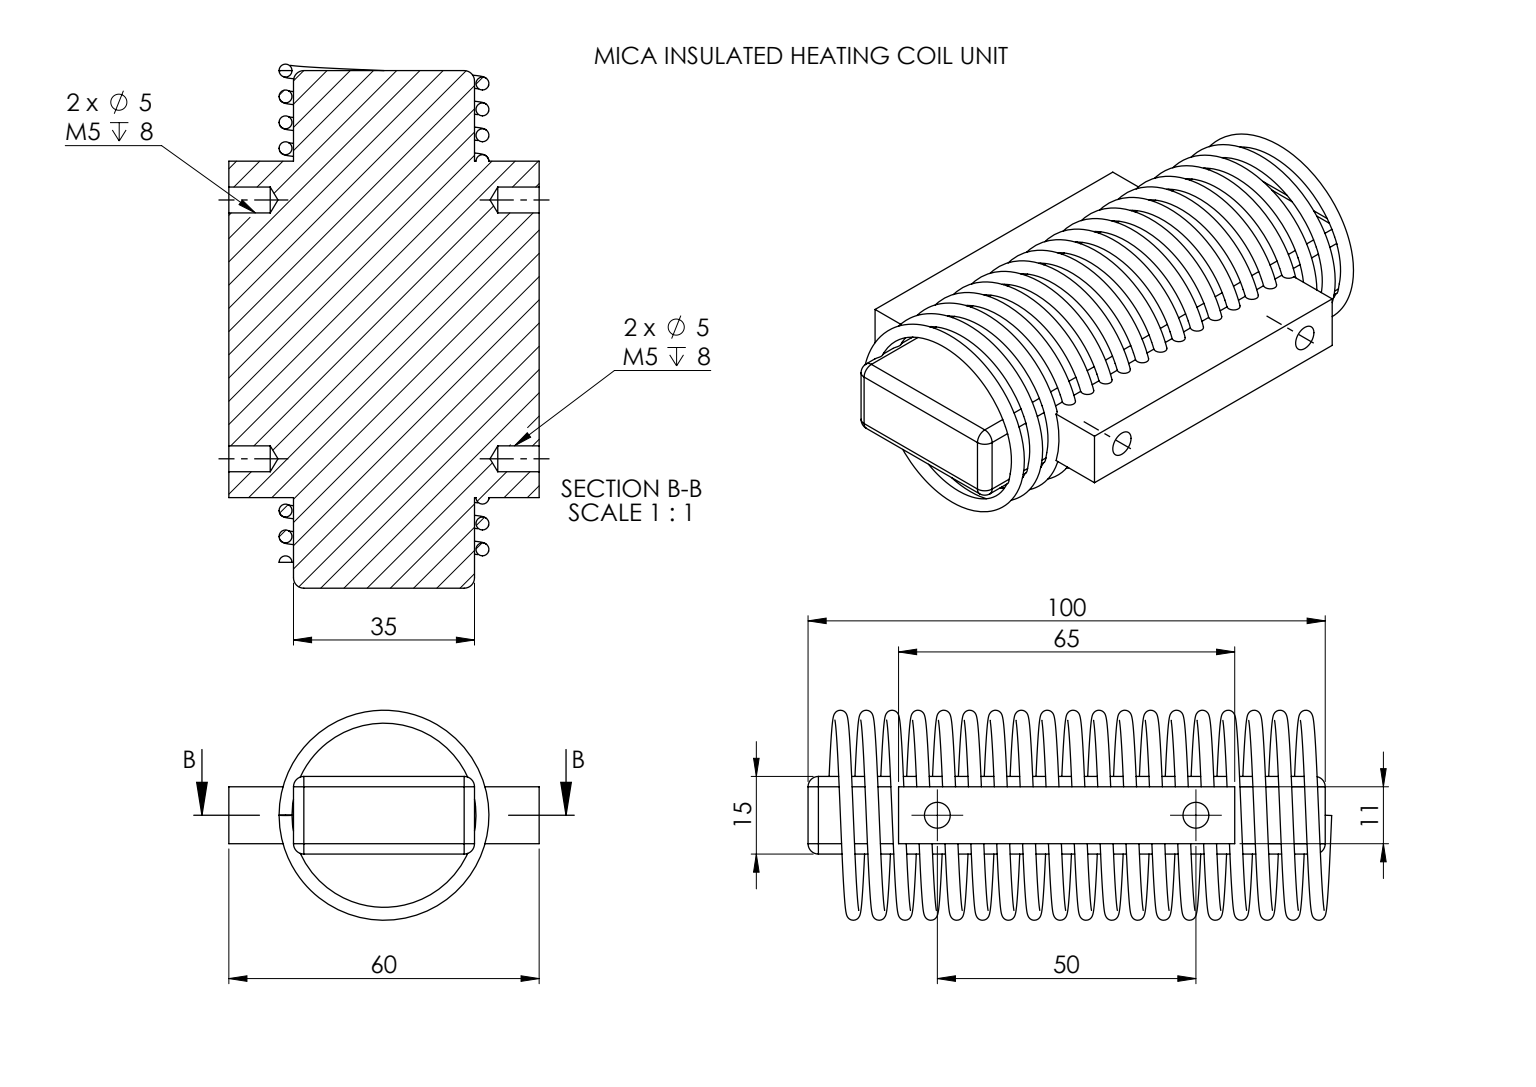
ISO-10303-21;
HEADER;
FILE_DESCRIPTION (('STEP AP214'),
    '1' );
FILE_NAME ('Mica Insulated Heating Coil Unit.step',
    '2026-10-04T13:31:42',
    ( '' ),
    ( '' ),
    'SwSTEP 2.0',
    'SolidWorks 2026',
    '' );
FILE_SCHEMA (( 'AUTOMOTIVE_DESIGN' ));
ENDSEC;

DATA;
#1=CARTESIAN_POINT ( 'NONE',  ( -19.03943276465977164, 0.05219959533909376836, 71.24890960531435269 ) ) ;
#2=CARTESIAN_POINT ( 'NONE',  ( 4.379528057220339221, -16.55341960407611168, 72.70724293864769550 ) ) ;
#3=CARTESIAN_POINT ( 'NONE',  ( 19.05341960407617918, -5.049401038297876454, 86.04275706135233293 ) ) ;
#4=CARTESIAN_POINT ( 'NONE',  ( 21.53943276465977519, -0.05219959533907433946, 43.74890960531435979 ) ) ;
#6=CARTESIAN_POINT ( 'NONE',  ( -19.05341960407611168, -5.049401038298163336, 21.45724293864768839 ) ) ;
#7=CARTESIAN_POINT ( 'NONE',  ( -16.18388926212240264, -7.379444403734405356, 30.43953151366152809 ) ) ;
#8=CARTESIAN_POINT ( 'NONE',  ( 5.049401038298161559, -19.05341960407611168, 77.70724293864765286 ) ) ;
#9=CARTESIAN_POINT ( 'NONE',  ( 21.53943276465977519, -0.05219959533907433946, 73.74890960531433848 ) ) ;
#10=CARTESIAN_POINT ( 'NONE',  ( -8.314922557961024197, 14.29746914071037800, 97.91775706135236135 ) ) ;
#11=CARTESIAN_POINT ( 'NONE',  ( -5.049401038298153566, 19.05341960407611168, 75.20724293864769550 ) ) ;
#12=CARTESIAN_POINT ( 'NONE',  ( -9.564922557961040184, 16.46253265017147172, 72.91775706135233293 ) ) ;
#13=CARTESIAN_POINT ( 'NONE',  ( 5.823673210054444382, -21.52544592524334988, 85.20942372801901854 ) ) ;
#14=CARTESIAN_POINT ( 'NONE',  ( -15.80617190586745835, -15.72974639402198527, 56.87390960531436690 ) ) ;
#15=CARTESIAN_POINT ( 'NONE',  ( 21.52544592524344225, -5.823673210054117533, 23.54057627198102765 ) ) ;
#16=CARTESIAN_POINT ( 'NONE',  ( -19.02544592524342804, 5.153800228976336051, 36.04057627198100988 ) ) ;
#17=CARTESIAN_POINT ( 'NONE',  ( -4.379528057220086978, -16.55341960407618274, 94.79275706135234714 ) ) ;
#18=CARTESIAN_POINT ( 'NONE',  ( -19.05341960407611168, -5.049401038298163336, 56.45724293864768129 ) ) ;
#19=CARTESIAN_POINT ( 'NONE',  ( 14.29746914071037800, 8.314922557961029526, 26.66775706135235424 ) ) ;
#21=CARTESIAN_POINT ( 'NONE',  ( 18.67979575497194134, -10.72451020669871369, 110.8344237280190043 ) ) ;
#22=CARTESIAN_POINT ( 'NONE',  ( -14.29746914071049879, 8.314922557960819915, 55.83224293864770260 ) ) ;
#23=CARTESIAN_POINT ( 'NONE',  ( -0.05219959533907301413, -21.53943276465977519, 102.4989096053143811 ) ) ;
#24=CARTESIAN_POINT ( 'NONE',  ( 10.81492255796078972, 18.62759615963270932, 99.58224293864770971 ) ) ;
#26=CARTESIAN_POINT ( 'NONE',  ( -15.72974639402197994, 15.80617190586746368, 40.62390960531435269 ) ) ;
#27=CARTESIAN_POINT ( 'NONE',  ( -12.06949235617739369, -12.14591786802326823, 74.37609039468568994 ) ) ;
#28=CARTESIAN_POINT ( 'NONE',  ( -4.483927247898539470, -16.52544592524342804, 92.29057627198103830 ) ) ;
#29=CARTESIAN_POINT ( 'NONE',  ( 19.03943276465977164, -0.05219959533909143690, 58.74890960531435979 ) ) ;
#30=SHAPE_REPRESENTATION_RELATIONSHIP ( 'NONE' , 'NONE' ,  #65015, #146166 ) ;
#32=CARTESIAN_POINT ( 'NONE',  ( -12.06949235617739369, -12.14591786802326823, 109.3760903946857042 ) ) ;
#33=CARTESIAN_POINT ( 'NONE',  ( -5.719274019375665041, -21.55341960407619695, 34.79275706135235424 ) ) ;
#34=CARTESIAN_POINT ( 'NONE',  ( -19.05341960407611168, -5.049401038298163336, 91.45724293864766707 ) ) ;
#35=CARTESIAN_POINT ( 'NONE',  ( 21.55341960407619695, -5.719274019375665929, 71.04275706135234714 ) ) ;
#38=ORIENTED_EDGE ( 'NONE', *, *, #138549, .T. ) ;
#39=CARTESIAN_POINT ( 'NONE',  ( 10.72451020669871369, 18.67979575497193778, 57.08442372801901854 ) ) ;
#40=CARTESIAN_POINT ( 'NONE',  ( -0.05219959533909027116, -19.03943276465977164, 57.49890960531435979 ) ) ;
#41=CARTESIAN_POINT ( 'NONE',  ( 9.564922557960805705, 16.46253265017160317, 84.58224293864769550 ) ) ;
#42=CARTESIAN_POINT ( 'NONE',  ( -9.564922557961040184, 16.46253265017147172, 67.91775706135233293 ) ) ;
#43=CARTESIAN_POINT ( 'NONE',  ( 5.719274019375673035, 21.55341960407619339, 47.29275706135234003 ) ) ;
#44=CARTESIAN_POINT ( 'NONE',  ( -19.05341960407617563, 5.049401038297882671, 103.5427570613523329 ) ) ;
#45=CARTESIAN_POINT ( 'NONE',  ( -5.049401038297874678, -19.05341960407617918, 69.79275706135233293 ) ) ;
#46=CARTESIAN_POINT ( 'NONE',  ( 13.89961937509977652, -13.97604488694527269, 38.12390960531436690 ) ) ;
#47=CARTESIAN_POINT ( 'NONE',  ( 19.05341960407617918, -5.049401038297876454, 86.04275706135233293 ) ) ;
#48=CARTESIAN_POINT ( 'NONE',  ( -16.52544592524335698, -4.483927247898792601, 98.95942372801903275 ) ) ;
#49=CARTESIAN_POINT ( 'NONE',  ( 0.05219959533936267826, -19.03943276465977164, 80.00109039468567573 ) ) ;
#50=CARTESIAN_POINT ( 'NONE',  ( -12.14591786802309592, -12.06949235617757132, 31.87390960531435979 ) ) ;
#51=CARTESIAN_POINT ( 'NONE',  ( 16.51473224551083163, -9.474510206698727899, 45.83442372801900433 ) ) ;
#52=CARTESIAN_POINT ( 'NONE',  ( 15.80617190586769283, -15.72974639402175789, 100.6260903946857184 ) ) ;
#54=CARTESIAN_POINT ( 'NONE',  ( 19.05341960407617918, -5.049401038297876454, 21.04275706135232582 ) ) ;
#56=CARTESIAN_POINT ( 'NONE',  ( 0.05219959533909260263, 19.03943276465977164, 24.99890960531435269 ) ) ;
#57=CARTESIAN_POINT ( 'NONE',  ( -21.53943276465977519, -0.05219959533937600094, 83.75109039468568994 ) ) ;
#58=CARTESIAN_POINT ( 'NONE',  ( 8.314922557961029526, -14.29746914071037800, 30.41775706135234358 ) ) ;
#59=CARTESIAN_POINT ( 'NONE',  ( 19.02544592524343514, -5.153800228976328945, 98.54057627198100988 ) ) ;
#61=CARTESIAN_POINT ( 'NONE',  ( 0.05219959533909260263, 19.03943276465977164, 79.99890960531436690 ) ) ;
#62=DIRECTION ( 'NONE',  ( -0.000000000000000000, -0.000000000000000000, 1.000000000000000000 ) ) ;
#64=CARTESIAN_POINT ( 'NONE',  ( -16.51473224551082808, 9.474510206698731452, 83.33442372801899012 ) ) ;
#66=CARTESIAN_POINT ( 'NONE',  ( 0.05219959533909260263, 19.03943276465977164, 114.9989096053143669 ) ) ;
#67=CARTESIAN_POINT ( 'NONE',  ( -10.72451020669870658, -18.67979575497194134, 109.5844237280190328 ) ) ;
#68=CARTESIAN_POINT ( 'NONE',  ( -13.97604488694547697, 13.89961937509957934, 103.1260903946856473 ) ) ;
#69=CARTESIAN_POINT ( 'NONE',  ( -4.483927247898539470, -16.52544592524342804, 97.29057627198105251 ) ) ;
#70=CARTESIAN_POINT ( 'NONE',  ( -5.153800228976328057, -19.02544592524343514, 22.29057627198102765 ) ) ;
#71=CARTESIAN_POINT ( 'NONE',  ( -5.823673210054116645, -21.52544592524344225, 62.29057627198102409 ) ) ;
#73=CARTESIAN_POINT ( 'NONE',  ( 10.72451020669898902, -18.67979575497178502, 47.91557627198102409 ) ) ;
#74=CARTESIAN_POINT ( 'NONE',  ( 13.89961937509977652, -13.97604488694527269, 28.12390960531435624 ) ) ;
#76=CARTESIAN_POINT ( 'NONE',  ( 16.51473224551083163, -9.474510206698727899, 55.83442372801899722 ) ) ;
#77=CARTESIAN_POINT ( 'NONE',  ( -14.29746914071049879, 8.314922557960819915, 35.83224293864768839 ) ) ;
#78=CARTESIAN_POINT ( 'NONE',  ( 9.474510206698971260, -16.51473224551069308, 112.9155762719810383 ) ) ;
#79=CARTESIAN_POINT ( 'NONE',  ( -15.80617190586768217, 15.72974639402176855, 83.12609039468568994 ) ) ;
#80=CARTESIAN_POINT ( 'NONE',  ( -10.72451020669898014, 18.67979575497178502, 65.41557627198102409 ) ) ;
#81=CARTESIAN_POINT ( 'NONE',  ( 18.67979575497194134, -10.72451020669871369, 55.83442372801901854 ) ) ;
#82=CARTESIAN_POINT ( 'NONE',  ( 15.80617190586769283, -15.72974639402175789, 45.62609039468567573 ) ) ;
#83=CARTESIAN_POINT ( 'NONE',  ( 13.89961937509977652, -13.97604488694527269, 78.12390960531433848 ) ) ;
#84=CARTESIAN_POINT ( 'NONE',  ( -8.314922557961024197, 14.29746914071037800, 97.91775706135236135 ) ) ;
#85=CARTESIAN_POINT ( 'NONE',  ( -5.049401038298153566, 19.05341960407611168, 25.20724293864768484 ) ) ;
#87=CARTESIAN_POINT ( 'NONE',  ( -14.29746914071049879, 8.314922557960819915, 70.83224293864770971 ) ) ;
#88=CARTESIAN_POINT ( 'NONE',  ( 8.224510206698953496, -14.34966873604960469, 37.91557627198102409 ) ) ;
#89=CARTESIAN_POINT ( 'NONE',  ( 19.05341960407611168, 5.049401038298154454, 63.95724293864769550 ) ) ;
#90=CARTESIAN_POINT ( 'NONE',  ( -19.03943276465977164, 0.05219959533909376836, 36.24890960531436690 ) ) ;
#91=CARTESIAN_POINT ( 'NONE',  ( 15.72974639402199770, -15.80617190586745480, 43.12390960531435269 ) ) ;
#92=CARTESIAN_POINT ( 'NONE',  ( -19.02544592524334988, -5.153800228976617603, 33.95942372801897591 ) ) ;
#94=CARTESIAN_POINT ( 'NONE',  ( 16.55341960407611168, 4.379528057220329451, 48.95724293864770971 ) ) ;
#95=CARTESIAN_POINT ( 'NONE',  ( -10.72451020669898014, 18.67979575497178502, 30.41557627198101699 ) ) ;
#98=CARTESIAN_POINT ( 'NONE',  ( -8.314922557961024197, 14.29746914071037800, 72.91775706135234714 ) ) ;
#99=CARTESIAN_POINT ( 'NONE',  ( 13.97604488694548053, -13.89961937509957401, 70.62609039468567573 ) ) ;
#100=CARTESIAN_POINT ( 'NONE',  ( 16.53943276465976808, -0.05219959533910856209, 43.74890960531435979 ) ) ;
#102=CARTESIAN_POINT ( 'NONE',  ( -8.314922557960811034, -14.29746914071050412, 27.08224293864769550 ) ) ;
#103=CARTESIAN_POINT ( 'NONE',  ( 16.46253265017160672, -9.564922557960803928, 48.33224293864769550 ) ) ;
#104=CARTESIAN_POINT ( 'NONE',  ( 19.05341960407611168, 5.049401038298154454, 73.95724293864768129 ) ) ;
#105=CARTESIAN_POINT ( 'NONE',  ( -5.049401038298153566, 19.05341960407611168, 35.20724293864768839 ) ) ;
#106=CARTESIAN_POINT ( 'NONE',  ( 21.55341960407619695, -5.719274019375665929, 41.04275706135236135 ) ) ;
#107=CARTESIAN_POINT ( 'NONE',  ( 16.46253265017160672, -9.564922557960803928, 63.33224293864769550 ) ) ;
#109=CARTESIAN_POINT ( 'NONE',  ( -19.03943276465977164, 0.05219959533909376836, 46.24890960531435979 ) ) ;
#110=CARTESIAN_POINT ( 'NONE',  ( -0.05219959533907301413, -21.53943276465977519, 32.49890960531435979 ) ) ;
#111=B_SPLINE_CURVE_WITH_KNOTS ( 'NONE', 3,
 ( #132361, #22184, #54519, #149527, #68676, #38352 ),
 .UNSPECIFIED., .F., .F.,
 ( 4, 2, 4 ),
 ( 0.007228050697041336729, 0.007608510107494812283, 0.007988969517948286969 ),
 .UNSPECIFIED. ) ;
#112=CARTESIAN_POINT ( 'NONE',  ( 10.72451020669871369, 18.67979575497193778, 67.08442372801901854 ) ) ;
#113=CARTESIAN_POINT ( 'NONE',  ( 12.06949235617757843, -12.14591786802309237, 113.1239096053143953 ) ) ;
#114=CARTESIAN_POINT ( 'NONE',  ( -21.55341960407610458, -5.719274019375992779, 31.45724293864769550 ) ) ;
#115=CARTESIAN_POINT ( 'NONE',  ( 8.314922557961029526, -14.29746914071037800, 95.41775706135234714 ) ) ;
#116=CARTESIAN_POINT ( 'NONE',  ( 10.81492255796106328, -18.62759615963255655, 110.4177570613523756 ) ) ;
#117=CARTESIAN_POINT ( 'NONE',  ( -8.314922557961024197, 14.29746914071037800, 67.91775706135234714 ) ) ;
#118=CARTESIAN_POINT ( 'NONE',  ( -9.564922557960796823, -16.46253265017161027, 112.0822429386476955 ) ) ;
#119=CARTESIAN_POINT ( 'NONE',  ( -14.29746914071037622, -8.314922557961029526, 59.16775706135234714 ) ) ;
#120=CARTESIAN_POINT ( 'NONE',  ( -8.314922557961024197, 14.29746914071037800, 37.91775706135235424 ) ) ;
#121=CARTESIAN_POINT ( 'NONE',  ( -0.05219959533934338120, 16.53943276465976808, 102.5010903946856899 ) ) ;
#122=CARTESIAN_POINT ( 'NONE',  ( -15.72974639402176322, -15.80617190586768395, 54.37609039468568994 ) ) ;
#123=CARTESIAN_POINT ( 'NONE',  ( 4.379528057220092307, 16.55341960407617563, 22.29275706135235069 ) ) ;
#124=CARTESIAN_POINT ( 'NONE',  ( 5.719274019375991003, -21.55341960407610458, 112.7072429386476955 ) ) ;
#125=CARTESIAN_POINT ( 'NONE',  ( 8.224510206698742110, 14.34966873604972548, 27.08442372801901854 ) ) ;
#126=CARTESIAN_POINT ( 'NONE',  ( -12.14591786802326823, 12.06949235617739902, 83.12609039468568994 ) ) ;
#128=CARTESIAN_POINT ( 'NONE',  ( 18.67979575497194134, -10.72451020669871369, 85.83442372801901854 ) ) ;
#129=CARTESIAN_POINT ( 'NONE',  ( 16.46253265017146816, 9.564922557961045513, 81.66775706135233293 ) ) ;
#130=CARTESIAN_POINT ( 'NONE',  ( -4.379528057220328563, 16.55341960407611168, 60.20724293864768839 ) ) ;
#131=CARTESIAN_POINT ( 'NONE',  ( -4.379528057220328563, 16.55341960407611168, 40.20724293864769550 ) ) ;
#132=CARTESIAN_POINT ( 'NONE',  ( -14.29746914071049879, 8.314922557960819915, 105.8322429386476955 ) ) ;
#133=CARTESIAN_POINT ( 'NONE',  ( -16.46253265017146816, -9.564922557961047289, 49.16775706135233293 ) ) ;
#135=CARTESIAN_POINT ( 'NONE',  ( 0.05219959533937995610, -21.53943276465977519, 45.00109039468568284 ) ) ;
#136=CARTESIAN_POINT ( 'NONE',  ( 0.05219959533934541429, -16.53943276465976808, 20.00109039468568639 ) ) ;
#137=DIRECTION ( 'NONE',  ( 0.000000000000000000, 0.000000000000000000, -1.000000000000000000 ) ) ;
#138=CARTESIAN_POINT ( 'NONE',  ( 16.46253265017160672, -9.564922557960803928, 108.3322429386476955 ) ) ;
#139=CARTESIAN_POINT ( 'NONE',  ( 15.80617190586746368, 15.72974639402197994, 69.37390960531436690 ) ) ;
#140=CARTESIAN_POINT ( 'NONE',  ( -19.02544592524334988, -5.153800228976617603, 98.95942372801900433 ) ) ;
#141=CARTESIAN_POINT ( 'NONE',  ( -16.51473224551069308, -9.474510206698971260, 106.6655762719810383 ) ) ;
#143=CARTESIAN_POINT ( 'NONE',  ( 14.29746914071049879, -8.314922557960816363, 113.3322429386476955 ) ) ;
#144=CARTESIAN_POINT ( 'NONE',  ( -21.55341960407619339, 5.719274019375674811, 98.54275706135234714 ) ) ;
#145=CARTESIAN_POINT ( 'NONE',  ( 13.89961937509977652, -13.97604488694527269, 28.12390960531435624 ) ) ;
#146=CARTESIAN_POINT ( 'NONE',  ( 21.52544592524334988, 5.823673210054432836, 51.45942372801901854 ) ) ;
#147=CARTESIAN_POINT ( 'NONE',  ( -21.53943276465977519, -0.05219959533937600094, 93.75109039468567573 ) ) ;
#148=CARTESIAN_POINT ( 'NONE',  ( 14.29746914071037800, 8.314922557961029526, 86.66775706135234714 ) ) ;
#149=CARTESIAN_POINT ( 'NONE',  ( -5.719274019375665041, -21.55341960407619695, 39.79275706135235424 ) ) ;
#150=CARTESIAN_POINT ( 'NONE',  ( 21.52544592524334988, 5.823673210054432836, 36.45942372801901143 ) ) ;
#151=CARTESIAN_POINT ( 'NONE',  ( 5.049401038297881783, 19.05341960407617563, 67.29275706135234714 ) ) ;
#152=CARTESIAN_POINT ( 'NONE',  ( -16.51473224551069308, -9.474510206698971260, 81.66557627198103830 ) ) ;
#153=CARTESIAN_POINT ( 'NONE',  ( -0.05219959533910754901, -16.53943276465976808, 107.4989096053143669 ) ) ;
#154=CARTESIAN_POINT ( 'NONE',  ( -0.05219959533907301413, -21.53943276465977519, 82.49890960531436690 ) ) ;
#155=CARTESIAN_POINT ( 'NONE',  ( 12.14591786802309770, 12.06949235617756955, 64.37390960531435269 ) ) ;
#156=CARTESIAN_POINT ( 'NONE',  ( -21.52544592524334988, -5.823673210054445271, 103.9594237280190185 ) ) ;
#157=CARTESIAN_POINT ( 'NONE',  ( -8.224510206698948167, 14.34966873604960824, 90.41557627198103830 ) ) ;
#158=CARTESIAN_POINT ( 'NONE',  ( -19.02544592524342804, 5.153800228976336051, 41.04057627198103120 ) ) ;
#159=CARTESIAN_POINT ( 'NONE',  ( 19.02544592524334988, 5.153800228976608722, 66.45942372801899012 ) ) ;
#160=AXIS2_PLACEMENT_3D ( 'NONE', #57198, #41025, #151201 ) ;
#161=CARTESIAN_POINT ( 'NONE',  ( -8.224510206698948167, 14.34966873604960824, 50.41557627198103120 ) ) ;
#162=CARTESIAN_POINT ( 'NONE',  ( 5.823673210054444382, -21.52544592524334988, 95.20942372801903275 ) ) ;
#163=CARTESIAN_POINT ( 'NONE',  ( 13.97604488694527802, 13.89961937509977652, 89.37390960531436690 ) ) ;
#164=CARTESIAN_POINT ( 'NONE',  ( 5.153800228976615827, -19.02544592524334988, 55.20942372801899722 ) ) ;
#165=CARTESIAN_POINT ( 'NONE',  ( 0.05219959533907565091, 21.53943276465977519, 69.99890960531435269 ) ) ;
#166=CARTESIAN_POINT ( 'NONE',  ( 18.67979575497178502, 10.72451020669898547, 109.1655762719810383 ) ) ;
#167=CARTESIAN_POINT ( 'NONE',  ( 5.153800228976615827, -19.02544592524334988, 110.2094237280189901 ) ) ;
#168=CARTESIAN_POINT ( 'NONE',  ( 0.05219959533934541429, -16.53943276465976808, 80.00109039468568994 ) ) ;
#169=CARTESIAN_POINT ( 'NONE',  ( -5.153800228976328057, -19.02544592524343514, 22.29057627198102765 ) ) ;
#170=CARTESIAN_POINT ( 'NONE',  ( -10.72451020669870658, -18.67979575497194134, 24.58442372801901499 ) ) ;
#171=CARTESIAN_POINT ( 'NONE',  ( -14.29746914071049879, 8.314922557960819915, 110.8322429386476955 ) ) ;
#173=CARTESIAN_POINT ( 'NONE',  ( 8.314922557961029526, -14.29746914071037800, 45.41775706135234003 ) ) ;
#175=CARTESIAN_POINT ( 'NONE',  ( 16.53943276465976808, -0.05219959533910856209, 78.74890960531436690 ) ) ;
#176=CARTESIAN_POINT ( 'NONE',  ( -18.67979575497178146, -10.72451020669898902, 81.66557627198103830 ) ) ;
#177=CARTESIAN_POINT ( 'NONE',  ( -8.224510206698735004, -14.34966873604973081, 104.5844237280190185 ) ) ;
#178=CARTESIAN_POINT ( 'NONE',  ( -4.483927247898782831, 16.52544592524335698, 32.70942372801900433 ) ) ;
#179=CARTESIAN_POINT ( 'NONE',  ( 19.03943276465977164, -0.05219959533909143690, 38.74890960531436690 ) ) ;
#180=CARTESIAN_POINT ( 'NONE',  ( -16.53943276465976808, -0.05219959533934237506, 83.75109039468568994 ) ) ;
#181=CARTESIAN_POINT ( 'NONE',  ( -5.153800228976607833, 19.02544592524334988, 77.70942372801900433 ) ) ;
#182=CARTESIAN_POINT ( 'NONE',  ( 21.55341960407610458, 5.719274019375980345, 68.95724293864769550 ) ) ;
#183=CARTESIAN_POINT ( 'NONE',  ( -4.379528057220086978, -16.55341960407618274, 109.7927570613523613 ) ) ;
#184=CARTESIAN_POINT ( 'NONE',  ( 15.72974639402176855, 15.80617190586768217, 86.87609039468568994 ) ) ;
#185=CARTESIAN_POINT ( 'NONE',  ( -18.67979575497178146, -10.72451020669898902, 41.66557627198103120 ) ) ;
#186=EDGE_LOOP ( 'NONE', ( #96983, #147295, #14374 ) ) ;
#187=CARTESIAN_POINT ( 'NONE',  ( -14.34966873604972548, 8.224510206698743886, 98.33442372801901854 ) ) ;
#188=CARTESIAN_POINT ( 'NONE',  ( -18.62759615963270932, 10.81492255796079327, 50.83224293864770971 ) ) ;
#190=CARTESIAN_POINT ( 'NONE',  ( -0.05219959533907301413, -21.53943276465977519, 22.49890960531436335 ) ) ;
#191=CARTESIAN_POINT ( 'NONE',  ( 17.50000000000000355, 3.565345528327941160, 108.0750551319352581 ) ) ;
#192=CARTESIAN_POINT ( 'NONE',  ( -16.46253265017160317, 9.564922557960807481, 25.83224293864769194 ) ) ;
#193=CARTESIAN_POINT ( 'NONE',  ( 15.72974639402199770, -15.80617190586745480, 78.12390960531436690 ) ) ;
#194=CARTESIAN_POINT ( 'NONE',  ( 0.05219959533934541429, -16.53943276465976808, 105.0010903946856757 ) ) ;
#195=CARTESIAN_POINT ( 'NONE',  ( 21.53943276465977519, 0.05219959533937863772, 61.25109039468567573 ) ) ;
#196=CARTESIAN_POINT ( 'NONE',  ( -14.29746914071037622, -8.314922557961029526, 24.16775706135235424 ) ) ;
#197=CARTESIAN_POINT ( 'NONE',  ( 12.14591786802309770, 12.06949235617756955, 114.3739096053143527 ) ) ;
#198=CARTESIAN_POINT ( 'NONE',  ( -19.05341960407617563, 5.049401038297882671, 113.5427570613523471 ) ) ;
#199=CARTESIAN_POINT ( 'NONE',  ( -5.049401038298153566, 19.05341960407611168, 35.20724293864768839 ) ) ;
#201=CARTESIAN_POINT ( 'NONE',  ( -19.03943276465977164, 0.05219959533909376836, 111.2489096053143669 ) ) ;
#202=CARTESIAN_POINT ( 'NONE',  ( 0.05219959533934541429, -16.53943276465976808, 85.00109039468568994 ) ) ;
#203=CARTESIAN_POINT ( 'NONE',  ( -9.564922557961040184, 16.46253265017147172, 82.91775706135233293 ) ) ;
#204=CARTESIAN_POINT ( 'NONE',  ( 9.564922557961047289, -16.46253265017146816, 30.41775706135232937 ) ) ;
#205=CARTESIAN_POINT ( 'NONE',  ( 0.05219959533907565091, 21.53943276465977519, 59.99890960531436690 ) ) ;
#206=CARTESIAN_POINT ( 'NONE',  ( -14.34966873604972548, 8.224510206698743886, 83.33442372801903275 ) ) ;
#207=CARTESIAN_POINT ( 'NONE',  ( -16.46253265017146816, -9.564922557961047289, 99.16775706135233293 ) ) ;
#208=CARTESIAN_POINT ( 'NONE',  ( 19.05341960407611168, 5.049401038298154454, 53.95724293864770260 ) ) ;
#209=CARTESIAN_POINT ( 'NONE',  ( 16.46253265017160672, -9.564922557960803928, 98.33224293864769550 ) ) ;
#210=CARTESIAN_POINT ( 'NONE',  ( -0.05219959533937732626, 21.53943276465977519, 47.50109039468568994 ) ) ;
#211=CARTESIAN_POINT ( 'NONE',  ( -19.05341960407611168, -5.049401038298163336, 41.45724293864769550 ) ) ;
#213=CARTESIAN_POINT ( 'NONE',  ( -13.89961937509977652, 13.97604488694528158, 110.6239096053143243 ) ) ;
#214=CARTESIAN_POINT ( 'NONE',  ( 8.314922557960818139, 14.29746914071049879, 64.58224293864769550 ) ) ;
#215=CARTESIAN_POINT ( 'NONE',  ( -5.719274019375978568, 21.55341960407610458, 55.20724293864770260 ) ) ;
#217=CARTESIAN_POINT ( 'NONE',  ( -16.46253265017146816, -9.564922557961047289, 49.16775706135233293 ) ) ;
#219=CARTESIAN_POINT ( 'NONE',  ( -16.46253265017160317, 9.564922557960807481, 60.83224293864769550 ) ) ;
#220=CARTESIAN_POINT ( 'NONE',  ( 5.049401038298161559, -19.05341960407611168, 67.70724293864769550 ) ) ;
#222=CARTESIAN_POINT ( 'NONE',  ( 12.06949235617739724, 12.14591786802326823, 46.87609039468568994 ) ) ;
#224=CARTESIAN_POINT ( 'NONE',  ( 16.51473224551083163, -9.474510206698727899, 30.83442372801900433 ) ) ;
#226=CARTESIAN_POINT ( 'NONE',  ( -0.05219959533934338120, 16.53943276465976808, 92.50109039468567573 ) ) ;
#228=CARTESIAN_POINT ( 'NONE',  ( 16.52544592524335698, 4.483927247898782831, 81.45942372801900433 ) ) ;
#229=CARTESIAN_POINT ( 'NONE',  ( 4.483927247898790824, -16.52544592524335698, 60.20942372801902565 ) ) ;
#230=CARTESIAN_POINT ( 'NONE',  ( -5.823673210054431948, 21.52544592524334988, 112.7094237280190328 ) ) ;
#231=CARTESIAN_POINT ( 'NONE',  ( -5.049401038298153566, 19.05341960407611168, 50.20724293864770260 ) ) ;
#233=CARTESIAN_POINT ( 'NONE',  ( -10.72451020669870658, -18.67979575497194134, 69.58442372801900433 ) ) ;
#234=CARTESIAN_POINT ( 'NONE',  ( -19.03943276465977164, -0.05219959533935918106, 73.75109039468566152 ) ) ;
#235=CARTESIAN_POINT ( 'NONE',  ( -18.67979575497193778, 10.72451020669871902, 113.3344237280190328 ) ) ;
#236=CARTESIAN_POINT ( 'NONE',  ( 16.51473224551069308, 9.474510206698969483, 29.16557627198103475 ) ) ;
#237=CARTESIAN_POINT ( 'NONE',  ( 17.50000000000006750, 5.663021631379938192, 23.82188452050911209 ) ) ;
#238=CARTESIAN_POINT ( 'NONE',  ( -10.72451020669898014, 18.67979575497178502, 70.41557627198102409 ) ) ;
#239=CARTESIAN_POINT ( 'NONE',  ( 18.67979575497178502, 10.72451020669898547, 24.16557627198103120 ) ) ;
#240=CARTESIAN_POINT ( 'NONE',  ( 0.05219959533910956823, 16.53943276465976808, 114.9989096053143669 ) ) ;
#241=CARTESIAN_POINT ( 'NONE',  ( 4.379528057220092307, 16.55341960407617563, 37.29275706135235424 ) ) ;
#242=CARTESIAN_POINT ( 'NONE',  ( 14.34966873604960469, 8.224510206698951720, 24.16557627198103120 ) ) ;
#244=CARTESIAN_POINT ( 'NONE',  ( -15.72974639402176322, -15.80617190586768395, 24.37609039468567573 ) ) ;
#245=CARTESIAN_POINT ( 'NONE',  ( 4.483927247898545687, 16.52544592524342804, 34.79057627198103120 ) ) ;
#247=CARTESIAN_POINT ( 'NONE',  ( -13.89961937509957401, -13.97604488694547875, 109.3760903946856331 ) ) ;
#248=CARTESIAN_POINT ( 'NONE',  ( 16.46253265017146816, 9.564922557961045513, 21.66775706135233648 ) ) ;
#249=CARTESIAN_POINT ( 'NONE',  ( 12.14591786802309770, 12.06949235617756955, 49.37390960531436690 ) ) ;
#250=CARTESIAN_POINT ( 'NONE',  ( 18.67979575497178502, 10.72451020669898547, 99.16557627198100988 ) ) ;
#251=CARTESIAN_POINT ( 'NONE',  ( 17.50000000000000355, 5.622605283950888655, 33.81207310596111881 ) ) ;
#252=CARTESIAN_POINT ( 'NONE',  ( -15.72974639402197994, 15.80617190586746368, 60.62390960531437401 ) ) ;
#253=CARTESIAN_POINT ( 'NONE',  ( -0.05219959533909027116, -19.03943276465977164, 77.49890960531435269 ) ) ;
#254=CARTESIAN_POINT ( 'NONE',  ( 8.314922557960818139, 14.29746914071049879, 49.58224293864769550 ) ) ;
#255=CARTESIAN_POINT ( 'NONE',  ( 0.05219959533909260263, 19.03943276465977164, 89.99890960531436690 ) ) ;
#256=B_SPLINE_CURVE_WITH_KNOTS ( 'NONE', 3,
 ( #135702, #179228, #194389, #162034, #102364, #70032, #58838, #148877, #56868, #196396, #118543, #180233, #23530, #41702, #119537, #146865, #181220, #193382, #54858, #116532, #178220, #17313, #108315, #14325, #1126, #186178, #60815, #44673, #78968, #169995, #75990, #62800 ),
 .UNSPECIFIED., .F., .F.,
 ( 4, 2, 2, 2, 2, 2, 2, 2, 2, 2, 2, 2, 2, 2, 2, 4 ),
 ( 1.646036181032119693E-15, 0.0003712461730052185930, 0.0007424923460087911502, 0.001113738519012363653, 0.001484984692015936265, 0.002227477038023079753, 0.002598723211026658653, 0.002969969384030237119, 0.003341215557033815585, 0.003712461730037394485, 0.004083707903040972517, 0.004454954076044551417, 0.004826200249048129449, 0.005197446422051708349, 0.005568692595055286382, 0.005939938768058865282 ),
 .UNSPECIFIED. ) ;
#258=CARTESIAN_POINT ( 'NONE',  ( 0.05219959533936267826, -19.03943276465977164, 60.00109039468566863 ) ) ;
#259=CARTESIAN_POINT ( 'NONE',  ( 5.823673210054125526, 21.52544592524343514, 99.79057627198103830 ) ) ;
#260=CARTESIAN_POINT ( 'NONE',  ( 19.05341960407611168, 5.049401038298154454, 43.95724293864769550 ) ) ;
#261=CARTESIAN_POINT ( 'NONE',  ( -0.05219959533910754901, -16.53943276465976808, 102.4989096053143811 ) ) ;
#262=CARTESIAN_POINT ( 'NONE',  ( -10.81492255796105439, 18.62759615963255655, 47.91775706135234714 ) ) ;
#264=CARTESIAN_POINT ( 'NONE',  ( -16.52544592524342804, 4.483927247898546575, 26.04057627198103475 ) ) ;
#265=CARTESIAN_POINT ( 'NONE',  ( -13.89961937509977652, 13.97604488694528158, 55.62390960531434558 ) ) ;
#266=CARTESIAN_POINT ( 'NONE',  ( -13.89961937509977652, 13.97604488694528158, 105.6239096053143527 ) ) ;
#267=CARTESIAN_POINT ( 'NONE',  ( 5.823673210054125526, 21.52544592524343514, 59.79057627198103120 ) ) ;
#269=CARTESIAN_POINT ( 'NONE',  ( 0.05219959533909260263, 19.03943276465977164, 34.99890960531435979 ) ) ;
#270=CARTESIAN_POINT ( 'NONE',  ( -15.72974639402197994, 15.80617190586746368, 50.62390960531435979 ) ) ;
#271=CARTESIAN_POINT ( 'NONE',  ( 15.72974639402176855, 15.80617190586768217, 91.87609039468568994 ) ) ;
#273=CARTESIAN_POINT ( 'NONE',  ( -16.52544592524335698, -4.483927247898792601, 83.95942372801900433 ) ) ;
#274=CARTESIAN_POINT ( 'NONE',  ( 12.06949235617739724, 12.14591786802326823, 91.87609039468568994 ) ) ;
#275=CARTESIAN_POINT ( 'NONE',  ( 5.153800228976335163, 19.02544592524342804, 54.79057627198103120 ) ) ;
#276=CARTESIAN_POINT ( 'NONE',  ( 13.89961937509977652, -13.97604488694527269, 68.12390960531436690 ) ) ;
#278=CARTESIAN_POINT ( 'NONE',  ( -19.03943276465977164, -0.05219959533935918106, 28.75109039468566507 ) ) ;
#279=CARTESIAN_POINT ( 'NONE',  ( 14.29746914071037800, 8.314922557961029526, 76.66775706135234714 ) ) ;
#280=CARTESIAN_POINT ( 'NONE',  ( -18.67979575497193778, 10.72451020669871902, 113.3344237280190328 ) ) ;
#281=CARTESIAN_POINT ( 'NONE',  ( -19.05341960407611168, -5.049401038298163336, 71.45724293864766707 ) ) ;
#282=CARTESIAN_POINT ( 'NONE',  ( -21.52544592524343514, 5.823673210054127303, 36.04057627198102409 ) ) ;
#283=CARTESIAN_POINT ( 'NONE',  ( 14.34966873604972726, -8.224510206698740333, 25.83442372801901499 ) ) ;
#284=CARTESIAN_POINT ( 'NONE',  ( 0.05219959533937995610, -21.53943276465977519, 80.00109039468568994 ) ) ;
#285=CARTESIAN_POINT ( 'NONE',  ( -0.05219959533934338120, 16.53943276465976808, 52.50109039468567573 ) ) ;
#286=CARTESIAN_POINT ( 'NONE',  ( 10.72451020669898902, -18.67979575497178502, 97.91557627198103830 ) ) ;
#287=CARTESIAN_POINT ( 'NONE',  ( -16.51473224551082808, 9.474510206698731452, 113.3344237280190043 ) ) ;
#288=CARTESIAN_POINT ( 'NONE',  ( 13.89961937509977652, -13.97604488694527269, 73.12390960531436690 ) ) ;
#289=CARTESIAN_POINT ( 'NONE',  ( 4.483927247898790824, -16.52544592524335698, 25.20942372801901854 ) ) ;
#290=CARTESIAN_POINT ( 'NONE',  ( 13.97604488694527802, 13.89961937509977652, 44.37390960531435269 ) ) ;
#291=CARTESIAN_POINT ( 'NONE',  ( 16.46253265017146816, 9.564922557961045513, 111.6677570613523329 ) ) ;
#292=CARTESIAN_POINT ( 'NONE',  ( -12.06949235617756955, 12.14591786802309770, 75.62390960531439532 ) ) ;
#293=CARTESIAN_POINT ( 'NONE',  ( 4.379528057220092307, 16.55341960407617563, 87.29275706135236135 ) ) ;
#294=EDGE_CURVE ( 'NONE', #2008, #55198, #134552, .T. ) ;
#295=CARTESIAN_POINT ( 'NONE',  ( 21.52544592524334988, 5.823673210054432836, 31.45942372801901854 ) ) ;
#296=CARTESIAN_POINT ( 'NONE',  ( 0.05219959533909260263, 19.03943276465977164, 69.99890960531435269 ) ) ;
#297=CARTESIAN_POINT ( 'NONE',  ( 13.89961937509977652, -13.97604488694527269, 63.12390960531435979 ) ) ;
#298=CARTESIAN_POINT ( 'NONE',  ( 4.483927247898790824, -16.52544592524335698, 80.20942372801901854 ) ) ;
#302=CARTESIAN_POINT ( 'NONE',  ( -19.02544592524334988, -5.153800228976617603, 28.95942372801900433 ) ) ;
#303=CARTESIAN_POINT ( 'NONE',  ( -5.049401038298153566, 19.05341960407611168, 35.20724293864768839 ) ) ;
#304=CARTESIAN_POINT ( 'NONE',  ( 0.05219959533909260263, 19.03943276465977164, 109.9989096053143669 ) ) ;
#305=ORIENTED_EDGE ( 'NONE', *, *, #5230, .T. ) ;
#306=CARTESIAN_POINT ( 'NONE',  ( -12.14591786802326823, 12.06949235617739902, 33.12609039468569705 ) ) ;
#307=CARTESIAN_POINT ( 'NONE',  ( 9.474510206698729675, 16.51473224551082808, 52.08442372801900433 ) ) ;
#308=CARTESIAN_POINT ( 'NONE',  ( -16.52544592524335698, -4.483927247898792601, 38.95942372801901854 ) ) ;
#309=CARTESIAN_POINT ( 'NONE',  ( 0.05219959533909260263, 19.03943276465977164, 109.9989096053143669 ) ) ;
#310=CARTESIAN_POINT ( 'NONE',  ( -0.05219959533909027116, -19.03943276465977164, 67.49890960531436690 ) ) ;
#311=CARTESIAN_POINT ( 'NONE',  ( 15.80617190586746368, 15.72974639402197994, 99.37390960531436690 ) ) ;
#312=CARTESIAN_POINT ( 'NONE',  ( 16.51473224551069308, 9.474510206698969483, 94.16557627198103830 ) ) ;
#313=CARTESIAN_POINT ( 'NONE',  ( 19.02544592524343514, -5.153800228976328945, 23.54057627198102054 ) ) ;
#314=CARTESIAN_POINT ( 'NONE',  ( -9.564922557960796823, -16.46253265017161027, 67.08224293864769550 ) ) ;
#315=CARTESIAN_POINT ( 'NONE',  ( -12.06949235617739369, -12.14591786802326823, 109.3760903946857042 ) ) ;
#316=CARTESIAN_POINT ( 'NONE',  ( 9.474510206698971260, -16.51473224551069308, 27.91557627198103120 ) ) ;
#317=CARTESIAN_POINT ( 'NONE',  ( -9.474510206698720793, -16.51473224551083518, 34.58442372801899722 ) ) ;
#318=CARTESIAN_POINT ( 'NONE',  ( 12.14591786802309770, 12.06949235617756955, 59.37390960531436690 ) ) ;
#319=CARTESIAN_POINT ( 'NONE',  ( 21.55341960407619695, -5.719274019375665929, 101.0427570613523756 ) ) ;
#320=CARTESIAN_POINT ( 'NONE',  ( 19.05341960407611168, 5.049401038298154454, 38.95724293864767418 ) ) ;
#321=CARTESIAN_POINT ( 'NONE',  ( -8.224510206698735004, -14.34966873604973081, 54.58442372801901143 ) ) ;
#322=CARTESIAN_POINT ( 'NONE',  ( -8.224510206698948167, 14.34966873604960824, 45.41557627198103830 ) ) ;
#323=CARTESIAN_POINT ( 'NONE',  ( 18.67979575497194134, -10.72451020669871369, 85.83442372801901854 ) ) ;
#324=CARTESIAN_POINT ( 'NONE',  ( 13.89961937509977652, -13.97604488694527269, 83.12390960531436690 ) ) ;
#325=CARTESIAN_POINT ( 'NONE',  ( 5.049401038298161559, -19.05341960407611168, 92.70724293864769550 ) ) ;
#326=CARTESIAN_POINT ( 'NONE',  ( 16.53943276465976808, -0.05219959533910856209, 103.7489096053143669 ) ) ;
#327=CARTESIAN_POINT ( 'NONE',  ( 14.29746914071049879, -8.314922557960816363, 78.33224293864770971 ) ) ;
#328=CARTESIAN_POINT ( 'NONE',  ( 15.80617190586746368, 15.72974639402197994, 84.37390960531438111 ) ) ;
#329=CARTESIAN_POINT ( 'NONE',  ( 19.02544592524343514, -5.153800228976328945, 78.54057627198099567 ) ) ;
#330=CARTESIAN_POINT ( 'NONE',  ( 21.52544592524344225, -5.823673210054117533, 93.54057627198103830 ) ) ;
#331=CARTESIAN_POINT ( 'NONE',  ( 16.46253265017146816, 9.564922557961045513, 71.66775706135233293 ) ) ;
#332=CARTESIAN_POINT ( 'NONE',  ( 19.53037848336981952, -5.499999999999893419, 47.35532783611446916 ) ) ;
#333=CARTESIAN_POINT ( 'NONE',  ( -12.14591786802309592, -12.06949235617757132, 91.87390960531436690 ) ) ;
#334=CARTESIAN_POINT ( 'NONE',  ( 5.049401038298161559, -19.05341960407611168, 57.70724293864769550 ) ) ;
#335=CARTESIAN_POINT ( 'NONE',  ( 21.52544592524344225, -5.823673210054117533, 63.54057627198103830 ) ) ;
#336=CARTESIAN_POINT ( 'NONE',  ( -18.09867054820431775, -5.499999999999926281, 83.98393025253589883 ) ) ;
#337=CARTESIAN_POINT ( 'NONE',  ( 16.53943276465976808, -0.05219959533910856209, 23.74890960531435269 ) ) ;
#339=CARTESIAN_POINT ( 'NONE',  ( -0.05219959533934338120, 16.53943276465976808, 22.50109039468567573 ) ) ;
#340=CARTESIAN_POINT ( 'NONE',  ( -8.314922557960811034, -14.29746914071050412, 77.08224293864769550 ) ) ;
#341=CARTESIAN_POINT ( 'NONE',  ( -19.20446147854526231, -5.499999999999955591, 94.38999695167676407 ) ) ;
#342=CARTESIAN_POINT ( 'NONE',  ( -19.03943276465977164, 0.05219959533909376836, 76.24890960531435269 ) ) ;
#343=CARTESIAN_POINT ( 'NONE',  ( -16.46253265017160317, 9.564922557960807481, 35.83224293864768839 ) ) ;
#344=CARTESIAN_POINT ( 'NONE',  ( -8.224510206698948167, 14.34966873604960824, 65.41557627198102409 ) ) ;
#345=CARTESIAN_POINT ( 'NONE',  ( -10.81492255796078084, -18.62759615963271287, 22.08224293864769194 ) ) ;
#346=CARTESIAN_POINT ( 'NONE',  ( 5.153800228976615827, -19.02544592524334988, 95.20942372801897591 ) ) ;
#347=CARTESIAN_POINT ( 'NONE',  ( -19.03943276465977164, 0.05219959533909376836, 96.24890960531436690 ) ) ;
#348=CARTESIAN_POINT ( 'NONE',  ( -10.72451020669898014, 18.67979575497178502, 70.41557627198102409 ) ) ;
#349=CARTESIAN_POINT ( 'NONE',  ( 8.314922557961029526, -14.29746914071037800, 75.41775706135233293 ) ) ;
#350=CARTESIAN_POINT ( 'NONE',  ( -16.29526858892909758, 7.335722546919977383, 94.20329402199732272 ) ) ;
#351=CARTESIAN_POINT ( 'NONE',  ( 16.51473224551069308, 9.474510206698969483, 69.16557627198102409 ) ) ;
#352=CARTESIAN_POINT ( 'NONE',  ( 18.67979575497178502, 10.72451020669898547, 64.16557627198102409 ) ) ;
#353=CARTESIAN_POINT ( 'NONE',  ( 19.02544592524334988, 5.153800228976608722, 106.4594237280190185 ) ) ;
#354=CARTESIAN_POINT ( 'NONE',  ( -8.314922557960811034, -14.29746914071050412, 37.08224293864768129 ) ) ;
#355=CARTESIAN_POINT ( 'NONE',  ( 18.67979575497194134, -10.72451020669871369, 40.83442372801901854 ) ) ;
#357=CARTESIAN_POINT ( 'NONE',  ( 16.53943276465976808, 0.05219959533934440121, 76.25109039468568994 ) ) ;
#358=CARTESIAN_POINT ( 'NONE',  ( -0.05219959533909027116, -19.03943276465977164, 102.4989096053143669 ) ) ;
#359=CARTESIAN_POINT ( 'NONE',  ( 9.564922557960805705, 16.46253265017160317, 104.5822429386476955 ) ) ;
#361=CARTESIAN_POINT ( 'NONE',  ( -12.06949235617739369, -12.14591786802326823, 99.37609039468568994 ) ) ;
#362=CARTESIAN_POINT ( 'NONE',  ( 12.06949235617739724, 12.14591786802326823, 51.87609039468568284 ) ) ;
#363=CARTESIAN_POINT ( 'NONE',  ( -19.02544592524342804, 5.153800228976336051, 61.04057627198103120 ) ) ;
#364=CARTESIAN_POINT ( 'NONE',  ( 0.05219959533909260263, 19.03943276465977164, 69.99890960531435269 ) ) ;
#365=CARTESIAN_POINT ( 'NONE',  ( -18.62759615963255300, -10.81492255796106328, 54.16775706135235424 ) ) ;
#366=CARTESIAN_POINT ( 'NONE',  ( 14.34966873604972726, -8.224510206698740333, 65.83442372801900433 ) ) ;
#367=CARTESIAN_POINT ( 'NONE',  ( -0.05219959533910754901, -16.53943276465976808, 32.49890960531435979 ) ) ;
#368=CARTESIAN_POINT ( 'NONE',  ( -16.46253265017160317, 9.564922557960807481, 40.83224293864769550 ) ) ;
#369=CARTESIAN_POINT ( 'NONE',  ( -9.474510206698964154, 16.51473224551069663, 30.41557627198102054 ) ) ;
#370=CARTESIAN_POINT ( 'NONE',  ( -12.06949235617739369, -12.14591786802326823, 24.37609039468567573 ) ) ;
#371=CARTESIAN_POINT ( 'NONE',  ( 19.05341960407617918, -5.049401038297876454, 76.04275706135230450 ) ) ;
#372=CARTESIAN_POINT ( 'NONE',  ( -14.34966873604960291, -8.224510206698953496, 81.66557627198103830 ) ) ;
#373=CARTESIAN_POINT ( 'NONE',  ( -16.46253265017160317, 9.564922557960807481, 55.83224293864769550 ) ) ;
#374=CARTESIAN_POINT ( 'NONE',  ( 0.05219959533936267826, -19.03943276465977164, 85.00109039468567573 ) ) ;
#376=CARTESIAN_POINT ( 'NONE',  ( -21.52544592524334988, -5.823673210054445271, 93.95942372801903275 ) ) ;
#377=CARTESIAN_POINT ( 'NONE',  ( -14.34966873604972548, 8.224510206698743886, 48.33442372801902565 ) ) ;
#379=CARTESIAN_POINT ( 'NONE',  ( -15.80617190586745835, -15.72974639402198527, 51.87390960531437401 ) ) ;
#380=CARTESIAN_POINT ( 'NONE',  ( 16.55341960407618274, -4.379528057220086978, 36.04275706135234714 ) ) ;
#381=CARTESIAN_POINT ( 'NONE',  ( -19.35633801406909527, 5.499999999999580780, 69.13373818172763663 ) ) ;
#382=CARTESIAN_POINT ( 'NONE',  ( 9.564922557961047289, -16.46253265017146816, 45.41775706135232582 ) ) ;
#383=CARTESIAN_POINT ( 'NONE',  ( -19.03943276465977164, 0.05219959533909376836, 76.24890960531435269 ) ) ;
#384=CARTESIAN_POINT ( 'NONE',  ( 13.89961937509977652, -13.97604488694527269, 58.12390960531436690 ) ) ;
#385=CARTESIAN_POINT ( 'NONE',  ( 16.46253265017160672, -9.564922557960803928, 73.33224293864769550 ) ) ;
#386=CARTESIAN_POINT ( 'NONE',  ( -16.51473224551069308, -9.474510206698971260, 91.66557627198103830 ) ) ;
#387=CARTESIAN_POINT ( 'NONE',  ( -9.474510206698720793, -16.51473224551083518, 39.58442372801899722 ) ) ;
#388=CARTESIAN_POINT ( 'NONE',  ( 9.564922557961047289, -16.46253265017146816, 20.41775706135233293 ) ) ;
#389=CARTESIAN_POINT ( 'NONE',  ( -14.34966873604960291, -8.224510206698953496, 41.66557627198103120 ) ) ;
#390=CARTESIAN_POINT ( 'NONE',  ( 13.89961937509977652, -13.97604488694527269, 38.12390960531436690 ) ) ;
#391=CARTESIAN_POINT ( 'NONE',  ( -5.049401038298153566, 19.05341960407611168, 105.2072429386476671 ) ) ;
#392=CARTESIAN_POINT ( 'NONE',  ( -0.05219959533937732626, 21.53943276465977519, 82.50109039468568994 ) ) ;
#393=CARTESIAN_POINT ( 'NONE',  ( -13.97604488694527625, -13.89961937509977652, 56.87390960531434558 ) ) ;
#395=CARTESIAN_POINT ( 'NONE',  ( 18.67979575497194134, -10.72451020669871369, 85.83442372801901854 ) ) ;
#396=CARTESIAN_POINT ( 'NONE',  ( 18.67979575497178502, 10.72451020669898547, 39.16557627198102409 ) ) ;
#397=CARTESIAN_POINT ( 'NONE',  ( -15.80617190586768217, 15.72974639402176855, 23.12609039468567573 ) ) ;
#398=CARTESIAN_POINT ( 'NONE',  ( 19.05341960407617918, -5.049401038297876454, 51.04275706135231871 ) ) ;
#399=CARTESIAN_POINT ( 'NONE',  ( -0.05219959533909027116, -19.03943276465977164, 22.49890960531436690 ) ) ;
#400=CARTESIAN_POINT ( 'NONE',  ( 19.05341960407611168, 5.049401038298154454, 78.95724293864769550 ) ) ;
#401=CARTESIAN_POINT ( 'NONE',  ( 12.14591786802327356, -12.06949235617739191, 30.62609039468567929 ) ) ;
#402=CARTESIAN_POINT ( 'NONE',  ( -12.06949235617756955, 12.14591786802309770, 90.62390960531436690 ) ) ;
#403=CARTESIAN_POINT ( 'NONE',  ( -19.03943276465977164, 0.05219959533909376836, 56.24890960531435979 ) ) ;
#404=CARTESIAN_POINT ( 'NONE',  ( 0.05219959533907565091, 21.53943276465977519, 34.99890960531435979 ) ) ;
#405=CARTESIAN_POINT ( 'NONE',  ( -16.51473224551082808, 9.474510206698731452, 103.3344237280190043 ) ) ;
#406=CARTESIAN_POINT ( 'NONE',  ( -21.55341960407610458, -5.719274019375992779, 101.4572429386476955 ) ) ;
#407=CARTESIAN_POINT ( 'NONE',  ( 18.62759615963255655, 10.81492255796105972, 61.66775706135235424 ) ) ;
#408=CARTESIAN_POINT ( 'NONE',  ( -8.314922557961024197, 14.29746914071037800, 52.91775706135235424 ) ) ;
#409=CARTESIAN_POINT ( 'NONE',  ( -16.53943276465976808, -0.05219959533934237506, 73.75109039468567573 ) ) ;
#410=CARTESIAN_POINT ( 'NONE',  ( -13.89961937509977652, 13.97604488694528158, 60.62390960531436690 ) ) ;
#411=CARTESIAN_POINT ( 'NONE',  ( -16.53943276465976808, -0.05219959533934237506, 83.75109039468568994 ) ) ;
#412=CARTESIAN_POINT ( 'NONE',  ( -10.72451020669898014, 18.67979575497178502, 115.4155762719810241 ) ) ;
#413=CARTESIAN_POINT ( 'NONE',  ( -14.34966873604960291, -8.224510206698953496, 66.66557627198102409 ) ) ;
#414=CARTESIAN_POINT ( 'NONE',  ( 9.564922557960805705, 16.46253265017160317, 84.58224293864769550 ) ) ;
#415=CARTESIAN_POINT ( 'NONE',  ( 0.05219959533934541429, -16.53943276465976808, 75.00109039468568994 ) ) ;
#416=CARTESIAN_POINT ( 'NONE',  ( -5.719274019375665041, -21.55341960407619695, 54.79275706135235424 ) ) ;
#417=CARTESIAN_POINT ( 'NONE',  ( -0.05219959533934338120, 16.53943276465976808, 22.50109039468567573 ) ) ;
#418=CARTESIAN_POINT ( 'NONE',  ( -21.53943276465977519, -0.05219959533937600094, 18.75109039468568639 ) ) ;
#419=CARTESIAN_POINT ( 'NONE',  ( -4.379528057220328563, 16.55341960407611168, 60.20724293864768839 ) ) ;
#421=CARTESIAN_POINT ( 'NONE',  ( -17.26058549869091863, 6.457015423128480869, 73.62254162523936429 ) ) ;
#422=CARTESIAN_POINT ( 'NONE',  ( 21.53943276465977519, -0.05219959533907433946, 88.74890960531436690 ) ) ;
#423=CARTESIAN_POINT ( 'NONE',  ( 12.14591786802309770, 12.06949235617756955, 34.37390960531435979 ) ) ;
#426=CARTESIAN_POINT ( 'NONE',  ( -10.81492255796078084, -18.62759615963271287, 112.0822429386477097 ) ) ;
#427=CARTESIAN_POINT ( 'NONE',  ( -9.474510206698964154, 16.51473224551069663, 110.4155762719810383 ) ) ;
#428=CARTESIAN_POINT ( 'NONE',  ( 21.55341960407619695, -5.719274019375665929, 21.04275706135234714 ) ) ;
#429=CARTESIAN_POINT ( 'NONE',  ( -16.52544592524342804, 4.483927247898546575, 56.04057627198102409 ) ) ;
#430=CARTESIAN_POINT ( 'NONE',  ( -12.14591786802326823, 12.06949235617739902, 68.12609039468567573 ) ) ;
#431=CARTESIAN_POINT ( 'NONE',  ( -5.153800228976328057, -19.02544592524343514, 57.29057627198103120 ) ) ;
#432=CARTESIAN_POINT ( 'NONE',  ( -19.02544592524334988, -5.153800228976617603, 68.95942372801896170 ) ) ;
#433=CARTESIAN_POINT ( 'NONE',  ( -16.46253265017160317, 9.564922557960807481, 75.83224293864769550 ) ) ;
#434=CARTESIAN_POINT ( 'NONE',  ( -18.62759615963270932, 10.81492255796079327, 45.83224293864769550 ) ) ;
#436=CARTESIAN_POINT ( 'NONE',  ( 5.049401038298161559, -19.05341960407611168, 62.70724293864769550 ) ) ;
#437=CARTESIAN_POINT ( 'NONE',  ( -4.379528057220086978, -16.55341960407618274, 29.79275706135234358 ) ) ;
#438=CARTESIAN_POINT ( 'NONE',  ( -19.02544592524334988, -5.153800228976617603, 63.95942372801899012 ) ) ;
#439=CARTESIAN_POINT ( 'NONE',  ( 21.55341960407610458, 5.719274019375980345, 113.9572429386477239 ) ) ;
#440=CARTESIAN_POINT ( 'NONE',  ( 0.05219959533910956823, 16.53943276465976808, 49.99890960531437401 ) ) ;
#441=CARTESIAN_POINT ( 'NONE',  ( -16.46253265017160317, 9.564922557960807481, 95.83224293864769550 ) ) ;
#442=CARTESIAN_POINT ( 'NONE',  ( 21.55341960407610458, 5.719274019375980345, 58.95724293864770971 ) ) ;
#443=CARTESIAN_POINT ( 'NONE',  ( 21.52544592524344225, -5.823673210054117533, 93.54057627198103830 ) ) ;
#444=CARTESIAN_POINT ( 'NONE',  ( -0.05219959533934338120, 16.53943276465976808, 32.50109039468568284 ) ) ;
#445=CARTESIAN_POINT ( 'NONE',  ( -21.55341960407610458, -5.719274019375992779, 41.45724293864769550 ) ) ;
#446=CARTESIAN_POINT ( 'NONE',  ( -0.05219959533937732626, 21.53943276465977519, 82.50109039468568994 ) ) ;
#447=CARTESIAN_POINT ( 'NONE',  ( -13.97604488694527625, -13.89961937509977652, 81.87390960531436690 ) ) ;
#448=CARTESIAN_POINT ( 'NONE',  ( -9.564922557960796823, -16.46253265017161027, 37.08224293864768839 ) ) ;
#449=CARTESIAN_POINT ( 'NONE',  ( -16.51473224551069308, -9.474510206698971260, 101.6655762719810241 ) ) ;
#450=CARTESIAN_POINT ( 'NONE',  ( 16.52544592524342804, -4.483927247898539470, 103.5405762719810383 ) ) ;
#451=CARTESIAN_POINT ( 'NONE',  ( -9.474510206698964154, 16.51473224551069663, 65.41557627198102409 ) ) ;
#452=CARTESIAN_POINT ( 'NONE',  ( -19.05341960407617563, 5.049401038297882671, 113.5427570613523471 ) ) ;
#453=CARTESIAN_POINT ( 'NONE',  ( 17.50000000000001776, 3.471454075611646761, 33.01667418855640790 ) ) ;
#454=CARTESIAN_POINT ( 'NONE',  ( 10.72451020669871369, 18.67979575497193778, 97.08442372801904696 ) ) ;
#455=CARTESIAN_POINT ( 'NONE',  ( -0.05219959533907301413, -21.53943276465977519, 32.49890960531435979 ) ) ;
#456=CARTESIAN_POINT ( 'NONE',  ( -4.483927247898782831, 16.52544592524335698, 87.70942372801901854 ) ) ;
#458=CARTESIAN_POINT ( 'NONE',  ( -19.03943276465977164, -0.05219959533935918106, 63.75109039468566863 ) ) ;
#459=CARTESIAN_POINT ( 'NONE',  ( -19.02544592524334988, -5.153800228976617603, 33.95942372801897591 ) ) ;
#461=CARTESIAN_POINT ( 'NONE',  ( 19.02544592524343514, -5.153800228976328945, 28.54057627198102409 ) ) ;
#462=CARTESIAN_POINT ( 'NONE',  ( -8.314922557960811034, -14.29746914071050412, 37.08224293864768129 ) ) ;
#463=CARTESIAN_POINT ( 'NONE',  ( -19.03943276465977164, 0.05219959533909376836, 21.24890960531436335 ) ) ;
#464=CARTESIAN_POINT ( 'NONE',  ( -14.29746914071049879, 8.314922557960819915, 25.83224293864769194 ) ) ;
#466=CARTESIAN_POINT ( 'NONE',  ( 8.224510206698742110, 14.34966873604972548, 92.08442372801901854 ) ) ;
#467=CARTESIAN_POINT ( 'NONE',  ( -16.51473224551069308, -9.474510206698971260, 31.66557627198102054 ) ) ;
#469=CARTESIAN_POINT ( 'NONE',  ( -19.03943276465977164, -0.05219959533935918106, 18.75109039468567218 ) ) ;
#470=CARTESIAN_POINT ( 'NONE',  ( -12.06949235617739369, -12.14591786802326823, 24.37609039468567573 ) ) ;
#471=CARTESIAN_POINT ( 'NONE',  ( 15.72974639402176855, 15.80617190586768217, 81.87609039468568994 ) ) ;
#472=CARTESIAN_POINT ( 'NONE',  ( -19.02544592524334988, -5.153800228976617603, 53.95942372801898301 ) ) ;
#473=CARTESIAN_POINT ( 'NONE',  ( 19.03943276465977164, -0.05219959533909143690, 93.74890960531435269 ) ) ;
#474=CARTESIAN_POINT ( 'NONE',  ( 13.89961937509977652, -13.97604488694527269, 73.12390960531436690 ) ) ;
#475=CARTESIAN_POINT ( 'NONE',  ( -18.22780087662122028, 5.500000000000031086, 38.51540105326107266 ) ) ;
#476=CARTESIAN_POINT ( 'NONE',  ( -10.81492255796078084, -18.62759615963271287, 102.0822429386476955 ) ) ;
#477=CARTESIAN_POINT ( 'NONE',  ( 16.53943276465976808, -0.05219959533910856209, 68.74890960531435269 ) ) ;
#478=CARTESIAN_POINT ( 'NONE',  ( -18.67979575497178146, -10.72451020669898902, 56.66557627198103830 ) ) ;
#479=CARTESIAN_POINT ( 'NONE',  ( -9.564922557960796823, -16.46253265017161027, 62.08224293864769550 ) ) ;
#480=CARTESIAN_POINT ( 'NONE',  ( 0.05219959533907565091, 21.53943276465977519, 89.99890960531438111 ) ) ;
#481=CARTESIAN_POINT ( 'NONE',  ( 14.29746914071037800, 8.314922557961029526, 76.66775706135234714 ) ) ;
#484=CARTESIAN_POINT ( 'NONE',  ( -16.46253265017160317, 9.564922557960807481, 50.83224293864770260 ) ) ;
#485=CARTESIAN_POINT ( 'NONE',  ( -16.55341960407611168, -4.379528057220339221, 91.45724293864769550 ) ) ;
#487=CARTESIAN_POINT ( 'NONE',  ( 16.51473224551069308, 9.474510206698969483, 44.16557627198103120 ) ) ;
#488=CARTESIAN_POINT ( 'NONE',  ( 14.34966873604960469, 8.224510206698951720, 114.1655762719810383 ) ) ;
#489=CARTESIAN_POINT ( 'NONE',  ( -5.153800228976607833, 19.02544592524334988, 62.70942372801899722 ) ) ;
#490=CARTESIAN_POINT ( 'NONE',  ( -8.314922557960811034, -14.29746914071050412, 87.08224293864769550 ) ) ;
#491=CARTESIAN_POINT ( 'NONE',  ( 5.823673210054444382, -21.52544592524334988, 45.20942372801901854 ) ) ;
#492=CARTESIAN_POINT ( 'NONE',  ( 19.03943276465977164, -0.05219959533909143690, 38.74890960531436690 ) ) ;
#493=CARTESIAN_POINT ( 'NONE',  ( 15.80617190586746368, 15.72974639402197994, 109.3739096053143811 ) ) ;
#494=CARTESIAN_POINT ( 'NONE',  ( 16.53943276465976808, -0.05219959533910856209, 83.74890960531435269 ) ) ;
#496=B_SPLINE_CURVE_WITH_KNOTS ( 'NONE', 3,
 ( #116941, #89601, #151289, #149289, #100764, #162446, #23947, #117955, #85601, #178634, #147288, #70447, #132113, #86606, #55272, #148289, #9783, #123892, #138089, #105763, #32904, #171418, #125899, #139075, #1553, #61237 ),
 .UNSPECIFIED., .F., .F.,
 ( 4, 2, 2, 2, 2, 2, 2, 2, 2, 2, 2, 2, 4 ),
 ( 0.000000000000000000, 0.0004878035110667099800, 0.0007317052666000649699, 0.0009756070221334199599, 0.001097557899900097455, 0.001219508777666774950, 0.001341459655433452445, 0.001463410533200129940, 0.001707312288733484930, 0.001951214044266839920, 0.002439017555333544696, 0.002926821066400249038, 0.003902428088533665095 ),
 .UNSPECIFIED. ) ;
#497=CARTESIAN_POINT ( 'NONE',  ( 13.97604488694527802, 13.89961937509977652, 64.37390960531436690 ) ) ;
#498=CARTESIAN_POINT ( 'NONE',  ( 19.39056639909671276, 5.500000000000041744, 48.28948781074346641 ) ) ;
#499=CARTESIAN_POINT ( 'NONE',  ( 19.03943276465977164, 0.05219959533936151252, 96.25109039468567573 ) ) ;
#500=CARTESIAN_POINT ( 'NONE',  ( 13.89961937509977652, -13.97604488694527269, 103.1239096053143527 ) ) ;
#501=CARTESIAN_POINT ( 'NONE',  ( 5.823673210054444382, -21.52544592524334988, 30.20942372801902565 ) ) ;
#502=CARTESIAN_POINT ( 'NONE',  ( 16.46253265017160672, -9.564922557960803928, 88.33224293864769550 ) ) ;
#503=CARTESIAN_POINT ( 'NONE',  ( -16.46253265017146816, -9.564922557961047289, 69.16775706135233293 ) ) ;
#504=CARTESIAN_POINT ( 'NONE',  ( 9.564922557960805705, 16.46253265017160317, 59.58224293864769550 ) ) ;
#505=CARTESIAN_POINT ( 'NONE',  ( -14.34966873604960291, -8.224510206698953496, 71.66557627198100988 ) ) ;
#506=CARTESIAN_POINT ( 'NONE',  ( -0.05219959533910754901, -16.53943276465976808, 67.49890960531436690 ) ) ;
#507=CARTESIAN_POINT ( 'NONE',  ( 0.05219959533909260263, 19.03943276465977164, 89.99890960531436690 ) ) ;
#508=CARTESIAN_POINT ( 'NONE',  ( 5.823673210054125526, 21.52544592524343514, 104.7905762719810241 ) ) ;
#509=CARTESIAN_POINT ( 'NONE',  ( -5.049401038298153566, 19.05341960407611168, 90.20724293864766707 ) ) ;
#510=CARTESIAN_POINT ( 'NONE',  ( -5.153800228976607833, 19.02544592524334988, 27.70942372801899722 ) ) ;
#511=CARTESIAN_POINT ( 'NONE',  ( -9.474510206698964154, 16.51473224551069663, 30.41557627198102054 ) ) ;
#512=CARTESIAN_POINT ( 'NONE',  ( 16.53943276465976808, -0.05219959533910856209, 28.74890960531435624 ) ) ;
#513=CARTESIAN_POINT ( 'NONE',  ( 14.34966873604960469, 8.224510206698951720, 114.1655762719810383 ) ) ;
#514=CARTESIAN_POINT ( 'NONE',  ( 19.03943276465977164, 0.05219959533936151252, 106.2510903946856615 ) ) ;
#516=CARTESIAN_POINT ( 'NONE',  ( -0.05219959533937732626, 21.53943276465977519, 32.50109039468568284 ) ) ;
#517=CARTESIAN_POINT ( 'NONE',  ( 19.02544592524334988, 5.153800228976608722, 71.45942372801900433 ) ) ;
#518=CARTESIAN_POINT ( 'NONE',  ( -16.55341960407611168, -4.379528057220339221, 26.45724293864768839 ) ) ;
#519=CARTESIAN_POINT ( 'NONE',  ( 18.67979575497178502, 10.72451020669898547, 84.16557627198103830 ) ) ;
#520=CARTESIAN_POINT ( 'NONE',  ( -13.89961937509977652, 13.97604488694528158, 115.6239096053143669 ) ) ;
#521=CARTESIAN_POINT ( 'NONE',  ( 12.14591786802309770, 12.06949235617756955, 64.37390960531435269 ) ) ;
#522=CARTESIAN_POINT ( 'NONE',  ( -0.05219959533909027116, -19.03943276465977164, 32.49890960531435979 ) ) ;
#523=CARTESIAN_POINT ( 'NONE',  ( -5.153800228976607833, 19.02544592524334988, 27.70942372801899722 ) ) ;
#524=CARTESIAN_POINT ( 'NONE',  ( -4.483927247898782831, 16.52544592524335698, 92.70942372801901854 ) ) ;
#525=CARTESIAN_POINT ( 'NONE',  ( 14.34966873604972726, -8.224510206698740333, 50.83442372801901143 ) ) ;
#526=CARTESIAN_POINT ( 'NONE',  ( -21.55341960407610458, -5.719274019375992779, 21.45724293864769550 ) ) ;
#527=CARTESIAN_POINT ( 'NONE',  ( -18.67979575497193778, 10.72451020669871902, 113.3344237280190328 ) ) ;
#528=CARTESIAN_POINT ( 'NONE',  ( 9.564922557960805705, 16.46253265017160317, 79.58224293864769550 ) ) ;
#529=CARTESIAN_POINT ( 'NONE',  ( 0.05219959533934541429, -16.53943276465976808, 60.00109039468568284 ) ) ;
#530=CARTESIAN_POINT ( 'NONE',  ( -9.564922557960796823, -16.46253265017161027, 27.08224293864769550 ) ) ;
#531=CARTESIAN_POINT ( 'NONE',  ( 16.52544592524342804, -4.483927247898539470, 33.54057627198102409 ) ) ;
#532=CARTESIAN_POINT ( 'NONE',  ( -17.97161686093727795, 5.499999999999975131, 70.99637206859166838 ) ) ;
#533=CARTESIAN_POINT ( 'NONE',  ( -19.05341960407611168, -5.049401038298163336, 106.4572429386476955 ) ) ;
#534=CARTESIAN_POINT ( 'NONE',  ( 13.97604488694527802, 13.89961937509977652, 89.37390960531436690 ) ) ;
#535=CARTESIAN_POINT ( 'NONE',  ( 19.05341960407611168, 5.049401038298154454, 113.9572429386477097 ) ) ;
#536=CARTESIAN_POINT ( 'NONE',  ( -8.314922557960811034, -14.29746914071050412, 57.08224293864769550 ) ) ;
#537=CARTESIAN_POINT ( 'NONE',  ( 16.55341960407611168, 4.379528057220329451, 33.95724293864769550 ) ) ;
#538=CARTESIAN_POINT ( 'NONE',  ( 16.52544592524342804, -4.483927247898539470, 58.54057627198103120 ) ) ;
#539=CARTESIAN_POINT ( 'NONE',  ( -14.29746914071037622, -8.314922557961029526, 44.16775706135234714 ) ) ;
#541=CARTESIAN_POINT ( 'NONE',  ( -13.89961937509957401, -13.97604488694547875, 54.37609039468565442 ) ) ;
#542=CARTESIAN_POINT ( 'NONE',  ( 16.51473224551069308, 9.474510206698969483, 74.16557627198103830 ) ) ;
#543=CARTESIAN_POINT ( 'NONE',  ( 19.03943276465977164, 0.05219959533936151252, 66.25109039468567573 ) ) ;
#545=CARTESIAN_POINT ( 'NONE',  ( 16.51473224551083163, -9.474510206698727899, 55.83442372801899722 ) ) ;
#546=CARTESIAN_POINT ( 'NONE',  ( 5.153800228976615827, -19.02544592524334988, 100.2094237280190043 ) ) ;
#547=CARTESIAN_POINT ( 'NONE',  ( -16.55341960407617563, 4.379528057220093196, 78.54275706135236135 ) ) ;
#549=CARTESIAN_POINT ( 'NONE',  ( 19.02544592524343514, -5.153800228976328945, 23.54057627198102054 ) ) ;
#550=CARTESIAN_POINT ( 'NONE',  ( -13.89961937509977652, 13.97604488694528158, 105.6239096053143527 ) ) ;
#551=CARTESIAN_POINT ( 'NONE',  ( -21.55341960407619339, 5.719274019375674811, 43.54275706135235424 ) ) ;
#552=CARTESIAN_POINT ( 'NONE',  ( 0.05219959533936267826, -19.03943276465977164, 100.0010903946856757 ) ) ;
#554=CARTESIAN_POINT ( 'NONE',  ( 9.474510206698971260, -16.51473224551069308, 57.91557627198103120 ) ) ;
#555=CARTESIAN_POINT ( 'NONE',  ( -0.05219959533909027116, -19.03943276465977164, 102.4989096053143669 ) ) ;
#556=CARTESIAN_POINT ( 'NONE',  ( -12.06949235617756955, 12.14591786802309770, 65.62390960531436690 ) ) ;
#557=CARTESIAN_POINT ( 'NONE',  ( -13.97604488694527625, -13.89961937509977652, 56.87390960531434558 ) ) ;
#558=CARTESIAN_POINT ( 'NONE',  ( 13.89961937509977652, -13.97604488694527269, 58.12390960531436690 ) ) ;
#559=CARTESIAN_POINT ( 'NONE',  ( 13.89961937509957401, 13.97604488694547697, 81.87609039468564731 ) ) ;
#560=CARTESIAN_POINT ( 'NONE',  ( -15.80617190586745835, -15.72974639402198527, 51.87390960531437401 ) ) ;
#561=CARTESIAN_POINT ( 'NONE',  ( -9.474510206698720793, -16.51473224551083518, 49.58442372801899722 ) ) ;
#562=CARTESIAN_POINT ( 'NONE',  ( -13.97604488694527625, -13.89961937509977652, 76.87390960531433848 ) ) ;
#563=CARTESIAN_POINT ( 'NONE',  ( -18.62759615963270932, 10.81492255796079327, 80.83224293864769550 ) ) ;
#564=CARTESIAN_POINT ( 'NONE',  ( 16.53943276465976808, -0.05219959533910856209, 83.74890960531435269 ) ) ;
#565=CARTESIAN_POINT ( 'NONE',  ( -9.564922557961040184, 16.46253265017147172, 37.91775706135233293 ) ) ;
#566=CARTESIAN_POINT ( 'NONE',  ( 0.05219959533907565091, 21.53943276465977519, 54.99890960531435269 ) ) ;
#567=CARTESIAN_POINT ( 'NONE',  ( 15.80617190586746368, 15.72974639402197994, 39.37390960531436690 ) ) ;
#568=CARTESIAN_POINT ( 'NONE',  ( -13.89961937509977652, 13.97604488694528158, 70.62390960531432427 ) ) ;
#569=CARTESIAN_POINT ( 'NONE',  ( 16.53943276465976808, -0.05219959533910856209, 108.7489096053143669 ) ) ;
#570=CARTESIAN_POINT ( 'NONE',  ( -21.53943276465977519, -0.05219959533937600094, 23.75109039468567929 ) ) ;
#571=CARTESIAN_POINT ( 'NONE',  ( -18.22780087662126647, -5.499999999999827693, 48.98236817873107185 ) ) ;
#572=CARTESIAN_POINT ( 'NONE',  ( 15.80617190586769283, -15.72974639402175789, 45.62609039468567573 ) ) ;
#573=CARTESIAN_POINT ( 'NONE',  ( -19.03943276465977164, 0.05219959533909376836, 31.24890960531435979 ) ) ;
#574=CARTESIAN_POINT ( 'NONE',  ( -18.67979575497178146, -10.72451020669898902, 111.6655762719810525 ) ) ;
#575=CARTESIAN_POINT ( 'NONE',  ( -13.97604488694547697, 13.89961937509957934, 43.12609039468566152 ) ) ;
#576=CARTESIAN_POINT ( 'NONE',  ( 0.05219959533909260263, 19.03943276465977164, 24.99890960531435269 ) ) ;
#577=CARTESIAN_POINT ( 'NONE',  ( 19.35633801406909171, -5.499999999999570122, 76.63373818172759400 ) ) ;
#578=CARTESIAN_POINT ( 'NONE',  ( 17.35746358384380628, -5.713263725054876119, 21.25662004187655185 ) ) ;
#579=CARTESIAN_POINT ( 'NONE',  ( 16.53943276465976808, 0.05219959533934440121, 56.25109039468568284 ) ) ;
#580=CARTESIAN_POINT ( 'NONE',  ( -9.564922557960796823, -16.46253265017161027, 22.08224293864768839 ) ) ;
#582=CARTESIAN_POINT ( 'NONE',  ( 5.153800228976335163, 19.02544592524342804, 74.79057627198103830 ) ) ;
#583=CARTESIAN_POINT ( 'NONE',  ( 16.53943276465976808, -0.05219959533910856209, 103.7489096053143669 ) ) ;
#585=CARTESIAN_POINT ( 'NONE',  ( 0.05219959533907565091, 21.53943276465977519, 64.99890960531435269 ) ) ;
#586=CARTESIAN_POINT ( 'NONE',  ( -4.379528057220086978, -16.55341960407618274, 39.79275706135235424 ) ) ;
#587=CARTESIAN_POINT ( 'NONE',  ( -0.05219959533937732626, 21.53943276465977519, 102.5010903946856899 ) ) ;
#588=EDGE_CURVE ( 'NONE', #47139, #178804, #190478, .T. ) ;
#590=CARTESIAN_POINT ( 'NONE',  ( 4.483927247898545687, 16.52544592524342804, 24.79057627198103120 ) ) ;
#591=CARTESIAN_POINT ( 'NONE',  ( 16.53943276465976808, -0.05219959533910856209, 48.74890960531435979 ) ) ;
#592=CARTESIAN_POINT ( 'NONE',  ( 16.46253265017160672, -9.564922557960803928, 48.33224293864769550 ) ) ;
#593=CARTESIAN_POINT ( 'NONE',  ( -21.52544592524334988, -5.823673210054445271, 93.95942372801903275 ) ) ;
#594=CARTESIAN_POINT ( 'NONE',  ( -5.823673210054116645, -21.52544592524344225, 112.2905762719810241 ) ) ;
#595=CARTESIAN_POINT ( 'NONE',  ( 10.72451020669871369, 18.67979575497193778, 67.08442372801901854 ) ) ;
#596=CARTESIAN_POINT ( 'NONE',  ( 14.29746914071037800, 8.314922557961029526, 56.66775706135235424 ) ) ;
#597=CARTESIAN_POINT ( 'NONE',  ( 16.55341960407611168, 4.379528057220329451, 73.95724293864769550 ) ) ;
#598=CARTESIAN_POINT ( 'NONE',  ( -5.719274019375665041, -21.55341960407619695, 104.7927570613523898 ) ) ;
#600=CARTESIAN_POINT ( 'NONE',  ( -8.314922557961024197, 14.29746914071037800, 112.9177570613523329 ) ) ;
#602=CARTESIAN_POINT ( 'NONE',  ( -14.29746914071037622, -8.314922557961029526, 44.16775706135234714 ) ) ;
#603=CARTESIAN_POINT ( 'NONE',  ( -12.06949235617756955, 12.14591786802309770, 40.62390960531435269 ) ) ;
#604=CARTESIAN_POINT ( 'NONE',  ( 16.55341960407618274, -4.379528057220086978, 81.04275706135236135 ) ) ;
#605=CARTESIAN_POINT ( 'NONE',  ( 5.153800228976335163, 19.02544592524342804, 94.79057627198103830 ) ) ;
#606=CARTESIAN_POINT ( 'NONE',  ( 5.153800228976335163, 19.02544592524342804, 109.7905762719810099 ) ) ;
#607=CARTESIAN_POINT ( 'NONE',  ( 10.81492255796106328, -18.62759615963255655, 95.41775706135234714 ) ) ;
#608=CARTESIAN_POINT ( 'NONE',  ( 16.53943276465976808, 0.05219959533934440121, 96.25109039468568994 ) ) ;
#609=CARTESIAN_POINT ( 'NONE',  ( -4.379528057220328563, 16.55341960407611168, 75.20724293864769550 ) ) ;
#610=CARTESIAN_POINT ( 'NONE',  ( -19.05341960407611168, -5.049401038298163336, 76.45724293864769550 ) ) ;
#612=CARTESIAN_POINT ( 'NONE',  ( 12.06949235617739724, 12.14591786802326823, 31.87609039468567929 ) ) ;
#613=CARTESIAN_POINT ( 'NONE',  ( -16.51473224551069308, -9.474510206698971260, 26.66557627198103120 ) ) ;
#614=CARTESIAN_POINT ( 'NONE',  ( 13.89961937509977652, -13.97604488694527269, 88.12390960531438111 ) ) ;
#615=CARTESIAN_POINT ( 'NONE',  ( -8.224510206698735004, -14.34966873604973081, 34.58442372801900433 ) ) ;
#617=CARTESIAN_POINT ( 'NONE',  ( -9.564922557961040184, 16.46253265017147172, 37.91775706135233293 ) ) ;
#618=CARTESIAN_POINT ( 'NONE',  ( -4.379528057220086978, -16.55341960407618274, 89.79275706135236135 ) ) ;
#619=CARTESIAN_POINT ( 'NONE',  ( 16.46253265017160672, -9.564922557960803928, 28.33224293864769550 ) ) ;
#620=CARTESIAN_POINT ( 'NONE',  ( 16.53943276465976808, 0.05219959533934440121, 81.25109039468568994 ) ) ;
#621=CARTESIAN_POINT ( 'NONE',  ( 16.52544592524335698, 4.483927247898782831, 71.45942372801901854 ) ) ;
#622=CARTESIAN_POINT ( 'NONE',  ( -16.51473224551082808, 9.474510206698731452, 88.33442372801900433 ) ) ;
#623=CARTESIAN_POINT ( 'NONE',  ( -16.46253265017146816, -9.564922557961047289, 34.16775706135233293 ) ) ;
#624=CARTESIAN_POINT ( 'NONE',  ( 5.049401038298161559, -19.05341960407611168, 42.70724293864767418 ) ) ;
#625=CARTESIAN_POINT ( 'NONE',  ( 16.53943276465976808, -0.05219959533910856209, 88.74890960531436690 ) ) ;
#626=CARTESIAN_POINT ( 'NONE',  ( 5.153800228976615827, -19.02544592524334988, 50.20942372801897591 ) ) ;
#627=CARTESIAN_POINT ( 'NONE',  ( 5.719274019375991003, -21.55341960407610458, 47.70724293864770260 ) ) ;
#628=CARTESIAN_POINT ( 'NONE',  ( -16.46253265017146816, -9.564922557961047289, 34.16775706135233293 ) ) ;
#629=CARTESIAN_POINT ( 'NONE',  ( 9.474510206698971260, -16.51473224551069308, 102.9155762719810241 ) ) ;
#631=CARTESIAN_POINT ( 'NONE',  ( -10.72451020669898014, 18.67979575497178502, 75.41557627198102409 ) ) ;
#632=CARTESIAN_POINT ( 'NONE',  ( 9.564922557960805705, 16.46253265017160317, 114.5822429386476955 ) ) ;
#633=CARTESIAN_POINT ( 'NONE',  ( -5.153800228976607833, 19.02544592524334988, 92.70942372801901854 ) ) ;
#634=CARTESIAN_POINT ( 'NONE',  ( -17.49999999999999645, 3.565345528327981128, 109.4249448680647561 ) ) ;
#635=CARTESIAN_POINT ( 'NONE',  ( -19.05341960407617563, 5.049401038297882671, 108.5427570613523187 ) ) ;
#636=CARTESIAN_POINT ( 'NONE',  ( -19.05341960407611168, -5.049401038298163336, 31.45724293864769550 ) ) ;
#637=CARTESIAN_POINT ( 'NONE',  ( -9.564922557960796823, -16.46253265017161027, 92.08224293864769550 ) ) ;
#638=CARTESIAN_POINT ( 'NONE',  ( -18.62759615963270932, 10.81492255796079327, 80.83224293864769550 ) ) ;
#639=CARTESIAN_POINT ( 'NONE',  ( 4.379528057220092307, 16.55341960407617563, 42.29275706135235424 ) ) ;
#640=CARTESIAN_POINT ( 'NONE',  ( -5.823673210054431948, 21.52544592524334988, 42.70942372801901854 ) ) ;
#641=CARTESIAN_POINT ( 'NONE',  ( -9.564922557961040184, 16.46253265017147172, 87.91775706135233293 ) ) ;
#642=CARTESIAN_POINT ( 'NONE',  ( 16.46253265017146816, 9.564922557961045513, 21.66775706135233648 ) ) ;
#643=CARTESIAN_POINT ( 'NONE',  ( -8.224510206698735004, -14.34966873604973081, 104.5844237280190185 ) ) ;
#644=CARTESIAN_POINT ( 'NONE',  ( 0.05219959533909260263, 19.03943276465977164, 104.9989096053143669 ) ) ;
#645=CARTESIAN_POINT ( 'NONE',  ( -14.29746914071049879, 8.314922557960819915, 85.83224293864768129 ) ) ;
#646=CARTESIAN_POINT ( 'NONE',  ( 16.55341960407611168, 4.379528057220329451, 38.95724293864768839 ) ) ;
#647=CARTESIAN_POINT ( 'NONE',  ( -19.02544592524334988, -5.153800228976617603, 83.95942372801901854 ) ) ;
#648=CARTESIAN_POINT ( 'NONE',  ( -21.52544592524334988, -5.823673210054445271, 63.95942372801901854 ) ) ;
#649=CARTESIAN_POINT ( 'NONE',  ( -19.05341960407617563, 5.049401038297882671, 23.54275706135233648 ) ) ;
#650=CARTESIAN_POINT ( 'NONE',  ( 4.379528057220339221, -16.55341960407611168, 107.7072429386476955 ) ) ;
#651=CARTESIAN_POINT ( 'NONE',  ( -10.72451020669898014, 18.67979575497178502, 35.41557627198102409 ) ) ;
#652=CARTESIAN_POINT ( 'NONE',  ( -14.34966873604960291, -8.224510206698953496, 26.66557627198103475 ) ) ;
#653=CARTESIAN_POINT ( 'NONE',  ( 21.55341960407619695, -5.719274019375665929, 101.0427570613523756 ) ) ;
#654=CARTESIAN_POINT ( 'NONE',  ( 4.483927247898790824, -16.52544592524335698, 55.20942372801902565 ) ) ;
#655=CARTESIAN_POINT ( 'NONE',  ( -14.34966873604960291, -8.224510206698953496, 21.66557627198102409 ) ) ;
#656=CARTESIAN_POINT ( 'NONE',  ( 10.72451020669871369, 18.67979575497193778, 57.08442372801901854 ) ) ;
#657=CARTESIAN_POINT ( 'NONE',  ( 21.53943276465977519, 0.05219959533937863772, 56.25109039468568284 ) ) ;
#658=VERTEX_POINT ( 'NONE', #196492 ) ;
#659=CARTESIAN_POINT ( 'NONE',  ( 16.46253265017160672, -9.564922557960803928, 63.33224293864769550 ) ) ;
#660=CARTESIAN_POINT ( 'NONE',  ( 21.52544592524334988, 5.823673210054432836, 31.45942372801901854 ) ) ;
#661=CARTESIAN_POINT ( 'NONE',  ( -8.314922557960811034, -14.29746914071050412, 102.0822429386476955 ) ) ;
#662=CARTESIAN_POINT ( 'NONE',  ( -13.89961937509977652, 13.97604488694528158, 30.62390960531435269 ) ) ;
#663=CARTESIAN_POINT ( 'NONE',  ( -4.379528057220328563, 16.55341960407611168, 85.20724293864770971 ) ) ;
#664=CARTESIAN_POINT ( 'NONE',  ( 9.474510206698971260, -16.51473224551069308, 67.91557627198102409 ) ) ;
#665=CARTESIAN_POINT ( 'NONE',  ( 14.29746914071049879, -8.314922557960816363, 28.33224293864769550 ) ) ;
#666=CARTESIAN_POINT ( 'NONE',  ( -18.67979575497178146, -10.72451020669898902, 51.66557627198102409 ) ) ;
#667=CARTESIAN_POINT ( 'NONE',  ( 4.483927247898545687, 16.52544592524342804, 89.79057627198103830 ) ) ;
#668=CARTESIAN_POINT ( 'NONE',  ( -21.52544592524343514, 5.823673210054127303, 91.04057627198103830 ) ) ;
#669=CARTESIAN_POINT ( 'NONE',  ( 19.03943276465977164, -0.05219959533909143690, 103.7489096053143669 ) ) ;
#670=CARTESIAN_POINT ( 'NONE',  ( -19.05341960407611168, -5.049401038298163336, 46.45724293864768129 ) ) ;
#671=CARTESIAN_POINT ( 'NONE',  ( -9.564922557961040184, 16.46253265017147172, 102.9177570613523329 ) ) ;
#672=CARTESIAN_POINT ( 'NONE',  ( -10.81492255796078084, -18.62759615963271287, 42.08224293864769550 ) ) ;
#673=CARTESIAN_POINT ( 'NONE',  ( 21.55341960407619695, -5.719274019375665929, 86.04275706135236135 ) ) ;
#674=CARTESIAN_POINT ( 'NONE',  ( 9.474510206698971260, -16.51473224551069308, 72.91557627198102409 ) ) ;
#675=CARTESIAN_POINT ( 'NONE',  ( 13.89961937509977652, -13.97604488694527269, 103.1239096053143527 ) ) ;
#676=CARTESIAN_POINT ( 'NONE',  ( 16.52544592524335698, 4.483927247898782831, 76.45942372801901854 ) ) ;
#677=CARTESIAN_POINT ( 'NONE',  ( 10.72451020669871369, 18.67979575497193778, 57.08442372801901854 ) ) ;
#678=CARTESIAN_POINT ( 'NONE',  ( 15.72974639402176855, 15.80617190586768217, 86.87609039468568994 ) ) ;
#679=CARTESIAN_POINT ( 'NONE',  ( -15.72974639402176322, -15.80617190586768395, 19.37609039468568639 ) ) ;
#680=CARTESIAN_POINT ( 'NONE',  ( -18.67979575497193778, 10.72451020669871902, 43.33442372801901143 ) ) ;
#681=CARTESIAN_POINT ( 'NONE',  ( -14.29746914071037622, -8.314922557961029526, 79.16775706135234714 ) ) ;
#682=CARTESIAN_POINT ( 'NONE',  ( -21.55341960407610458, -5.719274019375992779, 76.45724293864769550 ) ) ;
#683=CARTESIAN_POINT ( 'NONE',  ( -5.153800228976607833, 19.02544592524334988, 32.70942372801899722 ) ) ;
#684=CARTESIAN_POINT ( 'NONE',  ( 21.52544592524344225, -5.823673210054117533, 43.54057627198103830 ) ) ;
#685=CARTESIAN_POINT ( 'NONE',  ( -16.46253265017160317, 9.564922557960807481, 75.83224293864769550 ) ) ;
#686=CARTESIAN_POINT ( 'NONE',  ( -12.14591786802309592, -12.06949235617757132, 26.87390960531435979 ) ) ;
#687=CARTESIAN_POINT ( 'NONE',  ( -17.44270441346512612, 5.991230190323082461, 63.63664920735770636 ) ) ;
#688=CARTESIAN_POINT ( 'NONE',  ( -19.02544592524342804, 5.153800228976336051, 106.0405762719810241 ) ) ;
#690=CARTESIAN_POINT ( 'NONE',  ( 16.46253265017146816, 9.564922557961045513, 96.66775706135233293 ) ) ;
#691=CARTESIAN_POINT ( 'NONE',  ( -21.52544592524343514, 5.823673210054127303, 76.04057627198102409 ) ) ;
#692=CARTESIAN_POINT ( 'NONE',  ( 14.34966873604960469, 8.224510206698951720, 44.16557627198103120 ) ) ;
#693=CARTESIAN_POINT ( 'NONE',  ( -16.51473224551082808, 9.474510206698731452, 113.3344237280190043 ) ) ;
#694=CARTESIAN_POINT ( 'NONE',  ( -5.049401038298153566, 19.05341960407611168, 30.20724293864768839 ) ) ;
#695=CARTESIAN_POINT ( 'NONE',  ( -4.379528057220086978, -16.55341960407618274, 19.79275706135235069 ) ) ;
#696=CARTESIAN_POINT ( 'NONE',  ( -5.823673210054116645, -21.52544592524344225, 97.29057627198105251 ) ) ;
#697=CARTESIAN_POINT ( 'NONE',  ( -5.049401038297874678, -19.05341960407617918, 64.79275706135233293 ) ) ;
#698=CARTESIAN_POINT ( 'NONE',  ( 16.53943276465976808, 0.05219959533934440121, 76.25109039468568994 ) ) ;
#699=CARTESIAN_POINT ( 'NONE',  ( 19.05341960407611168, 5.049401038298154454, 83.95724293864766707 ) ) ;
#700=CARTESIAN_POINT ( 'NONE',  ( 16.55341960407611168, 4.379528057220329451, 73.95724293864769550 ) ) ;
#701=CARTESIAN_POINT ( 'NONE',  ( -9.474510206698964154, 16.51473224551069663, 55.41557627198103120 ) ) ;
#702=CARTESIAN_POINT ( 'NONE',  ( -8.314922557960811034, -14.29746914071050412, 72.08224293864769550 ) ) ;
#703=CARTESIAN_POINT ( 'NONE',  ( -19.02544592524342804, 5.153800228976336051, 31.04057627198102409 ) ) ;
#705=CARTESIAN_POINT ( 'NONE',  ( -8.224510206698948167, 14.34966873604960824, 40.41557627198103120 ) ) ;
#706=CARTESIAN_POINT ( 'NONE',  ( 13.89961937509977652, -13.97604488694527269, 73.12390960531436690 ) ) ;
#708=CARTESIAN_POINT ( 'NONE',  ( 9.474510206698729675, 16.51473224551082808, 52.08442372801900433 ) ) ;
#709=CARTESIAN_POINT ( 'NONE',  ( 16.55341960407618274, -4.379528057220086978, 61.04275706135234714 ) ) ;
#710=CARTESIAN_POINT ( 'NONE',  ( 15.72974639402199770, -15.80617190586745480, 68.12390960531436690 ) ) ;
#711=CARTESIAN_POINT ( 'NONE',  ( 9.474510206698729675, 16.51473224551082808, 22.08442372801899722 ) ) ;
#712=CARTESIAN_POINT ( 'NONE',  ( -16.46253265017160317, 9.564922557960807481, 90.83224293864769550 ) ) ;
#714=CARTESIAN_POINT ( 'NONE',  ( 10.81492255796078972, 18.62759615963270932, 24.58224293864768839 ) ) ;
#715=CARTESIAN_POINT ( 'NONE',  ( 19.02544592524343514, -5.153800228976328945, 63.54057627198103830 ) ) ;
#716=CARTESIAN_POINT ( 'NONE',  ( 5.823673210054444382, -21.52544592524334988, 50.20942372801901854 ) ) ;
#717=CARTESIAN_POINT ( 'NONE',  ( 0.05219959533910956823, 16.53943276465976808, 109.9989096053143527 ) ) ;
#718=CARTESIAN_POINT ( 'NONE',  ( -10.81492255796078084, -18.62759615963271287, 97.08224293864770971 ) ) ;
#719=CARTESIAN_POINT ( 'NONE',  ( 19.03943276465977164, -0.05219959533909143690, 93.74890960531435269 ) ) ;
#721=CARTESIAN_POINT ( 'NONE',  ( 0.05219959533937995610, -21.53943276465977519, 45.00109039468568284 ) ) ;
#724=CARTESIAN_POINT ( 'NONE',  ( -19.05341960407611168, -5.049401038298163336, 91.45724293864766707 ) ) ;
#725=CARTESIAN_POINT ( 'NONE',  ( 19.36337904590692460, -5.499999999999940492, 82.91494137495615746 ) ) ;
#726=CARTESIAN_POINT ( 'NONE',  ( 15.72974639402199770, -15.80617190586745480, 88.12390960531436690 ) ) ;
#727=CARTESIAN_POINT ( 'NONE',  ( 16.51473224551069308, 9.474510206698969483, 49.16557627198102409 ) ) ;
#728=CARTESIAN_POINT ( 'NONE',  ( 4.379528057220092307, 16.55341960407617563, 27.29275706135234358 ) ) ;
#730=CARTESIAN_POINT ( 'NONE',  ( 19.03943276465977164, -0.05219959533909143690, 28.74890960531435624 ) ) ;
#731=CARTESIAN_POINT ( 'NONE',  ( 21.53943276465977519, 0.05219959533937863772, 86.25109039468568994 ) ) ;
#732=CARTESIAN_POINT ( 'NONE',  ( 13.89961937509977652, -13.97604488694527269, 78.12390960531433848 ) ) ;
#733=CARTESIAN_POINT ( 'NONE',  ( -18.62759615963255300, -10.81492255796106328, 49.16775706135234003 ) ) ;
#734=CARTESIAN_POINT ( 'NONE',  ( 15.72974639402176855, 15.80617190586768217, 26.87609039468567218 ) ) ;
#736=CARTESIAN_POINT ( 'NONE',  ( 16.51473224551069308, 9.474510206698969483, 99.16557627198102409 ) ) ;
#737=CARTESIAN_POINT ( 'NONE',  ( 19.53091890409951858, 5.500000000000028422, 62.56097431831421574 ) ) ;
#738=CARTESIAN_POINT ( 'NONE',  ( -8.314922557961024197, 14.29746914071037800, 42.91775706135235424 ) ) ;
#739=CARTESIAN_POINT ( 'NONE',  ( 16.52544592524335698, 4.483927247898782831, 66.45942372801903275 ) ) ;
#740=CARTESIAN_POINT ( 'NONE',  ( -10.72451020669870658, -18.67979575497194134, 44.58442372801901854 ) ) ;
#741=CARTESIAN_POINT ( 'NONE',  ( -18.67979575497193778, 10.72451020669871902, 73.33442372801901854 ) ) ;
#743=CARTESIAN_POINT ( 'NONE',  ( -9.474510206698720793, -16.51473224551083518, 109.5844237280190043 ) ) ;
#744=CARTESIAN_POINT ( 'NONE',  ( -13.97604488694527625, -13.89961937509977652, 61.87390960531435979 ) ) ;
#745=CARTESIAN_POINT ( 'NONE',  ( 13.89961937509977652, -13.97604488694527269, 98.12390960531433848 ) ) ;
#746=CARTESIAN_POINT ( 'NONE',  ( 8.224510206698953496, -14.34966873604960469, 112.9155762719810383 ) ) ;
#747=CARTESIAN_POINT ( 'NONE',  ( 4.483927247898545687, 16.52544592524342804, 99.79057627198103830 ) ) ;
#748=CARTESIAN_POINT ( 'NONE',  ( -5.823673210054116645, -21.52544592524344225, 32.29057627198102409 ) ) ;
#750=CARTESIAN_POINT ( 'NONE',  ( -8.314922557961024197, 14.29746914071037800, 82.91775706135234714 ) ) ;
#751=CARTESIAN_POINT ( 'NONE',  ( 16.55341960407611168, 4.379528057220329451, 73.95724293864769550 ) ) ;
#752=CARTESIAN_POINT ( 'NONE',  ( 5.153800228976335163, 19.02544592524342804, 49.79057627198100988 ) ) ;
#753=CARTESIAN_POINT ( 'NONE',  ( 15.80617190586769283, -15.72974639402175789, 80.62609039468567573 ) ) ;
#754=CARTESIAN_POINT ( 'NONE',  ( -21.52544592524334988, -5.823673210054445271, 68.95942372801901854 ) ) ;
#755=CARTESIAN_POINT ( 'NONE',  ( -19.03943276465977164, -0.05219959533935918106, 108.7510903946856615 ) ) ;
#756=CARTESIAN_POINT ( 'NONE',  ( -14.34966873604960291, -8.224510206698953496, 71.66557627198100988 ) ) ;
#757=CARTESIAN_POINT ( 'NONE',  ( -15.80617190586768217, 15.72974639402176855, 23.12609039468567573 ) ) ;
#758=CARTESIAN_POINT ( 'NONE',  ( 21.52544592524344225, -5.823673210054117533, 58.54057627198103120 ) ) ;
#759=CARTESIAN_POINT ( 'NONE',  ( -17.44270441346516520, -5.991230190323039828, 106.3633507926423363 ) ) ;
#761=CARTESIAN_POINT ( 'NONE',  ( 13.89961937509977652, -13.97604488694527269, 68.12390960531436690 ) ) ;
#762=CARTESIAN_POINT ( 'NONE',  ( 4.483927247898545687, 16.52544592524342804, 49.79057627198102409 ) ) ;
#763=CARTESIAN_POINT ( 'NONE',  ( 14.29746914071037800, 8.314922557961029526, 111.6677570613523613 ) ) ;
#764=CARTESIAN_POINT ( 'NONE',  ( 12.14591786802327356, -12.06949235617739191, 90.62609039468567573 ) ) ;
#765=CARTESIAN_POINT ( 'NONE',  ( -16.51473224551082808, 9.474510206698731452, 53.33442372801900433 ) ) ;
#767=CARTESIAN_POINT ( 'NONE',  ( -9.474510206698964154, 16.51473224551069663, 105.4155762719810383 ) ) ;
#768=CARTESIAN_POINT ( 'NONE',  ( 0.05219959533910956823, 16.53943276465976808, 74.99890960531435269 ) ) ;
#769=CARTESIAN_POINT ( 'NONE',  ( -9.564922557961040184, 16.46253265017147172, 42.91775706135234003 ) ) ;
#770=CARTESIAN_POINT ( 'NONE',  ( 5.153800228976335163, 19.02544592524342804, 34.79057627198102409 ) ) ;
#771=CARTESIAN_POINT ( 'NONE',  ( 10.72451020669898902, -18.67979575497178502, 37.91557627198102409 ) ) ;
#772=CARTESIAN_POINT ( 'NONE',  ( 10.81492255796078972, 18.62759615963270932, 54.58224293864769550 ) ) ;
#774=CARTESIAN_POINT ( 'NONE',  ( -16.52544592524342804, 4.483927247898546575, 101.0405762719810383 ) ) ;
#775=CARTESIAN_POINT ( 'NONE',  ( 8.314922557961029526, -14.29746914071037800, 50.41775706135235424 ) ) ;
#776=CARTESIAN_POINT ( 'NONE',  ( 14.34966873604960469, 8.224510206698951720, 89.16557627198102409 ) ) ;
#777=CARTESIAN_POINT ( 'NONE',  ( 30.00000000000000000, -5.510910596163089556E-15, 45.00000000000000000 ) ) ;
#779=CARTESIAN_POINT ( 'NONE',  ( -15.80617190586745835, -15.72974639402198527, 21.87390960531436690 ) ) ;
#783=CARTESIAN_POINT ( 'NONE',  ( 16.55341960407618274, -4.379528057220086978, 41.04275706135236135 ) ) ;
#784=CARTESIAN_POINT ( 'NONE',  ( 12.06949235617757843, -12.14591786802309237, 28.12390960531435979 ) ) ;
#785=CARTESIAN_POINT ( 'NONE',  ( 10.81492255796078972, 18.62759615963270932, 59.58224293864770260 ) ) ;
#786=CARTESIAN_POINT ( 'NONE',  ( 13.97604488694548053, -13.89961937509957401, 80.62609039468567573 ) ) ;
#787=CARTESIAN_POINT ( 'NONE',  ( 10.72451020669898902, -18.67979575497178502, 57.91557627198103120 ) ) ;
#788=CARTESIAN_POINT ( 'NONE',  ( 15.80617190586769283, -15.72974639402175789, 75.62609039468567573 ) ) ;
#790=CARTESIAN_POINT ( 'NONE',  ( -0.05219959533934338120, 16.53943276465976808, 52.50109039468567573 ) ) ;
#791=CARTESIAN_POINT ( 'NONE',  ( 9.564922557960805705, 16.46253265017160317, 34.58224293864770260 ) ) ;
#792=CARTESIAN_POINT ( 'NONE',  ( -19.05341960407611168, -5.049401038298163336, 101.4572429386476955 ) ) ;
#793=CARTESIAN_POINT ( 'NONE',  ( -16.51473224551069308, -9.474510206698971260, 41.66557627198103120 ) ) ;
#794=CARTESIAN_POINT ( 'NONE',  ( -16.55341960407611168, -4.379528057220339221, 106.4572429386477097 ) ) ;
#796=CARTESIAN_POINT ( 'NONE',  ( -16.46253265017160317, 9.564922557960807481, 95.83224293864769550 ) ) ;
#797=ORIENTED_EDGE ( 'NONE', *, *, #148993, .T. ) ;
#798=CARTESIAN_POINT ( 'NONE',  ( 14.29746914071037800, 8.314922557961029526, 71.66775706135234714 ) ) ;
#799=CARTESIAN_POINT ( 'NONE',  ( -10.81492255796078084, -18.62759615963271287, 92.08224293864769550 ) ) ;
#800=CARTESIAN_POINT ( 'NONE',  ( -13.89961937509977652, 13.97604488694528158, 60.62390960531436690 ) ) ;
#801=CARTESIAN_POINT ( 'NONE',  ( -5.823673210054431948, 21.52544592524334988, 22.70942372801901499 ) ) ;
#802=CARTESIAN_POINT ( 'NONE',  ( -5.049401038298153566, 19.05341960407611168, 85.20724293864766707 ) ) ;
#804=ORIENTED_EDGE ( 'NONE', *, *, #97826, .F. ) ;
#805=CARTESIAN_POINT ( 'NONE',  ( -21.55341960407610458, -5.719274019375992779, 111.4572429386476813 ) ) ;
#806=CARTESIAN_POINT ( 'NONE',  ( -16.51473224551069308, -9.474510206698971260, 26.66557627198103120 ) ) ;
#807=CARTESIAN_POINT ( 'NONE',  ( 5.153800228976335163, 19.02544592524342804, 109.7905762719810099 ) ) ;
#808=CARTESIAN_POINT ( 'NONE',  ( 19.05341960407617918, -5.049401038297876454, 71.04275706135234714 ) ) ;
#809=CARTESIAN_POINT ( 'NONE',  ( -0.05219959533936034679, 19.03943276465977164, 27.50109039468566507 ) ) ;
#810=CARTESIAN_POINT ( 'NONE',  ( 15.80617190586746368, 15.72974639402197994, 99.37390960531436690 ) ) ;
#811=CARTESIAN_POINT ( 'NONE',  ( 5.049401038297881783, 19.05341960407617563, 42.29275706135234003 ) ) ;
#812=CARTESIAN_POINT ( 'NONE',  ( -0.05219959533934338120, 16.53943276465976808, 77.50109039468567573 ) ) ;
#813=CARTESIAN_POINT ( 'NONE',  ( 9.474510206698971260, -16.51473224551069308, 102.9155762719810241 ) ) ;
#814=CARTESIAN_POINT ( 'NONE',  ( -0.05219959533909027116, -19.03943276465977164, 52.49890960531436690 ) ) ;
#815=CARTESIAN_POINT ( 'NONE',  ( 10.81492255796106328, -18.62759615963255655, 60.41775706135235424 ) ) ;
#816=CARTESIAN_POINT ( 'NONE',  ( 18.67979575497194134, -10.72451020669871369, 75.83442372801900433 ) ) ;
#817=CARTESIAN_POINT ( 'NONE',  ( 16.46253265017160672, -9.564922557960803928, 68.33224293864770971 ) ) ;
#818=CARTESIAN_POINT ( 'NONE',  ( 21.52544592524334988, 5.823673210054432836, 46.45942372801901854 ) ) ;
#819=CARTESIAN_POINT ( 'NONE',  ( 13.89961937509957401, 13.97604488694547697, 91.87609039468567573 ) ) ;
#820=CARTESIAN_POINT ( 'NONE',  ( -5.153800228976328057, -19.02544592524343514, 47.29057627198102409 ) ) ;
#821=CARTESIAN_POINT ( 'NONE',  ( 0.05219959533909260263, 19.03943276465977164, 99.99890960531436690 ) ) ;
#822=CARTESIAN_POINT ( 'NONE',  ( -19.05341960407611168, -5.049401038298163336, 71.45724293864766707 ) ) ;
#824=CARTESIAN_POINT ( 'NONE',  ( 16.46253265017160672, -9.564922557960803928, 53.33224293864768839 ) ) ;
#825=CARTESIAN_POINT ( 'NONE',  ( 15.72974639402199770, -15.80617190586745480, 98.12390960531436690 ) ) ;
#826=CARTESIAN_POINT ( 'NONE',  ( -12.06949235617739369, -12.14591786802326823, 69.37609039468567573 ) ) ;
#828=CARTESIAN_POINT ( 'NONE',  ( -16.51473224551082808, 9.474510206698731452, 38.33442372801899722 ) ) ;
#830=CARTESIAN_POINT ( 'NONE',  ( -5.049401038298153566, 19.05341960407611168, 70.20724293864769550 ) ) ;
#831=CARTESIAN_POINT ( 'NONE',  ( 12.06949235617757843, -12.14591786802309237, 53.12390960531436690 ) ) ;
#832=CARTESIAN_POINT ( 'NONE',  ( 12.14591786802309770, 12.06949235617756955, 89.37390960531435269 ) ) ;
#833=CARTESIAN_POINT ( 'NONE',  ( -19.05341960407611168, -5.049401038298163336, 111.4572429386476671 ) ) ;
#835=CARTESIAN_POINT ( 'NONE',  ( -19.05341960407611168, -5.049401038298163336, 86.45724293864769550 ) ) ;
#836=CARTESIAN_POINT ( 'NONE',  ( 5.153800228976335163, 19.02544592524342804, 104.7905762719809957 ) ) ;
#837=CARTESIAN_POINT ( 'NONE',  ( -15.80617190586768217, 15.72974639402176855, 108.1260903946856757 ) ) ;
#838=CARTESIAN_POINT ( 'NONE',  ( -0.05219959533934338120, 16.53943276465976808, 87.50109039468568994 ) ) ;
#839=CARTESIAN_POINT ( 'NONE',  ( -16.46253265017160317, 9.564922557960807481, 75.83224293864769550 ) ) ;
#840=CARTESIAN_POINT ( 'NONE',  ( -21.55341960407619339, 5.719274019375674811, 33.54275706135234714 ) ) ;
#841=CARTESIAN_POINT ( 'NONE',  ( -5.823673210054116645, -21.52544592524344225, 27.29057627198103120 ) ) ;
#842=CARTESIAN_POINT ( 'NONE',  ( -0.05219959533907301413, -21.53943276465977519, 97.49890960531436690 ) ) ;
#843=CARTESIAN_POINT ( 'NONE',  ( 12.14591786802309770, 12.06949235617756955, 64.37390960531435269 ) ) ;
#844=CARTESIAN_POINT ( 'NONE',  ( 16.51473224551069308, 9.474510206698969483, 54.16557627198103120 ) ) ;
#845=CARTESIAN_POINT ( 'NONE',  ( -16.53943276465976808, 0.05219959533911058130, 86.24890960531436690 ) ) ;
#846=CARTESIAN_POINT ( 'NONE',  ( 13.97604488694548053, -13.89961937509957401, 45.62609039468566863 ) ) ;
#847=CARTESIAN_POINT ( 'NONE',  ( 12.14591786802309770, 12.06949235617756955, 109.3739096053143811 ) ) ;
#848=CARTESIAN_POINT ( 'NONE',  ( 16.55341960407618274, -4.379528057220086978, 66.04275706135236135 ) ) ;
#849=CARTESIAN_POINT ( 'NONE',  ( 19.05341960407611168, 5.049401038298154454, 83.95724293864766707 ) ) ;
#851=CARTESIAN_POINT ( 'NONE',  ( -4.483927247898539470, -16.52544592524342804, 102.2905762719810383 ) ) ;
#853=CARTESIAN_POINT ( 'NONE',  ( -4.483927247898782831, 16.52544592524335698, 112.7094237280190328 ) ) ;
#854=CARTESIAN_POINT ( 'NONE',  ( -0.05219959533934338120, 16.53943276465976808, 27.50109039468567929 ) ) ;
#855=CARTESIAN_POINT ( 'NONE',  ( 15.72974639402176855, 15.80617190586768217, 91.87609039468568994 ) ) ;
#856=CARTESIAN_POINT ( 'NONE',  ( -13.89961937509977652, 13.97604488694528158, 85.62390960531433848 ) ) ;
#857=CARTESIAN_POINT ( 'NONE',  ( 18.67979575497194134, -10.72451020669871369, 25.83442372801901499 ) ) ;
#858=CARTESIAN_POINT ( 'NONE',  ( 0.05219959533909260263, 19.03943276465977164, 29.99890960531435979 ) ) ;
#859=CARTESIAN_POINT ( 'NONE',  ( -16.55341960407617563, 4.379528057220093196, 33.54275706135234714 ) ) ;
#860=CARTESIAN_POINT ( 'NONE',  ( -9.564922557961040184, 16.46253265017147172, 92.91775706135233293 ) ) ;
#861=CARTESIAN_POINT ( 'NONE',  ( 10.81492255796078972, 18.62759615963270932, 89.58224293864768129 ) ) ;
#862=CARTESIAN_POINT ( 'NONE',  ( 5.049401038297881783, 19.05341960407617563, 72.29275706135234714 ) ) ;
#863=CARTESIAN_POINT ( 'NONE',  ( -17.97058386085787163, -5.500000000000058620, 64.00390968646217971 ) ) ;
#864=CARTESIAN_POINT ( 'NONE',  ( 18.67979575497194134, -10.72451020669871369, 25.83442372801901499 ) ) ;
#866=CARTESIAN_POINT ( 'NONE',  ( -0.05219959533909027116, -19.03943276465977164, 87.49890960531436690 ) ) ;
#867=CARTESIAN_POINT ( 'NONE',  ( -0.05219959533934338120, 16.53943276465976808, 27.50109039468567929 ) ) ;
#869=CARTESIAN_POINT ( 'NONE',  ( -19.03943276465977164, -0.05219959533935918106, 53.75109039468566863 ) ) ;
#870=CARTESIAN_POINT ( 'NONE',  ( -21.52544592524343514, 5.823673210054127303, 116.0405762719810383 ) ) ;
#871=CARTESIAN_POINT ( 'NONE',  ( 14.29746914071049879, -8.314922557960816363, 73.33224293864769550 ) ) ;
#872=CARTESIAN_POINT ( 'NONE',  ( -19.05341960407611168, -5.049401038298163336, 81.45724293864769550 ) ) ;
#873=CARTESIAN_POINT ( 'NONE',  ( 8.224510206698742110, 14.34966873604972548, 52.08442372801901854 ) ) ;
#874=CARTESIAN_POINT ( 'NONE',  ( 13.97604488694548053, -13.89961937509957401, 55.62609039468566863 ) ) ;
#875=CARTESIAN_POINT ( 'NONE',  ( 10.72451020669871369, 18.67979575497193778, 72.08442372801899012 ) ) ;
#876=CARTESIAN_POINT ( 'NONE',  ( -4.483927247898782831, 16.52544592524335698, 22.70942372801901499 ) ) ;
#877=CARTESIAN_POINT ( 'NONE',  ( 19.03943276465977164, -0.05219959533909143690, 68.74890960531436690 ) ) ;
#878=CARTESIAN_POINT ( 'NONE',  ( -19.03943276465977164, -0.05219959533935918106, 83.75109039468567573 ) ) ;
#879=CARTESIAN_POINT ( 'NONE',  ( -14.34966873604972548, 8.224510206698743886, 58.33442372801901143 ) ) ;
#880=CARTESIAN_POINT ( 'NONE',  ( -18.62759615963255300, -10.81492255796106328, 99.16775706135234714 ) ) ;
#881=CARTESIAN_POINT ( 'NONE',  ( 16.51473224551083163, -9.474510206698727899, 65.83442372801900433 ) ) ;
#882=CARTESIAN_POINT ( 'NONE',  ( 9.474510206698971260, -16.51473224551069308, 52.91557627198102409 ) ) ;
#883=CARTESIAN_POINT ( 'NONE',  ( -21.53943276465977519, 0.05219959533907696930, 71.24890960531435269 ) ) ;
#884=CARTESIAN_POINT ( 'NONE',  ( -8.224510206698948167, 14.34966873604960824, 70.41557627198102409 ) ) ;
#885=CARTESIAN_POINT ( 'NONE',  ( -19.03943276465977164, -0.05219959533935918106, 83.75109039468567573 ) ) ;
#886=CARTESIAN_POINT ( 'NONE',  ( 16.88567814943160172, -6.947325034625743356, 61.20998877347415856 ) ) ;
#887=CARTESIAN_POINT ( 'NONE',  ( 19.03943276465977164, 0.05219959533936151252, 46.25109039468566863 ) ) ;
#888=CARTESIAN_POINT ( 'NONE',  ( -8.314922557961024197, 14.29746914071037800, 102.9177570613523756 ) ) ;
#889=CARTESIAN_POINT ( 'NONE',  ( -12.14591786802309592, -12.06949235617757132, 66.87390960531436690 ) ) ;
#890=CARTESIAN_POINT ( 'NONE',  ( 0.05219959533937995610, -21.53943276465977519, 100.0010903946857042 ) ) ;
#892=CARTESIAN_POINT ( 'NONE',  ( -18.67979575497178146, -10.72451020669898902, 106.6655762719810383 ) ) ;
#893=( BOUNDED_SURFACE ( )  B_SPLINE_SURFACE ( 3, 2, ( 
 ( #10534, #53015, #163206, #193554, #178386, #114694, #23699, #69191, #130857, #72198, #68187, #86359, #133872, #40861, #191538, #115706, #99522, #71201, #39850, #161204, #176389, #195562, #8524, #57036, #100522, #7507, #118709, #22699, #70202, #84346, #162201, #85347, #146024, #9534, #177394, #147040, #180399, #41871, #131869, #101516, #24710, #148044, #129839, #103537, #132864, #194553, #56023, #117701, #165212, #88347, #6507, #156744, #198526, #59997, #89353, #166209, #136842, #134884, #28698, #121664, #125407, #79892, #3051, #32402, #126389, #187104, #110227, #48574, #18238, #171908, #120672, #135867, #111220, #167200, #33396, #17233, #74198, #105515, #155735, #64727, #58031, #78885, #140564, #27710, #119701, #95055, #2053, #141562, #75170, #183359, #188086, #94057, #11545, #63732, #49557, #73213, #181384, #182372, #13505, #172913, #197538, #34391, #150040, #196560, #42862, #104528, #151043, #12533, #59006, #44841, #43849, #90334, #152019, #106497, #168174, #53531, #65709, #66705, #116209, #176902, #174892, #38373, #21203, #175893, #142553, #4031, #54536, #20201, #143535, #127375, #23210, #19227, #113203, #160713, #81847, #6023, #5022, #36358, #68696, #22204, #128368, #51540, #99022, #8022, #189086, #83854, #145535, #173910, #50559, #130351, #7014, #100028, #82859, #144537, #131371, #37364, #157738, #192050, #193060, #80876, #112220, #190064, #159705, #177899, #98010, #96050, #115209, #161715, #35379, #84853, #146530, #97030, #69704, #67702, #158711, #129360, #191056, #52528, #114189, #197060, #9042, #10044, #59508, #120194, #118218, #181884, #164724, #119216, #85867, #147556, #198041, #163726, #86869, #70712, #166717, #162712, #56541, #104039, #25228, #149546, #148553, #43362, #101027, #180901, #105033, #73717, #24217, #71704, #132380, #165719, #11041, #194073, #55535, #28221, #41376, #58528, #133372, #40369, #89862, #117208, #103042, #178901, #195062, #179910, #102042, #42376, #26218, #87858, #12054, #151544, #72716, #134389, #196075, #57547, #27215, #135390, #88861, #150555, #13034, #74700, #136364, #121183, #39368, #186871, #31176, #92826, #122175, #199030, #169680, #167703, #61497, #154512, #155506, #109995, #33164, #62488, #156501, #17001, #140328, #78653, #48340, #1818, #153512, #168677, #141325, #60499, #152518, #63498, #47345, #125173, #107994, #16008, #18003, #124159, #44358, #109001, #79656, #106017, #14006, #15009, #46338, #2814, #30177, #64492, #171675, #93826, #29200, #94824, #182877, #75673, #90834, #77666, #170681, #32169, #137350, #91820, #76670, #183866, #45352, #138348, #107004, #200028, #123166, #184854, #139335, #185859, #814, #172670, #84617, #50328, #173675, #34155, #53293, #49324, #143297, #190820, #111983, #36126, #35142, #6782, #187855, #5790, #68461, #160479, #110984, #96795, #157501, #52295, #97778, #18994, #95815, #114972, #128134, #145299, #19971, #127137, #176664, #80640, #189835, #142317, #81614, #4783, #3797, #129121, #65475, #158483, #98786, #38141, #188844, #66472, #51308, #112968, #174661, #21970, #159465, #144299, #20961, #113952, #83622, #82618, #67463, #130115, #175651, #37126, #191811, #99794, #161481, #22969, #146296, #7783, #126160, #196826, #119962, #149311, #43127, #42143, #26980, #165484, #135153, #103804, #40120, #55295, #27982, #86629, #88623, #134148, #193830, #24983, #72474, #181648, #177663, #195836, #57308, #89621, #54303, #179669, #117979, #131134, #23971, #150321, #41139, #87625, #10805, #11816, #192821, #151310, #118984, #69467, #115975, #25982, #180667, #163486, #147313, #73480, #58293, #166484, #104795, #39132, #8802, #100787, #162470, #116967, #85627, #70472, #132138, #102803, #178658, #101799, #148312, #9806, #164489, #194824, #71468, #133133, #56296, #59272, #169433, #199789, #61257, #120941, #29942, #75440, #137114, #171434, #170434, #78403, #92585, #28965, #140079, #184615, #123908, #91581, #153270, #32921, #108758, #74464, #44124 ),
 ( #182641, #183632, #94576, #93580, #14772, #155265, #138108, #154273, #105783, #167470, #12799, #198801, #60266, #90606, #1570, #136130, #76432, #77423, #121937, #122927, #45114, #16755, #197806, #15764, #63246, #47097, #152288, #106771, #13772, #139095, #46096, #168446, #107751, #124925, #30938, #31926, #569, #62240, #186622, #185607, #48094, #109750, #50079, #34896, #172423, #159220, #95569, #3554, #128878, #6535, #49085, #125917, #111740, #96552, #33911, #20715, #157255, #65232, #190578, #68215, #110742, #142068, #18749, #80396, #17756, #52054, #158239, #174417, #126892, #144060, #113710, #51062, #79413, #160234, #4534, #66226, #188598, #173427, #143055, #141083, #19730, #127887, #175407, #83377, #129867, #35886, #191565, #36875, #98540, #21724, #145054, #53044, #81371, #189590, #114724, #112724, #176417, #82371, #97533, #5541, #67220, #37892, #64250, #156254, #2568, #187615, #69220, #133900, #164247, #41899, #24737, #86387, #134909, #40889, #161232, #25742, #196586, #22726, #130888, #70230, #163237, #119727, #85377, #58056, #195591, #10561, #84374, #57063, #72225, #192578, #118738, #71228, #87388, #149073, #180426, #147070, #131898, #103565, #54061, #193582, #181410, #165240, #178414, #26734, #148071, #179424, #146051, #7535, #99550, #23728, #8554, #115735, #88373, #177422, #116725, #150067, #55054, #9562, #39878, #11572, #38893, #102562, #73238, #100550, #162229, #101545, #132891, #194580, #56050, #117729, #151067, #170188, #44868, #61995, #136868, #43875, #31682, #89378, #106524, #122683, #16512, #15520, #327, #138847, #108509, #77177, #13531, #28724, #1317, #60023, #123661, #107506, #167226, #198553, #45853, #155016, #12558, #169182, #30688, #120698, #74224, #185358, #92339, #46849, #168201, #29698, #78160, #184372, #104553, #154025, #139828, #166235, #135892, #75197, #91329, #62996, #90361, #124674, #93331, #42888, #27735, #197564, #59031, #182397, #105540, #14520, #152046, #121690, #183386, #153021, #76181, #137861, #199541, #61011, #6292, #66976, #64988, #128636, #111491, #65977, #32674, #94327, #144809, #110492, #33659, #156005, #113466, #109503, #3315, #50824, #172174, #96311, #95320, #190330, #47850, #127646, #51807, #20469, #171185, #157005, #17502, #112481, #157997, #79159, #140830, #175160, #188349, #5293, #80151, #187369, #36627, #2319, #49827, #64001, #141822, #126646, #125671, #189346, #48838, #18503, #158977, #98284, #173176, #34652, #19489, #81134, #142815, #82119, #4295, #174174, #35644, #97290, #143811, #159985, #21472, #83133, #67971, #186371, #68974, #145807, #116484, #114465, #8308, #39638, #102317, #56821, #180186, #37637, #132654, #117482, #7290, #99301, #164007, #194342, #71976, #54809, #178173, #164999, #70986, #191320, #55810, #26493, #52797, #160986, #100307, #193335, #149819, #115489, #88135, #25503, #40648, #176167, #87147, #148830, #22480, #10320, #101299, #179180, #133650, #195341, #177177, #161985, #118495, #84128, #23481, #11325, #41655, #69985, #103319, #162988, #9321, #130638, #192333, #129625, #53814, #38650, #85130, #146814, #131653, #24493, #86144, #147835, #183143, #197327, #153782, #134664, #152785, #15277, #107269, #57818, #182150, #104311, #137620, #44628, #165994, #181172, #88, #74962, #92094, #166985, #73987, #61758, #119490, #136624, #42649, #28488, #151806, #89137, #75946, #12322, #120459, #45617, #123426, #27495, #58791, #150825, #135656, #196350, #168940, #198305, #91097, #43635, #60771, #30447, #167965, #105297, #76937, #121451, #106280, #90122, #13297, #59783, #29464, #14276, #199304, #138606, #185119, #46609, #122443, #108271, #169949, #31440, #93094, #154778, #72995, #184135, #2087, #174930, #33430, #189121, #80909, #140597, #171941, #19263, #128403, #155769, #63767, #50593, #66742, #109265, #125440, #94090, #17267, #77927, #112252, #18271, #34424, #187136, #4065, #173944, #111254, #139594, #20234, #64760, #126422, #78920, #32436 ),
 ( #35411, #48608, #110260, #36393, #95089, #97063, #142586, #156778, #79924, #65743, #190100, #124436, #127411, #158745, #141597, #186132, #81882, #143574, #5057, #51575, #3084, #113239, #98047, #96083, #188120, #16275, #49591, #1080, #172946, #157772, #62755, #47611, #170944, #191093, #59306, #53572, #10838, #119018, #180701, #192089, #44157, #42177, #52568, #115249, #161753, #23248, #82896, #176941, #119995, #43162, #151344, #11851, #37405, #120975, #28016, #38411, #182673, #149342, #104829, #159745, #165518, #100068, #166518, #136165, #99063, #150354, #21242, #27014, #72508, #87657, #196861, #160751, #88658, #58327, #181681, #134183, #83892, #114228, #68734, #144574, #73516, #195870, #89658, #57343, #175933, #135187, #103837, #6061, #22243, #12833, #74499, #197840, #67739, #129397, #145575, #7052, #130392, #171467, #154307, #75473, #78439, #167504, #31959, #141116, #28999, #137146, #76466, #169468, #125950, #91616, #2605, #140113, #16789, #90639, #1604, #63280, #198834, #124960, #77456, #170469, #155299, #186657, #153304, #138143, #48127, #60298, #199823, #187648, #109784, #184648, #32955, #30969, #185640, #152321, #13807, #64283, #29977, #14805, #121972, #94610, #183664, #122961, #93614, #61291, #15796, #46130, #156289, #45149, #47132, #17790, #79446, #106805, #107783, #168479, #105817, #139127, #92616, #604, #62274, #123942, #108790, #143091, #50113, #37924, #95603, #112758, #18784, #4570, #127922, #65266, #52088, #188633, #96586, #21758, #99584, #142103, #34933, #126926, #111773, #110776, #83410, #51098, #67254, #158275, #36911, #145087, #144093, #172458, #53079, #97566, #159254, #173461, #19764, #35920, #33945, #189624, #20750, #6570, #176451, #161265, #128912, #22759, #68249, #129900, #191600, #114757, #84408, #81405, #66262, #7569, #174451, #146085, #113745, #82405, #5574, #175441, #69255, #157288, #98574, #160268, #190613, #130921, #49119, #80430, #3588, #24776, #150107, #73276, #181447, #41936, #70265, #151105, #58093, #9600, #12597, #179462, #134946, #74261, #195629, #71265, #196623, #166275, #131934, #180464, #192612, #57102, #102600, #86423, #26771, #193617, #118776, #88411, #11608, #56088, #116760, #23765, #101586, #54094, #103602, #132929, #119763, #148109, #85414, #165277, #194616, #115768, #147106, #42925, #25779, #87425, #104589, #117769, #40927, #27773, #89416, #149110, #177456, #38926, #164286, #10600, #100583, #8591, #162265, #72261, #133939, #55089, #178451, #39918, #163274, #77213, #135931, #197601, #92374, #62033, #29733, #13566, #138882, #362, #32710, #123697, #185395, #75233, #31718, #156041, #183419, #17538, #124711, #182433, #107542, #46886, #136904, #105575, #94362, #169218, #61046, #184408, #108546, #93366, #43913, #154060, #122718, #45889, #167261, #153057, #186409, #109539, #30727, #47886, #1354, #15555, #152081, #63033, #170225, #155053, #14559, #76217, #59067, #16548, #120734, #28760, #90397, #91366, #78195, #139865, #171221, #168237, #198591, #60059, #121727, #44903, #106560, #137896, #199578, #125707, #49861, #175197, #98321, #158032, #36662, #190367, #189381, #172210, #51843, #142850, #159012, #111527, #173212, #83169, #82153, #140867, #48874, #21508, #188384, #19523, #127681, #50858, #126680, #144843, #112516, #110529, #34688, #96345, #81168, #2356, #65024, #143849, #67012, #160021, #97326, #33694, #79198, #64037, #4329, #187406, #174210, #95357, #157042, #113502, #35678, #18539, #80186, #66013, #141858, #3349, #20505, #5328, #128671, #94023, #137553, #186064, #155704, #17199, #123362, #184066, #91032, #168874, #121388, #47547, #19, #140532, #92024, #152718, #32370, #15212, #183080, #14209, #110195, #93027, #154715, #78853, #138541, #46543, #170879, #2021, #16208, #18203, #44563, #169884, #108203, #106218, #75877, #63700, #31377, #77863, #1013, #125375, #167902, #141529, #62687, #59716, #29402, #139530, #109200, #153716, #199236, #124369, #187071 ),
 ( #48541, #171873, #45549, #76871, #33362, #95021, #60701, #156710, #79861, #107204, #61693, #122377, #30379, #185055, #23172, #83819, #81813, #145499, #128334, #82822, #49522, #111185, #161676, #127338, #50525, #172875, #130315, #126355, #20168, #67667, #189050, #113169, #112187, #6980, #64694, #144503, #68660, #37329, #188052, #173875, #34356, #129325, #174857, #96017, #157702, #192012, #4985, #22169, #96996, #3997, #53496, #19192, #66671, #80841, #158679, #143501, #142518, #5987, #65676, #35345, #175857, #115173, #190033, #51507, #36323, #97977, #159670, #98988, #21166, #191020, #52495, #114155, #160677, #176866, #38335, #99991, #84816, #3017, #85832, #162676, #133336, #131336, #25191, #56504, #119182, #73682, #197026, #26183, #120159, #180867, #104005, #42343, #12020, #165683, #117170, #132344, #104997, #163689, #27181, #11006, #70678, #102007, #149509, #58493, #54501, #72680, #134355, #24182, #116173, #88828, #196039, #150521, #135354, #195027, #177863, #181850, #7986, #57514, #43329, #69669, #39332, #178865, #10009, #166684, #194036, #28186, #146495, #193024, #100991, #147522, #9010, #55500, #40332, #118182, #86833, #148519, #71669, #179873, #41341, #103003, #164688, #87823, #34119, #50290, #52258, #96756, #51271, #17965, #79620, #130075, #95778, #18957, #141288, #98749, #94784, #188807, #36090, #157464, #81576, #80602, #113916, #33128, #112931, #175614, #5751, #156465, #142279, #2778, #97741, #143261, #64454, #126124, #160442, #173636, #190784, #65437, #172631, #21932, #187819, #35105, #49288, #127098, #111947, #110946, #174625, #3760, #158446, #144264, #83583, #19934, #4745, #66434, #128095, #189799, #67427, #159429, #20925, #82583, #129084, #37090, #145262, #6744, #68423, #191774, #53256, #171638, #131096, #101764, #99757, #193793, #24949, #87593, #42111, #165452, #194789, #88591, #149279, #72439, #10774, #180636, #134115, #85590, #100753, #73448, #132102, #195804, #179635, #39097, #70436, #117945, #26949, #22933, #41105, #102769, #192784, #84579, #57276, #164456, #118950, #103773, #163451, #146259, #150289, #176627, #25950, #11784, #38102, #7743, #147277, #178623, #135121, #162435, #196795, #114934, #161441, #69429, #54267, #115939, #177629, #23936, #86596, #8767, #55261, #116930, #40086, #148279, #9772, #71436, #56262, #133100, #104765, #16727, #182608, #105751, #166453, #185578, #181617, #75409, #122896, #44093, #168415, #167437, #139063, #119932, #138077, #541, #92555, #43096, #28934, #89591, #184585, #29910, #151278, #27950, #47069, #60235, #77393, #152256, #59240, #108729, #12767, #121906, #74431, #13741, #137081, #136098, #61225, #197774, #90575, #30907, #170406, #120909, #198769, #183599, #45083, #106740, #154243, #91550, #76401, #153237, #46066, #15734, #14740, #199758, #62212, #107720, #169401, #123880, #31898, #93551, #155237, #78375, #140051, #58263, #131616, #54775, #81345, #178137, #174390, #159192, #97506, #69951, #35860, #172394, #187588, #162953, #18720, #23447, #66197, #125888, #157228, #4507, #116449, #109724, #127860, #189564, #79386, #171408, #85094, #51036, #146779, #193300, #50050, #32894, #8273, #63217, #112698, #39604, #124897, #94546, #33883, #65204, #24459, #49057, #101263, #86109, #1541, #186596, #48068, #156227, #17728, #141055, #173398, #2541, #64223, #110712, #95540, #80367, #142040, #3528, #34869, #126863, #96523, #188570, #111712, #158213, #19703, #143029, #9285, #179146, #44595, #41622, #196317, #104279, #165961, #180153, #29433, #27462, #40614, #103286, #149787, #11290, #72963, #198274, #194307, #135623, #136594, #197294, #25470, #106251, #13268, #164966, #167933, #134632, #28457, #147800, #150794, #26459, #151775, #121421, #87110, #58757, #70950, #12290, #57786, #88102, #182117, #148796, #73955, #43603, #105268, #119457, #71944, #102284, #56789, #132620, #120426, #181141, #90093, #42615, #163973, #166954, #89103, #55773, #10286, #59751, #74931 ),
 ( #183113, #117447, #133614, #195308, #118461, #152751, #172914, #32403, #91064, #14241, #47579, #17234, #185087, #168907, #94058, #155736, #188087, #78886, #140565, #30413, #187105, #111221, #138574, #75912, #79893, #137586, #62720, #2055, #92060, #60737, #49558, #124403, #16243, #139563, #63733, #48575, #199269, #109231, #77895, #1047, #122410, #108237, #141563, #64728, #186097, #3052, #156745, #170910, #107236, #126390, #153749, #125408, #184100, #110228, #171909, #123395, #33397, #15244, #95056, #18240, #45583, #154747, #76903, #52, #61727, #46576, #169917, #31409, #93060, #66707, #65710, #7015, #190065, #157739, #189087, #84854, #67703, #129361, #68697, #113204, #21204, #145536, #130352, #191057, #193061, #19228, #144538, #82861, #96051, #50561, #192051, #6024, #52529, #175894, #176903, #80877, #116210, #37366, #34393, #142554, #114190, #160714, #128369, #112221, #99024, #22205, #131373, #83855, #53533, #173911, #115210, #54537, #81848, #4032, #23211, #127376, #38374, #100029, #35380, #97031, #158712, #161716, #20202, #146531, #143536, #8024, #69706, #5023, #51541, #174893, #36359, #98011, #159706, #26219, #147558, #150557, #39369, #104040, #13035, #101028, #9043, #148554, #41377, #198042, #163728, #74701, #12056, #88863, #162713, #73718, #135391, #70713, #197061, #149547, #42377, #27216, #58529, #25229, #10045, #120195, #181885, #11042, #165720, #40370, #56543, #43363, #103043, #57548, #24219, #85869, #136365, #102044, #86870, #132381, #105035, #194074, #166719, #179911, #196077, #71705, #28223, #89863, #72718, #55536, #151545, #87859, #134391, #117209, #178902, #164725, #133373, #118220, #119217, #59509, #177900, #195063, #180902, #94825, #93827, #78654, #17002, #186872, #155507, #91821, #107005, #79658, #138349, #140329, #185861, #32171, #44360, #168678, #77667, #29201, #124160, #109003, #199032, #90835, #1819, #47347, #63500, #48342, #169682, #152519, #125175, #182878, #170682, #156502, #106018, #14007, #153514, #184855, #141327, #30178, #18004, #109996, #171676, #167705, #33165, #2815, #75674, #121185, #92828, #137352, #60501, #122176, #15011, #76672, #183868, #45353, #154513, #200030, #61498, #123167, #46339, #107995, #815, #31177, #16010, #139336, #62489, #111985, #172671, #191813, #187856, #81615, #129123, #50329, #174662, #188845, #145300, #126161, #144301, #6783, #98787, #49325, #173676, #95817, #190821, #36127, #157502, #34156, #53294, #66473, #83623, #158484, #65476, #114973, #110985, #128136, #18995, #19972, #143298, #80641, #67464, #3798, #35143, #37127, #176666, #142318, #96797, #127138, #4784, #189836, #20962, #52296, #51309, #112970, #113953, #5791, #161482, #175653, #160481, #97779, #21971, #84618, #159467, #146297, #38142, #82619, #68462, #130116, #99795, #22970, #64494, #27983, #178659, #134149, #118985, #165485, #54304, #164490, #194825, #56298, #115976, #24985, #58295, #181649, #117980, #119963, #73482, #87626, #23973, #135154, #179670, #180668, #86630, #148313, #89623, #103805, #69468, #39133, #104797, #101800, #41141, #25983, #149312, #40122, #7785, #10806, #100788, #163487, #9808, #71469, #133134, #43128, #177664, #195837, #196827, #57310, #85628, #166485, #131135, #102804, #192823, #72476, #88625, #162471, #42145, #26981, #11817, #147314, #8804, #150322, #70473, #132139, #193832, #55296, #116968, #28966, #77424, #47098, #185609, #14773, #75441, #182642, #60267, #12800, #139096, #91582, #31927, #183633, #44125, #123910, #106773, #74466, #105785, #1572, #184616, #46097, #108759, #29943, #138110, #62241, #170436, #107752, #109751, #136131, #61258, #199790, #197807, #167471, #93581, #122928, #169435, #92586, #155266, #59273, #32922, #154275, #151311, #120943, #570, #90608, #171435, #16756, #168448, #152289, #30939, #78404, #13773, #15765, #153272, #140080, #124926, #137116, #63247, #198802, #186624, #48095, #45115, #121939, #76433, #20716, #190579, #128879, #158240 ),
 ( #188599, #173428, #110743, #97534, #33913, #142069, #67221, #145055, #187616, #80397, #172424, #95570, #156255, #52055, #96553, #112725, #3555, #82373, #113711, #189591, #17758, #98542, #143057, #4535, #157256, #18751, #81372, #79414, #34898, #66228, #175408, #21725, #6536, #174418, #68216, #36876, #160235, #83378, #129868, #191566, #65233, #126893, #53045, #111741, #114725, #159221, #5542, #141084, #50080, #51064, #2570, #144061, #176418, #19731, #64251, #94577, #125918, #49086, #127888, #35887, #7536, #10562, #99551, #164248, #73239, #161233, #69221, #8555, #101546, #58057, #23729, #134910, #72226, #149074, #22727, #133901, #195592, #130889, #57064, #9563, #102563, #87389, #118739, #85378, #70231, #180427, #41900, #71229, #25743, #100551, #116726, #103566, #39879, #56051, #147071, #165241, #26735, #132892, #84375, #88374, #86388, #148072, #177423, #54062, #24738, #146052, #178415, #194581, #150068, #11573, #196587, #117730, #119728, #37893, #192579, #115736, #38894, #162230, #131899, #193583, #55055, #163238, #179425, #40890, #92340, #104554, #167227, #137862, #89379, #184373, #169183, #59032, #151068, #15521, #45854, #123662, #46850, #29699, #12559, #154026, #42889, #107507, #16513, #166236, #74225, #152047, #44869, #1318, #28725, #78161, #77178, #138848, #27736, #328, #61996, #135893, #185359, #153022, #30689, #108510, #170189, #90362, #13532, #31683, #93332, #14521, #155017, #43876, #60024, #139829, #106525, #61012, #197565, #120699, #62997, #105541, #75198, #182398, #181411, #136869, #198554, #121691, #183387, #91330, #168202, #76182, #199542, #122684, #5294, #158978, #109504, #33660, #156006, #189347, #34653, #17503, #32675, #51808, #126647, #143812, #18504, #125672, #113467, #171186, #188350, #94328, #80152, #3316, #140831, #127647, #64002, #172175, #97291, #175161, #79160, #110493, #2320, #187370, #186372, #64989, #48839, #50825, #95321, #157006, #20470, #36628, #141823, #49828, #111492, #173177, #47851, #82120, #96312, #142816, #157998, #112482, #66977, #19490, #81135, #128637, #4296, #65978, #174175, #35645, #190331, #98285, #159986, #21473, #83134, #144810, #6293, #124675, #41656, #40649, #25504, #164008, #133651, #102318, #38651, #53815, #26494, #85131, #87148, #132655, #179181, #191321, #115490, #24494, #176168, #70987, #55811, #145808, #37638, #148831, #194343, #10321, #195342, #116485, #99302, #71977, #129626, #117483, #103320, #52798, #160987, #100308, #131654, #88136, #177178, #165000, #56822, #118496, #114466, #180187, #149820, #22481, #67972, #39639, #84129, #7291, #68975, #161986, #23482, #130639, #192334, #101300, #146815, #8309, #69986, #193336, #54810, #147836, #178174, #162989, #86145, #9322, #58792, #119491, #141358, #134665, #28489, #78683, #197328, #121452, #135657, #94854, #72996, #91098, #156535, #48371, #196351, #120460, #42650, #140359, #183144, #104312, #181173, #2845, #13298, #33195, #105298, #12323, #64523, #57819, #74963, #165995, #166986, #90123, #198306, #125204, #110028, #167966, #172702, #27496, #44629, #59784, #89138, #150826, #186900, #106281, #29465, #152786, #18034, #73988, #95847, #14277, #11326, #182151, #1847, #63529, #151807, #43636, #171706, #79688, #111015, #126190, #187886, #136625, #49353, #34186, #4815, #177693, #146326, #3827, #129153, #98816, #96829, #127167, #145331, #39161, #128165, #83653, #68491, #115003, #65506, #113984, #144331, #5820, #188876, #174693, #7815, #131164, #67496, #69499, #23003, #37157, #173706, #84649, #190850, #130146, #36157, #97809, #157531, #53324, #19025, #50358, #54333, #51339, #52327, #175682, #160510, #189865, #80671, #22000, #112017, #112999, #159498, #20994, #82649, #192854, #35174, #6813, #116004, #191843, #158513, #142347, #20001, #176697, #81644, #38171, #99826, #143328, #161511, #66502, #104830, #74500, #178692, #88659, #59307, #165519, #10839, #133165, #135188, #40154, #27015, #196862, #58328 ),
 ( #55326, #151345, #134184, #195871, #119996, #120976, #89659, #147346, #72509, #42178, #101830, #70502, #150355, #182674, #71498, #11852, #73517, #181682, #8834, #57344, #87658, #149343, #132170, #118011, #12834, #136166, #119019, #197841, #166519, #180702, #116997, #28017, #103838, #43163, #179700, #41172, #100819, #162502, #24003, #193861, #85659, #194856, #163517, #25016, #86659, #56329, #148343, #9839, #102835, #164521, #26014, #46131, #107784, #94611, #90640, #31960, #32956, #93615, #121973, #2606, #109785, #61292, #64284, #30970, #124961, #125951, #47133, #122962, #48128, #17791, #183665, #155300, #44158, #108791, #154308, #76467, #78440, #45150, #170470, #140114, #1605, #169469, #168480, #75474, #153305, #105818, #16790, #184649, #186658, #138144, #137147, #63281, #199824, #167505, #198835, #156290, #77457, #139128, #171468, #92617, #15797, #79447, #141117, #605, #29000, #152322, #62275, #123943, #13808, #60299, #106806, #185641, #29978, #91617, #14806, #49120, #69256, #128913, #187649, #110777, #144094, #113746, #81406, #65267, #190614, #52089, #84409, #175442, #36912, #126927, #83411, #7570, #34934, #19765, #21759, #188634, #98575, #145088, #6571, #51099, #111774, #18785, #96587, #172459, #160269, #127923, #68250, #143092, #80431, #129901, #4571, #33946, #142104, #37925, #20751, #82406, #191601, #66263, #174452, #53080, #114758, #5575, #146086, #95604, #97567, #35921, #157289, #3589, #176452, #159255, #67255, #99585, #161266, #50114, #173462, #22760, #158276, #189625, #112759, #57103, #24777, #8592, #133940, #72262, #27774, #118777, #180465, #70266, #26772, #151106, #178452, #12598, #119764, #177457, #102601, #195630, #131935, #100584, #41937, #130922, #101587, #103603, #165278, #88412, #38927, #87426, #117770, #179463, #162266, #148110, #181448, #104590, #40928, #42926, #196624, #10601, #147107, #58094, #164287, #150108, #9601, #71266, #192613, #11609, #54095, #73277, #115769, #134947, #166276, #23766, #89417, #25780, #85415, #193618, #55090, #116761, #163275, #39919, #86424, #149111, #132930, #194617, #56089, #155054, #199579, #154061, #120735, #182434, #32711, #198592, #121728, #43914, #1355, #197602, #91367, #138883, #60060, #184409, #183420, #16549, #139866, #122719, #105576, #46887, #135932, #363, #109540, #59068, #167262, #44904, #137897, #94363, #63034, #28761, #90398, #62034, #152082, #170226, #108547, #13567, #31719, #45890, #123698, #185396, #78196, #106561, #168238, #93367, #124712, #107543, #186410, #136905, #153058, #47887, #61047, #15556, #75234, #29734, #156042, #14560, #76218, #169219, #171222, #30728, #92375, #74262, #77214, #127682, #141859, #98322, #79199, #97327, #160022, #51844, #2357, #126681, #48875, #82154, #189382, #110530, #125708, #144844, #19524, #36663, #111528, #18540, #6327, #64038, #81169, #187407, #173213, #96346, #33695, #20506, #157043, #65025, #190369, #68007, #172211, #3350, #95358, #80187, #140868, #113503, #142851, #35679, #188385, #5329, #175198, #112517, #49862, #21509, #66014, #50859, #34689, #158033, #4330, #174211, #159013, #143850, #83170, #129659, #191355, #67013, #52833, #114502, #176204, #37673, #99338, #17539, #128672, #162021, #103355, #131688, #102351, #194376, #40681, #84162, #23517, #147869, #7324, #55843, #117517, #115525, #69008, #164040, #179215, #10355, #192368, #85163, #177213, #38686, #22515, #25539, #116519, #9355, #146851, #87183, #148864, #86179, #145842, #72012, #101333, #163022, #100342, #53851, #24528, #130674, #193369, #71020, #133685, #195378, #56856, #132688, #118531, #180220, #41690, #165033, #26526, #161021, #8344, #70019, #54845, #178207, #39671, #5988, #52496, #64695, #127339, #97978, #49523, #144504, #129326, #19193, #111186, #175858, #67668, #83820, #6981, #190034, #172876, #114156, #3018, #191021, #176867, #126356, #34357, #112188, #4986, #161677, #68661, #188053, #157703, #37330, #96018, #98989, #160678 ) ),
 .UNSPECIFIED., .T., .F., .F. ) 
 B_SPLINE_SURFACE_WITH_KNOTS ( ( 4, 3, 4 ),
 ( 3, 2, 2, 2, 2, 2, 2, 2, 2, 2, 2, 2, 2, 2, 2, 2, 2, 2, 2, 2, 2, 2, 2, 2, 2, 2, 2, 2, 2, 2, 2, 2, 2, 2, 2, 2, 2, 2, 2, 2, 2, 2, 2, 2, 2, 2, 2, 2, 2, 2, 2, 2, 2, 2, 2, 2, 2, 2, 2, 2, 2, 2, 2, 2, 2, 2, 2, 2, 2, 2, 2, 2, 2, 2, 2, 2, 2, 2, 2, 2, 2, 2, 2, 2, 2, 2, 2, 2, 2, 2, 2, 2, 2, 2, 2, 2, 2, 2, 2, 2, 2, 2, 2, 2, 2, 2, 2, 2, 2, 2, 2, 2, 2, 2, 2, 2, 2, 2, 2, 2, 2, 2, 2, 2, 2, 2, 2, 2, 2, 2, 2, 2, 2, 2, 2, 2, 2, 2, 2, 2, 2, 2, 2, 2, 2, 2, 2, 2, 2, 2, 2, 2, 2, 2, 2, 2, 2, 2, 2, 2, 2, 2, 2, 2, 2, 2, 2, 2, 2, 2, 2, 2, 2, 2, 2, 2, 2, 2, 2, 2, 2, 2, 2, 2, 2, 2, 2, 2, 2, 2, 2, 2, 2, 2, 2, 2, 2, 2, 2, 2, 2, 2, 2, 2, 2, 2, 2, 2, 2, 2, 2, 2, 2, 2, 2, 2, 2, 2, 2, 2, 2, 2, 2, 2, 2, 2, 2, 2, 3 ),
 ( 0.000000000000000000, 0.5000000000000000000, 1.000000000000000000 ),
 ( 0.000000000000000000, 0.004385964912280701511, 0.008771929824561403022, 0.01315789473684210453, 0.01754385964912280604, 0.02192982456140350755, 0.02631578947368420907, 0.03070175438596491058, 0.03508771929824561209, 0.03947368421052631360, 0.04385964912280701511, 0.04824561403508771662, 0.05263157894736841813, 0.05701754385964911964, 0.06140350877192982115, 0.06578947368421052266, 0.07017543859649122417, 0.07456140350877192569, 0.07894736842105262720, 0.08333333333333332871, 0.08771929824561403022, 0.09210526315789473173, 0.09649122807017543324, 0.1008771929824561348, 0.1052631578947368363, 0.1096491228070175378, 0.1140350877192982393, 0.1184210526315789408, 0.1228070175438596423, 0.1271929824561403577, 0.1315789473684210453, 0.1359649122807017607, 0.1403508771929824483, 0.1447368421052631637, 0.1491228070175438514, 0.1535087719298245668, 0.1578947368421052544, 0.1622807017543859698, 0.1666666666666666574, 0.1710526315789473728, 0.1754385964912280604, 0.1798245614035087758, 0.1842105263157894635, 0.1885964912280701788, 0.1929824561403508665, 0.1973684210526315819, 0.2017543859649122695, 0.2061403508771929849, 0.2105263157894736725, 0.2149122807017543879, 0.2192982456140350755, 0.2236842105263157909, 0.2280701754385964786, 0.2324561403508771940, 0.2368421052631578816, 0.2412280701754385970, 0.2456140350877192846, 0.2500000000000000000, 0.2543859649122807154, 0.2587719298245614308, 0.2631578947368420907, 0.2675438596491228060, 0.2719298245614035214, 0.2763157894736842368, 0.2807017543859648967, 0.2850877192982456121, 0.2894736842105263275, 0.2938596491228070429, 0.2982456140350877027, 0.3026315789473684181, 0.3070175438596491335, 0.3114035087719298489, 0.3157894736842105088, 0.3201754385964912242, 0.3245614035087719396, 0.3289473684210526550, 0.3333333333333333148, 0.3377192982456140302, 0.3421052631578947456, 0.3464912280701754610, 0.3508771929824561209, 0.3552631578947368363, 0.3596491228070175517, 0.3640350877192982670, 0.3684210526315789269, 0.3728070175438596423, 0.3771929824561403577, 0.3815789473684210731, 0.3859649122807017330, 0.3903508771929824483, 0.3947368421052631637, 0.3991228070175438791, 0.4035087719298245390, 0.4078947368421052544, 0.4122807017543859698, 0.4166666666666666852, 0.4210526315789473450, 0.4254385964912280604, 0.4298245614035087758, 0.4342105263157894912, 0.4385964912280701511, 0.4429824561403508665, 0.4473684210526315819, 0.4517543859649122973, 0.4561403508771929571, 0.4605263157894736725, 0.4649122807017543879, 0.4692982456140351033, 0.4736842105263157632, 0.4780701754385964786, 0.4824561403508771940, 0.4868421052631579093, 0.4912280701754385692, 0.4956140350877192846, 0.5000000000000000000, 0.5043859649122807154, 0.5087719298245614308, 0.5131578947368421462, 0.5175438596491228616, 0.5219298245614034659, 0.5263157894736841813, 0.5307017543859648967, 0.5350877192982456121, 0.5394736842105263275, 0.5438596491228070429, 0.5482456140350877583, 0.5526315789473684736, 0.5570175438596490780, 0.5614035087719297934, 0.5657894736842105088, 0.5701754385964912242, 0.5745614035087719396, 0.5789473684210526550, 0.5833333333333333703, 0.5877192982456140857, 0.5921052631578946901, 0.5964912280701754055, 0.6008771929824561209, 0.6052631578947368363, 0.6096491228070175517, 0.6140350877192982670, 0.6184210526315789824, 0.6228070175438596978, 0.6271929824561403022, 0.6315789473684210176, 0.6359649122807017330, 0.6403508771929824483, 0.6447368421052631637, 0.6491228070175438791, 0.6535087719298245945, 0.6578947368421053099, 0.6622807017543859143, 0.6666666666666666297, 0.6710526315789473450, 0.6754385964912280604, 0.6798245614035087758, 0.6842105263157894912, 0.6885964912280702066, 0.6929824561403509220, 0.6973684210526315264, 0.7017543859649122417, 0.7061403508771929571, 0.7105263157894736725, 0.7149122807017543879, 0.7192982456140351033, 0.7236842105263158187, 0.7280701754385965341, 0.7324561403508771384, 0.7368421052631578538, 0.7412280701754385692, 0.7456140350877192846, 0.7500000000000000000, 0.7543859649122807154, 0.7587719298245614308, 0.7631578947368421462, 0.7675438596491228616, 0.7719298245614034659, 0.7763157894736841813, 0.7807017543859648967, 0.7850877192982456121, 0.7894736842105263275, 0.7938596491228070429, 0.7982456140350877583, 0.8026315789473684736, 0.8070175438596490780, 0.8114035087719297934, 0.8157894736842105088, 0.8201754385964912242, 0.8245614035087719396, 0.8289473684210526550, 0.8333333333333333703, 0.8377192982456140857, 0.8421052631578946901, 0.8464912280701754055, 0.8508771929824561209, 0.8552631578947368363, 0.8596491228070175517, 0.8640350877192982670, 0.8684210526315789824, 0.8728070175438596978, 0.8771929824561403022, 0.8815789473684210176, 0.8859649122807017330, 0.8903508771929824483, 0.8947368421052631637, 0.8991228070175438791, 0.9035087719298245945, 0.9078947368421053099, 0.9122807017543859143, 0.9166666666666666297, 0.9210526315789473450, 0.9254385964912280604, 0.9298245614035087758, 0.9342105263157894912, 0.9385964912280702066, 0.9429824561403509220, 0.9473684210526315264, 0.9517543859649122417, 0.9561403508771929571, 0.9605263157894736725, 0.9649122807017543879, 0.9692982456140351033, 0.9736842105263158187, 0.9780701754385965341, 0.9824561403508771384, 0.9868421052631578538, 0.9912280701754385692, 0.9956140350877192846, 1.000000000000000000 ),
 .UNSPECIFIED. ) 
 GEOMETRIC_REPRESENTATION_ITEM ( )  RATIONAL_B_SPLINE_SURFACE ( (
 ( 1.000000000000000000, 0.9659258262890683122, 1.000000000000000000, 0.9659258262890683122, 1.000000000000000000, 0.9659258262890683122, 1.000000000000000000, 0.9659258262890683122, 1.000000000000000000, 0.9659258262890683122, 1.000000000000000000, 0.9659258262890683122, 1.000000000000000000, 0.9659258262890683122, 1.000000000000000000, 0.9659258262890683122, 1.000000000000000000, 0.9659258262890683122, 1.000000000000000000, 0.9659258262890683122, 1.000000000000000000, 0.9659258262890683122, 1.000000000000000000, 0.9659258262890683122, 1.000000000000000000, 0.9659258262890683122, 1.000000000000000000, 0.9659258262890683122, 1.000000000000000000, 0.9659258262890683122, 1.000000000000000000, 0.9659258262890683122, 1.000000000000000000, 0.9659258262890683122, 1.000000000000000000, 0.9659258262890683122, 1.000000000000000000, 0.9659258262890683122, 1.000000000000000000, 0.9659258262890683122, 1.000000000000000000, 0.9659258262890683122, 1.000000000000000000, 0.9659258262890683122, 1.000000000000000000, 0.9659258262890683122, 1.000000000000000000, 0.9659258262890683122, 1.000000000000000000, 0.9659258262890683122, 1.000000000000000000, 0.9659258262890683122, 1.000000000000000000, 0.9659258262890683122, 1.000000000000000000, 0.9659258262890683122, 1.000000000000000000, 0.9659258262890683122, 1.000000000000000000, 0.9659258262890683122, 1.000000000000000000, 0.9659258262890683122, 1.000000000000000000, 0.9659258262890683122, 1.000000000000000000, 0.9659258262890683122, 1.000000000000000000, 0.9659258262890683122, 1.000000000000000000, 0.9659258262890683122, 1.000000000000000000, 0.9659258262890683122, 1.000000000000000000, 0.9659258262890683122, 1.000000000000000000, 0.9659258262890683122, 1.000000000000000000, 0.9659258262890683122, 1.000000000000000000, 0.9659258262890683122, 1.000000000000000000, 0.9659258262890683122, 1.000000000000000000, 0.9659258262890683122, 1.000000000000000000, 0.9659258262890683122, 1.000000000000000000, 0.9659258262890683122, 1.000000000000000000, 0.9659258262890683122, 1.000000000000000000, 0.9659258262890683122, 1.000000000000000000, 0.9659258262890683122, 1.000000000000000000, 0.9659258262890683122, 1.000000000000000000, 0.9659258262890683122, 1.000000000000000000, 0.9659258262890683122, 1.000000000000000000, 0.9659258262890683122, 1.000000000000000000, 0.9659258262890683122, 1.000000000000000000, 0.9659258262890683122, 1.000000000000000000, 0.9659258262890683122, 1.000000000000000000, 0.9659258262890683122, 1.000000000000000000, 0.9659258262890683122, 1.000000000000000000, 0.9659258262890683122, 1.000000000000000000, 0.9659258262890683122, 1.000000000000000000, 0.9659258262890683122, 1.000000000000000000, 0.9659258262890683122, 1.000000000000000000, 0.9659258262890683122, 1.000000000000000000, 0.9659258262890683122, 1.000000000000000000, 0.9659258262890683122, 1.000000000000000000, 0.9659258262890683122, 1.000000000000000000, 0.9659258262890683122, 1.000000000000000000, 0.9659258262890683122, 1.000000000000000000, 0.9659258262890683122, 1.000000000000000000, 0.9659258262890683122, 1.000000000000000000, 0.9659258262890683122, 1.000000000000000000, 0.9659258262890683122, 1.000000000000000000, 0.9659258262890683122, 1.000000000000000000, 0.9659258262890683122, 1.000000000000000000, 0.9659258262890683122, 1.000000000000000000, 0.9659258262890683122, 1.000000000000000000, 0.9659258262890683122, 1.000000000000000000, 0.9659258262890683122, 1.000000000000000000, 0.9659258262890683122, 1.000000000000000000, 0.9659258262890683122, 1.000000000000000000, 0.9659258262890683122, 1.000000000000000000, 0.9659258262890683122, 1.000000000000000000, 0.9659258262890683122, 1.000000000000000000, 0.9659258262890683122, 1.000000000000000000, 0.9659258262890683122, 1.000000000000000000, 0.9659258262890683122, 1.000000000000000000, 0.9659258262890683122, 1.000000000000000000, 0.9659258262890683122, 1.000000000000000000, 0.9659258262890683122, 1.000000000000000000, 0.9659258262890683122, 1.000000000000000000, 0.9659258262890683122, 1.000000000000000000, 0.9659258262890683122, 1.000000000000000000, 0.9659258262890683122, 1.000000000000000000, 0.9659258262890683122, 1.000000000000000000, 0.9659258262890683122, 1.000000000000000000, 0.9659258262890683122, 1.000000000000000000, 0.9659258262890683122, 1.000000000000000000, 0.9659258262890683122, 1.000000000000000000, 0.9659258262890683122, 1.000000000000000000, 0.9659258262890683122, 1.000000000000000000, 0.9659258262890683122, 1.000000000000000000, 0.9659258262890683122, 1.000000000000000000, 0.9659258262890683122, 1.000000000000000000, 0.9659258262890683122, 1.000000000000000000, 0.9659258262890683122, 1.000000000000000000, 0.9659258262890683122, 1.000000000000000000, 0.9659258262890683122, 1.000000000000000000, 0.9659258262890683122, 1.000000000000000000, 0.9659258262890683122, 1.000000000000000000, 0.9659258262890683122, 1.000000000000000000, 0.9659258262890683122, 1.000000000000000000, 0.9659258262890683122, 1.000000000000000000, 0.9659258262890683122, 1.000000000000000000, 0.9659258262890683122, 1.000000000000000000, 0.9659258262890683122, 1.000000000000000000, 0.9659258262890683122, 1.000000000000000000, 0.9659258262890683122, 1.000000000000000000, 0.9659258262890683122, 1.000000000000000000, 0.9659258262890683122, 1.000000000000000000, 0.9659258262890683122, 1.000000000000000000, 0.9659258262890683122, 1.000000000000000000, 0.9659258262890683122, 1.000000000000000000, 0.9659258262890683122, 1.000000000000000000, 0.9659258262890683122, 1.000000000000000000, 0.9659258262890683122, 1.000000000000000000, 0.9659258262890683122, 1.000000000000000000, 0.9659258262890683122, 1.000000000000000000, 0.9659258262890683122, 1.000000000000000000, 0.9659258262890683122, 1.000000000000000000, 0.9659258262890683122, 1.000000000000000000, 0.9659258262890683122, 1.000000000000000000, 0.9659258262890683122, 1.000000000000000000, 0.9659258262890683122, 1.000000000000000000, 0.9659258262890683122, 1.000000000000000000, 0.9659258262890683122, 1.000000000000000000, 0.9659258262890683122, 1.000000000000000000, 0.9659258262890683122, 1.000000000000000000, 0.9659258262890683122, 1.000000000000000000, 0.9659258262890683122, 1.000000000000000000, 0.9659258262890683122, 1.000000000000000000, 0.9659258262890683122, 1.000000000000000000, 0.9659258262890683122, 1.000000000000000000, 0.9659258262890683122, 1.000000000000000000, 0.9659258262890683122, 1.000000000000000000, 0.9659258262890683122, 1.000000000000000000, 0.9659258262890683122, 1.000000000000000000, 0.9659258262890683122, 1.000000000000000000, 0.9659258262890683122, 1.000000000000000000, 0.9659258262890683122, 1.000000000000000000, 0.9659258262890683122, 1.000000000000000000, 0.9659258262890683122, 1.000000000000000000, 0.9659258262890683122, 1.000000000000000000, 0.9659258262890683122, 1.000000000000000000, 0.9659258262890683122, 1.000000000000000000, 0.9659258262890683122, 1.000000000000000000, 0.9659258262890683122, 1.000000000000000000, 0.9659258262890683122, 1.000000000000000000, 0.9659258262890683122, 1.000000000000000000, 0.9659258262890683122, 1.000000000000000000, 0.9659258262890683122, 1.000000000000000000, 0.9659258262890683122, 1.000000000000000000, 0.9659258262890683122, 1.000000000000000000, 0.9659258262890683122, 1.000000000000000000, 0.9659258262890683122, 1.000000000000000000, 0.9659258262890683122, 1.000000000000000000, 0.9659258262890683122, 1.000000000000000000, 0.9659258262890683122, 1.000000000000000000, 0.9659258262890683122, 1.000000000000000000, 0.9659258262890683122, 1.000000000000000000, 0.9659258262890683122, 1.000000000000000000, 0.9659258262890683122, 1.000000000000000000, 0.9659258262890683122, 1.000000000000000000, 0.9659258262890683122, 1.000000000000000000, 0.9659258262890683122, 1.000000000000000000, 0.9659258262890683122, 1.000000000000000000, 0.9659258262890683122, 1.000000000000000000, 0.9659258262890683122, 1.000000000000000000, 0.9659258262890683122, 1.000000000000000000, 0.9659258262890683122, 1.000000000000000000, 0.9659258262890683122, 1.000000000000000000, 0.9659258262890683122, 1.000000000000000000, 0.9659258262890683122, 1.000000000000000000, 0.9659258262890683122, 1.000000000000000000, 0.9659258262890683122, 1.000000000000000000, 0.9659258262890683122, 1.000000000000000000, 0.9659258262890683122, 1.000000000000000000, 0.9659258262890683122, 1.000000000000000000, 0.9659258262890683122, 1.000000000000000000, 0.9659258262890683122, 1.000000000000000000, 0.9659258262890683122, 1.000000000000000000, 0.9659258262890683122, 1.000000000000000000, 0.9659258262890683122, 1.000000000000000000, 0.9659258262890683122, 1.000000000000000000, 0.9659258262890683122, 1.000000000000000000, 0.9659258262890683122, 1.000000000000000000, 0.9659258262890683122, 1.000000000000000000, 0.9659258262890683122, 1.000000000000000000, 0.9659258262890683122, 1.000000000000000000, 0.9659258262890683122, 1.000000000000000000, 0.9659258262890683122, 1.000000000000000000, 0.9659258262890683122, 1.000000000000000000, 0.9659258262890683122, 1.000000000000000000, 0.9659258262890683122, 1.000000000000000000, 0.9659258262890683122, 1.000000000000000000, 0.9659258262890683122, 1.000000000000000000, 0.9659258262890683122, 1.000000000000000000, 0.9659258262890683122, 1.000000000000000000, 0.9659258262890683122, 1.000000000000000000, 0.9659258262890683122, 1.000000000000000000, 0.9659258262890683122, 1.000000000000000000, 0.9659258262890683122, 1.000000000000000000, 0.9659258262890683122, 1.000000000000000000, 0.9659258262890683122, 1.000000000000000000, 0.9659258262890683122, 1.000000000000000000, 0.9659258262890683122, 1.000000000000000000, 0.9659258262890683122, 1.000000000000000000, 0.9659258262890683122, 1.000000000000000000, 0.9659258262890683122, 1.000000000000000000, 0.9659258262890683122, 1.000000000000000000, 0.9659258262890683122, 1.000000000000000000, 0.9659258262890683122, 1.000000000000000000, 0.9659258262890683122, 1.000000000000000000, 0.9659258262890683122, 1.000000000000000000, 0.9659258262890683122, 1.000000000000000000, 0.9659258262890683122, 1.000000000000000000, 0.9659258262890683122, 1.000000000000000000, 0.9659258262890683122, 1.000000000000000000, 0.9659258262890683122, 1.000000000000000000, 0.9659258262890683122, 1.000000000000000000, 0.9659258262890683122, 1.000000000000000000),
 ( 0.3333333333333333703, 0.3219752754296894559, 0.3333333333333333703, 0.3219752754296894559, 0.3333333333333333703, 0.3219752754296894559, 0.3333333333333333703, 0.3219752754296894559, 0.3333333333333333703, 0.3219752754296894559, 0.3333333333333333703, 0.3219752754296894559, 0.3333333333333333703, 0.3219752754296894559, 0.3333333333333333703, 0.3219752754296894559, 0.3333333333333333703, 0.3219752754296894559, 0.3333333333333333703, 0.3219752754296894559, 0.3333333333333333703, 0.3219752754296894559, 0.3333333333333333703, 0.3219752754296894559, 0.3333333333333333703, 0.3219752754296894559, 0.3333333333333333703, 0.3219752754296894559, 0.3333333333333333703, 0.3219752754296894559, 0.3333333333333333703, 0.3219752754296894559, 0.3333333333333333703, 0.3219752754296894559, 0.3333333333333333703, 0.3219752754296894559, 0.3333333333333333703, 0.3219752754296894559, 0.3333333333333333703, 0.3219752754296894559, 0.3333333333333333703, 0.3219752754296894559, 0.3333333333333333703, 0.3219752754296894559, 0.3333333333333333703, 0.3219752754296894559, 0.3333333333333333703, 0.3219752754296894559, 0.3333333333333333703, 0.3219752754296894559, 0.3333333333333333703, 0.3219752754296894559, 0.3333333333333333703, 0.3219752754296894559, 0.3333333333333333703, 0.3219752754296894559, 0.3333333333333333703, 0.3219752754296894559, 0.3333333333333333703, 0.3219752754296894559, 0.3333333333333333703, 0.3219752754296894559, 0.3333333333333333703, 0.3219752754296894559, 0.3333333333333333703, 0.3219752754296894559, 0.3333333333333333703, 0.3219752754296894559, 0.3333333333333333703, 0.3219752754296894559, 0.3333333333333333703, 0.3219752754296894559, 0.3333333333333333703, 0.3219752754296894559, 0.3333333333333333703, 0.3219752754296894559, 0.3333333333333333703, 0.3219752754296894559, 0.3333333333333333703, 0.3219752754296894559, 0.3333333333333333703, 0.3219752754296894559, 0.3333333333333333703, 0.3219752754296894559, 0.3333333333333333703, 0.3219752754296894559, 0.3333333333333333703, 0.3219752754296894559, 0.3333333333333333703, 0.3219752754296894559, 0.3333333333333333703, 0.3219752754296894559, 0.3333333333333333703, 0.3219752754296894559, 0.3333333333333333703, 0.3219752754296894559, 0.3333333333333333703, 0.3219752754296894559, 0.3333333333333333703, 0.3219752754296894559, 0.3333333333333333703, 0.3219752754296894559, 0.3333333333333333703, 0.3219752754296894559, 0.3333333333333333703, 0.3219752754296894559, 0.3333333333333333703, 0.3219752754296894559, 0.3333333333333333703, 0.3219752754296894559, 0.3333333333333333703, 0.3219752754296894559, 0.3333333333333333703, 0.3219752754296894559, 0.3333333333333333703, 0.3219752754296894559, 0.3333333333333333703, 0.3219752754296894559, 0.3333333333333333703, 0.3219752754296894559, 0.3333333333333333703, 0.3219752754296894559, 0.3333333333333333703, 0.3219752754296894559, 0.3333333333333333703, 0.3219752754296894559, 0.3333333333333333703, 0.3219752754296894559, 0.3333333333333333703, 0.3219752754296894559, 0.3333333333333333703, 0.3219752754296894559, 0.3333333333333333703, 0.3219752754296894559, 0.3333333333333333703, 0.3219752754296894559, 0.3333333333333333703, 0.3219752754296894559, 0.3333333333333333703, 0.3219752754296894559, 0.3333333333333333703, 0.3219752754296894559, 0.3333333333333333703, 0.3219752754296894559, 0.3333333333333333703, 0.3219752754296894559, 0.3333333333333333703, 0.3219752754296894559, 0.3333333333333333703, 0.3219752754296894559, 0.3333333333333333703, 0.3219752754296894559, 0.3333333333333333703, 0.3219752754296894559, 0.3333333333333333703, 0.3219752754296894559, 0.3333333333333333703, 0.3219752754296894559, 0.3333333333333333703, 0.3219752754296894559, 0.3333333333333333703, 0.3219752754296894559, 0.3333333333333333703, 0.3219752754296894559, 0.3333333333333333703, 0.3219752754296894559, 0.3333333333333333703, 0.3219752754296894559, 0.3333333333333333703, 0.3219752754296894559, 0.3333333333333333703, 0.3219752754296894559, 0.3333333333333333703, 0.3219752754296894559, 0.3333333333333333703, 0.3219752754296894559, 0.3333333333333333703, 0.3219752754296894559, 0.3333333333333333703, 0.3219752754296894559, 0.3333333333333333703, 0.3219752754296894559, 0.3333333333333333703, 0.3219752754296894559, 0.3333333333333333703, 0.3219752754296894559, 0.3333333333333333703, 0.3219752754296894559, 0.3333333333333333703, 0.3219752754296894559, 0.3333333333333333703, 0.3219752754296894559, 0.3333333333333333703, 0.3219752754296894559, 0.3333333333333333703, 0.3219752754296894559, 0.3333333333333333703, 0.3219752754296894559, 0.3333333333333333703, 0.3219752754296894559, 0.3333333333333333703, 0.3219752754296894559, 0.3333333333333333703, 0.3219752754296894559, 0.3333333333333333703, 0.3219752754296894559, 0.3333333333333333703, 0.3219752754296894559, 0.3333333333333333703, 0.3219752754296894559, 0.3333333333333333703, 0.3219752754296894559, 0.3333333333333333703, 0.3219752754296894559, 0.3333333333333333703, 0.3219752754296894559, 0.3333333333333333703, 0.3219752754296894559, 0.3333333333333333703, 0.3219752754296894559, 0.3333333333333333703, 0.3219752754296894559, 0.3333333333333333703, 0.3219752754296894559, 0.3333333333333333703, 0.3219752754296894559, 0.3333333333333333703, 0.3219752754296894559, 0.3333333333333333703, 0.3219752754296894559, 0.3333333333333333703, 0.3219752754296894559, 0.3333333333333333703, 0.3219752754296894559, 0.3333333333333333703, 0.3219752754296894559, 0.3333333333333333703, 0.3219752754296894559, 0.3333333333333333703, 0.3219752754296894559, 0.3333333333333333703, 0.3219752754296894559, 0.3333333333333333703, 0.3219752754296894559, 0.3333333333333333703, 0.3219752754296894559, 0.3333333333333333703, 0.3219752754296894559, 0.3333333333333333703, 0.3219752754296894559, 0.3333333333333333703, 0.3219752754296894559, 0.3333333333333333703, 0.3219752754296894559, 0.3333333333333333703, 0.3219752754296894559, 0.3333333333333333703, 0.3219752754296894559, 0.3333333333333333703, 0.3219752754296894559, 0.3333333333333333703, 0.3219752754296894559, 0.3333333333333333703, 0.3219752754296894559, 0.3333333333333333703, 0.3219752754296894559, 0.3333333333333333703, 0.3219752754296894559, 0.3333333333333333703, 0.3219752754296894559, 0.3333333333333333703, 0.3219752754296894559, 0.3333333333333333703, 0.3219752754296894559, 0.3333333333333333703, 0.3219752754296894559, 0.3333333333333333703, 0.3219752754296894559, 0.3333333333333333703, 0.3219752754296894559, 0.3333333333333333703, 0.3219752754296894559, 0.3333333333333333703, 0.3219752754296894559, 0.3333333333333333703, 0.3219752754296894559, 0.3333333333333333703, 0.3219752754296894559, 0.3333333333333333703, 0.3219752754296894559, 0.3333333333333333703, 0.3219752754296894559, 0.3333333333333333703, 0.3219752754296894559, 0.3333333333333333703, 0.3219752754296894559, 0.3333333333333333703, 0.3219752754296894559, 0.3333333333333333703, 0.3219752754296894559, 0.3333333333333333703, 0.3219752754296894559, 0.3333333333333333703, 0.3219752754296894559, 0.3333333333333333703, 0.3219752754296894559, 0.3333333333333333703, 0.3219752754296894559, 0.3333333333333333703, 0.3219752754296894559, 0.3333333333333333703, 0.3219752754296894559, 0.3333333333333333703, 0.3219752754296894559, 0.3333333333333333703, 0.3219752754296894559, 0.3333333333333333703, 0.3219752754296894559, 0.3333333333333333703, 0.3219752754296894559, 0.3333333333333333703, 0.3219752754296894559, 0.3333333333333333703, 0.3219752754296894559, 0.3333333333333333703, 0.3219752754296894559, 0.3333333333333333703, 0.3219752754296894559, 0.3333333333333333703, 0.3219752754296894559, 0.3333333333333333703, 0.3219752754296894559, 0.3333333333333333703, 0.3219752754296894559, 0.3333333333333333703, 0.3219752754296894559, 0.3333333333333333703, 0.3219752754296894559, 0.3333333333333333703, 0.3219752754296894559, 0.3333333333333333703, 0.3219752754296894559, 0.3333333333333333703, 0.3219752754296894559, 0.3333333333333333703, 0.3219752754296894559, 0.3333333333333333703, 0.3219752754296894559, 0.3333333333333333703, 0.3219752754296894559, 0.3333333333333333703, 0.3219752754296894559, 0.3333333333333333703, 0.3219752754296894559, 0.3333333333333333703, 0.3219752754296894559, 0.3333333333333333703, 0.3219752754296894559, 0.3333333333333333703, 0.3219752754296894559, 0.3333333333333333703, 0.3219752754296894559, 0.3333333333333333703, 0.3219752754296894559, 0.3333333333333333703, 0.3219752754296894559, 0.3333333333333333703, 0.3219752754296894559, 0.3333333333333333703, 0.3219752754296894559, 0.3333333333333333703, 0.3219752754296894559, 0.3333333333333333703, 0.3219752754296894559, 0.3333333333333333703, 0.3219752754296894559, 0.3333333333333333703, 0.3219752754296894559, 0.3333333333333333703, 0.3219752754296894559, 0.3333333333333333703, 0.3219752754296894559, 0.3333333333333333703, 0.3219752754296894559, 0.3333333333333333703, 0.3219752754296894559, 0.3333333333333333703, 0.3219752754296894559, 0.3333333333333333703, 0.3219752754296894559, 0.3333333333333333703, 0.3219752754296894559, 0.3333333333333333703, 0.3219752754296894559, 0.3333333333333333703, 0.3219752754296894559, 0.3333333333333333703, 0.3219752754296894559, 0.3333333333333333703, 0.3219752754296894559, 0.3333333333333333703, 0.3219752754296894559, 0.3333333333333333703, 0.3219752754296894559, 0.3333333333333333703, 0.3219752754296894559, 0.3333333333333333703, 0.3219752754296894559, 0.3333333333333333703, 0.3219752754296894559, 0.3333333333333333703, 0.3219752754296894559, 0.3333333333333333703, 0.3219752754296894559, 0.3333333333333333703, 0.3219752754296894559, 0.3333333333333333703, 0.3219752754296894559, 0.3333333333333333703, 0.3219752754296894559, 0.3333333333333333703, 0.3219752754296894559, 0.3333333333333333703, 0.3219752754296894559, 0.3333333333333333703, 0.3219752754296894559, 0.3333333333333333703, 0.3219752754296894559, 0.3333333333333333703, 0.3219752754296894559, 0.3333333333333333703, 0.3219752754296894559, 0.3333333333333333703, 0.3219752754296894559, 0.3333333333333333703, 0.3219752754296894559, 0.3333333333333333703, 0.3219752754296894559, 0.3333333333333333703, 0.3219752754296894559, 0.3333333333333333703, 0.3219752754296894559, 0.3333333333333333703, 0.3219752754296894559, 0.3333333333333333703, 0.3219752754296894559, 0.3333333333333333703, 0.3219752754296894559, 0.3333333333333333703, 0.3219752754296894559, 0.3333333333333333703, 0.3219752754296894559, 0.3333333333333333703, 0.3219752754296894559, 0.3333333333333333703, 0.3219752754296894559, 0.3333333333333333703),
 ( 0.3333333333333333703, 0.3219752754296894559, 0.3333333333333333703, 0.3219752754296894559, 0.3333333333333333703, 0.3219752754296894559, 0.3333333333333333703, 0.3219752754296894559, 0.3333333333333333703, 0.3219752754296894559, 0.3333333333333333703, 0.3219752754296894559, 0.3333333333333333703, 0.3219752754296894559, 0.3333333333333333703, 0.3219752754296894559, 0.3333333333333333703, 0.3219752754296894559, 0.3333333333333333703, 0.3219752754296894559, 0.3333333333333333703, 0.3219752754296894559, 0.3333333333333333703, 0.3219752754296894559, 0.3333333333333333703, 0.3219752754296894559, 0.3333333333333333703, 0.3219752754296894559, 0.3333333333333333703, 0.3219752754296894559, 0.3333333333333333703, 0.3219752754296894559, 0.3333333333333333703, 0.3219752754296894559, 0.3333333333333333703, 0.3219752754296894559, 0.3333333333333333703, 0.3219752754296894559, 0.3333333333333333703, 0.3219752754296894559, 0.3333333333333333703, 0.3219752754296894559, 0.3333333333333333703, 0.3219752754296894559, 0.3333333333333333703, 0.3219752754296894559, 0.3333333333333333703, 0.3219752754296894559, 0.3333333333333333703, 0.3219752754296894559, 0.3333333333333333703, 0.3219752754296894559, 0.3333333333333333703, 0.3219752754296894559, 0.3333333333333333703, 0.3219752754296894559, 0.3333333333333333703, 0.3219752754296894559, 0.3333333333333333703, 0.3219752754296894559, 0.3333333333333333703, 0.3219752754296894559, 0.3333333333333333703, 0.3219752754296894559, 0.3333333333333333703, 0.3219752754296894559, 0.3333333333333333703, 0.3219752754296894559, 0.3333333333333333703, 0.3219752754296894559, 0.3333333333333333703, 0.3219752754296894559, 0.3333333333333333703, 0.3219752754296894559, 0.3333333333333333703, 0.3219752754296894559, 0.3333333333333333703, 0.3219752754296894559, 0.3333333333333333703, 0.3219752754296894559, 0.3333333333333333703, 0.3219752754296894559, 0.3333333333333333703, 0.3219752754296894559, 0.3333333333333333703, 0.3219752754296894559, 0.3333333333333333703, 0.3219752754296894559, 0.3333333333333333703, 0.3219752754296894559, 0.3333333333333333703, 0.3219752754296894559, 0.3333333333333333703, 0.3219752754296894559, 0.3333333333333333703, 0.3219752754296894559, 0.3333333333333333703, 0.3219752754296894559, 0.3333333333333333703, 0.3219752754296894559, 0.3333333333333333703, 0.3219752754296894559, 0.3333333333333333703, 0.3219752754296894559, 0.3333333333333333703, 0.3219752754296894559, 0.3333333333333333703, 0.3219752754296894559, 0.3333333333333333703, 0.3219752754296894559, 0.3333333333333333703, 0.3219752754296894559, 0.3333333333333333703, 0.3219752754296894559, 0.3333333333333333703, 0.3219752754296894559, 0.3333333333333333703, 0.3219752754296894559, 0.3333333333333333703, 0.3219752754296894559, 0.3333333333333333703, 0.3219752754296894559, 0.3333333333333333703, 0.3219752754296894559, 0.3333333333333333703, 0.3219752754296894559, 0.3333333333333333703, 0.3219752754296894559, 0.3333333333333333703, 0.3219752754296894559, 0.3333333333333333703, 0.3219752754296894559, 0.3333333333333333703, 0.3219752754296894559, 0.3333333333333333703, 0.3219752754296894559, 0.3333333333333333703, 0.3219752754296894559, 0.3333333333333333703, 0.3219752754296894559, 0.3333333333333333703, 0.3219752754296894559, 0.3333333333333333703, 0.3219752754296894559, 0.3333333333333333703, 0.3219752754296894559, 0.3333333333333333703, 0.3219752754296894559, 0.3333333333333333703, 0.3219752754296894559, 0.3333333333333333703, 0.3219752754296894559, 0.3333333333333333703, 0.3219752754296894559, 0.3333333333333333703, 0.3219752754296894559, 0.3333333333333333703, 0.3219752754296894559, 0.3333333333333333703, 0.3219752754296894559, 0.3333333333333333703, 0.3219752754296894559, 0.3333333333333333703, 0.3219752754296894559, 0.3333333333333333703, 0.3219752754296894559, 0.3333333333333333703, 0.3219752754296894559, 0.3333333333333333703, 0.3219752754296894559, 0.3333333333333333703, 0.3219752754296894559, 0.3333333333333333703, 0.3219752754296894559, 0.3333333333333333703, 0.3219752754296894559, 0.3333333333333333703, 0.3219752754296894559, 0.3333333333333333703, 0.3219752754296894559, 0.3333333333333333703, 0.3219752754296894559, 0.3333333333333333703, 0.3219752754296894559, 0.3333333333333333703, 0.3219752754296894559, 0.3333333333333333703, 0.3219752754296894559, 0.3333333333333333703, 0.3219752754296894559, 0.3333333333333333703, 0.3219752754296894559, 0.3333333333333333703, 0.3219752754296894559, 0.3333333333333333703, 0.3219752754296894559, 0.3333333333333333703, 0.3219752754296894559, 0.3333333333333333703, 0.3219752754296894559, 0.3333333333333333703, 0.3219752754296894559, 0.3333333333333333703, 0.3219752754296894559, 0.3333333333333333703, 0.3219752754296894559, 0.3333333333333333703, 0.3219752754296894559, 0.3333333333333333703, 0.3219752754296894559, 0.3333333333333333703, 0.3219752754296894559, 0.3333333333333333703, 0.3219752754296894559, 0.3333333333333333703, 0.3219752754296894559, 0.3333333333333333703, 0.3219752754296894559, 0.3333333333333333703, 0.3219752754296894559, 0.3333333333333333703, 0.3219752754296894559, 0.3333333333333333703, 0.3219752754296894559, 0.3333333333333333703, 0.3219752754296894559, 0.3333333333333333703, 0.3219752754296894559, 0.3333333333333333703, 0.3219752754296894559, 0.3333333333333333703, 0.3219752754296894559, 0.3333333333333333703, 0.3219752754296894559, 0.3333333333333333703, 0.3219752754296894559, 0.3333333333333333703, 0.3219752754296894559, 0.3333333333333333703, 0.3219752754296894559, 0.3333333333333333703, 0.3219752754296894559, 0.3333333333333333703, 0.3219752754296894559, 0.3333333333333333703, 0.3219752754296894559, 0.3333333333333333703, 0.3219752754296894559, 0.3333333333333333703, 0.3219752754296894559, 0.3333333333333333703, 0.3219752754296894559, 0.3333333333333333703, 0.3219752754296894559, 0.3333333333333333703, 0.3219752754296894559, 0.3333333333333333703, 0.3219752754296894559, 0.3333333333333333703, 0.3219752754296894559, 0.3333333333333333703, 0.3219752754296894559, 0.3333333333333333703, 0.3219752754296894559, 0.3333333333333333703, 0.3219752754296894559, 0.3333333333333333703, 0.3219752754296894559, 0.3333333333333333703, 0.3219752754296894559, 0.3333333333333333703, 0.3219752754296894559, 0.3333333333333333703, 0.3219752754296894559, 0.3333333333333333703, 0.3219752754296894559, 0.3333333333333333703, 0.3219752754296894559, 0.3333333333333333703, 0.3219752754296894559, 0.3333333333333333703, 0.3219752754296894559, 0.3333333333333333703, 0.3219752754296894559, 0.3333333333333333703, 0.3219752754296894559, 0.3333333333333333703, 0.3219752754296894559, 0.3333333333333333703, 0.3219752754296894559, 0.3333333333333333703, 0.3219752754296894559, 0.3333333333333333703, 0.3219752754296894559, 0.3333333333333333703, 0.3219752754296894559, 0.3333333333333333703, 0.3219752754296894559, 0.3333333333333333703, 0.3219752754296894559, 0.3333333333333333703, 0.3219752754296894559, 0.3333333333333333703, 0.3219752754296894559, 0.3333333333333333703, 0.3219752754296894559, 0.3333333333333333703, 0.3219752754296894559, 0.3333333333333333703, 0.3219752754296894559, 0.3333333333333333703, 0.3219752754296894559, 0.3333333333333333703, 0.3219752754296894559, 0.3333333333333333703, 0.3219752754296894559, 0.3333333333333333703, 0.3219752754296894559, 0.3333333333333333703, 0.3219752754296894559, 0.3333333333333333703, 0.3219752754296894559, 0.3333333333333333703, 0.3219752754296894559, 0.3333333333333333703, 0.3219752754296894559, 0.3333333333333333703, 0.3219752754296894559, 0.3333333333333333703, 0.3219752754296894559, 0.3333333333333333703, 0.3219752754296894559, 0.3333333333333333703, 0.3219752754296894559, 0.3333333333333333703, 0.3219752754296894559, 0.3333333333333333703, 0.3219752754296894559, 0.3333333333333333703, 0.3219752754296894559, 0.3333333333333333703, 0.3219752754296894559, 0.3333333333333333703, 0.3219752754296894559, 0.3333333333333333703, 0.3219752754296894559, 0.3333333333333333703, 0.3219752754296894559, 0.3333333333333333703, 0.3219752754296894559, 0.3333333333333333703, 0.3219752754296894559, 0.3333333333333333703, 0.3219752754296894559, 0.3333333333333333703, 0.3219752754296894559, 0.3333333333333333703, 0.3219752754296894559, 0.3333333333333333703, 0.3219752754296894559, 0.3333333333333333703, 0.3219752754296894559, 0.3333333333333333703, 0.3219752754296894559, 0.3333333333333333703, 0.3219752754296894559, 0.3333333333333333703, 0.3219752754296894559, 0.3333333333333333703, 0.3219752754296894559, 0.3333333333333333703, 0.3219752754296894559, 0.3333333333333333703, 0.3219752754296894559, 0.3333333333333333703, 0.3219752754296894559, 0.3333333333333333703, 0.3219752754296894559, 0.3333333333333333703, 0.3219752754296894559, 0.3333333333333333703, 0.3219752754296894559, 0.3333333333333333703, 0.3219752754296894559, 0.3333333333333333703, 0.3219752754296894559, 0.3333333333333333703, 0.3219752754296894559, 0.3333333333333333703, 0.3219752754296894559, 0.3333333333333333703, 0.3219752754296894559, 0.3333333333333333703, 0.3219752754296894559, 0.3333333333333333703, 0.3219752754296894559, 0.3333333333333333703, 0.3219752754296894559, 0.3333333333333333703, 0.3219752754296894559, 0.3333333333333333703, 0.3219752754296894559, 0.3333333333333333703, 0.3219752754296894559, 0.3333333333333333703, 0.3219752754296894559, 0.3333333333333333703, 0.3219752754296894559, 0.3333333333333333703, 0.3219752754296894559, 0.3333333333333333703, 0.3219752754296894559, 0.3333333333333333703, 0.3219752754296894559, 0.3333333333333333703, 0.3219752754296894559, 0.3333333333333333703, 0.3219752754296894559, 0.3333333333333333703, 0.3219752754296894559, 0.3333333333333333703, 0.3219752754296894559, 0.3333333333333333703, 0.3219752754296894559, 0.3333333333333333703, 0.3219752754296894559, 0.3333333333333333703, 0.3219752754296894559, 0.3333333333333333703, 0.3219752754296894559, 0.3333333333333333703, 0.3219752754296894559, 0.3333333333333333703, 0.3219752754296894559, 0.3333333333333333703, 0.3219752754296894559, 0.3333333333333333703, 0.3219752754296894559, 0.3333333333333333703, 0.3219752754296894559, 0.3333333333333333703, 0.3219752754296894559, 0.3333333333333333703, 0.3219752754296894559, 0.3333333333333333703, 0.3219752754296894559, 0.3333333333333333703, 0.3219752754296894559, 0.3333333333333333703, 0.3219752754296894559, 0.3333333333333333703, 0.3219752754296894559, 0.3333333333333333703, 0.3219752754296894559, 0.3333333333333333703, 0.3219752754296894559, 0.3333333333333333703),
 ( 1.000000000000000000, 0.9659258262890683122, 1.000000000000000000, 0.9659258262890683122, 1.000000000000000000, 0.9659258262890683122, 1.000000000000000000, 0.9659258262890683122, 1.000000000000000000, 0.9659258262890683122, 1.000000000000000000, 0.9659258262890683122, 1.000000000000000000, 0.9659258262890683122, 1.000000000000000000, 0.9659258262890683122, 1.000000000000000000, 0.9659258262890683122, 1.000000000000000000, 0.9659258262890683122, 1.000000000000000000, 0.9659258262890683122, 1.000000000000000000, 0.9659258262890683122, 1.000000000000000000, 0.9659258262890683122, 1.000000000000000000, 0.9659258262890683122, 1.000000000000000000, 0.9659258262890683122, 1.000000000000000000, 0.9659258262890683122, 1.000000000000000000, 0.9659258262890683122, 1.000000000000000000, 0.9659258262890683122, 1.000000000000000000, 0.9659258262890683122, 1.000000000000000000, 0.9659258262890683122, 1.000000000000000000, 0.9659258262890683122, 1.000000000000000000, 0.9659258262890683122, 1.000000000000000000, 0.9659258262890683122, 1.000000000000000000, 0.9659258262890683122, 1.000000000000000000, 0.9659258262890683122, 1.000000000000000000, 0.9659258262890683122, 1.000000000000000000, 0.9659258262890683122, 1.000000000000000000, 0.9659258262890683122, 1.000000000000000000, 0.9659258262890683122, 1.000000000000000000, 0.9659258262890683122, 1.000000000000000000, 0.9659258262890683122, 1.000000000000000000, 0.9659258262890683122, 1.000000000000000000, 0.9659258262890683122, 1.000000000000000000, 0.9659258262890683122, 1.000000000000000000, 0.9659258262890683122, 1.000000000000000000, 0.9659258262890683122, 1.000000000000000000, 0.9659258262890683122, 1.000000000000000000, 0.9659258262890683122, 1.000000000000000000, 0.9659258262890683122, 1.000000000000000000, 0.9659258262890683122, 1.000000000000000000, 0.9659258262890683122, 1.000000000000000000, 0.9659258262890683122, 1.000000000000000000, 0.9659258262890683122, 1.000000000000000000, 0.9659258262890683122, 1.000000000000000000, 0.9659258262890683122, 1.000000000000000000, 0.9659258262890683122, 1.000000000000000000, 0.9659258262890683122, 1.000000000000000000, 0.9659258262890683122, 1.000000000000000000, 0.9659258262890683122, 1.000000000000000000, 0.9659258262890683122, 1.000000000000000000, 0.9659258262890683122, 1.000000000000000000, 0.9659258262890683122, 1.000000000000000000, 0.9659258262890683122, 1.000000000000000000, 0.9659258262890683122, 1.000000000000000000, 0.9659258262890683122, 1.000000000000000000, 0.9659258262890683122, 1.000000000000000000, 0.9659258262890683122, 1.000000000000000000, 0.9659258262890683122, 1.000000000000000000, 0.9659258262890683122, 1.000000000000000000, 0.9659258262890683122, 1.000000000000000000, 0.9659258262890683122, 1.000000000000000000, 0.9659258262890683122, 1.000000000000000000, 0.9659258262890683122, 1.000000000000000000, 0.9659258262890683122, 1.000000000000000000, 0.9659258262890683122, 1.000000000000000000, 0.9659258262890683122, 1.000000000000000000, 0.9659258262890683122, 1.000000000000000000, 0.9659258262890683122, 1.000000000000000000, 0.9659258262890683122, 1.000000000000000000, 0.9659258262890683122, 1.000000000000000000, 0.9659258262890683122, 1.000000000000000000, 0.9659258262890683122, 1.000000000000000000, 0.9659258262890683122, 1.000000000000000000, 0.9659258262890683122, 1.000000000000000000, 0.9659258262890683122, 1.000000000000000000, 0.9659258262890683122, 1.000000000000000000, 0.9659258262890683122, 1.000000000000000000, 0.9659258262890683122, 1.000000000000000000, 0.9659258262890683122, 1.000000000000000000, 0.9659258262890683122, 1.000000000000000000, 0.9659258262890683122, 1.000000000000000000, 0.9659258262890683122, 1.000000000000000000, 0.9659258262890683122, 1.000000000000000000, 0.9659258262890683122, 1.000000000000000000, 0.9659258262890683122, 1.000000000000000000, 0.9659258262890683122, 1.000000000000000000, 0.9659258262890683122, 1.000000000000000000, 0.9659258262890683122, 1.000000000000000000, 0.9659258262890683122, 1.000000000000000000, 0.9659258262890683122, 1.000000000000000000, 0.9659258262890683122, 1.000000000000000000, 0.9659258262890683122, 1.000000000000000000, 0.9659258262890683122, 1.000000000000000000, 0.9659258262890683122, 1.000000000000000000, 0.9659258262890683122, 1.000000000000000000, 0.9659258262890683122, 1.000000000000000000, 0.9659258262890683122, 1.000000000000000000, 0.9659258262890683122, 1.000000000000000000, 0.9659258262890683122, 1.000000000000000000, 0.9659258262890683122, 1.000000000000000000, 0.9659258262890683122, 1.000000000000000000, 0.9659258262890683122, 1.000000000000000000, 0.9659258262890683122, 1.000000000000000000, 0.9659258262890683122, 1.000000000000000000, 0.9659258262890683122, 1.000000000000000000, 0.9659258262890683122, 1.000000000000000000, 0.9659258262890683122, 1.000000000000000000, 0.9659258262890683122, 1.000000000000000000, 0.9659258262890683122, 1.000000000000000000, 0.9659258262890683122, 1.000000000000000000, 0.9659258262890683122, 1.000000000000000000, 0.9659258262890683122, 1.000000000000000000, 0.9659258262890683122, 1.000000000000000000, 0.9659258262890683122, 1.000000000000000000, 0.9659258262890683122, 1.000000000000000000, 0.9659258262890683122, 1.000000000000000000, 0.9659258262890683122, 1.000000000000000000, 0.9659258262890683122, 1.000000000000000000, 0.9659258262890683122, 1.000000000000000000, 0.9659258262890683122, 1.000000000000000000, 0.9659258262890683122, 1.000000000000000000, 0.9659258262890683122, 1.000000000000000000, 0.9659258262890683122, 1.000000000000000000, 0.9659258262890683122, 1.000000000000000000, 0.9659258262890683122, 1.000000000000000000, 0.9659258262890683122, 1.000000000000000000, 0.9659258262890683122, 1.000000000000000000, 0.9659258262890683122, 1.000000000000000000, 0.9659258262890683122, 1.000000000000000000, 0.9659258262890683122, 1.000000000000000000, 0.9659258262890683122, 1.000000000000000000, 0.9659258262890683122, 1.000000000000000000, 0.9659258262890683122, 1.000000000000000000, 0.9659258262890683122, 1.000000000000000000, 0.9659258262890683122, 1.000000000000000000, 0.9659258262890683122, 1.000000000000000000, 0.9659258262890683122, 1.000000000000000000, 0.9659258262890683122, 1.000000000000000000, 0.9659258262890683122, 1.000000000000000000, 0.9659258262890683122, 1.000000000000000000, 0.9659258262890683122, 1.000000000000000000, 0.9659258262890683122, 1.000000000000000000, 0.9659258262890683122, 1.000000000000000000, 0.9659258262890683122, 1.000000000000000000, 0.9659258262890683122, 1.000000000000000000, 0.9659258262890683122, 1.000000000000000000, 0.9659258262890683122, 1.000000000000000000, 0.9659258262890683122, 1.000000000000000000, 0.9659258262890683122, 1.000000000000000000, 0.9659258262890683122, 1.000000000000000000, 0.9659258262890683122, 1.000000000000000000, 0.9659258262890683122, 1.000000000000000000, 0.9659258262890683122, 1.000000000000000000, 0.9659258262890683122, 1.000000000000000000, 0.9659258262890683122, 1.000000000000000000, 0.9659258262890683122, 1.000000000000000000, 0.9659258262890683122, 1.000000000000000000, 0.9659258262890683122, 1.000000000000000000, 0.9659258262890683122, 1.000000000000000000, 0.9659258262890683122, 1.000000000000000000, 0.9659258262890683122, 1.000000000000000000, 0.9659258262890683122, 1.000000000000000000, 0.9659258262890683122, 1.000000000000000000, 0.9659258262890683122, 1.000000000000000000, 0.9659258262890683122, 1.000000000000000000, 0.9659258262890683122, 1.000000000000000000, 0.9659258262890683122, 1.000000000000000000, 0.9659258262890683122, 1.000000000000000000, 0.9659258262890683122, 1.000000000000000000, 0.9659258262890683122, 1.000000000000000000, 0.9659258262890683122, 1.000000000000000000, 0.9659258262890683122, 1.000000000000000000, 0.9659258262890683122, 1.000000000000000000, 0.9659258262890683122, 1.000000000000000000, 0.9659258262890683122, 1.000000000000000000, 0.9659258262890683122, 1.000000000000000000, 0.9659258262890683122, 1.000000000000000000, 0.9659258262890683122, 1.000000000000000000, 0.9659258262890683122, 1.000000000000000000, 0.9659258262890683122, 1.000000000000000000, 0.9659258262890683122, 1.000000000000000000, 0.9659258262890683122, 1.000000000000000000, 0.9659258262890683122, 1.000000000000000000, 0.9659258262890683122, 1.000000000000000000, 0.9659258262890683122, 1.000000000000000000, 0.9659258262890683122, 1.000000000000000000, 0.9659258262890683122, 1.000000000000000000, 0.9659258262890683122, 1.000000000000000000, 0.9659258262890683122, 1.000000000000000000, 0.9659258262890683122, 1.000000000000000000, 0.9659258262890683122, 1.000000000000000000, 0.9659258262890683122, 1.000000000000000000, 0.9659258262890683122, 1.000000000000000000, 0.9659258262890683122, 1.000000000000000000, 0.9659258262890683122, 1.000000000000000000, 0.9659258262890683122, 1.000000000000000000, 0.9659258262890683122, 1.000000000000000000, 0.9659258262890683122, 1.000000000000000000, 0.9659258262890683122, 1.000000000000000000, 0.9659258262890683122, 1.000000000000000000, 0.9659258262890683122, 1.000000000000000000, 0.9659258262890683122, 1.000000000000000000, 0.9659258262890683122, 1.000000000000000000, 0.9659258262890683122, 1.000000000000000000, 0.9659258262890683122, 1.000000000000000000, 0.9659258262890683122, 1.000000000000000000, 0.9659258262890683122, 1.000000000000000000, 0.9659258262890683122, 1.000000000000000000, 0.9659258262890683122, 1.000000000000000000, 0.9659258262890683122, 1.000000000000000000, 0.9659258262890683122, 1.000000000000000000, 0.9659258262890683122, 1.000000000000000000, 0.9659258262890683122, 1.000000000000000000, 0.9659258262890683122, 1.000000000000000000, 0.9659258262890683122, 1.000000000000000000, 0.9659258262890683122, 1.000000000000000000, 0.9659258262890683122, 1.000000000000000000, 0.9659258262890683122, 1.000000000000000000, 0.9659258262890683122, 1.000000000000000000, 0.9659258262890683122, 1.000000000000000000, 0.9659258262890683122, 1.000000000000000000, 0.9659258262890683122, 1.000000000000000000, 0.9659258262890683122, 1.000000000000000000, 0.9659258262890683122, 1.000000000000000000, 0.9659258262890683122, 1.000000000000000000, 0.9659258262890683122, 1.000000000000000000, 0.9659258262890683122, 1.000000000000000000, 0.9659258262890683122, 1.000000000000000000),
 ( 0.3333333333333333703, 0.3219752754296894559, 0.3333333333333333703, 0.3219752754296894559, 0.3333333333333333703, 0.3219752754296894559, 0.3333333333333333703, 0.3219752754296894559, 0.3333333333333333703, 0.3219752754296894559, 0.3333333333333333703, 0.3219752754296894559, 0.3333333333333333703, 0.3219752754296894559, 0.3333333333333333703, 0.3219752754296894559, 0.3333333333333333703, 0.3219752754296894559, 0.3333333333333333703, 0.3219752754296894559, 0.3333333333333333703, 0.3219752754296894559, 0.3333333333333333703, 0.3219752754296894559, 0.3333333333333333703, 0.3219752754296894559, 0.3333333333333333703, 0.3219752754296894559, 0.3333333333333333703, 0.3219752754296894559, 0.3333333333333333703, 0.3219752754296894559, 0.3333333333333333703, 0.3219752754296894559, 0.3333333333333333703, 0.3219752754296894559, 0.3333333333333333703, 0.3219752754296894559, 0.3333333333333333703, 0.3219752754296894559, 0.3333333333333333703, 0.3219752754296894559, 0.3333333333333333703, 0.3219752754296894559, 0.3333333333333333703, 0.3219752754296894559, 0.3333333333333333703, 0.3219752754296894559, 0.3333333333333333703, 0.3219752754296894559, 0.3333333333333333703, 0.3219752754296894559, 0.3333333333333333703, 0.3219752754296894559, 0.3333333333333333703, 0.3219752754296894559, 0.3333333333333333703, 0.3219752754296894559, 0.3333333333333333703, 0.3219752754296894559, 0.3333333333333333703, 0.3219752754296894559, 0.3333333333333333703, 0.3219752754296894559, 0.3333333333333333703, 0.3219752754296894559, 0.3333333333333333703, 0.3219752754296894559, 0.3333333333333333703, 0.3219752754296894559, 0.3333333333333333703, 0.3219752754296894559, 0.3333333333333333703, 0.3219752754296894559, 0.3333333333333333703, 0.3219752754296894559, 0.3333333333333333703, 0.3219752754296894559, 0.3333333333333333703, 0.3219752754296894559, 0.3333333333333333703, 0.3219752754296894559, 0.3333333333333333703, 0.3219752754296894559, 0.3333333333333333703, 0.3219752754296894559, 0.3333333333333333703, 0.3219752754296894559, 0.3333333333333333703, 0.3219752754296894559, 0.3333333333333333703, 0.3219752754296894559, 0.3333333333333333703, 0.3219752754296894559, 0.3333333333333333703, 0.3219752754296894559, 0.3333333333333333703, 0.3219752754296894559, 0.3333333333333333703, 0.3219752754296894559, 0.3333333333333333703, 0.3219752754296894559, 0.3333333333333333703, 0.3219752754296894559, 0.3333333333333333703, 0.3219752754296894559, 0.3333333333333333703, 0.3219752754296894559, 0.3333333333333333703, 0.3219752754296894559, 0.3333333333333333703, 0.3219752754296894559, 0.3333333333333333703, 0.3219752754296894559, 0.3333333333333333703, 0.3219752754296894559, 0.3333333333333333703, 0.3219752754296894559, 0.3333333333333333703, 0.3219752754296894559, 0.3333333333333333703, 0.3219752754296894559, 0.3333333333333333703, 0.3219752754296894559, 0.3333333333333333703, 0.3219752754296894559, 0.3333333333333333703, 0.3219752754296894559, 0.3333333333333333703, 0.3219752754296894559, 0.3333333333333333703, 0.3219752754296894559, 0.3333333333333333703, 0.3219752754296894559, 0.3333333333333333703, 0.3219752754296894559, 0.3333333333333333703, 0.3219752754296894559, 0.3333333333333333703, 0.3219752754296894559, 0.3333333333333333703, 0.3219752754296894559, 0.3333333333333333703, 0.3219752754296894559, 0.3333333333333333703, 0.3219752754296894559, 0.3333333333333333703, 0.3219752754296894559, 0.3333333333333333703, 0.3219752754296894559, 0.3333333333333333703, 0.3219752754296894559, 0.3333333333333333703, 0.3219752754296894559, 0.3333333333333333703, 0.3219752754296894559, 0.3333333333333333703, 0.3219752754296894559, 0.3333333333333333703, 0.3219752754296894559, 0.3333333333333333703, 0.3219752754296894559, 0.3333333333333333703, 0.3219752754296894559, 0.3333333333333333703, 0.3219752754296894559, 0.3333333333333333703, 0.3219752754296894559, 0.3333333333333333703, 0.3219752754296894559, 0.3333333333333333703, 0.3219752754296894559, 0.3333333333333333703, 0.3219752754296894559, 0.3333333333333333703, 0.3219752754296894559, 0.3333333333333333703, 0.3219752754296894559, 0.3333333333333333703, 0.3219752754296894559, 0.3333333333333333703, 0.3219752754296894559, 0.3333333333333333703, 0.3219752754296894559, 0.3333333333333333703, 0.3219752754296894559, 0.3333333333333333703, 0.3219752754296894559, 0.3333333333333333703, 0.3219752754296894559, 0.3333333333333333703, 0.3219752754296894559, 0.3333333333333333703, 0.3219752754296894559, 0.3333333333333333703, 0.3219752754296894559, 0.3333333333333333703, 0.3219752754296894559, 0.3333333333333333703, 0.3219752754296894559, 0.3333333333333333703, 0.3219752754296894559, 0.3333333333333333703, 0.3219752754296894559, 0.3333333333333333703, 0.3219752754296894559, 0.3333333333333333703, 0.3219752754296894559, 0.3333333333333333703, 0.3219752754296894559, 0.3333333333333333703, 0.3219752754296894559, 0.3333333333333333703, 0.3219752754296894559, 0.3333333333333333703, 0.3219752754296894559, 0.3333333333333333703, 0.3219752754296894559, 0.3333333333333333703, 0.3219752754296894559, 0.3333333333333333703, 0.3219752754296894559, 0.3333333333333333703, 0.3219752754296894559, 0.3333333333333333703, 0.3219752754296894559, 0.3333333333333333703, 0.3219752754296894559, 0.3333333333333333703, 0.3219752754296894559, 0.3333333333333333703, 0.3219752754296894559, 0.3333333333333333703, 0.3219752754296894559, 0.3333333333333333703, 0.3219752754296894559, 0.3333333333333333703, 0.3219752754296894559, 0.3333333333333333703, 0.3219752754296894559, 0.3333333333333333703, 0.3219752754296894559, 0.3333333333333333703, 0.3219752754296894559, 0.3333333333333333703, 0.3219752754296894559, 0.3333333333333333703, 0.3219752754296894559, 0.3333333333333333703, 0.3219752754296894559, 0.3333333333333333703, 0.3219752754296894559, 0.3333333333333333703, 0.3219752754296894559, 0.3333333333333333703, 0.3219752754296894559, 0.3333333333333333703, 0.3219752754296894559, 0.3333333333333333703, 0.3219752754296894559, 0.3333333333333333703, 0.3219752754296894559, 0.3333333333333333703, 0.3219752754296894559, 0.3333333333333333703, 0.3219752754296894559, 0.3333333333333333703, 0.3219752754296894559, 0.3333333333333333703, 0.3219752754296894559, 0.3333333333333333703, 0.3219752754296894559, 0.3333333333333333703, 0.3219752754296894559, 0.3333333333333333703, 0.3219752754296894559, 0.3333333333333333703, 0.3219752754296894559, 0.3333333333333333703, 0.3219752754296894559, 0.3333333333333333703, 0.3219752754296894559, 0.3333333333333333703, 0.3219752754296894559, 0.3333333333333333703, 0.3219752754296894559, 0.3333333333333333703, 0.3219752754296894559, 0.3333333333333333703, 0.3219752754296894559, 0.3333333333333333703, 0.3219752754296894559, 0.3333333333333333703, 0.3219752754296894559, 0.3333333333333333703, 0.3219752754296894559, 0.3333333333333333703, 0.3219752754296894559, 0.3333333333333333703, 0.3219752754296894559, 0.3333333333333333703, 0.3219752754296894559, 0.3333333333333333703, 0.3219752754296894559, 0.3333333333333333703, 0.3219752754296894559, 0.3333333333333333703, 0.3219752754296894559, 0.3333333333333333703, 0.3219752754296894559, 0.3333333333333333703, 0.3219752754296894559, 0.3333333333333333703, 0.3219752754296894559, 0.3333333333333333703, 0.3219752754296894559, 0.3333333333333333703, 0.3219752754296894559, 0.3333333333333333703, 0.3219752754296894559, 0.3333333333333333703, 0.3219752754296894559, 0.3333333333333333703, 0.3219752754296894559, 0.3333333333333333703, 0.3219752754296894559, 0.3333333333333333703, 0.3219752754296894559, 0.3333333333333333703, 0.3219752754296894559, 0.3333333333333333703, 0.3219752754296894559, 0.3333333333333333703, 0.3219752754296894559, 0.3333333333333333703, 0.3219752754296894559, 0.3333333333333333703, 0.3219752754296894559, 0.3333333333333333703, 0.3219752754296894559, 0.3333333333333333703, 0.3219752754296894559, 0.3333333333333333703, 0.3219752754296894559, 0.3333333333333333703, 0.3219752754296894559, 0.3333333333333333703, 0.3219752754296894559, 0.3333333333333333703, 0.3219752754296894559, 0.3333333333333333703, 0.3219752754296894559, 0.3333333333333333703, 0.3219752754296894559, 0.3333333333333333703, 0.3219752754296894559, 0.3333333333333333703, 0.3219752754296894559, 0.3333333333333333703, 0.3219752754296894559, 0.3333333333333333703, 0.3219752754296894559, 0.3333333333333333703, 0.3219752754296894559, 0.3333333333333333703, 0.3219752754296894559, 0.3333333333333333703, 0.3219752754296894559, 0.3333333333333333703, 0.3219752754296894559, 0.3333333333333333703, 0.3219752754296894559, 0.3333333333333333703, 0.3219752754296894559, 0.3333333333333333703, 0.3219752754296894559, 0.3333333333333333703, 0.3219752754296894559, 0.3333333333333333703, 0.3219752754296894559, 0.3333333333333333703, 0.3219752754296894559, 0.3333333333333333703, 0.3219752754296894559, 0.3333333333333333703, 0.3219752754296894559, 0.3333333333333333703, 0.3219752754296894559, 0.3333333333333333703, 0.3219752754296894559, 0.3333333333333333703, 0.3219752754296894559, 0.3333333333333333703, 0.3219752754296894559, 0.3333333333333333703, 0.3219752754296894559, 0.3333333333333333703, 0.3219752754296894559, 0.3333333333333333703, 0.3219752754296894559, 0.3333333333333333703, 0.3219752754296894559, 0.3333333333333333703, 0.3219752754296894559, 0.3333333333333333703, 0.3219752754296894559, 0.3333333333333333703, 0.3219752754296894559, 0.3333333333333333703, 0.3219752754296894559, 0.3333333333333333703, 0.3219752754296894559, 0.3333333333333333703, 0.3219752754296894559, 0.3333333333333333703, 0.3219752754296894559, 0.3333333333333333703, 0.3219752754296894559, 0.3333333333333333703, 0.3219752754296894559, 0.3333333333333333703, 0.3219752754296894559, 0.3333333333333333703, 0.3219752754296894559, 0.3333333333333333703, 0.3219752754296894559, 0.3333333333333333703, 0.3219752754296894559, 0.3333333333333333703, 0.3219752754296894559, 0.3333333333333333703, 0.3219752754296894559, 0.3333333333333333703, 0.3219752754296894559, 0.3333333333333333703, 0.3219752754296894559, 0.3333333333333333703, 0.3219752754296894559, 0.3333333333333333703, 0.3219752754296894559, 0.3333333333333333703, 0.3219752754296894559, 0.3333333333333333703, 0.3219752754296894559, 0.3333333333333333703, 0.3219752754296894559, 0.3333333333333333703, 0.3219752754296894559, 0.3333333333333333703, 0.3219752754296894559, 0.3333333333333333703, 0.3219752754296894559, 0.3333333333333333703, 0.3219752754296894559, 0.3333333333333333703, 0.3219752754296894559, 0.3333333333333333703),
 ( 0.3333333333333333703, 0.3219752754296894559, 0.3333333333333333703, 0.3219752754296894559, 0.3333333333333333703, 0.3219752754296894559, 0.3333333333333333703, 0.3219752754296894559, 0.3333333333333333703, 0.3219752754296894559, 0.3333333333333333703, 0.3219752754296894559, 0.3333333333333333703, 0.3219752754296894559, 0.3333333333333333703, 0.3219752754296894559, 0.3333333333333333703, 0.3219752754296894559, 0.3333333333333333703, 0.3219752754296894559, 0.3333333333333333703, 0.3219752754296894559, 0.3333333333333333703, 0.3219752754296894559, 0.3333333333333333703, 0.3219752754296894559, 0.3333333333333333703, 0.3219752754296894559, 0.3333333333333333703, 0.3219752754296894559, 0.3333333333333333703, 0.3219752754296894559, 0.3333333333333333703, 0.3219752754296894559, 0.3333333333333333703, 0.3219752754296894559, 0.3333333333333333703, 0.3219752754296894559, 0.3333333333333333703, 0.3219752754296894559, 0.3333333333333333703, 0.3219752754296894559, 0.3333333333333333703, 0.3219752754296894559, 0.3333333333333333703, 0.3219752754296894559, 0.3333333333333333703, 0.3219752754296894559, 0.3333333333333333703, 0.3219752754296894559, 0.3333333333333333703, 0.3219752754296894559, 0.3333333333333333703, 0.3219752754296894559, 0.3333333333333333703, 0.3219752754296894559, 0.3333333333333333703, 0.3219752754296894559, 0.3333333333333333703, 0.3219752754296894559, 0.3333333333333333703, 0.3219752754296894559, 0.3333333333333333703, 0.3219752754296894559, 0.3333333333333333703, 0.3219752754296894559, 0.3333333333333333703, 0.3219752754296894559, 0.3333333333333333703, 0.3219752754296894559, 0.3333333333333333703, 0.3219752754296894559, 0.3333333333333333703, 0.3219752754296894559, 0.3333333333333333703, 0.3219752754296894559, 0.3333333333333333703, 0.3219752754296894559, 0.3333333333333333703, 0.3219752754296894559, 0.3333333333333333703, 0.3219752754296894559, 0.3333333333333333703, 0.3219752754296894559, 0.3333333333333333703, 0.3219752754296894559, 0.3333333333333333703, 0.3219752754296894559, 0.3333333333333333703, 0.3219752754296894559, 0.3333333333333333703, 0.3219752754296894559, 0.3333333333333333703, 0.3219752754296894559, 0.3333333333333333703, 0.3219752754296894559, 0.3333333333333333703, 0.3219752754296894559, 0.3333333333333333703, 0.3219752754296894559, 0.3333333333333333703, 0.3219752754296894559, 0.3333333333333333703, 0.3219752754296894559, 0.3333333333333333703, 0.3219752754296894559, 0.3333333333333333703, 0.3219752754296894559, 0.3333333333333333703, 0.3219752754296894559, 0.3333333333333333703, 0.3219752754296894559, 0.3333333333333333703, 0.3219752754296894559, 0.3333333333333333703, 0.3219752754296894559, 0.3333333333333333703, 0.3219752754296894559, 0.3333333333333333703, 0.3219752754296894559, 0.3333333333333333703, 0.3219752754296894559, 0.3333333333333333703, 0.3219752754296894559, 0.3333333333333333703, 0.3219752754296894559, 0.3333333333333333703, 0.3219752754296894559, 0.3333333333333333703, 0.3219752754296894559, 0.3333333333333333703, 0.3219752754296894559, 0.3333333333333333703, 0.3219752754296894559, 0.3333333333333333703, 0.3219752754296894559, 0.3333333333333333703, 0.3219752754296894559, 0.3333333333333333703, 0.3219752754296894559, 0.3333333333333333703, 0.3219752754296894559, 0.3333333333333333703, 0.3219752754296894559, 0.3333333333333333703, 0.3219752754296894559, 0.3333333333333333703, 0.3219752754296894559, 0.3333333333333333703, 0.3219752754296894559, 0.3333333333333333703, 0.3219752754296894559, 0.3333333333333333703, 0.3219752754296894559, 0.3333333333333333703, 0.3219752754296894559, 0.3333333333333333703, 0.3219752754296894559, 0.3333333333333333703, 0.3219752754296894559, 0.3333333333333333703, 0.3219752754296894559, 0.3333333333333333703, 0.3219752754296894559, 0.3333333333333333703, 0.3219752754296894559, 0.3333333333333333703, 0.3219752754296894559, 0.3333333333333333703, 0.3219752754296894559, 0.3333333333333333703, 0.3219752754296894559, 0.3333333333333333703, 0.3219752754296894559, 0.3333333333333333703, 0.3219752754296894559, 0.3333333333333333703, 0.3219752754296894559, 0.3333333333333333703, 0.3219752754296894559, 0.3333333333333333703, 0.3219752754296894559, 0.3333333333333333703, 0.3219752754296894559, 0.3333333333333333703, 0.3219752754296894559, 0.3333333333333333703, 0.3219752754296894559, 0.3333333333333333703, 0.3219752754296894559, 0.3333333333333333703, 0.3219752754296894559, 0.3333333333333333703, 0.3219752754296894559, 0.3333333333333333703, 0.3219752754296894559, 0.3333333333333333703, 0.3219752754296894559, 0.3333333333333333703, 0.3219752754296894559, 0.3333333333333333703, 0.3219752754296894559, 0.3333333333333333703, 0.3219752754296894559, 0.3333333333333333703, 0.3219752754296894559, 0.3333333333333333703, 0.3219752754296894559, 0.3333333333333333703, 0.3219752754296894559, 0.3333333333333333703, 0.3219752754296894559, 0.3333333333333333703, 0.3219752754296894559, 0.3333333333333333703, 0.3219752754296894559, 0.3333333333333333703, 0.3219752754296894559, 0.3333333333333333703, 0.3219752754296894559, 0.3333333333333333703, 0.3219752754296894559, 0.3333333333333333703, 0.3219752754296894559, 0.3333333333333333703, 0.3219752754296894559, 0.3333333333333333703, 0.3219752754296894559, 0.3333333333333333703, 0.3219752754296894559, 0.3333333333333333703, 0.3219752754296894559, 0.3333333333333333703, 0.3219752754296894559, 0.3333333333333333703, 0.3219752754296894559, 0.3333333333333333703, 0.3219752754296894559, 0.3333333333333333703, 0.3219752754296894559, 0.3333333333333333703, 0.3219752754296894559, 0.3333333333333333703, 0.3219752754296894559, 0.3333333333333333703, 0.3219752754296894559, 0.3333333333333333703, 0.3219752754296894559, 0.3333333333333333703, 0.3219752754296894559, 0.3333333333333333703, 0.3219752754296894559, 0.3333333333333333703, 0.3219752754296894559, 0.3333333333333333703, 0.3219752754296894559, 0.3333333333333333703, 0.3219752754296894559, 0.3333333333333333703, 0.3219752754296894559, 0.3333333333333333703, 0.3219752754296894559, 0.3333333333333333703, 0.3219752754296894559, 0.3333333333333333703, 0.3219752754296894559, 0.3333333333333333703, 0.3219752754296894559, 0.3333333333333333703, 0.3219752754296894559, 0.3333333333333333703, 0.3219752754296894559, 0.3333333333333333703, 0.3219752754296894559, 0.3333333333333333703, 0.3219752754296894559, 0.3333333333333333703, 0.3219752754296894559, 0.3333333333333333703, 0.3219752754296894559, 0.3333333333333333703, 0.3219752754296894559, 0.3333333333333333703, 0.3219752754296894559, 0.3333333333333333703, 0.3219752754296894559, 0.3333333333333333703, 0.3219752754296894559, 0.3333333333333333703, 0.3219752754296894559, 0.3333333333333333703, 0.3219752754296894559, 0.3333333333333333703, 0.3219752754296894559, 0.3333333333333333703, 0.3219752754296894559, 0.3333333333333333703, 0.3219752754296894559, 0.3333333333333333703, 0.3219752754296894559, 0.3333333333333333703, 0.3219752754296894559, 0.3333333333333333703, 0.3219752754296894559, 0.3333333333333333703, 0.3219752754296894559, 0.3333333333333333703, 0.3219752754296894559, 0.3333333333333333703, 0.3219752754296894559, 0.3333333333333333703, 0.3219752754296894559, 0.3333333333333333703, 0.3219752754296894559, 0.3333333333333333703, 0.3219752754296894559, 0.3333333333333333703, 0.3219752754296894559, 0.3333333333333333703, 0.3219752754296894559, 0.3333333333333333703, 0.3219752754296894559, 0.3333333333333333703, 0.3219752754296894559, 0.3333333333333333703, 0.3219752754296894559, 0.3333333333333333703, 0.3219752754296894559, 0.3333333333333333703, 0.3219752754296894559, 0.3333333333333333703, 0.3219752754296894559, 0.3333333333333333703, 0.3219752754296894559, 0.3333333333333333703, 0.3219752754296894559, 0.3333333333333333703, 0.3219752754296894559, 0.3333333333333333703, 0.3219752754296894559, 0.3333333333333333703, 0.3219752754296894559, 0.3333333333333333703, 0.3219752754296894559, 0.3333333333333333703, 0.3219752754296894559, 0.3333333333333333703, 0.3219752754296894559, 0.3333333333333333703, 0.3219752754296894559, 0.3333333333333333703, 0.3219752754296894559, 0.3333333333333333703, 0.3219752754296894559, 0.3333333333333333703, 0.3219752754296894559, 0.3333333333333333703, 0.3219752754296894559, 0.3333333333333333703, 0.3219752754296894559, 0.3333333333333333703, 0.3219752754296894559, 0.3333333333333333703, 0.3219752754296894559, 0.3333333333333333703, 0.3219752754296894559, 0.3333333333333333703, 0.3219752754296894559, 0.3333333333333333703, 0.3219752754296894559, 0.3333333333333333703, 0.3219752754296894559, 0.3333333333333333703, 0.3219752754296894559, 0.3333333333333333703, 0.3219752754296894559, 0.3333333333333333703, 0.3219752754296894559, 0.3333333333333333703, 0.3219752754296894559, 0.3333333333333333703, 0.3219752754296894559, 0.3333333333333333703, 0.3219752754296894559, 0.3333333333333333703, 0.3219752754296894559, 0.3333333333333333703, 0.3219752754296894559, 0.3333333333333333703, 0.3219752754296894559, 0.3333333333333333703, 0.3219752754296894559, 0.3333333333333333703, 0.3219752754296894559, 0.3333333333333333703, 0.3219752754296894559, 0.3333333333333333703, 0.3219752754296894559, 0.3333333333333333703, 0.3219752754296894559, 0.3333333333333333703, 0.3219752754296894559, 0.3333333333333333703, 0.3219752754296894559, 0.3333333333333333703, 0.3219752754296894559, 0.3333333333333333703, 0.3219752754296894559, 0.3333333333333333703, 0.3219752754296894559, 0.3333333333333333703, 0.3219752754296894559, 0.3333333333333333703, 0.3219752754296894559, 0.3333333333333333703, 0.3219752754296894559, 0.3333333333333333703, 0.3219752754296894559, 0.3333333333333333703, 0.3219752754296894559, 0.3333333333333333703, 0.3219752754296894559, 0.3333333333333333703, 0.3219752754296894559, 0.3333333333333333703, 0.3219752754296894559, 0.3333333333333333703, 0.3219752754296894559, 0.3333333333333333703, 0.3219752754296894559, 0.3333333333333333703, 0.3219752754296894559, 0.3333333333333333703, 0.3219752754296894559, 0.3333333333333333703, 0.3219752754296894559, 0.3333333333333333703, 0.3219752754296894559, 0.3333333333333333703, 0.3219752754296894559, 0.3333333333333333703, 0.3219752754296894559, 0.3333333333333333703, 0.3219752754296894559, 0.3333333333333333703, 0.3219752754296894559, 0.3333333333333333703, 0.3219752754296894559, 0.3333333333333333703, 0.3219752754296894559, 0.3333333333333333703, 0.3219752754296894559, 0.3333333333333333703, 0.3219752754296894559, 0.3333333333333333703, 0.3219752754296894559, 0.3333333333333333703),
 ( 1.000000000000000000, 0.9659258262890683122, 1.000000000000000000, 0.9659258262890683122, 1.000000000000000000, 0.9659258262890683122, 1.000000000000000000, 0.9659258262890683122, 1.000000000000000000, 0.9659258262890683122, 1.000000000000000000, 0.9659258262890683122, 1.000000000000000000, 0.9659258262890683122, 1.000000000000000000, 0.9659258262890683122, 1.000000000000000000, 0.9659258262890683122, 1.000000000000000000, 0.9659258262890683122, 1.000000000000000000, 0.9659258262890683122, 1.000000000000000000, 0.9659258262890683122, 1.000000000000000000, 0.9659258262890683122, 1.000000000000000000, 0.9659258262890683122, 1.000000000000000000, 0.9659258262890683122, 1.000000000000000000, 0.9659258262890683122, 1.000000000000000000, 0.9659258262890683122, 1.000000000000000000, 0.9659258262890683122, 1.000000000000000000, 0.9659258262890683122, 1.000000000000000000, 0.9659258262890683122, 1.000000000000000000, 0.9659258262890683122, 1.000000000000000000, 0.9659258262890683122, 1.000000000000000000, 0.9659258262890683122, 1.000000000000000000, 0.9659258262890683122, 1.000000000000000000, 0.9659258262890683122, 1.000000000000000000, 0.9659258262890683122, 1.000000000000000000, 0.9659258262890683122, 1.000000000000000000, 0.9659258262890683122, 1.000000000000000000, 0.9659258262890683122, 1.000000000000000000, 0.9659258262890683122, 1.000000000000000000, 0.9659258262890683122, 1.000000000000000000, 0.9659258262890683122, 1.000000000000000000, 0.9659258262890683122, 1.000000000000000000, 0.9659258262890683122, 1.000000000000000000, 0.9659258262890683122, 1.000000000000000000, 0.9659258262890683122, 1.000000000000000000, 0.9659258262890683122, 1.000000000000000000, 0.9659258262890683122, 1.000000000000000000, 0.9659258262890683122, 1.000000000000000000, 0.9659258262890683122, 1.000000000000000000, 0.9659258262890683122, 1.000000000000000000, 0.9659258262890683122, 1.000000000000000000, 0.9659258262890683122, 1.000000000000000000, 0.9659258262890683122, 1.000000000000000000, 0.9659258262890683122, 1.000000000000000000, 0.9659258262890683122, 1.000000000000000000, 0.9659258262890683122, 1.000000000000000000, 0.9659258262890683122, 1.000000000000000000, 0.9659258262890683122, 1.000000000000000000, 0.9659258262890683122, 1.000000000000000000, 0.9659258262890683122, 1.000000000000000000, 0.9659258262890683122, 1.000000000000000000, 0.9659258262890683122, 1.000000000000000000, 0.9659258262890683122, 1.000000000000000000, 0.9659258262890683122, 1.000000000000000000, 0.9659258262890683122, 1.000000000000000000, 0.9659258262890683122, 1.000000000000000000, 0.9659258262890683122, 1.000000000000000000, 0.9659258262890683122, 1.000000000000000000, 0.9659258262890683122, 1.000000000000000000, 0.9659258262890683122, 1.000000000000000000, 0.9659258262890683122, 1.000000000000000000, 0.9659258262890683122, 1.000000000000000000, 0.9659258262890683122, 1.000000000000000000, 0.9659258262890683122, 1.000000000000000000, 0.9659258262890683122, 1.000000000000000000, 0.9659258262890683122, 1.000000000000000000, 0.9659258262890683122, 1.000000000000000000, 0.9659258262890683122, 1.000000000000000000, 0.9659258262890683122, 1.000000000000000000, 0.9659258262890683122, 1.000000000000000000, 0.9659258262890683122, 1.000000000000000000, 0.9659258262890683122, 1.000000000000000000, 0.9659258262890683122, 1.000000000000000000, 0.9659258262890683122, 1.000000000000000000, 0.9659258262890683122, 1.000000000000000000, 0.9659258262890683122, 1.000000000000000000, 0.9659258262890683122, 1.000000000000000000, 0.9659258262890683122, 1.000000000000000000, 0.9659258262890683122, 1.000000000000000000, 0.9659258262890683122, 1.000000000000000000, 0.9659258262890683122, 1.000000000000000000, 0.9659258262890683122, 1.000000000000000000, 0.9659258262890683122, 1.000000000000000000, 0.9659258262890683122, 1.000000000000000000, 0.9659258262890683122, 1.000000000000000000, 0.9659258262890683122, 1.000000000000000000, 0.9659258262890683122, 1.000000000000000000, 0.9659258262890683122, 1.000000000000000000, 0.9659258262890683122, 1.000000000000000000, 0.9659258262890683122, 1.000000000000000000, 0.9659258262890683122, 1.000000000000000000, 0.9659258262890683122, 1.000000000000000000, 0.9659258262890683122, 1.000000000000000000, 0.9659258262890683122, 1.000000000000000000, 0.9659258262890683122, 1.000000000000000000, 0.9659258262890683122, 1.000000000000000000, 0.9659258262890683122, 1.000000000000000000, 0.9659258262890683122, 1.000000000000000000, 0.9659258262890683122, 1.000000000000000000, 0.9659258262890683122, 1.000000000000000000, 0.9659258262890683122, 1.000000000000000000, 0.9659258262890683122, 1.000000000000000000, 0.9659258262890683122, 1.000000000000000000, 0.9659258262890683122, 1.000000000000000000, 0.9659258262890683122, 1.000000000000000000, 0.9659258262890683122, 1.000000000000000000, 0.9659258262890683122, 1.000000000000000000, 0.9659258262890683122, 1.000000000000000000, 0.9659258262890683122, 1.000000000000000000, 0.9659258262890683122, 1.000000000000000000, 0.9659258262890683122, 1.000000000000000000, 0.9659258262890683122, 1.000000000000000000, 0.9659258262890683122, 1.000000000000000000, 0.9659258262890683122, 1.000000000000000000, 0.9659258262890683122, 1.000000000000000000, 0.9659258262890683122, 1.000000000000000000, 0.9659258262890683122, 1.000000000000000000, 0.9659258262890683122, 1.000000000000000000, 0.9659258262890683122, 1.000000000000000000, 0.9659258262890683122, 1.000000000000000000, 0.9659258262890683122, 1.000000000000000000, 0.9659258262890683122, 1.000000000000000000, 0.9659258262890683122, 1.000000000000000000, 0.9659258262890683122, 1.000000000000000000, 0.9659258262890683122, 1.000000000000000000, 0.9659258262890683122, 1.000000000000000000, 0.9659258262890683122, 1.000000000000000000, 0.9659258262890683122, 1.000000000000000000, 0.9659258262890683122, 1.000000000000000000, 0.9659258262890683122, 1.000000000000000000, 0.9659258262890683122, 1.000000000000000000, 0.9659258262890683122, 1.000000000000000000, 0.9659258262890683122, 1.000000000000000000, 0.9659258262890683122, 1.000000000000000000, 0.9659258262890683122, 1.000000000000000000, 0.9659258262890683122, 1.000000000000000000, 0.9659258262890683122, 1.000000000000000000, 0.9659258262890683122, 1.000000000000000000, 0.9659258262890683122, 1.000000000000000000, 0.9659258262890683122, 1.000000000000000000, 0.9659258262890683122, 1.000000000000000000, 0.9659258262890683122, 1.000000000000000000, 0.9659258262890683122, 1.000000000000000000, 0.9659258262890683122, 1.000000000000000000, 0.9659258262890683122, 1.000000000000000000, 0.9659258262890683122, 1.000000000000000000, 0.9659258262890683122, 1.000000000000000000, 0.9659258262890683122, 1.000000000000000000, 0.9659258262890683122, 1.000000000000000000, 0.9659258262890683122, 1.000000000000000000, 0.9659258262890683122, 1.000000000000000000, 0.9659258262890683122, 1.000000000000000000, 0.9659258262890683122, 1.000000000000000000, 0.9659258262890683122, 1.000000000000000000, 0.9659258262890683122, 1.000000000000000000, 0.9659258262890683122, 1.000000000000000000, 0.9659258262890683122, 1.000000000000000000, 0.9659258262890683122, 1.000000000000000000, 0.9659258262890683122, 1.000000000000000000, 0.9659258262890683122, 1.000000000000000000, 0.9659258262890683122, 1.000000000000000000, 0.9659258262890683122, 1.000000000000000000, 0.9659258262890683122, 1.000000000000000000, 0.9659258262890683122, 1.000000000000000000, 0.9659258262890683122, 1.000000000000000000, 0.9659258262890683122, 1.000000000000000000, 0.9659258262890683122, 1.000000000000000000, 0.9659258262890683122, 1.000000000000000000, 0.9659258262890683122, 1.000000000000000000, 0.9659258262890683122, 1.000000000000000000, 0.9659258262890683122, 1.000000000000000000, 0.9659258262890683122, 1.000000000000000000, 0.9659258262890683122, 1.000000000000000000, 0.9659258262890683122, 1.000000000000000000, 0.9659258262890683122, 1.000000000000000000, 0.9659258262890683122, 1.000000000000000000, 0.9659258262890683122, 1.000000000000000000, 0.9659258262890683122, 1.000000000000000000, 0.9659258262890683122, 1.000000000000000000, 0.9659258262890683122, 1.000000000000000000, 0.9659258262890683122, 1.000000000000000000, 0.9659258262890683122, 1.000000000000000000, 0.9659258262890683122, 1.000000000000000000, 0.9659258262890683122, 1.000000000000000000, 0.9659258262890683122, 1.000000000000000000, 0.9659258262890683122, 1.000000000000000000, 0.9659258262890683122, 1.000000000000000000, 0.9659258262890683122, 1.000000000000000000, 0.9659258262890683122, 1.000000000000000000, 0.9659258262890683122, 1.000000000000000000, 0.9659258262890683122, 1.000000000000000000, 0.9659258262890683122, 1.000000000000000000, 0.9659258262890683122, 1.000000000000000000, 0.9659258262890683122, 1.000000000000000000, 0.9659258262890683122, 1.000000000000000000, 0.9659258262890683122, 1.000000000000000000, 0.9659258262890683122, 1.000000000000000000, 0.9659258262890683122, 1.000000000000000000, 0.9659258262890683122, 1.000000000000000000, 0.9659258262890683122, 1.000000000000000000, 0.9659258262890683122, 1.000000000000000000, 0.9659258262890683122, 1.000000000000000000, 0.9659258262890683122, 1.000000000000000000, 0.9659258262890683122, 1.000000000000000000, 0.9659258262890683122, 1.000000000000000000, 0.9659258262890683122, 1.000000000000000000, 0.9659258262890683122, 1.000000000000000000, 0.9659258262890683122, 1.000000000000000000, 0.9659258262890683122, 1.000000000000000000, 0.9659258262890683122, 1.000000000000000000, 0.9659258262890683122, 1.000000000000000000, 0.9659258262890683122, 1.000000000000000000, 0.9659258262890683122, 1.000000000000000000, 0.9659258262890683122, 1.000000000000000000, 0.9659258262890683122, 1.000000000000000000, 0.9659258262890683122, 1.000000000000000000, 0.9659258262890683122, 1.000000000000000000, 0.9659258262890683122, 1.000000000000000000, 0.9659258262890683122, 1.000000000000000000, 0.9659258262890683122, 1.000000000000000000, 0.9659258262890683122, 1.000000000000000000, 0.9659258262890683122, 1.000000000000000000, 0.9659258262890683122, 1.000000000000000000, 0.9659258262890683122, 1.000000000000000000, 0.9659258262890683122, 1.000000000000000000, 0.9659258262890683122, 1.000000000000000000, 0.9659258262890683122, 1.000000000000000000) ) ) 
 REPRESENTATION_ITEM ( '' )  SURFACE ( )  );
#894=CARTESIAN_POINT ( 'NONE',  ( 5.049401038298161559, -19.05341960407611168, 62.70724293864769550 ) ) ;
#895=CARTESIAN_POINT ( 'NONE',  ( 21.52544592524334988, 5.823673210054432836, 66.45942372801903275 ) ) ;
#896=CARTESIAN_POINT ( 'NONE',  ( 13.89961937509977652, -13.97604488694527269, 53.12390960531434558 ) ) ;
#897=CARTESIAN_POINT ( 'NONE',  ( 19.03943276465977164, -0.05219959533909143690, 28.74890960531435624 ) ) ;
#898=CARTESIAN_POINT ( 'NONE',  ( 9.564922557960805705, 16.46253265017160317, 114.5822429386476955 ) ) ;
#899=CARTESIAN_POINT ( 'NONE',  ( -4.379528057220328563, 16.55341960407611168, 65.20724293864768129 ) ) ;
#900=CARTESIAN_POINT ( 'NONE',  ( 19.05341960407611168, 5.049401038298154454, 23.95724293864769194 ) ) ;
#901=CARTESIAN_POINT ( 'NONE',  ( -8.314922557960811034, -14.29746914071050412, 87.08224293864769550 ) ) ;
#902=CARTESIAN_POINT ( 'NONE',  ( -21.55341960407610458, -5.719274019375992779, 101.4572429386476955 ) ) ;
#903=CARTESIAN_POINT ( 'NONE',  ( 5.719274019375673035, 21.55341960407619339, 37.29275706135235424 ) ) ;
#905=CARTESIAN_POINT ( 'NONE',  ( 16.53943276465976808, 0.05219959533934440121, 46.25109039468567573 ) ) ;
#906=CARTESIAN_POINT ( 'NONE',  ( 18.62759615963271287, -10.81492255796078972, 98.33224293864769550 ) ) ;
#907=CARTESIAN_POINT ( 'NONE',  ( 9.564922557961047289, -16.46253265017146816, 30.41775706135232937 ) ) ;
#908=CARTESIAN_POINT ( 'NONE',  ( 5.049401038298161559, -19.05341960407611168, 112.7072429386476813 ) ) ;
#909=CARTESIAN_POINT ( 'NONE',  ( -5.719274019375665041, -21.55341960407619695, 44.79275706135234714 ) ) ;
#911=CARTESIAN_POINT ( 'NONE',  ( -10.72451020669898014, 18.67979575497178502, 40.41557627198103120 ) ) ;
#912=CARTESIAN_POINT ( 'NONE',  ( -12.14591786802309592, -12.06949235617757132, 21.87390960531436690 ) ) ;
#913=CARTESIAN_POINT ( 'NONE',  ( 21.53943276465977519, 0.05219959533937863772, 61.25109039468567573 ) ) ;
#914=CARTESIAN_POINT ( 'NONE',  ( 18.62759615963255655, 10.81492255796105972, 96.66775706135234714 ) ) ;
#915=CARTESIAN_POINT ( 'NONE',  ( 0.05219959533936267826, -19.03943276465977164, 25.00109039468566152 ) ) ;
#916=CARTESIAN_POINT ( 'NONE',  ( -14.34966873604972548, 8.224510206698743886, 83.33442372801903275 ) ) ;
#917=CARTESIAN_POINT ( 'NONE',  ( 0.05219959533937995610, -21.53943276465977519, 50.00109039468568994 ) ) ;
#918=CARTESIAN_POINT ( 'NONE',  ( -19.03943276465977164, 0.05219959533909376836, 46.24890960531435979 ) ) ;
#919=CARTESIAN_POINT ( 'NONE',  ( -19.03943276465977164, -0.05219959533935918106, 23.75109039468566152 ) ) ;
#920=CARTESIAN_POINT ( 'NONE',  ( -0.05219959533907301413, -21.53943276465977519, 27.49890960531435269 ) ) ;
#921=CARTESIAN_POINT ( 'NONE',  ( 10.81492255796078972, 18.62759615963270932, 114.5822429386477097 ) ) ;
#922=CARTESIAN_POINT ( 'NONE',  ( -5.823673210054116645, -21.52544592524344225, 72.29057627198102409 ) ) ;
#923=CARTESIAN_POINT ( 'NONE',  ( -8.224510206698735004, -14.34966873604973081, 39.58442372801901143 ) ) ;
#925=CARTESIAN_POINT ( 'NONE',  ( 18.67979575497178502, 10.72451020669898547, 74.16557627198102409 ) ) ;
#926=CARTESIAN_POINT ( 'NONE',  ( -16.53943276465976808, -0.05219959533934237506, 68.75109039468568994 ) ) ;
#927=CARTESIAN_POINT ( 'NONE',  ( -4.483927247898539470, -16.52544592524342804, 57.29057627198103120 ) ) ;
#929=CARTESIAN_POINT ( 'NONE',  ( 19.05341960407617918, -5.049401038297876454, 106.0427570613523471 ) ) ;
#931=CARTESIAN_POINT ( 'NONE',  ( 4.483927247898790824, -16.52544592524335698, 45.20942372801901854 ) ) ;
#932=CARTESIAN_POINT ( 'NONE',  ( -21.53943276465977519, 0.05219959533907696930, 106.2489096053143811 ) ) ;
#933=CARTESIAN_POINT ( 'NONE',  ( 10.81492255796078972, 18.62759615963270932, 29.58224293864769905 ) ) ;
#934=CARTESIAN_POINT ( 'NONE',  ( 16.55341960407618274, -4.379528057220086978, 51.04275706135234714 ) ) ;
#935=CARTESIAN_POINT ( 'NONE',  ( -16.51473224551069308, -9.474510206698971260, 71.66557627198102409 ) ) ;
#936=CARTESIAN_POINT ( 'NONE',  ( -0.05219959533937732626, 21.53943276465977519, 42.50109039468567573 ) ) ;
#937=CARTESIAN_POINT ( 'NONE',  ( -19.05341960407617563, 5.049401038297882671, 113.5427570613523471 ) ) ;
#938=CARTESIAN_POINT ( 'NONE',  ( -0.05219959533907301413, -21.53943276465977519, 22.49890960531436335 ) ) ;
#939=CARTESIAN_POINT ( 'NONE',  ( -19.02544592524334988, -5.153800228976617603, 23.95942372801900078 ) ) ;
#940=CARTESIAN_POINT ( 'NONE',  ( 4.483927247898790824, -16.52544592524335698, 40.20942372801901854 ) ) ;
#941=CARTESIAN_POINT ( 'NONE',  ( -9.564922557960796823, -16.46253265017161027, 107.0822429386476955 ) ) ;
#942=CARTESIAN_POINT ( 'NONE',  ( 21.53943276465977519, -0.05219959533907433946, 98.74890960531438111 ) ) ;
#943=CARTESIAN_POINT ( 'NONE',  ( -9.474510206698964154, 16.51473224551069663, 70.41557627198102409 ) ) ;
#944=CARTESIAN_POINT ( 'NONE',  ( -17.48847506799967988, 5.747544572773784388, 25.82697437843280497 ) ) ;
#945=CARTESIAN_POINT ( 'NONE',  ( 16.53943276465976808, -0.05219959533910856209, 78.74890960531436690 ) ) ;
#946=CARTESIAN_POINT ( 'NONE',  ( -16.51473224551069308, -9.474510206698971260, 111.6655762719810383 ) ) ;
#948=CARTESIAN_POINT ( 'NONE',  ( 0.05219959533934541429, -16.53943276465976808, 70.00109039468568994 ) ) ;
#949=CARTESIAN_POINT ( 'NONE',  ( 15.80617190586746368, 15.72974639402197994, 99.37390960531436690 ) ) ;
#950=CARTESIAN_POINT ( 'NONE',  ( 5.049401038297881783, 19.05341960407617563, 67.29275706135234714 ) ) ;
#951=CARTESIAN_POINT ( 'NONE',  ( -15.80617190586745835, -15.72974639402198527, 26.87390960531435979 ) ) ;
#952=CARTESIAN_POINT ( 'NONE',  ( 9.564922557960805705, 16.46253265017160317, 29.58224293864769550 ) ) ;
#953=CARTESIAN_POINT ( 'NONE',  ( 15.80617190586746368, 15.72974639402197994, 74.37390960531436690 ) ) ;
#954=CARTESIAN_POINT ( 'NONE',  ( 5.049401038298161559, -19.05341960407611168, 102.7072429386476955 ) ) ;
#956=CARTESIAN_POINT ( 'NONE',  ( -18.67979575497193778, 10.72451020669871902, 93.33442372801901854 ) ) ;
#957=CARTESIAN_POINT ( 'NONE',  ( -0.05219959533909027116, -19.03943276465977164, 52.49890960531436690 ) ) ;
#958=CARTESIAN_POINT ( 'NONE',  ( -4.483927247898539470, -16.52544592524342804, 92.29057627198103830 ) ) ;
#959=CARTESIAN_POINT ( 'NONE',  ( 14.29746914071037800, 8.314922557961029526, 41.66775706135235424 ) ) ;
#960=CARTESIAN_POINT ( 'NONE',  ( -5.049401038298153566, 19.05341960407611168, 60.20724293864768129 ) ) ;
#961=CARTESIAN_POINT ( 'NONE',  ( 0.05219959533937995610, -21.53943276465977519, 80.00109039468568994 ) ) ;
#963=CARTESIAN_POINT ( 'NONE',  ( -19.02544592524334988, -5.153800228976617603, 38.95942372801900433 ) ) ;
#964=CARTESIAN_POINT ( 'NONE',  ( 19.03943276465977164, 0.05219959533936151252, 41.25109039468566152 ) ) ;
#965=CARTESIAN_POINT ( 'NONE',  ( 18.62759615963255655, 10.81492255796105972, 31.66775706135234358 ) ) ;
#967=CARTESIAN_POINT ( 'NONE',  ( 16.51473224551083163, -9.474510206698727899, 35.83442372801899722 ) ) ;
#968=CARTESIAN_POINT ( 'NONE',  ( -13.97604488694527625, -13.89961937509977652, 81.87390960531436690 ) ) ;
#969=CARTESIAN_POINT ( 'NONE',  ( 5.153800228976335163, 19.02544592524342804, 74.79057627198103830 ) ) ;
#970=CARTESIAN_POINT ( 'NONE',  ( -8.224510206698948167, 14.34966873604960824, 30.41557627198101699 ) ) ;
#971=CARTESIAN_POINT ( 'NONE',  ( -16.46253265017160317, 9.564922557960807481, 110.8322429386476955 ) ) ;
#972=CARTESIAN_POINT ( 'NONE',  ( -15.80617190586768217, 15.72974639402176855, 83.12609039468568994 ) ) ;
#975=CARTESIAN_POINT ( 'NONE',  ( 0.05219959533937995610, -21.53943276465977519, 100.0010903946857042 ) ) ;
#976=CARTESIAN_POINT ( 'NONE',  ( 17.40805194822031154, -6.112264579159331745, 43.33371272510611760 ) ) ;
#977=CARTESIAN_POINT ( 'NONE',  ( 13.97604488694527802, 13.89961937509977652, 114.3739096053143669 ) ) ;
#979=CARTESIAN_POINT ( 'NONE',  ( 14.34966873604972726, -8.224510206698740333, 50.83442372801901143 ) ) ;
#980=CARTESIAN_POINT ( 'NONE',  ( -15.72974639402197994, 15.80617190586746368, 75.62390960531439532 ) ) ;
#982=CARTESIAN_POINT ( 'NONE',  ( 8.314922557960818139, 14.29746914071049879, 29.58224293864769905 ) ) ;
#983=CARTESIAN_POINT ( 'NONE',  ( 4.483927247898545687, 16.52544592524342804, 114.7905762719810383 ) ) ;
#984=CARTESIAN_POINT ( 'NONE',  ( 9.564922557960805705, 16.46253265017160317, 99.58224293864770971 ) ) ;
#985=CARTESIAN_POINT ( 'NONE',  ( 19.03943276465977164, 0.05219959533936151252, 26.25109039468566507 ) ) ;
#986=CARTESIAN_POINT ( 'NONE',  ( 9.564922557960805705, 16.46253265017160317, 24.58224293864769194 ) ) ;
#987=CARTESIAN_POINT ( 'NONE',  ( -5.719274019375665041, -21.55341960407619695, 64.79275706135234714 ) ) ;
#988=CARTESIAN_POINT ( 'NONE',  ( -16.46253265017160317, 9.564922557960807481, 110.8322429386476955 ) ) ;
#989=CARTESIAN_POINT ( 'NONE',  ( -8.314922557961024197, 14.29746914071037800, 107.9177570613523471 ) ) ;
#990=CARTESIAN_POINT ( 'NONE',  ( 9.564922557961047289, -16.46253265017146816, 65.41775706135233293 ) ) ;
#992=CARTESIAN_POINT ( 'NONE',  ( -19.05341960407611168, -5.049401038298163336, 106.4572429386476955 ) ) ;
#993=CARTESIAN_POINT ( 'NONE',  ( 16.55341960407611168, 4.379528057220329451, 93.95724293864770971 ) ) ;
#994=CARTESIAN_POINT ( 'NONE',  ( 19.02544592524334988, 5.153800228976608722, 61.45942372801900433 ) ) ;
#995=CARTESIAN_POINT ( 'NONE',  ( 13.89961937509977652, -13.97604488694527269, 83.12390960531436690 ) ) ;
#996=CARTESIAN_POINT ( 'NONE',  ( -12.14591786802309592, -12.06949235617757132, 66.87390960531436690 ) ) ;
#997=CARTESIAN_POINT ( 'NONE',  ( 9.474510206698729675, 16.51473224551082808, 97.08442372801900433 ) ) ;
#998=CARTESIAN_POINT ( 'NONE',  ( -5.719274019375978568, 21.55341960407610458, 55.20724293864770260 ) ) ;
#1000=CARTESIAN_POINT ( 'NONE',  ( -13.89961937509977652, 13.97604488694528158, 25.62390960531434558 ) ) ;
#1001=CARTESIAN_POINT ( 'NONE',  ( -9.474510206698720793, -16.51473224551083518, 99.58442372801900433 ) ) ;
#1002=CARTESIAN_POINT ( 'NONE',  ( -19.03943276465977164, 0.05219959533909376836, 71.24890960531435269 ) ) ;
#1003=CARTESIAN_POINT ( 'NONE',  ( -18.67979575497178146, -10.72451020669898902, 81.66557627198103830 ) ) ;
#1004=CARTESIAN_POINT ( 'NONE',  ( 4.379528057220092307, 16.55341960407617563, 92.29275706135236135 ) ) ;
#1005=CARTESIAN_POINT ( 'NONE',  ( 9.474510206698971260, -16.51473224551069308, 67.91557627198102409 ) ) ;
#1006=CARTESIAN_POINT ( 'NONE',  ( -0.05219959533936034679, 19.03943276465977164, 67.50109039468566152 ) ) ;
#1007=CARTESIAN_POINT ( 'NONE',  ( 5.823673210054444382, -21.52544592524334988, 75.20942372801901854 ) ) ;
#1008=CARTESIAN_POINT ( 'NONE',  ( -15.80617190586745835, -15.72974639402198527, 66.87390960531436690 ) ) ;
#1009=CARTESIAN_POINT ( 'NONE',  ( 15.72974639402199770, -15.80617190586745480, 23.12390960531436335 ) ) ;
#1010=CARTESIAN_POINT ( 'NONE',  ( -5.153800228976328057, -19.02544592524343514, 42.29057627198101699 ) ) ;
#1011=CARTESIAN_POINT ( 'NONE',  ( 0.05219959533934541429, -16.53943276465976808, 105.0010903946856757 ) ) ;
#1012=CARTESIAN_POINT ( 'NONE',  ( 0.05219959533909260263, 19.03943276465977164, 54.99890960531435979 ) ) ;
#1013=CARTESIAN_POINT ( 'NONE',  ( 16.53943276465976808, 0.05219959533934440121, 21.25109039468567218 ) ) ;
#1015=CARTESIAN_POINT ( 'NONE',  ( -21.52544592524334988, -5.823673210054445271, 108.9594237280190185 ) ) ;
#1016=CARTESIAN_POINT ( 'NONE',  ( 12.14591786802309770, 12.06949235617756955, 59.37390960531436690 ) ) ;
#1018=CARTESIAN_POINT ( 'NONE',  ( -10.72451020669898014, 18.67979575497178502, 100.4155762719810241 ) ) ;
#1019=CARTESIAN_POINT ( 'NONE',  ( -15.80617190586745835, -15.72974639402198527, 106.8739096053143811 ) ) ;
#1020=CARTESIAN_POINT ( 'NONE',  ( 17.48853670773245383, -5.747243402303092275, 96.16671299749991420 ) ) ;
#1021=CARTESIAN_POINT ( 'NONE',  ( -10.72451020669898014, 18.67979575497178502, 50.41557627198103120 ) ) ;
#1022=CARTESIAN_POINT ( 'NONE',  ( 14.29746914071037800, 8.314922557961029526, 76.66775706135234714 ) ) ;
#1023=CARTESIAN_POINT ( 'NONE',  ( -14.29746914071049879, 8.314922557960819915, 85.83224293864768129 ) ) ;
#1024=CARTESIAN_POINT ( 'NONE',  ( -19.02544592524342804, 5.153800228976336051, 46.04057627198101699 ) ) ;
#1027=CARTESIAN_POINT ( 'NONE',  ( 4.379528057220339221, -16.55341960407611168, 22.70724293864769194 ) ) ;
#1028=CARTESIAN_POINT ( 'NONE',  ( -0.05219959533937732626, 21.53943276465977519, 27.50109039468567929 ) ) ;
#1029=CARTESIAN_POINT ( 'NONE',  ( -13.97604488694527625, -13.89961937509977652, 91.87390960531432427 ) ) ;
#1030=CARTESIAN_POINT ( 'NONE',  ( 10.72451020669871369, 18.67979575497193778, 62.08442372801901143 ) ) ;
#1032=CARTESIAN_POINT ( 'NONE',  ( 9.564922557960805705, 16.46253265017160317, 29.58224293864769550 ) ) ;
#1034=CARTESIAN_POINT ( 'NONE',  ( 18.67979575497194134, -10.72451020669871369, 60.83442372801901854 ) ) ;
#1035=CARTESIAN_POINT ( 'NONE',  ( -19.02544592524342804, 5.153800228976336051, 56.04057627198100988 ) ) ;
#1036=CARTESIAN_POINT ( 'NONE',  ( -19.05341960407611168, -5.049401038298163336, 111.4572429386476671 ) ) ;
#1037=CARTESIAN_POINT ( 'NONE',  ( 16.46253265017160672, -9.564922557960803928, 93.33224293864769550 ) ) ;
#1038=CARTESIAN_POINT ( 'NONE',  ( -19.02544592524334988, -5.153800228976617603, 68.95942372801896170 ) ) ;
#1039=CARTESIAN_POINT ( 'NONE',  ( -10.72451020669870658, -18.67979575497194134, 39.58442372801901143 ) ) ;
#1040=CARTESIAN_POINT ( 'NONE',  ( -13.97604488694547697, 13.89961937509957934, 103.1260903946856473 ) ) ;
#1041=CARTESIAN_POINT ( 'NONE',  ( -19.02544592524334988, -5.153800228976617603, 78.95942372801900433 ) ) ;
#1042=CARTESIAN_POINT ( 'NONE',  ( 19.03943276465977164, -0.05219959533909143690, 43.74890960531435979 ) ) ;
#1043=CARTESIAN_POINT ( 'NONE',  ( -16.52544592524335698, -4.483927247898792601, 103.9594237280190185 ) ) ;
#1044=CARTESIAN_POINT ( 'NONE',  ( 9.564922557961047289, -16.46253265017146816, 70.41775706135233293 ) ) ;
#1045=CARTESIAN_POINT ( 'NONE',  ( -14.29746914071049879, 8.314922557960819915, 25.83224293864769194 ) ) ;
#1046=CARTESIAN_POINT ( 'NONE',  ( 0.05219959533936267826, -19.03943276465977164, 45.00109039468566863 ) ) ;
#1047=CARTESIAN_POINT ( 'NONE',  ( 15.80617190586769283, -15.72974639402175789, 105.6260903946856899 ) ) ;
#1048=CARTESIAN_POINT ( 'NONE',  ( 16.51473224551083163, -9.474510206698727899, 30.83442372801900433 ) ) ;
#1049=CARTESIAN_POINT ( 'NONE',  ( -16.46253265017160317, 9.564922557960807481, 30.83224293864769550 ) ) ;
#1050=CARTESIAN_POINT ( 'NONE',  ( -21.55341960407619339, 5.719274019375674811, 93.54275706135234714 ) ) ;
#1051=CARTESIAN_POINT ( 'NONE',  ( 14.29746914071037800, 8.314922557961029526, 26.66775706135235424 ) ) ;
#1052=CARTESIAN_POINT ( 'NONE',  ( -5.153800228976328057, -19.02544592524343514, 87.29057627198103830 ) ) ;
#1053=AXIS2_PLACEMENT_3D ( 'NONE', #11334, #147844, #73005 ) ;
#1055=CARTESIAN_POINT ( 'NONE',  ( 19.05341960407611168, 5.049401038298154454, 83.95724293864766707 ) ) ;
#1056=CARTESIAN_POINT ( 'NONE',  ( -17.05587630539706367, 6.762274262136686254, 100.7418030903728408 ) ) ;
#1057=CARTESIAN_POINT ( 'NONE',  ( 13.89961937509957401, 13.97604488694547697, 81.87609039468564731 ) ) ;
#1058=CARTESIAN_POINT ( 'NONE',  ( -9.474510206698964154, 16.51473224551069663, 110.4155762719810383 ) ) ;
#1059=CARTESIAN_POINT ( 'NONE',  ( -18.67979575497193778, 10.72451020669871902, 98.33442372801901854 ) ) ;
#1060=CARTESIAN_POINT ( 'NONE',  ( 14.34966873604960469, 8.224510206698951720, 104.1655762719810241 ) ) ;
#1062=CARTESIAN_POINT ( 'NONE',  ( 0.05219959533907565091, 21.53943276465977519, 59.99890960531436690 ) ) ;
#1063=CARTESIAN_POINT ( 'NONE',  ( 10.72451020669898902, -18.67979575497178502, 42.91557627198103120 ) ) ;
#1064=CARTESIAN_POINT ( 'NONE',  ( -9.564922557960796823, -16.46253265017161027, 22.08224293864768839 ) ) ;
#1066=CARTESIAN_POINT ( 'NONE',  ( -16.46253265017146816, -9.564922557961047289, 54.16775706135234003 ) ) ;
#1067=CARTESIAN_POINT ( 'NONE',  ( -4.379528057220328563, 16.55341960407611168, 40.20724293864769550 ) ) ;
#1068=CARTESIAN_POINT ( 'NONE',  ( 5.719274019375991003, -21.55341960407610458, 22.70724293864769194 ) ) ;
#1069=CARTESIAN_POINT ( 'NONE',  ( -15.72974639402176322, -15.80617190586768395, 74.37609039468568994 ) ) ;
#1070=CARTESIAN_POINT ( 'NONE',  ( -10.81492255796078084, -18.62759615963271287, 72.08224293864769550 ) ) ;
#1071=CARTESIAN_POINT ( 'NONE',  ( -18.62759615963255300, -10.81492255796106328, 54.16775706135235424 ) ) ;
#1072=CARTESIAN_POINT ( 'NONE',  ( -5.823673210054116645, -21.52544592524344225, 97.29057627198105251 ) ) ;
#1073=CARTESIAN_POINT ( 'NONE',  ( -0.05219959533937732626, 21.53943276465977519, 52.50109039468567573 ) ) ;
#1074=CARTESIAN_POINT ( 'NONE',  ( -5.153800228976328057, -19.02544592524343514, 32.29057627198102409 ) ) ;
#1075=CARTESIAN_POINT ( 'NONE',  ( -13.97604488694527625, -13.89961937509977652, 76.87390960531433848 ) ) ;
#1076=CARTESIAN_POINT ( 'NONE',  ( 0.05219959533934541429, -16.53943276465976808, 85.00109039468568994 ) ) ;
#1077=CARTESIAN_POINT ( 'NONE',  ( 19.03943276465977164, -0.05219959533909143690, 28.74890960531435624 ) ) ;
#1079=CARTESIAN_POINT ( 'NONE',  ( -16.52544592524342804, 4.483927247898546575, 56.04057627198102409 ) ) ;
#1080=CARTESIAN_POINT ( 'NONE',  ( -12.14591786802326823, 12.06949235617739902, 108.1260903946856757 ) ) ;
#1081=CARTESIAN_POINT ( 'NONE',  ( -19.02544592524342804, 5.153800228976336051, 71.04057627198099567 ) ) ;
#1082=CARTESIAN_POINT ( 'NONE',  ( 19.02544592524343514, -5.153800228976328945, 38.54057627198103120 ) ) ;
#1083=CARTESIAN_POINT ( 'NONE',  ( 5.823673210054125526, 21.52544592524343514, 49.79057627198102409 ) ) ;
#1084=CARTESIAN_POINT ( 'NONE',  ( 9.474510206698729675, 16.51473224551082808, 42.08442372801900433 ) ) ;
#1086=CARTESIAN_POINT ( 'NONE',  ( 8.314922557960818139, 14.29746914071049879, 49.58224293864769550 ) ) ;
#1087=CARTESIAN_POINT ( 'NONE',  ( 5.823673210054125526, 21.52544592524343514, 29.79057627198102409 ) ) ;
#1089=CARTESIAN_POINT ( 'NONE',  ( -16.53943276465976808, -0.05219959533934237506, 68.75109039468568994 ) ) ;
#1090=CARTESIAN_POINT ( 'NONE',  ( -19.05341960407617563, 5.049401038297882671, 63.54275706135234003 ) ) ;
#1091=CARTESIAN_POINT ( 'NONE',  ( -16.55341960407611168, -4.379528057220339221, 36.45724293864768839 ) ) ;
#1093=CARTESIAN_POINT ( 'NONE',  ( -14.29746914071049879, 8.314922557960819915, 30.83224293864770260 ) ) ;
#1094=CARTESIAN_POINT ( 'NONE',  ( -16.46253265017160317, 9.564922557960807481, 40.83224293864769550 ) ) ;
#1095=CARTESIAN_POINT ( 'NONE',  ( 5.049401038298161559, -19.05341960407611168, 62.70724293864769550 ) ) ;
#1096=CARTESIAN_POINT ( 'NONE',  ( -19.05341960407611168, -5.049401038298163336, 21.45724293864768839 ) ) ;
#1097=CARTESIAN_POINT ( 'NONE',  ( 21.55341960407619695, -5.719274019375665929, 36.04275706135234714 ) ) ;
#1098=CARTESIAN_POINT ( 'NONE',  ( 16.46253265017160672, -9.564922557960803928, 58.33224293864769550 ) ) ;
#1100=CARTESIAN_POINT ( 'NONE',  ( 13.97604488694527802, 13.89961937509977652, 44.37390960531435269 ) ) ;
#1101=CARTESIAN_POINT ( 'NONE',  ( -10.72451020669898014, 18.67979575497178502, 35.41557627198102409 ) ) ;
#1102=CARTESIAN_POINT ( 'NONE',  ( 10.81492255796106328, -18.62759615963255655, 60.41775706135235424 ) ) ;
#1103=CARTESIAN_POINT ( 'NONE',  ( -19.05341960407611168, -5.049401038298163336, 21.45724293864768839 ) ) ;
#1104=CARTESIAN_POINT ( 'NONE',  ( 15.80617190586746368, 15.72974639402197994, 24.37390960531435979 ) ) ;
#1106=CARTESIAN_POINT ( 'NONE',  ( 16.52544592524335698, 4.483927247898782831, 96.45942372801901854 ) ) ;
#1108=CARTESIAN_POINT ( 'NONE',  ( -21.52544592524334988, -5.823673210054445271, 108.9594237280190185 ) ) ;
#1109=CARTESIAN_POINT ( 'NONE',  ( -12.14591786802326823, 12.06949235617739902, 63.12609039468568994 ) ) ;
#1110=CARTESIAN_POINT ( 'NONE',  ( -9.474510206698964154, 16.51473224551069663, 110.4155762719810383 ) ) ;
#1111=CARTESIAN_POINT ( 'NONE',  ( 16.53943276465976808, 0.05219959533934440121, 51.25109039468568994 ) ) ;
#1112=CARTESIAN_POINT ( 'NONE',  ( 4.379528057220092307, 16.55341960407617563, 32.29275706135235424 ) ) ;
#1113=CARTESIAN_POINT ( 'NONE',  ( -14.29746914071037622, -8.314922557961029526, 94.16775706135237556 ) ) ;
#1114=CARTESIAN_POINT ( 'NONE',  ( -18.62759615963255300, -10.81492255796106328, 49.16775706135234003 ) ) ;
#1115=CARTESIAN_POINT ( 'NONE',  ( 0.05219959533934541429, -16.53943276465976808, 20.00109039468568639 ) ) ;
#1116=CARTESIAN_POINT ( 'NONE',  ( 18.62759615963271287, -10.81492255796078972, 113.3322429386476955 ) ) ;
#1117=CARTESIAN_POINT ( 'NONE',  ( 4.379528057220092307, 16.55341960407617563, 27.29275706135234358 ) ) ;
#1118=CARTESIAN_POINT ( 'NONE',  ( -16.55341960407617563, 4.379528057220093196, 88.54275706135236135 ) ) ;
#1120=CARTESIAN_POINT ( 'NONE',  ( -21.53943276465977519, -0.05219959533937600094, 93.75109039468567573 ) ) ;
#1121=CARTESIAN_POINT ( 'NONE',  ( -9.564922557961040184, 16.46253265017147172, 87.91775706135233293 ) ) ;
#1122=CARTESIAN_POINT ( 'NONE',  ( 4.379528057220339221, -16.55341960407611168, 62.70724293864769550 ) ) ;
#1123=CARTESIAN_POINT ( 'NONE',  ( -4.483927247898539470, -16.52544592524342804, 37.29057627198102409 ) ) ;
#1124=CARTESIAN_POINT ( 'NONE',  ( -12.14591786802309592, -12.06949235617757132, 111.8739096053143669 ) ) ;
#1125=CARTESIAN_POINT ( 'NONE',  ( 19.05341960407617918, -5.049401038297876454, 51.04275706135231871 ) ) ;
#1126=CARTESIAN_POINT ( 'NONE',  ( 17.12812012977052589, -6.668231424565583154, 56.14051240676855059 ) ) ;
#1127=CARTESIAN_POINT ( 'NONE',  ( -18.67979575497193778, 10.72451020669871902, 53.33442372801901854 ) ) ;
#1128=CARTESIAN_POINT ( 'NONE',  ( 16.46253265017146816, 9.564922557961045513, 106.6677570613523471 ) ) ;
#1130=CARTESIAN_POINT ( 'NONE',  ( -19.02544592524342804, 5.153800228976336051, 101.0405762719810241 ) ) ;
#1131=CARTESIAN_POINT ( 'NONE',  ( 15.72974639402199770, -15.80617190586745480, 63.12390960531435979 ) ) ;
#1132=CARTESIAN_POINT ( 'NONE',  ( 0.05219959533936267826, -19.03943276465977164, 100.0010903946856757 ) ) ;
#1133=CARTESIAN_POINT ( 'NONE',  ( 13.97604488694527802, 13.89961937509977652, 89.37390960531436690 ) ) ;
#1134=CARTESIAN_POINT ( 'NONE',  ( -18.62759615963270932, 10.81492255796079327, 50.83224293864770971 ) ) ;
#1135=CARTESIAN_POINT ( 'NONE',  ( -12.06949235617756955, 12.14591786802309770, 110.6239096053143669 ) ) ;
#1136=CARTESIAN_POINT ( 'NONE',  ( -19.03943276465977164, 0.05219959533909376836, 76.24890960531435269 ) ) ;
#1137=CARTESIAN_POINT ( 'NONE',  ( 5.049401038298161559, -19.05341960407611168, 32.70724293864768129 ) ) ;
#1138=CARTESIAN_POINT ( 'NONE',  ( 10.81492255796106328, -18.62759615963255655, 35.41775706135234003 ) ) ;
#1139=CARTESIAN_POINT ( 'NONE',  ( 21.55341960407619695, -5.719274019375665929, 86.04275706135236135 ) ) ;
#1140=CARTESIAN_POINT ( 'NONE',  ( 14.34966873604972726, -8.224510206698740333, 95.83442372801903275 ) ) ;
#1141=CARTESIAN_POINT ( 'NONE',  ( -15.72974639402176322, -15.80617190586768395, 34.37609039468568284 ) ) ;
#1142=CARTESIAN_POINT ( 'NONE',  ( 5.719274019375673035, 21.55341960407619339, 37.29275706135235424 ) ) ;
#1143=CARTESIAN_POINT ( 'NONE',  ( 5.153800228976615827, -19.02544592524334988, 60.20942372801899012 ) ) ;
#1144=CARTESIAN_POINT ( 'NONE',  ( -5.049401038298153566, 19.05341960407611168, 75.20724293864769550 ) ) ;
#1145=CARTESIAN_POINT ( 'NONE',  ( 18.67979575497194134, -10.72451020669871369, 80.83442372801901854 ) ) ;
#1146=CARTESIAN_POINT ( 'NONE',  ( 15.80617190586746368, 15.72974639402197994, 89.37390960531435269 ) ) ;
#1147=CARTESIAN_POINT ( 'NONE',  ( -14.29746914071049879, 8.314922557960819915, 65.83224293864769550 ) ) ;
#1148=CARTESIAN_POINT ( 'NONE',  ( -5.823673210054431948, 21.52544592524334988, 107.7094237280190328 ) ) ;
#1149=CARTESIAN_POINT ( 'NONE',  ( -16.53943276465976808, 0.05219959533911058130, 86.24890960531436690 ) ) ;
#1150=CARTESIAN_POINT ( 'NONE',  ( -13.97604488694527625, -13.89961937509977652, 31.87390960531435979 ) ) ;
#1151=CARTESIAN_POINT ( 'NONE',  ( 0.05219959533936267826, -19.03943276465977164, 65.00109039468567573 ) ) ;
#1152=CARTESIAN_POINT ( 'NONE',  ( -12.06949235617756955, 12.14591786802309770, 30.62390960531436335 ) ) ;
#1153=CARTESIAN_POINT ( 'NONE',  ( -10.81492255796105439, 18.62759615963255655, 92.91775706135236135 ) ) ;
#1154=CARTESIAN_POINT ( 'NONE',  ( 9.564922557960805705, 16.46253265017160317, 94.58224293864769550 ) ) ;
#1155=CARTESIAN_POINT ( 'NONE',  ( 9.564922557961047289, -16.46253265017146816, 65.41775706135233293 ) ) ;
#1156=CARTESIAN_POINT ( 'NONE',  ( 10.81492255796078972, 18.62759615963270932, 64.58224293864769550 ) ) ;
#1157=CARTESIAN_POINT ( 'NONE',  ( -18.62759615963255300, -10.81492255796106328, 19.16775706135234714 ) ) ;
#1158=CARTESIAN_POINT ( 'NONE',  ( 19.05341960407617918, -5.049401038297876454, 106.0427570613523471 ) ) ;
#1159=CARTESIAN_POINT ( 'NONE',  ( 12.14591786802327356, -12.06949235617739191, 85.62609039468568994 ) ) ;
#1160=CARTESIAN_POINT ( 'NONE',  ( 16.31925111598459210, 7.325300261831489301, 62.33575461032749132 ) ) ;
#1161=CARTESIAN_POINT ( 'NONE',  ( -10.81492255796105439, 18.62759615963255655, 22.91775706135235069 ) ) ;
#1162=CARTESIAN_POINT ( 'NONE',  ( -16.53943276465976808, 0.05219959533911058130, 101.2489096053143669 ) ) ;
#1164=CARTESIAN_POINT ( 'NONE',  ( -12.14591786802326823, 12.06949235617739902, 43.12609039468568284 ) ) ;
#1165=CARTESIAN_POINT ( 'NONE',  ( 15.72974639402199770, -15.80617190586745480, 68.12390960531436690 ) ) ;
#1166=CARTESIAN_POINT ( 'NONE',  ( 14.34966873604972726, -8.224510206698740333, 110.8344237280190043 ) ) ;
#1167=CARTESIAN_POINT ( 'NONE',  ( -0.05219959533934338120, 16.53943276465976808, 42.50109039468567573 ) ) ;
#1168=CARTESIAN_POINT ( 'NONE',  ( 16.46253265017160672, -9.564922557960803928, 48.33224293864769550 ) ) ;
#1169=CARTESIAN_POINT ( 'NONE',  ( 14.29746914071037800, 8.314922557961029526, 81.66775706135236135 ) ) ;
#1170=CARTESIAN_POINT ( 'NONE',  ( -16.51473224551082808, 9.474510206698731452, 78.33442372801900433 ) ) ;
#1171=CARTESIAN_POINT ( 'NONE',  ( 18.67979575497178502, 10.72451020669898547, 69.16557627198102409 ) ) ;
#1172=CARTESIAN_POINT ( 'NONE',  ( 16.52544592524335698, 4.483927247898782831, 91.45942372801901854 ) ) ;
#1173=CARTESIAN_POINT ( 'NONE',  ( 5.719274019375673035, 21.55341960407619339, 82.29275706135234714 ) ) ;
#1174=CARTESIAN_POINT ( 'NONE',  ( 15.80617190586746368, 15.72974639402197994, 64.37390960531435269 ) ) ;
#1175=CARTESIAN_POINT ( 'NONE',  ( -0.05219959533907301413, -21.53943276465977519, 52.49890960531435979 ) ) ;
#1176=VERTEX_POINT ( 'NONE', #135799 ) ;
#1177=CARTESIAN_POINT ( 'NONE',  ( -8.314922557961024197, 14.29746914071037800, 77.91775706135231871 ) ) ;
#1178=CARTESIAN_POINT ( 'NONE',  ( -10.81492255796078084, -18.62759615963271287, 47.08224293864770260 ) ) ;
#1180=CARTESIAN_POINT ( 'NONE',  ( -19.02544592524342804, 5.153800228976336051, 116.0405762719810383 ) ) ;
#1182=CARTESIAN_POINT ( 'NONE',  ( -5.153800228976328057, -19.02544592524343514, 22.29057627198102765 ) ) ;
#1183=CARTESIAN_POINT ( 'NONE',  ( 10.81492255796078972, 18.62759615963270932, 74.58224293864768129 ) ) ;
#1184=CARTESIAN_POINT ( 'NONE',  ( -16.52544592524335698, -4.483927247898792601, 98.95942372801903275 ) ) ;
#1185=CARTESIAN_POINT ( 'NONE',  ( 21.52544592524334988, 5.823673210054432836, 51.45942372801901854 ) ) ;
#1186=CARTESIAN_POINT ( 'NONE',  ( -5.153800228976607833, 19.02544592524334988, 107.7094237280189759 ) ) ;
#1187=CARTESIAN_POINT ( 'NONE',  ( 12.06949235617757843, -12.14591786802309237, 113.1239096053143953 ) ) ;
#1188=CARTESIAN_POINT ( 'NONE',  ( 0.05219959533936267826, -19.03943276465977164, 105.0010903946856615 ) ) ;
#1189=CARTESIAN_POINT ( 'NONE',  ( -5.153800228976328057, -19.02544592524343514, 42.29057627198101699 ) ) ;
#1192=CARTESIAN_POINT ( 'NONE',  ( 5.153800228976335163, 19.02544592524342804, 94.79057627198103830 ) ) ;
#1193=CARTESIAN_POINT ( 'NONE',  ( 12.14591786802327356, -12.06949235617739191, 70.62609039468567573 ) ) ;
#1194=CARTESIAN_POINT ( 'NONE',  ( -16.46253265017146816, -9.564922557961047289, 84.16775706135233293 ) ) ;
#1195=CARTESIAN_POINT ( 'NONE',  ( 0.05219959533936267826, -19.03943276465977164, 20.00109039468567218 ) ) ;
#1196=CARTESIAN_POINT ( 'NONE',  ( 5.823673210054125526, 21.52544592524343514, 59.79057627198103120 ) ) ;
#1197=CARTESIAN_POINT ( 'NONE',  ( 12.06949235617739724, 12.14591786802326823, 81.87609039468568994 ) ) ;
#1199=CARTESIAN_POINT ( 'NONE',  ( 19.02544592524334988, 5.153800228976608722, 81.45942372801897591 ) ) ;
#1200=CARTESIAN_POINT ( 'NONE',  ( -0.05219959533909027116, -19.03943276465977164, 37.49890960531436690 ) ) ;
#1201=CARTESIAN_POINT ( 'NONE',  ( 5.049401038298161559, -19.05341960407611168, 97.70724293864766707 ) ) ;
#1202=CARTESIAN_POINT ( 'NONE',  ( -18.62759615963255300, -10.81492255796106328, 54.16775706135235424 ) ) ;
#1203=CARTESIAN_POINT ( 'NONE',  ( -16.51473224551069308, -9.474510206698971260, 46.66557627198102409 ) ) ;
#1205=CARTESIAN_POINT ( 'NONE',  ( -0.05219959533909027116, -19.03943276465977164, 112.4989096053143669 ) ) ;
#1206=CARTESIAN_POINT ( 'NONE',  ( -14.29746914071049879, 8.314922557960819915, 70.83224293864770971 ) ) ;
#1207=CARTESIAN_POINT ( 'NONE',  ( 5.823673210054125526, 21.52544592524343514, 64.79057627198103830 ) ) ;
#1209=CARTESIAN_POINT ( 'NONE',  ( 5.049401038297881783, 19.05341960407617563, 42.29275706135234003 ) ) ;
#1211=CARTESIAN_POINT ( 'NONE',  ( 19.05341960407611168, 5.049401038298154454, 58.95724293864768129 ) ) ;
#1212=CARTESIAN_POINT ( 'NONE',  ( -19.05341960407611168, -5.049401038298163336, 76.45724293864769550 ) ) ;
#1213=CARTESIAN_POINT ( 'NONE',  ( 8.224510206698742110, 14.34966873604972548, 52.08442372801901854 ) ) ;
#1216=CARTESIAN_POINT ( 'NONE',  ( -16.53943276465976808, -0.05219959533934237506, 83.75109039468568994 ) ) ;
#1218=CARTESIAN_POINT ( 'NONE',  ( -8.224510206698735004, -14.34966873604973081, 84.58442372801903275 ) ) ;
#1219=CARTESIAN_POINT ( 'NONE',  ( 12.14591786802327356, -12.06949235617739191, 50.62609039468568994 ) ) ;
#1220=CARTESIAN_POINT ( 'NONE',  ( -5.049401038297874678, -19.05341960407617918, 29.79275706135232227 ) ) ;
#1221=CARTESIAN_POINT ( 'NONE',  ( 19.03943276465977164, -0.05219959533909143690, 48.74890960531435979 ) ) ;
#1223=CARTESIAN_POINT ( 'NONE',  ( 0.05219959533937995610, -21.53943276465977519, 55.00109039468568284 ) ) ;
#1224=CARTESIAN_POINT ( 'NONE',  ( 13.97604488694548053, -13.89961937509957401, 55.62609039468566863 ) ) ;
#1225=CARTESIAN_POINT ( 'NONE',  ( -5.719274019375665041, -21.55341960407619695, 109.7927570613523613 ) ) ;
#1226=CARTESIAN_POINT ( 'NONE',  ( -0.05219959533909027116, -19.03943276465977164, 32.49890960531435979 ) ) ;
#1228=CARTESIAN_POINT ( 'NONE',  ( 0.05219959533907565091, 21.53943276465977519, 69.99890960531435269 ) ) ;
#1229=CARTESIAN_POINT ( 'NONE',  ( 9.474510206698971260, -16.51473224551069308, 112.9155762719810383 ) ) ;
#1230=CARTESIAN_POINT ( 'NONE',  ( 8.224510206698953496, -14.34966873604960469, 107.9155762719810241 ) ) ;
#1231=CARTESIAN_POINT ( 'NONE',  ( 8.224510206698742110, 14.34966873604972548, 37.08442372801901143 ) ) ;
#1232=CARTESIAN_POINT ( 'NONE',  ( -8.314922557960811034, -14.29746914071050412, 32.08224293864769550 ) ) ;
#1234=CARTESIAN_POINT ( 'NONE',  ( -21.53943276465977519, 0.05219959533907696930, 116.2489096053143669 ) ) ;
#1235=CARTESIAN_POINT ( 'NONE',  ( -4.483927247898539470, -16.52544592524342804, 42.29057627198103120 ) ) ;
#1236=CARTESIAN_POINT ( 'NONE',  ( 19.05341960407611168, 5.049401038298154454, 113.9572429386477097 ) ) ;
#1237=CARTESIAN_POINT ( 'NONE',  ( 0.05219959533936267826, -19.03943276465977164, 110.0010903946856757 ) ) ;
#1238=CARTESIAN_POINT ( 'NONE',  ( -5.153800228976607833, 19.02544592524334988, 22.70942372801899012 ) ) ;
#1239=CARTESIAN_POINT ( 'NONE',  ( -12.06949235617756955, 12.14591786802309770, 30.62390960531436335 ) ) ;
#1240=CARTESIAN_POINT ( 'NONE',  ( 21.52544592524344225, -5.823673210054117533, 103.5405762719810383 ) ) ;
#1241=DIRECTION ( 'NONE',  ( 0.000000000000000000, 0.000000000000000000, -1.000000000000000000 ) ) ;
#1242=CARTESIAN_POINT ( 'NONE',  ( -0.05219959533907301413, -21.53943276465977519, 62.49890960531436690 ) ) ;
#1243=CARTESIAN_POINT ( 'NONE',  ( -5.049401038298153566, 19.05341960407611168, 75.20724293864769550 ) ) ;
#1244=CARTESIAN_POINT ( 'NONE',  ( 8.314922557960818139, 14.29746914071049879, 54.58224293864769550 ) ) ;
#1245=CARTESIAN_POINT ( 'NONE',  ( 5.153800228976335163, 19.02544592524342804, 84.79057627198099567 ) ) ;
#1247=CARTESIAN_POINT ( 'NONE',  ( -19.02544592524334988, -5.153800228976617603, 58.95942372801900433 ) ) ;
#1248=CARTESIAN_POINT ( 'NONE',  ( 0.05219959533907565091, 21.53943276465977519, 99.99890960531436690 ) ) ;
#1249=CARTESIAN_POINT ( 'NONE',  ( 14.29746914071049879, -8.314922557960816363, 98.33224293864769550 ) ) ;
#1252=CARTESIAN_POINT ( 'NONE',  ( 0.05219959533937995610, -21.53943276465977519, 55.00109039468568284 ) ) ;
#1254=CARTESIAN_POINT ( 'NONE',  ( 4.379528057220339221, -16.55341960407611168, 27.70724293864769905 ) ) ;
#1255=CARTESIAN_POINT ( 'NONE',  ( -9.474510206698964154, 16.51473224551069663, 35.41557627198102409 ) ) ;
#1256=CARTESIAN_POINT ( 'NONE',  ( 16.51473224551069308, 9.474510206698969483, 99.16557627198102409 ) ) ;
#1257=CARTESIAN_POINT ( 'NONE',  ( -10.81492255796078084, -18.62759615963271287, 67.08224293864770971 ) ) ;
#1259=CARTESIAN_POINT ( 'NONE',  ( -0.05219959533909027116, -19.03943276465977164, 27.49890960531435624 ) ) ;
#1260=CARTESIAN_POINT ( 'NONE',  ( 15.80617190586746368, 15.72974639402197994, 54.37390960531435979 ) ) ;
#1261=CARTESIAN_POINT ( 'NONE',  ( 18.67979575497194134, -10.72451020669871369, 70.83442372801901854 ) ) ;
#1263=CARTESIAN_POINT ( 'NONE',  ( 16.53943276465976808, 0.05219959533934440121, 76.25109039468568994 ) ) ;
#1264=CARTESIAN_POINT ( 'NONE',  ( -9.564922557960796823, -16.46253265017161027, 57.08224293864769550 ) ) ;
#1265=CARTESIAN_POINT ( 'NONE',  ( 13.97604488694527802, 13.89961937509977652, 59.37390960531434558 ) ) ;
#1267=CARTESIAN_POINT ( 'NONE',  ( 13.89961937509957401, 13.97604488694547697, 21.87609039468566152 ) ) ;
#1268=CARTESIAN_POINT ( 'NONE',  ( 16.53943276465976808, 0.05219959533934440121, 81.25109039468568994 ) ) ;
#1269=CARTESIAN_POINT ( 'NONE',  ( 10.72451020669871369, 18.67979575497193778, 102.0844237280190185 ) ) ;
#1270=CARTESIAN_POINT ( 'NONE',  ( 13.89961937509977652, -13.97604488694527269, 73.12390960531436690 ) ) ;
#1271=CARTESIAN_POINT ( 'NONE',  ( -10.72451020669898014, 18.67979575497178502, 40.41557627198103120 ) ) ;
#1272=CARTESIAN_POINT ( 'NONE',  ( -19.03943276465977164, -0.05219959533935918106, 108.7510903946856615 ) ) ;
#1273=CARTESIAN_POINT ( 'NONE',  ( -10.72451020669870658, -18.67979575497194134, 79.58442372801903275 ) ) ;
#1274=CARTESIAN_POINT ( 'NONE',  ( -8.314922557961024197, 14.29746914071037800, 47.91775706135234714 ) ) ;
#1275=CARTESIAN_POINT ( 'NONE',  ( 15.80617190586746368, 15.72974639402197994, 94.37390960531436690 ) ) ;
#1276=CARTESIAN_POINT ( 'NONE',  ( -19.03943276465977164, -0.05219959533935918106, 113.7510903946856757 ) ) ;
#1277=CARTESIAN_POINT ( 'NONE',  ( -5.049401038298153566, 19.05341960407611168, 80.20724293864769550 ) ) ;
#1278=CARTESIAN_POINT ( 'NONE',  ( 9.474510206698729675, 16.51473224551082808, 112.0844237280190043 ) ) ;
#1279=CARTESIAN_POINT ( 'NONE',  ( 19.03943276465977164, -0.05219959533909143690, 43.74890960531435979 ) ) ;
#1281=CARTESIAN_POINT ( 'NONE',  ( 19.03943276465977164, 0.05219959533936151252, 111.2510903946856757 ) ) ;
#1282=CARTESIAN_POINT ( 'NONE',  ( -12.14591786802309592, -12.06949235617757132, 71.87390960531438111 ) ) ;
#1283=CARTESIAN_POINT ( 'NONE',  ( 16.55341960407618274, -4.379528057220086978, 71.04275706135234714 ) ) ;
#1284=CARTESIAN_POINT ( 'NONE',  ( -10.81492255796105439, 18.62759615963255655, 27.91775706135234358 ) ) ;
#1285=CARTESIAN_POINT ( 'NONE',  ( 13.89961937509977652, -13.97604488694527269, 53.12390960531434558 ) ) ;
#1286=CARTESIAN_POINT ( 'NONE',  ( 0.05219959533909260263, 19.03943276465977164, 69.99890960531435269 ) ) ;
#1287=CARTESIAN_POINT ( 'NONE',  ( 4.483927247898790824, -16.52544592524335698, 75.20942372801901854 ) ) ;
#1288=CARTESIAN_POINT ( 'NONE',  ( -17.50000000000000711, -5.499999999999944045, 81.28230962303565832 ) ) ;
#1290=CARTESIAN_POINT ( 'NONE',  ( -19.02544592524334988, -5.153800228976617603, 23.95942372801900078 ) ) ;
#1291=CARTESIAN_POINT ( 'NONE',  ( 19.03943276465977164, -0.05219959533909143690, 33.74890960531435979 ) ) ;
#1292=CARTESIAN_POINT ( 'NONE',  ( 17.50000000000000000, 5.499999999999992895, 66.70309617465828467 ) ) ;
#1294=CARTESIAN_POINT ( 'NONE',  ( -16.55341960407617563, 4.379528057220093196, 28.54275706135234358 ) ) ;
#1295=CARTESIAN_POINT ( 'NONE',  ( -19.05341960407617563, 5.049401038297882671, 58.54275706135234003 ) ) ;
#1296=CARTESIAN_POINT ( 'NONE',  ( -8.314922557961024197, 14.29746914071037800, 37.91775706135235424 ) ) ;
#1297=CARTESIAN_POINT ( 'NONE',  ( 5.049401038298161559, -19.05341960407611168, 37.70724293864768839 ) ) ;
#1298=CARTESIAN_POINT ( 'NONE',  ( 19.02544592524343514, -5.153800228976328945, 108.5405762719810383 ) ) ;
#1299=CARTESIAN_POINT ( 'NONE',  ( 13.97604488694527802, 13.89961937509977652, 59.37390960531434558 ) ) ;
#1300=CARTESIAN_POINT ( 'NONE',  ( 15.80617190586746368, 15.72974639402197994, 94.37390960531436690 ) ) ;
#1301=CARTESIAN_POINT ( 'NONE',  ( 9.474510206698971260, -16.51473224551069308, 87.91557627198102409 ) ) ;
#1303=CARTESIAN_POINT ( 'NONE',  ( 19.02544592524343514, -5.153800228976328945, 68.54057627198103830 ) ) ;
#1304=CARTESIAN_POINT ( 'NONE',  ( 14.34966873604972726, -8.224510206698740333, 110.8344237280190043 ) ) ;
#1306=CARTESIAN_POINT ( 'NONE',  ( -16.46253265017146816, -9.564922557961047289, 99.16775706135233293 ) ) ;
#1307=EDGE_CURVE ( 'NONE', #113002, #29646, #193703, .T. ) ;
#1308=CARTESIAN_POINT ( 'NONE',  ( 9.474510206698729675, 16.51473224551082808, 22.08442372801899722 ) ) ;
#1309=CARTESIAN_POINT ( 'NONE',  ( 4.379528057220339221, -16.55341960407611168, 62.70724293864769550 ) ) ;
#1310=CARTESIAN_POINT ( 'NONE',  ( 18.67979575497194134, -10.72451020669871369, 95.83442372801903275 ) ) ;
#1311=CARTESIAN_POINT ( 'NONE',  ( 16.51473224551069308, 9.474510206698969483, 44.16557627198103120 ) ) ;
#1312=CARTESIAN_POINT ( 'NONE',  ( 4.379528057220339221, -16.55341960407611168, 27.70724293864769905 ) ) ;
#1313=CARTESIAN_POINT ( 'NONE',  ( -15.72974639402176322, -15.80617190586768395, 84.37609039468570415 ) ) ;
#1314=CARTESIAN_POINT ( 'NONE',  ( -19.02544592524342804, 5.153800228976336051, 81.04057627198103830 ) ) ;
#1315=CARTESIAN_POINT ( 'NONE',  ( 19.05341960407611168, 5.049401038298154454, 93.95724293864769550 ) ) ;
#1316=CARTESIAN_POINT ( 'NONE',  ( 8.314922557960818139, 14.29746914071049879, 89.58224293864768129 ) ) ;
#1317=CARTESIAN_POINT ( 'NONE',  ( -8.314922557960811034, -14.29746914071050412, 77.08224293864769550 ) ) ;
#1318=CARTESIAN_POINT ( 'NONE',  ( -15.72974639402197994, 15.80617190586746368, 85.62390960531436690 ) ) ;
#1319=CARTESIAN_POINT ( 'NONE',  ( 13.89961937509977652, -13.97604488694527269, 78.12390960531433848 ) ) ;
#1320=CARTESIAN_POINT ( 'NONE',  ( 18.67979575497178502, 10.72451020669898547, 79.16557627198103830 ) ) ;
#1321=CARTESIAN_POINT ( 'NONE',  ( -13.97604488694547697, 13.89961937509957934, 73.12609039468568994 ) ) ;
#1323=CARTESIAN_POINT ( 'NONE',  ( -14.34966873604960291, -8.224510206698953496, 86.66557627198102409 ) ) ;
#1324=CARTESIAN_POINT ( 'NONE',  ( 5.049401038298161559, -19.05341960407611168, 62.70724293864769550 ) ) ;
#1325=CARTESIAN_POINT ( 'NONE',  ( 21.53943276465977519, -0.05219959533907433946, 63.74890960531435979 ) ) ;
#1327=CARTESIAN_POINT ( 'NONE',  ( -12.14591786802309592, -12.06949235617757132, 21.87390960531436690 ) ) ;
#1329=CARTESIAN_POINT ( 'NONE',  ( 5.049401038297881783, 19.05341960407617563, 112.2927570613523471 ) ) ;
#1330=CARTESIAN_POINT ( 'NONE',  ( -4.483927247898539470, -16.52544592524342804, 82.29057627198103830 ) ) ;
#1331=CARTESIAN_POINT ( 'NONE',  ( -19.35543954521080323, -5.499999999999531042, 94.58901960356449479 ) ) ;
#1332=CARTESIAN_POINT ( 'NONE',  ( -16.46253265017160317, 9.564922557960807481, 70.83224293864770971 ) ) ;
#1333=CARTESIAN_POINT ( 'NONE',  ( 19.02544592524343514, -5.153800228976328945, 38.54057627198103120 ) ) ;
#1334=CARTESIAN_POINT ( 'NONE',  ( -8.314922557960811034, -14.29746914071050412, 72.08224293864769550 ) ) ;
#1335=CARTESIAN_POINT ( 'NONE',  ( -19.02544592524342804, 5.153800228976336051, 101.0405762719810241 ) ) ;
#1336=CARTESIAN_POINT ( 'NONE',  ( -13.89961937509957401, -13.97604488694547875, 84.37609039468567573 ) ) ;
#1337=CARTESIAN_POINT ( 'NONE',  ( -9.564922557960796823, -16.46253265017161027, 82.08224293864768129 ) ) ;
#1338=CARTESIAN_POINT ( 'NONE',  ( -19.03943276465977164, 0.05219959533909376836, 86.24890960531436690 ) ) ;
#1339=CARTESIAN_POINT ( 'NONE',  ( 5.823673210054125526, 21.52544592524343514, 79.79057627198102409 ) ) ;
#1340=CARTESIAN_POINT ( 'NONE',  ( -4.483927247898782831, 16.52544592524335698, 67.70942372801901854 ) ) ;
#1341=CARTESIAN_POINT ( 'NONE',  ( 13.89961937509957579, 13.97604488694547520, 111.8760903946856757 ) ) ;
#1342=CARTESIAN_POINT ( 'NONE',  ( 19.05341960407611168, 5.049401038298154454, 68.95724293864769550 ) ) ;
#1343=CARTESIAN_POINT ( 'NONE',  ( -21.55341960407610458, -5.719274019375992779, 66.45724293864768129 ) ) ;
#1344=CARTESIAN_POINT ( 'NONE',  ( 13.89961937509957401, 13.97604488694547697, 91.87609039468567573 ) ) ;
#1345=CARTESIAN_POINT ( 'NONE',  ( 8.314922557960818139, 14.29746914071049879, 44.58224293864769550 ) ) ;
#1346=CARTESIAN_POINT ( 'NONE',  ( 21.52544592524334988, 5.823673210054432836, 46.45942372801901854 ) ) ;
#1349=CARTESIAN_POINT ( 'NONE',  ( -14.34966873604972548, 8.224510206698743886, 73.33442372801901854 ) ) ;
#1350=CARTESIAN_POINT ( 'NONE',  ( 16.46253265017160672, -9.564922557960803928, 103.3322429386476955 ) ) ;
#1353=CARTESIAN_POINT ( 'NONE',  ( -16.53943276465976808, -0.05219959533934237506, 88.75109039468567573 ) ) ;
#1354=CARTESIAN_POINT ( 'NONE',  ( 8.314922557961029526, -14.29746914071037800, 45.41775706135234003 ) ) ;
#1355=CARTESIAN_POINT ( 'NONE',  ( 19.03943276465977164, -0.05219959533909143690, 63.74890960531435979 ) ) ;
#1356=CARTESIAN_POINT ( 'NONE',  ( 0.05219959533909260263, 19.03943276465977164, 59.99890960531436690 ) ) ;
#1357=CARTESIAN_POINT ( 'NONE',  ( -15.80617190586768217, 15.72974639402176855, 53.12609039468568284 ) ) ;
#1358=CARTESIAN_POINT ( 'NONE',  ( 4.379528057220092307, 16.55341960407617563, 62.29275706135236845 ) ) ;
#1359=CARTESIAN_POINT ( 'NONE',  ( -16.55341960407611168, -4.379528057220339221, 31.45724293864769550 ) ) ;
#1360=CARTESIAN_POINT ( 'NONE',  ( -16.46253265017160317, 9.564922557960807481, 35.83224293864768839 ) ) ;
#1361=CARTESIAN_POINT ( 'NONE',  ( 19.02544592524343514, -5.153800228976328945, 28.54057627198102409 ) ) ;
#1362=CARTESIAN_POINT ( 'NONE',  ( -12.14591786802326823, 12.06949235617739902, 28.12609039468568284 ) ) ;
#1363=CARTESIAN_POINT ( 'NONE',  ( 5.049401038297881783, 19.05341960407617563, 87.29275706135234714 ) ) ;
#1364=CARTESIAN_POINT ( 'NONE',  ( 8.224510206698953496, -14.34966873604960469, 82.91557627198103830 ) ) ;
#1365=CARTESIAN_POINT ( 'NONE',  ( -0.05219959533909027116, -19.03943276465977164, 52.49890960531436690 ) ) ;
#1366=CARTESIAN_POINT ( 'NONE',  ( -13.89961937509957401, -13.97604488694547875, 84.37609039468567573 ) ) ;
#1368=CARTESIAN_POINT ( 'NONE',  ( 21.52544592524334988, 5.823673210054432836, 91.45942372801901854 ) ) ;
#1369=CARTESIAN_POINT ( 'NONE',  ( 8.224510206698742110, 14.34966873604972548, 52.08442372801901854 ) ) ;
#1371=CARTESIAN_POINT ( 'NONE',  ( 10.72451020669898902, -18.67979575497178502, 47.91557627198102409 ) ) ;
#1372=CARTESIAN_POINT ( 'NONE',  ( -8.224510206698735004, -14.34966873604973081, 44.58442372801901854 ) ) ;
#1373=CARTESIAN_POINT ( 'NONE',  ( -0.05219959533909027116, -19.03943276465977164, 32.49890960531435979 ) ) ;
#1374=CARTESIAN_POINT ( 'NONE',  ( 16.46253265017146816, 9.564922557961045513, 31.66775706135232937 ) ) ;
#1375=CARTESIAN_POINT ( 'NONE',  ( 13.89961937509977652, -13.97604488694527269, 73.12390960531436690 ) ) ;
#1376=CARTESIAN_POINT ( 'NONE',  ( 17.50000000000000000, -5.499999999999992895, 66.21769037696435589 ) ) ;
#1377=CARTESIAN_POINT ( 'NONE',  ( 19.02544592524343514, -5.153800228976328945, 58.54057627198102409 ) ) ;
#1379=CARTESIAN_POINT ( 'NONE',  ( 19.05341960407611168, 5.049401038298154454, 73.95724293864768129 ) ) ;
#1380=CARTESIAN_POINT ( 'NONE',  ( 17.50000000000014921, -3.292511757969696973, 112.5652027021053669 ) ) ;
#1381=CARTESIAN_POINT ( 'NONE',  ( -16.46253265017146816, -9.564922557961047289, 29.16775706135232937 ) ) ;
#1382=CARTESIAN_POINT ( 'NONE',  ( -13.89961937509957401, -13.97604488694547875, 19.37609039468566507 ) ) ;
#1383=CARTESIAN_POINT ( 'NONE',  ( -8.314922557960811034, -14.29746914071050412, 32.08224293864769550 ) ) ;
#1384=CARTESIAN_POINT ( 'NONE',  ( 13.89961937509977652, -13.97604488694527269, 48.12390960531435979 ) ) ;
#1385=CARTESIAN_POINT ( 'NONE',  ( -9.564922557960796823, -16.46253265017161027, 107.0822429386476955 ) ) ;
#1386=CARTESIAN_POINT ( 'NONE',  ( 15.72974639402176855, 15.80617190586768217, 66.87609039468568994 ) ) ;
#1387=CARTESIAN_POINT ( 'NONE',  ( 0.05219959533909260263, 19.03943276465977164, 49.99890960531435979 ) ) ;
#1388=CARTESIAN_POINT ( 'NONE',  ( -15.72974639402176322, -15.80617190586768395, 74.37609039468568994 ) ) ;
#1389=CARTESIAN_POINT ( 'NONE',  ( -10.81492255796078084, -18.62759615963271287, 27.08224293864769550 ) ) ;
#1390=CARTESIAN_POINT ( 'NONE',  ( 16.51473224551069308, 9.474510206698969483, 34.16557627198102409 ) ) ;
#1391=CARTESIAN_POINT ( 'NONE',  ( -15.72974639402176322, -15.80617190586768395, 29.37609039468568284 ) ) ;
#1392=CARTESIAN_POINT ( 'NONE',  ( 0.05219959533936267826, -19.03943276465977164, 50.00109039468566863 ) ) ;
#1393=CARTESIAN_POINT ( 'NONE',  ( 16.51473224551069308, 9.474510206698969483, 34.16557627198102409 ) ) ;
#1394=CARTESIAN_POINT ( 'NONE',  ( -16.46253265017160317, 9.564922557960807481, 80.83224293864769550 ) ) ;
#1395=CARTESIAN_POINT ( 'NONE',  ( 16.55341960407618274, -4.379528057220086978, 21.04275706135234714 ) ) ;
#1397=CARTESIAN_POINT ( 'NONE',  ( 12.14591786802309770, 12.06949235617756955, 69.37390960531436690 ) ) ;
#1398=CARTESIAN_POINT ( 'NONE',  ( -21.53943276465977519, 0.05219959533907696930, 36.24890960531435979 ) ) ;
#1399=CARTESIAN_POINT ( 'NONE',  ( 19.05341960407617918, -5.049401038297876454, 106.0427570613523471 ) ) ;
#1400=CARTESIAN_POINT ( 'NONE',  ( 5.823673210054125526, 21.52544592524343514, 104.7905762719810241 ) ) ;
#1401=CARTESIAN_POINT ( 'NONE',  ( 18.62759615963255655, 10.81492255796105972, 56.66775706135235424 ) ) ;
#1402=B_SPLINE_CURVE_WITH_KNOTS ( 'NONE', 3,
 ( #110750, #139103, #2578, #64258, #187623, #33920, #577, #123917, #81380, #159229, #23738, #191575, #192587, #22735, #98550, #160244, #99559, #144069, #20724, #65241 ),
 .UNSPECIFIED., .F., .F.,
 ( 4, 2, 2, 2, 2, 2, 2, 2, 2, 4 ),
 ( 0.004000878361811950439, 0.004499404418915936912, 0.004997930476019924254, 0.005496456533123910727, 0.005994982590227897201, 0.006244245618779890872, 0.006493508647331884542, 0.006992034704435875353, 0.007490560761539866164, 0.007989086818643856974 ),
 .UNSPECIFIED. ) ;
#1403=CARTESIAN_POINT ( 'NONE',  ( -0.05219959533934338120, 16.53943276465976808, 57.50109039468568994 ) ) ;
#1404=CARTESIAN_POINT ( 'NONE',  ( 16.53943276465976808, 0.05219959533934440121, 56.25109039468568284 ) ) ;
#1405=CARTESIAN_POINT ( 'NONE',  ( 19.03943276465977164, -0.05219959533909143690, 53.74890960531436690 ) ) ;
#1406=CARTESIAN_POINT ( 'NONE',  ( 12.14591786802327356, -12.06949235617739191, 85.62609039468568994 ) ) ;
#1407=CARTESIAN_POINT ( 'NONE',  ( -18.62759615963270932, 10.81492255796079327, 110.8322429386476955 ) ) ;
#1408=CARTESIAN_POINT ( 'NONE',  ( -8.314922557960811034, -14.29746914071050412, 47.08224293864770260 ) ) ;
#1409=CARTESIAN_POINT ( 'NONE',  ( 5.153800228976335163, 19.02544592524342804, 84.79057627198099567 ) ) ;
#1410=CARTESIAN_POINT ( 'NONE',  ( -12.06949235617739369, -12.14591786802326823, 69.37609039468567573 ) ) ;
#1411=CARTESIAN_POINT ( 'NONE',  ( 15.72974639402176855, 15.80617190586768217, 46.87609039468568994 ) ) ;
#1412=CARTESIAN_POINT ( 'NONE',  ( -5.153800228976607833, 19.02544592524334988, 107.7094237280189759 ) ) ;
#1413=CARTESIAN_POINT ( 'NONE',  ( 10.81492255796106328, -18.62759615963255655, 20.41775706135234714 ) ) ;
#1414=CARTESIAN_POINT ( 'NONE',  ( -0.05219959533910754901, -16.53943276465976808, 47.49890960531435979 ) ) ;
#1416=CARTESIAN_POINT ( 'NONE',  ( -17.49999999999999645, 5.499999999999992895, 73.71769037696435589 ) ) ;
#1417=CARTESIAN_POINT ( 'NONE',  ( -18.67979575497178146, -10.72451020669898902, 91.66557627198103830 ) ) ;
#1418=CARTESIAN_POINT ( 'NONE',  ( -12.14591786802309592, -12.06949235617757132, 26.87390960531435979 ) ) ;
#1421=CARTESIAN_POINT ( 'NONE',  ( 5.719274019375673035, 21.55341960407619339, 22.29275706135235069 ) ) ;
#1422=CARTESIAN_POINT ( 'NONE',  ( -0.05219959533909027116, -19.03943276465977164, 107.4989096053143527 ) ) ;
#1423=CARTESIAN_POINT ( 'NONE',  ( -10.72451020669870658, -18.67979575497194134, 19.58442372801901143 ) ) ;
#1424=CARTESIAN_POINT ( 'NONE',  ( -12.06949235617756955, 12.14591786802309770, 50.62390960531435979 ) ) ;
#1426=CARTESIAN_POINT ( 'NONE',  ( 4.483927247898790824, -16.52544592524335698, 60.20942372801902565 ) ) ;
#1427=CARTESIAN_POINT ( 'NONE',  ( -19.02544592524342804, 5.153800228976336051, 66.04057627198103830 ) ) ;
#1428=CARTESIAN_POINT ( 'NONE',  ( 19.03943276465977164, 0.05219959533936151252, 71.25109039468566152 ) ) ;
#1429=CARTESIAN_POINT ( 'NONE',  ( 5.049401038298161559, -19.05341960407611168, 77.70724293864765286 ) ) ;
#1431=CARTESIAN_POINT ( 'NONE',  ( 18.67979575497178502, 10.72451020669898547, 34.16557627198102409 ) ) ;
#1433=CARTESIAN_POINT ( 'NONE',  ( -19.05341960407611168, -5.049401038298163336, 41.45724293864769550 ) ) ;
#1434=CARTESIAN_POINT ( 'NONE',  ( 16.53943276465976808, 0.05219959533934440121, 21.25109039468567218 ) ) ;
#1435=CARTESIAN_POINT ( 'NONE',  ( 0.05219959533936267826, -19.03943276465977164, 60.00109039468566863 ) ) ;
#1436=CARTESIAN_POINT ( 'NONE',  ( -5.719274019375978568, 21.55341960407610458, 105.2072429386477097 ) ) ;
#1437=CARTESIAN_POINT ( 'NONE',  ( 16.52544592524342804, -4.483927247898539470, 38.54057627198103120 ) ) ;
#1438=CARTESIAN_POINT ( 'NONE',  ( -19.05341960407611168, -5.049401038298163336, 86.45724293864769550 ) ) ;
#1439=CARTESIAN_POINT ( 'NONE',  ( 21.53943276465977519, -0.05219959533907433946, 53.74890960531437401 ) ) ;
#1440=CARTESIAN_POINT ( 'NONE',  ( 15.80617190586746368, 15.72974639402197994, 99.37390960531436690 ) ) ;
#1441=CARTESIAN_POINT ( 'NONE',  ( -8.314922557961024197, 14.29746914071037800, 37.91775706135235424 ) ) ;
#1442=CARTESIAN_POINT ( 'NONE',  ( -5.823673210054116645, -21.52544592524344225, 37.29057627198102409 ) ) ;
#1443=CARTESIAN_POINT ( 'NONE',  ( 5.719274019375673035, 21.55341960407619339, 82.29275706135234714 ) ) ;
#1444=CARTESIAN_POINT ( 'NONE',  ( -5.153800228976328057, -19.02544592524343514, 92.29057627198099567 ) ) ;
#1445=CARTESIAN_POINT ( 'NONE',  ( 5.049401038298161559, -19.05341960407611168, 32.70724293864768129 ) ) ;
#1446=CARTESIAN_POINT ( 'NONE',  ( -13.89961937509977652, 13.97604488694528158, 90.62390960531432427 ) ) ;
#1447=CARTESIAN_POINT ( 'NONE',  ( -14.29746914071049879, 8.314922557960819915, 105.8322429386476955 ) ) ;
#1448=CARTESIAN_POINT ( 'NONE',  ( 13.97604488694527802, 13.89961937509977652, 64.37390960531436690 ) ) ;
#1449=CARTESIAN_POINT ( 'NONE',  ( -4.483927247898782831, 16.52544592524335698, 27.70942372801901854 ) ) ;
#1451=CARTESIAN_POINT ( 'NONE',  ( 21.55341960407619695, -5.719274019375665929, 101.0427570613523756 ) ) ;
#1452=CARTESIAN_POINT ( 'NONE',  ( -19.03943276465977164, 0.05219959533909376836, 111.2489096053143669 ) ) ;
#1453=CARTESIAN_POINT ( 'NONE',  ( 8.314922557961029526, -14.29746914071037800, 85.41775706135236135 ) ) ;
#1455=CARTESIAN_POINT ( 'NONE',  ( 9.474510206698729675, 16.51473224551082808, 67.08442372801900433 ) ) ;
#1456=CARTESIAN_POINT ( 'NONE',  ( -19.05341960407617563, 5.049401038297882671, 28.54275706135232937 ) ) ;
#1458=CARTESIAN_POINT ( 'NONE',  ( 16.51473224551069308, 9.474510206698969483, 24.16557627198102765 ) ) ;
#1459=CARTESIAN_POINT ( 'NONE',  ( 0.05219959533910956823, 16.53943276465976808, 34.99890960531435979 ) ) ;
#1460=CARTESIAN_POINT ( 'NONE',  ( 13.97604488694527802, 13.89961937509977652, 24.37390960531435624 ) ) ;
#1461=CARTESIAN_POINT ( 'NONE',  ( -12.06949235617756955, 12.14591786802309770, 30.62390960531436335 ) ) ;
#1463=CARTESIAN_POINT ( 'NONE',  ( -12.06949235617739369, -12.14591786802326823, 94.37609039468568994 ) ) ;
#1464=CARTESIAN_POINT ( 'NONE',  ( -19.02544592524342804, 5.153800228976336051, 41.04057627198103120 ) ) ;
#1465=CARTESIAN_POINT ( 'NONE',  ( 15.80617190586769283, -15.72974639402175789, 90.62609039468567573 ) ) ;
#1466=CARTESIAN_POINT ( 'NONE',  ( -19.03943276465977164, -0.05219959533935918106, 98.75109039468567573 ) ) ;
#1467=CARTESIAN_POINT ( 'NONE',  ( -15.80617190586768217, 15.72974639402176855, 78.12609039468570415 ) ) ;
#1468=CARTESIAN_POINT ( 'NONE',  ( -19.05341960407617563, 5.049401038297882671, 53.54275706135231871 ) ) ;
#1469=CARTESIAN_POINT ( 'NONE',  ( 19.03943276465977164, -0.05219959533909143690, 98.74890960531436690 ) ) ;
#1470=CARTESIAN_POINT ( 'NONE',  ( 16.46253265017160672, -9.564922557960803928, 68.33224293864770971 ) ) ;
#1471=CARTESIAN_POINT ( 'NONE',  ( 16.61371651742599909, 7.165104196376162804, 73.64584930007004004 ) ) ;
#1472=CARTESIAN_POINT ( 'NONE',  ( -12.14591786802309592, -12.06949235617757132, 66.87390960531436690 ) ) ;
#1473=CARTESIAN_POINT ( 'NONE',  ( 5.719274019375991003, -21.55341960407610458, 67.70724293864769550 ) ) ;
#1474=CARTESIAN_POINT ( 'NONE',  ( 5.049401038298161559, -19.05341960407611168, 57.70724293864769550 ) ) ;
#1475=CARTESIAN_POINT ( 'NONE',  ( -15.72974639402197994, 15.80617190586746368, 80.62390960531438111 ) ) ;
#1476=CARTESIAN_POINT ( 'NONE',  ( -14.29746914071037622, -8.314922557961029526, 74.16775706135231871 ) ) ;
#1477=ORIENTED_EDGE ( 'NONE', *, *, #126618, .F. ) ;
#1478=CARTESIAN_POINT ( 'NONE',  ( 19.05341960407611168, 5.049401038298154454, 48.95724293864768129 ) ) ;
#1480=CARTESIAN_POINT ( 'NONE',  ( -12.06949235617756955, 12.14591786802309770, 75.62390960531439532 ) ) ;
#1482=CARTESIAN_POINT ( 'NONE',  ( -9.474510206698964154, 16.51473224551069663, 50.41557627198102409 ) ) ;
#1483=CARTESIAN_POINT ( 'NONE',  ( -16.51473224551069308, -9.474510206698971260, 21.66557627198102765 ) ) ;
#1484=CARTESIAN_POINT ( 'NONE',  ( -13.89961937509957401, -13.97604488694547875, 69.37609039468564731 ) ) ;
#1485=CARTESIAN_POINT ( 'NONE',  ( -8.314922557960811034, -14.29746914071050412, 82.08224293864768129 ) ) ;
#1486=CARTESIAN_POINT ( 'NONE',  ( 21.55341960407619695, -5.719274019375665929, 41.04275706135236135 ) ) ;
#1487=CARTESIAN_POINT ( 'NONE',  ( -5.153800228976328057, -19.02544592524343514, 37.29057627198102409 ) ) ;
#1488=CARTESIAN_POINT ( 'NONE',  ( -15.72974639402197994, 15.80617190586746368, 100.6239096053143811 ) ) ;
#1489=CARTESIAN_POINT ( 'NONE',  ( 5.049401038298161559, -19.05341960407611168, 112.7072429386476813 ) ) ;
#1490=CARTESIAN_POINT ( 'NONE',  ( 8.224510206698953496, -14.34966873604960469, 87.91557627198103830 ) ) ;
#1492=CARTESIAN_POINT ( 'NONE',  ( 9.564922557960805705, 16.46253265017160317, 44.58224293864769550 ) ) ;
#1493=CARTESIAN_POINT ( 'NONE',  ( 16.88567814943161238, 6.947325034625693618, 113.7900112265259054 ) ) ;
#1494=CARTESIAN_POINT ( 'NONE',  ( -0.05219959533936034679, 19.03943276465977164, 97.50109039468567573 ) ) ;
#1495=CARTESIAN_POINT ( 'NONE',  ( 5.049401038298161559, -19.05341960407611168, 92.70724293864769550 ) ) ;
#1496=CARTESIAN_POINT ( 'NONE',  ( -15.72974639402176322, -15.80617190586768395, 39.37609039468567573 ) ) ;
#1497=CARTESIAN_POINT ( 'NONE',  ( -19.02544592524342804, 5.153800228976336051, 81.04057627198103830 ) ) ;
#1498=CARTESIAN_POINT ( 'NONE',  ( -5.049401038297874678, -19.05341960407617918, 69.79275706135233293 ) ) ;
#1499=CARTESIAN_POINT ( 'NONE',  ( -13.97604488694527625, -13.89961937509977652, 41.87390960531435979 ) ) ;
#1500=CARTESIAN_POINT ( 'NONE',  ( -8.224510206698948167, 14.34966873604960824, 70.41557627198102409 ) ) ;
#1501=CARTESIAN_POINT ( 'NONE',  ( 0.05219959533910956823, 16.53943276465976808, 69.99890960531435269 ) ) ;
#1502=CARTESIAN_POINT ( 'NONE',  ( 5.049401038298161559, -19.05341960407611168, 77.70724293864765286 ) ) ;
#1503=CARTESIAN_POINT ( 'NONE',  ( -10.72451020669898014, 18.67979575497178502, 100.4155762719810241 ) ) ;
#1504=CARTESIAN_POINT ( 'NONE',  ( -19.02544592524342804, 5.153800228976336051, 66.04057627198103830 ) ) ;
#1505=VECTOR ( 'NONE', #166542, 1000.000000000000000 ) ;
#1506=CARTESIAN_POINT ( 'NONE',  ( 5.049401038297881783, 19.05341960407617563, 22.29275706135233648 ) ) ;
#1507=CARTESIAN_POINT ( 'NONE',  ( -19.05341960407611168, -5.049401038298163336, 36.45724293864766707 ) ) ;
#1508=CARTESIAN_POINT ( 'NONE',  ( -4.483927247898539470, -16.52544592524342804, 27.29057627198103120 ) ) ;
#1509=CARTESIAN_POINT ( 'NONE',  ( -14.34966873604960291, -8.224510206698953496, 106.6655762719810383 ) ) ;
#1510=CARTESIAN_POINT ( 'NONE',  ( 5.049401038297881783, 19.05341960407617563, 102.2927570613523045 ) ) ;
#1512=CARTESIAN_POINT ( 'NONE',  ( 18.67979575497194134, -10.72451020669871369, 25.83442372801901499 ) ) ;
#1513=CARTESIAN_POINT ( 'NONE',  ( -13.97604488694547697, 13.89961937509957934, 63.12609039468566152 ) ) ;
#1514=CARTESIAN_POINT ( 'NONE',  ( -12.14591786802326823, 12.06949235617739902, 113.1260903946856899 ) ) ;
#1515=CARTESIAN_POINT ( 'NONE',  ( 15.72974639402199770, -15.80617190586745480, 68.12390960531436690 ) ) ;
#1516=CARTESIAN_POINT ( 'NONE',  ( -16.46253265017160317, 9.564922557960807481, 110.8322429386476955 ) ) ;
#1517=CARTESIAN_POINT ( 'NONE',  ( 4.379528057220339221, -16.55341960407611168, 57.70724293864770260 ) ) ;
#1518=CARTESIAN_POINT ( 'NONE',  ( 13.97604488694527802, 13.89961937509977652, 29.37390960531435979 ) ) ;
#1519=CARTESIAN_POINT ( 'NONE',  ( 13.97604488694548053, -13.89961937509957401, 20.62609039468567573 ) ) ;
#1520=CARTESIAN_POINT ( 'NONE',  ( -16.53943276465976808, -0.05219959533934237506, 83.75109039468568994 ) ) ;
#1521=CARTESIAN_POINT ( 'NONE',  ( -0.05219959533934338120, 16.53943276465976808, 52.50109039468567573 ) ) ;
#1522=CARTESIAN_POINT ( 'NONE',  ( 10.81492255796078972, 18.62759615963270932, 24.58224293864768839 ) ) ;
#1523=CARTESIAN_POINT ( 'NONE',  ( 5.719274019375673035, 21.55341960407619339, 112.2927570613523471 ) ) ;
#1524=CARTESIAN_POINT ( 'NONE',  ( -13.97604488694527625, -13.89961937509977652, 81.87390960531436690 ) ) ;
#1525=CARTESIAN_POINT ( 'NONE',  ( 16.55341960407618274, -4.379528057220086978, 66.04275706135236135 ) ) ;
#1526=CARTESIAN_POINT ( 'NONE',  ( -14.34966873604960291, -8.224510206698953496, 111.6655762719810525 ) ) ;
#1527=CARTESIAN_POINT ( 'NONE',  ( -4.483927247898539470, -16.52544592524342804, 22.29057627198102765 ) ) ;
#1529=CARTESIAN_POINT ( 'NONE',  ( -10.81492255796105439, 18.62759615963255655, 67.91775706135234714 ) ) ;
#1530=CARTESIAN_POINT ( 'NONE',  ( -19.05341960407611168, -5.049401038298163336, 91.45724293864766707 ) ) ;
#1531=CARTESIAN_POINT ( 'NONE',  ( 19.02544592524343514, -5.153800228976328945, 83.54057627198100988 ) ) ;
#1532=CARTESIAN_POINT ( 'NONE',  ( -5.049401038298153566, 19.05341960407611168, 105.2072429386476671 ) ) ;
#1534=CARTESIAN_POINT ( 'NONE',  ( 4.379528057220339221, -16.55341960407611168, 57.70724293864770260 ) ) ;
#1536=CARTESIAN_POINT ( 'NONE',  ( -14.34966873604972548, 8.224510206698743886, 108.3344237280190185 ) ) ;
#1537=CARTESIAN_POINT ( 'NONE',  ( 12.06949235617757843, -12.14591786802309237, 48.12390960531436690 ) ) ;
#1538=CARTESIAN_POINT ( 'NONE',  ( 0.05219959533934541429, -16.53943276465976808, 40.00109039468567573 ) ) ;
#1539=CARTESIAN_POINT ( 'NONE',  ( 18.22780087662125226, -5.499999999999864997, 61.01540105326109398 ) ) ;
#1541=CARTESIAN_POINT ( 'NONE',  ( 9.564922557961047289, -16.46253265017146816, 35.41775706135233293 ) ) ;
#1542=CARTESIAN_POINT ( 'NONE',  ( -9.564922557960796823, -16.46253265017161027, 82.08224293864768129 ) ) ;
#1543=CARTESIAN_POINT ( 'NONE',  ( 13.89961937509957401, 13.97604488694547697, 56.87609039468564731 ) ) ;
#1544=CARTESIAN_POINT ( 'NONE',  ( -9.564922557961040184, 16.46253265017147172, 57.91775706135233293 ) ) ;
#1545=CARTESIAN_POINT ( 'NONE',  ( 9.474510206698729675, 16.51473224551082808, 97.08442372801900433 ) ) ;
#1546=CARTESIAN_POINT ( 'NONE',  ( 14.34966873604972726, -8.224510206698740333, 80.83442372801901854 ) ) ;
#1549=CARTESIAN_POINT ( 'NONE',  ( -16.51473224551069308, -9.474510206698971260, 26.66557627198103120 ) ) ;
#1550=CARTESIAN_POINT ( 'NONE',  ( 19.05341960407611168, 5.049401038298154454, 103.9572429386476671 ) ) ;
#1551=CARTESIAN_POINT ( 'NONE',  ( -5.823673210054431948, 21.52544592524334988, 37.70942372801900433 ) ) ;
#1552=CARTESIAN_POINT ( 'NONE',  ( -13.89961937509957401, -13.97604488694547875, 84.37609039468567573 ) ) ;
#1553=CARTESIAN_POINT ( 'NONE',  ( 17.50000000000000355, 5.185212231016174123, 23.70589219561835392 ) ) ;
#1554=CARTESIAN_POINT ( 'NONE',  ( -19.03943276465977164, 0.05219959533909376836, 61.24890960531436690 ) ) ;
#1555=CARTESIAN_POINT ( 'NONE',  ( -9.564922557960796823, -16.46253265017161027, 102.0822429386477097 ) ) ;
#1556=CARTESIAN_POINT ( 'NONE',  ( -12.14591786802309592, -12.06949235617757132, 61.87390960531436690 ) ) ;
#1557=CARTESIAN_POINT ( 'NONE',  ( -16.46253265017160317, 9.564922557960807481, 65.83224293864769550 ) ) ;
#1558=CARTESIAN_POINT ( 'NONE',  ( -16.51473224551069308, -9.474510206698971260, 61.66557627198103120 ) ) ;
#1559=CARTESIAN_POINT ( 'NONE',  ( -16.46253265017146816, -9.564922557961047289, 59.16775706135233293 ) ) ;
#1560=CARTESIAN_POINT ( 'NONE',  ( 18.67979575497178502, 10.72451020669898547, 49.16557627198102409 ) ) ;
#1561=CARTESIAN_POINT ( 'NONE',  ( 5.049401038297881783, 19.05341960407617563, 42.29275706135234003 ) ) ;
#1562=CARTESIAN_POINT ( 'NONE',  ( -16.46253265017160317, 9.564922557960807481, 75.83224293864769550 ) ) ;
#1563=CARTESIAN_POINT ( 'NONE',  ( 5.719274019375991003, -21.55341960407610458, 82.70724293864770971 ) ) ;
#1564=CARTESIAN_POINT ( 'NONE',  ( 8.314922557960818139, 14.29746914071049879, 84.58224293864769550 ) ) ;
#1565=CARTESIAN_POINT ( 'NONE',  ( 0.05219959533936267826, -19.03943276465977164, 35.00109039468566863 ) ) ;
#1566=CARTESIAN_POINT ( 'NONE',  ( -18.67979575497178146, -10.72451020669898902, 46.66557627198102409 ) ) ;
#1567=CARTESIAN_POINT ( 'NONE',  ( 10.81492255796078972, 18.62759615963270932, 34.58224293864770260 ) ) ;
#1568=CARTESIAN_POINT ( 'NONE',  ( -19.03943276465977164, 0.05219959533909376836, 66.24890960531436690 ) ) ;
#1569=CARTESIAN_POINT ( 'NONE',  ( -13.97604488694527625, -13.89961937509977652, 56.87390960531434558 ) ) ;
#1570=CARTESIAN_POINT ( 'NONE',  ( 14.29746914071049879, -8.314922557960816363, 113.3322429386476955 ) ) ;
#1571=AXIS2_PLACEMENT_3D ( 'NONE', #136288, #181809, #132303 ) ;
#1572=CARTESIAN_POINT ( 'NONE',  ( -21.52544592524334988, -5.823673210054445271, 28.95942372801902209 ) ) ;
#1573=CARTESIAN_POINT ( 'NONE',  ( -9.474510206698964154, 16.51473224551069663, 110.4155762719810383 ) ) ;
#1574=CARTESIAN_POINT ( 'NONE',  ( -21.53943276465977519, -0.05219959533937600094, 33.75109039468568284 ) ) ;
#1575=CARTESIAN_POINT ( 'NONE',  ( 13.89961937509977652, -13.97604488694527269, 33.12390960531434558 ) ) ;
#1576=CARTESIAN_POINT ( 'NONE',  ( -10.81492255796078084, -18.62759615963271287, 112.0822429386477097 ) ) ;
#1577=CARTESIAN_POINT ( 'NONE',  ( -19.05341960407617563, 5.049401038297882671, 43.54275706135232582 ) ) ;
#1578=CARTESIAN_POINT ( 'NONE',  ( 13.89961937509977652, -13.97604488694527269, 28.12390960531435624 ) ) ;
#1580=CARTESIAN_POINT ( 'NONE',  ( 17.15686820162335025, -6.332220283772392655, 21.21893983122704341 ) ) ;
#1581=CARTESIAN_POINT ( 'NONE',  ( 4.379528057220092307, 16.55341960407617563, 62.29275706135236845 ) ) ;
#1582=CARTESIAN_POINT ( 'NONE',  ( -13.97604488694527625, -13.89961937509977652, 31.87390960531435979 ) ) ;
#1584=CARTESIAN_POINT ( 'NONE',  ( 13.97604488694527802, 13.89961937509977652, 69.37390960531436690 ) ) ;
#1585=CARTESIAN_POINT ( 'NONE',  ( -12.14591786802309592, -12.06949235617757132, 111.8739096053143669 ) ) ;
#1586=CARTESIAN_POINT ( 'NONE',  ( -21.53943276465977519, 0.05219959533907696930, 66.24890960531436690 ) ) ;
#1587=CARTESIAN_POINT ( 'NONE',  ( 4.379528057220339221, -16.55341960407611168, 82.70724293864770971 ) ) ;
#1588=CARTESIAN_POINT ( 'NONE',  ( -16.52544592524335698, -4.483927247898792601, 28.95942372801902209 ) ) ;
#1589=CARTESIAN_POINT ( 'NONE',  ( 5.719274019375673035, 21.55341960407619339, 92.29275706135236135 ) ) ;
#1590=CARTESIAN_POINT ( 'NONE',  ( 16.46253265017160672, -9.564922557960803928, 28.33224293864769550 ) ) ;
#1591=CARTESIAN_POINT ( 'NONE',  ( 0.05219959533934541429, -16.53943276465976808, 110.0010903946856757 ) ) ;
#1592=CARTESIAN_POINT ( 'NONE',  ( 16.55341960407611168, 4.379528057220329451, 58.95724293864770971 ) ) ;
#1593=CARTESIAN_POINT ( 'NONE',  ( -5.153800228976328057, -19.02544592524343514, 52.29057627198100988 ) ) ;
#1594=CARTESIAN_POINT ( 'NONE',  ( 21.53943276465977519, 0.05219959533937863772, 96.25109039468568994 ) ) ;
#1595=CARTESIAN_POINT ( 'NONE',  ( -5.719274019375978568, 21.55341960407610458, 110.2072429386477239 ) ) ;
#1596=CARTESIAN_POINT ( 'NONE',  ( 10.72451020669871369, 18.67979575497193778, 72.08442372801899012 ) ) ;
#1597=CARTESIAN_POINT ( 'NONE',  ( 12.14591786802327356, -12.06949235617739191, 45.62609039468567573 ) ) ;
#1598=CARTESIAN_POINT ( 'NONE',  ( -14.34966873604960291, -8.224510206698953496, 76.66557627198103830 ) ) ;
#1599=CARTESIAN_POINT ( 'NONE',  ( 5.719274019375673035, 21.55341960407619339, 87.29275706135236135 ) ) ;
#1600=CARTESIAN_POINT ( 'NONE',  ( -14.34966873604960291, -8.224510206698953496, 26.66557627198103475 ) ) ;
#1601=CARTESIAN_POINT ( 'NONE',  ( -17.40861289039002457, 6.110651285853324843, 113.6276752917256800 ) ) ;
#1602=CARTESIAN_POINT ( 'NONE',  ( 16.55341960407618274, -4.379528057220086978, 46.04275706135234714 ) ) ;
#1603=CARTESIAN_POINT ( 'NONE',  ( 12.06949235617757843, -12.14591786802309237, 38.12390960531436690 ) ) ;
#1604=CARTESIAN_POINT ( 'NONE',  ( 0.05219959533934541429, -16.53943276465976808, 90.00109039468567573 ) ) ;
#1605=CARTESIAN_POINT ( 'NONE',  ( 9.564922557960805705, 16.46253265017160317, 99.58224293864770971 ) ) ;
#1606=CARTESIAN_POINT ( 'NONE',  ( -0.05219959533907301413, -21.53943276465977519, 22.49890960531436335 ) ) ;
#1607=CARTESIAN_POINT ( 'NONE',  ( -5.823673210054431948, 21.52544592524334988, 102.7094237280190185 ) ) ;
#1608=CARTESIAN_POINT ( 'NONE',  ( 12.06949235617739724, 12.14591786802326823, 106.8760903946856899 ) ) ;
#1609=CARTESIAN_POINT ( 'NONE',  ( 14.29746914071049879, -8.314922557960816363, 73.33224293864769550 ) ) ;
#1610=CARTESIAN_POINT ( 'NONE',  ( 9.474510206698971260, -16.51473224551069308, 87.91557627198102409 ) ) ;
#1612=CARTESIAN_POINT ( 'NONE',  ( 4.483927247898790824, -16.52544592524335698, 25.20942372801901854 ) ) ;
#1613=CARTESIAN_POINT ( 'NONE',  ( 13.89961937509977652, -13.97604488694527269, 33.12390960531434558 ) ) ;
#1614=CARTESIAN_POINT ( 'NONE',  ( 19.02544592524343514, -5.153800228976328945, 88.54057627198102409 ) ) ;
#1615=CARTESIAN_POINT ( 'NONE',  ( -8.314922557961024197, 14.29746914071037800, 37.91775706135235424 ) ) ;
#1617=CARTESIAN_POINT ( 'NONE',  ( 19.03943276465977164, 0.05219959533936151252, 41.25109039468566152 ) ) ;
#1618=CARTESIAN_POINT ( 'NONE',  ( 16.55341960407618274, -4.379528057220086978, 96.04275706135236135 ) ) ;
#1619=CARTESIAN_POINT ( 'NONE',  ( 13.97604488694548053, -13.89961937509957401, 110.6260903946856615 ) ) ;
#1620=CARTESIAN_POINT ( 'NONE',  ( -9.564922557960796823, -16.46253265017161027, 32.08224293864769550 ) ) ;
#1621=CARTESIAN_POINT ( 'NONE',  ( -14.34966873604972548, 8.224510206698743886, 83.33442372801903275 ) ) ;
#1622=CARTESIAN_POINT ( 'NONE',  ( 14.29746914071037800, 8.314922557961029526, 71.66775706135234714 ) ) ;
#1623=CARTESIAN_POINT ( 'NONE',  ( 9.564922557961047289, -16.46253265017146816, 85.41775706135233293 ) ) ;
#1625=CARTESIAN_POINT ( 'NONE',  ( -21.53943276465977519, -0.05219959533937600094, 108.7510903946857042 ) ) ;
#1626=CARTESIAN_POINT ( 'NONE',  ( -19.05341960407611168, -5.049401038298163336, 41.45724293864769550 ) ) ;
#1627=CARTESIAN_POINT ( 'NONE',  ( -19.02544592524342804, 5.153800228976336051, 91.04057627198100988 ) ) ;
#1628=CARTESIAN_POINT ( 'NONE',  ( -8.224510206698948167, 14.34966873604960824, 80.41557627198103830 ) ) ;
#1630=CARTESIAN_POINT ( 'NONE',  ( -9.474510206698720793, -16.51473224551083518, 49.58442372801899722 ) ) ;
#1631=CARTESIAN_POINT ( 'NONE',  ( -21.53943276465977519, 0.05219959533907696930, 51.24890960531436690 ) ) ;
#1632=CARTESIAN_POINT ( 'NONE',  ( -5.153800228976607833, 19.02544592524334988, 27.70942372801899722 ) ) ;
#1633=CARTESIAN_POINT ( 'NONE',  ( -13.97604488694527625, -13.89961937509977652, 86.87390960531436690 ) ) ;
#1634=CARTESIAN_POINT ( 'NONE',  ( -13.97604488694547697, 13.89961937509957934, 28.12609039468565797 ) ) ;
#1635=CARTESIAN_POINT ( 'NONE',  ( 5.823673210054125526, 21.52544592524343514, 69.79057627198102409 ) ) ;
#1636=CARTESIAN_POINT ( 'NONE',  ( 5.049401038298161559, -19.05341960407611168, 107.7072429386476955 ) ) ;
#1637=CARTESIAN_POINT ( 'NONE',  ( 19.05341960407617918, -5.049401038297876454, 91.04275706135234714 ) ) ;
#1638=CARTESIAN_POINT ( 'NONE',  ( -17.50000000000002132, 4.049696124445919310, 109.1803967066594794 ) ) ;
#1639=CARTESIAN_POINT ( 'NONE',  ( 0.05219959533936267826, -19.03943276465977164, 105.0010903946856615 ) ) ;
#1640=CARTESIAN_POINT ( 'NONE',  ( 13.97604488694527802, 13.89961937509977652, 29.37390960531435979 ) ) ;
#1641=CARTESIAN_POINT ( 'NONE',  ( -19.02544592524342804, 5.153800228976336051, 91.04057627198100988 ) ) ;
#1642=CARTESIAN_POINT ( 'NONE',  ( 10.72451020669898902, -18.67979575497178502, 82.91557627198103830 ) ) ;
#1643=CARTESIAN_POINT ( 'NONE',  ( 16.52544592524335698, 4.483927247898782831, 46.45942372801901854 ) ) ;
#1644=CARTESIAN_POINT ( 'NONE',  ( 18.62759615963255655, 10.81492255796105972, 51.66775706135234714 ) ) ;
#1645=CARTESIAN_POINT ( 'NONE',  ( 16.51473224551083163, -9.474510206698727899, 95.83442372801900433 ) ) ;
#1646=CARTESIAN_POINT ( 'NONE',  ( 15.80617190586769283, -15.72974639402175789, 100.6260903946857184 ) ) ;
#1647=CARTESIAN_POINT ( 'NONE',  ( -16.53943276465976808, -0.05219959533934237506, 93.75109039468567573 ) ) ;
#1648=CARTESIAN_POINT ( 'NONE',  ( -16.46253265017160317, 9.564922557960807481, 105.8322429386476955 ) ) ;
#1649=CARTESIAN_POINT ( 'NONE',  ( 0.05219959533910956823, 16.53943276465976808, 84.99890960531436690 ) ) ;
#1650=CARTESIAN_POINT ( 'NONE',  ( 4.379528057220339221, -16.55341960407611168, 32.70724293864770260 ) ) ;
#1651=CARTESIAN_POINT ( 'NONE',  ( -16.46253265017146816, -9.564922557961047289, 74.16775706135234714 ) ) ;
#1652=CARTESIAN_POINT ( 'NONE',  ( 15.80617190586769283, -15.72974639402175789, 55.62609039468568284 ) ) ;
#1653=CARTESIAN_POINT ( 'NONE',  ( 16.46253265017146816, 9.564922557961045513, 31.66775706135232937 ) ) ;
#1654=CARTESIAN_POINT ( 'NONE',  ( 16.53943276465976808, -0.05219959533910856209, 93.74890960531436690 ) ) ;
#1655=CARTESIAN_POINT ( 'NONE',  ( 15.72974639402199770, -15.80617190586745480, 33.12390960531435979 ) ) ;
#1656=CARTESIAN_POINT ( 'NONE',  ( -0.05219959533934338120, 16.53943276465976808, 112.5010903946857042 ) ) ;
#1658=CARTESIAN_POINT ( 'NONE',  ( -18.67979575497193778, 10.72451020669871902, 103.3344237280190043 ) ) ;
#1659=CARTESIAN_POINT ( 'NONE',  ( -4.379528057220086978, -16.55341960407618274, 59.79275706135234714 ) ) ;
#1660=CARTESIAN_POINT ( 'NONE',  ( -12.06949235617739369, -12.14591786802326823, 109.3760903946857042 ) ) ;
#1661=CARTESIAN_POINT ( 'NONE',  ( -18.62759615963255300, -10.81492255796106328, 49.16775706135234003 ) ) ;
#1662=CARTESIAN_POINT ( 'NONE',  ( 15.80617190586769283, -15.72974639402175789, 60.62609039468567573 ) ) ;
#1663=ORIENTED_EDGE ( 'NONE', *, *, #80326, .T. ) ;
#1664=CARTESIAN_POINT ( 'NONE',  ( -10.81492255796105439, 18.62759615963255655, 32.91775706135234714 ) ) ;
#1665=CARTESIAN_POINT ( 'NONE',  ( 14.34966873604960469, 8.224510206698951720, 99.16557627198100988 ) ) ;
#1666=CARTESIAN_POINT ( 'NONE',  ( 13.89961937509977652, -13.97604488694527269, 23.12390960531436335 ) ) ;
#1667=CARTESIAN_POINT ( 'NONE',  ( -0.05219959533910754901, -16.53943276465976808, 62.49890960531436690 ) ) ;
#1668=CARTESIAN_POINT ( 'NONE',  ( 5.049401038298161559, -19.05341960407611168, 72.70724293864768129 ) ) ;
#1669=CARTESIAN_POINT ( 'NONE',  ( 14.34966873604972726, -8.224510206698740333, 110.8344237280190043 ) ) ;
#1670=CARTESIAN_POINT ( 'NONE',  ( 10.81492255796078972, 18.62759615963270932, 54.58224293864769550 ) ) ;
#1671=CARTESIAN_POINT ( 'NONE',  ( -12.14591786802309592, -12.06949235617757132, 96.87390960531436690 ) ) ;
#1672=CARTESIAN_POINT ( 'NONE',  ( -5.823673210054116645, -21.52544592524344225, 87.29057627198103830 ) ) ;
#1673=CARTESIAN_POINT ( 'NONE',  ( 19.02544592524343514, -5.153800228976328945, 103.5405762719809957 ) ) ;
#1674=CARTESIAN_POINT ( 'NONE',  ( -13.89961937509977652, 13.97604488694528158, 45.62390960531433848 ) ) ;
#1675=CARTESIAN_POINT ( 'NONE',  ( 19.05341960407617918, -5.049401038297876454, 111.0427570613523329 ) ) ;
#1676=CARTESIAN_POINT ( 'NONE',  ( 15.72974639402199770, -15.80617190586745480, 48.12390960531436690 ) ) ;
#1677=CARTESIAN_POINT ( 'NONE',  ( 5.823673210054444382, -21.52544592524334988, 70.20942372801904696 ) ) ;
#1678=CARTESIAN_POINT ( 'NONE',  ( 5.153800228976335163, 19.02544592524342804, 69.79057627198103830 ) ) ;
#1679=CARTESIAN_POINT ( 'NONE',  ( 19.02544592524343514, -5.153800228976328945, 93.54057627198102409 ) ) ;
#1680=CARTESIAN_POINT ( 'NONE',  ( -14.34966873604972548, 8.224510206698743886, 68.33442372801900433 ) ) ;
#1681=CARTESIAN_POINT ( 'NONE',  ( -0.05219959533937732626, 21.53943276465977519, 47.50109039468568994 ) ) ;
#1682=CARTESIAN_POINT ( 'NONE',  ( -18.67979575497193778, 10.72451020669871902, 83.33442372801903275 ) ) ;
#1683=CARTESIAN_POINT ( 'NONE',  ( -21.53943276465977519, 0.05219959533907696930, 96.24890960531435269 ) ) ;
#1685=CARTESIAN_POINT ( 'NONE',  ( 10.81492255796106328, -18.62759615963255655, 40.41775706135234714 ) ) ;
#1686=CARTESIAN_POINT ( 'NONE',  ( 14.34966873604972726, -8.224510206698740333, 80.83442372801901854 ) ) ;
#1687=CARTESIAN_POINT ( 'NONE',  ( -0.05219959533907301413, -21.53943276465977519, 77.49890960531433848 ) ) ;
#1688=CARTESIAN_POINT ( 'NONE',  ( -19.05341960407617563, 5.049401038297882671, 38.54275706135233293 ) ) ;
#1689=CIRCLE ( 'NONE', #85550, 2.500000000000002220 ) ;
#1690=CARTESIAN_POINT ( 'NONE',  ( 0.05219959533909260263, 19.03943276465977164, 79.99890960531436690 ) ) ;
#1691=CARTESIAN_POINT ( 'NONE',  ( 8.224510206698742110, 14.34966873604972548, 112.0844237280190185 ) ) ;
#1693=CARTESIAN_POINT ( 'NONE',  ( 13.89961937509977652, -13.97604488694527269, 98.12390960531433848 ) ) ;
#1695=CARTESIAN_POINT ( 'NONE',  ( -9.564922557961040184, 16.46253265017147172, 97.91775706135233293 ) ) ;
#1696=CARTESIAN_POINT ( 'NONE',  ( 5.823673210054125526, 21.52544592524343514, 54.79057627198104541 ) ) ;
#1697=CARTESIAN_POINT ( 'NONE',  ( 12.06949235617757843, -12.14591786802309237, 38.12390960531436690 ) ) ;
#1698=CARTESIAN_POINT ( 'NONE',  ( -9.564922557961040184, 16.46253265017147172, 107.9177570613523471 ) ) ;
#1699=CARTESIAN_POINT ( 'NONE',  ( 0.05219959533909260263, 19.03943276465977164, 24.99890960531435269 ) ) ;
#1700=CARTESIAN_POINT ( 'NONE',  ( -19.03943276465977164, -0.05219959533935918106, 108.7510903946856615 ) ) ;
#1701=CARTESIAN_POINT ( 'NONE',  ( -15.80617190586745835, -15.72974639402198527, 101.8739096053143811 ) ) ;
#1702=CARTESIAN_POINT ( 'NONE',  ( 19.05341960407617918, -5.049401038297876454, 76.04275706135230450 ) ) ;
#1703=CARTESIAN_POINT ( 'NONE',  ( 16.52544592524335698, 4.483927247898782831, 86.45942372801901854 ) ) ;
#1704=CARTESIAN_POINT ( 'NONE',  ( 9.564922557960805705, 16.46253265017160317, 64.58224293864769550 ) ) ;
#1705=CARTESIAN_POINT ( 'NONE',  ( -4.379528057220328563, 16.55341960407611168, 80.20724293864769550 ) ) ;
#1706=CARTESIAN_POINT ( 'NONE',  ( -19.05341960407611168, -5.049401038298163336, 56.45724293864768129 ) ) ;
#1707=CARTESIAN_POINT ( 'NONE',  ( 14.34966873604960469, 8.224510206698951720, 64.16557627198102409 ) ) ;
#1708=CARTESIAN_POINT ( 'NONE',  ( 16.46253265017160672, -9.564922557960803928, 23.33224293864769194 ) ) ;
#1710=CARTESIAN_POINT ( 'NONE',  ( 8.224510206698953496, -14.34966873604960469, 47.91557627198102409 ) ) ;
#1711=CARTESIAN_POINT ( 'NONE',  ( -13.89961937509977652, 13.97604488694528158, 75.62390960531438111 ) ) ;
#1713=CARTESIAN_POINT ( 'NONE',  ( 19.05341960407617918, -5.049401038297876454, 36.04275706135234003 ) ) ;
#1714=CARTESIAN_POINT ( 'NONE',  ( 8.224510206698742110, 14.34966873604972548, 62.08442372801901143 ) ) ;
#1715=CARTESIAN_POINT ( 'NONE',  ( 21.53943276465977519, -0.05219959533907433946, 68.74890960531435269 ) ) ;
#1716=CARTESIAN_POINT ( 'NONE',  ( 5.719274019375673035, 21.55341960407619339, 112.2927570613523471 ) ) ;
#1717=CARTESIAN_POINT ( 'NONE',  ( -9.564922557960796823, -16.46253265017161027, 72.08224293864770971 ) ) ;
#1719=CARTESIAN_POINT ( 'NONE',  ( -21.53943276465977519, 0.05219959533907696930, 21.24890960531436690 ) ) ;
#1720=CARTESIAN_POINT ( 'NONE',  ( 16.51473224551069308, 9.474510206698969483, 64.16557627198102409 ) ) ;
#1721=CARTESIAN_POINT ( 'NONE',  ( -21.52544592524334988, -5.823673210054445271, 38.95942372801901854 ) ) ;
#1722=CARTESIAN_POINT ( 'NONE',  ( -8.224510206698948167, 14.34966873604960824, 110.4155762719810383 ) ) ;
#1723=CARTESIAN_POINT ( 'NONE',  ( 18.62759615963271287, -10.81492255796078972, 103.3322429386476955 ) ) ;
#1724=CARTESIAN_POINT ( 'NONE',  ( 19.02544592524343514, -5.153800228976328945, 93.54057627198102409 ) ) ;
#1726=CARTESIAN_POINT ( 'NONE',  ( -0.05219959533937732626, 21.53943276465977519, 22.50109039468567573 ) ) ;
#1727=ORIENTED_EDGE ( 'NONE', *, *, #192158, .T. ) ;
#1728=CARTESIAN_POINT ( 'NONE',  ( -5.153800228976328057, -19.02544592524343514, 82.29057627198103830 ) ) ;
#1730=CARTESIAN_POINT ( 'NONE',  ( 10.81492255796078972, 18.62759615963270932, 99.58224293864770971 ) ) ;
#1731=CARTESIAN_POINT ( 'NONE',  ( -13.89961937509977652, 13.97604488694528158, 50.62390960531435979 ) ) ;
#1732=CARTESIAN_POINT ( 'NONE',  ( 9.474510206698729675, 16.51473224551082808, 102.0844237280190043 ) ) ;
#1734=CARTESIAN_POINT ( 'NONE',  ( -19.02544592524342804, 5.153800228976336051, 31.04057627198102409 ) ) ;
#1735=CARTESIAN_POINT ( 'NONE',  ( 21.52544592524334988, 5.823673210054432836, 91.45942372801901854 ) ) ;
#1736=CARTESIAN_POINT ( 'NONE',  ( -9.564922557960796823, -16.46253265017161027, 72.08224293864770971 ) ) ;
#1737=CARTESIAN_POINT ( 'NONE',  ( 15.72974639402176855, 15.80617190586768217, 41.87609039468568284 ) ) ;
#1738=CARTESIAN_POINT ( 'NONE',  ( -10.81492255796105439, 18.62759615963255655, 27.91775706135234358 ) ) ;
#1740=CARTESIAN_POINT ( 'NONE',  ( -16.51473224551069308, -9.474510206698971260, 86.66557627198102409 ) ) ;
#1741=CARTESIAN_POINT ( 'NONE',  ( 19.49671883438228193, 5.499999999999968914, 62.39279849105682985 ) ) ;
#1742=CARTESIAN_POINT ( 'NONE',  ( -12.06949235617739369, -12.14591786802326823, 44.37609039468567573 ) ) ;
#1743=CARTESIAN_POINT ( 'NONE',  ( -21.55341960407610458, -5.719274019375992779, 46.45724293864769550 ) ) ;
#1744=CARTESIAN_POINT ( 'NONE',  ( -10.72451020669870658, -18.67979575497194134, 39.58442372801901143 ) ) ;
#1745=CARTESIAN_POINT ( 'NONE',  ( -5.823673210054431948, 21.52544592524334988, 77.70942372801900433 ) ) ;
#1747=CARTESIAN_POINT ( 'NONE',  ( 0.05219959533936267826, -19.03943276465977164, 110.0010903946856757 ) ) ;
#1748=CARTESIAN_POINT ( 'NONE',  ( -19.02544592524342804, 5.153800228976336051, 56.04057627198100988 ) ) ;
#1749=CARTESIAN_POINT ( 'NONE',  ( 19.03943276465977164, -0.05219959533909143690, 88.74890960531436690 ) ) ;
#1750=CARTESIAN_POINT ( 'NONE',  ( 14.34966873604960469, 8.224510206698951720, 104.1655762719810241 ) ) ;
#1751=CARTESIAN_POINT ( 'NONE',  ( 16.53943276465976808, -0.05219959533910856209, 103.7489096053143669 ) ) ;
#1752=CARTESIAN_POINT ( 'NONE',  ( -15.80617190586745835, -15.72974639402198527, 21.87390960531436690 ) ) ;
#1753=CARTESIAN_POINT ( 'NONE',  ( -0.05219959533934338120, 16.53943276465976808, 82.50109039468568994 ) ) ;
#1754=CARTESIAN_POINT ( 'NONE',  ( -16.52544592524342804, 4.483927247898546575, 76.04057627198102409 ) ) ;
#1755=CARTESIAN_POINT ( 'NONE',  ( -16.46253265017160317, 9.564922557960807481, 55.83224293864769550 ) ) ;
#1756=CARTESIAN_POINT ( 'NONE',  ( -10.72451020669870658, -18.67979575497194134, 79.58442372801903275 ) ) ;
#1757=CARTESIAN_POINT ( 'NONE',  ( 18.62759615963255655, 10.81492255796105972, 71.66775706135234714 ) ) ;
#1758=CARTESIAN_POINT ( 'NONE',  ( 19.05341960407617918, -5.049401038297876454, 106.0427570613523471 ) ) ;
#1759=CARTESIAN_POINT ( 'NONE',  ( -8.224510206698948167, 14.34966873604960824, 65.41557627198102409 ) ) ;
#1760=CARTESIAN_POINT ( 'NONE',  ( 5.823673210054444382, -21.52544592524334988, 30.20942372801902565 ) ) ;
#1761=CARTESIAN_POINT ( 'NONE',  ( -10.81492255796078084, -18.62759615963271287, 67.08224293864770971 ) ) ;
#1763=CARTESIAN_POINT ( 'NONE',  ( 19.25176906914650843, 5.499999999999742428, 73.49927264242276692 ) ) ;
#1765=CARTESIAN_POINT ( 'NONE',  ( 13.89961937509977652, -13.97604488694527269, 73.12390960531436690 ) ) ;
#1766=CARTESIAN_POINT ( 'NONE',  ( 14.34966873604960469, 8.224510206698951720, 39.16557627198102409 ) ) ;
#1767=CARTESIAN_POINT ( 'NONE',  ( 0.05219959533934541429, -16.53943276465976808, 110.0010903946856757 ) ) ;
#1768=CARTESIAN_POINT ( 'NONE',  ( -16.55341960407617563, 4.379528057220093196, 93.54275706135234714 ) ) ;
#1769=CARTESIAN_POINT ( 'NONE',  ( 5.153800228976615827, -19.02544592524334988, 55.20942372801899722 ) ) ;
#1770=CARTESIAN_POINT ( 'NONE',  ( 16.19135201231368981, 7.376712067591808974, 47.68680854052031748 ) ) ;
#1771=CARTESIAN_POINT ( 'NONE',  ( -5.153800228976328057, -19.02544592524343514, 102.2905762719810383 ) ) ;
#1772=CARTESIAN_POINT ( 'NONE',  ( -14.29746914071049879, 8.314922557960819915, 80.83224293864769550 ) ) ;
#1773=CARTESIAN_POINT ( 'NONE',  ( 0.05219959533936267826, -19.03943276465977164, 40.00109039468566152 ) ) ;
#1774=CARTESIAN_POINT ( 'NONE',  ( -16.51473224551069308, -9.474510206698971260, 21.66557627198102765 ) ) ;
#1775=CARTESIAN_POINT ( 'NONE',  ( 18.62759615963271287, -10.81492255796078972, 28.33224293864769550 ) ) ;
#1776=CARTESIAN_POINT ( 'NONE',  ( 10.72451020669898902, -18.67979575497178502, 57.91557627198103120 ) ) ;
#1777=CARTESIAN_POINT ( 'NONE',  ( 8.314922557960818139, 14.29746914071049879, 94.58224293864769550 ) ) ;
#1778=CARTESIAN_POINT ( 'NONE',  ( -4.379528057220086978, -16.55341960407618274, 49.79275706135234714 ) ) ;
#1780=CARTESIAN_POINT ( 'NONE',  ( -16.52544592524342804, 4.483927247898546575, 96.04057627198102409 ) ) ;
#1782=CARTESIAN_POINT ( 'NONE',  ( -16.21995358207306381, 7.366697692864089042, 49.93551001512157939 ) ) ;
#1783=CARTESIAN_POINT ( 'NONE',  ( 0.05219959533909260263, 19.03943276465977164, 109.9989096053143669 ) ) ;
#1787=CARTESIAN_POINT ( 'NONE',  ( -8.314922557961024197, 14.29746914071037800, 42.91775706135235424 ) ) ;
#1788=CARTESIAN_POINT ( 'NONE',  ( 4.379528057220339221, -16.55341960407611168, 27.70724293864769905 ) ) ;
#1789=CARTESIAN_POINT ( 'NONE',  ( -18.62759615963270932, 10.81492255796079327, 55.83224293864770260 ) ) ;
#1790=CARTESIAN_POINT ( 'NONE',  ( 0.05219959533936267826, -19.03943276465977164, 90.00109039468567573 ) ) ;
#1791=CARTESIAN_POINT ( 'NONE',  ( 21.53943276465977519, -0.05219959533907433946, 53.74890960531437401 ) ) ;
#1792=CARTESIAN_POINT ( 'NONE',  ( -18.62759615963255300, -10.81492255796106328, 84.16775706135234714 ) ) ;
#1794=CARTESIAN_POINT ( 'NONE',  ( -4.483927247898782831, 16.52544592524335698, 37.70942372801900433 ) ) ;
#1795=CARTESIAN_POINT ( 'NONE',  ( -19.02544592524342804, 5.153800228976336051, 41.04057627198103120 ) ) ;
#1796=CARTESIAN_POINT ( 'NONE',  ( 9.474510206698971260, -16.51473224551069308, 97.91557627198102409 ) ) ;
#1797=CARTESIAN_POINT ( 'NONE',  ( -5.153800228976328057, -19.02544592524343514, 32.29057627198102409 ) ) ;
#1798=CARTESIAN_POINT ( 'NONE',  ( -16.52544592524342804, 4.483927247898546575, 101.0405762719810383 ) ) ;
#1799=CARTESIAN_POINT ( 'NONE',  ( -5.049401038298153566, 19.05341960407611168, 95.20724293864770971 ) ) ;
#1800=ORIENTED_EDGE ( 'NONE', *, *, #195432, .F. ) ;
#1801=CARTESIAN_POINT ( 'NONE',  ( 12.06949235617739724, 12.14591786802326823, 51.87609039468568284 ) ) ;
#1802=CARTESIAN_POINT ( 'NONE',  ( -21.55341960407610458, -5.719274019375992779, 96.45724293864770971 ) ) ;
#1803=CARTESIAN_POINT ( 'NONE',  ( -19.02544592524342804, 5.153800228976336051, 61.04057627198103120 ) ) ;
#1804=CARTESIAN_POINT ( 'NONE',  ( -10.72451020669870658, -18.67979575497194134, 24.58442372801901499 ) ) ;
#1805=CARTESIAN_POINT ( 'NONE',  ( 19.03943276465977164, -0.05219959533909143690, 83.74890960531436690 ) ) ;
#1808=CARTESIAN_POINT ( 'NONE',  ( 16.53943276465976808, 0.05219959533934440121, 41.25109039468568284 ) ) ;
#1809=CARTESIAN_POINT ( 'NONE',  ( 0.05219959533937995610, -21.53943276465977519, 25.00109039468567218 ) ) ;
#1810=CARTESIAN_POINT ( 'NONE',  ( 5.153800228976335163, 19.02544592524342804, 24.79057627198102765 ) ) ;
#1811=CARTESIAN_POINT ( 'NONE',  ( 9.474510206698971260, -16.51473224551069308, 102.9155762719810241 ) ) ;
#1812=CARTESIAN_POINT ( 'NONE',  ( 0.05219959533936267826, -19.03943276465977164, 70.00109039468566152 ) ) ;
#1813=CARTESIAN_POINT ( 'NONE',  ( 9.474510206698729675, 16.51473224551082808, 32.08442372801900433 ) ) ;
#1814=CARTESIAN_POINT ( 'NONE',  ( -21.53943276465977519, 0.05219959533907696930, 86.24890960531436690 ) ) ;
#1815=CARTESIAN_POINT ( 'NONE',  ( -16.46253265017146816, -9.564922557961047289, 39.16775706135234003 ) ) ;
#1816=CARTESIAN_POINT ( 'NONE',  ( -8.224510206698735004, -14.34966873604973081, 74.58442372801901854 ) ) ;
#1817=CARTESIAN_POINT ( 'NONE',  ( -9.564922557960796823, -16.46253265017161027, 112.0822429386476955 ) ) ;
#1818=CARTESIAN_POINT ( 'NONE',  ( -13.97604488694527625, -13.89961937509977652, 61.87390960531435979 ) ) ;
#1819=CARTESIAN_POINT ( 'NONE',  ( -18.67979575497193778, 10.72451020669871902, 68.33442372801900433 ) ) ;
#1820=CARTESIAN_POINT ( 'NONE',  ( 21.53943276465977519, 0.05219959533937863772, 86.25109039468568994 ) ) ;
#1821=CARTESIAN_POINT ( 'NONE',  ( -19.03943276465977164, 0.05219959533909376836, 71.24890960531435269 ) ) ;
#1822=CARTESIAN_POINT ( 'NONE',  ( 21.52544592524334988, 5.823673210054432836, 51.45942372801901854 ) ) ;
#1823=CARTESIAN_POINT ( 'NONE',  ( -19.05341960407617563, 5.049401038297882671, 93.54275706135234714 ) ) ;
#1824=CARTESIAN_POINT ( 'NONE',  ( -13.97604488694527625, -13.89961937509977652, 56.87390960531434558 ) ) ;
#1825=CARTESIAN_POINT ( 'NONE',  ( 19.02544592524343514, -5.153800228976328945, 103.5405762719809957 ) ) ;
#1826=CARTESIAN_POINT ( 'NONE',  ( -9.564922557960796823, -16.46253265017161027, 62.08224293864769550 ) ) ;
#1827=CARTESIAN_POINT ( 'NONE',  ( 16.46253265017160672, -9.564922557960803928, 113.3322429386476955 ) ) ;
#1828=CARTESIAN_POINT ( 'NONE',  ( -5.153800228976328057, -19.02544592524343514, 47.29057627198102409 ) ) ;
#1829=CARTESIAN_POINT ( 'NONE',  ( -5.823673210054116645, -21.52544592524344225, 102.2905762719810383 ) ) ;
#1830=CARTESIAN_POINT ( 'NONE',  ( -12.14591786802326823, 12.06949235617739902, 73.12609039468567573 ) ) ;
#1832=CARTESIAN_POINT ( 'NONE',  ( 16.51473224551083163, -9.474510206698727899, 30.83442372801900433 ) ) ;
#1833=CARTESIAN_POINT ( 'NONE',  ( -0.05219959533909027116, -19.03943276465977164, 72.49890960531435269 ) ) ;
#1834=CARTESIAN_POINT ( 'NONE',  ( -8.224510206698948167, 14.34966873604960824, 60.41557627198102409 ) ) ;
#1835=CARTESIAN_POINT ( 'NONE',  ( -8.314922557960811034, -14.29746914071050412, 92.08224293864769550 ) ) ;
#1836=CARTESIAN_POINT ( 'NONE',  ( 0.05219959533909260263, 19.03943276465977164, 94.99890960531436690 ) ) ;
#1837=CARTESIAN_POINT ( 'NONE',  ( 9.474510206698971260, -16.51473224551069308, 97.91557627198102409 ) ) ;
#1838=CARTESIAN_POINT ( 'NONE',  ( -16.46253265017160317, 9.564922557960807481, 105.8322429386476955 ) ) ;
#1839=CARTESIAN_POINT ( 'NONE',  ( 19.03943276465977164, 0.05219959533936151252, 21.25109039468565797 ) ) ;
#1840=CARTESIAN_POINT ( 'NONE',  ( -14.29746914071037622, -8.314922557961029526, 94.16775706135237556 ) ) ;
#1841=CARTESIAN_POINT ( 'NONE',  ( -10.81492255796105439, 18.62759615963255655, 37.91775706135235424 ) ) ;
#1842=CARTESIAN_POINT ( 'NONE',  ( 10.81492255796078972, 18.62759615963270932, 29.58224293864769905 ) ) ;
#1843=CARTESIAN_POINT ( 'NONE',  ( -5.823673210054116645, -21.52544592524344225, 102.2905762719810383 ) ) ;
#1844=CARTESIAN_POINT ( 'NONE',  ( -12.06949235617756955, 12.14591786802309770, 65.62390960531436690 ) ) ;
#1845=CARTESIAN_POINT ( 'NONE',  ( 0.05219959533909260263, 19.03943276465977164, 49.99890960531435979 ) ) ;
#1846=CARTESIAN_POINT ( 'NONE',  ( -16.52544592524342804, 4.483927247898546575, 81.04057627198102409 ) ) ;
#1847=CARTESIAN_POINT ( 'NONE',  ( 10.81492255796078972, 18.62759615963270932, 39.58224293864769550 ) ) ;
#1848=CARTESIAN_POINT ( 'NONE',  ( -5.049401038297874678, -19.05341960407617918, 49.79275706135231871 ) ) ;
#1849=CARTESIAN_POINT ( 'NONE',  ( -12.14591786802309592, -12.06949235617757132, 111.8739096053143669 ) ) ;
#1850=VERTEX_POINT ( 'NONE', #97199 ) ;
#1851=CARTESIAN_POINT ( 'NONE',  ( 8.224510206698742110, 14.34966873604972548, 67.08442372801901854 ) ) ;
#1852=CARTESIAN_POINT ( 'NONE',  ( 5.153800228976335163, 19.02544592524342804, 64.79057627198100988 ) ) ;
#1854=CARTESIAN_POINT ( 'NONE',  ( -16.55341960407611168, -4.379528057220339221, 86.45724293864770971 ) ) ;
#1855=CARTESIAN_POINT ( 'NONE',  ( -5.823673210054116645, -21.52544592524344225, 37.29057627198102409 ) ) ;
#1857=CARTESIAN_POINT ( 'NONE',  ( 16.55341960407618274, -4.379528057220086978, 106.0427570613523471 ) ) ;
#1858=CARTESIAN_POINT ( 'NONE',  ( 16.53943276465976808, 0.05219959533934440121, 31.25109039468568639 ) ) ;
#1859=CARTESIAN_POINT ( 'NONE',  ( -18.62759615963255300, -10.81492255796106328, 99.16775706135234714 ) ) ;
#1860=CARTESIAN_POINT ( 'NONE',  ( -19.02544592524342804, 5.153800228976336051, 86.04057627198103830 ) ) ;
#1861=CARTESIAN_POINT ( 'NONE',  ( -21.53943276465977519, 0.05219959533907696930, 116.2489096053143669 ) ) ;
#1862=CARTESIAN_POINT ( 'NONE',  ( -19.02544592524342804, 5.153800228976336051, 31.04057627198102409 ) ) ;
#1863=CARTESIAN_POINT ( 'NONE',  ( -8.224510206698735004, -14.34966873604973081, 24.58442372801901499 ) ) ;
#1865=CARTESIAN_POINT ( 'NONE',  ( -13.89961937509957401, -13.97604488694547875, 89.37609039468563310 ) ) ;
#1866=CARTESIAN_POINT ( 'NONE',  ( 21.55341960407610458, 5.719274019375980345, 88.95724293864769550 ) ) ;
#1867=CARTESIAN_POINT ( 'NONE',  ( 13.97604488694548053, -13.89961937509957401, 65.62609039468567573 ) ) ;
#1869=CARTESIAN_POINT ( 'NONE',  ( 15.80617190586746368, 15.72974639402197994, 114.3739096053143527 ) ) ;
#1870=CARTESIAN_POINT ( 'NONE',  ( 18.22780087662123805, -5.499999999999976019, 73.51763182126894947 ) ) ;
#1871=CARTESIAN_POINT ( 'NONE',  ( -9.474510206698964154, 16.51473224551069663, 80.41557627198103830 ) ) ;
#1872=CARTESIAN_POINT ( 'NONE',  ( 8.224510206698742110, 14.34966873604972548, 27.08442372801901854 ) ) ;
#1874=CARTESIAN_POINT ( 'NONE',  ( 9.564922557961047289, -16.46253265017146816, 65.41775706135233293 ) ) ;
#1875=CARTESIAN_POINT ( 'NONE',  ( -15.80617190586768217, 15.72974639402176855, 23.12609039468567573 ) ) ;
#1876=CARTESIAN_POINT ( 'NONE',  ( -16.55341960407611168, -4.379528057220339221, 71.45724293864769550 ) ) ;
#1877=CARTESIAN_POINT ( 'NONE',  ( 0.05219959533909260263, 19.03943276465977164, 79.99890960531436690 ) ) ;
#1878=CARTESIAN_POINT ( 'NONE',  ( -12.14591786802326823, 12.06949235617739902, 43.12609039468568284 ) ) ;
#1879=CARTESIAN_POINT ( 'NONE',  ( -16.51473224551082808, 9.474510206698731452, 38.33442372801899722 ) ) ;
#1880=CARTESIAN_POINT ( 'NONE',  ( -21.55341960407619339, 5.719274019375674811, 68.54275706135234714 ) ) ;
#1881=CARTESIAN_POINT ( 'NONE',  ( -9.474510206698720793, -16.51473224551083518, 104.5844237280190043 ) ) ;
#1882=CARTESIAN_POINT ( 'NONE',  ( 9.564922557960805705, 16.46253265017160317, 59.58224293864769550 ) ) ;
#1883=CARTESIAN_POINT ( 'NONE',  ( -19.03943276465977164, -0.05219959533935918106, 88.75109039468567573 ) ) ;
#1884=CARTESIAN_POINT ( 'NONE',  ( -16.53943276465976808, -0.05219959533934237506, 53.75109039468568994 ) ) ;
#1885=CARTESIAN_POINT ( 'NONE',  ( 10.81492255796106328, -18.62759615963255655, 100.4177570613523471 ) ) ;
#1886=CARTESIAN_POINT ( 'NONE',  ( -9.474510206698720793, -16.51473224551083518, 64.58442372801900433 ) ) ;
#1887=CARTESIAN_POINT ( 'NONE',  ( -19.05341960407611168, -5.049401038298163336, 56.45724293864768129 ) ) ;
#1888=CARTESIAN_POINT ( 'NONE',  ( -18.67979575497178146, -10.72451020669898902, 66.66557627198102409 ) ) ;
#1889=CARTESIAN_POINT ( 'NONE',  ( 16.55341960407611168, 4.379528057220329451, 68.95724293864769550 ) ) ;
#1890=CARTESIAN_POINT ( 'NONE',  ( -19.03943276465977164, -0.05219959533935918106, 63.75109039468566863 ) ) ;
#1892=CARTESIAN_POINT ( 'NONE',  ( 0.05219959533936267826, -19.03943276465977164, 40.00109039468566152 ) ) ;
#1894=CARTESIAN_POINT ( 'NONE',  ( -4.379528057220086978, -16.55341960407618274, 94.79275706135234714 ) ) ;
#1895=CARTESIAN_POINT ( 'NONE',  ( 12.06949235617757843, -12.14591786802309237, 68.12390960531436690 ) ) ;
#1896=CARTESIAN_POINT ( 'NONE',  ( 10.81492255796106328, -18.62759615963255655, 90.41775706135236135 ) ) ;
#1898=CARTESIAN_POINT ( 'NONE',  ( -10.81492255796078084, -18.62759615963271287, 92.08224293864769550 ) ) ;
#1899=CARTESIAN_POINT ( 'NONE',  ( 13.89961937509977652, -13.97604488694527269, 48.12390960531435979 ) ) ;
#1900=CARTESIAN_POINT ( 'NONE',  ( 18.62759615963255655, 10.81492255796105972, 76.66775706135234714 ) ) ;
#1901=CARTESIAN_POINT ( 'NONE',  ( 19.03943276465977164, -0.05219959533909143690, 53.74890960531436690 ) ) ;
#1903=CARTESIAN_POINT ( 'NONE',  ( 5.153800228976335163, 19.02544592524342804, 64.79057627198100988 ) ) ;
#1904=CARTESIAN_POINT ( 'NONE',  ( 12.14591786802309770, 12.06949235617756955, 114.3739096053143527 ) ) ;
#1905=CARTESIAN_POINT ( 'NONE',  ( -21.53943276465977519, 0.05219959533907696930, 21.24890960531436690 ) ) ;
#1907=CARTESIAN_POINT ( 'NONE',  ( 14.34966873604960469, 8.224510206698951720, 49.16557627198102409 ) ) ;
#1908=CARTESIAN_POINT ( 'NONE',  ( 9.474510206698971260, -16.51473224551069308, 27.91557627198103120 ) ) ;
#1909=CARTESIAN_POINT ( 'NONE',  ( -16.53943276465976808, 0.05219959533911058130, 86.24890960531436690 ) ) ;
#1910=CARTESIAN_POINT ( 'NONE',  ( -10.81492255796078084, -18.62759615963271287, 102.0822429386476955 ) ) ;
#1911=CARTESIAN_POINT ( 'NONE',  ( 21.53943276465977519, 0.05219959533937863772, 31.25109039468568639 ) ) ;
#1913=CARTESIAN_POINT ( 'NONE',  ( -14.29746914071037622, -8.314922557961029526, 49.16775706135234003 ) ) ;
#1914=CARTESIAN_POINT ( 'NONE',  ( -18.62759615963270932, 10.81492255796079327, 90.83224293864769550 ) ) ;
#1915=CARTESIAN_POINT ( 'NONE',  ( -21.53943276465977519, -0.05219959533937600094, 108.7510903946857042 ) ) ;
#1916=CARTESIAN_POINT ( 'NONE',  ( 0.05219959533909260263, 19.03943276465977164, 109.9989096053143669 ) ) ;
#1917=CARTESIAN_POINT ( 'NONE',  ( 0.05219959533937995610, -21.53943276465977519, 50.00109039468568994 ) ) ;
#1918=CARTESIAN_POINT ( 'NONE',  ( -18.62759615963270932, 10.81492255796079327, 40.83224293864769550 ) ) ;
#1919=CARTESIAN_POINT ( 'NONE',  ( 4.483927247898790824, -16.52544592524335698, 100.2094237280190043 ) ) ;
#1920=CARTESIAN_POINT ( 'NONE',  ( 5.823673210054444382, -21.52544592524334988, 60.20942372801902565 ) ) ;
#1921=CARTESIAN_POINT ( 'NONE',  ( 0.05219959533937995610, -21.53943276465977519, 100.0010903946857042 ) ) ;
#1922=CARTESIAN_POINT ( 'NONE',  ( 16.46253265017146816, 9.564922557961045513, 36.66775706135233293 ) ) ;
#1923=CARTESIAN_POINT ( 'NONE',  ( -14.34966873604972548, 8.224510206698743886, 93.33442372801901854 ) ) ;
#1924=CARTESIAN_POINT ( 'NONE',  ( 15.72974639402176855, 15.80617190586768217, 36.87609039468568994 ) ) ;
#1925=CARTESIAN_POINT ( 'NONE',  ( -0.05219959533909027116, -19.03943276465977164, 42.49890960531435269 ) ) ;
#1926=CARTESIAN_POINT ( 'NONE',  ( -5.153800228976607833, 19.02544592524334988, 27.70942372801899722 ) ) ;
#1927=CARTESIAN_POINT ( 'NONE',  ( 21.52544592524344225, -5.823673210054117533, 23.54057627198102765 ) ) ;
#1928=CARTESIAN_POINT ( 'NONE',  ( -18.67979575497178146, -10.72451020669898902, 111.6655762719810525 ) ) ;
#1929=CARTESIAN_POINT ( 'NONE',  ( 21.53943276465977519, -0.05219959533907433946, 78.74890960531436690 ) ) ;
#1930=CARTESIAN_POINT ( 'NONE',  ( 12.06949235617739724, 12.14591786802326823, 36.87609039468568994 ) ) ;
#1931=CARTESIAN_POINT ( 'NONE',  ( -17.49999999999999645, -7.500000000000000888, 22.00000000000000711 ) ) ;
#1932=CARTESIAN_POINT ( 'NONE',  ( -15.80617190586745835, -15.72974639402198527, 76.87390960531439532 ) ) ;
#1933=CARTESIAN_POINT ( 'NONE',  ( -4.379528057220086978, -16.55341960407618274, 69.79275706135234714 ) ) ;
#1934=CARTESIAN_POINT ( 'NONE',  ( 14.34966873604960469, 8.224510206698951720, 64.16557627198102409 ) ) ;
#1936=CARTESIAN_POINT ( 'NONE',  ( -0.05219959533936034679, 19.03943276465977164, 97.50109039468567573 ) ) ;
#1938=CARTESIAN_POINT ( 'NONE',  ( 16.55341960407618274, -4.379528057220086978, 41.04275706135236135 ) ) ;
#1939=CARTESIAN_POINT ( 'NONE',  ( 5.823673210054125526, 21.52544592524343514, 114.7905762719810383 ) ) ;
#1940=CARTESIAN_POINT ( 'NONE',  ( 18.67979575497178502, 10.72451020669898547, 69.16557627198102409 ) ) ;
#1941=CARTESIAN_POINT ( 'NONE',  ( -13.89961937509977652, 13.97604488694528158, 115.6239096053143669 ) ) ;
#1942=CARTESIAN_POINT ( 'NONE',  ( 12.14591786802327356, -12.06949235617739191, 60.62609039468567573 ) ) ;
#1943=CARTESIAN_POINT ( 'NONE',  ( 5.153800228976335163, 19.02544592524342804, 74.79057627198103830 ) ) ;
#1944=CARTESIAN_POINT ( 'NONE',  ( -21.52544592524334988, -5.823673210054445271, 43.95942372801902565 ) ) ;
#1945=CARTESIAN_POINT ( 'NONE',  ( 13.89961937509957401, 13.97604488694547697, 111.8760903946856757 ) ) ;
#1946=CARTESIAN_POINT ( 'NONE',  ( -19.02544592524342804, 5.153800228976336051, 106.0405762719810241 ) ) ;
#1948=CARTESIAN_POINT ( 'NONE',  ( 19.02544592524334988, 5.153800228976608722, 26.45942372801899722 ) ) ;
#1949=CARTESIAN_POINT ( 'NONE',  ( -16.53943276465976808, -0.05219959533934237506, 38.75109039468567573 ) ) ;
#1950=CARTESIAN_POINT ( 'NONE',  ( 13.97604488694527802, 13.89961937509977652, 104.3739096053143385 ) ) ;
#1951=CARTESIAN_POINT ( 'NONE',  ( 18.67979575497178502, 10.72451020669898547, 99.16557627198100988 ) ) ;
#1952=CARTESIAN_POINT ( 'NONE',  ( -5.153800228976328057, -19.02544592524343514, 57.29057627198103120 ) ) ;
#1953=CARTESIAN_POINT ( 'NONE',  ( -16.61371651742603461, 7.165104196376024248, 23.85415069992998482 ) ) ;
#1954=CARTESIAN_POINT ( 'NONE',  ( 8.224510206698953496, -14.34966873604960469, 77.91557627198102409 ) ) ;
#1955=CARTESIAN_POINT ( 'NONE',  ( 21.52544592524344225, -5.823673210054117533, 23.54057627198102765 ) ) ;
#1956=CARTESIAN_POINT ( 'NONE',  ( -16.18388926212241685, 7.379444403734376046, 34.56046848633846480 ) ) ;
#1957=CARTESIAN_POINT ( 'NONE',  ( 18.67979575497178502, 10.72451020669898547, 109.1655762719810383 ) ) ;
#1958=CARTESIAN_POINT ( 'NONE',  ( 19.03943276465977164, 0.05219959533936151252, 61.25109039468566863 ) ) ;
#1959=CARTESIAN_POINT ( 'NONE',  ( 21.53943276465977519, -0.05219959533907433946, 33.74890960531436690 ) ) ;
#1960=CARTESIAN_POINT ( 'NONE',  ( 13.97604488694527802, 13.89961937509977652, 29.37390960531435979 ) ) ;
#1961=CARTESIAN_POINT ( 'NONE',  ( 18.67979575497178502, 10.72451020669898547, 49.16557627198102409 ) ) ;
#1962=CARTESIAN_POINT ( 'NONE',  ( -19.03943276465977164, 0.05219959533909376836, 101.2489096053143669 ) ) ;
#1963=CARTESIAN_POINT ( 'NONE',  ( 10.72451020669871369, 18.67979575497193778, 82.08442372801901854 ) ) ;
#1964=CARTESIAN_POINT ( 'NONE',  ( 0.05219959533909260263, 19.03943276465977164, 49.99890960531435979 ) ) ;
#1965=CARTESIAN_POINT ( 'NONE',  ( 16.53943276465976808, -0.05219959533910856209, 88.74890960531436690 ) ) ;
#1966=CARTESIAN_POINT ( 'NONE',  ( 4.483927247898790824, -16.52544592524335698, 30.20942372801902565 ) ) ;
#1967=CARTESIAN_POINT ( 'NONE',  ( 5.153800228976335163, 19.02544592524342804, 54.79057627198103120 ) ) ;
#1968=CARTESIAN_POINT ( 'NONE',  ( 18.67979575497194134, -10.72451020669871369, 65.83442372801900433 ) ) ;
#1969=ORIENTED_EDGE ( 'NONE', *, *, #146153, .T. ) ;
#1970=CARTESIAN_POINT ( 'NONE',  ( 5.153800228976615827, -19.02544592524334988, 25.20942372801900433 ) ) ;
#1971=CARTESIAN_POINT ( 'NONE',  ( 5.049401038297881783, 19.05341960407617563, 42.29275706135234003 ) ) ;
#1973=CARTESIAN_POINT ( 'NONE',  ( -21.52544592524334988, -5.823673210054445271, 38.95942372801901854 ) ) ;
#1975=LINE ( 'NONE', #106172, #114116 ) ;
#1976=CARTESIAN_POINT ( 'NONE',  ( 5.049401038297881783, 19.05341960407617563, 32.29275706135233293 ) ) ;
#1977=CARTESIAN_POINT ( 'NONE',  ( -16.46253265017160317, 9.564922557960807481, 85.83224293864769550 ) ) ;
#1978=CARTESIAN_POINT ( 'NONE',  ( -19.03943276465977164, 0.05219959533909376836, 66.24890960531436690 ) ) ;
#1979=CARTESIAN_POINT ( 'NONE',  ( 12.06949235617757843, -12.14591786802309237, 23.12390960531436335 ) ) ;
#1980=CARTESIAN_POINT ( 'NONE',  ( 0.05219959533909260263, 19.03943276465977164, 114.9989096053143669 ) ) ;
#1981=CARTESIAN_POINT ( 'NONE',  ( 15.80617190586769283, -15.72974639402175789, 80.62609039468567573 ) ) ;
#1983=CARTESIAN_POINT ( 'NONE',  ( 16.36317988757058473, 7.306389748694949837, 58.40210391636776421 ) ) ;
#1984=CARTESIAN_POINT ( 'NONE',  ( 21.53943276465977519, 0.05219959533937863772, 81.25109039468568994 ) ) ;
#1985=CARTESIAN_POINT ( 'NONE',  ( 16.61371651742598843, -7.165104196376272938, 41.35415069992997417 ) ) ;
#1986=CARTESIAN_POINT ( 'NONE',  ( 5.153800228976335163, 19.02544592524342804, 104.7905762719809957 ) ) ;
#1989=CARTESIAN_POINT ( 'NONE',  ( 21.55341960407610458, 5.719274019375980345, 63.95724293864770260 ) ) ;
#1990=CARTESIAN_POINT ( 'NONE',  ( -8.314922557960811034, -14.29746914071050412, 22.08224293864769194 ) ) ;
#1991=CARTESIAN_POINT ( 'NONE',  ( 0.05219959533910956823, 16.53943276465976808, 109.9989096053143527 ) ) ;
#1992=CARTESIAN_POINT ( 'NONE',  ( 5.049401038298161559, -19.05341960407611168, 97.70724293864766707 ) ) ;
#1993=CARTESIAN_POINT ( 'NONE',  ( 10.72451020669871369, 18.67979575497193778, 112.0844237280190185 ) ) ;
#1994=CARTESIAN_POINT ( 'NONE',  ( -8.224510206698948167, 14.34966873604960824, 105.4155762719810383 ) ) ;
#1995=CARTESIAN_POINT ( 'NONE',  ( 21.52544592524334988, 5.823673210054432836, 66.45942372801903275 ) ) ;
#1996=CARTESIAN_POINT ( 'NONE',  ( 9.474510206698971260, -16.51473224551069308, 112.9155762719810383 ) ) ;
#1997=CARTESIAN_POINT ( 'NONE',  ( 8.314922557961029526, -14.29746914071037800, 105.4177570613523613 ) ) ;
#1998=CARTESIAN_POINT ( 'NONE',  ( -13.89961937509957401, -13.97604488694547875, 64.37609039468567573 ) ) ;
#2000=CARTESIAN_POINT ( 'NONE',  ( 19.02544592524343514, -5.153800228976328945, 103.5405762719809957 ) ) ;
#2001=CARTESIAN_POINT ( 'NONE',  ( 12.14591786802309770, 12.06949235617756955, 74.37390960531436690 ) ) ;
#2003=CARTESIAN_POINT ( 'NONE',  ( -13.89961937509957401, -13.97604488694547875, 59.37609039468566863 ) ) ;
#2004=CARTESIAN_POINT ( 'NONE',  ( 5.153800228976335163, 19.02544592524342804, 79.79057627198102409 ) ) ;
#2005=CARTESIAN_POINT ( 'NONE',  ( -16.52544592524342804, 4.483927247898546575, 66.04057627198103830 ) ) ;
#2006=CARTESIAN_POINT ( 'NONE',  ( -0.05219959533936034679, 19.03943276465977164, 97.50109039468567573 ) ) ;
#2007=CARTESIAN_POINT ( 'NONE',  ( 15.72974639402199770, -15.80617190586745480, 48.12390960531436690 ) ) ;
#2008=VERTEX_POINT ( 'NONE', #18414 ) ;
#2009=CARTESIAN_POINT ( 'NONE',  ( -13.97604488694527625, -13.89961937509977652, 21.87390960531435979 ) ) ;
#2010=CARTESIAN_POINT ( 'NONE',  ( 30.00000000000000000, -1.163414459189985801E-14, 92.50000000000000000 ) ) ;
#2011=CARTESIAN_POINT ( 'NONE',  ( -16.51473224551069308, -9.474510206698971260, 76.66557627198103830 ) ) ;
#2012=CARTESIAN_POINT ( 'NONE',  ( -15.72974639402197994, 15.80617190586746368, 65.62390960531436690 ) ) ;
#2013=CARTESIAN_POINT ( 'NONE',  ( -12.06949235617739369, -12.14591786802326823, 94.37609039468568994 ) ) ;
#2014=CARTESIAN_POINT ( 'NONE',  ( 16.46253265017160672, -9.564922557960803928, 78.33224293864769550 ) ) ;
#2015=CARTESIAN_POINT ( 'NONE',  ( 0.05219959533936267826, -19.03943276465977164, 50.00109039468566863 ) ) ;
#2016=CARTESIAN_POINT ( 'NONE',  ( 0.05219959533937995610, -21.53943276465977519, 80.00109039468568994 ) ) ;
#2017=CARTESIAN_POINT ( 'NONE',  ( -5.719274019375978568, 21.55341960407610458, 65.20724293864768129 ) ) ;
#2018=CARTESIAN_POINT ( 'NONE',  ( -5.153800228976328057, -19.02544592524343514, 112.2905762719810099 ) ) ;
#2019=CARTESIAN_POINT ( 'NONE',  ( 5.153800228976335163, 19.02544592524342804, 34.79057627198102409 ) ) ;
#2020=CARTESIAN_POINT ( 'NONE',  ( 4.379528057220092307, 16.55341960407617563, 107.2927570613523471 ) ) ;
#2021=CARTESIAN_POINT ( 'NONE',  ( -16.55341960407617563, 4.379528057220093196, 23.54275706135235424 ) ) ;
#2022=CARTESIAN_POINT ( 'NONE',  ( 16.61371651742603817, 7.165104196376042012, 53.64584930007004715 ) ) ;
#2023=CARTESIAN_POINT ( 'NONE',  ( -18.67979575497193778, 10.72451020669871902, 103.3344237280190043 ) ) ;
#2024=CARTESIAN_POINT ( 'NONE',  ( 16.55341960407611168, 4.379528057220329451, 53.95724293864770260 ) ) ;
#2025=CARTESIAN_POINT ( 'NONE',  ( 5.823673210054125526, 21.52544592524343514, 89.79057627198103830 ) ) ;
#2026=CARTESIAN_POINT ( 'NONE',  ( 18.62759615963271287, -10.81492255796078972, 88.33224293864769550 ) ) ;
#2028=CARTESIAN_POINT ( 'NONE',  ( 0.05219959533907565091, 21.53943276465977519, 39.99890960531436690 ) ) ;
#2029=CARTESIAN_POINT ( 'NONE',  ( 14.29746914071037800, 8.314922557961029526, 61.66775706135235424 ) ) ;
#2030=CARTESIAN_POINT ( 'NONE',  ( 12.14591786802309770, 12.06949235617756955, 89.37390960531435269 ) ) ;
#2031=CARTESIAN_POINT ( 'NONE',  ( -16.51473224551069308, -9.474510206698971260, 51.66557627198102409 ) ) ;
#2033=CARTESIAN_POINT ( 'NONE',  ( 16.52544592524335698, 4.483927247898782831, 101.4594237280190185 ) ) ;
#2034=CARTESIAN_POINT ( 'NONE',  ( -18.62759615963255300, -10.81492255796106328, 34.16775706135234714 ) ) ;
#2035=CARTESIAN_POINT ( 'NONE',  ( -0.05219959533909027116, -19.03943276465977164, 102.4989096053143669 ) ) ;
#2036=CARTESIAN_POINT ( 'NONE',  ( -5.823673210054431948, 21.52544592524334988, 67.70942372801901854 ) ) ;
#2038=CARTESIAN_POINT ( 'NONE',  ( -0.05219959533909027116, -19.03943276465977164, 27.49890960531435624 ) ) ;
#2040=CARTESIAN_POINT ( 'NONE',  ( 5.719274019375673035, 21.55341960407619339, 57.29275706135234714 ) ) ;
#2041=CARTESIAN_POINT ( 'NONE',  ( 5.153800228976335163, 19.02544592524342804, 49.79057627198100988 ) ) ;
#2042=CARTESIAN_POINT ( 'NONE',  ( 19.03943276465977164, -0.05219959533909143690, 113.7489096053143669 ) ) ;
#2043=CARTESIAN_POINT ( 'NONE',  ( 0.05219959533909260263, 19.03943276465977164, 89.99890960531436690 ) ) ;
#2044=CARTESIAN_POINT ( 'NONE',  ( 16.46253265017146816, 9.564922557961045513, 61.66775706135234003 ) ) ;
#2045=CARTESIAN_POINT ( 'NONE',  ( -5.823673210054431948, 21.52544592524334988, 47.70942372801902565 ) ) ;
#2047=CARTESIAN_POINT ( 'NONE',  ( 16.46253265017146816, 9.564922557961045513, 56.66775706135233293 ) ) ;
#2048=CARTESIAN_POINT ( 'NONE',  ( 13.97604488694527802, 13.89961937509977652, 39.37390960531435269 ) ) ;
#2049=CARTESIAN_POINT ( 'NONE',  ( -12.06949235617739369, -12.14591786802326823, 104.3760903946856899 ) ) ;
#2050=CARTESIAN_POINT ( 'NONE',  ( -9.474510206698720793, -16.51473224551083518, 74.58442372801900433 ) ) ;
#2051=CARTESIAN_POINT ( 'NONE',  ( -8.224510206698948167, 14.34966873604960824, 30.41557627198101699 ) ) ;
#2052=CARTESIAN_POINT ( 'NONE',  ( -5.049401038297874678, -19.05341960407617918, 49.79275706135231871 ) ) ;
#2053=CARTESIAN_POINT ( 'NONE',  ( 16.46253265017160672, -9.564922557960803928, 98.33224293864769550 ) ) ;
#2055=CARTESIAN_POINT ( 'NONE',  ( -15.80617190586768217, 15.72974639402176855, 108.1260903946856757 ) ) ;
#2056=CARTESIAN_POINT ( 'NONE',  ( 19.03943276465977164, 0.05219959533936151252, 31.25109039468566863 ) ) ;
#2057=CARTESIAN_POINT ( 'NONE',  ( 19.03943276465977164, -0.05219959533909143690, 33.74890960531435979 ) ) ;
#2058=CARTESIAN_POINT ( 'NONE',  ( 0.05219959533937995610, -21.53943276465977519, 90.00109039468567573 ) ) ;
#2059=CARTESIAN_POINT ( 'NONE',  ( -4.379528057220086978, -16.55341960407618274, 29.79275706135234358 ) ) ;
#2060=CARTESIAN_POINT ( 'NONE',  ( 5.049401038298161559, -19.05341960407611168, 92.70724293864769550 ) ) ;
#2062=CARTESIAN_POINT ( 'NONE',  ( 19.03943276465977164, -0.05219959533909143690, 73.74890960531435269 ) ) ;
#2063=CARTESIAN_POINT ( 'NONE',  ( -17.97161686094259636, 5.499999999999976907, 95.99637206859250682 ) ) ;
#2064=CARTESIAN_POINT ( 'NONE',  ( -19.02544592524334988, -5.153800228976617603, 88.95942372801897591 ) ) ;
#2065=CARTESIAN_POINT ( 'NONE',  ( 19.03943276465977164, -0.05219959533909143690, 103.7489096053143669 ) ) ;
#2066=CARTESIAN_POINT ( 'NONE',  ( -15.72974639402176322, -15.80617190586768395, 104.3760903946856899 ) ) ;
#2067=CARTESIAN_POINT ( 'NONE',  ( 8.314922557960818139, 14.29746914071049879, 99.58224293864770971 ) ) ;
#2069=CARTESIAN_POINT ( 'NONE',  ( -10.81492255796078084, -18.62759615963271287, 52.08224293864768839 ) ) ;
#2070=CARTESIAN_POINT ( 'NONE',  ( 18.67979575497178502, 10.72451020669898547, 39.16557627198102409 ) ) ;
#2071=CARTESIAN_POINT ( 'NONE',  ( -12.14591786802309592, -12.06949235617757132, 111.8739096053143669 ) ) ;
#2073=CARTESIAN_POINT ( 'NONE',  ( -9.564922557961040184, 16.46253265017147172, 62.91775706135233293 ) ) ;
#2074=CARTESIAN_POINT ( 'NONE',  ( 4.379528057220339221, -16.55341960407611168, 37.70724293864769550 ) ) ;
#2075=CARTESIAN_POINT ( 'NONE',  ( 0.05219959533907565091, 21.53943276465977519, 24.99890960531435624 ) ) ;
#2076=CARTESIAN_POINT ( 'NONE',  ( -0.05219959533937732626, 21.53943276465977519, 82.50109039468568994 ) ) ;
#2077=CARTESIAN_POINT ( 'NONE',  ( -18.67979575497178146, -10.72451020669898902, 76.66557627198103830 ) ) ;
#2078=CARTESIAN_POINT ( 'NONE',  ( -10.72451020669870658, -18.67979575497194134, 49.58442372801901143 ) ) ;
#2079=CARTESIAN_POINT ( 'NONE',  ( 15.72974639402199770, -15.80617190586745480, 93.12390960531436690 ) ) ;
#2080=CARTESIAN_POINT ( 'NONE',  ( 18.67979575497194134, -10.72451020669871369, 50.83442372801901143 ) ) ;
#2081=CARTESIAN_POINT ( 'NONE',  ( 19.03943276465977164, -0.05219959533909143690, 23.74890960531435269 ) ) ;
#2082=CARTESIAN_POINT ( 'NONE',  ( 19.05341960407611168, 5.049401038298154454, 83.95724293864766707 ) ) ;
#2083=CARTESIAN_POINT ( 'NONE',  ( -16.55341960407617563, 4.379528057220093196, 83.54275706135234714 ) ) ;
#2084=CARTESIAN_POINT ( 'NONE',  ( -16.53943276465976808, 0.05219959533911058130, 111.2489096053143669 ) ) ;
#2085=CARTESIAN_POINT ( 'NONE',  ( 19.05341960407611168, 5.049401038298154454, 108.9572429386477097 ) ) ;
#2086=CARTESIAN_POINT ( 'NONE',  ( 4.483927247898545687, 16.52544592524342804, 59.79057627198103120 ) ) ;
#2087=CARTESIAN_POINT ( 'NONE',  ( -0.05219959533910754901, -16.53943276465976808, 27.49890960531435269 ) ) ;
#2088=CARTESIAN_POINT ( 'NONE',  ( -5.049401038298153566, 19.05341960407611168, 70.20724293864769550 ) ) ;
#2089=CARTESIAN_POINT ( 'NONE',  ( 13.97604488694527802, 13.89961937509977652, 34.37390960531436690 ) ) ;
#2090=CARTESIAN_POINT ( 'NONE',  ( -21.53943276465977519, 0.05219959533907696930, 51.24890960531436690 ) ) ;
#2091=CARTESIAN_POINT ( 'NONE',  ( -9.474510206698720793, -16.51473224551083518, 34.58442372801899722 ) ) ;
#2092=CARTESIAN_POINT ( 'NONE',  ( -17.49999999999998579, -5.500000000000015099, 41.28230962303565832 ) ) ;
#2093=CARTESIAN_POINT ( 'NONE',  ( -8.314922557960811034, -14.29746914071050412, 32.08224293864769550 ) ) ;
#2094=CARTESIAN_POINT ( 'NONE',  ( 13.89961937509977652, -13.97604488694527269, 103.1239096053143527 ) ) ;
#2095=CARTESIAN_POINT ( 'NONE',  ( 21.52544592524334988, 5.823673210054432836, 66.45942372801903275 ) ) ;
#2096=CARTESIAN_POINT ( 'NONE',  ( 17.78921395495479629, -1.086248361263877582, 37.49999999999999289 ) ) ;
#2097=CARTESIAN_POINT ( 'NONE',  ( 16.53943276465976808, 0.05219959533934440121, 56.25109039468568284 ) ) ;
#2098=CARTESIAN_POINT ( 'NONE',  ( 19.02544592524334988, 5.153800228976608722, 56.45942372801898301 ) ) ;
#2099=CARTESIAN_POINT ( 'NONE',  ( -14.34966873604960291, -8.224510206698953496, 36.66557627198103120 ) ) ;
#2100=CARTESIAN_POINT ( 'NONE',  ( 16.79531203550644136, -7.028104445595668714, 51.24755011779560476 ) ) ;
#2101=CARTESIAN_POINT ( 'NONE',  ( 14.34966873604972726, -8.224510206698740333, 105.8344237280190328 ) ) ;
#2102=CARTESIAN_POINT ( 'NONE',  ( 5.153800228976335163, 19.02544592524342804, 39.79057627198100988 ) ) ;
#2103=CARTESIAN_POINT ( 'NONE',  ( -13.97604488694527625, -13.89961937509977652, 66.87390960531436690 ) ) ;
#2104=CARTESIAN_POINT ( 'NONE',  ( 9.564922557960805705, 16.46253265017160317, 29.58224293864769550 ) ) ;
#2105=CARTESIAN_POINT ( 'NONE',  ( 21.53943276465977519, 0.05219959533937863772, 26.25109039468567573 ) ) ;
#2106=CARTESIAN_POINT ( 'NONE',  ( -19.05341960407611168, -5.049401038298163336, 61.45724293864769550 ) ) ;
#2107=CARTESIAN_POINT ( 'NONE',  ( 16.51473224551069308, 9.474510206698969483, 114.1655762719810241 ) ) ;
#2108=CARTESIAN_POINT ( 'NONE',  ( 13.89961937509977652, -13.97604488694527269, 43.12390960531434558 ) ) ;
#2109=CARTESIAN_POINT ( 'NONE',  ( -21.55341960407610458, -5.719274019375992779, 26.45724293864768839 ) ) ;
#2110=CARTESIAN_POINT ( 'NONE',  ( -21.53943276465977519, -0.05219959533937600094, 53.75109039468568994 ) ) ;
#2111=CARTESIAN_POINT ( 'NONE',  ( 16.46253265017160672, -9.564922557960803928, 23.33224293864769194 ) ) ;
#2112=CARTESIAN_POINT ( 'NONE',  ( 21.52544592524344225, -5.823673210054117533, 33.54057627198102409 ) ) ;
#2113=CARTESIAN_POINT ( 'NONE',  ( -4.483927247898782831, 16.52544592524335698, 72.70942372801901854 ) ) ;
#2114=CARTESIAN_POINT ( 'NONE',  ( -15.80617190586768217, 15.72974639402176855, 103.1260903946856757 ) ) ;
#2115=CARTESIAN_POINT ( 'NONE',  ( 14.34966873604972726, -8.224510206698740333, 70.83442372801901854 ) ) ;
#2116=CARTESIAN_POINT ( 'NONE',  ( -19.03943276465977164, 0.05219959533909376836, 101.2489096053143669 ) ) ;
#2117=CARTESIAN_POINT ( 'NONE',  ( -14.34966873604972548, 8.224510206698743886, 48.33442372801902565 ) ) ;
#2118=CARTESIAN_POINT ( 'NONE',  ( 8.224510206698742110, 14.34966873604972548, 32.08442372801901854 ) ) ;
#2119=CARTESIAN_POINT ( 'NONE',  ( 8.224510206698742110, 14.34966873604972548, 102.0844237280190185 ) ) ;
#2120=CARTESIAN_POINT ( 'NONE',  ( -15.80617190586768217, 15.72974639402176855, 48.12609039468568284 ) ) ;
#2121=CARTESIAN_POINT ( 'NONE',  ( -19.02544592524334988, -5.153800228976617603, 108.9594237280189759 ) ) ;
#2122=CARTESIAN_POINT ( 'NONE',  ( -21.55341960407610458, -5.719274019375992779, 111.4572429386476813 ) ) ;
#2123=CARTESIAN_POINT ( 'NONE',  ( 4.379528057220339221, -16.55341960407611168, 102.7072429386476955 ) ) ;
#2124=CARTESIAN_POINT ( 'NONE',  ( 5.049401038297881783, 19.05341960407617563, 107.2927570613523187 ) ) ;
#2125=CARTESIAN_POINT ( 'NONE',  ( -16.53943276465976808, -0.05219959533934237506, 83.75109039468568994 ) ) ;
#2127=CARTESIAN_POINT ( 'NONE',  ( -16.51473224551082808, 9.474510206698731452, 88.33442372801900433 ) ) ;
#2129=CARTESIAN_POINT ( 'NONE',  ( -16.52544592524342804, 4.483927247898546575, 41.04057627198103120 ) ) ;
#2130=CARTESIAN_POINT ( 'NONE',  ( -4.483927247898539470, -16.52544592524342804, 47.29057627198103120 ) ) ;
#2131=CARTESIAN_POINT ( 'NONE',  ( 12.06949235617757843, -12.14591786802309237, 108.1239096053143811 ) ) ;
#2132=CARTESIAN_POINT ( 'NONE',  ( 13.89961937509957401, 13.97604488694547697, 46.87609039468565442 ) ) ;
#2133=CARTESIAN_POINT ( 'NONE',  ( -17.49999999999998579, 5.500000000000031974, 90.79690382534171533 ) ) ;
#2134=CARTESIAN_POINT ( 'NONE',  ( 0.05219959533937995610, -21.53943276465977519, 40.00109039468567573 ) ) ;
#2135=CARTESIAN_POINT ( 'NONE',  ( 8.314922557961029526, -14.29746914071037800, 20.41775706135234714 ) ) ;
#2137=CARTESIAN_POINT ( 'NONE',  ( -13.89961937509977652, 13.97604488694528158, 105.6239096053143527 ) ) ;
#2138=CARTESIAN_POINT ( 'NONE',  ( -10.72451020669898014, 18.67979575497178502, 60.41557627198102409 ) ) ;
#2139=CARTESIAN_POINT ( 'NONE',  ( 16.51473224551069308, 9.474510206698969483, 84.16557627198102409 ) ) ;
#2140=CARTESIAN_POINT ( 'NONE',  ( -21.52544592524343514, 5.823673210054127303, 51.04057627198103120 ) ) ;
#2141=CARTESIAN_POINT ( 'NONE',  ( 16.52544592524342804, -4.483927247898539470, 113.5405762719810383 ) ) ;
#2142=CARTESIAN_POINT ( 'NONE',  ( -9.474510206698964154, 16.51473224551069663, 70.41557627198102409 ) ) ;
#2144=CARTESIAN_POINT ( 'NONE',  ( -0.05219959533909027116, -19.03943276465977164, 32.49890960531435979 ) ) ;
#2146=CARTESIAN_POINT ( 'NONE',  ( 18.67979575497194134, -10.72451020669871369, 40.83442372801901854 ) ) ;
#2147=CARTESIAN_POINT ( 'NONE',  ( 18.62759615963255655, 10.81492255796105972, 76.66775706135234714 ) ) ;
#2148=CARTESIAN_POINT ( 'NONE',  ( -16.52544592524335698, -4.483927247898792601, 93.95942372801903275 ) ) ;
#2149=CARTESIAN_POINT ( 'NONE',  ( 21.52544592524334988, 5.823673210054432836, 31.45942372801901854 ) ) ;
#2150=CARTESIAN_POINT ( 'NONE',  ( -0.05219959533937732626, 21.53943276465977519, 32.50109039468568284 ) ) ;
#2151=CARTESIAN_POINT ( 'NONE',  ( 9.564922557961047289, -16.46253265017146816, 70.41775706135233293 ) ) ;
#2152=CARTESIAN_POINT ( 'NONE',  ( 16.51473224551069308, 9.474510206698969483, 79.16557627198103830 ) ) ;
#2153=CARTESIAN_POINT ( 'NONE',  ( 21.53943276465977519, 0.05219959533937863772, 86.25109039468568994 ) ) ;
#2154=CARTESIAN_POINT ( 'NONE',  ( 10.72451020669898902, -18.67979575497178502, 87.91557627198103830 ) ) ;
#2155=CARTESIAN_POINT ( 'NONE',  ( -12.06949235617756955, 12.14591786802309770, 60.62390960531437401 ) ) ;
#2156=CARTESIAN_POINT ( 'NONE',  ( -21.53943276465977519, -0.05219959533937600094, 98.75109039468568994 ) ) ;
#2157=CARTESIAN_POINT ( 'NONE',  ( 8.314922557960818139, 14.29746914071049879, 79.58224293864769550 ) ) ;
#2158=CARTESIAN_POINT ( 'NONE',  ( -9.564922557960796823, -16.46253265017161027, 27.08224293864769550 ) ) ;
#2159=CARTESIAN_POINT ( 'NONE',  ( -13.89961937509957401, -13.97604488694547875, 74.37609039468566152 ) ) ;
#2160=CARTESIAN_POINT ( 'NONE',  ( -14.34966873604960291, -8.224510206698953496, 31.66557627198102054 ) ) ;
#2161=CARTESIAN_POINT ( 'NONE',  ( -18.67979575497193778, 10.72451020669871902, 88.33442372801901854 ) ) ;
#2162=CARTESIAN_POINT ( 'NONE',  ( 13.89961937509977652, -13.97604488694527269, 88.12390960531438111 ) ) ;
#2163=CARTESIAN_POINT ( 'NONE',  ( 13.97604488694548053, -13.89961937509957401, 60.62609039468564731 ) ) ;
#2164=CARTESIAN_POINT ( 'NONE',  ( -21.55341960407610458, -5.719274019375992779, 71.45724293864769550 ) ) ;
#2165=CARTESIAN_POINT ( 'NONE',  ( -21.55341960407610458, -5.719274019375992779, 111.4572429386476813 ) ) ;
#2166=CARTESIAN_POINT ( 'NONE',  ( -19.02544592524334988, -5.153800228976617603, 108.9594237280189759 ) ) ;
#2167=CARTESIAN_POINT ( 'NONE',  ( 14.29746914071037800, 8.314922557961029526, 81.66775706135236135 ) ) ;
#2168=CARTESIAN_POINT ( 'NONE',  ( 17.31747979337950127, 6.344076630961019703, 63.87944868065186199 ) ) ;
#2169=CARTESIAN_POINT ( 'NONE',  ( -5.719274019375665041, -21.55341960407619695, 24.79275706135235779 ) ) ;
#2170=CARTESIAN_POINT ( 'NONE',  ( -12.14591786802309592, -12.06949235617757132, 106.8739096053143811 ) ) ;
#2172=CARTESIAN_POINT ( 'NONE',  ( -0.05219959533934338120, 16.53943276465976808, 32.50109039468568284 ) ) ;
#2173=CARTESIAN_POINT ( 'NONE',  ( -15.80617190586745835, -15.72974639402198527, 56.87390960531436690 ) ) ;
#2174=CARTESIAN_POINT ( 'NONE',  ( -12.06949235617739369, -12.14591786802326823, 109.3760903946857042 ) ) ;
#2175=CARTESIAN_POINT ( 'NONE',  ( 16.55341960407618274, -4.379528057220086978, 36.04275706135234714 ) ) ;
#2176=CARTESIAN_POINT ( 'NONE',  ( -9.564922557960796823, -16.46253265017161027, 37.08224293864768839 ) ) ;
#2177=CARTESIAN_POINT ( 'NONE',  ( -8.314922557961024197, 14.29746914071037800, 77.91775706135231871 ) ) ;
#2178=CARTESIAN_POINT ( 'NONE',  ( 13.97604488694548053, -13.89961937509957401, 75.62609039468564731 ) ) ;
#2179=CARTESIAN_POINT ( 'NONE',  ( 15.80617190586746368, 15.72974639402197994, 74.37390960531436690 ) ) ;
#2180=CARTESIAN_POINT ( 'NONE',  ( 16.53943276465976808, 0.05219959533934440121, 101.2510903946856757 ) ) ;
#2181=CARTESIAN_POINT ( 'NONE',  ( -18.67979575497193778, 10.72451020669871902, 88.33442372801901854 ) ) ;
#2182=CARTESIAN_POINT ( 'NONE',  ( -15.72974639402197994, 15.80617190586746368, 55.62390960531436690 ) ) ;
#2183=CARTESIAN_POINT ( 'NONE',  ( -5.823673210054116645, -21.52544592524344225, 47.29057627198103120 ) ) ;
#2184=CARTESIAN_POINT ( 'NONE',  ( -16.55341960407617563, 4.379528057220093196, 73.54275706135234714 ) ) ;
#2185=CARTESIAN_POINT ( 'NONE',  ( 5.823673210054125526, 21.52544592524343514, 49.79057627198102409 ) ) ;
#2186=ORIENTED_EDGE ( 'NONE', *, *, #107130, .T. ) ;
#2187=CARTESIAN_POINT ( 'NONE',  ( -5.153800228976328057, -19.02544592524343514, 112.2905762719810099 ) ) ;
#2189=CARTESIAN_POINT ( 'NONE',  ( 9.564922557960805705, 16.46253265017160317, 24.58224293864769194 ) ) ;
#2190=CARTESIAN_POINT ( 'NONE',  ( -21.52544592524343514, 5.823673210054127303, 56.04057627198102409 ) ) ;
#2191=CARTESIAN_POINT ( 'NONE',  ( 16.55341960407618274, -4.379528057220086978, 101.0427570613523756 ) ) ;
#2192=CARTESIAN_POINT ( 'NONE',  ( 5.823673210054444382, -21.52544592524334988, 40.20942372801901854 ) ) ;
#2193=CARTESIAN_POINT ( 'NONE',  ( -5.153800228976607833, 19.02544592524334988, 97.70942372801900433 ) ) ;
#2194=CARTESIAN_POINT ( 'NONE',  ( 4.483927247898545687, 16.52544592524342804, 114.7905762719810383 ) ) ;
#2195=CARTESIAN_POINT ( 'NONE',  ( 16.51473224551083163, -9.474510206698727899, 105.8344237280190043 ) ) ;
#2197=CARTESIAN_POINT ( 'NONE',  ( 13.97604488694527802, 13.89961937509977652, 39.37390960531435269 ) ) ;
#2199=CARTESIAN_POINT ( 'NONE',  ( 5.049401038298161559, -19.05341960407611168, 87.70724293864769550 ) ) ;
#2200=CARTESIAN_POINT ( 'NONE',  ( 8.224510206698742110, 14.34966873604972548, 72.08442372801899012 ) ) ;
#2201=CARTESIAN_POINT ( 'NONE',  ( -9.474510206698720793, -16.51473224551083518, 84.58442372801900433 ) ) ;
#2202=CARTESIAN_POINT ( 'NONE',  ( 5.049401038297881783, 19.05341960407617563, 22.29275706135233648 ) ) ;
#2203=CARTESIAN_POINT ( 'NONE',  ( -21.53943276465977519, 0.05219959533907696930, 56.24890960531436690 ) ) ;
#2204=CARTESIAN_POINT ( 'NONE',  ( -14.34966873604972548, 8.224510206698743886, 88.33442372801901854 ) ) ;
#2205=CARTESIAN_POINT ( 'NONE',  ( 19.03943276465977164, 0.05219959533936151252, 76.25109039468566152 ) ) ;
#2206=CARTESIAN_POINT ( 'NONE',  ( 0.05219959533909260263, 19.03943276465977164, 39.99890960531436690 ) ) ;
#2207=CARTESIAN_POINT ( 'NONE',  ( -5.049401038298153566, 19.05341960407611168, 75.20724293864769550 ) ) ;
#2208=CARTESIAN_POINT ( 'NONE',  ( -10.72451020669870658, -18.67979575497194134, 54.58442372801901143 ) ) ;
#2209=CARTESIAN_POINT ( 'NONE',  ( -13.89961937509977652, 13.97604488694528158, 45.62390960531433848 ) ) ;
#2210=CARTESIAN_POINT ( 'NONE',  ( -13.89961937509957401, -13.97604488694547875, 74.37609039468566152 ) ) ;
#2212=CARTESIAN_POINT ( 'NONE',  ( 0.05219959533909260263, 19.03943276465977164, 109.9989096053143669 ) ) ;
#2213=CARTESIAN_POINT ( 'NONE',  ( -12.14591786802309592, -12.06949235617757132, 66.87390960531436690 ) ) ;
#2214=CARTESIAN_POINT ( 'NONE',  ( 5.823673210054125526, 21.52544592524343514, 59.79057627198103120 ) ) ;
#2216=CARTESIAN_POINT ( 'NONE',  ( 19.03943276465977164, 0.05219959533936151252, 31.25109039468566863 ) ) ;
#2217=CARTESIAN_POINT ( 'NONE',  ( 5.049401038298161559, -19.05341960407611168, 57.70724293864769550 ) ) ;
#2218=CARTESIAN_POINT ( 'NONE',  ( 19.02544592524343514, -5.153800228976328945, 78.54057627198099567 ) ) ;
#2219=CARTESIAN_POINT ( 'NONE',  ( -4.379528057220086978, -16.55341960407618274, 44.79275706135234714 ) ) ;
#2221=CARTESIAN_POINT ( 'NONE',  ( -17.40805194822031510, 6.112264579159313982, 110.8337127251061247 ) ) ;
#2222=CARTESIAN_POINT ( 'NONE',  ( -14.29746914071037622, -8.314922557961029526, 89.16775706135236135 ) ) ;
#2223=CARTESIAN_POINT ( 'NONE',  ( -17.49999999999999645, 5.499999999999992895, 78.71769037696437010 ) ) ;
#2224=CARTESIAN_POINT ( 'NONE',  ( 0.05219959533934541429, -16.53943276465976808, 65.00109039468568994 ) ) ;
#2225=CARTESIAN_POINT ( 'NONE',  ( -16.52544592524335698, -4.483927247898792601, 38.95942372801901854 ) ) ;
#2226=CARTESIAN_POINT ( 'NONE',  ( 9.564922557960805705, 16.46253265017160317, 59.58224293864769550 ) ) ;
#2228=CARTESIAN_POINT ( 'NONE',  ( 21.55341960407619695, -5.719274019375665929, 56.04275706135235424 ) ) ;
#2229=CARTESIAN_POINT ( 'NONE',  ( 9.564922557961047289, -16.46253265017146816, 60.41775706135233293 ) ) ;
#2230=CARTESIAN_POINT ( 'NONE',  ( 0.05219959533937995610, -21.53943276465977519, 105.0010903946856757 ) ) ;
#2231=CARTESIAN_POINT ( 'NONE',  ( -19.02544592524342804, 5.153800228976336051, 36.04057627198100988 ) ) ;
#2233=CARTESIAN_POINT ( 'NONE',  ( 15.80617190586746368, 15.72974639402197994, 49.37390960531436690 ) ) ;
#2234=CARTESIAN_POINT ( 'NONE',  ( -19.05341960407611168, -5.049401038298163336, 111.4572429386476671 ) ) ;
#2235=CARTESIAN_POINT ( 'NONE',  ( -4.379528057220328563, 16.55341960407611168, 105.2072429386477097 ) ) ;
#2236=CARTESIAN_POINT ( 'NONE',  ( 16.53943276465976808, 0.05219959533934440121, 36.25109039468567573 ) ) ;
#2237=CARTESIAN_POINT ( 'NONE',  ( -16.55341960407611168, -4.379528057220339221, 31.45724293864769550 ) ) ;
#2239=CARTESIAN_POINT ( 'NONE',  ( -18.67979575497193778, 10.72451020669871902, 23.33442372801901499 ) ) ;
#2240=CARTESIAN_POINT ( 'NONE',  ( -4.379528057220328563, 16.55341960407611168, 40.20724293864769550 ) ) ;
#2241=CARTESIAN_POINT ( 'NONE',  ( 5.049401038298161559, -19.05341960407611168, 107.7072429386476955 ) ) ;
#2242=CARTESIAN_POINT ( 'NONE',  ( -13.97604488694547697, 13.89961937509957934, 113.1260903946856757 ) ) ;
#2243=CARTESIAN_POINT ( 'NONE',  ( -19.03943276465977164, -0.05219959533935918106, 23.75109039468566152 ) ) ;
#2244=CARTESIAN_POINT ( 'NONE',  ( 4.483927247898545687, 16.52544592524342804, 34.79057627198103120 ) ) ;
#2245=CARTESIAN_POINT ( 'NONE',  ( 21.53943276465977519, -0.05219959533907433946, 103.7489096053143669 ) ) ;
#2246=CARTESIAN_POINT ( 'NONE',  ( 18.62759615963271287, -10.81492255796078972, 63.33224293864770260 ) ) ;
#2247=CARTESIAN_POINT ( 'NONE',  ( -13.89961937509977652, 13.97604488694528158, 70.62390960531432427 ) ) ;
#2248=CARTESIAN_POINT ( 'NONE',  ( -12.14591786802309592, -12.06949235617757132, 51.87390960531437401 ) ) ;
#2249=CARTESIAN_POINT ( 'NONE',  ( 19.03943276465977164, -0.05219959533909143690, 93.74890960531435269 ) ) ;
#2250=B_SPLINE_CURVE_WITH_KNOTS ( 'NONE', 3,
 ( #76551, #27097, #62361, #16875, #170556, #81491 ),
 .UNSPECIFIED., .F., .F.,
 ( 4, 2, 4 ),
 ( 0.003989672132298188560, 0.004372778065220606601, 0.004755883998143024642 ),
 .UNSPECIFIED. ) ;
#2251=CARTESIAN_POINT ( 'NONE',  ( 0.05219959533909260263, 19.03943276465977164, 79.99890960531436690 ) ) ;
#2252=CARTESIAN_POINT ( 'NONE',  ( 19.02544592524334988, 5.153800228976608722, 41.45942372801900433 ) ) ;
#2253=CARTESIAN_POINT ( 'NONE',  ( -15.72974639402197994, 15.80617190586746368, 90.62390960531436690 ) ) ;
#2254=CARTESIAN_POINT ( 'NONE',  ( 14.29746914071049879, -8.314922557960816363, 93.33224293864769550 ) ) ;
#2255=CARTESIAN_POINT ( 'NONE',  ( -5.823673210054431948, 21.52544592524334988, 32.70942372801900433 ) ) ;
#2257=CARTESIAN_POINT ( 'NONE',  ( 16.55341960407611168, 4.379528057220329451, 23.95724293864769550 ) ) ;
#2258=CARTESIAN_POINT ( 'NONE',  ( 0.05219959533909260263, 19.03943276465977164, 29.99890960531435979 ) ) ;
#2259=CARTESIAN_POINT ( 'NONE',  ( 16.46253265017160672, -9.564922557960803928, 88.33224293864769550 ) ) ;
#2260=CARTESIAN_POINT ( 'NONE',  ( -21.55341960407610458, -5.719274019375992779, 61.45724293864770260 ) ) ;
#2262=CARTESIAN_POINT ( 'NONE',  ( -5.049401038298153566, 19.05341960407611168, 25.20724293864768484 ) ) ;
#2263=CARTESIAN_POINT ( 'NONE',  ( 5.719274019375991003, -21.55341960407610458, 57.70724293864770260 ) ) ;
#2264=CARTESIAN_POINT ( 'NONE',  ( 21.52544592524334988, 5.823673210054432836, 76.45942372801901854 ) ) ;
#2266=CARTESIAN_POINT ( 'NONE',  ( -8.224510206698735004, -14.34966873604973081, 69.58442372801900433 ) ) ;
#2267=CARTESIAN_POINT ( 'NONE',  ( -9.474510206698964154, 16.51473224551069663, 55.41557627198103120 ) ) ;
#2268=CARTESIAN_POINT ( 'NONE',  ( -9.474510206698964154, 16.51473224551069663, 70.41557627198102409 ) ) ;
#2270=CARTESIAN_POINT ( 'NONE',  ( -21.53943276465977519, -0.05219959533937600094, 113.7510903946856757 ) ) ;
#2271=CARTESIAN_POINT ( 'NONE',  ( 16.55341960407618274, -4.379528057220086978, 81.04275706135236135 ) ) ;
#2272=CARTESIAN_POINT ( 'NONE',  ( -21.55341960407619339, 5.719274019375674811, 103.5427570613523613 ) ) ;
#2273=CARTESIAN_POINT ( 'NONE',  ( 0.05219959533909260263, 19.03943276465977164, 59.99890960531436690 ) ) ;
#2274=CARTESIAN_POINT ( 'NONE',  ( 18.67979575497178502, 10.72451020669898547, 29.16557627198103120 ) ) ;
#2275=CARTESIAN_POINT ( 'NONE',  ( -9.564922557961040184, 16.46253265017147172, 102.9177570613523329 ) ) ;
#2276=CARTESIAN_POINT ( 'NONE',  ( 5.823673210054444382, -21.52544592524334988, 85.20942372801901854 ) ) ;
#2277=CARTESIAN_POINT ( 'NONE',  ( -8.314922557961024197, 14.29746914071037800, 42.91775706135235424 ) ) ;
#2278=CARTESIAN_POINT ( 'NONE',  ( -21.55341960407610458, -5.719274019375992779, 101.4572429386476955 ) ) ;
#2279=CARTESIAN_POINT ( 'NONE',  ( -19.03943276465977164, -0.05219959533935918106, 98.75109039468567573 ) ) ;
#2280=CARTESIAN_POINT ( 'NONE',  ( -16.46253265017160317, 9.564922557960807481, 80.83224293864769550 ) ) ;
#2281=CARTESIAN_POINT ( 'NONE',  ( 16.46253265017146816, 9.564922557961045513, 106.6677570613523471 ) ) ;
#2282=CARTESIAN_POINT ( 'NONE',  ( 0.05219959533909260263, 19.03943276465977164, 34.99890960531435979 ) ) ;
#2284=CARTESIAN_POINT ( 'NONE',  ( 0.05219959533934541429, -16.53943276465976808, 20.00109039468568639 ) ) ;
#2285=CARTESIAN_POINT ( 'NONE',  ( -16.52544592524342804, 4.483927247898546575, 61.04057627198103120 ) ) ;
#2286=CARTESIAN_POINT ( 'NONE',  ( 0.05219959533934541429, -16.53943276465976808, 75.00109039468568994 ) ) ;
#2287=CARTESIAN_POINT ( 'NONE',  ( 0.05219959533937995610, -21.53943276465977519, 30.00109039468568284 ) ) ;
#2288=CARTESIAN_POINT ( 'NONE',  ( -13.97604488694527625, -13.89961937509977652, 56.87390960531434558 ) ) ;
#2289=CARTESIAN_POINT ( 'NONE',  ( 5.049401038298161559, -19.05341960407611168, 67.70724293864769550 ) ) ;
#2290=CARTESIAN_POINT ( 'NONE',  ( -16.53943276465976808, -0.05219959533934237506, 73.75109039468567573 ) ) ;
#2293=CARTESIAN_POINT ( 'NONE',  ( 5.049401038297881783, 19.05341960407617563, 22.29275706135233648 ) ) ;
#2295=CARTESIAN_POINT ( 'NONE',  ( 9.564922557960805705, 16.46253265017160317, 29.58224293864769550 ) ) ;
#2297=CARTESIAN_POINT ( 'NONE',  ( 16.55341960407618274, -4.379528057220086978, 26.04275706135235779 ) ) ;
#2298=CARTESIAN_POINT ( 'NONE',  ( 19.03943276465977164, 0.05219959533936151252, 46.25109039468566863 ) ) ;
#2299=CARTESIAN_POINT ( 'NONE',  ( 12.06949235617739724, 12.14591786802326823, 41.87609039468568284 ) ) ;
#2300=CARTESIAN_POINT ( 'NONE',  ( 19.02544592524343514, -5.153800228976328945, 48.54057627198103120 ) ) ;
#2301=CARTESIAN_POINT ( 'NONE',  ( -13.97604488694527625, -13.89961937509977652, 101.8739096053143811 ) ) ;
#2302=CARTESIAN_POINT ( 'NONE',  ( -0.05219959533909027116, -19.03943276465977164, 57.49890960531435979 ) ) ;
#2303=CARTESIAN_POINT ( 'NONE',  ( -5.719274019375978568, 21.55341960407610458, 90.20724293864770971 ) ) ;
#2304=CARTESIAN_POINT ( 'NONE',  ( -19.05341960407611168, -5.049401038298163336, 76.45724293864769550 ) ) ;
#2305=CARTESIAN_POINT ( 'NONE',  ( -16.46253265017160317, 9.564922557960807481, 115.8322429386477097 ) ) ;
#2306=CARTESIAN_POINT ( 'NONE',  ( 16.46253265017160672, -9.564922557960803928, 63.33224293864769550 ) ) ;
#2308=CARTESIAN_POINT ( 'NONE',  ( -16.46253265017146816, -9.564922557961047289, 94.16775706135233293 ) ) ;
#2309=CARTESIAN_POINT ( 'NONE',  ( 19.05341960407617918, -5.049401038297876454, 21.04275706135232582 ) ) ;
#2310=CARTESIAN_POINT ( 'NONE',  ( -14.34966873604960291, -8.224510206698953496, 56.66557627198103830 ) ) ;
#2311=CARTESIAN_POINT ( 'NONE',  ( -10.72451020669870658, -18.67979575497194134, 89.58442372801901854 ) ) ;
#2312=CARTESIAN_POINT ( 'NONE',  ( -16.53943276465976808, 0.05219959533911058130, 116.2489096053143669 ) ) ;
#2313=CARTESIAN_POINT ( 'NONE',  ( -12.14591786802309592, -12.06949235617757132, 26.87390960531435979 ) ) ;
#2314=CARTESIAN_POINT ( 'NONE',  ( 21.52544592524334988, 5.823673210054432836, 91.45942372801901854 ) ) ;
#2315=CARTESIAN_POINT ( 'NONE',  ( 9.564922557960805705, 16.46253265017160317, 74.58224293864769550 ) ) ;
#2316=CARTESIAN_POINT ( 'NONE',  ( -10.72451020669870658, -18.67979575497194134, 44.58442372801901854 ) ) ;
#2317=CARTESIAN_POINT ( 'NONE',  ( 19.03943276465977164, -0.05219959533909143690, 78.74890960531436690 ) ) ;
#2318=CARTESIAN_POINT ( 'NONE',  ( 4.483927247898545687, 16.52544592524342804, 89.79057627198103830 ) ) ;
#2319=CARTESIAN_POINT ( 'NONE',  ( 4.483927247898545687, 16.52544592524342804, 59.79057627198103120 ) ) ;
#2320=CARTESIAN_POINT ( 'NONE',  ( -21.53943276465977519, 0.05219959533907696930, 71.24890960531435269 ) ) ;
#2321=CARTESIAN_POINT ( 'NONE',  ( 19.03943276465977164, -0.05219959533909143690, 78.74890960531436690 ) ) ;
#2322=CARTESIAN_POINT ( 'NONE',  ( -21.53943276465977519, 0.05219959533907696930, 91.24890960531436690 ) ) ;
#2323=CARTESIAN_POINT ( 'NONE',  ( 0.05219959533936267826, -19.03943276465977164, 80.00109039468567573 ) ) ;
#2324=CARTESIAN_POINT ( 'NONE',  ( 13.89961937509957579, 13.97604488694547520, 36.87609039468566863 ) ) ;
#2325=CARTESIAN_POINT ( 'NONE',  ( 12.14591786802309770, 12.06949235617756955, 79.37390960531436690 ) ) ;
#2327=CARTESIAN_POINT ( 'NONE',  ( -13.89961937509977652, 13.97604488694528158, 60.62390960531436690 ) ) ;
#2328=CARTESIAN_POINT ( 'NONE',  ( -5.823673210054116645, -21.52544592524344225, 72.29057627198102409 ) ) ;
#2329=CARTESIAN_POINT ( 'NONE',  ( 16.79531203550645202, -7.028104445595743321, 26.24755011779557989 ) ) ;
#2330=CARTESIAN_POINT ( 'NONE',  ( 8.314922557961029526, -14.29746914071037800, 110.4177570613523756 ) ) ;
#2332=CARTESIAN_POINT ( 'NONE',  ( 19.05341960407617918, -5.049401038297876454, 106.0427570613523471 ) ) ;
#2333=CARTESIAN_POINT ( 'NONE',  ( 4.379528057220339221, -16.55341960407611168, 87.70724293864769550 ) ) ;
#2334=CARTESIAN_POINT ( 'NONE',  ( -17.49999999999998579, 4.640572885337610920, 35.63788164548841308 ) ) ;
#2335=CARTESIAN_POINT ( 'NONE',  ( 5.153800228976335163, 19.02544592524342804, 79.79057627198102409 ) ) ;
#2336=CARTESIAN_POINT ( 'NONE',  ( -13.97604488694527625, -13.89961937509977652, 31.87390960531435979 ) ) ;
#2337=CARTESIAN_POINT ( 'NONE',  ( 0.05219959533910956823, 16.53943276465976808, 64.99890960531435269 ) ) ;
#2338=CARTESIAN_POINT ( 'NONE',  ( -19.03943276465977164, 0.05219959533909376836, 96.24890960531436690 ) ) ;
#2339=CARTESIAN_POINT ( 'NONE',  ( 9.564922557961047289, -16.46253265017146816, 95.41775706135233293 ) ) ;
#2340=CARTESIAN_POINT ( 'NONE',  ( -19.05341960407611168, -5.049401038298163336, 61.45724293864769550 ) ) ;
#2341=CARTESIAN_POINT ( 'NONE',  ( 9.564922557960805705, 16.46253265017160317, 89.58224293864769550 ) ) ;
#2342=CARTESIAN_POINT ( 'NONE',  ( 5.719274019375991003, -21.55341960407610458, 77.70724293864770971 ) ) ;
#2343=CARTESIAN_POINT ( 'NONE',  ( 14.29746914071037800, 8.314922557961029526, 71.66775706135234714 ) ) ;
#2344=CARTESIAN_POINT ( 'NONE',  ( -19.05341960407617918, 5.049401038297883559, 108.5427570613523329 ) ) ;
#2345=CARTESIAN_POINT ( 'NONE',  ( 5.049401038298161559, -19.05341960407611168, 62.70724293864769550 ) ) ;
#2346=CARTESIAN_POINT ( 'NONE',  ( 18.67979575497178502, 10.72451020669898547, 74.16557627198102409 ) ) ;
#2347=CARTESIAN_POINT ( 'NONE',  ( -5.153800228976607833, 19.02544592524334988, 97.70942372801900433 ) ) ;
#2348=CARTESIAN_POINT ( 'NONE',  ( 16.55341960407611168, 4.379528057220329451, 38.95724293864768839 ) ) ;
#2349=CARTESIAN_POINT ( 'NONE',  ( 21.55341960407619695, -5.719274019375665929, 46.04275706135234714 ) ) ;
#2351=CARTESIAN_POINT ( 'NONE',  ( 16.52544592524335698, 4.483927247898782831, 76.45942372801901854 ) ) ;
#2352=CARTESIAN_POINT ( 'NONE',  ( -0.05219959533909027116, -19.03943276465977164, 112.4989096053143669 ) ) ;
#2353=CARTESIAN_POINT ( 'NONE',  ( -5.049401038298153566, 19.05341960407611168, 105.2072429386476813 ) ) ;
#2354=CARTESIAN_POINT ( 'NONE',  ( -16.18388926212235290, -7.379444403734648716, 35.43953151366154941 ) ) ;
#2355=CARTESIAN_POINT ( 'NONE',  ( -16.53943276465976808, -0.05219959533934237506, 98.75109039468568994 ) ) ;
#2356=CARTESIAN_POINT ( 'NONE',  ( -16.52544592524335698, -4.483927247898792601, 33.95942372801901143 ) ) ;
#2357=CARTESIAN_POINT ( 'NONE',  ( -16.46253265017160317, 9.564922557960807481, 50.83224293864770260 ) ) ;
#2358=CARTESIAN_POINT ( 'NONE',  ( -9.474510206698964154, 16.51473224551069663, 55.41557627198103120 ) ) ;
#2359=CARTESIAN_POINT ( 'NONE',  ( 16.51473224551069308, 9.474510206698969483, 59.16557627198102409 ) ) ;
#2360=CARTESIAN_POINT ( 'NONE',  ( 15.80617190586769283, -15.72974639402175789, 50.62609039468568994 ) ) ;
#2361=CARTESIAN_POINT ( 'NONE',  ( -16.55341960407617563, 4.379528057220093196, 58.54275706135235424 ) ) ;
#2362=CARTESIAN_POINT ( 'NONE',  ( 14.34966873604960469, 8.224510206698951720, 34.16557627198102409 ) ) ;
#2363=CARTESIAN_POINT ( 'NONE',  ( -19.03943276465977164, 0.05219959533909376836, 46.24890960531435979 ) ) ;
#2364=CARTESIAN_POINT ( 'NONE',  ( -13.97604488694527625, -13.89961937509977652, 36.87390960531436690 ) ) ;
#2365=CARTESIAN_POINT ( 'NONE',  ( 14.34966873604972726, -8.224510206698740333, 25.83442372801901499 ) ) ;
#2367=CARTESIAN_POINT ( 'NONE',  ( 16.51473224551083163, -9.474510206698727899, 80.83442372801899012 ) ) ;
#2368=CARTESIAN_POINT ( 'NONE',  ( 14.34966873604960469, 8.224510206698951720, 79.16557627198103830 ) ) ;
#2369=CARTESIAN_POINT ( 'NONE',  ( -13.97604488694527625, -13.89961937509977652, 56.87390960531434558 ) ) ;
#2370=CARTESIAN_POINT ( 'NONE',  ( 9.474510206698729675, 16.51473224551082808, 82.08442372801899012 ) ) ;
#2372=CARTESIAN_POINT ( 'NONE',  ( -5.719274019375665041, -21.55341960407619695, 79.79275706135236135 ) ) ;
#2373=CARTESIAN_POINT ( 'NONE',  ( -16.55341960407617563, 4.379528057220093196, 58.54275706135235424 ) ) ;
#2375=CARTESIAN_POINT ( 'NONE',  ( -18.62759615963270932, 10.81492255796079327, 55.83224293864770260 ) ) ;
#2376=CARTESIAN_POINT ( 'NONE',  ( -0.05219959533934338120, 16.53943276465976808, 37.50109039468568284 ) ) ;
#2377=CARTESIAN_POINT ( 'NONE',  ( 19.05341960407611168, 5.049401038298154454, 23.95724293864769194 ) ) ;
#2378=CARTESIAN_POINT ( 'NONE',  ( -13.97604488694547697, 13.89961937509957934, 23.12609039468565442 ) ) ;
#2379=CARTESIAN_POINT ( 'NONE',  ( 19.02544592524343514, -5.153800228976328945, 83.54057627198100988 ) ) ;
#2381=CARTESIAN_POINT ( 'NONE',  ( 9.474510206698971260, -16.51473224551069308, 47.91557627198102409 ) ) ;
#2383=CARTESIAN_POINT ( 'NONE',  ( 5.153800228976335163, 19.02544592524342804, 69.79057627198103830 ) ) ;
#2384=CARTESIAN_POINT ( 'NONE',  ( 17.50000000000000355, -5.068104630630377194, 113.2281840534003265 ) ) ;
#2385=CARTESIAN_POINT ( 'NONE',  ( 19.03943276465977164, 0.05219959533936151252, 21.25109039468565797 ) ) ;
#2386=CARTESIAN_POINT ( 'NONE',  ( 12.06949235617757843, -12.14591786802309237, 38.12390960531436690 ) ) ;
#2387=CARTESIAN_POINT ( 'NONE',  ( 19.05341960407611168, 5.049401038298154454, 43.95724293864769550 ) ) ;
#2388=CARTESIAN_POINT ( 'NONE',  ( -13.89961937509977652, 13.97604488694528158, 110.6239096053143243 ) ) ;
#2389=CARTESIAN_POINT ( 'NONE',  ( -5.719274019375665041, -21.55341960407619695, 74.79275706135234714 ) ) ;
#2390=CARTESIAN_POINT ( 'NONE',  ( 13.97604488694527802, 13.89961937509977652, 54.37390960531435979 ) ) ;
#2391=CARTESIAN_POINT ( 'NONE',  ( -10.72451020669870658, -18.67979575497194134, 69.58442372801900433 ) ) ;
#2392=CARTESIAN_POINT ( 'NONE',  ( 21.52544592524344225, -5.823673210054117533, 28.54057627198103120 ) ) ;
#2393=CARTESIAN_POINT ( 'NONE',  ( -5.049401038298153566, 19.05341960407611168, 40.20724293864768839 ) ) ;
#2394=CARTESIAN_POINT ( 'NONE',  ( 15.80617190586769283, -15.72974639402175789, 30.62609039468567929 ) ) ;
#2395=CARTESIAN_POINT ( 'NONE',  ( -19.03943276465977164, -0.05219959533935918106, 48.75109039468566863 ) ) ;
#2396=CARTESIAN_POINT ( 'NONE',  ( -13.97604488694527625, -13.89961937509977652, 26.87390960531434558 ) ) ;
#2397=CARTESIAN_POINT ( 'NONE',  ( -19.05341960407611168, -5.049401038298163336, 71.45724293864766707 ) ) ;
#2398=CARTESIAN_POINT ( 'NONE',  ( 9.564922557961047289, -16.46253265017146816, 105.4177570613523471 ) ) ;
#2399=CARTESIAN_POINT ( 'NONE',  ( -14.34966873604960291, -8.224510206698953496, 71.66557627198100988 ) ) ;
#2400=CARTESIAN_POINT ( 'NONE',  ( 15.72974639402199770, -15.80617190586745480, 43.12390960531435269 ) ) ;
#2402=CARTESIAN_POINT ( 'NONE',  ( -9.474510206698720793, -16.51473224551083518, 99.58442372801900433 ) ) ;
#2403=CARTESIAN_POINT ( 'NONE',  ( 21.53943276465977519, -0.05219959533907433946, 103.7489096053143669 ) ) ;
#2404=CARTESIAN_POINT ( 'NONE',  ( 0.05219959533937995610, -21.53943276465977519, 55.00109039468568284 ) ) ;
#2405=CARTESIAN_POINT ( 'NONE',  ( 4.379528057220092307, 16.55341960407617563, 62.29275706135236845 ) ) ;
#2406=CARTESIAN_POINT ( 'NONE',  ( 16.53943276465976808, 0.05219959533934440121, 61.25109039468567573 ) ) ;
#2407=CARTESIAN_POINT ( 'NONE',  ( 5.823673210054125526, 21.52544592524343514, 69.79057627198102409 ) ) ;
#2408=CARTESIAN_POINT ( 'NONE',  ( 16.46253265017160672, -9.564922557960803928, 43.33224293864769550 ) ) ;
#2409=CARTESIAN_POINT ( 'NONE',  ( 16.52544592524335698, 4.483927247898782831, 91.45942372801901854 ) ) ;
#2410=CARTESIAN_POINT ( 'NONE',  ( -15.80617190586745835, -15.72974639402198527, 106.8739096053143811 ) ) ;
#2411=CARTESIAN_POINT ( 'NONE',  ( -8.314922557960811034, -14.29746914071050412, 57.08224293864769550 ) ) ;
#2412=CARTESIAN_POINT ( 'NONE',  ( -5.153800228976328057, -19.02544592524343514, 77.29057627198099567 ) ) ;
#2413=CARTESIAN_POINT ( 'NONE',  ( -12.14591786802326823, 12.06949235617739902, 78.12609039468570415 ) ) ;
#2414=CARTESIAN_POINT ( 'NONE',  ( -0.05219959533936034679, 19.03943276465977164, 112.5010903946856757 ) ) ;
#2415=CARTESIAN_POINT ( 'NONE',  ( -21.52544592524343514, 5.823673210054127303, 106.0405762719810525 ) ) ;
#2416=CARTESIAN_POINT ( 'NONE',  ( -14.29746914071049879, 8.314922557960819915, 45.83224293864769550 ) ) ;
#2418=CARTESIAN_POINT ( 'NONE',  ( -17.26058549869092573, 6.457015423128486198, 68.62254162523935008 ) ) ;
#2419=CARTESIAN_POINT ( 'NONE',  ( 10.72451020669898902, -18.67979575497178502, 87.91557627198103830 ) ) ;
#2420=ORIENTED_EDGE ( 'NONE', *, *, #94263, .F. ) ;
#2421=CARTESIAN_POINT ( 'NONE',  ( -16.52544592524342804, 4.483927247898546575, 26.04057627198103475 ) ) ;
#2422=ORIENTED_EDGE ( 'NONE', *, *, #150310, .F. ) ;
#2424=CARTESIAN_POINT ( 'NONE',  ( -21.53943276465977519, 0.05219959533907696930, 101.2489096053143669 ) ) ;
#2425=CARTESIAN_POINT ( 'NONE',  ( -13.89961937509977652, 13.97604488694528158, 105.6239096053143527 ) ) ;
#2426=CARTESIAN_POINT ( 'NONE',  ( 10.81492255796106328, -18.62759615963255655, 20.41775706135234714 ) ) ;
#2427=CARTESIAN_POINT ( 'NONE',  ( -8.224510206698948167, 14.34966873604960824, 50.41557627198103120 ) ) ;
#2428=CARTESIAN_POINT ( 'NONE',  ( 4.379528057220092307, 16.55341960407617563, 52.29275706135236135 ) ) ;
#2430=CARTESIAN_POINT ( 'NONE',  ( -9.474510206698964154, 16.51473224551069663, 55.41557627198103120 ) ) ;
#2431=CARTESIAN_POINT ( 'NONE',  ( 16.51473224551083163, -9.474510206698727899, 50.83442372801899722 ) ) ;
#2432=CARTESIAN_POINT ( 'NONE',  ( 5.153800228976335163, 19.02544592524342804, 79.79057627198102409 ) ) ;
#2433=CARTESIAN_POINT ( 'NONE',  ( 18.62759615963271287, -10.81492255796078972, 38.33224293864768839 ) ) ;
#2434=CARTESIAN_POINT ( 'NONE',  ( -9.474510206698964154, 16.51473224551069663, 40.41557627198103120 ) ) ;
#2435=CARTESIAN_POINT ( 'NONE',  ( -19.03943276465977164, -0.05219959533935918106, 113.7510903946856757 ) ) ;
#2436=CARTESIAN_POINT ( 'NONE',  ( 9.564922557961047289, -16.46253265017146816, 60.41775706135233293 ) ) ;
#2437=CARTESIAN_POINT ( 'NONE',  ( 15.80617190586746368, 15.72974639402197994, 104.3739096053143669 ) ) ;
#2438=CARTESIAN_POINT ( 'NONE',  ( -14.29746914071049879, 8.314922557960819915, 35.83224293864768839 ) ) ;
#2439=CARTESIAN_POINT ( 'NONE',  ( 9.564922557960805705, 16.46253265017160317, 74.58224293864769550 ) ) ;
#2440=CARTESIAN_POINT ( 'NONE',  ( -10.72451020669898014, 18.67979575497178502, 65.41557627198102409 ) ) ;
#2441=CARTESIAN_POINT ( 'NONE',  ( -15.72974639402197994, 15.80617190586746368, 95.62390960531436690 ) ) ;
#2442=CARTESIAN_POINT ( 'NONE',  ( 4.483927247898790824, -16.52544592524335698, 25.20942372801901854 ) ) ;
#2443=CARTESIAN_POINT ( 'NONE',  ( 9.474510206698971260, -16.51473224551069308, 112.9155762719810383 ) ) ;
#2444=CARTESIAN_POINT ( 'NONE',  ( -18.67979575497193778, 10.72451020669871902, 88.33442372801901854 ) ) ;
#2445=CARTESIAN_POINT ( 'NONE',  ( -19.02544592524342804, 5.153800228976336051, 81.04057627198103830 ) ) ;
#2446=CARTESIAN_POINT ( 'NONE',  ( -16.51473224551069308, -9.474510206698971260, 26.66557627198103120 ) ) ;
#2447=CARTESIAN_POINT ( 'NONE',  ( -19.02544592524342804, 5.153800228976336051, 81.04057627198103830 ) ) ;
#2448=CARTESIAN_POINT ( 'NONE',  ( 8.314922557960818139, 14.29746914071049879, 109.5822429386476955 ) ) ;
#2449=CARTESIAN_POINT ( 'NONE',  ( 19.02544592524343514, -5.153800228976328945, 68.54057627198103830 ) ) ;
#2450=CARTESIAN_POINT ( 'NONE',  ( 0.05219959533934541429, -16.53943276465976808, 25.00109039468567218 ) ) ;
#2451=CARTESIAN_POINT ( 'NONE',  ( 5.049401038297881783, 19.05341960407617918, 42.29275706135234003 ) ) ;
#2453=CARTESIAN_POINT ( 'NONE',  ( 21.53943276465977519, 0.05219959533937863772, 91.25109039468568994 ) ) ;
#2454=CARTESIAN_POINT ( 'NONE',  ( -19.03943276465977164, 0.05219959533909376836, 116.2489096053143669 ) ) ;
#2455=CARTESIAN_POINT ( 'NONE',  ( 14.29746914071037800, 8.314922557961029526, 86.66775706135234714 ) ) ;
#2457=CARTESIAN_POINT ( 'NONE',  ( -13.97604488694547697, 13.89961937509957934, 73.12609039468568994 ) ) ;
#2458=CARTESIAN_POINT ( 'NONE',  ( 9.564922557961047289, -16.46253265017146816, 25.41775706135234003 ) ) ;
#2460=CARTESIAN_POINT ( 'NONE',  ( -5.049401038298153566, 19.05341960407611168, 30.20724293864768839 ) ) ;
#2461=CARTESIAN_POINT ( 'NONE',  ( -16.52544592524342804, 4.483927247898546575, 36.04057627198102409 ) ) ;
#2463=CARTESIAN_POINT ( 'NONE',  ( 16.52544592524335698, 4.483927247898782831, 111.4594237280190328 ) ) ;
#2464=CARTESIAN_POINT ( 'NONE',  ( 16.62475595723700650, 7.163666690055261910, 66.97286648189530922 ) ) ;
#2465=CARTESIAN_POINT ( 'NONE',  ( -0.05219959533934338120, 16.53943276465976808, 82.50109039468568994 ) ) ;
#2466=CARTESIAN_POINT ( 'NONE',  ( 9.474510206698971260, -16.51473224551069308, 37.91557627198102409 ) ) ;
#2467=CARTESIAN_POINT ( 'NONE',  ( -15.72974639402176322, -15.80617190586768395, 99.37609039468568994 ) ) ;
#2468=CARTESIAN_POINT ( 'NONE',  ( 5.049401038297881783, 19.05341960407617563, 97.29275706135233293 ) ) ;
#2469=CARTESIAN_POINT ( 'NONE',  ( 0.05219959533937995610, -21.53943276465977519, 85.00109039468568994 ) ) ;
#2470=CARTESIAN_POINT ( 'NONE',  ( 13.97604488694548053, -13.89961937509957401, 50.62609039468566152 ) ) ;
#2471=CARTESIAN_POINT ( 'NONE',  ( -9.564922557960796823, -16.46253265017161027, 92.08224293864769550 ) ) ;
#2472=CARTESIAN_POINT ( 'NONE',  ( 19.02544592524343514, -5.153800228976328945, 73.54057627198103830 ) ) ;
#2473=CARTESIAN_POINT ( 'NONE',  ( 17.44279575226822843, 5.990770900252481823, 71.66442432485683867 ) ) ;
#2475=CARTESIAN_POINT ( 'NONE',  ( -14.29746914071049879, 8.314922557960819915, 65.83224293864769550 ) ) ;
#2476=CARTESIAN_POINT ( 'NONE',  ( -5.719274019375978568, 21.55341960407610458, 55.20724293864770260 ) ) ;
#2477=CARTESIAN_POINT ( 'NONE',  ( 9.564922557960805705, 16.46253265017160317, 49.58224293864770260 ) ) ;
#2478=CARTESIAN_POINT ( 'NONE',  ( 10.81492255796078972, 18.62759615963270932, 84.58224293864769550 ) ) ;
#2479=CARTESIAN_POINT ( 'NONE',  ( -8.224510206698735004, -14.34966873604973081, 74.58442372801901854 ) ) ;
#2480=VERTEX_POINT ( 'NONE', #101200 ) ;
#2481=CARTESIAN_POINT ( 'NONE',  ( 16.46253265017160672, -9.564922557960803928, 43.33224293864769550 ) ) ;
#2482=CARTESIAN_POINT ( 'NONE',  ( 14.29746914071049879, -8.314922557960816363, 73.33224293864769550 ) ) ;
#2484=CARTESIAN_POINT ( 'NONE',  ( 9.564922557960805705, 16.46253265017160317, 49.58224293864770260 ) ) ;
#2485=CARTESIAN_POINT ( 'NONE',  ( -19.02544592524342804, 5.153800228976336051, 26.04057627198103120 ) ) ;
#2486=CARTESIAN_POINT ( 'NONE',  ( 13.97604488694548053, -13.89961937509957401, 70.62609039468567573 ) ) ;
#2487=CARTESIAN_POINT ( 'NONE',  ( 14.34966873604960469, 8.224510206698951720, 74.16557627198102409 ) ) ;
#2488=CARTESIAN_POINT ( 'NONE',  ( -5.823673210054431948, 21.52544592524334988, 47.70942372801902565 ) ) ;
#2489=CARTESIAN_POINT ( 'NONE',  ( -9.564922557960796823, -16.46253265017161027, 37.08224293864768839 ) ) ;
#2490=CARTESIAN_POINT ( 'NONE',  ( 18.62759615963271287, -10.81492255796078972, 103.3322429386476955 ) ) ;
#2491=CARTESIAN_POINT ( 'NONE',  ( -5.049401038298153566, 19.05341960407611168, 115.2072429386477097 ) ) ;
#2492=CARTESIAN_POINT ( 'NONE',  ( 4.379528057220339221, -16.55341960407611168, 82.70724293864770971 ) ) ;
#2494=CARTESIAN_POINT ( 'NONE',  ( -19.03943276465977164, 0.05219959533909376836, 51.24890960531436690 ) ) ;
#2495=CARTESIAN_POINT ( 'NONE',  ( 19.25918095147781273, 5.499999999999579892, 46.95284276293937609 ) ) ;
#2496=CARTESIAN_POINT ( 'NONE',  ( 19.05341960407617918, -5.049401038297876454, 91.04275706135234714 ) ) ;
#2497=CARTESIAN_POINT ( 'NONE',  ( -21.53943276465977519, -0.05219959533937600094, 38.75109039468567573 ) ) ;
#2498=CARTESIAN_POINT ( 'NONE',  ( -19.03943276465977164, 0.05219959533909376836, 81.24890960531436690 ) ) ;
#2499=CARTESIAN_POINT ( 'NONE',  ( -19.03943276465977164, -0.05219959533935918106, 68.75109039468566152 ) ) ;
#2500=CARTESIAN_POINT ( 'NONE',  ( -9.474510206698964154, 16.51473224551069663, 40.41557627198103120 ) ) ;
#2502=CARTESIAN_POINT ( 'NONE',  ( -14.34966873604960291, -8.224510206698953496, 61.66557627198103120 ) ) ;
#2503=CARTESIAN_POINT ( 'NONE',  ( 4.379528057220339221, -16.55341960407611168, 67.70724293864769550 ) ) ;
#2504=CARTESIAN_POINT ( 'NONE',  ( -19.05341960407611168, -5.049401038298163336, 71.45724293864766707 ) ) ;
#2505=CARTESIAN_POINT ( 'NONE',  ( 10.81492255796078972, 18.62759615963270932, 99.58224293864770971 ) ) ;
#2506=CARTESIAN_POINT ( 'NONE',  ( 0.05219959533909260263, 19.03943276465977164, 74.99890960531435269 ) ) ;
#2507=CARTESIAN_POINT ( 'NONE',  ( -18.67979575497193778, 10.72451020669871902, 108.3344237280190185 ) ) ;
#2508=CARTESIAN_POINT ( 'NONE',  ( 13.97604488694527802, 13.89961937509977652, 39.37390960531435269 ) ) ;
#2509=CARTESIAN_POINT ( 'NONE',  ( -16.53943276465976808, 0.05219959533911058130, 21.24890960531436690 ) ) ;
#2510=CARTESIAN_POINT ( 'NONE',  ( -16.53943276465976808, 0.05219959533911058130, 111.2489096053143669 ) ) ;
#2511=CARTESIAN_POINT ( 'NONE',  ( -9.474510206698720793, -16.51473224551083518, 99.58442372801900433 ) ) ;
#2513=CARTESIAN_POINT ( 'NONE',  ( 10.72451020669871369, 18.67979575497193778, 37.08442372801901143 ) ) ;
#2514=CARTESIAN_POINT ( 'NONE',  ( 5.153800228976615827, -19.02544592524334988, 55.20942372801899722 ) ) ;
#2515=CARTESIAN_POINT ( 'NONE',  ( -8.314922557960811034, -14.29746914071050412, 22.08224293864769194 ) ) ;
#2516=CARTESIAN_POINT ( 'NONE',  ( -10.72451020669898014, 18.67979575497178502, 75.41557627198102409 ) ) ;
#2517=CARTESIAN_POINT ( 'NONE',  ( 18.67979575497178502, 10.72451020669898547, 24.16557627198103120 ) ) ;
#2518=CARTESIAN_POINT ( 'NONE',  ( -12.14591786802309592, -12.06949235617757132, 56.87390960531436690 ) ) ;
#2519=CARTESIAN_POINT ( 'NONE',  ( 19.03943276465977164, -0.05219959533909143690, 28.74890960531435624 ) ) ;
#2520=CARTESIAN_POINT ( 'NONE',  ( -19.03943276465977164, 0.05219959533909376836, 36.24890960531436690 ) ) ;
#2521=CARTESIAN_POINT ( 'NONE',  ( -19.02544592524334988, -5.153800228976617603, 28.95942372801900433 ) ) ;
#2522=CARTESIAN_POINT ( 'NONE',  ( 12.14591786802327356, -12.06949235617739191, 90.62609039468567573 ) ) ;
#2523=CARTESIAN_POINT ( 'NONE',  ( 16.53943276465976808, 0.05219959533934440121, 46.25109039468567573 ) ) ;
#2524=CARTESIAN_POINT ( 'NONE',  ( 5.823673210054125526, 21.52544592524343514, 24.79057627198103120 ) ) ;
#2525=CARTESIAN_POINT ( 'NONE',  ( 0.05219959533909260263, 19.03943276465977164, 59.99890960531436690 ) ) ;
#2526=CARTESIAN_POINT ( 'NONE',  ( -21.53943276465977519, -0.05219959533937600094, 88.75109039468567573 ) ) ;
#2527=CARTESIAN_POINT ( 'NONE',  ( -16.51473224551069308, -9.474510206698971260, 81.66557627198103830 ) ) ;
#2528=CARTESIAN_POINT ( 'NONE',  ( -14.29746914071037622, -8.314922557961029526, 64.16775706135234714 ) ) ;
#2529=CARTESIAN_POINT ( 'NONE',  ( 8.314922557960818139, 14.29746914071049879, 109.5822429386476955 ) ) ;
#2530=CARTESIAN_POINT ( 'NONE',  ( 8.314922557961029526, -14.29746914071037800, 110.4177570613523756 ) ) ;
#2532=CARTESIAN_POINT ( 'NONE',  ( 10.72451020669871369, 18.67979575497193778, 67.08442372801901854 ) ) ;
#2533=CARTESIAN_POINT ( 'NONE',  ( -13.97604488694527625, -13.89961937509977652, 86.87390960531436690 ) ) ;
#2534=CARTESIAN_POINT ( 'NONE',  ( -16.51473224551069308, -9.474510206698971260, 71.66557627198102409 ) ) ;
#2535=CARTESIAN_POINT ( 'NONE',  ( 16.51473224551069308, 9.474510206698969483, 114.1655762719810241 ) ) ;
#2536=CARTESIAN_POINT ( 'NONE',  ( -14.34966873604960291, -8.224510206698953496, 61.66557627198103120 ) ) ;
#2537=CARTESIAN_POINT ( 'NONE',  ( 12.06949235617739724, 12.14591786802326823, 111.8760903946856615 ) ) ;
#2538=CARTESIAN_POINT ( 'NONE',  ( 0.05219959533910956823, 16.53943276465976808, 34.99890960531435979 ) ) ;
#2539=CARTESIAN_POINT ( 'NONE',  ( -16.53943276465976808, -0.05219959533934237506, 43.75109039468568284 ) ) ;
#2541=CARTESIAN_POINT ( 'NONE',  ( -19.02544592524334988, -5.153800228976617603, 33.95942372801897591 ) ) ;
#2542=CARTESIAN_POINT ( 'NONE',  ( 5.153800228976335163, 19.02544592524342804, 74.79057627198103830 ) ) ;
#2543=CARTESIAN_POINT ( 'NONE',  ( 16.46253265017146816, 9.564922557961045513, 51.66775706135233293 ) ) ;
#2546=CARTESIAN_POINT ( 'NONE',  ( 0.05219959533936267826, -19.03943276465977164, 80.00109039468567573 ) ) ;
#2547=CARTESIAN_POINT ( 'NONE',  ( 4.483927247898790824, -16.52544592524335698, 80.20942372801901854 ) ) ;
#2549=CARTESIAN_POINT ( 'NONE',  ( -9.474510206698964154, 16.51473224551069663, 110.4155762719810383 ) ) ;
#2550=CARTESIAN_POINT ( 'NONE',  ( 0.05219959533937995610, -21.53943276465977519, 45.00109039468568284 ) ) ;
#2551=CARTESIAN_POINT ( 'NONE',  ( 5.153800228976615827, -19.02544592524334988, 95.20942372801897591 ) ) ;
#2553=CARTESIAN_POINT ( 'NONE',  ( -19.05341960407611168, -5.049401038298163336, 41.45724293864769550 ) ) ;
#2554=CARTESIAN_POINT ( 'NONE',  ( 19.05341960407611168, 5.049401038298154454, 108.9572429386477097 ) ) ;
#2555=CARTESIAN_POINT ( 'NONE',  ( -0.05219959533910754901, -16.53943276465976808, 62.49890960531436690 ) ) ;
#2556=CARTESIAN_POINT ( 'NONE',  ( 19.05341960407611168, 5.049401038298154454, 53.95724293864770260 ) ) ;
#2557=CARTESIAN_POINT ( 'NONE',  ( 5.049401038298161559, -19.05341960407611168, 62.70724293864769550 ) ) ;
#2558=CARTESIAN_POINT ( 'NONE',  ( -13.97604488694547697, 13.89961937509957934, 58.12609039468566863 ) ) ;
#2559=CARTESIAN_POINT ( 'NONE',  ( 19.05341960407617918, -5.049401038297876454, 46.04275706135233293 ) ) ;
#2560=CARTESIAN_POINT ( 'NONE',  ( 9.564922557960805705, 16.46253265017160317, 69.58224293864770971 ) ) ;
#2561=CARTESIAN_POINT ( 'NONE',  ( 5.823673210054125526, 21.52544592524343514, 74.79057627198105251 ) ) ;
#2562=CARTESIAN_POINT ( 'NONE',  ( -4.483927247898539470, -16.52544592524342804, 72.29057627198102409 ) ) ;
#2563=CARTESIAN_POINT ( 'NONE',  ( 5.153800228976615827, -19.02544592524334988, 40.20942372801898301 ) ) ;
#2564=CARTESIAN_POINT ( 'NONE',  ( -21.52544592524343514, 5.823673210054127303, 46.04057627198103830 ) ) ;
#2565=CARTESIAN_POINT ( 'NONE',  ( -21.52544592524343514, 5.823673210054127303, 36.04057627198102409 ) ) ;
#2566=CARTESIAN_POINT ( 'NONE',  ( -19.03943276465977164, 0.05219959533909376836, 61.24890960531436690 ) ) ;
#2567=CARTESIAN_POINT ( 'NONE',  ( -13.89961937509977652, 13.97604488694528158, 40.62390960531435979 ) ) ;
#2568=CARTESIAN_POINT ( 'NONE',  ( 8.314922557960818139, 14.29746914071049879, 94.58224293864769550 ) ) ;
#2570=CARTESIAN_POINT ( 'NONE',  ( -18.62759615963270932, 10.81492255796079327, 105.8322429386476955 ) ) ;
#2571=CARTESIAN_POINT ( 'NONE',  ( -0.05219959533909027116, -19.03943276465977164, 112.4989096053143669 ) ) ;
#2572=CARTESIAN_POINT ( 'NONE',  ( 10.72451020669871369, 18.67979575497193778, 27.08442372801901854 ) ) ;
#2573=CARTESIAN_POINT ( 'NONE',  ( -19.03943276465977164, 0.05219959533909376836, 41.24890960531435269 ) ) ;
#2574=CARTESIAN_POINT ( 'NONE',  ( 10.81492255796078972, 18.62759615963270932, 109.5822429386476955 ) ) ;
#2576=CARTESIAN_POINT ( 'NONE',  ( -9.474510206698720793, -16.51473224551083518, 49.58442372801899722 ) ) ;
#2577=CARTESIAN_POINT ( 'NONE',  ( 0.05219959533909260263, 19.03943276465977164, 29.99890960531435979 ) ) ;
#2578=CARTESIAN_POINT ( 'NONE',  ( 18.56197773271727414, -5.500000000000073719, 76.05066217314451649 ) ) ;
#2580=CARTESIAN_POINT ( 'NONE',  ( -16.55341960407617563, 4.379528057220093196, 48.54275706135234714 ) ) ;
#2581=CARTESIAN_POINT ( 'NONE',  ( -19.02544592524342804, 5.153800228976336051, 26.04057627198103120 ) ) ;
#2583=CARTESIAN_POINT ( 'NONE',  ( 5.153800228976335163, 19.02544592524342804, 69.79057627198103830 ) ) ;
#2584=CARTESIAN_POINT ( 'NONE',  ( -12.06949235617756955, 12.14591786802309770, 110.6239096053143669 ) ) ;
#2585=CARTESIAN_POINT ( 'NONE',  ( -5.823673210054116645, -21.52544592524344225, 52.29057627198102409 ) ) ;
#2586=CARTESIAN_POINT ( 'NONE',  ( -14.34966873604960291, -8.224510206698953496, 81.66557627198103830 ) ) ;
#2587=CARTESIAN_POINT ( 'NONE',  ( -4.483927247898782831, 16.52544592524335698, 37.70942372801900433 ) ) ;
#2588=CARTESIAN_POINT ( 'NONE',  ( 18.67979575497194134, -10.72451020669871369, 80.83442372801901854 ) ) ;
#2589=CARTESIAN_POINT ( 'NONE',  ( -19.03943276465977164, 0.05219959533909376836, 26.24890960531435624 ) ) ;
#2591=CARTESIAN_POINT ( 'NONE',  ( -4.483927247898782831, 16.52544592524335698, 107.7094237280190328 ) ) ;
#2592=CARTESIAN_POINT ( 'NONE',  ( -16.55341960407611168, -4.379528057220339221, 56.45724293864768839 ) ) ;
#2593=CARTESIAN_POINT ( 'NONE',  ( -16.46253265017160317, 9.564922557960807481, 50.83224293864770260 ) ) ;
#2594=CARTESIAN_POINT ( 'NONE',  ( -5.719274019375665041, -21.55341960407619695, 94.79275706135234714 ) ) ;
#2595=CARTESIAN_POINT ( 'NONE',  ( 21.52544592524344225, -5.823673210054117533, 103.5405762719810383 ) ) ;
#2596=CARTESIAN_POINT ( 'NONE',  ( -15.80617190586768217, 15.72974639402176855, 73.12609039468567573 ) ) ;
#2597=CARTESIAN_POINT ( 'NONE',  ( 16.55341960407618274, -4.379528057220086978, 36.04275706135234714 ) ) ;
#2598=CARTESIAN_POINT ( 'NONE',  ( -16.55341960407611168, -4.379528057220339221, 81.45724293864769550 ) ) ;
#2599=CARTESIAN_POINT ( 'NONE',  ( 18.62759615963255655, 10.81492255796105972, 91.66775706135234714 ) ) ;
#2601=CARTESIAN_POINT ( 'NONE',  ( 12.14591786802309770, 12.06949235617756955, 24.37390960531435979 ) ) ;
#2602=CARTESIAN_POINT ( 'NONE',  ( 18.22780087662125226, -5.499999999999864997, 61.01540105326109398 ) ) ;
#2603=CARTESIAN_POINT ( 'NONE',  ( 12.14591786802327356, -12.06949235617739191, 45.62609039468567573 ) ) ;
#2604=CARTESIAN_POINT ( 'NONE',  ( -16.53943276465976808, 0.05219959533911058130, 36.24890960531435979 ) ) ;
#2605=CARTESIAN_POINT ( 'NONE',  ( 14.34966873604972726, -8.224510206698740333, 90.83442372801901854 ) ) ;
#2606=CARTESIAN_POINT ( 'NONE',  ( 19.05341960407611168, 5.049401038298154454, 103.9572429386476671 ) ) ;
#2608=CARTESIAN_POINT ( 'NONE',  ( 9.564922557960805705, 16.46253265017160317, 94.58224293864769550 ) ) ;
#2609=CARTESIAN_POINT ( 'NONE',  ( 15.80617190586769283, -15.72974639402175789, 100.6260903946857184 ) ) ;
#2610=CARTESIAN_POINT ( 'NONE',  ( -16.52544592524335698, -4.483927247898792601, 98.95942372801903275 ) ) ;
#2611=CARTESIAN_POINT ( 'NONE',  ( -12.06949235617756955, 12.14591786802309770, 70.62390960531436690 ) ) ;
#2612=CARTESIAN_POINT ( 'NONE',  ( 16.46253265017160672, -9.564922557960803928, 83.33224293864768129 ) ) ;
#2614=CARTESIAN_POINT ( 'NONE',  ( 14.29746914071037800, 8.314922557961029526, 31.66775706135234358 ) ) ;
#2615=CARTESIAN_POINT ( 'NONE',  ( 5.153800228976335163, 19.02544592524342804, 24.79057627198102765 ) ) ;
#2616=CARTESIAN_POINT ( 'NONE',  ( -19.05341960407611168, -5.049401038298163336, 91.45724293864766707 ) ) ;
#2617=CARTESIAN_POINT ( 'NONE',  ( 16.53943276465976808, 0.05219959533934440121, 36.25109039468567573 ) ) ;
#2619=CARTESIAN_POINT ( 'NONE',  ( 0.05219959533936267826, -19.03943276465977164, 30.00109039468566863 ) ) ;
#2620=CARTESIAN_POINT ( 'NONE',  ( -14.34966873604972548, 8.224510206698743886, 93.33442372801901854 ) ) ;
#2621=CARTESIAN_POINT ( 'NONE',  ( 13.89961937509957401, 13.97604488694547697, 111.8760903946856757 ) ) ;
#2622=CARTESIAN_POINT ( 'NONE',  ( 13.97604488694527802, 13.89961937509977652, 29.37390960531435979 ) ) ;
#2623=CARTESIAN_POINT ( 'NONE',  ( -8.314922557961024197, 14.29746914071037800, 77.91775706135231871 ) ) ;
#2624=CARTESIAN_POINT ( 'NONE',  ( -16.52544592524335698, -4.483927247898792601, 63.95942372801901854 ) ) ;
#2625=CARTESIAN_POINT ( 'NONE',  ( -19.02544592524342804, 5.153800228976336051, 26.04057627198103120 ) ) ;
#2626=CARTESIAN_POINT ( 'NONE',  ( -13.97604488694547697, 13.89961937509957934, 68.12609039468563310 ) ) ;
#2627=CARTESIAN_POINT ( 'NONE',  ( -18.67979575497193778, 10.72451020669871902, 113.3344237280190328 ) ) ;
#2628=CARTESIAN_POINT ( 'NONE',  ( 5.049401038298161559, -19.05341960407611168, 47.70724293864770260 ) ) ;
#2629=CARTESIAN_POINT ( 'NONE',  ( 16.46253265017160672, -9.564922557960803928, 88.33224293864769550 ) ) ;
#2630=CARTESIAN_POINT ( 'NONE',  ( 14.34966873604960469, 8.224510206698951720, 84.16557627198103830 ) ) ;
#2632=CARTESIAN_POINT ( 'NONE',  ( 5.153800228976615827, -19.02544592524334988, 60.20942372801899012 ) ) ;
#2633=CARTESIAN_POINT ( 'NONE',  ( 21.53943276465977519, -0.05219959533907433946, 53.74890960531437401 ) ) ;
#2634=CARTESIAN_POINT ( 'NONE',  ( -19.02544592524334988, -5.153800228976617603, 18.95942372801899722 ) ) ;
#2635=CARTESIAN_POINT ( 'NONE',  ( 9.564922557960805705, 16.46253265017160317, 94.58224293864769550 ) ) ;
#2636=CARTESIAN_POINT ( 'NONE',  ( -13.97604488694547697, 13.89961937509957934, 23.12609039468565442 ) ) ;
#2637=CARTESIAN_POINT ( 'NONE',  ( -21.55341960407610458, -5.719274019375992779, 61.45724293864770260 ) ) ;
#2638=CARTESIAN_POINT ( 'NONE',  ( 19.05341960407611168, 5.049401038298154454, 113.9572429386477097 ) ) ;
#2639=CARTESIAN_POINT ( 'NONE',  ( 16.46253265017146816, 9.564922557961045513, 86.66775706135233293 ) ) ;
#2640=CARTESIAN_POINT ( 'NONE',  ( -17.50000000000148148, 3.202012800152246097, 109.9282241602726202 ) ) ;
#2641=CARTESIAN_POINT ( 'NONE',  ( -9.474510206698720793, -16.51473224551083518, 104.5844237280190043 ) ) ;
#2642=CARTESIAN_POINT ( 'NONE',  ( -8.224510206698948167, 14.34966873604960824, 110.4155762719810383 ) ) ;
#2643=CARTESIAN_POINT ( 'NONE',  ( 9.474510206698971260, -16.51473224551069308, 97.91557627198102409 ) ) ;
#2644=CARTESIAN_POINT ( 'NONE',  ( 15.72974639402199770, -15.80617190586745480, 73.12390960531436690 ) ) ;
#2645=CARTESIAN_POINT ( 'NONE',  ( -4.483927247898782831, 16.52544592524335698, 42.70942372801901854 ) ) ;
#2646=CARTESIAN_POINT ( 'NONE',  ( 5.719274019375673035, 21.55341960407619339, 47.29275706135234003 ) ) ;
#2647=CARTESIAN_POINT ( 'NONE',  ( 10.81492255796106328, -18.62759615963255655, 95.41775706135234714 ) ) ;
#2648=CARTESIAN_POINT ( 'NONE',  ( -16.53943276465976808, -0.05219959533934237506, 98.75109039468568994 ) ) ;
#2649=CARTESIAN_POINT ( 'NONE',  ( 19.02544592524343514, -5.153800228976328945, 93.54057627198102409 ) ) ;
#2650=CARTESIAN_POINT ( 'NONE',  ( -16.55341960407611168, -4.379528057220339221, 96.45724293864770971 ) ) ;
#2651=CARTESIAN_POINT ( 'NONE',  ( -14.34966873604960291, -8.224510206698953496, 36.66557627198103120 ) ) ;
#2652=CARTESIAN_POINT ( 'NONE',  ( -19.05341960407617563, 5.049401038297882671, 68.54275706135230450 ) ) ;
#2653=CARTESIAN_POINT ( 'NONE',  ( -5.719274019375665041, -21.55341960407619695, 44.79275706135234714 ) ) ;
#2654=CARTESIAN_POINT ( 'NONE',  ( -13.97604488694547697, 13.89961937509957934, 33.12609039468566863 ) ) ;
#2655=CARTESIAN_POINT ( 'NONE',  ( 12.14591786802309770, 12.06949235617756955, 89.37390960531435269 ) ) ;
#2656=CARTESIAN_POINT ( 'NONE',  ( -16.51473224551069308, -9.474510206698971260, 111.6655762719810383 ) ) ;
#2657=CARTESIAN_POINT ( 'NONE',  ( 16.53943276465976808, 0.05219959533934440121, 111.2510903946856899 ) ) ;
#2658=CARTESIAN_POINT ( 'NONE',  ( -0.05219959533937732626, 21.53943276465977519, 87.50109039468568994 ) ) ;
#2659=CARTESIAN_POINT ( 'NONE',  ( 4.379528057220092307, 16.55341960407617563, 62.29275706135236845 ) ) ;
#2660=CARTESIAN_POINT ( 'NONE',  ( -16.55341960407617563, 4.379528057220093196, 103.5427570613523613 ) ) ;
#2661=CARTESIAN_POINT ( 'NONE',  ( -15.80617190586768217, 15.72974639402176855, 48.12609039468568284 ) ) ;
#2663=CARTESIAN_POINT ( 'NONE',  ( -21.52544592524334988, -5.823673210054445271, 28.95942372801902209 ) ) ;
#2664=CARTESIAN_POINT ( 'NONE',  ( 12.06949235617757843, -12.14591786802309237, 103.1239096053143811 ) ) ;
#2665=CARTESIAN_POINT ( 'NONE',  ( -19.03943276465977164, 0.05219959533909376836, 21.24890960531436335 ) ) ;
#2666=CARTESIAN_POINT ( 'NONE',  ( -16.52544592524342804, 4.483927247898546575, 66.04057627198103830 ) ) ;
#2667=CARTESIAN_POINT ( 'NONE',  ( 16.51473224551069308, 9.474510206698969483, 74.16557627198103830 ) ) ;
#2668=CARTESIAN_POINT ( 'NONE',  ( 16.53943276465976808, 0.05219959533934440121, 101.2510903946856757 ) ) ;
#2669=CARTESIAN_POINT ( 'NONE',  ( -0.05219959533909027116, -19.03943276465977164, 42.49890960531435269 ) ) ;
#2670=CARTESIAN_POINT ( 'NONE',  ( 10.72451020669898902, -18.67979575497178502, 52.91557627198103830 ) ) ;
#2671=CARTESIAN_POINT ( 'NONE',  ( -0.05219959533910754901, -16.53943276465976808, 97.49890960531436690 ) ) ;
#2672=CARTESIAN_POINT ( 'NONE',  ( -10.81492255796078084, -18.62759615963271287, 97.08224293864770971 ) ) ;
#2673=CARTESIAN_POINT ( 'NONE',  ( 0.05219959533909260263, 19.03943276465977164, 94.99890960531436690 ) ) ;
#2674=CARTESIAN_POINT ( 'NONE',  ( 13.89961937509977652, -13.97604488694527269, 48.12390960531435979 ) ) ;
#2675=CARTESIAN_POINT ( 'NONE',  ( -5.153800228976607833, 19.02544592524334988, 97.70942372801900433 ) ) ;
#2676=CARTESIAN_POINT ( 'NONE',  ( -15.72974639402197994, 15.80617190586746368, 40.62390960531435269 ) ) ;
#2677=CARTESIAN_POINT ( 'NONE',  ( 0.05219959533937995610, -21.53943276465977519, 65.00109039468568994 ) ) ;
#2678=CARTESIAN_POINT ( 'NONE',  ( 13.97604488694527802, 13.89961937509977652, 59.37390960531434558 ) ) ;
#2679=CARTESIAN_POINT ( 'NONE',  ( 19.05341960407611168, 5.049401038298154454, 88.95724293864769550 ) ) ;
#2680=CARTESIAN_POINT ( 'NONE',  ( -0.05219959533934338120, 16.53943276465976808, 67.50109039468568994 ) ) ;
#2681=CARTESIAN_POINT ( 'NONE',  ( 0.05219959533937995610, -21.53943276465977519, 50.00109039468568994 ) ) ;
#2682=CARTESIAN_POINT ( 'NONE',  ( -5.823673210054431948, 21.52544592524334988, 92.70942372801901854 ) ) ;
#2683=CARTESIAN_POINT ( 'NONE',  ( 21.55341960407610458, 5.719274019375980345, 98.95724293864770971 ) ) ;
#2684=CARTESIAN_POINT ( 'NONE',  ( -10.72451020669870658, -18.67979575497194134, 39.58442372801901143 ) ) ;
#2685=CARTESIAN_POINT ( 'NONE',  ( 14.34966873604972726, -8.224510206698740333, 65.83442372801900433 ) ) ;
#2686=CARTESIAN_POINT ( 'NONE',  ( 15.72974639402199770, -15.80617190586745480, 63.12390960531435979 ) ) ;
#2687=CARTESIAN_POINT ( 'NONE',  ( 9.474510206698729675, 16.51473224551082808, 32.08442372801900433 ) ) ;
#2688=CARTESIAN_POINT ( 'NONE',  ( -9.564922557960796823, -16.46253265017161027, 62.08224293864769550 ) ) ;
#2689=CARTESIAN_POINT ( 'NONE',  ( 14.34966873604972726, -8.224510206698740333, 110.8344237280190043 ) ) ;
#2690=CARTESIAN_POINT ( 'NONE',  ( -17.50000000000000000, -5.500000000000000000, 106.2823096230357010 ) ) ;
#2691=CARTESIAN_POINT ( 'NONE',  ( -19.05341960407611168, -5.049401038298163336, 96.45724293864769550 ) ) ;
#2694=CARTESIAN_POINT ( 'NONE',  ( 9.564922557961047289, -16.46253265017146816, 85.41775706135233293 ) ) ;
#2695=CARTESIAN_POINT ( 'NONE',  ( 0.05219959533907565091, 21.53943276465977519, 54.99890960531435269 ) ) ;
#2696=CARTESIAN_POINT ( 'NONE',  ( -8.224510206698948167, 14.34966873604960824, 40.41557627198103120 ) ) ;
#2697=CARTESIAN_POINT ( 'NONE',  ( 5.153800228976615827, -19.02544592524334988, 110.2094237280189901 ) ) ;
#2698=CARTESIAN_POINT ( 'NONE',  ( -16.51473224551069308, -9.474510206698971260, 26.66557627198103120 ) ) ;
#2699=CARTESIAN_POINT ( 'NONE',  ( 5.153800228976615827, -19.02544592524334988, 110.2094237280189901 ) ) ;
#2700=CARTESIAN_POINT ( 'NONE',  ( -10.72451020669898014, 18.67979575497178502, 105.4155762719810383 ) ) ;
#2701=CARTESIAN_POINT ( 'NONE',  ( 9.474510206698729675, 16.51473224551082808, 67.08442372801900433 ) ) ;
#2702=CARTESIAN_POINT ( 'NONE',  ( 4.483927247898790824, -16.52544592524335698, 75.20942372801901854 ) ) ;
#2703=CARTESIAN_POINT ( 'NONE',  ( 16.46253265017160672, -9.564922557960803928, 73.33224293864769550 ) ) ;
#2704=CARTESIAN_POINT ( 'NONE',  ( -4.483927247898539470, -16.52544592524342804, 82.29057627198103830 ) ) ;
#2705=CARTESIAN_POINT ( 'NONE',  ( -19.02544592524342804, 5.153800228976336051, 61.04057627198103120 ) ) ;
#2706=CARTESIAN_POINT ( 'NONE',  ( 12.06949235617757843, -12.14591786802309237, 63.12390960531435979 ) ) ;
#2709=CARTESIAN_POINT ( 'NONE',  ( -4.483927247898539470, -16.52544592524342804, 47.29057627198103120 ) ) ;
#2710=CARTESIAN_POINT ( 'NONE',  ( -13.89961937509977652, 13.97604488694528158, 70.62390960531432427 ) ) ;
#2711=LINE ( 'NONE', #121077, #57362 ) ;
#2712=CARTESIAN_POINT ( 'NONE',  ( -16.46253265017146816, -9.564922557961047289, 44.16775706135232582 ) ) ;
#2713=CARTESIAN_POINT ( 'NONE',  ( 14.34966873604972726, -8.224510206698740333, 50.83442372801901143 ) ) ;
#2714=CARTESIAN_POINT ( 'NONE',  ( -5.719274019375978568, 21.55341960407610458, 60.20724293864768839 ) ) ;
#2715=CARTESIAN_POINT ( 'NONE',  ( -9.474510206698720793, -16.51473224551083518, 29.58442372801900433 ) ) ;
#2716=CARTESIAN_POINT ( 'NONE',  ( 19.02544592524343514, -5.153800228976328945, 78.54057627198099567 ) ) ;
#2718=CARTESIAN_POINT ( 'NONE',  ( -16.51473224551069308, -9.474510206698971260, 111.6655762719810383 ) ) ;
#2719=CARTESIAN_POINT ( 'NONE',  ( -10.81492255796105439, 18.62759615963255655, 42.91775706135235424 ) ) ;
#2720=CARTESIAN_POINT ( 'NONE',  ( 8.224510206698953496, -14.34966873604960469, 112.9155762719810383 ) ) ;
#2721=CARTESIAN_POINT ( 'NONE',  ( -18.62759615963270932, 10.81492255796079327, 95.83224293864770971 ) ) ;
#2722=CARTESIAN_POINT ( 'NONE',  ( 16.51473224551069308, 9.474510206698969483, 79.16557627198103830 ) ) ;
#2724=CARTESIAN_POINT ( 'NONE',  ( 0.05219959533937995610, -21.53943276465977519, 30.00109039468568284 ) ) ;
#2726=CARTESIAN_POINT ( 'NONE',  ( -19.03943276465977164, 0.05219959533909376836, 91.24890960531436690 ) ) ;
#2727=CARTESIAN_POINT ( 'NONE',  ( -17.97214573761834799, -5.500000000000021316, 76.46970049038655759 ) ) ;
#2728=CARTESIAN_POINT ( 'NONE',  ( 13.89961937509977652, -13.97604488694527269, 28.12390960531435624 ) ) ;
#2729=CARTESIAN_POINT ( 'NONE',  ( -13.97604488694547697, 13.89961937509957934, 103.1260903946856473 ) ) ;
#2731=CARTESIAN_POINT ( 'NONE',  ( -8.224510206698948167, 14.34966873604960824, 110.4155762719810383 ) ) ;
#2732=CARTESIAN_POINT ( 'NONE',  ( -21.52544592524334988, -5.823673210054445271, 78.95942372801901854 ) ) ;
#2733=CARTESIAN_POINT ( 'NONE',  ( -5.049401038298153566, 19.05341960407611168, 80.20724293864769550 ) ) ;
#2734=CARTESIAN_POINT ( 'NONE',  ( 5.823673210054444382, -21.52544592524334988, 45.20942372801901854 ) ) ;
#2735=CARTESIAN_POINT ( 'NONE',  ( 10.81492255796106328, -18.62759615963255655, 30.41775706135234358 ) ) ;
#2737=CARTESIAN_POINT ( 'NONE',  ( -19.05341960407611168, -5.049401038298163336, 86.45724293864769550 ) ) ;
#2739=CARTESIAN_POINT ( 'NONE',  ( 16.55341960407618274, -4.379528057220086978, 41.04275706135236135 ) ) ;
#2740=CARTESIAN_POINT ( 'NONE',  ( 18.62759615963271287, -10.81492255796078972, 38.33224293864768839 ) ) ;
#2741=CARTESIAN_POINT ( 'NONE',  ( 15.72974639402176855, 15.80617190586768217, 76.87609039468567573 ) ) ;
#2743=CARTESIAN_POINT ( 'NONE',  ( 13.89961937509957401, 13.97604488694547697, 111.8760903946856757 ) ) ;
#2744=CARTESIAN_POINT ( 'NONE',  ( -16.51473224551069308, -9.474510206698971260, 66.66557627198102409 ) ) ;
#2745=CARTESIAN_POINT ( 'NONE',  ( -16.46253265017160317, 9.564922557960807481, 85.83224293864769550 ) ) ;
#2747=CARTESIAN_POINT ( 'NONE',  ( -16.53943276465976808, 0.05219959533911058130, 106.2489096053143811 ) ) ;
#2748=CARTESIAN_POINT ( 'NONE',  ( 8.224510206698953496, -14.34966873604960469, 102.9155762719810383 ) ) ;
#2749=CARTESIAN_POINT ( 'NONE',  ( -9.474510206698964154, 16.51473224551069663, 105.4155762719810383 ) ) ;
#2750=CARTESIAN_POINT ( 'NONE',  ( 8.224510206698742110, 14.34966873604972548, 77.08442372801901854 ) ) ;
#2751=CARTESIAN_POINT ( 'NONE',  ( 14.34966873604960469, 8.224510206698951720, 54.16557627198103120 ) ) ;
#2752=CARTESIAN_POINT ( 'NONE',  ( 13.89961937509977652, -13.97604488694527269, 48.12390960531435979 ) ) ;
#2753=CARTESIAN_POINT ( 'NONE',  ( 21.53943276465977519, 0.05219959533937863772, 76.25109039468568994 ) ) ;
#2754=CARTESIAN_POINT ( 'NONE',  ( 5.719274019375673035, 21.55341960407619339, 77.29275706135234714 ) ) ;
#2755=CARTESIAN_POINT ( 'NONE',  ( -9.564922557961040184, 16.46253265017147172, 107.9177570613523471 ) ) ;
#2756=CARTESIAN_POINT ( 'NONE',  ( 16.55341960407611168, 4.379528057220329451, 68.95724293864769550 ) ) ;
#2757=CARTESIAN_POINT ( 'NONE',  ( -0.05219959533907301413, -21.53943276465977519, 107.4989096053143669 ) ) ;
#2758=CARTESIAN_POINT ( 'NONE',  ( -21.53943276465977519, 0.05219959533907696930, 66.24890960531436690 ) ) ;
#2759=CARTESIAN_POINT ( 'NONE',  ( 19.34837522270366961, 5.499999999999741540, 73.36337684832578532 ) ) ;
#2761=CARTESIAN_POINT ( 'NONE',  ( 16.46253265017160672, -9.564922557960803928, 63.33224293864769550 ) ) ;
#2762=CARTESIAN_POINT ( 'NONE',  ( 14.29746914071049879, -8.314922557960816363, 43.33224293864769550 ) ) ;
#2763=CARTESIAN_POINT ( 'NONE',  ( 8.314922557960818139, 14.29746914071049879, 24.58224293864768839 ) ) ;
#2764=CARTESIAN_POINT ( 'NONE',  ( -4.483927247898782831, 16.52544592524335698, 97.70942372801904696 ) ) ;
#2765=CARTESIAN_POINT ( 'NONE',  ( -19.02544592524334988, -5.153800228976617603, 48.95942372801900433 ) ) ;
#2766=CARTESIAN_POINT ( 'NONE',  ( -17.49999999999999645, -5.500000000000000888, 120.0000000000000142 ) ) ;
#2767=CARTESIAN_POINT ( 'NONE',  ( -16.51473224551069308, -9.474510206698971260, 86.66557627198102409 ) ) ;
#2769=CARTESIAN_POINT ( 'NONE',  ( -8.224510206698948167, 14.34966873604960824, 60.41557627198102409 ) ) ;
#2770=CARTESIAN_POINT ( 'NONE',  ( 16.51473224551069308, 9.474510206698969483, 24.16557627198102765 ) ) ;
#2771=CARTESIAN_POINT ( 'NONE',  ( -15.72974639402197994, 15.80617190586746368, 25.62390960531435624 ) ) ;
#2772=CARTESIAN_POINT ( 'NONE',  ( 15.80617190586746368, 15.72974639402197994, 49.37390960531436690 ) ) ;
#2774=CARTESIAN_POINT ( 'NONE',  ( 14.29746914071049879, -8.314922557960816363, 93.33224293864769550 ) ) ;
#2775=CARTESIAN_POINT ( 'NONE',  ( 12.06949235617739724, 12.14591786802326823, 56.87609039468568994 ) ) ;
#2776=CARTESIAN_POINT ( 'NONE',  ( -12.14591786802309592, -12.06949235617757132, 76.87390960531439532 ) ) ;
#2778=CARTESIAN_POINT ( 'NONE',  ( -19.02544592524334988, -5.153800228976617603, 78.95942372801900433 ) ) ;
#2779=CARTESIAN_POINT ( 'NONE',  ( -19.02544592524342804, 5.153800228976336051, 116.0405762719810383 ) ) ;
#2781=CARTESIAN_POINT ( 'NONE',  ( 19.17291183240702779, 5.499999999999965361, 101.8490549527296452 ) ) ;
#2782=CARTESIAN_POINT ( 'NONE',  ( -12.06949235617739369, -12.14591786802326823, 49.37609039468569705 ) ) ;
#2783=CARTESIAN_POINT ( 'NONE',  ( 16.52544592524342804, -4.483927247898539470, 28.54057627198103120 ) ) ;
#2784=CARTESIAN_POINT ( 'NONE',  ( -18.67979575497178146, -10.72451020669898902, 61.66557627198103120 ) ) ;
#2785=CARTESIAN_POINT ( 'NONE',  ( 9.564922557961047289, -16.46253265017146816, 80.41775706135234714 ) ) ;
#2786=CARTESIAN_POINT ( 'NONE',  ( 18.62759615963271287, -10.81492255796078972, 43.33224293864769550 ) ) ;
#2787=CARTESIAN_POINT ( 'NONE',  ( -21.55341960407619339, 5.719274019375674811, 78.54275706135236135 ) ) ;
#2788=CARTESIAN_POINT ( 'NONE',  ( -17.49999999999999289, 5.500000000000036415, 85.79690382534171533 ) ) ;
#2789=CARTESIAN_POINT ( 'NONE',  ( 14.34966873604972726, -8.224510206698740333, 30.83442372801902209 ) ) ;
#2790=CARTESIAN_POINT ( 'NONE',  ( -9.564922557960796823, -16.46253265017161027, 37.08224293864768839 ) ) ;
#2791=CARTESIAN_POINT ( 'NONE',  ( 16.51473224551069308, 9.474510206698969483, 104.1655762719810241 ) ) ;
#2792=CARTESIAN_POINT ( 'NONE',  ( -16.46253265017160317, 9.564922557960807481, 35.83224293864768839 ) ) ;
#2793=CARTESIAN_POINT ( 'NONE',  ( -12.14591786802309592, -12.06949235617757132, 106.8739096053143811 ) ) ;
#2795=CARTESIAN_POINT ( 'NONE',  ( 5.049401038298161559, -19.05341960407611168, 107.7072429386476955 ) ) ;
#2796=ORIENTED_EDGE ( 'NONE', *, *, #152637, .F. ) ;
#2797=CARTESIAN_POINT ( 'NONE',  ( -4.379528057220086978, -16.55341960407618274, 49.79275706135234714 ) ) ;
#2798=CARTESIAN_POINT ( 'NONE',  ( -5.719274019375978568, 21.55341960407610458, 90.20724293864770971 ) ) ;
#2799=CARTESIAN_POINT ( 'NONE',  ( -19.03943276465977164, 0.05219959533909376836, 41.24890960531435269 ) ) ;
#2800=CARTESIAN_POINT ( 'NONE',  ( -21.53943276465977519, -0.05219959533937600094, 33.75109039468568284 ) ) ;
#2801=CARTESIAN_POINT ( 'NONE',  ( 5.049401038298161559, -19.05341960407611168, 87.70724293864769550 ) ) ;
#2804=CARTESIAN_POINT ( 'NONE',  ( -14.34966873604972548, 8.224510206698743886, 48.33442372801902565 ) ) ;
#2805=CARTESIAN_POINT ( 'NONE',  ( -21.52544592524343514, 5.823673210054127303, 111.0405762719810525 ) ) ;
#2806=CARTESIAN_POINT ( 'NONE',  ( 4.379528057220339221, -16.55341960407611168, 102.7072429386476955 ) ) ;
#2807=CARTESIAN_POINT ( 'NONE',  ( 19.02544592524343514, -5.153800228976328945, 98.54057627198100988 ) ) ;
#2808=CARTESIAN_POINT ( 'NONE',  ( -19.03943276465977164, -0.05219959533935918106, 68.75109039468566152 ) ) ;
#2809=CARTESIAN_POINT ( 'NONE',  ( -13.97604488694547697, 13.89961937509957934, 33.12609039468566863 ) ) ;
#2810=CARTESIAN_POINT ( 'NONE',  ( -10.81492255796078084, -18.62759615963271287, 82.08224293864768129 ) ) ;
#2811=CARTESIAN_POINT ( 'NONE',  ( 9.474510206698729675, 16.51473224551082808, 27.08442372801900433 ) ) ;
#2812=CARTESIAN_POINT ( 'NONE',  ( -12.14591786802326823, 12.06949235617739902, 78.12609039468570415 ) ) ;
#2813=CARTESIAN_POINT ( 'NONE',  ( -16.51473224551069308, -9.474510206698971260, 101.6655762719810241 ) ) ;
#2814=CARTESIAN_POINT ( 'NONE',  ( 5.049401038298161559, -19.05341960407611168, 57.70724293864769550 ) ) ;
#2815=CARTESIAN_POINT ( 'NONE',  ( -21.52544592524334988, -5.823673210054445271, 63.95942372801901854 ) ) ;
#2816=CARTESIAN_POINT ( 'NONE',  ( 21.52544592524334988, 5.823673210054432836, 61.45942372801901854 ) ) ;
#2817=CARTESIAN_POINT ( 'NONE',  ( -5.049401038298153566, 19.05341960407611168, 70.20724293864769550 ) ) ;
#2818=CARTESIAN_POINT ( 'NONE',  ( -0.05219959533937732626, 21.53943276465977519, 47.50109039468568994 ) ) ;
#2820=CARTESIAN_POINT ( 'NONE',  ( -16.46253265017146816, -9.564922557961047289, 94.16775706135233293 ) ) ;
#2821=CARTESIAN_POINT ( 'NONE',  ( 16.51473224551069308, 9.474510206698969483, 49.16557627198102409 ) ) ;
#2822=CARTESIAN_POINT ( 'NONE',  ( 16.51473224551069308, 9.474510206698969483, 94.16557627198103830 ) ) ;
#2823=CARTESIAN_POINT ( 'NONE',  ( 5.049401038298161559, -19.05341960407611168, 62.70724293864769550 ) ) ;
#2824=CARTESIAN_POINT ( 'NONE',  ( 9.564922557960805705, 16.46253265017160317, 114.5822429386476955 ) ) ;
#2825=CARTESIAN_POINT ( 'NONE',  ( 0.05219959533909260263, 19.03943276465977164, 49.99890960531435979 ) ) ;
#2826=CARTESIAN_POINT ( 'NONE',  ( -15.72974639402197994, 15.80617190586746368, 80.62390960531438111 ) ) ;
#2827=CARTESIAN_POINT ( 'NONE',  ( -16.53943276465976808, -0.05219959533934237506, 78.75109039468568994 ) ) ;
#2829=CARTESIAN_POINT ( 'NONE',  ( 13.97604488694548053, -13.89961937509957401, 25.62609039468566507 ) ) ;
#2830=CARTESIAN_POINT ( 'NONE',  ( -19.02544592524342804, 5.153800228976336051, 71.04057627198099567 ) ) ;
#2831=CARTESIAN_POINT ( 'NONE',  ( 4.483927247898545687, 16.52544592524342804, 59.79057627198103120 ) ) ;
#2832=CARTESIAN_POINT ( 'NONE',  ( -4.483927247898539470, -16.52544592524342804, 92.29057627198103830 ) ) ;
#2833=CARTESIAN_POINT ( 'NONE',  ( -19.03943276465977164, 0.05219959533909376836, 96.24890960531436690 ) ) ;
#2834=CARTESIAN_POINT ( 'NONE',  ( 16.46253265017160672, -9.564922557960803928, 98.33224293864769550 ) ) ;
#2835=CARTESIAN_POINT ( 'NONE',  ( 0.05219959533937995610, -21.53943276465977519, 45.00109039468568284 ) ) ;
#2836=CARTESIAN_POINT ( 'NONE',  ( 16.46253265017160672, -9.564922557960803928, 103.3322429386476955 ) ) ;
#2837=CARTESIAN_POINT ( 'NONE',  ( 5.719274019375673035, 21.55341960407619339, 112.2927570613523471 ) ) ;
#2838=CARTESIAN_POINT ( 'NONE',  ( 14.34966873604972726, -8.224510206698740333, 75.83442372801900433 ) ) ;
#2839=CARTESIAN_POINT ( 'NONE',  ( -21.55341960407619339, 5.719274019375674811, 43.54275706135235424 ) ) ;
#2840=CARTESIAN_POINT ( 'NONE',  ( -10.72451020669898014, 18.67979575497178502, 25.41557627198103120 ) ) ;
#2841=CARTESIAN_POINT ( 'NONE',  ( 5.719274019375991003, -21.55341960407610458, 97.70724293864772392 ) ) ;
#2842=CARTESIAN_POINT ( 'NONE',  ( -14.29746914071049879, 8.314922557960819915, 60.83224293864769550 ) ) ;
#2843=CARTESIAN_POINT ( 'NONE',  ( 16.46253265017160672, -9.564922557960803928, 58.33224293864769550 ) ) ;
#2844=CARTESIAN_POINT ( 'NONE',  ( -8.314922557960811034, -14.29746914071050412, 77.08224293864769550 ) ) ;
#2845=CARTESIAN_POINT ( 'NONE',  ( -21.52544592524343514, 5.823673210054127303, 46.04057627198103830 ) ) ;
#2846=CARTESIAN_POINT ( 'NONE',  ( 5.049401038297881783, 19.05341960407617563, 47.29275706135231161 ) ) ;
#2847=CARTESIAN_POINT ( 'NONE',  ( -13.97604488694527625, -13.89961937509977652, 21.87390960531435979 ) ) ;
#2849=CARTESIAN_POINT ( 'NONE',  ( 4.483927247898790824, -16.52544592524335698, 70.20942372801904696 ) ) ;
#2850=CARTESIAN_POINT ( 'NONE',  ( 13.89961937509977652, -13.97604488694527269, 73.12390960531436690 ) ) ;
#2852=CARTESIAN_POINT ( 'NONE',  ( -16.55341960407611168, -4.379528057220339221, 91.45724293864769550 ) ) ;
#2853=CARTESIAN_POINT ( 'NONE',  ( -0.05219959533907301413, -21.53943276465977519, 42.49890960531435979 ) ) ;
#2855=CARTESIAN_POINT ( 'NONE',  ( -16.55341960407617563, 4.379528057220093196, 103.5427570613523613 ) ) ;
#2856=CARTESIAN_POINT ( 'NONE',  ( -19.03943276465977164, -0.05219959533935918106, 108.7510903946856615 ) ) ;
#2857=CARTESIAN_POINT ( 'NONE',  ( -21.53943276465977519, -0.05219959533937600094, 73.75109039468567573 ) ) ;
#2858=CARTESIAN_POINT ( 'NONE',  ( 13.89961937509977652, -13.97604488694527269, 93.12390960531436690 ) ) ;
#2859=CARTESIAN_POINT ( 'NONE',  ( -15.80617190586745835, -15.72974639402198527, 101.8739096053143811 ) ) ;
#2860=CARTESIAN_POINT ( 'NONE',  ( 16.53943276465976808, 0.05219959533934440121, 56.25109039468568284 ) ) ;
#2861=CARTESIAN_POINT ( 'NONE',  ( 0.05219959533909260263, 19.03943276465977164, 34.99890960531435979 ) ) ;
#2862=CARTESIAN_POINT ( 'NONE',  ( -8.314922557961024197, 14.29746914071037800, 32.91775706135234714 ) ) ;
#2863=CARTESIAN_POINT ( 'NONE',  ( -19.03943276465977164, -0.05219959533935918106, 98.75109039468567573 ) ) ;
#2864=B_SPLINE_CURVE_WITH_KNOTS ( 'NONE', 3,
 ( #190179, #24336, #51654, #25347, #83975, #85986 ),
 .UNSPECIFIED., .F., .F.,
 ( 4, 2, 4 ),
 ( 0.000000000000000000, 0.0003837532665634992165, 0.0007675065331269984329 ),
 .UNSPECIFIED. ) ;
#2865=CARTESIAN_POINT ( 'NONE',  ( -15.72974639402197994, 15.80617190586746368, 90.62390960531436690 ) ) ;
#2866=CARTESIAN_POINT ( 'NONE',  ( -16.51473224551082808, 9.474510206698731452, 53.33442372801900433 ) ) ;
#2867=DIRECTION ( 'NONE',  ( 0.000000000000000000, -1.000000000000000000, 0.000000000000000000 ) ) ;
#2868=CARTESIAN_POINT ( 'NONE',  ( -5.823673210054116645, -21.52544592524344225, 107.2905762719810525 ) ) ;
#2870=CARTESIAN_POINT ( 'NONE',  ( 19.03943276465977164, -0.05219959533909143690, 73.74890960531435269 ) ) ;
#2871=CARTESIAN_POINT ( 'NONE',  ( -12.06949235617739369, -12.14591786802326823, 39.37609039468567573 ) ) ;
#2872=CARTESIAN_POINT ( 'NONE',  ( -18.09805431107524143, 5.499999999999980460, 101.0160622929189032 ) ) ;
#2873=CARTESIAN_POINT ( 'NONE',  ( -19.05341960407617563, 5.049401038297882671, 58.54275706135234003 ) ) ;
#2874=CARTESIAN_POINT ( 'NONE',  ( 5.719274019375673035, 21.55341960407619339, 22.29275706135235069 ) ) ;
#2875=CARTESIAN_POINT ( 'NONE',  ( -8.224510206698948167, 14.34966873604960824, 60.41557627198102409 ) ) ;
#2876=CARTESIAN_POINT ( 'NONE',  ( -0.05219959533909027116, -19.03943276465977164, 72.49890960531435269 ) ) ;
#2877=CARTESIAN_POINT ( 'NONE',  ( 16.52544592524335698, 4.483927247898782831, 41.45942372801901143 ) ) ;
#2878=CARTESIAN_POINT ( 'NONE',  ( 13.89961937509957401, 13.97604488694547697, 41.87609039468566152 ) ) ;
#2879=CARTESIAN_POINT ( 'NONE',  ( 5.719274019375673035, 21.55341960407619339, 47.29275706135234003 ) ) ;
#2880=CARTESIAN_POINT ( 'NONE',  ( 16.51473224551083163, -9.474510206698727899, 110.8344237280190043 ) ) ;
#2881=CARTESIAN_POINT ( 'NONE',  ( 9.474510206698971260, -16.51473224551069308, 52.91557627198102409 ) ) ;
#2882=CARTESIAN_POINT ( 'NONE',  ( 16.51473224551083163, -9.474510206698727899, 75.83442372801900433 ) ) ;
#2883=CARTESIAN_POINT ( 'NONE',  ( -5.823673210054431948, 21.52544592524334988, 97.70942372801904696 ) ) ;
#2884=CARTESIAN_POINT ( 'NONE',  ( 13.89961937509957401, 13.97604488694547697, 66.87609039468567573 ) ) ;
#2885=CARTESIAN_POINT ( 'NONE',  ( 5.049401038298161559, -19.05341960407611168, 42.70724293864767418 ) ) ;
#2886=CARTESIAN_POINT ( 'NONE',  ( -10.72451020669898014, 18.67979575497178502, 75.41557627198102409 ) ) ;
#2887=CARTESIAN_POINT ( 'NONE',  ( 14.34966873604960469, 8.224510206698951720, 59.16557627198103120 ) ) ;
#2888=CARTESIAN_POINT ( 'NONE',  ( -16.46253265017146816, -9.564922557961047289, 64.16775706135233293 ) ) ;
#2890=CARTESIAN_POINT ( 'NONE',  ( 19.05341960407617918, -5.049401038297876454, 26.04275706135233293 ) ) ;
#2891=CARTESIAN_POINT ( 'NONE',  ( 4.379528057220092307, 16.55341960407617563, 92.29275706135236135 ) ) ;
#2892=CARTESIAN_POINT ( 'NONE',  ( -16.52544592524342804, 4.483927247898546575, 51.04057627198103120 ) ) ;
#2893=CARTESIAN_POINT ( 'NONE',  ( -15.72974639402176322, -15.80617190586768395, 84.37609039468570415 ) ) ;
#2895=CARTESIAN_POINT ( 'NONE',  ( 21.55341960407610458, 5.719274019375980345, 93.95724293864770971 ) ) ;
#2896=CARTESIAN_POINT ( 'NONE',  ( 19.05341960407611168, 5.049401038298154454, 48.95724293864768129 ) ) ;
#2897=CARTESIAN_POINT ( 'NONE',  ( 5.823673210054444382, -21.52544592524334988, 65.20942372801901854 ) ) ;
#2898=CARTESIAN_POINT ( 'NONE',  ( 16.51473224551069308, 9.474510206698969483, 44.16557627198103120 ) ) ;
#2900=CARTESIAN_POINT ( 'NONE',  ( 16.46253265017160672, -9.564922557960803928, 63.33224293864769550 ) ) ;
#2901=CARTESIAN_POINT ( 'NONE',  ( 16.52544592524342804, -4.483927247898539470, 108.5405762719810241 ) ) ;
#2902=CARTESIAN_POINT ( 'NONE',  ( -13.89961937509977652, 13.97604488694528158, 105.6239096053143527 ) ) ;
#2903=CARTESIAN_POINT ( 'NONE',  ( 4.483927247898545687, 16.52544592524342804, 59.79057627198103120 ) ) ;
#2904=CARTESIAN_POINT ( 'NONE',  ( -5.153800228976328057, -19.02544592524343514, 32.29057627198102409 ) ) ;
#2905=CARTESIAN_POINT ( 'NONE',  ( 16.52544592524342804, -4.483927247898539470, 88.54057627198103830 ) ) ;
#2906=CARTESIAN_POINT ( 'NONE',  ( -15.80617190586745835, -15.72974639402198527, 96.87390960531436690 ) ) ;
#2907=CARTESIAN_POINT ( 'NONE',  ( -21.52544592524334988, -5.823673210054445271, 28.95942372801902209 ) ) ;
#2909=CARTESIAN_POINT ( 'NONE',  ( -16.52544592524335698, -4.483927247898792601, 48.95942372801902565 ) ) ;
#2910=CARTESIAN_POINT ( 'NONE',  ( -21.53943276465977519, 0.05219959533907696930, 86.24890960531436690 ) ) ;
#2911=CARTESIAN_POINT ( 'NONE',  ( -18.62759615963255300, -10.81492255796106328, 104.1677570613523471 ) ) ;
#2912=CARTESIAN_POINT ( 'NONE',  ( -19.03943276465977164, 0.05219959533909376836, 96.24890960531436690 ) ) ;
#2913=CARTESIAN_POINT ( 'NONE',  ( -21.55341960407619339, 5.719274019375674811, 48.54275706135234714 ) ) ;
#2915=CARTESIAN_POINT ( 'NONE',  ( -18.62759615963270932, 10.81492255796079327, 35.83224293864768839 ) ) ;
#2916=CARTESIAN_POINT ( 'NONE',  ( -8.314922557961024197, 14.29746914071037800, 102.9177570613523756 ) ) ;
#2917=CARTESIAN_POINT ( 'NONE',  ( 0.05219959533937995610, -21.53943276465977519, 60.00109039468568284 ) ) ;
#2918=CARTESIAN_POINT ( 'NONE',  ( 21.53943276465977519, 0.05219959533937863772, 81.25109039468568994 ) ) ;
#2919=CARTESIAN_POINT ( 'NONE',  ( 5.049401038297881783, 19.05341960407617563, 37.29275706135232582 ) ) ;
#2920=CARTESIAN_POINT ( 'NONE',  ( -8.314922557961024197, 14.29746914071037800, 87.91775706135234714 ) ) ;
#2921=CARTESIAN_POINT ( 'NONE',  ( 5.719274019375673035, 21.55341960407619339, 42.29275706135235424 ) ) ;
#2922=CARTESIAN_POINT ( 'NONE',  ( 19.03943276465977164, -0.05219959533909143690, 43.74890960531435979 ) ) ;
#2923=CARTESIAN_POINT ( 'NONE',  ( -18.67979575497193778, 10.72451020669871902, 108.3344237280190185 ) ) ;
#2924=CARTESIAN_POINT ( 'NONE',  ( -21.55341960407610458, -5.719274019375992779, 21.45724293864769550 ) ) ;
#2925=CARTESIAN_POINT ( 'NONE',  ( 0.05219959533907565091, 21.53943276465977519, 114.9989096053143669 ) ) ;
#2926=CARTESIAN_POINT ( 'NONE',  ( 18.67979575497178502, 10.72451020669898547, 79.16557627198103830 ) ) ;
#2928=CARTESIAN_POINT ( 'NONE',  ( 0.05219959533907565091, 21.53943276465977519, 69.99890960531435269 ) ) ;
#2929=CARTESIAN_POINT ( 'NONE',  ( -16.52544592524335698, -4.483927247898792601, 53.95942372801900433 ) ) ;
#2930=CARTESIAN_POINT ( 'NONE',  ( 14.29746914071049879, -8.314922557960816363, 58.33224293864768839 ) ) ;
#2932=CARTESIAN_POINT ( 'NONE',  ( -19.03943276465977164, -0.05219959533935918106, 93.75109039468566152 ) ) ;
#2934=CARTESIAN_POINT ( 'NONE',  ( 14.29746914071037800, 8.314922557961029526, 26.66775706135235424 ) ) ;
#2935=CARTESIAN_POINT ( 'NONE',  ( 0.05219959533907565091, 21.53943276465977519, 99.99890960531436690 ) ) ;
#2936=CARTESIAN_POINT ( 'NONE',  ( -15.80617190586745835, -15.72974639402198527, 71.87390960531438111 ) ) ;
#2937=CARTESIAN_POINT ( 'NONE',  ( -16.51473224551069308, -9.474510206698971260, 111.6655762719810383 ) ) ;
#2938=CARTESIAN_POINT ( 'NONE',  ( 0.05219959533934541429, -16.53943276465976808, 55.00109039468568284 ) ) ;
#2939=CARTESIAN_POINT ( 'NONE',  ( -5.153800228976328057, -19.02544592524343514, 72.29057627198102409 ) ) ;
#2940=CARTESIAN_POINT ( 'NONE',  ( 15.80617190586769283, -15.72974639402175789, 45.62609039468567573 ) ) ;
#2941=CARTESIAN_POINT ( 'NONE',  ( -4.379528057220086978, -16.55341960407618274, 19.79275706135235069 ) ) ;
#2942=CARTESIAN_POINT ( 'NONE',  ( -13.89961937509977652, 13.97604488694528158, 110.6239096053143243 ) ) ;
#2943=CARTESIAN_POINT ( 'NONE',  ( -19.02544592524334988, -5.153800228976617603, 28.95942372801900433 ) ) ;
#2944=CARTESIAN_POINT ( 'NONE',  ( 0.05219959533909260263, 19.03943276465977164, 104.9989096053143669 ) ) ;
#2945=CARTESIAN_POINT ( 'NONE',  ( -10.72451020669898014, 18.67979575497178502, 105.4155762719810383 ) ) ;
#2946=CARTESIAN_POINT ( 'NONE',  ( 5.153800228976335163, 19.02544592524342804, 64.79057627198100988 ) ) ;
#2948=CARTESIAN_POINT ( 'NONE',  ( 12.06949235617757843, -12.14591786802309237, 83.12390960531436690 ) ) ;
#2949=CARTESIAN_POINT ( 'NONE',  ( -0.05219959533909027116, -19.03943276465977164, 112.4989096053143669 ) ) ;
#2950=CARTESIAN_POINT ( 'NONE',  ( -16.79531203550644491, 7.028104445595745098, 33.74755011779555502 ) ) ;
#2951=CARTESIAN_POINT ( 'NONE',  ( -10.81492255796078084, -18.62759615963271287, 107.0822429386476955 ) ) ;
#2952=CARTESIAN_POINT ( 'NONE',  ( -19.03943276465977164, -0.05219959533935918106, 63.75109039468566863 ) ) ;
#2953=CARTESIAN_POINT ( 'NONE',  ( 13.97604488694527802, 13.89961937509977652, 109.3739096053143669 ) ) ;
#2954=CARTESIAN_POINT ( 'NONE',  ( -9.564922557960796823, -16.46253265017161027, 32.08224293864769550 ) ) ;
#2955=CARTESIAN_POINT ( 'NONE',  ( -0.05219959533907301413, -21.53943276465977519, 57.49890960531435979 ) ) ;
#2956=CARTESIAN_POINT ( 'NONE',  ( -9.474510206698964154, 16.51473224551069663, 95.41557627198102409 ) ) ;
#2957=CARTESIAN_POINT ( 'NONE',  ( -18.62759615963255300, -10.81492255796106328, 79.16775706135234714 ) ) ;
#2958=CARTESIAN_POINT ( 'NONE',  ( -13.97604488694527625, -13.89961937509977652, 46.87390960531435979 ) ) ;
#2959=CARTESIAN_POINT ( 'NONE',  ( 4.483927247898545687, 16.52544592524342804, 84.79057627198102409 ) ) ;
#2960=CARTESIAN_POINT ( 'NONE',  ( -16.53943276465976808, -0.05219959533934237506, 33.75109039468568284 ) ) ;
#2961=CARTESIAN_POINT ( 'NONE',  ( 5.823673210054444382, -21.52544592524334988, 70.20942372801904696 ) ) ;
#2963=CARTESIAN_POINT ( 'NONE',  ( -16.51473224551082808, 9.474510206698731452, 23.33442372801900078 ) ) ;
#2964=CARTESIAN_POINT ( 'NONE',  ( -5.153800228976607833, 19.02544592524334988, 82.70942372801897591 ) ) ;
#2965=CARTESIAN_POINT ( 'NONE',  ( 5.049401038297881783, 19.05341960407617563, 37.29275706135232582 ) ) ;
#2967=CARTESIAN_POINT ( 'NONE',  ( 15.72974639402176855, 15.80617190586768217, 36.87609039468568994 ) ) ;
#2968=CARTESIAN_POINT ( 'NONE',  ( -19.52851543214742946, -5.500000000000037303, 45.39357721762583964 ) ) ;
#2969=CARTESIAN_POINT ( 'NONE',  ( -9.564922557961040184, 16.46253265017147172, 27.91775706135232582 ) ) ;
#2970=CARTESIAN_POINT ( 'NONE',  ( -5.153800228976328057, -19.02544592524343514, 72.29057627198102409 ) ) ;
#2971=CARTESIAN_POINT ( 'NONE',  ( -8.224510206698948167, 14.34966873604960824, 25.41557627198103120 ) ) ;
#2972=CARTESIAN_POINT ( 'NONE',  ( -10.81492255796078084, -18.62759615963271287, 27.08224293864769550 ) ) ;
#2973=CARTESIAN_POINT ( 'NONE',  ( -5.719274019375665041, -21.55341960407619695, 89.79275706135236135 ) ) ;
#2974=CIRCLE ( 'NONE', #183833, 2.500000000000002220 ) ;
#2976=CARTESIAN_POINT ( 'NONE',  ( -17.50000000000015277, -3.292511757969575292, 34.93479729789483201 ) ) ;
#2977=CARTESIAN_POINT ( 'NONE',  ( 15.80617190586769283, -15.72974639402175789, 80.62609039468567573 ) ) ;
#2978=CARTESIAN_POINT ( 'NONE',  ( 17.13100169013300089, -6.664070546373147330, 43.26789835699850784 ) ) ;
#2979=CARTESIAN_POINT ( 'NONE',  ( -19.05341960407611168, -5.049401038298163336, 106.4572429386476955 ) ) ;
#2981=CARTESIAN_POINT ( 'NONE',  ( 13.89961937509977652, -13.97604488694527269, 48.12390960531435979 ) ) ;
#2982=CARTESIAN_POINT ( 'NONE',  ( -5.823673210054116645, -21.52544592524344225, 52.29057627198102409 ) ) ;
#2983=CARTESIAN_POINT ( 'NONE',  ( -0.05219959533910754901, -16.53943276465976808, 32.49890960531435979 ) ) ;
#2984=CARTESIAN_POINT ( 'NONE',  ( -14.29746914071049879, 8.314922557960819915, 110.8322429386476955 ) ) ;
#2985=CARTESIAN_POINT ( 'NONE',  ( 19.02544592524343514, -5.153800228976328945, 88.54057627198102409 ) ) ;
#2986=CARTESIAN_POINT ( 'NONE',  ( 19.02544592524334988, 5.153800228976608722, 26.45942372801899722 ) ) ;
#2988=CARTESIAN_POINT ( 'NONE',  ( -16.53943276465976808, 0.05219959533911058130, 96.24890960531435269 ) ) ;
#2989=CARTESIAN_POINT ( 'NONE',  ( -21.53943276465977519, -0.05219959533937600094, 58.75109039468568994 ) ) ;
#2990=CARTESIAN_POINT ( 'NONE',  ( -0.05219959533909027116, -19.03943276465977164, 112.4989096053143669 ) ) ;
#2991=CARTESIAN_POINT ( 'NONE',  ( -16.52544592524335698, -4.483927247898792601, 103.9594237280190185 ) ) ;
#2992=CARTESIAN_POINT ( 'NONE',  ( -19.03943276465977164, -0.05219959533935918106, 63.75109039468566863 ) ) ;
#2994=CARTESIAN_POINT ( 'NONE',  ( 16.51473224551069308, 9.474510206698969483, 114.1655762719810241 ) ) ;
#2995=CARTESIAN_POINT ( 'NONE',  ( -16.53943276465976808, 0.05219959533911058130, 76.24890960531435269 ) ) ;
#2996=CARTESIAN_POINT ( 'NONE',  ( -13.97604488694547697, 13.89961937509957934, 63.12609039468566152 ) ) ;
#2997=CARTESIAN_POINT ( 'NONE',  ( 13.97604488694527802, 13.89961937509977652, 64.37390960531436690 ) ) ;
#2999=CARTESIAN_POINT ( 'NONE',  ( -16.52544592524342804, 4.483927247898546575, 56.04057627198102409 ) ) ;
#3000=CARTESIAN_POINT ( 'NONE',  ( -9.474510206698720793, -16.51473224551083518, 94.58442372801900433 ) ) ;
#3001=CARTESIAN_POINT ( 'NONE',  ( 21.53943276465977519, -0.05219959533907433946, 53.74890960531437401 ) ) ;
#3004=CARTESIAN_POINT ( 'NONE',  ( -16.55341960407611168, -4.379528057220339221, 101.4572429386476955 ) ) ;
#3005=CARTESIAN_POINT ( 'NONE',  ( -16.36317988757057762, -7.306389748694950725, 30.90210391636774290 ) ) ;
#3006=CARTESIAN_POINT ( 'NONE',  ( 5.153800228976335163, 19.02544592524342804, 64.79057627198100988 ) ) ;
#3007=CARTESIAN_POINT ( 'NONE',  ( 5.719274019375991003, -21.55341960407610458, 57.70724293864770260 ) ) ;
#3008=CARTESIAN_POINT ( 'NONE',  ( 12.14591786802327356, -12.06949235617739191, 90.62609039468567573 ) ) ;
#3009=CARTESIAN_POINT ( 'NONE',  ( 0.05219959533909260263, 19.03943276465977164, 79.99890960531436690 ) ) ;
#3010=CARTESIAN_POINT ( 'NONE',  ( -9.474510206698720793, -16.51473224551083518, 59.58442372801900433 ) ) ;
#3011=CARTESIAN_POINT ( 'NONE',  ( 15.72974639402176855, 15.80617190586768217, 81.87609039468568994 ) ) ;
#3012=ORIENTED_EDGE ( 'NONE', *, *, #25923, .F. ) ;
#3013=CARTESIAN_POINT ( 'NONE',  ( -18.62759615963270932, 10.81492255796079327, 65.83224293864769550 ) ) ;
#3014=CARTESIAN_POINT ( 'NONE',  ( -19.02544592524342804, 5.153800228976336051, 101.0405762719810241 ) ) ;
#3015=CARTESIAN_POINT ( 'NONE',  ( -19.03943276465977164, 0.05219959533909376836, 41.24890960531435269 ) ) ;
#3016=CARTESIAN_POINT ( 'NONE',  ( -14.29746914071037622, -8.314922557961029526, 89.16775706135236135 ) ) ;
#3017=CARTESIAN_POINT ( 'NONE',  ( -5.153800228976607833, 19.02544592524334988, 97.70942372801900433 ) ) ;
#3018=CARTESIAN_POINT ( 'NONE',  ( 16.51473224551069308, 9.474510206698969483, 24.16557627198102765 ) ) ;
#3019=CARTESIAN_POINT ( 'NONE',  ( 17.05116617787827238, 6.768360034955700932, 53.84324446740803438 ) ) ;
#3020=CARTESIAN_POINT ( 'NONE',  ( 10.72451020669871369, 18.67979575497193778, 92.08442372801901854 ) ) ;
#3022=CARTESIAN_POINT ( 'NONE',  ( 16.52544592524342804, -4.483927247898539470, 63.54057627198103830 ) ) ;
#3023=CARTESIAN_POINT ( 'NONE',  ( -16.53943276465976808, 0.05219959533911058130, 71.24890960531435269 ) ) ;
#3024=CARTESIAN_POINT ( 'NONE',  ( 10.81492255796078972, 18.62759615963270932, 94.58224293864769550 ) ) ;
#3025=CARTESIAN_POINT ( 'NONE',  ( -10.72451020669898014, 18.67979575497178502, 90.41557627198103830 ) ) ;
#3026=CARTESIAN_POINT ( 'NONE',  ( 16.29526858892875296, -7.335722546920107945, 96.70329402199793378 ) ) ;
#3027=CARTESIAN_POINT ( 'NONE',  ( 15.80617190586746368, 15.72974639402197994, 49.37390960531436690 ) ) ;
#3028=CARTESIAN_POINT ( 'NONE',  ( 8.314922557961029526, -14.29746914071037800, 65.41775706135234714 ) ) ;
#3029=CARTESIAN_POINT ( 'NONE',  ( -16.53943276465976808, 0.05219959533911058130, 91.24890960531436690 ) ) ;
#3030=CARTESIAN_POINT ( 'NONE',  ( -13.89961937509977652, 13.97604488694528158, 40.62390960531435979 ) ) ;
#3032=CARTESIAN_POINT ( 'NONE',  ( -4.483927247898782831, 16.52544592524335698, 92.70942372801901854 ) ) ;
#3033=CARTESIAN_POINT ( 'NONE',  ( -15.72974639402176322, -15.80617190586768395, 34.37609039468568284 ) ) ;
#3034=CARTESIAN_POINT ( 'NONE',  ( 13.97604488694527802, 13.89961937509977652, 79.37390960531435269 ) ) ;
#3035=CARTESIAN_POINT ( 'NONE',  ( -5.823673210054431948, 21.52544592524334988, 72.70942372801901854 ) ) ;
#3038=ORIENTED_EDGE ( 'NONE', *, *, #106448, .F. ) ;
#3039=CARTESIAN_POINT ( 'NONE',  ( 10.81492255796106328, -18.62759615963255655, 55.41775706135234714 ) ) ;
#3040=CARTESIAN_POINT ( 'NONE',  ( -19.05341960407611168, -5.049401038298163336, 36.45724293864766707 ) ) ;
#3041=CARTESIAN_POINT ( 'NONE',  ( 16.46253265017160672, -9.564922557960803928, 113.3322429386476955 ) ) ;
#3042=CARTESIAN_POINT ( 'NONE',  ( 16.46253265017160672, -9.564922557960803928, 88.33224293864769550 ) ) ;
#3043=CARTESIAN_POINT ( 'NONE',  ( 13.97604488694548053, -13.89961937509957401, 60.62609039468564731 ) ) ;
#3044=CARTESIAN_POINT ( 'NONE',  ( 15.80617190586769283, -15.72974639402175789, 30.62609039468567929 ) ) ;
#3045=CARTESIAN_POINT ( 'NONE',  ( -16.46253265017146816, -9.564922557961047289, 54.16775706135234003 ) ) ;
#3046=CARTESIAN_POINT ( 'NONE',  ( 16.46253265017160672, -9.564922557960803928, 43.33224293864769550 ) ) ;
#3047=CARTESIAN_POINT ( 'NONE',  ( -16.55341960407617563, 4.379528057220093196, 98.54275706135234714 ) ) ;
#3048=CARTESIAN_POINT ( 'NONE',  ( -13.89961937509957401, -13.97604488694547875, 69.37609039468564731 ) ) ;
#3049=CARTESIAN_POINT ( 'NONE',  ( -4.379528057220328563, 16.55341960407611168, 25.20724293864769550 ) ) ;
#3050=CARTESIAN_POINT ( 'NONE',  ( -19.03943276465977164, -0.05219959533935918106, 53.75109039468566863 ) ) ;
#3051=CARTESIAN_POINT ( 'NONE',  ( 16.46253265017160672, -9.564922557960803928, 103.3322429386476955 ) ) ;
#3052=CARTESIAN_POINT ( 'NONE',  ( -15.72974639402176322, -15.80617190586768395, 104.3760903946856899 ) ) ;
#3053=CARTESIAN_POINT ( 'NONE',  ( -18.67979575497193778, 10.72451020669871902, 108.3344237280190185 ) ) ;
#3055=CARTESIAN_POINT ( 'NONE',  ( 21.55341960407619695, -5.719274019375665929, 86.04275706135236135 ) ) ;
#3056=CARTESIAN_POINT ( 'NONE',  ( -12.06949235617739369, -12.14591786802326823, 29.37609039468568284 ) ) ;
#3057=CARTESIAN_POINT ( 'NONE',  ( -5.153800228976328057, -19.02544592524343514, 97.29057627198099567 ) ) ;
#3059=CARTESIAN_POINT ( 'NONE',  ( -5.049401038298153566, 19.05341960407611168, 85.20724293864766707 ) ) ;
#3060=DIRECTION ( 'NONE',  ( -1.000000000000000000, -0.000000000000000000, -0.000000000000000000 ) ) ;
#3061=CARTESIAN_POINT ( 'NONE',  ( -0.05219959533936034679, 19.03943276465977164, 67.50109039468566152 ) ) ;
#3062=CARTESIAN_POINT ( 'NONE',  ( -9.564922557960796823, -16.46253265017161027, 112.0822429386476955 ) ) ;
#3063=CARTESIAN_POINT ( 'NONE',  ( 21.53943276465977519, 0.05219959533937863772, 101.2510903946856757 ) ) ;
#3064=CARTESIAN_POINT ( 'NONE',  ( 14.34966873604960469, 8.224510206698951720, 99.16557627198100988 ) ) ;
#3065=CARTESIAN_POINT ( 'NONE',  ( -15.72974639402197994, 15.80617190586746368, 50.62390960531435979 ) ) ;
#3066=CARTESIAN_POINT ( 'NONE',  ( -21.55341960407610458, -5.719274019375992779, 31.45724293864769550 ) ) ;
#3067=CARTESIAN_POINT ( 'NONE',  ( -8.314922557960811034, -14.29746914071050412, 102.0822429386476955 ) ) ;
#3069=CARTESIAN_POINT ( 'NONE',  ( -19.02544592524334988, -5.153800228976617603, 53.95942372801898301 ) ) ;
#3070=CARTESIAN_POINT ( 'NONE',  ( -12.06949235617756955, 12.14591786802309770, 30.62390960531436335 ) ) ;
#3071=B_SPLINE_CURVE_WITH_KNOTS ( 'NONE', 3,
 ( #188981, #130245, #82752, #4917, #145428, #37259, #66600, #116102, #175785, #34287, #80772, #98917, #160609, #128264, #189962, #53425, #115102, #131265, #176794, #38267, #142450, #99921, #23100, #69598, #51437, #3928, #127268, #146423, #113097, #174788, #7914, #192953 ),
 .UNSPECIFIED., .F., .F.,
 ( 4, 2, 2, 2, 2, 2, 2, 2, 2, 2, 2, 2, 2, 2, 2, 4 ),
 ( 2.969368287472575283E-17, 0.0003712461730036993547, 0.0007424923460073690022, 0.001113738519011038758, 0.001484984692014708297, 0.002227477038022045424, 0.002598723211025721468, 0.002969969384029397079, 0.003341215557033072690, 0.003712461730036748300, 0.004083707903040423477, 0.004454954076044099522, 0.004826200249047774699, 0.005197446422051450743, 0.005568692595055125920, 0.005939938768058801964 ),
 .UNSPECIFIED. ) ;
#3072=CARTESIAN_POINT ( 'NONE',  ( -19.02544592524342804, 5.153800228976336051, 106.0405762719810241 ) ) ;
#3073=CARTESIAN_POINT ( 'NONE',  ( 15.72974639402176855, 15.80617190586768217, 81.87609039468568994 ) ) ;
#3074=CARTESIAN_POINT ( 'NONE',  ( 18.67979575497178502, 10.72451020669898547, 69.16557627198102409 ) ) ;
#3075=CARTESIAN_POINT ( 'NONE',  ( 15.72974639402176855, 15.80617190586768217, 41.87609039468568284 ) ) ;
#3076=CARTESIAN_POINT ( 'NONE',  ( 15.80617190586746368, 15.72974639402197994, 99.37390960531436690 ) ) ;
#3077=CARTESIAN_POINT ( 'NONE',  ( -15.72974639402176322, -15.80617190586768395, 49.37609039468569705 ) ) ;
#3078=CARTESIAN_POINT ( 'NONE',  ( 9.564922557960805705, 16.46253265017160317, 29.58224293864769550 ) ) ;
#3079=CARTESIAN_POINT ( 'NONE',  ( 19.03943276465977164, -0.05219959533909143690, 88.74890960531436690 ) ) ;
#3080=CARTESIAN_POINT ( 'NONE',  ( -14.29746914071037622, -8.314922557961029526, 79.16775706135234714 ) ) ;
#3081=CARTESIAN_POINT ( 'NONE',  ( -16.55341960407611168, -4.379528057220339221, 106.4572429386477097 ) ) ;
#3082=CARTESIAN_POINT ( 'NONE',  ( 19.02544592524343514, -5.153800228976328945, 113.5405762719810241 ) ) ;
#3083=CARTESIAN_POINT ( 'NONE',  ( 8.314922557960818139, 14.29746914071049879, 59.58224293864770260 ) ) ;
#3084=CARTESIAN_POINT ( 'NONE',  ( -8.224510206698735004, -14.34966873604973081, 109.5844237280190328 ) ) ;
#3085=CARTESIAN_POINT ( 'NONE',  ( 5.153800228976335163, 19.02544592524342804, 49.79057627198100988 ) ) ;
#3086=CARTESIAN_POINT ( 'NONE',  ( -19.02544592524342804, 5.153800228976336051, 31.04057627198102409 ) ) ;
#3087=CARTESIAN_POINT ( 'NONE',  ( -10.81492255796078084, -18.62759615963271287, 47.08224293864770260 ) ) ;
#3088=CARTESIAN_POINT ( 'NONE',  ( -19.03943276465977164, -0.05219959533935918106, 33.75109039468566863 ) ) ;
#3089=LINE ( 'NONE', #34429, #184950 ) ;
#3090=CARTESIAN_POINT ( 'NONE',  ( 0.05219959533910956823, 16.53943276465976808, 29.99890960531435979 ) ) ;
#3091=CARTESIAN_POINT ( 'NONE',  ( -21.52544592524334988, -5.823673210054445271, 43.95942372801902565 ) ) ;
#3093=CARTESIAN_POINT ( 'NONE',  ( -4.379528057220086978, -16.55341960407618274, 54.79275706135235424 ) ) ;
#3094=CARTESIAN_POINT ( 'NONE',  ( -16.46253265017146816, -9.564922557961047289, 64.16775706135233293 ) ) ;
#3095=CARTESIAN_POINT ( 'NONE',  ( -12.06949235617756955, 12.14591786802309770, 25.62390960531435624 ) ) ;
#3096=CARTESIAN_POINT ( 'NONE',  ( -18.22780087662123094, -5.499999999999984901, 76.48459894673894155 ) ) ;
#3097=CARTESIAN_POINT ( 'NONE',  ( -8.314922557961024197, 14.29746914071037800, 102.9177570613523756 ) ) ;
#3098=CARTESIAN_POINT ( 'NONE',  ( 19.03943276465977164, -0.05219959533909143690, 33.74890960531435979 ) ) ;
#3099=CARTESIAN_POINT ( 'NONE',  ( 0.05219959533909260263, 19.03943276465977164, 64.99890960531436690 ) ) ;
#3100=CARTESIAN_POINT ( 'NONE',  ( -13.89961937509977652, 13.97604488694528158, 30.62390960531435269 ) ) ;
#3101=CARTESIAN_POINT ( 'NONE',  ( -18.67979575497193778, 10.72451020669871902, 38.33442372801900433 ) ) ;
#3102=CARTESIAN_POINT ( 'NONE',  ( 5.049401038298161559, -19.05341960407611168, 42.70724293864767418 ) ) ;
#3103=CARTESIAN_POINT ( 'NONE',  ( -5.153800228976328057, -19.02544592524343514, 112.2905762719810099 ) ) ;
#3104=CARTESIAN_POINT ( 'NONE',  ( -5.153800228976328057, -19.02544592524343514, 42.29057627198101699 ) ) ;
#3106=CARTESIAN_POINT ( 'NONE',  ( 16.46253265017160672, -9.564922557960803928, 113.3322429386476955 ) ) ;
#3108=CARTESIAN_POINT ( 'NONE',  ( 15.80617190586769283, -15.72974639402175789, 55.62609039468568284 ) ) ;
#3109=CARTESIAN_POINT ( 'NONE',  ( -8.224510206698948167, 14.34966873604960824, 115.4155762719810241 ) ) ;
#3110=CARTESIAN_POINT ( 'NONE',  ( 0.05219959533907565091, 21.53943276465977519, 29.99890960531435979 ) ) ;
#3111=CARTESIAN_POINT ( 'NONE',  ( 14.29746914071037800, 8.314922557961029526, 71.66775706135234714 ) ) ;
#3112=CARTESIAN_POINT ( 'NONE',  ( 10.72451020669871369, 18.67979575497193778, 97.08442372801904696 ) ) ;
#3113=CARTESIAN_POINT ( 'NONE',  ( 0.05219959533934541429, -16.53943276465976808, 50.00109039468568994 ) ) ;
#3114=CARTESIAN_POINT ( 'NONE',  ( 9.474510206698971260, -16.51473224551069308, 92.91557627198103830 ) ) ;
#3115=ADVANCED_FACE ( 'NONE', ( #114370 ), #176313, .T. ) ;
#3116=CARTESIAN_POINT ( 'NONE',  ( -0.05219959533934338120, 16.53943276465976808, 47.50109039468568994 ) ) ;
#3117=CARTESIAN_POINT ( 'NONE',  ( -8.224510206698735004, -14.34966873604973081, 24.58442372801901499 ) ) ;
#3118=CARTESIAN_POINT ( 'NONE',  ( 12.14591786802327356, -12.06949235617739191, 95.62609039468568994 ) ) ;
#3119=CARTESIAN_POINT ( 'NONE',  ( 15.72974639402176855, 15.80617190586768217, 56.87609039468568994 ) ) ;
#3120=CARTESIAN_POINT ( 'NONE',  ( 19.03943276465977164, 0.05219959533936151252, 101.2510903946856757 ) ) ;
#3121=CARTESIAN_POINT ( 'NONE',  ( 5.719274019375991003, -21.55341960407610458, 107.7072429386476955 ) ) ;
#3122=CARTESIAN_POINT ( 'NONE',  ( -4.483927247898539470, -16.52544592524342804, 97.29057627198105251 ) ) ;
#3123=CARTESIAN_POINT ( 'NONE',  ( -19.03943276465977164, -0.05219959533935918106, 103.7510903946856757 ) ) ;
#3124=CARTESIAN_POINT ( 'NONE',  ( -4.379528057220086978, -16.55341960407618274, 74.79275706135234714 ) ) ;
#3125=CARTESIAN_POINT ( 'NONE',  ( -17.49999999999999645, 5.499999999999992895, 43.71769037696436300 ) ) ;
#3126=CARTESIAN_POINT ( 'NONE',  ( 9.474510206698729675, 16.51473224551082808, 77.08442372801900433 ) ) ;
#3127=CARTESIAN_POINT ( 'NONE',  ( -14.34966873604960291, -8.224510206698953496, 46.66557627198102409 ) ) ;
#3128=CARTESIAN_POINT ( 'NONE',  ( 14.29746914071049879, -8.314922557960816363, 48.33224293864770260 ) ) ;
#3129=CARTESIAN_POINT ( 'NONE',  ( -16.55341960407611168, -4.379528057220339221, 96.45724293864770971 ) ) ;
#3130=CARTESIAN_POINT ( 'NONE',  ( 19.02544592524334988, 5.153800228976608722, 31.45942372801900433 ) ) ;
#3131=CARTESIAN_POINT ( 'NONE',  ( -17.50000000000001066, 5.622605283950872668, 88.68792689403889540 ) ) ;
#3132=CARTESIAN_POINT ( 'NONE',  ( -15.72974639402176322, -15.80617190586768395, 34.37609039468568284 ) ) ;
#3133=CARTESIAN_POINT ( 'NONE',  ( 19.03943276465977164, 0.05219959533936151252, 101.2510903946856757 ) ) ;
#3135=CARTESIAN_POINT ( 'NONE',  ( 19.02544592524343514, -5.153800228976328945, 93.54057627198102409 ) ) ;
#3136=CARTESIAN_POINT ( 'NONE',  ( 16.46253265017160672, -9.564922557960803928, 93.33224293864769550 ) ) ;
#3137=CARTESIAN_POINT ( 'NONE',  ( 21.55341960407610458, 5.719274019375980345, 58.95724293864770971 ) ) ;
#3138=CARTESIAN_POINT ( 'NONE',  ( -16.52544592524342804, 4.483927247898546575, 96.04057627198102409 ) ) ;
#3139=CARTESIAN_POINT ( 'NONE',  ( -16.51473224551069308, -9.474510206698971260, 76.66557627198103830 ) ) ;
#3140=CARTESIAN_POINT ( 'NONE',  ( -19.02544592524342804, 5.153800228976336051, 26.04057627198103120 ) ) ;
#3141=CARTESIAN_POINT ( 'NONE',  ( 21.53943276465977519, 0.05219959533937863772, 41.25109039468568284 ) ) ;
#3143=CARTESIAN_POINT ( 'NONE',  ( -5.719274019375665041, -21.55341960407619695, 69.79275706135234714 ) ) ;
#3144=CARTESIAN_POINT ( 'NONE',  ( 0.05219959533934541429, -16.53943276465976808, 90.00109039468567573 ) ) ;
#3145=CARTESIAN_POINT ( 'NONE',  ( 18.67979575497194134, -10.72451020669871369, 30.83442372801902209 ) ) ;
#3146=CARTESIAN_POINT ( 'NONE',  ( 10.81492255796106328, -18.62759615963255655, 30.41775706135234358 ) ) ;
#3147=CARTESIAN_POINT ( 'NONE',  ( -9.564922557961040184, 16.46253265017147172, 57.91775706135233293 ) ) ;
#3148=CARTESIAN_POINT ( 'NONE',  ( -19.02544592524342804, 5.153800228976336051, 81.04057627198103830 ) ) ;
#3149=CARTESIAN_POINT ( 'NONE',  ( -10.72451020669870658, -18.67979575497194134, 89.58442372801901854 ) ) ;
#3151=CARTESIAN_POINT ( 'NONE',  ( 10.81492255796078972, 18.62759615963270932, 79.58224293864769550 ) ) ;
#3152=CARTESIAN_POINT ( 'NONE',  ( 14.29746914071049879, -8.314922557960816363, 53.33224293864769550 ) ) ;
#3153=CARTESIAN_POINT ( 'NONE',  ( 5.719274019375673035, 21.55341960407619339, 97.29275706135234714 ) ) ;
#3154=CARTESIAN_POINT ( 'NONE',  ( -0.05219959533936034679, 19.03943276465977164, 32.50109039468566863 ) ) ;
#3155=CARTESIAN_POINT ( 'NONE',  ( -16.55341960407611168, -4.379528057220339221, 71.45724293864769550 ) ) ;
#3156=CARTESIAN_POINT ( 'NONE',  ( -0.05219959533910754901, -16.53943276465976808, 112.4989096053143669 ) ) ;
#3157=CARTESIAN_POINT ( 'NONE',  ( 16.51473224551083163, -9.474510206698727899, 70.83442372801900433 ) ) ;
#3158=CARTESIAN_POINT ( 'NONE',  ( 8.314922557960818139, 14.29746914071049879, 39.58224293864769550 ) ) ;
#3159=CARTESIAN_POINT ( 'NONE',  ( 5.719274019375673035, 21.55341960407619339, 82.29275706135234714 ) ) ;
#3160=CARTESIAN_POINT ( 'NONE',  ( 19.03943276465977164, -0.05219959533909143690, 78.74890960531436690 ) ) ;
#3161=CARTESIAN_POINT ( 'NONE',  ( -9.564922557961040184, 16.46253265017147172, 62.91775706135233293 ) ) ;
#3162=CARTESIAN_POINT ( 'NONE',  ( 5.719274019375991003, -21.55341960407610458, 62.70724293864769550 ) ) ;
#3163=CARTESIAN_POINT ( 'NONE',  ( 21.52544592524344225, -5.823673210054117533, 113.5405762719810383 ) ) ;
#3164=CARTESIAN_POINT ( 'NONE',  ( -9.474510206698720793, -16.51473224551083518, 109.5844237280190043 ) ) ;
#3165=CARTESIAN_POINT ( 'NONE',  ( -16.55341960407617563, 4.379528057220093196, 78.54275706135236135 ) ) ;
#3166=CARTESIAN_POINT ( 'NONE',  ( 16.79531203550650176, 7.028104445595486638, 63.75244988220443787 ) ) ;
#3167=CARTESIAN_POINT ( 'NONE',  ( 21.53943276465977519, 0.05219959533937863772, 21.25109039468567218 ) ) ;
#3168=CARTESIAN_POINT ( 'NONE',  ( 14.34966873604960469, 8.224510206698951720, 104.1655762719810241 ) ) ;
#3170=CARTESIAN_POINT ( 'NONE',  ( -16.55341960407617563, 4.379528057220093196, 33.54275706135234714 ) ) ;
#3171=CARTESIAN_POINT ( 'NONE',  ( 5.719274019375991003, -21.55341960407610458, 62.70724293864769550 ) ) ;
#3172=CARTESIAN_POINT ( 'NONE',  ( 8.314922557961029526, -14.29746914071037800, 110.4177570613523756 ) ) ;
#3173=CARTESIAN_POINT ( 'NONE',  ( -13.89961937509977652, 13.97604488694528158, 35.62390960531435269 ) ) ;
#3174=CARTESIAN_POINT ( 'NONE',  ( 14.34966873604972726, -8.224510206698740333, 60.83442372801901854 ) ) ;
#3175=CARTESIAN_POINT ( 'NONE',  ( 5.049401038297881783, 19.05341960407617563, 77.29275706135231871 ) ) ;
#3176=CARTESIAN_POINT ( 'NONE',  ( 10.72451020669871369, 18.67979575497193778, 47.08442372801901854 ) ) ;
#3177=CARTESIAN_POINT ( 'NONE',  ( 5.823673210054125526, 21.52544592524343514, 54.79057627198104541 ) ) ;
#3178=CARTESIAN_POINT ( 'NONE',  ( -16.53943276465976808, -0.05219959533934237506, 98.75109039468568994 ) ) ;
#3179=CARTESIAN_POINT ( 'NONE',  ( 21.53943276465977519, 0.05219959533937863772, 86.25109039468568994 ) ) ;
#3180=CARTESIAN_POINT ( 'NONE',  ( 10.81492255796078972, 18.62759615963270932, 49.58224293864769550 ) ) ;
#3181=CARTESIAN_POINT ( 'NONE',  ( -5.823673210054116645, -21.52544592524344225, 52.29057627198102409 ) ) ;
#3182=CARTESIAN_POINT ( 'NONE',  ( 12.14591786802327356, -12.06949235617739191, 75.62609039468567573 ) ) ;
#3183=CARTESIAN_POINT ( 'NONE',  ( 21.53943276465977519, -0.05219959533907433946, 48.74890960531435979 ) ) ;
#3185=CARTESIAN_POINT ( 'NONE',  ( 13.89961937509977652, -13.97604488694527269, 103.1239096053143527 ) ) ;
#3187=CARTESIAN_POINT ( 'NONE',  ( -16.46253265017160317, 9.564922557960807481, 30.83224293864769550 ) ) ;
#3188=CARTESIAN_POINT ( 'NONE',  ( 5.719274019375991003, -21.55341960407610458, 62.70724293864769550 ) ) ;
#3189=CARTESIAN_POINT ( 'NONE',  ( 16.53943276465976808, 0.05219959533934440121, 91.25109039468568994 ) ) ;
#3190=CARTESIAN_POINT ( 'NONE',  ( 21.53943276465977519, 0.05219959533937863772, 46.25109039468567573 ) ) ;
#3191=CARTESIAN_POINT ( 'NONE',  ( -19.02544592524334988, -5.153800228976617603, 108.9594237280189759 ) ) ;
#3192=CARTESIAN_POINT ( 'NONE',  ( 14.34966873604960469, 8.224510206698951720, 104.1655762719810241 ) ) ;
#3193=CARTESIAN_POINT ( 'NONE',  ( 0.05219959533934541429, -16.53943276465976808, 20.00109039468568639 ) ) ;
#3194=CARTESIAN_POINT ( 'NONE',  ( 9.564922557960805705, 16.46253265017160317, 44.58224293864769550 ) ) ;
#3196=CARTESIAN_POINT ( 'NONE',  ( -9.564922557960796823, -16.46253265017161027, 92.08224293864769550 ) ) ;
#3197=CARTESIAN_POINT ( 'NONE',  ( -0.05219959533934338120, 16.53943276465976808, 77.50109039468567573 ) ) ;
#3198=CARTESIAN_POINT ( 'NONE',  ( -10.72451020669870658, -18.67979575497194134, 104.5844237280190185 ) ) ;
#3199=CARTESIAN_POINT ( 'NONE',  ( 18.62759615963271287, -10.81492255796078972, 68.33224293864769550 ) ) ;
#3200=CARTESIAN_POINT ( 'NONE',  ( 4.379528057220092307, 16.55341960407617563, 87.29275706135236135 ) ) ;
#3201=CARTESIAN_POINT ( 'NONE',  ( 16.51473224551083163, -9.474510206698727899, 80.83442372801899012 ) ) ;
#3202=CARTESIAN_POINT ( 'NONE',  ( -19.03943276465977164, 0.05219959533909376836, 31.24890960531435979 ) ) ;
#3203=CARTESIAN_POINT ( 'NONE',  ( 5.153800228976335163, 19.02544592524342804, 79.79057627198102409 ) ) ;
#3204=CARTESIAN_POINT ( 'NONE',  ( 9.564922557960805705, 16.46253265017160317, 29.58224293864769550 ) ) ;
#3205=CARTESIAN_POINT ( 'NONE',  ( 5.049401038297881783, 19.05341960407617563, 67.29275706135234714 ) ) ;
#3207=CARTESIAN_POINT ( 'NONE',  ( -0.05219959533909027116, -19.03943276465977164, 107.4989096053143527 ) ) ;
#3208=CARTESIAN_POINT ( 'NONE',  ( -4.379528057220328563, 16.55341960407611168, 70.20724293864769550 ) ) ;
#3209=CARTESIAN_POINT ( 'NONE',  ( -5.719274019375978568, 21.55341960407610458, 60.20724293864768839 ) ) ;
#3211=CARTESIAN_POINT ( 'NONE',  ( 13.89961937509957401, 13.97604488694547697, 31.87609039468566863 ) ) ;
#3213=CARTESIAN_POINT ( 'NONE',  ( 13.89961937509977652, -13.97604488694527269, 68.12390960531436690 ) ) ;
#3214=CARTESIAN_POINT ( 'NONE',  ( -13.97604488694527625, -13.89961937509977652, 76.87390960531433848 ) ) ;
#3215=CARTESIAN_POINT ( 'NONE',  ( -4.483927247898782831, 16.52544592524335698, 52.70942372801902565 ) ) ;
#3217=CARTESIAN_POINT ( 'NONE',  ( -16.62475595723701005, 7.163666690055290331, 110.5271335181047760 ) ) ;
#3218=CARTESIAN_POINT ( 'NONE',  ( -16.55341960407617563, 4.379528057220093196, 73.54275706135234714 ) ) ;
#3220=CARTESIAN_POINT ( 'NONE',  ( -12.14591786802326823, 12.06949235617739902, 63.12609039468568994 ) ) ;
#3221=CARTESIAN_POINT ( 'NONE',  ( 14.34966873604972726, -8.224510206698740333, 35.83442372801901143 ) ) ;
#3222=CARTESIAN_POINT ( 'NONE',  ( -5.049401038298153566, 19.05341960407611168, 60.20724293864768129 ) ) ;
#3224=CARTESIAN_POINT ( 'NONE',  ( -15.72974639402176322, -15.80617190586768395, 54.37609039468568994 ) ) ;
#3225=CARTESIAN_POINT ( 'NONE',  ( -19.05341960407617563, 5.049401038297882671, 63.54275706135234003 ) ) ;
#3226=CARTESIAN_POINT ( 'NONE',  ( 10.72451020669871369, 18.67979575497193778, 112.0844237280190185 ) ) ;
#3227=CARTESIAN_POINT ( 'NONE',  ( 19.05341960407611168, 5.049401038298154454, 28.95724293864769550 ) ) ;
#3229=CARTESIAN_POINT ( 'NONE',  ( 10.72451020669898902, -18.67979575497178502, 57.91557627198103120 ) ) ;
#3230=CARTESIAN_POINT ( 'NONE',  ( -19.03943276465977164, 0.05219959533909376836, 106.2489096053143669 ) ) ;
#3231=CARTESIAN_POINT ( 'NONE',  ( 14.34966873604960469, 8.224510206698951720, 104.1655762719810241 ) ) ;
#3232=CARTESIAN_POINT ( 'NONE',  ( -0.05219959533934338120, 16.53943276465976808, 42.50109039468567573 ) ) ;
#3233=CARTESIAN_POINT ( 'NONE',  ( 8.224510206698953496, -14.34966873604960469, 27.91557627198103830 ) ) ;
#3234=ORIENTED_EDGE ( 'NONE', *, *, #131252, .T. ) ;
#3235=CARTESIAN_POINT ( 'NONE',  ( 5.719274019375991003, -21.55341960407610458, 97.70724293864772392 ) ) ;
#3236=CARTESIAN_POINT ( 'NONE',  ( -14.29746914071049879, 8.314922557960819915, 40.83224293864769550 ) ) ;
#3237=CARTESIAN_POINT ( 'NONE',  ( 16.46253265017160672, -9.564922557960803928, 113.3322429386476955 ) ) ;
#3238=CARTESIAN_POINT ( 'NONE',  ( 9.564922557961047289, -16.46253265017146816, 90.41775706135234714 ) ) ;
#3239=CARTESIAN_POINT ( 'NONE',  ( -19.05341960407617563, 5.049401038297882671, 23.54275706135233648 ) ) ;
#3240=CARTESIAN_POINT ( 'NONE',  ( -4.483927247898539470, -16.52544592524342804, 27.29057627198103120 ) ) ;
#3241=CARTESIAN_POINT ( 'NONE',  ( -21.52544592524343514, 5.823673210054127303, 101.0405762719810383 ) ) ;
#3242=CARTESIAN_POINT ( 'NONE',  ( 15.80617190586746368, 15.72974639402197994, 49.37390960531436690 ) ) ;
#3243=CARTESIAN_POINT ( 'NONE',  ( -19.03943276465977164, 0.05219959533909376836, 76.24890960531435269 ) ) ;
#3244=CARTESIAN_POINT ( 'NONE',  ( -0.05219959533910754901, -16.53943276465976808, 42.49890960531435979 ) ) ;
#3245=CARTESIAN_POINT ( 'NONE',  ( -5.153800228976328057, -19.02544592524343514, 92.29057627198099567 ) ) ;
#3246=VECTOR ( 'NONE', #122823, 1000.000000000000000 ) ;
#3249=CARTESIAN_POINT ( 'NONE',  ( 9.474510206698729675, 16.51473224551082808, 37.08442372801899722 ) ) ;
#3250=CARTESIAN_POINT ( 'NONE',  ( 21.53943276465977519, -0.05219959533907433946, 83.74890960531435269 ) ) ;
#3251=CARTESIAN_POINT ( 'NONE',  ( 0.05219959533910956823, 16.53943276465976808, 104.9989096053143669 ) ) ;
#3252=CARTESIAN_POINT ( 'NONE',  ( -18.67979575497193778, 10.72451020669871902, 33.33442372801900433 ) ) ;
#3254=CARTESIAN_POINT ( 'NONE',  ( -8.314922557961024197, 14.29746914071037800, 112.9177570613523329 ) ) ;
#3255=CARTESIAN_POINT ( 'NONE',  ( -16.51473224551069308, -9.474510206698971260, 41.66557627198103120 ) ) ;
#3256=CARTESIAN_POINT ( 'NONE',  ( -16.51473224551069308, -9.474510206698971260, 81.66557627198103830 ) ) ;
#3257=CARTESIAN_POINT ( 'NONE',  ( -19.52217212775657273, 5.500000000000115463, 44.93993709005262360 ) ) ;
#3258=CARTESIAN_POINT ( 'NONE',  ( 19.03943276465977164, -0.05219959533909143690, 33.74890960531435979 ) ) ;
#3259=CARTESIAN_POINT ( 'NONE',  ( -0.05219959533910754901, -16.53943276465976808, 37.49890960531436690 ) ) ;
#3261=CARTESIAN_POINT ( 'NONE',  ( -0.05219959533937732626, 21.53943276465977519, 72.50109039468568994 ) ) ;
#3263=CARTESIAN_POINT ( 'NONE',  ( -14.29746914071037622, -8.314922557961029526, 69.16775706135234714 ) ) ;
#3264=CARTESIAN_POINT ( 'NONE',  ( 5.049401038298161559, -19.05341960407611168, 57.70724293864769550 ) ) ;
#3265=CARTESIAN_POINT ( 'NONE',  ( -16.51473224551069308, -9.474510206698971260, 66.66557627198102409 ) ) ;
#3268=CARTESIAN_POINT ( 'NONE',  ( 5.719274019375673035, 21.55341960407619339, 102.2927570613523613 ) ) ;
#3269=CARTESIAN_POINT ( 'NONE',  ( -12.06949235617739369, -12.14591786802326823, 69.37609039468567573 ) ) ;
#3270=CARTESIAN_POINT ( 'NONE',  ( -15.72974639402176322, -15.80617190586768395, 99.37609039468568994 ) ) ;
#3271=CARTESIAN_POINT ( 'NONE',  ( -19.03943276465977164, 0.05219959533909376836, 61.24890960531436690 ) ) ;
#3272=CARTESIAN_POINT ( 'NONE',  ( 5.719274019375991003, -21.55341960407610458, 32.70724293864770260 ) ) ;
#3273=CARTESIAN_POINT ( 'NONE',  ( 13.97604488694548053, -13.89961937509957401, 100.6260903946856615 ) ) ;
#3274=CARTESIAN_POINT ( 'NONE',  ( 21.55341960407619695, -5.719274019375665929, 66.04275706135236135 ) ) ;
#3275=CARTESIAN_POINT ( 'NONE',  ( -4.379528057220086978, -16.55341960407618274, 54.79275706135235424 ) ) ;
#3276=CARTESIAN_POINT ( 'NONE',  ( -15.80617190586745835, -15.72974639402198527, 101.8739096053143811 ) ) ;
#3277=CARTESIAN_POINT ( 'NONE',  ( -19.02544592524334988, -5.153800228976617603, 103.9594237280190043 ) ) ;
#3278=CARTESIAN_POINT ( 'NONE',  ( 5.049401038298161559, -19.05341960407611168, 77.70724293864765286 ) ) ;
#3279=CARTESIAN_POINT ( 'NONE',  ( -9.474510206698720793, -16.51473224551083518, 104.5844237280190043 ) ) ;
#3281=CARTESIAN_POINT ( 'NONE',  ( -19.03943276465977164, -0.05219959533935918106, 113.7510903946856757 ) ) ;
#3282=CARTESIAN_POINT ( 'NONE',  ( -12.14591786802309592, -12.06949235617757132, 61.87390960531436690 ) ) ;
#3283=CARTESIAN_POINT ( 'NONE',  ( -0.05219959533934338120, 16.53943276465976808, 67.50109039468568994 ) ) ;
#3284=CARTESIAN_POINT ( 'NONE',  ( 5.823673210054444382, -21.52544592524334988, 20.20942372801900788 ) ) ;
#3285=CARTESIAN_POINT ( 'NONE',  ( -19.05341960407611168, -5.049401038298163336, 46.45724293864768129 ) ) ;
#3286=CARTESIAN_POINT ( 'NONE',  ( -0.05219959533909027116, -19.03943276465977164, 67.49890960531436690 ) ) ;
#3287=CARTESIAN_POINT ( 'NONE',  ( -4.379528057220086978, -16.55341960407618274, 74.79275706135234714 ) ) ;
#3290=CARTESIAN_POINT ( 'NONE',  ( -19.05341960407617563, 5.049401038297882671, 23.54275706135233648 ) ) ;
#3291=CARTESIAN_POINT ( 'NONE',  ( -16.46253265017160317, 9.564922557960807481, 40.83224293864769550 ) ) ;
#3293=CARTESIAN_POINT ( 'NONE',  ( 8.224510206698742110, 14.34966873604972548, 22.08442372801901143 ) ) ;
#3294=CARTESIAN_POINT ( 'NONE',  ( 0.05219959533936267826, -19.03943276465977164, 40.00109039468566152 ) ) ;
#3295=CARTESIAN_POINT ( 'NONE',  ( -14.29746914071037622, -8.314922557961029526, 29.16775706135234003 ) ) ;
#3296=CARTESIAN_POINT ( 'NONE',  ( 19.02544592524343514, -5.153800228976328945, 38.54057627198103120 ) ) ;
#3297=CARTESIAN_POINT ( 'NONE',  ( 19.05341960407611168, 5.049401038298154454, 68.95724293864769550 ) ) ;
#3298=CARTESIAN_POINT ( 'NONE',  ( -18.67979575497178146, -10.72451020669898902, 86.66557627198102409 ) ) ;
#3299=CARTESIAN_POINT ( 'NONE',  ( 16.51473224551069308, 9.474510206698969483, 114.1655762719810241 ) ) ;
#3300=CARTESIAN_POINT ( 'NONE',  ( -9.474510206698964154, 16.51473224551069663, 55.41557627198103120 ) ) ;
#3302=CARTESIAN_POINT ( 'NONE',  ( 16.51473224551083163, -9.474510206698727899, 95.83442372801900433 ) ) ;
#3303=CARTESIAN_POINT ( 'NONE',  ( -10.72451020669898014, 18.67979575497178502, 70.41557627198102409 ) ) ;
#3304=CARTESIAN_POINT ( 'NONE',  ( -16.51473224551082808, 9.474510206698731452, 23.33442372801900078 ) ) ;
#3305=CARTESIAN_POINT ( 'NONE',  ( 8.224510206698953496, -14.34966873604960469, 62.91557627198102409 ) ) ;
#3306=CARTESIAN_POINT ( 'NONE',  ( 15.72974639402176855, 15.80617190586768217, 91.87609039468568994 ) ) ;
#3307=CARTESIAN_POINT ( 'NONE',  ( 13.97604488694527802, 13.89961937509977652, 29.37390960531435979 ) ) ;
#3308=CARTESIAN_POINT ( 'NONE',  ( -18.62759615963255300, -10.81492255796106328, 94.16775706135237556 ) ) ;
#3309=CARTESIAN_POINT ( 'NONE',  ( 0.05219959533910956823, 16.53943276465976808, 24.99890960531435624 ) ) ;
#3310=CARTESIAN_POINT ( 'NONE',  ( -10.81492255796105439, 18.62759615963255655, 87.91775706135234714 ) ) ;
#3311=CARTESIAN_POINT ( 'NONE',  ( 19.03943276465977164, -0.05219959533909143690, 73.74890960531435269 ) ) ;
#3312=CARTESIAN_POINT ( 'NONE',  ( -18.62759615963255300, -10.81492255796106328, 39.16775706135235424 ) ) ;
#3313=CARTESIAN_POINT ( 'NONE',  ( -16.46253265017160317, 9.564922557960807481, 75.83224293864769550 ) ) ;
#3314=CARTESIAN_POINT ( 'NONE',  ( -16.55341960407611168, -4.379528057220339221, 96.45724293864770971 ) ) ;
#3315=CARTESIAN_POINT ( 'NONE',  ( 8.314922557960818139, 14.29746914071049879, 64.58224293864769550 ) ) ;
#3316=CARTESIAN_POINT ( 'NONE',  ( 15.72974639402199770, -15.80617190586745480, 73.12390960531436690 ) ) ;
#3317=CARTESIAN_POINT ( 'NONE',  ( -9.474510206698964154, 16.51473224551069663, 75.41557627198103830 ) ) ;
#3318=CARTESIAN_POINT ( 'NONE',  ( -10.72451020669898014, 18.67979575497178502, 90.41557627198103830 ) ) ;
#3319=CARTESIAN_POINT ( 'NONE',  ( -9.564922557961040184, 16.46253265017147172, 82.91775706135233293 ) ) ;
#3320=CARTESIAN_POINT ( 'NONE',  ( 16.51473224551083163, -9.474510206698727899, 30.83442372801900433 ) ) ;
#3321=CARTESIAN_POINT ( 'NONE',  ( -8.314922557960811034, -14.29746914071050412, 82.08224293864768129 ) ) ;
#3322=CARTESIAN_POINT ( 'NONE',  ( -21.55341960407610458, -5.719274019375992779, 51.45724293864770260 ) ) ;
#3324=CARTESIAN_POINT ( 'NONE',  ( -12.14591786802326823, 12.06949235617739902, 103.1260903946856757 ) ) ;
#3326=CARTESIAN_POINT ( 'NONE',  ( -0.05219959533936034679, 19.03943276465977164, 107.5010903946856615 ) ) ;
#3327=CARTESIAN_POINT ( 'NONE',  ( 8.224510206698953496, -14.34966873604960469, 67.91557627198102409 ) ) ;
#3329=CARTESIAN_POINT ( 'NONE',  ( -16.46253265017160317, 9.564922557960807481, 60.83224293864769550 ) ) ;
#3330=CARTESIAN_POINT ( 'NONE',  ( -12.14591786802309592, -12.06949235617757132, 56.87390960531436690 ) ) ;
#3331=CARTESIAN_POINT ( 'NONE',  ( 19.02544592524343514, -5.153800228976328945, 103.5405762719809957 ) ) ;
#3332=CARTESIAN_POINT ( 'NONE',  ( 9.564922557961047289, -16.46253265017146816, 90.41775706135234714 ) ) ;
#3333=CARTESIAN_POINT ( 'NONE',  ( -0.05219959533909027116, -19.03943276465977164, 62.49890960531435979 ) ) ;
#3334=CARTESIAN_POINT ( 'NONE',  ( -19.02544592524342804, 5.153800228976336051, 86.04057627198103830 ) ) ;
#3335=CARTESIAN_POINT ( 'NONE',  ( 13.89961937509977652, -13.97604488694527269, 83.12390960531436690 ) ) ;
#3336=CARTESIAN_POINT ( 'NONE',  ( 18.67979575497178502, 10.72451020669898547, 59.16557627198103120 ) ) ;
#3337=CARTESIAN_POINT ( 'NONE',  ( -14.34966873604972548, 8.224510206698743886, 58.33442372801901143 ) ) ;
#3338=CARTESIAN_POINT ( 'NONE',  ( -13.89961937509957401, -13.97604488694547697, 104.3760903946856757 ) ) ;
#3339=CARTESIAN_POINT ( 'NONE',  ( -19.03943276465977164, 0.05219959533909376836, 61.24890960531436690 ) ) ;
#3340=CARTESIAN_POINT ( 'NONE',  ( -18.62759615963270932, 10.81492255796079327, 65.83224293864769550 ) ) ;
#3341=CARTESIAN_POINT ( 'NONE',  ( 16.51473224551083163, -9.474510206698727899, 95.83442372801900433 ) ) ;
#3342=CARTESIAN_POINT ( 'NONE',  ( -14.34966873604960291, -8.224510206698953496, 26.66557627198103475 ) ) ;
#3343=CARTESIAN_POINT ( 'NONE',  ( 0.05219959533937995610, -21.53943276465977519, 50.00109039468568994 ) ) ;
#3345=CARTESIAN_POINT ( 'NONE',  ( -16.55341960407617563, 4.379528057220093196, 68.54275706135234714 ) ) ;
#3346=CARTESIAN_POINT ( 'NONE',  ( -8.314922557961024197, 14.29746914071037800, 97.91775706135236135 ) ) ;
#3347=CARTESIAN_POINT ( 'NONE',  ( 19.52837319214027900, -5.499999999999891642, 42.10471352585535953 ) ) ;
#3348=CARTESIAN_POINT ( 'NONE',  ( -16.52544592524335698, -4.483927247898792601, 78.95942372801901854 ) ) ;
#3349=CARTESIAN_POINT ( 'NONE',  ( -4.379528057220086978, -16.55341960407618274, 29.79275706135234358 ) ) ;
#3350=CARTESIAN_POINT ( 'NONE',  ( -13.89961937509977652, 13.97604488694528158, 45.62390960531433848 ) ) ;
#3351=CARTESIAN_POINT ( 'NONE',  ( 5.153800228976335163, 19.02544592524342804, 54.79057627198103120 ) ) ;
#3352=CARTESIAN_POINT ( 'NONE',  ( -19.03943276465977164, 0.05219959533909376836, 61.24890960531436690 ) ) ;
#3353=CARTESIAN_POINT ( 'NONE',  ( 18.62759615963255655, 10.81492255796105972, 51.66775706135234714 ) ) ;
#3354=CARTESIAN_POINT ( 'NONE',  ( 16.55341960407618274, -4.379528057220086978, 46.04275706135234714 ) ) ;
#3355=CARTESIAN_POINT ( 'NONE',  ( 16.55341960407611168, 4.379528057220329451, 38.95724293864768839 ) ) ;
#3356=CARTESIAN_POINT ( 'NONE',  ( 19.03943276465977164, -0.05219959533909143690, 33.74890960531435979 ) ) ;
#3357=CARTESIAN_POINT ( 'NONE',  ( 0.05219959533909260263, 19.03943276465977164, 39.99890960531436690 ) ) ;
#3358=CARTESIAN_POINT ( 'NONE',  ( 16.52544592524335698, 4.483927247898782831, 31.45942372801901854 ) ) ;
#3359=CARTESIAN_POINT ( 'NONE',  ( 5.049401038297881783, 19.05341960407617563, 82.29275706135229029 ) ) ;
#3360=CARTESIAN_POINT ( 'NONE',  ( 12.06949235617757843, -12.14591786802309237, 88.12390960531436690 ) ) ;
#3361=CARTESIAN_POINT ( 'NONE',  ( -0.05219959533909027116, -19.03943276465977164, 57.49890960531435979 ) ) ;
#3362=CARTESIAN_POINT ( 'NONE',  ( -9.474510206698720793, -16.51473224551083518, 79.58442372801899012 ) ) ;
#3363=CARTESIAN_POINT ( 'NONE',  ( 17.44279575226822132, 5.990770900252482711, 76.66442432485679603 ) ) ;
#3364=CARTESIAN_POINT ( 'NONE',  ( -21.53943276465977519, -0.05219959533937600094, 78.75109039468568994 ) ) ;
#3365=CARTESIAN_POINT ( 'NONE',  ( -16.55341960407617563, 4.379528057220093196, 53.54275706135234714 ) ) ;
#3366=CARTESIAN_POINT ( 'NONE',  ( 17.31728774477273092, 6.344390552232407998, 36.68093348310681279 ) ) ;
#3367=CARTESIAN_POINT ( 'NONE',  ( -15.80617190586745835, -15.72974639402198527, 36.87390960531435979 ) ) ;
#3368=CARTESIAN_POINT ( 'NONE',  ( 8.224510206698742110, 14.34966873604972548, 32.08442372801901854 ) ) ;
#3370=CARTESIAN_POINT ( 'NONE',  ( 19.03943276465977164, 0.05219959533936151252, 26.25109039468566507 ) ) ;
#3372=CARTESIAN_POINT ( 'NONE',  ( -13.97604488694527625, -13.89961937509977652, 41.87390960531435979 ) ) ;
#3374=CARTESIAN_POINT ( 'NONE',  ( 19.05341960407611168, 5.049401038298154454, 68.95724293864769550 ) ) ;
#3375=CARTESIAN_POINT ( 'NONE',  ( -19.49190055781010145, -5.500000000000053291, 55.56116087098782685 ) ) ;
#3376=CARTESIAN_POINT ( 'NONE',  ( 15.80617190586769283, -15.72974639402175789, 110.6260903946857042 ) ) ;
#3377=CARTESIAN_POINT ( 'NONE',  ( 8.314922557960818139, 14.29746914071049879, 34.58224293864770260 ) ) ;
#3378=CARTESIAN_POINT ( 'NONE',  ( 19.05341960407611168, 5.049401038298154454, 38.95724293864767418 ) ) ;
#3379=CARTESIAN_POINT ( 'NONE',  ( -19.05341960407611168, -5.049401038298163336, 111.4572429386476671 ) ) ;
#3380=CARTESIAN_POINT ( 'NONE',  ( 18.67979575497194134, -10.72451020669871369, 75.83442372801900433 ) ) ;
#3381=CARTESIAN_POINT ( 'NONE',  ( -13.89961937509977652, 13.97604488694528158, 55.62390960531434558 ) ) ;
#3382=CARTESIAN_POINT ( 'NONE',  ( 21.53943276465977519, 0.05219959533937863772, 71.25109039468568994 ) ) ;
#3383=CARTESIAN_POINT ( 'NONE',  ( 5.049401038298161559, -19.05341960407611168, 112.7072429386476813 ) ) ;
#3384=CARTESIAN_POINT ( 'NONE',  ( 19.03943276465977164, -0.05219959533909143690, 38.74890960531436690 ) ) ;
#3385=CARTESIAN_POINT ( 'NONE',  ( -21.55341960407619339, 5.719274019375674811, 23.54275706135235424 ) ) ;
#3386=CARTESIAN_POINT ( 'NONE',  ( 5.049401038297881783, 19.05341960407617563, 42.29275706135234003 ) ) ;
#3387=CARTESIAN_POINT ( 'NONE',  ( -12.14591786802309592, -12.06949235617757132, 106.8739096053143811 ) ) ;
#3388=CARTESIAN_POINT ( 'NONE',  ( -9.474510206698964154, 16.51473224551069663, 65.41557627198102409 ) ) ;
#3389=CARTESIAN_POINT ( 'NONE',  ( 14.29746914071037800, 8.314922557961029526, 21.66775706135235069 ) ) ;
#3390=CARTESIAN_POINT ( 'NONE',  ( -8.224510206698948167, 14.34966873604960824, 75.41557627198102409 ) ) ;
#3391=CARTESIAN_POINT ( 'NONE',  ( 18.62759615963271287, -10.81492255796078972, 28.33224293864769550 ) ) ;
#3392=CARTESIAN_POINT ( 'NONE',  ( -9.564922557961040184, 16.46253265017147172, 107.9177570613523471 ) ) ;
#3393=CARTESIAN_POINT ( 'NONE',  ( -15.72974639402197994, 15.80617190586746368, 110.6239096053143669 ) ) ;
#3394=CARTESIAN_POINT ( 'NONE',  ( -10.81492255796105439, 18.62759615963255655, 52.91775706135235424 ) ) ;
#3395=CARTESIAN_POINT ( 'NONE',  ( 16.53943276465976808, 0.05219959533934440121, 61.25109039468567573 ) ) ;
#3396=CARTESIAN_POINT ( 'NONE',  ( 14.29746914071037800, 8.314922557961029526, 56.66775706135235424 ) ) ;
#3397=CARTESIAN_POINT ( 'NONE',  ( -5.823673210054116645, -21.52544592524344225, 52.29057627198102409 ) ) ;
#3398=CARTESIAN_POINT ( 'NONE',  ( -5.049401038298153566, 19.05341960407611168, 50.20724293864770260 ) ) ;
#3399=CARTESIAN_POINT ( 'NONE',  ( 16.55341960407618274, -4.379528057220086978, 81.04275706135236135 ) ) ;
#3400=CARTESIAN_POINT ( 'NONE',  ( -21.52544592524343514, 5.823673210054127303, 96.04057627198102409 ) ) ;
#3401=CARTESIAN_POINT ( 'NONE',  ( 16.55341960407611168, 4.379528057220329451, 48.95724293864770971 ) ) ;
#3402=CARTESIAN_POINT ( 'NONE',  ( -19.02544592524342804, 5.153800228976336051, 71.04057627198099567 ) ) ;
#3403=CARTESIAN_POINT ( 'NONE',  ( -4.483927247898782831, 16.52544592524335698, 77.70942372801900433 ) ) ;
#3404=CARTESIAN_POINT ( 'NONE',  ( -19.03943276465977164, -0.05219959533935918106, 113.7510903946856757 ) ) ;
#3405=CARTESIAN_POINT ( 'NONE',  ( -15.72974639402197994, 15.80617190586746368, 100.6239096053143811 ) ) ;
#3406=CARTESIAN_POINT ( 'NONE',  ( 8.224510206698953496, -14.34966873604960469, 47.91557627198102409 ) ) ;
#3408=CARTESIAN_POINT ( 'NONE',  ( -16.62475595723698518, 7.163666690055228159, 75.52713351810470499 ) ) ;
#3409=CARTESIAN_POINT ( 'NONE',  ( -15.72974639402197994, 15.80617190586746368, 85.62390960531436690 ) ) ;
#3410=CARTESIAN_POINT ( 'NONE',  ( 12.06949235617757843, -12.14591786802309237, 23.12390960531436335 ) ) ;
#3413=CARTESIAN_POINT ( 'NONE',  ( -15.80617190586745835, -15.72974639402198527, 101.8739096053143811 ) ) ;
#3414=CARTESIAN_POINT ( 'NONE',  ( 19.02544592524343514, -5.153800228976328945, 98.54057627198100988 ) ) ;
#3415=CARTESIAN_POINT ( 'NONE',  ( -5.823673210054431948, 21.52544592524334988, 22.70942372801901499 ) ) ;
#3416=CARTESIAN_POINT ( 'NONE',  ( 12.06949235617757843, -12.14591786802309237, 33.12390960531435979 ) ) ;
#3417=CARTESIAN_POINT ( 'NONE',  ( -12.06949235617739369, -12.14591786802326823, 44.37609039468567573 ) ) ;
#3418=CARTESIAN_POINT ( 'NONE',  ( 5.153800228976335163, 19.02544592524342804, 44.79057627198103830 ) ) ;
#3419=CARTESIAN_POINT ( 'NONE',  ( 16.46253265017146816, 9.564922557961045513, 46.66775706135233293 ) ) ;
#3420=CARTESIAN_POINT ( 'NONE',  ( 9.564922557960805705, 16.46253265017160317, 79.58224293864769550 ) ) ;
#3421=CARTESIAN_POINT ( 'NONE',  ( 10.81492255796078972, 18.62759615963270932, 34.58224293864770260 ) ) ;
#3423=CARTESIAN_POINT ( 'NONE',  ( -4.483927247898782831, 16.52544592524335698, 22.70942372801901499 ) ) ;
#3424=CARTESIAN_POINT ( 'NONE',  ( 0.05219959533936267826, -19.03943276465977164, 50.00109039468566863 ) ) ;
#3425=CARTESIAN_POINT ( 'NONE',  ( 18.62759615963271287, -10.81492255796078972, 103.3322429386476955 ) ) ;
#3426=CARTESIAN_POINT ( 'NONE',  ( -8.224510206698948167, 14.34966873604960824, 35.41557627198102409 ) ) ;
#3427=CARTESIAN_POINT ( 'NONE',  ( -16.46253265017160317, 9.564922557960807481, 80.83224293864769550 ) ) ;
#3428=CARTESIAN_POINT ( 'NONE',  ( -21.52544592524343514, 5.823673210054127303, 66.04057627198103830 ) ) ;
#3429=CARTESIAN_POINT ( 'NONE',  ( -18.67979575497178146, -10.72451020669898902, 101.6655762719810383 ) ) ;
#3430=CARTESIAN_POINT ( 'NONE',  ( -16.53943276465976808, -0.05219959533934237506, 28.75109039468567929 ) ) ;
#3431=CARTESIAN_POINT ( 'NONE',  ( 18.67979575497178502, 10.72451020669898547, 29.16557627198103120 ) ) ;
#3432=CARTESIAN_POINT ( 'NONE',  ( -0.05219959533937732626, 21.53943276465977519, 87.50109039468568994 ) ) ;
#3433=CARTESIAN_POINT ( 'NONE',  ( 5.049401038298161559, -19.05341960407611168, 82.70724293864770971 ) ) ;
#3434=CARTESIAN_POINT ( 'NONE',  ( 19.05341960407611168, 5.049401038298154454, 23.95724293864769194 ) ) ;
#3435=CARTESIAN_POINT ( 'NONE',  ( 19.02544592524343514, -5.153800228976328945, 88.54057627198102409 ) ) ;
#3436=CARTESIAN_POINT ( 'NONE',  ( 14.29746914071049879, -8.314922557960816363, 108.3322429386477097 ) ) ;
#3437=CARTESIAN_POINT ( 'NONE',  ( -16.51473224551069308, -9.474510206698971260, 66.66557627198102409 ) ) ;
#3438=CARTESIAN_POINT ( 'NONE',  ( 14.29746914071037800, 8.314922557961029526, 26.66775706135235424 ) ) ;
#3439=CARTESIAN_POINT ( 'NONE',  ( 17.50000000000147082, 3.202012800152225669, 32.57177583972737978 ) ) ;
#3440=CARTESIAN_POINT ( 'NONE',  ( 5.049401038298161559, -19.05341960407611168, 72.70724293864768129 ) ) ;
#3441=CARTESIAN_POINT ( 'NONE',  ( -15.80617190586768217, 15.72974639402176855, 103.1260903946856757 ) ) ;
#3442=CARTESIAN_POINT ( 'NONE',  ( 5.719274019375991003, -21.55341960407610458, 22.70724293864769194 ) ) ;
#3443=CARTESIAN_POINT ( 'NONE',  ( -8.224510206698735004, -14.34966873604973081, 89.58442372801901854 ) ) ;
#3445=CARTESIAN_POINT ( 'NONE',  ( 5.049401038297881783, 19.05341960407617563, 72.29275706135234714 ) ) ;
#3446=CARTESIAN_POINT ( 'NONE',  ( 18.67979575497194134, -10.72451020669871369, 110.8344237280190043 ) ) ;
#3447=CARTESIAN_POINT ( 'NONE',  ( -17.40861289039002813, -6.110651285853281323, 46.37232470827434838 ) ) ;
#3448=CARTESIAN_POINT ( 'NONE',  ( -5.049401038298153566, 19.05341960407611168, 25.20724293864768484 ) ) ;
#3449=CARTESIAN_POINT ( 'NONE',  ( -12.14591786802309592, -12.06949235617757132, 31.87390960531435979 ) ) ;
#3451=CARTESIAN_POINT ( 'NONE',  ( -12.14591786802326823, 12.06949235617739902, 103.1260903946856757 ) ) ;
#3452=CARTESIAN_POINT ( 'NONE',  ( -18.87255363501902750, -5.500000000000067502, 86.32513748171830059 ) ) ;
#3453=CARTESIAN_POINT ( 'NONE',  ( 8.314922557961029526, -14.29746914071037800, 80.41775706135234714 ) ) ;
#3454=CARTESIAN_POINT ( 'NONE',  ( -9.564922557960796823, -16.46253265017161027, 37.08224293864768839 ) ) ;
#3455=CARTESIAN_POINT ( 'NONE',  ( 21.53943276465977519, 0.05219959533937863772, 96.25109039468568994 ) ) ;
#3456=CARTESIAN_POINT ( 'NONE',  ( 13.97604488694548053, -13.89961937509957401, 95.62609039468563310 ) ) ;
#3457=CARTESIAN_POINT ( 'NONE',  ( -18.67979575497193778, 10.72451020669871902, 78.33442372801901854 ) ) ;
#3458=CARTESIAN_POINT ( 'NONE',  ( -16.51473224551082808, 9.474510206698731452, 48.33442372801900433 ) ) ;
#3459=CARTESIAN_POINT ( 'NONE',  ( -5.153800228976328057, -19.02544592524343514, 77.29057627198099567 ) ) ;
#3460=CARTESIAN_POINT ( 'NONE',  ( 5.153800228976335163, 19.02544592524342804, 69.79057627198103830 ) ) ;
#3461=CARTESIAN_POINT ( 'NONE',  ( 17.50000000000000000, 5.499999999999997335, 120.0000000000000142 ) ) ;
#3462=CARTESIAN_POINT ( 'NONE',  ( 8.224510206698953496, -14.34966873604960469, 67.91557627198102409 ) ) ;
#3463=CARTESIAN_POINT ( 'NONE',  ( 18.62759615963271287, -10.81492255796078972, 53.33224293864769550 ) ) ;
#3464=CARTESIAN_POINT ( 'NONE',  ( 5.049401038298161559, -19.05341960407611168, 47.70724293864770260 ) ) ;
#3465=CARTESIAN_POINT ( 'NONE',  ( 15.80617190586746368, 15.72974639402197994, 84.37390960531438111 ) ) ;
#3466=CARTESIAN_POINT ( 'NONE',  ( 16.52544592524335698, 4.483927247898782831, 81.45942372801900433 ) ) ;
#3468=CARTESIAN_POINT ( 'NONE',  ( 8.224510206698953496, -14.34966873604960469, 77.91557627198102409 ) ) ;
#3470=CARTESIAN_POINT ( 'NONE',  ( -8.224510206698735004, -14.34966873604973081, 44.58442372801901854 ) ) ;
#3471=CARTESIAN_POINT ( 'NONE',  ( -14.29746914071049879, 8.314922557960819915, 110.8322429386476955 ) ) ;
#3472=CARTESIAN_POINT ( 'NONE',  ( -0.05219959533936034679, 19.03943276465977164, 72.50109039468566152 ) ) ;
#3473=CARTESIAN_POINT ( 'NONE',  ( -12.06949235617756955, 12.14591786802309770, 65.62390960531436690 ) ) ;
#3474=CARTESIAN_POINT ( 'NONE',  ( -5.719274019375665041, -21.55341960407619695, 44.79275706135234714 ) ) ;
#3475=DIRECTION ( 'NONE',  ( 0.000000000000000000, -1.000000000000000000, 0.000000000000000000 ) ) ;
#3476=CARTESIAN_POINT ( 'NONE',  ( -21.52544592524343514, 5.823673210054127303, 96.04057627198102409 ) ) ;
#3477=CARTESIAN_POINT ( 'NONE',  ( 17.50000000000000000, 5.499999999999992895, 91.70309617465828467 ) ) ;
#3478=CARTESIAN_POINT ( 'NONE',  ( -14.34966873604960291, -8.224510206698953496, 81.66557627198103830 ) ) ;
#3480=CARTESIAN_POINT ( 'NONE',  ( 9.564922557960805705, 16.46253265017160317, 39.58224293864768839 ) ) ;
#3482=CARTESIAN_POINT ( 'NONE',  ( -19.02544592524334988, -5.153800228976617603, 78.95942372801900433 ) ) ;
#3483=CARTESIAN_POINT ( 'NONE',  ( -21.53943276465977519, -0.05219959533937600094, 33.75109039468568284 ) ) ;
#3484=CARTESIAN_POINT ( 'NONE',  ( 19.03943276465977164, -0.05219959533909143690, 68.74890960531436690 ) ) ;
#3485=CARTESIAN_POINT ( 'NONE',  ( 0.05219959533936267826, -19.03943276465977164, 55.00109039468566863 ) ) ;
#3486=CARTESIAN_POINT ( 'NONE',  ( -13.89961937509977652, 13.97604488694528158, 50.62390960531435979 ) ) ;
#3487=CARTESIAN_POINT ( 'NONE',  ( 16.52544592524342804, -4.483927247898539470, 58.54057627198103120 ) ) ;
#3488=CARTESIAN_POINT ( 'NONE',  ( -4.483927247898539470, -16.52544592524342804, 57.29057627198103120 ) ) ;
#3489=CARTESIAN_POINT ( 'NONE',  ( 5.153800228976335163, 19.02544592524342804, 69.79057627198103830 ) ) ;
#3490=CARTESIAN_POINT ( 'NONE',  ( -21.55341960407610458, -5.719274019375992779, 101.4572429386476955 ) ) ;
#3491=CARTESIAN_POINT ( 'NONE',  ( -13.97604488694527625, -13.89961937509977652, 66.87390960531436690 ) ) ;
#3492=CARTESIAN_POINT ( 'NONE',  ( -15.72974639402197994, 15.80617190586746368, 80.62390960531438111 ) ) ;
#3493=EDGE_CURVE ( 'NONE', #90870, #121091, #171835, .T. ) ;
#3494=CARTESIAN_POINT ( 'NONE',  ( -18.67979575497193778, 10.72451020669871902, 113.3344237280190328 ) ) ;
#3495=CARTESIAN_POINT ( 'NONE',  ( -0.05219959533909027116, -19.03943276465977164, 32.49890960531435979 ) ) ;
#3496=CARTESIAN_POINT ( 'NONE',  ( -12.06949235617739369, -12.14591786802326823, 104.3760903946856899 ) ) ;
#3497=CARTESIAN_POINT ( 'NONE',  ( -4.379528057220328563, 16.55341960407611168, 100.2072429386476955 ) ) ;
#3498=CARTESIAN_POINT ( 'NONE',  ( 13.97604488694548053, -13.89961937509957401, 110.6260903946856615 ) ) ;
#3500=CARTESIAN_POINT ( 'NONE',  ( 0.05219959533937995610, -21.53943276465977519, 30.00109039468568284 ) ) ;
#3501=CARTESIAN_POINT ( 'NONE',  ( -5.049401038297874678, -19.05341960407617918, 59.79275706135231871 ) ) ;
#3502=CARTESIAN_POINT ( 'NONE',  ( -12.14591786802309592, -12.06949235617757132, 26.87390960531435979 ) ) ;
#3503=CARTESIAN_POINT ( 'NONE',  ( -21.52544592524343514, 5.823673210054127303, 76.04057627198102409 ) ) ;
#3504=CARTESIAN_POINT ( 'NONE',  ( -13.97604488694527625, -13.89961937509977652, 101.8739096053143811 ) ) ;
#3505=CARTESIAN_POINT ( 'NONE',  ( -16.52544592524342804, 4.483927247898546575, 61.04057627198103120 ) ) ;
#3506=CARTESIAN_POINT ( 'NONE',  ( -5.153800228976328057, -19.02544592524343514, 27.29057627198103120 ) ) ;
#3507=CARTESIAN_POINT ( 'NONE',  ( -9.474510206698964154, 16.51473224551069663, 40.41557627198103120 ) ) ;
#3508=CARTESIAN_POINT ( 'NONE',  ( 5.153800228976615827, -19.02544592524334988, 30.20942372801900433 ) ) ;
#3509=CARTESIAN_POINT ( 'NONE',  ( -0.05219959533934338120, 16.53943276465976808, 92.50109039468567573 ) ) ;
#3510=CARTESIAN_POINT ( 'NONE',  ( 10.81492255796106328, -18.62759615963255655, 40.41775706135234714 ) ) ;
#3511=CARTESIAN_POINT ( 'NONE',  ( -8.314922557961024197, 14.29746914071037800, 47.91775706135234714 ) ) ;
#3512=CARTESIAN_POINT ( 'NONE',  ( 21.55341960407610458, 5.719274019375980345, 28.95724293864769905 ) ) ;
#3513=CARTESIAN_POINT ( 'NONE',  ( 5.049401038298161559, -19.05341960407611168, 47.70724293864770260 ) ) ;
#3514=CARTESIAN_POINT ( 'NONE',  ( -0.05219959533937732626, 21.53943276465977519, 92.50109039468567573 ) ) ;
#3515=CARTESIAN_POINT ( 'NONE',  ( -5.049401038298153566, 19.05341960407611168, 75.20724293864769550 ) ) ;
#3516=CARTESIAN_POINT ( 'NONE',  ( -14.34966873604972548, 8.224510206698743886, 58.33442372801901143 ) ) ;
#3517=CARTESIAN_POINT ( 'NONE',  ( -16.52544592524342804, 4.483927247898546575, 101.0405762719810383 ) ) ;
#3518=CARTESIAN_POINT ( 'NONE',  ( -4.379528057220086978, -16.55341960407618274, 109.7927570613523613 ) ) ;
#3520=CARTESIAN_POINT ( 'NONE',  ( 10.72451020669871369, 18.67979575497193778, 62.08442372801901143 ) ) ;
#3521=CARTESIAN_POINT ( 'NONE',  ( 9.474510206698971260, -16.51473224551069308, 97.91557627198102409 ) ) ;
#3522=CARTESIAN_POINT ( 'NONE',  ( -19.03943276465977164, 0.05219959533909376836, 81.24890960531436690 ) ) ;
#3523=CARTESIAN_POINT ( 'NONE',  ( 16.46253265017160672, -9.564922557960803928, 113.3322429386476955 ) ) ;
#3524=CARTESIAN_POINT ( 'NONE',  ( 0.05219959533910956823, 16.53943276465976808, 44.99890960531435979 ) ) ;
#3525=CARTESIAN_POINT ( 'NONE',  ( 8.314922557960818139, 14.29746914071049879, 24.58224293864768839 ) ) ;
#3526=CARTESIAN_POINT ( 'NONE',  ( 4.379528057220339221, -16.55341960407611168, 37.70724293864769550 ) ) ;
#3528=CARTESIAN_POINT ( 'NONE',  ( -5.153800228976607833, 19.02544592524334988, 32.70942372801899722 ) ) ;
#3529=CARTESIAN_POINT ( 'NONE',  ( 5.153800228976335163, 19.02544592524342804, 79.79057627198102409 ) ) ;
#3530=CARTESIAN_POINT ( 'NONE',  ( -0.05219959533936034679, 19.03943276465977164, 57.50109039468566863 ) ) ;
#3532=CARTESIAN_POINT ( 'NONE',  ( -0.05219959533936034679, 19.03943276465977164, 82.50109039468567573 ) ) ;
#3533=CARTESIAN_POINT ( 'NONE',  ( -12.14591786802326823, 12.06949235617739902, 73.12609039468567573 ) ) ;
#3535=CARTESIAN_POINT ( 'NONE',  ( 0.05219959533909260263, 19.03943276465977164, 109.9989096053143669 ) ) ;
#3536=CARTESIAN_POINT ( 'NONE',  ( 18.62759615963255655, 10.81492255796105972, 26.66775706135235424 ) ) ;
#3537=CARTESIAN_POINT ( 'NONE',  ( 19.05341960407617918, -5.049401038297876454, 96.04275706135231871 ) ) ;
#3538=CARTESIAN_POINT ( 'NONE',  ( 19.05341960407611168, 5.049401038298154454, 53.95724293864770260 ) ) ;
#3539=CARTESIAN_POINT ( 'NONE',  ( -16.46253265017160317, 9.564922557960807481, 95.83224293864769550 ) ) ;
#3540=CARTESIAN_POINT ( 'NONE',  ( -12.14591786802309592, -12.06949235617757132, 56.87390960531436690 ) ) ;
#3541=CARTESIAN_POINT ( 'NONE',  ( 5.049401038298161559, -19.05341960407611168, 52.70724293864767418 ) ) ;
#3542=CARTESIAN_POINT ( 'NONE',  ( 5.153800228976335163, 19.02544592524342804, 59.79057627198100988 ) ) ;
#3543=CARTESIAN_POINT ( 'NONE',  ( 9.474510206698729675, 16.51473224551082808, 67.08442372801900433 ) ) ;
#3544=CARTESIAN_POINT ( 'NONE',  ( -19.03943276465977164, -0.05219959533935918106, 28.75109039468566507 ) ) ;
#3545=CARTESIAN_POINT ( 'NONE',  ( -13.89961937509977652, 13.97604488694528158, 60.62390960531436690 ) ) ;
#3546=CARTESIAN_POINT ( 'NONE',  ( -0.05219959533907301413, -21.53943276465977519, 67.49890960531436690 ) ) ;
#3547=CARTESIAN_POINT ( 'NONE',  ( -14.34966873604960291, -8.224510206698953496, 71.66557627198100988 ) ) ;
#3548=CARTESIAN_POINT ( 'NONE',  ( 9.564922557961047289, -16.46253265017146816, 30.41775706135232937 ) ) ;
#3549=CARTESIAN_POINT ( 'NONE',  ( 30.00000000000000000, -5.204748896376250896E-15, 47.50000000000000000 ) ) ;
#3550=CARTESIAN_POINT ( 'NONE',  ( 15.72974639402199770, -15.80617190586745480, 48.12390960531436690 ) ) ;
#3551=CARTESIAN_POINT ( 'NONE',  ( 18.62759615963271287, -10.81492255796078972, 23.33224293864769194 ) ) ;
#3552=CARTESIAN_POINT ( 'NONE',  ( 13.97604488694527802, 13.89961937509977652, 54.37390960531435979 ) ) ;
#3553=CARTESIAN_POINT ( 'NONE',  ( -19.03943276465977164, 0.05219959533909376836, 41.24890960531435269 ) ) ;
#3554=CARTESIAN_POINT ( 'NONE',  ( -16.55341960407611168, -4.379528057220339221, 106.4572429386477097 ) ) ;
#3555=CARTESIAN_POINT ( 'NONE',  ( 10.72451020669898902, -18.67979575497178502, 112.9155762719810383 ) ) ;
#3556=CARTESIAN_POINT ( 'NONE',  ( 13.89961937509977652, -13.97604488694527269, 108.1239096053143669 ) ) ;
#3557=CARTESIAN_POINT ( 'NONE',  ( -21.55341960407619339, 5.719274019375674811, 33.54275706135234714 ) ) ;
#3558=CARTESIAN_POINT ( 'NONE',  ( 12.06949235617757843, -12.14591786802309237, 113.1239096053143953 ) ) ;
#3559=CARTESIAN_POINT ( 'NONE',  ( -10.72451020669870658, -18.67979575497194134, 84.58442372801903275 ) ) ;
#3560=CARTESIAN_POINT ( 'NONE',  ( 10.72451020669898902, -18.67979575497178502, 87.91557627198103830 ) ) ;
#3561=CARTESIAN_POINT ( 'NONE',  ( -16.46253265017146816, -9.564922557961047289, 39.16775706135234003 ) ) ;
#3563=CARTESIAN_POINT ( 'NONE',  ( 9.564922557960805705, 16.46253265017160317, 24.58224293864769194 ) ) ;
#3565=CARTESIAN_POINT ( 'NONE',  ( 16.55341960407618274, -4.379528057220086978, 41.04275706135236135 ) ) ;
#3566=CARTESIAN_POINT ( 'NONE',  ( -9.474510206698964154, 16.51473224551069663, 30.41557627198102054 ) ) ;
#3568=CARTESIAN_POINT ( 'NONE',  ( -0.05219959533909027116, -19.03943276465977164, 67.49890960531436690 ) ) ;
#3569=CARTESIAN_POINT ( 'NONE',  ( 4.379528057220339221, -16.55341960407611168, 87.70724293864769550 ) ) ;
#3570=CARTESIAN_POINT ( 'NONE',  ( -10.72451020669898014, 18.67979575497178502, 50.41557627198103120 ) ) ;
#3571=CARTESIAN_POINT ( 'NONE',  ( 8.224510206698953496, -14.34966873604960469, 82.91557627198103830 ) ) ;
#3572=CARTESIAN_POINT ( 'NONE',  ( 0.05219959533934541429, -16.53943276465976808, 30.00109039468568284 ) ) ;
#3573=CARTESIAN_POINT ( 'NONE',  ( -21.52544592524334988, -5.823673210054445271, 83.95942372801900433 ) ) ;
#3574=CARTESIAN_POINT ( 'NONE',  ( 5.049401038298161559, -19.05341960407611168, 32.70724293864768129 ) ) ;
#3575=CARTESIAN_POINT ( 'NONE',  ( 16.52544592524335698, 4.483927247898782831, 101.4594237280190185 ) ) ;
#3576=CARTESIAN_POINT ( 'NONE',  ( -8.314922557960811034, -14.29746914071050412, 47.08224293864770260 ) ) ;
#3577=CARTESIAN_POINT ( 'NONE',  ( -0.05219959533909027116, -19.03943276465977164, 52.49890960531436690 ) ) ;
#3578=CARTESIAN_POINT ( 'NONE',  ( -5.823673210054431948, 21.52544592524334988, 97.70942372801904696 ) ) ;
#3579=CARTESIAN_POINT ( 'NONE',  ( -10.81492255796078084, -18.62759615963271287, 102.0822429386476955 ) ) ;
#3580=CARTESIAN_POINT ( 'NONE',  ( -18.62759615963255300, -10.81492255796106328, 54.16775706135235424 ) ) ;
#3581=CARTESIAN_POINT ( 'NONE',  ( 4.483927247898790824, -16.52544592524335698, 35.20942372801901854 ) ) ;
#3582=CARTESIAN_POINT ( 'NONE',  ( -14.29746914071049879, 8.314922557960819915, 60.83224293864769550 ) ) ;
#3583=CARTESIAN_POINT ( 'NONE',  ( -5.823673210054431948, 21.52544592524334988, 92.70942372801901854 ) ) ;
#3584=CARTESIAN_POINT ( 'NONE',  ( 12.06949235617757843, -12.14591786802309237, 23.12390960531436335 ) ) ;
#3585=CARTESIAN_POINT ( 'NONE',  ( 16.21995358207275117, -7.366697692864356384, 47.43551001512066989 ) ) ;
#3586=CARTESIAN_POINT ( 'NONE',  ( -19.25176906914649422, -5.499999999999740652, 65.99927264242279534 ) ) ;
#3587=CARTESIAN_POINT ( 'NONE',  ( 4.483927247898545687, 16.52544592524342804, 39.79057627198103830 ) ) ;
#3588=CARTESIAN_POINT ( 'NONE',  ( 8.224510206698742110, 14.34966873604972548, 67.08442372801901854 ) ) ;
#3589=CARTESIAN_POINT ( 'NONE',  ( -19.05341960407611168, -5.049401038298163336, 81.45724293864769550 ) ) ;
#3590=CARTESIAN_POINT ( 'NONE',  ( -19.03943276465977164, 0.05219959533909376836, 106.2489096053143669 ) ) ;
#3591=CARTESIAN_POINT ( 'NONE',  ( -18.62759615963255300, -10.81492255796106328, 84.16775706135234714 ) ) ;
#3592=CARTESIAN_POINT ( 'NONE',  ( -4.379528057220086978, -16.55341960407618274, 84.79275706135234714 ) ) ;
#3593=CARTESIAN_POINT ( 'NONE',  ( 16.52544592524342804, -4.483927247898539470, 73.54057627198102409 ) ) ;
#3594=CARTESIAN_POINT ( 'NONE',  ( 19.02544592524343514, -5.153800228976328945, 78.54057627198099567 ) ) ;
#3596=CARTESIAN_POINT ( 'NONE',  ( -8.224510206698735004, -14.34966873604973081, 29.58442372801901854 ) ) ;
#3597=CARTESIAN_POINT ( 'NONE',  ( 19.03943276465977164, -0.05219959533909143690, 23.74890960531435269 ) ) ;
#3598=CARTESIAN_POINT ( 'NONE',  ( 5.049401038298161559, -19.05341960407611168, 97.70724293864766707 ) ) ;
#3599=CARTESIAN_POINT ( 'NONE',  ( -8.314922557961024197, 14.29746914071037800, 27.91775706135234358 ) ) ;
#3601=CARTESIAN_POINT ( 'NONE',  ( 21.52544592524334988, 5.823673210054432836, 111.4594237280190328 ) ) ;
#3602=CARTESIAN_POINT ( 'NONE',  ( -12.06949235617739369, -12.14591786802326823, 89.37609039468568994 ) ) ;
#3603=CARTESIAN_POINT ( 'NONE',  ( 16.46253265017146816, 9.564922557961045513, 106.6677570613523471 ) ) ;
#3604=CARTESIAN_POINT ( 'NONE',  ( 0.05219959533909260263, 19.03943276465977164, 29.99890960531435979 ) ) ;
#3605=CARTESIAN_POINT ( 'NONE',  ( 14.34966873604972726, -8.224510206698740333, 80.83442372801901854 ) ) ;
#3606=CARTESIAN_POINT ( 'NONE',  ( 0.05219959533934541429, -16.53943276465976808, 70.00109039468568994 ) ) ;
#3608=CARTESIAN_POINT ( 'NONE',  ( 16.46253265017146816, 9.564922557961045513, 66.66775706135233293 ) ) ;
#3609=CARTESIAN_POINT ( 'NONE',  ( 16.46253265017146816, 9.564922557961045513, 21.66775706135233648 ) ) ;
#3610=CARTESIAN_POINT ( 'NONE',  ( -16.51473224551069308, -9.474510206698971260, 46.66557627198102409 ) ) ;
#3611=CARTESIAN_POINT ( 'NONE',  ( -16.46253265017160317, 9.564922557960807481, 95.83224293864769550 ) ) ;
#3612=CARTESIAN_POINT ( 'NONE',  ( -16.53943276465976808, 0.05219959533911058130, 91.24890960531436690 ) ) ;
#3613=CARTESIAN_POINT ( 'NONE',  ( 16.46253265017146816, 9.564922557961045513, 51.66775706135233293 ) ) ;
#3614=CARTESIAN_POINT ( 'NONE',  ( -18.67979575497178146, -10.72451020669898902, 46.66557627198102409 ) ) ;
#3615=CARTESIAN_POINT ( 'NONE',  ( -15.72974639402176322, -15.80617190586768395, 104.3760903946856899 ) ) ;
#3616=CARTESIAN_POINT ( 'NONE',  ( -9.564922557960796823, -16.46253265017161027, 87.08224293864769550 ) ) ;
#3617=CARTESIAN_POINT ( 'NONE',  ( -10.72451020669870658, -18.67979575497194134, 109.5844237280190328 ) ) ;
#3618=CARTESIAN_POINT ( 'NONE',  ( 21.53943276465977519, -0.05219959533907433946, 68.74890960531435269 ) ) ;
#3619=CARTESIAN_POINT ( 'NONE',  ( -0.05219959533909027116, -19.03943276465977164, 92.49890960531436690 ) ) ;
#3620=CARTESIAN_POINT ( 'NONE',  ( 0.05219959533936267826, -19.03943276465977164, 85.00109039468567573 ) ) ;
#3621=CARTESIAN_POINT ( 'NONE',  ( 13.89961937509977652, -13.97604488694527269, 108.1239096053143669 ) ) ;
#3622=CARTESIAN_POINT ( 'NONE',  ( -16.46253265017146816, -9.564922557961047289, 104.1677570613523329 ) ) ;
#3623=CARTESIAN_POINT ( 'NONE',  ( -12.14591786802309592, -12.06949235617757132, 111.8739096053143669 ) ) ;
#3624=CARTESIAN_POINT ( 'NONE',  ( 0.05219959533909260263, 19.03943276465977164, 79.99890960531436690 ) ) ;
#3625=CARTESIAN_POINT ( 'NONE',  ( -21.53943276465977519, 0.05219959533907696930, 76.24890960531435269 ) ) ;
#3626=CARTESIAN_POINT ( 'NONE',  ( -0.05219959533934338120, 16.53943276465976808, 42.50109039468567573 ) ) ;
#3627=CARTESIAN_POINT ( 'NONE',  ( -5.823673210054431948, 21.52544592524334988, 47.70942372801902565 ) ) ;
#3628=CARTESIAN_POINT ( 'NONE',  ( -10.81492255796105439, 18.62759615963255655, 102.9177570613523756 ) ) ;
#3629=CARTESIAN_POINT ( 'NONE',  ( -4.379528057220086978, -16.55341960407618274, 89.79275706135236135 ) ) ;
#3630=CARTESIAN_POINT ( 'NONE',  ( -9.474510206698964154, 16.51473224551069663, 85.41557627198102409 ) ) ;
#3631=CARTESIAN_POINT ( 'NONE',  ( -0.05219959533910754901, -16.53943276465976808, 97.49890960531436690 ) ) ;
#3632=CARTESIAN_POINT ( 'NONE',  ( 4.379528057220339221, -16.55341960407611168, 27.70724293864769905 ) ) ;
#3633=CARTESIAN_POINT ( 'NONE',  ( -19.03943276465977164, -0.05219959533935918106, 63.75109039468566863 ) ) ;
#3634=ADVANCED_FACE ( 'NONE', ( #17223 ), #51107, .T. ) ;
#3635=CARTESIAN_POINT ( 'NONE',  ( 21.53943276465977519, 0.05219959533937863772, 41.25109039468568284 ) ) ;
#3636=CARTESIAN_POINT ( 'NONE',  ( -9.474510206698720793, -16.51473224551083518, 24.58442372801900078 ) ) ;
#3637=CARTESIAN_POINT ( 'NONE',  ( -8.314922557960811034, -14.29746914071050412, 97.08224293864770971 ) ) ;
#3638=CARTESIAN_POINT ( 'NONE',  ( 13.89961937509977652, -13.97604488694527269, 113.1239096053143527 ) ) ;
#3639=CARTESIAN_POINT ( 'NONE',  ( -8.224510206698948167, 14.34966873604960824, 25.41557627198103120 ) ) ;
#3640=CARTESIAN_POINT ( 'NONE',  ( -21.52544592524334988, -5.823673210054445271, 78.95942372801901854 ) ) ;
#3641=CARTESIAN_POINT ( 'NONE',  ( -4.483927247898782831, 16.52544592524335698, 52.70942372801902565 ) ) ;
#3642=CARTESIAN_POINT ( 'NONE',  ( 0.05219959533934541429, -16.53943276465976808, 100.0010903946857042 ) ) ;
#3643=CARTESIAN_POINT ( 'NONE',  ( 18.67979575497194134, -10.72451020669871369, 55.83442372801901854 ) ) ;
#3645=CARTESIAN_POINT ( 'NONE',  ( 18.67979575497194134, -10.72451020669871369, 25.83442372801901499 ) ) ;
#3646=CARTESIAN_POINT ( 'NONE',  ( -16.53943276465976808, 0.05219959533911058130, 101.2489096053143669 ) ) ;
#3647=CARTESIAN_POINT ( 'NONE',  ( 19.05341960407611168, 5.049401038298154454, 28.95724293864769550 ) ) ;
#3648=CARTESIAN_POINT ( 'NONE',  ( -8.314922557960811034, -14.29746914071050412, 72.08224293864769550 ) ) ;
#3649=CARTESIAN_POINT ( 'NONE',  ( 19.02544592524343514, -5.153800228976328945, 68.54057627198103830 ) ) ;
#3650=CARTESIAN_POINT ( 'NONE',  ( 8.224510206698742110, 14.34966873604972548, 102.0844237280190185 ) ) ;
#3651=CARTESIAN_POINT ( 'NONE',  ( -5.153800228976328057, -19.02544592524343514, 37.29057627198102409 ) ) ;
#3652=CARTESIAN_POINT ( 'NONE',  ( -10.72451020669898014, 18.67979575497178502, 50.41557627198103120 ) ) ;
#3653=CARTESIAN_POINT ( 'NONE',  ( 12.06949235617757843, -12.14591786802309237, 88.12390960531436690 ) ) ;
#3654=CARTESIAN_POINT ( 'NONE',  ( 21.53943276465977519, -0.05219959533907433946, 88.74890960531436690 ) ) ;
#3655=CARTESIAN_POINT ( 'NONE',  ( 0.05219959533909260263, 19.03943276465977164, 89.99890960531436690 ) ) ;
#3656=CARTESIAN_POINT ( 'NONE',  ( -19.02544592524342804, 5.153800228976336051, 46.04057627198101699 ) ) ;
#3657=CARTESIAN_POINT ( 'NONE',  ( 19.02544592524334988, 5.153800228976608722, 86.45942372801900433 ) ) ;
#3658=CARTESIAN_POINT ( 'NONE',  ( 15.80617190586746368, 15.72974639402197994, 39.37390960531436690 ) ) ;
#3659=CARTESIAN_POINT ( 'NONE',  ( -18.62759615963255300, -10.81492255796106328, 74.16775706135231871 ) ) ;
#3660=CARTESIAN_POINT ( 'NONE',  ( 9.474510206698971260, -16.51473224551069308, 57.91557627198103120 ) ) ;
#3661=CARTESIAN_POINT ( 'NONE',  ( 5.049401038298161559, -19.05341960407611168, 87.70724293864769550 ) ) ;
#3662=CARTESIAN_POINT ( 'NONE',  ( 16.52544592524335698, 4.483927247898782831, 66.45942372801903275 ) ) ;
#3663=CARTESIAN_POINT ( 'NONE',  ( -10.81492255796105439, 18.62759615963255655, 37.91775706135235424 ) ) ;
#3664=CARTESIAN_POINT ( 'NONE',  ( 5.719274019375673035, 21.55341960407619339, 72.29275706135236135 ) ) ;
#3665=CARTESIAN_POINT ( 'NONE',  ( 9.564922557960805705, 16.46253265017160317, 114.5822429386476955 ) ) ;
#3666=CARTESIAN_POINT ( 'NONE',  ( 18.62759615963271287, -10.81492255796078972, 103.3322429386476955 ) ) ;
#3667=CARTESIAN_POINT ( 'NONE',  ( -21.55341960407619339, 5.719274019375674811, 33.54275706135234714 ) ) ;
#3668=CARTESIAN_POINT ( 'NONE',  ( 0.05219959533934541429, -16.53943276465976808, 70.00109039468568994 ) ) ;
#3669=CARTESIAN_POINT ( 'NONE',  ( 21.53943276465977519, -0.05219959533907433946, 68.74890960531435269 ) ) ;
#3670=CARTESIAN_POINT ( 'NONE',  ( -19.03943276465977164, -0.05219959533935918106, 38.75109039468566152 ) ) ;
#3671=CARTESIAN_POINT ( 'NONE',  ( 19.03943276465977164, -0.05219959533909143690, 68.74890960531436690 ) ) ;
#3672=CARTESIAN_POINT ( 'NONE',  ( -12.06949235617739369, -12.14591786802326823, 109.3760903946857042 ) ) ;
#3674=CARTESIAN_POINT ( 'NONE',  ( 5.153800228976335163, 19.02544592524342804, 104.7905762719809957 ) ) ;
#3675=CARTESIAN_POINT ( 'NONE',  ( 17.50000000000000000, 5.499999999999992895, 96.70309617465829888 ) ) ;
#3676=CARTESIAN_POINT ( 'NONE',  ( 16.46253265017146816, 9.564922557961045513, 81.66775706135233293 ) ) ;
#3677=CARTESIAN_POINT ( 'NONE',  ( -5.719274019375978568, 21.55341960407610458, 60.20724293864768839 ) ) ;
#3678=CARTESIAN_POINT ( 'NONE',  ( -8.314922557960811034, -14.29746914071050412, 37.08224293864768129 ) ) ;
#3679=CARTESIAN_POINT ( 'NONE',  ( -9.564922557961040184, 16.46253265017147172, 112.9177570613523329 ) ) ;
#3680=CARTESIAN_POINT ( 'NONE',  ( 9.474510206698971260, -16.51473224551069308, 37.91557627198102409 ) ) ;
#3681=CARTESIAN_POINT ( 'NONE',  ( 13.89961937509957401, 13.97604488694547697, 106.8760903946856757 ) ) ;
#3682=CARTESIAN_POINT ( 'NONE',  ( 10.72451020669898902, -18.67979575497178502, 92.91557627198103830 ) ) ;
#3683=CARTESIAN_POINT ( 'NONE',  ( -5.153800228976607833, 19.02544592524334988, 62.70942372801899722 ) ) ;
#3684=CARTESIAN_POINT ( 'NONE',  ( 8.314922557961029526, -14.29746914071037800, 75.41775706135233293 ) ) ;
#3685=CARTESIAN_POINT ( 'NONE',  ( -19.05341960407611168, -5.049401038298163336, 66.45724293864769550 ) ) ;
#3686=CARTESIAN_POINT ( 'NONE',  ( -8.314922557960811034, -14.29746914071050412, 72.08224293864769550 ) ) ;
#3687=CARTESIAN_POINT ( 'NONE',  ( -19.03943276465977164, 0.05219959533909376836, 51.24890960531436690 ) ) ;
#3688=CARTESIAN_POINT ( 'NONE',  ( -16.53943276465976808, 0.05219959533911058130, 51.24890960531436690 ) ) ;
#3689=CARTESIAN_POINT ( 'NONE',  ( 19.03943276465977164, -0.05219959533909143690, 23.74890960531435269 ) ) ;
#3691=CARTESIAN_POINT ( 'NONE',  ( 12.06949235617757843, -12.14591786802309237, 23.12390960531436335 ) ) ;
#3692=CARTESIAN_POINT ( 'NONE',  ( 19.03943276465977164, -0.05219959533909143690, 73.74890960531435269 ) ) ;
#3694=CARTESIAN_POINT ( 'NONE',  ( -5.153800228976607833, 19.02544592524334988, 42.70942372801901143 ) ) ;
#3695=CARTESIAN_POINT ( 'NONE',  ( 8.314922557961029526, -14.29746914071037800, 40.41775706135234714 ) ) ;
#3696=CARTESIAN_POINT ( 'NONE',  ( 18.62759615963271287, -10.81492255796078972, 63.33224293864770260 ) ) ;
#3697=CARTESIAN_POINT ( 'NONE',  ( 19.05341960407617918, -5.049401038297876454, 21.04275706135232582 ) ) ;
#3698=CARTESIAN_POINT ( 'NONE',  ( -9.474510206698964154, 16.51473224551069663, 80.41557627198103830 ) ) ;
#3700=CARTESIAN_POINT ( 'NONE',  ( 19.05341960407611168, 5.049401038298154454, 103.9572429386476671 ) ) ;
#3701=CARTESIAN_POINT ( 'NONE',  ( -18.67979575497193778, 10.72451020669871902, 38.33442372801900433 ) ) ;
#3702=CARTESIAN_POINT ( 'NONE',  ( 16.53943276465976808, -0.05219959533910856209, 108.7489096053143669 ) ) ;
#3704=CARTESIAN_POINT ( 'NONE',  ( -5.823673210054116645, -21.52544592524344225, 102.2905762719810383 ) ) ;
#3705=CARTESIAN_POINT ( 'NONE',  ( 9.474510206698971260, -16.51473224551069308, 82.91557627198103830 ) ) ;
#3707=CARTESIAN_POINT ( 'NONE',  ( -0.05219959533937732626, 21.53943276465977519, 27.50109039468567929 ) ) ;
#3709=CARTESIAN_POINT ( 'NONE',  ( -0.05219959533909027116, -19.03943276465977164, 82.49890960531436690 ) ) ;
#3710=CARTESIAN_POINT ( 'NONE',  ( 18.87075004821567603, -5.500000000000079936, 81.17408112101045958 ) ) ;
#3712=CARTESIAN_POINT ( 'NONE',  ( -14.29746914071049879, 8.314922557960819915, 115.8322429386477097 ) ) ;
#3713=CARTESIAN_POINT ( 'NONE',  ( -0.05219959533909027116, -19.03943276465977164, 27.49890960531435624 ) ) ;
#3714=CARTESIAN_POINT ( 'NONE',  ( -19.03943276465977164, -0.05219959533935918106, 103.7510903946856757 ) ) ;
#3716=CARTESIAN_POINT ( 'NONE',  ( 16.52544592524342804, -4.483927247898539470, 108.5405762719810241 ) ) ;
#3717=CARTESIAN_POINT ( 'NONE',  ( 5.823673210054444382, -21.52544592524334988, 85.20942372801901854 ) ) ;
#3718=CARTESIAN_POINT ( 'NONE',  ( 19.03943276465977164, -0.05219959533909143690, 68.74890960531436690 ) ) ;
#3719=CARTESIAN_POINT ( 'NONE',  ( 0.05219959533937995610, -21.53943276465977519, 50.00109039468568994 ) ) ;
#3720=CARTESIAN_POINT ( 'NONE',  ( 18.62759615963255655, 10.81492255796105972, 26.66775706135235424 ) ) ;
#3722=CARTESIAN_POINT ( 'NONE',  ( 13.89961937509977652, -13.97604488694527269, 88.12390960531438111 ) ) ;
#3724=CARTESIAN_POINT ( 'NONE',  ( 14.29746914071037800, 8.314922557961029526, 31.66775706135234358 ) ) ;
#3725=CARTESIAN_POINT ( 'NONE',  ( -18.62759615963270932, 10.81492255796079327, 40.83224293864769550 ) ) ;
#3726=CARTESIAN_POINT ( 'NONE',  ( 5.719274019375673035, 21.55341960407619339, 77.29275706135234714 ) ) ;
#3727=CARTESIAN_POINT ( 'NONE',  ( 13.97604488694527802, 13.89961937509977652, 109.3739096053143669 ) ) ;
#3728=CARTESIAN_POINT ( 'NONE',  ( -0.05219959533936034679, 19.03943276465977164, 102.5010903946856757 ) ) ;
#3729=CARTESIAN_POINT ( 'NONE',  ( -9.564922557960796823, -16.46253265017161027, 62.08224293864769550 ) ) ;
#3730=CARTESIAN_POINT ( 'NONE',  ( 19.05341960407611168, 5.049401038298154454, 88.95724293864769550 ) ) ;
#3731=CARTESIAN_POINT ( 'NONE',  ( -4.379528057220328563, 16.55341960407611168, 105.2072429386477097 ) ) ;
#3732=CARTESIAN_POINT ( 'NONE',  ( 0.05219959533910956823, 16.53943276465976808, 104.9989096053143669 ) ) ;
#3733=CARTESIAN_POINT ( 'NONE',  ( -16.46253265017160317, 9.564922557960807481, 115.8322429386477097 ) ) ;
#3734=CARTESIAN_POINT ( 'NONE',  ( 16.52544592524335698, 4.483927247898782831, 76.45942372801901854 ) ) ;
#3735=CARTESIAN_POINT ( 'NONE',  ( -14.34966873604960291, -8.224510206698953496, 61.66557627198103120 ) ) ;
#3736=CARTESIAN_POINT ( 'NONE',  ( -19.03943276465977164, 0.05219959533909376836, 36.24890960531436690 ) ) ;
#3737=CARTESIAN_POINT ( 'NONE',  ( -5.823673210054431948, 21.52544592524334988, 72.70942372801901854 ) ) ;
#3738=CARTESIAN_POINT ( 'NONE',  ( -16.51473224551082808, 9.474510206698731452, 88.33442372801900433 ) ) ;
#3739=CARTESIAN_POINT ( 'NONE',  ( 4.379528057220339221, -16.55341960407611168, 67.70724293864769550 ) ) ;
#3740=CARTESIAN_POINT ( 'NONE',  ( -18.62759615963255300, -10.81492255796106328, 19.16775706135234714 ) ) ;
#3741=CARTESIAN_POINT ( 'NONE',  ( 5.823673210054125526, 21.52544592524343514, 49.79057627198102409 ) ) ;
#3742=LINE ( 'NONE', #186814, #122762 ) ;
#3744=CARTESIAN_POINT ( 'NONE',  ( 5.153800228976335163, 19.02544592524342804, 69.79057627198103830 ) ) ;
#3745=CARTESIAN_POINT ( 'NONE',  ( 12.06949235617757843, -12.14591786802309237, 43.12390960531435269 ) ) ;
#3746=CARTESIAN_POINT ( 'NONE',  ( 4.379528057220339221, -16.55341960407611168, 22.70724293864769194 ) ) ;
#3747=CARTESIAN_POINT ( 'NONE',  ( -16.55341960407617563, 4.379528057220093196, 83.54275706135234714 ) ) ;
#3748=CARTESIAN_POINT ( 'NONE',  ( -5.049401038297874678, -19.05341960407617918, 44.79275706135232582 ) ) ;
#3750=CARTESIAN_POINT ( 'NONE',  ( 13.89961937509977652, -13.97604488694527269, 98.12390960531433848 ) ) ;
#3751=CARTESIAN_POINT ( 'NONE',  ( -12.14591786802309592, -12.06949235617757132, 56.87390960531436690 ) ) ;
#3752=CARTESIAN_POINT ( 'NONE',  ( 16.20579543436678094, -7.371946100355078357, 101.9347916582813127 ) ) ;
#3753=CARTESIAN_POINT ( 'NONE',  ( -19.02544592524342804, 5.153800228976336051, 116.0405762719810383 ) ) ;
#3754=CARTESIAN_POINT ( 'NONE',  ( -15.72974639402197994, 15.80617190586746368, 50.62390960531435979 ) ) ;
#3756=CARTESIAN_POINT ( 'NONE',  ( -16.53943276465976808, 0.05219959533911058130, 101.2489096053143669 ) ) ;
#3757=CARTESIAN_POINT ( 'NONE',  ( -8.224510206698735004, -14.34966873604973081, 39.58442372801901143 ) ) ;
#3758=CARTESIAN_POINT ( 'NONE',  ( 4.483927247898545687, 16.52544592524342804, 84.79057627198102409 ) ) ;
#3760=CARTESIAN_POINT ( 'NONE',  ( 5.153800228976615827, -19.02544592524334988, 75.20942372801896170 ) ) ;
#3761=CARTESIAN_POINT ( 'NONE',  ( -0.05219959533907301413, -21.53943276465977519, 27.49890960531435269 ) ) ;
#3764=CARTESIAN_POINT ( 'NONE',  ( 14.34966873604972726, -8.224510206698740333, 35.83442372801901143 ) ) ;
#3765=CARTESIAN_POINT ( 'NONE',  ( -16.55341960407611168, -4.379528057220339221, 31.45724293864769550 ) ) ;
#3766=CARTESIAN_POINT ( 'NONE',  ( -21.55341960407610458, -5.719274019375992779, 51.45724293864770260 ) ) ;
#3767=CARTESIAN_POINT ( 'NONE',  ( -9.564922557961040184, 16.46253265017147172, 72.91775706135233293 ) ) ;
#3768=CARTESIAN_POINT ( 'NONE',  ( 18.62759615963271287, -10.81492255796078972, 53.33224293864769550 ) ) ;
#3769=CARTESIAN_POINT ( 'NONE',  ( -10.81492255796105439, 18.62759615963255655, 62.91775706135236135 ) ) ;
#3771=CARTESIAN_POINT ( 'NONE',  ( -16.53943276465976808, -0.05219959533934237506, 38.75109039468567573 ) ) ;
#3772=CARTESIAN_POINT ( 'NONE',  ( -13.89961937509977652, 13.97604488694528158, 30.62390960531435269 ) ) ;
#3773=CARTESIAN_POINT ( 'NONE',  ( -16.46253265017160317, 9.564922557960807481, 90.83224293864769550 ) ) ;
#3774=CARTESIAN_POINT ( 'NONE',  ( -16.51473224551069308, -9.474510206698971260, 31.66557627198102054 ) ) ;
#3775=CARTESIAN_POINT ( 'NONE',  ( -0.05219959533910754901, -16.53943276465976808, 102.4989096053143811 ) ) ;
#3777=CARTESIAN_POINT ( 'NONE',  ( 0.05219959533909260263, 19.03943276465977164, 99.99890960531436690 ) ) ;
#3778=VERTEX_POINT ( 'NONE', #101192 ) ;
#3779=CARTESIAN_POINT ( 'NONE',  ( -4.379528057220086978, -16.55341960407618274, 59.79275706135234714 ) ) ;
#3780=CARTESIAN_POINT ( 'NONE',  ( -21.52544592524343514, 5.823673210054127303, 91.04057627198103830 ) ) ;
#3781=CARTESIAN_POINT ( 'NONE',  ( 13.97604488694527802, 13.89961937509977652, 49.37390960531434558 ) ) ;
#3782=CARTESIAN_POINT ( 'NONE',  ( 0.05219959533936267826, -19.03943276465977164, 75.00109039468566152 ) ) ;
#3783=CARTESIAN_POINT ( 'NONE',  ( 18.62759615963255655, 10.81492255796105972, 31.66775706135234358 ) ) ;
#3784=CARTESIAN_POINT ( 'NONE',  ( 19.03943276465977164, -0.05219959533909143690, 73.74890960531435269 ) ) ;
#3785=CARTESIAN_POINT ( 'NONE',  ( -13.89961937509977652, 13.97604488694528158, 100.6239096053143669 ) ) ;
#3787=CARTESIAN_POINT ( 'NONE',  ( -4.483927247898782831, 16.52544592524335698, 37.70942372801900433 ) ) ;
#3788=CARTESIAN_POINT ( 'NONE',  ( 5.719274019375673035, 21.55341960407619339, 22.29275706135235069 ) ) ;
#3789=CARTESIAN_POINT ( 'NONE',  ( -4.379528057220328563, 16.55341960407611168, 105.2072429386477097 ) ) ;
#3790=CARTESIAN_POINT ( 'NONE',  ( -19.02544592524342804, 5.153800228976336051, 96.04057627198103830 ) ) ;
#3791=CARTESIAN_POINT ( 'NONE',  ( 19.02544592524334988, 5.153800228976608722, 71.45942372801900433 ) ) ;
#3792=CARTESIAN_POINT ( 'NONE',  ( 18.67979575497178502, 10.72451020669898547, 89.16557627198102409 ) ) ;
#3793=CARTESIAN_POINT ( 'NONE',  ( 0.05219959533910956823, 16.53943276465976808, 49.99890960531437401 ) ) ;
#3794=CARTESIAN_POINT ( 'NONE',  ( 19.03943276465977164, 0.05219959533936151252, 26.25109039468566507 ) ) ;
#3795=CARTESIAN_POINT ( 'NONE',  ( -12.06949235617739369, -12.14591786802326823, 74.37609039468568994 ) ) ;
#3796=CARTESIAN_POINT ( 'NONE',  ( 5.153800228976335163, 19.02544592524342804, 89.79057627198102409 ) ) ;
#3797=CARTESIAN_POINT ( 'NONE',  ( 0.05219959533909260263, 19.03943276465977164, 44.99890960531435979 ) ) ;
#3798=CARTESIAN_POINT ( 'NONE',  ( 5.719274019375673035, 21.55341960407619339, 52.29275706135236135 ) ) ;
#3799=CARTESIAN_POINT ( 'NONE',  ( 21.53943276465977519, 0.05219959533937863772, 71.25109039468568994 ) ) ;
#3800=CARTESIAN_POINT ( 'NONE',  ( -9.474510206698964154, 16.51473224551069663, 55.41557627198103120 ) ) ;
#3801=CARTESIAN_POINT ( 'NONE',  ( 10.72451020669871369, 18.67979575497193778, 37.08442372801901143 ) ) ;
#3802=CARTESIAN_POINT ( 'NONE',  ( -19.03943276465977164, -0.05219959533935918106, 83.75109039468567573 ) ) ;
#3803=CARTESIAN_POINT ( 'NONE',  ( -9.564922557960796823, -16.46253265017161027, 37.08224293864768839 ) ) ;
#3804=CARTESIAN_POINT ( 'NONE',  ( 8.224510206698742110, 14.34966873604972548, 92.08442372801901854 ) ) ;
#3805=CARTESIAN_POINT ( 'NONE',  ( -9.564922557960796823, -16.46253265017161027, 67.08224293864769550 ) ) ;
#3806=CARTESIAN_POINT ( 'NONE',  ( -9.474510206698964154, 16.51473224551069663, 110.4155762719810383 ) ) ;
#3807=CARTESIAN_POINT ( 'NONE',  ( -16.46253265017160317, 9.564922557960807481, 50.83224293864770260 ) ) ;
#3808=CARTESIAN_POINT ( 'NONE',  ( 0.05219959533907565091, 21.53943276465977519, 89.99890960531438111 ) ) ;
#3809=CARTESIAN_POINT ( 'NONE',  ( -8.314922557961024197, 14.29746914071037800, 77.91775706135231871 ) ) ;
#3811=CARTESIAN_POINT ( 'NONE',  ( 5.049401038297881783, 19.05341960407617563, 32.29275706135233293 ) ) ;
#3812=CARTESIAN_POINT ( 'NONE',  ( -16.51473224551069308, -9.474510206698971260, 61.66557627198103120 ) ) ;
#3813=CARTESIAN_POINT ( 'NONE',  ( -4.483927247898539470, -16.52544592524342804, 52.29057627198102409 ) ) ;
#3814=CARTESIAN_POINT ( 'NONE',  ( 12.06949235617757843, -12.14591786802309237, 78.12390960531436690 ) ) ;
#3815=CARTESIAN_POINT ( 'NONE',  ( -9.474510206698964154, 16.51473224551069663, 100.4155762719810241 ) ) ;
#3816=CARTESIAN_POINT ( 'NONE',  ( 16.46253265017160672, -9.564922557960803928, 93.33224293864769550 ) ) ;
#3817=CARTESIAN_POINT ( 'NONE',  ( 18.62759615963255655, 10.81492255796105972, 51.66775706135234714 ) ) ;
#3818=CARTESIAN_POINT ( 'NONE',  ( 19.03943276465977164, -0.05219959533909143690, 108.7489096053143527 ) ) ;
#3819=CARTESIAN_POINT ( 'NONE',  ( 5.823673210054444382, -21.52544592524334988, 110.2094237280190185 ) ) ;
#3820=CARTESIAN_POINT ( 'NONE',  ( 16.52544592524335698, 4.483927247898782831, 76.45942372801901854 ) ) ;
#3821=CARTESIAN_POINT ( 'NONE',  ( 15.72974639402176855, 15.80617190586768217, 36.87609039468568994 ) ) ;
#3822=CARTESIAN_POINT ( 'NONE',  ( 19.02544592524343514, -5.153800228976328945, 108.5405762719810383 ) ) ;
#3823=CARTESIAN_POINT ( 'NONE',  ( 21.53943276465977519, -0.05219959533907433946, 108.7489096053143669 ) ) ;
#3824=CARTESIAN_POINT ( 'NONE',  ( 12.14591786802309770, 12.06949235617756955, 54.37390960531435979 ) ) ;
#3825=CARTESIAN_POINT ( 'NONE',  ( 19.02544592524343514, -5.153800228976328945, 58.54057627198102409 ) ) ;
#3826=CARTESIAN_POINT ( 'NONE',  ( 14.34966873604960469, 8.224510206698951720, 79.16557627198103830 ) ) ;
#3827=CARTESIAN_POINT ( 'NONE',  ( -21.55341960407610458, -5.719274019375992779, 36.45724293864768839 ) ) ;
#3828=CARTESIAN_POINT ( 'NONE',  ( -19.02544592524334988, -5.153800228976617603, 38.95942372801900433 ) ) ;
#3829=CARTESIAN_POINT ( 'NONE',  ( 8.224510206698953496, -14.34966873604960469, 112.9155762719810383 ) ) ;
#3830=VERTEX_POINT ( 'NONE', #148727 ) ;
#3831=CARTESIAN_POINT ( 'NONE',  ( -16.53943276465976808, -0.05219959533934237506, 63.75109039468568284 ) ) ;
#3832=CARTESIAN_POINT ( 'NONE',  ( -9.474510206698964154, 16.51473224551069663, 65.41557627198102409 ) ) ;
#3834=CARTESIAN_POINT ( 'NONE',  ( -16.52544592524342804, 4.483927247898546575, 91.04057627198103830 ) ) ;
#3835=CARTESIAN_POINT ( 'NONE',  ( -21.52544592524343514, 5.823673210054127303, 41.04057627198103120 ) ) ;
#3836=ORIENTED_EDGE ( 'NONE', *, *, #177334, .F. ) ;
#3837=CARTESIAN_POINT ( 'NONE',  ( -14.34966873604972548, 8.224510206698743886, 108.3344237280190185 ) ) ;
#3838=CARTESIAN_POINT ( 'NONE',  ( -13.89961937509957401, -13.97604488694547875, 104.3760903946856757 ) ) ;
#3839=CARTESIAN_POINT ( 'NONE',  ( -15.80617190586768217, 15.72974639402176855, 78.12609039468570415 ) ) ;
#3840=CARTESIAN_POINT ( 'NONE',  ( 16.46253265017160672, -9.564922557960803928, 88.33224293864769550 ) ) ;
#3841=CARTESIAN_POINT ( 'NONE',  ( 15.80617190586746368, 15.72974639402197994, 104.3739096053143669 ) ) ;
#3842=CARTESIAN_POINT ( 'NONE',  ( -14.29746914071037622, -8.314922557961029526, 49.16775706135234003 ) ) ;
#3843=CARTESIAN_POINT ( 'NONE',  ( 13.89961937509977652, -13.97604488694527269, 28.12390960531435624 ) ) ;
#3844=CARTESIAN_POINT ( 'NONE',  ( 8.224510206698742110, 14.34966873604972548, 27.08442372801901854 ) ) ;
#3845=CARTESIAN_POINT ( 'NONE',  ( 5.153800228976615827, -19.02544592524334988, 95.20942372801897591 ) ) ;
#3846=CARTESIAN_POINT ( 'NONE',  ( 21.53943276465977519, -0.05219959533907433946, 93.74890960531436690 ) ) ;
#3847=CARTESIAN_POINT ( 'NONE',  ( -13.89961937509957401, -13.97604488694547875, 59.37609039468566863 ) ) ;
#3848=CARTESIAN_POINT ( 'NONE',  ( -17.49999999999999645, 5.499999999999997335, 120.0000000000000142 ) ) ;
#3849=CARTESIAN_POINT ( 'NONE',  ( 21.55341960407610458, 5.719274019375980345, 108.9572429386476955 ) ) ;
#3850=CARTESIAN_POINT ( 'NONE',  ( 16.46253265017160672, -9.564922557960803928, 73.33224293864769550 ) ) ;
#3851=CARTESIAN_POINT ( 'NONE',  ( 5.049401038298161559, -19.05341960407611168, 72.70724293864768129 ) ) ;
#3853=CARTESIAN_POINT ( 'NONE',  ( -16.55341960407617563, 4.379528057220093196, 33.54275706135234714 ) ) ;
#3855=CARTESIAN_POINT ( 'NONE',  ( -10.72451020669870658, -18.67979575497194134, 24.58442372801901499 ) ) ;
#3856=CARTESIAN_POINT ( 'NONE',  ( 8.224510206698953496, -14.34966873604960469, 62.91557627198102409 ) ) ;
#3857=CARTESIAN_POINT ( 'NONE',  ( 5.153800228976335163, 19.02544592524342804, 74.79057627198103830 ) ) ;
#3858=CARTESIAN_POINT ( 'NONE',  ( -14.34966873604972548, 8.224510206698743886, 43.33442372801901143 ) ) ;
#3859=CARTESIAN_POINT ( 'NONE',  ( 16.46253265017146816, 9.564922557961045513, 46.66775706135233293 ) ) ;
#3860=CARTESIAN_POINT ( 'NONE',  ( 5.719274019375673035, 21.55341960407619339, 57.29275706135234714 ) ) ;
#3861=CARTESIAN_POINT ( 'NONE',  ( -16.46253265017146816, -9.564922557961047289, 104.1677570613523329 ) ) ;
#3862=CARTESIAN_POINT ( 'NONE',  ( -19.05341960407611168, -5.049401038298163336, 56.45724293864768129 ) ) ;
#3863=EDGE_CURVE ( 'NONE', #25133, #53699, #36920, .T. ) ;
#3864=CARTESIAN_POINT ( 'NONE',  ( -19.02544592524334988, -5.153800228976617603, 83.95942372801901854 ) ) ;
#3865=CARTESIAN_POINT ( 'NONE',  ( 5.823673210054444382, -21.52544592524334988, 85.20942372801901854 ) ) ;
#3866=CARTESIAN_POINT ( 'NONE',  ( 19.02544592524334988, 5.153800228976608722, 66.45942372801899012 ) ) ;
#3867=CARTESIAN_POINT ( 'NONE',  ( 13.89961937509977652, -13.97604488694527269, 38.12390960531436690 ) ) ;
#3868=CARTESIAN_POINT ( 'NONE',  ( -21.55341960407610458, -5.719274019375992779, 56.45724293864768839 ) ) ;
#3869=CARTESIAN_POINT ( 'NONE',  ( -16.55341960407611168, -4.379528057220339221, 61.45724293864770260 ) ) ;
#3870=CARTESIAN_POINT ( 'NONE',  ( -9.474510206698720793, -16.51473224551083518, 64.58442372801900433 ) ) ;
#3871=CARTESIAN_POINT ( 'NONE',  ( -16.18388926212235646, -7.379444403734649605, 25.43953151366155296 ) ) ;
#3872=CARTESIAN_POINT ( 'NONE',  ( 13.97604488694548053, -13.89961937509957401, 25.62609039468566507 ) ) ;
#3873=CARTESIAN_POINT ( 'NONE',  ( -4.379528057220086978, -16.55341960407618274, 99.79275706135234714 ) ) ;
#3874=CARTESIAN_POINT ( 'NONE',  ( 12.06949235617757843, -12.14591786802309237, 58.12390960531435979 ) ) ;
#3875=CARTESIAN_POINT ( 'NONE',  ( -21.55341960407619339, 5.719274019375674811, 93.54275706135234714 ) ) ;
#3877=CARTESIAN_POINT ( 'NONE',  ( -18.67979575497193778, 10.72451020669871902, 93.33442372801901854 ) ) ;
#3878=CARTESIAN_POINT ( 'NONE',  ( 0.05219959533907565091, 21.53943276465977519, 94.99890960531436690 ) ) ;
#3879=CARTESIAN_POINT ( 'NONE',  ( 9.564922557960805705, 16.46253265017160317, 54.58224293864769550 ) ) ;
#3880=CARTESIAN_POINT ( 'NONE',  ( 21.53943276465977519, 0.05219959533937863772, 66.25109039468567573 ) ) ;
#3881=CARTESIAN_POINT ( 'NONE',  ( 5.153800228976335163, 19.02544592524342804, 54.79057627198103120 ) ) ;
#3882=CARTESIAN_POINT ( 'NONE',  ( -5.049401038298153566, 19.05341960407611168, 70.20724293864769550 ) ) ;
#3883=CARTESIAN_POINT ( 'NONE',  ( -12.06949235617756955, 12.14591786802309770, 110.6239096053143669 ) ) ;
#3884=CARTESIAN_POINT ( 'NONE',  ( 10.72451020669898902, -18.67979575497178502, 22.91557627198102765 ) ) ;
#3885=CARTESIAN_POINT ( 'NONE',  ( -8.314922557960811034, -14.29746914071050412, 52.08224293864768839 ) ) ;
#3886=CARTESIAN_POINT ( 'NONE',  ( -16.51473224551069308, -9.474510206698971260, 26.66557627198103120 ) ) ;
#3887=CARTESIAN_POINT ( 'NONE',  ( -8.314922557960811034, -14.29746914071050412, 77.08224293864769550 ) ) ;
#3888=CARTESIAN_POINT ( 'NONE',  ( -21.53943276465977519, 0.05219959533907696930, 91.24890960531436690 ) ) ;
#3889=CARTESIAN_POINT ( 'NONE',  ( 21.53943276465977519, 0.05219959533937863772, 36.25109039468567573 ) ) ;
#3891=CARTESIAN_POINT ( 'NONE',  ( -14.29746914071037622, -8.314922557961029526, 39.16775706135235424 ) ) ;
#3892=CARTESIAN_POINT ( 'NONE',  ( 15.80617190586746368, 15.72974639402197994, 84.37390960531438111 ) ) ;
#3893=PRODUCT_DEFINITION_CONTEXT ( 'detailed design', #36479, 'design' ) ;
#3894=CARTESIAN_POINT ( 'NONE',  ( -21.55341960407619339, 5.719274019375674811, 113.5427570613523756 ) ) ;
#3895=CARTESIAN_POINT ( 'NONE',  ( 5.049401038298161559, -19.05341960407611168, 87.70724293864769550 ) ) ;
#3896=CARTESIAN_POINT ( 'NONE',  ( 10.72451020669871369, 18.67979575497193778, 47.08442372801901854 ) ) ;
#3897=CARTESIAN_POINT ( 'NONE',  ( -18.62759615963270932, 10.81492255796079327, 25.83224293864769194 ) ) ;
#3898=CARTESIAN_POINT ( 'NONE',  ( -16.53943276465976808, -0.05219959533934237506, 98.75109039468568994 ) ) ;
#3899=CARTESIAN_POINT ( 'NONE',  ( -15.72974639402176322, -15.80617190586768395, 49.37609039468569705 ) ) ;
#3900=CARTESIAN_POINT ( 'NONE',  ( -21.53943276465977519, -0.05219959533937600094, 88.75109039468567573 ) ) ;
#3901=CARTESIAN_POINT ( 'NONE',  ( -13.89961937509957401, -13.97604488694547875, 29.37609039468565797 ) ) ;
#3902=CARTESIAN_POINT ( 'NONE',  ( -4.379528057220086978, -16.55341960407618274, 89.79275706135236135 ) ) ;
#3903=CARTESIAN_POINT ( 'NONE',  ( 10.81492255796106328, -18.62759615963255655, 45.41775706135234003 ) ) ;
#3904=CARTESIAN_POINT ( 'NONE',  ( -5.153800228976328057, -19.02544592524343514, 32.29057627198102409 ) ) ;
#3905=CARTESIAN_POINT ( 'NONE',  ( -21.55341960407619339, 5.719274019375674811, 98.54275706135234714 ) ) ;
#3906=CARTESIAN_POINT ( 'NONE',  ( 5.153800228976335163, 19.02544592524342804, 104.7905762719809957 ) ) ;
#3907=CARTESIAN_POINT ( 'NONE',  ( 5.719274019375991003, -21.55341960407610458, 107.7072429386476955 ) ) ;
#3908=CARTESIAN_POINT ( 'NONE',  ( -18.67979575497178146, -10.72451020669898902, 61.66557627198103120 ) ) ;
#3909=DIRECTION ( 'NONE',  ( 0.000000000000000000, -1.000000000000000000, 0.000000000000000000 ) ) ;
#3910=CARTESIAN_POINT ( 'NONE',  ( 10.72451020669898902, -18.67979575497178502, 62.91557627198102409 ) ) ;
#3911=CARTESIAN_POINT ( 'NONE',  ( 12.06949235617739724, 12.14591786802326823, 46.87609039468568994 ) ) ;
#3912=CARTESIAN_POINT ( 'NONE',  ( -12.14591786802309592, -12.06949235617757132, 56.87390960531436690 ) ) ;
#3914=CARTESIAN_POINT ( 'NONE',  ( 19.02544592524334988, 5.153800228976608722, 96.45942372801897591 ) ) ;
#3916=CARTESIAN_POINT ( 'NONE',  ( 16.52544592524335698, 4.483927247898782831, 21.45942372801901499 ) ) ;
#3917=CARTESIAN_POINT ( 'NONE',  ( -0.05219959533907301413, -21.53943276465977519, 92.49890960531436690 ) ) ;
#3918=CARTESIAN_POINT ( 'NONE',  ( -21.53943276465977519, 0.05219959533907696930, 76.24890960531435269 ) ) ;
#3919=CARTESIAN_POINT ( 'NONE',  ( -5.049401038298153566, 19.05341960407611168, 110.2072429386476671 ) ) ;
#3920=CARTESIAN_POINT ( 'NONE',  ( -8.314922557961024197, 14.29746914071037800, 52.91775706135235424 ) ) ;
#3921=CARTESIAN_POINT ( 'NONE',  ( 19.03943276465977164, -0.05219959533909143690, 73.74890960531435269 ) ) ;
#3922=CARTESIAN_POINT ( 'NONE',  ( -5.719274019375665041, -21.55341960407619695, 29.79275706135234358 ) ) ;
#3923=CARTESIAN_POINT ( 'NONE',  ( 16.51473224551083163, -9.474510206698727899, 105.8344237280190043 ) ) ;
#3924=CARTESIAN_POINT ( 'NONE',  ( -13.97604488694527625, -13.89961937509977652, 106.8739096053143669 ) ) ;
#3925=CARTESIAN_POINT ( 'NONE',  ( 16.51473224551069308, 9.474510206698969483, 84.16557627198102409 ) ) ;
#3926=CARTESIAN_POINT ( 'NONE',  ( -5.719274019375978568, 21.55341960407610458, 85.20724293864770971 ) ) ;
#3927=CARTESIAN_POINT ( 'NONE',  ( 5.049401038298161559, -19.05341960407611168, 62.70724293864769550 ) ) ;
#3928=CARTESIAN_POINT ( 'NONE',  ( -17.26058549869089376, -6.457015423128632747, 61.37745837476070676 ) ) ;
#3929=CARTESIAN_POINT ( 'NONE',  ( 14.34966873604960469, 8.224510206698951720, 64.16557627198102409 ) ) ;
#3930=CARTESIAN_POINT ( 'NONE',  ( -16.46253265017160317, 9.564922557960807481, 115.8322429386477097 ) ) ;
#3932=CARTESIAN_POINT ( 'NONE',  ( 15.72974639402199770, -15.80617190586745480, 108.1239096053143811 ) ) ;
#3933=CARTESIAN_POINT ( 'NONE',  ( 16.51473224551083163, -9.474510206698727899, 60.83442372801900433 ) ) ;
#3934=CARTESIAN_POINT ( 'NONE',  ( 19.02544592524343514, -5.153800228976328945, 108.5405762719810383 ) ) ;
#3935=CARTESIAN_POINT ( 'NONE',  ( 9.474510206698971260, -16.51473224551069308, 27.91557627198103120 ) ) ;
#3936=CARTESIAN_POINT ( 'NONE',  ( 21.52544592524344225, -5.823673210054117533, 58.54057627198103120 ) ) ;
#3937=CARTESIAN_POINT ( 'NONE',  ( -13.97604488694527625, -13.89961937509977652, 86.87390960531436690 ) ) ;
#3938=CARTESIAN_POINT ( 'NONE',  ( 5.719274019375673035, 21.55341960407619339, 82.29275706135234714 ) ) ;
#3939=CARTESIAN_POINT ( 'NONE',  ( -19.02544592524342804, 5.153800228976336051, 56.04057627198100988 ) ) ;
#3941=CARTESIAN_POINT ( 'NONE',  ( -16.55341960407611168, -4.379528057220339221, 81.45724293864769550 ) ) ;
#3942=CARTESIAN_POINT ( 'NONE',  ( -14.29746914071037622, -8.314922557961029526, 34.16775706135234714 ) ) ;
#3943=CARTESIAN_POINT ( 'NONE',  ( -15.72974639402176322, -15.80617190586768395, 69.37609039468567573 ) ) ;
#3945=CARTESIAN_POINT ( 'NONE',  ( -19.02544592524334988, -5.153800228976617603, 23.95942372801900078 ) ) ;
#3946=CARTESIAN_POINT ( 'NONE',  ( 5.049401038297881783, 19.05341960407617563, 77.29275706135231871 ) ) ;
#3947=CARTESIAN_POINT ( 'NONE',  ( -19.03943276465977164, -0.05219959533935918106, 38.75109039468566152 ) ) ;
#3949=CARTESIAN_POINT ( 'NONE',  ( -18.67979575497193778, 10.72451020669871902, 43.33442372801901143 ) ) ;
#3950=DIRECTION ( 'NONE',  ( 4.336808689942018229E-16, -1.000000000000000000, -0.000000000000000000 ) ) ;
#3951=CARTESIAN_POINT ( 'NONE',  ( -0.05219959533936034679, 19.03943276465977164, 32.50109039468566863 ) ) ;
#3952=CARTESIAN_POINT ( 'NONE',  ( -9.474510206698964154, 16.51473224551069663, 50.41557627198102409 ) ) ;
#3953=CARTESIAN_POINT ( 'NONE',  ( -5.049401038297874678, -19.05341960407617918, 29.79275706135232227 ) ) ;
#3954=CARTESIAN_POINT ( 'NONE',  ( -16.52544592524335698, -4.483927247898792601, 98.95942372801903275 ) ) ;
#3955=CARTESIAN_POINT ( 'NONE',  ( 13.97604488694527802, 13.89961937509977652, 109.3739096053143669 ) ) ;
#3956=CARTESIAN_POINT ( 'NONE',  ( -0.05219959533937732626, 21.53943276465977519, 82.50109039468568994 ) ) ;
#3959=CARTESIAN_POINT ( 'NONE',  ( -15.72974639402176322, -15.80617190586768395, 89.37609039468568994 ) ) ;
#3961=CARTESIAN_POINT ( 'NONE',  ( -16.51473224551069308, -9.474510206698971260, 106.6655762719810383 ) ) ;
#3963=CARTESIAN_POINT ( 'NONE',  ( -13.89961937509977652, 13.97604488694528158, 55.62390960531434558 ) ) ;
#3964=CARTESIAN_POINT ( 'NONE',  ( 21.53943276465977519, -0.05219959533907433946, 53.74890960531437401 ) ) ;
#3965=CARTESIAN_POINT ( 'NONE',  ( 14.34966873604960469, 8.224510206698951720, 24.16557627198103120 ) ) ;
#3966=CARTESIAN_POINT ( 'NONE',  ( 12.06949235617757843, -12.14591786802309237, 98.12390960531436690 ) ) ;
#3967=CARTESIAN_POINT ( 'NONE',  ( 13.89961937509977652, -13.97604488694527269, 93.12390960531436690 ) ) ;
#3968=CARTESIAN_POINT ( 'NONE',  ( 9.564922557961047289, -16.46253265017146816, 25.41775706135234003 ) ) ;
#3969=CARTESIAN_POINT ( 'NONE',  ( -19.03943276465977164, 0.05219959533909376836, 36.24890960531436690 ) ) ;
#3970=CARTESIAN_POINT ( 'NONE',  ( 4.379528057220339221, -16.55341960407611168, 107.7072429386476955 ) ) ;
#3971=CARTESIAN_POINT ( 'NONE',  ( -15.80617190586768217, 15.72974639402176855, 53.12609039468568284 ) ) ;
#3972=CARTESIAN_POINT ( 'NONE',  ( -16.53943276465976808, -0.05219959533934237506, 108.7510903946857042 ) ) ;
#3973=CARTESIAN_POINT ( 'NONE',  ( 5.049401038297881783, 19.05341960407617563, 62.29275706135234003 ) ) ;
#3975=CARTESIAN_POINT ( 'NONE',  ( -16.46253265017160317, 9.564922557960807481, 110.8322429386476955 ) ) ;
#3976=CARTESIAN_POINT ( 'NONE',  ( 14.34966873604960469, 8.224510206698951720, 79.16557627198103830 ) ) ;
#3977=CARTESIAN_POINT ( 'NONE',  ( -19.05341960407617563, 5.049401038297882671, 43.54275706135232582 ) ) ;
#3978=CARTESIAN_POINT ( 'NONE',  ( 0.05219959533909260263, 19.03943276465977164, 64.99890960531436690 ) ) ;
#3979=CARTESIAN_POINT ( 'NONE',  ( -4.483927247898539470, -16.52544592524342804, 57.29057627198103120 ) ) ;
#3980=CARTESIAN_POINT ( 'NONE',  ( 5.153800228976615827, -19.02544592524334988, 85.20942372801900433 ) ) ;
#3981=CARTESIAN_POINT ( 'NONE',  ( -21.55341960407610458, -5.719274019375992779, 36.45724293864768839 ) ) ;
#3982=ORIENTED_EDGE ( 'NONE', *, *, #6380, .F. ) ;
#3983=CARTESIAN_POINT ( 'NONE',  ( 8.224510206698953496, -14.34966873604960469, 107.9155762719810241 ) ) ;
#3985=CARTESIAN_POINT ( 'NONE',  ( 16.51473224551069308, 9.474510206698969483, 59.16557627198102409 ) ) ;
#3986=CARTESIAN_POINT ( 'NONE',  ( 5.823673210054125526, 21.52544592524343514, 59.79057627198103120 ) ) ;
#3987=CARTESIAN_POINT ( 'NONE',  ( -13.97604488694527625, -13.89961937509977652, 41.87390960531435979 ) ) ;
#3988=CARTESIAN_POINT ( 'NONE',  ( 16.52544592524335698, 4.483927247898782831, 91.45942372801901854 ) ) ;
#3989=CARTESIAN_POINT ( 'NONE',  ( 13.89961937509977652, -13.97604488694527269, 78.12390960531433848 ) ) ;
#3990=CARTESIAN_POINT ( 'NONE',  ( -5.049401038297874678, -19.05341960407617918, 59.79275706135231871 ) ) ;
#3991=CARTESIAN_POINT ( 'NONE',  ( -15.80617190586768217, 15.72974639402176855, 73.12609039468567573 ) ) ;
#3992=CARTESIAN_POINT ( 'NONE',  ( -5.719274019375978568, 21.55341960407610458, 45.20724293864769550 ) ) ;
#3993=CARTESIAN_POINT ( 'NONE',  ( -0.05219959533909027116, -19.03943276465977164, 102.4989096053143669 ) ) ;
#3994=CARTESIAN_POINT ( 'NONE',  ( 9.564922557960805705, 16.46253265017160317, 29.58224293864769550 ) ) ;
#3995=CARTESIAN_POINT ( 'NONE',  ( -14.34966873604972548, 8.224510206698743886, 88.33442372801901854 ) ) ;
#3997=CARTESIAN_POINT ( 'NONE',  ( -19.05341960407617563, 5.049401038297882671, 103.5427570613523329 ) ) ;
#4000=CARTESIAN_POINT ( 'NONE',  ( 21.52544592524334988, 5.823673210054432836, 96.45942372801901854 ) ) ;
#4001=CARTESIAN_POINT ( 'NONE',  ( 16.52544592524342804, -4.483927247898539470, 58.54057627198103120 ) ) ;
#4002=CARTESIAN_POINT ( 'NONE',  ( 16.52544592524342804, -4.483927247898539470, 68.54057627198103830 ) ) ;
#4003=CARTESIAN_POINT ( 'NONE',  ( 5.719274019375991003, -21.55341960407610458, 97.70724293864772392 ) ) ;
#4004=CARTESIAN_POINT ( 'NONE',  ( 10.72451020669898902, -18.67979575497178502, 82.91557627198103830 ) ) ;
#4006=CARTESIAN_POINT ( 'NONE',  ( 21.55341960407610458, 5.719274019375980345, 38.95724293864768839 ) ) ;
#4007=CARTESIAN_POINT ( 'NONE',  ( -4.483927247898782831, 16.52544592524335698, 62.70942372801902565 ) ) ;
#4008=CARTESIAN_POINT ( 'NONE',  ( 8.314922557960818139, 14.29746914071049879, 89.58224293864768129 ) ) ;
#4009=CARTESIAN_POINT ( 'NONE',  ( 0.05219959533909260263, 19.03943276465977164, 39.99890960531436690 ) ) ;
#4012=CARTESIAN_POINT ( 'NONE',  ( 14.29746914071037800, 8.314922557961029526, 96.66775706135234714 ) ) ;
#4013=CARTESIAN_POINT ( 'NONE',  ( 15.72974639402176855, 15.80617190586768217, 31.87609039468567929 ) ) ;
#4014=CARTESIAN_POINT ( 'NONE',  ( 19.05341960407611168, 5.049401038298154454, 78.95724293864769550 ) ) ;
#4015=CARTESIAN_POINT ( 'NONE',  ( 15.80617190586769283, -15.72974639402175789, 65.62609039468568994 ) ) ;
#4016=CARTESIAN_POINT ( 'NONE',  ( 9.564922557960805705, 16.46253265017160317, 109.5822429386476955 ) ) ;
#4019=CARTESIAN_POINT ( 'NONE',  ( -18.67979575497193778, 10.72451020669871902, 63.33442372801900433 ) ) ;
#4020=CARTESIAN_POINT ( 'NONE',  ( -19.03943276465977164, 0.05219959533909376836, 41.24890960531435269 ) ) ;
#4021=CARTESIAN_POINT ( 'NONE',  ( 5.153800228976335163, 19.02544592524342804, 114.7905762719810241 ) ) ;
#4022=CARTESIAN_POINT ( 'NONE',  ( 0.05219959533936267826, -19.03943276465977164, 65.00109039468567573 ) ) ;
#4023=CARTESIAN_POINT ( 'NONE',  ( -5.823673210054431948, 21.52544592524334988, 22.70942372801901499 ) ) ;
#4024=CARTESIAN_POINT ( 'NONE',  ( -9.474510206698720793, -16.51473224551083518, 54.58442372801899722 ) ) ;
#4025=CARTESIAN_POINT ( 'NONE',  ( 5.049401038298161559, -19.05341960407611168, 27.70724293864769550 ) ) ;
#4026=CARTESIAN_POINT ( 'NONE',  ( -12.14591786802326823, 12.06949235617739902, 98.12609039468570415 ) ) ;
#4027=CARTESIAN_POINT ( 'NONE',  ( -19.02544592524334988, -5.153800228976617603, 63.95942372801899012 ) ) ;
#4028=CARTESIAN_POINT ( 'NONE',  ( 4.379528057220339221, -16.55341960407611168, 22.70724293864769194 ) ) ;
#4029=CARTESIAN_POINT ( 'NONE',  ( 16.46253265017146816, 9.564922557961045513, 46.66775706135233293 ) ) ;
#4031=CARTESIAN_POINT ( 'NONE',  ( -5.049401038298153566, 19.05341960407611168, 90.20724293864766707 ) ) ;
#4032=CARTESIAN_POINT ( 'NONE',  ( 5.823673210054444382, -21.52544592524334988, 90.20942372801903275 ) ) ;
#4033=CARTESIAN_POINT ( 'NONE',  ( -18.67979575497193778, 10.72451020669871902, 113.3344237280190328 ) ) ;
#4034=CARTESIAN_POINT ( 'NONE',  ( -22.00000000000000000, -1.163414459189985801E-14, 95.00000000000000000 ) ) ;
#4035=CARTESIAN_POINT ( 'NONE',  ( -18.62759615963255300, -10.81492255796106328, 89.16775706135236135 ) ) ;
#4036=CARTESIAN_POINT ( 'NONE',  ( 14.29746914071037800, 8.314922557961029526, 36.66775706135234714 ) ) ;
#4037=CARTESIAN_POINT ( 'NONE',  ( 9.474510206698971260, -16.51473224551069308, 87.91557627198102409 ) ) ;
#4038=CARTESIAN_POINT ( 'NONE',  ( -0.05219959533907301413, -21.53943276465977519, 32.49890960531435979 ) ) ;
#4041=CARTESIAN_POINT ( 'NONE',  ( -13.97604488694527625, -13.89961937509977652, 81.87390960531436690 ) ) ;
#4042=CARTESIAN_POINT ( 'NONE',  ( -19.25176906914649777, -5.499999999999744205, 40.99927264242279534 ) ) ;
#4043=CARTESIAN_POINT ( 'NONE',  ( 19.05341960407617918, -5.049401038297876454, 66.04275706135233293 ) ) ;
#4044=CARTESIAN_POINT ( 'NONE',  ( -13.89961937509977652, 13.97604488694528158, 100.6239096053143669 ) ) ;
#4045=CARTESIAN_POINT ( 'NONE',  ( -21.53943276465977519, -0.05219959533937600094, 103.7510903946857042 ) ) ;
#4046=CARTESIAN_POINT ( 'NONE',  ( 12.14591786802309770, 12.06949235617756955, 99.37390960531436690 ) ) ;
#4047=CARTESIAN_POINT ( 'NONE',  ( -21.55341960407610458, -5.719274019375992779, 46.45724293864769550 ) ) ;
#4048=CARTESIAN_POINT ( 'NONE',  ( -10.72451020669898014, 18.67979575497178502, 35.41557627198102409 ) ) ;
#4049=CARTESIAN_POINT ( 'NONE',  ( 16.55341960407611168, 4.379528057220329451, 108.9572429386476955 ) ) ;
#4051=CARTESIAN_POINT ( 'NONE',  ( 19.02544592524334988, 5.153800228976608722, 61.45942372801900433 ) ) ;
#4052=CARTESIAN_POINT ( 'NONE',  ( -14.34966873604972548, 8.224510206698743886, 113.3344237280190328 ) ) ;
#4053=CARTESIAN_POINT ( 'NONE',  ( -19.05341960407611168, -5.049401038298163336, 96.45724293864769550 ) ) ;
#4054=CARTESIAN_POINT ( 'NONE',  ( -18.67979575497193778, 10.72451020669871902, 78.33442372801901854 ) ) ;
#4055=CARTESIAN_POINT ( 'NONE',  ( -21.53943276465977519, 0.05219959533907696930, 61.24890960531435979 ) ) ;
#4056=CARTESIAN_POINT ( 'NONE',  ( 21.53943276465977519, 0.05219959533937863772, 41.25109039468568284 ) ) ;
#4057=CARTESIAN_POINT ( 'NONE',  ( 10.81492255796078972, 18.62759615963270932, 94.58224293864769550 ) ) ;
#4058=CARTESIAN_POINT ( 'NONE',  ( -10.72451020669870658, -18.67979575497194134, 39.58442372801901143 ) ) ;
#4059=CARTESIAN_POINT ( 'NONE',  ( 9.474510206698971260, -16.51473224551069308, 27.91557627198103120 ) ) ;
#4060=CARTESIAN_POINT ( 'NONE',  ( -9.474510206698964154, 16.51473224551069663, 80.41557627198103830 ) ) ;
#4061=CARTESIAN_POINT ( 'NONE',  ( 8.224510206698742110, 14.34966873604972548, 77.08442372801901854 ) ) ;
#4062=CARTESIAN_POINT ( 'NONE',  ( -14.34966873604960291, -8.224510206698953496, 101.6655762719810383 ) ) ;
#4063=CARTESIAN_POINT ( 'NONE',  ( 13.89961937509977652, -13.97604488694527269, 113.1239096053143527 ) ) ;
#4064=CARTESIAN_POINT ( 'NONE',  ( -16.53943276465976808, 0.05219959533911058130, 56.24890960531436690 ) ) ;
#4065=CARTESIAN_POINT ( 'NONE',  ( 8.224510206698953496, -14.34966873604960469, 22.91557627198102765 ) ) ;
#4066=CARTESIAN_POINT ( 'NONE',  ( 9.474510206698971260, -16.51473224551069308, 47.91557627198102409 ) ) ;
#4067=CARTESIAN_POINT ( 'NONE',  ( -13.89961937509977652, 13.97604488694528158, 30.62390960531435269 ) ) ;
#4068=CARTESIAN_POINT ( 'NONE',  ( -18.67979575497178146, -10.72451020669898902, 41.66557627198103120 ) ) ;
#4070=CARTESIAN_POINT ( 'NONE',  ( 19.02544592524334988, 5.153800228976608722, 21.45942372801899012 ) ) ;
#4071=CARTESIAN_POINT ( 'NONE',  ( -17.49999999999998934, -5.622605283950890431, 41.31207310596112592 ) ) ;
#4072=CARTESIAN_POINT ( 'NONE',  ( 4.379528057220339221, -16.55341960407611168, 32.70724293864770260 ) ) ;
#4073=CARTESIAN_POINT ( 'NONE',  ( -5.719274019375665041, -21.55341960407619695, 49.79275706135234714 ) ) ;
#4074=CARTESIAN_POINT ( 'NONE',  ( 16.51473224551069308, 9.474510206698969483, 114.1655762719810241 ) ) ;
#4075=CARTESIAN_POINT ( 'NONE',  ( -8.314922557961024197, 14.29746914071037800, 62.91775706135236135 ) ) ;
#4076=CARTESIAN_POINT ( 'NONE',  ( 19.05341960407617918, -5.049401038297876454, 66.04275706135233293 ) ) ;
#4077=CARTESIAN_POINT ( 'NONE',  ( -14.34966873604960291, -8.224510206698953496, 31.66557627198102054 ) ) ;
#4078=CARTESIAN_POINT ( 'NONE',  ( 12.14591786802327356, -12.06949235617739191, 100.6260903946857184 ) ) ;
#4079=CARTESIAN_POINT ( 'NONE',  ( -0.05219959533909027116, -19.03943276465977164, 37.49890960531436690 ) ) ;
#4080=CARTESIAN_POINT ( 'NONE',  ( 5.153800228976335163, 19.02544592524342804, 59.79057627198100988 ) ) ;
#4081=CARTESIAN_POINT ( 'NONE',  ( -9.474510206698964154, 16.51473224551069663, 25.41557627198103120 ) ) ;
#4082=CARTESIAN_POINT ( 'NONE',  ( 15.80617190586769283, -15.72974639402175789, 30.62609039468567929 ) ) ;
#4083=CARTESIAN_POINT ( 'NONE',  ( -19.03943276465977164, 0.05219959533909376836, 51.24890960531436690 ) ) ;
#4085=CARTESIAN_POINT ( 'NONE',  ( -9.564922557960796823, -16.46253265017161027, 47.08224293864769550 ) ) ;
#4086=CARTESIAN_POINT ( 'NONE',  ( 13.97604488694527802, 13.89961937509977652, 114.3739096053143669 ) ) ;
#4087=CARTESIAN_POINT ( 'NONE',  ( 10.72451020669871369, 18.67979575497193778, 62.08442372801901143 ) ) ;
#4088=CARTESIAN_POINT ( 'NONE',  ( -8.224510206698948167, 14.34966873604960824, 110.4155762719810383 ) ) ;
#4089=CARTESIAN_POINT ( 'NONE',  ( 19.03943276465977164, -0.05219959533909143690, 108.7489096053143527 ) ) ;
#4090=CARTESIAN_POINT ( 'NONE',  ( 16.53943276465976808, 0.05219959533934440121, 81.25109039468568994 ) ) ;
#4091=CARTESIAN_POINT ( 'NONE',  ( 15.72974639402176855, 15.80617190586768217, 86.87609039468568994 ) ) ;
#4092=CARTESIAN_POINT ( 'NONE',  ( -8.224510206698735004, -14.34966873604973081, 49.58442372801901143 ) ) ;
#4093=CARTESIAN_POINT ( 'NONE',  ( -5.049401038298153566, 19.05341960407611168, 100.2072429386476955 ) ) ;
#4094=CARTESIAN_POINT ( 'NONE',  ( -14.29746914071037622, -8.314922557961029526, 44.16775706135234714 ) ) ;
#4095=CARTESIAN_POINT ( 'NONE',  ( 14.29746914071037800, 8.314922557961029526, 26.66775706135235424 ) ) ;
#4096=CARTESIAN_POINT ( 'NONE',  ( 12.06949235617739724, 12.14591786802326823, 86.87609039468568994 ) ) ;
#4097=CARTESIAN_POINT ( 'NONE',  ( 13.97604488694548053, -13.89961937509957401, 110.6260903946856615 ) ) ;
#4098=CARTESIAN_POINT ( 'NONE',  ( 21.55341960407610458, 5.719274019375980345, 103.9572429386476813 ) ) ;
#4099=CARTESIAN_POINT ( 'NONE',  ( 4.483927247898545687, 16.52544592524342804, 109.7905762719810383 ) ) ;
#4100=CARTESIAN_POINT ( 'NONE',  ( -16.46253265017146816, -9.564922557961047289, 99.16775706135233293 ) ) ;
#4101=CARTESIAN_POINT ( 'NONE',  ( -12.14591786802326823, 12.06949235617739902, 68.12609039468567573 ) ) ;
#4103=CARTESIAN_POINT ( 'NONE',  ( 5.153800228976615827, -19.02544592524334988, 65.20942372801900433 ) ) ;
#4104=CARTESIAN_POINT ( 'NONE',  ( 8.224510206698953496, -14.34966873604960469, 42.91557627198103120 ) ) ;
#4105=CARTESIAN_POINT ( 'NONE',  ( 0.05219959533910956823, 16.53943276465976808, 34.99890960531435979 ) ) ;
#4106=CARTESIAN_POINT ( 'NONE',  ( -16.52544592524342804, 4.483927247898546575, 91.04057627198103830 ) ) ;
#4107=CARTESIAN_POINT ( 'NONE',  ( -5.049401038297874678, -19.05341960407617918, 29.79275706135232227 ) ) ;
#4109=CARTESIAN_POINT ( 'NONE',  ( 18.67979575497194134, -10.72451020669871369, 40.83442372801901854 ) ) ;
#4110=CARTESIAN_POINT ( 'NONE',  ( 0.05219959533936267826, -19.03943276465977164, 100.0010903946856757 ) ) ;
#4112=CARTESIAN_POINT ( 'NONE',  ( 9.474510206698971260, -16.51473224551069308, 87.91557627198102409 ) ) ;
#4113=CARTESIAN_POINT ( 'NONE',  ( 0.05219959533909260263, 19.03943276465977164, 89.99890960531436690 ) ) ;
#4114=CARTESIAN_POINT ( 'NONE',  ( -10.72451020669898014, 18.67979575497178502, 55.41557627198102409 ) ) ;
#4115=CARTESIAN_POINT ( 'NONE',  ( 14.29746914071049879, -8.314922557960816363, 88.33224293864769550 ) ) ;
#4116=CARTESIAN_POINT ( 'NONE',  ( -5.049401038298153566, 19.05341960407611168, 75.20724293864769550 ) ) ;
#4117=CARTESIAN_POINT ( 'NONE',  ( 19.02544592524343514, -5.153800228976328945, 33.54057627198102409 ) ) ;
#4118=CARTESIAN_POINT ( 'NONE',  ( 15.80617190586769283, -15.72974639402175789, 35.62609039468568994 ) ) ;
#4119=CARTESIAN_POINT ( 'NONE',  ( 5.719274019375673035, 21.55341960407619339, 77.29275706135234714 ) ) ;
#4120=CARTESIAN_POINT ( 'NONE',  ( 13.97604488694527802, 13.89961937509977652, 59.37390960531434558 ) ) ;
#4121=CARTESIAN_POINT ( 'NONE',  ( -16.55341960407617563, 4.379528057220093196, 78.54275706135236135 ) ) ;
#4123=CARTESIAN_POINT ( 'NONE',  ( 10.72451020669871369, 18.67979575497193778, 32.08442372801901854 ) ) ;
#4124=CARTESIAN_POINT ( 'NONE',  ( 0.05219959533937995610, -21.53943276465977519, 20.00109039468568639 ) ) ;
#4125=CARTESIAN_POINT ( 'NONE',  ( -19.05341960407617563, 5.049401038297882671, 48.54275706135233293 ) ) ;
#4126=CARTESIAN_POINT ( 'NONE',  ( 13.89961937509977652, -13.97604488694527269, 78.12390960531433848 ) ) ;
#4127=CARTESIAN_POINT ( 'NONE',  ( -19.05341960407617563, 5.049401038297882671, 28.54275706135232937 ) ) ;
#4128=CARTESIAN_POINT ( 'NONE',  ( -10.72451020669870658, -18.67979575497194134, 84.58442372801903275 ) ) ;
#4129=CARTESIAN_POINT ( 'NONE',  ( 18.67979575497178502, 10.72451020669898547, 69.16557627198102409 ) ) ;
#4130=CARTESIAN_POINT ( 'NONE',  ( -16.53943276465976808, 0.05219959533911058130, 56.24890960531436690 ) ) ;
#4131=CARTESIAN_POINT ( 'NONE',  ( 0.05219959533937995610, -21.53943276465977519, 95.00109039468568994 ) ) ;
#4132=CARTESIAN_POINT ( 'NONE',  ( 13.97604488694548053, -13.89961937509957401, 25.62609039468566507 ) ) ;
#4133=CARTESIAN_POINT ( 'NONE',  ( 4.379528057220339221, -16.55341960407611168, 72.70724293864769550 ) ) ;
#4134=CARTESIAN_POINT ( 'NONE',  ( 9.474510206698971260, -16.51473224551069308, 27.91557627198103120 ) ) ;
#4135=CARTESIAN_POINT ( 'NONE',  ( 0.05219959533936267826, -19.03943276465977164, 75.00109039468566152 ) ) ;
#4136=CARTESIAN_POINT ( 'NONE',  ( -4.379528057220328563, 16.55341960407611168, 40.20724293864769550 ) ) ;
#4137=CARTESIAN_POINT ( 'NONE',  ( -15.72974639402176322, -15.80617190586768395, 79.37609039468567573 ) ) ;
#4138=CARTESIAN_POINT ( 'NONE',  ( -9.564922557960796823, -16.46253265017161027, 77.08224293864769550 ) ) ;
#4139=CARTESIAN_POINT ( 'NONE',  ( -13.89961937509957401, -13.97604488694547875, 44.37609039468566863 ) ) ;
#4140=CARTESIAN_POINT ( 'NONE',  ( -10.81492255796078084, -18.62759615963271287, 52.08224293864768839 ) ) ;
#4141=CARTESIAN_POINT ( 'NONE',  ( -21.52544592524334988, -5.823673210054445271, 18.95942372801901143 ) ) ;
#4142=CARTESIAN_POINT ( 'NONE',  ( 16.52544592524335698, 4.483927247898782831, 21.45942372801901499 ) ) ;
#4143=CARTESIAN_POINT ( 'NONE',  ( -4.483927247898782831, 16.52544592524335698, 72.70942372801901854 ) ) ;
#4145=CARTESIAN_POINT ( 'NONE',  ( -15.80617190586745835, -15.72974639402198527, 111.8739096053143669 ) ) ;
#4146=CARTESIAN_POINT ( 'NONE',  ( -14.34966873604960291, -8.224510206698953496, 106.6655762719810383 ) ) ;
#4147=CARTESIAN_POINT ( 'NONE',  ( -17.49999999999998579, -3.237210098469594399, 30.28763012620448691 ) ) ;
#4148=CARTESIAN_POINT ( 'NONE',  ( 16.53943276465976808, 0.05219959533934440121, 41.25109039468568284 ) ) ;
#4149=CARTESIAN_POINT ( 'NONE',  ( -18.67979575497178146, -10.72451020669898902, 66.66557627198102409 ) ) ;
#4150=CARTESIAN_POINT ( 'NONE',  ( 4.483927247898790824, -16.52544592524335698, 105.2094237280190328 ) ) ;
#4151=CARTESIAN_POINT ( 'NONE',  ( -0.05219959533909027116, -19.03943276465977164, 37.49890960531436690 ) ) ;
#4152=CARTESIAN_POINT ( 'NONE',  ( -14.34966873604972548, 8.224510206698743886, 68.33442372801900433 ) ) ;
#4153=CARTESIAN_POINT ( 'NONE',  ( -16.51473224551082808, 9.474510206698731452, 58.33442372801900433 ) ) ;
#4154=CARTESIAN_POINT ( 'NONE',  ( -5.719274019375665041, -21.55341960407619695, 39.79275706135235424 ) ) ;
#4155=CARTESIAN_POINT ( 'NONE',  ( -10.81492255796078084, -18.62759615963271287, 62.08224293864769550 ) ) ;
#4156=CARTESIAN_POINT ( 'NONE',  ( 14.29746914071037800, 8.314922557961029526, 101.6677570613523613 ) ) ;
#4157=CARTESIAN_POINT ( 'NONE',  ( 21.55341960407619695, -5.719274019375665929, 81.04275706135236135 ) ) ;
#4158=CARTESIAN_POINT ( 'NONE',  ( 21.53943276465977519, -0.05219959533907433946, 58.74890960531436690 ) ) ;
#4159=CARTESIAN_POINT ( 'NONE',  ( -21.52544592524343514, 5.823673210054127303, 41.04057627198103120 ) ) ;
#4161=CARTESIAN_POINT ( 'NONE',  ( -4.483927247898782831, 16.52544592524335698, 82.70942372801900433 ) ) ;
#4162=CARTESIAN_POINT ( 'NONE',  ( 15.72974639402199770, -15.80617190586745480, 43.12390960531435269 ) ) ;
#4164=CARTESIAN_POINT ( 'NONE',  ( -19.05341960407611168, -5.049401038298163336, 96.45724293864769550 ) ) ;
#4165=CARTESIAN_POINT ( 'NONE',  ( 12.06949235617739724, 12.14591786802326823, 111.8760903946856615 ) ) ;
#4167=CARTESIAN_POINT ( 'NONE',  ( -19.03943276465977164, 0.05219959533909376836, 26.24890960531435624 ) ) ;
#4168=CARTESIAN_POINT ( 'NONE',  ( -18.67979575497178146, -10.72451020669898902, 61.66557627198103120 ) ) ;
#4169=CARTESIAN_POINT ( 'NONE',  ( -16.55341960407617563, 4.379528057220093196, 88.54275706135236135 ) ) ;
#4170=CARTESIAN_POINT ( 'NONE',  ( -21.55341960407619339, 5.719274019375674811, 43.54275706135235424 ) ) ;
#4171=CARTESIAN_POINT ( 'NONE',  ( -16.51473224551082808, 9.474510206698731452, 108.3344237280190043 ) ) ;
#4172=CARTESIAN_POINT ( 'NONE',  ( 12.06949235617757843, -12.14591786802309237, 103.1239096053143811 ) ) ;
#4173=CARTESIAN_POINT ( 'NONE',  ( 0.05219959533936267826, -19.03943276465977164, 110.0010903946856757 ) ) ;
#4174=CARTESIAN_POINT ( 'NONE',  ( 16.46253265017160672, -9.564922557960803928, 38.33224293864768839 ) ) ;
#4176=CARTESIAN_POINT ( 'NONE',  ( -19.05341960407611168, -5.049401038298163336, 91.45724293864766707 ) ) ;
#4177=CARTESIAN_POINT ( 'NONE',  ( 12.06949235617739724, 12.14591786802326823, 71.87609039468568994 ) ) ;
#4178=CARTESIAN_POINT ( 'NONE',  ( 15.72974639402176855, 15.80617190586768217, 101.8760903946857042 ) ) ;
#4179=CARTESIAN_POINT ( 'NONE',  ( 18.62759615963271287, -10.81492255796078972, 58.33224293864768839 ) ) ;
#4180=CARTESIAN_POINT ( 'NONE',  ( 14.29746914071037800, 8.314922557961029526, 91.66775706135234714 ) ) ;
#4181=CARTESIAN_POINT ( 'NONE',  ( -19.02544592524334988, -5.153800228976617603, 78.95942372801900433 ) ) ;
#4182=CARTESIAN_POINT ( 'NONE',  ( -19.02544592524342804, 5.153800228976336051, 31.04057627198102409 ) ) ;
#4183=CARTESIAN_POINT ( 'NONE',  ( 19.05341960407611168, 5.049401038298154454, 83.95724293864766707 ) ) ;
#4184=CARTESIAN_POINT ( 'NONE',  ( 13.89961937509977652, -13.97604488694527269, 28.12390960531435624 ) ) ;
#4185=CARTESIAN_POINT ( 'NONE',  ( -13.97604488694547697, 13.89961937509957934, 68.12609039468563310 ) ) ;
#4187=CARTESIAN_POINT ( 'NONE',  ( 9.564922557960805705, 16.46253265017160317, 94.58224293864769550 ) ) ;
#4188=CARTESIAN_POINT ( 'NONE',  ( -0.05219959533910754901, -16.53943276465976808, 47.49890960531435979 ) ) ;
#4189=CARTESIAN_POINT ( 'NONE',  ( -18.67979575497178146, -10.72451020669898902, 56.66557627198103830 ) ) ;
#4190=CARTESIAN_POINT ( 'NONE',  ( 17.50000000000000000, -5.499999999999992895, 91.21769037696437010 ) ) ;
#4191=( BOUNDED_SURFACE ( )  B_SPLINE_SURFACE ( 3, 2, ( 
 ( #118549, #161040, #22534, #147888, #41708, #84181, #148883, #165051, #145861, #53870, #115544, #193388, #24548, #177232, #38704, #100361, #23536, #40700, #164059, #39690, #85182, #70038, #86198, #8363, #9374, #116538, #178226, #71039, #55862, #25558, #87202, #10374, #136678, #90175, #106333, #168993, #16328, #92148, #42703, #105350, #166048, #44680, #30497, #121504, #45669, #122496, #141, #135709, #138660, #77978, #15331, #76989, #75997, #153834, #14332, #107320, #119544, #137671, #198360, #27548, #59835, #61810, #197380, #89189, #123480, #12375, #168019, #152838, #75013, #199357, #60822, #184187, #28539, #196402, #74038, #46663, #185172, #170002, #29515, #108322, #91149, #57872, #31493, #151858, #181227, #93146, #183198, #154830, #104364, #150881, #58845, #13349, #120512, #182204, #43688, #167037, #65792, #173991, #79978, #18321, #110311, #95139, #141646, #188170, #80959, #125491, #66787, #51622, #98097, #50639, #3136, #112301, #157821, #156828, #19311, #49643, #35460, #111306, #189167, #34473, #96132, #36442, #190147, #126472, #97111, #142635, #4113, #47666, #158794, #1133, #109318, #127461, #128451, #62807, #20283, #5106, #32490, #159795, #94143, #64811, #172995, #186185, #155822, #139645, #113287, #81929, #143621, #174978, #21290, #124489, #170998, #17319, #78974, #140649, #2139, #63818, #187188, #48659, #171993, #33481, #23295, #176991, #193145, #55620, #103130, #178988, #129446, #192141, #52619, #131458, #117293, #8112, #132465, #9131, #86957, #22293, #25315, #164811, #102129, #163813, #162796, #40455, #101110, #148641, #41465, #82947, #24305, #191145, #70797, #179998, #53622, #177982, #39449, #144625, #133461, #69790, #10131, #85954, #147642, #114281, #71792, #6108, #175984, #194156, #195151, #67789, #56632, #118306, #37452, #99113, #160805, #161800, #54617, #83944, #145624, #7103, #68785, #130442, #115298, #116292, #38461, #100117, #84939, #146620, #121267, #104125, #28305, #45431, #138427, #149634, #165807, #44444, #166805, #120276, #136445, #199113, #46420, #122256, #72807, #135475, #196162, #74783, #60580, #151626, #75756, #152599, #30259, #27304, #168756, #108078, #107084, #91902, #106098, #183946, #167784, #137433, #200107, #61575, #26306, #59593, #90914, #76752, #14090, #57636, #182961, #153594, #29283, #87946, #42461, #15092, #197143, #105119, #13119, #88951, #11132, #123244, #134477, #184935, #119302, #181968, #180985, #150642, #12138, #73802, #58610, #43451, #89945, #198126, #127220, #92907, #157583, #34238, #78736, #80724, #139413, #3881, #33249, #124247, #77747, #81696, #1901, #126242, #31257, #896, #169762, #143379, #51391, #35227, #63581, #185942, #142402, #64577, #47427, #171760, #188933, #4871, #154593, #109083, #187937, #110080, #125255, #79741, #65560, #189916, #50411, #16089, #140412, #62570, #18086, #112071, #94907, #19076, #95900, #173759, #170762, #96880, #32251, #158564, #20053, #49406, #66555, #111069, #128219, #93909, #155587, #17082, #2898, #186954, #48424, #156591, #141410, #172758, #132223, #131218, #174744, #129206, #147400, #83705, #191895, #38223, #114037, #113052, #193916, #194908, #117049, #86712, #6865, #177747, #55379, #71552, #148397, #24059, #101887, #36207, #178744, #70556, #97861, #100872, #39216, #22054, #85714, #82702, #8888, #176749, #67548, #21048, #25069, #145383, #69554, #159551, #144386, #5872, #9891, #190904, #40208, #68544, #52380, #163569, #133217, #175735, #37213, #54386, #98869, #162554, #160565, #130200, #7868, #192909, #53379, #115057, #99878, #161562, #116059, #23055, #84700, #146380, #118065, #26065, #151397, #45205, #179755, #152375, #122029, #149394, #153360, #10889, #135241, #166571, #102886, #72562, #56383, #183719, #121030, #182728, #43215, #76523, #73568, #28071, #14862, #74550, #196913, #150409, #89712, #29052, #138200, #13860, #164571, #165569, #87708, #104883, #90692, #181734, #105871, #44212, #60356, #195922, #198888 ),
 ( #167558, #134237, #12887, #75527, #136217, #41225, #57398, #137202, #27068, #58380, #197892, #119070, #180752, #106859, #42228, #168533, #30031, #11904, #91669, #103889, #88714, #120047, #59361, #188691, #199882, #18843, #157348, #123017, #187705, #64341, #108848, #110835, #169524, #34004, #63343, #154362, #107840, #111829, #32018, #156348, #61346, #31024, #184702, #173517, #81461, #65324, #93676, #15856, #172519, #80488, #158331, #46187, #141174, #92674, #49177, #96643, #170528, #94669, #17848, #19820, #50172, #186716, #95660, #2664, #126010, #77514, #142162, #139186, #661, #79505, #34989, #62331, #3646, #126984, #124001, #185699, #47188, #78499, #109841, #155359, #16848, #140172, #1665, #125020, #48186, #171526, #33014, #160327, #53138, #42737, #37987, #20807, #145146, #165084, #57905, #66318, #82463, #180272, #113803, #21817, #68308, #144149, #143147, #26578, #27584, #149905, #119577, #36971, #7630, #88221, #104399, #181260, #54154, #134753, #4628, #11412, #103406, #127979, #130980, #69314, #52146, #118582, #112815, #41742, #6629, #97622, #51154, #166081, #175498, #99643, #189682, #174508, #35975, #159312, #5634, #73082, #98632, #67311, #196435, #128970, #190670, #83469, #84465, #129959, #192671, #191659, #114817, #161326, #22819, #176509, #146143, #168051, #92183, #60854, #122529, #135742, #15365, #150916, #197413, #14365, #123512, #12409, #153867, #61843, #120545, #170036, #58879, #121537, #91181, #74071, #43723, #89222, #154864, #77021, #138693, #184220, #182238, #137706, #107352, #105384, #175, #183232, #45701, #93179, #167071, #90209, #44713, #185205, #169025, #199390, #30530, #31526, #28573, #151892, #198393, #46696, #106369, #108357, #13382, #75046, #136712, #59870, #29548, #152870, #76030, #63383, #60393, #168570, #33055, #154403, #153403, #44250, #702, #61385, #152410, #123057, #78539, #122065, #13898, #32060, #137240, #31066, #77555, #199922, #139227, #94710, #105907, #198925, #62374, #184743, #14901, #92714, #93716, #141216, #16888, #167593, #30068, #90727, #169569, #155398, #46228, #170569, #47231, #125060, #186757, #29088, #75564, #183757, #140214, #124044, #1707, #185743, #48227, #156388, #17892, #2706, #15897, #108890, #171566, #109882, #45243, #79546, #121072, #182766, #106897, #91709, #76563, #138238, #107882, #189726, #65367, #64383, #83511, #146186, #68350, #38030, #158375, #129014, #145188, #22861, #99686, #175541, #53185, #126051, #6672, #21861, #187748, #52187, #190714, #173563, #37016, #34047, #98677, #128024, #18885, #172561, #176555, #96687, #20854, #49218, #95704, #110876, #161370, #157392, #130001, #19864, #80531, #160370, #191701, #84508, #142205, #5678, #3688, #113845, #127027, #35032, #159356, #82510, #188734, #114860, #51199, #50219, #67354, #111873, #81504, #143192, #4672, #66364, #144192, #112860, #174551, #36018, #97667, #100682, #104693, #162364, #86524, #117873, #54197, #23865, #7671, #135051, #72366, #134040, #194720, #27877, #24875, #179563, #166381, #102699, #85516, #9702, #26876, #148208, #196727, #71366, #133030, #56190, #195733, #42039, #41033, #164387, #178550, #163378, #25880, #87525, #149212, #193722, #58195, #119863, #89518, #118881, #10703, #180565, #57206, #103703, #165383, #88519, #115869, #132033, #69355, #131024, #150215, #181548, #11712, #43027, #73379, #192713, #177558, #39027, #147204, #8695, #70365, #55190, #116859, #40016, #101689, #186518, #155159, #76324, #60162, #14663, #138001, #199685, #197702, #93472, #61150, #15659, #170329, #77318, #47992, #1461, #105679, #92479, #183525, #184512, #137006, #122822, #198696, #16651, #120837, #123803, #78298, #31822, #63139, #45992, #109646, #138986, #107647, #151208, #91474, #139972, #44018, #90503, #464, #121831, #182536, #124818, #32816, #74362, #171328, #152185, #45008, #12696, #169324, #106668, #136028, #30831, #153162, #167365, #154168, #108651, #13669, #28863, #62139, #75336, #185501 ),
 ( #168341, #46992, #59168, #29837, #129764, #5435, #83275, #94467, #113609, #51949, #17646, #2463, #175303, #156148, #64145, #189485, #144949, #79306, #190476, #160129, #187512, #191460, #48978, #173319, #4432, #140975, #110633, #125809, #21617, #159117, #20612, #81270, #114612, #111634, #66120, #52938, #50963, #172314, #96449, #36769, #6430, #33803, #95463, #112622, #34794, #188491, #127785, #67119, #176311, #98433, #157149, #3451, #18644, #142952, #128777, #19628, #143955, #82263, #68112, #80290, #141962, #65128, #126785, #49970, #174314, #158136, #35784, #97431, #11468, #149962, #57959, #71125, #102457, #88274, #164145, #7431, #132791, #56961, #55950, #99446, #53956, #72121, #8451, #116624, #163131, #38791, #37782, #118634, #119630, #41794, #73139, #131796, #25642, #180326, #196489, #134809, #148971, #26631, #161126, #103461, #195486, #22622, #87287, #10460, #146963, #133794, #69115, #165140, #101440, #192473, #145950, #84269, #70124, #194478, #130781, #115631, #177320, #100448, #162128, #23624, #193475, #85272, #54952, #178313, #39776, #24634, #179324, #86282, #147973, #9462, #117626, #40788, #137757, #78061, #31581, #168101, #15418, #184272, #45755, #153924, #1218, #77076, #27639, #90262, #150970, #29599, #138746, #106420, #30586, #107407, #185261, #46753, #166137, #89280, #12465, #228, #60909, #61896, #199441, #92238, #154916, #93231, #62895, #14417, #169080, #16414, #123566, #74125, #76081, #108412, #122585, #42792, #197467, #170087, #151945, #59922, #91230, #182296, #181313, #139729, #104454, #135796, #58933, #75098, #120602, #43776, #105440, #167125, #28625, #13434, #136765, #198451, #121590, #183285, #44767, #152921, #33566, #38298, #94228, #161638, #188255, #79062, #32575, #39293, #156914, #81044, #186272, #155909, #124576, #100950, #8969, #192986, #18411, #140735, #99952, #146455, #85793, #47751, #65878, #171084, #115134, #24141, #95228, #19395, #142720, #147479, #177823, #111397, #23132, #127552, #189253, #17405, #7948, #109405, #2224, #4200, #116134, #63906, #84777, #54464, #125576, #187274, #48743, #3220, #34559, #110397, #172079, #80060, #162634, #53458, #176826, #173082, #141730, #64894, #96217, #126555, #69631, #49729, #157906, #131297, #182802, #193996, #148479, #88788, #10965, #164648, #180826, #178822, #89785, #150481, #28145, #11976, #120119, #44285, #105943, #90763, #103965, #135312, #121108, #196985, #40293, #165643, #151470, #73641, #132304, #86792, #104957, #41302, #149470, #196000, #71630, #70638, #12959, #152446, #74623, #167628, #26143, #58451, #136289, #29125, #55458, #181810, #59435, #117129, #197965, #101967, #163648, #43288, #166643, #179832, #25150, #9970, #133296, #134314, #194986, #56464, #118142, #102963, #27141, #87785, #72639, #57473, #119145, #42304, #79581, #46264, #30104, #125095, #33089, #172595, #95739, #155433, #60427, #1742, #110909, #184778, #108925, #170605, #34081, #64416, #738, #48264, #16923, #78576, #122101, #94745, #75599, #183791, #32095, #2739, #137278, #109918, #141250, #106931, #13932, #168604, #92750, #124080, #45278, #91744, #198960, #126085, #140250, #63420, #62410, #153439, #31102, #185781, #14937, #93752, #76597, #15932, #156425, #187781, #138273, #199956, #186793, #154438, #107919, #47268, #171601, #61421, #17926, #123092, #169604, #77591, #49251, #139262, #82547, #6706, #83545, #161403, #22895, #142239, #3724, #113879, #20889, #80564, #96721, #190748, #98712, #192747, #65401, #111909, #50253, #54230, #84541, #144229, #66398, #5713, #67390, #129047, #127062, #99719, #52222, #21895, #176589, #145224, #115901, #7706, #173597, #160406, #189762, #175576, #143226, #37053, #4708, #146218, #188769, #130036, #69389, #38063, #131058, #68384, #177591, #191735, #53217, #157425, #97703, #39058, #35066, #158409, #114895, #128060, #19898, #18919, #81539, #51234, #112895, #174589, #36054, #159394, #134075, #133063, #23899, #180597, #41068 ),
 ( #194753, #100716, #178585, #151238, #27909, #74393, #149244, #12727, #195765, #162396, #42071, #56225, #85552, #89552, #179596, #136058, #182568, #57239, #58225, #117907, #197733, #102731, #164420, #87557, #26908, #135082, #25913, #10735, #71399, #72399, #118913, #103735, #165415, #86557, #59199, #120868, #147238, #11744, #88551, #73411, #150250, #196758, #119894, #181579, #8730, #24910, #70399, #132067, #43057, #193756, #104723, #55224, #166415, #116893, #40049, #101725, #163414, #148241, #9735, #137037, #183556, #108684, #153193, #75367, #186551, #125842, #167398, #48023, #45042, #91506, #156181, #77352, #76359, #28894, #123835, #184543, #198728, #46023, #1494, #106700, #60194, #155193, #121864, #154201, #499, #122855, #62171, #185533, #170362, #138036, #44051, #168373, #94499, #171361, #17680, #92512, #79338, #139019, #105711, #47026, #199717, #90534, #32849, #107679, #141008, #152216, #31854, #63172, #61183, #2496, #169356, #30866, #15691, #93507, #78332, #16682, #140005, #14697, #124851, #109680, #64177, #13700, #29869, #114644, #99475, #145978, #98465, #66151, #160159, #5467, #142984, #67149, #97460, #33835, #111666, #187544, #7460, #128807, #176342, #143986, #37814, #21650, #190506, #50992, #110666, #126818, #20642, #51980, #22652, #172346, #141994, #80321, #84299, #191489, #112653, #96479, #174344, #35814, #159146, #95495, #129792, #82295, #113638, #6460, #175333, #69144, #161156, #3482, #36800, #19659, #83303, #173353, #144980, #34824, #52967, #157181, #68141, #49011, #18675, #65159, #188524, #50001, #158167, #81300, #4462, #127814, #189519, #70154, #164173, #72149, #166167, #115659, #85300, #23652, #27668, #134838, #55979, #39804, #194506, #117656, #179353, #177349, #73168, #40816, #195516, #149991, #56989, #89308, #181341, #146992, #133825, #163160, #25671, #116651, #102486, #178342, #196517, #100477, #103490, #57988, #11497, #42820, #87316, #151001, #118663, #149000, #130811, #71154, #119659, #8479, #131824, #180354, #101470, #162156, #104483, #12492, #53986, #192502, #193505, #24663, #38819, #10489, #86312, #54982, #41823, #132820, #148001, #165168, #88303, #9491, #26661, #185290, #90290, #184304, #30616, #152949, #92269, #153953, #258, #106451, #74154, #151974, #124606, #1247, #47781, #122614, #186301, #107437, #135825, #15449, #168130, #197495, #62926, #14448, #109433, #155938, #169109, #31611, #91258, #171115, #76111, #137788, #60939, #61927, #108441, #199472, #45785, #44796, #29626, #77107, #138777, #123596, #59952, #32605, #94258, #58962, #46782, #170117, #93261, #154947, #16443, #78092, #139761, #120630, #198480, #182327, #43806, #105469, #167155, #28655, #13462, #75126, #136794, #121619, #183314, #64922, #129560, #50760, #49758, #140763, #97225, #157933, #48772, #19424, #175093, #156941, #110427, #128570, #33594, #127582, #174109, #96245, #35579, #158912, #143746, #111426, #17434, #95258, #67907, #144741, #191259, #65909, #52734, #112417, #79090, #20403, #173112, #2252, #6228, #81071, #114401, #99235, #82051, #36562, #34588, #176102, #142750, #4230, #189282, #5225, #51742, #66907, #190265, #188284, #113403, #98217, #159920, #21409, #3249, #37572, #63934, #125603, #83066, #187301, #172108, #18438, #80089, #141757, #126582, #7225, #85063, #160922, #119425, #179115, #88069, #117417, #149755, #71912, #40583, #24428, #84065, #100239, #194276, #102253, #196286, #145744, #115423, #53749, #57755, #164936, #86076, #69918, #147767, #9253, #70920, #68910, #103254, #132587, #25438, #180122, #87079, #181109, #11258, #177112, #163941, #193268, #55743, #146745, #148764, #8240, #26429, #130570, #133584, #72931, #41590, #134600, #10253, #42583, #195274, #56757, #22415, #101231, #192267, #38583, #161921, #118429, #131584, #23415, #54742, #116414, #178104, #39572, #162919, #77865, #16210, #124371, #137555, #168876, #154717, #30381, #73922, #199238, #123364, #122379, #165929, #120395, #138543 ),
 ( #198245, #27426, #93029, #183082, #31379, #186066, #60703, #61695, #121390, #139532, #44565, #106220, #91034, #92026, #21, #167904, #29404, #74901, #59718, #152720, #14211, #45551, #90063, #1015, #62689, #104246, #15214, #75879, #76873, #184068, #107206, #153718, #185057, #150762, #28426, #89071, #12259, #46545, #135592, #108205, #197264, #169886, #58726, #182089, #43572, #105237, #166925, #151745, #13238, #136564, #2023, #140534, #82826, #51510, #172878, #156712, #111188, #34359, #96020, #94025, #190036, #157705, #112190, #66674, #173878, #144507, #97981, #63702, #189053, #79863, #80844, #33364, #19195, #95023, #113172, #17201, #20170, #174861, #128337, #159674, #142521, #5991, #35348, #4000, #47549, #188055, #36327, #125377, #187073, #96999, #18205, #78855, #21170, #129329, #170881, #67671, #49525, #64697, #65679, #158682, #81816, #127341, #126358, #141532, #3020, #50528, #143504, #4988, #109202, #32372, #155706, #48543, #110197, #171875, #163694, #9015, #146500, #70683, #100996, #37333, #115178, #191024, #149514, #132349, #118187, #147527, #179878, #102012, #194041, #54506, #114159, #130320, #24187, #55505, #26188, #175861, #145504, #83823, #87828, #195032, #116178, #99996, #177868, #39337, #162681, #98992, #133341, #85837, #117175, #10014, #178870, #11011, #41346, #6985, #40337, #23177, #25196, #176871, #86838, #38340, #56509, #160681, #148524, #103008, #71674, #164693, #72685, #52499, #22173, #68665, #192017, #131341, #53501, #161681, #84821, #7991, #69674, #193029, #79375, #18712, #57519, #141046, #73687, #181855, #49047, #170397, #166688, #119187, #16716, #74668, #165688, #136335, #94535, #135359, #27186, #48059, #150526, #44329, #93542, #13005, #155227, #78366, #63208, #28191, #134360, #12025, #187579, #64213, #110702, #182846, #172382, #31888, #196044, #140040, #89833, #180872, #125879, #198009, #33873, #42348, #1529, #156217, #151513, #95532, #2532, #17717, #157219, #124888, #104010, #186587, #109715, #88833, #59479, #197031, #58498, #120164, #171398, #43334, #105002, #121153, #108720, #32885, #22690, #19695, #127851, #192541, #113675, #112689, #3520, #160197, #20678, #111704, #82333, #37854, #81337, #173390, #191529, #96515, #190542, #36837, #159183, #98502, #21687, #6498, #174381, #80359, #158205, #130849, #7499, #54024, #128843, #115697, #175369, #142032, #83340, #35851, #65196, #69183, #144023, #177386, #162193, #145017, #99513, #97497, #38857, #5504, #67186, #52016, #68178, #114685, #129830, #53006, #51028, #176380, #161194, #84337, #146016, #66189, #100514, #126855, #188561, #50040, #34860, #143020, #4498, #189556, #103529, #133863, #70194, #148037, #23691, #182363, #41863, #151036, #180392, #12526, #134876, #165204, #87352, #147032, #163198, #57028, #26699, #58999, #8516, #178378, #116688, #120665, #27702, #149038, #132856, #10526, #72189, #195554, #131861, #166201, #118701, #88339, #42855, #150030, #43841, #74191, #39842, #11537, #56015, #73205, #9526, #196553, #71192, #89345, #193545, #58024, #119694, #181377, #85339, #164210, #135860, #101508, #24702, #104520, #194544, #55018, #197531, #105506, #86351, #117693, #179390, #40853, #102527, #25707, #199509, #90326, #46816, #107472, #198517, #169149, #124641, #106488, #59988, #78127, #183350, #77144, #123630, #45821, #185326, #108476, #93296, #60975, #167193, #44833, #17469, #94293, #140798, #15487, #79125, #295, #28690, #170154, #122651, #152011, #155972, #30653, #2287, #48806, #61963, #186336, #184339, #63969, #92307, #153990, #138814, #154982, #1284, #31647, #16477, #137826, #139795, #62960, #47818, #109467, #152986, #125639, #187336, #13497, #171151, #32639, #75162, #136834, #121656, #168166, #29663, #91295, #14485, #76147, #52764, #158944, #144775, #20433, #83099, #190296, #97256, #65943, #33628, #126614, #35611, #82084, #129592, #95290, #141790, #3284, #191288, #159951, #189314, #34620, #127614, #67939, #6259 ),
 ( #36593, #114433, #172141, #64955, #143777, #4263, #19457, #112450, #51773, #176134, #5258, #110460, #66941, #156974, #98249, #128603, #174139, #188316, #96279, #113433, #175126, #18471, #49794, #111460, #173145, #80121, #157965, #21439, #81104, #142782, #50791, #63630, #47475, #76803, #77793, #155637, #110129, #17132, #126286, #141461, #45480, #32303, #123293, #124295, #138474, #16138, #200155, #94954, #60632, #125306, #156638, #171807, #2945, #185992, #49453, #78784, #109132, #90963, #31304, #79788, #183997, #30310, #140461, #61625, #122306, #33295, #172804, #14140, #18134, #91953, #184985, #64624, #170810, #46469, #75807, #93958, #92957, #107136, #154643, #48472, #153646, #168806, #1951, #15141, #942, #187002, #169813, #187983, #111115, #152650, #108129, #137485, #139462, #199165, #62617, #7912, #82750, #146421, #67593, #34285, #114082, #128262, #95945, #23098, #113095, #161604, #116100, #129252, #191939, #51435, #84745, #174786, #36252, #21093, #160607, #68587, #97905, #159596, #4915, #189960, #144430, #5916, #175783, #20098, #69596, #131263, #192951, #145426, #190947, #6909, #52424, #37257, #98915, #22097, #80770, #158608, #157631, #83747, #66598, #130243, #53423, #115100, #176792, #81742, #54430, #19120, #142448, #38265, #99919, #3926, #65606, #127266, #188979, #50455, #112114, #143429, #173806, #35271, #96926, #104922, #134278, #166609, #88754, #195966, #41266, #100914, #117093, #10931, #119111, #12922, #162599, #132268, #70601, #74586, #181773, #102928, #86757, #164613, #135278, #150447, #57438, #163612, #26107, #42271, #196950, #103929, #136254, #28111, #193959, #180792, #9935, #72604, #25113, #87750, #148440, #43254, #147444, #11943, #89749, #58418, #151435, #165609, #197930, #27108, #73607, #177788, #118108, #59398, #55422, #178788, #120085, #71594, #8932, #39258, #24103, #85757, #40257, #101930, #133260, #194951, #56428, #179797, #149435, #40567, #149740, #72916, #104231, #90048, #165912, #9237, #134585, #58710, #57740, #101214, #55727, #73907, #10236, #118413, #164919, #102237, #39557, #120380, #121373, #43556, #13223, #133567, #27410, #182073, #198229, #74886, #150747, #28411, #162903, #105222, #197249, #24412, #89056, #12245, #148748, #135577, #70904, #166910, #103237, #194260, #147750, #86061, #151730, #180106, #136548, #132571, #196271, #59701, #56742, #117400, #41574, #26413, #88052, #179098, #163925, #11241, #119410, #71896, #195258, #181093, #42568, #25421, #87063, #110181, #95007, #141515, #94009, #61678, #155690, #998, #138526, #62672, #93012, #29387, #107188, #183066, #3001, #124353, #171860, #139515, #33348, #17185, #186048, #46527, #106204, #122362, #16193, #47531, #18189, #167888, #137539, #75863, #79846, #187057, #108187, #92007, #169868, #140517, #78839, #109186, #168859, #31362, #170865, #2007, #32356, #64678, #156695, #199221, #63686, #15196, #77848, #30364, #154698, #153701, #48527, #152704, #125360, #44549, #91018, #14193, #60687, #184051, #45534, #76855, #4, #123347, #185040, #19177, #65661, #191006, #35329, #157686, #68647, #7973, #49507, #130303, #127323, #173861, #38323, #159656, #158663, #52482, #6967, #20154, #114141, #128320, #83807, #189035, #80825, #37316, #142503, #36309, #82808, #4971, #144490, #5973, #175842, #81799, #126340, #3981, #176854, #53483, #99979, #174844, #161664, #21153, #188037, #67653, #143486, #23160, #129310, #50510, #190019, #145487, #84803, #111170, #112173, #98974, #66657, #51493, #97964, #160664, #146482, #22156, #172860, #96982, #96002, #191997, #115161, #113154, #34341, #196027, #73669, #135341, #54489, #116161, #177851, #88817, #149498, #27170, #87812, #147507, #39320, #70665, #179860, #102990, #134344, #120147, #57502, #100979, #164676, #150510, #10995, #131323, #85820, #103992, #40318, #148507, #195015, #132332, #69656, #12008, #151497, #197015, #43318, #163676, #119171, #58480, #28174, #104985, #180855, #181838, #193012 ),
 ( #101994, #25178, #71657, #118169, #72667, #55486, #166672, #89816, #162663, #42331, #9997, #165671, #24169, #86820, #8997, #41330, #194023, #117156, #178852, #133324, #56491, #26171, #169634, #140279, #124111, #31130, #76624, #136318, #152474, #46291, #154468, #48292, #197993, #167657, #105972, #109948, #16951, #138302, #122130, #199983, #170634, #185811, #92779, #198987, #61450, #77620, #32123, #139290, #171629, #63449, #29153, #123120, #767, #93780, #62437, #33117, #125125, #90790, #15960, #45307, #107948, #60455, #184805, #183817, #78605, #182831, #47297, #1771, #155461, #186822, #108954, #94774, #12989, #74652, #59464, #153467, #121137, #13960, #75627, #44313, #106957, #137306, #168631, #30131, #91773, #14964, #95767, #3750, #68411, #189789, #188797, #20915, #37080, #50280, #144254, #158436, #113905, #157453, #49278, #67417, #172622, #66424, #112920, #35094, #174615, #36080, #82573, #111937, #156456, #34110, #6733, #83573, #130064, #4735, #191763, #51260, #17955, #97729, #173624, #79608, #145252, #96746, #53246, #38092, #159419, #175603, #19923, #114924, #81565, #143251, #128085, #5741, #190773, #129072, #52248, #127088, #98739, #160432, #21922, #176617, #142267, #141278, #2767, #64443, #126114, #187809, #110936, #18947, #80592, #65427, #9760, #146247, #23925, #99747, #58252, #117934, #26936, #56252, #88578, #10762, #179623, #163441, #22923, #39087, #133088, #41095, #135108, #84569, #54258, #192774, #196784, #103762, #24938, #8756, #86584, #57266, #72426, #102759, #85580, #161431, #164446, #193782, #7733, #150276, #178612, #11772, #181606, #194778, #118940, #116919, #73437, #40075, #101753, #148268, #25940, #134104, #71424, #87583, #70427, #55251, #149270, #195794, #180625, #147266, #119920, #69419, #131085, #42097, #165441, #115929, #177619, #100743, #162424, #132093, #92288, #170134, #43084, #4245, #63951, #173128, #2268, #34603, #156956, #125620, #109449, #169130, #185307, #79106, #187318, #81087, #30635, #276, #138795, #142765, #49776, #171132, #154963, #32621, #3265, #18453, #48789, #31628, #94275, #110443, #64938, #172124, #65925, #96262, #61945, #33610, #78108, #140779, #93278, #155953, #16459, #111441, #15469, #80104, #157948, #126597, #19439, #95273, #127598, #141772, #188299, #104751, #186317, #153972, #123612, #46798, #77126, #139777, #108457, #1265, #62942, #124622, #47799, #17450, #36576, #101246, #22428, #21421, #53762, #69934, #83081, #177127, #191271, #146760, #128585, #82067, #100254, #5241, #99249, #145757, #67921, #7239, #68924, #115436, #144757, #189297, #66921, #39587, #116431, #162935, #37587, #24442, #84078, #175107, #193283, #158928, #161935, #54757, #8254, #86091, #130586, #147782, #38598, #192281, #50774, #129574, #178119, #143760, #190279, #23430, #98231, #20417, #131598, #70934, #112434, #9268, #51755, #159934, #174123, #85077, #6242, #35594, #97240, #52746, #113416, #114415, #176116, #160936, #25454, #43587, #148779, #42598, #89086, #11272, #150778, #12273, #58741, #164949, #132601, #10268, #183098, #59735, #106235, #181124, #44579, #165944, #194291, #73938, #26442, #55757, #121404, #72945, #167918, #14226, #27444, #90077, #149770, #29418, #134615, #196299, #119439, #120410, #166939, #57769, #104261, #103269, #88084, #135607, #197278, #182102, #118442, #91049, #152736, #117431, #105253, #28442, #151760, #13253, #74916, #136579, #198259, #179129, #56770, #40597, #102268, #163956, #87094, #71927, #133597, #195289, #180135, #41604, #199254, #15229, #109217, #17218, #111205, #60721, #30397, #168892, #172897, #79879, #1032, #185072, #139547, #33381, #48560, #32388, #61710, #62704, #140550, #95039, #2038, #34376, #126375, #92044, #78870, #108222, #170896, #123380, #124387, #96036, #46560, #94043, #155721, #157723, #188072, #186082, #110213, #63718, #125393, #184084, #156730, #137571, #45568, #187090, #64713, #122395, #171894, #141548, #153733, #75896, #76888 ) ),
 .UNSPECIFIED., .T., .F., .F. ) 
 B_SPLINE_SURFACE_WITH_KNOTS ( ( 4, 3, 4 ),
 ( 3, 2, 2, 2, 2, 2, 2, 2, 2, 2, 2, 2, 2, 2, 2, 2, 2, 2, 2, 2, 2, 2, 2, 2, 2, 2, 2, 2, 2, 2, 2, 2, 2, 2, 2, 2, 2, 2, 2, 2, 2, 2, 2, 2, 2, 2, 2, 2, 2, 2, 2, 2, 2, 2, 2, 2, 2, 2, 2, 2, 2, 2, 2, 2, 2, 2, 2, 2, 2, 2, 2, 2, 2, 2, 2, 2, 2, 2, 2, 2, 2, 2, 2, 2, 2, 2, 2, 2, 2, 2, 2, 2, 2, 2, 2, 2, 2, 2, 2, 2, 2, 2, 2, 2, 2, 2, 2, 2, 2, 2, 2, 2, 2, 2, 2, 2, 2, 2, 2, 2, 2, 2, 2, 2, 2, 2, 2, 2, 2, 2, 2, 2, 2, 2, 2, 2, 2, 2, 2, 2, 2, 2, 2, 2, 2, 2, 2, 2, 2, 2, 2, 2, 2, 2, 2, 2, 2, 2, 2, 2, 2, 2, 2, 2, 2, 2, 2, 2, 2, 2, 2, 2, 2, 2, 2, 2, 2, 2, 2, 2, 2, 2, 2, 2, 2, 2, 2, 2, 2, 2, 2, 2, 2, 2, 2, 2, 2, 2, 2, 2, 2, 2, 2, 2, 2, 2, 2, 2, 2, 2, 2, 2, 2, 2, 2, 2, 2, 2, 2, 2, 2, 2, 2, 2, 2, 2, 2, 2, 3 ),
 ( 0.000000000000000000, 0.5000000000000000000, 1.000000000000000000 ),
 ( 0.000000000000000000, 0.004385964912280701511, 0.008771929824561403022, 0.01315789473684210453, 0.01754385964912280604, 0.02192982456140350755, 0.02631578947368420907, 0.03070175438596491058, 0.03508771929824561209, 0.03947368421052631360, 0.04385964912280701511, 0.04824561403508771662, 0.05263157894736841813, 0.05701754385964911964, 0.06140350877192982115, 0.06578947368421052266, 0.07017543859649122417, 0.07456140350877192569, 0.07894736842105262720, 0.08333333333333332871, 0.08771929824561403022, 0.09210526315789473173, 0.09649122807017543324, 0.1008771929824561348, 0.1052631578947368363, 0.1096491228070175378, 0.1140350877192982393, 0.1184210526315789408, 0.1228070175438596423, 0.1271929824561403577, 0.1315789473684210453, 0.1359649122807017607, 0.1403508771929824483, 0.1447368421052631637, 0.1491228070175438514, 0.1535087719298245668, 0.1578947368421052544, 0.1622807017543859698, 0.1666666666666666574, 0.1710526315789473728, 0.1754385964912280604, 0.1798245614035087758, 0.1842105263157894635, 0.1885964912280701788, 0.1929824561403508665, 0.1973684210526315819, 0.2017543859649122695, 0.2061403508771929849, 0.2105263157894736725, 0.2149122807017543879, 0.2192982456140350755, 0.2236842105263157909, 0.2280701754385964786, 0.2324561403508771940, 0.2368421052631578816, 0.2412280701754385970, 0.2456140350877192846, 0.2500000000000000000, 0.2543859649122807154, 0.2587719298245614308, 0.2631578947368420907, 0.2675438596491228060, 0.2719298245614035214, 0.2763157894736842368, 0.2807017543859648967, 0.2850877192982456121, 0.2894736842105263275, 0.2938596491228070429, 0.2982456140350877027, 0.3026315789473684181, 0.3070175438596491335, 0.3114035087719298489, 0.3157894736842105088, 0.3201754385964912242, 0.3245614035087719396, 0.3289473684210526550, 0.3333333333333333148, 0.3377192982456140302, 0.3421052631578947456, 0.3464912280701754610, 0.3508771929824561209, 0.3552631578947368363, 0.3596491228070175517, 0.3640350877192982670, 0.3684210526315789269, 0.3728070175438596423, 0.3771929824561403577, 0.3815789473684210731, 0.3859649122807017330, 0.3903508771929824483, 0.3947368421052631637, 0.3991228070175438791, 0.4035087719298245390, 0.4078947368421052544, 0.4122807017543859698, 0.4166666666666666852, 0.4210526315789473450, 0.4254385964912280604, 0.4298245614035087758, 0.4342105263157894912, 0.4385964912280701511, 0.4429824561403508665, 0.4473684210526315819, 0.4517543859649122973, 0.4561403508771929571, 0.4605263157894736725, 0.4649122807017543879, 0.4692982456140351033, 0.4736842105263157632, 0.4780701754385964786, 0.4824561403508771940, 0.4868421052631579093, 0.4912280701754385692, 0.4956140350877192846, 0.5000000000000000000, 0.5043859649122807154, 0.5087719298245614308, 0.5131578947368421462, 0.5175438596491228616, 0.5219298245614034659, 0.5263157894736841813, 0.5307017543859648967, 0.5350877192982456121, 0.5394736842105263275, 0.5438596491228070429, 0.5482456140350877583, 0.5526315789473684736, 0.5570175438596490780, 0.5614035087719297934, 0.5657894736842105088, 0.5701754385964912242, 0.5745614035087719396, 0.5789473684210526550, 0.5833333333333333703, 0.5877192982456140857, 0.5921052631578946901, 0.5964912280701754055, 0.6008771929824561209, 0.6052631578947368363, 0.6096491228070175517, 0.6140350877192982670, 0.6184210526315789824, 0.6228070175438596978, 0.6271929824561403022, 0.6315789473684210176, 0.6359649122807017330, 0.6403508771929824483, 0.6447368421052631637, 0.6491228070175438791, 0.6535087719298245945, 0.6578947368421053099, 0.6622807017543859143, 0.6666666666666666297, 0.6710526315789473450, 0.6754385964912280604, 0.6798245614035087758, 0.6842105263157894912, 0.6885964912280702066, 0.6929824561403509220, 0.6973684210526315264, 0.7017543859649122417, 0.7061403508771929571, 0.7105263157894736725, 0.7149122807017543879, 0.7192982456140351033, 0.7236842105263158187, 0.7280701754385965341, 0.7324561403508771384, 0.7368421052631578538, 0.7412280701754385692, 0.7456140350877192846, 0.7500000000000000000, 0.7543859649122807154, 0.7587719298245614308, 0.7631578947368421462, 0.7675438596491228616, 0.7719298245614034659, 0.7763157894736841813, 0.7807017543859648967, 0.7850877192982456121, 0.7894736842105263275, 0.7938596491228070429, 0.7982456140350877583, 0.8026315789473684736, 0.8070175438596490780, 0.8114035087719297934, 0.8157894736842105088, 0.8201754385964912242, 0.8245614035087719396, 0.8289473684210526550, 0.8333333333333333703, 0.8377192982456140857, 0.8421052631578946901, 0.8464912280701754055, 0.8508771929824561209, 0.8552631578947368363, 0.8596491228070175517, 0.8640350877192982670, 0.8684210526315789824, 0.8728070175438596978, 0.8771929824561403022, 0.8815789473684210176, 0.8859649122807017330, 0.8903508771929824483, 0.8947368421052631637, 0.8991228070175438791, 0.9035087719298245945, 0.9078947368421053099, 0.9122807017543859143, 0.9166666666666666297, 0.9210526315789473450, 0.9254385964912280604, 0.9298245614035087758, 0.9342105263157894912, 0.9385964912280702066, 0.9429824561403509220, 0.9473684210526315264, 0.9517543859649122417, 0.9561403508771929571, 0.9605263157894736725, 0.9649122807017543879, 0.9692982456140351033, 0.9736842105263158187, 0.9780701754385965341, 0.9824561403508771384, 0.9868421052631578538, 0.9912280701754385692, 0.9956140350877192846, 1.000000000000000000 ),
 .UNSPECIFIED. ) 
 GEOMETRIC_REPRESENTATION_ITEM ( )  RATIONAL_B_SPLINE_SURFACE ( (
 ( 1.000000000000000000, 0.9659258262890683122, 1.000000000000000000, 0.9659258262890683122, 1.000000000000000000, 0.9659258262890683122, 1.000000000000000000, 0.9659258262890683122, 1.000000000000000000, 0.9659258262890683122, 1.000000000000000000, 0.9659258262890683122, 1.000000000000000000, 0.9659258262890683122, 1.000000000000000000, 0.9659258262890683122, 1.000000000000000000, 0.9659258262890683122, 1.000000000000000000, 0.9659258262890683122, 1.000000000000000000, 0.9659258262890683122, 1.000000000000000000, 0.9659258262890683122, 1.000000000000000000, 0.9659258262890683122, 1.000000000000000000, 0.9659258262890683122, 1.000000000000000000, 0.9659258262890683122, 1.000000000000000000, 0.9659258262890683122, 1.000000000000000000, 0.9659258262890683122, 1.000000000000000000, 0.9659258262890683122, 1.000000000000000000, 0.9659258262890683122, 1.000000000000000000, 0.9659258262890683122, 1.000000000000000000, 0.9659258262890683122, 1.000000000000000000, 0.9659258262890683122, 1.000000000000000000, 0.9659258262890683122, 1.000000000000000000, 0.9659258262890683122, 1.000000000000000000, 0.9659258262890683122, 1.000000000000000000, 0.9659258262890683122, 1.000000000000000000, 0.9659258262890683122, 1.000000000000000000, 0.9659258262890683122, 1.000000000000000000, 0.9659258262890683122, 1.000000000000000000, 0.9659258262890683122, 1.000000000000000000, 0.9659258262890683122, 1.000000000000000000, 0.9659258262890683122, 1.000000000000000000, 0.9659258262890683122, 1.000000000000000000, 0.9659258262890683122, 1.000000000000000000, 0.9659258262890683122, 1.000000000000000000, 0.9659258262890683122, 1.000000000000000000, 0.9659258262890683122, 1.000000000000000000, 0.9659258262890683122, 1.000000000000000000, 0.9659258262890683122, 1.000000000000000000, 0.9659258262890683122, 1.000000000000000000, 0.9659258262890683122, 1.000000000000000000, 0.9659258262890683122, 1.000000000000000000, 0.9659258262890683122, 1.000000000000000000, 0.9659258262890683122, 1.000000000000000000, 0.9659258262890683122, 1.000000000000000000, 0.9659258262890683122, 1.000000000000000000, 0.9659258262890683122, 1.000000000000000000, 0.9659258262890683122, 1.000000000000000000, 0.9659258262890683122, 1.000000000000000000, 0.9659258262890683122, 1.000000000000000000, 0.9659258262890683122, 1.000000000000000000, 0.9659258262890683122, 1.000000000000000000, 0.9659258262890683122, 1.000000000000000000, 0.9659258262890683122, 1.000000000000000000, 0.9659258262890683122, 1.000000000000000000, 0.9659258262890683122, 1.000000000000000000, 0.9659258262890683122, 1.000000000000000000, 0.9659258262890683122, 1.000000000000000000, 0.9659258262890683122, 1.000000000000000000, 0.9659258262890683122, 1.000000000000000000, 0.9659258262890683122, 1.000000000000000000, 0.9659258262890683122, 1.000000000000000000, 0.9659258262890683122, 1.000000000000000000, 0.9659258262890683122, 1.000000000000000000, 0.9659258262890683122, 1.000000000000000000, 0.9659258262890683122, 1.000000000000000000, 0.9659258262890683122, 1.000000000000000000, 0.9659258262890683122, 1.000000000000000000, 0.9659258262890683122, 1.000000000000000000, 0.9659258262890683122, 1.000000000000000000, 0.9659258262890683122, 1.000000000000000000, 0.9659258262890683122, 1.000000000000000000, 0.9659258262890683122, 1.000000000000000000, 0.9659258262890683122, 1.000000000000000000, 0.9659258262890683122, 1.000000000000000000, 0.9659258262890683122, 1.000000000000000000, 0.9659258262890683122, 1.000000000000000000, 0.9659258262890683122, 1.000000000000000000, 0.9659258262890683122, 1.000000000000000000, 0.9659258262890683122, 1.000000000000000000, 0.9659258262890683122, 1.000000000000000000, 0.9659258262890683122, 1.000000000000000000, 0.9659258262890683122, 1.000000000000000000, 0.9659258262890683122, 1.000000000000000000, 0.9659258262890683122, 1.000000000000000000, 0.9659258262890683122, 1.000000000000000000, 0.9659258262890683122, 1.000000000000000000, 0.9659258262890683122, 1.000000000000000000, 0.9659258262890683122, 1.000000000000000000, 0.9659258262890683122, 1.000000000000000000, 0.9659258262890683122, 1.000000000000000000, 0.9659258262890683122, 1.000000000000000000, 0.9659258262890683122, 1.000000000000000000, 0.9659258262890683122, 1.000000000000000000, 0.9659258262890683122, 1.000000000000000000, 0.9659258262890683122, 1.000000000000000000, 0.9659258262890683122, 1.000000000000000000, 0.9659258262890683122, 1.000000000000000000, 0.9659258262890683122, 1.000000000000000000, 0.9659258262890683122, 1.000000000000000000, 0.9659258262890683122, 1.000000000000000000, 0.9659258262890683122, 1.000000000000000000, 0.9659258262890683122, 1.000000000000000000, 0.9659258262890683122, 1.000000000000000000, 0.9659258262890683122, 1.000000000000000000, 0.9659258262890683122, 1.000000000000000000, 0.9659258262890683122, 1.000000000000000000, 0.9659258262890683122, 1.000000000000000000, 0.9659258262890683122, 1.000000000000000000, 0.9659258262890683122, 1.000000000000000000, 0.9659258262890683122, 1.000000000000000000, 0.9659258262890683122, 1.000000000000000000, 0.9659258262890683122, 1.000000000000000000, 0.9659258262890683122, 1.000000000000000000, 0.9659258262890683122, 1.000000000000000000, 0.9659258262890683122, 1.000000000000000000, 0.9659258262890683122, 1.000000000000000000, 0.9659258262890683122, 1.000000000000000000, 0.9659258262890683122, 1.000000000000000000, 0.9659258262890683122, 1.000000000000000000, 0.9659258262890683122, 1.000000000000000000, 0.9659258262890683122, 1.000000000000000000, 0.9659258262890683122, 1.000000000000000000, 0.9659258262890683122, 1.000000000000000000, 0.9659258262890683122, 1.000000000000000000, 0.9659258262890683122, 1.000000000000000000, 0.9659258262890683122, 1.000000000000000000, 0.9659258262890683122, 1.000000000000000000, 0.9659258262890683122, 1.000000000000000000, 0.9659258262890683122, 1.000000000000000000, 0.9659258262890683122, 1.000000000000000000, 0.9659258262890683122, 1.000000000000000000, 0.9659258262890683122, 1.000000000000000000, 0.9659258262890683122, 1.000000000000000000, 0.9659258262890683122, 1.000000000000000000, 0.9659258262890683122, 1.000000000000000000, 0.9659258262890683122, 1.000000000000000000, 0.9659258262890683122, 1.000000000000000000, 0.9659258262890683122, 1.000000000000000000, 0.9659258262890683122, 1.000000000000000000, 0.9659258262890683122, 1.000000000000000000, 0.9659258262890683122, 1.000000000000000000, 0.9659258262890683122, 1.000000000000000000, 0.9659258262890683122, 1.000000000000000000, 0.9659258262890683122, 1.000000000000000000, 0.9659258262890683122, 1.000000000000000000, 0.9659258262890683122, 1.000000000000000000, 0.9659258262890683122, 1.000000000000000000, 0.9659258262890683122, 1.000000000000000000, 0.9659258262890683122, 1.000000000000000000, 0.9659258262890683122, 1.000000000000000000, 0.9659258262890683122, 1.000000000000000000, 0.9659258262890683122, 1.000000000000000000, 0.9659258262890683122, 1.000000000000000000, 0.9659258262890683122, 1.000000000000000000, 0.9659258262890683122, 1.000000000000000000, 0.9659258262890683122, 1.000000000000000000, 0.9659258262890683122, 1.000000000000000000, 0.9659258262890683122, 1.000000000000000000, 0.9659258262890683122, 1.000000000000000000, 0.9659258262890683122, 1.000000000000000000, 0.9659258262890683122, 1.000000000000000000, 0.9659258262890683122, 1.000000000000000000, 0.9659258262890683122, 1.000000000000000000, 0.9659258262890683122, 1.000000000000000000, 0.9659258262890683122, 1.000000000000000000, 0.9659258262890683122, 1.000000000000000000, 0.9659258262890683122, 1.000000000000000000, 0.9659258262890683122, 1.000000000000000000, 0.9659258262890683122, 1.000000000000000000, 0.9659258262890683122, 1.000000000000000000, 0.9659258262890683122, 1.000000000000000000, 0.9659258262890683122, 1.000000000000000000, 0.9659258262890683122, 1.000000000000000000, 0.9659258262890683122, 1.000000000000000000, 0.9659258262890683122, 1.000000000000000000, 0.9659258262890683122, 1.000000000000000000, 0.9659258262890683122, 1.000000000000000000, 0.9659258262890683122, 1.000000000000000000, 0.9659258262890683122, 1.000000000000000000, 0.9659258262890683122, 1.000000000000000000, 0.9659258262890683122, 1.000000000000000000, 0.9659258262890683122, 1.000000000000000000, 0.9659258262890683122, 1.000000000000000000, 0.9659258262890683122, 1.000000000000000000, 0.9659258262890683122, 1.000000000000000000, 0.9659258262890683122, 1.000000000000000000, 0.9659258262890683122, 1.000000000000000000, 0.9659258262890683122, 1.000000000000000000, 0.9659258262890683122, 1.000000000000000000, 0.9659258262890683122, 1.000000000000000000, 0.9659258262890683122, 1.000000000000000000, 0.9659258262890683122, 1.000000000000000000, 0.9659258262890683122, 1.000000000000000000, 0.9659258262890683122, 1.000000000000000000, 0.9659258262890683122, 1.000000000000000000, 0.9659258262890683122, 1.000000000000000000, 0.9659258262890683122, 1.000000000000000000, 0.9659258262890683122, 1.000000000000000000, 0.9659258262890683122, 1.000000000000000000, 0.9659258262890683122, 1.000000000000000000, 0.9659258262890683122, 1.000000000000000000, 0.9659258262890683122, 1.000000000000000000, 0.9659258262890683122, 1.000000000000000000, 0.9659258262890683122, 1.000000000000000000, 0.9659258262890683122, 1.000000000000000000, 0.9659258262890683122, 1.000000000000000000, 0.9659258262890683122, 1.000000000000000000, 0.9659258262890683122, 1.000000000000000000, 0.9659258262890683122, 1.000000000000000000, 0.9659258262890683122, 1.000000000000000000, 0.9659258262890683122, 1.000000000000000000, 0.9659258262890683122, 1.000000000000000000, 0.9659258262890683122, 1.000000000000000000, 0.9659258262890683122, 1.000000000000000000, 0.9659258262890683122, 1.000000000000000000, 0.9659258262890683122, 1.000000000000000000, 0.9659258262890683122, 1.000000000000000000, 0.9659258262890683122, 1.000000000000000000, 0.9659258262890683122, 1.000000000000000000, 0.9659258262890683122, 1.000000000000000000, 0.9659258262890683122, 1.000000000000000000, 0.9659258262890683122, 1.000000000000000000, 0.9659258262890683122, 1.000000000000000000, 0.9659258262890683122, 1.000000000000000000, 0.9659258262890683122, 1.000000000000000000, 0.9659258262890683122, 1.000000000000000000, 0.9659258262890683122, 1.000000000000000000),
 ( 0.3333333333333333703, 0.3219752754296894559, 0.3333333333333333703, 0.3219752754296894559, 0.3333333333333333703, 0.3219752754296894559, 0.3333333333333333703, 0.3219752754296894559, 0.3333333333333333703, 0.3219752754296894559, 0.3333333333333333703, 0.3219752754296894559, 0.3333333333333333703, 0.3219752754296894559, 0.3333333333333333703, 0.3219752754296894559, 0.3333333333333333703, 0.3219752754296894559, 0.3333333333333333703, 0.3219752754296894559, 0.3333333333333333703, 0.3219752754296894559, 0.3333333333333333703, 0.3219752754296894559, 0.3333333333333333703, 0.3219752754296894559, 0.3333333333333333703, 0.3219752754296894559, 0.3333333333333333703, 0.3219752754296894559, 0.3333333333333333703, 0.3219752754296894559, 0.3333333333333333703, 0.3219752754296894559, 0.3333333333333333703, 0.3219752754296894559, 0.3333333333333333703, 0.3219752754296894559, 0.3333333333333333703, 0.3219752754296894559, 0.3333333333333333703, 0.3219752754296894559, 0.3333333333333333703, 0.3219752754296894559, 0.3333333333333333703, 0.3219752754296894559, 0.3333333333333333703, 0.3219752754296894559, 0.3333333333333333703, 0.3219752754296894559, 0.3333333333333333703, 0.3219752754296894559, 0.3333333333333333703, 0.3219752754296894559, 0.3333333333333333703, 0.3219752754296894559, 0.3333333333333333703, 0.3219752754296894559, 0.3333333333333333703, 0.3219752754296894559, 0.3333333333333333703, 0.3219752754296894559, 0.3333333333333333703, 0.3219752754296894559, 0.3333333333333333703, 0.3219752754296894559, 0.3333333333333333703, 0.3219752754296894559, 0.3333333333333333703, 0.3219752754296894559, 0.3333333333333333703, 0.3219752754296894559, 0.3333333333333333703, 0.3219752754296894559, 0.3333333333333333703, 0.3219752754296894559, 0.3333333333333333703, 0.3219752754296894559, 0.3333333333333333703, 0.3219752754296894559, 0.3333333333333333703, 0.3219752754296894559, 0.3333333333333333703, 0.3219752754296894559, 0.3333333333333333703, 0.3219752754296894559, 0.3333333333333333703, 0.3219752754296894559, 0.3333333333333333703, 0.3219752754296894559, 0.3333333333333333703, 0.3219752754296894559, 0.3333333333333333703, 0.3219752754296894559, 0.3333333333333333703, 0.3219752754296894559, 0.3333333333333333703, 0.3219752754296894559, 0.3333333333333333703, 0.3219752754296894559, 0.3333333333333333703, 0.3219752754296894559, 0.3333333333333333703, 0.3219752754296894559, 0.3333333333333333703, 0.3219752754296894559, 0.3333333333333333703, 0.3219752754296894559, 0.3333333333333333703, 0.3219752754296894559, 0.3333333333333333703, 0.3219752754296894559, 0.3333333333333333703, 0.3219752754296894559, 0.3333333333333333703, 0.3219752754296894559, 0.3333333333333333703, 0.3219752754296894559, 0.3333333333333333703, 0.3219752754296894559, 0.3333333333333333703, 0.3219752754296894559, 0.3333333333333333703, 0.3219752754296894559, 0.3333333333333333703, 0.3219752754296894559, 0.3333333333333333703, 0.3219752754296894559, 0.3333333333333333703, 0.3219752754296894559, 0.3333333333333333703, 0.3219752754296894559, 0.3333333333333333703, 0.3219752754296894559, 0.3333333333333333703, 0.3219752754296894559, 0.3333333333333333703, 0.3219752754296894559, 0.3333333333333333703, 0.3219752754296894559, 0.3333333333333333703, 0.3219752754296894559, 0.3333333333333333703, 0.3219752754296894559, 0.3333333333333333703, 0.3219752754296894559, 0.3333333333333333703, 0.3219752754296894559, 0.3333333333333333703, 0.3219752754296894559, 0.3333333333333333703, 0.3219752754296894559, 0.3333333333333333703, 0.3219752754296894559, 0.3333333333333333703, 0.3219752754296894559, 0.3333333333333333703, 0.3219752754296894559, 0.3333333333333333703, 0.3219752754296894559, 0.3333333333333333703, 0.3219752754296894559, 0.3333333333333333703, 0.3219752754296894559, 0.3333333333333333703, 0.3219752754296894559, 0.3333333333333333703, 0.3219752754296894559, 0.3333333333333333703, 0.3219752754296894559, 0.3333333333333333703, 0.3219752754296894559, 0.3333333333333333703, 0.3219752754296894559, 0.3333333333333333703, 0.3219752754296894559, 0.3333333333333333703, 0.3219752754296894559, 0.3333333333333333703, 0.3219752754296894559, 0.3333333333333333703, 0.3219752754296894559, 0.3333333333333333703, 0.3219752754296894559, 0.3333333333333333703, 0.3219752754296894559, 0.3333333333333333703, 0.3219752754296894559, 0.3333333333333333703, 0.3219752754296894559, 0.3333333333333333703, 0.3219752754296894559, 0.3333333333333333703, 0.3219752754296894559, 0.3333333333333333703, 0.3219752754296894559, 0.3333333333333333703, 0.3219752754296894559, 0.3333333333333333703, 0.3219752754296894559, 0.3333333333333333703, 0.3219752754296894559, 0.3333333333333333703, 0.3219752754296894559, 0.3333333333333333703, 0.3219752754296894559, 0.3333333333333333703, 0.3219752754296894559, 0.3333333333333333703, 0.3219752754296894559, 0.3333333333333333703, 0.3219752754296894559, 0.3333333333333333703, 0.3219752754296894559, 0.3333333333333333703, 0.3219752754296894559, 0.3333333333333333703, 0.3219752754296894559, 0.3333333333333333703, 0.3219752754296894559, 0.3333333333333333703, 0.3219752754296894559, 0.3333333333333333703, 0.3219752754296894559, 0.3333333333333333703, 0.3219752754296894559, 0.3333333333333333703, 0.3219752754296894559, 0.3333333333333333703, 0.3219752754296894559, 0.3333333333333333703, 0.3219752754296894559, 0.3333333333333333703, 0.3219752754296894559, 0.3333333333333333703, 0.3219752754296894559, 0.3333333333333333703, 0.3219752754296894559, 0.3333333333333333703, 0.3219752754296894559, 0.3333333333333333703, 0.3219752754296894559, 0.3333333333333333703, 0.3219752754296894559, 0.3333333333333333703, 0.3219752754296894559, 0.3333333333333333703, 0.3219752754296894559, 0.3333333333333333703, 0.3219752754296894559, 0.3333333333333333703, 0.3219752754296894559, 0.3333333333333333703, 0.3219752754296894559, 0.3333333333333333703, 0.3219752754296894559, 0.3333333333333333703, 0.3219752754296894559, 0.3333333333333333703, 0.3219752754296894559, 0.3333333333333333703, 0.3219752754296894559, 0.3333333333333333703, 0.3219752754296894559, 0.3333333333333333703, 0.3219752754296894559, 0.3333333333333333703, 0.3219752754296894559, 0.3333333333333333703, 0.3219752754296894559, 0.3333333333333333703, 0.3219752754296894559, 0.3333333333333333703, 0.3219752754296894559, 0.3333333333333333703, 0.3219752754296894559, 0.3333333333333333703, 0.3219752754296894559, 0.3333333333333333703, 0.3219752754296894559, 0.3333333333333333703, 0.3219752754296894559, 0.3333333333333333703, 0.3219752754296894559, 0.3333333333333333703, 0.3219752754296894559, 0.3333333333333333703, 0.3219752754296894559, 0.3333333333333333703, 0.3219752754296894559, 0.3333333333333333703, 0.3219752754296894559, 0.3333333333333333703, 0.3219752754296894559, 0.3333333333333333703, 0.3219752754296894559, 0.3333333333333333703, 0.3219752754296894559, 0.3333333333333333703, 0.3219752754296894559, 0.3333333333333333703, 0.3219752754296894559, 0.3333333333333333703, 0.3219752754296894559, 0.3333333333333333703, 0.3219752754296894559, 0.3333333333333333703, 0.3219752754296894559, 0.3333333333333333703, 0.3219752754296894559, 0.3333333333333333703, 0.3219752754296894559, 0.3333333333333333703, 0.3219752754296894559, 0.3333333333333333703, 0.3219752754296894559, 0.3333333333333333703, 0.3219752754296894559, 0.3333333333333333703, 0.3219752754296894559, 0.3333333333333333703, 0.3219752754296894559, 0.3333333333333333703, 0.3219752754296894559, 0.3333333333333333703, 0.3219752754296894559, 0.3333333333333333703, 0.3219752754296894559, 0.3333333333333333703, 0.3219752754296894559, 0.3333333333333333703, 0.3219752754296894559, 0.3333333333333333703, 0.3219752754296894559, 0.3333333333333333703, 0.3219752754296894559, 0.3333333333333333703, 0.3219752754296894559, 0.3333333333333333703, 0.3219752754296894559, 0.3333333333333333703, 0.3219752754296894559, 0.3333333333333333703, 0.3219752754296894559, 0.3333333333333333703, 0.3219752754296894559, 0.3333333333333333703, 0.3219752754296894559, 0.3333333333333333703, 0.3219752754296894559, 0.3333333333333333703, 0.3219752754296894559, 0.3333333333333333703, 0.3219752754296894559, 0.3333333333333333703, 0.3219752754296894559, 0.3333333333333333703, 0.3219752754296894559, 0.3333333333333333703, 0.3219752754296894559, 0.3333333333333333703, 0.3219752754296894559, 0.3333333333333333703, 0.3219752754296894559, 0.3333333333333333703, 0.3219752754296894559, 0.3333333333333333703, 0.3219752754296894559, 0.3333333333333333703, 0.3219752754296894559, 0.3333333333333333703, 0.3219752754296894559, 0.3333333333333333703, 0.3219752754296894559, 0.3333333333333333703, 0.3219752754296894559, 0.3333333333333333703, 0.3219752754296894559, 0.3333333333333333703, 0.3219752754296894559, 0.3333333333333333703, 0.3219752754296894559, 0.3333333333333333703, 0.3219752754296894559, 0.3333333333333333703, 0.3219752754296894559, 0.3333333333333333703, 0.3219752754296894559, 0.3333333333333333703, 0.3219752754296894559, 0.3333333333333333703, 0.3219752754296894559, 0.3333333333333333703, 0.3219752754296894559, 0.3333333333333333703, 0.3219752754296894559, 0.3333333333333333703, 0.3219752754296894559, 0.3333333333333333703, 0.3219752754296894559, 0.3333333333333333703, 0.3219752754296894559, 0.3333333333333333703, 0.3219752754296894559, 0.3333333333333333703, 0.3219752754296894559, 0.3333333333333333703, 0.3219752754296894559, 0.3333333333333333703, 0.3219752754296894559, 0.3333333333333333703, 0.3219752754296894559, 0.3333333333333333703, 0.3219752754296894559, 0.3333333333333333703, 0.3219752754296894559, 0.3333333333333333703, 0.3219752754296894559, 0.3333333333333333703, 0.3219752754296894559, 0.3333333333333333703, 0.3219752754296894559, 0.3333333333333333703, 0.3219752754296894559, 0.3333333333333333703, 0.3219752754296894559, 0.3333333333333333703, 0.3219752754296894559, 0.3333333333333333703, 0.3219752754296894559, 0.3333333333333333703, 0.3219752754296894559, 0.3333333333333333703, 0.3219752754296894559, 0.3333333333333333703, 0.3219752754296894559, 0.3333333333333333703, 0.3219752754296894559, 0.3333333333333333703, 0.3219752754296894559, 0.3333333333333333703, 0.3219752754296894559, 0.3333333333333333703, 0.3219752754296894559, 0.3333333333333333703, 0.3219752754296894559, 0.3333333333333333703, 0.3219752754296894559, 0.3333333333333333703, 0.3219752754296894559, 0.3333333333333333703, 0.3219752754296894559, 0.3333333333333333703, 0.3219752754296894559, 0.3333333333333333703, 0.3219752754296894559, 0.3333333333333333703),
 ( 0.3333333333333333703, 0.3219752754296894559, 0.3333333333333333703, 0.3219752754296894559, 0.3333333333333333703, 0.3219752754296894559, 0.3333333333333333703, 0.3219752754296894559, 0.3333333333333333703, 0.3219752754296894559, 0.3333333333333333703, 0.3219752754296894559, 0.3333333333333333703, 0.3219752754296894559, 0.3333333333333333703, 0.3219752754296894559, 0.3333333333333333703, 0.3219752754296894559, 0.3333333333333333703, 0.3219752754296894559, 0.3333333333333333703, 0.3219752754296894559, 0.3333333333333333703, 0.3219752754296894559, 0.3333333333333333703, 0.3219752754296894559, 0.3333333333333333703, 0.3219752754296894559, 0.3333333333333333703, 0.3219752754296894559, 0.3333333333333333703, 0.3219752754296894559, 0.3333333333333333703, 0.3219752754296894559, 0.3333333333333333703, 0.3219752754296894559, 0.3333333333333333703, 0.3219752754296894559, 0.3333333333333333703, 0.3219752754296894559, 0.3333333333333333703, 0.3219752754296894559, 0.3333333333333333703, 0.3219752754296894559, 0.3333333333333333703, 0.3219752754296894559, 0.3333333333333333703, 0.3219752754296894559, 0.3333333333333333703, 0.3219752754296894559, 0.3333333333333333703, 0.3219752754296894559, 0.3333333333333333703, 0.3219752754296894559, 0.3333333333333333703, 0.3219752754296894559, 0.3333333333333333703, 0.3219752754296894559, 0.3333333333333333703, 0.3219752754296894559, 0.3333333333333333703, 0.3219752754296894559, 0.3333333333333333703, 0.3219752754296894559, 0.3333333333333333703, 0.3219752754296894559, 0.3333333333333333703, 0.3219752754296894559, 0.3333333333333333703, 0.3219752754296894559, 0.3333333333333333703, 0.3219752754296894559, 0.3333333333333333703, 0.3219752754296894559, 0.3333333333333333703, 0.3219752754296894559, 0.3333333333333333703, 0.3219752754296894559, 0.3333333333333333703, 0.3219752754296894559, 0.3333333333333333703, 0.3219752754296894559, 0.3333333333333333703, 0.3219752754296894559, 0.3333333333333333703, 0.3219752754296894559, 0.3333333333333333703, 0.3219752754296894559, 0.3333333333333333703, 0.3219752754296894559, 0.3333333333333333703, 0.3219752754296894559, 0.3333333333333333703, 0.3219752754296894559, 0.3333333333333333703, 0.3219752754296894559, 0.3333333333333333703, 0.3219752754296894559, 0.3333333333333333703, 0.3219752754296894559, 0.3333333333333333703, 0.3219752754296894559, 0.3333333333333333703, 0.3219752754296894559, 0.3333333333333333703, 0.3219752754296894559, 0.3333333333333333703, 0.3219752754296894559, 0.3333333333333333703, 0.3219752754296894559, 0.3333333333333333703, 0.3219752754296894559, 0.3333333333333333703, 0.3219752754296894559, 0.3333333333333333703, 0.3219752754296894559, 0.3333333333333333703, 0.3219752754296894559, 0.3333333333333333703, 0.3219752754296894559, 0.3333333333333333703, 0.3219752754296894559, 0.3333333333333333703, 0.3219752754296894559, 0.3333333333333333703, 0.3219752754296894559, 0.3333333333333333703, 0.3219752754296894559, 0.3333333333333333703, 0.3219752754296894559, 0.3333333333333333703, 0.3219752754296894559, 0.3333333333333333703, 0.3219752754296894559, 0.3333333333333333703, 0.3219752754296894559, 0.3333333333333333703, 0.3219752754296894559, 0.3333333333333333703, 0.3219752754296894559, 0.3333333333333333703, 0.3219752754296894559, 0.3333333333333333703, 0.3219752754296894559, 0.3333333333333333703, 0.3219752754296894559, 0.3333333333333333703, 0.3219752754296894559, 0.3333333333333333703, 0.3219752754296894559, 0.3333333333333333703, 0.3219752754296894559, 0.3333333333333333703, 0.3219752754296894559, 0.3333333333333333703, 0.3219752754296894559, 0.3333333333333333703, 0.3219752754296894559, 0.3333333333333333703, 0.3219752754296894559, 0.3333333333333333703, 0.3219752754296894559, 0.3333333333333333703, 0.3219752754296894559, 0.3333333333333333703, 0.3219752754296894559, 0.3333333333333333703, 0.3219752754296894559, 0.3333333333333333703, 0.3219752754296894559, 0.3333333333333333703, 0.3219752754296894559, 0.3333333333333333703, 0.3219752754296894559, 0.3333333333333333703, 0.3219752754296894559, 0.3333333333333333703, 0.3219752754296894559, 0.3333333333333333703, 0.3219752754296894559, 0.3333333333333333703, 0.3219752754296894559, 0.3333333333333333703, 0.3219752754296894559, 0.3333333333333333703, 0.3219752754296894559, 0.3333333333333333703, 0.3219752754296894559, 0.3333333333333333703, 0.3219752754296894559, 0.3333333333333333703, 0.3219752754296894559, 0.3333333333333333703, 0.3219752754296894559, 0.3333333333333333703, 0.3219752754296894559, 0.3333333333333333703, 0.3219752754296894559, 0.3333333333333333703, 0.3219752754296894559, 0.3333333333333333703, 0.3219752754296894559, 0.3333333333333333703, 0.3219752754296894559, 0.3333333333333333703, 0.3219752754296894559, 0.3333333333333333703, 0.3219752754296894559, 0.3333333333333333703, 0.3219752754296894559, 0.3333333333333333703, 0.3219752754296894559, 0.3333333333333333703, 0.3219752754296894559, 0.3333333333333333703, 0.3219752754296894559, 0.3333333333333333703, 0.3219752754296894559, 0.3333333333333333703, 0.3219752754296894559, 0.3333333333333333703, 0.3219752754296894559, 0.3333333333333333703, 0.3219752754296894559, 0.3333333333333333703, 0.3219752754296894559, 0.3333333333333333703, 0.3219752754296894559, 0.3333333333333333703, 0.3219752754296894559, 0.3333333333333333703, 0.3219752754296894559, 0.3333333333333333703, 0.3219752754296894559, 0.3333333333333333703, 0.3219752754296894559, 0.3333333333333333703, 0.3219752754296894559, 0.3333333333333333703, 0.3219752754296894559, 0.3333333333333333703, 0.3219752754296894559, 0.3333333333333333703, 0.3219752754296894559, 0.3333333333333333703, 0.3219752754296894559, 0.3333333333333333703, 0.3219752754296894559, 0.3333333333333333703, 0.3219752754296894559, 0.3333333333333333703, 0.3219752754296894559, 0.3333333333333333703, 0.3219752754296894559, 0.3333333333333333703, 0.3219752754296894559, 0.3333333333333333703, 0.3219752754296894559, 0.3333333333333333703, 0.3219752754296894559, 0.3333333333333333703, 0.3219752754296894559, 0.3333333333333333703, 0.3219752754296894559, 0.3333333333333333703, 0.3219752754296894559, 0.3333333333333333703, 0.3219752754296894559, 0.3333333333333333703, 0.3219752754296894559, 0.3333333333333333703, 0.3219752754296894559, 0.3333333333333333703, 0.3219752754296894559, 0.3333333333333333703, 0.3219752754296894559, 0.3333333333333333703, 0.3219752754296894559, 0.3333333333333333703, 0.3219752754296894559, 0.3333333333333333703, 0.3219752754296894559, 0.3333333333333333703, 0.3219752754296894559, 0.3333333333333333703, 0.3219752754296894559, 0.3333333333333333703, 0.3219752754296894559, 0.3333333333333333703, 0.3219752754296894559, 0.3333333333333333703, 0.3219752754296894559, 0.3333333333333333703, 0.3219752754296894559, 0.3333333333333333703, 0.3219752754296894559, 0.3333333333333333703, 0.3219752754296894559, 0.3333333333333333703, 0.3219752754296894559, 0.3333333333333333703, 0.3219752754296894559, 0.3333333333333333703, 0.3219752754296894559, 0.3333333333333333703, 0.3219752754296894559, 0.3333333333333333703, 0.3219752754296894559, 0.3333333333333333703, 0.3219752754296894559, 0.3333333333333333703, 0.3219752754296894559, 0.3333333333333333703, 0.3219752754296894559, 0.3333333333333333703, 0.3219752754296894559, 0.3333333333333333703, 0.3219752754296894559, 0.3333333333333333703, 0.3219752754296894559, 0.3333333333333333703, 0.3219752754296894559, 0.3333333333333333703, 0.3219752754296894559, 0.3333333333333333703, 0.3219752754296894559, 0.3333333333333333703, 0.3219752754296894559, 0.3333333333333333703, 0.3219752754296894559, 0.3333333333333333703, 0.3219752754296894559, 0.3333333333333333703, 0.3219752754296894559, 0.3333333333333333703, 0.3219752754296894559, 0.3333333333333333703, 0.3219752754296894559, 0.3333333333333333703, 0.3219752754296894559, 0.3333333333333333703, 0.3219752754296894559, 0.3333333333333333703, 0.3219752754296894559, 0.3333333333333333703, 0.3219752754296894559, 0.3333333333333333703, 0.3219752754296894559, 0.3333333333333333703, 0.3219752754296894559, 0.3333333333333333703, 0.3219752754296894559, 0.3333333333333333703, 0.3219752754296894559, 0.3333333333333333703, 0.3219752754296894559, 0.3333333333333333703, 0.3219752754296894559, 0.3333333333333333703, 0.3219752754296894559, 0.3333333333333333703, 0.3219752754296894559, 0.3333333333333333703, 0.3219752754296894559, 0.3333333333333333703, 0.3219752754296894559, 0.3333333333333333703, 0.3219752754296894559, 0.3333333333333333703, 0.3219752754296894559, 0.3333333333333333703, 0.3219752754296894559, 0.3333333333333333703, 0.3219752754296894559, 0.3333333333333333703, 0.3219752754296894559, 0.3333333333333333703, 0.3219752754296894559, 0.3333333333333333703, 0.3219752754296894559, 0.3333333333333333703, 0.3219752754296894559, 0.3333333333333333703, 0.3219752754296894559, 0.3333333333333333703, 0.3219752754296894559, 0.3333333333333333703, 0.3219752754296894559, 0.3333333333333333703, 0.3219752754296894559, 0.3333333333333333703, 0.3219752754296894559, 0.3333333333333333703, 0.3219752754296894559, 0.3333333333333333703, 0.3219752754296894559, 0.3333333333333333703, 0.3219752754296894559, 0.3333333333333333703, 0.3219752754296894559, 0.3333333333333333703, 0.3219752754296894559, 0.3333333333333333703, 0.3219752754296894559, 0.3333333333333333703, 0.3219752754296894559, 0.3333333333333333703, 0.3219752754296894559, 0.3333333333333333703, 0.3219752754296894559, 0.3333333333333333703, 0.3219752754296894559, 0.3333333333333333703, 0.3219752754296894559, 0.3333333333333333703, 0.3219752754296894559, 0.3333333333333333703, 0.3219752754296894559, 0.3333333333333333703, 0.3219752754296894559, 0.3333333333333333703, 0.3219752754296894559, 0.3333333333333333703, 0.3219752754296894559, 0.3333333333333333703, 0.3219752754296894559, 0.3333333333333333703, 0.3219752754296894559, 0.3333333333333333703, 0.3219752754296894559, 0.3333333333333333703, 0.3219752754296894559, 0.3333333333333333703, 0.3219752754296894559, 0.3333333333333333703, 0.3219752754296894559, 0.3333333333333333703, 0.3219752754296894559, 0.3333333333333333703, 0.3219752754296894559, 0.3333333333333333703, 0.3219752754296894559, 0.3333333333333333703, 0.3219752754296894559, 0.3333333333333333703, 0.3219752754296894559, 0.3333333333333333703, 0.3219752754296894559, 0.3333333333333333703, 0.3219752754296894559, 0.3333333333333333703, 0.3219752754296894559, 0.3333333333333333703, 0.3219752754296894559, 0.3333333333333333703, 0.3219752754296894559, 0.3333333333333333703),
 ( 1.000000000000000000, 0.9659258262890683122, 1.000000000000000000, 0.9659258262890683122, 1.000000000000000000, 0.9659258262890683122, 1.000000000000000000, 0.9659258262890683122, 1.000000000000000000, 0.9659258262890683122, 1.000000000000000000, 0.9659258262890683122, 1.000000000000000000, 0.9659258262890683122, 1.000000000000000000, 0.9659258262890683122, 1.000000000000000000, 0.9659258262890683122, 1.000000000000000000, 0.9659258262890683122, 1.000000000000000000, 0.9659258262890683122, 1.000000000000000000, 0.9659258262890683122, 1.000000000000000000, 0.9659258262890683122, 1.000000000000000000, 0.9659258262890683122, 1.000000000000000000, 0.9659258262890683122, 1.000000000000000000, 0.9659258262890683122, 1.000000000000000000, 0.9659258262890683122, 1.000000000000000000, 0.9659258262890683122, 1.000000000000000000, 0.9659258262890683122, 1.000000000000000000, 0.9659258262890683122, 1.000000000000000000, 0.9659258262890683122, 1.000000000000000000, 0.9659258262890683122, 1.000000000000000000, 0.9659258262890683122, 1.000000000000000000, 0.9659258262890683122, 1.000000000000000000, 0.9659258262890683122, 1.000000000000000000, 0.9659258262890683122, 1.000000000000000000, 0.9659258262890683122, 1.000000000000000000, 0.9659258262890683122, 1.000000000000000000, 0.9659258262890683122, 1.000000000000000000, 0.9659258262890683122, 1.000000000000000000, 0.9659258262890683122, 1.000000000000000000, 0.9659258262890683122, 1.000000000000000000, 0.9659258262890683122, 1.000000000000000000, 0.9659258262890683122, 1.000000000000000000, 0.9659258262890683122, 1.000000000000000000, 0.9659258262890683122, 1.000000000000000000, 0.9659258262890683122, 1.000000000000000000, 0.9659258262890683122, 1.000000000000000000, 0.9659258262890683122, 1.000000000000000000, 0.9659258262890683122, 1.000000000000000000, 0.9659258262890683122, 1.000000000000000000, 0.9659258262890683122, 1.000000000000000000, 0.9659258262890683122, 1.000000000000000000, 0.9659258262890683122, 1.000000000000000000, 0.9659258262890683122, 1.000000000000000000, 0.9659258262890683122, 1.000000000000000000, 0.9659258262890683122, 1.000000000000000000, 0.9659258262890683122, 1.000000000000000000, 0.9659258262890683122, 1.000000000000000000, 0.9659258262890683122, 1.000000000000000000, 0.9659258262890683122, 1.000000000000000000, 0.9659258262890683122, 1.000000000000000000, 0.9659258262890683122, 1.000000000000000000, 0.9659258262890683122, 1.000000000000000000, 0.9659258262890683122, 1.000000000000000000, 0.9659258262890683122, 1.000000000000000000, 0.9659258262890683122, 1.000000000000000000, 0.9659258262890683122, 1.000000000000000000, 0.9659258262890683122, 1.000000000000000000, 0.9659258262890683122, 1.000000000000000000, 0.9659258262890683122, 1.000000000000000000, 0.9659258262890683122, 1.000000000000000000, 0.9659258262890683122, 1.000000000000000000, 0.9659258262890683122, 1.000000000000000000, 0.9659258262890683122, 1.000000000000000000, 0.9659258262890683122, 1.000000000000000000, 0.9659258262890683122, 1.000000000000000000, 0.9659258262890683122, 1.000000000000000000, 0.9659258262890683122, 1.000000000000000000, 0.9659258262890683122, 1.000000000000000000, 0.9659258262890683122, 1.000000000000000000, 0.9659258262890683122, 1.000000000000000000, 0.9659258262890683122, 1.000000000000000000, 0.9659258262890683122, 1.000000000000000000, 0.9659258262890683122, 1.000000000000000000, 0.9659258262890683122, 1.000000000000000000, 0.9659258262890683122, 1.000000000000000000, 0.9659258262890683122, 1.000000000000000000, 0.9659258262890683122, 1.000000000000000000, 0.9659258262890683122, 1.000000000000000000, 0.9659258262890683122, 1.000000000000000000, 0.9659258262890683122, 1.000000000000000000, 0.9659258262890683122, 1.000000000000000000, 0.9659258262890683122, 1.000000000000000000, 0.9659258262890683122, 1.000000000000000000, 0.9659258262890683122, 1.000000000000000000, 0.9659258262890683122, 1.000000000000000000, 0.9659258262890683122, 1.000000000000000000, 0.9659258262890683122, 1.000000000000000000, 0.9659258262890683122, 1.000000000000000000, 0.9659258262890683122, 1.000000000000000000, 0.9659258262890683122, 1.000000000000000000, 0.9659258262890683122, 1.000000000000000000, 0.9659258262890683122, 1.000000000000000000, 0.9659258262890683122, 1.000000000000000000, 0.9659258262890683122, 1.000000000000000000, 0.9659258262890683122, 1.000000000000000000, 0.9659258262890683122, 1.000000000000000000, 0.9659258262890683122, 1.000000000000000000, 0.9659258262890683122, 1.000000000000000000, 0.9659258262890683122, 1.000000000000000000, 0.9659258262890683122, 1.000000000000000000, 0.9659258262890683122, 1.000000000000000000, 0.9659258262890683122, 1.000000000000000000, 0.9659258262890683122, 1.000000000000000000, 0.9659258262890683122, 1.000000000000000000, 0.9659258262890683122, 1.000000000000000000, 0.9659258262890683122, 1.000000000000000000, 0.9659258262890683122, 1.000000000000000000, 0.9659258262890683122, 1.000000000000000000, 0.9659258262890683122, 1.000000000000000000, 0.9659258262890683122, 1.000000000000000000, 0.9659258262890683122, 1.000000000000000000, 0.9659258262890683122, 1.000000000000000000, 0.9659258262890683122, 1.000000000000000000, 0.9659258262890683122, 1.000000000000000000, 0.9659258262890683122, 1.000000000000000000, 0.9659258262890683122, 1.000000000000000000, 0.9659258262890683122, 1.000000000000000000, 0.9659258262890683122, 1.000000000000000000, 0.9659258262890683122, 1.000000000000000000, 0.9659258262890683122, 1.000000000000000000, 0.9659258262890683122, 1.000000000000000000, 0.9659258262890683122, 1.000000000000000000, 0.9659258262890683122, 1.000000000000000000, 0.9659258262890683122, 1.000000000000000000, 0.9659258262890683122, 1.000000000000000000, 0.9659258262890683122, 1.000000000000000000, 0.9659258262890683122, 1.000000000000000000, 0.9659258262890683122, 1.000000000000000000, 0.9659258262890683122, 1.000000000000000000, 0.9659258262890683122, 1.000000000000000000, 0.9659258262890683122, 1.000000000000000000, 0.9659258262890683122, 1.000000000000000000, 0.9659258262890683122, 1.000000000000000000, 0.9659258262890683122, 1.000000000000000000, 0.9659258262890683122, 1.000000000000000000, 0.9659258262890683122, 1.000000000000000000, 0.9659258262890683122, 1.000000000000000000, 0.9659258262890683122, 1.000000000000000000, 0.9659258262890683122, 1.000000000000000000, 0.9659258262890683122, 1.000000000000000000, 0.9659258262890683122, 1.000000000000000000, 0.9659258262890683122, 1.000000000000000000, 0.9659258262890683122, 1.000000000000000000, 0.9659258262890683122, 1.000000000000000000, 0.9659258262890683122, 1.000000000000000000, 0.9659258262890683122, 1.000000000000000000, 0.9659258262890683122, 1.000000000000000000, 0.9659258262890683122, 1.000000000000000000, 0.9659258262890683122, 1.000000000000000000, 0.9659258262890683122, 1.000000000000000000, 0.9659258262890683122, 1.000000000000000000, 0.9659258262890683122, 1.000000000000000000, 0.9659258262890683122, 1.000000000000000000, 0.9659258262890683122, 1.000000000000000000, 0.9659258262890683122, 1.000000000000000000, 0.9659258262890683122, 1.000000000000000000, 0.9659258262890683122, 1.000000000000000000, 0.9659258262890683122, 1.000000000000000000, 0.9659258262890683122, 1.000000000000000000, 0.9659258262890683122, 1.000000000000000000, 0.9659258262890683122, 1.000000000000000000, 0.9659258262890683122, 1.000000000000000000, 0.9659258262890683122, 1.000000000000000000, 0.9659258262890683122, 1.000000000000000000, 0.9659258262890683122, 1.000000000000000000, 0.9659258262890683122, 1.000000000000000000, 0.9659258262890683122, 1.000000000000000000, 0.9659258262890683122, 1.000000000000000000, 0.9659258262890683122, 1.000000000000000000, 0.9659258262890683122, 1.000000000000000000, 0.9659258262890683122, 1.000000000000000000, 0.9659258262890683122, 1.000000000000000000, 0.9659258262890683122, 1.000000000000000000, 0.9659258262890683122, 1.000000000000000000, 0.9659258262890683122, 1.000000000000000000, 0.9659258262890683122, 1.000000000000000000, 0.9659258262890683122, 1.000000000000000000, 0.9659258262890683122, 1.000000000000000000, 0.9659258262890683122, 1.000000000000000000, 0.9659258262890683122, 1.000000000000000000, 0.9659258262890683122, 1.000000000000000000, 0.9659258262890683122, 1.000000000000000000, 0.9659258262890683122, 1.000000000000000000, 0.9659258262890683122, 1.000000000000000000, 0.9659258262890683122, 1.000000000000000000, 0.9659258262890683122, 1.000000000000000000, 0.9659258262890683122, 1.000000000000000000, 0.9659258262890683122, 1.000000000000000000, 0.9659258262890683122, 1.000000000000000000, 0.9659258262890683122, 1.000000000000000000, 0.9659258262890683122, 1.000000000000000000, 0.9659258262890683122, 1.000000000000000000, 0.9659258262890683122, 1.000000000000000000, 0.9659258262890683122, 1.000000000000000000, 0.9659258262890683122, 1.000000000000000000, 0.9659258262890683122, 1.000000000000000000, 0.9659258262890683122, 1.000000000000000000, 0.9659258262890683122, 1.000000000000000000, 0.9659258262890683122, 1.000000000000000000, 0.9659258262890683122, 1.000000000000000000, 0.9659258262890683122, 1.000000000000000000, 0.9659258262890683122, 1.000000000000000000, 0.9659258262890683122, 1.000000000000000000, 0.9659258262890683122, 1.000000000000000000, 0.9659258262890683122, 1.000000000000000000, 0.9659258262890683122, 1.000000000000000000, 0.9659258262890683122, 1.000000000000000000, 0.9659258262890683122, 1.000000000000000000, 0.9659258262890683122, 1.000000000000000000, 0.9659258262890683122, 1.000000000000000000, 0.9659258262890683122, 1.000000000000000000, 0.9659258262890683122, 1.000000000000000000, 0.9659258262890683122, 1.000000000000000000, 0.9659258262890683122, 1.000000000000000000, 0.9659258262890683122, 1.000000000000000000, 0.9659258262890683122, 1.000000000000000000, 0.9659258262890683122, 1.000000000000000000, 0.9659258262890683122, 1.000000000000000000, 0.9659258262890683122, 1.000000000000000000, 0.9659258262890683122, 1.000000000000000000, 0.9659258262890683122, 1.000000000000000000, 0.9659258262890683122, 1.000000000000000000, 0.9659258262890683122, 1.000000000000000000, 0.9659258262890683122, 1.000000000000000000, 0.9659258262890683122, 1.000000000000000000, 0.9659258262890683122, 1.000000000000000000),
 ( 0.3333333333333333703, 0.3219752754296894559, 0.3333333333333333703, 0.3219752754296894559, 0.3333333333333333703, 0.3219752754296894559, 0.3333333333333333703, 0.3219752754296894559, 0.3333333333333333703, 0.3219752754296894559, 0.3333333333333333703, 0.3219752754296894559, 0.3333333333333333703, 0.3219752754296894559, 0.3333333333333333703, 0.3219752754296894559, 0.3333333333333333703, 0.3219752754296894559, 0.3333333333333333703, 0.3219752754296894559, 0.3333333333333333703, 0.3219752754296894559, 0.3333333333333333703, 0.3219752754296894559, 0.3333333333333333703, 0.3219752754296894559, 0.3333333333333333703, 0.3219752754296894559, 0.3333333333333333703, 0.3219752754296894559, 0.3333333333333333703, 0.3219752754296894559, 0.3333333333333333703, 0.3219752754296894559, 0.3333333333333333703, 0.3219752754296894559, 0.3333333333333333703, 0.3219752754296894559, 0.3333333333333333703, 0.3219752754296894559, 0.3333333333333333703, 0.3219752754296894559, 0.3333333333333333703, 0.3219752754296894559, 0.3333333333333333703, 0.3219752754296894559, 0.3333333333333333703, 0.3219752754296894559, 0.3333333333333333703, 0.3219752754296894559, 0.3333333333333333703, 0.3219752754296894559, 0.3333333333333333703, 0.3219752754296894559, 0.3333333333333333703, 0.3219752754296894559, 0.3333333333333333703, 0.3219752754296894559, 0.3333333333333333703, 0.3219752754296894559, 0.3333333333333333703, 0.3219752754296894559, 0.3333333333333333703, 0.3219752754296894559, 0.3333333333333333703, 0.3219752754296894559, 0.3333333333333333703, 0.3219752754296894559, 0.3333333333333333703, 0.3219752754296894559, 0.3333333333333333703, 0.3219752754296894559, 0.3333333333333333703, 0.3219752754296894559, 0.3333333333333333703, 0.3219752754296894559, 0.3333333333333333703, 0.3219752754296894559, 0.3333333333333333703, 0.3219752754296894559, 0.3333333333333333703, 0.3219752754296894559, 0.3333333333333333703, 0.3219752754296894559, 0.3333333333333333703, 0.3219752754296894559, 0.3333333333333333703, 0.3219752754296894559, 0.3333333333333333703, 0.3219752754296894559, 0.3333333333333333703, 0.3219752754296894559, 0.3333333333333333703, 0.3219752754296894559, 0.3333333333333333703, 0.3219752754296894559, 0.3333333333333333703, 0.3219752754296894559, 0.3333333333333333703, 0.3219752754296894559, 0.3333333333333333703, 0.3219752754296894559, 0.3333333333333333703, 0.3219752754296894559, 0.3333333333333333703, 0.3219752754296894559, 0.3333333333333333703, 0.3219752754296894559, 0.3333333333333333703, 0.3219752754296894559, 0.3333333333333333703, 0.3219752754296894559, 0.3333333333333333703, 0.3219752754296894559, 0.3333333333333333703, 0.3219752754296894559, 0.3333333333333333703, 0.3219752754296894559, 0.3333333333333333703, 0.3219752754296894559, 0.3333333333333333703, 0.3219752754296894559, 0.3333333333333333703, 0.3219752754296894559, 0.3333333333333333703, 0.3219752754296894559, 0.3333333333333333703, 0.3219752754296894559, 0.3333333333333333703, 0.3219752754296894559, 0.3333333333333333703, 0.3219752754296894559, 0.3333333333333333703, 0.3219752754296894559, 0.3333333333333333703, 0.3219752754296894559, 0.3333333333333333703, 0.3219752754296894559, 0.3333333333333333703, 0.3219752754296894559, 0.3333333333333333703, 0.3219752754296894559, 0.3333333333333333703, 0.3219752754296894559, 0.3333333333333333703, 0.3219752754296894559, 0.3333333333333333703, 0.3219752754296894559, 0.3333333333333333703, 0.3219752754296894559, 0.3333333333333333703, 0.3219752754296894559, 0.3333333333333333703, 0.3219752754296894559, 0.3333333333333333703, 0.3219752754296894559, 0.3333333333333333703, 0.3219752754296894559, 0.3333333333333333703, 0.3219752754296894559, 0.3333333333333333703, 0.3219752754296894559, 0.3333333333333333703, 0.3219752754296894559, 0.3333333333333333703, 0.3219752754296894559, 0.3333333333333333703, 0.3219752754296894559, 0.3333333333333333703, 0.3219752754296894559, 0.3333333333333333703, 0.3219752754296894559, 0.3333333333333333703, 0.3219752754296894559, 0.3333333333333333703, 0.3219752754296894559, 0.3333333333333333703, 0.3219752754296894559, 0.3333333333333333703, 0.3219752754296894559, 0.3333333333333333703, 0.3219752754296894559, 0.3333333333333333703, 0.3219752754296894559, 0.3333333333333333703, 0.3219752754296894559, 0.3333333333333333703, 0.3219752754296894559, 0.3333333333333333703, 0.3219752754296894559, 0.3333333333333333703, 0.3219752754296894559, 0.3333333333333333703, 0.3219752754296894559, 0.3333333333333333703, 0.3219752754296894559, 0.3333333333333333703, 0.3219752754296894559, 0.3333333333333333703, 0.3219752754296894559, 0.3333333333333333703, 0.3219752754296894559, 0.3333333333333333703, 0.3219752754296894559, 0.3333333333333333703, 0.3219752754296894559, 0.3333333333333333703, 0.3219752754296894559, 0.3333333333333333703, 0.3219752754296894559, 0.3333333333333333703, 0.3219752754296894559, 0.3333333333333333703, 0.3219752754296894559, 0.3333333333333333703, 0.3219752754296894559, 0.3333333333333333703, 0.3219752754296894559, 0.3333333333333333703, 0.3219752754296894559, 0.3333333333333333703, 0.3219752754296894559, 0.3333333333333333703, 0.3219752754296894559, 0.3333333333333333703, 0.3219752754296894559, 0.3333333333333333703, 0.3219752754296894559, 0.3333333333333333703, 0.3219752754296894559, 0.3333333333333333703, 0.3219752754296894559, 0.3333333333333333703, 0.3219752754296894559, 0.3333333333333333703, 0.3219752754296894559, 0.3333333333333333703, 0.3219752754296894559, 0.3333333333333333703, 0.3219752754296894559, 0.3333333333333333703, 0.3219752754296894559, 0.3333333333333333703, 0.3219752754296894559, 0.3333333333333333703, 0.3219752754296894559, 0.3333333333333333703, 0.3219752754296894559, 0.3333333333333333703, 0.3219752754296894559, 0.3333333333333333703, 0.3219752754296894559, 0.3333333333333333703, 0.3219752754296894559, 0.3333333333333333703, 0.3219752754296894559, 0.3333333333333333703, 0.3219752754296894559, 0.3333333333333333703, 0.3219752754296894559, 0.3333333333333333703, 0.3219752754296894559, 0.3333333333333333703, 0.3219752754296894559, 0.3333333333333333703, 0.3219752754296894559, 0.3333333333333333703, 0.3219752754296894559, 0.3333333333333333703, 0.3219752754296894559, 0.3333333333333333703, 0.3219752754296894559, 0.3333333333333333703, 0.3219752754296894559, 0.3333333333333333703, 0.3219752754296894559, 0.3333333333333333703, 0.3219752754296894559, 0.3333333333333333703, 0.3219752754296894559, 0.3333333333333333703, 0.3219752754296894559, 0.3333333333333333703, 0.3219752754296894559, 0.3333333333333333703, 0.3219752754296894559, 0.3333333333333333703, 0.3219752754296894559, 0.3333333333333333703, 0.3219752754296894559, 0.3333333333333333703, 0.3219752754296894559, 0.3333333333333333703, 0.3219752754296894559, 0.3333333333333333703, 0.3219752754296894559, 0.3333333333333333703, 0.3219752754296894559, 0.3333333333333333703, 0.3219752754296894559, 0.3333333333333333703, 0.3219752754296894559, 0.3333333333333333703, 0.3219752754296894559, 0.3333333333333333703, 0.3219752754296894559, 0.3333333333333333703, 0.3219752754296894559, 0.3333333333333333703, 0.3219752754296894559, 0.3333333333333333703, 0.3219752754296894559, 0.3333333333333333703, 0.3219752754296894559, 0.3333333333333333703, 0.3219752754296894559, 0.3333333333333333703, 0.3219752754296894559, 0.3333333333333333703, 0.3219752754296894559, 0.3333333333333333703, 0.3219752754296894559, 0.3333333333333333703, 0.3219752754296894559, 0.3333333333333333703, 0.3219752754296894559, 0.3333333333333333703, 0.3219752754296894559, 0.3333333333333333703, 0.3219752754296894559, 0.3333333333333333703, 0.3219752754296894559, 0.3333333333333333703, 0.3219752754296894559, 0.3333333333333333703, 0.3219752754296894559, 0.3333333333333333703, 0.3219752754296894559, 0.3333333333333333703, 0.3219752754296894559, 0.3333333333333333703, 0.3219752754296894559, 0.3333333333333333703, 0.3219752754296894559, 0.3333333333333333703, 0.3219752754296894559, 0.3333333333333333703, 0.3219752754296894559, 0.3333333333333333703, 0.3219752754296894559, 0.3333333333333333703, 0.3219752754296894559, 0.3333333333333333703, 0.3219752754296894559, 0.3333333333333333703, 0.3219752754296894559, 0.3333333333333333703, 0.3219752754296894559, 0.3333333333333333703, 0.3219752754296894559, 0.3333333333333333703, 0.3219752754296894559, 0.3333333333333333703, 0.3219752754296894559, 0.3333333333333333703, 0.3219752754296894559, 0.3333333333333333703, 0.3219752754296894559, 0.3333333333333333703, 0.3219752754296894559, 0.3333333333333333703, 0.3219752754296894559, 0.3333333333333333703, 0.3219752754296894559, 0.3333333333333333703, 0.3219752754296894559, 0.3333333333333333703, 0.3219752754296894559, 0.3333333333333333703, 0.3219752754296894559, 0.3333333333333333703, 0.3219752754296894559, 0.3333333333333333703, 0.3219752754296894559, 0.3333333333333333703, 0.3219752754296894559, 0.3333333333333333703, 0.3219752754296894559, 0.3333333333333333703, 0.3219752754296894559, 0.3333333333333333703, 0.3219752754296894559, 0.3333333333333333703, 0.3219752754296894559, 0.3333333333333333703, 0.3219752754296894559, 0.3333333333333333703, 0.3219752754296894559, 0.3333333333333333703, 0.3219752754296894559, 0.3333333333333333703, 0.3219752754296894559, 0.3333333333333333703, 0.3219752754296894559, 0.3333333333333333703, 0.3219752754296894559, 0.3333333333333333703, 0.3219752754296894559, 0.3333333333333333703, 0.3219752754296894559, 0.3333333333333333703, 0.3219752754296894559, 0.3333333333333333703, 0.3219752754296894559, 0.3333333333333333703, 0.3219752754296894559, 0.3333333333333333703, 0.3219752754296894559, 0.3333333333333333703, 0.3219752754296894559, 0.3333333333333333703, 0.3219752754296894559, 0.3333333333333333703, 0.3219752754296894559, 0.3333333333333333703, 0.3219752754296894559, 0.3333333333333333703, 0.3219752754296894559, 0.3333333333333333703, 0.3219752754296894559, 0.3333333333333333703, 0.3219752754296894559, 0.3333333333333333703, 0.3219752754296894559, 0.3333333333333333703, 0.3219752754296894559, 0.3333333333333333703, 0.3219752754296894559, 0.3333333333333333703, 0.3219752754296894559, 0.3333333333333333703, 0.3219752754296894559, 0.3333333333333333703, 0.3219752754296894559, 0.3333333333333333703, 0.3219752754296894559, 0.3333333333333333703, 0.3219752754296894559, 0.3333333333333333703, 0.3219752754296894559, 0.3333333333333333703, 0.3219752754296894559, 0.3333333333333333703, 0.3219752754296894559, 0.3333333333333333703, 0.3219752754296894559, 0.3333333333333333703),
 ( 0.3333333333333333703, 0.3219752754296894559, 0.3333333333333333703, 0.3219752754296894559, 0.3333333333333333703, 0.3219752754296894559, 0.3333333333333333703, 0.3219752754296894559, 0.3333333333333333703, 0.3219752754296894559, 0.3333333333333333703, 0.3219752754296894559, 0.3333333333333333703, 0.3219752754296894559, 0.3333333333333333703, 0.3219752754296894559, 0.3333333333333333703, 0.3219752754296894559, 0.3333333333333333703, 0.3219752754296894559, 0.3333333333333333703, 0.3219752754296894559, 0.3333333333333333703, 0.3219752754296894559, 0.3333333333333333703, 0.3219752754296894559, 0.3333333333333333703, 0.3219752754296894559, 0.3333333333333333703, 0.3219752754296894559, 0.3333333333333333703, 0.3219752754296894559, 0.3333333333333333703, 0.3219752754296894559, 0.3333333333333333703, 0.3219752754296894559, 0.3333333333333333703, 0.3219752754296894559, 0.3333333333333333703, 0.3219752754296894559, 0.3333333333333333703, 0.3219752754296894559, 0.3333333333333333703, 0.3219752754296894559, 0.3333333333333333703, 0.3219752754296894559, 0.3333333333333333703, 0.3219752754296894559, 0.3333333333333333703, 0.3219752754296894559, 0.3333333333333333703, 0.3219752754296894559, 0.3333333333333333703, 0.3219752754296894559, 0.3333333333333333703, 0.3219752754296894559, 0.3333333333333333703, 0.3219752754296894559, 0.3333333333333333703, 0.3219752754296894559, 0.3333333333333333703, 0.3219752754296894559, 0.3333333333333333703, 0.3219752754296894559, 0.3333333333333333703, 0.3219752754296894559, 0.3333333333333333703, 0.3219752754296894559, 0.3333333333333333703, 0.3219752754296894559, 0.3333333333333333703, 0.3219752754296894559, 0.3333333333333333703, 0.3219752754296894559, 0.3333333333333333703, 0.3219752754296894559, 0.3333333333333333703, 0.3219752754296894559, 0.3333333333333333703, 0.3219752754296894559, 0.3333333333333333703, 0.3219752754296894559, 0.3333333333333333703, 0.3219752754296894559, 0.3333333333333333703, 0.3219752754296894559, 0.3333333333333333703, 0.3219752754296894559, 0.3333333333333333703, 0.3219752754296894559, 0.3333333333333333703, 0.3219752754296894559, 0.3333333333333333703, 0.3219752754296894559, 0.3333333333333333703, 0.3219752754296894559, 0.3333333333333333703, 0.3219752754296894559, 0.3333333333333333703, 0.3219752754296894559, 0.3333333333333333703, 0.3219752754296894559, 0.3333333333333333703, 0.3219752754296894559, 0.3333333333333333703, 0.3219752754296894559, 0.3333333333333333703, 0.3219752754296894559, 0.3333333333333333703, 0.3219752754296894559, 0.3333333333333333703, 0.3219752754296894559, 0.3333333333333333703, 0.3219752754296894559, 0.3333333333333333703, 0.3219752754296894559, 0.3333333333333333703, 0.3219752754296894559, 0.3333333333333333703, 0.3219752754296894559, 0.3333333333333333703, 0.3219752754296894559, 0.3333333333333333703, 0.3219752754296894559, 0.3333333333333333703, 0.3219752754296894559, 0.3333333333333333703, 0.3219752754296894559, 0.3333333333333333703, 0.3219752754296894559, 0.3333333333333333703, 0.3219752754296894559, 0.3333333333333333703, 0.3219752754296894559, 0.3333333333333333703, 0.3219752754296894559, 0.3333333333333333703, 0.3219752754296894559, 0.3333333333333333703, 0.3219752754296894559, 0.3333333333333333703, 0.3219752754296894559, 0.3333333333333333703, 0.3219752754296894559, 0.3333333333333333703, 0.3219752754296894559, 0.3333333333333333703, 0.3219752754296894559, 0.3333333333333333703, 0.3219752754296894559, 0.3333333333333333703, 0.3219752754296894559, 0.3333333333333333703, 0.3219752754296894559, 0.3333333333333333703, 0.3219752754296894559, 0.3333333333333333703, 0.3219752754296894559, 0.3333333333333333703, 0.3219752754296894559, 0.3333333333333333703, 0.3219752754296894559, 0.3333333333333333703, 0.3219752754296894559, 0.3333333333333333703, 0.3219752754296894559, 0.3333333333333333703, 0.3219752754296894559, 0.3333333333333333703, 0.3219752754296894559, 0.3333333333333333703, 0.3219752754296894559, 0.3333333333333333703, 0.3219752754296894559, 0.3333333333333333703, 0.3219752754296894559, 0.3333333333333333703, 0.3219752754296894559, 0.3333333333333333703, 0.3219752754296894559, 0.3333333333333333703, 0.3219752754296894559, 0.3333333333333333703, 0.3219752754296894559, 0.3333333333333333703, 0.3219752754296894559, 0.3333333333333333703, 0.3219752754296894559, 0.3333333333333333703, 0.3219752754296894559, 0.3333333333333333703, 0.3219752754296894559, 0.3333333333333333703, 0.3219752754296894559, 0.3333333333333333703, 0.3219752754296894559, 0.3333333333333333703, 0.3219752754296894559, 0.3333333333333333703, 0.3219752754296894559, 0.3333333333333333703, 0.3219752754296894559, 0.3333333333333333703, 0.3219752754296894559, 0.3333333333333333703, 0.3219752754296894559, 0.3333333333333333703, 0.3219752754296894559, 0.3333333333333333703, 0.3219752754296894559, 0.3333333333333333703, 0.3219752754296894559, 0.3333333333333333703, 0.3219752754296894559, 0.3333333333333333703, 0.3219752754296894559, 0.3333333333333333703, 0.3219752754296894559, 0.3333333333333333703, 0.3219752754296894559, 0.3333333333333333703, 0.3219752754296894559, 0.3333333333333333703, 0.3219752754296894559, 0.3333333333333333703, 0.3219752754296894559, 0.3333333333333333703, 0.3219752754296894559, 0.3333333333333333703, 0.3219752754296894559, 0.3333333333333333703, 0.3219752754296894559, 0.3333333333333333703, 0.3219752754296894559, 0.3333333333333333703, 0.3219752754296894559, 0.3333333333333333703, 0.3219752754296894559, 0.3333333333333333703, 0.3219752754296894559, 0.3333333333333333703, 0.3219752754296894559, 0.3333333333333333703, 0.3219752754296894559, 0.3333333333333333703, 0.3219752754296894559, 0.3333333333333333703, 0.3219752754296894559, 0.3333333333333333703, 0.3219752754296894559, 0.3333333333333333703, 0.3219752754296894559, 0.3333333333333333703, 0.3219752754296894559, 0.3333333333333333703, 0.3219752754296894559, 0.3333333333333333703, 0.3219752754296894559, 0.3333333333333333703, 0.3219752754296894559, 0.3333333333333333703, 0.3219752754296894559, 0.3333333333333333703, 0.3219752754296894559, 0.3333333333333333703, 0.3219752754296894559, 0.3333333333333333703, 0.3219752754296894559, 0.3333333333333333703, 0.3219752754296894559, 0.3333333333333333703, 0.3219752754296894559, 0.3333333333333333703, 0.3219752754296894559, 0.3333333333333333703, 0.3219752754296894559, 0.3333333333333333703, 0.3219752754296894559, 0.3333333333333333703, 0.3219752754296894559, 0.3333333333333333703, 0.3219752754296894559, 0.3333333333333333703, 0.3219752754296894559, 0.3333333333333333703, 0.3219752754296894559, 0.3333333333333333703, 0.3219752754296894559, 0.3333333333333333703, 0.3219752754296894559, 0.3333333333333333703, 0.3219752754296894559, 0.3333333333333333703, 0.3219752754296894559, 0.3333333333333333703, 0.3219752754296894559, 0.3333333333333333703, 0.3219752754296894559, 0.3333333333333333703, 0.3219752754296894559, 0.3333333333333333703, 0.3219752754296894559, 0.3333333333333333703, 0.3219752754296894559, 0.3333333333333333703, 0.3219752754296894559, 0.3333333333333333703, 0.3219752754296894559, 0.3333333333333333703, 0.3219752754296894559, 0.3333333333333333703, 0.3219752754296894559, 0.3333333333333333703, 0.3219752754296894559, 0.3333333333333333703, 0.3219752754296894559, 0.3333333333333333703, 0.3219752754296894559, 0.3333333333333333703, 0.3219752754296894559, 0.3333333333333333703, 0.3219752754296894559, 0.3333333333333333703, 0.3219752754296894559, 0.3333333333333333703, 0.3219752754296894559, 0.3333333333333333703, 0.3219752754296894559, 0.3333333333333333703, 0.3219752754296894559, 0.3333333333333333703, 0.3219752754296894559, 0.3333333333333333703, 0.3219752754296894559, 0.3333333333333333703, 0.3219752754296894559, 0.3333333333333333703, 0.3219752754296894559, 0.3333333333333333703, 0.3219752754296894559, 0.3333333333333333703, 0.3219752754296894559, 0.3333333333333333703, 0.3219752754296894559, 0.3333333333333333703, 0.3219752754296894559, 0.3333333333333333703, 0.3219752754296894559, 0.3333333333333333703, 0.3219752754296894559, 0.3333333333333333703, 0.3219752754296894559, 0.3333333333333333703, 0.3219752754296894559, 0.3333333333333333703, 0.3219752754296894559, 0.3333333333333333703, 0.3219752754296894559, 0.3333333333333333703, 0.3219752754296894559, 0.3333333333333333703, 0.3219752754296894559, 0.3333333333333333703, 0.3219752754296894559, 0.3333333333333333703, 0.3219752754296894559, 0.3333333333333333703, 0.3219752754296894559, 0.3333333333333333703, 0.3219752754296894559, 0.3333333333333333703, 0.3219752754296894559, 0.3333333333333333703, 0.3219752754296894559, 0.3333333333333333703, 0.3219752754296894559, 0.3333333333333333703, 0.3219752754296894559, 0.3333333333333333703, 0.3219752754296894559, 0.3333333333333333703, 0.3219752754296894559, 0.3333333333333333703, 0.3219752754296894559, 0.3333333333333333703, 0.3219752754296894559, 0.3333333333333333703, 0.3219752754296894559, 0.3333333333333333703, 0.3219752754296894559, 0.3333333333333333703, 0.3219752754296894559, 0.3333333333333333703, 0.3219752754296894559, 0.3333333333333333703, 0.3219752754296894559, 0.3333333333333333703, 0.3219752754296894559, 0.3333333333333333703, 0.3219752754296894559, 0.3333333333333333703, 0.3219752754296894559, 0.3333333333333333703, 0.3219752754296894559, 0.3333333333333333703, 0.3219752754296894559, 0.3333333333333333703, 0.3219752754296894559, 0.3333333333333333703, 0.3219752754296894559, 0.3333333333333333703, 0.3219752754296894559, 0.3333333333333333703, 0.3219752754296894559, 0.3333333333333333703, 0.3219752754296894559, 0.3333333333333333703, 0.3219752754296894559, 0.3333333333333333703, 0.3219752754296894559, 0.3333333333333333703, 0.3219752754296894559, 0.3333333333333333703, 0.3219752754296894559, 0.3333333333333333703, 0.3219752754296894559, 0.3333333333333333703, 0.3219752754296894559, 0.3333333333333333703, 0.3219752754296894559, 0.3333333333333333703, 0.3219752754296894559, 0.3333333333333333703, 0.3219752754296894559, 0.3333333333333333703, 0.3219752754296894559, 0.3333333333333333703, 0.3219752754296894559, 0.3333333333333333703, 0.3219752754296894559, 0.3333333333333333703, 0.3219752754296894559, 0.3333333333333333703, 0.3219752754296894559, 0.3333333333333333703, 0.3219752754296894559, 0.3333333333333333703, 0.3219752754296894559, 0.3333333333333333703, 0.3219752754296894559, 0.3333333333333333703, 0.3219752754296894559, 0.3333333333333333703, 0.3219752754296894559, 0.3333333333333333703, 0.3219752754296894559, 0.3333333333333333703),
 ( 1.000000000000000000, 0.9659258262890683122, 1.000000000000000000, 0.9659258262890683122, 1.000000000000000000, 0.9659258262890683122, 1.000000000000000000, 0.9659258262890683122, 1.000000000000000000, 0.9659258262890683122, 1.000000000000000000, 0.9659258262890683122, 1.000000000000000000, 0.9659258262890683122, 1.000000000000000000, 0.9659258262890683122, 1.000000000000000000, 0.9659258262890683122, 1.000000000000000000, 0.9659258262890683122, 1.000000000000000000, 0.9659258262890683122, 1.000000000000000000, 0.9659258262890683122, 1.000000000000000000, 0.9659258262890683122, 1.000000000000000000, 0.9659258262890683122, 1.000000000000000000, 0.9659258262890683122, 1.000000000000000000, 0.9659258262890683122, 1.000000000000000000, 0.9659258262890683122, 1.000000000000000000, 0.9659258262890683122, 1.000000000000000000, 0.9659258262890683122, 1.000000000000000000, 0.9659258262890683122, 1.000000000000000000, 0.9659258262890683122, 1.000000000000000000, 0.9659258262890683122, 1.000000000000000000, 0.9659258262890683122, 1.000000000000000000, 0.9659258262890683122, 1.000000000000000000, 0.9659258262890683122, 1.000000000000000000, 0.9659258262890683122, 1.000000000000000000, 0.9659258262890683122, 1.000000000000000000, 0.9659258262890683122, 1.000000000000000000, 0.9659258262890683122, 1.000000000000000000, 0.9659258262890683122, 1.000000000000000000, 0.9659258262890683122, 1.000000000000000000, 0.9659258262890683122, 1.000000000000000000, 0.9659258262890683122, 1.000000000000000000, 0.9659258262890683122, 1.000000000000000000, 0.9659258262890683122, 1.000000000000000000, 0.9659258262890683122, 1.000000000000000000, 0.9659258262890683122, 1.000000000000000000, 0.9659258262890683122, 1.000000000000000000, 0.9659258262890683122, 1.000000000000000000, 0.9659258262890683122, 1.000000000000000000, 0.9659258262890683122, 1.000000000000000000, 0.9659258262890683122, 1.000000000000000000, 0.9659258262890683122, 1.000000000000000000, 0.9659258262890683122, 1.000000000000000000, 0.9659258262890683122, 1.000000000000000000, 0.9659258262890683122, 1.000000000000000000, 0.9659258262890683122, 1.000000000000000000, 0.9659258262890683122, 1.000000000000000000, 0.9659258262890683122, 1.000000000000000000, 0.9659258262890683122, 1.000000000000000000, 0.9659258262890683122, 1.000000000000000000, 0.9659258262890683122, 1.000000000000000000, 0.9659258262890683122, 1.000000000000000000, 0.9659258262890683122, 1.000000000000000000, 0.9659258262890683122, 1.000000000000000000, 0.9659258262890683122, 1.000000000000000000, 0.9659258262890683122, 1.000000000000000000, 0.9659258262890683122, 1.000000000000000000, 0.9659258262890683122, 1.000000000000000000, 0.9659258262890683122, 1.000000000000000000, 0.9659258262890683122, 1.000000000000000000, 0.9659258262890683122, 1.000000000000000000, 0.9659258262890683122, 1.000000000000000000, 0.9659258262890683122, 1.000000000000000000, 0.9659258262890683122, 1.000000000000000000, 0.9659258262890683122, 1.000000000000000000, 0.9659258262890683122, 1.000000000000000000, 0.9659258262890683122, 1.000000000000000000, 0.9659258262890683122, 1.000000000000000000, 0.9659258262890683122, 1.000000000000000000, 0.9659258262890683122, 1.000000000000000000, 0.9659258262890683122, 1.000000000000000000, 0.9659258262890683122, 1.000000000000000000, 0.9659258262890683122, 1.000000000000000000, 0.9659258262890683122, 1.000000000000000000, 0.9659258262890683122, 1.000000000000000000, 0.9659258262890683122, 1.000000000000000000, 0.9659258262890683122, 1.000000000000000000, 0.9659258262890683122, 1.000000000000000000, 0.9659258262890683122, 1.000000000000000000, 0.9659258262890683122, 1.000000000000000000, 0.9659258262890683122, 1.000000000000000000, 0.9659258262890683122, 1.000000000000000000, 0.9659258262890683122, 1.000000000000000000, 0.9659258262890683122, 1.000000000000000000, 0.9659258262890683122, 1.000000000000000000, 0.9659258262890683122, 1.000000000000000000, 0.9659258262890683122, 1.000000000000000000, 0.9659258262890683122, 1.000000000000000000, 0.9659258262890683122, 1.000000000000000000, 0.9659258262890683122, 1.000000000000000000, 0.9659258262890683122, 1.000000000000000000, 0.9659258262890683122, 1.000000000000000000, 0.9659258262890683122, 1.000000000000000000, 0.9659258262890683122, 1.000000000000000000, 0.9659258262890683122, 1.000000000000000000, 0.9659258262890683122, 1.000000000000000000, 0.9659258262890683122, 1.000000000000000000, 0.9659258262890683122, 1.000000000000000000, 0.9659258262890683122, 1.000000000000000000, 0.9659258262890683122, 1.000000000000000000, 0.9659258262890683122, 1.000000000000000000, 0.9659258262890683122, 1.000000000000000000, 0.9659258262890683122, 1.000000000000000000, 0.9659258262890683122, 1.000000000000000000, 0.9659258262890683122, 1.000000000000000000, 0.9659258262890683122, 1.000000000000000000, 0.9659258262890683122, 1.000000000000000000, 0.9659258262890683122, 1.000000000000000000, 0.9659258262890683122, 1.000000000000000000, 0.9659258262890683122, 1.000000000000000000, 0.9659258262890683122, 1.000000000000000000, 0.9659258262890683122, 1.000000000000000000, 0.9659258262890683122, 1.000000000000000000, 0.9659258262890683122, 1.000000000000000000, 0.9659258262890683122, 1.000000000000000000, 0.9659258262890683122, 1.000000000000000000, 0.9659258262890683122, 1.000000000000000000, 0.9659258262890683122, 1.000000000000000000, 0.9659258262890683122, 1.000000000000000000, 0.9659258262890683122, 1.000000000000000000, 0.9659258262890683122, 1.000000000000000000, 0.9659258262890683122, 1.000000000000000000, 0.9659258262890683122, 1.000000000000000000, 0.9659258262890683122, 1.000000000000000000, 0.9659258262890683122, 1.000000000000000000, 0.9659258262890683122, 1.000000000000000000, 0.9659258262890683122, 1.000000000000000000, 0.9659258262890683122, 1.000000000000000000, 0.9659258262890683122, 1.000000000000000000, 0.9659258262890683122, 1.000000000000000000, 0.9659258262890683122, 1.000000000000000000, 0.9659258262890683122, 1.000000000000000000, 0.9659258262890683122, 1.000000000000000000, 0.9659258262890683122, 1.000000000000000000, 0.9659258262890683122, 1.000000000000000000, 0.9659258262890683122, 1.000000000000000000, 0.9659258262890683122, 1.000000000000000000, 0.9659258262890683122, 1.000000000000000000, 0.9659258262890683122, 1.000000000000000000, 0.9659258262890683122, 1.000000000000000000, 0.9659258262890683122, 1.000000000000000000, 0.9659258262890683122, 1.000000000000000000, 0.9659258262890683122, 1.000000000000000000, 0.9659258262890683122, 1.000000000000000000, 0.9659258262890683122, 1.000000000000000000, 0.9659258262890683122, 1.000000000000000000, 0.9659258262890683122, 1.000000000000000000, 0.9659258262890683122, 1.000000000000000000, 0.9659258262890683122, 1.000000000000000000, 0.9659258262890683122, 1.000000000000000000, 0.9659258262890683122, 1.000000000000000000, 0.9659258262890683122, 1.000000000000000000, 0.9659258262890683122, 1.000000000000000000, 0.9659258262890683122, 1.000000000000000000, 0.9659258262890683122, 1.000000000000000000, 0.9659258262890683122, 1.000000000000000000, 0.9659258262890683122, 1.000000000000000000, 0.9659258262890683122, 1.000000000000000000, 0.9659258262890683122, 1.000000000000000000, 0.9659258262890683122, 1.000000000000000000, 0.9659258262890683122, 1.000000000000000000, 0.9659258262890683122, 1.000000000000000000, 0.9659258262890683122, 1.000000000000000000, 0.9659258262890683122, 1.000000000000000000, 0.9659258262890683122, 1.000000000000000000, 0.9659258262890683122, 1.000000000000000000, 0.9659258262890683122, 1.000000000000000000, 0.9659258262890683122, 1.000000000000000000, 0.9659258262890683122, 1.000000000000000000, 0.9659258262890683122, 1.000000000000000000, 0.9659258262890683122, 1.000000000000000000, 0.9659258262890683122, 1.000000000000000000, 0.9659258262890683122, 1.000000000000000000, 0.9659258262890683122, 1.000000000000000000, 0.9659258262890683122, 1.000000000000000000, 0.9659258262890683122, 1.000000000000000000, 0.9659258262890683122, 1.000000000000000000, 0.9659258262890683122, 1.000000000000000000, 0.9659258262890683122, 1.000000000000000000, 0.9659258262890683122, 1.000000000000000000, 0.9659258262890683122, 1.000000000000000000, 0.9659258262890683122, 1.000000000000000000, 0.9659258262890683122, 1.000000000000000000, 0.9659258262890683122, 1.000000000000000000, 0.9659258262890683122, 1.000000000000000000, 0.9659258262890683122, 1.000000000000000000, 0.9659258262890683122, 1.000000000000000000, 0.9659258262890683122, 1.000000000000000000, 0.9659258262890683122, 1.000000000000000000, 0.9659258262890683122, 1.000000000000000000, 0.9659258262890683122, 1.000000000000000000, 0.9659258262890683122, 1.000000000000000000, 0.9659258262890683122, 1.000000000000000000, 0.9659258262890683122, 1.000000000000000000, 0.9659258262890683122, 1.000000000000000000, 0.9659258262890683122, 1.000000000000000000, 0.9659258262890683122, 1.000000000000000000, 0.9659258262890683122, 1.000000000000000000, 0.9659258262890683122, 1.000000000000000000, 0.9659258262890683122, 1.000000000000000000, 0.9659258262890683122, 1.000000000000000000, 0.9659258262890683122, 1.000000000000000000, 0.9659258262890683122, 1.000000000000000000, 0.9659258262890683122, 1.000000000000000000, 0.9659258262890683122, 1.000000000000000000, 0.9659258262890683122, 1.000000000000000000, 0.9659258262890683122, 1.000000000000000000, 0.9659258262890683122, 1.000000000000000000, 0.9659258262890683122, 1.000000000000000000, 0.9659258262890683122, 1.000000000000000000, 0.9659258262890683122, 1.000000000000000000, 0.9659258262890683122, 1.000000000000000000, 0.9659258262890683122, 1.000000000000000000, 0.9659258262890683122, 1.000000000000000000, 0.9659258262890683122, 1.000000000000000000, 0.9659258262890683122, 1.000000000000000000, 0.9659258262890683122, 1.000000000000000000, 0.9659258262890683122, 1.000000000000000000, 0.9659258262890683122, 1.000000000000000000, 0.9659258262890683122, 1.000000000000000000, 0.9659258262890683122, 1.000000000000000000, 0.9659258262890683122, 1.000000000000000000, 0.9659258262890683122, 1.000000000000000000, 0.9659258262890683122, 1.000000000000000000, 0.9659258262890683122, 1.000000000000000000, 0.9659258262890683122, 1.000000000000000000, 0.9659258262890683122, 1.000000000000000000) ) ) 
 REPRESENTATION_ITEM ( '' )  SURFACE ( )  );
#4192=CARTESIAN_POINT ( 'NONE',  ( -16.51473224551082808, 9.474510206698731452, 28.33442372801900433 ) ) ;
#4194=CARTESIAN_POINT ( 'NONE',  ( -13.97604488694527625, -13.89961937509977652, 51.87390960531436690 ) ) ;
#4195=CARTESIAN_POINT ( 'NONE',  ( 19.02544592524343514, -5.153800228976328945, 68.54057627198103830 ) ) ;
#4196=CARTESIAN_POINT ( 'NONE',  ( 8.224510206698742110, 14.34966873604972548, 32.08442372801901854 ) ) ;
#4198=CARTESIAN_POINT ( 'NONE',  ( -16.79531203550645913, 7.028104445595614536, 108.7475501177955834 ) ) ;
#4199=CARTESIAN_POINT ( 'NONE',  ( 8.314922557961029526, -14.29746914071037800, 80.41775706135234714 ) ) ;
#4200=CARTESIAN_POINT ( 'NONE',  ( -4.379528057220086978, -16.55341960407618274, 64.79275706135234714 ) ) ;
#4201=CARTESIAN_POINT ( 'NONE',  ( -5.719274019375978568, 21.55341960407610458, 90.20724293864770971 ) ) ;
#4202=CARTESIAN_POINT ( 'NONE',  ( -8.314922557961024197, 14.29746914071037800, 47.91775706135234714 ) ) ;
#4203=CARTESIAN_POINT ( 'NONE',  ( -16.51473224551069308, -9.474510206698971260, 41.66557627198103120 ) ) ;
#4205=CARTESIAN_POINT ( 'NONE',  ( -21.53943276465977519, -0.05219959533937600094, 58.75109039468568994 ) ) ;
#4206=CARTESIAN_POINT ( 'NONE',  ( -13.97604488694547697, 13.89961937509957934, 68.12609039468563310 ) ) ;
#4207=CARTESIAN_POINT ( 'NONE',  ( -10.81492255796105439, 18.62759615963255655, 97.91775706135236135 ) ) ;
#4208=CARTESIAN_POINT ( 'NONE',  ( 5.049401038298161559, -19.05341960407611168, 32.70724293864768129 ) ) ;
#4210=CARTESIAN_POINT ( 'NONE',  ( -21.52544592524343514, 5.823673210054127303, 56.04057627198102409 ) ) ;
#4211=CARTESIAN_POINT ( 'NONE',  ( 5.153800228976335163, 19.02544592524342804, 99.79057627198102409 ) ) ;
#4212=CARTESIAN_POINT ( 'NONE',  ( 12.06949235617757843, -12.14591786802309237, 103.1239096053143811 ) ) ;
#4213=CARTESIAN_POINT ( 'NONE',  ( 4.379528057220092307, 16.55341960407617563, 42.29275706135235424 ) ) ;
#4214=CARTESIAN_POINT ( 'NONE',  ( -16.55341960407617563, 4.379528057220093196, 108.5427570613523756 ) ) ;
#4215=VERTEX_POINT ( 'NONE', #91986 ) ;
#4216=CARTESIAN_POINT ( 'NONE',  ( 18.62759615963271287, -10.81492255796078972, 108.3322429386477097 ) ) ;
#4218=CARTESIAN_POINT ( 'NONE',  ( 0.05219959533910956823, 16.53943276465976808, 34.99890960531435979 ) ) ;
#4219=CARTESIAN_POINT ( 'NONE',  ( -19.02544592524342804, 5.153800228976336051, 111.0405762719810099 ) ) ;
#4220=CARTESIAN_POINT ( 'NONE',  ( 9.564922557961047289, -16.46253265017146816, 95.41775706135233293 ) ) ;
#4221=CARTESIAN_POINT ( 'NONE',  ( -0.05219959533936034679, 19.03943276465977164, 22.50109039468566152 ) ) ;
#4222=CARTESIAN_POINT ( 'NONE',  ( -8.224510206698948167, 14.34966873604960824, 25.41557627198103120 ) ) ;
#4223=CARTESIAN_POINT ( 'NONE',  ( 0.05219959533907565091, 21.53943276465977519, 94.99890960531436690 ) ) ;
#4224=CARTESIAN_POINT ( 'NONE',  ( 10.72451020669898902, -18.67979575497178502, 52.91557627198103830 ) ) ;
#4225=CARTESIAN_POINT ( 'NONE',  ( -9.474510206698964154, 16.51473224551069663, 60.41557627198102409 ) ) ;
#4226=CARTESIAN_POINT ( 'NONE',  ( -8.224510206698948167, 14.34966873604960824, 35.41557627198102409 ) ) ;
#4227=CARTESIAN_POINT ( 'NONE',  ( -5.049401038298153566, 19.05341960407611168, 85.20724293864766707 ) ) ;
#4229=CARTESIAN_POINT ( 'NONE',  ( 18.22780087662125226, -5.499999999999864997, 61.01540105326109398 ) ) ;
#4230=CARTESIAN_POINT ( 'NONE',  ( -13.89961937509957401, -13.97604488694547875, 39.37609039468566152 ) ) ;
#4231=CARTESIAN_POINT ( 'NONE',  ( -21.52544592524343514, 5.823673210054127303, 86.04057627198102409 ) ) ;
#4232=CARTESIAN_POINT ( 'NONE',  ( 4.379528057220339221, -16.55341960407611168, 97.70724293864772392 ) ) ;
#4233=CARTESIAN_POINT ( 'NONE',  ( 10.72451020669871369, 18.67979575497193778, 37.08442372801901143 ) ) ;
#4235=CARTESIAN_POINT ( 'NONE',  ( -12.06949235617739369, -12.14591786802326823, 104.3760903946856899 ) ) ;
#4236=CARTESIAN_POINT ( 'NONE',  ( 5.049401038298161559, -19.05341960407611168, 37.70724293864768839 ) ) ;
#4237=CARTESIAN_POINT ( 'NONE',  ( -16.46253265017160317, 9.564922557960807481, 85.83224293864769550 ) ) ;
#4238=CARTESIAN_POINT ( 'NONE',  ( -19.26498983726237313, 5.499999999999599432, 45.55319577422005750 ) ) ;
#4239=CARTESIAN_POINT ( 'NONE',  ( 9.564922557960805705, 16.46253265017160317, 29.58224293864769550 ) ) ;
#4240=CARTESIAN_POINT ( 'NONE',  ( 8.224510206698953496, -14.34966873604960469, 47.91557627198102409 ) ) ;
#4241=CARTESIAN_POINT ( 'NONE',  ( -5.823673210054431948, 21.52544592524334988, 67.70942372801901854 ) ) ;
#4243=CARTESIAN_POINT ( 'NONE',  ( -12.14591786802326823, 12.06949235617739902, 73.12609039468567573 ) ) ;
#4244=CARTESIAN_POINT ( 'NONE',  ( 13.97604488694527802, 13.89961937509977652, 54.37390960531435979 ) ) ;
#4245=CARTESIAN_POINT ( 'NONE',  ( -19.02544592524342804, 5.153800228976336051, 71.04057627198099567 ) ) ;
#4247=CARTESIAN_POINT ( 'NONE',  ( 21.52544592524334988, 5.823673210054432836, 106.4594237280190328 ) ) ;
#4248=CARTESIAN_POINT ( 'NONE',  ( -16.55341960407617563, 4.379528057220093196, 78.54275706135236135 ) ) ;
#4249=B_SPLINE_CURVE_WITH_KNOTS ( 'NONE', 3,
 ( #199002, #121154, #154481, #199997, #182847, #186838 ),
 .UNSPECIFIED., .F., .F.,
 ( 4, 2, 4 ),
 ( 0.003239945802372220466, 0.003620412082092073526, 0.004000878361811927020 ),
 .UNSPECIFIED. ) ;
#4250=CARTESIAN_POINT ( 'NONE',  ( -18.67979575497193778, 10.72451020669871902, 98.33442372801901854 ) ) ;
#4251=CARTESIAN_POINT ( 'NONE',  ( -13.97604488694527625, -13.89961937509977652, 56.87390960531434558 ) ) ;
#4252=CARTESIAN_POINT ( 'NONE',  ( 21.53943276465977519, -0.05219959533907433946, 33.74890960531436690 ) ) ;
#4253=CARTESIAN_POINT ( 'NONE',  ( 5.153800228976615827, -19.02544592524334988, 110.2094237280189901 ) ) ;
#4254=CARTESIAN_POINT ( 'NONE',  ( -18.62759615963255300, -10.81492255796106328, 69.16775706135234714 ) ) ;
#4255=CARTESIAN_POINT ( 'NONE',  ( -16.52544592524335698, -4.483927247898792601, 48.95942372801902565 ) ) ;
#4256=CARTESIAN_POINT ( 'NONE',  ( 21.55341960407610458, 5.719274019375980345, 98.95724293864770971 ) ) ;
#4257=CARTESIAN_POINT ( 'NONE',  ( -9.564922557961040184, 16.46253265017147172, 92.91775706135233293 ) ) ;
#4258=CARTESIAN_POINT ( 'NONE',  ( -5.049401038298153566, 19.05341960407611168, 75.20724293864769550 ) ) ;
#4259=CARTESIAN_POINT ( 'NONE',  ( -19.05341960407617563, 5.049401038297882671, 103.5427570613523329 ) ) ;
#4260=CARTESIAN_POINT ( 'NONE',  ( -19.03943276465977164, -0.05219959533935918106, 108.7510903946856615 ) ) ;
#4261=CARTESIAN_POINT ( 'NONE',  ( -16.55341960407611168, -4.379528057220339221, 61.45724293864770260 ) ) ;
#4262=CARTESIAN_POINT ( 'NONE',  ( -0.05219959533934338120, 16.53943276465976808, 77.50109039468567573 ) ) ;
#4263=CARTESIAN_POINT ( 'NONE',  ( -5.719274019375978568, 21.55341960407610458, 115.2072429386476955 ) ) ;
#4264=CARTESIAN_POINT ( 'NONE',  ( 16.46253265017160672, -9.564922557960803928, 48.33224293864769550 ) ) ;
#4265=CARTESIAN_POINT ( 'NONE',  ( 5.153800228976335163, 19.02544592524342804, 59.79057627198100988 ) ) ;
#4266=CARTESIAN_POINT ( 'NONE',  ( 0.05219959533934541429, -16.53943276465976808, 75.00109039468568994 ) ) ;
#4267=ADVANCED_FACE ( 'NONE', ( #27388 ), #85950, .T. ) ;
#4270=CARTESIAN_POINT ( 'NONE',  ( 19.03943276465977164, 0.05219959533936151252, 21.25109039468565797 ) ) ;
#4271=CARTESIAN_POINT ( 'NONE',  ( 5.049401038298161559, -19.05341960407611168, 22.70724293864769194 ) ) ;
#4272=CARTESIAN_POINT ( 'NONE',  ( 14.29746914071037800, 8.314922557961029526, 21.66775706135235069 ) ) ;
#4273=CARTESIAN_POINT ( 'NONE',  ( 19.05341960407617918, -5.049401038297876454, 46.04275706135233293 ) ) ;
#4274=CARTESIAN_POINT ( 'NONE',  ( -16.55341960407617563, 4.379528057220093196, 23.54275706135235424 ) ) ;
#4275=CARTESIAN_POINT ( 'NONE',  ( -0.05219959533909027116, -19.03943276465977164, 37.49890960531436690 ) ) ;
#4276=B_SPLINE_CURVE_WITH_KNOTS ( 'NONE', 3,
 ( #133701, #28535, #45665, #168015, #199353, #10371, #13345, #135705, #165048, #30493, #148880, #59830, #12371, #73044, #137666, #90171, #72028, #26541, #182199, #103370, #29511, #121500, #91145, #60818, #75009, #195393, #151854, #197376, #122492, #89185, #104360, #149869 ),
 .UNSPECIFIED., .F., .F.,
 ( 4, 2, 2, 2, 2, 2, 2, 2, 2, 2, 2, 2, 2, 2, 2, 4 ),
 ( 2.453269466693398313E-17, 0.0003712461730037028783, 0.0007424923460073811453, 0.001113738519011059358, 0.001484984692014737788, 0.002227477038022087925, 0.002598723211025748790, 0.002969969384029409656, 0.003341215557033070088, 0.003712461730036730519, 0.004083707903040390517, 0.004454954076044050949, 0.004826200249047711381, 0.005197446422051372680, 0.005568692595055032245, 0.005939938768058692677 ),
 .UNSPECIFIED. ) ;
#4277=CARTESIAN_POINT ( 'NONE',  ( 5.153800228976335163, 19.02544592524342804, 59.79057627198100988 ) ) ;
#4278=CARTESIAN_POINT ( 'NONE',  ( -18.62759615963270932, 10.81492255796079327, 85.83224293864768129 ) ) ;
#4279=CARTESIAN_POINT ( 'NONE',  ( 5.153800228976335163, 19.02544592524342804, 114.7905762719810241 ) ) ;
#4280=CARTESIAN_POINT ( 'NONE',  ( -16.51473224551069308, -9.474510206698971260, 46.66557627198102409 ) ) ;
#4282=CARTESIAN_POINT ( 'NONE',  ( 13.89961937509957401, 13.97604488694547697, 101.8760903946856331 ) ) ;
#4283=CARTESIAN_POINT ( 'NONE',  ( -16.55341960407611168, -4.379528057220339221, 66.45724293864768129 ) ) ;
#4284=CARTESIAN_POINT ( 'NONE',  ( 13.97604488694548053, -13.89961937509957401, 20.62609039468567573 ) ) ;
#4285=CARTESIAN_POINT ( 'NONE',  ( -16.53943276465976808, 0.05219959533911058130, 61.24890960531435979 ) ) ;
#4286=CARTESIAN_POINT ( 'NONE',  ( 0.05219959533937995610, -21.53943276465977519, 90.00109039468567573 ) ) ;
#4287=CARTESIAN_POINT ( 'NONE',  ( 13.89961937509977652, -13.97604488694527269, 28.12390960531435624 ) ) ;
#4288=CARTESIAN_POINT ( 'NONE',  ( -0.05219959533937732626, 21.53943276465977519, 97.50109039468567573 ) ) ;
#4289=CARTESIAN_POINT ( 'NONE',  ( 14.29746914071049879, -8.314922557960816363, 23.33224293864769194 ) ) ;
#4290=CARTESIAN_POINT ( 'NONE',  ( 10.81492255796106328, -18.62759615963255655, 70.41775706135236135 ) ) ;
#4291=CARTESIAN_POINT ( 'NONE',  ( -19.02544592524342804, 5.153800228976336051, 86.04057627198103830 ) ) ;
#4292=CARTESIAN_POINT ( 'NONE',  ( -21.55341960407619339, 5.719274019375674811, 48.54275706135234714 ) ) ;
#4293=CARTESIAN_POINT ( 'NONE',  ( -16.51473224551069308, -9.474510206698971260, 81.66557627198103830 ) ) ;
#4294=CARTESIAN_POINT ( 'NONE',  ( 14.34966873604960469, 8.224510206698951720, 94.16557627198103830 ) ) ;
#4295=CARTESIAN_POINT ( 'NONE',  ( -16.53943276465976808, 0.05219959533911058130, 56.24890960531436690 ) ) ;
#4296=CARTESIAN_POINT ( 'NONE',  ( -21.53943276465977519, 0.05219959533907696930, 66.24890960531436690 ) ) ;
#4297=CARTESIAN_POINT ( 'NONE',  ( 16.51473224551069308, 9.474510206698969483, 74.16557627198103830 ) ) ;
#4298=CARTESIAN_POINT ( 'NONE',  ( 0.05219959533907565091, 21.53943276465977519, 79.99890960531435269 ) ) ;
#4299=CARTESIAN_POINT ( 'NONE',  ( -16.46253265017146816, -9.564922557961047289, 64.16775706135233293 ) ) ;
#4300=CARTESIAN_POINT ( 'NONE',  ( -13.97604488694547520, 13.89961937509957934, 28.12609039468566152 ) ) ;
#4301=CARTESIAN_POINT ( 'NONE',  ( -8.314922557960811034, -14.29746914071050412, 72.08224293864769550 ) ) ;
#4302=CARTESIAN_POINT ( 'NONE',  ( 15.72974639402199770, -15.80617190586745480, 48.12390960531436690 ) ) ;
#4304=CARTESIAN_POINT ( 'NONE',  ( -4.379528057220086978, -16.55341960407618274, 99.79275706135234714 ) ) ;
#4306=CARTESIAN_POINT ( 'NONE',  ( 9.474510206698729675, 16.51473224551082808, 97.08442372801900433 ) ) ;
#4307=CARTESIAN_POINT ( 'NONE',  ( 14.34966873604960469, 8.224510206698951720, 64.16557627198102409 ) ) ;
#4308=CARTESIAN_POINT ( 'NONE',  ( -17.50000000000001776, 3.305555262949595452, 34.62517152156593170 ) ) ;
#4309=CARTESIAN_POINT ( 'NONE',  ( 0.05219959533909260263, 19.03943276465977164, 54.99890960531435979 ) ) ;
#4310=CARTESIAN_POINT ( 'NONE',  ( 14.29746914071049879, -8.314922557960816363, 53.33224293864769550 ) ) ;
#4311=CARTESIAN_POINT ( 'NONE',  ( 9.564922557960805705, 16.46253265017160317, 99.58224293864770971 ) ) ;
#4312=CARTESIAN_POINT ( 'NONE',  ( 19.02544592524334988, 5.153800228976608722, 81.45942372801897591 ) ) ;
#4313=CARTESIAN_POINT ( 'NONE',  ( -13.89961937509977652, 13.97604488694528158, 70.62390960531432427 ) ) ;
#4314=CARTESIAN_POINT ( 'NONE',  ( -13.97604488694527625, -13.89961937509977652, 91.87390960531432427 ) ) ;
#4315=CARTESIAN_POINT ( 'NONE',  ( -16.46253265017160317, 9.564922557960807481, 80.83224293864769550 ) ) ;
#4316=CARTESIAN_POINT ( 'NONE',  ( 5.719274019375991003, -21.55341960407610458, 67.70724293864769550 ) ) ;
#4317=CARTESIAN_POINT ( 'NONE',  ( -4.379528057220086978, -16.55341960407618274, 54.79275706135235424 ) ) ;
#4319=CARTESIAN_POINT ( 'NONE',  ( -19.05341960407611168, -5.049401038298163336, 46.45724293864768129 ) ) ;
#4320=CARTESIAN_POINT ( 'NONE',  ( 5.719274019375991003, -21.55341960407610458, 52.70724293864769550 ) ) ;
#4321=CARTESIAN_POINT ( 'NONE',  ( -9.474510206698720793, -16.51473224551083518, 99.58442372801900433 ) ) ;
#4322=CARTESIAN_POINT ( 'NONE',  ( -4.379528057220328563, 16.55341960407611168, 30.20724293864769550 ) ) ;
#4323=CARTESIAN_POINT ( 'NONE',  ( 18.62759615963255655, 10.81492255796105972, 46.66775706135234714 ) ) ;
#4324=CARTESIAN_POINT ( 'NONE',  ( 5.049401038297881783, 19.05341960407617563, 37.29275706135232582 ) ) ;
#4325=CARTESIAN_POINT ( 'NONE',  ( -12.06949235617739369, -12.14591786802326823, 54.37609039468568994 ) ) ;
#4326=CARTESIAN_POINT ( 'NONE',  ( -16.53943276465976808, -0.05219959533934237506, 93.75109039468567573 ) ) ;
#4327=CARTESIAN_POINT ( 'NONE',  ( 18.87580814761073711, -5.500000000000038192, 43.37172394265759579 ) ) ;
#4328=CARTESIAN_POINT ( 'NONE',  ( 12.14591786802327356, -12.06949235617739191, 75.62609039468567573 ) ) ;
#4329=CARTESIAN_POINT ( 'NONE',  ( 8.224510206698742110, 14.34966873604972548, 32.08442372801901854 ) ) ;
#4330=CARTESIAN_POINT ( 'NONE',  ( -9.564922557960796823, -16.46253265017161027, 42.08224293864769550 ) ) ;
#4331=CARTESIAN_POINT ( 'NONE',  ( 9.474510206698971260, -16.51473224551069308, 52.91557627198102409 ) ) ;
#4332=CARTESIAN_POINT ( 'NONE',  ( -16.51473224551069308, -9.474510206698971260, 61.66557627198103120 ) ) ;
#4333=CARTESIAN_POINT ( 'NONE',  ( -15.72974639402176322, -15.80617190586768395, 54.37609039468568994 ) ) ;
#4334=CARTESIAN_POINT ( 'NONE',  ( 4.483927247898790824, -16.52544592524335698, 50.20942372801901854 ) ) ;
#4335=CARTESIAN_POINT ( 'NONE',  ( -8.314922557961024197, 14.29746914071037800, 112.9177570613523329 ) ) ;
#4336=CARTESIAN_POINT ( 'NONE',  ( -0.05219959533909027116, -19.03943276465977164, 22.49890960531436690 ) ) ;
#4337=CARTESIAN_POINT ( 'NONE',  ( -9.474510206698720793, -16.51473224551083518, 19.58442372801899722 ) ) ;
#4338=CARTESIAN_POINT ( 'NONE',  ( 9.474510206698729675, 16.51473224551082808, 112.0844237280190043 ) ) ;
#4339=CARTESIAN_POINT ( 'NONE',  ( -13.89961937509957401, -13.97604488694547875, 69.37609039468564731 ) ) ;
#4340=CARTESIAN_POINT ( 'NONE',  ( -12.14591786802309592, -12.06949235617757132, 81.87390960531435269 ) ) ;
#4341=CARTESIAN_POINT ( 'NONE',  ( 0.05219959533909260263, 19.03943276465977164, 39.99890960531436690 ) ) ;
#4342=CARTESIAN_POINT ( 'NONE',  ( 16.46253265017146816, 9.564922557961045513, 76.66775706135234714 ) ) ;
#4344=CARTESIAN_POINT ( 'NONE',  ( -10.81492255796105439, 18.62759615963255655, 82.91775706135234714 ) ) ;
#4345=CARTESIAN_POINT ( 'NONE',  ( 8.314922557961029526, -14.29746914071037800, 35.41775706135234003 ) ) ;
#4346=CARTESIAN_POINT ( 'NONE',  ( -17.50000000000000711, 4.049696124445808287, 24.18039670665952201 ) ) ;
#4347=CARTESIAN_POINT ( 'NONE',  ( -10.72451020669898014, 18.67979575497178502, 40.41557627198103120 ) ) ;
#4348=CARTESIAN_POINT ( 'NONE',  ( -4.379528057220086978, -16.55341960407618274, 24.79275706135235779 ) ) ;
#4349=CARTESIAN_POINT ( 'NONE',  ( 9.564922557960805705, 16.46253265017160317, 29.58224293864769550 ) ) ;
#4350=CARTESIAN_POINT ( 'NONE',  ( -19.03943276465977164, -0.05219959533935918106, 33.75109039468566863 ) ) ;
#4352=CARTESIAN_POINT ( 'NONE',  ( -5.049401038298153566, 19.05341960407611168, 35.20724293864768839 ) ) ;
#4354=CARTESIAN_POINT ( 'NONE',  ( 0.05219959533909260263, 19.03943276465977164, 64.99890960531436690 ) ) ;
#4355=CARTESIAN_POINT ( 'NONE',  ( 17.50000000000000355, -3.345213924137376171, 112.0876862309434756 ) ) ;
#4356=CARTESIAN_POINT ( 'NONE',  ( -21.52544592524334988, -5.823673210054445271, 108.9594237280190185 ) ) ;
#4357=CARTESIAN_POINT ( 'NONE',  ( 14.29746914071049879, -8.314922557960816363, 33.33224293864769550 ) ) ;
#4358=CARTESIAN_POINT ( 'NONE',  ( 9.474510206698971260, -16.51473224551069308, 47.91557627198102409 ) ) ;
#4360=CARTESIAN_POINT ( 'NONE',  ( -5.049401038298153566, 19.05341960407611168, 90.20724293864766707 ) ) ;
#4361=CARTESIAN_POINT ( 'NONE',  ( -5.823673210054431948, 21.52544592524334988, 67.70942372801901854 ) ) ;
#4362=CARTESIAN_POINT ( 'NONE',  ( 16.51473224551069308, 9.474510206698969483, 49.16557627198102409 ) ) ;
#4364=CARTESIAN_POINT ( 'NONE',  ( -15.72974639402176322, -15.80617190586768395, 69.37609039468567573 ) ) ;
#4365=CARTESIAN_POINT ( 'NONE',  ( 15.80617190586746368, 15.72974639402197994, 24.37390960531435979 ) ) ;
#4366=CARTESIAN_POINT ( 'NONE',  ( 13.97604488694527802, 13.89961937509977652, 34.37390960531436690 ) ) ;
#4367=CARTESIAN_POINT ( 'NONE',  ( 5.823673210054125526, 21.52544592524343514, 114.7905762719810383 ) ) ;
#4368=CARTESIAN_POINT ( 'NONE',  ( 19.05341960407617918, -5.049401038297876454, 31.04275706135232227 ) ) ;
#4369=CARTESIAN_POINT ( 'NONE',  ( -0.05219959533910754901, -16.53943276465976808, 107.4989096053143669 ) ) ;
#4370=CARTESIAN_POINT ( 'NONE',  ( -13.97604488694527625, -13.89961937509977652, 66.87390960531436690 ) ) ;
#4371=CARTESIAN_POINT ( 'NONE',  ( -16.52544592524335698, -4.483927247898792601, 18.95942372801901143 ) ) ;
#4372=CARTESIAN_POINT ( 'NONE',  ( 8.314922557960818139, 14.29746914071049879, 74.58224293864768129 ) ) ;
#4373=CARTESIAN_POINT ( 'NONE',  ( -21.53943276465977519, 0.05219959533907696930, 26.24890960531435624 ) ) ;
#4374=CARTESIAN_POINT ( 'NONE',  ( 16.46253265017146816, 9.564922557961045513, 86.66775706135233293 ) ) ;
#4375=CARTESIAN_POINT ( 'NONE',  ( -18.67979575497178146, -10.72451020669898902, 111.6655762719810525 ) ) ;
#4376=CARTESIAN_POINT ( 'NONE',  ( 21.55341960407619695, -5.719274019375665929, 56.04275706135235424 ) ) ;
#4377=CARTESIAN_POINT ( 'NONE',  ( 14.29746914071037800, 8.314922557961029526, 61.66775706135235424 ) ) ;
#4378=CARTESIAN_POINT ( 'NONE',  ( -4.483927247898782831, 16.52544592524335698, 57.70942372801901143 ) ) ;
#4379=CARTESIAN_POINT ( 'NONE',  ( -10.81492255796078084, -18.62759615963271287, 52.08224293864768839 ) ) ;
#4380=CARTESIAN_POINT ( 'NONE',  ( -19.02544592524342804, 5.153800228976336051, 51.04057627198103120 ) ) ;
#4382=CARTESIAN_POINT ( 'NONE',  ( -0.05219959533934338120, 16.53943276465976808, 77.50109039468567573 ) ) ;
#4383=CARTESIAN_POINT ( 'NONE',  ( -18.62759615963270932, 10.81492255796079327, 100.8322429386477097 ) ) ;
#4384=CARTESIAN_POINT ( 'NONE',  ( -0.05219959533910754901, -16.53943276465976808, 52.49890960531435979 ) ) ;
#4385=CARTESIAN_POINT ( 'NONE',  ( 14.29746914071037800, 8.314922557961029526, 76.66775706135234714 ) ) ;
#4386=CARTESIAN_POINT ( 'NONE',  ( 16.51473224551083163, -9.474510206698727899, 105.8344237280190043 ) ) ;
#4387=CARTESIAN_POINT ( 'NONE',  ( 18.67979575497178502, 10.72451020669898547, 94.16557627198103830 ) ) ;
#4388=CARTESIAN_POINT ( 'NONE',  ( -0.05219959533910754901, -16.53943276465976808, 42.49890960531435979 ) ) ;
#4391=CARTESIAN_POINT ( 'NONE',  ( -16.29526858892875651, 7.335722546920117715, 69.20329402199793378 ) ) ;
#4392=CARTESIAN_POINT ( 'NONE',  ( 18.67979575497178502, 10.72451020669898547, 79.16557627198103830 ) ) ;
#4393=CARTESIAN_POINT ( 'NONE',  ( -14.34966873604972548, 8.224510206698743886, 113.3344237280190328 ) ) ;
#4395=CARTESIAN_POINT ( 'NONE',  ( -17.31728774477271671, -6.344390552232407110, 54.18093348310682700 ) ) ;
#4396=CARTESIAN_POINT ( 'NONE',  ( -18.62759615963270932, 10.81492255796079327, 95.83224293864770971 ) ) ;
#4397=CARTESIAN_POINT ( 'NONE',  ( -5.719274019375665041, -21.55341960407619695, 24.79275706135235779 ) ) ;
#4398=CARTESIAN_POINT ( 'NONE',  ( 4.483927247898545687, 16.52544592524342804, 34.79057627198103120 ) ) ;
#4399=CARTESIAN_POINT ( 'NONE',  ( -4.483927247898782831, 16.52544592524335698, 47.70942372801902565 ) ) ;
#4400=CARTESIAN_POINT ( 'NONE',  ( 19.03943276465977164, -0.05219959533909143690, 53.74890960531436690 ) ) ;
#4401=CARTESIAN_POINT ( 'NONE',  ( -13.97604488694527625, -13.89961937509977652, 81.87390960531436690 ) ) ;
#4403=CARTESIAN_POINT ( 'NONE',  ( 21.53943276465977519, -0.05219959533907433946, 28.74890960531435624 ) ) ;
#4405=CARTESIAN_POINT ( 'NONE',  ( 12.06949235617739724, 12.14591786802326823, 21.87609039468567573 ) ) ;
#4406=CARTESIAN_POINT ( 'NONE',  ( -9.474510206698720793, -16.51473224551083518, 49.58442372801899722 ) ) ;
#4407=CARTESIAN_POINT ( 'NONE',  ( 5.719274019375991003, -21.55341960407610458, 97.70724293864772392 ) ) ;
#4408=CARTESIAN_POINT ( 'NONE',  ( 0.05219959533910956823, 16.53943276465976808, 34.99890960531435979 ) ) ;
#4409=CARTESIAN_POINT ( 'NONE',  ( 0.05219959533909260263, 19.03943276465977164, 79.99890960531436690 ) ) ;
#4410=CARTESIAN_POINT ( 'NONE',  ( 5.719274019375991003, -21.55341960407610458, 57.70724293864770260 ) ) ;
#4411=CARTESIAN_POINT ( 'NONE',  ( 5.823673210054125526, 21.52544592524343514, 99.79057627198103830 ) ) ;
#4412=CARTESIAN_POINT ( 'NONE',  ( 16.55341960407618274, -4.379528057220086978, 26.04275706135235779 ) ) ;
#4413=CARTESIAN_POINT ( 'NONE',  ( 5.049401038298161559, -19.05341960407611168, 112.7072429386476813 ) ) ;
#4414=CARTESIAN_POINT ( 'NONE',  ( -15.80617190586768217, 15.72974639402176855, 83.12609039468568994 ) ) ;
#4415=CARTESIAN_POINT ( 'NONE',  ( -5.153800228976328057, -19.02544592524343514, 77.29057627198099567 ) ) ;
#4416=CARTESIAN_POINT ( 'NONE',  ( -19.03943276465977164, 0.05219959533909376836, 31.24890960531435979 ) ) ;
#4417=CARTESIAN_POINT ( 'NONE',  ( -13.97604488694527625, -13.89961937509977652, 86.87390960531436690 ) ) ;
#4418=CARTESIAN_POINT ( 'NONE',  ( 4.483927247898545687, 16.52544592524342804, 99.79057627198103830 ) ) ;
#4419=CARTESIAN_POINT ( 'NONE',  ( 5.153800228976615827, -19.02544592524334988, 110.2094237280189901 ) ) ;
#4422=CARTESIAN_POINT ( 'NONE',  ( 9.564922557960805705, 16.46253265017160317, 74.58224293864769550 ) ) ;
#4423=CARTESIAN_POINT ( 'NONE',  ( -5.719274019375665041, -21.55341960407619695, 94.79275706135234714 ) ) ;
#4424=CARTESIAN_POINT ( 'NONE',  ( -21.55341960407610458, -5.719274019375992779, 21.45724293864769550 ) ) ;
#4425=CARTESIAN_POINT ( 'NONE',  ( -4.483927247898782831, 16.52544592524335698, 92.70942372801901854 ) ) ;
#4427=CARTESIAN_POINT ( 'NONE',  ( -5.153800228976607833, 19.02544592524334988, 57.70942372801899012 ) ) ;
#4428=CARTESIAN_POINT ( 'NONE',  ( -19.05341960407617563, 5.049401038297882671, 23.54275706135233648 ) ) ;
#4429=CARTESIAN_POINT ( 'NONE',  ( -19.05341960407611168, -5.049401038298163336, 26.45724293864769550 ) ) ;
#4430=CARTESIAN_POINT ( 'NONE',  ( -16.55341960407611168, -4.379528057220339221, 26.45724293864768839 ) ) ;
#4432=CARTESIAN_POINT ( 'NONE',  ( -16.53943276465976808, -0.05219959533934237506, 108.7510903946857042 ) ) ;
#4434=CARTESIAN_POINT ( 'NONE',  ( 0.05219959533934541429, -16.53943276465976808, 80.00109039468568994 ) ) ;
#4435=CARTESIAN_POINT ( 'NONE',  ( -9.564922557960796823, -16.46253265017161027, 22.08224293864768839 ) ) ;
#4436=CARTESIAN_POINT ( 'NONE',  ( -15.72974639402176322, -15.80617190586768395, 89.37609039468568994 ) ) ;
#4437=CARTESIAN_POINT ( 'NONE',  ( 0.05219959533936267826, -19.03943276465977164, 105.0010903946856615 ) ) ;
#4438=CARTESIAN_POINT ( 'NONE',  ( -10.72451020669870658, -18.67979575497194134, 64.58442372801900433 ) ) ;
#4439=CARTESIAN_POINT ( 'NONE',  ( 0.05219959533936267826, -19.03943276465977164, 35.00109039468566863 ) ) ;
#4440=CARTESIAN_POINT ( 'NONE',  ( 0.05219959533909260263, 19.03943276465977164, 84.99890960531436690 ) ) ;
#4441=CARTESIAN_POINT ( 'NONE',  ( -16.51473224551069308, -9.474510206698971260, 76.66557627198103830 ) ) ;
#4443=CARTESIAN_POINT ( 'NONE',  ( 5.719274019375991003, -21.55341960407610458, 52.70724293864769550 ) ) ;
#4444=CARTESIAN_POINT ( 'NONE',  ( 9.474510206698971260, -16.51473224551069308, 47.91557627198102409 ) ) ;
#4445=CARTESIAN_POINT ( 'NONE',  ( -8.224510206698735004, -14.34966873604973081, 79.58442372801903275 ) ) ;
#4446=ORIENTED_EDGE ( 'NONE', *, *, #59341, .T. ) ;
#4447=CARTESIAN_POINT ( 'NONE',  ( -4.379528057220328563, 16.55341960407611168, 75.20724293864769550 ) ) ;
#4449=CARTESIAN_POINT ( 'NONE',  ( -16.52544592524335698, -4.483927247898792601, 43.95942372801902565 ) ) ;
#4450=CARTESIAN_POINT ( 'NONE',  ( -16.52544592524342804, 4.483927247898546575, 116.0405762719810383 ) ) ;
#4451=CARTESIAN_POINT ( 'NONE',  ( -0.05219959533936034679, 19.03943276465977164, 62.50109039468566863 ) ) ;
#4452=CARTESIAN_POINT ( 'NONE',  ( -14.34966873604960291, -8.224510206698953496, 71.66557627198100988 ) ) ;
#4453=CARTESIAN_POINT ( 'NONE',  ( -21.55341960407619339, 5.719274019375674811, 48.54275706135234714 ) ) ;
#4455=CYLINDRICAL_SURFACE ( 'NONE', #82707, 2.000000000000001776 ) ;
#4456=CARTESIAN_POINT ( 'NONE',  ( 21.55341960407610458, 5.719274019375980345, 88.95724293864769550 ) ) ;
#4457=CARTESIAN_POINT ( 'NONE',  ( 19.02544592524343514, -5.153800228976328945, 113.5405762719810241 ) ) ;
#4458=CARTESIAN_POINT ( 'NONE',  ( 14.34966873604960469, 8.224510206698951720, 69.16557627198102409 ) ) ;
#4460=CARTESIAN_POINT ( 'NONE',  ( 0.05219959533909260263, 19.03943276465977164, 39.99890960531436690 ) ) ;
#4462=CARTESIAN_POINT ( 'NONE',  ( 9.564922557961047289, -16.46253265017146816, 75.41775706135234714 ) ) ;
#4463=CARTESIAN_POINT ( 'NONE',  ( -10.81492255796105439, 18.62759615963255655, 22.91775706135235069 ) ) ;
#4464=CARTESIAN_POINT ( 'NONE',  ( 9.564922557960805705, 16.46253265017160317, 74.58224293864769550 ) ) ;
#4465=CARTESIAN_POINT ( 'NONE',  ( 9.564922557961047289, -16.46253265017146816, 50.41775706135233293 ) ) ;
#4466=CARTESIAN_POINT ( 'NONE',  ( -16.51473224551069308, -9.474510206698971260, 41.66557627198103120 ) ) ;
#4467=CARTESIAN_POINT ( 'NONE',  ( 14.29746914071049879, -8.314922557960816363, 58.33224293864768839 ) ) ;
#4468=CARTESIAN_POINT ( 'NONE',  ( 14.34966873604960469, 8.224510206698951720, 54.16557627198103120 ) ) ;
#4469=CARTESIAN_POINT ( 'NONE',  ( 0.05219959533909260263, 19.03943276465977164, 79.99890960531436690 ) ) ;
#4470=CARTESIAN_POINT ( 'NONE',  ( 21.55341960407610458, 5.719274019375980345, 83.95724293864770971 ) ) ;
#4471=CARTESIAN_POINT ( 'NONE',  ( -13.97604488694527625, -13.89961937509977652, 76.87390960531433848 ) ) ;
#4472=CARTESIAN_POINT ( 'NONE',  ( -0.05219959533907301413, -21.53943276465977519, 77.49890960531433848 ) ) ;
#4473=CARTESIAN_POINT ( 'NONE',  ( 5.153800228976615827, -19.02544592524334988, 20.20942372801899722 ) ) ;
#4474=CARTESIAN_POINT ( 'NONE',  ( 16.51473224551069308, 9.474510206698969483, 24.16557627198102765 ) ) ;
#4475=CARTESIAN_POINT ( 'NONE',  ( -12.14591786802326823, 12.06949235617739902, 103.1260903946856757 ) ) ;
#4476=CARTESIAN_POINT ( 'NONE',  ( 8.224510206698953496, -14.34966873604960469, 102.9155762719810383 ) ) ;
#4477=CARTESIAN_POINT ( 'NONE',  ( -19.05341960407617563, 5.049401038297882671, 108.5427570613523187 ) ) ;
#4478=ORIENTED_EDGE ( 'NONE', *, *, #588, .F. ) ;
#4479=CARTESIAN_POINT ( 'NONE',  ( 21.53943276465977519, 0.05219959533937863772, 36.25109039468567573 ) ) ;
#4480=CARTESIAN_POINT ( 'NONE',  ( -0.05219959533936034679, 19.03943276465977164, 47.50109039468566863 ) ) ;
#4481=CARTESIAN_POINT ( 'NONE',  ( 4.379528057220339221, -16.55341960407611168, 22.70724293864769194 ) ) ;
#4482=CARTESIAN_POINT ( 'NONE',  ( -18.62759615963270932, 10.81492255796079327, 70.83224293864770971 ) ) ;
#4483=CARTESIAN_POINT ( 'NONE',  ( 19.03943276465977164, -0.05219959533909143690, 103.7489096053143669 ) ) ;
#4484=CARTESIAN_POINT ( 'NONE',  ( -4.483927247898539470, -16.52544592524342804, 62.29057627198102409 ) ) ;
#4486=CARTESIAN_POINT ( 'NONE',  ( -16.51473224551069308, -9.474510206698971260, 36.66557627198102409 ) ) ;
#4487=CARTESIAN_POINT ( 'NONE',  ( -21.55341960407619339, 5.719274019375674811, 103.5427570613523613 ) ) ;
#4488=CARTESIAN_POINT ( 'NONE',  ( 14.34966873604972726, -8.224510206698740333, 85.83442372801901854 ) ) ;
#4489=CARTESIAN_POINT ( 'NONE',  ( 5.719274019375673035, 21.55341960407619339, 42.29275706135235424 ) ) ;
#4490=CARTESIAN_POINT ( 'NONE',  ( 14.34966873604972726, -8.224510206698740333, 45.83442372801901854 ) ) ;
#4491=CARTESIAN_POINT ( 'NONE',  ( 18.67979575497178502, 10.72451020669898547, 29.16557627198103120 ) ) ;
#4492=CARTESIAN_POINT ( 'NONE',  ( 0.05219959533909260263, 19.03943276465977164, 49.99890960531435979 ) ) ;
#4493=CARTESIAN_POINT ( 'NONE',  ( 0.05219959533909260263, 19.03943276465977164, 69.99890960531435269 ) ) ;
#4494=CARTESIAN_POINT ( 'NONE',  ( 14.29746914071037800, 8.314922557961029526, 56.66775706135235424 ) ) ;
#4495=CARTESIAN_POINT ( 'NONE',  ( 14.29746914071049879, -8.314922557960816363, 103.3322429386476955 ) ) ;
#4496=CARTESIAN_POINT ( 'NONE',  ( -8.224510206698735004, -14.34966873604973081, 109.5844237280190328 ) ) ;
#4498=CARTESIAN_POINT ( 'NONE',  ( 10.81492255796106328, -18.62759615963255655, 50.41775706135235424 ) ) ;
#4499=CARTESIAN_POINT ( 'NONE',  ( 0.05219959533909260263, 19.03943276465977164, 94.99890960531436690 ) ) ;
#4500=CARTESIAN_POINT ( 'NONE',  ( 16.51473224551069308, 9.474510206698969483, 84.16557627198102409 ) ) ;
#4501=CARTESIAN_POINT ( 'NONE',  ( 0.05219959533909260263, 19.03943276465977164, 99.99890960531436690 ) ) ;
#4502=CARTESIAN_POINT ( 'NONE',  ( -8.224510206698948167, 14.34966873604960824, 50.41557627198103120 ) ) ;
#4503=CARTESIAN_POINT ( 'NONE',  ( -16.55341960407617563, 4.379528057220093196, 113.5427570613523756 ) ) ;
#4505=CARTESIAN_POINT ( 'NONE',  ( -14.29746914071049879, 8.314922557960819915, 40.83224293864769550 ) ) ;
#4507=CARTESIAN_POINT ( 'NONE',  ( 13.97604488694548053, -13.89961937509957401, 40.62609039468564731 ) ) ;
#4508=CARTESIAN_POINT ( 'NONE',  ( -16.51473224551069308, -9.474510206698971260, 71.66557627198102409 ) ) ;
#4509=CARTESIAN_POINT ( 'NONE',  ( -19.02544592524334988, -5.153800228976617603, 58.95942372801900433 ) ) ;
#4512=CARTESIAN_POINT ( 'NONE',  ( 5.153800228976615827, -19.02544592524334988, 80.20942372801901854 ) ) ;
#4513=CARTESIAN_POINT ( 'NONE',  ( 16.53943276465976808, 0.05219959533934440121, 71.25109039468568994 ) ) ;
#4515=CARTESIAN_POINT ( 'NONE',  ( 9.564922557960805705, 16.46253265017160317, 104.5822429386476955 ) ) ;
#4516=CARTESIAN_POINT ( 'NONE',  ( 15.80617190586769283, -15.72974639402175789, 30.62609039468567929 ) ) ;
#4517=CARTESIAN_POINT ( 'NONE',  ( -19.02544592524334988, -5.153800228976617603, 88.95942372801897591 ) ) ;
#4518=CARTESIAN_POINT ( 'NONE',  ( 16.18388926212237067, 7.379444403734554569, 87.93953151366153520 ) ) ;
#4519=CARTESIAN_POINT ( 'NONE',  ( 19.05341960407611168, 5.049401038298154454, 48.95724293864768129 ) ) ;
#4520=CARTESIAN_POINT ( 'NONE',  ( -16.51473224551069308, -9.474510206698971260, 86.66557627198102409 ) ) ;
#4521=CARTESIAN_POINT ( 'NONE',  ( -12.06949235617756955, 12.14591786802309770, 45.62390960531436690 ) ) ;
#4522=CARTESIAN_POINT ( 'NONE',  ( 16.46253265017160672, -9.564922557960803928, 53.33224293864768839 ) ) ;
#4523=CARTESIAN_POINT ( 'NONE',  ( -0.05219959533936034679, 19.03943276465977164, 67.50109039468566152 ) ) ;
#4524=CARTESIAN_POINT ( 'NONE',  ( 16.46253265017146816, 9.564922557961045513, 26.66775706135234003 ) ) ;
#4525=CARTESIAN_POINT ( 'NONE',  ( -16.46253265017160317, 9.564922557960807481, 60.83224293864769550 ) ) ;
#4527=CARTESIAN_POINT ( 'NONE',  ( 5.823673210054125526, 21.52544592524343514, 59.79057627198103120 ) ) ;
#4528=CARTESIAN_POINT ( 'NONE',  ( 14.34966873604960469, 8.224510206698951720, 69.16557627198102409 ) ) ;
#4529=CARTESIAN_POINT ( 'NONE',  ( 5.719274019375673035, 21.55341960407619339, 112.2927570613523471 ) ) ;
#4531=CARTESIAN_POINT ( 'NONE',  ( -16.46253265017160317, 9.564922557960807481, 115.8322429386477097 ) ) ;
#4532=CARTESIAN_POINT ( 'NONE',  ( 19.02544592524343514, -5.153800228976328945, 53.54057627198102409 ) ) ;
#4533=CARTESIAN_POINT ( 'NONE',  ( -5.153800228976328057, -19.02544592524343514, 37.29057627198102409 ) ) ;
#4534=CARTESIAN_POINT ( 'NONE',  ( -14.29746914071049879, 8.314922557960819915, 100.8322429386477097 ) ) ;
#4535=CARTESIAN_POINT ( 'NONE',  ( -21.55341960407610458, -5.719274019375992779, 111.4572429386476813 ) ) ;
#4537=CARTESIAN_POINT ( 'NONE',  ( 5.823673210054444382, -21.52544592524334988, 30.20942372801902565 ) ) ;
#4538=CARTESIAN_POINT ( 'NONE',  ( -19.03943276465977164, 0.05219959533909376836, 26.24890960531435624 ) ) ;
#4539=CARTESIAN_POINT ( 'NONE',  ( -18.67979575497193778, 10.72451020669871902, 78.33442372801901854 ) ) ;
#4540=CARTESIAN_POINT ( 'NONE',  ( 15.72974639402199770, -15.80617190586745480, 93.12390960531436690 ) ) ;
#4541=CARTESIAN_POINT ( 'NONE',  ( 13.89961937509957401, 13.97604488694547697, 36.87609039468565442 ) ) ;
#4542=CARTESIAN_POINT ( 'NONE',  ( -16.51473224551069308, -9.474510206698971260, 21.66557627198102765 ) ) ;
#4545=CARTESIAN_POINT ( 'NONE',  ( -14.29746914071037622, -8.314922557961029526, 49.16775706135234003 ) ) ;
#4546=CARTESIAN_POINT ( 'NONE',  ( 4.379528057220339221, -16.55341960407611168, 102.7072429386476955 ) ) ;
#4549=CARTESIAN_POINT ( 'NONE',  ( 16.51473224551069308, 9.474510206698969483, 74.16557627198103830 ) ) ;
#4550=CARTESIAN_POINT ( 'NONE',  ( -14.34966873604960291, -8.224510206698953496, 96.66557627198102409 ) ) ;
#4551=CARTESIAN_POINT ( 'NONE',  ( -21.55341960407610458, -5.719274019375992779, 51.45724293864770260 ) ) ;
#4552=CARTESIAN_POINT ( 'NONE',  ( 14.34966873604960469, 8.224510206698951720, 69.16557627198102409 ) ) ;
#4553=CARTESIAN_POINT ( 'NONE',  ( 12.14591786802327356, -12.06949235617739191, 30.62609039468567929 ) ) ;
#4554=CARTESIAN_POINT ( 'NONE',  ( -21.53943276465977519, -0.05219959533937600094, 83.75109039468568994 ) ) ;
#4557=CARTESIAN_POINT ( 'NONE',  ( 12.06949235617739724, 12.14591786802326823, 91.87609039468568994 ) ) ;
#4558=CARTESIAN_POINT ( 'NONE',  ( 4.483927247898545687, 16.52544592524342804, 44.79057627198103120 ) ) ;
#4559=CARTESIAN_POINT ( 'NONE',  ( -19.02544592524342804, 5.153800228976336051, 36.04057627198100988 ) ) ;
#4560=CARTESIAN_POINT ( 'NONE',  ( 9.474510206698971260, -16.51473224551069308, 82.91557627198103830 ) ) ;
#4561=CARTESIAN_POINT ( 'NONE',  ( 15.80617190586746368, 15.72974639402197994, 114.3739096053143527 ) ) ;
#4562=CARTESIAN_POINT ( 'NONE',  ( 18.62759615963255655, 10.81492255796105972, 56.66775706135235424 ) ) ;
#4563=CARTESIAN_POINT ( 'NONE',  ( -8.314922557961024197, 14.29746914071037800, 37.91775706135235424 ) ) ;
#4564=CARTESIAN_POINT ( 'NONE',  ( -16.53943276465976808, 0.05219959533911058130, 61.24890960531435979 ) ) ;
#4565=CARTESIAN_POINT ( 'NONE',  ( 0.05219959533937995610, -21.53943276465977519, 85.00109039468568994 ) ) ;
#4566=CARTESIAN_POINT ( 'NONE',  ( -12.06949235617739369, -12.14591786802326823, 99.37609039468568994 ) ) ;
#4567=CARTESIAN_POINT ( 'NONE',  ( 16.18388926212245948, -7.379444403734571445, 47.06046848633767610 ) ) ;
#4568=CARTESIAN_POINT ( 'NONE',  ( -17.49999999999999645, 5.499999999999992895, 48.71769037696437010 ) ) ;
#4569=CARTESIAN_POINT ( 'NONE',  ( 12.14591786802309770, 12.06949235617756955, 34.37390960531435979 ) ) ;
#4570=CARTESIAN_POINT ( 'NONE',  ( -16.52544592524335698, -4.483927247898792601, 78.95942372801901854 ) ) ;
#4571=CARTESIAN_POINT ( 'NONE',  ( 0.05219959533909260263, 19.03943276465977164, 84.99890960531436690 ) ) ;
#4572=CARTESIAN_POINT ( 'NONE',  ( -9.564922557960796823, -16.46253265017161027, 97.08224293864769550 ) ) ;
#4573=CARTESIAN_POINT ( 'NONE',  ( -5.719274019375665041, -21.55341960407619695, 79.79275706135236135 ) ) ;
#4574=CARTESIAN_POINT ( 'NONE',  ( 16.53943276465976808, 0.05219959533934440121, 91.25109039468568994 ) ) ;
#4575=CARTESIAN_POINT ( 'NONE',  ( 16.52544592524342804, -4.483927247898539470, 58.54057627198103120 ) ) ;
#4576=CARTESIAN_POINT ( 'NONE',  ( 13.89961937509977652, -13.97604488694527269, 73.12390960531436690 ) ) ;
#4577=VERTEX_POINT ( 'NONE', #180648 ) ;
#4578=CARTESIAN_POINT ( 'NONE',  ( 14.34966873604972726, -8.224510206698740333, 25.83442372801901499 ) ) ;
#4579=CARTESIAN_POINT ( 'NONE',  ( -19.05341960407611168, -5.049401038298163336, 31.45724293864769550 ) ) ;
#4580=CARTESIAN_POINT ( 'NONE',  ( -16.51473224551069308, -9.474510206698971260, 81.66557627198103830 ) ) ;
#4581=CARTESIAN_POINT ( 'NONE',  ( -5.153800228976607833, 19.02544592524334988, 112.7094237280190043 ) ) ;
#4583=CARTESIAN_POINT ( 'NONE',  ( 16.46253265017146816, 9.564922557961045513, 21.66775706135233648 ) ) ;
#4584=CARTESIAN_POINT ( 'NONE',  ( 8.224510206698742110, 14.34966873604972548, 87.08442372801901854 ) ) ;
#4585=CARTESIAN_POINT ( 'NONE',  ( 5.153800228976615827, -19.02544592524334988, 110.2094237280189901 ) ) ;
#4586=CARTESIAN_POINT ( 'NONE',  ( 16.46253265017160672, -9.564922557960803928, 23.33224293864769194 ) ) ;
#4587=CARTESIAN_POINT ( 'NONE',  ( -16.53943276465976808, -0.05219959533934237506, 63.75109039468568284 ) ) ;
#4588=CARTESIAN_POINT ( 'NONE',  ( 16.55341960407618274, -4.379528057220086978, 56.04275706135235424 ) ) ;
#4589=CARTESIAN_POINT ( 'NONE',  ( 19.05341960407611168, 5.049401038298154454, 23.95724293864769194 ) ) ;
#4590=CARTESIAN_POINT ( 'NONE',  ( -9.474510206698720793, -16.51473224551083518, 74.58442372801900433 ) ) ;
#4591=CARTESIAN_POINT ( 'NONE',  ( -0.05219959533937732626, 21.53943276465977519, 107.5010903946856899 ) ) ;
#4592=CARTESIAN_POINT ( 'NONE',  ( -13.89961937509977652, 13.97604488694528158, 30.62390960531435269 ) ) ;
#4593=CARTESIAN_POINT ( 'NONE',  ( 9.564922557960805705, 16.46253265017160317, 84.58224293864769550 ) ) ;
#4594=CARTESIAN_POINT ( 'NONE',  ( -0.05219959533910754901, -16.53943276465976808, 77.49890960531433848 ) ) ;
#4596=CARTESIAN_POINT ( 'NONE',  ( -19.03943276465977164, -0.05219959533935918106, 38.75109039468566152 ) ) ;
#4597=CARTESIAN_POINT ( 'NONE',  ( -15.80617190586745835, -15.72974639402198527, 41.87390960531435979 ) ) ;
#4598=CARTESIAN_POINT ( 'NONE',  ( -5.049401038297874678, -19.05341960407617918, 19.79275706135233293 ) ) ;
#4599=CARTESIAN_POINT ( 'NONE',  ( 5.153800228976335163, 19.02544592524342804, 89.79057627198102409 ) ) ;
#4600=CARTESIAN_POINT ( 'NONE',  ( -21.55341960407619339, 5.719274019375674811, 103.5427570613523613 ) ) ;
#4601=CARTESIAN_POINT ( 'NONE',  ( 15.80617190586746368, 15.72974639402197994, 59.37390960531436690 ) ) ;
#4602=CARTESIAN_POINT ( 'NONE',  ( -9.564922557960796823, -16.46253265017161027, 102.0822429386477097 ) ) ;
#4603=CARTESIAN_POINT ( 'NONE',  ( -9.564922557961040184, 16.46253265017147172, 82.91775706135233293 ) ) ;
#4604=CARTESIAN_POINT ( 'NONE',  ( -13.97604488694527625, -13.89961937509977652, 101.8739096053143811 ) ) ;
#4605=CARTESIAN_POINT ( 'NONE',  ( -5.153800228976607833, 19.02544592524334988, 97.70942372801900433 ) ) ;
#4606=CARTESIAN_POINT ( 'NONE',  ( -8.224510206698948167, 14.34966873604960824, 115.4155762719810241 ) ) ;
#4607=CARTESIAN_POINT ( 'NONE',  ( 5.049401038298161559, -19.05341960407611168, 82.70724293864770971 ) ) ;
#4608=CARTESIAN_POINT ( 'NONE',  ( 21.55341960407610458, 5.719274019375980345, 63.95724293864770260 ) ) ;
#4609=CARTESIAN_POINT ( 'NONE',  ( -12.14591786802326823, 12.06949235617739902, 43.12609039468568284 ) ) ;
#4610=CARTESIAN_POINT ( 'NONE',  ( 0.05219959533937995610, -21.53943276465977519, 50.00109039468568994 ) ) ;
#4611=CARTESIAN_POINT ( 'NONE',  ( 10.81492255796106328, -18.62759615963255655, 100.4177570613523471 ) ) ;
#4612=CARTESIAN_POINT ( 'NONE',  ( 4.379528057220092307, 16.55341960407617563, 92.29275706135236135 ) ) ;
#4613=CARTESIAN_POINT ( 'NONE',  ( 9.564922557960805705, 16.46253265017160317, 89.58224293864769550 ) ) ;
#4614=CARTESIAN_POINT ( 'NONE',  ( -8.314922557960811034, -14.29746914071050412, 87.08224293864769550 ) ) ;
#4615=CARTESIAN_POINT ( 'NONE',  ( -16.52544592524342804, 4.483927247898546575, 26.04057627198103475 ) ) ;
#4616=CARTESIAN_POINT ( 'NONE',  ( -13.97604488694547697, 13.89961937509957934, 63.12609039468566152 ) ) ;
#4617=CARTESIAN_POINT ( 'NONE',  ( -10.72451020669870658, -18.67979575497194134, 39.58442372801901143 ) ) ;
#4619=CARTESIAN_POINT ( 'NONE',  ( -4.379528057220328563, 16.55341960407611168, 95.20724293864769550 ) ) ;
#4620=CARTESIAN_POINT ( 'NONE',  ( -13.97604488694527625, -13.89961937509977652, 106.8739096053143669 ) ) ;
#4621=CARTESIAN_POINT ( 'NONE',  ( 8.314922557961029526, -14.29746914071037800, 110.4177570613523756 ) ) ;
#4622=CARTESIAN_POINT ( 'NONE',  ( 21.53943276465977519, 0.05219959533937863772, 91.25109039468568994 ) ) ;
#4623=CARTESIAN_POINT ( 'NONE',  ( -14.29746914071037622, -8.314922557961029526, 64.16775706135234714 ) ) ;
#4624=CARTESIAN_POINT ( 'NONE',  ( 5.719274019375673035, 21.55341960407619339, 42.29275706135235424 ) ) ;
#4627=CARTESIAN_POINT ( 'NONE',  ( 0.05219959533937995610, -21.53943276465977519, 35.00109039468568284 ) ) ;
#4628=CARTESIAN_POINT ( 'NONE',  ( -0.05219959533910754901, -16.53943276465976808, 92.49890960531436690 ) ) ;
#4629=CARTESIAN_POINT ( 'NONE',  ( 19.05341960407611168, 5.049401038298154454, 23.95724293864769194 ) ) ;
#4630=CARTESIAN_POINT ( 'NONE',  ( 12.14591786802309770, 12.06949235617756955, 64.37390960531435269 ) ) ;
#4631=CARTESIAN_POINT ( 'NONE',  ( -5.049401038298153566, 19.05341960407611168, 60.20724293864768129 ) ) ;
#4632=CARTESIAN_POINT ( 'NONE',  ( 16.52544592524335698, 4.483927247898782831, 111.4594237280190328 ) ) ;
#4633=CARTESIAN_POINT ( 'NONE',  ( 16.46253265017160672, -9.564922557960803928, 38.33224293864768839 ) ) ;
#4634=CARTESIAN_POINT ( 'NONE',  ( 18.67979575497178502, 10.72451020669898547, 49.16557627198102409 ) ) ;
#4635=CARTESIAN_POINT ( 'NONE',  ( -16.53943276465976808, 0.05219959533911058130, 76.24890960531435269 ) ) ;
#4636=CARTESIAN_POINT ( 'NONE',  ( 18.62759615963271287, -10.81492255796078972, 88.33224293864769550 ) ) ;
#4637=CARTESIAN_POINT ( 'NONE',  ( -9.564922557960796823, -16.46253265017161027, 82.08224293864768129 ) ) ;
#4638=CARTESIAN_POINT ( 'NONE',  ( -5.049401038298153566, 19.05341960407611168, 50.20724293864770260 ) ) ;
#4639=CARTESIAN_POINT ( 'NONE',  ( 16.46253265017146816, 9.564922557961045513, 91.66775706135234714 ) ) ;
#4640=CARTESIAN_POINT ( 'NONE',  ( 18.67979575497178502, 10.72451020669898547, 44.16557627198103120 ) ) ;
#4641=CARTESIAN_POINT ( 'NONE',  ( -15.72974639402176322, -15.80617190586768395, 74.37609039468568994 ) ) ;
#4642=CARTESIAN_POINT ( 'NONE',  ( 16.46253265017160672, -9.564922557960803928, 48.33224293864769550 ) ) ;
#4643=CARTESIAN_POINT ( 'NONE',  ( 19.02544592524343514, -5.153800228976328945, 88.54057627198102409 ) ) ;
#4645=CARTESIAN_POINT ( 'NONE',  ( 12.06949235617739724, 12.14591786802326823, 61.87609039468568284 ) ) ;
#4646=CARTESIAN_POINT ( 'NONE',  ( 18.67979575497194134, -10.72451020669871369, 40.83442372801901854 ) ) ;
#4647=CARTESIAN_POINT ( 'NONE',  ( -0.05219959533937732626, 21.53943276465977519, 67.50109039468568994 ) ) ;
#4648=CARTESIAN_POINT ( 'NONE',  ( 10.72451020669898902, -18.67979575497178502, 22.91557627198102765 ) ) ;
#4649=CARTESIAN_POINT ( 'NONE',  ( -18.62759615963270932, 10.81492255796079327, 100.8322429386477097 ) ) ;
#4650=CARTESIAN_POINT ( 'NONE',  ( 15.72974639402176855, 15.80617190586768217, 31.87609039468567929 ) ) ;
#4651=CARTESIAN_POINT ( 'NONE',  ( 16.52544592524335698, 4.483927247898782831, 71.45942372801901854 ) ) ;
#4652=CARTESIAN_POINT ( 'NONE',  ( -5.719274019375978568, 21.55341960407610458, 60.20724293864768839 ) ) ;
#4653=CARTESIAN_POINT ( 'NONE',  ( 19.05341960407617918, -5.049401038297876454, 36.04275706135234003 ) ) ;
#4654=CARTESIAN_POINT ( 'NONE',  ( -16.46253265017160317, 9.564922557960807481, 65.83224293864769550 ) ) ;
#4655=CARTESIAN_POINT ( 'NONE',  ( 12.14591786802327356, -12.06949235617739191, 105.6260903946856899 ) ) ;
#4656=CARTESIAN_POINT ( 'NONE',  ( 18.22780087662123805, -5.499999999999976019, 83.51763182126894947 ) ) ;
#4657=CARTESIAN_POINT ( 'NONE',  ( -16.46253265017160317, 9.564922557960807481, 100.8322429386477097 ) ) ;
#4659=CARTESIAN_POINT ( 'NONE',  ( -0.05219959533936034679, 19.03943276465977164, 87.50109039468567573 ) ) ;
#4660=CARTESIAN_POINT ( 'NONE',  ( -15.80617190586745835, -15.72974639402198527, 51.87390960531437401 ) ) ;
#4661=CARTESIAN_POINT ( 'NONE',  ( 4.379528057220339221, -16.55341960407611168, 32.70724293864770260 ) ) ;
#4662=CARTESIAN_POINT ( 'NONE',  ( -9.474510206698720793, -16.51473224551083518, 104.5844237280190043 ) ) ;
#4664=CARTESIAN_POINT ( 'NONE',  ( -19.02544592524334988, -5.153800228976617603, 93.95942372801900433 ) ) ;
#4665=CARTESIAN_POINT ( 'NONE',  ( -10.81492255796078084, -18.62759615963271287, 82.08224293864768129 ) ) ;
#4666=CARTESIAN_POINT ( 'NONE',  ( -16.51473224551082808, 9.474510206698731452, 63.33442372801900433 ) ) ;
#4667=CARTESIAN_POINT ( 'NONE',  ( 16.55341960407618274, -4.379528057220086978, 76.04275706135237556 ) ) ;
#4668=CARTESIAN_POINT ( 'NONE',  ( 19.03943276465977164, -0.05219959533909143690, 63.74890960531435979 ) ) ;
#4669=CARTESIAN_POINT ( 'NONE',  ( 4.379528057220339221, -16.55341960407611168, 62.70724293864769550 ) ) ;
#4671=CARTESIAN_POINT ( 'NONE',  ( 9.474510206698971260, -16.51473224551069308, 52.91557627198102409 ) ) ;
#4672=CARTESIAN_POINT ( 'NONE',  ( 14.29746914071049879, -8.314922557960816363, 48.33224293864770260 ) ) ;
#4673=CARTESIAN_POINT ( 'NONE',  ( -19.05341960407611168, -5.049401038298163336, 21.45724293864768839 ) ) ;
#4675=CARTESIAN_POINT ( 'NONE',  ( 14.34966873604960469, 8.224510206698951720, 34.16557627198102409 ) ) ;
#4676=CARTESIAN_POINT ( 'NONE',  ( -0.05219959533909027116, -19.03943276465977164, 77.49890960531435269 ) ) ;
#4677=CARTESIAN_POINT ( 'NONE',  ( -18.22780087662122028, 5.500000000000031086, 73.51540105326107266 ) ) ;
#4678=CARTESIAN_POINT ( 'NONE',  ( -19.03943276465977164, -0.05219959533935918106, 43.75109039468566863 ) ) ;
#4679=CARTESIAN_POINT ( 'NONE',  ( 4.379528057220092307, 16.55341960407617563, 52.29275706135236135 ) ) ;
#4680=CARTESIAN_POINT ( 'NONE',  ( 18.67979575497178502, 10.72451020669898547, 54.16557627198103120 ) ) ;
#4681=CARTESIAN_POINT ( 'NONE',  ( 0.05219959533937995610, -21.53943276465977519, 100.0010903946857042 ) ) ;
#4682=CARTESIAN_POINT ( 'NONE',  ( 5.049401038298161559, -19.05341960407611168, 72.70724293864768129 ) ) ;
#4683=LINE ( 'NONE', #52198, #69514 ) ;
#4684=CARTESIAN_POINT ( 'NONE',  ( -13.89961937509977652, 13.97604488694528158, 105.6239096053143527 ) ) ;
#4685=CARTESIAN_POINT ( 'NONE',  ( 15.72974639402176855, 15.80617190586768217, 41.87609039468568284 ) ) ;
#4686=CARTESIAN_POINT ( 'NONE',  ( 0.05219959533910956823, 16.53943276465976808, 94.99890960531436690 ) ) ;
#4687=CARTESIAN_POINT ( 'NONE',  ( 21.52544592524344225, -5.823673210054117533, 83.54057627198102409 ) ) ;
#4688=CARTESIAN_POINT ( 'NONE',  ( -19.02544592524342804, 5.153800228976336051, 86.04057627198103830 ) ) ;
#4690=CARTESIAN_POINT ( 'NONE',  ( -21.52544592524334988, -5.823673210054445271, 28.95942372801902209 ) ) ;
#4693=CARTESIAN_POINT ( 'NONE',  ( 9.564922557960805705, 16.46253265017160317, 84.58224293864769550 ) ) ;
#4694=FACE_OUTER_BOUND ( 'NONE', #155307, .T. ) ;
#4695=CARTESIAN_POINT ( 'NONE',  ( 16.51473224551069308, 9.474510206698969483, 24.16557627198102765 ) ) ;
#4696=CARTESIAN_POINT ( 'NONE',  ( -9.564922557960796823, -16.46253265017161027, 37.08224293864768839 ) ) ;
#4697=CARTESIAN_POINT ( 'NONE',  ( -9.564922557961040184, 16.46253265017147172, 112.9177570613523329 ) ) ;
#4700=CARTESIAN_POINT ( 'NONE',  ( 14.34966873604960469, 8.224510206698951720, 109.1655762719810383 ) ) ;
#4701=CARTESIAN_POINT ( 'NONE',  ( 21.53943276465977519, 0.05219959533937863772, 91.25109039468568994 ) ) ;
#4702=CARTESIAN_POINT ( 'NONE',  ( -5.153800228976328057, -19.02544592524343514, 62.29057627198100988 ) ) ;
#4703=CARTESIAN_POINT ( 'NONE',  ( 15.72974639402176855, 15.80617190586768217, 31.87609039468567929 ) ) ;
#4704=CARTESIAN_POINT ( 'NONE',  ( 5.719274019375673035, 21.55341960407619339, 32.29275706135235424 ) ) ;
#4706=CARTESIAN_POINT ( 'NONE',  ( -5.153800228976328057, -19.02544592524343514, 87.29057627198103830 ) ) ;
#4708=CARTESIAN_POINT ( 'NONE',  ( 0.05219959533934541429, -16.53943276465976808, 25.00109039468567218 ) ) ;
#4709=CARTESIAN_POINT ( 'NONE',  ( 18.67979575497178502, 10.72451020669898547, 49.16557627198102409 ) ) ;
#4710=CARTESIAN_POINT ( 'NONE',  ( 5.719274019375673035, 21.55341960407619339, 57.29275706135234714 ) ) ;
#4712=CARTESIAN_POINT ( 'NONE',  ( 0.05219959533909260263, 19.03943276465977164, 109.9989096053143669 ) ) ;
#4713=CARTESIAN_POINT ( 'NONE',  ( -0.05219959533936034679, 19.03943276465977164, 97.50109039468567573 ) ) ;
#4714=CARTESIAN_POINT ( 'NONE',  ( -13.97604488694527625, -13.89961937509977652, 66.87390960531436690 ) ) ;
#4715=CARTESIAN_POINT ( 'NONE',  ( -16.46253265017160317, 9.564922557960807481, 90.83224293864769550 ) ) ;
#4716=CARTESIAN_POINT ( 'NONE',  ( -0.05219959533910754901, -16.53943276465976808, 92.49890960531436690 ) ) ;
#4717=CARTESIAN_POINT ( 'NONE',  ( -0.05219959533910754901, -16.53943276465976808, 107.4989096053143669 ) ) ;
#4718=CARTESIAN_POINT ( 'NONE',  ( 13.89961937509977652, -13.97604488694527269, 113.1239096053143527 ) ) ;
#4719=CARTESIAN_POINT ( 'NONE',  ( -16.55341960407611168, -4.379528057220339221, 51.45724293864770260 ) ) ;
#4720=CARTESIAN_POINT ( 'NONE',  ( -16.46253265017160317, 9.564922557960807481, 35.83224293864768839 ) ) ;
#4721=CARTESIAN_POINT ( 'NONE',  ( -10.72451020669870658, -18.67979575497194134, 74.58442372801901854 ) ) ;
#4722=CARTESIAN_POINT ( 'NONE',  ( 16.51473224551083163, -9.474510206698727899, 90.83442372801900433 ) ) ;
#4723=CARTESIAN_POINT ( 'NONE',  ( -8.224510206698948167, 14.34966873604960824, 60.41557627198102409 ) ) ;
#4724=CARTESIAN_POINT ( 'NONE',  ( -15.80617190586745835, -15.72974639402198527, 106.8739096053143811 ) ) ;
#4725=CARTESIAN_POINT ( 'NONE',  ( 15.80617190586746368, 15.72974639402197994, 44.37390960531435979 ) ) ;
#4726=CARTESIAN_POINT ( 'NONE',  ( -16.51473224551069308, -9.474510206698971260, 111.6655762719810383 ) ) ;
#4728=CARTESIAN_POINT ( 'NONE',  ( -13.89961937509977652, 13.97604488694528158, 70.62390960531432427 ) ) ;
#4729=CARTESIAN_POINT ( 'NONE',  ( 14.34966873604960469, 8.224510206698951720, 34.16557627198102409 ) ) ;
#4731=CARTESIAN_POINT ( 'NONE',  ( 16.53943276465976808, 0.05219959533934440121, 106.2510903946856757 ) ) ;
#4732=CARTESIAN_POINT ( 'NONE',  ( 16.52544592524335698, 4.483927247898782831, 86.45942372801901854 ) ) ;
#4733=CARTESIAN_POINT ( 'NONE',  ( -9.474510206698720793, -16.51473224551083518, 44.58442372801900433 ) ) ;
#4735=CARTESIAN_POINT ( 'NONE',  ( 5.049401038298161559, -19.05341960407611168, 92.70724293864769550 ) ) ;
#4736=CARTESIAN_POINT ( 'NONE',  ( 13.97604488694527802, 13.89961937509977652, 44.37390960531435269 ) ) ;
#4737=CARTESIAN_POINT ( 'NONE',  ( 14.34966873604960469, 8.224510206698951720, 59.16557627198103120 ) ) ;
#4738=CARTESIAN_POINT ( 'NONE',  ( 17.13100169013300444, -6.664070546373146442, 103.2678983569984581 ) ) ;
#4739=CARTESIAN_POINT ( 'NONE',  ( 5.719274019375991003, -21.55341960407610458, 22.70724293864769194 ) ) ;
#4740=CARTESIAN_POINT ( 'NONE',  ( 15.72974639402199770, -15.80617190586745480, 58.12390960531435979 ) ) ;
#4741=CARTESIAN_POINT ( 'NONE',  ( -16.55341960407611168, -4.379528057220339221, 81.45724293864769550 ) ) ;
#4742=CARTESIAN_POINT ( 'NONE',  ( -16.55341960407617563, 4.379528057220093196, 33.54275706135234714 ) ) ;
#4743=CARTESIAN_POINT ( 'NONE',  ( 14.29746914071049879, -8.314922557960816363, 83.33224293864769550 ) ) ;
#4744=CARTESIAN_POINT ( 'NONE',  ( -19.49149378614657735, 5.499999999999777955, 64.43757513605362419 ) ) ;
#4745=CARTESIAN_POINT ( 'NONE',  ( -16.46253265017146816, -9.564922557961047289, 74.16775706135234714 ) ) ;
#4746=CARTESIAN_POINT ( 'NONE',  ( 13.89961937509977652, -13.97604488694527269, 113.1239096053143527 ) ) ;
#4749=CARTESIAN_POINT ( 'NONE',  ( -16.55341960407617563, 4.379528057220093196, 33.54275706135234714 ) ) ;
#4750=CARTESIAN_POINT ( 'NONE',  ( 12.14591786802327356, -12.06949235617739191, 105.6260903946856899 ) ) ;
#4751=CARTESIAN_POINT ( 'NONE',  ( -13.89961937509957401, -13.97604488694547875, 69.37609039468564731 ) ) ;
#4752=CARTESIAN_POINT ( 'NONE',  ( -21.55341960407610458, -5.719274019375992779, 46.45724293864769550 ) ) ;
#4753=CARTESIAN_POINT ( 'NONE',  ( -21.52544592524334988, -5.823673210054445271, 73.95942372801901854 ) ) ;
#4755=CARTESIAN_POINT ( 'NONE',  ( 12.06949235617739724, 12.14591786802326823, 31.87609039468567929 ) ) ;
#4757=CARTESIAN_POINT ( 'NONE',  ( -19.05341960407611168, -5.049401038298163336, 91.45724293864766707 ) ) ;
#4759=CARTESIAN_POINT ( 'NONE',  ( -9.564922557960796823, -16.46253265017161027, 22.08224293864768839 ) ) ;
#4760=CARTESIAN_POINT ( 'NONE',  ( -0.05219959533910754901, -16.53943276465976808, 97.49890960531436690 ) ) ;
#4762=CARTESIAN_POINT ( 'NONE',  ( 19.03943276465977164, -0.05219959533909143690, 103.7489096053143669 ) ) ;
#4764=CARTESIAN_POINT ( 'NONE',  ( -12.06949235617739369, -12.14591786802326823, 59.37609039468568284 ) ) ;
#4765=CARTESIAN_POINT ( 'NONE',  ( -5.153800228976607833, 19.02544592524334988, 102.7094237280189759 ) ) ;
#4766=CARTESIAN_POINT ( 'NONE',  ( 18.62759615963271287, -10.81492255796078972, 83.33224293864769550 ) ) ;
#4767=CARTESIAN_POINT ( 'NONE',  ( 5.153800228976335163, 19.02544592524342804, 44.79057627198103830 ) ) ;
#4768=CARTESIAN_POINT ( 'NONE',  ( 5.049401038297881783, 19.05341960407617563, 72.29275706135234714 ) ) ;
#4769=CARTESIAN_POINT ( 'NONE',  ( -21.52544592524334988, -5.823673210054445271, 18.95942372801901143 ) ) ;
#4770=CARTESIAN_POINT ( 'NONE',  ( 16.51473224551069308, 9.474510206698969483, 69.16557627198102409 ) ) ;
#4771=CARTESIAN_POINT ( 'NONE',  ( 19.03943276465977164, -0.05219959533909143690, 108.7489096053143527 ) ) ;
#4772=ORIENTED_EDGE ( 'NONE', *, *, #189415, .T. ) ;
#4773=CARTESIAN_POINT ( 'NONE',  ( -8.224510206698735004, -14.34966873604973081, 29.58442372801901854 ) ) ;
#4774=CARTESIAN_POINT ( 'NONE',  ( 21.55341960407610458, 5.719274019375980345, 103.9572429386476813 ) ) ;
#4775=CARTESIAN_POINT ( 'NONE',  ( -0.05219959533910754901, -16.53943276465976808, 107.4989096053143669 ) ) ;
#4776=CARTESIAN_POINT ( 'NONE',  ( -9.474510206698964154, 16.51473224551069663, 95.41557627198102409 ) ) ;
#4777=CARTESIAN_POINT ( 'NONE',  ( -19.03943276465977164, -0.05219959533935918106, 73.75109039468566152 ) ) ;
#4778=CARTESIAN_POINT ( 'NONE',  ( 0.05219959533907565091, 21.53943276465977519, 84.99890960531436690 ) ) ;
#4779=CARTESIAN_POINT ( 'NONE',  ( 14.29746914071049879, -8.314922557960816363, 43.33224293864769550 ) ) ;
#4780=CARTESIAN_POINT ( 'NONE',  ( -10.81492255796105439, 18.62759615963255655, 112.9177570613523329 ) ) ;
#4781=CARTESIAN_POINT ( 'NONE',  ( -12.14591786802326823, 12.06949235617739902, 68.12609039468567573 ) ) ;
#4782=CARTESIAN_POINT ( 'NONE',  ( -9.474510206698964154, 16.51473224551069663, 90.41557627198103830 ) ) ;
#4783=CARTESIAN_POINT ( 'NONE',  ( -5.049401038298153566, 19.05341960407611168, 45.20724293864769550 ) ) ;
#4784=CARTESIAN_POINT ( 'NONE',  ( 18.67979575497194134, -10.72451020669871369, 50.83442372801901143 ) ) ;
#4785=CARTESIAN_POINT ( 'NONE',  ( 15.72974639402176855, 15.80617190586768217, 61.87609039468568284 ) ) ;
#4786=CARTESIAN_POINT ( 'NONE',  ( 5.153800228976335163, 19.02544592524342804, 59.79057627198100988 ) ) ;
#4787=CARTESIAN_POINT ( 'NONE',  ( 21.52544592524334988, 5.823673210054432836, 31.45942372801901854 ) ) ;
#4788=CARTESIAN_POINT ( 'NONE',  ( 9.564922557961047289, -16.46253265017146816, 70.41775706135233293 ) ) ;
#4789=CARTESIAN_POINT ( 'NONE',  ( -19.02544592524342804, 5.153800228976336051, 41.04057627198103120 ) ) ;
#4790=CARTESIAN_POINT ( 'NONE',  ( -8.224510206698735004, -14.34966873604973081, 84.58442372801903275 ) ) ;
#4791=CARTESIAN_POINT ( 'NONE',  ( -16.46253265017160317, 9.564922557960807481, 50.83224293864770260 ) ) ;
#4792=CARTESIAN_POINT ( 'NONE',  ( -19.05341960407611168, -5.049401038298163336, 106.4572429386476955 ) ) ;
#4793=CARTESIAN_POINT ( 'NONE',  ( -19.02544592524342804, 5.153800228976336051, 41.04057627198103120 ) ) ;
#4795=CARTESIAN_POINT ( 'NONE',  ( -21.52544592524343514, 5.823673210054127303, 81.04057627198102409 ) ) ;
#4796=CARTESIAN_POINT ( 'NONE',  ( -14.34966873604972548, 8.224510206698743886, 78.33442372801901854 ) ) ;
#4798=CARTESIAN_POINT ( 'NONE',  ( -9.564922557961040184, 16.46253265017147172, 32.91775706135233293 ) ) ;
#4799=CARTESIAN_POINT ( 'NONE',  ( -9.564922557960796823, -16.46253265017161027, 57.08224293864769550 ) ) ;
#4800=CARTESIAN_POINT ( 'NONE',  ( 14.29746914071049879, -8.314922557960816363, 43.33224293864769550 ) ) ;
#4801=CARTESIAN_POINT ( 'NONE',  ( 8.314922557960818139, 14.29746914071049879, 79.58224293864769550 ) ) ;
#4802=CARTESIAN_POINT ( 'NONE',  ( -16.51473224551069308, -9.474510206698971260, 106.6655762719810383 ) ) ;
#4803=CARTESIAN_POINT ( 'NONE',  ( 9.564922557960805705, 16.46253265017160317, 79.58224293864769550 ) ) ;
#4804=CARTESIAN_POINT ( 'NONE',  ( -15.72974639402176322, -15.80617190586768395, 54.37609039468568994 ) ) ;
#4805=CARTESIAN_POINT ( 'NONE',  ( 19.03943276465977164, -0.05219959533909143690, 98.74890960531436690 ) ) ;
#4806=CARTESIAN_POINT ( 'NONE',  ( -0.05219959533937732626, 21.53943276465977519, 102.5010903946856899 ) ) ;
#4807=CARTESIAN_POINT ( 'NONE',  ( 16.53943276465976808, 0.05219959533934440121, 81.25109039468568994 ) ) ;
#4809=CARTESIAN_POINT ( 'NONE',  ( 18.67979575497194134, -10.72451020669871369, 25.83442372801901499 ) ) ;
#4810=CARTESIAN_POINT ( 'NONE',  ( 18.67979575497178502, 10.72451020669898547, 109.1655762719810383 ) ) ;
#4811=CARTESIAN_POINT ( 'NONE',  ( -4.379528057220328563, 16.55341960407611168, 55.20724293864770260 ) ) ;
#4812=AXIS2_PLACEMENT_3D ( 'NONE', #26522, #196381, #195373 ) ;
#4813=CARTESIAN_POINT ( 'NONE',  ( -16.46253265017160317, 9.564922557960807481, 40.83224293864769550 ) ) ;
#4814=CARTESIAN_POINT ( 'NONE',  ( -4.379528057220328563, 16.55341960407611168, 65.20724293864768129 ) ) ;
#4815=CARTESIAN_POINT ( 'NONE',  ( -10.81492255796078084, -18.62759615963271287, 37.08224293864768129 ) ) ;
#4816=CARTESIAN_POINT ( 'NONE',  ( 9.474510206698729675, 16.51473224551082808, 37.08442372801899722 ) ) ;
#4817=CARTESIAN_POINT ( 'NONE',  ( -16.55341960407611168, -4.379528057220339221, 96.45724293864770971 ) ) ;
#4819=CARTESIAN_POINT ( 'NONE',  ( 16.53943276465976808, 0.05219959533934440121, 66.25109039468567573 ) ) ;
#4820=CARTESIAN_POINT ( 'NONE',  ( 19.03943276465977164, -0.05219959533909143690, 68.74890960531436690 ) ) ;
#4821=CARTESIAN_POINT ( 'NONE',  ( -16.99472585857189699, -5.499999999999960032, 20.67116795353343051 ) ) ;
#4822=CARTESIAN_POINT ( 'NONE',  ( 16.55341960407611168, 4.379528057220329451, 83.95724293864770971 ) ) ;
#4823=CARTESIAN_POINT ( 'NONE',  ( -21.55341960407610458, -5.719274019375992779, 31.45724293864769550 ) ) ;
#4824=CARTESIAN_POINT ( 'NONE',  ( 12.14591786802327356, -12.06949235617739191, 90.62609039468567573 ) ) ;
#4825=CARTESIAN_POINT ( 'NONE',  ( 4.483927247898790824, -16.52544592524335698, 20.20942372801900788 ) ) ;
#4826=CARTESIAN_POINT ( 'NONE',  ( -18.67979575497193778, 10.72451020669871902, 73.33442372801901854 ) ) ;
#4827=CARTESIAN_POINT ( 'NONE',  ( 13.97604488694527802, 13.89961937509977652, 94.37390960531436690 ) ) ;
#4828=CARTESIAN_POINT ( 'NONE',  ( 0.05219959533907565091, 21.53943276465977519, 104.9989096053143669 ) ) ;
#4829=CARTESIAN_POINT ( 'NONE',  ( -14.29746914071037622, -8.314922557961029526, 59.16775706135234714 ) ) ;
#4831=CARTESIAN_POINT ( 'NONE',  ( 16.53943276465976808, -0.05219959533910856209, 108.7489096053143669 ) ) ;
#4832=CARTESIAN_POINT ( 'NONE',  ( -14.29746914071037622, -8.314922557961029526, 19.16775706135234714 ) ) ;
#4833=CARTESIAN_POINT ( 'NONE',  ( 0.05219959533936267826, -19.03943276465977164, 75.00109039468566152 ) ) ;
#4834=CARTESIAN_POINT ( 'NONE',  ( 5.719274019375991003, -21.55341960407610458, 92.70724293864770971 ) ) ;
#4835=CARTESIAN_POINT ( 'NONE',  ( 19.02544592524334988, 5.153800228976608722, 51.45942372801900433 ) ) ;
#4836=CARTESIAN_POINT ( 'NONE',  ( 19.49149378614661998, -5.499999999999574563, 86.93757513605363840 ) ) ;
#4837=CARTESIAN_POINT ( 'NONE',  ( -21.53943276465977519, 0.05219959533907696930, 106.2489096053143811 ) ) ;
#4838=CARTESIAN_POINT ( 'NONE',  ( -17.49999999999999289, 5.500000000000036415, 85.79690382534171533 ) ) ;
#4839=CARTESIAN_POINT ( 'NONE',  ( -9.564922557960796823, -16.46253265017161027, 77.08224293864769550 ) ) ;
#4842=CARTESIAN_POINT ( 'NONE',  ( 4.483927247898790824, -16.52544592524335698, 35.20942372801901854 ) ) ;
#4844=CARTESIAN_POINT ( 'NONE',  ( 21.53943276465977519, -0.05219959533907433946, 98.74890960531438111 ) ) ;
#4845=CARTESIAN_POINT ( 'NONE',  ( -4.379528057220328563, 16.55341960407611168, 65.20724293864768129 ) ) ;
#4846=CARTESIAN_POINT ( 'NONE',  ( 5.153800228976335163, 19.02544592524342804, 64.79057627198100988 ) ) ;
#4848=CARTESIAN_POINT ( 'NONE',  ( 21.55341960407619695, -5.719274019375665929, 91.04275706135236135 ) ) ;
#4849=CARTESIAN_POINT ( 'NONE',  ( -4.379528057220328563, 16.55341960407611168, 95.20724293864769550 ) ) ;
#4850=CARTESIAN_POINT ( 'NONE',  ( -16.52544592524335698, -4.483927247898792601, 43.95942372801902565 ) ) ;
#4851=CARTESIAN_POINT ( 'NONE',  ( 16.46253265017146816, 9.564922557961045513, 41.66775706135234003 ) ) ;
#4852=CARTESIAN_POINT ( 'NONE',  ( -5.719274019375665041, -21.55341960407619695, 54.79275706135235424 ) ) ;
#4853=CARTESIAN_POINT ( 'NONE',  ( -13.97604488694547697, 13.89961937509957934, 113.1260903946856757 ) ) ;
#4854=CARTESIAN_POINT ( 'NONE',  ( -0.05219959533909027116, -19.03943276465977164, 52.49890960531436690 ) ) ;
#4855=CARTESIAN_POINT ( 'NONE',  ( 19.02544592524334988, 5.153800228976608722, 81.45942372801897591 ) ) ;
#4856=CARTESIAN_POINT ( 'NONE',  ( 18.67979575497194134, -10.72451020669871369, 80.83442372801901854 ) ) ;
#4857=CARTESIAN_POINT ( 'NONE',  ( -0.05219959533936034679, 19.03943276465977164, 72.50109039468566152 ) ) ;
#4858=CARTESIAN_POINT ( 'NONE',  ( 16.51473224551069308, 9.474510206698969483, 34.16557627198102409 ) ) ;
#4859=CARTESIAN_POINT ( 'NONE',  ( -10.72451020669898014, 18.67979575497178502, 60.41557627198102409 ) ) ;
#4860=CARTESIAN_POINT ( 'NONE',  ( 4.379528057220339221, -16.55341960407611168, 62.70724293864769550 ) ) ;
#4862=CARTESIAN_POINT ( 'NONE',  ( -9.564922557961040184, 16.46253265017147172, 27.91775706135232582 ) ) ;
#4863=CARTESIAN_POINT ( 'NONE',  ( -12.06949235617739369, -12.14591786802326823, 99.37609039468568994 ) ) ;
#4864=CARTESIAN_POINT ( 'NONE',  ( 8.314922557960818139, 14.29746914071049879, 59.58224293864770260 ) ) ;
#4865=CARTESIAN_POINT ( 'NONE',  ( -21.53943276465977519, -0.05219959533937600094, 88.75109039468567573 ) ) ;
#4866=CARTESIAN_POINT ( 'NONE',  ( -18.67979575497193778, 10.72451020669871902, 78.33442372801901854 ) ) ;
#4867=CARTESIAN_POINT ( 'NONE',  ( -18.62759615963270932, 10.81492255796079327, 90.83224293864769550 ) ) ;
#4869=CARTESIAN_POINT ( 'NONE',  ( 19.03943276465977164, -0.05219959533909143690, 53.74890960531436690 ) ) ;
#4870=CARTESIAN_POINT ( 'NONE',  ( 15.80617190586769283, -15.72974639402175789, 75.62609039468567573 ) ) ;
#4871=CARTESIAN_POINT ( 'NONE',  ( -13.89961937509977652, 13.97604488694528158, 50.62390960531435979 ) ) ;
#4873=CARTESIAN_POINT ( 'NONE',  ( 0.05219959533909260263, 19.03943276465977164, 69.99890960531435269 ) ) ;
#4874=CARTESIAN_POINT ( 'NONE',  ( 12.06949235617757843, -12.14591786802309237, 108.1239096053143811 ) ) ;
#4875=CARTESIAN_POINT ( 'NONE',  ( 9.474510206698971260, -16.51473224551069308, 92.91557627198103830 ) ) ;
#4876=CARTESIAN_POINT ( 'NONE',  ( 0.05219959533910956823, 16.53943276465976808, 59.99890960531436690 ) ) ;
#4877=CARTESIAN_POINT ( 'NONE',  ( 16.55341960407611168, 4.379528057220329451, 108.9572429386476955 ) ) ;
#4879=CARTESIAN_POINT ( 'NONE',  ( 10.72451020669898902, -18.67979575497178502, 82.91557627198103830 ) ) ;
#4880=CARTESIAN_POINT ( 'NONE',  ( -21.52544592524334988, -5.823673210054445271, 33.95942372801901143 ) ) ;
#4882=CARTESIAN_POINT ( 'NONE',  ( 16.55341960407618274, -4.379528057220086978, 36.04275706135234714 ) ) ;
#4883=CARTESIAN_POINT ( 'NONE',  ( -5.823673210054116645, -21.52544592524344225, 82.29057627198103830 ) ) ;
#4884=CARTESIAN_POINT ( 'NONE',  ( 21.53943276465977519, 0.05219959533937863772, 111.2510903946856899 ) ) ;
#4885=CARTESIAN_POINT ( 'NONE',  ( 16.51473224551069308, 9.474510206698969483, 94.16557627198103830 ) ) ;
#4886=CARTESIAN_POINT ( 'NONE',  ( -5.823673210054431948, 21.52544592524334988, 27.70942372801901854 ) ) ;
#4887=CARTESIAN_POINT ( 'NONE',  ( 21.55341960407610458, 5.719274019375980345, 28.95724293864769905 ) ) ;
#4888=CARTESIAN_POINT ( 'NONE',  ( -4.379528057220086978, -16.55341960407618274, 99.79275706135234714 ) ) ;
#4889=CARTESIAN_POINT ( 'NONE',  ( -0.05219959533937732626, 21.53943276465977519, 47.50109039468568994 ) ) ;
#4890=CARTESIAN_POINT ( 'NONE',  ( -0.05219959533937732626, 21.53943276465977519, 87.50109039468568994 ) ) ;
#4891=CARTESIAN_POINT ( 'NONE',  ( -21.53943276465977519, -0.05219959533937600094, 113.7510903946856757 ) ) ;
#4892=CARTESIAN_POINT ( 'NONE',  ( 0.05219959533934541429, -16.53943276465976808, 70.00109039468568994 ) ) ;
#4893=CARTESIAN_POINT ( 'NONE',  ( 15.72974639402176855, 15.80617190586768217, 46.87609039468568994 ) ) ;
#4894=CARTESIAN_POINT ( 'NONE',  ( -13.97604488694527625, -13.89961937509977652, 36.87390960531436690 ) ) ;
#4895=CARTESIAN_POINT ( 'NONE',  ( 21.53943276465977519, 0.05219959533937863772, 106.2510903946856757 ) ) ;
#4896=CARTESIAN_POINT ( 'NONE',  ( 19.03943276465977164, -0.05219959533909143690, 103.7489096053143669 ) ) ;
#4897=CARTESIAN_POINT ( 'NONE',  ( 15.80617190586746368, 15.72974639402197994, 99.37390960531436690 ) ) ;
#4899=CARTESIAN_POINT ( 'NONE',  ( 21.52544592524344225, -5.823673210054117533, 73.54057627198102409 ) ) ;
#4900=CARTESIAN_POINT ( 'NONE',  ( 16.53943276465976808, 0.05219959533934440121, 56.25109039468568284 ) ) ;
#4901=CARTESIAN_POINT ( 'NONE',  ( 16.52544592524342804, -4.483927247898539470, 43.54057627198103830 ) ) ;
#4902=CARTESIAN_POINT ( 'NONE',  ( 18.41295718396491310, -5.500000000000023093, 101.0176815517915969 ) ) ;
#4903=CARTESIAN_POINT ( 'NONE',  ( 9.564922557961047289, -16.46253265017146816, 95.41775706135233293 ) ) ;
#4905=CARTESIAN_POINT ( 'NONE',  ( 16.53943276465976808, 0.05219959533934440121, 26.25109039468567573 ) ) ;
#4906=CARTESIAN_POINT ( 'NONE',  ( 15.80617190586746368, 15.72974639402197994, 104.3739096053143669 ) ) ;
#4907=CARTESIAN_POINT ( 'NONE',  ( 0.05219959533907565091, 21.53943276465977519, 74.99890960531435269 ) ) ;
#4908=CARTESIAN_POINT ( 'NONE',  ( -9.474510206698964154, 16.51473224551069663, 110.4155762719810383 ) ) ;
#4909=CARTESIAN_POINT ( 'NONE',  ( 16.55341960407618274, -4.379528057220086978, 46.04275706135234714 ) ) ;
#4910=CARTESIAN_POINT ( 'NONE',  ( 19.05341960407611168, 5.049401038298154454, 73.95724293864768129 ) ) ;
#4911=CARTESIAN_POINT ( 'NONE',  ( -18.62759615963255300, -10.81492255796106328, 24.16775706135235424 ) ) ;
#4912=CARTESIAN_POINT ( 'NONE',  ( 13.89961937509957401, 13.97604488694547697, 101.8760903946856331 ) ) ;
#4913=CARTESIAN_POINT ( 'NONE',  ( 5.153800228976335163, 19.02544592524342804, 114.7905762719810241 ) ) ;
#4914=CARTESIAN_POINT ( 'NONE',  ( 9.564922557960805705, 16.46253265017160317, 89.58224293864769550 ) ) ;
#4915=CARTESIAN_POINT ( 'NONE',  ( -18.67979575497178146, -10.72451020669898902, 91.66557627198103830 ) ) ;
#4916=CARTESIAN_POINT ( 'NONE',  ( 9.564922557960805705, 16.46253265017160317, 54.58224293864769550 ) ) ;
#4917=CARTESIAN_POINT ( 'NONE',  ( -17.44279575226822487, -5.990770900252486264, 59.16442432485682446 ) ) ;
#4918=CARTESIAN_POINT ( 'NONE',  ( -4.483927247898539470, -16.52544592524342804, 62.29057627198102409 ) ) ;
#4919=CARTESIAN_POINT ( 'NONE',  ( -18.67979575497178146, -10.72451020669898902, 21.66557627198102409 ) ) ;
#4922=CARTESIAN_POINT ( 'NONE',  ( -10.81492255796078084, -18.62759615963271287, 92.08224293864769550 ) ) ;
#4923=CARTESIAN_POINT ( 'NONE',  ( -5.049401038297874678, -19.05341960407617918, 69.79275706135233293 ) ) ;
#4924=CARTESIAN_POINT ( 'NONE',  ( 21.52544592524344225, -5.823673210054117533, 23.54057627198102765 ) ) ;
#4925=CARTESIAN_POINT ( 'NONE',  ( 19.49671883438228548, 5.499999999999968026, 67.39279849105682274 ) ) ;
#4926=CARTESIAN_POINT ( 'NONE',  ( -21.52544592524343514, 5.823673210054127303, 61.04057627198103120 ) ) ;
#4927=CARTESIAN_POINT ( 'NONE',  ( 19.05341960407611168, 5.049401038298154454, 83.95724293864766707 ) ) ;
#4928=CARTESIAN_POINT ( 'NONE',  ( -18.62759615963255300, -10.81492255796106328, 84.16775706135234714 ) ) ;
#4929=CARTESIAN_POINT ( 'NONE',  ( -13.89961937509977652, 13.97604488694528158, 50.62390960531435979 ) ) ;
#4930=CARTESIAN_POINT ( 'NONE',  ( -8.314922557960811034, -14.29746914071050412, 77.08224293864769550 ) ) ;
#4931=CARTESIAN_POINT ( 'NONE',  ( -4.483927247898782831, 16.52544592524335698, 32.70942372801900433 ) ) ;
#4932=CARTESIAN_POINT ( 'NONE',  ( 21.53943276465977519, 0.05219959533937863772, 71.25109039468568994 ) ) ;
#4934=CARTESIAN_POINT ( 'NONE',  ( -13.89961937509957401, -13.97604488694547875, 19.37609039468566507 ) ) ;
#4935=CARTESIAN_POINT ( 'NONE',  ( 16.51473224551083163, -9.474510206698727899, 75.83442372801900433 ) ) ;
#4936=CARTESIAN_POINT ( 'NONE',  ( -18.62759615963255300, -10.81492255796106328, 39.16775706135235424 ) ) ;
#4938=CARTESIAN_POINT ( 'NONE',  ( 5.049401038297881783, 19.05341960407617563, 27.29275706135232937 ) ) ;
#4939=CARTESIAN_POINT ( 'NONE',  ( -19.02544592524342804, 5.153800228976336051, 56.04057627198100988 ) ) ;
#4940=CARTESIAN_POINT ( 'NONE',  ( -16.51473224551082808, 9.474510206698731452, 28.33442372801900433 ) ) ;
#4941=CARTESIAN_POINT ( 'NONE',  ( -8.314922557961024197, 14.29746914071037800, 107.9177570613523471 ) ) ;
#4942=CARTESIAN_POINT ( 'NONE',  ( 0.05219959533909260263, 19.03943276465977164, 99.99890960531436690 ) ) ;
#4943=CARTESIAN_POINT ( 'NONE',  ( -0.05219959533937732626, 21.53943276465977519, 72.50109039468568994 ) ) ;
#4946=CARTESIAN_POINT ( 'NONE',  ( -15.72974639402176322, -15.80617190586768395, 84.37609039468570415 ) ) ;
#4948=CARTESIAN_POINT ( 'NONE',  ( 5.153800228976335163, 19.02544592524342804, 99.79057627198102409 ) ) ;
#4949=CARTESIAN_POINT ( 'NONE',  ( -9.564922557961040184, 16.46253265017147172, 27.91775706135232582 ) ) ;
#4951=CARTESIAN_POINT ( 'NONE',  ( 5.153800228976335163, 19.02544592524342804, 34.79057627198102409 ) ) ;
#4952=CARTESIAN_POINT ( 'NONE',  ( 21.52544592524344225, -5.823673210054117533, 53.54057627198103120 ) ) ;
#4953=CARTESIAN_POINT ( 'NONE',  ( 12.14591786802309770, 12.06949235617756955, 24.37390960531435979 ) ) ;
#4954=CARTESIAN_POINT ( 'NONE',  ( -14.34966873604960291, -8.224510206698953496, 91.66557627198103830 ) ) ;
#4955=CARTESIAN_POINT ( 'NONE',  ( -9.474510206698964154, 16.51473224551069663, 75.41557627198103830 ) ) ;
#4956=CARTESIAN_POINT ( 'NONE',  ( 21.55341960407619695, -5.719274019375665929, 101.0427570613523756 ) ) ;
#4957=CARTESIAN_POINT ( 'NONE',  ( -9.474510206698964154, 16.51473224551069663, 35.41557627198102409 ) ) ;
#4958=CARTESIAN_POINT ( 'NONE',  ( 4.483927247898545687, 16.52544592524342804, 104.7905762719810241 ) ) ;
#4959=CARTESIAN_POINT ( 'NONE',  ( -0.05219959533937732626, 21.53943276465977519, 57.50109039468568994 ) ) ;
#4960=CARTESIAN_POINT ( 'NONE',  ( -15.72974639402197994, 15.80617190586746368, 80.62390960531438111 ) ) ;
#4961=CARTESIAN_POINT ( 'NONE',  ( 5.153800228976615827, -19.02544592524334988, 50.20942372801897591 ) ) ;
#4963=CARTESIAN_POINT ( 'NONE',  ( -9.474510206698964154, 16.51473224551069663, 105.4155762719810383 ) ) ;
#4964=CARTESIAN_POINT ( 'NONE',  ( -8.314922557960811034, -14.29746914071050412, 82.08224293864768129 ) ) ;
#4966=CARTESIAN_POINT ( 'NONE',  ( -5.049401038297874678, -19.05341960407617918, 44.79275706135232582 ) ) ;
#4967=CARTESIAN_POINT ( 'NONE',  ( -13.97604488694527625, -13.89961937509977652, 61.87390960531435979 ) ) ;
#4968=CARTESIAN_POINT ( 'NONE',  ( -16.53943276465976808, 0.05219959533911058130, 56.24890960531436690 ) ) ;
#4969=CARTESIAN_POINT ( 'NONE',  ( -19.05341960407617563, 5.049401038297882671, 73.54275706135233293 ) ) ;
#4971=CARTESIAN_POINT ( 'NONE',  ( 5.719274019375991003, -21.55341960407610458, 37.70724293864769550 ) ) ;
#4973=CARTESIAN_POINT ( 'NONE',  ( 12.06949235617757843, -12.14591786802309237, 98.12390960531436690 ) ) ;
#4974=CARTESIAN_POINT ( 'NONE',  ( -17.49999999999997158, -3.805241302050501151, 24.62647527217407628 ) ) ;
#4975=CARTESIAN_POINT ( 'NONE',  ( 9.474510206698971260, -16.51473224551069308, 62.91557627198102409 ) ) ;
#4976=CARTESIAN_POINT ( 'NONE',  ( 5.719274019375991003, -21.55341960407610458, 67.70724293864769550 ) ) ;
#4977=CARTESIAN_POINT ( 'NONE',  ( 19.05341960407611168, 5.049401038298154454, 33.95724293864769550 ) ) ;
#4978=CARTESIAN_POINT ( 'NONE',  ( -4.483927247898782831, 16.52544592524335698, 77.70942372801900433 ) ) ;
#4979=CARTESIAN_POINT ( 'NONE',  ( -13.97604488694527625, -13.89961937509977652, 66.87390960531436690 ) ) ;
#4980=CARTESIAN_POINT ( 'NONE',  ( 5.153800228976615827, -19.02544592524334988, 50.20942372801897591 ) ) ;
#4981=CARTESIAN_POINT ( 'NONE',  ( 21.52544592524334988, 5.823673210054432836, 66.45942372801903275 ) ) ;
#4982=CARTESIAN_POINT ( 'NONE',  ( 18.67979575497178502, 10.72451020669898547, 44.16557627198103120 ) ) ;
#4983=CARTESIAN_POINT ( 'NONE',  ( 5.153800228976335163, 19.02544592524342804, 29.79057627198102409 ) ) ;
#4984=CARTESIAN_POINT ( 'NONE',  ( 12.14591786802327356, -12.06949235617739191, 85.62609039468568994 ) ) ;
#4985=CARTESIAN_POINT ( 'NONE',  ( -16.46253265017146816, -9.564922557961047289, 104.1677570613523329 ) ) ;
#4986=CARTESIAN_POINT ( 'NONE',  ( 9.474510206698971260, -16.51473224551069308, 22.91557627198102765 ) ) ;
#4987=DIRECTION ( 'NONE',  ( -1.000000000000000000, 0.000000000000000000, 0.000000000000000000 ) ) ;
#4988=CARTESIAN_POINT ( 'NONE',  ( 21.52544592524334988, 5.823673210054432836, 91.45942372801901854 ) ) ;
#4991=CARTESIAN_POINT ( 'NONE',  ( -4.379528057220328563, 16.55341960407611168, 40.20724293864769550 ) ) ;
#4992=CARTESIAN_POINT ( 'NONE',  ( -4.379528057220328563, 16.55341960407611168, 55.20724293864770260 ) ) ;
#4993=CARTESIAN_POINT ( 'NONE',  ( 21.52544592524344225, -5.823673210054117533, 93.54057627198103830 ) ) ;
#4994=CARTESIAN_POINT ( 'NONE',  ( 18.62759615963271287, -10.81492255796078972, 93.33224293864769550 ) ) ;
#4996=CARTESIAN_POINT ( 'NONE',  ( -15.72974639402197994, 15.80617190586746368, 35.62390960531437401 ) ) ;
#4997=ADVANCED_FACE ( 'NONE', ( #193808 ), #113093, .T. ) ;
#4998=CARTESIAN_POINT ( 'NONE',  ( -8.314922557961024197, 14.29746914071037800, 72.91775706135234714 ) ) ;
#5000=CARTESIAN_POINT ( 'NONE',  ( 14.34966873604960469, 8.224510206698951720, 84.16557627198103830 ) ) ;
#5001=CARTESIAN_POINT ( 'NONE',  ( -9.564922557960796823, -16.46253265017161027, 47.08224293864769550 ) ) ;
#5004=CARTESIAN_POINT ( 'NONE',  ( 14.34966873604972726, -8.224510206698740333, 100.8344237280190185 ) ) ;
#5005=CARTESIAN_POINT ( 'NONE',  ( 21.53943276465977519, -0.05219959533907433946, 113.7489096053143527 ) ) ;
#5006=CARTESIAN_POINT ( 'NONE',  ( -16.46253265017160317, 9.564922557960807481, 80.83224293864769550 ) ) ;
#5007=CARTESIAN_POINT ( 'NONE',  ( 21.52544592524334988, 5.823673210054432836, 51.45942372801901854 ) ) ;
#5008=CARTESIAN_POINT ( 'NONE',  ( 0.05219959533909260263, 19.03943276465977164, 104.9989096053143669 ) ) ;
#5011=CARTESIAN_POINT ( 'NONE',  ( 5.823673210054444382, -21.52544592524334988, 45.20942372801901854 ) ) ;
#5012=CARTESIAN_POINT ( 'NONE',  ( 0.05219959533909260263, 19.03943276465977164, 39.99890960531436690 ) ) ;
#5013=CARTESIAN_POINT ( 'NONE',  ( -19.05341960407611168, -5.049401038298163336, 21.45724293864768839 ) ) ;
#5014=CARTESIAN_POINT ( 'NONE',  ( -13.89961937509957401, -13.97604488694547875, 59.37609039468566863 ) ) ;
#5015=CARTESIAN_POINT ( 'NONE',  ( -5.823673210054431948, 21.52544592524334988, 27.70942372801901854 ) ) ;
#5016=CARTESIAN_POINT ( 'NONE',  ( -9.474510206698720793, -16.51473224551083518, 64.58442372801900433 ) ) ;
#5017=CARTESIAN_POINT ( 'NONE',  ( -16.46253265017160317, 9.564922557960807481, 30.83224293864769550 ) ) ;
#5018=CARTESIAN_POINT ( 'NONE',  ( 16.55341960407618274, -4.379528057220086978, 96.04275706135236135 ) ) ;
#5019=CARTESIAN_POINT ( 'NONE',  ( 19.05341960407617918, -5.049401038297876454, 66.04275706135233293 ) ) ;
#5020=CARTESIAN_POINT ( 'NONE',  ( 14.34966873604972726, -8.224510206698740333, 110.8344237280190043 ) ) ;
#5022=CARTESIAN_POINT ( 'NONE',  ( 9.474510206698971260, -16.51473224551069308, 87.91557627198102409 ) ) ;
#5023=CARTESIAN_POINT ( 'NONE',  ( 5.719274019375673035, 21.55341960407619339, 87.29275706135236135 ) ) ;
#5024=CARTESIAN_POINT ( 'NONE',  ( -21.55341960407619339, 5.719274019375674811, 103.5427570613523613 ) ) ;
#5026=CARTESIAN_POINT ( 'NONE',  ( 0.05219959533909260263, 19.03943276465977164, 94.99890960531436690 ) ) ;
#5027=CARTESIAN_POINT ( 'NONE',  ( 15.72974639402176855, 15.80617190586768217, 71.87609039468568994 ) ) ;
#5028=CARTESIAN_POINT ( 'NONE',  ( 0.05219959533934541429, -16.53943276465976808, 25.00109039468567218 ) ) ;
#5029=CARTESIAN_POINT ( 'NONE',  ( 16.46253265017160672, -9.564922557960803928, 78.33224293864769550 ) ) ;
#5030=CARTESIAN_POINT ( 'NONE',  ( -15.80617190586745835, -15.72974639402198527, 31.87390960531435979 ) ) ;
#5032=CARTESIAN_POINT ( 'NONE',  ( 13.97604488694527802, 13.89961937509977652, 59.37390960531434558 ) ) ;
#5033=CARTESIAN_POINT ( 'NONE',  ( 16.55341960407618274, -4.379528057220086978, 111.0427570613523613 ) ) ;
#5034=CARTESIAN_POINT ( 'NONE',  ( -16.19135201231352639, 7.376712067591985722, 99.81319145947878724 ) ) ;
#5035=CARTESIAN_POINT ( 'NONE',  ( 19.02544592524334988, 5.153800228976608722, 71.45942372801900433 ) ) ;
#5036=CARTESIAN_POINT ( 'NONE',  ( -19.03943276465977164, 0.05219959533909376836, 101.2489096053143669 ) ) ;
#5037=CARTESIAN_POINT ( 'NONE',  ( 10.72451020669871369, 18.67979575497193778, 102.0844237280190185 ) ) ;
#5038=CARTESIAN_POINT ( 'NONE',  ( 8.314922557960818139, 14.29746914071049879, 84.58224293864769550 ) ) ;
#5039=CARTESIAN_POINT ( 'NONE',  ( -15.80617190586745835, -15.72974639402198527, 51.87390960531437401 ) ) ;
#5040=CARTESIAN_POINT ( 'NONE',  ( -15.72974639402197994, 15.80617190586746368, 35.62390960531437401 ) ) ;
#5041=CARTESIAN_POINT ( 'NONE',  ( -14.29746914071049879, 8.314922557960819915, 110.8322429386476955 ) ) ;
#5043=CARTESIAN_POINT ( 'NONE',  ( 19.03943276465977164, 0.05219959533936151252, 41.25109039468566152 ) ) ;
#5044=CARTESIAN_POINT ( 'NONE',  ( 8.224510206698953496, -14.34966873604960469, 22.91557627198102765 ) ) ;
#5045=CARTESIAN_POINT ( 'NONE',  ( 9.564922557960805705, 16.46253265017160317, 99.58224293864770971 ) ) ;
#5046=CARTESIAN_POINT ( 'NONE',  ( 15.80617190586769283, -15.72974639402175789, 70.62609039468567573 ) ) ;
#5047=CARTESIAN_POINT ( 'NONE',  ( 15.80617190586746368, 15.72974639402197994, 54.37390960531435979 ) ) ;
#5048=CARTESIAN_POINT ( 'NONE',  ( -5.719274019375665041, -21.55341960407619695, 44.79275706135234714 ) ) ;
#5049=CARTESIAN_POINT ( 'NONE',  ( 5.719274019375991003, -21.55341960407610458, 97.70724293864772392 ) ) ;
#5050=CARTESIAN_POINT ( 'NONE',  ( -18.67979575497193778, 10.72451020669871902, 33.33442372801900433 ) ) ;
#5051=CARTESIAN_POINT ( 'NONE',  ( 16.46253265017160672, -9.564922557960803928, 28.33224293864769550 ) ) ;
#5052=CARTESIAN_POINT ( 'NONE',  ( 0.05219959533936267826, -19.03943276465977164, 65.00109039468567573 ) ) ;
#5053=CARTESIAN_POINT ( 'NONE',  ( -8.224510206698948167, 14.34966873604960824, 110.4155762719810383 ) ) ;
#5054=CARTESIAN_POINT ( 'NONE',  ( -19.05341960407611168, -5.049401038298163336, 106.4572429386476955 ) ) ;
#5056=CARTESIAN_POINT ( 'NONE',  ( 8.224510206698953496, -14.34966873604960469, 57.91557627198103120 ) ) ;
#5057=CARTESIAN_POINT ( 'NONE',  ( 0.05219959533934541429, -16.53943276465976808, 110.0010903946856757 ) ) ;
#5058=CARTESIAN_POINT ( 'NONE',  ( -19.05341960407611168, -5.049401038298163336, 46.45724293864768129 ) ) ;
#5059=CARTESIAN_POINT ( 'NONE',  ( 16.53943276465976808, -0.05219959533910856209, 113.7489096053143527 ) ) ;
#5060=CARTESIAN_POINT ( 'NONE',  ( -15.72974639402197994, 15.80617190586746368, 30.62390960531436335 ) ) ;
#5061=CARTESIAN_POINT ( 'NONE',  ( -5.049401038297874678, -19.05341960407617918, 29.79275706135232227 ) ) ;
#5063=CARTESIAN_POINT ( 'NONE',  ( 16.53943276465976808, -0.05219959533910856209, 33.74890960531436690 ) ) ;
#5064=CARTESIAN_POINT ( 'NONE',  ( 10.72451020669871369, 18.67979575497193778, 47.08442372801901854 ) ) ;
#5065=CARTESIAN_POINT ( 'NONE',  ( 17.50000000000000000, -7.500000000000000888, 120.0000000000000142 ) ) ;
#5066=CARTESIAN_POINT ( 'NONE',  ( 8.224510206698742110, 14.34966873604972548, 62.08442372801901143 ) ) ;
#5068=CARTESIAN_POINT ( 'NONE',  ( 9.474510206698729675, 16.51473224551082808, 62.08442372801899722 ) ) ;
#5069=CARTESIAN_POINT ( 'NONE',  ( 4.483927247898545687, 16.52544592524342804, 29.79057627198102409 ) ) ;
#5070=CARTESIAN_POINT ( 'NONE',  ( 4.379528057220092307, 16.55341960407617563, 107.2927570613523471 ) ) ;
#5071=CARTESIAN_POINT ( 'NONE',  ( 19.05341960407611168, 5.049401038298154454, 33.95724293864769550 ) ) ;
#5072=CARTESIAN_POINT ( 'NONE',  ( 9.474510206698971260, -16.51473224551069308, 67.91557627198102409 ) ) ;
#5073=CARTESIAN_POINT ( 'NONE',  ( -5.153800228976328057, -19.02544592524343514, 27.29057627198103120 ) ) ;
#5074=CARTESIAN_POINT ( 'NONE',  ( 18.67979575497194134, -10.72451020669871369, 30.83442372801902209 ) ) ;
#5075=CARTESIAN_POINT ( 'NONE',  ( 19.03943276465977164, -0.05219959533909143690, 48.74890960531435979 ) ) ;
#5077=CARTESIAN_POINT ( 'NONE',  ( 19.03943276465977164, -0.05219959533909143690, 33.74890960531435979 ) ) ;
#5078=CARTESIAN_POINT ( 'NONE',  ( -0.05219959533909027116, -19.03943276465977164, 112.4989096053143669 ) ) ;
#5080=CARTESIAN_POINT ( 'NONE',  ( -10.72451020669870658, -18.67979575497194134, 64.58442372801900433 ) ) ;
#5081=CARTESIAN_POINT ( 'NONE',  ( -16.53943276465976808, 0.05219959533911058130, 101.2489096053143669 ) ) ;
#5082=CARTESIAN_POINT ( 'NONE',  ( -16.46253265017160317, 9.564922557960807481, 115.8322429386477097 ) ) ;
#5083=CARTESIAN_POINT ( 'NONE',  ( -14.29746914071037622, -8.314922557961029526, 84.16775706135234714 ) ) ;
#5084=CARTESIAN_POINT ( 'NONE',  ( -5.719274019375665041, -21.55341960407619695, 94.79275706135234714 ) ) ;
#5085=CARTESIAN_POINT ( 'NONE',  ( -12.14591786802326823, 12.06949235617739902, 48.12609039468568284 ) ) ;
#5086=CARTESIAN_POINT ( 'NONE',  ( 13.97604488694527802, 13.89961937509977652, 94.37390960531436690 ) ) ;
#5087=CARTESIAN_POINT ( 'NONE',  ( 16.55341960407618274, -4.379528057220086978, 36.04275706135234714 ) ) ;
#5088=CARTESIAN_POINT ( 'NONE',  ( 16.52544592524335698, 4.483927247898782831, 21.45942372801901499 ) ) ;
#5089=CARTESIAN_POINT ( 'NONE',  ( 16.52544592524335698, 4.483927247898782831, 81.45942372801900433 ) ) ;
#5090=CARTESIAN_POINT ( 'NONE',  ( -13.89961937509957401, -13.97604488694547875, 109.3760903946856331 ) ) ;
#5091=CARTESIAN_POINT ( 'NONE',  ( 18.62759615963271287, -10.81492255796078972, 93.33224293864769550 ) ) ;
#5092=CARTESIAN_POINT ( 'NONE',  ( 16.55341960407611168, 4.379528057220329451, 103.9572429386476813 ) ) ;
#5093=CARTESIAN_POINT ( 'NONE',  ( -16.51473224551082808, 9.474510206698731452, 98.33442372801900433 ) ) ;
#5094=CARTESIAN_POINT ( 'NONE',  ( 4.379528057220092307, 16.55341960407617563, 77.29275706135234714 ) ) ;
#5096=CARTESIAN_POINT ( 'NONE',  ( -19.02544592524334988, -5.153800228976617603, 63.95942372801899012 ) ) ;
#5097=CARTESIAN_POINT ( 'NONE',  ( -8.224510206698948167, 14.34966873604960824, 45.41557627198103830 ) ) ;
#5098=CARTESIAN_POINT ( 'NONE',  ( 8.224510206698953496, -14.34966873604960469, 92.91557627198103830 ) ) ;
#5099=CARTESIAN_POINT ( 'NONE',  ( 5.153800228976615827, -19.02544592524334988, 35.20942372801899722 ) ) ;
#5100=CARTESIAN_POINT ( 'NONE',  ( -19.49149378614659867, 5.499999999999578115, 89.43757513605359577 ) ) ;
#5101=CARTESIAN_POINT ( 'NONE',  ( 5.823673210054444382, -21.52544592524334988, 40.20942372801901854 ) ) ;
#5102=CARTESIAN_POINT ( 'NONE',  ( 16.51473224551083163, -9.474510206698727899, 95.83442372801900433 ) ) ;
#5103=CARTESIAN_POINT ( 'NONE',  ( -19.05341960407611168, -5.049401038298163336, 111.4572429386476671 ) ) ;
#5104=CARTESIAN_POINT ( 'NONE',  ( 16.51473224551069308, 9.474510206698969483, 94.16557627198103830 ) ) ;
#5105=CARTESIAN_POINT ( 'NONE',  ( 21.52544592524334988, 5.823673210054432836, 111.4594237280190328 ) ) ;
#5106=CARTESIAN_POINT ( 'NONE',  ( 13.89961937509977652, -13.97604488694527269, 88.12390960531438111 ) ) ;
#5107=CARTESIAN_POINT ( 'NONE',  ( -21.53943276465977519, 0.05219959533907696930, 61.24890960531435979 ) ) ;
#5108=CARTESIAN_POINT ( 'NONE',  ( 4.379528057220339221, -16.55341960407611168, 87.70724293864769550 ) ) ;
#5109=CARTESIAN_POINT ( 'NONE',  ( -19.05341960407611168, -5.049401038298163336, 66.45724293864769550 ) ) ;
#5110=CARTESIAN_POINT ( 'NONE',  ( 12.06949235617757843, -12.14591786802309237, 108.1239096053143811 ) ) ;
#5111=CARTESIAN_POINT ( 'NONE',  ( -21.52544592524334988, -5.823673210054445271, 43.95942372801902565 ) ) ;
#5112=CARTESIAN_POINT ( 'NONE',  ( -18.67979575497193778, 10.72451020669871902, 78.33442372801901854 ) ) ;
#5113=CARTESIAN_POINT ( 'NONE',  ( 5.153800228976335163, 19.02544592524342804, 49.79057627198100988 ) ) ;
#5114=CARTESIAN_POINT ( 'NONE',  ( -8.314922557961024197, 14.29746914071037800, 72.91775706135234714 ) ) ;
#5115=CARTESIAN_POINT ( 'NONE',  ( 21.53943276465977519, 0.05219959533937863772, 36.25109039468567573 ) ) ;
#5116=CARTESIAN_POINT ( 'NONE',  ( 21.55341960407619695, -5.719274019375665929, 26.04275706135235779 ) ) ;
#5117=CARTESIAN_POINT ( 'NONE',  ( -16.51473224551082808, 9.474510206698731452, 53.33442372801900433 ) ) ;
#5118=CARTESIAN_POINT ( 'NONE',  ( -13.97604488694527625, -13.89961937509977652, 66.87390960531436690 ) ) ;
#5119=CARTESIAN_POINT ( 'NONE',  ( 16.46253265017146816, 9.564922557961045513, 26.66775706135234003 ) ) ;
#5120=CARTESIAN_POINT ( 'NONE',  ( -0.05219959533937732626, 21.53943276465977519, 87.50109039468568994 ) ) ;
#5121=CARTESIAN_POINT ( 'NONE',  ( 21.53943276465977519, -0.05219959533907433946, 73.74890960531433848 ) ) ;
#5122=CARTESIAN_POINT ( 'NONE',  ( 8.314922557960818139, 14.29746914071049879, 49.58224293864769550 ) ) ;
#5123=CARTESIAN_POINT ( 'NONE',  ( 10.81492255796106328, -18.62759615963255655, 85.41775706135236135 ) ) ;
#5124=CARTESIAN_POINT ( 'NONE',  ( -16.46253265017146816, -9.564922557961047289, 24.16775706135233648 ) ) ;
#5125=CARTESIAN_POINT ( 'NONE',  ( -12.14591786802309592, -12.06949235617757132, 76.87390960531439532 ) ) ;
#5126=CARTESIAN_POINT ( 'NONE',  ( -16.46253265017160317, 9.564922557960807481, 25.83224293864769194 ) ) ;
#5127=CARTESIAN_POINT ( 'NONE',  ( -16.46253265017146816, -9.564922557961047289, 54.16775706135234003 ) ) ;
#5128=CARTESIAN_POINT ( 'NONE',  ( -12.14591786802309592, -12.06949235617757132, 31.87390960531435979 ) ) ;
#5129=CARTESIAN_POINT ( 'NONE',  ( 18.62759615963255655, 10.81492255796105972, 86.66775706135234714 ) ) ;
#5130=CARTESIAN_POINT ( 'NONE',  ( 16.51473224551069308, 9.474510206698969483, 79.16557627198103830 ) ) ;
#5131=CARTESIAN_POINT ( 'NONE',  ( 13.89961937509957401, 13.97604488694547697, 51.87609039468566863 ) ) ;
#5132=CARTESIAN_POINT ( 'NONE',  ( -18.67979575497178146, -10.72451020669898902, 46.66557627198102409 ) ) ;
#5134=CARTESIAN_POINT ( 'NONE',  ( -21.55341960407619339, 5.719274019375674811, 48.54275706135234714 ) ) ;
#5135=CARTESIAN_POINT ( 'NONE',  ( -21.55341960407610458, -5.719274019375992779, 96.45724293864770971 ) ) ;
#5136=CARTESIAN_POINT ( 'NONE',  ( 13.97604488694548053, -13.89961937509957401, 100.6260903946856615 ) ) ;
#5137=CARTESIAN_POINT ( 'NONE',  ( 8.224510206698742110, 14.34966873604972548, 62.08442372801901143 ) ) ;
#5139=CARTESIAN_POINT ( 'NONE',  ( 15.72974639402199770, -15.80617190586745480, 108.1239096053143811 ) ) ;
#5140=CARTESIAN_POINT ( 'NONE',  ( -12.14591786802309592, -12.06949235617757132, 96.87390960531436690 ) ) ;
#5141=DIRECTION ( 'NONE',  ( 0.000000000000000000, 0.000000000000000000, -1.000000000000000000 ) ) ;
#5142=CARTESIAN_POINT ( 'NONE',  ( 16.55341960407618274, -4.379528057220086978, 31.04275706135234714 ) ) ;
#5143=CARTESIAN_POINT ( 'NONE',  ( -10.72451020669898014, 18.67979575497178502, 65.41557627198102409 ) ) ;
#5144=CARTESIAN_POINT ( 'NONE',  ( -12.14591786802326823, 12.06949235617739902, 98.12609039468570415 ) ) ;
#5145=CARTESIAN_POINT ( 'NONE',  ( 13.89961937509977652, -13.97604488694527269, 28.12390960531435624 ) ) ;
#5146=CARTESIAN_POINT ( 'NONE',  ( -8.224510206698735004, -14.34966873604973081, 64.58442372801900433 ) ) ;
#5147=CARTESIAN_POINT ( 'NONE',  ( -16.46253265017146816, -9.564922557961047289, 59.16775706135233293 ) ) ;
#5148=CARTESIAN_POINT ( 'NONE',  ( -18.67979575497193778, 10.72451020669871902, 43.33442372801901143 ) ) ;
#5149=CARTESIAN_POINT ( 'NONE',  ( 21.55341960407610458, 5.719274019375980345, 58.95724293864770971 ) ) ;
#5150=CARTESIAN_POINT ( 'NONE',  ( -4.483927247898782831, 16.52544592524335698, 87.70942372801901854 ) ) ;
#5151=CARTESIAN_POINT ( 'NONE',  ( -21.53943276465977519, -0.05219959533937600094, 73.75109039468567573 ) ) ;
#5152=CARTESIAN_POINT ( 'NONE',  ( 5.719274019375991003, -21.55341960407610458, 57.70724293864770260 ) ) ;
#5153=CARTESIAN_POINT ( 'NONE',  ( 0.05219959533907565091, 21.53943276465977519, 39.99890960531436690 ) ) ;
#5154=CARTESIAN_POINT ( 'NONE',  ( 4.483927247898790824, -16.52544592524335698, 60.20942372801902565 ) ) ;
#5155=CARTESIAN_POINT ( 'NONE',  ( -18.62759615963270932, 10.81492255796079327, 35.83224293864768839 ) ) ;
#5157=CARTESIAN_POINT ( 'NONE',  ( 19.05341960407611168, 5.049401038298154454, 93.95724293864769550 ) ) ;
#5158=CARTESIAN_POINT ( 'NONE',  ( -12.14591786802326823, 12.06949235617739902, 113.1260903946856899 ) ) ;
#5160=CARTESIAN_POINT ( 'NONE',  ( 8.224510206698953496, -14.34966873604960469, 102.9155762719810383 ) ) ;
#5161=CARTESIAN_POINT ( 'NONE',  ( -15.72974639402197994, 15.80617190586746368, 65.62390960531436690 ) ) ;
#5162=CARTESIAN_POINT ( 'NONE',  ( 14.34966873604972726, -8.224510206698740333, 85.83442372801901854 ) ) ;
#5163=CARTESIAN_POINT ( 'NONE',  ( -15.72974639402176322, -15.80617190586768395, 49.37609039468569705 ) ) ;
#5164=CARTESIAN_POINT ( 'NONE',  ( -0.05219959533936034679, 19.03943276465977164, 107.5010903946856615 ) ) ;
#5165=CARTESIAN_POINT ( 'NONE',  ( 4.379528057220339221, -16.55341960407611168, 102.7072429386476955 ) ) ;
#5166=CARTESIAN_POINT ( 'NONE',  ( -9.564922557960796823, -16.46253265017161027, 52.08224293864768839 ) ) ;
#5168=CARTESIAN_POINT ( 'NONE',  ( 9.564922557960805705, 16.46253265017160317, 29.58224293864769550 ) ) ;
#5170=CARTESIAN_POINT ( 'NONE',  ( 5.153800228976335163, 19.02544592524342804, 89.79057627198102409 ) ) ;
#5171=CARTESIAN_POINT ( 'NONE',  ( -8.314922557961024197, 14.29746914071037800, 77.91775706135231871 ) ) ;
#5172=CARTESIAN_POINT ( 'NONE',  ( -5.719274019375665041, -21.55341960407619695, 99.79275706135234714 ) ) ;
#5173=CARTESIAN_POINT ( 'NONE',  ( 10.72451020669898902, -18.67979575497178502, 47.91557627198102409 ) ) ;
#5175=CARTESIAN_POINT ( 'NONE',  ( -14.34966873604972548, 8.224510206698743886, 78.33442372801901854 ) ) ;
#5176=CARTESIAN_POINT ( 'NONE',  ( 13.97604488694548053, -13.89961937509957401, 80.62609039468567573 ) ) ;
#5178=CARTESIAN_POINT ( 'NONE',  ( -13.97604488694527625, -13.89961937509977652, 36.87390960531436690 ) ) ;
#5179=CARTESIAN_POINT ( 'NONE',  ( -13.89961937509977652, 13.97604488694528158, 80.62390960531436690 ) ) ;
#5180=CARTESIAN_POINT ( 'NONE',  ( 13.89961937509977652, -13.97604488694527269, 38.12390960531436690 ) ) ;
#5181=CARTESIAN_POINT ( 'NONE',  ( -13.97604488694547697, 13.89961937509957934, 78.12609039468567573 ) ) ;
#5183=CARTESIAN_POINT ( 'NONE',  ( -0.05219959533909027116, -19.03943276465977164, 102.4989096053143669 ) ) ;
#5184=CARTESIAN_POINT ( 'NONE',  ( -12.06949235617756955, 12.14591786802309770, 55.62390960531436690 ) ) ;
#5185=CARTESIAN_POINT ( 'NONE',  ( -10.72451020669898014, 18.67979575497178502, 50.41557627198103120 ) ) ;
#5186=CARTESIAN_POINT ( 'NONE',  ( -17.50000000000000000, 3.209263204892625954, 104.7619682560627297 ) ) ;
#5187=CARTESIAN_POINT ( 'NONE',  ( 9.564922557961047289, -16.46253265017146816, 30.41775706135232937 ) ) ;
#5188=CARTESIAN_POINT ( 'NONE',  ( -17.50000000000000711, -5.499999999999944045, 81.28230962303565832 ) ) ;
#5189=CARTESIAN_POINT ( 'NONE',  ( -5.153800228976328057, -19.02544592524343514, 47.29057627198102409 ) ) ;
#5190=CARTESIAN_POINT ( 'NONE',  ( 16.55341960407618274, -4.379528057220086978, 36.04275706135234714 ) ) ;
#5191=CARTESIAN_POINT ( 'NONE',  ( -18.56399227203342051, -5.499999999999968914, 98.97830131249901342 ) ) ;
#5193=CARTESIAN_POINT ( 'NONE',  ( 4.379528057220092307, 16.55341960407617563, 82.29275706135234714 ) ) ;
#5194=CARTESIAN_POINT ( 'NONE',  ( 21.55341960407610458, 5.719274019375980345, 93.95724293864770971 ) ) ;
#5195=CARTESIAN_POINT ( 'NONE',  ( -0.05219959533934338120, 16.53943276465976808, 42.50109039468567573 ) ) ;
#5196=CARTESIAN_POINT ( 'NONE',  ( 13.89961937509977652, -13.97604488694527269, 38.12390960531436690 ) ) ;
#5197=CARTESIAN_POINT ( 'NONE',  ( -5.049401038298153566, 19.05341960407611168, 115.2072429386477097 ) ) ;
#5198=CARTESIAN_POINT ( 'NONE',  ( -21.55341960407619339, 5.719274019375674811, 38.54275706135234714 ) ) ;
#5199=CARTESIAN_POINT ( 'NONE',  ( 19.05341960407617918, -5.049401038297876454, 56.04275706135234714 ) ) ;
#5200=CARTESIAN_POINT ( 'NONE',  ( 21.55341960407619695, -5.719274019375665929, 96.04275706135236135 ) ) ;
#5203=CARTESIAN_POINT ( 'NONE',  ( -4.379528057220328563, 16.55341960407611168, 35.20724293864768839 ) ) ;
#5205=CARTESIAN_POINT ( 'NONE',  ( -15.80617190586745835, -15.72974639402198527, 56.87390960531436690 ) ) ;
#5207=CARTESIAN_POINT ( 'NONE',  ( -16.51473224551069308, -9.474510206698971260, 106.6655762719810383 ) ) ;
#5208=CARTESIAN_POINT ( 'NONE',  ( 14.29746914071049879, -8.314922557960816363, 108.3322429386477097 ) ) ;
#5209=CARTESIAN_POINT ( 'NONE',  ( -12.06949235617739369, -12.14591786802326823, 19.37609039468568639 ) ) ;
#5210=CARTESIAN_POINT ( 'NONE',  ( -4.379528057220086978, -16.55341960407618274, 109.7927570613523613 ) ) ;
#5212=CARTESIAN_POINT ( 'NONE',  ( 19.02544592524343514, -5.153800228976328945, 103.5405762719809957 ) ) ;
#5213=CARTESIAN_POINT ( 'NONE',  ( 5.719274019375991003, -21.55341960407610458, 102.7072429386476955 ) ) ;
#5214=CARTESIAN_POINT ( 'NONE',  ( -16.53943276465976808, 0.05219959533911058130, 31.24890960531435979 ) ) ;
#5215=CARTESIAN_POINT ( 'NONE',  ( -13.97604488694527625, -13.89961937509977652, 111.8739096053143243 ) ) ;
#5216=CARTESIAN_POINT ( 'NONE',  ( 13.97604488694548053, -13.89961937509957401, 90.62609039468567573 ) ) ;
#5217=CARTESIAN_POINT ( 'NONE',  ( 5.719274019375673035, 21.55341960407619339, 102.2927570613523613 ) ) ;
#5218=CARTESIAN_POINT ( 'NONE',  ( -4.379528057220328563, 16.55341960407611168, 30.20724293864769550 ) ) ;
#5219=CARTESIAN_POINT ( 'NONE',  ( -18.67979575497178146, -10.72451020669898902, 86.66557627198102409 ) ) ;
#5220=CARTESIAN_POINT ( 'NONE',  ( 21.55341960407610458, 5.719274019375980345, 48.95724293864770971 ) ) ;
#5221=CARTESIAN_POINT ( 'NONE',  ( 16.46253265017160672, -9.564922557960803928, 63.33224293864769550 ) ) ;
#5222=CARTESIAN_POINT ( 'NONE',  ( 0.05219959533910956823, 16.53943276465976808, 29.99890960531435979 ) ) ;
#5223=CARTESIAN_POINT ( 'NONE',  ( 5.049401038298161559, -19.05341960407611168, 77.70724293864765286 ) ) ;
#5224=CARTESIAN_POINT ( 'NONE',  ( 19.53037848336977333, -5.500000000000093259, 62.35532783611444074 ) ) ;
#5225=CARTESIAN_POINT ( 'NONE',  ( -19.02544592524334988, -5.153800228976617603, 38.95942372801900433 ) ) ;
#5226=CARTESIAN_POINT ( 'NONE',  ( -10.81492255796078084, -18.62759615963271287, 87.08224293864769550 ) ) ;
#5227=CARTESIAN_POINT ( 'NONE',  ( 0.05219959533910956823, 16.53943276465976808, 84.99890960531436690 ) ) ;
#5228=CARTESIAN_POINT ( 'NONE',  ( 10.72451020669871369, 18.67979575497193778, 42.08442372801901854 ) ) ;
#5230=EDGE_CURVE ( 'NONE', #13916, #15707, #123918, .T. ) ;
#5231=CARTESIAN_POINT ( 'NONE',  ( -14.34966873604972548, 8.224510206698743886, 108.3344237280190185 ) ) ;
#5232=CARTESIAN_POINT ( 'NONE',  ( -0.05219959533909027116, -19.03943276465977164, 22.49890960531436690 ) ) ;
#5233=CARTESIAN_POINT ( 'NONE',  ( -16.46253265017160317, 9.564922557960807481, 90.83224293864769550 ) ) ;
#5236=CARTESIAN_POINT ( 'NONE',  ( -16.52544592524342804, 4.483927247898546575, 41.04057627198103120 ) ) ;
#5237=CARTESIAN_POINT ( 'NONE',  ( 10.72451020669871369, 18.67979575497193778, 77.08442372801901854 ) ) ;
#5239=CARTESIAN_POINT ( 'NONE',  ( -4.379528057220086978, -16.55341960407618274, 69.79275706135234714 ) ) ;
#5240=CARTESIAN_POINT ( 'NONE',  ( -16.46253265017160317, 9.564922557960807481, 40.83224293864769550 ) ) ;
#5241=CARTESIAN_POINT ( 'NONE',  ( -13.89961937509977652, 13.97604488694528158, 55.62390960531434558 ) ) ;
#5243=CARTESIAN_POINT ( 'NONE',  ( 5.823673210054444382, -21.52544592524334988, 110.2094237280190185 ) ) ;
#5244=CARTESIAN_POINT ( 'NONE',  ( 14.34966873604972726, -8.224510206698740333, 65.83442372801900433 ) ) ;
#5245=CARTESIAN_POINT ( 'NONE',  ( 5.823673210054444382, -21.52544592524334988, 95.20942372801903275 ) ) ;
#5246=CARTESIAN_POINT ( 'NONE',  ( -13.89961937509977652, 13.97604488694528158, 115.6239096053143669 ) ) ;
#5247=CARTESIAN_POINT ( 'NONE',  ( -5.153800228976607833, 19.02544592524334988, 102.7094237280189759 ) ) ;
#5248=CARTESIAN_POINT ( 'NONE',  ( -5.823673210054431948, 21.52544592524334988, 72.70942372801901854 ) ) ;
#5249=CARTESIAN_POINT ( 'NONE',  ( 16.52544592524335698, 4.483927247898782831, 31.45942372801901854 ) ) ;
#5250=CARTESIAN_POINT ( 'NONE',  ( -10.81492255796078084, -18.62759615963271287, 92.08224293864769550 ) ) ;
#5251=CARTESIAN_POINT ( 'NONE',  ( -16.46253265017146816, -9.564922557961047289, 99.16775706135233293 ) ) ;
#5252=CARTESIAN_POINT ( 'NONE',  ( -19.03943276465977164, 0.05219959533909376836, 66.24890960531436690 ) ) ;
#5253=CARTESIAN_POINT ( 'NONE',  ( 5.153800228976615827, -19.02544592524334988, 110.2094237280189901 ) ) ;
#5254=CARTESIAN_POINT ( 'NONE',  ( 13.97604488694548053, -13.89961937509957401, 100.6260903946856615 ) ) ;
#5255=CARTESIAN_POINT ( 'NONE',  ( -4.483927247898539470, -16.52544592524342804, 62.29057627198102409 ) ) ;
#5256=CARTESIAN_POINT ( 'NONE',  ( 5.049401038297881783, 19.05341960407617563, 82.29275706135229029 ) ) ;
#5257=CARTESIAN_POINT ( 'NONE',  ( -4.483927247898782831, 16.52544592524335698, 72.70942372801901854 ) ) ;
#5258=CARTESIAN_POINT ( 'NONE',  ( 18.67979575497178502, 10.72451020669898547, 114.1655762719810383 ) ) ;
#5259=CARTESIAN_POINT ( 'NONE',  ( -9.474510206698964154, 16.51473224551069663, 35.41557627198102409 ) ) ;
#5260=CARTESIAN_POINT ( 'NONE',  ( -9.564922557960796823, -16.46253265017161027, 52.08224293864768839 ) ) ;
#5262=CARTESIAN_POINT ( 'NONE',  ( -16.53943276465976808, -0.05219959533934237506, 78.75109039468568994 ) ) ;
#5265=ORIENTED_EDGE ( 'NONE', *, *, #135302, .F. ) ;
#5266=CARTESIAN_POINT ( 'NONE',  ( -5.153800228976607833, 19.02544592524334988, 22.70942372801899012 ) ) ;
#5269=CARTESIAN_POINT ( 'NONE',  ( 4.379528057220092307, 16.55341960407617563, 22.29275706135235069 ) ) ;
#5270=B_SPLINE_CURVE_WITH_KNOTS ( 'NONE', 3,
 ( #154319, #121986, #64295, #157300, #139139, #155312 ),
 .UNSPECIFIED., .F., .F.,
 ( 4, 2, 4 ),
 ( 0.007228050697041574386, 0.007608510107495053409, 0.007988969517948531565 ),
 .UNSPECIFIED. ) ;
#5271=CARTESIAN_POINT ( 'NONE',  ( -15.72974639402197994, 15.80617190586746368, 45.62390960531436690 ) ) ;
#5272=CARTESIAN_POINT ( 'NONE',  ( -9.564922557961040184, 16.46253265017147172, 47.91775706135233293 ) ) ;
#5273=CARTESIAN_POINT ( 'NONE',  ( -16.52544592524335698, -4.483927247898792601, 33.95942372801901143 ) ) ;
#5274=CARTESIAN_POINT ( 'NONE',  ( 13.89961937509977652, -13.97604488694527269, 48.12390960531435979 ) ) ;
#5275=CARTESIAN_POINT ( 'NONE',  ( -9.474510206698964154, 16.51473224551069663, 55.41557627198103120 ) ) ;
#5276=CARTESIAN_POINT ( 'NONE',  ( 5.823673210054125526, 21.52544592524343514, 89.79057627198103830 ) ) ;
#5277=CARTESIAN_POINT ( 'NONE',  ( -19.03943276465977164, 0.05219959533909376836, 106.2489096053143669 ) ) ;
#5278=CARTESIAN_POINT ( 'NONE',  ( 19.05341960407611168, 5.049401038298154454, 48.95724293864768129 ) ) ;
#5280=CARTESIAN_POINT ( 'NONE',  ( -5.153800228976607833, 19.02544592524334988, 92.70942372801901854 ) ) ;
#5281=CARTESIAN_POINT ( 'NONE',  ( -4.483927247898539470, -16.52544592524342804, 62.29057627198102409 ) ) ;
#5282=CARTESIAN_POINT ( 'NONE',  ( -9.474510206698720793, -16.51473224551083518, 19.58442372801899722 ) ) ;
#5283=CARTESIAN_POINT ( 'NONE',  ( 5.823673210054125526, 21.52544592524343514, 99.79057627198103830 ) ) ;
#5284=CARTESIAN_POINT ( 'NONE',  ( 18.62759615963255655, 10.81492255796105972, 81.66775706135236135 ) ) ;
#5285=CARTESIAN_POINT ( 'NONE',  ( 16.46253265017160672, -9.564922557960803928, 23.33224293864769194 ) ) ;
#5286=CARTESIAN_POINT ( 'NONE',  ( -18.62759615963255300, -10.81492255796106328, 84.16775706135234714 ) ) ;
#5287=CARTESIAN_POINT ( 'NONE',  ( -14.34966873604972548, 8.224510206698743886, 113.3344237280190328 ) ) ;
#5288=CARTESIAN_POINT ( 'NONE',  ( 18.62759615963255655, 10.81492255796105972, 76.66775706135234714 ) ) ;
#5289=CARTESIAN_POINT ( 'NONE',  ( -5.049401038298153566, 19.05341960407611168, 65.20724293864765286 ) ) ;
#5290=CARTESIAN_POINT ( 'NONE',  ( -10.81492255796105439, 18.62759615963255655, 37.91775706135235424 ) ) ;
#5291=CARTESIAN_POINT ( 'NONE',  ( 16.46253265017160672, -9.564922557960803928, 78.33224293864769550 ) ) ;
#5292=CARTESIAN_POINT ( 'NONE',  ( 8.224510206698953496, -14.34966873604960469, 92.91557627198103830 ) ) ;
#5293=CARTESIAN_POINT ( 'NONE',  ( -12.06949235617756955, 12.14591786802309770, 60.62390960531437401 ) ) ;
#5294=CARTESIAN_POINT ( 'NONE',  ( -10.81492255796078084, -18.62759615963271287, 77.08224293864769550 ) ) ;
#5295=CARTESIAN_POINT ( 'NONE',  ( -13.89961937509977652, 13.97604488694528158, 60.62390960531436690 ) ) ;
#5296=CARTESIAN_POINT ( 'NONE',  ( 10.81492255796078972, 18.62759615963270932, 89.58224293864768129 ) ) ;
#5297=CARTESIAN_POINT ( 'NONE',  ( 16.51473224551083163, -9.474510206698727899, 60.83442372801900433 ) ) ;
#5298=CARTESIAN_POINT ( 'NONE',  ( 17.50000000000000000, 5.499999999999997335, 36.70309617465829177 ) ) ;
#5299=CARTESIAN_POINT ( 'NONE',  ( -8.314922557960811034, -14.29746914071050412, 77.08224293864769550 ) ) ;
#5300=CARTESIAN_POINT ( 'NONE',  ( -5.719274019375978568, 21.55341960407610458, 50.20724293864769550 ) ) ;
#5302=CARTESIAN_POINT ( 'NONE',  ( 16.53943276465976808, 0.05219959533934440121, 96.25109039468568994 ) ) ;
#5304=CARTESIAN_POINT ( 'NONE',  ( 16.46253265017146816, 9.564922557961045513, 96.66775706135233293 ) ) ;
#5305=CARTESIAN_POINT ( 'NONE',  ( 14.29746914071049879, -8.314922557960816363, 68.33224293864769550 ) ) ;
#5306=CARTESIAN_POINT ( 'NONE',  ( -17.50000000000001066, -5.499999999999943157, 86.28230962303568674 ) ) ;
#5307=CARTESIAN_POINT ( 'NONE',  ( -5.049401038298153566, 19.05341960407611168, 55.20724293864769550 ) ) ;
#5308=CARTESIAN_POINT ( 'NONE',  ( 14.29746914071049879, -8.314922557960816363, 58.33224293864768839 ) ) ;
#5309=CARTESIAN_POINT ( 'NONE',  ( -13.89961937509977652, 13.97604488694528158, 105.6239096053143527 ) ) ;
#5310=CARTESIAN_POINT ( 'NONE',  ( -13.97604488694547697, 13.89961937509957934, 73.12609039468568994 ) ) ;
#5311=CARTESIAN_POINT ( 'NONE',  ( -19.02544592524342804, 5.153800228976336051, 66.04057627198103830 ) ) ;
#5312=CARTESIAN_POINT ( 'NONE',  ( 13.89961937509977652, -13.97604488694527269, 88.12390960531438111 ) ) ;
#5313=CARTESIAN_POINT ( 'NONE',  ( 19.05341960407611168, 5.049401038298154454, 78.95724293864769550 ) ) ;
#5314=CARTESIAN_POINT ( 'NONE',  ( -5.823673210054116645, -21.52544592524344225, 67.29057627198103830 ) ) ;
#5315=CARTESIAN_POINT ( 'NONE',  ( -12.14591786802326823, 12.06949235617739902, 63.12609039468568994 ) ) ;
#5317=CARTESIAN_POINT ( 'NONE',  ( 9.564922557960805705, 16.46253265017160317, 44.58224293864769550 ) ) ;
#5318=CARTESIAN_POINT ( 'NONE',  ( 5.823673210054125526, 21.52544592524343514, 49.79057627198102409 ) ) ;
#5319=CARTESIAN_POINT ( 'NONE',  ( 9.474510206698729675, 16.51473224551082808, 92.08442372801900433 ) ) ;
#5320=CARTESIAN_POINT ( 'NONE',  ( -16.52544592524342804, 4.483927247898546575, 31.04057627198102409 ) ) ;
#5321=CARTESIAN_POINT ( 'NONE',  ( -10.72451020669870658, -18.67979575497194134, 29.58442372801901854 ) ) ;
#5322=CARTESIAN_POINT ( 'NONE',  ( 19.02544592524334988, 5.153800228976608722, 31.45942372801900433 ) ) ;
#5323=CARTESIAN_POINT ( 'NONE',  ( -0.05219959533934338120, 16.53943276465976808, 62.50109039468568284 ) ) ;
#5324=CARTESIAN_POINT ( 'NONE',  ( -0.05219959533934338120, 16.53943276465976808, 97.50109039468567573 ) ) ;
#5326=CARTESIAN_POINT ( 'NONE',  ( 4.483927247898790824, -16.52544592524335698, 80.20942372801901854 ) ) ;
#5327=CARTESIAN_POINT ( 'NONE',  ( 21.52544592524344225, -5.823673210054117533, 23.54057627198102765 ) ) ;
#5328=CARTESIAN_POINT ( 'NONE',  ( -12.06949235617739369, -12.14591786802326823, 29.37609039468568284 ) ) ;
#5329=CARTESIAN_POINT ( 'NONE',  ( 19.05341960407611168, 5.049401038298154454, 43.95724293864769550 ) ) ;
#5330=CARTESIAN_POINT ( 'NONE',  ( 9.564922557960805705, 16.46253265017160317, 49.58224293864770260 ) ) ;
#5331=CARTESIAN_POINT ( 'NONE',  ( 19.05341960407611168, 5.049401038298154454, 63.95724293864769550 ) ) ;
#5332=CARTESIAN_POINT ( 'NONE',  ( -0.05219959533937732626, 21.53943276465977519, 42.50109039468567573 ) ) ;
#5333=CARTESIAN_POINT ( 'NONE',  ( -8.224510206698735004, -14.34966873604973081, 49.58442372801901143 ) ) ;
#5334=CARTESIAN_POINT ( 'NONE',  ( -14.29746914071037622, -8.314922557961029526, 109.1677570613523613 ) ) ;
#5335=CARTESIAN_POINT ( 'NONE',  ( -19.02544592524342804, 5.153800228976336051, 31.04057627198102409 ) ) ;
#5336=CARTESIAN_POINT ( 'NONE',  ( -0.05219959533937732626, 21.53943276465977519, 107.5010903946856899 ) ) ;
#5337=CARTESIAN_POINT ( 'NONE',  ( -13.89961937509957401, -13.97604488694547875, 109.3760903946856331 ) ) ;
#5338=CARTESIAN_POINT ( 'NONE',  ( -19.03943276465977164, -0.05219959533935918106, 63.75109039468566863 ) ) ;
#5339=CARTESIAN_POINT ( 'NONE',  ( 12.14591786802309770, 12.06949235617756955, 64.37390960531435269 ) ) ;
#5340=CARTESIAN_POINT ( 'NONE',  ( 16.46253265017160672, -9.564922557960803928, 33.33224293864770260 ) ) ;
#5341=CARTESIAN_POINT ( 'NONE',  ( -0.05219959533936034679, 19.03943276465977164, 67.50109039468566152 ) ) ;
#5342=CARTESIAN_POINT ( 'NONE',  ( 17.48853670773245028, -5.747243402303091386, 91.16671299749991420 ) ) ;
#5343=CARTESIAN_POINT ( 'NONE',  ( -10.72451020669870658, -18.67979575497194134, 79.58442372801903275 ) ) ;
#5344=CARTESIAN_POINT ( 'NONE',  ( -4.379528057220086978, -16.55341960407618274, 34.79275706135235424 ) ) ;
#5345=CARTESIAN_POINT ( 'NONE',  ( 18.22780087662119897, -5.500000000000096811, 58.51763182126894947 ) ) ;
#5346=CARTESIAN_POINT ( 'NONE',  ( 10.81492255796078972, 18.62759615963270932, 39.58224293864769550 ) ) ;
#5347=CARTESIAN_POINT ( 'NONE',  ( -0.05219959533934338120, 16.53943276465976808, 32.50109039468568284 ) ) ;
#5348=CARTESIAN_POINT ( 'NONE',  ( 19.03943276465977164, -0.05219959533909143690, 23.74890960531435269 ) ) ;
#5349=CARTESIAN_POINT ( 'NONE',  ( 13.97604488694548053, -13.89961937509957401, 30.62609039468566863 ) ) ;
#5351=CARTESIAN_POINT ( 'NONE',  ( -19.03943276465977164, 0.05219959533909376836, 36.24890960531436690 ) ) ;
#5352=CARTESIAN_POINT ( 'NONE',  ( 13.89961937509957579, 13.97604488694547520, 56.87609039468566863 ) ) ;
#5353=CARTESIAN_POINT ( 'NONE',  ( -19.02544592524342804, 5.153800228976336051, 61.04057627198103120 ) ) ;
#5355=CARTESIAN_POINT ( 'NONE',  ( -19.25176906914649422, -5.499999999999741540, 55.99927264242278824 ) ) ;
#5356=CARTESIAN_POINT ( 'NONE',  ( -21.55341960407619339, 5.719274019375674811, 113.5427570613523756 ) ) ;
#5357=CARTESIAN_POINT ( 'NONE',  ( 14.34966873604960469, 8.224510206698951720, 24.16557627198103120 ) ) ;
#5358=CARTESIAN_POINT ( 'NONE',  ( -13.97604488694527625, -13.89961937509977652, 31.87390960531435979 ) ) ;
#5359=CARTESIAN_POINT ( 'NONE',  ( -19.03943276465977164, 0.05219959533909376836, 96.24890960531436690 ) ) ;
#5360=CARTESIAN_POINT ( 'NONE',  ( 21.52544592524334988, 5.823673210054432836, 71.45942372801901854 ) ) ;
#5361=CARTESIAN_POINT ( 'NONE',  ( 16.51473224551069308, 9.474510206698969483, 44.16557627198103120 ) ) ;
#5362=CARTESIAN_POINT ( 'NONE',  ( -15.72974639402176322, -15.80617190586768395, 64.37609039468568994 ) ) ;
#5363=CARTESIAN_POINT ( 'NONE',  ( 13.97604488694548053, -13.89961937509957401, 95.62609039468563310 ) ) ;
#5364=CARTESIAN_POINT ( 'NONE',  ( 10.72451020669898902, -18.67979575497178502, 22.91557627198102765 ) ) ;
#5365=CARTESIAN_POINT ( 'NONE',  ( -16.46253265017160317, 9.564922557960807481, 30.83224293864769550 ) ) ;
#5366=CARTESIAN_POINT ( 'NONE',  ( -18.67979575497178146, -10.72451020669898902, 106.6655762719810383 ) ) ;
#5367=CARTESIAN_POINT ( 'NONE',  ( 19.03943276465977164, 0.05219959533936151252, 31.25109039468566863 ) ) ;
#5368=CARTESIAN_POINT ( 'NONE',  ( 14.34966873604960469, 8.224510206698951720, 104.1655762719810241 ) ) ;
#5369=CARTESIAN_POINT ( 'NONE',  ( -19.03943276465977164, 0.05219959533909376836, 61.24890960531436690 ) ) ;
#5370=CARTESIAN_POINT ( 'NONE',  ( -5.153800228976607833, 19.02544592524334988, 107.7094237280189759 ) ) ;
#5371=CARTESIAN_POINT ( 'NONE',  ( 4.379528057220339221, -16.55341960407611168, 72.70724293864769550 ) ) ;
#5372=CARTESIAN_POINT ( 'NONE',  ( -5.049401038298153566, 19.05341960407611168, 115.2072429386477097 ) ) ;
#5373=CARTESIAN_POINT ( 'NONE',  ( -13.97604488694547697, 13.89961937509957934, 83.12609039468564731 ) ) ;
#5374=CARTESIAN_POINT ( 'NONE',  ( 21.52544592524344225, -5.823673210054117533, 88.54057627198103830 ) ) ;
#5375=CARTESIAN_POINT ( 'NONE',  ( 21.52544592524334988, 5.823673210054432836, 41.45942372801901143 ) ) ;
#5376=CARTESIAN_POINT ( 'NONE',  ( -8.224510206698735004, -14.34966873604973081, 49.58442372801901143 ) ) ;
#5377=CARTESIAN_POINT ( 'NONE',  ( 4.483927247898790824, -16.52544592524335698, 50.20942372801901854 ) ) ;
#5378=CARTESIAN_POINT ( 'NONE',  ( 5.823673210054444382, -21.52544592524334988, 55.20942372801902565 ) ) ;
#5379=CARTESIAN_POINT ( 'NONE',  ( -21.53943276465977519, 0.05219959533907696930, 61.24890960531435979 ) ) ;
#5380=( BOUNDED_CURVE ( )  B_SPLINE_CURVE ( 2, ( #51492, #21152, #144489, #25177, #86819, #148506, #52481, #66656, #115160, #99978, #113153, #114140, #37315 ),
 .UNSPECIFIED., .F., .F. ) 
 B_SPLINE_CURVE_WITH_KNOTS ( ( 3, 2, 2, 2, 2, 2, 3 ),
 ( 0.2393182215122932333, 0.2412280701754385970, 0.2456140350877192846, 0.2500000000000000000, 0.2543859649122807154, 0.2587719298245614308, 0.2607274583097970999 ),
 .UNSPECIFIED. ) 
 CURVE ( )  GEOMETRIC_REPRESENTATION_ITEM ( )  RATIONAL_B_SPLINE_CURVE ( ( 0.9832469066685285419, 0.9851625545550100060, 1.000000000000000000, 0.9659258262890683122, 1.000000000000000000, 0.9659258262890683122, 1.000000000000000000, 0.9659258262890683122, 1.000000000000000000, 0.9659258262890683122, 1.000000000000000000, 0.9848076720550081875, 0.9831626618144004848 ) ) 
 REPRESENTATION_ITEM ( '' )  );
#5381=CARTESIAN_POINT ( 'NONE',  ( 9.564922557960805705, 16.46253265017160317, 49.58224293864770260 ) ) ;
#5383=CARTESIAN_POINT ( 'NONE',  ( 14.34966873604972726, -8.224510206698740333, 75.83442372801900433 ) ) ;
#5384=CARTESIAN_POINT ( 'NONE',  ( -5.823673210054116645, -21.52544592524344225, 102.2905762719810383 ) ) ;
#5385=CARTESIAN_POINT ( 'NONE',  ( -12.14591786802309592, -12.06949235617757132, 56.87390960531436690 ) ) ;
#5386=CARTESIAN_POINT ( 'NONE',  ( 14.29746914071037800, 8.314922557961029526, 66.66775706135234714 ) ) ;
#5387=CARTESIAN_POINT ( 'NONE',  ( 19.02544592524334988, 5.153800228976608722, 96.45942372801897591 ) ) ;
#5388=CARTESIAN_POINT ( 'NONE',  ( -10.72451020669898014, 18.67979575497178502, 100.4155762719810241 ) ) ;
#5389=CARTESIAN_POINT ( 'NONE',  ( -8.224510206698948167, 14.34966873604960824, 45.41557627198103830 ) ) ;
#5391=CARTESIAN_POINT ( 'NONE',  ( 18.22780087662123805, -5.499999999999976019, 93.51763182126896368 ) ) ;
#5392=CARTESIAN_POINT ( 'NONE',  ( 18.62759615963271287, -10.81492255796078972, 78.33224293864770971 ) ) ;
#5393=CARTESIAN_POINT ( 'NONE',  ( -8.224510206698948167, 14.34966873604960824, 25.41557627198103120 ) ) ;
#5396=CARTESIAN_POINT ( 'NONE',  ( 5.719274019375991003, -21.55341960407610458, 107.7072429386476955 ) ) ;
#5397=CARTESIAN_POINT ( 'NONE',  ( -18.67979575497178146, -10.72451020669898902, 111.6655762719810525 ) ) ;
#5398=CARTESIAN_POINT ( 'NONE',  ( 8.224510206698953496, -14.34966873604960469, 42.91557627198103120 ) ) ;
#5399=CARTESIAN_POINT ( 'NONE',  ( 12.14591786802327356, -12.06949235617739191, 50.62609039468568994 ) ) ;
#5400=CARTESIAN_POINT ( 'NONE',  ( 19.02544592524343514, -5.153800228976328945, 53.54057627198102409 ) ) ;
#5401=CARTESIAN_POINT ( 'NONE',  ( 0.05219959533909260263, 19.03943276465977164, 69.99890960531435269 ) ) ;
#5403=CARTESIAN_POINT ( 'NONE',  ( 10.72451020669898902, -18.67979575497178502, 37.91557627198102409 ) ) ;
#5405=CARTESIAN_POINT ( 'NONE',  ( -5.153800228976607833, 19.02544592524334988, 107.7094237280189759 ) ) ;
#5406=CARTESIAN_POINT ( 'NONE',  ( -13.97604488694547697, 13.89961937509957934, 53.12609039468565442 ) ) ;
#5407=CARTESIAN_POINT ( 'NONE',  ( 21.53943276465977519, -0.05219959533907433946, 103.7489096053143669 ) ) ;
#5409=CARTESIAN_POINT ( 'NONE',  ( -8.314922557960811034, -14.29746914071050412, 32.08224293864769550 ) ) ;
#5410=CARTESIAN_POINT ( 'NONE',  ( 19.02544592524343514, -5.153800228976328945, 78.54057627198099567 ) ) ;
#5411=CARTESIAN_POINT ( 'NONE',  ( 21.52544592524344225, -5.823673210054117533, 43.54057627198103830 ) ) ;
#5412=CARTESIAN_POINT ( 'NONE',  ( -0.05219959533907301413, -21.53943276465977519, 87.49890960531436690 ) ) ;
#5413=CARTESIAN_POINT ( 'NONE',  ( 8.224510206698742110, 14.34966873604972548, 22.08442372801901143 ) ) ;
#5414=CARTESIAN_POINT ( 'NONE',  ( -9.474510206698964154, 16.51473224551069663, 115.4155762719810241 ) ) ;
#5415=CARTESIAN_POINT ( 'NONE',  ( 15.80617190586769283, -15.72974639402175789, 70.62609039468567573 ) ) ;
#5416=CARTESIAN_POINT ( 'NONE',  ( 16.46253265017160672, -9.564922557960803928, 78.33224293864769550 ) ) ;
#5417=CARTESIAN_POINT ( 'NONE',  ( 5.153800228976335163, 19.02544592524342804, 24.79057627198102765 ) ) ;
#5418=CARTESIAN_POINT ( 'NONE',  ( 0.05219959533909260263, 19.03943276465977164, 79.99890960531436690 ) ) ;
#5419=CARTESIAN_POINT ( 'NONE',  ( 8.314922557960818139, 14.29746914071049879, 94.58224293864769550 ) ) ;
#5421=CARTESIAN_POINT ( 'NONE',  ( -19.05341960407617563, 5.049401038297882671, 103.5427570613523329 ) ) ;
#5423=CARTESIAN_POINT ( 'NONE',  ( 16.46253265017160672, -9.564922557960803928, 78.33224293864769550 ) ) ;
#5424=CARTESIAN_POINT ( 'NONE',  ( 10.72451020669871369, 18.67979575497193778, 82.08442372801901854 ) ) ;
#5425=CARTESIAN_POINT ( 'NONE',  ( -16.46253265017160317, 9.564922557960807481, 110.8322429386476955 ) ) ;
#5426=CARTESIAN_POINT ( 'NONE',  ( -16.55341960407617563, 4.379528057220093196, 78.54275706135236135 ) ) ;
#5427=CARTESIAN_POINT ( 'NONE',  ( -17.26172910966779384, -6.454744622555833367, 74.19353091350777163 ) ) ;
#5428=CARTESIAN_POINT ( 'NONE',  ( -5.153800228976607833, 19.02544592524334988, 52.70942372801900433 ) ) ;
#5429=CARTESIAN_POINT ( 'NONE',  ( -0.05219959533936034679, 19.03943276465977164, 22.50109039468566152 ) ) ;
#5433=CARTESIAN_POINT ( 'NONE',  ( 12.06949235617757843, -12.14591786802309237, 28.12390960531435979 ) ) ;
#5435=CARTESIAN_POINT ( 'NONE',  ( -4.483927247898782831, 16.52544592524335698, 112.7094237280190328 ) ) ;
#5437=CARTESIAN_POINT ( 'NONE',  ( -0.05219959533934338120, 16.53943276465976808, 87.50109039468568994 ) ) ;
#5438=CARTESIAN_POINT ( 'NONE',  ( 15.80617190586769283, -15.72974639402175789, 100.6260903946857184 ) ) ;
#5439=CARTESIAN_POINT ( 'NONE',  ( 13.89961937509957401, 13.97604488694547697, 101.8760903946856331 ) ) ;
#5440=CARTESIAN_POINT ( 'NONE',  ( 21.55341960407619695, -5.719274019375665929, 61.04275706135234714 ) ) ;
#5441=CARTESIAN_POINT ( 'NONE',  ( 13.89961937509957401, 13.97604488694547697, 41.87609039468566152 ) ) ;
#5442=CARTESIAN_POINT ( 'NONE',  ( 16.46253265017160672, -9.564922557960803928, 83.33224293864768129 ) ) ;
#5443=CARTESIAN_POINT ( 'NONE',  ( -13.97604488694527625, -13.89961937509977652, 51.87390960531436690 ) ) ;
#5445=CARTESIAN_POINT ( 'NONE',  ( -0.05219959533907301413, -21.53943276465977519, 92.49890960531436690 ) ) ;
#5447=CARTESIAN_POINT ( 'NONE',  ( 18.67979575497178502, 10.72451020669898547, 49.16557627198102409 ) ) ;
#5448=CARTESIAN_POINT ( 'NONE',  ( 13.97604488694527802, 13.89961937509977652, 44.37390960531435269 ) ) ;
#5449=CARTESIAN_POINT ( 'NONE',  ( 14.29746914071037800, 8.314922557961029526, 66.66775706135234714 ) ) ;
#5452=CARTESIAN_POINT ( 'NONE',  ( -21.53943276465977519, -0.05219959533937600094, 38.75109039468567573 ) ) ;
#5453=CARTESIAN_POINT ( 'NONE',  ( -16.52544592524342804, 4.483927247898546575, 81.04057627198102409 ) ) ;
#5455=CARTESIAN_POINT ( 'NONE',  ( -4.483927247898782831, 16.52544592524335698, 42.70942372801901854 ) ) ;
#5456=CARTESIAN_POINT ( 'NONE',  ( 8.224510206698953496, -14.34966873604960469, 107.9155762719810241 ) ) ;
#5457=CARTESIAN_POINT ( 'NONE',  ( 19.02544592524334988, 5.153800228976608722, 51.45942372801900433 ) ) ;
#5458=VECTOR ( 'NONE', #88989, 1000.000000000000000 ) ;
#5459=CARTESIAN_POINT ( 'NONE',  ( -16.52544592524342804, 4.483927247898546575, 71.04057627198103830 ) ) ;
#5460=CARTESIAN_POINT ( 'NONE',  ( 21.52544592524334988, 5.823673210054432836, 36.45942372801901143 ) ) ;
#5461=CARTESIAN_POINT ( 'NONE',  ( 19.05341960407611168, 5.049401038298154454, 28.95724293864769550 ) ) ;
#5462=CARTESIAN_POINT ( 'NONE',  ( 5.823673210054125526, 21.52544592524343514, 84.79057627198102409 ) ) ;
#5463=CARTESIAN_POINT ( 'NONE',  ( 0.05219959533909260263, 19.03943276465977164, 99.99890960531436690 ) ) ;
#5464=CARTESIAN_POINT ( 'NONE',  ( 14.29746914071049879, -8.314922557960816363, 68.33224293864769550 ) ) ;
#5467=CARTESIAN_POINT ( 'NONE',  ( 13.89961937509957401, 13.97604488694547697, 86.87609039468567573 ) ) ;
#5468=CARTESIAN_POINT ( 'NONE',  ( -21.53943276465977519, -0.05219959533937600094, 28.75109039468567929 ) ) ;
#5469=CARTESIAN_POINT ( 'NONE',  ( -19.02544592524342804, 5.153800228976336051, 66.04057627198103830 ) ) ;
#5470=CARTESIAN_POINT ( 'NONE',  ( 0.05219959533936267826, -19.03943276465977164, 60.00109039468566863 ) ) ;
#5471=CARTESIAN_POINT ( 'NONE',  ( 9.564922557960805705, 16.46253265017160317, 44.58224293864769550 ) ) ;
#5472=CARTESIAN_POINT ( 'NONE',  ( -8.224510206698948167, 14.34966873604960824, 60.41557627198102409 ) ) ;
#5473=CARTESIAN_POINT ( 'NONE',  ( -8.224510206698948167, 14.34966873604960824, 55.41557627198102409 ) ) ;
#5474=CARTESIAN_POINT ( 'NONE',  ( 13.89961937509977652, -13.97604488694527269, 73.12390960531436690 ) ) ;
#5475=CARTESIAN_POINT ( 'NONE',  ( 18.67979575497178502, 10.72451020669898547, 89.16557627198102409 ) ) ;
#5476=CARTESIAN_POINT ( 'NONE',  ( 13.89961937509977652, -13.97604488694527269, 68.12390960531436690 ) ) ;
#5477=CARTESIAN_POINT ( 'NONE',  ( -18.62759615963270932, 10.81492255796079327, 85.83224293864768129 ) ) ;
#5478=CARTESIAN_POINT ( 'NONE',  ( -0.05219959533937732626, 21.53943276465977519, 112.5010903946857042 ) ) ;
#5479=CARTESIAN_POINT ( 'NONE',  ( -17.49999999999999645, -7.500000000000000888, 120.0000000000000142 ) ) ;
#5480=CARTESIAN_POINT ( 'NONE',  ( -0.05219959533910754901, -16.53943276465976808, 22.49890960531436335 ) ) ;
#5481=CARTESIAN_POINT ( 'NONE',  ( -0.05219959533910754901, -16.53943276465976808, 97.49890960531436690 ) ) ;
#5482=CARTESIAN_POINT ( 'NONE',  ( 13.89961937509957401, 13.97604488694547697, 91.87609039468567573 ) ) ;
#5483=EDGE_LOOP ( 'NONE', ( #52442, #128612, #179339 ) ) ;
#5484=CARTESIAN_POINT ( 'NONE',  ( 21.52544592524334988, 5.823673210054432836, 21.45942372801901499 ) ) ;
#5485=CARTESIAN_POINT ( 'NONE',  ( 9.564922557961047289, -16.46253265017146816, 50.41775706135233293 ) ) ;
#5486=CARTESIAN_POINT ( 'NONE',  ( -14.34966873604972548, 8.224510206698743886, 108.3344237280190185 ) ) ;
#5487=CARTESIAN_POINT ( 'NONE',  ( 16.46253265017146816, 9.564922557961045513, 46.66775706135233293 ) ) ;
#5488=CARTESIAN_POINT ( 'NONE',  ( 5.049401038298161559, -19.05341960407611168, 107.7072429386476955 ) ) ;
#5489=CARTESIAN_POINT ( 'NONE',  ( -8.314922557960811034, -14.29746914071050412, 62.08224293864769550 ) ) ;
#5490=CARTESIAN_POINT ( 'NONE',  ( -19.53037848336980886, 5.499999999999898748, 49.85532783611443364 ) ) ;
#5491=CARTESIAN_POINT ( 'NONE',  ( 13.89961937509977652, -13.97604488694527269, 33.12390960531434558 ) ) ;
#5492=CARTESIAN_POINT ( 'NONE',  ( 21.52544592524334988, 5.823673210054432836, 111.4594237280190328 ) ) ;
#5493=CARTESIAN_POINT ( 'NONE',  ( -4.379528057220086978, -16.55341960407618274, 79.79275706135236135 ) ) ;
#5494=CARTESIAN_POINT ( 'NONE',  ( -21.53943276465977519, -0.05219959533937600094, 43.75109039468568284 ) ) ;
#5495=CARTESIAN_POINT ( 'NONE',  ( -14.34966873604972548, 8.224510206698743886, 43.33442372801901143 ) ) ;
#5496=CARTESIAN_POINT ( 'NONE',  ( -9.564922557960796823, -16.46253265017161027, 102.0822429386477097 ) ) ;
#5497=CARTESIAN_POINT ( 'NONE',  ( 0.05219959533909260263, 19.03943276465977164, 54.99890960531435979 ) ) ;
#5498=CARTESIAN_POINT ( 'NONE',  ( -9.474510206698964154, 16.51473224551069663, 70.41557627198102409 ) ) ;
#5500=CARTESIAN_POINT ( 'NONE',  ( -12.06949235617739369, -12.14591786802326823, 49.37609039468569705 ) ) ;
#5501=CARTESIAN_POINT ( 'NONE',  ( 16.55341960407611168, 4.379528057220329451, 103.9572429386476813 ) ) ;
#5502=CARTESIAN_POINT ( 'NONE',  ( 12.14591786802309770, 12.06949235617756955, 24.37390960531435979 ) ) ;
#5504=CARTESIAN_POINT ( 'NONE',  ( -15.72974639402176322, -15.80617190586768395, 54.37609039468568994 ) ) ;
#5505=CARTESIAN_POINT ( 'NONE',  ( 16.46253265017160672, -9.564922557960803928, 88.33224293864769550 ) ) ;
#5506=CARTESIAN_POINT ( 'NONE',  ( -9.474510206698964154, 16.51473224551069663, 65.41557627198102409 ) ) ;
#5507=CARTESIAN_POINT ( 'NONE',  ( -5.153800228976328057, -19.02544592524343514, 97.29057627198099567 ) ) ;
#5509=CARTESIAN_POINT ( 'NONE',  ( 14.29746914071049879, -8.314922557960816363, 48.33224293864770260 ) ) ;
#5510=CARTESIAN_POINT ( 'NONE',  ( 4.379528057220339221, -16.55341960407611168, 22.70724293864769194 ) ) ;
#5511=CARTESIAN_POINT ( 'NONE',  ( -16.55341960407611168, -4.379528057220339221, 36.45724293864768839 ) ) ;
#5512=VERTEX_POINT ( 'NONE', #91590 ) ;
#5514=CARTESIAN_POINT ( 'NONE',  ( -5.153800228976328057, -19.02544592524343514, 67.29057627198102409 ) ) ;
#5515=CARTESIAN_POINT ( 'NONE',  ( 19.05341960407617918, -5.049401038297876454, 36.04275706135234003 ) ) ;
#5517=CARTESIAN_POINT ( 'NONE',  ( -5.153800228976328057, -19.02544592524343514, 67.29057627198102409 ) ) ;
#5518=CARTESIAN_POINT ( 'NONE',  ( -16.51473224551082808, 9.474510206698731452, 88.33442372801900433 ) ) ;
#5519=CARTESIAN_POINT ( 'NONE',  ( -8.314922557961024197, 14.29746914071037800, 62.91775706135236135 ) ) ;
#5521=CARTESIAN_POINT ( 'NONE',  ( -19.03943276465977164, 0.05219959533909376836, 96.24890960531436690 ) ) ;
#5522=CARTESIAN_POINT ( 'NONE',  ( 18.67979575497194134, -10.72451020669871369, 25.83442372801901499 ) ) ;
#5523=CARTESIAN_POINT ( 'NONE',  ( 16.46253265017146816, 9.564922557961045513, 86.66775706135233293 ) ) ;
#5524=CARTESIAN_POINT ( 'NONE',  ( 19.05341960407611168, 5.049401038298154454, 113.9572429386477097 ) ) ;
#5525=CARTESIAN_POINT ( 'NONE',  ( -9.564922557960796823, -16.46253265017161027, 42.08224293864769550 ) ) ;
#5526=CARTESIAN_POINT ( 'NONE',  ( -13.97604488694527625, -13.89961937509977652, 86.87390960531436690 ) ) ;
#5527=CARTESIAN_POINT ( 'NONE',  ( 12.06949235617757843, -12.14591786802309237, 53.12390960531436690 ) ) ;
#5528=CARTESIAN_POINT ( 'NONE',  ( -9.474510206698964154, 16.51473224551069663, 50.41557627198102409 ) ) ;
#5529=CARTESIAN_POINT ( 'NONE',  ( -5.049401038297874678, -19.05341960407617918, 69.79275706135233293 ) ) ;
#5530=ORIENTED_EDGE ( 'NONE', *, *, #127855, .T. ) ;
#5531=CARTESIAN_POINT ( 'NONE',  ( 12.06949235617757843, -12.14591786802309237, 83.12390960531436690 ) ) ;
#5532=CARTESIAN_POINT ( 'NONE',  ( -9.474510206698720793, -16.51473224551083518, 24.58442372801900078 ) ) ;
#5533=CARTESIAN_POINT ( 'NONE',  ( -9.564922557960796823, -16.46253265017161027, 72.08224293864770971 ) ) ;
#5534=CARTESIAN_POINT ( 'NONE',  ( -0.05219959533907301413, -21.53943276465977519, 57.49890960531435979 ) ) ;
#5535=CARTESIAN_POINT ( 'NONE',  ( -8.314922557960811034, -14.29746914071050412, 72.08224293864769550 ) ) ;
#5536=CARTESIAN_POINT ( 'NONE',  ( -9.474510206698720793, -16.51473224551083518, 24.58442372801900078 ) ) ;
#5537=CARTESIAN_POINT ( 'NONE',  ( 0.05219959533909260263, 19.03943276465977164, 109.9989096053143669 ) ) ;
#5538=CARTESIAN_POINT ( 'NONE',  ( 10.72451020669898902, -18.67979575497178502, 27.91557627198103830 ) ) ;
#5539=CARTESIAN_POINT ( 'NONE',  ( 19.02544592524343514, -5.153800228976328945, 48.54057627198103120 ) ) ;
#5540=CARTESIAN_POINT ( 'NONE',  ( 19.02544592524343514, -5.153800228976328945, 38.54057627198103120 ) ) ;
#5541=CARTESIAN_POINT ( 'NONE',  ( -12.06949235617756955, 12.14591786802309770, 95.62390960531436690 ) ) ;
#5542=CARTESIAN_POINT ( 'NONE',  ( -18.67979575497178146, -10.72451020669898902, 106.6655762719810383 ) ) ;
#5543=CARTESIAN_POINT ( 'NONE',  ( -19.03943276465977164, 0.05219959533909376836, 111.2489096053143669 ) ) ;
#5544=CARTESIAN_POINT ( 'NONE',  ( -15.80617190586768217, 15.72974639402176855, 23.12609039468567573 ) ) ;
#5545=CARTESIAN_POINT ( 'NONE',  ( -5.049401038298153566, 19.05341960407611168, 105.2072429386476671 ) ) ;
#5546=CARTESIAN_POINT ( 'NONE',  ( 9.474510206698971260, -16.51473224551069308, 22.91557627198102765 ) ) ;
#5547=CARTESIAN_POINT ( 'NONE',  ( 10.72451020669871369, 18.67979575497193778, 72.08442372801899012 ) ) ;
#5548=CARTESIAN_POINT ( 'NONE',  ( 5.719274019375991003, -21.55341960407610458, 92.70724293864770971 ) ) ;
#5549=CARTESIAN_POINT ( 'NONE',  ( 17.50000000000000000, -5.500000000000000888, 33.29690382534174375 ) ) ;
#5550=CARTESIAN_POINT ( 'NONE',  ( -5.153800228976328057, -19.02544592524343514, 52.29057627198101699 ) ) ;
#5552=CARTESIAN_POINT ( 'NONE',  ( 8.314922557961029526, -14.29746914071037800, 50.41775706135235424 ) ) ;
#5553=CARTESIAN_POINT ( 'NONE',  ( -4.379528057220328563, 16.55341960407611168, 110.2072429386477239 ) ) ;
#5555=CARTESIAN_POINT ( 'NONE',  ( -9.564922557960796823, -16.46253265017161027, 57.08224293864769550 ) ) ;
#5556=CARTESIAN_POINT ( 'NONE',  ( -14.34966873604960291, -8.224510206698953496, 91.66557627198103830 ) ) ;
#5557=CARTESIAN_POINT ( 'NONE',  ( 15.72974639402199770, -15.80617190586745480, 43.12390960531435269 ) ) ;
#5558=CARTESIAN_POINT ( 'NONE',  ( 14.29746914071049879, -8.314922557960816363, 68.33224293864769550 ) ) ;
#5559=CARTESIAN_POINT ( 'NONE',  ( -0.05219959533934338120, 16.53943276465976808, 22.50109039468567573 ) ) ;
#5560=CARTESIAN_POINT ( 'NONE',  ( 15.72974639402176855, 15.80617190586768217, 81.87609039468568994 ) ) ;
#5561=CARTESIAN_POINT ( 'NONE',  ( 17.40861289039004944, -6.110651285853252901, 76.12767529172570846 ) ) ;
#5562=CARTESIAN_POINT ( 'NONE',  ( -0.05219959533934338120, 16.53943276465976808, 97.50109039468567573 ) ) ;
#5563=CARTESIAN_POINT ( 'NONE',  ( -8.314922557960811034, -14.29746914071050412, 37.08224293864768129 ) ) ;
#5564=CARTESIAN_POINT ( 'NONE',  ( 19.03943276465977164, -0.05219959533909143690, 38.74890960531436690 ) ) ;
#5565=CARTESIAN_POINT ( 'NONE',  ( -16.51473224551069308, -9.474510206698971260, 86.66557627198102409 ) ) ;
#5566=CARTESIAN_POINT ( 'NONE',  ( 10.81492255796078972, 18.62759615963270932, 89.58224293864768129 ) ) ;
#5567=CARTESIAN_POINT ( 'NONE',  ( 8.314922557961029526, -14.29746914071037800, 45.41775706135234003 ) ) ;
#5568=CARTESIAN_POINT ( 'NONE',  ( 4.483927247898545687, 16.52544592524342804, 69.79057627198102409 ) ) ;
#5569=CARTESIAN_POINT ( 'NONE',  ( 18.67979575497194134, -10.72451020669871369, 80.83442372801901854 ) ) ;
#5570=CARTESIAN_POINT ( 'NONE',  ( -12.06949235617739369, -12.14591786802326823, 94.37609039468568994 ) ) ;
#5571=CARTESIAN_POINT ( 'NONE',  ( 17.31728774477213051, -6.344390552233675429, 48.31906651689307353 ) ) ;
#5572=CARTESIAN_POINT ( 'NONE',  ( -19.01529144963331674, -5.500000000000166978, 66.23431955728440812 ) ) ;
#5573=CARTESIAN_POINT ( 'NONE',  ( 16.53943276465976808, -0.05219959533910856209, 33.74890960531436690 ) ) ;
#5574=CARTESIAN_POINT ( 'NONE',  ( -14.29746914071037622, -8.314922557961029526, 69.16775706135234714 ) ) ;
#5575=CARTESIAN_POINT ( 'NONE',  ( 5.049401038298161559, -19.05341960407611168, 82.70724293864770971 ) ) ;
#5576=CARTESIAN_POINT ( 'NONE',  ( -19.02544592524342804, 5.153800228976336051, 96.04057627198103830 ) ) ;
#5577=CARTESIAN_POINT ( 'NONE',  ( 10.72451020669871369, 18.67979575497193778, 87.08442372801901854 ) ) ;
#5578=CARTESIAN_POINT ( 'NONE',  ( 8.224510206698742110, 14.34966873604972548, 87.08442372801901854 ) ) ;
#5579=CARTESIAN_POINT ( 'NONE',  ( -8.224510206698948167, 14.34966873604960824, 55.41557627198102409 ) ) ;
#5580=CARTESIAN_POINT ( 'NONE',  ( 13.89961937509977652, -13.97604488694527269, 63.12390960531435979 ) ) ;
#5581=ORIENTED_EDGE ( 'NONE', *, *, #50316, .F. ) ;
#5582=CARTESIAN_POINT ( 'NONE',  ( 19.03943276465977164, 0.05219959533936151252, 106.2510903946856615 ) ) ;
#5583=CARTESIAN_POINT ( 'NONE',  ( -4.379528057220328563, 16.55341960407611168, 110.2072429386477239 ) ) ;
#5584=CARTESIAN_POINT ( 'NONE',  ( -0.05219959533909027116, -19.03943276465977164, 72.49890960531435269 ) ) ;
#5585=CARTESIAN_POINT ( 'NONE',  ( -16.52544592524335698, -4.483927247898792601, 18.95942372801901143 ) ) ;
#5587=CARTESIAN_POINT ( 'NONE',  ( 5.153800228976615827, -19.02544592524334988, 20.20942372801899722 ) ) ;
#5588=CARTESIAN_POINT ( 'NONE',  ( -12.06949235617739369, -12.14591786802326823, 74.37609039468568994 ) ) ;
#5589=CARTESIAN_POINT ( 'NONE',  ( 19.02544592524334988, 5.153800228976608722, 106.4594237280190185 ) ) ;
#5590=CARTESIAN_POINT ( 'NONE',  ( -8.224510206698948167, 14.34966873604960824, 110.4155762719810383 ) ) ;
#5591=CARTESIAN_POINT ( 'NONE',  ( 0.05219959533934541429, -16.53943276465976808, 60.00109039468568284 ) ) ;
#5592=CARTESIAN_POINT ( 'NONE',  ( 4.379528057220092307, 16.55341960407617563, 52.29275706135236135 ) ) ;
#5593=CARTESIAN_POINT ( 'NONE',  ( -5.153800228976328057, -19.02544592524343514, 22.29057627198102765 ) ) ;
#5594=CARTESIAN_POINT ( 'NONE',  ( -16.46253265017146816, -9.564922557961047289, 64.16775706135233293 ) ) ;
#5595=CARTESIAN_POINT ( 'NONE',  ( -15.72974639402176322, -15.80617190586768395, 109.3760903946857042 ) ) ;
#5596=CARTESIAN_POINT ( 'NONE',  ( 19.05341960407611168, 5.049401038298154454, 33.95724293864769550 ) ) ;
#5597=CARTESIAN_POINT ( 'NONE',  ( 0.05219959533909260263, 19.03943276465977164, 84.99890960531436690 ) ) ;
#5598=CARTESIAN_POINT ( 'NONE',  ( 8.314922557960818139, 14.29746914071049879, 74.58224293864768129 ) ) ;
#5600=CARTESIAN_POINT ( 'NONE',  ( 5.153800228976615827, -19.02544592524334988, 35.20942372801899722 ) ) ;
#5601=CARTESIAN_POINT ( 'NONE',  ( -5.823673210054116645, -21.52544592524344225, 32.29057627198102409 ) ) ;
#5602=CARTESIAN_POINT ( 'NONE',  ( -16.46253265017146816, -9.564922557961047289, 19.16775706135233293 ) ) ;
#5603=CARTESIAN_POINT ( 'NONE',  ( -19.03943276465977164, 0.05219959533909376836, 86.24890960531436690 ) ) ;
#5604=CARTESIAN_POINT ( 'NONE',  ( -0.05219959533937732626, 21.53943276465977519, 112.5010903946857042 ) ) ;
#5605=CARTESIAN_POINT ( 'NONE',  ( -0.05219959533907301413, -21.53943276465977519, 62.49890960531436690 ) ) ;
#5606=CARTESIAN_POINT ( 'NONE',  ( -16.46253265017160317, 9.564922557960807481, 90.83224293864769550 ) ) ;
#5607=CARTESIAN_POINT ( 'NONE',  ( -19.03943276465977164, -0.05219959533935918106, 78.75109039468567573 ) ) ;
#5608=CARTESIAN_POINT ( 'NONE',  ( 19.03943276465977164, -0.05219959533909143690, 98.74890960531436690 ) ) ;
#5610=CARTESIAN_POINT ( 'NONE',  ( 9.474510206698729675, 16.51473224551082808, 102.0844237280190043 ) ) ;
#5611=CARTESIAN_POINT ( 'NONE',  ( 8.224510206698742110, 14.34966873604972548, 57.08442372801901854 ) ) ;
#5612=CARTESIAN_POINT ( 'NONE',  ( -16.53943276465976808, 0.05219959533911058130, 111.2489096053143669 ) ) ;
#5613=CARTESIAN_POINT ( 'NONE',  ( 9.564922557960805705, 16.46253265017160317, 79.58224293864769550 ) ) ;
#5614=CARTESIAN_POINT ( 'NONE',  ( 21.52544592524344225, -5.823673210054117533, 68.54057627198103830 ) ) ;
#5615=CARTESIAN_POINT ( 'NONE',  ( -4.379528057220086978, -16.55341960407618274, 34.79275706135235424 ) ) ;
#5616=CARTESIAN_POINT ( 'NONE',  ( -21.52544592524334988, -5.823673210054445271, 28.95942372801902209 ) ) ;
#5617=CARTESIAN_POINT ( 'NONE',  ( -15.72974639402176322, -15.80617190586768395, 84.37609039468570415 ) ) ;
#5618=CARTESIAN_POINT ( 'NONE',  ( -16.55341960407617563, 4.379528057220093196, 93.54275706135234714 ) ) ;
#5619=CARTESIAN_POINT ( 'NONE',  ( 16.46253265017160672, -9.564922557960803928, 93.33224293864769550 ) ) ;
#5620=CARTESIAN_POINT ( 'NONE',  ( -4.379528057220328563, 16.55341960407611168, 80.20724293864769550 ) ) ;
#5621=CARTESIAN_POINT ( 'NONE',  ( -16.53943276465976808, 0.05219959533911058130, 26.24890960531435624 ) ) ;
#5622=CARTESIAN_POINT ( 'NONE',  ( 9.564922557961047289, -16.46253265017146816, 75.41775706135234714 ) ) ;
#5624=CARTESIAN_POINT ( 'NONE',  ( -18.67979575497193778, 10.72451020669871902, 43.33442372801901143 ) ) ;
#5625=EDGE_CURVE ( 'NONE', #199940, #38283, #53651, .T. ) ;
#5626=CARTESIAN_POINT ( 'NONE',  ( -0.05219959533910754901, -16.53943276465976808, 87.49890960531436690 ) ) ;
#5627=CARTESIAN_POINT ( 'NONE',  ( -13.97604488694527625, -13.89961937509977652, 111.8739096053143243 ) ) ;
#5628=CARTESIAN_POINT ( 'NONE',  ( 12.14591786802327356, -12.06949235617739191, 105.6260903946856899 ) ) ;
#5629=CARTESIAN_POINT ( 'NONE',  ( -21.55341960407619339, 5.719274019375674811, 83.54275706135234714 ) ) ;
#5630=CARTESIAN_POINT ( 'NONE',  ( 0.05219959533934541429, -16.53943276465976808, 45.00109039468568284 ) ) ;
#5631=CARTESIAN_POINT ( 'NONE',  ( -18.67979575497193778, 10.72451020669871902, 43.33442372801901143 ) ) ;
#5632=ORIENTED_EDGE ( 'NONE', *, *, #5625, .T. ) ;
#5633=CARTESIAN_POINT ( 'NONE',  ( 18.62759615963255655, 10.81492255796105972, 21.66775706135235069 ) ) ;
#5634=CARTESIAN_POINT ( 'NONE',  ( 14.29746914071049879, -8.314922557960816363, 88.33224293864769550 ) ) ;
#5636=CARTESIAN_POINT ( 'NONE',  ( 12.06949235617757843, -12.14591786802309237, 63.12390960531435979 ) ) ;
#5637=CARTESIAN_POINT ( 'NONE',  ( -4.379528057220086978, -16.55341960407618274, 104.7927570613523898 ) ) ;
#5638=CARTESIAN_POINT ( 'NONE',  ( 16.51473224551069308, 9.474510206698969483, 34.16557627198102409 ) ) ;
#5639=CARTESIAN_POINT ( 'NONE',  ( -10.72451020669898014, 18.67979575497178502, 45.41557627198103830 ) ) ;
#5640=CARTESIAN_POINT ( 'NONE',  ( 4.379528057220339221, -16.55341960407611168, 72.70724293864769550 ) ) ;
#5641=CARTESIAN_POINT ( 'NONE',  ( -10.81492255796078084, -18.62759615963271287, 82.08224293864768129 ) ) ;
#5642=CARTESIAN_POINT ( 'NONE',  ( 5.153800228976335163, 19.02544592524342804, 84.79057627198099567 ) ) ;
#5643=CARTESIAN_POINT ( 'NONE',  ( -13.97604488694527625, -13.89961937509977652, 36.87390960531436690 ) ) ;
#5644=CARTESIAN_POINT ( 'NONE',  ( 19.03943276465977164, 0.05219959533936151252, 96.25109039468567573 ) ) ;
#5645=CARTESIAN_POINT ( 'NONE',  ( -10.81492255796078084, -18.62759615963271287, 37.08224293864768129 ) ) ;
#5646=CARTESIAN_POINT ( 'NONE',  ( -21.52544592524334988, -5.823673210054445271, 73.95942372801901854 ) ) ;
#5647=CARTESIAN_POINT ( 'NONE',  ( 16.51473224551069308, 9.474510206698969483, 59.16557627198102409 ) ) ;
#5648=CARTESIAN_POINT ( 'NONE',  ( -9.474510206698964154, 16.51473224551069663, 90.41557627198103830 ) ) ;
#5650=CARTESIAN_POINT ( 'NONE',  ( 12.06949235617739724, 12.14591786802326823, 66.87609039468568994 ) ) ;
#5651=CARTESIAN_POINT ( 'NONE',  ( -21.53943276465977519, -0.05219959533937600094, 48.75109039468568284 ) ) ;
#5652=ADVANCED_FACE ( 'NONE', ( #169444 ), #46105, .F. ) ;
#5653=CARTESIAN_POINT ( 'NONE',  ( 21.53943276465977519, 0.05219959533937863772, 76.25109039468568994 ) ) ;
#5654=CARTESIAN_POINT ( 'NONE',  ( 15.72974639402199770, -15.80617190586745480, 28.12390960531435979 ) ) ;
#5655=CARTESIAN_POINT ( 'NONE',  ( 0.05219959533907565091, 21.53943276465977519, 89.99890960531438111 ) ) ;
#5656=CARTESIAN_POINT ( 'NONE',  ( 18.67979575497194134, -10.72451020669871369, 25.83442372801901499 ) ) ;
#5657=CARTESIAN_POINT ( 'NONE',  ( -16.53943276465976808, -0.05219959533934237506, 58.75109039468568994 ) ) ;
#5658=CARTESIAN_POINT ( 'NONE',  ( 18.62759615963271287, -10.81492255796078972, 63.33224293864770260 ) ) ;
#5659=CARTESIAN_POINT ( 'NONE',  ( -19.02544592524334988, -5.153800228976617603, 18.95942372801899722 ) ) ;
#5660=CARTESIAN_POINT ( 'NONE',  ( -19.02544592524342804, 5.153800228976336051, 71.04057627198099567 ) ) ;
#5661=CARTESIAN_POINT ( 'NONE',  ( -16.52544592524335698, -4.483927247898792601, 103.9594237280190185 ) ) ;
#5663=CARTESIAN_POINT ( 'NONE',  ( 16.46253265017160672, -9.564922557960803928, 88.33224293864769550 ) ) ;
#5664=CARTESIAN_POINT ( 'NONE',  ( 4.379528057220092307, 16.55341960407617563, 37.29275706135235424 ) ) ;
#5665=CARTESIAN_POINT ( 'NONE',  ( 17.49999999999999645, 3.190838340304485321, 102.6087687570488498 ) ) ;
#5666=CARTESIAN_POINT ( 'NONE',  ( 5.153800228976615827, -19.02544592524334988, 80.20942372801901854 ) ) ;
#5667=CARTESIAN_POINT ( 'NONE',  ( 15.72974639402199770, -15.80617190586745480, 63.12390960531435979 ) ) ;
#5668=CARTESIAN_POINT ( 'NONE',  ( -8.314922557960811034, -14.29746914071050412, 22.08224293864769194 ) ) ;
#5669=CARTESIAN_POINT ( 'NONE',  ( 19.03943276465977164, 0.05219959533936151252, 96.25109039468567573 ) ) ;
#5670=CARTESIAN_POINT ( 'NONE',  ( -17.58332526062525858, 7.635886036038558977, 40.92334959558466778 ) ) ;
#5671=CARTESIAN_POINT ( 'NONE',  ( -5.153800228976607833, 19.02544592524334988, 97.70942372801900433 ) ) ;
#5672=CARTESIAN_POINT ( 'NONE',  ( -15.80617190586745835, -15.72974639402198527, 86.87390960531438111 ) ) ;
#5673=CARTESIAN_POINT ( 'NONE',  ( 19.02544592524334988, 5.153800228976608722, 61.45942372801900433 ) ) ;
#5675=CARTESIAN_POINT ( 'NONE',  ( 5.153800228976335163, 19.02544592524342804, 54.79057627198103120 ) ) ;
#5676=CARTESIAN_POINT ( 'NONE',  ( 8.224510206698953496, -14.34966873604960469, 57.91557627198103120 ) ) ;
#5677=CARTESIAN_POINT ( 'NONE',  ( 19.03943276465977164, -0.05219959533909143690, 48.74890960531435979 ) ) ;
#5678=CARTESIAN_POINT ( 'NONE',  ( -16.55341960407611168, -4.379528057220339221, 51.45724293864770260 ) ) ;
#5681=CARTESIAN_POINT ( 'NONE',  ( -16.55341960407611168, -4.379528057220339221, 31.45724293864769550 ) ) ;
#5682=CARTESIAN_POINT ( 'NONE',  ( -9.474510206698964154, 16.51473224551069663, 60.41557627198102409 ) ) ;
#5683=CARTESIAN_POINT ( 'NONE',  ( -13.97604488694547520, 13.89961937509957934, 73.12609039468567573 ) ) ;
#5684=CARTESIAN_POINT ( 'NONE',  ( 0.05219959533936267826, -19.03943276465977164, 45.00109039468566863 ) ) ;
#5685=CARTESIAN_POINT ( 'NONE',  ( 8.224510206698742110, 14.34966873604972548, 52.08442372801901854 ) ) ;
#5686=CARTESIAN_POINT ( 'NONE',  ( 10.72451020669898902, -18.67979575497178502, 47.91557627198102409 ) ) ;
#5687=CARTESIAN_POINT ( 'NONE',  ( -21.52544592524334988, -5.823673210054445271, 108.9594237280190185 ) ) ;
#5688=CARTESIAN_POINT ( 'NONE',  ( -19.02544592524342804, 5.153800228976336051, 71.04057627198099567 ) ) ;
#5690=CARTESIAN_POINT ( 'NONE',  ( -16.46253265017160317, 9.564922557960807481, 105.8322429386476955 ) ) ;
#5692=CARTESIAN_POINT ( 'NONE',  ( 15.72974639402176855, 15.80617190586768217, 36.87609039468568994 ) ) ;
#5693=CARTESIAN_POINT ( 'NONE',  ( 4.379528057220339221, -16.55341960407611168, 87.70724293864769550 ) ) ;
#5694=CARTESIAN_POINT ( 'NONE',  ( -10.81492255796078084, -18.62759615963271287, 82.08224293864768129 ) ) ;
#5695=CARTESIAN_POINT ( 'NONE',  ( 9.474510206698971260, -16.51473224551069308, 87.91557627198102409 ) ) ;
#5696=CARTESIAN_POINT ( 'NONE',  ( 13.89961937509977652, -13.97604488694527269, 93.12390960531436690 ) ) ;
#5697=CARTESIAN_POINT ( 'NONE',  ( -18.62759615963255300, -10.81492255796106328, 29.16775706135234003 ) ) ;
#5699=CARTESIAN_POINT ( 'NONE',  ( 5.153800228976335163, 19.02544592524342804, 74.79057627198103830 ) ) ;
#5701=CARTESIAN_POINT ( 'NONE',  ( 19.02544592524343514, -5.153800228976328945, 23.54057627198102054 ) ) ;
#5702=CARTESIAN_POINT ( 'NONE',  ( -9.474510206698964154, 16.51473224551069663, 30.41557627198102054 ) ) ;
#5703=CARTESIAN_POINT ( 'NONE',  ( 19.02544592524334988, 5.153800228976608722, 111.4594237280190043 ) ) ;
#5705=CARTESIAN_POINT ( 'NONE',  ( 14.29746914071049879, -8.314922557960816363, 108.3322429386477097 ) ) ;
#5706=CARTESIAN_POINT ( 'NONE',  ( -5.823673210054431948, 21.52544592524334988, 77.70942372801900433 ) ) ;
#5707=CARTESIAN_POINT ( 'NONE',  ( 9.474510206698971260, -16.51473224551069308, 62.91557627198102409 ) ) ;
#5708=CARTESIAN_POINT ( 'NONE',  ( 10.81492255796106328, -18.62759615963255655, 30.41775706135234358 ) ) ;
#5709=CARTESIAN_POINT ( 'NONE',  ( 18.62759615963271287, -10.81492255796078972, 113.3322429386476955 ) ) ;
#5711=CARTESIAN_POINT ( 'NONE',  ( 5.049401038298161559, -19.05341960407611168, 87.70724293864769550 ) ) ;
#5713=CARTESIAN_POINT ( 'NONE',  ( -16.55341960407617563, 4.379528057220093196, 28.54275706135234358 ) ) ;
#5714=CARTESIAN_POINT ( 'NONE',  ( 21.52544592524344225, -5.823673210054117533, 38.54057627198103120 ) ) ;
#5715=CARTESIAN_POINT ( 'NONE',  ( 5.719274019375673035, 21.55341960407619339, 67.29275706135234714 ) ) ;
#5716=CARTESIAN_POINT ( 'NONE',  ( -9.474510206698964154, 16.51473224551069663, 110.4155762719810383 ) ) ;
#5717=CARTESIAN_POINT ( 'NONE',  ( 13.97604488694548053, -13.89961937509957401, 100.6260903946856615 ) ) ;
#5718=CARTESIAN_POINT ( 'NONE',  ( -0.05219959533909027116, -19.03943276465977164, 47.49890960531435979 ) ) ;
#5719=CARTESIAN_POINT ( 'NONE',  ( -0.05219959533909027116, -19.03943276465977164, 82.49890960531436690 ) ) ;
#5720=CARTESIAN_POINT ( 'NONE',  ( -8.314922557960811034, -14.29746914071050412, 92.08224293864769550 ) ) ;
#5721=CARTESIAN_POINT ( 'NONE',  ( 12.06949235617757843, -12.14591786802309237, 93.12390960531436690 ) ) ;
#5722=CARTESIAN_POINT ( 'NONE',  ( 19.02544592524343514, -5.153800228976328945, 108.5405762719810383 ) ) ;
#5723=CARTESIAN_POINT ( 'NONE',  ( 0.05219959533910956823, 16.53943276465976808, 54.99890960531435269 ) ) ;
#5724=CARTESIAN_POINT ( 'NONE',  ( -19.05341960407611168, -5.049401038298163336, 46.45724293864768129 ) ) ;
#5725=CARTESIAN_POINT ( 'NONE',  ( 15.80617190586769283, -15.72974639402175789, 60.62609039468567573 ) ) ;
#5726=CARTESIAN_POINT ( 'NONE',  ( -5.049401038297874678, -19.05341960407617918, 99.79275706135234714 ) ) ;
#5727=CARTESIAN_POINT ( 'NONE',  ( 16.55341960407611168, 4.379528057220329451, 58.95724293864770971 ) ) ;
#5728=CARTESIAN_POINT ( 'NONE',  ( -15.72974639402197994, 15.80617190586746368, 110.6239096053143669 ) ) ;
#5729=CARTESIAN_POINT ( 'NONE',  ( -18.67979575497178146, -10.72451020669898902, 46.66557627198102409 ) ) ;
#5730=CARTESIAN_POINT ( 'NONE',  ( -19.02544592524342804, 5.153800228976336051, 116.0405762719810383 ) ) ;
#5732=CARTESIAN_POINT ( 'NONE',  ( -16.46253265017160317, 9.564922557960807481, 55.83224293864769550 ) ) ;
#5733=CARTESIAN_POINT ( 'NONE',  ( -4.483927247898539470, -16.52544592524342804, 32.29057627198102409 ) ) ;
#5734=AXIS2_PLACEMENT_3D ( 'NONE', #61704, #10514, #133851 ) ;
#5736=CARTESIAN_POINT ( 'NONE',  ( 16.52544592524335698, 4.483927247898782831, 106.4594237280190328 ) ) ;
#5737=CARTESIAN_POINT ( 'NONE',  ( -4.379528057220086978, -16.55341960407618274, 89.79275706135236135 ) ) ;
#5738=CARTESIAN_POINT ( 'NONE',  ( -5.049401038297874678, -19.05341960407617918, 34.79275706135233293 ) ) ;
#5741=CARTESIAN_POINT ( 'NONE',  ( 19.05341960407611168, 5.049401038298154454, 88.95724293864769550 ) ) ;
#5742=CARTESIAN_POINT ( 'NONE',  ( -0.05219959533909027116, -19.03943276465977164, 52.49890960531436690 ) ) ;
#5743=CARTESIAN_POINT ( 'NONE',  ( -14.29746914071049879, 8.314922557960819915, 60.83224293864769550 ) ) ;
#5744=CARTESIAN_POINT ( 'NONE',  ( 16.52216118717207394, -7.221426719304488984, 101.4240097895301034 ) ) ;
#5745=CARTESIAN_POINT ( 'NONE',  ( -21.52544592524343514, 5.823673210054127303, 26.04057627198103475 ) ) ;
#5746=CARTESIAN_POINT ( 'NONE',  ( -15.80617190586745835, -15.72974639402198527, 46.87390960531435979 ) ) ;
#5747=CARTESIAN_POINT ( 'NONE',  ( -14.34966873604960291, -8.224510206698953496, 81.66557627198103830 ) ) ;
#5748=CARTESIAN_POINT ( 'NONE',  ( -0.05219959533934338120, 16.53943276465976808, 32.50109039468568284 ) ) ;
#5749=CARTESIAN_POINT ( 'NONE',  ( -16.55341960407611168, -4.379528057220339221, 76.45724293864769550 ) ) ;
#5751=CARTESIAN_POINT ( 'NONE',  ( -9.474510206698720793, -16.51473224551083518, 79.58442372801899012 ) ) ;
#5752=CARTESIAN_POINT ( 'NONE',  ( 5.049401038298161559, -19.05341960407611168, 107.7072429386476955 ) ) ;
#5754=CARTESIAN_POINT ( 'NONE',  ( -0.05219959533909027116, -19.03943276465977164, 42.49890960531435269 ) ) ;
#5755=CARTESIAN_POINT ( 'NONE',  ( -8.224510206698735004, -14.34966873604973081, 29.58442372801901854 ) ) ;
#5756=CARTESIAN_POINT ( 'NONE',  ( -16.53943276465976808, -0.05219959533934237506, 103.7510903946857042 ) ) ;
#5757=CARTESIAN_POINT ( 'NONE',  ( -19.05341960407617563, 5.049401038297882671, 68.54275706135230450 ) ) ;
#5758=CARTESIAN_POINT ( 'NONE',  ( 18.67979575497178502, 10.72451020669898547, 44.16557627198103120 ) ) ;
#5759=CARTESIAN_POINT ( 'NONE',  ( -15.72974639402176322, -15.80617190586768395, 69.37609039468567573 ) ) ;
#5761=CARTESIAN_POINT ( 'NONE',  ( 16.55341960407618274, -4.379528057220086978, 41.04275706135236135 ) ) ;
#5762=CARTESIAN_POINT ( 'NONE',  ( 0.05219959533909260263, 19.03943276465977164, 29.99890960531435979 ) ) ;
#5763=CARTESIAN_POINT ( 'NONE',  ( -16.51473224551069308, -9.474510206698971260, 81.66557627198103830 ) ) ;
#5765=CARTESIAN_POINT ( 'NONE',  ( -19.05341960407611168, -5.049401038298163336, 26.45724293864769550 ) ) ;
#5766=CARTESIAN_POINT ( 'NONE',  ( 4.483927247898545687, 16.52544592524342804, 84.79057627198102409 ) ) ;
#5768=CARTESIAN_POINT ( 'NONE',  ( 0.05219959533909260263, 19.03943276465977164, 84.99890960531436690 ) ) ;
#5770=CARTESIAN_POINT ( 'NONE',  ( 19.05341960407617918, -5.049401038297876454, 101.0427570613523045 ) ) ;
#5771=CARTESIAN_POINT ( 'NONE',  ( 21.53943276465977519, -0.05219959533907433946, 78.74890960531436690 ) ) ;
#5772=CARTESIAN_POINT ( 'NONE',  ( -19.02544592524342804, 5.153800228976336051, 46.04057627198101699 ) ) ;
#5773=CARTESIAN_POINT ( 'NONE',  ( -5.049401038297874678, -19.05341960407617918, 69.79275706135233293 ) ) ;
#5774=CARTESIAN_POINT ( 'NONE',  ( 5.719274019375991003, -21.55341960407610458, 112.7072429386476955 ) ) ;
#5775=CARTESIAN_POINT ( 'NONE',  ( 5.153800228976335163, 19.02544592524342804, 64.79057627198100988 ) ) ;
#5776=CARTESIAN_POINT ( 'NONE',  ( 5.153800228976335163, 19.02544592524342804, 109.7905762719810099 ) ) ;
#5779=CARTESIAN_POINT ( 'NONE',  ( -16.53943276465976808, -0.05219959533934237506, 33.75109039468568284 ) ) ;
#5780=CARTESIAN_POINT ( 'NONE',  ( -10.72451020669898014, 18.67979575497178502, 105.4155762719810383 ) ) ;
#5781=CARTESIAN_POINT ( 'NONE',  ( -0.05219959533910754901, -16.53943276465976808, 112.4989096053143669 ) ) ;
#5782=CARTESIAN_POINT ( 'NONE',  ( -19.02544592524342804, 5.153800228976336051, 91.04057627198100988 ) ) ;
#5783=CARTESIAN_POINT ( 'NONE',  ( 5.153800228976615827, -19.02544592524334988, 55.20942372801899722 ) ) ;
#5784=CARTESIAN_POINT ( 'NONE',  ( 10.72451020669898902, -18.67979575497178502, 82.91557627198103830 ) ) ;
#5785=CARTESIAN_POINT ( 'NONE',  ( -12.06949235617756955, 12.14591786802309770, 45.62390960531436690 ) ) ;
#5786=CARTESIAN_POINT ( 'NONE',  ( -13.89961937509957401, -13.97604488694547875, 24.37609039468565442 ) ) ;
#5787=CARTESIAN_POINT ( 'NONE',  ( -14.29746914071037622, -8.314922557961029526, 64.16775706135234714 ) ) ;
#5789=CARTESIAN_POINT ( 'NONE',  ( 19.05341960407611168, 5.049401038298154454, 98.95724293864766707 ) ) ;
#5790=CARTESIAN_POINT ( 'NONE',  ( 13.97604488694527802, 13.89961937509977652, 49.37390960531434558 ) ) ;
#5791=CARTESIAN_POINT ( 'NONE',  ( -15.72974639402176322, -15.80617190586768395, 49.37609039468569705 ) ) ;
#5792=CARTESIAN_POINT ( 'NONE',  ( -5.823673210054431948, 21.52544592524334988, 67.70942372801901854 ) ) ;
#5793=CARTESIAN_POINT ( 'NONE',  ( -19.05341960407611168, -5.049401038298163336, 66.45724293864769550 ) ) ;
#5794=CARTESIAN_POINT ( 'NONE',  ( 15.80617190586769283, -15.72974639402175789, 30.62609039468567929 ) ) ;
#5795=CARTESIAN_POINT ( 'NONE',  ( -16.51473224551082808, 9.474510206698731452, 73.33442372801900433 ) ) ;
#5796=CARTESIAN_POINT ( 'NONE',  ( -13.97604488694547697, 13.89961937509957934, 73.12609039468568994 ) ) ;
#5797=CARTESIAN_POINT ( 'NONE',  ( 19.05341960407611168, 5.049401038298154454, 33.95724293864769550 ) ) ;
#5798=CARTESIAN_POINT ( 'NONE',  ( -4.379528057220086978, -16.55341960407618274, 89.79275706135236135 ) ) ;
#5799=CARTESIAN_POINT ( 'NONE',  ( 19.02544592524343514, -5.153800228976328945, 48.54057627198103120 ) ) ;
#5800=CARTESIAN_POINT ( 'NONE',  ( 5.153800228976335163, 19.02544592524342804, 24.79057627198102765 ) ) ;
#5801=CARTESIAN_POINT ( 'NONE',  ( -5.153800228976328057, -19.02544592524343514, 102.2905762719810383 ) ) ;
#5802=CARTESIAN_POINT ( 'NONE',  ( -5.153800228976328057, -19.02544592524343514, 32.29057627198102409 ) ) ;
#5803=CARTESIAN_POINT ( 'NONE',  ( -5.719274019375978568, 21.55341960407610458, 90.20724293864770971 ) ) ;
#5804=CARTESIAN_POINT ( 'NONE',  ( 8.314922557961029526, -14.29746914071037800, 60.41775706135235424 ) ) ;
#5805=CARTESIAN_POINT ( 'NONE',  ( 19.02544592524334988, 5.153800228976608722, 36.45942372801900433 ) ) ;
#5806=CARTESIAN_POINT ( 'NONE',  ( -13.97604488694527625, -13.89961937509977652, 46.87390960531435979 ) ) ;
#5807=CARTESIAN_POINT ( 'NONE',  ( 8.314922557960818139, 14.29746914071049879, 39.58224293864769550 ) ) ;
#5808=CARTESIAN_POINT ( 'NONE',  ( -16.52544592524342804, 4.483927247898546575, 76.04057627198102409 ) ) ;
#5809=CARTESIAN_POINT ( 'NONE',  ( -19.05341960407611168, -5.049401038298163336, 81.45724293864769550 ) ) ;
#5810=CARTESIAN_POINT ( 'NONE',  ( -9.564922557960796823, -16.46253265017161027, 77.08224293864769550 ) ) ;
#5811=CARTESIAN_POINT ( 'NONE',  ( 10.72451020669871369, 18.67979575497193778, 32.08442372801901854 ) ) ;
#5812=CARTESIAN_POINT ( 'NONE',  ( -9.564922557960796823, -16.46253265017161027, 87.08224293864769550 ) ) ;
#5813=CARTESIAN_POINT ( 'NONE',  ( -21.52544592524334988, -5.823673210054445271, 103.9594237280190185 ) ) ;
#5814=CARTESIAN_POINT ( 'NONE',  ( 16.53943276465976808, 0.05219959533934440121, 76.25109039468568994 ) ) ;
#5815=CARTESIAN_POINT ( 'NONE',  ( 5.719274019375673035, 21.55341960407619339, 22.29275706135235069 ) ) ;
#5816=CARTESIAN_POINT ( 'NONE',  ( 10.72451020669898902, -18.67979575497178502, 87.91557627198103830 ) ) ;
#5817=CARTESIAN_POINT ( 'NONE',  ( 8.224510206698953496, -14.34966873604960469, 47.91557627198102409 ) ) ;
#5818=CARTESIAN_POINT ( 'NONE',  ( -19.05341960407611168, -5.049401038298163336, 41.45724293864769550 ) ) ;
#5819=CARTESIAN_POINT ( 'NONE',  ( 12.06949235617757843, -12.14591786802309237, 73.12390960531436690 ) ) ;
#5820=CARTESIAN_POINT ( 'NONE',  ( 21.52544592524344225, -5.823673210054117533, 33.54057627198102409 ) ) ;
#5821=CARTESIAN_POINT ( 'NONE',  ( -5.049401038297874678, -19.05341960407617918, 29.79275706135232227 ) ) ;
#5822=CARTESIAN_POINT ( 'NONE',  ( -16.53943276465976808, 0.05219959533911058130, 106.2489096053143811 ) ) ;
#5823=CARTESIAN_POINT ( 'NONE',  ( -13.97604488694527625, -13.89961937509977652, 106.8739096053143669 ) ) ;
#5824=EDGE_LOOP ( 'NONE', ( #66134, #59358 ) ) ;
#5825=CARTESIAN_POINT ( 'NONE',  ( 16.55341960407618274, -4.379528057220086978, 51.04275706135234714 ) ) ;
#5826=CARTESIAN_POINT ( 'NONE',  ( 13.89961937509977652, -13.97604488694527269, 63.12390960531435979 ) ) ;
#5828=CARTESIAN_POINT ( 'NONE',  ( 15.72974639402199770, -15.80617190586745480, 23.12390960531436335 ) ) ;
#5829=CARTESIAN_POINT ( 'NONE',  ( -12.06949235617739369, -12.14591786802326823, 89.37609039468568994 ) ) ;
#5830=CARTESIAN_POINT ( 'NONE',  ( -8.224510206698735004, -14.34966873604973081, 19.58442372801901143 ) ) ;
#5831=CARTESIAN_POINT ( 'NONE',  ( 21.55341960407619695, -5.719274019375665929, 86.04275706135236135 ) ) ;
#5832=CARTESIAN_POINT ( 'NONE',  ( -9.474510206698964154, 16.51473224551069663, 75.41557627198103830 ) ) ;
#5833=CARTESIAN_POINT ( 'NONE',  ( 15.72974639402199770, -15.80617190586745480, 103.1239096053143811 ) ) ;
#5834=CARTESIAN_POINT ( 'NONE',  ( 16.53943276465976808, 0.05219959533934440121, 61.25109039468567573 ) ) ;
#5835=CARTESIAN_POINT ( 'NONE',  ( 12.14591786802309770, 12.06949235617756955, 114.3739096053143527 ) ) ;
#5836=CARTESIAN_POINT ( 'NONE',  ( 14.29746914071037800, 8.314922557961029526, 21.66775706135235069 ) ) ;
#5837=CARTESIAN_POINT ( 'NONE',  ( 9.564922557961047289, -16.46253265017146816, 85.41775706135233293 ) ) ;
#5838=CARTESIAN_POINT ( 'NONE',  ( -10.72451020669898014, 18.67979575497178502, 80.41557627198103830 ) ) ;
#5839=CARTESIAN_POINT ( 'NONE',  ( 19.05341960407617918, -5.049401038297876454, 56.04275706135234714 ) ) ;
#5841=CARTESIAN_POINT ( 'NONE',  ( -15.80617190586745835, -15.72974639402198527, 101.8739096053143811 ) ) ;
#5843=CARTESIAN_POINT ( 'NONE',  ( 19.02544592524343514, -5.153800228976328945, 78.54057627198099567 ) ) ;
#5845=CARTESIAN_POINT ( 'NONE',  ( 16.53943276465976808, 0.05219959533934440121, 21.25109039468567218 ) ) ;
#5847=CARTESIAN_POINT ( 'NONE',  ( -10.81492255796078084, -18.62759615963271287, 97.08224293864770971 ) ) ;
#5848=CARTESIAN_POINT ( 'NONE',  ( -4.379528057220328563, 16.55341960407611168, 70.20724293864769550 ) ) ;
#5849=CARTESIAN_POINT ( 'NONE',  ( 19.05341960407611168, 5.049401038298154454, 63.95724293864769550 ) ) ;
#5850=CARTESIAN_POINT ( 'NONE',  ( 0.05219959533937995610, -21.53943276465977519, 75.00109039468568994 ) ) ;
#5851=CARTESIAN_POINT ( 'NONE',  ( -0.05219959533934338120, 16.53943276465976808, 37.50109039468568284 ) ) ;
#5852=CARTESIAN_POINT ( 'NONE',  ( -0.05219959533936034679, 19.03943276465977164, 37.50109039468567573 ) ) ;
#5853=CARTESIAN_POINT ( 'NONE',  ( 21.53943276465977519, 0.05219959533937863772, 56.25109039468568284 ) ) ;
#5854=CARTESIAN_POINT ( 'NONE',  ( -5.719274019375978568, 21.55341960407610458, 65.20724293864768129 ) ) ;
#5855=CARTESIAN_POINT ( 'NONE',  ( 19.03943276465977164, 0.05219959533936151252, 106.2510903946856615 ) ) ;
#5856=CARTESIAN_POINT ( 'NONE',  ( -19.02544592524342804, 5.153800228976336051, 51.04057627198103120 ) ) ;
#5857=CARTESIAN_POINT ( 'NONE',  ( -9.474510206698720793, -16.51473224551083518, 74.58442372801900433 ) ) ;
#5858=CARTESIAN_POINT ( 'NONE',  ( -15.80617190586768217, 15.72974639402176855, 78.12609039468570415 ) ) ;
#5859=CARTESIAN_POINT ( 'NONE',  ( -13.97604488694547697, 13.89961937509957934, 48.12609039468566863 ) ) ;
#5860=CARTESIAN_POINT ( 'NONE',  ( -19.05341960407611168, -5.049401038298163336, 41.45724293864769550 ) ) ;
#5861=CARTESIAN_POINT ( 'NONE',  ( 21.55341960407610458, 5.719274019375980345, 63.95724293864770260 ) ) ;
#5862=CARTESIAN_POINT ( 'NONE',  ( -16.55341960407611168, -4.379528057220339221, 46.45724293864769550 ) ) ;
#5864=CARTESIAN_POINT ( 'NONE',  ( 9.564922557961047289, -16.46253265017146816, 25.41775706135234003 ) ) ;
#5865=CARTESIAN_POINT ( 'NONE',  ( 14.29746914071037800, 8.314922557961029526, 91.66775706135234714 ) ) ;
#5866=CARTESIAN_POINT ( 'NONE',  ( -0.05219959533910754901, -16.53943276465976808, 57.49890960531435979 ) ) ;
#5867=CARTESIAN_POINT ( 'NONE',  ( -18.67979575497193778, 10.72451020669871902, 83.33442372801903275 ) ) ;
#5868=CARTESIAN_POINT ( 'NONE',  ( -15.72974639402176322, -15.80617190586768395, 79.37609039468567573 ) ) ;
#5869=CARTESIAN_POINT ( 'NONE',  ( -21.52544592524343514, 5.823673210054127303, 76.04057627198102409 ) ) ;
#5870=CARTESIAN_POINT ( 'NONE',  ( 16.51473224551069308, 9.474510206698969483, 54.16557627198103120 ) ) ;
#5871=CARTESIAN_POINT ( 'NONE',  ( 21.55341960407619695, -5.719274019375665929, 56.04275706135235424 ) ) ;
#5872=CARTESIAN_POINT ( 'NONE',  ( 5.153800228976335163, 19.02544592524342804, 34.79057627198102409 ) ) ;
#5873=CARTESIAN_POINT ( 'NONE',  ( -9.474510206698964154, 16.51473224551069663, 50.41557627198102409 ) ) ;
#5874=CARTESIAN_POINT ( 'NONE',  ( 0.05219959533910956823, 16.53943276465976808, 109.9989096053143527 ) ) ;
#5875=CARTESIAN_POINT ( 'NONE',  ( -5.153800228976328057, -19.02544592524343514, 97.29057627198099567 ) ) ;
#5876=CARTESIAN_POINT ( 'NONE',  ( -4.483927247898539470, -16.52544592524342804, 47.29057627198103120 ) ) ;
#5877=CARTESIAN_POINT ( 'NONE',  ( 14.29746914071049879, -8.314922557960816363, 108.3322429386477097 ) ) ;
#5878=CARTESIAN_POINT ( 'NONE',  ( -0.05219959533907301413, -21.53943276465977519, 82.49890960531436690 ) ) ;
#5879=CARTESIAN_POINT ( 'NONE',  ( 15.80617190586769283, -15.72974639402175789, 20.62609039468568639 ) ) ;
#5881=CARTESIAN_POINT ( 'NONE',  ( 8.224510206698742110, 14.34966873604972548, 42.08442372801901854 ) ) ;
#5882=EDGE_LOOP ( 'NONE', ( #15030, #54670, #59880, #149688, #178120, #2796, #66506, #131779 ) ) ;
#5883=CARTESIAN_POINT ( 'NONE',  ( 10.72451020669898902, -18.67979575497178502, 67.91557627198102409 ) ) ;
#5885=CARTESIAN_POINT ( 'NONE',  ( 15.72974639402176855, 15.80617190586768217, 106.8760903946856899 ) ) ;
#5886=CARTESIAN_POINT ( 'NONE',  ( -19.02544592524342804, 5.153800228976336051, 96.04057627198103830 ) ) ;
#5887=CARTESIAN_POINT ( 'NONE',  ( 5.719274019375673035, 21.55341960407619339, 27.29275706135234358 ) ) ;
#5888=CARTESIAN_POINT ( 'NONE',  ( 5.823673210054125526, 21.52544592524343514, 29.79057627198102409 ) ) ;
#5889=CARTESIAN_POINT ( 'NONE',  ( 8.314922557961029526, -14.29746914071037800, 105.4177570613523613 ) ) ;
#5890=CARTESIAN_POINT ( 'NONE',  ( -18.67979575497193778, 10.72451020669871902, 53.33442372801901854 ) ) ;
#5891=CARTESIAN_POINT ( 'NONE',  ( -18.67979575497193778, 10.72451020669871902, 78.33442372801901854 ) ) ;
#5892=CARTESIAN_POINT ( 'NONE',  ( 10.81492255796106328, -18.62759615963255655, 110.4177570613523756 ) ) ;
#5893=CARTESIAN_POINT ( 'NONE',  ( 12.14591786802327356, -12.06949235617739191, 70.62609039468567573 ) ) ;
#5894=CARTESIAN_POINT ( 'NONE',  ( 21.53943276465977519, 0.05219959533937863772, 36.25109039468567573 ) ) ;
#5895=CARTESIAN_POINT ( 'NONE',  ( 9.474510206698971260, -16.51473224551069308, 27.91557627198103120 ) ) ;
#5896=CARTESIAN_POINT ( 'NONE',  ( -5.823673210054431948, 21.52544592524334988, 107.7094237280190328 ) ) ;
#5897=CARTESIAN_POINT ( 'NONE',  ( -19.02544592524342804, 5.153800228976336051, 106.0405762719810241 ) ) ;
#5898=CARTESIAN_POINT ( 'NONE',  ( 18.62759615963271287, -10.81492255796078972, 108.3322429386477097 ) ) ;
#5900=CARTESIAN_POINT ( 'NONE',  ( -21.52544592524343514, 5.823673210054127303, 71.04057627198103830 ) ) ;
#5901=CARTESIAN_POINT ( 'NONE',  ( -16.53943276465976808, -0.05219959533934237506, 53.75109039468568994 ) ) ;
#5902=CARTESIAN_POINT ( 'NONE',  ( 16.53943276465976808, -0.05219959533910856209, 43.74890960531435979 ) ) ;
#5904=CARTESIAN_POINT ( 'NONE',  ( 9.564922557961047289, -16.46253265017146816, 85.41775706135233293 ) ) ;
#5906=CARTESIAN_POINT ( 'NONE',  ( -16.53943276465976808, -0.05219959533934237506, 23.75109039468567929 ) ) ;
#5907=CARTESIAN_POINT ( 'NONE',  ( 21.52544592524344225, -5.823673210054117533, 93.54057627198103830 ) ) ;
#5908=CARTESIAN_POINT ( 'NONE',  ( 15.80617190586746368, 15.72974639402197994, 69.37390960531436690 ) ) ;
#5909=CARTESIAN_POINT ( 'NONE',  ( 9.474510206698971260, -16.51473224551069308, 107.9155762719810383 ) ) ;
#5910=CARTESIAN_POINT ( 'NONE',  ( -8.314922557961024197, 14.29746914071037800, 47.91775706135234714 ) ) ;
#5911=CARTESIAN_POINT ( 'NONE',  ( -9.474510206698964154, 16.51473224551069663, 55.41557627198103120 ) ) ;
#5912=CARTESIAN_POINT ( 'NONE',  ( 18.67979575497194134, -10.72451020669871369, 35.83442372801901143 ) ) ;
#5913=CARTESIAN_POINT ( 'NONE',  ( -0.05219959533936034679, 19.03943276465977164, 92.50109039468566152 ) ) ;
#5914=CARTESIAN_POINT ( 'NONE',  ( 16.46253265017160672, -9.564922557960803928, 103.3322429386476955 ) ) ;
#5915=CARTESIAN_POINT ( 'NONE',  ( 16.51473224551069308, 9.474510206698969483, 94.16557627198103830 ) ) ;
#5916=CARTESIAN_POINT ( 'NONE',  ( -21.52544592524343514, 5.823673210054127303, 91.04057627198103830 ) ) ;
#5917=CARTESIAN_POINT ( 'NONE',  ( -5.153800228976328057, -19.02544592524343514, 62.29057627198100988 ) ) ;
#5919=CARTESIAN_POINT ( 'NONE',  ( 8.314922557960818139, 14.29746914071049879, 69.58224293864769550 ) ) ;
#5920=CARTESIAN_POINT ( 'NONE',  ( 19.02544592524343514, -5.153800228976328945, 98.54057627198100988 ) ) ;
#5922=CARTESIAN_POINT ( 'NONE',  ( -5.049401038297874678, -19.05341960407617918, 79.79275706135233293 ) ) ;
#5923=CARTESIAN_POINT ( 'NONE',  ( -18.67979575497178146, -10.72451020669898902, 86.66557627198102409 ) ) ;
#5924=CARTESIAN_POINT ( 'NONE',  ( 19.03943276465977164, 0.05219959533936151252, 46.25109039468566863 ) ) ;
#5925=CARTESIAN_POINT ( 'NONE',  ( 15.80617190586746368, 15.72974639402197994, 24.37390960531435979 ) ) ;
#5926=SURFACE_STYLE_USAGE ( .BOTH. , #173815 ) ;
#5927=CARTESIAN_POINT ( 'NONE',  ( 21.55341960407610458, 5.719274019375980345, 58.95724293864770971 ) ) ;
#5928=CARTESIAN_POINT ( 'NONE',  ( 13.89961937509977652, -13.97604488694527269, 88.12390960531438111 ) ) ;
#5929=CARTESIAN_POINT ( 'NONE',  ( 21.53943276465977519, 0.05219959533937863772, 76.25109039468568994 ) ) ;
#5930=CARTESIAN_POINT ( 'NONE',  ( 5.049401038298161559, -19.05341960407611168, 37.70724293864768839 ) ) ;
#5931=CARTESIAN_POINT ( 'NONE',  ( -8.314922557960811034, -14.29746914071050412, 72.08224293864769550 ) ) ;
#5932=CARTESIAN_POINT ( 'NONE',  ( 4.379528057220092307, 16.55341960407617563, 27.29275706135234358 ) ) ;
#5933=CARTESIAN_POINT ( 'NONE',  ( 15.80617190586769283, -15.72974639402175789, 60.62609039468567573 ) ) ;
#5935=CARTESIAN_POINT ( 'NONE',  ( -13.97604488694547697, 13.89961937509957934, 28.12609039468565797 ) ) ;
#5936=CARTESIAN_POINT ( 'NONE',  ( 19.05341960407617918, -5.049401038297876454, 81.04275706135231871 ) ) ;
#5937=CARTESIAN_POINT ( 'NONE',  ( -17.60779699588841751, -5.499999999999947597, 91.34981316670105400 ) ) ;
#5938=CARTESIAN_POINT ( 'NONE',  ( -21.52544592524334988, -5.823673210054445271, 23.95942372801901143 ) ) ;
#5940=CARTESIAN_POINT ( 'NONE',  ( 10.81492255796106328, -18.62759615963255655, 110.4177570613523756 ) ) ;
#5941=CARTESIAN_POINT ( 'NONE',  ( -5.153800228976328057, -19.02544592524343514, 57.29057627198103120 ) ) ;
#5942=CARTESIAN_POINT ( 'NONE',  ( 19.03943276465977164, 0.05219959533936151252, 21.25109039468565797 ) ) ;
#5943=CARTESIAN_POINT ( 'NONE',  ( -8.224510206698735004, -14.34966873604973081, 104.5844237280190185 ) ) ;
#5944=CARTESIAN_POINT ( 'NONE',  ( -9.474510206698964154, 16.51473224551069663, 105.4155762719810383 ) ) ;
#5945=CARTESIAN_POINT ( 'NONE',  ( -21.55341960407619339, 5.719274019375674811, 78.54275706135236135 ) ) ;
#5948=CARTESIAN_POINT ( 'NONE',  ( 18.67979575497194134, -10.72451020669871369, 90.83442372801901854 ) ) ;
#5949=CARTESIAN_POINT ( 'NONE',  ( 21.52544592524334988, 5.823673210054432836, 101.4594237280190185 ) ) ;
#5951=CARTESIAN_POINT ( 'NONE',  ( 9.474510206698971260, -16.51473224551069308, 102.9155762719810241 ) ) ;
#5952=CARTESIAN_POINT ( 'NONE',  ( 9.564922557961047289, -16.46253265017146816, 20.41775706135233293 ) ) ;
#5954=CARTESIAN_POINT ( 'NONE',  ( -19.05341960407611168, -5.049401038298163336, 36.45724293864766707 ) ) ;
#5955=CARTESIAN_POINT ( 'NONE',  ( 10.72451020669898902, -18.67979575497178502, 57.91557627198103120 ) ) ;
#5956=CARTESIAN_POINT ( 'NONE',  ( 12.14591786802327356, -12.06949235617739191, 105.6260903946856899 ) ) ;
#5957=CARTESIAN_POINT ( 'NONE',  ( -14.29746914071049879, 8.314922557960819915, 100.8322429386477097 ) ) ;
#5958=CARTESIAN_POINT ( 'NONE',  ( 5.049401038298161559, -19.05341960407611168, 87.70724293864769550 ) ) ;
#5959=CARTESIAN_POINT ( 'NONE',  ( -21.53943276465977519, -0.05219959533937600094, 103.7510903946857042 ) ) ;
#5960=CARTESIAN_POINT ( 'NONE',  ( -5.049401038298153566, 19.05341960407611168, 35.20724293864768839 ) ) ;
#5961=CARTESIAN_POINT ( 'NONE',  ( 4.379528057220339221, -16.55341960407611168, 97.70724293864772392 ) ) ;
#5962=CARTESIAN_POINT ( 'NONE',  ( 15.80617190586769283, -15.72974639402175789, 60.62609039468567573 ) ) ;
#5963=CARTESIAN_POINT ( 'NONE',  ( 18.62759615963271287, -10.81492255796078972, 93.33224293864769550 ) ) ;
#5964=CARTESIAN_POINT ( 'NONE',  ( -9.474510206698720793, -16.51473224551083518, 54.58442372801899722 ) ) ;
#5965=CARTESIAN_POINT ( 'NONE',  ( 17.58332526062526568, -7.635886036038552760, 48.42334959558466778 ) ) ;
#5966=CARTESIAN_POINT ( 'NONE',  ( -16.51473224551069308, -9.474510206698971260, 96.66557627198102409 ) ) ;
#5967=CARTESIAN_POINT ( 'NONE',  ( -16.55341960407611168, -4.379528057220339221, 71.45724293864769550 ) ) ;
#5968=CARTESIAN_POINT ( 'NONE',  ( -16.51473224551082808, 9.474510206698731452, 38.33442372801899722 ) ) ;
#5969=CARTESIAN_POINT ( 'NONE',  ( -13.89961937509977652, 13.97604488694528158, 60.62390960531436690 ) ) ;
#5970=CARTESIAN_POINT ( 'NONE',  ( -8.314922557960811034, -14.29746914071050412, 47.08224293864770260 ) ) ;
#5971=CARTESIAN_POINT ( 'NONE',  ( -19.03943276465977164, -0.05219959533935918106, 73.75109039468566152 ) ) ;
#5972=CARTESIAN_POINT ( 'NONE',  ( 17.50000000000000000, -5.499999999999992895, 101.2176903769643559 ) ) ;
#5973=CARTESIAN_POINT ( 'NONE',  ( -5.823673210054116645, -21.52544592524344225, 37.29057627198102409 ) ) ;
#5974=CARTESIAN_POINT ( 'NONE',  ( -16.52544592524342804, 4.483927247898546575, 101.0405762719810383 ) ) ;
#5976=CARTESIAN_POINT ( 'NONE',  ( 5.049401038298161559, -19.05341960407611168, 57.70724293864769550 ) ) ;
#5977=CARTESIAN_POINT ( 'NONE',  ( 21.55341960407610458, 5.719274019375980345, 58.95724293864770971 ) ) ;
#5978=CARTESIAN_POINT ( 'NONE',  ( -19.02544592524342804, 5.153800228976336051, 31.04057627198102409 ) ) ;
#5979=CARTESIAN_POINT ( 'NONE',  ( -0.05219959533934338120, 16.53943276465976808, 72.50109039468568994 ) ) ;
#5980=CARTESIAN_POINT ( 'NONE',  ( -19.03943276465977164, 0.05219959533909376836, 61.24890960531436690 ) ) ;
#5981=CARTESIAN_POINT ( 'NONE',  ( 0.05219959533936267826, -19.03943276465977164, 55.00109039468566863 ) ) ;
#5982=CARTESIAN_POINT ( 'NONE',  ( -18.62759615963255300, -10.81492255796106328, 74.16775706135231871 ) ) ;
#5984=CARTESIAN_POINT ( 'NONE',  ( 5.719274019375991003, -21.55341960407610458, 47.70724293864770260 ) ) ;
#5985=CARTESIAN_POINT ( 'NONE',  ( 13.97604488694527802, 13.89961937509977652, 29.37390960531435979 ) ) ;
#5986=CARTESIAN_POINT ( 'NONE',  ( 4.379528057220092307, 16.55341960407617563, 82.29275706135234714 ) ) ;
#5987=CARTESIAN_POINT ( 'NONE',  ( 13.89961937509957401, 13.97604488694547697, 101.8760903946856331 ) ) ;
#5988=CARTESIAN_POINT ( 'NONE',  ( 5.049401038298161559, -19.05341960407611168, 27.70724293864769550 ) ) ;
#5990=CARTESIAN_POINT ( 'NONE',  ( -15.80617190586745835, -15.72974639402198527, 56.87390960531436690 ) ) ;
#5991=CARTESIAN_POINT ( 'NONE',  ( 15.72974639402176855, 15.80617190586768217, 96.87609039468568994 ) ) ;
#5993=CARTESIAN_POINT ( 'NONE',  ( 8.224510206698953496, -14.34966873604960469, 47.91557627198102409 ) ) ;
#5994=CARTESIAN_POINT ( 'NONE',  ( -16.55341960407611168, -4.379528057220339221, 51.45724293864770260 ) ) ;
#5995=CARTESIAN_POINT ( 'NONE',  ( -15.72974639402197994, 15.80617190586746368, 85.62390960531436690 ) ) ;
#5996=CARTESIAN_POINT ( 'NONE',  ( 15.72974639402199770, -15.80617190586745480, 93.12390960531436690 ) ) ;
#5998=CARTESIAN_POINT ( 'NONE',  ( 21.52544592524344225, -5.823673210054117533, 28.54057627198103120 ) ) ;
#5999=CARTESIAN_POINT ( 'NONE',  ( 8.224510206698742110, 14.34966873604972548, 67.08442372801901854 ) ) ;
#6000=CARTESIAN_POINT ( 'NONE',  ( 8.224510206698953496, -14.34966873604960469, 77.91557627198102409 ) ) ;
#6001=CARTESIAN_POINT ( 'NONE',  ( -5.153800228976328057, -19.02544592524343514, 32.29057627198102409 ) ) ;
#6004=CARTESIAN_POINT ( 'NONE',  ( 8.314922557961029526, -14.29746914071037800, 90.41775706135236135 ) ) ;
#6005=CARTESIAN_POINT ( 'NONE',  ( -21.53943276465977519, 0.05219959533907696930, 116.2489096053143669 ) ) ;
#6006=CARTESIAN_POINT ( 'NONE',  ( 5.049401038298161559, -19.05341960407611168, 77.70724293864765286 ) ) ;
#6007=CARTESIAN_POINT ( 'NONE',  ( -21.52544592524334988, -5.823673210054445271, 53.95942372801900433 ) ) ;
#6008=CARTESIAN_POINT ( 'NONE',  ( 5.049401038298161559, -19.05341960407611168, 107.7072429386476955 ) ) ;
#6012=CARTESIAN_POINT ( 'NONE',  ( 21.53943276465977519, 0.05219959533937863772, 41.25109039468568284 ) ) ;
#6013=CARTESIAN_POINT ( 'NONE',  ( 16.51473224551069308, 9.474510206698969483, 39.16557627198103120 ) ) ;
#6014=CARTESIAN_POINT ( 'NONE',  ( 9.474510206698971260, -16.51473224551069308, 97.91557627198102409 ) ) ;
#6015=CARTESIAN_POINT ( 'NONE',  ( 19.03943276465977164, 0.05219959533936151252, 56.25109039468566863 ) ) ;
#6016=CARTESIAN_POINT ( 'NONE',  ( -18.62759615963255300, -10.81492255796106328, 29.16775706135234003 ) ) ;
#6017=CARTESIAN_POINT ( 'NONE',  ( 9.564922557961047289, -16.46253265017146816, 45.41775706135232582 ) ) ;
#6018=CARTESIAN_POINT ( 'NONE',  ( 13.97604488694527802, 13.89961937509977652, 29.37390960531435979 ) ) ;
#6019=CARTESIAN_POINT ( 'NONE',  ( 16.52544592524335698, 4.483927247898782831, 96.45942372801901854 ) ) ;
#6020=CARTESIAN_POINT ( 'NONE',  ( 5.049401038297881783, 19.05341960407617563, 57.29275706135231871 ) ) ;
#6021=CARTESIAN_POINT ( 'NONE',  ( -16.53943276465976808, -0.05219959533934237506, 108.7510903946857042 ) ) ;
#6022=CARTESIAN_POINT ( 'NONE',  ( 17.72560187377285601, 5.500000000000046185, 86.57814504131317790 ) ) ;
#6023=CARTESIAN_POINT ( 'NONE',  ( 13.89961937509977652, -13.97604488694527269, 88.12390960531438111 ) ) ;
#6024=CARTESIAN_POINT ( 'NONE',  ( -5.719274019375665041, -21.55341960407619695, 94.79275706135234714 ) ) ;
#6025=CARTESIAN_POINT ( 'NONE',  ( 10.72451020669871369, 18.67979575497193778, 107.0844237280190043 ) ) ;
#6027=CARTESIAN_POINT ( 'NONE',  ( -9.564922557960796823, -16.46253265017161027, 107.0822429386476955 ) ) ;
#6028=CARTESIAN_POINT ( 'NONE',  ( -21.55341960407619339, 5.719274019375674811, 73.54275706135234714 ) ) ;
#6029=CARTESIAN_POINT ( 'NONE',  ( -5.153800228976607833, 19.02544592524334988, 112.7094237280190043 ) ) ;
#6030=CARTESIAN_POINT ( 'NONE',  ( 5.049401038298161559, -19.05341960407611168, 82.70724293864770971 ) ) ;
#6031=CARTESIAN_POINT ( 'NONE',  ( 21.52544592524344225, -5.823673210054117533, 33.54057627198102409 ) ) ;
#6032=CARTESIAN_POINT ( 'NONE',  ( -0.05219959533909027116, -19.03943276465977164, 92.49890960531436690 ) ) ;
#6034=CARTESIAN_POINT ( 'NONE',  ( 5.049401038298161559, -19.05341960407611168, 77.70724293864765286 ) ) ;
#6035=CARTESIAN_POINT ( 'NONE',  ( -9.564922557960796823, -16.46253265017161027, 62.08224293864769550 ) ) ;
#6036=CARTESIAN_POINT ( 'NONE',  ( 14.29746914071037800, 8.314922557961029526, 111.6677570613523613 ) ) ;
#6037=CARTESIAN_POINT ( 'NONE',  ( -16.20579543436698700, 7.371946100355027731, 99.43479165828048849 ) ) ;
#6038=CARTESIAN_POINT ( 'NONE',  ( -5.153800228976607833, 19.02544592524334988, 67.70942372801900433 ) ) ;
#6039=CARTESIAN_POINT ( 'NONE',  ( 9.564922557960805705, 16.46253265017160317, 99.58224293864770971 ) ) ;
#6040=CARTESIAN_POINT ( 'NONE',  ( 8.314922557960818139, 14.29746914071049879, 89.58224293864768129 ) ) ;
#6042=CARTESIAN_POINT ( 'NONE',  ( 10.72451020669898902, -18.67979575497178502, 47.91557627198102409 ) ) ;
#6043=CARTESIAN_POINT ( 'NONE',  ( 18.67979575497178502, 10.72451020669898547, 29.16557627198103120 ) ) ;
#6044=CARTESIAN_POINT ( 'NONE',  ( -12.14591786802309592, -12.06949235617757132, 106.8739096053143811 ) ) ;
#6045=CARTESIAN_POINT ( 'NONE',  ( -17.44270441346513678, 5.991230190323085125, 53.63664920735775610 ) ) ;
#6046=CARTESIAN_POINT ( 'NONE',  ( 5.049401038297881783, 19.05341960407617563, 42.29275706135234003 ) ) ;
#6047=CARTESIAN_POINT ( 'NONE',  ( -4.379528057220328563, 16.55341960407611168, 30.20724293864769550 ) ) ;
#6048=CARTESIAN_POINT ( 'NONE',  ( -13.97604488694527625, -13.89961937509977652, 106.8739096053143669 ) ) ;
#6049=CARTESIAN_POINT ( 'NONE',  ( 15.72974639402176855, 15.80617190586768217, 71.87609039468568994 ) ) ;
#6050=CARTESIAN_POINT ( 'NONE',  ( -18.67979575497178146, -10.72451020669898902, 61.66557627198103120 ) ) ;
#6051=CARTESIAN_POINT ( 'NONE',  ( 18.67979575497194134, -10.72451020669871369, 50.83442372801901143 ) ) ;
#6052=CARTESIAN_POINT ( 'NONE',  ( -5.823673210054116645, -21.52544592524344225, 82.29057627198103830 ) ) ;
#6053=CARTESIAN_POINT ( 'NONE',  ( 18.62759615963255655, 10.81492255796105972, 41.66775706135235424 ) ) ;
#6054=CARTESIAN_POINT ( 'NONE',  ( 12.06949235617757843, -12.14591786802309237, 113.1239096053143953 ) ) ;
#6055=CARTESIAN_POINT ( 'NONE',  ( -5.049401038297874678, -19.05341960407617918, 74.79275706135231871 ) ) ;
#6056=CARTESIAN_POINT ( 'NONE',  ( 16.51473224551069308, 9.474510206698969483, 39.16557627198103120 ) ) ;
#6057=CARTESIAN_POINT ( 'NONE',  ( -16.53943276465976808, 0.05219959533911058130, 86.24890960531436690 ) ) ;
#6058=CARTESIAN_POINT ( 'NONE',  ( 16.51473224551069308, 9.474510206698969483, 104.1655762719810241 ) ) ;
#6059=CARTESIAN_POINT ( 'NONE',  ( -19.05341960407611168, -5.049401038298163336, 26.45724293864769550 ) ) ;
#6060=CARTESIAN_POINT ( 'NONE',  ( 16.52544592524342804, -4.483927247898539470, 43.54057627198103830 ) ) ;
#6061=CARTESIAN_POINT ( 'NONE',  ( 12.14591786802327356, -12.06949235617739191, 95.62609039468568994 ) ) ;
#6062=CARTESIAN_POINT ( 'NONE',  ( 5.049401038298161559, -19.05341960407611168, 57.70724293864769550 ) ) ;
#6063=CARTESIAN_POINT ( 'NONE',  ( -13.89961937509977652, 13.97604488694528158, 25.62390960531434558 ) ) ;
#6064=CARTESIAN_POINT ( 'NONE',  ( -13.97604488694547697, 13.89961937509957934, 28.12609039468565797 ) ) ;
#6065=CARTESIAN_POINT ( 'NONE',  ( 0.05219959533909260263, 19.03943276465977164, 109.9989096053143669 ) ) ;
#6066=CARTESIAN_POINT ( 'NONE',  ( -14.29746914071049879, 8.314922557960819915, 35.83224293864768839 ) ) ;
#6067=CARTESIAN_POINT ( 'NONE',  ( 21.55341960407619695, -5.719274019375665929, 46.04275706135234714 ) ) ;
#6069=CARTESIAN_POINT ( 'NONE',  ( 14.29746914071037800, 8.314922557961029526, 61.66775706135235424 ) ) ;
#6070=CARTESIAN_POINT ( 'NONE',  ( 4.379528057220339221, -16.55341960407611168, 22.70724293864769194 ) ) ;
#6071=CARTESIAN_POINT ( 'NONE',  ( -4.379528057220086978, -16.55341960407618274, 109.7927570613523613 ) ) ;
#6072=CARTESIAN_POINT ( 'NONE',  ( -16.53943276465976808, -0.05219959533934237506, 23.75109039468567929 ) ) ;
#6073=CARTESIAN_POINT ( 'NONE',  ( -5.049401038298153566, 19.05341960407611168, 50.20724293864770260 ) ) ;
#6074=CARTESIAN_POINT ( 'NONE',  ( 16.53943276465976808, -0.05219959533910856209, 108.7489096053143669 ) ) ;
#6075=CARTESIAN_POINT ( 'NONE',  ( 5.823673210054125526, 21.52544592524343514, 114.7905762719810383 ) ) ;
#6076=CARTESIAN_POINT ( 'NONE',  ( -5.049401038298153566, 19.05341960407611168, 50.20724293864770260 ) ) ;
#6078=CARTESIAN_POINT ( 'NONE',  ( 9.474510206698971260, -16.51473224551069308, 27.91557627198103120 ) ) ;
#6079=CARTESIAN_POINT ( 'NONE',  ( -18.67979575497178146, -10.72451020669898902, 21.66557627198102409 ) ) ;
#6080=CARTESIAN_POINT ( 'NONE',  ( -17.44270441346516876, -5.991230190323022065, 36.36335079264227232 ) ) ;
#6081=CARTESIAN_POINT ( 'NONE',  ( 16.46253265017160672, -9.564922557960803928, 98.33224293864769550 ) ) ;
#6082=CARTESIAN_POINT ( 'NONE',  ( 5.719274019375673035, 21.55341960407619339, 47.29275706135234003 ) ) ;
#6083=CARTESIAN_POINT ( 'NONE',  ( -8.314922557960811034, -14.29746914071050412, 102.0822429386476955 ) ) ;
#6084=CARTESIAN_POINT ( 'NONE',  ( -5.049401038298153566, 19.05341960407611168, 105.2072429386476671 ) ) ;
#6086=CARTESIAN_POINT ( 'NONE',  ( 4.379528057220092307, 16.55341960407617563, 77.29275706135234714 ) ) ;
#6087=CARTESIAN_POINT ( 'NONE',  ( -21.53943276465977519, -0.05219959533937600094, 98.75109039468568994 ) ) ;
#6088=CARTESIAN_POINT ( 'NONE',  ( -12.06949235617739369, -12.14591786802326823, 54.37609039468568994 ) ) ;
#6089=CARTESIAN_POINT ( 'NONE',  ( 16.46253265017160672, -9.564922557960803928, 98.33224293864769550 ) ) ;
#6090=CARTESIAN_POINT ( 'NONE',  ( 0.05219959533934541429, -16.53943276465976808, 40.00109039468567573 ) ) ;
#6091=CARTESIAN_POINT ( 'NONE',  ( -5.153800228976607833, 19.02544592524334988, 107.7094237280189759 ) ) ;
#6092=CARTESIAN_POINT ( 'NONE',  ( -8.224510206698735004, -14.34966873604973081, 79.58442372801903275 ) ) ;
#6093=CARTESIAN_POINT ( 'NONE',  ( -16.46253265017146816, -9.564922557961047289, 109.1677570613523471 ) ) ;
#6094=CARTESIAN_POINT ( 'NONE',  ( -5.049401038298153566, 19.05341960407611168, 75.20724293864769550 ) ) ;
#6095=CARTESIAN_POINT ( 'NONE',  ( 18.62759615963271287, -10.81492255796078972, 103.3322429386476955 ) ) ;
#6096=CARTESIAN_POINT ( 'NONE',  ( 16.53943276465976808, -0.05219959533910856209, 103.7489096053143669 ) ) ;
#6097=CARTESIAN_POINT ( 'NONE',  ( 16.46253265017146816, 9.564922557961045513, 106.6677570613523471 ) ) ;
#6098=CARTESIAN_POINT ( 'NONE',  ( -14.29746914071037622, -8.314922557961029526, 69.16775706135234714 ) ) ;
#6099=CARTESIAN_POINT ( 'NONE',  ( 19.02544592524334988, 5.153800228976608722, 76.45942372801897591 ) ) ;
#6100=CARTESIAN_POINT ( 'NONE',  ( 4.483927247898545687, 16.52544592524342804, 34.79057627198103120 ) ) ;
#6101=CARTESIAN_POINT ( 'NONE',  ( 8.314922557960818139, 14.29746914071049879, 99.58224293864770971 ) ) ;
#6102=CARTESIAN_POINT ( 'NONE',  ( -19.03943276465977164, -0.05219959533935918106, 33.75109039468566863 ) ) ;
#6103=CARTESIAN_POINT ( 'NONE',  ( -5.823673210054431948, 21.52544592524334988, 42.70942372801901854 ) ) ;
#6104=CARTESIAN_POINT ( 'NONE',  ( -13.89961937509957401, -13.97604488694547875, 94.37609039468566152 ) ) ;
#6105=CARTESIAN_POINT ( 'NONE',  ( 13.89961937509977652, -13.97604488694527269, 113.1239096053143527 ) ) ;
#6106=CARTESIAN_POINT ( 'NONE',  ( 19.02544592524343514, -5.153800228976328945, 88.54057627198102409 ) ) ;
#6107=CARTESIAN_POINT ( 'NONE',  ( -18.62759615963255300, -10.81492255796106328, 109.1677570613523613 ) ) ;
#6108=CARTESIAN_POINT ( 'NONE',  ( 13.97604488694527802, 13.89961937509977652, 74.37390960531436690 ) ) ;
#6109=CARTESIAN_POINT ( 'NONE',  ( 21.52544592524344225, -5.823673210054117533, 43.54057627198103830 ) ) ;
#6110=CARTESIAN_POINT ( 'NONE',  ( 12.14591786802309770, 12.06949235617756955, 94.37390960531436690 ) ) ;
#6111=CARTESIAN_POINT ( 'NONE',  ( 9.564922557960805705, 16.46253265017160317, 59.58224293864769550 ) ) ;
#6112=CARTESIAN_POINT ( 'NONE',  ( -14.29746914071049879, 8.314922557960819915, 115.8322429386477097 ) ) ;
#6113=CARTESIAN_POINT ( 'NONE',  ( -0.05219959533937732626, 21.53943276465977519, 27.50109039468567929 ) ) ;
#6114=CARTESIAN_POINT ( 'NONE',  ( 15.80617190586769283, -15.72974639402175789, 80.62609039468567573 ) ) ;
#6115=CARTESIAN_POINT ( 'NONE',  ( -0.05219959533909027116, -19.03943276465977164, 42.49890960531435269 ) ) ;
#6116=CARTESIAN_POINT ( 'NONE',  ( 16.52544592524335698, 4.483927247898782831, 81.45942372801900433 ) ) ;
#6117=CARTESIAN_POINT ( 'NONE',  ( -15.72974639402176322, -15.80617190586768395, 19.37609039468568639 ) ) ;
#6119=CARTESIAN_POINT ( 'NONE',  ( -5.719274019375665041, -21.55341960407619695, 29.79275706135234358 ) ) ;
#6120=CARTESIAN_POINT ( 'NONE',  ( -13.97604488694547697, 13.89961937509957934, 48.12609039468566863 ) ) ;
#6121=CARTESIAN_POINT ( 'NONE',  ( -13.97604488694527625, -13.89961937509977652, 61.87390960531435979 ) ) ;
#6122=CARTESIAN_POINT ( 'NONE',  ( -0.05219959533936034679, 19.03943276465977164, 32.50109039468566863 ) ) ;
#6123=CARTESIAN_POINT ( 'NONE',  ( 5.719274019375673035, 21.55341960407619339, 77.29275706135234714 ) ) ;
#6124=CARTESIAN_POINT ( 'NONE',  ( 21.55341960407610458, 5.719274019375980345, 68.95724293864769550 ) ) ;
#6125=CARTESIAN_POINT ( 'NONE',  ( -16.53943276465976808, 0.05219959533911058130, 46.24890960531435979 ) ) ;
#6126=CARTESIAN_POINT ( 'NONE',  ( 21.52544592524334988, 5.823673210054432836, 86.45942372801901854 ) ) ;
#6127=CARTESIAN_POINT ( 'NONE',  ( 19.02544592524334988, 5.153800228976608722, 31.45942372801900433 ) ) ;
#6128=CARTESIAN_POINT ( 'NONE',  ( -4.379528057220328563, 16.55341960407611168, 75.20724293864769550 ) ) ;
#6129=CARTESIAN_POINT ( 'NONE',  ( -19.05341960407611168, -5.049401038298163336, 26.45724293864769550 ) ) ;
#6130=CARTESIAN_POINT ( 'NONE',  ( 13.89961937509957401, 13.97604488694547697, 61.87609039468566863 ) ) ;
#6131=CARTESIAN_POINT ( 'NONE',  ( -14.34966873604960291, -8.224510206698953496, 26.66557627198103475 ) ) ;
#6132=CARTESIAN_POINT ( 'NONE',  ( 18.67979575497194134, -10.72451020669871369, 80.83442372801901854 ) ) ;
#6133=CARTESIAN_POINT ( 'NONE',  ( -5.049401038297874678, -19.05341960407617918, 44.79275706135232582 ) ) ;
#6134=CARTESIAN_POINT ( 'NONE',  ( -15.80617190586745835, -15.72974639402198527, 56.87390960531436690 ) ) ;
#6135=CARTESIAN_POINT ( 'NONE',  ( 21.53943276465977519, 0.05219959533937863772, 41.25109039468568284 ) ) ;
#6137=CARTESIAN_POINT ( 'NONE',  ( 18.62759615963271287, -10.81492255796078972, 98.33224293864769550 ) ) ;
#6138=CARTESIAN_POINT ( 'NONE',  ( 16.51473224551083163, -9.474510206698727899, 100.8344237280190043 ) ) ;
#6139=CARTESIAN_POINT ( 'NONE',  ( 12.14591786802327356, -12.06949235617739191, 70.62609039468567573 ) ) ;
#6140=CARTESIAN_POINT ( 'NONE',  ( 17.50000000000000000, -5.500000000000031086, 98.29690382534174375 ) ) ;
#6141=CARTESIAN_POINT ( 'NONE',  ( -21.52544592524343514, 5.823673210054127303, 106.0405762719810525 ) ) ;
#6142=CARTESIAN_POINT ( 'NONE',  ( -4.379528057220328563, 16.55341960407611168, 95.20724293864769550 ) ) ;
#6143=LINE ( 'NONE', #113321, #114368 ) ;
#6144=CARTESIAN_POINT ( 'NONE',  ( 12.06949235617739724, 12.14591786802326823, 41.87609039468568284 ) ) ;
#6146=CARTESIAN_POINT ( 'NONE',  ( 15.72974639402199770, -15.80617190586745480, 43.12390960531435269 ) ) ;
#6147=CARTESIAN_POINT ( 'NONE',  ( 16.53943276465976808, 0.05219959533934440121, 96.25109039468568994 ) ) ;
#6148=CARTESIAN_POINT ( 'NONE',  ( 13.97604488694527802, 13.89961937509977652, 24.37390960531435624 ) ) ;
#6150=CARTESIAN_POINT ( 'NONE',  ( -16.53943276465976808, -0.05219959533934237506, 63.75109039468568284 ) ) ;
#6151=CARTESIAN_POINT ( 'NONE',  ( 0.05219959533937995610, -21.53943276465977519, 40.00109039468567573 ) ) ;
#6152=CARTESIAN_POINT ( 'NONE',  ( 18.62759615963271287, -10.81492255796078972, 63.33224293864770260 ) ) ;
#6153=CARTESIAN_POINT ( 'NONE',  ( 8.314922557961029526, -14.29746914071037800, 80.41775706135234714 ) ) ;
#6154=CARTESIAN_POINT ( 'NONE',  ( 18.67979575497194134, -10.72451020669871369, 70.83442372801901854 ) ) ;
#6155=CARTESIAN_POINT ( 'NONE',  ( 15.72974639402199770, -15.80617190586745480, 58.12390960531435979 ) ) ;
#6156=CARTESIAN_POINT ( 'NONE',  ( 15.72974639402199770, -15.80617190586745480, 38.12390960531436690 ) ) ;
#6157=CARTESIAN_POINT ( 'NONE',  ( 0.05219959533934541429, -16.53943276465976808, 60.00109039468568284 ) ) ;
#6158=CARTESIAN_POINT ( 'NONE',  ( -21.55341960407610458, -5.719274019375992779, 36.45724293864768839 ) ) ;
#6160=CARTESIAN_POINT ( 'NONE',  ( -0.05219959533909027116, -19.03943276465977164, 102.4989096053143669 ) ) ;
#6161=CARTESIAN_POINT ( 'NONE',  ( 8.224510206698742110, 14.34966873604972548, 107.0844237280190043 ) ) ;
#6162=CARTESIAN_POINT ( 'NONE',  ( -18.09867054820431775, -5.499999999999927169, 78.98393025253584199 ) ) ;
#6163=CARTESIAN_POINT ( 'NONE',  ( 0.05219959533910956823, 16.53943276465976808, 114.9989096053143669 ) ) ;
#6164=CARTESIAN_POINT ( 'NONE',  ( 18.67979575497178502, 10.72451020669898547, 59.16557627198103120 ) ) ;
#6165=CARTESIAN_POINT ( 'NONE',  ( 19.05341960407611168, 5.049401038298154454, 38.95724293864767418 ) ) ;
#6166=CARTESIAN_POINT ( 'NONE',  ( 16.53943276465976808, 0.05219959533934440121, 96.25109039468568994 ) ) ;
#6167=CARTESIAN_POINT ( 'NONE',  ( 10.72451020669871369, 18.67979575497193778, 37.08442372801901143 ) ) ;
#6168=CARTESIAN_POINT ( 'NONE',  ( 0.05219959533936267826, -19.03943276465977164, 95.00109039468567573 ) ) ;
#6169=CARTESIAN_POINT ( 'NONE',  ( 12.06949235617757843, -12.14591786802309237, 108.1239096053143811 ) ) ;
#6170=CARTESIAN_POINT ( 'NONE',  ( 9.564922557960805705, 16.46253265017160317, 59.58224293864769550 ) ) ;
#6172=FACE_BOUND ( 'NONE', #14736, .T. ) ;
#6173=CARTESIAN_POINT ( 'NONE',  ( 9.564922557960805705, 16.46253265017160317, 79.58224293864769550 ) ) ;
#6174=CARTESIAN_POINT ( 'NONE',  ( 16.52544592524335698, 4.483927247898782831, 61.45942372801901854 ) ) ;
#6175=CARTESIAN_POINT ( 'NONE',  ( 10.81492255796106328, -18.62759615963255655, 100.4177570613523471 ) ) ;
#6176=CARTESIAN_POINT ( 'NONE',  ( 21.53943276465977519, -0.05219959533907433946, 48.74890960531435979 ) ) ;
#6177=CARTESIAN_POINT ( 'NONE',  ( -0.05219959533934338120, 16.53943276465976808, 72.50109039468568994 ) ) ;
#6178=CARTESIAN_POINT ( 'NONE',  ( -16.46253265017146816, -9.564922557961047289, 64.16775706135233293 ) ) ;
#6180=CARTESIAN_POINT ( 'NONE',  ( -15.72974639402176322, -15.80617190586768395, 69.37609039468567573 ) ) ;
#6181=CARTESIAN_POINT ( 'NONE',  ( 5.153800228976335163, 19.02544592524342804, 69.79057627198103830 ) ) ;
#6182=CARTESIAN_POINT ( 'NONE',  ( 9.474510206698971260, -16.51473224551069308, 32.91557627198102409 ) ) ;
#6183=CARTESIAN_POINT ( 'NONE',  ( 9.474510206698729675, 16.51473224551082808, 62.08442372801899722 ) ) ;
#6184=CARTESIAN_POINT ( 'NONE',  ( 5.153800228976335163, 19.02544592524342804, 109.7905762719810099 ) ) ;
#6185=CARTESIAN_POINT ( 'NONE',  ( 13.97604488694527802, 13.89961937509977652, 99.37390960531436690 ) ) ;
#6186=CARTESIAN_POINT ( 'NONE',  ( -16.52544592524342804, 4.483927247898546575, 56.04057627198102409 ) ) ;
#6187=CARTESIAN_POINT ( 'NONE',  ( -10.81492255796078084, -18.62759615963271287, 52.08224293864768839 ) ) ;
#6189=CARTESIAN_POINT ( 'NONE',  ( 5.153800228976615827, -19.02544592524334988, 30.20942372801900433 ) ) ;
#6191=CARTESIAN_POINT ( 'NONE',  ( 9.564922557960805705, 16.46253265017160317, 49.58224293864770260 ) ) ;
#6192=CARTESIAN_POINT ( 'NONE',  ( 12.14591786802327356, -12.06949235617739191, 35.62609039468568994 ) ) ;
#6195=CARTESIAN_POINT ( 'NONE',  ( -14.29746914071037622, -8.314922557961029526, 74.16775706135231871 ) ) ;
#6196=CARTESIAN_POINT ( 'NONE',  ( -15.80617190586745835, -15.72974639402198527, 96.87390960531436690 ) ) ;
#6198=CARTESIAN_POINT ( 'NONE',  ( -19.05341960407611168, -5.049401038298163336, 36.45724293864766707 ) ) ;
#6200=CARTESIAN_POINT ( 'NONE',  ( 5.719274019375673035, 21.55341960407619339, 37.29275706135235424 ) ) ;
#6201=CARTESIAN_POINT ( 'NONE',  ( -19.05341960407617563, 5.049401038297882671, 48.54275706135233293 ) ) ;
#6202=CARTESIAN_POINT ( 'NONE',  ( 9.564922557960805705, 16.46253265017160317, 44.58224293864769550 ) ) ;
#6203=CARTESIAN_POINT ( 'NONE',  ( 21.53943276465977519, 0.05219959533937863772, 101.2510903946856757 ) ) ;
#6204=CARTESIAN_POINT ( 'NONE',  ( 16.52216118717209525, 7.221426719304514741, 98.57599021046996768 ) ) ;
#6205=CARTESIAN_POINT ( 'NONE',  ( 8.314922557960818139, 14.29746914071049879, 34.58224293864770260 ) ) ;
#6206=CARTESIAN_POINT ( 'NONE',  ( 18.56399227203344893, 5.499999999999817923, 41.47830131249902763 ) ) ;
#6207=CARTESIAN_POINT ( 'NONE',  ( -0.05219959533907301413, -21.53943276465977519, 57.49890960531435979 ) ) ;
#6209=CARTESIAN_POINT ( 'NONE',  ( -16.51473224551069308, -9.474510206698971260, 96.66557627198102409 ) ) ;
#6210=CARTESIAN_POINT ( 'NONE',  ( -4.483927247898539470, -16.52544592524342804, 92.29057627198103830 ) ) ;
#6211=CARTESIAN_POINT ( 'NONE',  ( -19.03943276465977164, -0.05219959533935918106, 113.7510903946856757 ) ) ;
#6212=EDGE_CURVE ( 'NONE', #48812, #162452, #31629, .T. ) ;
#6213=CARTESIAN_POINT ( 'NONE',  ( -16.53943276465976808, -0.05219959533934237506, 103.7510903946857042 ) ) ;
#6215=CARTESIAN_POINT ( 'NONE',  ( 9.474510206698971260, -16.51473224551069308, 97.91557627198102409 ) ) ;
#6216=CARTESIAN_POINT ( 'NONE',  ( 5.823673210054125526, 21.52544592524343514, 99.79057627198103830 ) ) ;
#6217=CARTESIAN_POINT ( 'NONE',  ( -14.34966873604960291, -8.224510206698953496, 21.66557627198102409 ) ) ;
#6218=CARTESIAN_POINT ( 'NONE',  ( 9.474510206698971260, -16.51473224551069308, 97.91557627198102409 ) ) ;
#6219=CARTESIAN_POINT ( 'NONE',  ( -9.474510206698720793, -16.51473224551083518, 99.58442372801900433 ) ) ;
#6220=CARTESIAN_POINT ( 'NONE',  ( -21.52544592524334988, -5.823673210054445271, 108.9594237280190185 ) ) ;
#6221=CARTESIAN_POINT ( 'NONE',  ( 21.55341960407610458, 5.719274019375980345, 83.95724293864770971 ) ) ;
#6222=CARTESIAN_POINT ( 'NONE',  ( -10.72451020669898014, 18.67979575497178502, 45.41557627198103830 ) ) ;
#6223=CARTESIAN_POINT ( 'NONE',  ( 13.89961937509977652, -13.97604488694527269, 58.12390960531436690 ) ) ;
#6224=CARTESIAN_POINT ( 'NONE',  ( 12.06949235617757843, -12.14591786802309237, 38.12390960531436690 ) ) ;
#6225=CARTESIAN_POINT ( 'NONE',  ( 16.46253265017160672, -9.564922557960803928, 83.33224293864768129 ) ) ;
#6227=CARTESIAN_POINT ( 'NONE',  ( 18.87255363501903105, 5.499999999999944045, 58.82513748171828638 ) ) ;
#6228=CARTESIAN_POINT ( 'NONE',  ( 19.03943276465977164, 0.05219959533936151252, 41.25109039468566152 ) ) ;
#6229=CARTESIAN_POINT ( 'NONE',  ( -5.719274019375978568, 21.55341960407610458, 80.20724293864769550 ) ) ;
#6230=CARTESIAN_POINT ( 'NONE',  ( -8.224510206698948167, 14.34966873604960824, 80.41557627198103830 ) ) ;
#6231=CARTESIAN_POINT ( 'NONE',  ( -5.719274019375978568, 21.55341960407610458, 115.2072429386476955 ) ) ;
#6233=CARTESIAN_POINT ( 'NONE',  ( -4.483927247898782831, 16.52544592524335698, 112.7094237280190328 ) ) ;
#6234=CARTESIAN_POINT ( 'NONE',  ( 19.03943276465977164, -0.05219959533909143690, 28.74890960531435624 ) ) ;
#6235=CARTESIAN_POINT ( 'NONE',  ( -0.05219959533909027116, -19.03943276465977164, 92.49890960531436690 ) ) ;
#6238=CARTESIAN_POINT ( 'NONE',  ( 16.52544592524342804, -4.483927247898539470, 48.54057627198103120 ) ) ;
#6239=CARTESIAN_POINT ( 'NONE',  ( -15.80617190586768217, 15.72974639402176855, 63.12609039468568994 ) ) ;
#6241=CARTESIAN_POINT ( 'NONE',  ( 9.474510206698971260, -16.51473224551069308, 37.91557627198102409 ) ) ;
#6242=CARTESIAN_POINT ( 'NONE',  ( -16.51473224551069308, -9.474510206698971260, 46.66557627198102409 ) ) ;
#6243=ORIENTED_EDGE ( 'NONE', *, *, #128983, .F. ) ;
#6244=CARTESIAN_POINT ( 'NONE',  ( 21.53943276465977519, 0.05219959533937863772, 111.2510903946856899 ) ) ;
#6245=CARTESIAN_POINT ( 'NONE',  ( -16.52544592524335698, -4.483927247898792601, 63.95942372801901854 ) ) ;
#6246=CARTESIAN_POINT ( 'NONE',  ( 15.72974639402176855, 15.80617190586768217, 86.87609039468568994 ) ) ;
#6247=CARTESIAN_POINT ( 'NONE',  ( 13.97604488694527802, 13.89961937509977652, 114.3739096053143669 ) ) ;
#6248=CARTESIAN_POINT ( 'NONE',  ( 16.46253265017146816, 9.564922557961045513, 96.66775706135233293 ) ) ;
#6249=CARTESIAN_POINT ( 'NONE',  ( -21.55341960407619339, 5.719274019375674811, 63.54275706135234003 ) ) ;
#6250=CARTESIAN_POINT ( 'NONE',  ( -8.224510206698735004, -14.34966873604973081, 29.58442372801901854 ) ) ;
#6251=CARTESIAN_POINT ( 'NONE',  ( -18.67979575497178146, -10.72451020669898902, 81.66557627198103830 ) ) ;
#6252=CARTESIAN_POINT ( 'NONE',  ( -16.51473224551082808, 9.474510206698731452, 103.3344237280190043 ) ) ;
#6253=CARTESIAN_POINT ( 'NONE',  ( -5.153800228976328057, -19.02544592524343514, 62.29057627198100988 ) ) ;
#6254=CARTESIAN_POINT ( 'NONE',  ( 5.049401038297881783, 19.05341960407617563, 97.29275706135233293 ) ) ;
#6255=CARTESIAN_POINT ( 'NONE',  ( 16.51473224551083163, -9.474510206698727899, 100.8344237280190043 ) ) ;
#6256=CARTESIAN_POINT ( 'NONE',  ( -14.34966873604960291, -8.224510206698953496, 56.66557627198103830 ) ) ;
#6257=CARTESIAN_POINT ( 'NONE',  ( 0.05219959533936267826, -19.03943276465977164, 80.00109039468567573 ) ) ;
#6258=CARTESIAN_POINT ( 'NONE',  ( -12.14591786802326823, 12.06949235617739902, 63.12609039468568994 ) ) ;
#6259=CARTESIAN_POINT ( 'NONE',  ( -21.53943276465977519, -0.05219959533937600094, 18.75109039468568639 ) ) ;
#6260=CARTESIAN_POINT ( 'NONE',  ( -9.564922557960796823, -16.46253265017161027, 32.08224293864769550 ) ) ;
#6261=CARTESIAN_POINT ( 'NONE',  ( 16.51473224551069308, 9.474510206698969483, 54.16557627198103120 ) ) ;
#6262=CARTESIAN_POINT ( 'NONE',  ( -8.314922557961024197, 14.29746914071037800, 62.91775706135236135 ) ) ;
#6265=CARTESIAN_POINT ( 'NONE',  ( 9.564922557960805705, 16.46253265017160317, 104.5822429386476955 ) ) ;
#6268=CARTESIAN_POINT ( 'NONE',  ( 19.05341960407617918, -5.049401038297876454, 111.0427570613523329 ) ) ;
#6270=CARTESIAN_POINT ( 'NONE',  ( 18.62759615963271287, -10.81492255796078972, 38.33224293864768839 ) ) ;
#6271=CARTESIAN_POINT ( 'NONE',  ( -0.05219959533936034679, 19.03943276465977164, 42.50109039468566152 ) ) ;
#6272=CARTESIAN_POINT ( 'NONE',  ( 16.55341960407618274, -4.379528057220086978, 26.04275706135235779 ) ) ;
#6273=CARTESIAN_POINT ( 'NONE',  ( 19.05341960407611168, 5.049401038298154454, 23.95724293864769194 ) ) ;
#6274=CARTESIAN_POINT ( 'NONE',  ( -19.02544592524342804, 5.153800228976336051, 51.04057627198103120 ) ) ;
#6275=CARTESIAN_POINT ( 'NONE',  ( -21.55341960407610458, -5.719274019375992779, 86.45724293864770971 ) ) ;
#6276=CARTESIAN_POINT ( 'NONE',  ( -16.46253265017160317, 9.564922557960807481, 110.8322429386476955 ) ) ;
#6277=CARTESIAN_POINT ( 'NONE',  ( 16.51473224551069308, 9.474510206698969483, 54.16557627198103120 ) ) ;
#6279=CARTESIAN_POINT ( 'NONE',  ( -16.51473224551082808, 9.474510206698731452, 83.33442372801899012 ) ) ;
#6280=CARTESIAN_POINT ( 'NONE',  ( -4.483927247898539470, -16.52544592524342804, 67.29057627198103830 ) ) ;
#6281=CARTESIAN_POINT ( 'NONE',  ( 21.55341960407619695, -5.719274019375665929, 106.0427570613523471 ) ) ;
#6282=CARTESIAN_POINT ( 'NONE',  ( 18.67979575497178502, 10.72451020669898547, 104.1655762719810241 ) ) ;
#6283=CARTESIAN_POINT ( 'NONE',  ( 21.55341960407619695, -5.719274019375665929, 86.04275706135236135 ) ) ;
#6284=CARTESIAN_POINT ( 'NONE',  ( 21.52544592524334988, 5.823673210054432836, 81.45942372801900433 ) ) ;
#6285=CARTESIAN_POINT ( 'NONE',  ( 16.46253265017160672, -9.564922557960803928, 103.3322429386476955 ) ) ;
#6286=CARTESIAN_POINT ( 'NONE',  ( 8.314922557961029526, -14.29746914071037800, 110.4177570613523756 ) ) ;
#6287=CARTESIAN_POINT ( 'NONE',  ( 5.823673210054444382, -21.52544592524334988, 80.20942372801901854 ) ) ;
#6288=CARTESIAN_POINT ( 'NONE',  ( -19.05341960407611168, -5.049401038298163336, 61.45724293864769550 ) ) ;
#6289=CARTESIAN_POINT ( 'NONE',  ( 21.55341960407619695, -5.719274019375665929, 46.04275706135234714 ) ) ;
#6290=CARTESIAN_POINT ( 'NONE',  ( 5.153800228976335163, 19.02544592524342804, 84.79057627198099567 ) ) ;
#6291=CARTESIAN_POINT ( 'NONE',  ( 14.29746914071049879, -8.314922557960816363, 83.33224293864769550 ) ) ;
#6292=CARTESIAN_POINT ( 'NONE',  ( -0.05219959533910754901, -16.53943276465976808, 67.49890960531436690 ) ) ;
#6293=CARTESIAN_POINT ( 'NONE',  ( 18.67979575497178502, 10.72451020669898547, 64.16557627198102409 ) ) ;
#6294=CARTESIAN_POINT ( 'NONE',  ( -19.03943276465977164, 0.05219959533909376836, 56.24890960531435979 ) ) ;
#6295=CARTESIAN_POINT ( 'NONE',  ( -21.52544592524343514, 5.823673210054127303, 71.04057627198103830 ) ) ;
#6296=CARTESIAN_POINT ( 'NONE',  ( -19.02544592524334988, -5.153800228976617603, 58.95942372801900433 ) ) ;
#6297=CARTESIAN_POINT ( 'NONE',  ( 9.474510206698729675, 16.51473224551082808, 37.08442372801899722 ) ) ;
#6298=CARTESIAN_POINT ( 'NONE',  ( 12.06949235617757843, -12.14591786802309237, 73.12390960531436690 ) ) ;
#6299=CARTESIAN_POINT ( 'NONE',  ( -15.80617190586745835, -15.72974639402198527, 51.87390960531437401 ) ) ;
#6302=CARTESIAN_POINT ( 'NONE',  ( 12.14591786802327356, -12.06949235617739191, 100.6260903946857184 ) ) ;
#6304=CARTESIAN_POINT ( 'NONE',  ( -5.153800228976607833, 19.02544592524334988, 107.7094237280189759 ) ) ;
#6305=CARTESIAN_POINT ( 'NONE',  ( -4.379528057220328563, 16.55341960407611168, 65.20724293864768129 ) ) ;
#6306=CARTESIAN_POINT ( 'NONE',  ( -17.49999999999999645, 5.499999999999992895, 68.71769037696435589 ) ) ;
#6307=CARTESIAN_POINT ( 'NONE',  ( 13.89961937509977652, -13.97604488694527269, 63.12390960531435979 ) ) ;
#6308=CARTESIAN_POINT ( 'NONE',  ( 14.34966873604960469, 8.224510206698951720, 49.16557627198102409 ) ) ;
#6309=CARTESIAN_POINT ( 'NONE',  ( 19.05341960407611168, 5.049401038298154454, 88.95724293864769550 ) ) ;
#6310=CARTESIAN_POINT ( 'NONE',  ( 5.049401038297881783, 19.05341960407617563, 77.29275706135231871 ) ) ;
#6311=CARTESIAN_POINT ( 'NONE',  ( 5.153800228976335163, 19.02544592524342804, 64.79057627198100988 ) ) ;
#6312=CARTESIAN_POINT ( 'NONE',  ( 19.03943276465977164, -0.05219959533909143690, 83.74890960531436690 ) ) ;
#6313=CARTESIAN_POINT ( 'NONE',  ( 5.049401038298161559, -19.05341960407611168, 67.70724293864769550 ) ) ;
#6314=CARTESIAN_POINT ( 'NONE',  ( -15.80617190586745835, -15.72974639402198527, 61.87390960531436690 ) ) ;
#6315=CARTESIAN_POINT ( 'NONE',  ( -0.05219959533934338120, 16.53943276465976808, 62.50109039468568284 ) ) ;
#6316=CARTESIAN_POINT ( 'NONE',  ( -9.474510206698720793, -16.51473224551083518, 104.5844237280190043 ) ) ;
#6317=CARTESIAN_POINT ( 'NONE',  ( -5.049401038298153566, 19.05341960407611168, 55.20724293864769550 ) ) ;
#6318=CARTESIAN_POINT ( 'NONE',  ( 0.05219959533907565091, 21.53943276465977519, 54.99890960531435269 ) ) ;
#6319=CARTESIAN_POINT ( 'NONE',  ( 5.049401038297881783, 19.05341960407617563, 82.29275706135229029 ) ) ;
#6320=CARTESIAN_POINT ( 'NONE',  ( -0.05219959533934338120, 16.53943276465976808, 112.5010903946857042 ) ) ;
#6321=CARTESIAN_POINT ( 'NONE',  ( -0.05219959533936034679, 19.03943276465977164, 42.50109039468566152 ) ) ;
#6322=CARTESIAN_POINT ( 'NONE',  ( -12.06949235617739369, -12.14591786802326823, 64.37609039468568994 ) ) ;
#6323=CARTESIAN_POINT ( 'NONE',  ( -0.05219959533934338120, 16.53943276465976808, 92.50109039468567573 ) ) ;
#6325=CARTESIAN_POINT ( 'NONE',  ( 12.06949235617739724, 12.14591786802326823, 81.87609039468568994 ) ) ;
#6326=CARTESIAN_POINT ( 'NONE',  ( 15.72974639402199770, -15.80617190586745480, 28.12390960531435979 ) ) ;
#6327=CARTESIAN_POINT ( 'NONE',  ( 16.46253265017160672, -9.564922557960803928, 48.33224293864769550 ) ) ;
#6328=CARTESIAN_POINT ( 'NONE',  ( -9.564922557960796823, -16.46253265017161027, 47.08224293864769550 ) ) ;
#6329=CARTESIAN_POINT ( 'NONE',  ( -5.153800228976328057, -19.02544592524343514, 47.29057627198102409 ) ) ;
#6330=CARTESIAN_POINT ( 'NONE',  ( 18.67979575497194134, -10.72451020669871369, 35.83442372801901143 ) ) ;
#6331=CARTESIAN_POINT ( 'NONE',  ( 16.52544592524335698, 4.483927247898782831, 51.45942372801901854 ) ) ;
#6332=CARTESIAN_POINT ( 'NONE',  ( -12.06949235617756955, 12.14591786802309770, 25.62390960531435624 ) ) ;
#6333=CARTESIAN_POINT ( 'NONE',  ( -5.153800228976328057, -19.02544592524343514, 27.29057627198103120 ) ) ;
#6334=CARTESIAN_POINT ( 'NONE',  ( 9.564922557961047289, -16.46253265017146816, 20.41775706135233293 ) ) ;
#6335=CARTESIAN_POINT ( 'NONE',  ( -9.564922557961040184, 16.46253265017147172, 112.9177570613523329 ) ) ;
#6336=CARTESIAN_POINT ( 'NONE',  ( -13.97604488694547697, 13.89961937509957934, 63.12609039468566152 ) ) ;
#6337=CARTESIAN_POINT ( 'NONE',  ( -12.06949235617756955, 12.14591786802309770, 65.62390960531436690 ) ) ;
#6338=CARTESIAN_POINT ( 'NONE',  ( -5.049401038298153566, 19.05341960407611168, 40.20724293864768839 ) ) ;
#6339=CARTESIAN_POINT ( 'NONE',  ( 9.474510206698729675, 16.51473224551082808, 77.08442372801900433 ) ) ;
#6340=CARTESIAN_POINT ( 'NONE',  ( 16.81555441253551564, 7.025013491695499823, 76.86314554665744936 ) ) ;
#6341=CARTESIAN_POINT ( 'NONE',  ( -18.62759615963255300, -10.81492255796106328, 79.16775706135234714 ) ) ;
#6342=CARTESIAN_POINT ( 'NONE',  ( -8.224510206698735004, -14.34966873604973081, 39.58442372801901143 ) ) ;
#6344=CARTESIAN_POINT ( 'NONE',  ( 21.52544592524344225, -5.823673210054117533, 33.54057627198102409 ) ) ;
#6345=CARTESIAN_POINT ( 'NONE',  ( 14.29746914071037800, 8.314922557961029526, 31.66775706135234358 ) ) ;
#6346=CARTESIAN_POINT ( 'NONE',  ( 17.97214573761835510, 5.499999999999910294, 88.96970049038655759 ) ) ;
#6347=CARTESIAN_POINT ( 'NONE',  ( 0.05219959533937995610, -21.53943276465977519, 110.0010903946856757 ) ) ;
#6349=CARTESIAN_POINT ( 'NONE',  ( 0.05219959533909260263, 19.03943276465977164, 34.99890960531435979 ) ) ;
#6351=CARTESIAN_POINT ( 'NONE',  ( -19.03943276465977164, 0.05219959533909376836, 51.24890960531436690 ) ) ;
#6352=CARTESIAN_POINT ( 'NONE',  ( 21.55341960407619695, -5.719274019375665929, 66.04275706135236135 ) ) ;
#6353=CARTESIAN_POINT ( 'NONE',  ( 5.049401038297881783, 19.05341960407617563, 22.29275706135233648 ) ) ;
#6354=CARTESIAN_POINT ( 'NONE',  ( 0.05219959533910956823, 16.53943276465976808, 29.99890960531435979 ) ) ;
#6355=CARTESIAN_POINT ( 'NONE',  ( 9.564922557960805705, 16.46253265017160317, 29.58224293864769550 ) ) ;
#6356=CARTESIAN_POINT ( 'NONE',  ( -5.153800228976328057, -19.02544592524343514, 97.29057627198099567 ) ) ;
#6357=CARTESIAN_POINT ( 'NONE',  ( 5.823673210054444382, -21.52544592524334988, 50.20942372801901854 ) ) ;
#6358=CARTESIAN_POINT ( 'NONE',  ( 9.474510206698971260, -16.51473224551069308, 37.91557627198102409 ) ) ;
#6359=CARTESIAN_POINT ( 'NONE',  ( -21.52544592524334988, -5.823673210054445271, 63.95942372801901854 ) ) ;
#6360=CARTESIAN_POINT ( 'NONE',  ( 9.564922557961047289, -16.46253265017146816, 90.41775706135234714 ) ) ;
#6361=CARTESIAN_POINT ( 'NONE',  ( 5.153800228976335163, 19.02544592524342804, 109.7905762719810099 ) ) ;
#6362=CARTESIAN_POINT ( 'NONE',  ( -16.51473224551069308, -9.474510206698971260, 21.66557627198102765 ) ) ;
#6363=CARTESIAN_POINT ( 'NONE',  ( -21.53943276465977519, 0.05219959533907696930, 106.2489096053143811 ) ) ;
#6364=CARTESIAN_POINT ( 'NONE',  ( -9.564922557961040184, 16.46253265017147172, 32.91775706135233293 ) ) ;
#6365=CARTESIAN_POINT ( 'NONE',  ( 16.55341960407611168, 4.379528057220329451, 108.9572429386476955 ) ) ;
#6366=CARTESIAN_POINT ( 'NONE',  ( 5.153800228976335163, 19.02544592524342804, 59.79057627198100988 ) ) ;
#6367=CARTESIAN_POINT ( 'NONE',  ( 5.153800228976615827, -19.02544592524334988, 100.2094237280190043 ) ) ;
#6368=CARTESIAN_POINT ( 'NONE',  ( 14.34966873604960469, 8.224510206698951720, 64.16557627198102409 ) ) ;
#6369=CARTESIAN_POINT ( 'NONE',  ( 0.05219959533907565091, 21.53943276465977519, 24.99890960531435624 ) ) ;
#6370=CARTESIAN_POINT ( 'NONE',  ( 19.03943276465977164, 0.05219959533936151252, 91.25109039468566152 ) ) ;
#6371=CARTESIAN_POINT ( 'NONE',  ( -10.81492255796078084, -18.62759615963271287, 97.08224293864770971 ) ) ;
#6372=CARTESIAN_POINT ( 'NONE',  ( 10.72451020669871369, 18.67979575497193778, 42.08442372801901854 ) ) ;
#6373=CARTESIAN_POINT ( 'NONE',  ( -16.55341960407617563, 4.379528057220093196, 38.54275706135234714 ) ) ;
#6374=CARTESIAN_POINT ( 'NONE',  ( 12.06949235617739724, 12.14591786802326823, 41.87609039468568284 ) ) ;
#6375=CARTESIAN_POINT ( 'NONE',  ( 15.80617190586769283, -15.72974639402175789, 55.62609039468568284 ) ) ;
#6376=CARTESIAN_POINT ( 'NONE',  ( 18.62759615963271287, -10.81492255796078972, 53.33224293864769550 ) ) ;
#6377=CARTESIAN_POINT ( 'NONE',  ( 13.97604488694527802, 13.89961937509977652, 34.37390960531436690 ) ) ;
#6379=CARTESIAN_POINT ( 'NONE',  ( 0.05219959533934541429, -16.53943276465976808, 70.00109039468568994 ) ) ;
#6380=EDGE_CURVE ( 'NONE', #65463, #186347, #182275, .T. ) ;
#6381=CARTESIAN_POINT ( 'NONE',  ( 10.81492255796078972, 18.62759615963270932, 104.5822429386477097 ) ) ;
#6382=CARTESIAN_POINT ( 'NONE',  ( -8.314922557960811034, -14.29746914071050412, 42.08224293864769550 ) ) ;
#6383=CARTESIAN_POINT ( 'NONE',  ( 14.29746914071037800, 8.314922557961029526, 61.66775706135235424 ) ) ;
#6384=CARTESIAN_POINT ( 'NONE',  ( 19.02544592524334988, 5.153800228976608722, 101.4594237280189759 ) ) ;
#6385=CARTESIAN_POINT ( 'NONE',  ( 21.55341960407610458, 5.719274019375980345, 93.95724293864770971 ) ) ;
#6386=CARTESIAN_POINT ( 'NONE',  ( -14.34966873604960291, -8.224510206698953496, 31.66557627198102054 ) ) ;
#6388=CARTESIAN_POINT ( 'NONE',  ( -12.06949235617739369, -12.14591786802326823, 74.37609039468568994 ) ) ;
#6390=CARTESIAN_POINT ( 'NONE',  ( -5.719274019375978568, 21.55341960407610458, 70.20724293864769550 ) ) ;
#6391=CARTESIAN_POINT ( 'NONE',  ( 14.29746914071037800, 8.314922557961029526, 111.6677570613523613 ) ) ;
#6394=CARTESIAN_POINT ( 'NONE',  ( -10.72451020669898014, 18.67979575497178502, 105.4155762719810383 ) ) ;
#6395=CARTESIAN_POINT ( 'NONE',  ( -0.05219959533907301413, -21.53943276465977519, 112.4989096053143669 ) ) ;
#6396=CARTESIAN_POINT ( 'NONE',  ( -4.379528057220328563, 16.55341960407611168, 35.20724293864768839 ) ) ;
#6397=CARTESIAN_POINT ( 'NONE',  ( -14.34966873604972548, 8.224510206698743886, 43.33442372801901143 ) ) ;
#6398=CARTESIAN_POINT ( 'NONE',  ( 13.89961937509977652, -13.97604488694527269, 53.12390960531434558 ) ) ;
#6399=CARTESIAN_POINT ( 'NONE',  ( 9.474510206698971260, -16.51473224551069308, 67.91557627198102409 ) ) ;
#6400=CARTESIAN_POINT ( 'NONE',  ( -19.02544592524342804, 5.153800228976336051, 111.0405762719810099 ) ) ;
#6402=CARTESIAN_POINT ( 'NONE',  ( 19.03943276465977164, 0.05219959533936151252, 101.2510903946856757 ) ) ;
#6403=CARTESIAN_POINT ( 'NONE',  ( 9.564922557961047289, -16.46253265017146816, 50.41775706135233293 ) ) ;
#6404=CARTESIAN_POINT ( 'NONE',  ( 18.62759615963271287, -10.81492255796078972, 93.33224293864769550 ) ) ;
#6405=CARTESIAN_POINT ( 'NONE',  ( -8.314922557961024197, 14.29746914071037800, 112.9177570613523329 ) ) ;
#6406=CARTESIAN_POINT ( 'NONE',  ( 0.05219959533907565091, 21.53943276465977519, 49.99890960531437401 ) ) ;
#6407=CARTESIAN_POINT ( 'NONE',  ( -10.81492255796078084, -18.62759615963271287, 77.08224293864769550 ) ) ;
#6408=CARTESIAN_POINT ( 'NONE',  ( 19.03943276465977164, 0.05219959533936151252, 111.2510903946856757 ) ) ;
#6409=CARTESIAN_POINT ( 'NONE',  ( 16.46253265017160672, -9.564922557960803928, 113.3322429386476955 ) ) ;
#6410=CARTESIAN_POINT ( 'NONE',  ( -15.72974639402176322, -15.80617190586768395, 79.37609039468567573 ) ) ;
#6411=CARTESIAN_POINT ( 'NONE',  ( -19.02544592524342804, 5.153800228976336051, 76.04057627198102409 ) ) ;
#6414=CARTESIAN_POINT ( 'NONE',  ( 5.153800228976335163, 19.02544592524342804, 69.79057627198103830 ) ) ;
#6415=CARTESIAN_POINT ( 'NONE',  ( -14.29746914071049879, 8.314922557960819915, 85.83224293864768129 ) ) ;
#6417=CARTESIAN_POINT ( 'NONE',  ( 13.97604488694548053, -13.89961937509957401, 110.6260903946856615 ) ) ;
#6419=CARTESIAN_POINT ( 'NONE',  ( -9.564922557960796823, -16.46253265017161027, 77.08224293864769550 ) ) ;
#6420=CARTESIAN_POINT ( 'NONE',  ( -5.719274019375665041, -21.55341960407619695, 89.79275706135236135 ) ) ;
#6421=CARTESIAN_POINT ( 'NONE',  ( -19.03943276465977164, 0.05219959533909376836, 106.2489096053143669 ) ) ;
#6422=CARTESIAN_POINT ( 'NONE',  ( 12.14591786802327356, -12.06949235617739191, 80.62609039468567573 ) ) ;
#6423=CARTESIAN_POINT ( 'NONE',  ( -16.61371651742603106, -7.165104196376148593, 76.14584930007006847 ) ) ;
#6424=CARTESIAN_POINT ( 'NONE',  ( 19.03943276465977164, 0.05219959533936151252, 51.25109039468567573 ) ) ;
#6425=CARTESIAN_POINT ( 'NONE',  ( -5.719274019375665041, -21.55341960407619695, 109.7927570613523613 ) ) ;
#6428=CARTESIAN_POINT ( 'NONE',  ( -8.224510206698948167, 14.34966873604960824, 25.41557627198103120 ) ) ;
#6430=CARTESIAN_POINT ( 'NONE',  ( 8.314922557961029526, -14.29746914071037800, 105.4177570613523613 ) ) ;
#6432=CARTESIAN_POINT ( 'NONE',  ( 16.55341960407618274, -4.379528057220086978, 81.04275706135236135 ) ) ;
#6433=CARTESIAN_POINT ( 'NONE',  ( -18.62759615963255300, -10.81492255796106328, 79.16775706135234714 ) ) ;
#6434=CARTESIAN_POINT ( 'NONE',  ( -5.049401038297874678, -19.05341960407617918, 89.79275706135230450 ) ) ;
#6435=CARTESIAN_POINT ( 'NONE',  ( -16.51473224551082808, 9.474510206698731452, 33.33442372801899722 ) ) ;
#6436=CARTESIAN_POINT ( 'NONE',  ( 9.564922557960805705, 16.46253265017160317, 74.58224293864769550 ) ) ;
#6437=CARTESIAN_POINT ( 'NONE',  ( 16.51473224551069308, 9.474510206698969483, 54.16557627198103120 ) ) ;
#6438=CARTESIAN_POINT ( 'NONE',  ( 17.50000000000000711, -5.499999999999978684, 41.21769037696436300 ) ) ;
#6439=CARTESIAN_POINT ( 'NONE',  ( 5.823673210054125526, 21.52544592524343514, 89.79057627198103830 ) ) ;
#6441=CARTESIAN_POINT ( 'NONE',  ( 5.823673210054125526, 21.52544592524343514, 44.79057627198103120 ) ) ;
#6442=CARTESIAN_POINT ( 'NONE',  ( 19.02544592524343514, -5.153800228976328945, 43.54057627198103120 ) ) ;
#6443=CARTESIAN_POINT ( 'NONE',  ( -0.05219959533934338120, 16.53943276465976808, 67.50109039468568994 ) ) ;
#6444=EDGE_CURVE ( 'NONE', #40791, #194062, #8567, .T. ) ;
#6446=CARTESIAN_POINT ( 'NONE',  ( 10.72451020669871369, 18.67979575497193778, 47.08442372801901854 ) ) ;
#6447=CARTESIAN_POINT ( 'NONE',  ( 4.379528057220339221, -16.55341960407611168, 67.70724293864769550 ) ) ;
#6449=CARTESIAN_POINT ( 'NONE',  ( -12.14591786802326823, 12.06949235617739902, 33.12609039468569705 ) ) ;
#6450=CARTESIAN_POINT ( 'NONE',  ( -8.314922557960811034, -14.29746914071050412, 97.08224293864770971 ) ) ;
#6451=CARTESIAN_POINT ( 'NONE',  ( 13.89961937509957401, 13.97604488694547697, 46.87609039468565442 ) ) ;
#6452=CARTESIAN_POINT ( 'NONE',  ( -8.314922557960811034, -14.29746914071050412, 77.08224293864769550 ) ) ;
#6453=CARTESIAN_POINT ( 'NONE',  ( 21.52544592524334988, 5.823673210054432836, 31.45942372801901854 ) ) ;
#6454=CARTESIAN_POINT ( 'NONE',  ( -19.02544592524342804, 5.153800228976336051, 26.04057627198103120 ) ) ;
#6455=CARTESIAN_POINT ( 'NONE',  ( -15.72974639402197994, 15.80617190586746368, 95.62390960531436690 ) ) ;
#6456=CARTESIAN_POINT ( 'NONE',  ( -13.89961937509977652, 13.97604488694528158, 100.6239096053143669 ) ) ;
#6457=CARTESIAN_POINT ( 'NONE',  ( -14.29746914071049879, 8.314922557960819915, 70.83224293864770971 ) ) ;
#6458=CARTESIAN_POINT ( 'NONE',  ( -9.474510206698964154, 16.51473224551069663, 115.4155762719810241 ) ) ;
#6460=CARTESIAN_POINT ( 'NONE',  ( -5.049401038297874678, -19.05341960407617918, 79.79275706135233293 ) ) ;
#6461=CARTESIAN_POINT ( 'NONE',  ( -21.55341960407619339, 5.719274019375674811, 23.54275706135235424 ) ) ;
#6462=CARTESIAN_POINT ( 'NONE',  ( -19.05341960407611168, -5.049401038298163336, 66.45724293864769550 ) ) ;
#6463=CARTESIAN_POINT ( 'NONE',  ( 5.049401038297881783, 19.05341960407617563, 52.29275706135234003 ) ) ;
#6464=CARTESIAN_POINT ( 'NONE',  ( -16.46253265017160317, 9.564922557960807481, 30.83224293864769550 ) ) ;
#6465=CARTESIAN_POINT ( 'NONE',  ( 10.72451020669871369, 18.67979575497193778, 77.08442372801901854 ) ) ;
#6466=CARTESIAN_POINT ( 'NONE',  ( 0.05219959533910956823, 16.53943276465976808, 64.99890960531435269 ) ) ;
#6467=CARTESIAN_POINT ( 'NONE',  ( 16.52544592524342804, -4.483927247898539470, 53.54057627198103120 ) ) ;
#6468=CARTESIAN_POINT ( 'NONE',  ( -5.153800228976328057, -19.02544592524343514, 62.29057627198100988 ) ) ;
#6469=CARTESIAN_POINT ( 'NONE',  ( 10.72451020669898902, -18.67979575497178502, 82.91557627198103830 ) ) ;
#6470=CARTESIAN_POINT ( 'NONE',  ( 13.97604488694527802, 13.89961937509977652, 54.37390960531435979 ) ) ;
#6471=ORIENTED_EDGE ( 'NONE', *, *, #12002, .T. ) ;
#6472=CARTESIAN_POINT ( 'NONE',  ( -15.80617190586745835, -15.72974639402198527, 76.87390960531439532 ) ) ;
#6473=CARTESIAN_POINT ( 'NONE',  ( 15.80617190586769283, -15.72974639402175789, 100.6260903946857184 ) ) ;
#6475=CARTESIAN_POINT ( 'NONE',  ( 14.34966873604972726, -8.224510206698740333, 110.8344237280190043 ) ) ;
#6476=CARTESIAN_POINT ( 'NONE',  ( -16.55341960407611168, -4.379528057220339221, 101.4572429386476955 ) ) ;
#6477=CARTESIAN_POINT ( 'NONE',  ( 19.05341960407617918, -5.049401038297876454, 91.04275706135234714 ) ) ;
#6479=CARTESIAN_POINT ( 'NONE',  ( 15.72974639402176855, 15.80617190586768217, 21.87609039468567573 ) ) ;
#6480=CARTESIAN_POINT ( 'NONE',  ( -13.89961937509957401, -13.97604488694547875, 59.37609039468566863 ) ) ;
#6481=CARTESIAN_POINT ( 'NONE',  ( -16.55341960407617563, 4.379528057220093196, 98.54275706135234714 ) ) ;
#6482=CARTESIAN_POINT ( 'NONE',  ( 9.474510206698729675, 16.51473224551082808, 37.08442372801899722 ) ) ;
#6483=CARTESIAN_POINT ( 'NONE',  ( 16.46253265017160672, -9.564922557960803928, 98.33224293864769550 ) ) ;
#6484=CARTESIAN_POINT ( 'NONE',  ( 5.719274019375991003, -21.55341960407610458, 67.70724293864769550 ) ) ;
#6486=CARTESIAN_POINT ( 'NONE',  ( 13.97604488694527802, 13.89961937509977652, 29.37390960531435979 ) ) ;
#6487=CARTESIAN_POINT ( 'NONE',  ( -15.72974639402176322, -15.80617190586768395, 109.3760903946857042 ) ) ;
#6488=CARTESIAN_POINT ( 'NONE',  ( 12.14591786802327356, -12.06949235617739191, 70.62609039468567573 ) ) ;
#6489=CARTESIAN_POINT ( 'NONE',  ( 10.81492255796106328, -18.62759615963255655, 25.41775706135235779 ) ) ;
#6490=CARTESIAN_POINT ( 'NONE',  ( -14.34966873604972548, 8.224510206698743886, 48.33442372801902565 ) ) ;
#6491=CARTESIAN_POINT ( 'NONE',  ( 13.89961937509977652, -13.97604488694527269, 108.1239096053143669 ) ) ;
#6492=CARTESIAN_POINT ( 'NONE',  ( 16.51473224551069308, 9.474510206698969483, 54.16557627198103120 ) ) ;
#6493=CARTESIAN_POINT ( 'NONE',  ( -19.05341960407611168, -5.049401038298163336, 71.45724293864766707 ) ) ;
#6494=CARTESIAN_POINT ( 'NONE',  ( 16.55341960407618274, -4.379528057220086978, 41.04275706135236135 ) ) ;
#6495=CARTESIAN_POINT ( 'NONE',  ( -16.55341960407611168, -4.379528057220339221, 96.45724293864770971 ) ) ;
#6496=CARTESIAN_POINT ( 'NONE',  ( 16.52544592524335698, 4.483927247898782831, 106.4594237280190328 ) ) ;
#6498=CARTESIAN_POINT ( 'NONE',  ( -21.52544592524334988, -5.823673210054445271, 58.95942372801902565 ) ) ;
#6499=CARTESIAN_POINT ( 'NONE',  ( 16.46253265017160672, -9.564922557960803928, 78.33224293864769550 ) ) ;
#6500=CARTESIAN_POINT ( 'NONE',  ( 13.89961937509977652, -13.97604488694527269, 63.12390960531435979 ) ) ;
#6501=CARTESIAN_POINT ( 'NONE',  ( -13.97604488694527625, -13.89961937509977652, 96.87390960531433848 ) ) ;
#6502=CARTESIAN_POINT ( 'NONE',  ( -16.53943276465976808, 0.05219959533911058130, 51.24890960531436690 ) ) ;
#6503=CARTESIAN_POINT ( 'NONE',  ( 14.34966873604972726, -8.224510206698740333, 95.83442372801903275 ) ) ;
#6504=CARTESIAN_POINT ( 'NONE',  ( 8.224510206698953496, -14.34966873604960469, 42.91557627198103120 ) ) ;
#6506=CARTESIAN_POINT ( 'NONE',  ( -16.51473224551082808, 9.474510206698731452, 38.33442372801899722 ) ) ;
#6507=CARTESIAN_POINT ( 'NONE',  ( -16.46253265017160317, 9.564922557960807481, 105.8322429386476955 ) ) ;
#6508=CARTESIAN_POINT ( 'NONE',  ( -19.05341960407611168, -5.049401038298163336, 66.45724293864769550 ) ) ;
#6509=CARTESIAN_POINT ( 'NONE',  ( 16.46253265017146816, 9.564922557961045513, 41.66775706135234003 ) ) ;
#6512=CARTESIAN_POINT ( 'NONE',  ( 17.72662750342724891, 5.500000000000079048, 58.90179492283742491 ) ) ;
#6513=CARTESIAN_POINT ( 'NONE',  ( 16.51473224551083163, -9.474510206698727899, 90.83442372801900433 ) ) ;
#6514=CARTESIAN_POINT ( 'NONE',  ( 16.55341960407618274, -4.379528057220086978, 71.04275706135234714 ) ) ;
#6516=CARTESIAN_POINT ( 'NONE',  ( 9.474510206698971260, -16.51473224551069308, 87.91557627198102409 ) ) ;
#6517=CARTESIAN_POINT ( 'NONE',  ( -15.72974639402176322, -15.80617190586768395, 34.37609039468568284 ) ) ;
#6518=CARTESIAN_POINT ( 'NONE',  ( -16.46253265017146816, -9.564922557961047289, 79.16775706135234714 ) ) ;
#6520=CARTESIAN_POINT ( 'NONE',  ( -13.97604488694527625, -13.89961937509977652, 41.87390960531435979 ) ) ;
#6521=CARTESIAN_POINT ( 'NONE',  ( 9.474510206698971260, -16.51473224551069308, 92.91557627198103830 ) ) ;
#6522=CARTESIAN_POINT ( 'NONE',  ( -16.52544592524342804, 4.483927247898546575, 51.04057627198103120 ) ) ;
#6523=CARTESIAN_POINT ( 'NONE',  ( 9.564922557960805705, 16.46253265017160317, 34.58224293864770260 ) ) ;
#6524=CARTESIAN_POINT ( 'NONE',  ( -9.564922557961040184, 16.46253265017147172, 47.91775706135233293 ) ) ;
#6525=CARTESIAN_POINT ( 'NONE',  ( -4.483927247898539470, -16.52544592524342804, 92.29057627198103830 ) ) ;
#6526=CARTESIAN_POINT ( 'NONE',  ( -9.474510206698720793, -16.51473224551083518, 29.58442372801900433 ) ) ;
#6527=CARTESIAN_POINT ( 'NONE',  ( 19.05341960407611168, 5.049401038298154454, 63.95724293864769550 ) ) ;
#6528=CARTESIAN_POINT ( 'NONE',  ( 5.823673210054125526, 21.52544592524343514, 69.79057627198102409 ) ) ;
#6529=CARTESIAN_POINT ( 'NONE',  ( 16.53943276465976808, -0.05219959533910856209, 68.74890960531435269 ) ) ;
#6530=CARTESIAN_POINT ( 'NONE',  ( -16.46253265017146816, -9.564922557961047289, 19.16775706135233293 ) ) ;
#6531=CARTESIAN_POINT ( 'NONE',  ( 0.05219959533909260263, 19.03943276465977164, 99.99890960531436690 ) ) ;
#6532=CARTESIAN_POINT ( 'NONE',  ( -21.52544592524343514, 5.823673210054127303, 26.04057627198103475 ) ) ;
#6533=CARTESIAN_POINT ( 'NONE',  ( 16.51473224551069308, 9.474510206698969483, 49.16557627198102409 ) ) ;
#6534=CARTESIAN_POINT ( 'NONE',  ( -9.474510206698964154, 16.51473224551069663, 35.41557627198102409 ) ) ;
#6535=CARTESIAN_POINT ( 'NONE',  ( -16.52544592524342804, 4.483927247898546575, 106.0405762719810525 ) ) ;
#6536=CARTESIAN_POINT ( 'NONE',  ( 10.81492255796078972, 18.62759615963270932, 109.5822429386476955 ) ) ;
#6537=CARTESIAN_POINT ( 'NONE',  ( -5.049401038298153566, 19.05341960407611168, 95.20724293864770971 ) ) ;
#6538=CARTESIAN_POINT ( 'NONE',  ( 10.81492255796078972, 18.62759615963270932, 109.5822429386476955 ) ) ;
#6539=CARTESIAN_POINT ( 'NONE',  ( 9.564922557960805705, 16.46253265017160317, 104.5822429386476955 ) ) ;
#6540=CARTESIAN_POINT ( 'NONE',  ( -16.53943276465976808, 0.05219959533911058130, 116.2489096053143669 ) ) ;
#6541=CARTESIAN_POINT ( 'NONE',  ( -21.53943276465977519, -0.05219959533937600094, 83.75109039468568994 ) ) ;
#6542=CARTESIAN_POINT ( 'NONE',  ( -10.72451020669898014, 18.67979575497178502, 90.41557627198103830 ) ) ;
#6544=CARTESIAN_POINT ( 'NONE',  ( -19.03943276465977164, -0.05219959533935918106, 18.75109039468567218 ) ) ;
#6545=CARTESIAN_POINT ( 'NONE',  ( 5.153800228976335163, 19.02544592524342804, 59.79057627198101699 ) ) ;
#6546=CARTESIAN_POINT ( 'NONE',  ( 16.53943276465976808, 0.05219959533934440121, 46.25109039468567573 ) ) ;
#6547=CARTESIAN_POINT ( 'NONE',  ( 14.34966873604960469, 8.224510206698951720, 109.1655762719810383 ) ) ;
#6548=CARTESIAN_POINT ( 'NONE',  ( -17.50000000000147082, -3.202012800152271854, 110.0717758397273798 ) ) ;
#6549=CARTESIAN_POINT ( 'NONE',  ( -5.153800228976328057, -19.02544592524343514, 57.29057627198103120 ) ) ;
#6550=CARTESIAN_POINT ( 'NONE',  ( -8.224510206698948167, 14.34966873604960824, 100.4155762719810241 ) ) ;
#6552=CARTESIAN_POINT ( 'NONE',  ( 18.62759615963271287, -10.81492255796078972, 43.33224293864769550 ) ) ;
#6553=CARTESIAN_POINT ( 'NONE',  ( -16.55341960407611168, -4.379528057220339221, 66.45724293864768129 ) ) ;
#6554=CARTESIAN_POINT ( 'NONE',  ( -16.51473224551082808, 9.474510206698731452, 113.3344237280190043 ) ) ;
#6555=CARTESIAN_POINT ( 'NONE',  ( -18.67979575497193778, 10.72451020669871902, 68.33442372801900433 ) ) ;
#6557=CARTESIAN_POINT ( 'NONE',  ( -16.52544592524335698, -4.483927247898792601, 103.9594237280190185 ) ) ;
#6558=CARTESIAN_POINT ( 'NONE',  ( -16.53943276465976808, 0.05219959533911058130, 41.24890960531435269 ) ) ;
#6559=CARTESIAN_POINT ( 'NONE',  ( -9.564922557960796823, -16.46253265017161027, 42.08224293864769550 ) ) ;
#6560=CARTESIAN_POINT ( 'NONE',  ( 19.03943276465977164, -0.05219959533909143690, 93.74890960531435269 ) ) ;
#6561=CARTESIAN_POINT ( 'NONE',  ( 18.67979575497178502, 10.72451020669898547, 94.16557627198103830 ) ) ;
#6562=( BOUNDED_SURFACE ( )  B_SPLINE_SURFACE ( 3, 2, ( 
 ( #143243, #5730, #54248, #146237, #11506, #73177, #68402, #175595, #99737, #81557, #36072, #196526, #21913, #97721, #57997, #26671, #52240, #88312, #35085, #160424, #98731, #83564, #4726, #66416, #7724, #150000, #159411, #69410, #114914, #115920, #53237, #119667, #96738, #20906, #190765, #158427, #84559, #128077, #192765, #130054, #131076, #177610, #113897, #145243, #189780, #82565, #144246, #67409, #6724, #30624, #169119, #266, #13471, #90298, #93269, #137797, #58970, #16450, #75134, #61934, #120638, #31619, #60947, #154954, #92277, #74162, #44804, #122622, #42828, #138785, #104493, #181349, #78099, #170124, #199481, #76119, #106459, #184312, #29634, #166175, #27676, #182336, #1256, #168138, #153961, #14456, #123603, #89316, #135834, #197503, #139768, #45793, #15459, #151009, #107445, #12500, #91267, #62933, #108448, #43814, #77115, #185298, #167164, #105477, #28663, #46789, #151983, #136804, #198488, #59961, #121627, #183323, #152958, #36569, #6235, #35586, #96253, #189289, #187309, #141764, #49768, #155945, #5233, #48780, #17441, #34595, #95265, #157940, #79097, #50767, #140770, #19431, #128578, #81078, #2259, #126589, #63942, #159927, #110434, #125610, #82059, #124613, #142757, #97232, #51749, #172116, #4237, #113410, #112425, #175101, #158920, #65917, #94266, #127590, #98224, #21416, #83074, #143753, #156948, #33602, #174116, #18445, #80096, #20410, #66914, #144750, #3256, #47789, #111433, #64930, #188291, #186308, #173120, #190272, #109440, #171123, #32612, #37578, #71920, #25446, #69925, #39579, #84071, #54749, #52740, #146752, #178111, #40590, #195282, #149763, #179122, #101238, #132594, #130578, #85070, #193276, #99241, #148771, #192273, #160930, #162927, #38591, #24435, #22421, #194284, #145750, #86083, #133591, #147774, #7231, #131591, #68916, #103261, #53755, #115429, #87086, #67914, #9261, #102261, #56764, #177120, #70927, #118436, #55750, #180129, #163948, #117424, #100246, #10260, #41597, #164943, #26436, #88077, #161928, #23422, #129567, #8247, #116423, #191265, #114407, #176108, #73931, #134607, #198253, #135600, #120404, #169894, #59728, #30389, #61703, #90071, #105246, #181117, #15222, #168884, #13246, #183091, #27436, #121398, #196293, #151753, #44573, #184076, #138552, #123372, #91042, #185065, #199246, #104254, #74909, #152729, #72938, #92036, #57763, #11266, #46553, #29, #167912, #106228, #136573, #29412, #14219, #119433, #42591, #12267, #31388, #75888, #60713, #137563, #153726, #165937, #89079, #150770, #108215, #122387, #45560, #197272, #107214, #58734, #76881, #93037, #182097, #43581, #166933, #28435, #140543, #16220, #155714, #20180, #170889, #2031, #173889, #128346, #63711, #51519, #66684, #190045, #35358, #65688, #113181, #174871, #188064, #95032, #19205, #139540, #17210, #36337, #141541, #78863, #154725, #143513, #171886, #5001, #77873, #79872, #18214, #156722, #1024, #62697, #127352, #124379, #32381, #189066, #34368, #97009, #172889, #186074, #96029, #111197, #80854, #81826, #47557, #112199, #125386, #94035, #157715, #187083, #48552, #142531, #126368, #109210, #110206, #33374, #3030, #64706, #49535, #4009, #50537, #158691, #148534, #176881, #192027, #67680, #102022, #55515, #100006, #69685, #114168, #84831, #82836, #38351, #8001, #70693, #25207, #10025, #177879, #71685, #85846, #191033, #161693, #39347, #159684, #117186, #21181, #97990, #133351, #86849, #54518, #193040, #23188, #116190, #146511, #144516, #6001, #99001, #118197, #131352, #147536, #101006, #40347, #129338, #52508, #175871, #195042, #162690, #9024, #37343, #24196, #160691, #132360, #179889, #56519, #22182, #194052, #178880, #83832, #145513, #6994, #163705, #68675, #130330, #53511, #115188, #88842, #138328, #153493, #14989, #123146, #152498, #13014, #105996, #104019, #58507, #166697, #74678, #73697, #44339, #26199, #30156, #89842, #167683, #150534, #136345, #91799, #164703, #137330, #134369 ),
 ( #76650, #149525, #60479, #199011, #197040, #87838, #11021, #122154, #198020, #200009, #105013, #61475, #72694, #29179, #59489, #196053, #12034, #183843, #13986, #41356, #103020, #121164, #181864, #90815, #57528, #42357, #119197, #28200, #165698, #180882, #27196, #120173, #135369, #43343, #151523, #182857, #75652, #45332, #106982, #168656, #173651, #62466, #157480, #64472, #65452, #2793, #46319, #794, #18972, #155486, #143276, #110962, #111961, #142295, #17981, #79635, #80618, #63476, #78632, #184833, #77646, #187834, #31157, #140307, #34134, #172646, #3775, #16978, #93807, #96771, #141304, #124139, #19949, #1798, #127115, #185838, #47325, #188821, #126139, #95793, #125151, #108981, #49304, #50304, #81590, #35119, #158460, #186850, #48319, #107974, #4760, #169661, #109974, #92806, #66448, #170661, #171654, #154493, #15988, #33143, #139315, #32149, #94801, #156480, #146273, #86609, #68437, #83597, #163466, #162449, #129098, #24963, #36104, #147291, #23950, #145277, #174639, #97756, #85605, #22947, #148292, #191789, #178637, #159444, #115954, #161456, #20939, #98763, #8781, #39111, #101778, #9786, #84593, #130091, #192799, #112946, #190798, #128109, #114948, #52272, #189814, #116944, #6758, #40100, #51285, #53270, #176641, #38117, #82596, #144278, #100767, #5766, #67441, #70451, #7760, #132116, #69443, #113930, #175630, #193809, #160456, #37104, #54282, #55274, #21948, #131111, #177643, #99771, #150301, #165466, #71448, #164469, #74447, #117958, #26962, #120924, #59255, #90590, #103786, #180649, #183615, #27963, #149292, #106755, #88605, #152272, #10786, #72453, #75424, #89604, #197789, #11797, #134128, #136113, #12781, #168430, #182623, #137098, #73461, #135135, #194801, #44108, #56275, #196809, #179649, #105766, #195817, #58276, #198784, #167453, #119945, #151293, #60250, #43110, #181630, #28949, #41119, #121921, #104778, #13756, #118965, #166466, #45098, #102783, #29926, #25963, #91565, #153253, #133113, #87606, #57289, #42124, #32907, #64237, #122912, #79399, #184600, #140065, #34883, #142054, #46081, #141070, #187602, #556, #76416, #15749, #80382, #30922, #62227, #33897, #188584, #123895, #111726, #126878, #50065, #96538, #125903, #186609, #2555, #77408, #31912, #1556, #107736, #95554, #139078, #169417, #124911, #185594, #48081, #92570, #49071, #154258, #109737, #18735, #171421, #47083, #16740, #108744, #173412, #170420, #93565, #172408, #14755, #94561, #110727, #3540, #155251, #156240, #65218, #157241, #138092, #199773, #78389, #17742, #61240, #63232, #85363, #55041, #115721, #128865, #174405, #161218, #97520, #5527, #37878, #129854, #131884, #20701, #81359, #145040, #82357, #67207, #116711, #6522, #177409, #8539, #36860, #52040, #127874, #162216, #38880, #160220, #191552, #35874, #68201, #143043, #98527, #53029, #130874, #147055, #70217, #99536, #193569, #146038, #51050, #21710, #22713, #19717, #100537, #4521, #158227, #178401, #39865, #114710, #176403, #83364, #84360, #7522, #66214, #189578, #159207, #112712, #69206, #192564, #54047, #23715, #144045, #190565, #113696, #175392, #181398, #73226, #75183, #164233, #24724, #88361, #25729, #10548, #60011, #150054, #120686, #152033, #180413, #195577, #71215, #105528, #59019, #103552, #134897, #117715, #11560, #86373, #41885, #196574, #74212, #28711, #13518, #42876, #136855, #89366, #194567, #165227, #104541, #163223, #182385, #148058, #101531, #198540, #90347, #58044, #119714, #26722, #166222, #27723, #9549, #132878, #102549, #121678, #151055, #12546, #135880, #43863, #56037, #179411, #40876, #183374, #197551, #167214, #87375, #149060, #72212, #133886, #57050, #118725, #153008, #171173, #20211, #30674, #106511, #45841, #113216, #60999, #92327, #66719, #21216, #154013, #144551, #159719, #82873, #129373, #155992, #16500, #109490, #107493, #61983, #170176, #76169, #128380, #169170, #137849, #155003, #15508, #78148, #199530, #32660, #122671, #139817 ),
 ( #36370, #184360, #81859, #124662, #190076, #62983, #168188, #77165, #143547, #138835, #6036, #94314, #174906, #5033, #1304, #186358, #51552, #47838, #185347, #98024, #29685, #315, #67715, #31669, #123649, #44855, #91317, #46837, #14507, #108497, #93319, #54550, #193075, #175907, #37379, #102057, #179924, #68709, #163742, #70727, #71718, #9056, #52542, #7027, #25242, #161728, #149560, #117222, #118233, #148568, #24232, #85883, #86883, #69719, #84866, #191069, #83867, #194087, #99036, #146544, #40383, #178916, #10058, #23223, #100042, #103056, #147571, #130366, #26233, #8037, #133386, #192063, #53545, #195077, #132394, #56556, #131386, #115223, #55549, #41391, #87872, #164738, #11056, #116223, #177914, #114203, #72731, #160726, #39382, #22218, #145549, #176915, #101041, #38386, #162727, #182891, #152532, #138360, #106030, #166732, #137364, #119231, #123179, #44374, #199043, #181898, #29214, #184868, #57561, #30191, #27229, #167716, #200041, #16021, #61510, #88877, #104053, #14019, #92839, #74715, #89876, #169693, #168690, #135404, #31187, #42390, #153526, #91833, #151559, #180915, #165733, #15023, #90847, #154524, #198055, #46350, #150570, #122188, #75685, #12069, #105048, #76684, #45365, #108008, #134404, #196091, #60513, #183880, #59521, #107018, #73731, #197075, #58542, #120208, #43376, #121198, #28236, #13048, #136378, #62501, #32182, #170693, #112982, #95829, #127149, #185873, #142329, #47359, #2827, #97792, #4796, #109014, #3809, #50340, #63512, #139347, #78665, #143309, #93838, #125187, #96810, #51321, #186883, #174675, #189847, #36140, #159481, #188857, #49335, #65487, #140342, #94836, #64505, #155518, #158496, #1830, #17013, #187867, #48353, #110997, #110007, #111997, #171688, #172683, #81626, #34167, #33177, #79669, #156515, #77678, #18016, #141340, #35154, #826, #157513, #173688, #66485, #126172, #19007, #128147, #19983, #124172, #80653, #99809, #39146, #177678, #147329, #148327, #117995, #178673, #191827, #37141, #23986, #160494, #68475, #100801, #192836, #194839, #83636, #144314, #7799, #145313, #130130, #179684, #69483, #40137, #71483, #161495, #114986, #190834, #25000, #101814, #22983, #54317, #98800, #131148, #5804, #84633, #115989, #193845, #9822, #133148, #162485, #56312, #8816, #113967, #146310, #85643, #82632, #163502, #67477, #20975, #41156, #102819, #129137, #52310, #175666, #132152, #70486, #55309, #6797, #38155, #116981, #21984, #86644, #53308, #176679, #74481, #135169, #197822, #195852, #28981, #57324, #59288, #168462, #120957, #180683, #166500, #103819, #199806, #150336, #42159, #121954, #164504, #182656, #75455, #91597, #88640, #44140, #153287, #152304, #14788, #198816, #43142, #105799, #167485, #90622, #76448, #61273, #183647, #196842, #165499, #13789, #26995, #11831, #137129, #136146, #138125, #73497, #87640, #151326, #58309, #119977, #122943, #12814, #45129, #184632, #104811, #181663, #134163, #29960, #106788, #27998, #60281, #89637, #46113, #149326, #25998, #10820, #72490, #119000, #158258, #187632, #19748, #95587, #586, #171451, #49102, #169451, #65250, #30953, #107766, #81389, #96570, #64267, #2587, #32939, #125933, #156272, #92600, #154290, #108774, #127906, #94594, #157271, #141100, #50097, #15780, #62258, #123926, #143075, #110760, #18767, #77439, #172441, #139111, #17774, #189608, #34914, #185624, #33929, #80414, #93597, #47115, #170452, #173446, #31943, #155283, #126910, #4553, #16773, #142086, #3572, #78421, #188616, #140097, #79429, #1588, #66246, #63263, #111757, #124943, #186640, #48111, #109767, #116744, #67238, #36894, #70250, #24760, #98559, #148092, #163258, #86407, #132913, #162250, #22744, #115753, #113729, #68232, #176436, #82390, #131918, #175426, #144078, #161250, #21743, #84393, #5559, #177441, #128897, #146069, #55074, #7554, #190596, #53063, #52073, #9583, #160253, #83395, #69240, #23749, #35905, #85398, #39902, #145072, #147091 ),
 ( #8575, #129885, #6554, #51082, #191585, #54079, #97551, #114742, #100568, #38911, #193602, #37910, #99569, #71249, #130906, #192596, #112742, #178434, #101567, #174435, #159239, #20733, #151088, #120718, #88395, #72245, #197584, #135913, #91349, #182416, #198573, #196606, #58077, #117752, #59051, #179445, #119747, #102584, #167245, #133922, #134929, #60043, #43896, #42908, #12579, #121711, #166256, #26755, #105559, #40911, #183404, #104574, #28744, #41920, #89399, #44887, #164268, #90380, #25763, #149094, #87409, #29717, #74244, #152065, #10584, #13550, #195613, #181430, #14540, #106544, #57085, #75216, #136888, #180448, #56072, #118759, #168220, #103586, #165261, #153041, #76201, #150088, #194600, #11592, #73260, #27756, #48856, #109522, #2339, #346, #155036, #63016, #169202, #18522, #62015, #30708, #47869, #108529, #171204, #92358, #64020, #154044, #32694, #141841, #94345, #15539, #139847, #77197, #173194, #123679, #107525, #126663, #3332, #137880, #110511, #65006, #185378, #156024, #188367, #125689, #49844, #172192, #16531, #17521, #79179, #187388, #111508, #34670, #95339, #170208, #138866, #140850, #46868, #31701, #33677, #157024, #96328, #93350, #61030, #124695, #78178, #1336, #158015, #186392, #80169, #19506, #199561, #122702, #184392, #45872, #7308, #175178, #144826, #174192, #21491, #4312, #113484, #83152, #22499, #53834, #177196, #191338, #38669, #37656, #112498, #98303, #52816, #81151, #68993, #65995, #142833, #23499, #162003, #114484, #176187, #6310, #99321, #67988, #189364, #35660, #143830, #127664, #129642, #130658, #161005, #100324, #50841, #97308, #84146, #158994, #20487, #145825, #85147, #192351, #146833, #5310, #82136, #66994, #115508, #128653, #190348, #51824, #36644, #160003, #77840, #95993, #32348, #20145, #188029, #189026, #19168, #95000, #156686, #157678, #140509, #155682, #61670, #154690, #64670, #108178, #17177, #111162, #49500, #80817, #94001, #170857, #173853, #18180, #139507, #96973, #78831, #142495, #990, #62664, #65653, #79837, #172851, #1998, #124344, #126332, #2992, #158654, #34332, #127315, #63677, #125352, #185032, #3973, #46519, #187049, #169859, #50500, #186039, #48519, #112164, #35319, #110173, #141507, #81790, #33340, #171852, #143477, #31353, #123339, #93004, #16185, #109178, #47522, #194015, #128309, #100970, #97955, #38316, #70657, #86812, #132323, #159647, #174835, #23151, #163668, #145477, #160655, #40311, #39311, #5964, #101987, #113145, #24161, #162655, #22147, #51483, #36300, #85812, #99971, #25170, #68638, #55478, #21143, #193005, #161655, #82798, #175833, #147498, #116152, #178843, #4961, #84795, #6958, #69649, #190009, #67642, #66647, #191988, #129301, #177843, #190997, #144480, #52473, #117148, #114132, #37306, #8989, #98965, #83797, #130294, #53475, #115152, #176845, #146474, #7966, #131315, #54482, #165663, #73661, #179851, #29145, #72659, #41322, #58472, #119163, #181830, #102982, #12980, #164667, #43309, #152466, #104977, #26163, #150501, #87804, #183810, #134334, #118161, #137298, #13952, #148498, #59455, #75618, #196018, #166664, #198979, #136310, #60446, #182823, #27161, #28165, #89807, #74644, #122121, #45298, #105964, #180846, #149490, #151489, #10986, #57494, #197985, #120139, #106950, #42323, #71649, #135333, #103984, #88809, #168623, #197006, #167649, #30123, #11998, #121129, #44305, #9989, #90782, #133316, #195005, #56483, #181944, #58587, #64312, #29259, #167761, #125980, #16817, #32986, #28283, #89922, #149610, #93644, #11108, #151604, #134453, #1634, #165784, #166782, #94639, #155329, #74761, #44421, #156320, #198103, #120253, #78468, #72783, #17820, #136423, #140142, #73778, #121244, #79478, #196138, #124990, #119278, #59569, #141146, #110806, #2636, #180961, #57609, #106074, #187678, #13095, #43427, #27279, #88927, #49148, #26281, #105096, #182938, #87923, #63311, #186686, #42438, #48156, #104101, #109814, #171497, #150619 ),
 ( #12115, #135451, #197120, #192642, #35949, #160299, #5604, #114789, #157319, #126955, #65296, #7600, #190643, #21789, #80459, #36943, #142133, #97595, #54125, #99616, #3617, #98605, #145118, #158305, #33976, #173491, #37958, #188664, #19793, #191631, #146116, #81434, #69286, #84438, #130952, #172488, #83440, #144123, #6602, #34964, #189655, #159283, #50143, #53111, #96616, #111803, #82435, #143120, #67284, #4600, #68281, #66292, #128942, #176482, #52119, #127951, #174482, #51128, #95632, #112788, #20780, #161296, #22792, #18815, #129932, #113775, #175471, #133972, #42958, #103635, #166310, #150141, #194650, #195663, #72293, #41968, #104621, #12628, #73309, #86455, #131964, #118810, #55121, #163308, #57134, #87456, #89448, #178482, #38957, #102632, #39948, #24806, #74293, #164317, #134980, #27807, #56120, #9631, #85446, #119795, #148140, #135962, #165312, #151137, #196657, #149142, #10633, #11643, #117802, #71298, #115798, #8624, #180496, #162296, #132961, #26806, #88446, #58126, #179495, #40960, #197632, #181479, #193649, #177488, #25810, #100614, #116790, #101619, #23796, #147136, #70296, #91403, #94396, #62067, #395, #156077, #46921, #63069, #61079, #122752, #182465, #123732, #43946, #184442, #167296, #31752, #198627, #199613, #124748, #185431, #107576, #77246, #186444, #30761, #153091, #108581, #105608, #47920, #169254, #170258, #106595, #154094, #109574, #28792, #155087, #152117, #92408, #171257, #140905, #32744, #13600, #90431, #138914, #17573, #45922, #14595, #79234, #93401, #60093, #59099, #75268, #78229, #16581, #76251, #136938, #121761, #139900, #15588, #120764, #1388, #183454, #44939, #168271, #29768, #137929, #173246, #21542, #113536, #176236, #37707, #35712, #142882, #67046, #187440, #3382, #99369, #189416, #65057, #161052, #191388, #19557, #52865, #2391, #4364, #51877, #159045, #175230, #48908, #36695, #114536, #80220, #98356, #82188, #83202, #20539, #64070, #18573, #160055, #125740, #144877, #129691, #22547, #143881, #84193, #190401, #95391, #66047, #5362, #110562, #6359, #172243, #33730, #157077, #141891, #128704, #97359, #127714, #68039, #50891, #126714, #188418, #49895, #111562, #112549, #34721, #96379, #158066, #81201, #174244, #38716, #181237, #164069, #195407, #53882, #10384, #115557, #71050, #166058, #73058, #177244, #72041, #118559, #131719, #7356, #146884, #11388, #162052, #193401, #165061, #119554, #54876, #42713, #57882, #104375, #27559, #56885, #117547, #133715, #8376, #163052, #132716, #100374, #26555, #70051, #23548, #55874, #116550, #179246, #85196, #180249, #178239, #40712, #149882, #102381, #39700, #147898, #101363, #145873, #24559, #86208, #134730, #196412, #69041, #41719, #130706, #9384, #25568, #192400, #103383, #194404, #88198, #87212, #148894, #45678, #15342, #16338, #186195, #46672, #59847, #105361, #92157, #28549, #136688, #169002, #60831, #62816, #151869, #12386, #76007, #13359, #198370, #47676, #137682, #108332, #139654, #168028, #183209, #58855, #93156, #170012, #91158, #122506, #167048, #30506, #89199, #171009, #107329, #154841, #184196, #121514, #153844, #74048, #77987, #199367, #76998, #44690, #138670, #1142, #135719, #185182, #182215, #150, #124500, #150892, #109327, #43699, #120522, #61819, #197390, #29525, #106344, #90186, #123489, #75023, #152847, #14341, #31503, #128461, #188180, #78983, #2150, #190157, #127471, #67802, #96142, #82959, #140658, #20293, #65803, #63828, #3146, #51633, #143632, #6119, #129457, #189177, #173005, #97121, #17328, #33490, #191156, #19322, #95148, #52629, #21302, #49652, #144636, #32500, #34484, #81941, #50650, #5116, #125500, #66798, #114293, #110321, #113297, #112311, #174988, #174001, #94152, #48669, #36452, #64820, #155831, #158804, #159807, #98110, #35472, #187198, #172002, #111316, #126482, #156837, #18332, #79987, #141655, #157831, #80969, #142645, #4124, #8123, #84949, #87958, #132477, #53634, #11144 ),
 ( #180009, #177992, #39459, #99126, #40467, #160816, #101120, #83955, #148654, #115311, #116303, #41476, #102139, #24315, #177003, #103140, #164822, #131469, #69801, #72818, #178999, #117303, #134487, #163824, #26318, #162806, #85964, #22304, #25325, #145635, #147653, #7115, #10142, #38472, #9141, #149646, #86967, #70808, #194166, #196174, #55630, #193156, #71802, #68797, #57646, #133471, #195162, #23305, #56643, #175995, #130456, #118316, #192153, #37465, #100129, #161810, #146631, #54628, #88963, #137447, #77758, #59607, #74794, #154605, #153607, #120288, #16100, #27316, #138437, #15103, #136456, #165819, #150653, #76764, #14101, #139424, #182973, #169774, #12151, #107096, #152611, #73816, #89957, #200118, #30269, #92919, #906, #75769, #121280, #183956, #104137, #181981, #119312, #106111, #43463, #180998, #108090, #135486, #91914, #105131, #197156, #31268, #123255, #42474, #61587, #46431, #166817, #199126, #58621, #168766, #28318, #184946, #198137, #60593, #122268, #45443, #151637, #13132, #44457, #167795, #29295, #90925, #1914, #110093, #142414, #34251, #36218, #125268, #185954, #49419, #186966, #171771, #21061, #111081, #81708, #113062, #141423, #156604, #32264, #66565, #20064, #64588, #144398, #155599, #2910, #112082, #19087, #35238, #47438, #173772, #51402, #140424, #96892, #3892, #143392, #80735, #124259, #78747, #158575, #33260, #82715, #188946, #189927, #4883, #95911, #157595, #128230, #126253, #18098, #62581, #17094, #65572, #109095, #79753, #174754, #50423, #97871, #94918, #187950, #159562, #127231, #63593, #170774, #172771, #93921, #48436, #145394, #9903, #71563, #161573, #38233, #41236, #8899, #147411, #102897, #193927, #133228, #7878, #69564, #129218, #70567, #190915, #131230, #114049, #178755, #6877, #146390, #194919, #132235, #54397, #24069, #56394, #177757, #99888, #55390, #52392, #118077, #116069, #117060, #53391, #100882, #179767, #175747, #101898, #98882, #39226, #164582, #87720, #26076, #160576, #37225, #85724, #5883, #192919, #23066, #67560, #40220, #68555, #22065, #83716, #25080, #163580, #84712, #130211, #191906, #86723, #162565, #115069, #148408, #176761, #195935, #137212, #182740, #57409, #120058, #168543, #60367, #123028, #184714, #44224, #89723, #13870, #134248, #150421, #46198, #136228, #11916, #107851, #29063, #196924, #61357, #31036, #122039, #121044, #75537, #73580, #166583, #74561, #180763, #30041, #135252, #42239, #59372, #181745, #105882, #103900, #198899, #165581, #167569, #153372, #90702, #27079, #138211, #119081, #183729, #58391, #88725, #199893, #14874, #149405, #45215, #76535, #43227, #152385, #169536, #106870, #10900, #91680, #28083, #72573, #104894, #151409, #12897, #197903, #50185, #63354, #108860, #95675, #32029, #140184, #172531, #64353, #66331, #155370, #15867, #79517, #16859, #1676, #51168, #141187, #111842, #143160, #171537, #186727, #62343, #96656, #173532, #94680, #126022, #170539, #34017, #92685, #174520, #154373, #65336, #19832, #4640, #157361, #127992, #80501, #185710, #156359, #18855, #77525, #35001, #139197, #672, #189695, #81473, #49189, #187718, #17862, #110847, #2676, #124012, #47200, #93687, #112828, #142174, #3658, #126996, #158343, #78510, #125031, #48198, #109852, #188703, #33025, #144160, #103420, #5645, #161337, #58894, #166097, #67322, #165099, #11426, #21828, #97634, #36983, #104414, #52157, #83480, #57920, #12424, #145158, #135757, #150931, #56922, #197428, #176522, #191670, #74087, #73096, #98645, #120560, #128984, #119591, #134767, #53149, #82475, #190682, #196450, #133753, #35987, #99653, #89237, #113814, #26592, #72079, #175509, #6642, #181274, #149920, #159323, #20819, #195447, #37998, #88235, #160339, #68320, #129970, #22829, #114828, #84476, #118597, #148931, #10421, #180287, #41755, #42751, #27599, #154880, #167086, #93195, #171047, #59886, #16378, #61859, #62857, #190, #43739, #198409, #78025, #152885, #140697, #108376 ),
 ( #170052, #1180, #14380, #91195, #94190, #138709, #121552, #17367, #76046, #124539, #183248, #44729, #186236, #47715, #137722, #199406, #79022, #185222, #123528, #2187, #31543, #109365, #184236, #45717, #105400, #46713, #28588, #107370, #90224, #139694, #106385, #122546, #32537, #155870, #30548, #63869, #182254, #153884, #60869, #151908, #13397, #75061, #92200, #136727, #29564, #77038, #168066, #169042, #15381, #18373, #158846, #191195, #7158, #52670, #80025, #95190, #175030, #113338, #144675, #157872, #34523, #37504, #81983, #3185, #160856, #19361, #6160, #64858, #126520, #129496, #114333, #81010, #142685, #22346, #128503, #66840, #83997, #36495, #176036, #127512, #189216, #48706, #190198, #110359, #50695, #33528, #98149, #188219, #65842, #99166, #51676, #174044, #143676, #145676, #97161, #4164, #159849, #172041, #125540, #35513, #21342, #173046, #20334, #187236, #156876, #83000, #141694, #5157, #49692, #111357, #96183, #112353, #67840, #87011, #27357, #9185, #24357, #104179, #103185, #69844, #165861, #177045, #88001, #164866, #86008, #115355, #38515, #26361, #163870, #89003, #132519, #119357, #100171, #56686, #102182, #161853, #39502, #149689, #180053, #42516, #150694, #25369, #70850, #133514, #53678, #131512, #68841, #55673, #193198, #130500, #148697, #116345, #192196, #23347, #194208, #118360, #10185, #41522, #84992, #11187, #57689, #146673, #72862, #71845, #134532, #195206, #8168, #54671, #196219, #101162, #178034, #181041, #162850, #147697, #117347, #179043, #40511, #90964, #106152, #12192, #105170, #15142, #58660, #167834, #120326, #138475, #184986, #198176, #73857, #13171, #77794, #28358, #59646, #31305, #185993, #121320, #109133, #124296, #47476, #93959, #123294, #183998, #76804, #74834, #29335, #137486, #43504, #92958, #136496, #166856, #122307, #183012, #45481, #89996, #200156, #151678, #107137, #16139, #168807, #44496, #943, #182021, #46470, #152651, #14141, #62618, #139463, #135526, #108130, #170811, #75808, #30311, #32304, #61626, #197197, #169814, #199166, #91954, #153647, #154644, #60633, #52425, #113096, #126287, #171808, #158609, #94955, #2946, #35272, #127267, #129253, #18135, #78785, #142449, #79789, #64625, #114083, #3927, #174787, #5917, #34286, #49454, #125307, #159597, #36253, #157632, #188980, #33296, #96927, #155638, #37258, #17133, #128263, #82751, #67594, #20099, #190948, #143430, #48473, #19121, #81743, #140462, #97906, #1952, #63631, #175784, #144431, #112115, #50456, #80771, #173807, #65607, #187003, #110130, #156639, #141462, #4916, #66599, #189961, #21094, #187984, #111116, #172805, #95946, #51436, #148441, #6910, #163613, #68588, #24104, #119112, #26108, #87751, #23099, #117094, #149436, #86758, #10932, #133261, #177789, #178789, #55423, #25114, #72605, #195967, #56429, #69597, #115101, #101931, #38266, #146422, #40258, #70602, #134279, #161605, #22098, #85758, #84746, #7913, #57439, #147445, #118109, #180793, #39259, #192952, #130244, #102929, #179798, #100915, #132269, #176793, #9936, #98916, #160608, #83748, #71595, #145427, #191940, #194952, #53424, #41267, #99920, #162600, #164614, #131264, #54431, #116101, #8933, #193960, #31067, #198926, #137241, #105908, #60394, #90728, #103930, #88755, #43255, #62375, #167594, #30069, #75565, #184744, #27109, #196951, #135279, #77556, #122066, #91710, #150448, #106898, #11944, #29089, #124045, #169570, #73608, #168571, #14902, #28112, #165610, #104923, #107883, #58419, #89750, #61386, #15898, #151436, #139228, #154404, #703, #42272, #153404, #13899, #76564, #166610, #59399, #152411, #120086, #123058, #12923, #181774, #183758, #74587, #45244, #136255, #138239, #197931, #199923, #46229, #92715, #121073, #182767, #44251, #96688, #109883, #155399, #174552, #189727, #185744, #158376, #63384, #19865, #65368, #66365, #3689, #47232, #1708, #81505, #156389, #144193, #111874, #112861, #143193, #18886, #80532, #4673, #64384 ) ),
 .UNSPECIFIED., .T., .F., .T. ) 
 B_SPLINE_SURFACE_WITH_KNOTS ( ( 4, 3, 4 ),
 ( 3, 2, 2, 2, 2, 2, 2, 2, 2, 2, 2, 2, 2, 2, 2, 2, 2, 2, 2, 2, 2, 2, 2, 2, 2, 2, 2, 2, 2, 2, 2, 2, 2, 2, 2, 2, 2, 2, 2, 2, 2, 2, 2, 2, 2, 2, 2, 2, 2, 2, 2, 2, 2, 2, 2, 2, 2, 2, 2, 2, 2, 2, 2, 2, 2, 2, 2, 2, 2, 2, 2, 2, 2, 2, 2, 2, 2, 2, 2, 2, 2, 2, 2, 2, 2, 2, 2, 2, 2, 2, 2, 2, 2, 2, 2, 2, 2, 2, 2, 2, 2, 2, 2, 2, 2, 2, 2, 2, 2, 2, 2, 2, 2, 2, 2, 2, 2, 2, 2, 2, 2, 2, 2, 2, 2, 2, 2, 2, 2, 2, 2, 2, 2, 2, 2, 2, 2, 2, 2, 2, 2, 2, 2, 2, 2, 2, 2, 2, 2, 2, 2, 2, 2, 2, 2, 2, 2, 2, 2, 2, 2, 2, 2, 2, 2, 2, 2, 2, 2, 2, 2, 2, 2, 2, 2, 2, 2, 2, 2, 2, 2, 2, 2, 2, 2, 2, 2, 2, 2, 2, 2, 2, 2, 2, 2, 2, 2, 2, 2, 2, 2, 2, 2, 2, 2, 2, 2, 2, 2, 2, 2, 2, 2, 2, 2, 2, 2, 2, 2, 2, 2, 2, 2, 2, 2, 2, 2, 2, 3 ),
 ( 0.000000000000000000, 0.5000000000000000000, 1.000000000000000000 ),
 ( 0.000000000000000000, 0.004385964912280701511, 0.008771929824561403022, 0.01315789473684210453, 0.01754385964912280604, 0.02192982456140350755, 0.02631578947368420907, 0.03070175438596491058, 0.03508771929824561209, 0.03947368421052631360, 0.04385964912280701511, 0.04824561403508771662, 0.05263157894736841813, 0.05701754385964911964, 0.06140350877192982115, 0.06578947368421052266, 0.07017543859649122417, 0.07456140350877192569, 0.07894736842105262720, 0.08333333333333332871, 0.08771929824561403022, 0.09210526315789473173, 0.09649122807017543324, 0.1008771929824561348, 0.1052631578947368363, 0.1096491228070175378, 0.1140350877192982393, 0.1184210526315789408, 0.1228070175438596423, 0.1271929824561403577, 0.1315789473684210453, 0.1359649122807017607, 0.1403508771929824483, 0.1447368421052631637, 0.1491228070175438514, 0.1535087719298245668, 0.1578947368421052544, 0.1622807017543859698, 0.1666666666666666574, 0.1710526315789473728, 0.1754385964912280604, 0.1798245614035087758, 0.1842105263157894635, 0.1885964912280701788, 0.1929824561403508665, 0.1973684210526315819, 0.2017543859649122695, 0.2061403508771929849, 0.2105263157894736725, 0.2149122807017543879, 0.2192982456140350755, 0.2236842105263157909, 0.2280701754385964786, 0.2324561403508771940, 0.2368421052631578816, 0.2412280701754385970, 0.2456140350877192846, 0.2500000000000000000, 0.2543859649122807154, 0.2587719298245614308, 0.2631578947368420907, 0.2675438596491228060, 0.2719298245614035214, 0.2763157894736842368, 0.2807017543859648967, 0.2850877192982456121, 0.2894736842105263275, 0.2938596491228070429, 0.2982456140350877027, 0.3026315789473684181, 0.3070175438596491335, 0.3114035087719298489, 0.3157894736842105088, 0.3201754385964912242, 0.3245614035087719396, 0.3289473684210526550, 0.3333333333333333148, 0.3377192982456140302, 0.3421052631578947456, 0.3464912280701754610, 0.3508771929824561209, 0.3552631578947368363, 0.3596491228070175517, 0.3640350877192982670, 0.3684210526315789269, 0.3728070175438596423, 0.3771929824561403577, 0.3815789473684210731, 0.3859649122807017330, 0.3903508771929824483, 0.3947368421052631637, 0.3991228070175438791, 0.4035087719298245390, 0.4078947368421052544, 0.4122807017543859698, 0.4166666666666666852, 0.4210526315789473450, 0.4254385964912280604, 0.4298245614035087758, 0.4342105263157894912, 0.4385964912280701511, 0.4429824561403508665, 0.4473684210526315819, 0.4517543859649122973, 0.4561403508771929571, 0.4605263157894736725, 0.4649122807017543879, 0.4692982456140351033, 0.4736842105263157632, 0.4780701754385964786, 0.4824561403508771940, 0.4868421052631579093, 0.4912280701754385692, 0.4956140350877192846, 0.5000000000000000000, 0.5043859649122807154, 0.5087719298245614308, 0.5131578947368421462, 0.5175438596491228616, 0.5219298245614034659, 0.5263157894736841813, 0.5307017543859648967, 0.5350877192982456121, 0.5394736842105263275, 0.5438596491228070429, 0.5482456140350877583, 0.5526315789473684736, 0.5570175438596490780, 0.5614035087719297934, 0.5657894736842105088, 0.5701754385964912242, 0.5745614035087719396, 0.5789473684210526550, 0.5833333333333333703, 0.5877192982456140857, 0.5921052631578946901, 0.5964912280701754055, 0.6008771929824561209, 0.6052631578947368363, 0.6096491228070175517, 0.6140350877192982670, 0.6184210526315789824, 0.6228070175438596978, 0.6271929824561403022, 0.6315789473684210176, 0.6359649122807017330, 0.6403508771929824483, 0.6447368421052631637, 0.6491228070175438791, 0.6535087719298245945, 0.6578947368421053099, 0.6622807017543859143, 0.6666666666666666297, 0.6710526315789473450, 0.6754385964912280604, 0.6798245614035087758, 0.6842105263157894912, 0.6885964912280702066, 0.6929824561403509220, 0.6973684210526315264, 0.7017543859649122417, 0.7061403508771929571, 0.7105263157894736725, 0.7149122807017543879, 0.7192982456140351033, 0.7236842105263158187, 0.7280701754385965341, 0.7324561403508771384, 0.7368421052631578538, 0.7412280701754385692, 0.7456140350877192846, 0.7500000000000000000, 0.7543859649122807154, 0.7587719298245614308, 0.7631578947368421462, 0.7675438596491228616, 0.7719298245614034659, 0.7763157894736841813, 0.7807017543859648967, 0.7850877192982456121, 0.7894736842105263275, 0.7938596491228070429, 0.7982456140350877583, 0.8026315789473684736, 0.8070175438596490780, 0.8114035087719297934, 0.8157894736842105088, 0.8201754385964912242, 0.8245614035087719396, 0.8289473684210526550, 0.8333333333333333703, 0.8377192982456140857, 0.8421052631578946901, 0.8464912280701754055, 0.8508771929824561209, 0.8552631578947368363, 0.8596491228070175517, 0.8640350877192982670, 0.8684210526315789824, 0.8728070175438596978, 0.8771929824561403022, 0.8815789473684210176, 0.8859649122807017330, 0.8903508771929824483, 0.8947368421052631637, 0.8991228070175438791, 0.9035087719298245945, 0.9078947368421053099, 0.9122807017543859143, 0.9166666666666666297, 0.9210526315789473450, 0.9254385964912280604, 0.9298245614035087758, 0.9342105263157894912, 0.9385964912280702066, 0.9429824561403509220, 0.9473684210526315264, 0.9517543859649122417, 0.9561403508771929571, 0.9605263157894736725, 0.9649122807017543879, 0.9692982456140351033, 0.9736842105263158187, 0.9780701754385965341, 0.9824561403508771384, 0.9868421052631578538, 0.9912280701754385692, 0.9956140350877192846, 1.000000000000000000 ),
 .UNSPECIFIED. ) 
 GEOMETRIC_REPRESENTATION_ITEM ( )  RATIONAL_B_SPLINE_SURFACE ( (
 ( 1.000000000000000000, 0.9659258262890683122, 1.000000000000000000, 0.9659258262890683122, 1.000000000000000000, 0.9659258262890683122, 1.000000000000000000, 0.9659258262890683122, 1.000000000000000000, 0.9659258262890683122, 1.000000000000000000, 0.9659258262890683122, 1.000000000000000000, 0.9659258262890683122, 1.000000000000000000, 0.9659258262890683122, 1.000000000000000000, 0.9659258262890683122, 1.000000000000000000, 0.9659258262890683122, 1.000000000000000000, 0.9659258262890683122, 1.000000000000000000, 0.9659258262890683122, 1.000000000000000000, 0.9659258262890683122, 1.000000000000000000, 0.9659258262890683122, 1.000000000000000000, 0.9659258262890683122, 1.000000000000000000, 0.9659258262890683122, 1.000000000000000000, 0.9659258262890683122, 1.000000000000000000, 0.9659258262890683122, 1.000000000000000000, 0.9659258262890683122, 1.000000000000000000, 0.9659258262890683122, 1.000000000000000000, 0.9659258262890683122, 1.000000000000000000, 0.9659258262890683122, 1.000000000000000000, 0.9659258262890683122, 1.000000000000000000, 0.9659258262890683122, 1.000000000000000000, 0.9659258262890683122, 1.000000000000000000, 0.9659258262890683122, 1.000000000000000000, 0.9659258262890683122, 1.000000000000000000, 0.9659258262890683122, 1.000000000000000000, 0.9659258262890683122, 1.000000000000000000, 0.9659258262890683122, 1.000000000000000000, 0.9659258262890683122, 1.000000000000000000, 0.9659258262890683122, 1.000000000000000000, 0.9659258262890683122, 1.000000000000000000, 0.9659258262890683122, 1.000000000000000000, 0.9659258262890683122, 1.000000000000000000, 0.9659258262890683122, 1.000000000000000000, 0.9659258262890683122, 1.000000000000000000, 0.9659258262890683122, 1.000000000000000000, 0.9659258262890683122, 1.000000000000000000, 0.9659258262890683122, 1.000000000000000000, 0.9659258262890683122, 1.000000000000000000, 0.9659258262890683122, 1.000000000000000000, 0.9659258262890683122, 1.000000000000000000, 0.9659258262890683122, 1.000000000000000000, 0.9659258262890683122, 1.000000000000000000, 0.9659258262890683122, 1.000000000000000000, 0.9659258262890683122, 1.000000000000000000, 0.9659258262890683122, 1.000000000000000000, 0.9659258262890683122, 1.000000000000000000, 0.9659258262890683122, 1.000000000000000000, 0.9659258262890683122, 1.000000000000000000, 0.9659258262890683122, 1.000000000000000000, 0.9659258262890683122, 1.000000000000000000, 0.9659258262890683122, 1.000000000000000000, 0.9659258262890683122, 1.000000000000000000, 0.9659258262890683122, 1.000000000000000000, 0.9659258262890683122, 1.000000000000000000, 0.9659258262890683122, 1.000000000000000000, 0.9659258262890683122, 1.000000000000000000, 0.9659258262890683122, 1.000000000000000000, 0.9659258262890683122, 1.000000000000000000, 0.9659258262890683122, 1.000000000000000000, 0.9659258262890683122, 1.000000000000000000, 0.9659258262890683122, 1.000000000000000000, 0.9659258262890683122, 1.000000000000000000, 0.9659258262890683122, 1.000000000000000000, 0.9659258262890683122, 1.000000000000000000, 0.9659258262890683122, 1.000000000000000000, 0.9659258262890683122, 1.000000000000000000, 0.9659258262890683122, 1.000000000000000000, 0.9659258262890683122, 1.000000000000000000, 0.9659258262890683122, 1.000000000000000000, 0.9659258262890683122, 1.000000000000000000, 0.9659258262890683122, 1.000000000000000000, 0.9659258262890683122, 1.000000000000000000, 0.9659258262890683122, 1.000000000000000000, 0.9659258262890683122, 1.000000000000000000, 0.9659258262890683122, 1.000000000000000000, 0.9659258262890683122, 1.000000000000000000, 0.9659258262890683122, 1.000000000000000000, 0.9659258262890683122, 1.000000000000000000, 0.9659258262890683122, 1.000000000000000000, 0.9659258262890683122, 1.000000000000000000, 0.9659258262890683122, 1.000000000000000000, 0.9659258262890683122, 1.000000000000000000, 0.9659258262890683122, 1.000000000000000000, 0.9659258262890683122, 1.000000000000000000, 0.9659258262890683122, 1.000000000000000000, 0.9659258262890683122, 1.000000000000000000, 0.9659258262890683122, 1.000000000000000000, 0.9659258262890683122, 1.000000000000000000, 0.9659258262890683122, 1.000000000000000000, 0.9659258262890683122, 1.000000000000000000, 0.9659258262890683122, 1.000000000000000000, 0.9659258262890683122, 1.000000000000000000, 0.9659258262890683122, 1.000000000000000000, 0.9659258262890683122, 1.000000000000000000, 0.9659258262890683122, 1.000000000000000000, 0.9659258262890683122, 1.000000000000000000, 0.9659258262890683122, 1.000000000000000000, 0.9659258262890683122, 1.000000000000000000, 0.9659258262890683122, 1.000000000000000000, 0.9659258262890683122, 1.000000000000000000, 0.9659258262890683122, 1.000000000000000000, 0.9659258262890683122, 1.000000000000000000, 0.9659258262890683122, 1.000000000000000000, 0.9659258262890683122, 1.000000000000000000, 0.9659258262890683122, 1.000000000000000000, 0.9659258262890683122, 1.000000000000000000, 0.9659258262890683122, 1.000000000000000000, 0.9659258262890683122, 1.000000000000000000, 0.9659258262890683122, 1.000000000000000000, 0.9659258262890683122, 1.000000000000000000, 0.9659258262890683122, 1.000000000000000000, 0.9659258262890683122, 1.000000000000000000, 0.9659258262890683122, 1.000000000000000000, 0.9659258262890683122, 1.000000000000000000, 0.9659258262890683122, 1.000000000000000000, 0.9659258262890683122, 1.000000000000000000, 0.9659258262890683122, 1.000000000000000000, 0.9659258262890683122, 1.000000000000000000, 0.9659258262890683122, 1.000000000000000000, 0.9659258262890683122, 1.000000000000000000, 0.9659258262890683122, 1.000000000000000000, 0.9659258262890683122, 1.000000000000000000, 0.9659258262890683122, 1.000000000000000000, 0.9659258262890683122, 1.000000000000000000, 0.9659258262890683122, 1.000000000000000000, 0.9659258262890683122, 1.000000000000000000, 0.9659258262890683122, 1.000000000000000000, 0.9659258262890683122, 1.000000000000000000, 0.9659258262890683122, 1.000000000000000000, 0.9659258262890683122, 1.000000000000000000, 0.9659258262890683122, 1.000000000000000000, 0.9659258262890683122, 1.000000000000000000, 0.9659258262890683122, 1.000000000000000000, 0.9659258262890683122, 1.000000000000000000, 0.9659258262890683122, 1.000000000000000000, 0.9659258262890683122, 1.000000000000000000, 0.9659258262890683122, 1.000000000000000000, 0.9659258262890683122, 1.000000000000000000, 0.9659258262890683122, 1.000000000000000000, 0.9659258262890683122, 1.000000000000000000, 0.9659258262890683122, 1.000000000000000000, 0.9659258262890683122, 1.000000000000000000, 0.9659258262890683122, 1.000000000000000000, 0.9659258262890683122, 1.000000000000000000, 0.9659258262890683122, 1.000000000000000000, 0.9659258262890683122, 1.000000000000000000, 0.9659258262890683122, 1.000000000000000000, 0.9659258262890683122, 1.000000000000000000, 0.9659258262890683122, 1.000000000000000000, 0.9659258262890683122, 1.000000000000000000, 0.9659258262890683122, 1.000000000000000000, 0.9659258262890683122, 1.000000000000000000, 0.9659258262890683122, 1.000000000000000000, 0.9659258262890683122, 1.000000000000000000, 0.9659258262890683122, 1.000000000000000000, 0.9659258262890683122, 1.000000000000000000, 0.9659258262890683122, 1.000000000000000000, 0.9659258262890683122, 1.000000000000000000, 0.9659258262890683122, 1.000000000000000000, 0.9659258262890683122, 1.000000000000000000, 0.9659258262890683122, 1.000000000000000000, 0.9659258262890683122, 1.000000000000000000, 0.9659258262890683122, 1.000000000000000000, 0.9659258262890683122, 1.000000000000000000, 0.9659258262890683122, 1.000000000000000000, 0.9659258262890683122, 1.000000000000000000, 0.9659258262890683122, 1.000000000000000000, 0.9659258262890683122, 1.000000000000000000, 0.9659258262890683122, 1.000000000000000000, 0.9659258262890683122, 1.000000000000000000, 0.9659258262890683122, 1.000000000000000000, 0.9659258262890683122, 1.000000000000000000, 0.9659258262890683122, 1.000000000000000000, 0.9659258262890683122, 1.000000000000000000, 0.9659258262890683122, 1.000000000000000000, 0.9659258262890683122, 1.000000000000000000, 0.9659258262890683122, 1.000000000000000000, 0.9659258262890683122, 1.000000000000000000, 0.9659258262890683122, 1.000000000000000000, 0.9659258262890683122, 1.000000000000000000, 0.9659258262890683122, 1.000000000000000000, 0.9659258262890683122, 1.000000000000000000, 0.9659258262890683122, 1.000000000000000000, 0.9659258262890683122, 1.000000000000000000, 0.9659258262890683122, 1.000000000000000000, 0.9659258262890683122, 1.000000000000000000, 0.9659258262890683122, 1.000000000000000000, 0.9659258262890683122, 1.000000000000000000, 0.9659258262890683122, 1.000000000000000000, 0.9659258262890683122, 1.000000000000000000, 0.9659258262890683122, 1.000000000000000000, 0.9659258262890683122, 1.000000000000000000, 0.9659258262890683122, 1.000000000000000000, 0.9659258262890683122, 1.000000000000000000, 0.9659258262890683122, 1.000000000000000000, 0.9659258262890683122, 1.000000000000000000, 0.9659258262890683122, 1.000000000000000000, 0.9659258262890683122, 1.000000000000000000, 0.9659258262890683122, 1.000000000000000000, 0.9659258262890683122, 1.000000000000000000, 0.9659258262890683122, 1.000000000000000000, 0.9659258262890683122, 1.000000000000000000, 0.9659258262890683122, 1.000000000000000000, 0.9659258262890683122, 1.000000000000000000, 0.9659258262890683122, 1.000000000000000000, 0.9659258262890683122, 1.000000000000000000, 0.9659258262890683122, 1.000000000000000000, 0.9659258262890683122, 1.000000000000000000, 0.9659258262890683122, 1.000000000000000000, 0.9659258262890683122, 1.000000000000000000, 0.9659258262890683122, 1.000000000000000000, 0.9659258262890683122, 1.000000000000000000, 0.9659258262890683122, 1.000000000000000000, 0.9659258262890683122, 1.000000000000000000, 0.9659258262890683122, 1.000000000000000000, 0.9659258262890683122, 1.000000000000000000, 0.9659258262890683122, 1.000000000000000000, 0.9659258262890683122, 1.000000000000000000, 0.9659258262890683122, 1.000000000000000000, 0.9659258262890683122, 1.000000000000000000, 0.9659258262890683122, 1.000000000000000000, 0.9659258262890683122, 1.000000000000000000, 0.9659258262890683122, 1.000000000000000000, 0.9659258262890683122, 1.000000000000000000, 0.9659258262890683122, 1.000000000000000000),
 ( 0.3333333333333333703, 0.3219752754296894559, 0.3333333333333333703, 0.3219752754296894559, 0.3333333333333333703, 0.3219752754296894559, 0.3333333333333333703, 0.3219752754296894559, 0.3333333333333333703, 0.3219752754296894559, 0.3333333333333333703, 0.3219752754296894559, 0.3333333333333333703, 0.3219752754296894559, 0.3333333333333333703, 0.3219752754296894559, 0.3333333333333333703, 0.3219752754296894559, 0.3333333333333333703, 0.3219752754296894559, 0.3333333333333333703, 0.3219752754296894559, 0.3333333333333333703, 0.3219752754296894559, 0.3333333333333333703, 0.3219752754296894559, 0.3333333333333333703, 0.3219752754296894559, 0.3333333333333333703, 0.3219752754296894559, 0.3333333333333333703, 0.3219752754296894559, 0.3333333333333333703, 0.3219752754296894559, 0.3333333333333333703, 0.3219752754296894559, 0.3333333333333333703, 0.3219752754296894559, 0.3333333333333333703, 0.3219752754296894559, 0.3333333333333333703, 0.3219752754296894559, 0.3333333333333333703, 0.3219752754296894559, 0.3333333333333333703, 0.3219752754296894559, 0.3333333333333333703, 0.3219752754296894559, 0.3333333333333333703, 0.3219752754296894559, 0.3333333333333333703, 0.3219752754296894559, 0.3333333333333333703, 0.3219752754296894559, 0.3333333333333333703, 0.3219752754296894559, 0.3333333333333333703, 0.3219752754296894559, 0.3333333333333333703, 0.3219752754296894559, 0.3333333333333333703, 0.3219752754296894559, 0.3333333333333333703, 0.3219752754296894559, 0.3333333333333333703, 0.3219752754296894559, 0.3333333333333333703, 0.3219752754296894559, 0.3333333333333333703, 0.3219752754296894559, 0.3333333333333333703, 0.3219752754296894559, 0.3333333333333333703, 0.3219752754296894559, 0.3333333333333333703, 0.3219752754296894559, 0.3333333333333333703, 0.3219752754296894559, 0.3333333333333333703, 0.3219752754296894559, 0.3333333333333333703, 0.3219752754296894559, 0.3333333333333333703, 0.3219752754296894559, 0.3333333333333333703, 0.3219752754296894559, 0.3333333333333333703, 0.3219752754296894559, 0.3333333333333333703, 0.3219752754296894559, 0.3333333333333333703, 0.3219752754296894559, 0.3333333333333333703, 0.3219752754296894559, 0.3333333333333333703, 0.3219752754296894559, 0.3333333333333333703, 0.3219752754296894559, 0.3333333333333333703, 0.3219752754296894559, 0.3333333333333333703, 0.3219752754296894559, 0.3333333333333333703, 0.3219752754296894559, 0.3333333333333333703, 0.3219752754296894559, 0.3333333333333333703, 0.3219752754296894559, 0.3333333333333333703, 0.3219752754296894559, 0.3333333333333333703, 0.3219752754296894559, 0.3333333333333333703, 0.3219752754296894559, 0.3333333333333333703, 0.3219752754296894559, 0.3333333333333333703, 0.3219752754296894559, 0.3333333333333333703, 0.3219752754296894559, 0.3333333333333333703, 0.3219752754296894559, 0.3333333333333333703, 0.3219752754296894559, 0.3333333333333333703, 0.3219752754296894559, 0.3333333333333333703, 0.3219752754296894559, 0.3333333333333333703, 0.3219752754296894559, 0.3333333333333333703, 0.3219752754296894559, 0.3333333333333333703, 0.3219752754296894559, 0.3333333333333333703, 0.3219752754296894559, 0.3333333333333333703, 0.3219752754296894559, 0.3333333333333333703, 0.3219752754296894559, 0.3333333333333333703, 0.3219752754296894559, 0.3333333333333333703, 0.3219752754296894559, 0.3333333333333333703, 0.3219752754296894559, 0.3333333333333333703, 0.3219752754296894559, 0.3333333333333333703, 0.3219752754296894559, 0.3333333333333333703, 0.3219752754296894559, 0.3333333333333333703, 0.3219752754296894559, 0.3333333333333333703, 0.3219752754296894559, 0.3333333333333333703, 0.3219752754296894559, 0.3333333333333333703, 0.3219752754296894559, 0.3333333333333333703, 0.3219752754296894559, 0.3333333333333333703, 0.3219752754296894559, 0.3333333333333333703, 0.3219752754296894559, 0.3333333333333333703, 0.3219752754296894559, 0.3333333333333333703, 0.3219752754296894559, 0.3333333333333333703, 0.3219752754296894559, 0.3333333333333333703, 0.3219752754296894559, 0.3333333333333333703, 0.3219752754296894559, 0.3333333333333333703, 0.3219752754296894559, 0.3333333333333333703, 0.3219752754296894559, 0.3333333333333333703, 0.3219752754296894559, 0.3333333333333333703, 0.3219752754296894559, 0.3333333333333333703, 0.3219752754296894559, 0.3333333333333333703, 0.3219752754296894559, 0.3333333333333333703, 0.3219752754296894559, 0.3333333333333333703, 0.3219752754296894559, 0.3333333333333333703, 0.3219752754296894559, 0.3333333333333333703, 0.3219752754296894559, 0.3333333333333333703, 0.3219752754296894559, 0.3333333333333333703, 0.3219752754296894559, 0.3333333333333333703, 0.3219752754296894559, 0.3333333333333333703, 0.3219752754296894559, 0.3333333333333333703, 0.3219752754296894559, 0.3333333333333333703, 0.3219752754296894559, 0.3333333333333333703, 0.3219752754296894559, 0.3333333333333333703, 0.3219752754296894559, 0.3333333333333333703, 0.3219752754296894559, 0.3333333333333333703, 0.3219752754296894559, 0.3333333333333333703, 0.3219752754296894559, 0.3333333333333333703, 0.3219752754296894559, 0.3333333333333333703, 0.3219752754296894559, 0.3333333333333333703, 0.3219752754296894559, 0.3333333333333333703, 0.3219752754296894559, 0.3333333333333333703, 0.3219752754296894559, 0.3333333333333333703, 0.3219752754296894559, 0.3333333333333333703, 0.3219752754296894559, 0.3333333333333333703, 0.3219752754296894559, 0.3333333333333333703, 0.3219752754296894559, 0.3333333333333333703, 0.3219752754296894559, 0.3333333333333333703, 0.3219752754296894559, 0.3333333333333333703, 0.3219752754296894559, 0.3333333333333333703, 0.3219752754296894559, 0.3333333333333333703, 0.3219752754296894559, 0.3333333333333333703, 0.3219752754296894559, 0.3333333333333333703, 0.3219752754296894559, 0.3333333333333333703, 0.3219752754296894559, 0.3333333333333333703, 0.3219752754296894559, 0.3333333333333333703, 0.3219752754296894559, 0.3333333333333333703, 0.3219752754296894559, 0.3333333333333333703, 0.3219752754296894559, 0.3333333333333333703, 0.3219752754296894559, 0.3333333333333333703, 0.3219752754296894559, 0.3333333333333333703, 0.3219752754296894559, 0.3333333333333333703, 0.3219752754296894559, 0.3333333333333333703, 0.3219752754296894559, 0.3333333333333333703, 0.3219752754296894559, 0.3333333333333333703, 0.3219752754296894559, 0.3333333333333333703, 0.3219752754296894559, 0.3333333333333333703, 0.3219752754296894559, 0.3333333333333333703, 0.3219752754296894559, 0.3333333333333333703, 0.3219752754296894559, 0.3333333333333333703, 0.3219752754296894559, 0.3333333333333333703, 0.3219752754296894559, 0.3333333333333333703, 0.3219752754296894559, 0.3333333333333333703, 0.3219752754296894559, 0.3333333333333333703, 0.3219752754296894559, 0.3333333333333333703, 0.3219752754296894559, 0.3333333333333333703, 0.3219752754296894559, 0.3333333333333333703, 0.3219752754296894559, 0.3333333333333333703, 0.3219752754296894559, 0.3333333333333333703, 0.3219752754296894559, 0.3333333333333333703, 0.3219752754296894559, 0.3333333333333333703, 0.3219752754296894559, 0.3333333333333333703, 0.3219752754296894559, 0.3333333333333333703, 0.3219752754296894559, 0.3333333333333333703, 0.3219752754296894559, 0.3333333333333333703, 0.3219752754296894559, 0.3333333333333333703, 0.3219752754296894559, 0.3333333333333333703, 0.3219752754296894559, 0.3333333333333333703, 0.3219752754296894559, 0.3333333333333333703, 0.3219752754296894559, 0.3333333333333333703, 0.3219752754296894559, 0.3333333333333333703, 0.3219752754296894559, 0.3333333333333333703, 0.3219752754296894559, 0.3333333333333333703, 0.3219752754296894559, 0.3333333333333333703, 0.3219752754296894559, 0.3333333333333333703, 0.3219752754296894559, 0.3333333333333333703, 0.3219752754296894559, 0.3333333333333333703, 0.3219752754296894559, 0.3333333333333333703, 0.3219752754296894559, 0.3333333333333333703, 0.3219752754296894559, 0.3333333333333333703, 0.3219752754296894559, 0.3333333333333333703, 0.3219752754296894559, 0.3333333333333333703, 0.3219752754296894559, 0.3333333333333333703, 0.3219752754296894559, 0.3333333333333333703, 0.3219752754296894559, 0.3333333333333333703, 0.3219752754296894559, 0.3333333333333333703, 0.3219752754296894559, 0.3333333333333333703, 0.3219752754296894559, 0.3333333333333333703, 0.3219752754296894559, 0.3333333333333333703, 0.3219752754296894559, 0.3333333333333333703, 0.3219752754296894559, 0.3333333333333333703, 0.3219752754296894559, 0.3333333333333333703, 0.3219752754296894559, 0.3333333333333333703, 0.3219752754296894559, 0.3333333333333333703, 0.3219752754296894559, 0.3333333333333333703, 0.3219752754296894559, 0.3333333333333333703, 0.3219752754296894559, 0.3333333333333333703, 0.3219752754296894559, 0.3333333333333333703, 0.3219752754296894559, 0.3333333333333333703, 0.3219752754296894559, 0.3333333333333333703, 0.3219752754296894559, 0.3333333333333333703, 0.3219752754296894559, 0.3333333333333333703, 0.3219752754296894559, 0.3333333333333333703, 0.3219752754296894559, 0.3333333333333333703, 0.3219752754296894559, 0.3333333333333333703, 0.3219752754296894559, 0.3333333333333333703, 0.3219752754296894559, 0.3333333333333333703, 0.3219752754296894559, 0.3333333333333333703, 0.3219752754296894559, 0.3333333333333333703, 0.3219752754296894559, 0.3333333333333333703, 0.3219752754296894559, 0.3333333333333333703, 0.3219752754296894559, 0.3333333333333333703, 0.3219752754296894559, 0.3333333333333333703, 0.3219752754296894559, 0.3333333333333333703, 0.3219752754296894559, 0.3333333333333333703, 0.3219752754296894559, 0.3333333333333333703, 0.3219752754296894559, 0.3333333333333333703, 0.3219752754296894559, 0.3333333333333333703, 0.3219752754296894559, 0.3333333333333333703, 0.3219752754296894559, 0.3333333333333333703, 0.3219752754296894559, 0.3333333333333333703, 0.3219752754296894559, 0.3333333333333333703, 0.3219752754296894559, 0.3333333333333333703, 0.3219752754296894559, 0.3333333333333333703, 0.3219752754296894559, 0.3333333333333333703, 0.3219752754296894559, 0.3333333333333333703, 0.3219752754296894559, 0.3333333333333333703, 0.3219752754296894559, 0.3333333333333333703, 0.3219752754296894559, 0.3333333333333333703, 0.3219752754296894559, 0.3333333333333333703, 0.3219752754296894559, 0.3333333333333333703, 0.3219752754296894559, 0.3333333333333333703, 0.3219752754296894559, 0.3333333333333333703, 0.3219752754296894559, 0.3333333333333333703, 0.3219752754296894559, 0.3333333333333333703, 0.3219752754296894559, 0.3333333333333333703, 0.3219752754296894559, 0.3333333333333333703),
 ( 0.3333333333333333703, 0.3219752754296894559, 0.3333333333333333703, 0.3219752754296894559, 0.3333333333333333703, 0.3219752754296894559, 0.3333333333333333703, 0.3219752754296894559, 0.3333333333333333703, 0.3219752754296894559, 0.3333333333333333703, 0.3219752754296894559, 0.3333333333333333703, 0.3219752754296894559, 0.3333333333333333703, 0.3219752754296894559, 0.3333333333333333703, 0.3219752754296894559, 0.3333333333333333703, 0.3219752754296894559, 0.3333333333333333703, 0.3219752754296894559, 0.3333333333333333703, 0.3219752754296894559, 0.3333333333333333703, 0.3219752754296894559, 0.3333333333333333703, 0.3219752754296894559, 0.3333333333333333703, 0.3219752754296894559, 0.3333333333333333703, 0.3219752754296894559, 0.3333333333333333703, 0.3219752754296894559, 0.3333333333333333703, 0.3219752754296894559, 0.3333333333333333703, 0.3219752754296894559, 0.3333333333333333703, 0.3219752754296894559, 0.3333333333333333703, 0.3219752754296894559, 0.3333333333333333703, 0.3219752754296894559, 0.3333333333333333703, 0.3219752754296894559, 0.3333333333333333703, 0.3219752754296894559, 0.3333333333333333703, 0.3219752754296894559, 0.3333333333333333703, 0.3219752754296894559, 0.3333333333333333703, 0.3219752754296894559, 0.3333333333333333703, 0.3219752754296894559, 0.3333333333333333703, 0.3219752754296894559, 0.3333333333333333703, 0.3219752754296894559, 0.3333333333333333703, 0.3219752754296894559, 0.3333333333333333703, 0.3219752754296894559, 0.3333333333333333703, 0.3219752754296894559, 0.3333333333333333703, 0.3219752754296894559, 0.3333333333333333703, 0.3219752754296894559, 0.3333333333333333703, 0.3219752754296894559, 0.3333333333333333703, 0.3219752754296894559, 0.3333333333333333703, 0.3219752754296894559, 0.3333333333333333703, 0.3219752754296894559, 0.3333333333333333703, 0.3219752754296894559, 0.3333333333333333703, 0.3219752754296894559, 0.3333333333333333703, 0.3219752754296894559, 0.3333333333333333703, 0.3219752754296894559, 0.3333333333333333703, 0.3219752754296894559, 0.3333333333333333703, 0.3219752754296894559, 0.3333333333333333703, 0.3219752754296894559, 0.3333333333333333703, 0.3219752754296894559, 0.3333333333333333703, 0.3219752754296894559, 0.3333333333333333703, 0.3219752754296894559, 0.3333333333333333703, 0.3219752754296894559, 0.3333333333333333703, 0.3219752754296894559, 0.3333333333333333703, 0.3219752754296894559, 0.3333333333333333703, 0.3219752754296894559, 0.3333333333333333703, 0.3219752754296894559, 0.3333333333333333703, 0.3219752754296894559, 0.3333333333333333703, 0.3219752754296894559, 0.3333333333333333703, 0.3219752754296894559, 0.3333333333333333703, 0.3219752754296894559, 0.3333333333333333703, 0.3219752754296894559, 0.3333333333333333703, 0.3219752754296894559, 0.3333333333333333703, 0.3219752754296894559, 0.3333333333333333703, 0.3219752754296894559, 0.3333333333333333703, 0.3219752754296894559, 0.3333333333333333703, 0.3219752754296894559, 0.3333333333333333703, 0.3219752754296894559, 0.3333333333333333703, 0.3219752754296894559, 0.3333333333333333703, 0.3219752754296894559, 0.3333333333333333703, 0.3219752754296894559, 0.3333333333333333703, 0.3219752754296894559, 0.3333333333333333703, 0.3219752754296894559, 0.3333333333333333703, 0.3219752754296894559, 0.3333333333333333703, 0.3219752754296894559, 0.3333333333333333703, 0.3219752754296894559, 0.3333333333333333703, 0.3219752754296894559, 0.3333333333333333703, 0.3219752754296894559, 0.3333333333333333703, 0.3219752754296894559, 0.3333333333333333703, 0.3219752754296894559, 0.3333333333333333703, 0.3219752754296894559, 0.3333333333333333703, 0.3219752754296894559, 0.3333333333333333703, 0.3219752754296894559, 0.3333333333333333703, 0.3219752754296894559, 0.3333333333333333703, 0.3219752754296894559, 0.3333333333333333703, 0.3219752754296894559, 0.3333333333333333703, 0.3219752754296894559, 0.3333333333333333703, 0.3219752754296894559, 0.3333333333333333703, 0.3219752754296894559, 0.3333333333333333703, 0.3219752754296894559, 0.3333333333333333703, 0.3219752754296894559, 0.3333333333333333703, 0.3219752754296894559, 0.3333333333333333703, 0.3219752754296894559, 0.3333333333333333703, 0.3219752754296894559, 0.3333333333333333703, 0.3219752754296894559, 0.3333333333333333703, 0.3219752754296894559, 0.3333333333333333703, 0.3219752754296894559, 0.3333333333333333703, 0.3219752754296894559, 0.3333333333333333703, 0.3219752754296894559, 0.3333333333333333703, 0.3219752754296894559, 0.3333333333333333703, 0.3219752754296894559, 0.3333333333333333703, 0.3219752754296894559, 0.3333333333333333703, 0.3219752754296894559, 0.3333333333333333703, 0.3219752754296894559, 0.3333333333333333703, 0.3219752754296894559, 0.3333333333333333703, 0.3219752754296894559, 0.3333333333333333703, 0.3219752754296894559, 0.3333333333333333703, 0.3219752754296894559, 0.3333333333333333703, 0.3219752754296894559, 0.3333333333333333703, 0.3219752754296894559, 0.3333333333333333703, 0.3219752754296894559, 0.3333333333333333703, 0.3219752754296894559, 0.3333333333333333703, 0.3219752754296894559, 0.3333333333333333703, 0.3219752754296894559, 0.3333333333333333703, 0.3219752754296894559, 0.3333333333333333703, 0.3219752754296894559, 0.3333333333333333703, 0.3219752754296894559, 0.3333333333333333703, 0.3219752754296894559, 0.3333333333333333703, 0.3219752754296894559, 0.3333333333333333703, 0.3219752754296894559, 0.3333333333333333703, 0.3219752754296894559, 0.3333333333333333703, 0.3219752754296894559, 0.3333333333333333703, 0.3219752754296894559, 0.3333333333333333703, 0.3219752754296894559, 0.3333333333333333703, 0.3219752754296894559, 0.3333333333333333703, 0.3219752754296894559, 0.3333333333333333703, 0.3219752754296894559, 0.3333333333333333703, 0.3219752754296894559, 0.3333333333333333703, 0.3219752754296894559, 0.3333333333333333703, 0.3219752754296894559, 0.3333333333333333703, 0.3219752754296894559, 0.3333333333333333703, 0.3219752754296894559, 0.3333333333333333703, 0.3219752754296894559, 0.3333333333333333703, 0.3219752754296894559, 0.3333333333333333703, 0.3219752754296894559, 0.3333333333333333703, 0.3219752754296894559, 0.3333333333333333703, 0.3219752754296894559, 0.3333333333333333703, 0.3219752754296894559, 0.3333333333333333703, 0.3219752754296894559, 0.3333333333333333703, 0.3219752754296894559, 0.3333333333333333703, 0.3219752754296894559, 0.3333333333333333703, 0.3219752754296894559, 0.3333333333333333703, 0.3219752754296894559, 0.3333333333333333703, 0.3219752754296894559, 0.3333333333333333703, 0.3219752754296894559, 0.3333333333333333703, 0.3219752754296894559, 0.3333333333333333703, 0.3219752754296894559, 0.3333333333333333703, 0.3219752754296894559, 0.3333333333333333703, 0.3219752754296894559, 0.3333333333333333703, 0.3219752754296894559, 0.3333333333333333703, 0.3219752754296894559, 0.3333333333333333703, 0.3219752754296894559, 0.3333333333333333703, 0.3219752754296894559, 0.3333333333333333703, 0.3219752754296894559, 0.3333333333333333703, 0.3219752754296894559, 0.3333333333333333703, 0.3219752754296894559, 0.3333333333333333703, 0.3219752754296894559, 0.3333333333333333703, 0.3219752754296894559, 0.3333333333333333703, 0.3219752754296894559, 0.3333333333333333703, 0.3219752754296894559, 0.3333333333333333703, 0.3219752754296894559, 0.3333333333333333703, 0.3219752754296894559, 0.3333333333333333703, 0.3219752754296894559, 0.3333333333333333703, 0.3219752754296894559, 0.3333333333333333703, 0.3219752754296894559, 0.3333333333333333703, 0.3219752754296894559, 0.3333333333333333703, 0.3219752754296894559, 0.3333333333333333703, 0.3219752754296894559, 0.3333333333333333703, 0.3219752754296894559, 0.3333333333333333703, 0.3219752754296894559, 0.3333333333333333703, 0.3219752754296894559, 0.3333333333333333703, 0.3219752754296894559, 0.3333333333333333703, 0.3219752754296894559, 0.3333333333333333703, 0.3219752754296894559, 0.3333333333333333703, 0.3219752754296894559, 0.3333333333333333703, 0.3219752754296894559, 0.3333333333333333703, 0.3219752754296894559, 0.3333333333333333703, 0.3219752754296894559, 0.3333333333333333703, 0.3219752754296894559, 0.3333333333333333703, 0.3219752754296894559, 0.3333333333333333703, 0.3219752754296894559, 0.3333333333333333703, 0.3219752754296894559, 0.3333333333333333703, 0.3219752754296894559, 0.3333333333333333703, 0.3219752754296894559, 0.3333333333333333703, 0.3219752754296894559, 0.3333333333333333703, 0.3219752754296894559, 0.3333333333333333703, 0.3219752754296894559, 0.3333333333333333703, 0.3219752754296894559, 0.3333333333333333703, 0.3219752754296894559, 0.3333333333333333703, 0.3219752754296894559, 0.3333333333333333703, 0.3219752754296894559, 0.3333333333333333703, 0.3219752754296894559, 0.3333333333333333703, 0.3219752754296894559, 0.3333333333333333703, 0.3219752754296894559, 0.3333333333333333703, 0.3219752754296894559, 0.3333333333333333703, 0.3219752754296894559, 0.3333333333333333703, 0.3219752754296894559, 0.3333333333333333703, 0.3219752754296894559, 0.3333333333333333703, 0.3219752754296894559, 0.3333333333333333703, 0.3219752754296894559, 0.3333333333333333703, 0.3219752754296894559, 0.3333333333333333703, 0.3219752754296894559, 0.3333333333333333703, 0.3219752754296894559, 0.3333333333333333703, 0.3219752754296894559, 0.3333333333333333703, 0.3219752754296894559, 0.3333333333333333703, 0.3219752754296894559, 0.3333333333333333703, 0.3219752754296894559, 0.3333333333333333703, 0.3219752754296894559, 0.3333333333333333703, 0.3219752754296894559, 0.3333333333333333703, 0.3219752754296894559, 0.3333333333333333703, 0.3219752754296894559, 0.3333333333333333703, 0.3219752754296894559, 0.3333333333333333703, 0.3219752754296894559, 0.3333333333333333703, 0.3219752754296894559, 0.3333333333333333703, 0.3219752754296894559, 0.3333333333333333703, 0.3219752754296894559, 0.3333333333333333703, 0.3219752754296894559, 0.3333333333333333703, 0.3219752754296894559, 0.3333333333333333703, 0.3219752754296894559, 0.3333333333333333703, 0.3219752754296894559, 0.3333333333333333703, 0.3219752754296894559, 0.3333333333333333703, 0.3219752754296894559, 0.3333333333333333703, 0.3219752754296894559, 0.3333333333333333703, 0.3219752754296894559, 0.3333333333333333703, 0.3219752754296894559, 0.3333333333333333703, 0.3219752754296894559, 0.3333333333333333703, 0.3219752754296894559, 0.3333333333333333703, 0.3219752754296894559, 0.3333333333333333703, 0.3219752754296894559, 0.3333333333333333703, 0.3219752754296894559, 0.3333333333333333703, 0.3219752754296894559, 0.3333333333333333703),
 ( 1.000000000000000000, 0.9659258262890683122, 1.000000000000000000, 0.9659258262890683122, 1.000000000000000000, 0.9659258262890683122, 1.000000000000000000, 0.9659258262890683122, 1.000000000000000000, 0.9659258262890683122, 1.000000000000000000, 0.9659258262890683122, 1.000000000000000000, 0.9659258262890683122, 1.000000000000000000, 0.9659258262890683122, 1.000000000000000000, 0.9659258262890683122, 1.000000000000000000, 0.9659258262890683122, 1.000000000000000000, 0.9659258262890683122, 1.000000000000000000, 0.9659258262890683122, 1.000000000000000000, 0.9659258262890683122, 1.000000000000000000, 0.9659258262890683122, 1.000000000000000000, 0.9659258262890683122, 1.000000000000000000, 0.9659258262890683122, 1.000000000000000000, 0.9659258262890683122, 1.000000000000000000, 0.9659258262890683122, 1.000000000000000000, 0.9659258262890683122, 1.000000000000000000, 0.9659258262890683122, 1.000000000000000000, 0.9659258262890683122, 1.000000000000000000, 0.9659258262890683122, 1.000000000000000000, 0.9659258262890683122, 1.000000000000000000, 0.9659258262890683122, 1.000000000000000000, 0.9659258262890683122, 1.000000000000000000, 0.9659258262890683122, 1.000000000000000000, 0.9659258262890683122, 1.000000000000000000, 0.9659258262890683122, 1.000000000000000000, 0.9659258262890683122, 1.000000000000000000, 0.9659258262890683122, 1.000000000000000000, 0.9659258262890683122, 1.000000000000000000, 0.9659258262890683122, 1.000000000000000000, 0.9659258262890683122, 1.000000000000000000, 0.9659258262890683122, 1.000000000000000000, 0.9659258262890683122, 1.000000000000000000, 0.9659258262890683122, 1.000000000000000000, 0.9659258262890683122, 1.000000000000000000, 0.9659258262890683122, 1.000000000000000000, 0.9659258262890683122, 1.000000000000000000, 0.9659258262890683122, 1.000000000000000000, 0.9659258262890683122, 1.000000000000000000, 0.9659258262890683122, 1.000000000000000000, 0.9659258262890683122, 1.000000000000000000, 0.9659258262890683122, 1.000000000000000000, 0.9659258262890683122, 1.000000000000000000, 0.9659258262890683122, 1.000000000000000000, 0.9659258262890683122, 1.000000000000000000, 0.9659258262890683122, 1.000000000000000000, 0.9659258262890683122, 1.000000000000000000, 0.9659258262890683122, 1.000000000000000000, 0.9659258262890683122, 1.000000000000000000, 0.9659258262890683122, 1.000000000000000000, 0.9659258262890683122, 1.000000000000000000, 0.9659258262890683122, 1.000000000000000000, 0.9659258262890683122, 1.000000000000000000, 0.9659258262890683122, 1.000000000000000000, 0.9659258262890683122, 1.000000000000000000, 0.9659258262890683122, 1.000000000000000000, 0.9659258262890683122, 1.000000000000000000, 0.9659258262890683122, 1.000000000000000000, 0.9659258262890683122, 1.000000000000000000, 0.9659258262890683122, 1.000000000000000000, 0.9659258262890683122, 1.000000000000000000, 0.9659258262890683122, 1.000000000000000000, 0.9659258262890683122, 1.000000000000000000, 0.9659258262890683122, 1.000000000000000000, 0.9659258262890683122, 1.000000000000000000, 0.9659258262890683122, 1.000000000000000000, 0.9659258262890683122, 1.000000000000000000, 0.9659258262890683122, 1.000000000000000000, 0.9659258262890683122, 1.000000000000000000, 0.9659258262890683122, 1.000000000000000000, 0.9659258262890683122, 1.000000000000000000, 0.9659258262890683122, 1.000000000000000000, 0.9659258262890683122, 1.000000000000000000, 0.9659258262890683122, 1.000000000000000000, 0.9659258262890683122, 1.000000000000000000, 0.9659258262890683122, 1.000000000000000000, 0.9659258262890683122, 1.000000000000000000, 0.9659258262890683122, 1.000000000000000000, 0.9659258262890683122, 1.000000000000000000, 0.9659258262890683122, 1.000000000000000000, 0.9659258262890683122, 1.000000000000000000, 0.9659258262890683122, 1.000000000000000000, 0.9659258262890683122, 1.000000000000000000, 0.9659258262890683122, 1.000000000000000000, 0.9659258262890683122, 1.000000000000000000, 0.9659258262890683122, 1.000000000000000000, 0.9659258262890683122, 1.000000000000000000, 0.9659258262890683122, 1.000000000000000000, 0.9659258262890683122, 1.000000000000000000, 0.9659258262890683122, 1.000000000000000000, 0.9659258262890683122, 1.000000000000000000, 0.9659258262890683122, 1.000000000000000000, 0.9659258262890683122, 1.000000000000000000, 0.9659258262890683122, 1.000000000000000000, 0.9659258262890683122, 1.000000000000000000, 0.9659258262890683122, 1.000000000000000000, 0.9659258262890683122, 1.000000000000000000, 0.9659258262890683122, 1.000000000000000000, 0.9659258262890683122, 1.000000000000000000, 0.9659258262890683122, 1.000000000000000000, 0.9659258262890683122, 1.000000000000000000, 0.9659258262890683122, 1.000000000000000000, 0.9659258262890683122, 1.000000000000000000, 0.9659258262890683122, 1.000000000000000000, 0.9659258262890683122, 1.000000000000000000, 0.9659258262890683122, 1.000000000000000000, 0.9659258262890683122, 1.000000000000000000, 0.9659258262890683122, 1.000000000000000000, 0.9659258262890683122, 1.000000000000000000, 0.9659258262890683122, 1.000000000000000000, 0.9659258262890683122, 1.000000000000000000, 0.9659258262890683122, 1.000000000000000000, 0.9659258262890683122, 1.000000000000000000, 0.9659258262890683122, 1.000000000000000000, 0.9659258262890683122, 1.000000000000000000, 0.9659258262890683122, 1.000000000000000000, 0.9659258262890683122, 1.000000000000000000, 0.9659258262890683122, 1.000000000000000000, 0.9659258262890683122, 1.000000000000000000, 0.9659258262890683122, 1.000000000000000000, 0.9659258262890683122, 1.000000000000000000, 0.9659258262890683122, 1.000000000000000000, 0.9659258262890683122, 1.000000000000000000, 0.9659258262890683122, 1.000000000000000000, 0.9659258262890683122, 1.000000000000000000, 0.9659258262890683122, 1.000000000000000000, 0.9659258262890683122, 1.000000000000000000, 0.9659258262890683122, 1.000000000000000000, 0.9659258262890683122, 1.000000000000000000, 0.9659258262890683122, 1.000000000000000000, 0.9659258262890683122, 1.000000000000000000, 0.9659258262890683122, 1.000000000000000000, 0.9659258262890683122, 1.000000000000000000, 0.9659258262890683122, 1.000000000000000000, 0.9659258262890683122, 1.000000000000000000, 0.9659258262890683122, 1.000000000000000000, 0.9659258262890683122, 1.000000000000000000, 0.9659258262890683122, 1.000000000000000000, 0.9659258262890683122, 1.000000000000000000, 0.9659258262890683122, 1.000000000000000000, 0.9659258262890683122, 1.000000000000000000, 0.9659258262890683122, 1.000000000000000000, 0.9659258262890683122, 1.000000000000000000, 0.9659258262890683122, 1.000000000000000000, 0.9659258262890683122, 1.000000000000000000, 0.9659258262890683122, 1.000000000000000000, 0.9659258262890683122, 1.000000000000000000, 0.9659258262890683122, 1.000000000000000000, 0.9659258262890683122, 1.000000000000000000, 0.9659258262890683122, 1.000000000000000000, 0.9659258262890683122, 1.000000000000000000, 0.9659258262890683122, 1.000000000000000000, 0.9659258262890683122, 1.000000000000000000, 0.9659258262890683122, 1.000000000000000000, 0.9659258262890683122, 1.000000000000000000, 0.9659258262890683122, 1.000000000000000000, 0.9659258262890683122, 1.000000000000000000, 0.9659258262890683122, 1.000000000000000000, 0.9659258262890683122, 1.000000000000000000, 0.9659258262890683122, 1.000000000000000000, 0.9659258262890683122, 1.000000000000000000, 0.9659258262890683122, 1.000000000000000000, 0.9659258262890683122, 1.000000000000000000, 0.9659258262890683122, 1.000000000000000000, 0.9659258262890683122, 1.000000000000000000, 0.9659258262890683122, 1.000000000000000000, 0.9659258262890683122, 1.000000000000000000, 0.9659258262890683122, 1.000000000000000000, 0.9659258262890683122, 1.000000000000000000, 0.9659258262890683122, 1.000000000000000000, 0.9659258262890683122, 1.000000000000000000, 0.9659258262890683122, 1.000000000000000000, 0.9659258262890683122, 1.000000000000000000, 0.9659258262890683122, 1.000000000000000000, 0.9659258262890683122, 1.000000000000000000, 0.9659258262890683122, 1.000000000000000000, 0.9659258262890683122, 1.000000000000000000, 0.9659258262890683122, 1.000000000000000000, 0.9659258262890683122, 1.000000000000000000, 0.9659258262890683122, 1.000000000000000000, 0.9659258262890683122, 1.000000000000000000, 0.9659258262890683122, 1.000000000000000000, 0.9659258262890683122, 1.000000000000000000, 0.9659258262890683122, 1.000000000000000000, 0.9659258262890683122, 1.000000000000000000, 0.9659258262890683122, 1.000000000000000000, 0.9659258262890683122, 1.000000000000000000, 0.9659258262890683122, 1.000000000000000000, 0.9659258262890683122, 1.000000000000000000, 0.9659258262890683122, 1.000000000000000000, 0.9659258262890683122, 1.000000000000000000, 0.9659258262890683122, 1.000000000000000000, 0.9659258262890683122, 1.000000000000000000, 0.9659258262890683122, 1.000000000000000000, 0.9659258262890683122, 1.000000000000000000, 0.9659258262890683122, 1.000000000000000000, 0.9659258262890683122, 1.000000000000000000, 0.9659258262890683122, 1.000000000000000000, 0.9659258262890683122, 1.000000000000000000, 0.9659258262890683122, 1.000000000000000000, 0.9659258262890683122, 1.000000000000000000, 0.9659258262890683122, 1.000000000000000000, 0.9659258262890683122, 1.000000000000000000, 0.9659258262890683122, 1.000000000000000000, 0.9659258262890683122, 1.000000000000000000, 0.9659258262890683122, 1.000000000000000000, 0.9659258262890683122, 1.000000000000000000, 0.9659258262890683122, 1.000000000000000000, 0.9659258262890683122, 1.000000000000000000, 0.9659258262890683122, 1.000000000000000000, 0.9659258262890683122, 1.000000000000000000, 0.9659258262890683122, 1.000000000000000000, 0.9659258262890683122, 1.000000000000000000, 0.9659258262890683122, 1.000000000000000000, 0.9659258262890683122, 1.000000000000000000, 0.9659258262890683122, 1.000000000000000000, 0.9659258262890683122, 1.000000000000000000, 0.9659258262890683122, 1.000000000000000000, 0.9659258262890683122, 1.000000000000000000, 0.9659258262890683122, 1.000000000000000000, 0.9659258262890683122, 1.000000000000000000, 0.9659258262890683122, 1.000000000000000000, 0.9659258262890683122, 1.000000000000000000, 0.9659258262890683122, 1.000000000000000000, 0.9659258262890683122, 1.000000000000000000, 0.9659258262890683122, 1.000000000000000000),
 ( 0.3333333333333333703, 0.3219752754296894559, 0.3333333333333333703, 0.3219752754296894559, 0.3333333333333333703, 0.3219752754296894559, 0.3333333333333333703, 0.3219752754296894559, 0.3333333333333333703, 0.3219752754296894559, 0.3333333333333333703, 0.3219752754296894559, 0.3333333333333333703, 0.3219752754296894559, 0.3333333333333333703, 0.3219752754296894559, 0.3333333333333333703, 0.3219752754296894559, 0.3333333333333333703, 0.3219752754296894559, 0.3333333333333333703, 0.3219752754296894559, 0.3333333333333333703, 0.3219752754296894559, 0.3333333333333333703, 0.3219752754296894559, 0.3333333333333333703, 0.3219752754296894559, 0.3333333333333333703, 0.3219752754296894559, 0.3333333333333333703, 0.3219752754296894559, 0.3333333333333333703, 0.3219752754296894559, 0.3333333333333333703, 0.3219752754296894559, 0.3333333333333333703, 0.3219752754296894559, 0.3333333333333333703, 0.3219752754296894559, 0.3333333333333333703, 0.3219752754296894559, 0.3333333333333333703, 0.3219752754296894559, 0.3333333333333333703, 0.3219752754296894559, 0.3333333333333333703, 0.3219752754296894559, 0.3333333333333333703, 0.3219752754296894559, 0.3333333333333333703, 0.3219752754296894559, 0.3333333333333333703, 0.3219752754296894559, 0.3333333333333333703, 0.3219752754296894559, 0.3333333333333333703, 0.3219752754296894559, 0.3333333333333333703, 0.3219752754296894559, 0.3333333333333333703, 0.3219752754296894559, 0.3333333333333333703, 0.3219752754296894559, 0.3333333333333333703, 0.3219752754296894559, 0.3333333333333333703, 0.3219752754296894559, 0.3333333333333333703, 0.3219752754296894559, 0.3333333333333333703, 0.3219752754296894559, 0.3333333333333333703, 0.3219752754296894559, 0.3333333333333333703, 0.3219752754296894559, 0.3333333333333333703, 0.3219752754296894559, 0.3333333333333333703, 0.3219752754296894559, 0.3333333333333333703, 0.3219752754296894559, 0.3333333333333333703, 0.3219752754296894559, 0.3333333333333333703, 0.3219752754296894559, 0.3333333333333333703, 0.3219752754296894559, 0.3333333333333333703, 0.3219752754296894559, 0.3333333333333333703, 0.3219752754296894559, 0.3333333333333333703, 0.3219752754296894559, 0.3333333333333333703, 0.3219752754296894559, 0.3333333333333333703, 0.3219752754296894559, 0.3333333333333333703, 0.3219752754296894559, 0.3333333333333333703, 0.3219752754296894559, 0.3333333333333333703, 0.3219752754296894559, 0.3333333333333333703, 0.3219752754296894559, 0.3333333333333333703, 0.3219752754296894559, 0.3333333333333333703, 0.3219752754296894559, 0.3333333333333333703, 0.3219752754296894559, 0.3333333333333333703, 0.3219752754296894559, 0.3333333333333333703, 0.3219752754296894559, 0.3333333333333333703, 0.3219752754296894559, 0.3333333333333333703, 0.3219752754296894559, 0.3333333333333333703, 0.3219752754296894559, 0.3333333333333333703, 0.3219752754296894559, 0.3333333333333333703, 0.3219752754296894559, 0.3333333333333333703, 0.3219752754296894559, 0.3333333333333333703, 0.3219752754296894559, 0.3333333333333333703, 0.3219752754296894559, 0.3333333333333333703, 0.3219752754296894559, 0.3333333333333333703, 0.3219752754296894559, 0.3333333333333333703, 0.3219752754296894559, 0.3333333333333333703, 0.3219752754296894559, 0.3333333333333333703, 0.3219752754296894559, 0.3333333333333333703, 0.3219752754296894559, 0.3333333333333333703, 0.3219752754296894559, 0.3333333333333333703, 0.3219752754296894559, 0.3333333333333333703, 0.3219752754296894559, 0.3333333333333333703, 0.3219752754296894559, 0.3333333333333333703, 0.3219752754296894559, 0.3333333333333333703, 0.3219752754296894559, 0.3333333333333333703, 0.3219752754296894559, 0.3333333333333333703, 0.3219752754296894559, 0.3333333333333333703, 0.3219752754296894559, 0.3333333333333333703, 0.3219752754296894559, 0.3333333333333333703, 0.3219752754296894559, 0.3333333333333333703, 0.3219752754296894559, 0.3333333333333333703, 0.3219752754296894559, 0.3333333333333333703, 0.3219752754296894559, 0.3333333333333333703, 0.3219752754296894559, 0.3333333333333333703, 0.3219752754296894559, 0.3333333333333333703, 0.3219752754296894559, 0.3333333333333333703, 0.3219752754296894559, 0.3333333333333333703, 0.3219752754296894559, 0.3333333333333333703, 0.3219752754296894559, 0.3333333333333333703, 0.3219752754296894559, 0.3333333333333333703, 0.3219752754296894559, 0.3333333333333333703, 0.3219752754296894559, 0.3333333333333333703, 0.3219752754296894559, 0.3333333333333333703, 0.3219752754296894559, 0.3333333333333333703, 0.3219752754296894559, 0.3333333333333333703, 0.3219752754296894559, 0.3333333333333333703, 0.3219752754296894559, 0.3333333333333333703, 0.3219752754296894559, 0.3333333333333333703, 0.3219752754296894559, 0.3333333333333333703, 0.3219752754296894559, 0.3333333333333333703, 0.3219752754296894559, 0.3333333333333333703, 0.3219752754296894559, 0.3333333333333333703, 0.3219752754296894559, 0.3333333333333333703, 0.3219752754296894559, 0.3333333333333333703, 0.3219752754296894559, 0.3333333333333333703, 0.3219752754296894559, 0.3333333333333333703, 0.3219752754296894559, 0.3333333333333333703, 0.3219752754296894559, 0.3333333333333333703, 0.3219752754296894559, 0.3333333333333333703, 0.3219752754296894559, 0.3333333333333333703, 0.3219752754296894559, 0.3333333333333333703, 0.3219752754296894559, 0.3333333333333333703, 0.3219752754296894559, 0.3333333333333333703, 0.3219752754296894559, 0.3333333333333333703, 0.3219752754296894559, 0.3333333333333333703, 0.3219752754296894559, 0.3333333333333333703, 0.3219752754296894559, 0.3333333333333333703, 0.3219752754296894559, 0.3333333333333333703, 0.3219752754296894559, 0.3333333333333333703, 0.3219752754296894559, 0.3333333333333333703, 0.3219752754296894559, 0.3333333333333333703, 0.3219752754296894559, 0.3333333333333333703, 0.3219752754296894559, 0.3333333333333333703, 0.3219752754296894559, 0.3333333333333333703, 0.3219752754296894559, 0.3333333333333333703, 0.3219752754296894559, 0.3333333333333333703, 0.3219752754296894559, 0.3333333333333333703, 0.3219752754296894559, 0.3333333333333333703, 0.3219752754296894559, 0.3333333333333333703, 0.3219752754296894559, 0.3333333333333333703, 0.3219752754296894559, 0.3333333333333333703, 0.3219752754296894559, 0.3333333333333333703, 0.3219752754296894559, 0.3333333333333333703, 0.3219752754296894559, 0.3333333333333333703, 0.3219752754296894559, 0.3333333333333333703, 0.3219752754296894559, 0.3333333333333333703, 0.3219752754296894559, 0.3333333333333333703, 0.3219752754296894559, 0.3333333333333333703, 0.3219752754296894559, 0.3333333333333333703, 0.3219752754296894559, 0.3333333333333333703, 0.3219752754296894559, 0.3333333333333333703, 0.3219752754296894559, 0.3333333333333333703, 0.3219752754296894559, 0.3333333333333333703, 0.3219752754296894559, 0.3333333333333333703, 0.3219752754296894559, 0.3333333333333333703, 0.3219752754296894559, 0.3333333333333333703, 0.3219752754296894559, 0.3333333333333333703, 0.3219752754296894559, 0.3333333333333333703, 0.3219752754296894559, 0.3333333333333333703, 0.3219752754296894559, 0.3333333333333333703, 0.3219752754296894559, 0.3333333333333333703, 0.3219752754296894559, 0.3333333333333333703, 0.3219752754296894559, 0.3333333333333333703, 0.3219752754296894559, 0.3333333333333333703, 0.3219752754296894559, 0.3333333333333333703, 0.3219752754296894559, 0.3333333333333333703, 0.3219752754296894559, 0.3333333333333333703, 0.3219752754296894559, 0.3333333333333333703, 0.3219752754296894559, 0.3333333333333333703, 0.3219752754296894559, 0.3333333333333333703, 0.3219752754296894559, 0.3333333333333333703, 0.3219752754296894559, 0.3333333333333333703, 0.3219752754296894559, 0.3333333333333333703, 0.3219752754296894559, 0.3333333333333333703, 0.3219752754296894559, 0.3333333333333333703, 0.3219752754296894559, 0.3333333333333333703, 0.3219752754296894559, 0.3333333333333333703, 0.3219752754296894559, 0.3333333333333333703, 0.3219752754296894559, 0.3333333333333333703, 0.3219752754296894559, 0.3333333333333333703, 0.3219752754296894559, 0.3333333333333333703, 0.3219752754296894559, 0.3333333333333333703, 0.3219752754296894559, 0.3333333333333333703, 0.3219752754296894559, 0.3333333333333333703, 0.3219752754296894559, 0.3333333333333333703, 0.3219752754296894559, 0.3333333333333333703, 0.3219752754296894559, 0.3333333333333333703, 0.3219752754296894559, 0.3333333333333333703, 0.3219752754296894559, 0.3333333333333333703, 0.3219752754296894559, 0.3333333333333333703, 0.3219752754296894559, 0.3333333333333333703, 0.3219752754296894559, 0.3333333333333333703, 0.3219752754296894559, 0.3333333333333333703, 0.3219752754296894559, 0.3333333333333333703, 0.3219752754296894559, 0.3333333333333333703, 0.3219752754296894559, 0.3333333333333333703, 0.3219752754296894559, 0.3333333333333333703, 0.3219752754296894559, 0.3333333333333333703, 0.3219752754296894559, 0.3333333333333333703, 0.3219752754296894559, 0.3333333333333333703, 0.3219752754296894559, 0.3333333333333333703, 0.3219752754296894559, 0.3333333333333333703, 0.3219752754296894559, 0.3333333333333333703, 0.3219752754296894559, 0.3333333333333333703, 0.3219752754296894559, 0.3333333333333333703, 0.3219752754296894559, 0.3333333333333333703, 0.3219752754296894559, 0.3333333333333333703, 0.3219752754296894559, 0.3333333333333333703, 0.3219752754296894559, 0.3333333333333333703, 0.3219752754296894559, 0.3333333333333333703, 0.3219752754296894559, 0.3333333333333333703, 0.3219752754296894559, 0.3333333333333333703, 0.3219752754296894559, 0.3333333333333333703, 0.3219752754296894559, 0.3333333333333333703, 0.3219752754296894559, 0.3333333333333333703, 0.3219752754296894559, 0.3333333333333333703, 0.3219752754296894559, 0.3333333333333333703, 0.3219752754296894559, 0.3333333333333333703, 0.3219752754296894559, 0.3333333333333333703, 0.3219752754296894559, 0.3333333333333333703, 0.3219752754296894559, 0.3333333333333333703, 0.3219752754296894559, 0.3333333333333333703, 0.3219752754296894559, 0.3333333333333333703, 0.3219752754296894559, 0.3333333333333333703, 0.3219752754296894559, 0.3333333333333333703, 0.3219752754296894559, 0.3333333333333333703, 0.3219752754296894559, 0.3333333333333333703, 0.3219752754296894559, 0.3333333333333333703, 0.3219752754296894559, 0.3333333333333333703, 0.3219752754296894559, 0.3333333333333333703, 0.3219752754296894559, 0.3333333333333333703, 0.3219752754296894559, 0.3333333333333333703, 0.3219752754296894559, 0.3333333333333333703, 0.3219752754296894559, 0.3333333333333333703, 0.3219752754296894559, 0.3333333333333333703),
 ( 0.3333333333333333703, 0.3219752754296894559, 0.3333333333333333703, 0.3219752754296894559, 0.3333333333333333703, 0.3219752754296894559, 0.3333333333333333703, 0.3219752754296894559, 0.3333333333333333703, 0.3219752754296894559, 0.3333333333333333703, 0.3219752754296894559, 0.3333333333333333703, 0.3219752754296894559, 0.3333333333333333703, 0.3219752754296894559, 0.3333333333333333703, 0.3219752754296894559, 0.3333333333333333703, 0.3219752754296894559, 0.3333333333333333703, 0.3219752754296894559, 0.3333333333333333703, 0.3219752754296894559, 0.3333333333333333703, 0.3219752754296894559, 0.3333333333333333703, 0.3219752754296894559, 0.3333333333333333703, 0.3219752754296894559, 0.3333333333333333703, 0.3219752754296894559, 0.3333333333333333703, 0.3219752754296894559, 0.3333333333333333703, 0.3219752754296894559, 0.3333333333333333703, 0.3219752754296894559, 0.3333333333333333703, 0.3219752754296894559, 0.3333333333333333703, 0.3219752754296894559, 0.3333333333333333703, 0.3219752754296894559, 0.3333333333333333703, 0.3219752754296894559, 0.3333333333333333703, 0.3219752754296894559, 0.3333333333333333703, 0.3219752754296894559, 0.3333333333333333703, 0.3219752754296894559, 0.3333333333333333703, 0.3219752754296894559, 0.3333333333333333703, 0.3219752754296894559, 0.3333333333333333703, 0.3219752754296894559, 0.3333333333333333703, 0.3219752754296894559, 0.3333333333333333703, 0.3219752754296894559, 0.3333333333333333703, 0.3219752754296894559, 0.3333333333333333703, 0.3219752754296894559, 0.3333333333333333703, 0.3219752754296894559, 0.3333333333333333703, 0.3219752754296894559, 0.3333333333333333703, 0.3219752754296894559, 0.3333333333333333703, 0.3219752754296894559, 0.3333333333333333703, 0.3219752754296894559, 0.3333333333333333703, 0.3219752754296894559, 0.3333333333333333703, 0.3219752754296894559, 0.3333333333333333703, 0.3219752754296894559, 0.3333333333333333703, 0.3219752754296894559, 0.3333333333333333703, 0.3219752754296894559, 0.3333333333333333703, 0.3219752754296894559, 0.3333333333333333703, 0.3219752754296894559, 0.3333333333333333703, 0.3219752754296894559, 0.3333333333333333703, 0.3219752754296894559, 0.3333333333333333703, 0.3219752754296894559, 0.3333333333333333703, 0.3219752754296894559, 0.3333333333333333703, 0.3219752754296894559, 0.3333333333333333703, 0.3219752754296894559, 0.3333333333333333703, 0.3219752754296894559, 0.3333333333333333703, 0.3219752754296894559, 0.3333333333333333703, 0.3219752754296894559, 0.3333333333333333703, 0.3219752754296894559, 0.3333333333333333703, 0.3219752754296894559, 0.3333333333333333703, 0.3219752754296894559, 0.3333333333333333703, 0.3219752754296894559, 0.3333333333333333703, 0.3219752754296894559, 0.3333333333333333703, 0.3219752754296894559, 0.3333333333333333703, 0.3219752754296894559, 0.3333333333333333703, 0.3219752754296894559, 0.3333333333333333703, 0.3219752754296894559, 0.3333333333333333703, 0.3219752754296894559, 0.3333333333333333703, 0.3219752754296894559, 0.3333333333333333703, 0.3219752754296894559, 0.3333333333333333703, 0.3219752754296894559, 0.3333333333333333703, 0.3219752754296894559, 0.3333333333333333703, 0.3219752754296894559, 0.3333333333333333703, 0.3219752754296894559, 0.3333333333333333703, 0.3219752754296894559, 0.3333333333333333703, 0.3219752754296894559, 0.3333333333333333703, 0.3219752754296894559, 0.3333333333333333703, 0.3219752754296894559, 0.3333333333333333703, 0.3219752754296894559, 0.3333333333333333703, 0.3219752754296894559, 0.3333333333333333703, 0.3219752754296894559, 0.3333333333333333703, 0.3219752754296894559, 0.3333333333333333703, 0.3219752754296894559, 0.3333333333333333703, 0.3219752754296894559, 0.3333333333333333703, 0.3219752754296894559, 0.3333333333333333703, 0.3219752754296894559, 0.3333333333333333703, 0.3219752754296894559, 0.3333333333333333703, 0.3219752754296894559, 0.3333333333333333703, 0.3219752754296894559, 0.3333333333333333703, 0.3219752754296894559, 0.3333333333333333703, 0.3219752754296894559, 0.3333333333333333703, 0.3219752754296894559, 0.3333333333333333703, 0.3219752754296894559, 0.3333333333333333703, 0.3219752754296894559, 0.3333333333333333703, 0.3219752754296894559, 0.3333333333333333703, 0.3219752754296894559, 0.3333333333333333703, 0.3219752754296894559, 0.3333333333333333703, 0.3219752754296894559, 0.3333333333333333703, 0.3219752754296894559, 0.3333333333333333703, 0.3219752754296894559, 0.3333333333333333703, 0.3219752754296894559, 0.3333333333333333703, 0.3219752754296894559, 0.3333333333333333703, 0.3219752754296894559, 0.3333333333333333703, 0.3219752754296894559, 0.3333333333333333703, 0.3219752754296894559, 0.3333333333333333703, 0.3219752754296894559, 0.3333333333333333703, 0.3219752754296894559, 0.3333333333333333703, 0.3219752754296894559, 0.3333333333333333703, 0.3219752754296894559, 0.3333333333333333703, 0.3219752754296894559, 0.3333333333333333703, 0.3219752754296894559, 0.3333333333333333703, 0.3219752754296894559, 0.3333333333333333703, 0.3219752754296894559, 0.3333333333333333703, 0.3219752754296894559, 0.3333333333333333703, 0.3219752754296894559, 0.3333333333333333703, 0.3219752754296894559, 0.3333333333333333703, 0.3219752754296894559, 0.3333333333333333703, 0.3219752754296894559, 0.3333333333333333703, 0.3219752754296894559, 0.3333333333333333703, 0.3219752754296894559, 0.3333333333333333703, 0.3219752754296894559, 0.3333333333333333703, 0.3219752754296894559, 0.3333333333333333703, 0.3219752754296894559, 0.3333333333333333703, 0.3219752754296894559, 0.3333333333333333703, 0.3219752754296894559, 0.3333333333333333703, 0.3219752754296894559, 0.3333333333333333703, 0.3219752754296894559, 0.3333333333333333703, 0.3219752754296894559, 0.3333333333333333703, 0.3219752754296894559, 0.3333333333333333703, 0.3219752754296894559, 0.3333333333333333703, 0.3219752754296894559, 0.3333333333333333703, 0.3219752754296894559, 0.3333333333333333703, 0.3219752754296894559, 0.3333333333333333703, 0.3219752754296894559, 0.3333333333333333703, 0.3219752754296894559, 0.3333333333333333703, 0.3219752754296894559, 0.3333333333333333703, 0.3219752754296894559, 0.3333333333333333703, 0.3219752754296894559, 0.3333333333333333703, 0.3219752754296894559, 0.3333333333333333703, 0.3219752754296894559, 0.3333333333333333703, 0.3219752754296894559, 0.3333333333333333703, 0.3219752754296894559, 0.3333333333333333703, 0.3219752754296894559, 0.3333333333333333703, 0.3219752754296894559, 0.3333333333333333703, 0.3219752754296894559, 0.3333333333333333703, 0.3219752754296894559, 0.3333333333333333703, 0.3219752754296894559, 0.3333333333333333703, 0.3219752754296894559, 0.3333333333333333703, 0.3219752754296894559, 0.3333333333333333703, 0.3219752754296894559, 0.3333333333333333703, 0.3219752754296894559, 0.3333333333333333703, 0.3219752754296894559, 0.3333333333333333703, 0.3219752754296894559, 0.3333333333333333703, 0.3219752754296894559, 0.3333333333333333703, 0.3219752754296894559, 0.3333333333333333703, 0.3219752754296894559, 0.3333333333333333703, 0.3219752754296894559, 0.3333333333333333703, 0.3219752754296894559, 0.3333333333333333703, 0.3219752754296894559, 0.3333333333333333703, 0.3219752754296894559, 0.3333333333333333703, 0.3219752754296894559, 0.3333333333333333703, 0.3219752754296894559, 0.3333333333333333703, 0.3219752754296894559, 0.3333333333333333703, 0.3219752754296894559, 0.3333333333333333703, 0.3219752754296894559, 0.3333333333333333703, 0.3219752754296894559, 0.3333333333333333703, 0.3219752754296894559, 0.3333333333333333703, 0.3219752754296894559, 0.3333333333333333703, 0.3219752754296894559, 0.3333333333333333703, 0.3219752754296894559, 0.3333333333333333703, 0.3219752754296894559, 0.3333333333333333703, 0.3219752754296894559, 0.3333333333333333703, 0.3219752754296894559, 0.3333333333333333703, 0.3219752754296894559, 0.3333333333333333703, 0.3219752754296894559, 0.3333333333333333703, 0.3219752754296894559, 0.3333333333333333703, 0.3219752754296894559, 0.3333333333333333703, 0.3219752754296894559, 0.3333333333333333703, 0.3219752754296894559, 0.3333333333333333703, 0.3219752754296894559, 0.3333333333333333703, 0.3219752754296894559, 0.3333333333333333703, 0.3219752754296894559, 0.3333333333333333703, 0.3219752754296894559, 0.3333333333333333703, 0.3219752754296894559, 0.3333333333333333703, 0.3219752754296894559, 0.3333333333333333703, 0.3219752754296894559, 0.3333333333333333703, 0.3219752754296894559, 0.3333333333333333703, 0.3219752754296894559, 0.3333333333333333703, 0.3219752754296894559, 0.3333333333333333703, 0.3219752754296894559, 0.3333333333333333703, 0.3219752754296894559, 0.3333333333333333703, 0.3219752754296894559, 0.3333333333333333703, 0.3219752754296894559, 0.3333333333333333703, 0.3219752754296894559, 0.3333333333333333703, 0.3219752754296894559, 0.3333333333333333703, 0.3219752754296894559, 0.3333333333333333703, 0.3219752754296894559, 0.3333333333333333703, 0.3219752754296894559, 0.3333333333333333703, 0.3219752754296894559, 0.3333333333333333703, 0.3219752754296894559, 0.3333333333333333703, 0.3219752754296894559, 0.3333333333333333703, 0.3219752754296894559, 0.3333333333333333703, 0.3219752754296894559, 0.3333333333333333703, 0.3219752754296894559, 0.3333333333333333703, 0.3219752754296894559, 0.3333333333333333703, 0.3219752754296894559, 0.3333333333333333703, 0.3219752754296894559, 0.3333333333333333703, 0.3219752754296894559, 0.3333333333333333703, 0.3219752754296894559, 0.3333333333333333703, 0.3219752754296894559, 0.3333333333333333703, 0.3219752754296894559, 0.3333333333333333703, 0.3219752754296894559, 0.3333333333333333703, 0.3219752754296894559, 0.3333333333333333703, 0.3219752754296894559, 0.3333333333333333703, 0.3219752754296894559, 0.3333333333333333703, 0.3219752754296894559, 0.3333333333333333703, 0.3219752754296894559, 0.3333333333333333703, 0.3219752754296894559, 0.3333333333333333703, 0.3219752754296894559, 0.3333333333333333703, 0.3219752754296894559, 0.3333333333333333703, 0.3219752754296894559, 0.3333333333333333703, 0.3219752754296894559, 0.3333333333333333703, 0.3219752754296894559, 0.3333333333333333703, 0.3219752754296894559, 0.3333333333333333703, 0.3219752754296894559, 0.3333333333333333703, 0.3219752754296894559, 0.3333333333333333703, 0.3219752754296894559, 0.3333333333333333703, 0.3219752754296894559, 0.3333333333333333703, 0.3219752754296894559, 0.3333333333333333703, 0.3219752754296894559, 0.3333333333333333703, 0.3219752754296894559, 0.3333333333333333703, 0.3219752754296894559, 0.3333333333333333703),
 ( 1.000000000000000000, 0.9659258262890683122, 1.000000000000000000, 0.9659258262890683122, 1.000000000000000000, 0.9659258262890683122, 1.000000000000000000, 0.9659258262890683122, 1.000000000000000000, 0.9659258262890683122, 1.000000000000000000, 0.9659258262890683122, 1.000000000000000000, 0.9659258262890683122, 1.000000000000000000, 0.9659258262890683122, 1.000000000000000000, 0.9659258262890683122, 1.000000000000000000, 0.9659258262890683122, 1.000000000000000000, 0.9659258262890683122, 1.000000000000000000, 0.9659258262890683122, 1.000000000000000000, 0.9659258262890683122, 1.000000000000000000, 0.9659258262890683122, 1.000000000000000000, 0.9659258262890683122, 1.000000000000000000, 0.9659258262890683122, 1.000000000000000000, 0.9659258262890683122, 1.000000000000000000, 0.9659258262890683122, 1.000000000000000000, 0.9659258262890683122, 1.000000000000000000, 0.9659258262890683122, 1.000000000000000000, 0.9659258262890683122, 1.000000000000000000, 0.9659258262890683122, 1.000000000000000000, 0.9659258262890683122, 1.000000000000000000, 0.9659258262890683122, 1.000000000000000000, 0.9659258262890683122, 1.000000000000000000, 0.9659258262890683122, 1.000000000000000000, 0.9659258262890683122, 1.000000000000000000, 0.9659258262890683122, 1.000000000000000000, 0.9659258262890683122, 1.000000000000000000, 0.9659258262890683122, 1.000000000000000000, 0.9659258262890683122, 1.000000000000000000, 0.9659258262890683122, 1.000000000000000000, 0.9659258262890683122, 1.000000000000000000, 0.9659258262890683122, 1.000000000000000000, 0.9659258262890683122, 1.000000000000000000, 0.9659258262890683122, 1.000000000000000000, 0.9659258262890683122, 1.000000000000000000, 0.9659258262890683122, 1.000000000000000000, 0.9659258262890683122, 1.000000000000000000, 0.9659258262890683122, 1.000000000000000000, 0.9659258262890683122, 1.000000000000000000, 0.9659258262890683122, 1.000000000000000000, 0.9659258262890683122, 1.000000000000000000, 0.9659258262890683122, 1.000000000000000000, 0.9659258262890683122, 1.000000000000000000, 0.9659258262890683122, 1.000000000000000000, 0.9659258262890683122, 1.000000000000000000, 0.9659258262890683122, 1.000000000000000000, 0.9659258262890683122, 1.000000000000000000, 0.9659258262890683122, 1.000000000000000000, 0.9659258262890683122, 1.000000000000000000, 0.9659258262890683122, 1.000000000000000000, 0.9659258262890683122, 1.000000000000000000, 0.9659258262890683122, 1.000000000000000000, 0.9659258262890683122, 1.000000000000000000, 0.9659258262890683122, 1.000000000000000000, 0.9659258262890683122, 1.000000000000000000, 0.9659258262890683122, 1.000000000000000000, 0.9659258262890683122, 1.000000000000000000, 0.9659258262890683122, 1.000000000000000000, 0.9659258262890683122, 1.000000000000000000, 0.9659258262890683122, 1.000000000000000000, 0.9659258262890683122, 1.000000000000000000, 0.9659258262890683122, 1.000000000000000000, 0.9659258262890683122, 1.000000000000000000, 0.9659258262890683122, 1.000000000000000000, 0.9659258262890683122, 1.000000000000000000, 0.9659258262890683122, 1.000000000000000000, 0.9659258262890683122, 1.000000000000000000, 0.9659258262890683122, 1.000000000000000000, 0.9659258262890683122, 1.000000000000000000, 0.9659258262890683122, 1.000000000000000000, 0.9659258262890683122, 1.000000000000000000, 0.9659258262890683122, 1.000000000000000000, 0.9659258262890683122, 1.000000000000000000, 0.9659258262890683122, 1.000000000000000000, 0.9659258262890683122, 1.000000000000000000, 0.9659258262890683122, 1.000000000000000000, 0.9659258262890683122, 1.000000000000000000, 0.9659258262890683122, 1.000000000000000000, 0.9659258262890683122, 1.000000000000000000, 0.9659258262890683122, 1.000000000000000000, 0.9659258262890683122, 1.000000000000000000, 0.9659258262890683122, 1.000000000000000000, 0.9659258262890683122, 1.000000000000000000, 0.9659258262890683122, 1.000000000000000000, 0.9659258262890683122, 1.000000000000000000, 0.9659258262890683122, 1.000000000000000000, 0.9659258262890683122, 1.000000000000000000, 0.9659258262890683122, 1.000000000000000000, 0.9659258262890683122, 1.000000000000000000, 0.9659258262890683122, 1.000000000000000000, 0.9659258262890683122, 1.000000000000000000, 0.9659258262890683122, 1.000000000000000000, 0.9659258262890683122, 1.000000000000000000, 0.9659258262890683122, 1.000000000000000000, 0.9659258262890683122, 1.000000000000000000, 0.9659258262890683122, 1.000000000000000000, 0.9659258262890683122, 1.000000000000000000, 0.9659258262890683122, 1.000000000000000000, 0.9659258262890683122, 1.000000000000000000, 0.9659258262890683122, 1.000000000000000000, 0.9659258262890683122, 1.000000000000000000, 0.9659258262890683122, 1.000000000000000000, 0.9659258262890683122, 1.000000000000000000, 0.9659258262890683122, 1.000000000000000000, 0.9659258262890683122, 1.000000000000000000, 0.9659258262890683122, 1.000000000000000000, 0.9659258262890683122, 1.000000000000000000, 0.9659258262890683122, 1.000000000000000000, 0.9659258262890683122, 1.000000000000000000, 0.9659258262890683122, 1.000000000000000000, 0.9659258262890683122, 1.000000000000000000, 0.9659258262890683122, 1.000000000000000000, 0.9659258262890683122, 1.000000000000000000, 0.9659258262890683122, 1.000000000000000000, 0.9659258262890683122, 1.000000000000000000, 0.9659258262890683122, 1.000000000000000000, 0.9659258262890683122, 1.000000000000000000, 0.9659258262890683122, 1.000000000000000000, 0.9659258262890683122, 1.000000000000000000, 0.9659258262890683122, 1.000000000000000000, 0.9659258262890683122, 1.000000000000000000, 0.9659258262890683122, 1.000000000000000000, 0.9659258262890683122, 1.000000000000000000, 0.9659258262890683122, 1.000000000000000000, 0.9659258262890683122, 1.000000000000000000, 0.9659258262890683122, 1.000000000000000000, 0.9659258262890683122, 1.000000000000000000, 0.9659258262890683122, 1.000000000000000000, 0.9659258262890683122, 1.000000000000000000, 0.9659258262890683122, 1.000000000000000000, 0.9659258262890683122, 1.000000000000000000, 0.9659258262890683122, 1.000000000000000000, 0.9659258262890683122, 1.000000000000000000, 0.9659258262890683122, 1.000000000000000000, 0.9659258262890683122, 1.000000000000000000, 0.9659258262890683122, 1.000000000000000000, 0.9659258262890683122, 1.000000000000000000, 0.9659258262890683122, 1.000000000000000000, 0.9659258262890683122, 1.000000000000000000, 0.9659258262890683122, 1.000000000000000000, 0.9659258262890683122, 1.000000000000000000, 0.9659258262890683122, 1.000000000000000000, 0.9659258262890683122, 1.000000000000000000, 0.9659258262890683122, 1.000000000000000000, 0.9659258262890683122, 1.000000000000000000, 0.9659258262890683122, 1.000000000000000000, 0.9659258262890683122, 1.000000000000000000, 0.9659258262890683122, 1.000000000000000000, 0.9659258262890683122, 1.000000000000000000, 0.9659258262890683122, 1.000000000000000000, 0.9659258262890683122, 1.000000000000000000, 0.9659258262890683122, 1.000000000000000000, 0.9659258262890683122, 1.000000000000000000, 0.9659258262890683122, 1.000000000000000000, 0.9659258262890683122, 1.000000000000000000, 0.9659258262890683122, 1.000000000000000000, 0.9659258262890683122, 1.000000000000000000, 0.9659258262890683122, 1.000000000000000000, 0.9659258262890683122, 1.000000000000000000, 0.9659258262890683122, 1.000000000000000000, 0.9659258262890683122, 1.000000000000000000, 0.9659258262890683122, 1.000000000000000000, 0.9659258262890683122, 1.000000000000000000, 0.9659258262890683122, 1.000000000000000000, 0.9659258262890683122, 1.000000000000000000, 0.9659258262890683122, 1.000000000000000000, 0.9659258262890683122, 1.000000000000000000, 0.9659258262890683122, 1.000000000000000000, 0.9659258262890683122, 1.000000000000000000, 0.9659258262890683122, 1.000000000000000000, 0.9659258262890683122, 1.000000000000000000, 0.9659258262890683122, 1.000000000000000000, 0.9659258262890683122, 1.000000000000000000, 0.9659258262890683122, 1.000000000000000000, 0.9659258262890683122, 1.000000000000000000, 0.9659258262890683122, 1.000000000000000000, 0.9659258262890683122, 1.000000000000000000, 0.9659258262890683122, 1.000000000000000000, 0.9659258262890683122, 1.000000000000000000, 0.9659258262890683122, 1.000000000000000000, 0.9659258262890683122, 1.000000000000000000, 0.9659258262890683122, 1.000000000000000000, 0.9659258262890683122, 1.000000000000000000, 0.9659258262890683122, 1.000000000000000000, 0.9659258262890683122, 1.000000000000000000, 0.9659258262890683122, 1.000000000000000000, 0.9659258262890683122, 1.000000000000000000, 0.9659258262890683122, 1.000000000000000000, 0.9659258262890683122, 1.000000000000000000, 0.9659258262890683122, 1.000000000000000000, 0.9659258262890683122, 1.000000000000000000, 0.9659258262890683122, 1.000000000000000000, 0.9659258262890683122, 1.000000000000000000, 0.9659258262890683122, 1.000000000000000000, 0.9659258262890683122, 1.000000000000000000, 0.9659258262890683122, 1.000000000000000000, 0.9659258262890683122, 1.000000000000000000, 0.9659258262890683122, 1.000000000000000000, 0.9659258262890683122, 1.000000000000000000, 0.9659258262890683122, 1.000000000000000000, 0.9659258262890683122, 1.000000000000000000, 0.9659258262890683122, 1.000000000000000000, 0.9659258262890683122, 1.000000000000000000, 0.9659258262890683122, 1.000000000000000000, 0.9659258262890683122, 1.000000000000000000, 0.9659258262890683122, 1.000000000000000000, 0.9659258262890683122, 1.000000000000000000, 0.9659258262890683122, 1.000000000000000000, 0.9659258262890683122, 1.000000000000000000, 0.9659258262890683122, 1.000000000000000000, 0.9659258262890683122, 1.000000000000000000, 0.9659258262890683122, 1.000000000000000000, 0.9659258262890683122, 1.000000000000000000, 0.9659258262890683122, 1.000000000000000000, 0.9659258262890683122, 1.000000000000000000, 0.9659258262890683122, 1.000000000000000000, 0.9659258262890683122, 1.000000000000000000, 0.9659258262890683122, 1.000000000000000000, 0.9659258262890683122, 1.000000000000000000, 0.9659258262890683122, 1.000000000000000000, 0.9659258262890683122, 1.000000000000000000, 0.9659258262890683122, 1.000000000000000000, 0.9659258262890683122, 1.000000000000000000, 0.9659258262890683122, 1.000000000000000000, 0.9659258262890683122, 1.000000000000000000, 0.9659258262890683122, 1.000000000000000000) ) ) 
 REPRESENTATION_ITEM ( '' )  SURFACE ( )  );
#6563=CARTESIAN_POINT ( 'NONE',  ( -8.314922557961024197, 14.29746914071037800, 27.91775706135234358 ) ) ;
#6564=CARTESIAN_POINT ( 'NONE',  ( -14.29746914071049879, 8.314922557960819915, 65.83224293864769550 ) ) ;
#6565=CARTESIAN_POINT ( 'NONE',  ( 15.72974639402176855, 15.80617190586768217, 76.87609039468567573 ) ) ;
#6566=CARTESIAN_POINT ( 'NONE',  ( 4.483927247898790824, -16.52544592524335698, 100.2094237280190043 ) ) ;
#6567=CARTESIAN_POINT ( 'NONE',  ( 17.40861289039011339, -6.110651285853056613, 46.12767529172570136 ) ) ;
#6568=CARTESIAN_POINT ( 'NONE',  ( -18.56399227203345959, -5.499999999999829470, 63.97830131249904184 ) ) ;
#6569=CARTESIAN_POINT ( 'NONE',  ( -16.52544592524342804, 4.483927247898546575, 26.04057627198103475 ) ) ;
#6570=CARTESIAN_POINT ( 'NONE',  ( -4.483927247898782831, 16.52544592524335698, 72.70942372801901854 ) ) ;
#6571=CARTESIAN_POINT ( 'NONE',  ( -0.05219959533909027116, -19.03943276465977164, 87.49890960531436690 ) ) ;
#6572=CARTESIAN_POINT ( 'NONE',  ( 16.46253265017160672, -9.564922557960803928, 98.33224293864769550 ) ) ;
#6573=CARTESIAN_POINT ( 'NONE',  ( -10.81492255796105439, 18.62759615963255655, 82.91775706135234714 ) ) ;
#6574=CARTESIAN_POINT ( 'NONE',  ( -14.29746914071037622, -8.314922557961029526, 94.16775706135237556 ) ) ;
#6575=CARTESIAN_POINT ( 'NONE',  ( -14.29746914071049879, 8.314922557960819915, 60.83224293864769550 ) ) ;
#6576=CARTESIAN_POINT ( 'NONE',  ( -13.89961937509977652, 13.97604488694528158, 65.62390960531436690 ) ) ;
#6578=CARTESIAN_POINT ( 'NONE',  ( -19.05341960407617563, 5.049401038297882671, 108.5427570613523187 ) ) ;
#6579=CARTESIAN_POINT ( 'NONE',  ( -16.53943276465976808, 0.05219959533911058130, 111.2489096053143669 ) ) ;
#6580=CARTESIAN_POINT ( 'NONE',  ( 19.05341960407611168, 5.049401038298154454, 73.95724293864768129 ) ) ;
#6581=CARTESIAN_POINT ( 'NONE',  ( -4.379528057220086978, -16.55341960407618274, 19.79275706135235069 ) ) ;
#6583=CARTESIAN_POINT ( 'NONE',  ( -19.03943276465977164, -0.05219959533935918106, 23.75109039468566152 ) ) ;
#6584=CARTESIAN_POINT ( 'NONE',  ( 4.379528057220092307, 16.55341960407617563, 77.29275706135234714 ) ) ;
#6585=CARTESIAN_POINT ( 'NONE',  ( -13.97604488694547697, 13.89961937509957934, 98.12609039468566152 ) ) ;
#6586=CARTESIAN_POINT ( 'NONE',  ( 19.03943276465977164, -0.05219959533909143690, 23.74890960531435269 ) ) ;
#6587=CARTESIAN_POINT ( 'NONE',  ( 0.05219959533934541429, -16.53943276465976808, 65.00109039468568994 ) ) ;
#6588=CARTESIAN_POINT ( 'NONE',  ( 0.05219959533934541429, -16.53943276465976808, 50.00109039468568994 ) ) ;
#6589=CARTESIAN_POINT ( 'NONE',  ( -5.153800228976328057, -19.02544592524343514, 27.29057627198103120 ) ) ;
#6590=CARTESIAN_POINT ( 'NONE',  ( 13.89961937509957401, 13.97604488694547697, 51.87609039468566863 ) ) ;
#6591=CARTESIAN_POINT ( 'NONE',  ( -5.823673210054431948, 21.52544592524334988, 92.70942372801901854 ) ) ;
#6592=CARTESIAN_POINT ( 'NONE',  ( -19.02544592524342804, 5.153800228976336051, 31.04057627198102409 ) ) ;
#6593=CARTESIAN_POINT ( 'NONE',  ( 5.153800228976335163, 19.02544592524342804, 74.79057627198103830 ) ) ;
#6594=CARTESIAN_POINT ( 'NONE',  ( -8.314922557960811034, -14.29746914071050412, 72.08224293864769550 ) ) ;
#6596=CARTESIAN_POINT ( 'NONE',  ( 21.55341960407619695, -5.719274019375665929, 96.04275706135236135 ) ) ;
#6597=CARTESIAN_POINT ( 'NONE',  ( 0.05219959533936267826, -19.03943276465977164, 60.00109039468566863 ) ) ;
#6598=CARTESIAN_POINT ( 'NONE',  ( 13.97604488694548053, -13.89961937509957401, 40.62609039468564731 ) ) ;
#6599=CARTESIAN_POINT ( 'NONE',  ( 10.72451020669898902, -18.67979575497178502, 37.91557627198102409 ) ) ;
#6600=CARTESIAN_POINT ( 'NONE',  ( 21.53943276465977519, 0.05219959533937863772, 106.2510903946856757 ) ) ;
#6601=CARTESIAN_POINT ( 'NONE',  ( -13.97604488694527625, -13.89961937509977652, 71.87390960531433848 ) ) ;
#6602=CARTESIAN_POINT ( 'NONE',  ( 18.67979575497194134, -10.72451020669871369, 105.8344237280190328 ) ) ;
#6603=CARTESIAN_POINT ( 'NONE',  ( -5.719274019375978568, 21.55341960407610458, 45.20724293864769550 ) ) ;
#6604=CARTESIAN_POINT ( 'NONE',  ( 9.474510206698971260, -16.51473224551069308, 102.9155762719810241 ) ) ;
#6605=CARTESIAN_POINT ( 'NONE',  ( -5.049401038297874678, -19.05341960407617918, 69.79275706135233293 ) ) ;
#6606=CARTESIAN_POINT ( 'NONE',  ( -19.03943276465977164, 0.05219959533909376836, 106.2489096053143669 ) ) ;
#6607=CARTESIAN_POINT ( 'NONE',  ( -16.51473224551082808, 9.474510206698731452, 98.33442372801900433 ) ) ;
#6608=CARTESIAN_POINT ( 'NONE',  ( 16.53943276465976808, 0.05219959533934440121, 41.25109039468568284 ) ) ;
#6609=CARTESIAN_POINT ( 'NONE',  ( -16.46253265017160317, 9.564922557960807481, 25.83224293864769194 ) ) ;
#6610=CARTESIAN_POINT ( 'NONE',  ( 13.89961937509977652, -13.97604488694527269, 78.12390960531433848 ) ) ;
#6611=CARTESIAN_POINT ( 'NONE',  ( 18.62759615963271287, -10.81492255796078972, 68.33224293864769550 ) ) ;
#6612=CARTESIAN_POINT ( 'NONE',  ( -12.14591786802326823, 12.06949235617739902, 38.12609039468567573 ) ) ;
#6613=CARTESIAN_POINT ( 'NONE',  ( 5.823673210054444382, -21.52544592524334988, 40.20942372801901854 ) ) ;
#6614=CARTESIAN_POINT ( 'NONE',  ( 5.823673210054444382, -21.52544592524334988, 80.20942372801901854 ) ) ;
#6615=CARTESIAN_POINT ( 'NONE',  ( -12.06949235617739369, -12.14591786802326823, 79.37609039468567573 ) ) ;
#6616=CARTESIAN_POINT ( 'NONE',  ( 16.51473224551069308, 9.474510206698969483, 89.16557627198103830 ) ) ;
#6617=CARTESIAN_POINT ( 'NONE',  ( -16.55341960407611168, -4.379528057220339221, 71.45724293864769550 ) ) ;
#6618=CARTESIAN_POINT ( 'NONE',  ( 8.224510206698953496, -14.34966873604960469, 27.91557627198103830 ) ) ;
#6619=CARTESIAN_POINT ( 'NONE',  ( -19.03943276465977164, -0.05219959533935918106, 53.75109039468566863 ) ) ;
#6620=CARTESIAN_POINT ( 'NONE',  ( -15.80617190586768217, 15.72974639402176855, 43.12609039468568284 ) ) ;
#6621=CARTESIAN_POINT ( 'NONE',  ( 16.53943276465976808, -0.05219959533910856209, 83.74890960531435269 ) ) ;
#6622=CARTESIAN_POINT ( 'NONE',  ( 15.72974639402199770, -15.80617190586745480, 23.12390960531436335 ) ) ;
#6623=CARTESIAN_POINT ( 'NONE',  ( 16.52544592524335698, 4.483927247898782831, 96.45942372801901854 ) ) ;
#6624=CARTESIAN_POINT ( 'NONE',  ( 10.81492255796106328, -18.62759615963255655, 80.41775706135234714 ) ) ;
#6625=CARTESIAN_POINT ( 'NONE',  ( 0.05219959533934541429, -16.53943276465976808, 50.00109039468568994 ) ) ;
#6626=CARTESIAN_POINT ( 'NONE',  ( -21.55341960407619339, 5.719274019375674811, 43.54275706135235424 ) ) ;
#6628=CARTESIAN_POINT ( 'NONE',  ( 18.67979575497178502, 10.72451020669898547, 109.1655762719810383 ) ) ;
#6629=CARTESIAN_POINT ( 'NONE',  ( -8.224510206698948167, 14.34966873604960824, 90.41557627198103830 ) ) ;
#6630=EDGE_CURVE ( 'NONE', #122538, #2008, #46499, .T. ) ;
#6632=CARTESIAN_POINT ( 'NONE',  ( 8.314922557960818139, 14.29746914071049879, 49.58224293864769550 ) ) ;
#6633=CARTESIAN_POINT ( 'NONE',  ( -14.29746914071037622, -8.314922557961029526, 94.16775706135237556 ) ) ;
#6634=CARTESIAN_POINT ( 'NONE',  ( -9.564922557960796823, -16.46253265017161027, 42.08224293864769550 ) ) ;
#6635=CARTESIAN_POINT ( 'NONE',  ( 15.80617190586746368, 15.72974639402197994, 44.37390960531435979 ) ) ;
#6636=CARTESIAN_POINT ( 'NONE',  ( -14.34966873604960291, -8.224510206698953496, 71.66557627198100988 ) ) ;
#6637=CARTESIAN_POINT ( 'NONE',  ( -21.53943276465977519, 0.05219959533907696930, 76.24890960531435269 ) ) ;
#6638=CARTESIAN_POINT ( 'NONE',  ( -16.51473224551069308, -9.474510206698971260, 86.66557627198102409 ) ) ;
#6639=CARTESIAN_POINT ( 'NONE',  ( 5.153800228976335163, 19.02544592524342804, 34.79057627198102409 ) ) ;
#6640=CARTESIAN_POINT ( 'NONE',  ( 0.05219959533936267826, -19.03943276465977164, 95.00109039468567573 ) ) ;
#6642=CARTESIAN_POINT ( 'NONE',  ( 21.52544592524344225, -5.823673210054117533, 28.54057627198103120 ) ) ;
#6643=CARTESIAN_POINT ( 'NONE',  ( 15.72974639402176855, 15.80617190586768217, 56.87609039468568994 ) ) ;
#6644=CARTESIAN_POINT ( 'NONE',  ( 9.564922557960805705, 16.46253265017160317, 49.58224293864770260 ) ) ;
#6645=CARTESIAN_POINT ( 'NONE',  ( 0.05219959533909260263, 19.03943276465977164, 84.99890960531436690 ) ) ;
#6647=CARTESIAN_POINT ( 'NONE',  ( -16.53943276465976808, -0.05219959533934237506, 53.75109039468568994 ) ) ;
#6648=CARTESIAN_POINT ( 'NONE',  ( 10.72451020669871369, 18.67979575497193778, 32.08442372801901854 ) ) ;
#6649=CARTESIAN_POINT ( 'NONE',  ( 21.55341960407619695, -5.719274019375665929, 71.04275706135234714 ) ) ;
#6650=CARTESIAN_POINT ( 'NONE',  ( -10.81492255796078084, -18.62759615963271287, 27.08224293864769550 ) ) ;
#6651=CARTESIAN_POINT ( 'NONE',  ( 15.72974639402199770, -15.80617190586745480, 83.12390960531436690 ) ) ;
#6652=CARTESIAN_POINT ( 'NONE',  ( -21.52544592524334988, -5.823673210054445271, 18.95942372801901143 ) ) ;
#6653=CARTESIAN_POINT ( 'NONE',  ( 12.06949235617739724, 12.14591786802326823, 61.87609039468568284 ) ) ;
#6654=CARTESIAN_POINT ( 'NONE',  ( -15.72974639402197994, 15.80617190586746368, 65.62390960531436690 ) ) ;
#6655=CARTESIAN_POINT ( 'NONE',  ( -16.46253265017146816, -9.564922557961047289, 19.16775706135233293 ) ) ;
#6656=CARTESIAN_POINT ( 'NONE',  ( -5.153800228976328057, -19.02544592524343514, 67.29057627198102409 ) ) ;
#6657=CARTESIAN_POINT ( 'NONE',  ( 16.51473224551069308, 9.474510206698969483, 104.1655762719810241 ) ) ;
#6658=CARTESIAN_POINT ( 'NONE',  ( 19.05341960407611168, 5.049401038298154454, 88.95724293864769550 ) ) ;
#6660=CARTESIAN_POINT ( 'NONE',  ( -19.05341960407617563, 5.049401038297882671, 63.54275706135234003 ) ) ;
#6661=CARTESIAN_POINT ( 'NONE',  ( -10.72451020669898014, 18.67979575497178502, 50.41557627198103120 ) ) ;
#6662=CARTESIAN_POINT ( 'NONE',  ( 16.52544592524342804, -4.483927247898539470, 23.54057627198102765 ) ) ;
#6663=CARTESIAN_POINT ( 'NONE',  ( -16.46253265017146816, -9.564922557961047289, 104.1677570613523329 ) ) ;
#6664=CARTESIAN_POINT ( 'NONE',  ( 9.474510206698971260, -16.51473224551069308, 22.91557627198102765 ) ) ;
#6665=CARTESIAN_POINT ( 'NONE',  ( 19.02544592524334988, 5.153800228976608722, 101.4594237280189759 ) ) ;
#6666=CARTESIAN_POINT ( 'NONE',  ( 5.823673210054125526, 21.52544592524343514, 84.79057627198102409 ) ) ;
#6667=CARTESIAN_POINT ( 'NONE',  ( -13.97604488694547697, 13.89961937509957934, 53.12609039468565442 ) ) ;
#6668=CARTESIAN_POINT ( 'NONE',  ( 17.26172910966779739, 6.454744622555832478, 106.6935309135077432 ) ) ;
#6669=CARTESIAN_POINT ( 'NONE',  ( -13.97604488694527625, -13.89961937509977652, 51.87390960531436690 ) ) ;
#6670=CARTESIAN_POINT ( 'NONE',  ( 12.14591786802309770, 12.06949235617756955, 64.37390960531435269 ) ) ;
#6671=CARTESIAN_POINT ( 'NONE',  ( 19.03943276465977164, -0.05219959533909143690, 43.74890960531435979 ) ) ;
#6672=CARTESIAN_POINT ( 'NONE',  ( -8.314922557960811034, -14.29746914071050412, 57.08224293864769550 ) ) ;
#6674=CARTESIAN_POINT ( 'NONE',  ( -16.53943276465976808, 0.05219959533911058130, 26.24890960531435624 ) ) ;
#6675=CARTESIAN_POINT ( 'NONE',  ( 9.564922557960805705, 16.46253265017160317, 64.58224293864769550 ) ) ;
#6676=CARTESIAN_POINT ( 'NONE',  ( -17.72517630440429670, 5.500000000000146549, 50.92175719257211597 ) ) ;
#6677=CARTESIAN_POINT ( 'NONE',  ( 13.89961937509957401, 13.97604488694547697, 31.87609039468566863 ) ) ;
#6678=CARTESIAN_POINT ( 'NONE',  ( 8.224510206698742110, 14.34966873604972548, 42.08442372801901854 ) ) ;
#6679=CARTESIAN_POINT ( 'NONE',  ( -18.62759615963270932, 10.81492255796079327, 55.83224293864770260 ) ) ;
#6680=CARTESIAN_POINT ( 'NONE',  ( 18.62759615963255655, 10.81492255796105972, 106.6677570613523756 ) ) ;
#6682=CARTESIAN_POINT ( 'NONE',  ( -0.05219959533909027116, -19.03943276465977164, 57.49890960531435979 ) ) ;
#6684=CARTESIAN_POINT ( 'NONE',  ( 5.049401038298161559, -19.05341960407611168, 102.7072429386476955 ) ) ;
#6685=CARTESIAN_POINT ( 'NONE',  ( -17.60691670004650433, -5.500000000000067502, 44.13333313366439370 ) ) ;
#6686=CARTESIAN_POINT ( 'NONE',  ( 18.67979575497194134, -10.72451020669871369, 25.83442372801901499 ) ) ;
#6687=CARTESIAN_POINT ( 'NONE',  ( 12.06949235617757843, -12.14591786802309237, 98.12390960531436690 ) ) ;
#6688=CARTESIAN_POINT ( 'NONE',  ( -5.823673210054116645, -21.52544592524344225, 87.29057627198103830 ) ) ;
#6689=CARTESIAN_POINT ( 'NONE',  ( 16.46253265017160672, -9.564922557960803928, 88.33224293864769550 ) ) ;
#6690=CARTESIAN_POINT ( 'NONE',  ( -19.02544592524342804, 5.153800228976336051, 91.04057627198100988 ) ) ;
#6691=CARTESIAN_POINT ( 'NONE',  ( 5.823673210054125526, 21.52544592524343514, 114.7905762719810383 ) ) ;
#6693=CARTESIAN_POINT ( 'NONE',  ( 19.03943276465977164, -0.05219959533909143690, 68.74890960531436690 ) ) ;
#6694=CARTESIAN_POINT ( 'NONE',  ( 18.22780087662122384, -5.500000000000022204, 96.01540105326108687 ) ) ;
#6695=CARTESIAN_POINT ( 'NONE',  ( -8.224510206698948167, 14.34966873604960824, 100.4155762719810241 ) ) ;
#6696=CARTESIAN_POINT ( 'NONE',  ( 19.02544592524343514, -5.153800228976328945, 38.54057627198103120 ) ) ;
#6697=CARTESIAN_POINT ( 'NONE',  ( 13.97604488694548053, -13.89961937509957401, 95.62609039468563310 ) ) ;
#6698=CARTESIAN_POINT ( 'NONE',  ( 16.53943276465976808, -0.05219959533910856209, 108.7489096053143669 ) ) ;
#6699=CARTESIAN_POINT ( 'NONE',  ( 15.80617190586769283, -15.72974639402175789, 75.62609039468567573 ) ) ;
#6700=CARTESIAN_POINT ( 'NONE',  ( 9.474510206698971260, -16.51473224551069308, 57.91557627198103120 ) ) ;
#6701=CARTESIAN_POINT ( 'NONE',  ( 10.72451020669871369, 18.67979575497193778, 37.08442372801901143 ) ) ;
#6702=CARTESIAN_POINT ( 'NONE',  ( -5.719274019375978568, 21.55341960407610458, 105.2072429386477097 ) ) ;
#6704=CARTESIAN_POINT ( 'NONE',  ( 5.153800228976335163, 19.02544592524342804, 69.79057627198103830 ) ) ;
#6706=CARTESIAN_POINT ( 'NONE',  ( -4.483927247898782831, 16.52544592524335698, 32.70942372801900433 ) ) ;
#6707=CARTESIAN_POINT ( 'NONE',  ( 18.67979575497178502, 10.72451020669898547, 29.16557627198103120 ) ) ;
#6708=CARTESIAN_POINT ( 'NONE',  ( -5.823673210054431948, 21.52544592524334988, 62.70942372801902565 ) ) ;
#6709=CARTESIAN_POINT ( 'NONE',  ( 19.02544592524343514, -5.153800228976328945, 113.5405762719810241 ) ) ;
#6710=CARTESIAN_POINT ( 'NONE',  ( 9.474510206698729675, 16.51473224551082808, 92.08442372801900433 ) ) ;
#6711=CARTESIAN_POINT ( 'NONE',  ( -9.564922557960796823, -16.46253265017161027, 52.08224293864768839 ) ) ;
#6712=CARTESIAN_POINT ( 'NONE',  ( 5.153800228976335163, 19.02544592524342804, 74.79057627198103830 ) ) ;
#6713=CARTESIAN_POINT ( 'NONE',  ( -12.06949235617756955, 12.14591786802309770, 100.6239096053143811 ) ) ;
#6714=CARTESIAN_POINT ( 'NONE',  ( 16.51473224551069308, 9.474510206698969483, 104.1655762719810241 ) ) ;
#6715=CARTESIAN_POINT ( 'NONE',  ( 16.55341960407611168, 4.379528057220329451, 88.95724293864769550 ) ) ;
#6716=CARTESIAN_POINT ( 'NONE',  ( 19.03943276465977164, -0.05219959533909143690, 103.7489096053143669 ) ) ;
#6717=CARTESIAN_POINT ( 'NONE',  ( -8.314922557960811034, -14.29746914071050412, 57.08224293864769550 ) ) ;
#6718=CARTESIAN_POINT ( 'NONE',  ( -16.51473224551069308, -9.474510206698971260, 36.66557627198102409 ) ) ;
#6719=CARTESIAN_POINT ( 'NONE',  ( -18.62759615963255300, -10.81492255796106328, 64.16775706135234714 ) ) ;
#6720=CARTESIAN_POINT ( 'NONE',  ( 16.51473224551083163, -9.474510206698727899, 95.83442372801900433 ) ) ;
#6721=CARTESIAN_POINT ( 'NONE',  ( 0.05219959533910956823, 16.53943276465976808, 54.99890960531435269 ) ) ;
#6722=CARTESIAN_POINT ( 'NONE',  ( -21.55341960407610458, -5.719274019375992779, 111.4572429386476813 ) ) ;
#6723=CARTESIAN_POINT ( 'NONE',  ( -21.55341960407610458, -5.719274019375992779, 46.45724293864769550 ) ) ;
#6724=CARTESIAN_POINT ( 'NONE',  ( -19.03943276465977164, 0.05219959533909376836, 106.2489096053143669 ) ) ;
#6725=CARTESIAN_POINT ( 'NONE',  ( 12.06949235617757843, -12.14591786802309237, 83.12390960531436690 ) ) ;
#6727=CARTESIAN_POINT ( 'NONE',  ( -19.05341960407611168, -5.049401038298163336, 56.45724293864768129 ) ) ;
#6728=CARTESIAN_POINT ( 'NONE',  ( 16.55341960407611168, 4.379528057220329451, 23.95724293864769550 ) ) ;
#6729=CARTESIAN_POINT ( 'NONE',  ( 8.224510206698742110, 14.34966873604972548, 97.08442372801904696 ) ) ;
#6730=CARTESIAN_POINT ( 'NONE',  ( 16.55341960407618274, -4.379528057220086978, 81.04275706135236135 ) ) ;
#6731=CARTESIAN_POINT ( 'NONE',  ( -13.89961937509957401, -13.97604488694547875, 44.37609039468566863 ) ) ;
#6733=CARTESIAN_POINT ( 'NONE',  ( 16.46253265017160672, -9.564922557960803928, 93.33224293864769550 ) ) ;
#6734=CARTESIAN_POINT ( 'NONE',  ( 9.564922557960805705, 16.46253265017160317, 49.58224293864770260 ) ) ;
#6735=CARTESIAN_POINT ( 'NONE',  ( -14.34966873604960291, -8.224510206698953496, 61.66557627198103120 ) ) ;
#6737=CARTESIAN_POINT ( 'NONE',  ( -9.564922557960796823, -16.46253265017161027, 107.0822429386476955 ) ) ;
#6738=CARTESIAN_POINT ( 'NONE',  ( -15.72974639402197994, 15.80617190586746368, 40.62390960531435269 ) ) ;
#6739=CARTESIAN_POINT ( 'NONE',  ( -16.55341960407611168, -4.379528057220339221, 91.45724293864769550 ) ) ;
#6740=CARTESIAN_POINT ( 'NONE',  ( -16.52544592524335698, -4.483927247898792601, 43.95942372801902565 ) ) ;
#6741=CARTESIAN_POINT ( 'NONE',  ( 12.14591786802309770, 12.06949235617756955, 84.37390960531438111 ) ) ;
#6743=CARTESIAN_POINT ( 'NONE',  ( -18.22780087662121673, -5.500000000000063061, 51.48459894673893444 ) ) ;
#6744=CARTESIAN_POINT ( 'NONE',  ( 13.89961937509957401, 13.97604488694547697, 71.87609039468567573 ) ) ;
#6745=CARTESIAN_POINT ( 'NONE',  ( 13.89961937509977652, -13.97604488694527269, 103.1239096053143527 ) ) ;
#6746=CARTESIAN_POINT ( 'NONE',  ( -19.02544592524334988, -5.153800228976617603, 73.95942372801900433 ) ) ;
#6748=CARTESIAN_POINT ( 'NONE',  ( 16.52544592524335698, 4.483927247898782831, 26.45942372801901854 ) ) ;
#6749=CARTESIAN_POINT ( 'NONE',  ( -14.34966873604972548, 8.224510206698743886, 113.3344237280190328 ) ) ;
#6750=CARTESIAN_POINT ( 'NONE',  ( -0.05219959533936034679, 19.03943276465977164, 72.50109039468566152 ) ) ;
#6751=CARTESIAN_POINT ( 'NONE',  ( 21.52544592524344225, -5.823673210054117533, 33.54057627198102409 ) ) ;
#6752=CARTESIAN_POINT ( 'NONE',  ( -21.53943276465977519, -0.05219959533937600094, 73.75109039468567573 ) ) ;
#6754=CARTESIAN_POINT ( 'NONE',  ( 16.53943276465976808, 0.05219959533934440121, 26.25109039468567573 ) ) ;
#6755=CARTESIAN_POINT ( 'NONE',  ( 13.89961937509977652, -13.97604488694527269, 28.12390960531435624 ) ) ;
#6756=CARTESIAN_POINT ( 'NONE',  ( -13.97604488694527625, -13.89961937509977652, 86.87390960531436690 ) ) ;
#6757=CARTESIAN_POINT ( 'NONE',  ( 19.05341960407611168, 5.049401038298154454, 23.95724293864769194 ) ) ;
#6758=CARTESIAN_POINT ( 'NONE',  ( -14.34966873604960291, -8.224510206698953496, 86.66557627198102409 ) ) ;
#6759=CARTESIAN_POINT ( 'NONE',  ( -19.03943276465977164, 0.05219959533909376836, 86.24890960531436690 ) ) ;
#6761=CARTESIAN_POINT ( 'NONE',  ( -9.564922557960796823, -16.46253265017161027, 82.08224293864768129 ) ) ;
#6762=ORIENTED_EDGE ( 'NONE', *, *, #100373, .T. ) ;
#6763=CARTESIAN_POINT ( 'NONE',  ( 13.89961937509957401, 13.97604488694547697, 91.87609039468567573 ) ) ;
#6764=CARTESIAN_POINT ( 'NONE',  ( -18.67979575497178146, -10.72451020669898902, 81.66557627198103830 ) ) ;
#6765=CARTESIAN_POINT ( 'NONE',  ( -16.46253265017160317, 9.564922557960807481, 40.83224293864769550 ) ) ;
#6766=CARTESIAN_POINT ( 'NONE',  ( -19.05341960407617563, 5.049401038297882671, 73.54275706135233293 ) ) ;
#6767=CARTESIAN_POINT ( 'NONE',  ( 21.55341960407610458, 5.719274019375980345, 113.9572429386477239 ) ) ;
#6768=CARTESIAN_POINT ( 'NONE',  ( -0.05219959533909027116, -19.03943276465977164, 72.49890960531435269 ) ) ;
#6769=CARTESIAN_POINT ( 'NONE',  ( -19.02544592524342804, 5.153800228976336051, 111.0405762719810099 ) ) ;
#6770=EDGE_LOOP ( 'NONE', ( #148749, #114399 ) ) ;
#6771=CARTESIAN_POINT ( 'NONE',  ( -16.53943276465976808, -0.05219959533934237506, 38.75109039468567573 ) ) ;
#6772=CARTESIAN_POINT ( 'NONE',  ( 5.719274019375991003, -21.55341960407610458, 102.7072429386476955 ) ) ;
#6773=CARTESIAN_POINT ( 'NONE',  ( 14.34966873604960469, 8.224510206698951720, 109.1655762719810383 ) ) ;
#6774=CARTESIAN_POINT ( 'NONE',  ( -9.564922557960796823, -16.46253265017161027, 87.08224293864769550 ) ) ;
#6775=CARTESIAN_POINT ( 'NONE',  ( -9.564922557961040184, 16.46253265017147172, 57.91775706135233293 ) ) ;
#6776=CARTESIAN_POINT ( 'NONE',  ( 18.62759615963271287, -10.81492255796078972, 88.33224293864769550 ) ) ;
#6777=CARTESIAN_POINT ( 'NONE',  ( 0.05219959533907565091, 21.53943276465977519, 69.99890960531435269 ) ) ;
#6778=CARTESIAN_POINT ( 'NONE',  ( -16.52544592524342804, 4.483927247898546575, 51.04057627198103120 ) ) ;
#6779=CARTESIAN_POINT ( 'NONE',  ( -5.823673210054431948, 21.52544592524334988, 112.7094237280190328 ) ) ;
#6780=CARTESIAN_POINT ( 'NONE',  ( 0.05219959533934541429, -16.53943276465976808, 60.00109039468568284 ) ) ;
#6781=CARTESIAN_POINT ( 'NONE',  ( 5.049401038298161559, -19.05341960407611168, 97.70724293864766707 ) ) ;
#6782=CARTESIAN_POINT ( 'NONE',  ( 5.153800228976335163, 19.02544592524342804, 49.79057627198100988 ) ) ;
#6783=CARTESIAN_POINT ( 'NONE',  ( 15.72974639402176855, 15.80617190586768217, 56.87609039468568994 ) ) ;
#6784=CARTESIAN_POINT ( 'NONE',  ( 15.80617190586769283, -15.72974639402175789, 65.62609039468568994 ) ) ;
#6785=CARTESIAN_POINT ( 'NONE',  ( -19.02544592524342804, 5.153800228976336051, 61.04057627198103120 ) ) ;
#6786=CARTESIAN_POINT ( 'NONE',  ( -18.67979575497193778, 10.72451020669871902, 38.33442372801900433 ) ) ;
#6787=CARTESIAN_POINT ( 'NONE',  ( 19.03943276465977164, 0.05219959533936151252, 71.25109039468566152 ) ) ;
#6788=CARTESIAN_POINT ( 'NONE',  ( -19.03943276465977164, -0.05219959533935918106, 68.75109039468566152 ) ) ;
#6789=CARTESIAN_POINT ( 'NONE',  ( 9.474510206698971260, -16.51473224551069308, 32.91557627198102409 ) ) ;
#6790=CARTESIAN_POINT ( 'NONE',  ( 14.34966873604972726, -8.224510206698740333, 90.83442372801901854 ) ) ;
#6791=CARTESIAN_POINT ( 'NONE',  ( 13.89961937509977652, -13.97604488694527269, 58.12390960531436690 ) ) ;
#6793=CARTESIAN_POINT ( 'NONE',  ( 19.05341960407611168, 5.049401038298154454, 98.95724293864766707 ) ) ;
#6794=CARTESIAN_POINT ( 'NONE',  ( 13.89961937509977652, -13.97604488694527269, 38.12390960531436690 ) ) ;
#6796=CARTESIAN_POINT ( 'NONE',  ( 10.81492255796078972, 18.62759615963270932, 84.58224293864769550 ) ) ;
#6797=CARTESIAN_POINT ( 'NONE',  ( 8.314922557961029526, -14.29746914071037800, 55.41775706135234714 ) ) ;
#6798=CARTESIAN_POINT ( 'NONE',  ( 5.823673210054444382, -21.52544592524334988, 110.2094237280190185 ) ) ;
#6799=CARTESIAN_POINT ( 'NONE',  ( 16.51473224551069308, 9.474510206698969483, 59.16557627198102409 ) ) ;
#6800=CARTESIAN_POINT ( 'NONE',  ( -14.34966873604960291, -8.224510206698953496, 51.66557627198102409 ) ) ;
#6801=CARTESIAN_POINT ( 'NONE',  ( 16.55341960407611168, 4.379528057220329451, 78.95724293864769550 ) ) ;
#6802=CARTESIAN_POINT ( 'NONE',  ( 13.97604488694527802, 13.89961937509977652, 84.37390960531433848 ) ) ;
#6803=CARTESIAN_POINT ( 'NONE',  ( -5.719274019375665041, -21.55341960407619695, 39.79275706135235424 ) ) ;
#6804=CARTESIAN_POINT ( 'NONE',  ( 5.153800228976335163, 19.02544592524342804, 89.79057627198102409 ) ) ;
#6805=CARTESIAN_POINT ( 'NONE',  ( 15.72974639402176855, 15.80617190586768217, 96.87609039468568994 ) ) ;
#6806=CARTESIAN_POINT ( 'NONE',  ( -14.34966873604972548, 8.224510206698743886, 78.33442372801901854 ) ) ;
#6807=CARTESIAN_POINT ( 'NONE',  ( -5.823673210054431948, 21.52544592524334988, 27.70942372801901854 ) ) ;
#6808=CARTESIAN_POINT ( 'NONE',  ( -19.03943276465977164, 0.05219959533909376836, 111.2489096053143669 ) ) ;
#6809=CARTESIAN_POINT ( 'NONE',  ( 0.05219959533907565091, 21.53943276465977519, 84.99890960531436690 ) ) ;
#6810=CARTESIAN_POINT ( 'NONE',  ( 16.53943276465976808, -0.05219959533910856209, 53.74890960531437401 ) ) ;
#6811=CARTESIAN_POINT ( 'NONE',  ( 13.89961937509977652, -13.97604488694527269, 38.12390960531436690 ) ) ;
#6812=CARTESIAN_POINT ( 'NONE',  ( 16.52544592524342804, -4.483927247898539470, 73.54057627198102409 ) ) ;
#6813=CARTESIAN_POINT ( 'NONE',  ( -21.55341960407610458, -5.719274019375992779, 26.45724293864768839 ) ) ;
#6814=CARTESIAN_POINT ( 'NONE',  ( 13.97604488694548053, -13.89961937509957401, 30.62609039468566863 ) ) ;
#6815=CARTESIAN_POINT ( 'NONE',  ( 16.55341960407611168, 4.379528057220329451, 93.95724293864770971 ) ) ;
#6816=CARTESIAN_POINT ( 'NONE',  ( -9.564922557960796823, -16.46253265017161027, 112.0822429386476955 ) ) ;
#6818=CARTESIAN_POINT ( 'NONE',  ( -4.379528057220086978, -16.55341960407618274, 49.79275706135234714 ) ) ;
#6819=CARTESIAN_POINT ( 'NONE',  ( -19.02544592524342804, 5.153800228976336051, 61.04057627198103120 ) ) ;
#6821=CARTESIAN_POINT ( 'NONE',  ( 12.14591786802327356, -12.06949235617739191, 95.62609039468568994 ) ) ;
#6822=CARTESIAN_POINT ( 'NONE',  ( -19.03943276465977164, -0.05219959533935918106, 103.7510903946856757 ) ) ;
#6823=CARTESIAN_POINT ( 'NONE',  ( 10.72451020669871369, 18.67979575497193778, 77.08442372801901854 ) ) ;
#6824=CARTESIAN_POINT ( 'NONE',  ( -13.89961937509977652, 13.97604488694528158, 75.62390960531438111 ) ) ;
#6825=CARTESIAN_POINT ( 'NONE',  ( 10.81492255796078972, 18.62759615963270932, 109.5822429386476955 ) ) ;
#6826=CARTESIAN_POINT ( 'NONE',  ( -0.05219959533934338120, 16.53943276465976808, 57.50109039468568994 ) ) ;
#6827=CARTESIAN_POINT ( 'NONE',  ( 5.049401038298161559, -19.05341960407611168, 22.70724293864769194 ) ) ;
#6828=CARTESIAN_POINT ( 'NONE',  ( -16.51473224551082808, 9.474510206698731452, 113.3344237280190043 ) ) ;
#6829=CARTESIAN_POINT ( 'NONE',  ( 16.46253265017146816, 9.564922557961045513, 81.66775706135233293 ) ) ;
#6830=CARTESIAN_POINT ( 'NONE',  ( -21.53943276465977519, 0.05219959533907696930, 81.24890960531436690 ) ) ;
#6831=CARTESIAN_POINT ( 'NONE',  ( -0.05219959533936034679, 19.03943276465977164, 57.50109039468566863 ) ) ;
#6832=CARTESIAN_POINT ( 'NONE',  ( -13.97604488694527625, -13.89961937509977652, 111.8739096053143243 ) ) ;
#6833=CARTESIAN_POINT ( 'NONE',  ( 10.81492255796078972, 18.62759615963270932, 104.5822429386477097 ) ) ;
#6835=CARTESIAN_POINT ( 'NONE',  ( -19.03943276465977164, 0.05219959533909376836, 71.24890960531435269 ) ) ;
#6836=DIRECTION ( 'NONE',  ( -1.000000000000000000, 0.000000000000000000, 0.000000000000000000 ) ) ;
#6837=CARTESIAN_POINT ( 'NONE',  ( -0.05219959533936034679, 19.03943276465977164, 112.5010903946856757 ) ) ;
#6839=CARTESIAN_POINT ( 'NONE',  ( -0.05219959533937732626, 21.53943276465977519, 57.50109039468568994 ) ) ;
#6840=CARTESIAN_POINT ( 'NONE',  ( -21.55341960407610458, -5.719274019375992779, 106.4572429386477097 ) ) ;
#6841=CARTESIAN_POINT ( 'NONE',  ( 16.53943276465976808, -0.05219959533910856209, 68.74890960531435269 ) ) ;
#6842=CARTESIAN_POINT ( 'NONE',  ( -5.049401038298153566, 19.05341960407611168, 75.20724293864769550 ) ) ;
#6843=CARTESIAN_POINT ( 'NONE',  ( -15.80617190586768217, 15.72974639402176855, 68.12609039468567573 ) ) ;
#6844=CARTESIAN_POINT ( 'NONE',  ( 12.14591786802327356, -12.06949235617739191, 30.62609039468567929 ) ) ;
#6845=CARTESIAN_POINT ( 'NONE',  ( -19.05341960407617563, 5.049401038297882671, 33.54275706135231871 ) ) ;
#6846=CARTESIAN_POINT ( 'NONE',  ( 21.52544592524334988, 5.823673210054432836, 56.45942372801902565 ) ) ;
#6847=CARTESIAN_POINT ( 'NONE',  ( 10.72451020669898902, -18.67979575497178502, 112.9155762719810383 ) ) ;
#6848=CARTESIAN_POINT ( 'NONE',  ( 15.80617190586746368, 15.72974639402197994, 64.37390960531435269 ) ) ;
#6849=CARTESIAN_POINT ( 'NONE',  ( -16.46253265017146816, -9.564922557961047289, 99.16775706135233293 ) ) ;
#6850=CARTESIAN_POINT ( 'NONE',  ( -16.51473224551082808, 9.474510206698731452, 68.33442372801900433 ) ) ;
#6851=CARTESIAN_POINT ( 'NONE',  ( -18.62759615963255300, -10.81492255796106328, 89.16775706135236135 ) ) ;
#6852=CARTESIAN_POINT ( 'NONE',  ( -0.05219959533936034679, 19.03943276465977164, 57.50109039468566863 ) ) ;
#6853=CARTESIAN_POINT ( 'NONE',  ( -19.05341960407611168, -5.049401038298163336, 31.45724293864769550 ) ) ;
#6854=CARTESIAN_POINT ( 'NONE',  ( -21.53943276465977519, 0.05219959533907696930, 51.24890960531436690 ) ) ;
#6855=CARTESIAN_POINT ( 'NONE',  ( -16.52544592524342804, 4.483927247898546575, 46.04057627198103830 ) ) ;
#6856=CARTESIAN_POINT ( 'NONE',  ( -19.02130022317636104, 5.499999999999802824, 95.78188669246574705 ) ) ;
#6857=CARTESIAN_POINT ( 'NONE',  ( -16.51473224551082808, 9.474510206698731452, 33.33442372801899722 ) ) ;
#6858=CARTESIAN_POINT ( 'NONE',  ( -14.34966873604972548, 8.224510206698743886, 88.33442372801901854 ) ) ;
#6859=CARTESIAN_POINT ( 'NONE',  ( -16.52544592524342804, 4.483927247898546575, 56.04057627198102409 ) ) ;
#6860=CARTESIAN_POINT ( 'NONE',  ( 21.53943276465977519, 0.05219959533937863772, 81.25109039468568994 ) ) ;
#6861=CARTESIAN_POINT ( 'NONE',  ( 5.823673210054444382, -21.52544592524334988, 80.20942372801901854 ) ) ;
#6862=CARTESIAN_POINT ( 'NONE',  ( -21.53943276465977519, 0.05219959533907696930, 81.24890960531436690 ) ) ;
#6863=CARTESIAN_POINT ( 'NONE',  ( 9.474510206698971260, -16.51473224551069308, 37.91557627198102409 ) ) ;
#6864=CARTESIAN_POINT ( 'NONE',  ( 21.53943276465977519, 0.05219959533937863772, 51.25109039468568994 ) ) ;
#6865=CARTESIAN_POINT ( 'NONE',  ( 0.05219959533909260263, 19.03943276465977164, 39.99890960531436690 ) ) ;
#6866=CARTESIAN_POINT ( 'NONE',  ( -5.153800228976328057, -19.02544592524343514, 47.29057627198102409 ) ) ;
#6867=CARTESIAN_POINT ( 'NONE',  ( -14.29746914071049879, 8.314922557960819915, 110.8322429386476955 ) ) ;
#6868=CARTESIAN_POINT ( 'NONE',  ( 9.564922557960805705, 16.46253265017160317, 104.5822429386476955 ) ) ;
#6869=CARTESIAN_POINT ( 'NONE',  ( -4.379528057220328563, 16.55341960407611168, 40.20724293864769550 ) ) ;
#6870=CARTESIAN_POINT ( 'NONE',  ( 0.05219959533910956823, 16.53943276465976808, 114.9989096053143669 ) ) ;
#6871=CARTESIAN_POINT ( 'NONE',  ( -18.62759615963270932, 10.81492255796079327, 85.83224293864768129 ) ) ;
#6872=CARTESIAN_POINT ( 'NONE',  ( 21.53943276465977519, 0.05219959533937863772, 21.25109039468567218 ) ) ;
#6874=CARTESIAN_POINT ( 'NONE',  ( -16.55341960407617563, 4.379528057220093196, 33.54275706135234714 ) ) ;
#6877=CARTESIAN_POINT ( 'NONE',  ( 21.52544592524344225, -5.823673210054117533, 73.54057627198102409 ) ) ;
#6878=CARTESIAN_POINT ( 'NONE',  ( -10.81492255796105439, 18.62759615963255655, 97.91775706135236135 ) ) ;
#6879=CARTESIAN_POINT ( 'NONE',  ( 9.564922557960805705, 16.46253265017160317, 89.58224293864769550 ) ) ;
#6880=CARTESIAN_POINT ( 'NONE',  ( 21.52544592524334988, 5.823673210054432836, 36.45942372801901143 ) ) ;
#6881=CARTESIAN_POINT ( 'NONE',  ( -21.52544592524343514, 5.823673210054127303, 26.04057627198103475 ) ) ;
#6882=CARTESIAN_POINT ( 'NONE',  ( 14.29746914071037800, 8.314922557961029526, 86.66775706135234714 ) ) ;
#6883=CARTESIAN_POINT ( 'NONE',  ( -21.52544592524334988, -5.823673210054445271, 78.95942372801901854 ) ) ;
#6884=CARTESIAN_POINT ( 'NONE',  ( -9.474510206698720793, -16.51473224551083518, 19.58442372801899722 ) ) ;
#6885=CARTESIAN_POINT ( 'NONE',  ( -8.314922557961024197, 14.29746914071037800, 72.91775706135234714 ) ) ;
#6886=CARTESIAN_POINT ( 'NONE',  ( -21.55341960407619339, 5.719274019375674811, 23.54275706135235424 ) ) ;
#6887=CARTESIAN_POINT ( 'NONE',  ( -9.564922557960796823, -16.46253265017161027, 37.08224293864768839 ) ) ;
#6888=CARTESIAN_POINT ( 'NONE',  ( 15.80617190586769283, -15.72974639402175789, 100.6260903946857184 ) ) ;
#6889=CARTESIAN_POINT ( 'NONE',  ( -5.153800228976328057, -19.02544592524343514, 112.2905762719810099 ) ) ;
#6890=CARTESIAN_POINT ( 'NONE',  ( 15.72974639402199770, -15.80617190586745480, 98.12390960531436690 ) ) ;
#6891=CARTESIAN_POINT ( 'NONE',  ( 17.97161686094262123, -5.499999999999981348, 88.49637206859249261 ) ) ;
#6892=CARTESIAN_POINT ( 'NONE',  ( -21.53943276465977519, 0.05219959533907696930, 61.24890960531435979 ) ) ;
#6893=CARTESIAN_POINT ( 'NONE',  ( -4.379528057220086978, -16.55341960407618274, 54.79275706135235424 ) ) ;
#6894=CARTESIAN_POINT ( 'NONE',  ( -8.224510206698948167, 14.34966873604960824, 50.41557627198103120 ) ) ;
#6895=CARTESIAN_POINT ( 'NONE',  ( 19.15291303114473820, -5.500000000000005329, 101.3916229363312311 ) ) ;
#6896=CARTESIAN_POINT ( 'NONE',  ( 5.153800228976615827, -19.02544592524334988, 75.20942372801896170 ) ) ;
#6897=CARTESIAN_POINT ( 'NONE',  ( -16.38665767535054485, 7.295008042176108987, 105.2640086421455266 ) ) ;
#6898=CARTESIAN_POINT ( 'NONE',  ( -0.05219959533934338120, 16.53943276465976808, 32.50109039468568284 ) ) ;
#6899=CARTESIAN_POINT ( 'NONE',  ( 18.62759615963271287, -10.81492255796078972, 93.33224293864769550 ) ) ;
#6900=CARTESIAN_POINT ( 'NONE',  ( 16.55341960407611168, 4.379528057220329451, 58.95724293864770971 ) ) ;
#6901=CARTESIAN_POINT ( 'NONE',  ( 19.05341960407611168, 5.049401038298154454, 98.95724293864766707 ) ) ;
#6902=CARTESIAN_POINT ( 'NONE',  ( 0.05219959533934541429, -16.53943276465976808, 50.00109039468568994 ) ) ;
#6903=CARTESIAN_POINT ( 'NONE',  ( 13.89961937509977652, -13.97604488694527269, 53.12390960531434558 ) ) ;
#6904=CARTESIAN_POINT ( 'NONE',  ( -18.67979575497193778, 10.72451020669871902, 28.33442372801902209 ) ) ;
#6905=CARTESIAN_POINT ( 'NONE',  ( -5.049401038297874678, -19.05341960407617918, 94.79275706135230450 ) ) ;
#6907=CARTESIAN_POINT ( 'NONE',  ( -13.89961937509977652, 13.97604488694528158, 90.62390960531432427 ) ) ;
#6908=CARTESIAN_POINT ( 'NONE',  ( -19.02544592524342804, 5.153800228976336051, 91.04057627198100988 ) ) ;
#6909=CARTESIAN_POINT ( 'NONE',  ( 15.80617190586746368, 15.72974639402197994, 89.37390960531435269 ) ) ;
#6910=CARTESIAN_POINT ( 'NONE',  ( -0.05219959533909027116, -19.03943276465977164, 52.49890960531436690 ) ) ;
#6912=CARTESIAN_POINT ( 'NONE',  ( -16.55341960407611168, -4.379528057220339221, 66.45724293864768129 ) ) ;
#6913=CARTESIAN_POINT ( 'NONE',  ( -0.05219959533909027116, -19.03943276465977164, 97.49890960531436690 ) ) ;
#6915=CARTESIAN_POINT ( 'NONE',  ( -16.51473224551082808, 9.474510206698731452, 83.33442372801899012 ) ) ;
#6916=CARTESIAN_POINT ( 'NONE',  ( -21.52544592524343514, 5.823673210054127303, 86.04057627198102409 ) ) ;
#6917=CARTESIAN_POINT ( 'NONE',  ( 5.153800228976615827, -19.02544592524334988, 50.20942372801897591 ) ) ;
#6918=CARTESIAN_POINT ( 'NONE',  ( 21.53943276465977519, -0.05219959533907433946, 23.74890960531435269 ) ) ;
#6919=CARTESIAN_POINT ( 'NONE',  ( 18.09867054820430710, 5.500000000000001776, 76.48393025253584199 ) ) ;
#6920=CARTESIAN_POINT ( 'NONE',  ( -10.81492255796078084, -18.62759615963271287, 42.08224293864769550 ) ) ;
#6921=CARTESIAN_POINT ( 'NONE',  ( 16.46253265017160672, -9.564922557960803928, 83.33224293864768129 ) ) ;
#6922=CARTESIAN_POINT ( 'NONE',  ( -15.80617190586768217, 15.72974639402176855, 68.12609039468567573 ) ) ;
#6923=CARTESIAN_POINT ( 'NONE',  ( 13.97604488694527802, 13.89961937509977652, 34.37390960531436690 ) ) ;
#6924=CARTESIAN_POINT ( 'NONE',  ( -14.34966873604960291, -8.224510206698953496, 71.66557627198100988 ) ) ;
#6925=CARTESIAN_POINT ( 'NONE',  ( -19.03943276465977164, -0.05219959533935918106, 113.7510903946856757 ) ) ;
#6926=CARTESIAN_POINT ( 'NONE',  ( -5.823673210054431948, 21.52544592524334988, 52.70942372801902565 ) ) ;
#6927=VERTEX_POINT ( 'NONE', #148083 ) ;
#6928=CARTESIAN_POINT ( 'NONE',  ( 16.51473224551069308, 9.474510206698969483, 109.1655762719810383 ) ) ;
#6929=CARTESIAN_POINT ( 'NONE',  ( -13.97604488694547697, 13.89961937509957934, 78.12609039468567573 ) ) ;
#6931=CARTESIAN_POINT ( 'NONE',  ( -5.719274019375665041, -21.55341960407619695, 24.79275706135235779 ) ) ;
#6933=CARTESIAN_POINT ( 'NONE',  ( 21.55341960407619695, -5.719274019375665929, 111.0427570613523613 ) ) ;
#6934=CARTESIAN_POINT ( 'NONE',  ( -5.049401038298153566, 19.05341960407611168, 50.20724293864770260 ) ) ;
#6935=CARTESIAN_POINT ( 'NONE',  ( 21.55341960407619695, -5.719274019375665929, 111.0427570613523613 ) ) ;
#6936=CARTESIAN_POINT ( 'NONE',  ( 16.53943276465976808, 0.05219959533934440121, 106.2510903946856757 ) ) ;
#6937=CARTESIAN_POINT ( 'NONE',  ( 16.46253265017160672, -9.564922557960803928, 98.33224293864769550 ) ) ;
#6938=CARTESIAN_POINT ( 'NONE',  ( -5.719274019375665041, -21.55341960407619695, 74.79275706135234714 ) ) ;
#6940=CARTESIAN_POINT ( 'NONE',  ( -17.72696623605162713, 5.499999999999965361, 98.59811031808418136 ) ) ;
#6942=CARTESIAN_POINT ( 'NONE',  ( -5.823673210054431948, 21.52544592524334988, 72.70942372801901854 ) ) ;
#6943=CARTESIAN_POINT ( 'NONE',  ( -18.67979575497193778, 10.72451020669871902, 108.3344237280190185 ) ) ;
#6945=CARTESIAN_POINT ( 'NONE',  ( -5.049401038298153566, 19.05341960407611168, 90.20724293864766707 ) ) ;
#6946=CARTESIAN_POINT ( 'NONE',  ( -16.46253265017146816, -9.564922557961047289, 24.16775706135233648 ) ) ;
#6948=CARTESIAN_POINT ( 'NONE',  ( -9.474510206698964154, 16.51473224551069663, 35.41557627198102409 ) ) ;
#6949=CARTESIAN_POINT ( 'NONE',  ( 21.55341960407610458, 5.719274019375980345, 53.95724293864770260 ) ) ;
#6950=CARTESIAN_POINT ( 'NONE',  ( 16.55341960407618274, -4.379528057220086978, 106.0427570613523471 ) ) ;
#6951=CARTESIAN_POINT ( 'NONE',  ( 8.224510206698953496, -14.34966873604960469, 102.9155762719810383 ) ) ;
#6952=CARTESIAN_POINT ( 'NONE',  ( -16.51473224551069308, -9.474510206698971260, 81.66557627198103830 ) ) ;
#6953=CARTESIAN_POINT ( 'NONE',  ( -18.67979575497193778, 10.72451020669871902, 103.3344237280190043 ) ) ;
#6954=CARTESIAN_POINT ( 'NONE',  ( -16.51473224551069308, -9.474510206698971260, 41.66557627198103120 ) ) ;
#6955=CARTESIAN_POINT ( 'NONE',  ( 4.483927247898545687, 16.52544592524342804, 89.79057627198103830 ) ) ;
#6956=CARTESIAN_POINT ( 'NONE',  ( -15.72974639402176322, -15.80617190586768395, 49.37609039468569705 ) ) ;
#6957=CARTESIAN_POINT ( 'NONE',  ( -15.80617190586745835, -15.72974639402198527, 86.87390960531438111 ) ) ;
#6958=CARTESIAN_POINT ( 'NONE',  ( -5.049401038297874678, -19.05341960407617918, 49.79275706135231871 ) ) ;
#6960=CARTESIAN_POINT ( 'NONE',  ( -9.564922557960796823, -16.46253265017161027, 92.08224293864769550 ) ) ;
#6961=CARTESIAN_POINT ( 'NONE',  ( 14.29746914071049879, -8.314922557960816363, 63.33224293864770260 ) ) ;
#6962=CARTESIAN_POINT ( 'NONE',  ( 13.89961937509957401, 13.97604488694547697, 46.87609039468565442 ) ) ;
#6963=CARTESIAN_POINT ( 'NONE',  ( 19.03943276465977164, -0.05219959533909143690, 53.74890960531436690 ) ) ;
#6964=CARTESIAN_POINT ( 'NONE',  ( 12.06949235617757843, -12.14591786802309237, 43.12390960531435269 ) ) ;
#6965=CARTESIAN_POINT ( 'NONE',  ( 5.049401038297881783, 19.05341960407617563, 82.29275706135229029 ) ) ;
#6967=CARTESIAN_POINT ( 'NONE',  ( 0.05219959533907565091, 21.53943276465977519, 39.99890960531436690 ) ) ;
#6968=CARTESIAN_POINT ( 'NONE',  ( -16.52544592524342804, 4.483927247898546575, 96.04057627198102409 ) ) ;
#6969=CARTESIAN_POINT ( 'NONE',  ( -17.49999999999996447, -4.013004640162789904, 24.55394279005590619 ) ) ;
#6970=CARTESIAN_POINT ( 'NONE',  ( 19.03943276465977164, -0.05219959533909143690, 58.74890960531435979 ) ) ;
#6971=CARTESIAN_POINT ( 'NONE',  ( 15.80617190586746368, 15.72974639402197994, 54.37390960531435979 ) ) ;
#6972=CARTESIAN_POINT ( 'NONE',  ( -19.02544592524342804, 5.153800228976336051, 36.04057627198100988 ) ) ;
#6973=CARTESIAN_POINT ( 'NONE',  ( -12.06949235617739369, -12.14591786802326823, 79.37609039468567573 ) ) ;
#6974=CARTESIAN_POINT ( 'NONE',  ( 13.97604488694527802, 13.89961937509977652, 54.37390960531435979 ) ) ;
#6975=CARTESIAN_POINT ( 'NONE',  ( 9.474510206698729675, 16.51473224551082808, 37.08442372801899722 ) ) ;
#6976=CARTESIAN_POINT ( 'NONE',  ( 5.823673210054444382, -21.52544592524334988, 70.20942372801904696 ) ) ;
#6977=CARTESIAN_POINT ( 'NONE',  ( -15.80617190586745835, -15.72974639402198527, 51.87390960531437401 ) ) ;
#6978=CARTESIAN_POINT ( 'NONE',  ( 19.05341960407611168, 5.049401038298154454, 28.95724293864769550 ) ) ;
#6980=CARTESIAN_POINT ( 'NONE',  ( 13.89961937509957401, 13.97604488694547697, 106.8760903946856757 ) ) ;
#6981=CARTESIAN_POINT ( 'NONE',  ( 0.05219959533909260263, 19.03943276465977164, 24.99890960531435269 ) ) ;
#6983=CARTESIAN_POINT ( 'NONE',  ( 10.72451020669898902, -18.67979575497178502, 42.91557627198103120 ) ) ;
#6984=CARTESIAN_POINT ( 'NONE',  ( 16.36317988757059894, -7.306389748694922304, 66.59789608363222158 ) ) ;
#6985=CARTESIAN_POINT ( 'NONE',  ( 15.72974639402176855, 15.80617190586768217, 81.87609039468568994 ) ) ;
#6986=CARTESIAN_POINT ( 'NONE',  ( 14.34966873604960469, 8.224510206698951720, 49.16557627198102409 ) ) ;
#6987=CARTESIAN_POINT ( 'NONE',  ( -12.14591786802309592, -12.06949235617757132, 61.87390960531436690 ) ) ;
#6988=CARTESIAN_POINT ( 'NONE',  ( 18.62759615963271287, -10.81492255796078972, 78.33224293864770971 ) ) ;
#6989=CARTESIAN_POINT ( 'NONE',  ( -5.719274019375978568, 21.55341960407610458, 80.20724293864769550 ) ) ;
#6991=CARTESIAN_POINT ( 'NONE',  ( 0.05219959533907565091, 21.53943276465977519, 29.99890960531435979 ) ) ;
#6992=CARTESIAN_POINT ( 'NONE',  ( -14.34966873604972548, 8.224510206698743886, 48.33442372801902565 ) ) ;
#6993=CARTESIAN_POINT ( 'NONE',  ( 16.55341960407611168, 4.379528057220329451, 78.95724293864769550 ) ) ;
#6994=CARTESIAN_POINT ( 'NONE',  ( -5.153800228976328057, -19.02544592524343514, 27.29057627198103120 ) ) ;
#6996=CARTESIAN_POINT ( 'NONE',  ( -16.55341960407617563, 4.379528057220093196, 78.54275706135236135 ) ) ;
#6997=CARTESIAN_POINT ( 'NONE',  ( 5.719274019375673035, 21.55341960407619339, 22.29275706135235069 ) ) ;
#6998=CARTESIAN_POINT ( 'NONE',  ( 9.474510206698971260, -16.51473224551069308, 87.91557627198102409 ) ) ;
#6999=CARTESIAN_POINT ( 'NONE',  ( -5.823673210054431948, 21.52544592524334988, 57.70942372801901143 ) ) ;
#7000=CARTESIAN_POINT ( 'NONE',  ( -19.02544592524342804, 5.153800228976336051, 116.0405762719810383 ) ) ;
#7003=CARTESIAN_POINT ( 'NONE',  ( 10.81492255796106328, -18.62759615963255655, 50.41775706135235424 ) ) ;
#7004=CARTESIAN_POINT ( 'NONE',  ( 5.153800228976335163, 19.02544592524342804, 34.79057627198102409 ) ) ;
#7005=CARTESIAN_POINT ( 'NONE',  ( -5.049401038298153566, 19.05341960407611168, 105.2072429386476671 ) ) ;
#7006=CARTESIAN_POINT ( 'NONE',  ( 5.153800228976615827, -19.02544592524334988, 55.20942372801899722 ) ) ;
#7007=CARTESIAN_POINT ( 'NONE',  ( 18.67979575497194134, -10.72451020669871369, 30.83442372801902209 ) ) ;
#7008=CARTESIAN_POINT ( 'NONE',  ( 19.05341960407617918, -5.049401038297876454, 46.04275706135233293 ) ) ;
#7009=CARTESIAN_POINT ( 'NONE',  ( -5.153800228976328057, -19.02544592524343514, 27.29057627198103120 ) ) ;
#7010=CARTESIAN_POINT ( 'NONE',  ( 16.53943276465976808, 0.05219959533934440121, 96.25109039468568994 ) ) ;
#7011=CARTESIAN_POINT ( 'NONE',  ( -16.51473224551082808, 9.474510206698731452, 63.33442372801900433 ) ) ;
#7012=CARTESIAN_POINT ( 'NONE',  ( -14.29746914071037622, -8.314922557961029526, 99.16775706135234714 ) ) ;
#7014=CARTESIAN_POINT ( 'NONE',  ( 0.05219959533909260263, 19.03943276465977164, 84.99890960531436690 ) ) ;
#7015=CARTESIAN_POINT ( 'NONE',  ( -21.52544592524334988, -5.823673210054445271, 98.95942372801903275 ) ) ;
#7016=CARTESIAN_POINT ( 'NONE',  ( 21.52544592524334988, 5.823673210054432836, 111.4594237280190328 ) ) ;
#7018=CARTESIAN_POINT ( 'NONE',  ( 9.564922557960805705, 16.46253265017160317, 104.5822429386476955 ) ) ;
#7019=CARTESIAN_POINT ( 'NONE',  ( -0.05219959533937732626, 21.53943276465977519, 72.50109039468568994 ) ) ;
#7020=CARTESIAN_POINT ( 'NONE',  ( 13.97604488694548053, -13.89961937509957401, 110.6260903946856615 ) ) ;
#7021=CARTESIAN_POINT ( 'NONE',  ( -5.049401038298153566, 19.05341960407611168, 80.20724293864769550 ) ) ;
#7022=CARTESIAN_POINT ( 'NONE',  ( -10.81492255796078084, -18.62759615963271287, 32.08224293864769550 ) ) ;
#7023=CARTESIAN_POINT ( 'NONE',  ( 16.46253265017160672, -9.564922557960803928, 88.33224293864769550 ) ) ;
#7024=CARTESIAN_POINT ( 'NONE',  ( -16.36317988757058828, -7.306389748694930297, 90.90210391636776421 ) ) ;
#7025=CARTESIAN_POINT ( 'NONE',  ( -16.51473224551069308, -9.474510206698971260, 76.66557627198103830 ) ) ;
#7026=CARTESIAN_POINT ( 'NONE',  ( -16.51473224551069308, -9.474510206698971260, 66.66557627198102409 ) ) ;
#7027=CARTESIAN_POINT ( 'NONE',  ( -4.379528057220086978, -16.55341960407618274, 104.7927570613523898 ) ) ;
#7029=CARTESIAN_POINT ( 'NONE',  ( 13.89961937509957401, 13.97604488694547697, 71.87609039468567573 ) ) ;
#7030=CARTESIAN_POINT ( 'NONE',  ( -19.02544592524342804, 5.153800228976336051, 91.04057627198100988 ) ) ;
#7031=CARTESIAN_POINT ( 'NONE',  ( 4.483927247898545687, 16.52544592524342804, 79.79057627198102409 ) ) ;
#7032=CARTESIAN_POINT ( 'NONE',  ( 21.53943276465977519, -0.05219959533907433946, 33.74890960531436690 ) ) ;
#7033=CARTESIAN_POINT ( 'NONE',  ( 0.05219959533909260263, 19.03943276465977164, 114.9989096053143669 ) ) ;
#7034=CARTESIAN_POINT ( 'NONE',  ( -14.29746914071049879, 8.314922557960819915, 95.83224293864770971 ) ) ;
#7036=CARTESIAN_POINT ( 'NONE',  ( 9.474510206698729675, 16.51473224551082808, 42.08442372801900433 ) ) ;
#7037=CARTESIAN_POINT ( 'NONE',  ( -16.52544592524342804, 4.483927247898546575, 31.04057627198102409 ) ) ;
#7038=CARTESIAN_POINT ( 'NONE',  ( 5.153800228976335163, 19.02544592524342804, 104.7905762719809957 ) ) ;
#7039=CARTESIAN_POINT ( 'NONE',  ( 5.823673210054444382, -21.52544592524334988, 60.20942372801902565 ) ) ;
#7040=CARTESIAN_POINT ( 'NONE',  ( -5.719274019375978568, 21.55341960407610458, 60.20724293864768839 ) ) ;
#7041=CARTESIAN_POINT ( 'NONE',  ( -15.80617190586768217, 15.72974639402176855, 33.12609039468569705 ) ) ;
#7042=CARTESIAN_POINT ( 'NONE',  ( -10.81492255796078084, -18.62759615963271287, 77.08224293864769550 ) ) ;
#7043=CARTESIAN_POINT ( 'NONE',  ( 10.81492255796106328, -18.62759615963255655, 40.41775706135234714 ) ) ;
#7044=CARTESIAN_POINT ( 'NONE',  ( 8.314922557960818139, 14.29746914071049879, 104.5822429386477097 ) ) ;
#7045=CARTESIAN_POINT ( 'NONE',  ( -19.03943276465977164, -0.05219959533935918106, 73.75109039468566152 ) ) ;
#7046=CARTESIAN_POINT ( 'NONE',  ( 16.46253265017160672, -9.564922557960803928, 48.33224293864769550 ) ) ;
#7047=CARTESIAN_POINT ( 'NONE',  ( -16.52544592524342804, 4.483927247898546575, 96.04057627198102409 ) ) ;
#7048=CARTESIAN_POINT ( 'NONE',  ( -5.153800228976328057, -19.02544592524343514, 92.29057627198099567 ) ) ;
#7049=CARTESIAN_POINT ( 'NONE',  ( -16.46253265017160317, 9.564922557960807481, 95.83224293864769550 ) ) ;
#7050=CARTESIAN_POINT ( 'NONE',  ( 4.483927247898545687, 16.52544592524342804, 114.7905762719810383 ) ) ;
#7051=CARTESIAN_POINT ( 'NONE',  ( -16.55341960407611168, -4.379528057220339221, 36.45724293864768839 ) ) ;
#7052=CARTESIAN_POINT ( 'NONE',  ( -16.52544592524335698, -4.483927247898792601, 93.95942372801903275 ) ) ;
#7053=CARTESIAN_POINT ( 'NONE',  ( -13.97604488694527625, -13.89961937509977652, 56.87390960531434558 ) ) ;
#7054=CARTESIAN_POINT ( 'NONE',  ( 13.89961937509977652, -13.97604488694527269, 23.12390960531436335 ) ) ;
#7055=CARTESIAN_POINT ( 'NONE',  ( 5.153800228976615827, -19.02544592524334988, 25.20942372801900433 ) ) ;
#7057=CARTESIAN_POINT ( 'NONE',  ( -8.314922557960811034, -14.29746914071050412, 27.08224293864769550 ) ) ;
#7059=CARTESIAN_POINT ( 'NONE',  ( -15.80617190586768217, 15.72974639402176855, 48.12609039468568284 ) ) ;
#7060=CARTESIAN_POINT ( 'NONE',  ( -9.474510206698964154, 16.51473224551069663, 115.4155762719810241 ) ) ;
#7061=CARTESIAN_POINT ( 'NONE',  ( 4.483927247898790824, -16.52544592524335698, 50.20942372801901854 ) ) ;
#7062=CARTESIAN_POINT ( 'NONE',  ( -14.34966873604960291, -8.224510206698953496, 21.66557627198102409 ) ) ;
#7063=CARTESIAN_POINT ( 'NONE',  ( 19.02544592524343514, -5.153800228976328945, 48.54057627198103120 ) ) ;
#7064=CARTESIAN_POINT ( 'NONE',  ( 12.06949235617739724, 12.14591786802326823, 91.87609039468568994 ) ) ;
#7065=CARTESIAN_POINT ( 'NONE',  ( 0.05219959533934541429, -16.53943276465976808, 20.00109039468568639 ) ) ;
#7066=CARTESIAN_POINT ( 'NONE',  ( 9.474510206698971260, -16.51473224551069308, 42.91557627198103120 ) ) ;
#7067=CARTESIAN_POINT ( 'NONE',  ( 16.53943276465976808, -0.05219959533910856209, 103.7489096053143669 ) ) ;
#7068=CARTESIAN_POINT ( 'NONE',  ( -21.55341960407610458, -5.719274019375992779, 111.4572429386476813 ) ) ;
#7069=CARTESIAN_POINT ( 'NONE',  ( -9.474510206698964154, 16.51473224551069663, 50.41557627198102409 ) ) ;
#7071=CARTESIAN_POINT ( 'NONE',  ( 19.05341960407611168, 5.049401038298154454, 108.9572429386477097 ) ) ;
#7072=CARTESIAN_POINT ( 'NONE',  ( 19.05341960407611168, 5.049401038298154454, 38.95724293864767418 ) ) ;
#7073=CARTESIAN_POINT ( 'NONE',  ( 5.153800228976335163, 19.02544592524342804, 104.7905762719809957 ) ) ;
#7075=CARTESIAN_POINT ( 'NONE',  ( -9.564922557960796823, -16.46253265017161027, 92.08224293864769550 ) ) ;
#7076=CARTESIAN_POINT ( 'NONE',  ( 10.72451020669871369, 18.67979575497193778, 42.08442372801901854 ) ) ;
#7077=CARTESIAN_POINT ( 'NONE',  ( 12.14591786802309770, 12.06949235617756955, 104.3739096053143669 ) ) ;
#7078=CARTESIAN_POINT ( 'NONE',  ( -16.51473224551069308, -9.474510206698971260, 106.6655762719810383 ) ) ;
#7079=CARTESIAN_POINT ( 'NONE',  ( -17.58332526062526213, -7.635886036038624702, 69.07665040441534643 ) ) ;
#7080=CARTESIAN_POINT ( 'NONE',  ( -16.53943276465976808, -0.05219959533934237506, 63.75109039468568284 ) ) ;
#7081=CARTESIAN_POINT ( 'NONE',  ( -5.719274019375665041, -21.55341960407619695, 89.79275706135236135 ) ) ;
#7082=CARTESIAN_POINT ( 'NONE',  ( 14.29746914071037800, 8.314922557961029526, 51.66775706135234714 ) ) ;
#7083=CARTESIAN_POINT ( 'NONE',  ( 19.03943276465977164, -0.05219959533909143690, 83.74890960531436690 ) ) ;
#7084=CARTESIAN_POINT ( 'NONE',  ( -8.224510206698735004, -14.34966873604973081, 44.58442372801901854 ) ) ;
#7085=CARTESIAN_POINT ( 'NONE',  ( -9.564922557961040184, 16.46253265017147172, 102.9177570613523329 ) ) ;
#7086=CARTESIAN_POINT ( 'NONE',  ( -16.55341960407617563, 4.379528057220093196, 78.54275706135236135 ) ) ;
#7087=CARTESIAN_POINT ( 'NONE',  ( 0.05219959533936267826, -19.03943276465977164, 95.00109039468567573 ) ) ;
#7088=CARTESIAN_POINT ( 'NONE',  ( 0.05219959533909260263, 19.03943276465977164, 79.99890960531436690 ) ) ;
#7089=CARTESIAN_POINT ( 'NONE',  ( -18.67979575497178146, -10.72451020669898902, 96.66557627198102409 ) ) ;
#7090=CARTESIAN_POINT ( 'NONE',  ( 0.05219959533910956823, 16.53943276465976808, 84.99890960531436690 ) ) ;
#7091=CARTESIAN_POINT ( 'NONE',  ( -9.564922557961040184, 16.46253265017147172, 87.91775706135233293 ) ) ;
#7092=CARTESIAN_POINT ( 'NONE',  ( -16.52544592524335698, -4.483927247898792601, 78.95942372801901854 ) ) ;
#7094=CARTESIAN_POINT ( 'NONE',  ( 9.564922557961047289, -16.46253265017146816, 75.41775706135234714 ) ) ;
#7095=CARTESIAN_POINT ( 'NONE',  ( 8.314922557960818139, 14.29746914071049879, 29.58224293864769905 ) ) ;
#7096=CARTESIAN_POINT ( 'NONE',  ( 4.379528057220339221, -16.55341960407611168, 97.70724293864772392 ) ) ;
#7097=CARTESIAN_POINT ( 'NONE',  ( 13.89961937509957401, 13.97604488694547697, 36.87609039468565442 ) ) ;
#7098=CARTESIAN_POINT ( 'NONE',  ( -17.31747979337962562, 6.344076630960745256, 38.62055131934819485 ) ) ;
#7099=CARTESIAN_POINT ( 'NONE',  ( -21.53943276465977519, 0.05219959533907696930, 116.2489096053143669 ) ) ;
#7100=CARTESIAN_POINT ( 'NONE',  ( -9.474510206698964154, 16.51473224551069663, 110.4155762719810383 ) ) ;
#7101=CARTESIAN_POINT ( 'NONE',  ( 16.46253265017160672, -9.564922557960803928, 93.33224293864769550 ) ) ;
#7102=CARTESIAN_POINT ( 'NONE',  ( 21.53943276465977519, 0.05219959533937863772, 96.25109039468568994 ) ) ;
#7103=CARTESIAN_POINT ( 'NONE',  ( -19.05341960407611168, -5.049401038298163336, 71.45724293864766707 ) ) ;
#7105=CARTESIAN_POINT ( 'NONE',  ( 10.72451020669898902, -18.67979575497178502, 42.91557627198103120 ) ) ;
#7106=CARTESIAN_POINT ( 'NONE',  ( 8.314922557960818139, 14.29746914071049879, 99.58224293864770971 ) ) ;
#7107=CARTESIAN_POINT ( 'NONE',  ( -19.05341960407611168, -5.049401038298163336, 61.45724293864769550 ) ) ;
#7108=CARTESIAN_POINT ( 'NONE',  ( -12.06949235617756955, 12.14591786802309770, 110.6239096053143669 ) ) ;
#7109=CARTESIAN_POINT ( 'NONE',  ( 5.823673210054444382, -21.52544592524334988, 30.20942372801902565 ) ) ;
#7110=CARTESIAN_POINT ( 'NONE',  ( -15.80617190586768217, 15.72974639402176855, 58.12609039468568994 ) ) ;
#7111=CARTESIAN_POINT ( 'NONE',  ( 13.89961937509977652, -13.97604488694527269, 38.12390960531436690 ) ) ;
#7112=CARTESIAN_POINT ( 'NONE',  ( 8.224510206698742110, 14.34966873604972548, 77.08442372801901854 ) ) ;
#7113=CARTESIAN_POINT ( 'NONE',  ( 21.52544592524344225, -5.823673210054117533, 113.5405762719810383 ) ) ;
#7115=CARTESIAN_POINT ( 'NONE',  ( 5.823673210054125526, 21.52544592524343514, 109.7905762719810383 ) ) ;
#7116=CARTESIAN_POINT ( 'NONE',  ( -5.049401038297874678, -19.05341960407617918, 54.79275706135234003 ) ) ;
#7117=CARTESIAN_POINT ( 'NONE',  ( -19.05341960407611168, -5.049401038298163336, 71.45724293864766707 ) ) ;
#7118=CARTESIAN_POINT ( 'NONE',  ( -0.05219959533936034679, 19.03943276465977164, 37.50109039468567573 ) ) ;
#7119=CARTESIAN_POINT ( 'NONE',  ( 21.52544592524334988, 5.823673210054432836, 76.45942372801901854 ) ) ;
#7120=CARTESIAN_POINT ( 'NONE',  ( 0.05219959533907565091, 21.53943276465977519, 74.99890960531435269 ) ) ;
#7121=CARTESIAN_POINT ( 'NONE',  ( -8.224510206698948167, 14.34966873604960824, 55.41557627198102409 ) ) ;
#7122=CARTESIAN_POINT ( 'NONE',  ( -15.72974639402176322, -15.80617190586768395, 84.37609039468570415 ) ) ;
#7123=CARTESIAN_POINT ( 'NONE',  ( -5.049401038297874678, -19.05341960407617918, 34.79275706135233293 ) ) ;
#7124=CARTESIAN_POINT ( 'NONE',  ( -12.14591786802309592, -12.06949235617757132, 66.87390960531436690 ) ) ;
#7125=CARTESIAN_POINT ( 'NONE',  ( 12.14591786802309770, 12.06949235617756955, 109.3739096053143811 ) ) ;
#7126=CARTESIAN_POINT ( 'NONE',  ( 16.46253265017146816, 9.564922557961045513, 51.66775706135233293 ) ) ;
#7127=CARTESIAN_POINT ( 'NONE',  ( -16.53943276465976808, -0.05219959533934237506, 108.7510903946857042 ) ) ;
#7128=CARTESIAN_POINT ( 'NONE',  ( 0.05219959533937995610, -21.53943276465977519, 75.00109039468568994 ) ) ;
#7129=CARTESIAN_POINT ( 'NONE',  ( 5.049401038298161559, -19.05341960407611168, 72.70724293864768129 ) ) ;
#7130=CARTESIAN_POINT ( 'NONE',  ( 13.89961937509957401, 13.97604488694547697, 46.87609039468565442 ) ) ;
#7131=CARTESIAN_POINT ( 'NONE',  ( 0.05219959533907565091, 21.53943276465977519, 54.99890960531435269 ) ) ;
#7132=CARTESIAN_POINT ( 'NONE',  ( 0.05219959533937995610, -21.53943276465977519, 45.00109039468568284 ) ) ;
#7133=CARTESIAN_POINT ( 'NONE',  ( 21.53943276465977519, -0.05219959533907433946, 103.7489096053143669 ) ) ;
#7134=CARTESIAN_POINT ( 'NONE',  ( 5.049401038297881783, 19.05341960407617563, 97.29275706135233293 ) ) ;
#7135=CARTESIAN_POINT ( 'NONE',  ( 8.314922557961029526, -14.29746914071037800, 60.41775706135235424 ) ) ;
#7137=CARTESIAN_POINT ( 'NONE',  ( -10.81492255796078084, -18.62759615963271287, 102.0822429386476955 ) ) ;
#7138=CARTESIAN_POINT ( 'NONE',  ( -4.379528057220328563, 16.55341960407611168, 90.20724293864770971 ) ) ;
#7140=CARTESIAN_POINT ( 'NONE',  ( 16.53943276465976808, 0.05219959533934440121, 21.25109039468567218 ) ) ;
#7141=CARTESIAN_POINT ( 'NONE',  ( 18.67979575497178502, 10.72451020669898547, 49.16557627198102409 ) ) ;
#7142=CARTESIAN_POINT ( 'NONE',  ( 4.483927247898790824, -16.52544592524335698, 85.20942372801901854 ) ) ;
#7144=CARTESIAN_POINT ( 'NONE',  ( -0.05219959533934338120, 16.53943276465976808, 62.50109039468568284 ) ) ;
#7145=CARTESIAN_POINT ( 'NONE',  ( 10.81492255796106328, -18.62759615963255655, 35.41775706135234003 ) ) ;
#7146=CARTESIAN_POINT ( 'NONE',  ( 10.81492255796078972, 18.62759615963270932, 64.58224293864769550 ) ) ;
#7147=CARTESIAN_POINT ( 'NONE',  ( -12.14591786802326823, 12.06949235617739902, 88.12609039468570415 ) ) ;
#7148=CARTESIAN_POINT ( 'NONE',  ( 9.474510206698971260, -16.51473224551069308, 92.91557627198103830 ) ) ;
#7149=CARTESIAN_POINT ( 'NONE',  ( 15.72974639402176855, 15.80617190586768217, 71.87609039468568994 ) ) ;
#7150=EDGE_CURVE ( 'NONE', #179366, #27205, #179436, .T. ) ;
#7151=CARTESIAN_POINT ( 'NONE',  ( -21.52544592524343514, 5.823673210054127303, 46.04057627198103830 ) ) ;
#7152=CARTESIAN_POINT ( 'NONE',  ( -21.55341960407610458, -5.719274019375992779, 31.45724293864769550 ) ) ;
#7154=CARTESIAN_POINT ( 'NONE',  ( -16.51473224551082808, 9.474510206698731452, 48.33442372801900433 ) ) ;
#7155=CARTESIAN_POINT ( 'NONE',  ( 0.05219959533934541429, -16.53943276465976808, 70.00109039468568994 ) ) ;
#7156=CARTESIAN_POINT ( 'NONE',  ( 5.823673210054125526, 21.52544592524343514, 34.79057627198103120 ) ) ;
#7158=CARTESIAN_POINT ( 'NONE',  ( -9.474510206698964154, 16.51473224551069663, 105.4155762719810383 ) ) ;
#7159=CARTESIAN_POINT ( 'NONE',  ( 8.224510206698742110, 14.34966873604972548, 112.0844237280190185 ) ) ;
#7161=CARTESIAN_POINT ( 'NONE',  ( 4.379528057220339221, -16.55341960407611168, 112.7072429386476955 ) ) ;
#7162=CARTESIAN_POINT ( 'NONE',  ( 21.52544592524344225, -5.823673210054117533, 53.54057627198103120 ) ) ;
#7163=CARTESIAN_POINT ( 'NONE',  ( -19.02544592524342804, 5.153800228976336051, 51.04057627198103120 ) ) ;
#7164=CARTESIAN_POINT ( 'NONE',  ( 8.314922557961029526, -14.29746914071037800, 95.41775706135234714 ) ) ;
#7165=CARTESIAN_POINT ( 'NONE',  ( -21.53943276465977519, -0.05219959533937600094, 28.75109039468567929 ) ) ;
#7166=CARTESIAN_POINT ( 'NONE',  ( 13.89961937509957401, 13.97604488694547697, 91.87609039468567573 ) ) ;
#7167=CARTESIAN_POINT ( 'NONE',  ( -14.29746914071049879, 8.314922557960819915, 95.83224293864770971 ) ) ;
#7168=CARTESIAN_POINT ( 'NONE',  ( 13.89961937509977652, -13.97604488694527269, 53.12390960531434558 ) ) ;
#7169=CARTESIAN_POINT ( 'NONE',  ( -0.05219959533909027116, -19.03943276465977164, 32.49890960531435979 ) ) ;
#7170=FACE_BOUND ( 'NONE', #125078, .T. ) ;
#7171=CARTESIAN_POINT ( 'NONE',  ( -13.97604488694527625, -13.89961937509977652, 71.87390960531433848 ) ) ;
#7172=CARTESIAN_POINT ( 'NONE',  ( 16.52544592524335698, 4.483927247898782831, 56.45942372801902565 ) ) ;
#7173=CARTESIAN_POINT ( 'NONE',  ( 15.80617190586769283, -15.72974639402175789, 110.6260903946857042 ) ) ;
#7174=CARTESIAN_POINT ( 'NONE',  ( 5.719274019375991003, -21.55341960407610458, 52.70724293864769550 ) ) ;
#7175=CARTESIAN_POINT ( 'NONE',  ( -12.14591786802326823, 12.06949235617739902, 73.12609039468567573 ) ) ;
#7176=CARTESIAN_POINT ( 'NONE',  ( 16.46253265017146816, 9.564922557961045513, 46.66775706135233293 ) ) ;
#7177=CARTESIAN_POINT ( 'NONE',  ( 19.03943276465977164, 0.05219959533936151252, 61.25109039468566863 ) ) ;
#7178=CARTESIAN_POINT ( 'NONE',  ( 15.80617190586769283, -15.72974639402175789, 65.62609039468568994 ) ) ;
#7179=CARTESIAN_POINT ( 'NONE',  ( -5.049401038298153566, 19.05341960407611168, 70.20724293864769550 ) ) ;
#7180=CARTESIAN_POINT ( 'NONE',  ( 16.51473224551069308, 9.474510206698969483, 34.16557627198102409 ) ) ;
#7181=CARTESIAN_POINT ( 'NONE',  ( 5.049401038297881783, 19.05341960407617563, 62.29275706135234003 ) ) ;
#7182=CARTESIAN_POINT ( 'NONE',  ( -9.474510206698964154, 16.51473224551069663, 110.4155762719810383 ) ) ;
#7183=CARTESIAN_POINT ( 'NONE',  ( -19.05341960407611168, -5.049401038298163336, 91.45724293864766707 ) ) ;
#7184=CARTESIAN_POINT ( 'NONE',  ( 16.53943276465976808, -0.05219959533910856209, 48.74890960531435979 ) ) ;
#7185=CARTESIAN_POINT ( 'NONE',  ( -5.823673210054116645, -21.52544592524344225, 42.29057627198103120 ) ) ;
#7187=CARTESIAN_POINT ( 'NONE',  ( -21.55341960407619339, 5.719274019375674811, 108.5427570613523756 ) ) ;
#7189=CARTESIAN_POINT ( 'NONE',  ( 5.049401038298161559, -19.05341960407611168, 52.70724293864767418 ) ) ;
#7190=CARTESIAN_POINT ( 'NONE',  ( -18.22780087662122028, -5.500000000000014211, 101.4845989467389273 ) ) ;
#7192=CARTESIAN_POINT ( 'NONE',  ( 12.14591786802327356, -12.06949235617739191, 70.62609039468567573 ) ) ;
#7193=CARTESIAN_POINT ( 'NONE',  ( 10.81492255796078972, 18.62759615963270932, 99.58224293864770971 ) ) ;
#7194=CARTESIAN_POINT ( 'NONE',  ( 12.06949235617757843, -12.14591786802309237, 48.12390960531436690 ) ) ;
#7195=CARTESIAN_POINT ( 'NONE',  ( -13.89961937509977652, 13.97604488694528158, 35.62390960531435269 ) ) ;
#7197=CARTESIAN_POINT ( 'NONE',  ( 5.823673210054444382, -21.52544592524334988, 35.20942372801901854 ) ) ;
#7198=CARTESIAN_POINT ( 'NONE',  ( -9.564922557961040184, 16.46253265017147172, 52.91775706135233293 ) ) ;
#7199=CARTESIAN_POINT ( 'NONE',  ( 9.474510206698971260, -16.51473224551069308, 52.91557627198102409 ) ) ;
#7200=CARTESIAN_POINT ( 'NONE',  ( -18.62759615963255300, -10.81492255796106328, 99.16775706135234714 ) ) ;
#7201=CARTESIAN_POINT ( 'NONE',  ( 16.31925111598457079, 7.325300261831539927, 97.33575461032749843 ) ) ;
#7203=CARTESIAN_POINT ( 'NONE',  ( 8.314922557960818139, 14.29746914071049879, 39.58224293864769550 ) ) ;
#7204=CARTESIAN_POINT ( 'NONE',  ( 18.39639308325437383, 5.500000000000037303, 43.98252246182197922 ) ) ;
#7205=CARTESIAN_POINT ( 'NONE',  ( -21.52544592524343514, 5.823673210054127303, 36.04057627198102409 ) ) ;
#7207=CARTESIAN_POINT ( 'NONE',  ( 19.03943276465977164, -0.05219959533909143690, 98.74890960531436690 ) ) ;
#7208=CARTESIAN_POINT ( 'NONE',  ( -8.224510206698948167, 14.34966873604960824, 85.41557627198102409 ) ) ;
#7209=CARTESIAN_POINT ( 'NONE',  ( -16.52544592524335698, -4.483927247898792601, 23.95942372801901143 ) ) ;
#7210=CARTESIAN_POINT ( 'NONE',  ( 16.52544592524335698, 4.483927247898782831, 111.4594237280190328 ) ) ;
#7212=CARTESIAN_POINT ( 'NONE',  ( 16.51473224551069308, 9.474510206698969483, 94.16557627198103830 ) ) ;
#7213=CARTESIAN_POINT ( 'NONE',  ( 5.823673210054125526, 21.52544592524343514, 104.7905762719810241 ) ) ;
#7214=CARTESIAN_POINT ( 'NONE',  ( -8.314922557961024197, 14.29746914071037800, 112.9177570613523329 ) ) ;
#7215=CARTESIAN_POINT ( 'NONE',  ( 16.51473224551069308, 9.474510206698969483, 94.16557627198103830 ) ) ;
#7216=CARTESIAN_POINT ( 'NONE',  ( -13.89961937509957401, -13.97604488694547875, 94.37609039468566152 ) ) ;
#7217=CARTESIAN_POINT ( 'NONE',  ( 18.67979575497194134, -10.72451020669871369, 110.8344237280190043 ) ) ;
#7218=CARTESIAN_POINT ( 'NONE',  ( 21.53943276465977519, -0.05219959533907433946, 93.74890960531436690 ) ) ;
#7219=CARTESIAN_POINT ( 'NONE',  ( -10.81492255796078084, -18.62759615963271287, 52.08224293864768839 ) ) ;
#7220=CARTESIAN_POINT ( 'NONE',  ( -19.02544592524342804, 5.153800228976336051, 66.04057627198103830 ) ) ;
#7221=CARTESIAN_POINT ( 'NONE',  ( -8.314922557960811034, -14.29746914071050412, 32.08224293864769550 ) ) ;
#7222=CARTESIAN_POINT ( 'NONE',  ( -16.51473224551069308, -9.474510206698971260, 76.66557627198103830 ) ) ;
#7223=ORIENTED_EDGE ( 'NONE', *, *, #175162, .T. ) ;
#7225=CARTESIAN_POINT ( 'NONE',  ( -5.049401038297874678, -19.05341960407617918, 34.79275706135233293 ) ) ;
#7226=CARTESIAN_POINT ( 'NONE',  ( -16.52544592524342804, 4.483927247898546575, 86.04057627198102409 ) ) ;
#7227=CARTESIAN_POINT ( 'NONE',  ( -15.72974639402176322, -15.80617190586768395, 24.37609039468567573 ) ) ;
#7229=CARTESIAN_POINT ( 'NONE',  ( 14.34966873604972726, -8.224510206698740333, 100.8344237280190185 ) ) ;
#7230=CARTESIAN_POINT ( 'NONE',  ( 4.379528057220339221, -16.55341960407611168, 112.7072429386476955 ) ) ;
#7231=CARTESIAN_POINT ( 'NONE',  ( 5.049401038298161559, -19.05341960407611168, 72.70724293864768129 ) ) ;
#7233=CARTESIAN_POINT ( 'NONE',  ( -5.153800228976328057, -19.02544592524343514, 22.29057627198102765 ) ) ;
#7234=CARTESIAN_POINT ( 'NONE',  ( -4.483927247898539470, -16.52544592524342804, 32.29057627198102409 ) ) ;
#7235=CARTESIAN_POINT ( 'NONE',  ( -21.55341960407619339, 5.719274019375674811, 53.54275706135234714 ) ) ;
#7237=CARTESIAN_POINT ( 'NONE',  ( 18.62759615963255655, 10.81492255796105972, 96.66775706135234714 ) ) ;
#7238=CARTESIAN_POINT ( 'NONE',  ( -9.474510206698964154, 16.51473224551069663, 45.41557627198103120 ) ) ;
#7239=CARTESIAN_POINT ( 'NONE',  ( 5.153800228976335163, 19.02544592524342804, 54.79057627198103120 ) ) ;
#7241=CARTESIAN_POINT ( 'NONE',  ( -18.62759615963255300, -10.81492255796106328, 89.16775706135236135 ) ) ;
#7242=CARTESIAN_POINT ( 'NONE',  ( -4.483927247898782831, 16.52544592524335698, 67.70942372801901854 ) ) ;
#7243=CARTESIAN_POINT ( 'NONE',  ( 10.72451020669871369, 18.67979575497193778, 87.08442372801901854 ) ) ;
#7244=CARTESIAN_POINT ( 'NONE',  ( -5.049401038298153566, 19.05341960407611168, 110.2072429386476671 ) ) ;
#7245=CARTESIAN_POINT ( 'NONE',  ( -5.049401038297874678, -19.05341960407617918, 99.79275706135234714 ) ) ;
#7246=CARTESIAN_POINT ( 'NONE',  ( -15.72974639402176322, -15.80617190586768395, 69.37609039468567573 ) ) ;
#7247=CARTESIAN_POINT ( 'NONE',  ( 8.224510206698742110, 14.34966873604972548, 42.08442372801901854 ) ) ;
#7248=CARTESIAN_POINT ( 'NONE',  ( 10.81492255796078972, 18.62759615963270932, 84.58224293864769550 ) ) ;
#7249=CARTESIAN_POINT ( 'NONE',  ( 19.05341960407617918, -5.049401038297876454, 81.04275706135231871 ) ) ;
#7250=CARTESIAN_POINT ( 'NONE',  ( -5.049401038298153566, 19.05341960407611168, 70.20724293864769550 ) ) ;
#7251=CARTESIAN_POINT ( 'NONE',  ( -0.05219959533936034679, 19.03943276465977164, 97.50109039468567573 ) ) ;
#7252=CARTESIAN_POINT ( 'NONE',  ( 0.05219959533936267826, -19.03943276465977164, 105.0010903946856615 ) ) ;
#7253=CARTESIAN_POINT ( 'NONE',  ( -16.52544592524342804, 4.483927247898546575, 46.04057627198103830 ) ) ;
#7254=CARTESIAN_POINT ( 'NONE',  ( -9.564922557961040184, 16.46253265017147172, 82.91775706135233293 ) ) ;
#7255=CARTESIAN_POINT ( 'NONE',  ( 16.52544592524335698, 4.483927247898782831, 66.45942372801903275 ) ) ;
#7256=CARTESIAN_POINT ( 'NONE',  ( -0.05219959533909027116, -19.03943276465977164, 42.49890960531435269 ) ) ;
#7257=CARTESIAN_POINT ( 'NONE',  ( -5.153800228976328057, -19.02544592524343514, 62.29057627198100988 ) ) ;
#7258=CARTESIAN_POINT ( 'NONE',  ( 14.34966873604972726, -8.224510206698740333, 65.83442372801900433 ) ) ;
#7261=CARTESIAN_POINT ( 'NONE',  ( -19.02544592524342804, 5.153800228976336051, 111.0405762719810099 ) ) ;
#7264=CARTESIAN_POINT ( 'NONE',  ( 19.03943276465977164, 0.05219959533936151252, 111.2510903946856757 ) ) ;
#7266=CARTESIAN_POINT ( 'NONE',  ( -10.81492255796078084, -18.62759615963271287, 37.08224293864768129 ) ) ;
#7267=CARTESIAN_POINT ( 'NONE',  ( -5.049401038297874678, -19.05341960407617918, 34.79275706135233293 ) ) ;
#7268=CARTESIAN_POINT ( 'NONE',  ( -16.55341960407617563, 4.379528057220093196, 33.54275706135234714 ) ) ;
#7269=CARTESIAN_POINT ( 'NONE',  ( 19.03943276465977164, -0.05219959533909143690, 28.74890960531435624 ) ) ;
#7270=CARTESIAN_POINT ( 'NONE',  ( -16.51473224551069308, -9.474510206698971260, 51.66557627198102409 ) ) ;
#7271=CARTESIAN_POINT ( 'NONE',  ( 10.72451020669898902, -18.67979575497178502, 77.91557627198102409 ) ) ;
#7272=CARTESIAN_POINT ( 'NONE',  ( -13.97604488694527625, -13.89961937509977652, 96.87390960531433848 ) ) ;
#7273=EDGE_CURVE ( 'NONE', #179892, #165007, #168212, .T. ) ;
#7274=CARTESIAN_POINT ( 'NONE',  ( -13.97604488694527625, -13.89961937509977652, 46.87390960531435979 ) ) ;
#7276=CARTESIAN_POINT ( 'NONE',  ( 9.474510206698729675, 16.51473224551082808, 82.08442372801899012 ) ) ;
#7277=CARTESIAN_POINT ( 'NONE',  ( 4.483927247898545687, 16.52544592524342804, 64.79057627198103830 ) ) ;
#7278=CARTESIAN_POINT ( 'NONE',  ( -10.81492255796078084, -18.62759615963271287, 42.08224293864769550 ) ) ;
#7279=CARTESIAN_POINT ( 'NONE',  ( 5.719274019375673035, 21.55341960407619339, 112.2927570613523471 ) ) ;
#7280=CARTESIAN_POINT ( 'NONE',  ( -15.72974639402197994, 15.80617190586746368, 100.6239096053143811 ) ) ;
#7281=CARTESIAN_POINT ( 'NONE',  ( 5.719274019375673035, 21.55341960407619339, 72.29275706135236135 ) ) ;
#7282=CARTESIAN_POINT ( 'NONE',  ( 18.67979575497194134, -10.72451020669871369, 80.83442372801901854 ) ) ;
#7283=CARTESIAN_POINT ( 'NONE',  ( -13.89961937509977652, 13.97604488694528158, 115.6239096053143669 ) ) ;
#7284=CARTESIAN_POINT ( 'NONE',  ( -12.14591786802326823, 12.06949235617739902, 103.1260903946856757 ) ) ;
#7285=CARTESIAN_POINT ( 'NONE',  ( -5.823673210054431948, 21.52544592524334988, 72.70942372801901854 ) ) ;
#7286=CARTESIAN_POINT ( 'NONE',  ( -13.97604488694527625, -13.89961937509977652, 71.87390960531433848 ) ) ;
#7287=CARTESIAN_POINT ( 'NONE',  ( 21.53943276465977519, 0.05219959533937863772, 31.25109039468568639 ) ) ;
#7288=CARTESIAN_POINT ( 'NONE',  ( -19.02544592524342804, 5.153800228976336051, 66.04057627198103830 ) ) ;
#7289=CARTESIAN_POINT ( 'NONE',  ( -8.314922557960811034, -14.29746914071050412, 77.08224293864769550 ) ) ;
#7290=CARTESIAN_POINT ( 'NONE',  ( -14.34966873604960291, -8.224510206698953496, 51.66557627198102409 ) ) ;
#7291=CARTESIAN_POINT ( 'NONE',  ( 21.55341960407610458, 5.719274019375980345, 53.95724293864770260 ) ) ;
#7292=CARTESIAN_POINT ( 'NONE',  ( 19.05341960407611168, 5.049401038298154454, 58.95724293864768129 ) ) ;
#7293=CARTESIAN_POINT ( 'NONE',  ( -18.67979575497178146, -10.72451020669898902, 76.66557627198103830 ) ) ;
#7294=CARTESIAN_POINT ( 'NONE',  ( 19.02544592524334988, 5.153800228976608722, 61.45942372801900433 ) ) ;
#7295=CARTESIAN_POINT ( 'NONE',  ( -13.89961937509957401, -13.97604488694547697, 19.37609039468566863 ) ) ;
#7296=CARTESIAN_POINT ( 'NONE',  ( 14.34966873604960469, 8.224510206698951720, 69.16557627198102409 ) ) ;
#7297=CARTESIAN_POINT ( 'NONE',  ( 15.72974639402199770, -15.80617190586745480, 38.12390960531436690 ) ) ;
#7298=ORIENTED_EDGE ( 'NONE', *, *, #35651, .T. ) ;
#7299=LINE ( 'NONE', #52807, #17240 ) ;
#7300=CARTESIAN_POINT ( 'NONE',  ( 8.224510206698742110, 14.34966873604972548, 102.0844237280190185 ) ) ;
#7302=CARTESIAN_POINT ( 'NONE',  ( -19.02544592524334988, -5.153800228976617603, 83.95942372801901854 ) ) ;
#7303=CARTESIAN_POINT ( 'NONE',  ( 14.29746914071049879, -8.314922557960816363, 73.33224293864769550 ) ) ;
#7305=CARTESIAN_POINT ( 'NONE',  ( -5.153800228976328057, -19.02544592524343514, 57.29057627198103120 ) ) ;
#7306=CARTESIAN_POINT ( 'NONE',  ( -8.314922557960811034, -14.29746914071050412, 52.08224293864768839 ) ) ;
#7307=CARTESIAN_POINT ( 'NONE',  ( -0.05219959533909027116, -19.03943276465977164, 82.49890960531436690 ) ) ;
#7308=CARTESIAN_POINT ( 'NONE',  ( -0.05219959533936034679, 19.03943276465977164, 82.50109039468567573 ) ) ;
#7309=CARTESIAN_POINT ( 'NONE',  ( -13.97604488694527625, -13.89961937509977652, 56.87390960531434558 ) ) ;
#7310=CARTESIAN_POINT ( 'NONE',  ( -19.02544592524342804, 5.153800228976336051, 81.04057627198103830 ) ) ;
#7311=CARTESIAN_POINT ( 'NONE',  ( -16.51473224551069308, -9.474510206698971260, 66.66557627198102409 ) ) ;
#7312=CARTESIAN_POINT ( 'NONE',  ( -5.823673210054116645, -21.52544592524344225, 62.29057627198102409 ) ) ;
#7313=CARTESIAN_POINT ( 'NONE',  ( -9.474510206698964154, 16.51473224551069663, 50.41557627198102409 ) ) ;
#7314=CARTESIAN_POINT ( 'NONE',  ( 10.72451020669898902, -18.67979575497178502, 52.91557627198103830 ) ) ;
#7315=CARTESIAN_POINT ( 'NONE',  ( 19.05341960407617918, -5.049401038297876454, 76.04275706135230450 ) ) ;
#7316=CARTESIAN_POINT ( 'NONE',  ( 4.483927247898545687, 16.52544592524342804, 29.79057627198102409 ) ) ;
#7318=CARTESIAN_POINT ( 'NONE',  ( -0.05219959533936034679, 19.03943276465977164, 32.50109039468566863 ) ) ;
#7319=CARTESIAN_POINT ( 'NONE',  ( 14.29746914071037800, 8.314922557961029526, 61.66775706135235424 ) ) ;
#7320=CARTESIAN_POINT ( 'NONE',  ( 14.29746914071037800, 8.314922557961029526, 96.66775706135234714 ) ) ;
#7321=CARTESIAN_POINT ( 'NONE',  ( 18.56197773271726348, -5.499999999999867661, 41.05066217314450938 ) ) ;
#7322=CARTESIAN_POINT ( 'NONE',  ( 16.52544592524335698, 4.483927247898782831, 81.45942372801900433 ) ) ;
#7323=CARTESIAN_POINT ( 'NONE',  ( 10.72451020669898902, -18.67979575497178502, 32.91557627198102409 ) ) ;
#7324=CARTESIAN_POINT ( 'NONE',  ( -9.564922557960796823, -16.46253265017161027, 37.08224293864768839 ) ) ;
#7325=CARTESIAN_POINT ( 'NONE',  ( -14.29746914071037622, -8.314922557961029526, 34.16775706135234714 ) ) ;
#7326=CARTESIAN_POINT ( 'NONE',  ( 5.049401038298161559, -19.05341960407611168, 47.70724293864770260 ) ) ;
#7327=CARTESIAN_POINT ( 'NONE',  ( -10.81492255796105439, 18.62759615963255655, 42.91775706135235424 ) ) ;
#7328=CARTESIAN_POINT ( 'NONE',  ( 8.224510206698742110, 14.34966873604972548, 47.08442372801901854 ) ) ;
#7329=CARTESIAN_POINT ( 'NONE',  ( 14.29746914071049879, -8.314922557960816363, 23.33224293864769194 ) ) ;
#7330=CARTESIAN_POINT ( 'NONE',  ( 19.02544592524343514, -5.153800228976328945, 23.54057627198102054 ) ) ;
#7331=CARTESIAN_POINT ( 'NONE',  ( -19.02544592524334988, -5.153800228976617603, 23.95942372801900078 ) ) ;
#7332=CARTESIAN_POINT ( 'NONE',  ( 5.153800228976615827, -19.02544592524334988, 110.2094237280189901 ) ) ;
#7333=CARTESIAN_POINT ( 'NONE',  ( -5.049401038297874678, -19.05341960407617918, 74.79275706135231871 ) ) ;
#7334=CARTESIAN_POINT ( 'NONE',  ( 14.34966873604960469, 8.224510206698951720, 74.16557627198102409 ) ) ;
#7335=CARTESIAN_POINT ( 'NONE',  ( -5.049401038298153566, 19.05341960407611168, 35.20724293864768839 ) ) ;
#7336=CARTESIAN_POINT ( 'NONE',  ( -13.89961937509957401, -13.97604488694547875, 69.37609039468564731 ) ) ;
#7337=CARTESIAN_POINT ( 'NONE',  ( 17.50000000000000355, -5.622605283950865562, 91.18792689403888119 ) ) ;
#7338=CARTESIAN_POINT ( 'NONE',  ( 0.05219959533937995610, -21.53943276465977519, 70.00109039468568994 ) ) ;
#7339=CARTESIAN_POINT ( 'NONE',  ( 4.483927247898790824, -16.52544592524335698, 45.20942372801901854 ) ) ;
#7341=CARTESIAN_POINT ( 'NONE',  ( -18.67979575497178146, -10.72451020669898902, 31.66557627198102054 ) ) ;
#7342=CARTESIAN_POINT ( 'NONE',  ( -8.314922557961024197, 14.29746914071037800, 27.91775706135234358 ) ) ;
#7345=CARTESIAN_POINT ( 'NONE',  ( 19.03943276465977164, -0.05219959533909143690, 38.74890960531436690 ) ) ;
#7346=CARTESIAN_POINT ( 'NONE',  ( -5.153800228976607833, 19.02544592524335343, 57.70942372801899722 ) ) ;
#7347=CARTESIAN_POINT ( 'NONE',  ( -13.97604488694527625, -13.89961937509977652, 61.87390960531435979 ) ) ;
#7348=CARTESIAN_POINT ( 'NONE',  ( -15.72974639402176322, -15.80617190586768395, 59.37609039468568284 ) ) ;
#7350=CARTESIAN_POINT ( 'NONE',  ( 10.81492255796106328, -18.62759615963255655, 100.4177570613523471 ) ) ;
#7351=CARTESIAN_POINT ( 'NONE',  ( 16.53943276465976808, -0.05219959533910856209, 28.74890960531435624 ) ) ;
#7352=CARTESIAN_POINT ( 'NONE',  ( 19.03943276465977164, -0.05219959533909143690, 28.74890960531435624 ) ) ;
#7353=CARTESIAN_POINT ( 'NONE',  ( 16.46253265017160672, -9.564922557960803928, 93.33224293864769550 ) ) ;
#7354=CARTESIAN_POINT ( 'NONE',  ( 21.55341960407619695, -5.719274019375665929, 56.04275706135235424 ) ) ;
#7355=CARTESIAN_POINT ( 'NONE',  ( 5.153800228976335163, 19.02544592524342804, 34.79057627198102409 ) ) ;
#7356=CARTESIAN_POINT ( 'NONE',  ( 15.72974639402176855, 15.80617190586768217, 56.87609039468568994 ) ) ;
#7357=CARTESIAN_POINT ( 'NONE',  ( -5.153800228976607833, 19.02544592524334988, 97.70942372801900433 ) ) ;
#7358=CARTESIAN_POINT ( 'NONE',  ( 13.97604488694527802, 13.89961937509977652, 104.3739096053143385 ) ) ;
#7359=CARTESIAN_POINT ( 'NONE',  ( -19.05341960407611168, -5.049401038298163336, 21.45724293864768839 ) ) ;
#7360=CARTESIAN_POINT ( 'NONE',  ( -5.823673210054116645, -21.52544592524344225, 107.2905762719810525 ) ) ;
#7361=CARTESIAN_POINT ( 'NONE',  ( -19.02544592524334988, -5.153800228976617603, 38.95942372801900433 ) ) ;
#7362=CARTESIAN_POINT ( 'NONE',  ( -9.564922557960796823, -16.46253265017161027, 22.08224293864768839 ) ) ;
#7363=CARTESIAN_POINT ( 'NONE',  ( -9.564922557960796823, -16.46253265017161027, 67.08224293864769550 ) ) ;
#7364=CARTESIAN_POINT ( 'NONE',  ( 16.51473224551083163, -9.474510206698727899, 100.8344237280190043 ) ) ;
#7365=CARTESIAN_POINT ( 'NONE',  ( 16.53943276465976808, -0.05219959533910856209, 68.74890960531435269 ) ) ;
#7366=CARTESIAN_POINT ( 'NONE',  ( 19.02544592524334988, 5.153800228976608722, 26.45942372801899722 ) ) ;
#7367=CARTESIAN_POINT ( 'NONE',  ( 10.81492255796078972, 18.62759615963270932, 24.58224293864768839 ) ) ;
#7368=CARTESIAN_POINT ( 'NONE',  ( -19.05341960407617563, 5.049401038297882671, 93.54275706135234714 ) ) ;
#7369=CARTESIAN_POINT ( 'NONE',  ( -0.05219959533907301413, -21.53943276465977519, 92.49890960531436690 ) ) ;
#7370=CARTESIAN_POINT ( 'NONE',  ( 10.81492255796106328, -18.62759615963255655, 40.41775706135234714 ) ) ;
#7371=CARTESIAN_POINT ( 'NONE',  ( 16.52544592524335698, 4.483927247898782831, 36.45942372801901143 ) ) ;
#7372=CARTESIAN_POINT ( 'NONE',  ( -8.314922557961024197, 14.29746914071037800, 102.9177570613523756 ) ) ;
#7373=CARTESIAN_POINT ( 'NONE',  ( 4.483927247898790824, -16.52544592524335698, 35.20942372801901854 ) ) ;
#7374=CARTESIAN_POINT ( 'NONE',  ( 10.72451020669871369, 18.67979575497193778, 52.08442372801901854 ) ) ;
#7375=CARTESIAN_POINT ( 'NONE',  ( -15.72974639402197994, 15.80617190586746368, 50.62390960531435979 ) ) ;
#7376=CARTESIAN_POINT ( 'NONE',  ( 16.46253265017160672, -9.564922557960803928, 28.33224293864769550 ) ) ;
#7378=CARTESIAN_POINT ( 'NONE',  ( 16.53943276465976808, 0.05219959533934440121, 56.25109039468568284 ) ) ;
#7380=CARTESIAN_POINT ( 'NONE',  ( -10.72451020669898014, 18.67979575497178502, 90.41557627198103830 ) ) ;
#7381=CARTESIAN_POINT ( 'NONE',  ( 8.224510206698953496, -14.34966873604960469, 32.91557627198102409 ) ) ;
#7382=CARTESIAN_POINT ( 'NONE',  ( 12.14591786802327356, -12.06949235617739191, 60.62609039468567573 ) ) ;
#7383=CARTESIAN_POINT ( 'NONE',  ( -16.46253265017146816, -9.564922557961047289, 104.1677570613523329 ) ) ;
#7384=CARTESIAN_POINT ( 'NONE',  ( 21.55341960407610458, 5.719274019375980345, 98.95724293864770971 ) ) ;
#7385=CARTESIAN_POINT ( 'NONE',  ( 0.05219959533910956823, 16.53943276465976808, 24.99890960531435624 ) ) ;
#7387=CARTESIAN_POINT ( 'NONE',  ( 14.34966873604972726, -8.224510206698740333, 75.83442372801900433 ) ) ;
#7389=( BOUNDED_SURFACE ( )  B_SPLINE_SURFACE ( 3, 2, ( 
 ( #25226, #12052, #135388, #148552, #182876, #57546, #28220, #121182, #10043, #71703, #197058, #134387, #198039, #196073, #59507, #90833, #186870, #154511, #138347, #63496, #1817, #157500, #48339, #170680, #183864, #169679, #124158, #45351, #18993, #31175, #107993, #140327, #109994, #46337, #61496, #171674, #153511, #142316, #33163, #141324, #47344, #172669, #60498, #16007, #184853, #77665, #122174, #123165, #92825, #80639, #18002, #126158, #125171, #76668, #187854, #30176, #49323, #16999, #62486, #139334, #107003, #94822, #110983, #168676, #813, #108999, #78652, #200027, #15008, #185858, #2813, #32168, #93825, #34154, #155505, #156500, #91819, #79655, #64491, #95814, #53292, #81612, #162469, #5789, #161480, #160478, #96793, #84616, #23970, #6781, #20960, #7782, #177662, #143296, #191810, #68460, #112967, #131133, #130114, #99793, #115974, #39131, #100786, #38140, #67462, #128133, #35141, #65473, #37125, #113951, #176663, #146295, #36125, #158482, #22968, #129120, #114971, #127136, #85626, #174660, #51306, #83621, #69466, #189834, #4782, #192820, #19970, #3796, #54302, #188842, #190819, #50327, #111982, #97777, #159464, #82617, #173674, #66470, #144298, #52294, #175650, #98785, #145298, #21969, #12798, #116966, #74463, #103803, #149310, #9805, #8801, #73479, #136129, #44123, #41138, #195835, #165483, #86628, #101798, #71467, #89620, #163485, #24982, #197805, #148311, #133132, #105782, #70471, #25981, #59271, #196825, #194823, #167469, #10804, #104794, #26979, #40119, #27981, #28964, #150320, #164488, #151309, #120940, #56295, #135152, #11815, #117978, #182640, #58292, #43126, #147312, #132137, #193829, #181647, #72473, #179668, #178657, #55294, #180666, #57307, #119961, #102802, #87624, #134147, #166483, #118983, #42142, #88622, #153269, #187613, #106770, #171432, #16753, #14771, #141081, #125915, #186620, #49083, #75439, #568, #139094, #121936, #156252, #30937, #78401, #94574, #137113, #198800, #77422, #172421, #31924, #90605, #152287, #47096, #140077, #184614, #168445, #93578, #155263, #110740, #1568, #62239, #13771, #199788, #154272, #183631, #17754, #92584, #63244, #79411, #60265, #45113, #123907, #29941, #124923, #91580, #76431, #108756, #48092, #46095, #138107, #109748, #32919, #61256, #2566, #185606, #122926, #107750, #15763, #169432, #170432, #64248, #81369, #113708, #160232, #19728, #34894, #145052, #126890, #115733, #21722, #114722, #20713, #146049, #33909, #127885, #158237, #189588, #95567, #96550, #143053, #192576, #191563, #99548, #175405, #50077, #161230, #3552, #22724, #190576, #35884, #4532, #157253, #83375, #84372, #130886, #51060, #82369, #52052, #173425, #188596, #66224, #176415, #111738, #112722, #7533, #174415, #97531, #54059, #18747, #159218, #69218, #6533, #144058, #80394, #5539, #53042, #36873, #67218, #37890, #142066, #98538, #128876, #65230, #68213, #129865, #165238, #180424, #86385, #104551, #41897, #73236, #89376, #12556, #151065, #11570, #40887, #101543, #8552, #38891, #10559, #87386, #150065, #58054, #9560, #70228, #134907, #102560, #103563, #72223, #39876, #74222, #193580, #119725, #26732, #163235, #27733, #135890, #196584, #197562, #162227, #149071, #25740, #88371, #133898, #24735, #59029, #55052, #181408, #42886, #148069, #177420, #100548, #166233, #23726, #85375, #195589, #57061, #131896, #147068, #117727, #116723, #178412, #71226, #132889, #164245, #194578, #118736, #56048, #179422, #79918, #49585, #17261, #1074, #126416, #64754, #20229, #111248, #33424, #43873, #32430, #187130, #105538, #81877, #94084, #170938, #3078, #172939, #109259, #124429, #34418, #13529, #5051, #96077, #4059, #110254, #35406, #120696, #78914, #47605, #140591, #182395, #186125, #155763, #143569, #80903, #189114, #188113, #136866, #50587, #90359, #112247, #141590, #125434, #2081, #167224, #157766, #173938, #28722, #63760, #171935, #19256, #62749, #75195, #48602, #65737, #95083 ),
 ( #156771, #18265, #142580, #127405, #152044, #97057, #158740, #83884, #131403, #52559, #176933, #114220, #38403, #144568, #194104, #6054, #193091, #162743, #101058, #130383, #191086, #98041, #128397, #100060, #161745, #39398, #147589, #99055, #159738, #24251, #192081, #175925, #21235, #54567, #23240, #82890, #163759, #146563, #67732, #53563, #160743, #129390, #55566, #113233, #51569, #174923, #115241, #85901, #37396, #116239, #9074, #178933, #84884, #70744, #22235, #145566, #7044, #68726, #190094, #132412, #8058, #69735, #177931, #36387, #117240, #40403, #102074, #25259, #86902, #148585, #66737, #26251, #197092, #195094, #88895, #120225, #182907, #137381, #60529, #89893, #122204, #59538, #198072, #71735, #165753, #57579, #119249, #196109, #133405, #43395, #14036, #121217, #10077, #28254, #56577, #152548, #103074, #105066, #166750, #151576, #45381, #168706, #149578, #44391, #135421, #58559, #107034, #13065, #118251, #136395, #30208, #179942, #74731, #106046, #91850, #41409, #12086, #11074, #87892, #181915, #164756, #167732, #29230, #72752, #90863, #134423, #75701, #199060, #180933, #183896, #42408, #104071, #27246, #150587, #73749, #76701, #32200, #34185, #78682, #33194, #47376, #93857, #140358, #110027, #845, #61526, #80670, #138377, #170710, #18033, #139364, #63528, #62518, #125203, #31205, #142346, #95846, #187885, #200057, #77696, #184885, #15040, #186899, #48370, #126189, #157530, #185891, #46367, #49352, #1846, #79687, #171705, #16038, #50357, #169712, #19024, #141357, #124190, #3826, #188875, #111014, #112016, #123195, #94853, #156534, #108025, #65505, #155534, #2844, #127166, #92856, #154543, #64522, #35173, #172701, #153543, #109031, #173705, #17029, #190849, #174692, #99825, #38170, #193860, #84648, #6812, #19999, #5819, #160509, #81643, #55325, #67495, #144330, #176696, #23002, #82647, #97808, #7814, #189864, #178691, #146325, #177692, #83652, #8833, #96828, #52326, #20993, #113983, #158512, #159497, #129152, #116996, #54332, #162501, #161510, #112998, #24002, #66501, #85658, #53323, #98815, #175681, #143327, #69498, #147345, #4814, #37156, #145330, #115002, #36156, #51338, #21999, #39160, #68490, #130145, #70501, #191842, #131163, #128164, #192853, #116003, #132169, #100818, #118010, #198833, #42176, #197839, #196860, #133163, #120974, #60297, #43161, #57342, #44156, #13806, #179699, #28015, #104828, #149341, #167503, #166517, #74498, #41171, #89657, #136164, #59305, #103836, #28998, #151343, #182672, #102834, #12832, #105816, #90638, #165517, #164520, #71497, #101829, #73515, #150353, #152320, #75472, #72507, #194855, #137145, #27013, #121971, #135186, #26013, #40153, #56328, #163516, #25015, #87656, #86658, #148342, #9838, #10837, #134182, #11850, #88657, #195869, #119017, #180700, #58326, #119994, #181680, #168478, #170468, #65265, #124959, #183663, #45148, #140112, #109783, #77455, #61290, #186656, #48126, #80429, #171466, #93613, #106804, #92615, #47131, #29976, #142102, #154306, #30968, #63279, #32954, #169467, #184647, #94609, #76465, #91615, #156288, #64282, #31958, #95602, #153303, #139126, #107782, #603, #14804, #46128, #15795, #3587, #141115, #49118, #17789, #199822, #110775, #138142, #172457, #1603, #185639, #62273, #122960, #79445, #33944, #123941, #108789, #155298, #2604, #16788, #78438, #125949, #187647, #157287, #18783, #115767, #81404, #4569, #85413, #50112, #5573, #177455, #176450, #66261, #147105, #128911, #84407, #83409, #19763, #7568, #8590, #129899, #144092, #130920, #100582, #127921, #114756, #191599, #35919, #173460, #111772, #34932, #175440, #161264, #112757, #37923, #99583, #38925, #160267, #146084, #143090, #97565, #189623, #51097, #188632, #22758, #174450, #6569, #145086, #96585, #159253, #69254, #192611, #82404, #36910, #98573, #20749, #67253, #113744, #158274, #190612, #21757, #54093, #162264, #23764, #68248, #126925, #52087, #53078, #131933, #25778 ),
 ( #165276, #26770, #105574, #28759, #9599, #42924, #195628, #57101, #167260, #11607, #193616, #196622, #90396, #55088, #88410, #134945, #152080, #116759, #72260, #71264, #86422, #41935, #178450, #166274, #104588, #39917, #58092, #70264, #73275, #197600, #101585, #119762, #12596, #40926, #118775, #181446, #27772, #163273, #149109, #151104, #180463, #150106, #164285, #10599, #103601, #89415, #117768, #24775, #59066, #148108, #87424, #74260, #56087, #135930, #179461, #120733, #132928, #182432, #43912, #194615, #102599, #133938, #44902, #78194, #123696, #106559, #110528, #93365, #14558, #361, #107541, #76216, #2355, #95356, #169217, #137895, #30726, #13565, #199577, #61045, #172209, #171220, #79197, #155052, #29732, #140866, #183418, #64036, #170224, #15554, #122717, #75232, #139864, #125706, #33693, #92373, #62032, #31717, #153056, #168236, #184407, #156040, #91365, #45888, #187405, #154059, #77212, #136903, #198590, #138881, #48873, #63032, #185394, #60058, #46885, #32709, #16547, #108545, #94361, #121726, #1353, #124710, #17537, #186408, #47885, #109538, #160019, #66012, #84160, #21506, #191353, #34687, #83167, #52831, #114500, #20503, #81167, #188383, #18538, #190365, #67010, #129657, #37671, #189380, #49860, #176202, #82151, #144841, #51841, #19522, #53849, #173211, #99336, #6325, #142849, #7322, #192366, #161019, #115523, #141857, #128669, #5326, #111526, #22513, #97324, #68005, #145840, #3348, #65023, #143847, #38684, #98319, #157041, #80185, #113500, #69006, #50857, #96344, #130672, #177211, #126679, #158031, #175195, #4328, #127680, #36660, #112515, #174208, #35676, #159010, #180217, #26523, #86177, #101331, #11356, #193367, #182182, #88168, #181206, #87180, #12354, #149852, #162019, #55841, #147867, #9353, #71018, #23515, #133682, #104343, #73027, #100340, #118528, #85161, #42682, #54843, #195374, #56853, #41687, #135687, #58824, #39669, #134699, #25536, #148861, #197359, #103352, #146848, #196382, #120491, #8342, #165030, #57851, #70017, #131686, #102349, #163019, #116517, #72009, #178205, #119523, #166027, #24526, #27527, #132686, #89168, #150860, #194374, #74017, #117515, #179212, #10352, #40679, #164038, #167017, #122474, #124466, #168970, #123458, #137649, #184165, #30475, #119, #91127, #151837, #170975, #28518, #60801, #108300, #29494, #153813, #152817, #15308, #121483, #32468, #186163, #77956, #90154, #14310, #74992, #169980, #76967, #136657, #140627, #185150, #44659, #92126, #199336, #106312, #94121, #13327, #198337, #59813, #138638, #139623, #75976, #31471, #16306, #155800, #61788, #1111, #183177, #45647, #167998, #107298, #105329, #62785, #46640, #93123, #154808, #47645, #109296, #17298, #78952, #2117, #63799, #125472, #43667, #3116, #173972, #171973, #65773, #97092, #159775, #114260, #37433, #66769, #99093, #36422, #143603, #79957, #67769, #7084, #190127, #4094, #191124, #160785, #64791, #174958, #51602, #96113, #175964, #113266, #21270, #126452, #98077, #82927, #144605, #50621, #111285, #18301, #48639, #20264, #158776, #6090, #129426, #19292, #141626, #52598, #112282, #22273, #81910, #49623, #83924, #188150, #145605, #68765, #172975, #187168, #110291, #33461, #95119, #156809, #5087, #35440, #34454, #157801, #127442, #80940, #142615, #189148, #128430, #120021, #14835, #74526, #130423, #192122, #89685, #59333, #27041, #10864, #136191, #197866, #30007, #121003, #43187, #53603, #42203, #196887, #118037, #91645, #103863, #180727, #12861, #182701, #119045, #134210, #44186, #26038, #179728, #105845, #13834, #181706, #45180, #41198, #88687, #57372, #150383, #102860, #195897, #165544, #153334, #90667, #198862, #167532, #149368, #60329, #164545, #122003, #151370, #135215, #11879, #87683, #29027, #183694, #72534, #73542, #104856, #152349, #58354, #166545, #28044, #75500, #137174, #106834, #168509, #30998, #154336, #34969, #199855, #155334, #65301, #125985, #15827, #96621, #78473, #33981 ),
 ( #185672, #107815, #141152, #186691, #169499, #173496, #156325, #77488, #63316, #170501, #139158, #126960, #122992, #61321, #184678, #124996, #110811, #62305, #64317, #49153, #188669, #109819, #95637, #92647, #47163, #635, #123975, #138174, #172494, #108822, #17825, #32991, #46161, #31991, #157325, #18820, #93649, #48161, #171502, #16823, #140147, #94645, #1639, #79483, #2641, #80464, #3622, #50149, #187683, #111808, #142138, #158310, #76498, #175476, #67289, #128947, #5610, #81439, #53116, #23801, #69291, #19798, #37963, #143125, #162301, #112793, #114794, #176487, #99621, #55126, #178487, #159288, #192647, #145123, #6607, #116796, #161302, #4605, #146121, #39954, #66297, #22797, #84443, #101625, #127957, #21794, #20785, #35954, #191636, #189660, #115803, #54130, #51133, #7605, #174487, #130957, #147141, #97600, #177493, #85451, #190648, #68286, #38963, #100619, #82440, #98610, #8629, #129937, #70301, #113780, #160304, #131970, #193654, #52124, #144128, #36948, #83446, #149149, #118816, #9637, #103641, #163314, #40966, #41974, #133978, #71304, #165319, #102638, #57140, #87462, #132967, #180502, #24812, #72300, #164323, #86461, #148146, #25816, #194657, #56126, #10639, #117808, #179501, #195669, #21436, #69949, #39602, #178135, #7254, #67937, #175124, #5256, #177142, #53777, #116447, #24457, #176132, #36591, #101261, #68939, #8270, #38613, #6257, #40612, #159949, #86107, #131614, #129590, #194305, #179144, #162951, #102282, #128600, #115452, #192298, #98247, #9283, #84094, #193298, #147798, #190294, #51771, #130603, #25468, #85092, #143775, #66938, #100269, #54773, #37602, #83097, #146777, #70948, #163971, #132618, #161950, #113431, #52762, #23445, #144772, #191286, #114431, #99265, #55771, #117445, #160951, #22444, #145772, #180151, #168906, #74929, #167931, #73953, #199268, #87108, #181139, #11288, #42613, #148794, #149785, #72961, #45582, #44593, #152749, #166952, #103284, #14239, #56787, #75911, #43601, #89101, #134630, #10284, #13266, #137585, #184099, #104277, #135621, #105266, #26457, #41620, #196315, #29431, #197292, #28455, #88099, #164964, #57784, #91062, #119455, #71942, #90091, #60736, #165959, #107235, #133612, #27460, #122409, #136592, #150792, #195306, #12288, #106249, #151773, #58755, #118459, #120424, #198272, #182115, #59749, #121419, #183111, #18237, #33395, #139562, #157736, #95054, #64726, #108236, #156743, #126388, #188085, #94056, #154746, #61726, #92059, #63731, #140563, #3050, #111219, #62719, #123394, #49556, #155734, #79891, #125406, #93059, #127373, #46575, #172911, #141561, #16242, #80875, #65707, #34389, #189085, #15243, #2052, #78884, #185086, #96049, #170909, #19225, #142551, #76902, #138573, #17232, #112218, #171907, #30412, #153748, #187103, #4029, #124402, #169916, #50558, #51, #31408, #77894, #48573, #1046, #186096, #110226, #47578, #109230, #32401, #49856, #111521, #21502, #192362, #37667, #188379, #6321, #173207, #130668, #81163, #83163, #144837, #68001, #23511, #146844, #127676, #161015, #113496, #175191, #85158, #129653, #34683, #114496, #8338, #96340, #191349, #52827, #70013, #158027, #190361, #189376, #4324, #160015, #19518, #142845, #66008, #98315, #36657, #50853, #53845, #128665, #176198, #115519, #112511, #174204, #99332, #35672, #22509, #97320, #159006, #84156, #145836, #82147, #20499, #7318, #69002, #143843, #177207, #38680, #5322, #67006, #51837, #100336, #162014, #148857, #193363, #11352, #57847, #117510, #132682, #42678, #24522, #13324, #119519, #12350, #118524, #43664, #131682, #25532, #55837, #87176, #54839, #194370, #179208, #90151, #89164, #197355, #73023, #147863, #58819, #101327, #120487, #88164, #133678, #40675, #116514, #181201, #182178, #28515, #10348, #180213, #149848, #71014, #86173, #102345, #74013, #9349, #178201, #134695, #135683, #164034, #151834, #39665, #72005, #105326, #104339, #195369, #163015, #56849, #150855, #196378 ),
 ( #166023, #41683, #27523, #167014, #103347, #165026, #26519, #106309, #136653, #108297, #185147, #47640, #155797, #107295, #167995, #109293, #116, #139620, #169976, #137646, #171970, #91124, #17295, #1108, #199333, #125468, #110288, #170972, #63795, #121480, #59810, #183173, #123455, #32465, #60798, #62782, #94118, #187165, #31468, #78949, #29491, #45644, #152814, #14306, #198334, #140624, #75973, #154805, #93120, #44656, #122471, #2114, #48636, #30472, #46637, #16303, #184162, #168967, #61785, #92122, #153810, #77953, #33458, #95116, #156806, #124463, #74989, #186160, #15304, #76964, #138635, #50618, #6087, #79953, #141623, #51599, #22270, #67766, #18298, #36418, #3112, #160781, #111282, #113263, #174955, #98074, #53600, #176969, #157798, #191121, #143600, #5084, #115276, #159772, #64788, #144601, #38439, #126449, #21267, #82924, #100095, #188147, #20261, #19289, #34451, #190124, #49620, #114256, #52595, #172972, #129423, #96109, #175961, #145602, #128427, #7081, #81907, #80936, #66766, #37430, #99090, #142612, #97089, #83921, #68762, #130420, #112278, #158772, #192118, #4091, #65770, #127439, #189145, #173969, #35437, #26283, #147621, #71769, #9108, #133439, #39429, #88929, #42440, #196140, #146598, #70775, #193123, #87925, #195129, #54597, #58589, #41442, #162775, #148618, #55599, #24283, #163791, #85932, #23274, #149612, #150621, #120255, #117273, #10109, #118284, #101089, #116271, #132444, #104103, #177961, #84918, #179975, #165786, #194135, #181946, #8091, #40434, #12117, #11110, #178967, #43429, #25292, #119280, #103108, #102106, #27283, #161779, #164789, #86935, #73780, #135453, #56610, #72785, #134455, #57611, #197122, #180963, #69769, #131437, #31237, #875, #139393, #168735, #29262, #136425, #166784, #138406, #15070, #77727, #185922, #137412, #198106, #62550, #30239, #169742, #200087, #167764, #1880, #121247, #47407, #92886, #90893, #155567, #140392, #124226, #63561, #89924, #76731, #153573, #59572, #170741, #45411, #154573, #109063, #151606, #13098, #91882, #186933, #46399, #105098, #28285, #61555, #16069, #199093, #182941, #108058, #32231, #125235, #93889, #123224, #74763, #14069, #184915, #17062, #44424, #122235, #106077, #78716, #152579, #75736, #60560, #183926, #107064, #130180, #36188, #129186, #35208, #160545, #48403, #142382, #172738, #3860, #110060, #111050, #34218, #6846, #5853, #114017, #128200, #64558, #175714, #18067, #37193, #4852, #190884, #173739, #189897, #65540, #188913, #96861, #66536, #95881, #156572, #98850, #171740, #127199, #113033, #157564, #158545, #19057, #20035, #126222, #22034, #52360, #82682, #33229, #80704, #79722, #174725, #81677, #141391, #145364, #51372, #49387, #143360, #50391, #112051, #83686, #94888, #2879, #187918, #97842, #144366, #159530, #21029, #67529, #68525, #27810, #152120, #84681, #162535, #69535, #131199, #53360, #28795, #192889, #74296, #151140, #115037, #177728, #13602, #75270, #147380, #42961, #104624, #54367, #7848, #181483, #176730, #70536, #166313, #167299, #121763, #44942, #135965, #106597, #43949, #182468, #38203, #89451, #24039, #105611, #99859, #161543, #12631, #198629, #90434, #191876, #197636, #23036, #136940, #146361, #59102, #120767, #60095, #29770, #153093, #116039, #183456, #119798, #168273, #91405, #14597, #39197, #76253, #100853, #85694, #8869, #132205, #196660, #58129, #139902, #77248, #154096, #109577, #199615, #33733, #110565, #107579, #2394, #96382, #79237, #65060, #47923, #126717, #1391, #45924, #63072, #64073, #95394, #61081, #16583, #80223, #30763, #122754, #94399, #141894, #15590, #158069, #184444, #78231, #188421, #187443, #138916, #19560, #124751, #157080, #156080, #92410, #18576, #137931, #140908, #155089, #3385, #111565, #397, #125743, #48911, #46923, #49898, #172246, #173249, #62069, #34724, #169256, #123734, #186447, #185433, #108583, #170260, #171260, #32748, #31754, #93403, #17576, #112553, #53886 ),
 ( #159049, #20543, #142885, #115561, #82192, #161056, #37711, #4367, #67050, #100378, #162056, #36699, #129695, #191392, #143885, #97363, #68043, #66050, #160059, #52869, #177248, #8380, #131723, #22551, #193405, #130710, #69045, #127718, #114540, #113540, #192404, #189420, #50895, #176240, #85200, #38720, #81204, #99373, #174248, #23552, #35716, #84197, #145877, #7360, #116554, #39704, #5366, #146888, #6363, #70055, #178243, #54880, #128708, #101367, #163056, #190405, #51881, #175234, #98360, #21546, #83206, #144881, #40716, #196416, #86212, #120526, #197394, #194408, #89203, #183213, #166062, #58860, #55878, #150896, #44694, #27563, #151873, #134734, #13363, #26559, #132720, #149886, #12390, #182219, #147902, #103387, #105365, #11392, #104379, #118563, #165065, #73062, #181241, #72045, #117551, #75027, #9388, #41723, #74052, #10388, #57886, #133719, #119558, #102385, #136693, #167052, #43703, #71054, #195411, #179250, #135723, #42717, #164073, #121518, #28553, #25572, #90190, #180253, #87216, #198374, #148898, #56889, #88202, #59851, #106348, #24563, #155835, #140662, #79991, #1146, #125505, #60835, #138674, #45682, #107333, #29529, #2154, #169006, #47681, #124504, #91162, #153848, #187202, #48673, #123493, #16342, #77991, #30510, #184200, #154845, #152851, #46677, #139658, #63832, #95153, #18336, #109331, #141659, #17332, #78988, #14346, #62821, #154, #110325, #76011, #137686, #186199, #172006, #33494, #168032, #171013, #199371, #156841, #122510, #32504, #94156, #3151, #64824, #126486, #92162, #188184, #93160, #49656, #15346, #77002, #61823, #185186, #108336, #170017, #31507, #176001, #193161, #96147, #113302, #50655, #127477, #82964, #173010, #7120, #52634, #111320, #34489, #67807, #37470, #5121, #189182, #114299, #99131, #8129, #160821, #21307, #157836, #20298, #174993, #191161, #146636, #128466, #19327, #22309, #83960, #97126, #144641, #80975, #129462, #142650, #53639, #4129, #6124, #145640, #68802, #69807, #131474, #112316, #130461, #36458, #98115, #65808, #192159, #174006, #115316, #35477, #158810, #177008, #38477, #81946, #143638, #159812, #66803, #190162, #100134, #51638, #161815, #23310, #84954, #119317, #13137, #196179, #181986, #164827, #43468, #56648, #162811, #180014, #181004, #12156, #177997, #133475, #135491, #41481, #134492, #148659, #195167, #103146, #11149, #102144, #24320, #105136, #39464, #71807, #42479, #40472, #26323, #163829, #87963, #132482, #166822, #197161, #88968, #101125, #25331, #85969, #104142, #149651, #147659, #151642, #57651, #55635, #72823, #10147, #117308, #28323, #9146, #70813, #194171, #165824, #150658, #86972, #27321, #73821, #89962, #58627, #120293, #179004, #118321, #74799, #136462, #116308, #54633, #137452, #77762, #154609, #59612, #183961, #17099, #78751, #153612, #108094, #45448, #169779, #75774, #125273, #140428, #32268, #182978, #107102, #29300, #62585, #31272, #90930, #94923, #139428, #199131, #184951, #91920, #60598, #186970, #44462, #106116, #167800, #46435, #93925, #168772, #185958, #170778, #110097, #92923, #155603, #152616, #30274, #122273, #15108, #121285, #1918, #76769, #911, #16104, #14107, #138441, #63597, #48440, #200122, #124263, #47443, #61591, #123259, #109099, #171775, #33264, #156608, #18103, #79757, #198142, #21065, #53395, #190919, #129222, #2915, #128234, #173776, #52396, #64593, #143398, #50427, #51406, #174758, #141428, #159567, #126257, #83720, #34256, #36224, #97876, #82721, #176765, #99892, #80740, #114055, #66569, #189931, #38237, #144402, #187954, #67564, #161577, #49424, #5888, #175752, #23070, #111085, #4887, #142418, #157600, #113066, #172775, #37229, #98886, #95915, #160580, #19091, #22069, #68559, #145399, #130216, #6881, #3897, #191911, #115073, #65577, #127236, #20069, #188950, #112086, #35242, #96896, #81713, #158580, #41240, #132239, #192923, #11919, #7883, #101902, #149409, #70571, #43231, #26080, #73583 ),
 ( #25085, #9907, #102902, #193931, #54401, #135255, #69569, #163584, #10905, #55394, #194924, #117064, #56399, #162570, #196927, #165585, #119086, #131235, #178760, #116073, #72578, #118081, #177761, #181749, #164586, #85728, #71567, #40225, #147416, #58395, #39230, #100886, #24073, #133232, #180768, #86727, #134252, #57413, #120061, #179771, #42243, #8903, #148412, #87724, #195939, #146394, #103904, #27083, #88729, #150424, #104897, #166586, #84716, #47204, #183732, #76538, #138214, #167572, #44228, #14877, #12900, #106873, #199896, #675, #155373, #78513, #107855, #140187, #77528, #15870, #89726, #61360, #60370, #139200, #151412, #30044, #137215, #123031, #184717, #28086, #46201, #74564, #170542, #121048, #169540, #31039, #92688, #63357, #186730, #29066, #62346, #153375, #154376, #125034, #124016, #136232, #185713, #48201, #197906, #108863, #32033, #109855, #59376, #91685, #90705, #105885, #93690, #182743, #16862, #1679, #152388, #13874, #75541, #198902, #122042, #45218, #168546, #145161, #49192, #159326, #174523, #80504, #98648, #35990, #5648, #110850, #97637, #67325, #128987, #35004, #95678, #2679, #33028, #4643, #81476, #144163, #52160, #3661, #64356, #190685, #96659, #20822, #66334, #34020, #68323, #187721, #113817, #82479, #157364, #21831, #6645, #175512, #129973, #156362, #143163, #19835, #126025, #36986, #111845, #160342, #83483, #17865, #79520, #158346, #53153, #112831, #171540, #94683, #127995, #191673, #65339, #172534, #141190, #18858, #142177, #126999, #189698, #188706, #50188, #51171, #173535, #150183, #132005, #176526, #84480, #195704, #130993, #38002, #25853, #7643, #196698, #102672, #57176, #101660, #26847, #114832, #8665, #38999, #70338, #99657, #177530, #100655, #73350, #72337, #180536, #194692, #192685, #42010, #146157, #103675, #71339, #116831, #162337, #161341, #41005, #165353, #11684, #193693, #163351, #133002, #54168, #69327, #23838, #118853, #115841, #22833, #56162, #88488, #85487, #135023, #147176, #55161, #178522, #164357, #39989, #24847, #86496, #134012, #117844, #148181, #87496, #9674, #179536, #149185, #10673, #137972, #93442, #75307, #119835, #27849, #138957, #74336, #181520, #169295, #151181, #139943, #45963, #436, #44979, #170300, #58168, #152157, #182507, #13640, #42999, #120808, #43987, #16622, #15630, #123774, #199654, #136002, #185473, #89490, #46963, #14635, #60134, #105648, #104666, #184484, #108622, #155129, #136978, #106639, #76294, #197673, #12669, #167337, #62111, #59138, #166351, #61120, #31793, #28834, #78270, #90475, #198667, #121802, #107617, #183495, #168312, #29808, #77287, #122794, #91444, #153132, #30801, #92450, #154138, #8173, #178039, #79277, #192201, #7163, #113343, #131517, #68846, #38520, #140947, #130505, #100176, #161858, #67845, #125781, #32786, #63111, #37509, #114338, #177050, #84997, #36500, #94438, #23352, #129500, #53683, #99171, #64116, #101167, #17618, #146678, #115360, #187483, #54676, #39507, #69849, #162855, #186488, #176041, #52675, #156119, #193203, #144680, #116350, #24362, #47964, #109616, #191200, #86013, #145681, #1433, #124789, #160861, #171300, #98154, #2434, #51681, #175035, #159854, #21347, #22351, #83005, #6165, #84002, #147702, #104184, #73862, #41527, #25374, #150699, #89008, #44501, #135531, #57694, #70855, #56691, #11192, #27362, #183017, #164871, #9190, #117352, #28363, #163875, #132524, #58665, #40516, #29340, #197202, #90001, #134536, #59651, #194213, #103190, #71850, #26366, #55678, #10190, #133519, #106157, #105175, #13175, #12197, #87016, #74838, #179048, #136501, #165866, #149694, #195211, #102187, #120331, #198181, #167839, #88006, #196224, #182026, #148702, #118365, #180058, #151683, #72867, #119362, #43509, #121325, #181046, #42521, #166861, #169818, #79793, #140466, #168811, #49458, #92962, #48477, #47480, #184003, #171812, #111120, #93962, #108134, #94959, #64629, #30315, #78789, #155642, #200160, #18139 ) ),
 .UNSPECIFIED., .T., .F., .F. ) 
 B_SPLINE_SURFACE_WITH_KNOTS ( ( 4, 3, 4 ),
 ( 3, 2, 2, 2, 2, 2, 2, 2, 2, 2, 2, 2, 2, 2, 2, 2, 2, 2, 2, 2, 2, 2, 2, 2, 2, 2, 2, 2, 2, 2, 2, 2, 2, 2, 2, 2, 2, 2, 2, 2, 2, 2, 2, 2, 2, 2, 2, 2, 2, 2, 2, 2, 2, 2, 2, 2, 2, 2, 2, 2, 2, 2, 2, 2, 2, 2, 2, 2, 2, 2, 2, 2, 2, 2, 2, 2, 2, 2, 2, 2, 2, 2, 2, 2, 2, 2, 2, 2, 2, 2, 2, 2, 2, 2, 2, 2, 2, 2, 2, 2, 2, 2, 2, 2, 2, 2, 2, 2, 2, 2, 2, 2, 2, 2, 2, 2, 2, 2, 2, 2, 2, 2, 2, 2, 2, 2, 2, 2, 2, 2, 2, 2, 2, 2, 2, 2, 2, 2, 2, 2, 2, 2, 2, 2, 2, 2, 2, 2, 2, 2, 2, 2, 2, 2, 2, 2, 2, 2, 2, 2, 2, 2, 2, 2, 2, 2, 2, 2, 2, 2, 2, 2, 2, 2, 2, 2, 2, 2, 2, 2, 2, 2, 2, 2, 2, 2, 2, 2, 2, 2, 2, 2, 2, 2, 2, 2, 2, 2, 2, 2, 2, 2, 2, 2, 2, 2, 2, 2, 2, 2, 2, 2, 2, 2, 2, 2, 2, 2, 2, 2, 2, 2, 2, 2, 2, 2, 2, 2, 3 ),
 ( 0.000000000000000000, 0.5000000000000000000, 1.000000000000000000 ),
 ( 0.000000000000000000, 0.004385964912280701511, 0.008771929824561403022, 0.01315789473684210453, 0.01754385964912280604, 0.02192982456140350755, 0.02631578947368420907, 0.03070175438596491058, 0.03508771929824561209, 0.03947368421052631360, 0.04385964912280701511, 0.04824561403508771662, 0.05263157894736841813, 0.05701754385964911964, 0.06140350877192982115, 0.06578947368421052266, 0.07017543859649122417, 0.07456140350877192569, 0.07894736842105262720, 0.08333333333333332871, 0.08771929824561403022, 0.09210526315789473173, 0.09649122807017543324, 0.1008771929824561348, 0.1052631578947368363, 0.1096491228070175378, 0.1140350877192982393, 0.1184210526315789408, 0.1228070175438596423, 0.1271929824561403577, 0.1315789473684210453, 0.1359649122807017607, 0.1403508771929824483, 0.1447368421052631637, 0.1491228070175438514, 0.1535087719298245668, 0.1578947368421052544, 0.1622807017543859698, 0.1666666666666666574, 0.1710526315789473728, 0.1754385964912280604, 0.1798245614035087758, 0.1842105263157894635, 0.1885964912280701788, 0.1929824561403508665, 0.1973684210526315819, 0.2017543859649122695, 0.2061403508771929849, 0.2105263157894736725, 0.2149122807017543879, 0.2192982456140350755, 0.2236842105263157909, 0.2280701754385964786, 0.2324561403508771940, 0.2368421052631578816, 0.2412280701754385970, 0.2456140350877192846, 0.2500000000000000000, 0.2543859649122807154, 0.2587719298245614308, 0.2631578947368420907, 0.2675438596491228060, 0.2719298245614035214, 0.2763157894736842368, 0.2807017543859648967, 0.2850877192982456121, 0.2894736842105263275, 0.2938596491228070429, 0.2982456140350877027, 0.3026315789473684181, 0.3070175438596491335, 0.3114035087719298489, 0.3157894736842105088, 0.3201754385964912242, 0.3245614035087719396, 0.3289473684210526550, 0.3333333333333333148, 0.3377192982456140302, 0.3421052631578947456, 0.3464912280701754610, 0.3508771929824561209, 0.3552631578947368363, 0.3596491228070175517, 0.3640350877192982670, 0.3684210526315789269, 0.3728070175438596423, 0.3771929824561403577, 0.3815789473684210731, 0.3859649122807017330, 0.3903508771929824483, 0.3947368421052631637, 0.3991228070175438791, 0.4035087719298245390, 0.4078947368421052544, 0.4122807017543859698, 0.4166666666666666852, 0.4210526315789473450, 0.4254385964912280604, 0.4298245614035087758, 0.4342105263157894912, 0.4385964912280701511, 0.4429824561403508665, 0.4473684210526315819, 0.4517543859649122973, 0.4561403508771929571, 0.4605263157894736725, 0.4649122807017543879, 0.4692982456140351033, 0.4736842105263157632, 0.4780701754385964786, 0.4824561403508771940, 0.4868421052631579093, 0.4912280701754385692, 0.4956140350877192846, 0.5000000000000000000, 0.5043859649122807154, 0.5087719298245614308, 0.5131578947368421462, 0.5175438596491228616, 0.5219298245614034659, 0.5263157894736841813, 0.5307017543859648967, 0.5350877192982456121, 0.5394736842105263275, 0.5438596491228070429, 0.5482456140350877583, 0.5526315789473684736, 0.5570175438596490780, 0.5614035087719297934, 0.5657894736842105088, 0.5701754385964912242, 0.5745614035087719396, 0.5789473684210526550, 0.5833333333333333703, 0.5877192982456140857, 0.5921052631578946901, 0.5964912280701754055, 0.6008771929824561209, 0.6052631578947368363, 0.6096491228070175517, 0.6140350877192982670, 0.6184210526315789824, 0.6228070175438596978, 0.6271929824561403022, 0.6315789473684210176, 0.6359649122807017330, 0.6403508771929824483, 0.6447368421052631637, 0.6491228070175438791, 0.6535087719298245945, 0.6578947368421053099, 0.6622807017543859143, 0.6666666666666666297, 0.6710526315789473450, 0.6754385964912280604, 0.6798245614035087758, 0.6842105263157894912, 0.6885964912280702066, 0.6929824561403509220, 0.6973684210526315264, 0.7017543859649122417, 0.7061403508771929571, 0.7105263157894736725, 0.7149122807017543879, 0.7192982456140351033, 0.7236842105263158187, 0.7280701754385965341, 0.7324561403508771384, 0.7368421052631578538, 0.7412280701754385692, 0.7456140350877192846, 0.7500000000000000000, 0.7543859649122807154, 0.7587719298245614308, 0.7631578947368421462, 0.7675438596491228616, 0.7719298245614034659, 0.7763157894736841813, 0.7807017543859648967, 0.7850877192982456121, 0.7894736842105263275, 0.7938596491228070429, 0.7982456140350877583, 0.8026315789473684736, 0.8070175438596490780, 0.8114035087719297934, 0.8157894736842105088, 0.8201754385964912242, 0.8245614035087719396, 0.8289473684210526550, 0.8333333333333333703, 0.8377192982456140857, 0.8421052631578946901, 0.8464912280701754055, 0.8508771929824561209, 0.8552631578947368363, 0.8596491228070175517, 0.8640350877192982670, 0.8684210526315789824, 0.8728070175438596978, 0.8771929824561403022, 0.8815789473684210176, 0.8859649122807017330, 0.8903508771929824483, 0.8947368421052631637, 0.8991228070175438791, 0.9035087719298245945, 0.9078947368421053099, 0.9122807017543859143, 0.9166666666666666297, 0.9210526315789473450, 0.9254385964912280604, 0.9298245614035087758, 0.9342105263157894912, 0.9385964912280702066, 0.9429824561403509220, 0.9473684210526315264, 0.9517543859649122417, 0.9561403508771929571, 0.9605263157894736725, 0.9649122807017543879, 0.9692982456140351033, 0.9736842105263158187, 0.9780701754385965341, 0.9824561403508771384, 0.9868421052631578538, 0.9912280701754385692, 0.9956140350877192846, 1.000000000000000000 ),
 .UNSPECIFIED. ) 
 GEOMETRIC_REPRESENTATION_ITEM ( )  RATIONAL_B_SPLINE_SURFACE ( (
 ( 1.000000000000000000, 0.9659258262890683122, 1.000000000000000000, 0.9659258262890683122, 1.000000000000000000, 0.9659258262890683122, 1.000000000000000000, 0.9659258262890683122, 1.000000000000000000, 0.9659258262890683122, 1.000000000000000000, 0.9659258262890683122, 1.000000000000000000, 0.9659258262890683122, 1.000000000000000000, 0.9659258262890683122, 1.000000000000000000, 0.9659258262890683122, 1.000000000000000000, 0.9659258262890683122, 1.000000000000000000, 0.9659258262890683122, 1.000000000000000000, 0.9659258262890683122, 1.000000000000000000, 0.9659258262890683122, 1.000000000000000000, 0.9659258262890683122, 1.000000000000000000, 0.9659258262890683122, 1.000000000000000000, 0.9659258262890683122, 1.000000000000000000, 0.9659258262890683122, 1.000000000000000000, 0.9659258262890683122, 1.000000000000000000, 0.9659258262890683122, 1.000000000000000000, 0.9659258262890683122, 1.000000000000000000, 0.9659258262890683122, 1.000000000000000000, 0.9659258262890683122, 1.000000000000000000, 0.9659258262890683122, 1.000000000000000000, 0.9659258262890683122, 1.000000000000000000, 0.9659258262890683122, 1.000000000000000000, 0.9659258262890683122, 1.000000000000000000, 0.9659258262890683122, 1.000000000000000000, 0.9659258262890683122, 1.000000000000000000, 0.9659258262890683122, 1.000000000000000000, 0.9659258262890683122, 1.000000000000000000, 0.9659258262890683122, 1.000000000000000000, 0.9659258262890683122, 1.000000000000000000, 0.9659258262890683122, 1.000000000000000000, 0.9659258262890683122, 1.000000000000000000, 0.9659258262890683122, 1.000000000000000000, 0.9659258262890683122, 1.000000000000000000, 0.9659258262890683122, 1.000000000000000000, 0.9659258262890683122, 1.000000000000000000, 0.9659258262890683122, 1.000000000000000000, 0.9659258262890683122, 1.000000000000000000, 0.9659258262890683122, 1.000000000000000000, 0.9659258262890683122, 1.000000000000000000, 0.9659258262890683122, 1.000000000000000000, 0.9659258262890683122, 1.000000000000000000, 0.9659258262890683122, 1.000000000000000000, 0.9659258262890683122, 1.000000000000000000, 0.9659258262890683122, 1.000000000000000000, 0.9659258262890683122, 1.000000000000000000, 0.9659258262890683122, 1.000000000000000000, 0.9659258262890683122, 1.000000000000000000, 0.9659258262890683122, 1.000000000000000000, 0.9659258262890683122, 1.000000000000000000, 0.9659258262890683122, 1.000000000000000000, 0.9659258262890683122, 1.000000000000000000, 0.9659258262890683122, 1.000000000000000000, 0.9659258262890683122, 1.000000000000000000, 0.9659258262890683122, 1.000000000000000000, 0.9659258262890683122, 1.000000000000000000, 0.9659258262890683122, 1.000000000000000000, 0.9659258262890683122, 1.000000000000000000, 0.9659258262890683122, 1.000000000000000000, 0.9659258262890683122, 1.000000000000000000, 0.9659258262890683122, 1.000000000000000000, 0.9659258262890683122, 1.000000000000000000, 0.9659258262890683122, 1.000000000000000000, 0.9659258262890683122, 1.000000000000000000, 0.9659258262890683122, 1.000000000000000000, 0.9659258262890683122, 1.000000000000000000, 0.9659258262890683122, 1.000000000000000000, 0.9659258262890683122, 1.000000000000000000, 0.9659258262890683122, 1.000000000000000000, 0.9659258262890683122, 1.000000000000000000, 0.9659258262890683122, 1.000000000000000000, 0.9659258262890683122, 1.000000000000000000, 0.9659258262890683122, 1.000000000000000000, 0.9659258262890683122, 1.000000000000000000, 0.9659258262890683122, 1.000000000000000000, 0.9659258262890683122, 1.000000000000000000, 0.9659258262890683122, 1.000000000000000000, 0.9659258262890683122, 1.000000000000000000, 0.9659258262890683122, 1.000000000000000000, 0.9659258262890683122, 1.000000000000000000, 0.9659258262890683122, 1.000000000000000000, 0.9659258262890683122, 1.000000000000000000, 0.9659258262890683122, 1.000000000000000000, 0.9659258262890683122, 1.000000000000000000, 0.9659258262890683122, 1.000000000000000000, 0.9659258262890683122, 1.000000000000000000, 0.9659258262890683122, 1.000000000000000000, 0.9659258262890683122, 1.000000000000000000, 0.9659258262890683122, 1.000000000000000000, 0.9659258262890683122, 1.000000000000000000, 0.9659258262890683122, 1.000000000000000000, 0.9659258262890683122, 1.000000000000000000, 0.9659258262890683122, 1.000000000000000000, 0.9659258262890683122, 1.000000000000000000, 0.9659258262890683122, 1.000000000000000000, 0.9659258262890683122, 1.000000000000000000, 0.9659258262890683122, 1.000000000000000000, 0.9659258262890683122, 1.000000000000000000, 0.9659258262890683122, 1.000000000000000000, 0.9659258262890683122, 1.000000000000000000, 0.9659258262890683122, 1.000000000000000000, 0.9659258262890683122, 1.000000000000000000, 0.9659258262890683122, 1.000000000000000000, 0.9659258262890683122, 1.000000000000000000, 0.9659258262890683122, 1.000000000000000000, 0.9659258262890683122, 1.000000000000000000, 0.9659258262890683122, 1.000000000000000000, 0.9659258262890683122, 1.000000000000000000, 0.9659258262890683122, 1.000000000000000000, 0.9659258262890683122, 1.000000000000000000, 0.9659258262890683122, 1.000000000000000000, 0.9659258262890683122, 1.000000000000000000, 0.9659258262890683122, 1.000000000000000000, 0.9659258262890683122, 1.000000000000000000, 0.9659258262890683122, 1.000000000000000000, 0.9659258262890683122, 1.000000000000000000, 0.9659258262890683122, 1.000000000000000000, 0.9659258262890683122, 1.000000000000000000, 0.9659258262890683122, 1.000000000000000000, 0.9659258262890683122, 1.000000000000000000, 0.9659258262890683122, 1.000000000000000000, 0.9659258262890683122, 1.000000000000000000, 0.9659258262890683122, 1.000000000000000000, 0.9659258262890683122, 1.000000000000000000, 0.9659258262890683122, 1.000000000000000000, 0.9659258262890683122, 1.000000000000000000, 0.9659258262890683122, 1.000000000000000000, 0.9659258262890683122, 1.000000000000000000, 0.9659258262890683122, 1.000000000000000000, 0.9659258262890683122, 1.000000000000000000, 0.9659258262890683122, 1.000000000000000000, 0.9659258262890683122, 1.000000000000000000, 0.9659258262890683122, 1.000000000000000000, 0.9659258262890683122, 1.000000000000000000, 0.9659258262890683122, 1.000000000000000000, 0.9659258262890683122, 1.000000000000000000, 0.9659258262890683122, 1.000000000000000000, 0.9659258262890683122, 1.000000000000000000, 0.9659258262890683122, 1.000000000000000000, 0.9659258262890683122, 1.000000000000000000, 0.9659258262890683122, 1.000000000000000000, 0.9659258262890683122, 1.000000000000000000, 0.9659258262890683122, 1.000000000000000000, 0.9659258262890683122, 1.000000000000000000, 0.9659258262890683122, 1.000000000000000000, 0.9659258262890683122, 1.000000000000000000, 0.9659258262890683122, 1.000000000000000000, 0.9659258262890683122, 1.000000000000000000, 0.9659258262890683122, 1.000000000000000000, 0.9659258262890683122, 1.000000000000000000, 0.9659258262890683122, 1.000000000000000000, 0.9659258262890683122, 1.000000000000000000, 0.9659258262890683122, 1.000000000000000000, 0.9659258262890683122, 1.000000000000000000, 0.9659258262890683122, 1.000000000000000000, 0.9659258262890683122, 1.000000000000000000, 0.9659258262890683122, 1.000000000000000000, 0.9659258262890683122, 1.000000000000000000, 0.9659258262890683122, 1.000000000000000000, 0.9659258262890683122, 1.000000000000000000, 0.9659258262890683122, 1.000000000000000000, 0.9659258262890683122, 1.000000000000000000, 0.9659258262890683122, 1.000000000000000000, 0.9659258262890683122, 1.000000000000000000, 0.9659258262890683122, 1.000000000000000000, 0.9659258262890683122, 1.000000000000000000, 0.9659258262890683122, 1.000000000000000000, 0.9659258262890683122, 1.000000000000000000, 0.9659258262890683122, 1.000000000000000000, 0.9659258262890683122, 1.000000000000000000, 0.9659258262890683122, 1.000000000000000000, 0.9659258262890683122, 1.000000000000000000, 0.9659258262890683122, 1.000000000000000000, 0.9659258262890683122, 1.000000000000000000, 0.9659258262890683122, 1.000000000000000000, 0.9659258262890683122, 1.000000000000000000, 0.9659258262890683122, 1.000000000000000000, 0.9659258262890683122, 1.000000000000000000, 0.9659258262890683122, 1.000000000000000000, 0.9659258262890683122, 1.000000000000000000, 0.9659258262890683122, 1.000000000000000000, 0.9659258262890683122, 1.000000000000000000, 0.9659258262890683122, 1.000000000000000000, 0.9659258262890683122, 1.000000000000000000, 0.9659258262890683122, 1.000000000000000000, 0.9659258262890683122, 1.000000000000000000, 0.9659258262890683122, 1.000000000000000000, 0.9659258262890683122, 1.000000000000000000, 0.9659258262890683122, 1.000000000000000000, 0.9659258262890683122, 1.000000000000000000, 0.9659258262890683122, 1.000000000000000000, 0.9659258262890683122, 1.000000000000000000, 0.9659258262890683122, 1.000000000000000000, 0.9659258262890683122, 1.000000000000000000, 0.9659258262890683122, 1.000000000000000000, 0.9659258262890683122, 1.000000000000000000, 0.9659258262890683122, 1.000000000000000000, 0.9659258262890683122, 1.000000000000000000, 0.9659258262890683122, 1.000000000000000000, 0.9659258262890683122, 1.000000000000000000, 0.9659258262890683122, 1.000000000000000000, 0.9659258262890683122, 1.000000000000000000, 0.9659258262890683122, 1.000000000000000000, 0.9659258262890683122, 1.000000000000000000, 0.9659258262890683122, 1.000000000000000000, 0.9659258262890683122, 1.000000000000000000, 0.9659258262890683122, 1.000000000000000000, 0.9659258262890683122, 1.000000000000000000, 0.9659258262890683122, 1.000000000000000000, 0.9659258262890683122, 1.000000000000000000, 0.9659258262890683122, 1.000000000000000000, 0.9659258262890683122, 1.000000000000000000, 0.9659258262890683122, 1.000000000000000000, 0.9659258262890683122, 1.000000000000000000, 0.9659258262890683122, 1.000000000000000000, 0.9659258262890683122, 1.000000000000000000, 0.9659258262890683122, 1.000000000000000000, 0.9659258262890683122, 1.000000000000000000, 0.9659258262890683122, 1.000000000000000000, 0.9659258262890683122, 1.000000000000000000, 0.9659258262890683122, 1.000000000000000000, 0.9659258262890683122, 1.000000000000000000, 0.9659258262890683122, 1.000000000000000000, 0.9659258262890683122, 1.000000000000000000, 0.9659258262890683122, 1.000000000000000000, 0.9659258262890683122, 1.000000000000000000),
 ( 0.3333333333333333703, 0.3219752754296894559, 0.3333333333333333703, 0.3219752754296894559, 0.3333333333333333703, 0.3219752754296894559, 0.3333333333333333703, 0.3219752754296894559, 0.3333333333333333703, 0.3219752754296894559, 0.3333333333333333703, 0.3219752754296894559, 0.3333333333333333703, 0.3219752754296894559, 0.3333333333333333703, 0.3219752754296894559, 0.3333333333333333703, 0.3219752754296894559, 0.3333333333333333703, 0.3219752754296894559, 0.3333333333333333703, 0.3219752754296894559, 0.3333333333333333703, 0.3219752754296894559, 0.3333333333333333703, 0.3219752754296894559, 0.3333333333333333703, 0.3219752754296894559, 0.3333333333333333703, 0.3219752754296894559, 0.3333333333333333703, 0.3219752754296894559, 0.3333333333333333703, 0.3219752754296894559, 0.3333333333333333703, 0.3219752754296894559, 0.3333333333333333703, 0.3219752754296894559, 0.3333333333333333703, 0.3219752754296894559, 0.3333333333333333703, 0.3219752754296894559, 0.3333333333333333703, 0.3219752754296894559, 0.3333333333333333703, 0.3219752754296894559, 0.3333333333333333703, 0.3219752754296894559, 0.3333333333333333703, 0.3219752754296894559, 0.3333333333333333703, 0.3219752754296894559, 0.3333333333333333703, 0.3219752754296894559, 0.3333333333333333703, 0.3219752754296894559, 0.3333333333333333703, 0.3219752754296894559, 0.3333333333333333703, 0.3219752754296894559, 0.3333333333333333703, 0.3219752754296894559, 0.3333333333333333703, 0.3219752754296894559, 0.3333333333333333703, 0.3219752754296894559, 0.3333333333333333703, 0.3219752754296894559, 0.3333333333333333703, 0.3219752754296894559, 0.3333333333333333703, 0.3219752754296894559, 0.3333333333333333703, 0.3219752754296894559, 0.3333333333333333703, 0.3219752754296894559, 0.3333333333333333703, 0.3219752754296894559, 0.3333333333333333703, 0.3219752754296894559, 0.3333333333333333703, 0.3219752754296894559, 0.3333333333333333703, 0.3219752754296894559, 0.3333333333333333703, 0.3219752754296894559, 0.3333333333333333703, 0.3219752754296894559, 0.3333333333333333703, 0.3219752754296894559, 0.3333333333333333703, 0.3219752754296894559, 0.3333333333333333703, 0.3219752754296894559, 0.3333333333333333703, 0.3219752754296894559, 0.3333333333333333703, 0.3219752754296894559, 0.3333333333333333703, 0.3219752754296894559, 0.3333333333333333703, 0.3219752754296894559, 0.3333333333333333703, 0.3219752754296894559, 0.3333333333333333703, 0.3219752754296894559, 0.3333333333333333703, 0.3219752754296894559, 0.3333333333333333703, 0.3219752754296894559, 0.3333333333333333703, 0.3219752754296894559, 0.3333333333333333703, 0.3219752754296894559, 0.3333333333333333703, 0.3219752754296894559, 0.3333333333333333703, 0.3219752754296894559, 0.3333333333333333703, 0.3219752754296894559, 0.3333333333333333703, 0.3219752754296894559, 0.3333333333333333703, 0.3219752754296894559, 0.3333333333333333703, 0.3219752754296894559, 0.3333333333333333703, 0.3219752754296894559, 0.3333333333333333703, 0.3219752754296894559, 0.3333333333333333703, 0.3219752754296894559, 0.3333333333333333703, 0.3219752754296894559, 0.3333333333333333703, 0.3219752754296894559, 0.3333333333333333703, 0.3219752754296894559, 0.3333333333333333703, 0.3219752754296894559, 0.3333333333333333703, 0.3219752754296894559, 0.3333333333333333703, 0.3219752754296894559, 0.3333333333333333703, 0.3219752754296894559, 0.3333333333333333703, 0.3219752754296894559, 0.3333333333333333703, 0.3219752754296894559, 0.3333333333333333703, 0.3219752754296894559, 0.3333333333333333703, 0.3219752754296894559, 0.3333333333333333703, 0.3219752754296894559, 0.3333333333333333703, 0.3219752754296894559, 0.3333333333333333703, 0.3219752754296894559, 0.3333333333333333703, 0.3219752754296894559, 0.3333333333333333703, 0.3219752754296894559, 0.3333333333333333703, 0.3219752754296894559, 0.3333333333333333703, 0.3219752754296894559, 0.3333333333333333703, 0.3219752754296894559, 0.3333333333333333703, 0.3219752754296894559, 0.3333333333333333703, 0.3219752754296894559, 0.3333333333333333703, 0.3219752754296894559, 0.3333333333333333703, 0.3219752754296894559, 0.3333333333333333703, 0.3219752754296894559, 0.3333333333333333703, 0.3219752754296894559, 0.3333333333333333703, 0.3219752754296894559, 0.3333333333333333703, 0.3219752754296894559, 0.3333333333333333703, 0.3219752754296894559, 0.3333333333333333703, 0.3219752754296894559, 0.3333333333333333703, 0.3219752754296894559, 0.3333333333333333703, 0.3219752754296894559, 0.3333333333333333703, 0.3219752754296894559, 0.3333333333333333703, 0.3219752754296894559, 0.3333333333333333703, 0.3219752754296894559, 0.3333333333333333703, 0.3219752754296894559, 0.3333333333333333703, 0.3219752754296894559, 0.3333333333333333703, 0.3219752754296894559, 0.3333333333333333703, 0.3219752754296894559, 0.3333333333333333703, 0.3219752754296894559, 0.3333333333333333703, 0.3219752754296894559, 0.3333333333333333703, 0.3219752754296894559, 0.3333333333333333703, 0.3219752754296894559, 0.3333333333333333703, 0.3219752754296894559, 0.3333333333333333703, 0.3219752754296894559, 0.3333333333333333703, 0.3219752754296894559, 0.3333333333333333703, 0.3219752754296894559, 0.3333333333333333703, 0.3219752754296894559, 0.3333333333333333703, 0.3219752754296894559, 0.3333333333333333703, 0.3219752754296894559, 0.3333333333333333703, 0.3219752754296894559, 0.3333333333333333703, 0.3219752754296894559, 0.3333333333333333703, 0.3219752754296894559, 0.3333333333333333703, 0.3219752754296894559, 0.3333333333333333703, 0.3219752754296894559, 0.3333333333333333703, 0.3219752754296894559, 0.3333333333333333703, 0.3219752754296894559, 0.3333333333333333703, 0.3219752754296894559, 0.3333333333333333703, 0.3219752754296894559, 0.3333333333333333703, 0.3219752754296894559, 0.3333333333333333703, 0.3219752754296894559, 0.3333333333333333703, 0.3219752754296894559, 0.3333333333333333703, 0.3219752754296894559, 0.3333333333333333703, 0.3219752754296894559, 0.3333333333333333703, 0.3219752754296894559, 0.3333333333333333703, 0.3219752754296894559, 0.3333333333333333703, 0.3219752754296894559, 0.3333333333333333703, 0.3219752754296894559, 0.3333333333333333703, 0.3219752754296894559, 0.3333333333333333703, 0.3219752754296894559, 0.3333333333333333703, 0.3219752754296894559, 0.3333333333333333703, 0.3219752754296894559, 0.3333333333333333703, 0.3219752754296894559, 0.3333333333333333703, 0.3219752754296894559, 0.3333333333333333703, 0.3219752754296894559, 0.3333333333333333703, 0.3219752754296894559, 0.3333333333333333703, 0.3219752754296894559, 0.3333333333333333703, 0.3219752754296894559, 0.3333333333333333703, 0.3219752754296894559, 0.3333333333333333703, 0.3219752754296894559, 0.3333333333333333703, 0.3219752754296894559, 0.3333333333333333703, 0.3219752754296894559, 0.3333333333333333703, 0.3219752754296894559, 0.3333333333333333703, 0.3219752754296894559, 0.3333333333333333703, 0.3219752754296894559, 0.3333333333333333703, 0.3219752754296894559, 0.3333333333333333703, 0.3219752754296894559, 0.3333333333333333703, 0.3219752754296894559, 0.3333333333333333703, 0.3219752754296894559, 0.3333333333333333703, 0.3219752754296894559, 0.3333333333333333703, 0.3219752754296894559, 0.3333333333333333703, 0.3219752754296894559, 0.3333333333333333703, 0.3219752754296894559, 0.3333333333333333703, 0.3219752754296894559, 0.3333333333333333703, 0.3219752754296894559, 0.3333333333333333703, 0.3219752754296894559, 0.3333333333333333703, 0.3219752754296894559, 0.3333333333333333703, 0.3219752754296894559, 0.3333333333333333703, 0.3219752754296894559, 0.3333333333333333703, 0.3219752754296894559, 0.3333333333333333703, 0.3219752754296894559, 0.3333333333333333703, 0.3219752754296894559, 0.3333333333333333703, 0.3219752754296894559, 0.3333333333333333703, 0.3219752754296894559, 0.3333333333333333703, 0.3219752754296894559, 0.3333333333333333703, 0.3219752754296894559, 0.3333333333333333703, 0.3219752754296894559, 0.3333333333333333703, 0.3219752754296894559, 0.3333333333333333703, 0.3219752754296894559, 0.3333333333333333703, 0.3219752754296894559, 0.3333333333333333703, 0.3219752754296894559, 0.3333333333333333703, 0.3219752754296894559, 0.3333333333333333703, 0.3219752754296894559, 0.3333333333333333703, 0.3219752754296894559, 0.3333333333333333703, 0.3219752754296894559, 0.3333333333333333703, 0.3219752754296894559, 0.3333333333333333703, 0.3219752754296894559, 0.3333333333333333703, 0.3219752754296894559, 0.3333333333333333703, 0.3219752754296894559, 0.3333333333333333703, 0.3219752754296894559, 0.3333333333333333703, 0.3219752754296894559, 0.3333333333333333703, 0.3219752754296894559, 0.3333333333333333703, 0.3219752754296894559, 0.3333333333333333703, 0.3219752754296894559, 0.3333333333333333703, 0.3219752754296894559, 0.3333333333333333703, 0.3219752754296894559, 0.3333333333333333703, 0.3219752754296894559, 0.3333333333333333703, 0.3219752754296894559, 0.3333333333333333703, 0.3219752754296894559, 0.3333333333333333703, 0.3219752754296894559, 0.3333333333333333703, 0.3219752754296894559, 0.3333333333333333703, 0.3219752754296894559, 0.3333333333333333703, 0.3219752754296894559, 0.3333333333333333703, 0.3219752754296894559, 0.3333333333333333703, 0.3219752754296894559, 0.3333333333333333703, 0.3219752754296894559, 0.3333333333333333703, 0.3219752754296894559, 0.3333333333333333703, 0.3219752754296894559, 0.3333333333333333703, 0.3219752754296894559, 0.3333333333333333703, 0.3219752754296894559, 0.3333333333333333703, 0.3219752754296894559, 0.3333333333333333703, 0.3219752754296894559, 0.3333333333333333703, 0.3219752754296894559, 0.3333333333333333703, 0.3219752754296894559, 0.3333333333333333703, 0.3219752754296894559, 0.3333333333333333703, 0.3219752754296894559, 0.3333333333333333703, 0.3219752754296894559, 0.3333333333333333703, 0.3219752754296894559, 0.3333333333333333703, 0.3219752754296894559, 0.3333333333333333703, 0.3219752754296894559, 0.3333333333333333703, 0.3219752754296894559, 0.3333333333333333703, 0.3219752754296894559, 0.3333333333333333703, 0.3219752754296894559, 0.3333333333333333703, 0.3219752754296894559, 0.3333333333333333703, 0.3219752754296894559, 0.3333333333333333703, 0.3219752754296894559, 0.3333333333333333703, 0.3219752754296894559, 0.3333333333333333703, 0.3219752754296894559, 0.3333333333333333703, 0.3219752754296894559, 0.3333333333333333703, 0.3219752754296894559, 0.3333333333333333703, 0.3219752754296894559, 0.3333333333333333703, 0.3219752754296894559, 0.3333333333333333703, 0.3219752754296894559, 0.3333333333333333703),
 ( 0.3333333333333333703, 0.3219752754296894559, 0.3333333333333333703, 0.3219752754296894559, 0.3333333333333333703, 0.3219752754296894559, 0.3333333333333333703, 0.3219752754296894559, 0.3333333333333333703, 0.3219752754296894559, 0.3333333333333333703, 0.3219752754296894559, 0.3333333333333333703, 0.3219752754296894559, 0.3333333333333333703, 0.3219752754296894559, 0.3333333333333333703, 0.3219752754296894559, 0.3333333333333333703, 0.3219752754296894559, 0.3333333333333333703, 0.3219752754296894559, 0.3333333333333333703, 0.3219752754296894559, 0.3333333333333333703, 0.3219752754296894559, 0.3333333333333333703, 0.3219752754296894559, 0.3333333333333333703, 0.3219752754296894559, 0.3333333333333333703, 0.3219752754296894559, 0.3333333333333333703, 0.3219752754296894559, 0.3333333333333333703, 0.3219752754296894559, 0.3333333333333333703, 0.3219752754296894559, 0.3333333333333333703, 0.3219752754296894559, 0.3333333333333333703, 0.3219752754296894559, 0.3333333333333333703, 0.3219752754296894559, 0.3333333333333333703, 0.3219752754296894559, 0.3333333333333333703, 0.3219752754296894559, 0.3333333333333333703, 0.3219752754296894559, 0.3333333333333333703, 0.3219752754296894559, 0.3333333333333333703, 0.3219752754296894559, 0.3333333333333333703, 0.3219752754296894559, 0.3333333333333333703, 0.3219752754296894559, 0.3333333333333333703, 0.3219752754296894559, 0.3333333333333333703, 0.3219752754296894559, 0.3333333333333333703, 0.3219752754296894559, 0.3333333333333333703, 0.3219752754296894559, 0.3333333333333333703, 0.3219752754296894559, 0.3333333333333333703, 0.3219752754296894559, 0.3333333333333333703, 0.3219752754296894559, 0.3333333333333333703, 0.3219752754296894559, 0.3333333333333333703, 0.3219752754296894559, 0.3333333333333333703, 0.3219752754296894559, 0.3333333333333333703, 0.3219752754296894559, 0.3333333333333333703, 0.3219752754296894559, 0.3333333333333333703, 0.3219752754296894559, 0.3333333333333333703, 0.3219752754296894559, 0.3333333333333333703, 0.3219752754296894559, 0.3333333333333333703, 0.3219752754296894559, 0.3333333333333333703, 0.3219752754296894559, 0.3333333333333333703, 0.3219752754296894559, 0.3333333333333333703, 0.3219752754296894559, 0.3333333333333333703, 0.3219752754296894559, 0.3333333333333333703, 0.3219752754296894559, 0.3333333333333333703, 0.3219752754296894559, 0.3333333333333333703, 0.3219752754296894559, 0.3333333333333333703, 0.3219752754296894559, 0.3333333333333333703, 0.3219752754296894559, 0.3333333333333333703, 0.3219752754296894559, 0.3333333333333333703, 0.3219752754296894559, 0.3333333333333333703, 0.3219752754296894559, 0.3333333333333333703, 0.3219752754296894559, 0.3333333333333333703, 0.3219752754296894559, 0.3333333333333333703, 0.3219752754296894559, 0.3333333333333333703, 0.3219752754296894559, 0.3333333333333333703, 0.3219752754296894559, 0.3333333333333333703, 0.3219752754296894559, 0.3333333333333333703, 0.3219752754296894559, 0.3333333333333333703, 0.3219752754296894559, 0.3333333333333333703, 0.3219752754296894559, 0.3333333333333333703, 0.3219752754296894559, 0.3333333333333333703, 0.3219752754296894559, 0.3333333333333333703, 0.3219752754296894559, 0.3333333333333333703, 0.3219752754296894559, 0.3333333333333333703, 0.3219752754296894559, 0.3333333333333333703, 0.3219752754296894559, 0.3333333333333333703, 0.3219752754296894559, 0.3333333333333333703, 0.3219752754296894559, 0.3333333333333333703, 0.3219752754296894559, 0.3333333333333333703, 0.3219752754296894559, 0.3333333333333333703, 0.3219752754296894559, 0.3333333333333333703, 0.3219752754296894559, 0.3333333333333333703, 0.3219752754296894559, 0.3333333333333333703, 0.3219752754296894559, 0.3333333333333333703, 0.3219752754296894559, 0.3333333333333333703, 0.3219752754296894559, 0.3333333333333333703, 0.3219752754296894559, 0.3333333333333333703, 0.3219752754296894559, 0.3333333333333333703, 0.3219752754296894559, 0.3333333333333333703, 0.3219752754296894559, 0.3333333333333333703, 0.3219752754296894559, 0.3333333333333333703, 0.3219752754296894559, 0.3333333333333333703, 0.3219752754296894559, 0.3333333333333333703, 0.3219752754296894559, 0.3333333333333333703, 0.3219752754296894559, 0.3333333333333333703, 0.3219752754296894559, 0.3333333333333333703, 0.3219752754296894559, 0.3333333333333333703, 0.3219752754296894559, 0.3333333333333333703, 0.3219752754296894559, 0.3333333333333333703, 0.3219752754296894559, 0.3333333333333333703, 0.3219752754296894559, 0.3333333333333333703, 0.3219752754296894559, 0.3333333333333333703, 0.3219752754296894559, 0.3333333333333333703, 0.3219752754296894559, 0.3333333333333333703, 0.3219752754296894559, 0.3333333333333333703, 0.3219752754296894559, 0.3333333333333333703, 0.3219752754296894559, 0.3333333333333333703, 0.3219752754296894559, 0.3333333333333333703, 0.3219752754296894559, 0.3333333333333333703, 0.3219752754296894559, 0.3333333333333333703, 0.3219752754296894559, 0.3333333333333333703, 0.3219752754296894559, 0.3333333333333333703, 0.3219752754296894559, 0.3333333333333333703, 0.3219752754296894559, 0.3333333333333333703, 0.3219752754296894559, 0.3333333333333333703, 0.3219752754296894559, 0.3333333333333333703, 0.3219752754296894559, 0.3333333333333333703, 0.3219752754296894559, 0.3333333333333333703, 0.3219752754296894559, 0.3333333333333333703, 0.3219752754296894559, 0.3333333333333333703, 0.3219752754296894559, 0.3333333333333333703, 0.3219752754296894559, 0.3333333333333333703, 0.3219752754296894559, 0.3333333333333333703, 0.3219752754296894559, 0.3333333333333333703, 0.3219752754296894559, 0.3333333333333333703, 0.3219752754296894559, 0.3333333333333333703, 0.3219752754296894559, 0.3333333333333333703, 0.3219752754296894559, 0.3333333333333333703, 0.3219752754296894559, 0.3333333333333333703, 0.3219752754296894559, 0.3333333333333333703, 0.3219752754296894559, 0.3333333333333333703, 0.3219752754296894559, 0.3333333333333333703, 0.3219752754296894559, 0.3333333333333333703, 0.3219752754296894559, 0.3333333333333333703, 0.3219752754296894559, 0.3333333333333333703, 0.3219752754296894559, 0.3333333333333333703, 0.3219752754296894559, 0.3333333333333333703, 0.3219752754296894559, 0.3333333333333333703, 0.3219752754296894559, 0.3333333333333333703, 0.3219752754296894559, 0.3333333333333333703, 0.3219752754296894559, 0.3333333333333333703, 0.3219752754296894559, 0.3333333333333333703, 0.3219752754296894559, 0.3333333333333333703, 0.3219752754296894559, 0.3333333333333333703, 0.3219752754296894559, 0.3333333333333333703, 0.3219752754296894559, 0.3333333333333333703, 0.3219752754296894559, 0.3333333333333333703, 0.3219752754296894559, 0.3333333333333333703, 0.3219752754296894559, 0.3333333333333333703, 0.3219752754296894559, 0.3333333333333333703, 0.3219752754296894559, 0.3333333333333333703, 0.3219752754296894559, 0.3333333333333333703, 0.3219752754296894559, 0.3333333333333333703, 0.3219752754296894559, 0.3333333333333333703, 0.3219752754296894559, 0.3333333333333333703, 0.3219752754296894559, 0.3333333333333333703, 0.3219752754296894559, 0.3333333333333333703, 0.3219752754296894559, 0.3333333333333333703, 0.3219752754296894559, 0.3333333333333333703, 0.3219752754296894559, 0.3333333333333333703, 0.3219752754296894559, 0.3333333333333333703, 0.3219752754296894559, 0.3333333333333333703, 0.3219752754296894559, 0.3333333333333333703, 0.3219752754296894559, 0.3333333333333333703, 0.3219752754296894559, 0.3333333333333333703, 0.3219752754296894559, 0.3333333333333333703, 0.3219752754296894559, 0.3333333333333333703, 0.3219752754296894559, 0.3333333333333333703, 0.3219752754296894559, 0.3333333333333333703, 0.3219752754296894559, 0.3333333333333333703, 0.3219752754296894559, 0.3333333333333333703, 0.3219752754296894559, 0.3333333333333333703, 0.3219752754296894559, 0.3333333333333333703, 0.3219752754296894559, 0.3333333333333333703, 0.3219752754296894559, 0.3333333333333333703, 0.3219752754296894559, 0.3333333333333333703, 0.3219752754296894559, 0.3333333333333333703, 0.3219752754296894559, 0.3333333333333333703, 0.3219752754296894559, 0.3333333333333333703, 0.3219752754296894559, 0.3333333333333333703, 0.3219752754296894559, 0.3333333333333333703, 0.3219752754296894559, 0.3333333333333333703, 0.3219752754296894559, 0.3333333333333333703, 0.3219752754296894559, 0.3333333333333333703, 0.3219752754296894559, 0.3333333333333333703, 0.3219752754296894559, 0.3333333333333333703, 0.3219752754296894559, 0.3333333333333333703, 0.3219752754296894559, 0.3333333333333333703, 0.3219752754296894559, 0.3333333333333333703, 0.3219752754296894559, 0.3333333333333333703, 0.3219752754296894559, 0.3333333333333333703, 0.3219752754296894559, 0.3333333333333333703, 0.3219752754296894559, 0.3333333333333333703, 0.3219752754296894559, 0.3333333333333333703, 0.3219752754296894559, 0.3333333333333333703, 0.3219752754296894559, 0.3333333333333333703, 0.3219752754296894559, 0.3333333333333333703, 0.3219752754296894559, 0.3333333333333333703, 0.3219752754296894559, 0.3333333333333333703, 0.3219752754296894559, 0.3333333333333333703, 0.3219752754296894559, 0.3333333333333333703, 0.3219752754296894559, 0.3333333333333333703, 0.3219752754296894559, 0.3333333333333333703, 0.3219752754296894559, 0.3333333333333333703, 0.3219752754296894559, 0.3333333333333333703, 0.3219752754296894559, 0.3333333333333333703, 0.3219752754296894559, 0.3333333333333333703, 0.3219752754296894559, 0.3333333333333333703, 0.3219752754296894559, 0.3333333333333333703, 0.3219752754296894559, 0.3333333333333333703, 0.3219752754296894559, 0.3333333333333333703, 0.3219752754296894559, 0.3333333333333333703, 0.3219752754296894559, 0.3333333333333333703, 0.3219752754296894559, 0.3333333333333333703, 0.3219752754296894559, 0.3333333333333333703, 0.3219752754296894559, 0.3333333333333333703, 0.3219752754296894559, 0.3333333333333333703, 0.3219752754296894559, 0.3333333333333333703, 0.3219752754296894559, 0.3333333333333333703, 0.3219752754296894559, 0.3333333333333333703, 0.3219752754296894559, 0.3333333333333333703, 0.3219752754296894559, 0.3333333333333333703, 0.3219752754296894559, 0.3333333333333333703, 0.3219752754296894559, 0.3333333333333333703, 0.3219752754296894559, 0.3333333333333333703, 0.3219752754296894559, 0.3333333333333333703, 0.3219752754296894559, 0.3333333333333333703, 0.3219752754296894559, 0.3333333333333333703, 0.3219752754296894559, 0.3333333333333333703, 0.3219752754296894559, 0.3333333333333333703, 0.3219752754296894559, 0.3333333333333333703, 0.3219752754296894559, 0.3333333333333333703),
 ( 1.000000000000000000, 0.9659258262890683122, 1.000000000000000000, 0.9659258262890683122, 1.000000000000000000, 0.9659258262890683122, 1.000000000000000000, 0.9659258262890683122, 1.000000000000000000, 0.9659258262890683122, 1.000000000000000000, 0.9659258262890683122, 1.000000000000000000, 0.9659258262890683122, 1.000000000000000000, 0.9659258262890683122, 1.000000000000000000, 0.9659258262890683122, 1.000000000000000000, 0.9659258262890683122, 1.000000000000000000, 0.9659258262890683122, 1.000000000000000000, 0.9659258262890683122, 1.000000000000000000, 0.9659258262890683122, 1.000000000000000000, 0.9659258262890683122, 1.000000000000000000, 0.9659258262890683122, 1.000000000000000000, 0.9659258262890683122, 1.000000000000000000, 0.9659258262890683122, 1.000000000000000000, 0.9659258262890683122, 1.000000000000000000, 0.9659258262890683122, 1.000000000000000000, 0.9659258262890683122, 1.000000000000000000, 0.9659258262890683122, 1.000000000000000000, 0.9659258262890683122, 1.000000000000000000, 0.9659258262890683122, 1.000000000000000000, 0.9659258262890683122, 1.000000000000000000, 0.9659258262890683122, 1.000000000000000000, 0.9659258262890683122, 1.000000000000000000, 0.9659258262890683122, 1.000000000000000000, 0.9659258262890683122, 1.000000000000000000, 0.9659258262890683122, 1.000000000000000000, 0.9659258262890683122, 1.000000000000000000, 0.9659258262890683122, 1.000000000000000000, 0.9659258262890683122, 1.000000000000000000, 0.9659258262890683122, 1.000000000000000000, 0.9659258262890683122, 1.000000000000000000, 0.9659258262890683122, 1.000000000000000000, 0.9659258262890683122, 1.000000000000000000, 0.9659258262890683122, 1.000000000000000000, 0.9659258262890683122, 1.000000000000000000, 0.9659258262890683122, 1.000000000000000000, 0.9659258262890683122, 1.000000000000000000, 0.9659258262890683122, 1.000000000000000000, 0.9659258262890683122, 1.000000000000000000, 0.9659258262890683122, 1.000000000000000000, 0.9659258262890683122, 1.000000000000000000, 0.9659258262890683122, 1.000000000000000000, 0.9659258262890683122, 1.000000000000000000, 0.9659258262890683122, 1.000000000000000000, 0.9659258262890683122, 1.000000000000000000, 0.9659258262890683122, 1.000000000000000000, 0.9659258262890683122, 1.000000000000000000, 0.9659258262890683122, 1.000000000000000000, 0.9659258262890683122, 1.000000000000000000, 0.9659258262890683122, 1.000000000000000000, 0.9659258262890683122, 1.000000000000000000, 0.9659258262890683122, 1.000000000000000000, 0.9659258262890683122, 1.000000000000000000, 0.9659258262890683122, 1.000000000000000000, 0.9659258262890683122, 1.000000000000000000, 0.9659258262890683122, 1.000000000000000000, 0.9659258262890683122, 1.000000000000000000, 0.9659258262890683122, 1.000000000000000000, 0.9659258262890683122, 1.000000000000000000, 0.9659258262890683122, 1.000000000000000000, 0.9659258262890683122, 1.000000000000000000, 0.9659258262890683122, 1.000000000000000000, 0.9659258262890683122, 1.000000000000000000, 0.9659258262890683122, 1.000000000000000000, 0.9659258262890683122, 1.000000000000000000, 0.9659258262890683122, 1.000000000000000000, 0.9659258262890683122, 1.000000000000000000, 0.9659258262890683122, 1.000000000000000000, 0.9659258262890683122, 1.000000000000000000, 0.9659258262890683122, 1.000000000000000000, 0.9659258262890683122, 1.000000000000000000, 0.9659258262890683122, 1.000000000000000000, 0.9659258262890683122, 1.000000000000000000, 0.9659258262890683122, 1.000000000000000000, 0.9659258262890683122, 1.000000000000000000, 0.9659258262890683122, 1.000000000000000000, 0.9659258262890683122, 1.000000000000000000, 0.9659258262890683122, 1.000000000000000000, 0.9659258262890683122, 1.000000000000000000, 0.9659258262890683122, 1.000000000000000000, 0.9659258262890683122, 1.000000000000000000, 0.9659258262890683122, 1.000000000000000000, 0.9659258262890683122, 1.000000000000000000, 0.9659258262890683122, 1.000000000000000000, 0.9659258262890683122, 1.000000000000000000, 0.9659258262890683122, 1.000000000000000000, 0.9659258262890683122, 1.000000000000000000, 0.9659258262890683122, 1.000000000000000000, 0.9659258262890683122, 1.000000000000000000, 0.9659258262890683122, 1.000000000000000000, 0.9659258262890683122, 1.000000000000000000, 0.9659258262890683122, 1.000000000000000000, 0.9659258262890683122, 1.000000000000000000, 0.9659258262890683122, 1.000000000000000000, 0.9659258262890683122, 1.000000000000000000, 0.9659258262890683122, 1.000000000000000000, 0.9659258262890683122, 1.000000000000000000, 0.9659258262890683122, 1.000000000000000000, 0.9659258262890683122, 1.000000000000000000, 0.9659258262890683122, 1.000000000000000000, 0.9659258262890683122, 1.000000000000000000, 0.9659258262890683122, 1.000000000000000000, 0.9659258262890683122, 1.000000000000000000, 0.9659258262890683122, 1.000000000000000000, 0.9659258262890683122, 1.000000000000000000, 0.9659258262890683122, 1.000000000000000000, 0.9659258262890683122, 1.000000000000000000, 0.9659258262890683122, 1.000000000000000000, 0.9659258262890683122, 1.000000000000000000, 0.9659258262890683122, 1.000000000000000000, 0.9659258262890683122, 1.000000000000000000, 0.9659258262890683122, 1.000000000000000000, 0.9659258262890683122, 1.000000000000000000, 0.9659258262890683122, 1.000000000000000000, 0.9659258262890683122, 1.000000000000000000, 0.9659258262890683122, 1.000000000000000000, 0.9659258262890683122, 1.000000000000000000, 0.9659258262890683122, 1.000000000000000000, 0.9659258262890683122, 1.000000000000000000, 0.9659258262890683122, 1.000000000000000000, 0.9659258262890683122, 1.000000000000000000, 0.9659258262890683122, 1.000000000000000000, 0.9659258262890683122, 1.000000000000000000, 0.9659258262890683122, 1.000000000000000000, 0.9659258262890683122, 1.000000000000000000, 0.9659258262890683122, 1.000000000000000000, 0.9659258262890683122, 1.000000000000000000, 0.9659258262890683122, 1.000000000000000000, 0.9659258262890683122, 1.000000000000000000, 0.9659258262890683122, 1.000000000000000000, 0.9659258262890683122, 1.000000000000000000, 0.9659258262890683122, 1.000000000000000000, 0.9659258262890683122, 1.000000000000000000, 0.9659258262890683122, 1.000000000000000000, 0.9659258262890683122, 1.000000000000000000, 0.9659258262890683122, 1.000000000000000000, 0.9659258262890683122, 1.000000000000000000, 0.9659258262890683122, 1.000000000000000000, 0.9659258262890683122, 1.000000000000000000, 0.9659258262890683122, 1.000000000000000000, 0.9659258262890683122, 1.000000000000000000, 0.9659258262890683122, 1.000000000000000000, 0.9659258262890683122, 1.000000000000000000, 0.9659258262890683122, 1.000000000000000000, 0.9659258262890683122, 1.000000000000000000, 0.9659258262890683122, 1.000000000000000000, 0.9659258262890683122, 1.000000000000000000, 0.9659258262890683122, 1.000000000000000000, 0.9659258262890683122, 1.000000000000000000, 0.9659258262890683122, 1.000000000000000000, 0.9659258262890683122, 1.000000000000000000, 0.9659258262890683122, 1.000000000000000000, 0.9659258262890683122, 1.000000000000000000, 0.9659258262890683122, 1.000000000000000000, 0.9659258262890683122, 1.000000000000000000, 0.9659258262890683122, 1.000000000000000000, 0.9659258262890683122, 1.000000000000000000, 0.9659258262890683122, 1.000000000000000000, 0.9659258262890683122, 1.000000000000000000, 0.9659258262890683122, 1.000000000000000000, 0.9659258262890683122, 1.000000000000000000, 0.9659258262890683122, 1.000000000000000000, 0.9659258262890683122, 1.000000000000000000, 0.9659258262890683122, 1.000000000000000000, 0.9659258262890683122, 1.000000000000000000, 0.9659258262890683122, 1.000000000000000000, 0.9659258262890683122, 1.000000000000000000, 0.9659258262890683122, 1.000000000000000000, 0.9659258262890683122, 1.000000000000000000, 0.9659258262890683122, 1.000000000000000000, 0.9659258262890683122, 1.000000000000000000, 0.9659258262890683122, 1.000000000000000000, 0.9659258262890683122, 1.000000000000000000, 0.9659258262890683122, 1.000000000000000000, 0.9659258262890683122, 1.000000000000000000, 0.9659258262890683122, 1.000000000000000000, 0.9659258262890683122, 1.000000000000000000, 0.9659258262890683122, 1.000000000000000000, 0.9659258262890683122, 1.000000000000000000, 0.9659258262890683122, 1.000000000000000000, 0.9659258262890683122, 1.000000000000000000, 0.9659258262890683122, 1.000000000000000000, 0.9659258262890683122, 1.000000000000000000, 0.9659258262890683122, 1.000000000000000000, 0.9659258262890683122, 1.000000000000000000, 0.9659258262890683122, 1.000000000000000000, 0.9659258262890683122, 1.000000000000000000, 0.9659258262890683122, 1.000000000000000000, 0.9659258262890683122, 1.000000000000000000, 0.9659258262890683122, 1.000000000000000000, 0.9659258262890683122, 1.000000000000000000, 0.9659258262890683122, 1.000000000000000000, 0.9659258262890683122, 1.000000000000000000, 0.9659258262890683122, 1.000000000000000000, 0.9659258262890683122, 1.000000000000000000, 0.9659258262890683122, 1.000000000000000000, 0.9659258262890683122, 1.000000000000000000, 0.9659258262890683122, 1.000000000000000000, 0.9659258262890683122, 1.000000000000000000, 0.9659258262890683122, 1.000000000000000000, 0.9659258262890683122, 1.000000000000000000, 0.9659258262890683122, 1.000000000000000000, 0.9659258262890683122, 1.000000000000000000, 0.9659258262890683122, 1.000000000000000000, 0.9659258262890683122, 1.000000000000000000, 0.9659258262890683122, 1.000000000000000000, 0.9659258262890683122, 1.000000000000000000, 0.9659258262890683122, 1.000000000000000000, 0.9659258262890683122, 1.000000000000000000, 0.9659258262890683122, 1.000000000000000000, 0.9659258262890683122, 1.000000000000000000, 0.9659258262890683122, 1.000000000000000000, 0.9659258262890683122, 1.000000000000000000, 0.9659258262890683122, 1.000000000000000000, 0.9659258262890683122, 1.000000000000000000, 0.9659258262890683122, 1.000000000000000000, 0.9659258262890683122, 1.000000000000000000, 0.9659258262890683122, 1.000000000000000000, 0.9659258262890683122, 1.000000000000000000, 0.9659258262890683122, 1.000000000000000000, 0.9659258262890683122, 1.000000000000000000, 0.9659258262890683122, 1.000000000000000000, 0.9659258262890683122, 1.000000000000000000, 0.9659258262890683122, 1.000000000000000000, 0.9659258262890683122, 1.000000000000000000),
 ( 0.3333333333333333703, 0.3219752754296894559, 0.3333333333333333703, 0.3219752754296894559, 0.3333333333333333703, 0.3219752754296894559, 0.3333333333333333703, 0.3219752754296894559, 0.3333333333333333703, 0.3219752754296894559, 0.3333333333333333703, 0.3219752754296894559, 0.3333333333333333703, 0.3219752754296894559, 0.3333333333333333703, 0.3219752754296894559, 0.3333333333333333703, 0.3219752754296894559, 0.3333333333333333703, 0.3219752754296894559, 0.3333333333333333703, 0.3219752754296894559, 0.3333333333333333703, 0.3219752754296894559, 0.3333333333333333703, 0.3219752754296894559, 0.3333333333333333703, 0.3219752754296894559, 0.3333333333333333703, 0.3219752754296894559, 0.3333333333333333703, 0.3219752754296894559, 0.3333333333333333703, 0.3219752754296894559, 0.3333333333333333703, 0.3219752754296894559, 0.3333333333333333703, 0.3219752754296894559, 0.3333333333333333703, 0.3219752754296894559, 0.3333333333333333703, 0.3219752754296894559, 0.3333333333333333703, 0.3219752754296894559, 0.3333333333333333703, 0.3219752754296894559, 0.3333333333333333703, 0.3219752754296894559, 0.3333333333333333703, 0.3219752754296894559, 0.3333333333333333703, 0.3219752754296894559, 0.3333333333333333703, 0.3219752754296894559, 0.3333333333333333703, 0.3219752754296894559, 0.3333333333333333703, 0.3219752754296894559, 0.3333333333333333703, 0.3219752754296894559, 0.3333333333333333703, 0.3219752754296894559, 0.3333333333333333703, 0.3219752754296894559, 0.3333333333333333703, 0.3219752754296894559, 0.3333333333333333703, 0.3219752754296894559, 0.3333333333333333703, 0.3219752754296894559, 0.3333333333333333703, 0.3219752754296894559, 0.3333333333333333703, 0.3219752754296894559, 0.3333333333333333703, 0.3219752754296894559, 0.3333333333333333703, 0.3219752754296894559, 0.3333333333333333703, 0.3219752754296894559, 0.3333333333333333703, 0.3219752754296894559, 0.3333333333333333703, 0.3219752754296894559, 0.3333333333333333703, 0.3219752754296894559, 0.3333333333333333703, 0.3219752754296894559, 0.3333333333333333703, 0.3219752754296894559, 0.3333333333333333703, 0.3219752754296894559, 0.3333333333333333703, 0.3219752754296894559, 0.3333333333333333703, 0.3219752754296894559, 0.3333333333333333703, 0.3219752754296894559, 0.3333333333333333703, 0.3219752754296894559, 0.3333333333333333703, 0.3219752754296894559, 0.3333333333333333703, 0.3219752754296894559, 0.3333333333333333703, 0.3219752754296894559, 0.3333333333333333703, 0.3219752754296894559, 0.3333333333333333703, 0.3219752754296894559, 0.3333333333333333703, 0.3219752754296894559, 0.3333333333333333703, 0.3219752754296894559, 0.3333333333333333703, 0.3219752754296894559, 0.3333333333333333703, 0.3219752754296894559, 0.3333333333333333703, 0.3219752754296894559, 0.3333333333333333703, 0.3219752754296894559, 0.3333333333333333703, 0.3219752754296894559, 0.3333333333333333703, 0.3219752754296894559, 0.3333333333333333703, 0.3219752754296894559, 0.3333333333333333703, 0.3219752754296894559, 0.3333333333333333703, 0.3219752754296894559, 0.3333333333333333703, 0.3219752754296894559, 0.3333333333333333703, 0.3219752754296894559, 0.3333333333333333703, 0.3219752754296894559, 0.3333333333333333703, 0.3219752754296894559, 0.3333333333333333703, 0.3219752754296894559, 0.3333333333333333703, 0.3219752754296894559, 0.3333333333333333703, 0.3219752754296894559, 0.3333333333333333703, 0.3219752754296894559, 0.3333333333333333703, 0.3219752754296894559, 0.3333333333333333703, 0.3219752754296894559, 0.3333333333333333703, 0.3219752754296894559, 0.3333333333333333703, 0.3219752754296894559, 0.3333333333333333703, 0.3219752754296894559, 0.3333333333333333703, 0.3219752754296894559, 0.3333333333333333703, 0.3219752754296894559, 0.3333333333333333703, 0.3219752754296894559, 0.3333333333333333703, 0.3219752754296894559, 0.3333333333333333703, 0.3219752754296894559, 0.3333333333333333703, 0.3219752754296894559, 0.3333333333333333703, 0.3219752754296894559, 0.3333333333333333703, 0.3219752754296894559, 0.3333333333333333703, 0.3219752754296894559, 0.3333333333333333703, 0.3219752754296894559, 0.3333333333333333703, 0.3219752754296894559, 0.3333333333333333703, 0.3219752754296894559, 0.3333333333333333703, 0.3219752754296894559, 0.3333333333333333703, 0.3219752754296894559, 0.3333333333333333703, 0.3219752754296894559, 0.3333333333333333703, 0.3219752754296894559, 0.3333333333333333703, 0.3219752754296894559, 0.3333333333333333703, 0.3219752754296894559, 0.3333333333333333703, 0.3219752754296894559, 0.3333333333333333703, 0.3219752754296894559, 0.3333333333333333703, 0.3219752754296894559, 0.3333333333333333703, 0.3219752754296894559, 0.3333333333333333703, 0.3219752754296894559, 0.3333333333333333703, 0.3219752754296894559, 0.3333333333333333703, 0.3219752754296894559, 0.3333333333333333703, 0.3219752754296894559, 0.3333333333333333703, 0.3219752754296894559, 0.3333333333333333703, 0.3219752754296894559, 0.3333333333333333703, 0.3219752754296894559, 0.3333333333333333703, 0.3219752754296894559, 0.3333333333333333703, 0.3219752754296894559, 0.3333333333333333703, 0.3219752754296894559, 0.3333333333333333703, 0.3219752754296894559, 0.3333333333333333703, 0.3219752754296894559, 0.3333333333333333703, 0.3219752754296894559, 0.3333333333333333703, 0.3219752754296894559, 0.3333333333333333703, 0.3219752754296894559, 0.3333333333333333703, 0.3219752754296894559, 0.3333333333333333703, 0.3219752754296894559, 0.3333333333333333703, 0.3219752754296894559, 0.3333333333333333703, 0.3219752754296894559, 0.3333333333333333703, 0.3219752754296894559, 0.3333333333333333703, 0.3219752754296894559, 0.3333333333333333703, 0.3219752754296894559, 0.3333333333333333703, 0.3219752754296894559, 0.3333333333333333703, 0.3219752754296894559, 0.3333333333333333703, 0.3219752754296894559, 0.3333333333333333703, 0.3219752754296894559, 0.3333333333333333703, 0.3219752754296894559, 0.3333333333333333703, 0.3219752754296894559, 0.3333333333333333703, 0.3219752754296894559, 0.3333333333333333703, 0.3219752754296894559, 0.3333333333333333703, 0.3219752754296894559, 0.3333333333333333703, 0.3219752754296894559, 0.3333333333333333703, 0.3219752754296894559, 0.3333333333333333703, 0.3219752754296894559, 0.3333333333333333703, 0.3219752754296894559, 0.3333333333333333703, 0.3219752754296894559, 0.3333333333333333703, 0.3219752754296894559, 0.3333333333333333703, 0.3219752754296894559, 0.3333333333333333703, 0.3219752754296894559, 0.3333333333333333703, 0.3219752754296894559, 0.3333333333333333703, 0.3219752754296894559, 0.3333333333333333703, 0.3219752754296894559, 0.3333333333333333703, 0.3219752754296894559, 0.3333333333333333703, 0.3219752754296894559, 0.3333333333333333703, 0.3219752754296894559, 0.3333333333333333703, 0.3219752754296894559, 0.3333333333333333703, 0.3219752754296894559, 0.3333333333333333703, 0.3219752754296894559, 0.3333333333333333703, 0.3219752754296894559, 0.3333333333333333703, 0.3219752754296894559, 0.3333333333333333703, 0.3219752754296894559, 0.3333333333333333703, 0.3219752754296894559, 0.3333333333333333703, 0.3219752754296894559, 0.3333333333333333703, 0.3219752754296894559, 0.3333333333333333703, 0.3219752754296894559, 0.3333333333333333703, 0.3219752754296894559, 0.3333333333333333703, 0.3219752754296894559, 0.3333333333333333703, 0.3219752754296894559, 0.3333333333333333703, 0.3219752754296894559, 0.3333333333333333703, 0.3219752754296894559, 0.3333333333333333703, 0.3219752754296894559, 0.3333333333333333703, 0.3219752754296894559, 0.3333333333333333703, 0.3219752754296894559, 0.3333333333333333703, 0.3219752754296894559, 0.3333333333333333703, 0.3219752754296894559, 0.3333333333333333703, 0.3219752754296894559, 0.3333333333333333703, 0.3219752754296894559, 0.3333333333333333703, 0.3219752754296894559, 0.3333333333333333703, 0.3219752754296894559, 0.3333333333333333703, 0.3219752754296894559, 0.3333333333333333703, 0.3219752754296894559, 0.3333333333333333703, 0.3219752754296894559, 0.3333333333333333703, 0.3219752754296894559, 0.3333333333333333703, 0.3219752754296894559, 0.3333333333333333703, 0.3219752754296894559, 0.3333333333333333703, 0.3219752754296894559, 0.3333333333333333703, 0.3219752754296894559, 0.3333333333333333703, 0.3219752754296894559, 0.3333333333333333703, 0.3219752754296894559, 0.3333333333333333703, 0.3219752754296894559, 0.3333333333333333703, 0.3219752754296894559, 0.3333333333333333703, 0.3219752754296894559, 0.3333333333333333703, 0.3219752754296894559, 0.3333333333333333703, 0.3219752754296894559, 0.3333333333333333703, 0.3219752754296894559, 0.3333333333333333703, 0.3219752754296894559, 0.3333333333333333703, 0.3219752754296894559, 0.3333333333333333703, 0.3219752754296894559, 0.3333333333333333703, 0.3219752754296894559, 0.3333333333333333703, 0.3219752754296894559, 0.3333333333333333703, 0.3219752754296894559, 0.3333333333333333703, 0.3219752754296894559, 0.3333333333333333703, 0.3219752754296894559, 0.3333333333333333703, 0.3219752754296894559, 0.3333333333333333703, 0.3219752754296894559, 0.3333333333333333703, 0.3219752754296894559, 0.3333333333333333703, 0.3219752754296894559, 0.3333333333333333703, 0.3219752754296894559, 0.3333333333333333703, 0.3219752754296894559, 0.3333333333333333703, 0.3219752754296894559, 0.3333333333333333703, 0.3219752754296894559, 0.3333333333333333703, 0.3219752754296894559, 0.3333333333333333703, 0.3219752754296894559, 0.3333333333333333703, 0.3219752754296894559, 0.3333333333333333703, 0.3219752754296894559, 0.3333333333333333703, 0.3219752754296894559, 0.3333333333333333703, 0.3219752754296894559, 0.3333333333333333703, 0.3219752754296894559, 0.3333333333333333703, 0.3219752754296894559, 0.3333333333333333703, 0.3219752754296894559, 0.3333333333333333703, 0.3219752754296894559, 0.3333333333333333703, 0.3219752754296894559, 0.3333333333333333703, 0.3219752754296894559, 0.3333333333333333703, 0.3219752754296894559, 0.3333333333333333703, 0.3219752754296894559, 0.3333333333333333703, 0.3219752754296894559, 0.3333333333333333703, 0.3219752754296894559, 0.3333333333333333703, 0.3219752754296894559, 0.3333333333333333703, 0.3219752754296894559, 0.3333333333333333703, 0.3219752754296894559, 0.3333333333333333703, 0.3219752754296894559, 0.3333333333333333703, 0.3219752754296894559, 0.3333333333333333703, 0.3219752754296894559, 0.3333333333333333703, 0.3219752754296894559, 0.3333333333333333703, 0.3219752754296894559, 0.3333333333333333703, 0.3219752754296894559, 0.3333333333333333703, 0.3219752754296894559, 0.3333333333333333703),
 ( 0.3333333333333333703, 0.3219752754296894559, 0.3333333333333333703, 0.3219752754296894559, 0.3333333333333333703, 0.3219752754296894559, 0.3333333333333333703, 0.3219752754296894559, 0.3333333333333333703, 0.3219752754296894559, 0.3333333333333333703, 0.3219752754296894559, 0.3333333333333333703, 0.3219752754296894559, 0.3333333333333333703, 0.3219752754296894559, 0.3333333333333333703, 0.3219752754296894559, 0.3333333333333333703, 0.3219752754296894559, 0.3333333333333333703, 0.3219752754296894559, 0.3333333333333333703, 0.3219752754296894559, 0.3333333333333333703, 0.3219752754296894559, 0.3333333333333333703, 0.3219752754296894559, 0.3333333333333333703, 0.3219752754296894559, 0.3333333333333333703, 0.3219752754296894559, 0.3333333333333333703, 0.3219752754296894559, 0.3333333333333333703, 0.3219752754296894559, 0.3333333333333333703, 0.3219752754296894559, 0.3333333333333333703, 0.3219752754296894559, 0.3333333333333333703, 0.3219752754296894559, 0.3333333333333333703, 0.3219752754296894559, 0.3333333333333333703, 0.3219752754296894559, 0.3333333333333333703, 0.3219752754296894559, 0.3333333333333333703, 0.3219752754296894559, 0.3333333333333333703, 0.3219752754296894559, 0.3333333333333333703, 0.3219752754296894559, 0.3333333333333333703, 0.3219752754296894559, 0.3333333333333333703, 0.3219752754296894559, 0.3333333333333333703, 0.3219752754296894559, 0.3333333333333333703, 0.3219752754296894559, 0.3333333333333333703, 0.3219752754296894559, 0.3333333333333333703, 0.3219752754296894559, 0.3333333333333333703, 0.3219752754296894559, 0.3333333333333333703, 0.3219752754296894559, 0.3333333333333333703, 0.3219752754296894559, 0.3333333333333333703, 0.3219752754296894559, 0.3333333333333333703, 0.3219752754296894559, 0.3333333333333333703, 0.3219752754296894559, 0.3333333333333333703, 0.3219752754296894559, 0.3333333333333333703, 0.3219752754296894559, 0.3333333333333333703, 0.3219752754296894559, 0.3333333333333333703, 0.3219752754296894559, 0.3333333333333333703, 0.3219752754296894559, 0.3333333333333333703, 0.3219752754296894559, 0.3333333333333333703, 0.3219752754296894559, 0.3333333333333333703, 0.3219752754296894559, 0.3333333333333333703, 0.3219752754296894559, 0.3333333333333333703, 0.3219752754296894559, 0.3333333333333333703, 0.3219752754296894559, 0.3333333333333333703, 0.3219752754296894559, 0.3333333333333333703, 0.3219752754296894559, 0.3333333333333333703, 0.3219752754296894559, 0.3333333333333333703, 0.3219752754296894559, 0.3333333333333333703, 0.3219752754296894559, 0.3333333333333333703, 0.3219752754296894559, 0.3333333333333333703, 0.3219752754296894559, 0.3333333333333333703, 0.3219752754296894559, 0.3333333333333333703, 0.3219752754296894559, 0.3333333333333333703, 0.3219752754296894559, 0.3333333333333333703, 0.3219752754296894559, 0.3333333333333333703, 0.3219752754296894559, 0.3333333333333333703, 0.3219752754296894559, 0.3333333333333333703, 0.3219752754296894559, 0.3333333333333333703, 0.3219752754296894559, 0.3333333333333333703, 0.3219752754296894559, 0.3333333333333333703, 0.3219752754296894559, 0.3333333333333333703, 0.3219752754296894559, 0.3333333333333333703, 0.3219752754296894559, 0.3333333333333333703, 0.3219752754296894559, 0.3333333333333333703, 0.3219752754296894559, 0.3333333333333333703, 0.3219752754296894559, 0.3333333333333333703, 0.3219752754296894559, 0.3333333333333333703, 0.3219752754296894559, 0.3333333333333333703, 0.3219752754296894559, 0.3333333333333333703, 0.3219752754296894559, 0.3333333333333333703, 0.3219752754296894559, 0.3333333333333333703, 0.3219752754296894559, 0.3333333333333333703, 0.3219752754296894559, 0.3333333333333333703, 0.3219752754296894559, 0.3333333333333333703, 0.3219752754296894559, 0.3333333333333333703, 0.3219752754296894559, 0.3333333333333333703, 0.3219752754296894559, 0.3333333333333333703, 0.3219752754296894559, 0.3333333333333333703, 0.3219752754296894559, 0.3333333333333333703, 0.3219752754296894559, 0.3333333333333333703, 0.3219752754296894559, 0.3333333333333333703, 0.3219752754296894559, 0.3333333333333333703, 0.3219752754296894559, 0.3333333333333333703, 0.3219752754296894559, 0.3333333333333333703, 0.3219752754296894559, 0.3333333333333333703, 0.3219752754296894559, 0.3333333333333333703, 0.3219752754296894559, 0.3333333333333333703, 0.3219752754296894559, 0.3333333333333333703, 0.3219752754296894559, 0.3333333333333333703, 0.3219752754296894559, 0.3333333333333333703, 0.3219752754296894559, 0.3333333333333333703, 0.3219752754296894559, 0.3333333333333333703, 0.3219752754296894559, 0.3333333333333333703, 0.3219752754296894559, 0.3333333333333333703, 0.3219752754296894559, 0.3333333333333333703, 0.3219752754296894559, 0.3333333333333333703, 0.3219752754296894559, 0.3333333333333333703, 0.3219752754296894559, 0.3333333333333333703, 0.3219752754296894559, 0.3333333333333333703, 0.3219752754296894559, 0.3333333333333333703, 0.3219752754296894559, 0.3333333333333333703, 0.3219752754296894559, 0.3333333333333333703, 0.3219752754296894559, 0.3333333333333333703, 0.3219752754296894559, 0.3333333333333333703, 0.3219752754296894559, 0.3333333333333333703, 0.3219752754296894559, 0.3333333333333333703, 0.3219752754296894559, 0.3333333333333333703, 0.3219752754296894559, 0.3333333333333333703, 0.3219752754296894559, 0.3333333333333333703, 0.3219752754296894559, 0.3333333333333333703, 0.3219752754296894559, 0.3333333333333333703, 0.3219752754296894559, 0.3333333333333333703, 0.3219752754296894559, 0.3333333333333333703, 0.3219752754296894559, 0.3333333333333333703, 0.3219752754296894559, 0.3333333333333333703, 0.3219752754296894559, 0.3333333333333333703, 0.3219752754296894559, 0.3333333333333333703, 0.3219752754296894559, 0.3333333333333333703, 0.3219752754296894559, 0.3333333333333333703, 0.3219752754296894559, 0.3333333333333333703, 0.3219752754296894559, 0.3333333333333333703, 0.3219752754296894559, 0.3333333333333333703, 0.3219752754296894559, 0.3333333333333333703, 0.3219752754296894559, 0.3333333333333333703, 0.3219752754296894559, 0.3333333333333333703, 0.3219752754296894559, 0.3333333333333333703, 0.3219752754296894559, 0.3333333333333333703, 0.3219752754296894559, 0.3333333333333333703, 0.3219752754296894559, 0.3333333333333333703, 0.3219752754296894559, 0.3333333333333333703, 0.3219752754296894559, 0.3333333333333333703, 0.3219752754296894559, 0.3333333333333333703, 0.3219752754296894559, 0.3333333333333333703, 0.3219752754296894559, 0.3333333333333333703, 0.3219752754296894559, 0.3333333333333333703, 0.3219752754296894559, 0.3333333333333333703, 0.3219752754296894559, 0.3333333333333333703, 0.3219752754296894559, 0.3333333333333333703, 0.3219752754296894559, 0.3333333333333333703, 0.3219752754296894559, 0.3333333333333333703, 0.3219752754296894559, 0.3333333333333333703, 0.3219752754296894559, 0.3333333333333333703, 0.3219752754296894559, 0.3333333333333333703, 0.3219752754296894559, 0.3333333333333333703, 0.3219752754296894559, 0.3333333333333333703, 0.3219752754296894559, 0.3333333333333333703, 0.3219752754296894559, 0.3333333333333333703, 0.3219752754296894559, 0.3333333333333333703, 0.3219752754296894559, 0.3333333333333333703, 0.3219752754296894559, 0.3333333333333333703, 0.3219752754296894559, 0.3333333333333333703, 0.3219752754296894559, 0.3333333333333333703, 0.3219752754296894559, 0.3333333333333333703, 0.3219752754296894559, 0.3333333333333333703, 0.3219752754296894559, 0.3333333333333333703, 0.3219752754296894559, 0.3333333333333333703, 0.3219752754296894559, 0.3333333333333333703, 0.3219752754296894559, 0.3333333333333333703, 0.3219752754296894559, 0.3333333333333333703, 0.3219752754296894559, 0.3333333333333333703, 0.3219752754296894559, 0.3333333333333333703, 0.3219752754296894559, 0.3333333333333333703, 0.3219752754296894559, 0.3333333333333333703, 0.3219752754296894559, 0.3333333333333333703, 0.3219752754296894559, 0.3333333333333333703, 0.3219752754296894559, 0.3333333333333333703, 0.3219752754296894559, 0.3333333333333333703, 0.3219752754296894559, 0.3333333333333333703, 0.3219752754296894559, 0.3333333333333333703, 0.3219752754296894559, 0.3333333333333333703, 0.3219752754296894559, 0.3333333333333333703, 0.3219752754296894559, 0.3333333333333333703, 0.3219752754296894559, 0.3333333333333333703, 0.3219752754296894559, 0.3333333333333333703, 0.3219752754296894559, 0.3333333333333333703, 0.3219752754296894559, 0.3333333333333333703, 0.3219752754296894559, 0.3333333333333333703, 0.3219752754296894559, 0.3333333333333333703, 0.3219752754296894559, 0.3333333333333333703, 0.3219752754296894559, 0.3333333333333333703, 0.3219752754296894559, 0.3333333333333333703, 0.3219752754296894559, 0.3333333333333333703, 0.3219752754296894559, 0.3333333333333333703, 0.3219752754296894559, 0.3333333333333333703, 0.3219752754296894559, 0.3333333333333333703, 0.3219752754296894559, 0.3333333333333333703, 0.3219752754296894559, 0.3333333333333333703, 0.3219752754296894559, 0.3333333333333333703, 0.3219752754296894559, 0.3333333333333333703, 0.3219752754296894559, 0.3333333333333333703, 0.3219752754296894559, 0.3333333333333333703, 0.3219752754296894559, 0.3333333333333333703, 0.3219752754296894559, 0.3333333333333333703, 0.3219752754296894559, 0.3333333333333333703, 0.3219752754296894559, 0.3333333333333333703, 0.3219752754296894559, 0.3333333333333333703, 0.3219752754296894559, 0.3333333333333333703, 0.3219752754296894559, 0.3333333333333333703, 0.3219752754296894559, 0.3333333333333333703, 0.3219752754296894559, 0.3333333333333333703, 0.3219752754296894559, 0.3333333333333333703, 0.3219752754296894559, 0.3333333333333333703, 0.3219752754296894559, 0.3333333333333333703, 0.3219752754296894559, 0.3333333333333333703, 0.3219752754296894559, 0.3333333333333333703, 0.3219752754296894559, 0.3333333333333333703, 0.3219752754296894559, 0.3333333333333333703, 0.3219752754296894559, 0.3333333333333333703, 0.3219752754296894559, 0.3333333333333333703, 0.3219752754296894559, 0.3333333333333333703, 0.3219752754296894559, 0.3333333333333333703, 0.3219752754296894559, 0.3333333333333333703, 0.3219752754296894559, 0.3333333333333333703, 0.3219752754296894559, 0.3333333333333333703, 0.3219752754296894559, 0.3333333333333333703, 0.3219752754296894559, 0.3333333333333333703, 0.3219752754296894559, 0.3333333333333333703, 0.3219752754296894559, 0.3333333333333333703, 0.3219752754296894559, 0.3333333333333333703, 0.3219752754296894559, 0.3333333333333333703, 0.3219752754296894559, 0.3333333333333333703, 0.3219752754296894559, 0.3333333333333333703),
 ( 1.000000000000000000, 0.9659258262890683122, 1.000000000000000000, 0.9659258262890683122, 1.000000000000000000, 0.9659258262890683122, 1.000000000000000000, 0.9659258262890683122, 1.000000000000000000, 0.9659258262890683122, 1.000000000000000000, 0.9659258262890683122, 1.000000000000000000, 0.9659258262890683122, 1.000000000000000000, 0.9659258262890683122, 1.000000000000000000, 0.9659258262890683122, 1.000000000000000000, 0.9659258262890683122, 1.000000000000000000, 0.9659258262890683122, 1.000000000000000000, 0.9659258262890683122, 1.000000000000000000, 0.9659258262890683122, 1.000000000000000000, 0.9659258262890683122, 1.000000000000000000, 0.9659258262890683122, 1.000000000000000000, 0.9659258262890683122, 1.000000000000000000, 0.9659258262890683122, 1.000000000000000000, 0.9659258262890683122, 1.000000000000000000, 0.9659258262890683122, 1.000000000000000000, 0.9659258262890683122, 1.000000000000000000, 0.9659258262890683122, 1.000000000000000000, 0.9659258262890683122, 1.000000000000000000, 0.9659258262890683122, 1.000000000000000000, 0.9659258262890683122, 1.000000000000000000, 0.9659258262890683122, 1.000000000000000000, 0.9659258262890683122, 1.000000000000000000, 0.9659258262890683122, 1.000000000000000000, 0.9659258262890683122, 1.000000000000000000, 0.9659258262890683122, 1.000000000000000000, 0.9659258262890683122, 1.000000000000000000, 0.9659258262890683122, 1.000000000000000000, 0.9659258262890683122, 1.000000000000000000, 0.9659258262890683122, 1.000000000000000000, 0.9659258262890683122, 1.000000000000000000, 0.9659258262890683122, 1.000000000000000000, 0.9659258262890683122, 1.000000000000000000, 0.9659258262890683122, 1.000000000000000000, 0.9659258262890683122, 1.000000000000000000, 0.9659258262890683122, 1.000000000000000000, 0.9659258262890683122, 1.000000000000000000, 0.9659258262890683122, 1.000000000000000000, 0.9659258262890683122, 1.000000000000000000, 0.9659258262890683122, 1.000000000000000000, 0.9659258262890683122, 1.000000000000000000, 0.9659258262890683122, 1.000000000000000000, 0.9659258262890683122, 1.000000000000000000, 0.9659258262890683122, 1.000000000000000000, 0.9659258262890683122, 1.000000000000000000, 0.9659258262890683122, 1.000000000000000000, 0.9659258262890683122, 1.000000000000000000, 0.9659258262890683122, 1.000000000000000000, 0.9659258262890683122, 1.000000000000000000, 0.9659258262890683122, 1.000000000000000000, 0.9659258262890683122, 1.000000000000000000, 0.9659258262890683122, 1.000000000000000000, 0.9659258262890683122, 1.000000000000000000, 0.9659258262890683122, 1.000000000000000000, 0.9659258262890683122, 1.000000000000000000, 0.9659258262890683122, 1.000000000000000000, 0.9659258262890683122, 1.000000000000000000, 0.9659258262890683122, 1.000000000000000000, 0.9659258262890683122, 1.000000000000000000, 0.9659258262890683122, 1.000000000000000000, 0.9659258262890683122, 1.000000000000000000, 0.9659258262890683122, 1.000000000000000000, 0.9659258262890683122, 1.000000000000000000, 0.9659258262890683122, 1.000000000000000000, 0.9659258262890683122, 1.000000000000000000, 0.9659258262890683122, 1.000000000000000000, 0.9659258262890683122, 1.000000000000000000, 0.9659258262890683122, 1.000000000000000000, 0.9659258262890683122, 1.000000000000000000, 0.9659258262890683122, 1.000000000000000000, 0.9659258262890683122, 1.000000000000000000, 0.9659258262890683122, 1.000000000000000000, 0.9659258262890683122, 1.000000000000000000, 0.9659258262890683122, 1.000000000000000000, 0.9659258262890683122, 1.000000000000000000, 0.9659258262890683122, 1.000000000000000000, 0.9659258262890683122, 1.000000000000000000, 0.9659258262890683122, 1.000000000000000000, 0.9659258262890683122, 1.000000000000000000, 0.9659258262890683122, 1.000000000000000000, 0.9659258262890683122, 1.000000000000000000, 0.9659258262890683122, 1.000000000000000000, 0.9659258262890683122, 1.000000000000000000, 0.9659258262890683122, 1.000000000000000000, 0.9659258262890683122, 1.000000000000000000, 0.9659258262890683122, 1.000000000000000000, 0.9659258262890683122, 1.000000000000000000, 0.9659258262890683122, 1.000000000000000000, 0.9659258262890683122, 1.000000000000000000, 0.9659258262890683122, 1.000000000000000000, 0.9659258262890683122, 1.000000000000000000, 0.9659258262890683122, 1.000000000000000000, 0.9659258262890683122, 1.000000000000000000, 0.9659258262890683122, 1.000000000000000000, 0.9659258262890683122, 1.000000000000000000, 0.9659258262890683122, 1.000000000000000000, 0.9659258262890683122, 1.000000000000000000, 0.9659258262890683122, 1.000000000000000000, 0.9659258262890683122, 1.000000000000000000, 0.9659258262890683122, 1.000000000000000000, 0.9659258262890683122, 1.000000000000000000, 0.9659258262890683122, 1.000000000000000000, 0.9659258262890683122, 1.000000000000000000, 0.9659258262890683122, 1.000000000000000000, 0.9659258262890683122, 1.000000000000000000, 0.9659258262890683122, 1.000000000000000000, 0.9659258262890683122, 1.000000000000000000, 0.9659258262890683122, 1.000000000000000000, 0.9659258262890683122, 1.000000000000000000, 0.9659258262890683122, 1.000000000000000000, 0.9659258262890683122, 1.000000000000000000, 0.9659258262890683122, 1.000000000000000000, 0.9659258262890683122, 1.000000000000000000, 0.9659258262890683122, 1.000000000000000000, 0.9659258262890683122, 1.000000000000000000, 0.9659258262890683122, 1.000000000000000000, 0.9659258262890683122, 1.000000000000000000, 0.9659258262890683122, 1.000000000000000000, 0.9659258262890683122, 1.000000000000000000, 0.9659258262890683122, 1.000000000000000000, 0.9659258262890683122, 1.000000000000000000, 0.9659258262890683122, 1.000000000000000000, 0.9659258262890683122, 1.000000000000000000, 0.9659258262890683122, 1.000000000000000000, 0.9659258262890683122, 1.000000000000000000, 0.9659258262890683122, 1.000000000000000000, 0.9659258262890683122, 1.000000000000000000, 0.9659258262890683122, 1.000000000000000000, 0.9659258262890683122, 1.000000000000000000, 0.9659258262890683122, 1.000000000000000000, 0.9659258262890683122, 1.000000000000000000, 0.9659258262890683122, 1.000000000000000000, 0.9659258262890683122, 1.000000000000000000, 0.9659258262890683122, 1.000000000000000000, 0.9659258262890683122, 1.000000000000000000, 0.9659258262890683122, 1.000000000000000000, 0.9659258262890683122, 1.000000000000000000, 0.9659258262890683122, 1.000000000000000000, 0.9659258262890683122, 1.000000000000000000, 0.9659258262890683122, 1.000000000000000000, 0.9659258262890683122, 1.000000000000000000, 0.9659258262890683122, 1.000000000000000000, 0.9659258262890683122, 1.000000000000000000, 0.9659258262890683122, 1.000000000000000000, 0.9659258262890683122, 1.000000000000000000, 0.9659258262890683122, 1.000000000000000000, 0.9659258262890683122, 1.000000000000000000, 0.9659258262890683122, 1.000000000000000000, 0.9659258262890683122, 1.000000000000000000, 0.9659258262890683122, 1.000000000000000000, 0.9659258262890683122, 1.000000000000000000, 0.9659258262890683122, 1.000000000000000000, 0.9659258262890683122, 1.000000000000000000, 0.9659258262890683122, 1.000000000000000000, 0.9659258262890683122, 1.000000000000000000, 0.9659258262890683122, 1.000000000000000000, 0.9659258262890683122, 1.000000000000000000, 0.9659258262890683122, 1.000000000000000000, 0.9659258262890683122, 1.000000000000000000, 0.9659258262890683122, 1.000000000000000000, 0.9659258262890683122, 1.000000000000000000, 0.9659258262890683122, 1.000000000000000000, 0.9659258262890683122, 1.000000000000000000, 0.9659258262890683122, 1.000000000000000000, 0.9659258262890683122, 1.000000000000000000, 0.9659258262890683122, 1.000000000000000000, 0.9659258262890683122, 1.000000000000000000, 0.9659258262890683122, 1.000000000000000000, 0.9659258262890683122, 1.000000000000000000, 0.9659258262890683122, 1.000000000000000000, 0.9659258262890683122, 1.000000000000000000, 0.9659258262890683122, 1.000000000000000000, 0.9659258262890683122, 1.000000000000000000, 0.9659258262890683122, 1.000000000000000000, 0.9659258262890683122, 1.000000000000000000, 0.9659258262890683122, 1.000000000000000000, 0.9659258262890683122, 1.000000000000000000, 0.9659258262890683122, 1.000000000000000000, 0.9659258262890683122, 1.000000000000000000, 0.9659258262890683122, 1.000000000000000000, 0.9659258262890683122, 1.000000000000000000, 0.9659258262890683122, 1.000000000000000000, 0.9659258262890683122, 1.000000000000000000, 0.9659258262890683122, 1.000000000000000000, 0.9659258262890683122, 1.000000000000000000, 0.9659258262890683122, 1.000000000000000000, 0.9659258262890683122, 1.000000000000000000, 0.9659258262890683122, 1.000000000000000000, 0.9659258262890683122, 1.000000000000000000, 0.9659258262890683122, 1.000000000000000000, 0.9659258262890683122, 1.000000000000000000, 0.9659258262890683122, 1.000000000000000000, 0.9659258262890683122, 1.000000000000000000, 0.9659258262890683122, 1.000000000000000000, 0.9659258262890683122, 1.000000000000000000, 0.9659258262890683122, 1.000000000000000000, 0.9659258262890683122, 1.000000000000000000, 0.9659258262890683122, 1.000000000000000000, 0.9659258262890683122, 1.000000000000000000, 0.9659258262890683122, 1.000000000000000000, 0.9659258262890683122, 1.000000000000000000, 0.9659258262890683122, 1.000000000000000000, 0.9659258262890683122, 1.000000000000000000, 0.9659258262890683122, 1.000000000000000000, 0.9659258262890683122, 1.000000000000000000, 0.9659258262890683122, 1.000000000000000000, 0.9659258262890683122, 1.000000000000000000, 0.9659258262890683122, 1.000000000000000000, 0.9659258262890683122, 1.000000000000000000, 0.9659258262890683122, 1.000000000000000000, 0.9659258262890683122, 1.000000000000000000, 0.9659258262890683122, 1.000000000000000000, 0.9659258262890683122, 1.000000000000000000, 0.9659258262890683122, 1.000000000000000000, 0.9659258262890683122, 1.000000000000000000, 0.9659258262890683122, 1.000000000000000000, 0.9659258262890683122, 1.000000000000000000, 0.9659258262890683122, 1.000000000000000000, 0.9659258262890683122, 1.000000000000000000, 0.9659258262890683122, 1.000000000000000000, 0.9659258262890683122, 1.000000000000000000, 0.9659258262890683122, 1.000000000000000000, 0.9659258262890683122, 1.000000000000000000, 0.9659258262890683122, 1.000000000000000000, 0.9659258262890683122, 1.000000000000000000) ) ) 
 REPRESENTATION_ITEM ( '' )  SURFACE ( )  );
#7390=CARTESIAN_POINT ( 'NONE',  ( 18.67979575497178502, 10.72451020669898547, 69.16557627198102409 ) ) ;
#7391=CARTESIAN_POINT ( 'NONE',  ( 8.314922557961029526, -14.29746914071037800, 110.4177570613523756 ) ) ;
#7394=CARTESIAN_POINT ( 'NONE',  ( -10.72451020669898014, 18.67979575497178502, 90.41557627198103830 ) ) ;
#7395=CARTESIAN_POINT ( 'NONE',  ( 5.719274019375991003, -21.55341960407610458, 112.7072429386476955 ) ) ;
#7396=CARTESIAN_POINT ( 'NONE',  ( -16.55341960407611168, -4.379528057220339221, 41.45724293864769550 ) ) ;
#7397=CARTESIAN_POINT ( 'NONE',  ( -8.224510206698735004, -14.34966873604973081, 29.58442372801901854 ) ) ;
#7398=CARTESIAN_POINT ( 'NONE',  ( 19.05341960407611168, 5.049401038298154454, 53.95724293864770260 ) ) ;
#7399=CARTESIAN_POINT ( 'NONE',  ( -0.05219959533909027116, -19.03943276465977164, 67.49890960531436690 ) ) ;
#7400=CARTESIAN_POINT ( 'NONE',  ( -10.72451020669898014, 18.67979575497178502, 25.41557627198103120 ) ) ;
#7401=CARTESIAN_POINT ( 'NONE',  ( -17.49999999999999645, 5.499999999999997335, 22.00000000000000711 ) ) ;
#7402=CARTESIAN_POINT ( 'NONE',  ( -19.02544592524334988, -5.153800228976617603, 98.95942372801900433 ) ) ;
#7403=CARTESIAN_POINT ( 'NONE',  ( 19.05341960407617918, -5.049401038297876454, 51.04275706135231871 ) ) ;
#7404=CARTESIAN_POINT ( 'NONE',  ( 5.823673210054125526, 21.52544592524343514, 89.79057627198103830 ) ) ;
#7405=CARTESIAN_POINT ( 'NONE',  ( 4.379528057220092307, 16.55341960407617563, 107.2927570613523471 ) ) ;
#7407=CARTESIAN_POINT ( 'NONE',  ( -0.05219959533907301413, -21.53943276465977519, 47.49890960531435979 ) ) ;
#7408=CARTESIAN_POINT ( 'NONE',  ( -15.72974639402197994, 15.80617190586746368, 75.62390960531439532 ) ) ;
#7409=CARTESIAN_POINT ( 'NONE',  ( -13.97604488694547697, 13.89961937509957934, 103.1260903946856473 ) ) ;
#7410=CARTESIAN_POINT ( 'NONE',  ( -19.02544592524342804, 5.153800228976336051, 101.0405762719810241 ) ) ;
#7411=CARTESIAN_POINT ( 'NONE',  ( -10.72451020669870658, -18.67979575497194134, 69.58442372801900433 ) ) ;
#7412=CARTESIAN_POINT ( 'NONE',  ( 19.02544592524343514, -5.153800228976328945, 68.54057627198103830 ) ) ;
#7414=CARTESIAN_POINT ( 'NONE',  ( -16.46253265017160317, 9.564922557960807481, 70.83224293864770971 ) ) ;
#7415=CARTESIAN_POINT ( 'NONE',  ( -14.29746914071049879, 8.314922557960819915, 90.83224293864769550 ) ) ;
#7417=CARTESIAN_POINT ( 'NONE',  ( 19.03943276465977164, 0.05219959533936151252, 106.2510903946856615 ) ) ;
#7418=CARTESIAN_POINT ( 'NONE',  ( 17.44279575226823908, -5.990770900252459619, 83.33557567514316133 ) ) ;
#7419=CARTESIAN_POINT ( 'NONE',  ( 5.153800228976335163, 19.02544592524342804, 69.79057627198103830 ) ) ;
#7420=CARTESIAN_POINT ( 'NONE',  ( 5.719274019375673035, 21.55341960407619339, 87.29275706135236135 ) ) ;
#7421=CARTESIAN_POINT ( 'NONE',  ( 0.05219959533909260263, 19.03943276465977164, 99.99890960531436690 ) ) ;
#7422=CARTESIAN_POINT ( 'NONE',  ( 4.379528057220092307, 16.55341960407617563, 72.29275706135236135 ) ) ;
#7424=CARTESIAN_POINT ( 'NONE',  ( 13.97604488694548053, -13.89961937509957401, 50.62609039468566152 ) ) ;
#7425=CARTESIAN_POINT ( 'NONE',  ( -15.80617190586768217, 15.72974639402176855, 108.1260903946856757 ) ) ;
#7429=CARTESIAN_POINT ( 'NONE',  ( 8.314922557961029526, -14.29746914071037800, 110.4177570613523756 ) ) ;
#7430=CARTESIAN_POINT ( 'NONE',  ( 16.51473224551083163, -9.474510206698727899, 75.83442372801900433 ) ) ;
#7431=CARTESIAN_POINT ( 'NONE',  ( -12.14591786802326823, 12.06949235617739902, 98.12609039468570415 ) ) ;
#7433=CARTESIAN_POINT ( 'NONE',  ( 14.34966873604972726, -8.224510206698740333, 70.83442372801901854 ) ) ;
#7434=CARTESIAN_POINT ( 'NONE',  ( -15.80617190586768217, 15.72974639402176855, 78.12609039468570415 ) ) ;
#7435=CARTESIAN_POINT ( 'NONE',  ( -19.02544592524334988, -5.153800228976617603, 88.95942372801897591 ) ) ;
#7436=CARTESIAN_POINT ( 'NONE',  ( -13.97604488694547697, 13.89961937509957934, 38.12609039468566152 ) ) ;
#7437=CARTESIAN_POINT ( 'NONE',  ( -5.049401038298153566, 19.05341960407611168, 85.20724293864766707 ) ) ;
#7438=CARTESIAN_POINT ( 'NONE',  ( -5.153800228976328057, -19.02544592524343514, 57.29057627198103120 ) ) ;
#7439=CARTESIAN_POINT ( 'NONE',  ( -18.39635199886966177, 5.500000000000103029, 41.01967076359999709 ) ) ;
#7440=CARTESIAN_POINT ( 'NONE',  ( -5.823673210054116645, -21.52544592524344225, 77.29057627198102409 ) ) ;
#7441=CARTESIAN_POINT ( 'NONE',  ( 10.81492255796078972, 18.62759615963270932, 54.58224293864769550 ) ) ;
#7442=CARTESIAN_POINT ( 'NONE',  ( -19.03943276465977164, 0.05219959533909376836, 31.24890960531435979 ) ) ;
#7443=CARTESIAN_POINT ( 'NONE',  ( -14.29746914071037622, -8.314922557961029526, 64.16775706135234714 ) ) ;
#7446=CARTESIAN_POINT ( 'NONE',  ( 21.53943276465977519, 0.05219959533937863772, 51.25109039468568994 ) ) ;
#7447=CARTESIAN_POINT ( 'NONE',  ( -16.53943276465976808, 0.05219959533911058130, 71.24890960531435269 ) ) ;
#7449=CARTESIAN_POINT ( 'NONE',  ( -16.52544592524335698, -4.483927247898792601, 38.95942372801901854 ) ) ;
#7450=CARTESIAN_POINT ( 'NONE',  ( -14.34966873604960291, -8.224510206698953496, 106.6655762719810383 ) ) ;
#7451=CARTESIAN_POINT ( 'NONE',  ( -9.474510206698720793, -16.51473224551083518, 54.58442372801899722 ) ) ;
#7452=CARTESIAN_POINT ( 'NONE',  ( 8.224510206698953496, -14.34966873604960469, 62.91557627198102409 ) ) ;
#7453=CARTESIAN_POINT ( 'NONE',  ( -21.55341960407619339, 5.719274019375674811, 38.54275706135234714 ) ) ;
#7455=CARTESIAN_POINT ( 'NONE',  ( 18.62759615963271287, -10.81492255796078972, 88.33224293864769550 ) ) ;
#7456=CARTESIAN_POINT ( 'NONE',  ( 16.51473224551069308, 9.474510206698969483, 109.1655762719810383 ) ) ;
#7457=CARTESIAN_POINT ( 'NONE',  ( 16.55341960407611168, 4.379528057220329451, 73.95724293864769550 ) ) ;
#7460=CARTESIAN_POINT ( 'NONE',  ( 9.564922557961047289, -16.46253265017146816, 85.41775706135233293 ) ) ;
#7461=CARTESIAN_POINT ( 'NONE',  ( 21.52544592524334988, 5.823673210054432836, 26.45942372801901854 ) ) ;
#7462=CARTESIAN_POINT ( 'NONE',  ( 19.02544592524343514, -5.153800228976328945, 63.54057627198103830 ) ) ;
#7463=CARTESIAN_POINT ( 'NONE',  ( -13.97604488694547697, 13.89961937509957934, 53.12609039468565442 ) ) ;
#7464=CARTESIAN_POINT ( 'NONE',  ( -16.51473224551069308, -9.474510206698971260, 36.66557627198102409 ) ) ;
#7465=CARTESIAN_POINT ( 'NONE',  ( -18.62759615963255300, -10.81492255796106328, 69.16775706135234714 ) ) ;
#7467=CARTESIAN_POINT ( 'NONE',  ( -17.40805194822030089, -6.112264579159311317, 69.16628727489386108 ) ) ;
#7468=CARTESIAN_POINT ( 'NONE',  ( -0.05219959533910754901, -16.53943276465976808, 52.49890960531435979 ) ) ;
#7469=CARTESIAN_POINT ( 'NONE',  ( 13.89961937509977652, -13.97604488694527269, 58.12390960531436690 ) ) ;
#7470=CARTESIAN_POINT ( 'NONE',  ( -21.52544592524343514, 5.823673210054127303, 91.04057627198103830 ) ) ;
#7471=CARTESIAN_POINT ( 'NONE',  ( -9.564922557960796823, -16.46253265017161027, 57.08224293864769550 ) ) ;
#7473=CARTESIAN_POINT ( 'NONE',  ( 21.55341960407610458, 5.719274019375980345, 78.95724293864769550 ) ) ;
#7474=CARTESIAN_POINT ( 'NONE',  ( -21.53943276465977519, -0.05219959533937600094, 93.75109039468567573 ) ) ;
#7475=CARTESIAN_POINT ( 'NONE',  ( -5.049401038298153566, 19.05341960407611168, 25.20724293864768484 ) ) ;
#7476=CARTESIAN_POINT ( 'NONE',  ( -14.34966873604972548, 8.224510206698743886, 98.33442372801901854 ) ) ;
#7477=CARTESIAN_POINT ( 'NONE',  ( 4.483927247898545687, 16.52544592524342804, 99.79057627198103830 ) ) ;
#7478=CARTESIAN_POINT ( 'NONE',  ( 5.049401038297881783, 19.05341960407617563, 87.29275706135234714 ) ) ;
#7480=CARTESIAN_POINT ( 'NONE',  ( -15.80617190586745835, -15.72974639402198527, 111.8739096053143669 ) ) ;
#7481=CARTESIAN_POINT ( 'NONE',  ( 0.05219959533936267826, -19.03943276465977164, 40.00109039468566152 ) ) ;
#7482=CARTESIAN_POINT ( 'NONE',  ( 0.05219959533934541429, -16.53943276465976808, 100.0010903946857042 ) ) ;
#7483=CARTESIAN_POINT ( 'NONE',  ( -9.474510206698720793, -16.51473224551083518, 24.58442372801900078 ) ) ;
#7484=CARTESIAN_POINT ( 'NONE',  ( -16.51473224551069308, -9.474510206698971260, 101.6655762719810241 ) ) ;
#7485=CARTESIAN_POINT ( 'NONE',  ( 21.52544592524344225, -5.823673210054117533, 58.54057627198103120 ) ) ;
#7487=CARTESIAN_POINT ( 'NONE',  ( -13.97604488694527625, -13.89961937509977652, 26.87390960531434558 ) ) ;
#7488=CARTESIAN_POINT ( 'NONE',  ( 5.823673210054444382, -21.52544592524334988, 110.2094237280190185 ) ) ;
#7489=CARTESIAN_POINT ( 'NONE',  ( -8.224510206698735004, -14.34966873604973081, 69.58442372801900433 ) ) ;
#7490=CARTESIAN_POINT ( 'NONE',  ( -5.823673210054431948, 21.52544592524334988, 22.70942372801901499 ) ) ;
#7491=CARTESIAN_POINT ( 'NONE',  ( 16.52544592524335698, 4.483927247898782831, 36.45942372801901143 ) ) ;
#7492=CARTESIAN_POINT ( 'NONE',  ( -19.02544592524342804, 5.153800228976336051, 106.0405762719810241 ) ) ;
#7493=CARTESIAN_POINT ( 'NONE',  ( 19.05341960407611168, 5.049401038298154454, 43.95724293864769550 ) ) ;
#7494=CARTESIAN_POINT ( 'NONE',  ( -16.51473224551069308, -9.474510206698971260, 71.66557627198102409 ) ) ;
#7495=CARTESIAN_POINT ( 'NONE',  ( -16.55341960407617563, 4.379528057220093196, 53.54275706135234714 ) ) ;
#7496=CARTESIAN_POINT ( 'NONE',  ( 14.29746914071049879, -8.314922557960816363, 88.33224293864769550 ) ) ;
#7497=CARTESIAN_POINT ( 'NONE',  ( -16.53943276465976808, -0.05219959533934237506, 103.7510903946857042 ) ) ;
#7499=CARTESIAN_POINT ( 'NONE',  ( -10.81492255796105439, 18.62759615963255655, 57.91775706135234714 ) ) ;
#7500=CARTESIAN_POINT ( 'NONE',  ( 13.97604488694527802, 13.89961937509977652, 74.37390960531436690 ) ) ;
#7501=CARTESIAN_POINT ( 'NONE',  ( 16.51473224551069308, 9.474510206698969483, 59.16557627198102409 ) ) ;
#7502=CARTESIAN_POINT ( 'NONE',  ( 5.049401038298161559, -19.05341960407611168, 92.70724293864769550 ) ) ;
#7503=CARTESIAN_POINT ( 'NONE',  ( -0.05219959533910754901, -16.53943276465976808, 42.49890960531435979 ) ) ;
#7504=CARTESIAN_POINT ( 'NONE',  ( 16.53943276465976808, 0.05219959533934440121, 101.2510903946856757 ) ) ;
#7505=EDGE_LOOP ( 'NONE', ( #18975, #111133, #32322, #195295, #124314, #19951 ) ) ;
#7506=CARTESIAN_POINT ( 'NONE',  ( 9.474510206698729675, 16.51473224551082808, 42.08442372801900433 ) ) ;
#7507=CARTESIAN_POINT ( 'NONE',  ( -19.02544592524342804, 5.153800228976336051, 111.0405762719810099 ) ) ;
#7508=CARTESIAN_POINT ( 'NONE',  ( -16.46253265017160317, 9.564922557960807481, 65.83224293864769550 ) ) ;
#7509=CARTESIAN_POINT ( 'NONE',  ( -19.03943276465977164, -0.05219959533935918106, 33.75109039468566863 ) ) ;
#7511=CARTESIAN_POINT ( 'NONE',  ( 19.01533133064925352, -5.499999999999438671, 71.26586590595739779 ) ) ;
#7512=CARTESIAN_POINT ( 'NONE',  ( 13.97604488694548053, -13.89961937509957401, 65.62609039468567573 ) ) ;
#7513=CARTESIAN_POINT ( 'NONE',  ( 14.29746914071037800, 8.314922557961029526, 66.66775706135234714 ) ) ;
#7514=CARTESIAN_POINT ( 'NONE',  ( 17.40861289039003523, 6.110651285853315962, 93.87232470827436259 ) ) ;
#7515=CARTESIAN_POINT ( 'NONE',  ( 9.564922557960805705, 16.46253265017160317, 84.58224293864769550 ) ) ;
#7516=CARTESIAN_POINT ( 'NONE',  ( -18.62759615963255300, -10.81492255796106328, 29.16775706135234003 ) ) ;
#7517=CARTESIAN_POINT ( 'NONE',  ( -19.05341960407617563, 5.049401038297882671, 78.54275706135233293 ) ) ;
#7518=CARTESIAN_POINT ( 'NONE',  ( 13.97604488694527802, 13.89961937509977652, 114.3739096053143669 ) ) ;
#7519=CARTESIAN_POINT ( 'NONE',  ( 0.05219959533909260263, 19.03943276465977164, 39.99890960531436690 ) ) ;
#7521=CARTESIAN_POINT ( 'NONE',  ( -9.474510206698964154, 16.51473224551069663, 85.41557627198102409 ) ) ;
#7522=CARTESIAN_POINT ( 'NONE',  ( 16.55341960407611168, 4.379528057220329451, 43.95724293864769550 ) ) ;
#7523=CARTESIAN_POINT ( 'NONE',  ( -5.049401038298153566, 19.05341960407611168, 35.20724293864768839 ) ) ;
#7524=CARTESIAN_POINT ( 'NONE',  ( 13.97604488694548053, -13.89961937509957401, 45.62609039468566863 ) ) ;
#7525=CARTESIAN_POINT ( 'NONE',  ( -16.55341960407611168, -4.379528057220339221, 81.45724293864769550 ) ) ;
#7526=CARTESIAN_POINT ( 'NONE',  ( 5.719274019375673035, 21.55341960407619339, 107.2927570613523471 ) ) ;
#7527=CARTESIAN_POINT ( 'NONE',  ( 13.89961937509977652, -13.97604488694527269, 53.12390960531434558 ) ) ;
#7528=CARTESIAN_POINT ( 'NONE',  ( -5.719274019375978568, 21.55341960407610458, 60.20724293864768839 ) ) ;
#7529=CARTESIAN_POINT ( 'NONE',  ( -4.483927247898539470, -16.52544592524342804, 57.29057627198103120 ) ) ;
#7530=CARTESIAN_POINT ( 'NONE',  ( -13.89961937509957401, -13.97604488694547875, 24.37609039468565442 ) ) ;
#7531=CARTESIAN_POINT ( 'NONE',  ( -13.97604488694527625, -13.89961937509977652, 106.8739096053143669 ) ) ;
#7532=CARTESIAN_POINT ( 'NONE',  ( -15.80617190586745835, -15.72974639402198527, 21.87390960531436690 ) ) ;
#7533=CARTESIAN_POINT ( 'NONE',  ( -13.89961937509977652, 13.97604488694528158, 50.62390960531435979 ) ) ;
#7534=CARTESIAN_POINT ( 'NONE',  ( -16.46253265017160317, 9.564922557960807481, 25.83224293864769194 ) ) ;
#7535=CARTESIAN_POINT ( 'NONE',  ( -12.06949235617756955, 12.14591786802309770, 85.62390960531436690 ) ) ;
#7536=CARTESIAN_POINT ( 'NONE',  ( 21.53943276465977519, -0.05219959533907433946, 103.7489096053143669 ) ) ;
#7537=CARTESIAN_POINT ( 'NONE',  ( 5.049401038298161559, -19.05341960407611168, 107.7072429386476955 ) ) ;
#7538=CARTESIAN_POINT ( 'NONE',  ( -15.72974639402197994, 15.80617190586746368, 115.6239096053143669 ) ) ;
#7539=CARTESIAN_POINT ( 'NONE',  ( 19.03943276465977164, -0.05219959533909143690, 103.7489096053143669 ) ) ;
#7540=CARTESIAN_POINT ( 'NONE',  ( -16.51473224551069308, -9.474510206698971260, 21.66557627198102765 ) ) ;
#7541=CARTESIAN_POINT ( 'NONE',  ( -5.719274019375665041, -21.55341960407619695, 74.79275706135234714 ) ) ;
#7542=CARTESIAN_POINT ( 'NONE',  ( -15.80617190586745835, -15.72974639402198527, 91.87390960531436690 ) ) ;
#7546=CARTESIAN_POINT ( 'NONE',  ( -14.34966873604972548, 8.224510206698743886, 38.33442372801900433 ) ) ;
#7547=CARTESIAN_POINT ( 'NONE',  ( -8.224510206698948167, 14.34966873604960824, 105.4155762719810383 ) ) ;
#7548=CARTESIAN_POINT ( 'NONE',  ( 19.01533133064921799, -5.499999999999651834, 51.26586590595738357 ) ) ;
#7549=CARTESIAN_POINT ( 'NONE',  ( -9.564922557960796823, -16.46253265017161027, 62.08224293864769550 ) ) ;
#7550=CARTESIAN_POINT ( 'NONE',  ( -0.05219959533910754901, -16.53943276465976808, 97.49890960531436690 ) ) ;
#7552=CARTESIAN_POINT ( 'NONE',  ( 15.80617190586746368, 15.72974639402197994, 29.37390960531435269 ) ) ;
#7553=CARTESIAN_POINT ( 'NONE',  ( 0.05219959533910956823, 16.53943276465976808, 69.99890960531435269 ) ) ;
#7554=CARTESIAN_POINT ( 'NONE',  ( 16.52544592524335698, 4.483927247898782831, 21.45942372801901499 ) ) ;
#7555=CARTESIAN_POINT ( 'NONE',  ( 5.719274019375673035, 21.55341960407619339, 67.29275706135234714 ) ) ;
#7556=CARTESIAN_POINT ( 'NONE',  ( 16.81555441253551919, -7.025013491695474954, 78.13685445334255064 ) ) ;
#7557=CARTESIAN_POINT ( 'NONE',  ( -16.46253265017160317, 9.564922557960807481, 110.8322429386476955 ) ) ;
#7558=CARTESIAN_POINT ( 'NONE',  ( -0.05219959533934338120, 16.53943276465976808, 102.5010903946856899 ) ) ;
#7559=CARTESIAN_POINT ( 'NONE',  ( 13.89961937509977652, -13.97604488694527269, 43.12390960531434558 ) ) ;
#7560=CARTESIAN_POINT ( 'NONE',  ( -19.05341960407611168, -5.049401038298163336, 86.45724293864769550 ) ) ;
#7561=CARTESIAN_POINT ( 'NONE',  ( 0.05219959533907565091, 21.53943276465977519, 99.99890960531436690 ) ) ;
#7562=CARTESIAN_POINT ( 'NONE',  ( 4.483927247898790824, -16.52544592524335698, 20.20942372801900788 ) ) ;
#7563=CARTESIAN_POINT ( 'NONE',  ( 16.52544592524342804, -4.483927247898539470, 63.54057627198103830 ) ) ;
#7564=CARTESIAN_POINT ( 'NONE',  ( -21.55341960407619339, 5.719274019375674811, 78.54275706135236135 ) ) ;
#7565=CARTESIAN_POINT ( 'NONE',  ( -4.379528057220086978, -16.55341960407618274, 104.7927570613523898 ) ) ;
#7566=CARTESIAN_POINT ( 'NONE',  ( 16.88567814943192857, -6.947325034625397855, 46.20998877347406619 ) ) ;
#7568=CARTESIAN_POINT ( 'NONE',  ( -12.14591786802309592, -12.06949235617757132, 31.87390960531435979 ) ) ;
#7569=CARTESIAN_POINT ( 'NONE',  ( 4.483927247898790824, -16.52544592524335698, 70.20942372801904696 ) ) ;
#7570=CARTESIAN_POINT ( 'NONE',  ( 19.05341960407611168, 5.049401038298154454, 88.95724293864769550 ) ) ;
#7571=CARTESIAN_POINT ( 'NONE',  ( 0.05219959533909260263, 19.03943276465977164, 84.99890960531436690 ) ) ;
#7572=CARTESIAN_POINT ( 'NONE',  ( -21.53943276465977519, -0.05219959533937600094, 83.75109039468568994 ) ) ;
#7573=CARTESIAN_POINT ( 'NONE',  ( 8.314922557961029526, -14.29746914071037800, 90.41775706135236135 ) ) ;
#7574=CARTESIAN_POINT ( 'NONE',  ( -16.53943276465976808, 0.05219959533911058130, 66.24890960531436690 ) ) ;
#7575=CARTESIAN_POINT ( 'NONE',  ( 9.474510206698971260, -16.51473224551069308, 67.91557627198102409 ) ) ;
#7577=CARTESIAN_POINT ( 'NONE',  ( -13.89961937509957401, -13.97604488694547875, 109.3760903946856331 ) ) ;
#7578=CARTESIAN_POINT ( 'NONE',  ( 12.06949235617757843, -12.14591786802309237, 108.1239096053143811 ) ) ;
#7579=CARTESIAN_POINT ( 'NONE',  ( -19.03943276465977164, 0.05219959533909376836, 81.24890960531436690 ) ) ;
#7580=CARTESIAN_POINT ( 'NONE',  ( -13.97604488694547697, 13.89961937509957934, 113.1260903946856757 ) ) ;
#7582=CARTESIAN_POINT ( 'NONE',  ( 16.51473224551083163, -9.474510206698727899, 20.83442372801899722 ) ) ;
#7583=CARTESIAN_POINT ( 'NONE',  ( 16.55341960407618274, -4.379528057220086978, 81.04275706135236135 ) ) ;
#7584=CARTESIAN_POINT ( 'NONE',  ( -13.97604488694547697, 13.89961937509957934, 93.12609039468566152 ) ) ;
#7585=CARTESIAN_POINT ( 'NONE',  ( 5.049401038298161559, -19.05341960407611168, 22.70724293864769194 ) ) ;
#7586=CARTESIAN_POINT ( 'NONE',  ( -4.379528057220086978, -16.55341960407618274, 64.79275706135234714 ) ) ;
#7588=CARTESIAN_POINT ( 'NONE',  ( -5.049401038297874678, -19.05341960407617918, 49.79275706135231871 ) ) ;
#7589=CARTESIAN_POINT ( 'NONE',  ( 18.67979575497194134, -10.72451020669871369, 100.8344237280190185 ) ) ;
#7590=CARTESIAN_POINT ( 'NONE',  ( 0.05219959533909260263, 19.03943276465977164, 34.99890960531435979 ) ) ;
#7591=CARTESIAN_POINT ( 'NONE',  ( 16.46253265017160672, -9.564922557960803928, 78.33224293864769550 ) ) ;
#7592=CARTESIAN_POINT ( 'NONE',  ( 16.53943276465976808, -0.05219959533910856209, 68.74890960531435269 ) ) ;
#7593=CARTESIAN_POINT ( 'NONE',  ( -15.72974639402176322, -15.80617190586768395, 84.37609039468570415 ) ) ;
#7595=CARTESIAN_POINT ( 'NONE',  ( 5.153800228976615827, -19.02544592524334988, 60.20942372801899012 ) ) ;
#7596=CARTESIAN_POINT ( 'NONE',  ( -5.049401038297874678, -19.05341960407617918, 39.79275706135232582 ) ) ;
#7597=CARTESIAN_POINT ( 'NONE',  ( 21.53943276465977519, -0.05219959533907433946, 33.74890960531436690 ) ) ;
#7598=CARTESIAN_POINT ( 'NONE',  ( 15.72974639402176855, 15.80617190586768217, 96.87609039468568994 ) ) ;
#7599=CARTESIAN_POINT ( 'NONE',  ( 13.97604488694527802, 13.89961937509977652, 74.37390960531436690 ) ) ;
#7600=CARTESIAN_POINT ( 'NONE',  ( 21.52544592524334988, 5.823673210054432836, 111.4594237280190328 ) ) ;
#7601=CARTESIAN_POINT ( 'NONE',  ( -21.53943276465977519, 0.05219959533907696930, 51.24890960531436690 ) ) ;
#7602=CARTESIAN_POINT ( 'NONE',  ( 13.89961937509977652, -13.97604488694527269, 93.12390960531436690 ) ) ;
#7603=CARTESIAN_POINT ( 'NONE',  ( 9.564922557961047289, -16.46253265017146816, 80.41775706135234714 ) ) ;
#7604=CARTESIAN_POINT ( 'NONE',  ( 19.02544592524343514, -5.153800228976328945, 108.5405762719810383 ) ) ;
#7605=CARTESIAN_POINT ( 'NONE',  ( -13.89961937509957401, -13.97604488694547875, 94.37609039468566152 ) ) ;
#7606=CARTESIAN_POINT ( 'NONE',  ( -14.34966873604972548, 8.224510206698743886, 48.33442372801902565 ) ) ;
#7607=CARTESIAN_POINT ( 'NONE',  ( -12.06949235617756955, 12.14591786802309770, 100.6239096053143811 ) ) ;
#7608=CARTESIAN_POINT ( 'NONE',  ( 13.89961937509977652, -13.97604488694527269, 88.12390960531438111 ) ) ;
#7610=CARTESIAN_POINT ( 'NONE',  ( -15.80617190586745835, -15.72974639402198527, 61.87390960531436690 ) ) ;
#7611=CARTESIAN_POINT ( 'NONE',  ( 8.224510206698742110, 14.34966873604972548, 37.08442372801901143 ) ) ;
#7612=CARTESIAN_POINT ( 'NONE',  ( 18.62759615963255655, 10.81492255796105972, 36.66775706135234714 ) ) ;
#7613=CARTESIAN_POINT ( 'NONE',  ( -15.72974639402176322, -15.80617190586768395, 79.37609039468567573 ) ) ;
#7614=CARTESIAN_POINT ( 'NONE',  ( 14.34966873604972726, -8.224510206698740333, 80.83442372801901854 ) ) ;
#7616=CARTESIAN_POINT ( 'NONE',  ( 19.02544592524343514, -5.153800228976328945, 78.54057627198099567 ) ) ;
#7617=CARTESIAN_POINT ( 'NONE',  ( 16.52544592524342804, -4.483927247898539470, 73.54057627198102409 ) ) ;
#7618=CARTESIAN_POINT ( 'NONE',  ( -4.379528057220086978, -16.55341960407618274, 109.7927570613523613 ) ) ;
#7619=CARTESIAN_POINT ( 'NONE',  ( 9.564922557961047289, -16.46253265017146816, 60.41775706135233293 ) ) ;
#7620=CARTESIAN_POINT ( 'NONE',  ( 21.55341960407619695, -5.719274019375665929, 31.04275706135234714 ) ) ;
#7621=CARTESIAN_POINT ( 'NONE',  ( -4.483927247898539470, -16.52544592524342804, 77.29057627198102409 ) ) ;
#7622=CARTESIAN_POINT ( 'NONE',  ( 0.05219959533909260263, 19.03943276465977164, 99.99890960531436690 ) ) ;
#7623=CARTESIAN_POINT ( 'NONE',  ( -16.55341960407617563, 4.379528057220093196, 108.5427570613523756 ) ) ;
#7624=CARTESIAN_POINT ( 'NONE',  ( -15.72974639402176322, -15.80617190586768395, 74.37609039468568994 ) ) ;
#7625=CARTESIAN_POINT ( 'NONE',  ( -0.05219959533934338120, 16.53943276465976808, 47.50109039468568994 ) ) ;
#7626=CARTESIAN_POINT ( 'NONE',  ( -10.72451020669870658, -18.67979575497194134, 34.58442372801900433 ) ) ;
#7627=CARTESIAN_POINT ( 'NONE',  ( -16.55341960407611168, -4.379528057220339221, 71.45724293864769550 ) ) ;
#7629=CARTESIAN_POINT ( 'NONE',  ( -5.719274019375978568, 21.55341960407610458, 110.2072429386477239 ) ) ;
#7630=CARTESIAN_POINT ( 'NONE',  ( 16.53943276465976808, -0.05219959533910856209, 93.74890960531436690 ) ) ;
#7631=CARTESIAN_POINT ( 'NONE',  ( -19.52851543214742236, -5.500000000000036415, 50.39357721762583964 ) ) ;
#7632=CARTESIAN_POINT ( 'NONE',  ( -4.379528057220328563, 16.55341960407611168, 55.20724293864770260 ) ) ;
#7633=CARTESIAN_POINT ( 'NONE',  ( -5.049401038298153566, 19.05341960407611168, 30.20724293864768839 ) ) ;
#7634=CARTESIAN_POINT ( 'NONE',  ( -10.81492255796078084, -18.62759615963271287, 47.08224293864770260 ) ) ;
#7635=CARTESIAN_POINT ( 'NONE',  ( 16.55341960407611168, 4.379528057220329451, 83.95724293864770971 ) ) ;
#7636=CARTESIAN_POINT ( 'NONE',  ( 18.67979575497178502, 10.72451020669898547, 84.16557627198103830 ) ) ;
#7637=CARTESIAN_POINT ( 'NONE',  ( 19.03943276465977164, -0.05219959533909143690, 93.74890960531435269 ) ) ;
#7638=CARTESIAN_POINT ( 'NONE',  ( 19.05341960407611168, 5.049401038298154454, 38.95724293864767418 ) ) ;
#7639=CARTESIAN_POINT ( 'NONE',  ( -16.46253265017146816, -9.564922557961047289, 79.16775706135234714 ) ) ;
#7640=CARTESIAN_POINT ( 'NONE',  ( -18.62759615963255300, -10.81492255796106328, 59.16775706135234714 ) ) ;
#7641=CARTESIAN_POINT ( 'NONE',  ( 0.05219959533907565091, 21.53943276465977519, 64.99890960531435269 ) ) ;
#7642=CARTESIAN_POINT ( 'NONE',  ( 0.05219959533909260263, 19.03943276465977164, 34.99890960531435979 ) ) ;
#7643=CARTESIAN_POINT ( 'NONE',  ( -13.97604488694527625, -13.89961937509977652, 76.87390960531433848 ) ) ;
#7644=ORIENTED_EDGE ( 'NONE', *, *, #25526, .F. ) ;
#7645=CARTESIAN_POINT ( 'NONE',  ( 14.29746914071037800, 8.314922557961029526, 56.66775706135235424 ) ) ;
#7646=CARTESIAN_POINT ( 'NONE',  ( 5.719274019375673035, 21.55341960407619339, 37.29275706135235424 ) ) ;
#7647=CARTESIAN_POINT ( 'NONE',  ( 15.72974639402176855, 15.80617190586768217, 76.87609039468567573 ) ) ;
#7648=CARTESIAN_POINT ( 'NONE',  ( 5.049401038298161559, -19.05341960407611168, 112.7072429386476813 ) ) ;
#7649=CARTESIAN_POINT ( 'NONE',  ( -18.62759615963270932, 10.81492255796079327, 80.83224293864769550 ) ) ;
#7650=CARTESIAN_POINT ( 'NONE',  ( 18.67979575497194134, -10.72451020669871369, 20.83442372801901143 ) ) ;
#7651=CARTESIAN_POINT ( 'NONE',  ( 4.483927247898790824, -16.52544592524335698, 55.20942372801902565 ) ) ;
#7652=CARTESIAN_POINT ( 'NONE',  ( 18.62759615963271287, -10.81492255796078972, 48.33224293864770260 ) ) ;
#7653=CARTESIAN_POINT ( 'NONE',  ( 5.823673210054444382, -21.52544592524334988, 110.2094237280190185 ) ) ;
#7654=CARTESIAN_POINT ( 'NONE',  ( 16.51473224551069308, 9.474510206698969483, 54.16557627198103120 ) ) ;
#7655=CARTESIAN_POINT ( 'NONE',  ( -16.46253265017160317, 9.564922557960807481, 110.8322429386476955 ) ) ;
#7656=CARTESIAN_POINT ( 'NONE',  ( -5.049401038298153566, 19.05341960407611168, 90.20724293864766707 ) ) ;
#7658=CARTESIAN_POINT ( 'NONE',  ( -13.97604488694547697, 13.89961937509957934, 63.12609039468566152 ) ) ;
#7659=CARTESIAN_POINT ( 'NONE',  ( 10.72451020669898902, -18.67979575497178502, 47.91557627198102409 ) ) ;
#7660=CARTESIAN_POINT ( 'NONE',  ( 12.06949235617757843, -12.14591786802309237, 28.12390960531435979 ) ) ;
#7661=CARTESIAN_POINT ( 'NONE',  ( 19.05341960407617918, -5.049401038297876454, 106.0427570613523471 ) ) ;
#7662=CARTESIAN_POINT ( 'NONE',  ( 17.49999999999999289, 5.500000000000007994, 83.78230962303564411 ) ) ;
#7663=CARTESIAN_POINT ( 'NONE',  ( 5.153800228976615827, -19.02544592524334988, 20.20942372801899722 ) ) ;
#7664=CARTESIAN_POINT ( 'NONE',  ( -19.03943276465977164, -0.05219959533935918106, 98.75109039468567573 ) ) ;
#7665=CARTESIAN_POINT ( 'NONE',  ( -0.05219959533907301413, -21.53943276465977519, 82.49890960531436690 ) ) ;
#7666=CARTESIAN_POINT ( 'NONE',  ( -13.97604488694547697, 13.89961937509957934, 58.12609039468566863 ) ) ;
#7668=CARTESIAN_POINT ( 'NONE',  ( -19.05341960407611168, -5.049401038298163336, 61.45724293864769550 ) ) ;
#7669=CARTESIAN_POINT ( 'NONE',  ( 16.52544592524342804, -4.483927247898539470, 68.54057627198103830 ) ) ;
#7670=CARTESIAN_POINT ( 'NONE',  ( 13.89961937509977652, -13.97604488694527269, 48.12390960531435979 ) ) ;
#7671=CARTESIAN_POINT ( 'NONE',  ( -8.224510206698948167, 14.34966873604960824, 45.41557627198103830 ) ) ;
#7673=CARTESIAN_POINT ( 'NONE',  ( -14.34966873604960291, -8.224510206698953496, 31.66557627198102054 ) ) ;
#7674=CARTESIAN_POINT ( 'NONE',  ( 19.03943276465977164, -0.05219959533909143690, 58.74890960531435979 ) ) ;
#7675=CARTESIAN_POINT ( 'NONE',  ( 13.97604488694548053, -13.89961937509957401, 30.62609039468566863 ) ) ;
#7676=CARTESIAN_POINT ( 'NONE',  ( -4.483927247898782831, 16.52544592524335698, 37.70942372801900433 ) ) ;
#7677=CARTESIAN_POINT ( 'NONE',  ( -21.53943276465977519, 0.05219959533907696930, 56.24890960531436690 ) ) ;
#7678=CARTESIAN_POINT ( 'NONE',  ( -21.55341960407619339, 5.719274019375674811, 103.5427570613523613 ) ) ;
#7679=VERTEX_POINT ( 'NONE', #61022 ) ;
#7680=CARTESIAN_POINT ( 'NONE',  ( -16.46253265017160317, 9.564922557960807481, 65.83224293864769550 ) ) ;
#7681=CARTESIAN_POINT ( 'NONE',  ( -9.474510206698964154, 16.51473224551069663, 115.4155762719810241 ) ) ;
#7682=CARTESIAN_POINT ( 'NONE',  ( -16.46253265017160317, 9.564922557960807481, 90.83224293864769550 ) ) ;
#7684=CARTESIAN_POINT ( 'NONE',  ( 18.62759615963255655, 10.81492255796105972, 31.66775706135234358 ) ) ;
#7685=CARTESIAN_POINT ( 'NONE',  ( -16.53943276465976808, 0.05219959533911058130, 96.24890960531435269 ) ) ;
#7686=CARTESIAN_POINT ( 'NONE',  ( 15.72974639402199770, -15.80617190586745480, 93.12390960531436690 ) ) ;
#7687=CARTESIAN_POINT ( 'NONE',  ( -19.02544592524342804, 5.153800228976336051, 66.04057627198103830 ) ) ;
#7688=CARTESIAN_POINT ( 'NONE',  ( 19.05341960407611168, 5.049401038298154454, 73.95724293864768129 ) ) ;
#7689=CARTESIAN_POINT ( 'NONE',  ( -10.81492255796078084, -18.62759615963271287, 112.0822429386477097 ) ) ;
#7690=ORIENTED_EDGE ( 'NONE', *, *, #48933, .F. ) ;
#7691=CARTESIAN_POINT ( 'NONE',  ( 0.05219959533909260263, 19.03943276465977164, 74.99890960531435269 ) ) ;
#7695=CARTESIAN_POINT ( 'NONE',  ( 16.55341960407611168, 4.379528057220329451, 108.9572429386476955 ) ) ;
#7696=CARTESIAN_POINT ( 'NONE',  ( -19.03943276465977164, 0.05219959533909376836, 26.24890960531435624 ) ) ;
#7697=CARTESIAN_POINT ( 'NONE',  ( -9.564922557961040184, 16.46253265017147172, 97.91775706135233293 ) ) ;
#7698=CARTESIAN_POINT ( 'NONE',  ( -8.314922557960811034, -14.29746914071050412, 102.0822429386476955 ) ) ;
#7699=CARTESIAN_POINT ( 'NONE',  ( 18.67979575497194134, -10.72451020669871369, 70.83442372801901854 ) ) ;
#7700=CARTESIAN_POINT ( 'NONE',  ( -0.05219959533909027116, -19.03943276465977164, 67.49890960531436690 ) ) ;
#7701=CARTESIAN_POINT ( 'NONE',  ( 21.52544592524334988, 5.823673210054432836, 36.45942372801901143 ) ) ;
#7702=CARTESIAN_POINT ( 'NONE',  ( 10.72451020669898902, -18.67979575497178502, 112.9155762719810383 ) ) ;
#7704=CARTESIAN_POINT ( 'NONE',  ( 9.474510206698971260, -16.51473224551069308, 77.91557627198103830 ) ) ;
#7706=CARTESIAN_POINT ( 'NONE',  ( 16.52544592524335698, 4.483927247898782831, 26.45942372801901854 ) ) ;
#7707=CARTESIAN_POINT ( 'NONE',  ( 15.80617190586746368, 15.72974639402197994, 24.37390960531435979 ) ) ;
#7708=CARTESIAN_POINT ( 'NONE',  ( -0.05219959533937732626, 21.53943276465977519, 67.50109039468568994 ) ) ;
#7709=CARTESIAN_POINT ( 'NONE',  ( -9.474510206698964154, 16.51473224551069663, 105.4155762719810383 ) ) ;
#7710=CARTESIAN_POINT ( 'NONE',  ( -5.049401038297874678, -19.05341960407617918, 94.79275706135230450 ) ) ;
#7711=CARTESIAN_POINT ( 'NONE',  ( 5.153800228976335163, 19.02544592524342804, 49.79057627198100988 ) ) ;
#7712=CARTESIAN_POINT ( 'NONE',  ( 19.05341960407611168, 5.049401038298154454, 73.95724293864768129 ) ) ;
#7713=CARTESIAN_POINT ( 'NONE',  ( 14.34966873604960469, 8.224510206698951720, 99.16557627198100988 ) ) ;
#7714=CARTESIAN_POINT ( 'NONE',  ( 13.97604488694527802, 13.89961937509977652, 99.37390960531436690 ) ) ;
#7715=CARTESIAN_POINT ( 'NONE',  ( -4.483927247898539470, -16.52544592524342804, 97.29057627198105251 ) ) ;
#7716=CARTESIAN_POINT ( 'NONE',  ( 9.564922557960805705, 16.46253265017160317, 104.5822429386476955 ) ) ;
#7717=CARTESIAN_POINT ( 'NONE',  ( -8.224510206698948167, 14.34966873604960824, 45.41557627198103830 ) ) ;
#7718=CARTESIAN_POINT ( 'NONE',  ( 19.05341960407611168, 5.049401038298154454, 43.95724293864769550 ) ) ;
#7719=CARTESIAN_POINT ( 'NONE',  ( -0.05219959533937732626, 21.53943276465977519, 52.50109039468567573 ) ) ;
#7720=CARTESIAN_POINT ( 'NONE',  ( 13.89961937509957401, 13.97604488694547697, 96.87609039468566152 ) ) ;
#7721=CARTESIAN_POINT ( 'NONE',  ( 14.34966873604960469, 8.224510206698951720, 44.16557627198103120 ) ) ;
#7722=CARTESIAN_POINT ( 'NONE',  ( 18.67979575497178502, 10.72451020669898547, 104.1655762719810241 ) ) ;
#7723=CARTESIAN_POINT ( 'NONE',  ( -0.05219959533907301413, -21.53943276465977519, 52.49890960531435979 ) ) ;
#7724=CARTESIAN_POINT ( 'NONE',  ( -19.03943276465977164, 0.05219959533909376836, 111.2489096053143669 ) ) ;
#7725=CARTESIAN_POINT ( 'NONE',  ( -14.29746914071049879, 8.314922557960819915, 85.83224293864768129 ) ) ;
#7726=CARTESIAN_POINT ( 'NONE',  ( -19.03943276465977164, 0.05219959533909376836, 51.24890960531436690 ) ) ;
#7727=CARTESIAN_POINT ( 'NONE',  ( -8.224510206698735004, -14.34966873604973081, 109.5844237280190328 ) ) ;
#7728=CARTESIAN_POINT ( 'NONE',  ( 8.314922557961029526, -14.29746914071037800, 100.4177570613523471 ) ) ;
#7729=CARTESIAN_POINT ( 'NONE',  ( 14.29746914071037800, 8.314922557961029526, 86.66775706135234714 ) ) ;
#7730=CARTESIAN_POINT ( 'NONE',  ( 5.153800228976615827, -19.02544592524334988, 45.20942372801901143 ) ) ;
#7731=LINE ( 'NONE', #22921, #105403 ) ;
#7732=CARTESIAN_POINT ( 'NONE',  ( 5.153800228976335163, 19.02544592524342804, 104.7905762719809957 ) ) ;
#7733=CARTESIAN_POINT ( 'NONE',  ( 16.46253265017160672, -9.564922557960803928, 78.33224293864769550 ) ) ;
#7734=CARTESIAN_POINT ( 'NONE',  ( -16.46253265017160317, 9.564922557960807481, 35.83224293864768839 ) ) ;
#7735=CARTESIAN_POINT ( 'NONE',  ( 14.29746914071049879, -8.314922557960816363, 43.33224293864769550 ) ) ;
#7736=CARTESIAN_POINT ( 'NONE',  ( 13.97604488694527802, 13.89961937509977652, 114.3739096053143669 ) ) ;
#7737=CARTESIAN_POINT ( 'NONE',  ( 19.03943276465977164, -0.05219959533909143690, 103.7489096053143669 ) ) ;
#7738=CARTESIAN_POINT ( 'NONE',  ( 18.67979575497178502, 10.72451020669898547, 34.16557627198102409 ) ) ;
#7739=CARTESIAN_POINT ( 'NONE',  ( -0.05219959533910754901, -16.53943276465976808, 87.49890960531436690 ) ) ;
#7740=CARTESIAN_POINT ( 'NONE',  ( 16.53943276465976808, 0.05219959533934440121, 36.25109039468567573 ) ) ;
#7741=CARTESIAN_POINT ( 'NONE',  ( -12.14591786802309592, -12.06949235617757132, 61.87390960531436690 ) ) ;
#7743=CARTESIAN_POINT ( 'NONE',  ( 5.049401038297881783, 19.05341960407617563, 62.29275706135234003 ) ) ;
#7744=CARTESIAN_POINT ( 'NONE',  ( 19.03943276465977164, -0.05219959533909143690, 98.74890960531436690 ) ) ;
#7745=CARTESIAN_POINT ( 'NONE',  ( 13.97604488694548053, -13.89961937509957401, 75.62609039468564731 ) ) ;
#7747=CARTESIAN_POINT ( 'NONE',  ( 16.55341960407618274, -4.379528057220086978, 36.04275706135234714 ) ) ;
#7748=CARTESIAN_POINT ( 'NONE',  ( -12.14591786802326823, 12.06949235617739902, 103.1260903946856757 ) ) ;
#7749=VECTOR ( 'NONE', #34804, 1000.000000000000000 ) ;
#7750=CARTESIAN_POINT ( 'NONE',  ( 9.564922557961047289, -16.46253265017146816, 70.41775706135233293 ) ) ;
#7752=CARTESIAN_POINT ( 'NONE',  ( -15.72974639402197994, 15.80617190586746368, 30.62390960531436335 ) ) ;
#7753=CARTESIAN_POINT ( 'NONE',  ( -18.67979575497193778, 10.72451020669871902, 73.33442372801901854 ) ) ;
#7755=CARTESIAN_POINT ( 'NONE',  ( 19.02544592524334988, 5.153800228976608722, 111.4594237280190043 ) ) ;
#7756=CARTESIAN_POINT ( 'NONE',  ( -9.564922557960796823, -16.46253265017161027, 27.08224293864769550 ) ) ;
#7757=CARTESIAN_POINT ( 'NONE',  ( 5.153800228976335163, 19.02544592524342804, 74.79057627198103830 ) ) ;
#7760=CARTESIAN_POINT ( 'NONE',  ( 14.34966873604960469, 8.224510206698951720, 84.16557627198103830 ) ) ;
#7761=CARTESIAN_POINT ( 'NONE',  ( 5.049401038298161559, -19.05341960407611168, 72.70724293864768129 ) ) ;
#7763=CARTESIAN_POINT ( 'NONE',  ( 16.46253265017160672, -9.564922557960803928, 93.33224293864769550 ) ) ;
#7765=CARTESIAN_POINT ( 'NONE',  ( -5.153800228976607833, 19.02544592524334988, 87.70942372801897591 ) ) ;
#7766=CARTESIAN_POINT ( 'NONE',  ( -21.55341960407610458, -5.719274019375992779, 81.45724293864769550 ) ) ;
#7767=CARTESIAN_POINT ( 'NONE',  ( -5.153800228976328057, -19.02544592524343514, 27.29057627198103120 ) ) ;
#7768=CARTESIAN_POINT ( 'NONE',  ( -19.02544592524334988, -5.153800228976617603, 68.95942372801896170 ) ) ;
#7769=CARTESIAN_POINT ( 'NONE',  ( 15.80617190586746368, 15.72974639402197994, 109.3739096053143811 ) ) ;
#7770=CARTESIAN_POINT ( 'NONE',  ( 9.564922557960805705, 16.46253265017160317, 69.58224293864770971 ) ) ;
#7771=CARTESIAN_POINT ( 'NONE',  ( 9.564922557960805705, 16.46253265017160317, 104.5822429386476955 ) ) ;
#7772=ORIENTED_EDGE ( 'NONE', *, *, #98256, .F. ) ;
#7773=CARTESIAN_POINT ( 'NONE',  ( -5.719274019375978568, 21.55341960407610458, 100.2072429386476955 ) ) ;
#7774=CARTESIAN_POINT ( 'NONE',  ( 14.29746914071049879, -8.314922557960816363, 88.33224293864769550 ) ) ;
#7775=CARTESIAN_POINT ( 'NONE',  ( -19.05341960407611168, -5.049401038298163336, 81.45724293864769550 ) ) ;
#7776=CARTESIAN_POINT ( 'NONE',  ( -19.03943276465977164, -0.05219959533935918106, 63.75109039468566863 ) ) ;
#7777=CARTESIAN_POINT ( 'NONE',  ( -15.80617190586745835, -15.72974639402198527, 91.87390960531436690 ) ) ;
#7778=CARTESIAN_POINT ( 'NONE',  ( 10.81492255796078972, 18.62759615963270932, 74.58224293864768129 ) ) ;
#7779=CARTESIAN_POINT ( 'NONE',  ( -8.224510206698948167, 14.34966873604960824, 40.41557627198103120 ) ) ;
#7780=CARTESIAN_POINT ( 'NONE',  ( 18.62759615963255655, 10.81492255796105972, 101.6677570613523613 ) ) ;
#7781=CARTESIAN_POINT ( 'NONE',  ( -14.29746914071037622, -8.314922557961029526, 69.16775706135234714 ) ) ;
#7782=CARTESIAN_POINT ( 'NONE',  ( -5.153800228976328057, -19.02544592524343514, 97.29057627198099567 ) ) ;
#7783=CARTESIAN_POINT ( 'NONE',  ( 13.97604488694527802, 13.89961937509977652, 39.37390960531435269 ) ) ;
#7785=CARTESIAN_POINT ( 'NONE',  ( -18.62759615963255300, -10.81492255796106328, 39.16775706135235424 ) ) ;
#7786=CARTESIAN_POINT ( 'NONE',  ( 0.05219959533937995610, -21.53943276465977519, 50.00109039468568994 ) ) ;
#7787=CARTESIAN_POINT ( 'NONE',  ( 0.05219959533909260263, 19.03943276465977164, 64.99890960531436690 ) ) ;
#7788=CARTESIAN_POINT ( 'NONE',  ( -0.05219959533937732626, 21.53943276465977519, 37.50109039468568284 ) ) ;
#7789=CARTESIAN_POINT ( 'NONE',  ( 13.97604488694548053, -13.89961937509957401, 80.62609039468567573 ) ) ;
#7791=CARTESIAN_POINT ( 'NONE',  ( 19.02544592524334988, 5.153800228976608722, 71.45942372801900433 ) ) ;
#7792=CARTESIAN_POINT ( 'NONE',  ( -16.51473224551069308, -9.474510206698971260, 41.66557627198103120 ) ) ;
#7793=CARTESIAN_POINT ( 'NONE',  ( -12.14591786802326823, 12.06949235617739902, 93.12609039468568994 ) ) ;
#7794=CARTESIAN_POINT ( 'NONE',  ( -19.02544592524342804, 5.153800228976336051, 51.04057627198103120 ) ) ;
#7795=CARTESIAN_POINT ( 'NONE',  ( 22.00000000000000000, -5.204748896376250896E-15, 47.50000000000000000 ) ) ;
#7796=CARTESIAN_POINT ( 'NONE',  ( 19.05341960407611168, 5.049401038298154454, 103.9572429386476671 ) ) ;
#7797=CARTESIAN_POINT ( 'NONE',  ( 9.564922557960805705, 16.46253265017160317, 39.58224293864768839 ) ) ;
#7798=CARTESIAN_POINT ( 'NONE',  ( 21.52544592524344225, -5.823673210054117533, 68.54057627198103830 ) ) ;
#7799=CARTESIAN_POINT ( 'NONE',  ( -16.53943276465976808, -0.05219959533934237506, 63.75109039468568284 ) ) ;
#7800=CARTESIAN_POINT ( 'NONE',  ( 5.153800228976615827, -19.02544592524334988, 20.20942372801899722 ) ) ;
#7801=CARTESIAN_POINT ( 'NONE',  ( 19.02544592524343514, -5.153800228976328945, 48.54057627198103120 ) ) ;
#7802=CARTESIAN_POINT ( 'NONE',  ( -4.483927247898539470, -16.52544592524342804, 47.29057627198103120 ) ) ;
#7803=CARTESIAN_POINT ( 'NONE',  ( -14.34966873604960291, -8.224510206698953496, 81.66557627198103830 ) ) ;
#7804=CARTESIAN_POINT ( 'NONE',  ( -19.05341960407611168, -5.049401038298163336, 81.45724293864769550 ) ) ;
#7805=CARTESIAN_POINT ( 'NONE',  ( -15.72974639402176322, -15.80617190586768395, 34.37609039468568284 ) ) ;
#7806=CARTESIAN_POINT ( 'NONE',  ( 16.46253265017160672, -9.564922557960803928, 98.33224293864769550 ) ) ;
#7807=CARTESIAN_POINT ( 'NONE',  ( -21.52544592524334988, -5.823673210054445271, 93.95942372801903275 ) ) ;
#7808=CARTESIAN_POINT ( 'NONE',  ( -4.379528057220086978, -16.55341960407618274, 64.79275706135234714 ) ) ;
#7809=CARTESIAN_POINT ( 'NONE',  ( -21.52544592524334988, -5.823673210054445271, 28.95942372801902209 ) ) ;
#7810=CARTESIAN_POINT ( 'NONE',  ( -0.05219959533909027116, -19.03943276465977164, 102.4989096053143669 ) ) ;
#7811=CARTESIAN_POINT ( 'NONE',  ( 0.05219959533907565091, 21.53943276465977519, 89.99890960531438111 ) ) ;
#7812=CARTESIAN_POINT ( 'NONE',  ( -12.06949235617756955, 12.14591786802309770, 40.62390960531435269 ) ) ;
#7813=CARTESIAN_POINT ( 'NONE',  ( -13.89961937509977652, 13.97604488694528158, 35.62390960531435269 ) ) ;
#7814=CARTESIAN_POINT ( 'NONE',  ( -16.52544592524342804, 4.483927247898546575, 71.04057627198103830 ) ) ;
#7815=CARTESIAN_POINT ( 'NONE',  ( 10.72451020669898902, -18.67979575497178502, 32.91557627198102409 ) ) ;
#7816=CARTESIAN_POINT ( 'NONE',  ( 19.05341960407617918, -5.049401038297876454, 31.04275706135232227 ) ) ;
#7817=CARTESIAN_POINT ( 'NONE',  ( -14.34966873604960291, -8.224510206698953496, 96.66557627198102409 ) ) ;
#7818=CARTESIAN_POINT ( 'NONE',  ( -0.05219959533909027116, -19.03943276465977164, 112.4989096053143669 ) ) ;
#7819=ORIENTED_EDGE ( 'NONE', *, *, #40745, .F. ) ;
#7820=CARTESIAN_POINT ( 'NONE',  ( -8.314922557961024197, 14.29746914071037800, 57.91775706135234714 ) ) ;
#7821=CARTESIAN_POINT ( 'NONE',  ( 19.05341960407611168, 5.049401038298154454, 48.95724293864768129 ) ) ;
#7822=DIRECTION ( 'NONE',  ( -0.000000000000000000, -0.000000000000000000, 1.000000000000000000 ) ) ;
#7823=CARTESIAN_POINT ( 'NONE',  ( -14.34966873604972548, 8.224510206698743886, 93.33442372801901854 ) ) ;
#7824=CARTESIAN_POINT ( 'NONE',  ( 13.97604488694548053, -13.89961937509957401, 95.62609039468563310 ) ) ;
#7825=CARTESIAN_POINT ( 'NONE',  ( 18.62759615963255655, 10.81492255796105972, 66.66775706135234714 ) ) ;
#7826=CARTESIAN_POINT ( 'NONE',  ( 19.02544592524343514, -5.153800228976328945, 73.54057627198103830 ) ) ;
#7827=CARTESIAN_POINT ( 'NONE',  ( -18.67979575497178146, -10.72451020669898902, 86.66557627198102409 ) ) ;
#7828=CARTESIAN_POINT ( 'NONE',  ( 4.483927247898790824, -16.52544592524335698, 45.20942372801901854 ) ) ;
#7829=CARTESIAN_POINT ( 'NONE',  ( 9.474510206698971260, -16.51473224551069308, 22.91557627198102765 ) ) ;
#7830=CARTESIAN_POINT ( 'NONE',  ( 9.474510206698729675, 16.51473224551082808, 77.08442372801900433 ) ) ;
#7831=CARTESIAN_POINT ( 'NONE',  ( 21.52544592524344225, -5.823673210054117533, 73.54057627198102409 ) ) ;
#7832=CARTESIAN_POINT ( 'NONE',  ( -16.51473224551082808, 9.474510206698731452, 43.33442372801900433 ) ) ;
#7833=CARTESIAN_POINT ( 'NONE',  ( -9.564922557960796823, -16.46253265017161027, 112.0822429386476955 ) ) ;
#7834=CARTESIAN_POINT ( 'NONE',  ( -10.72451020669898014, 18.67979575497178502, 90.41557627198103830 ) ) ;
#7835=CARTESIAN_POINT ( 'NONE',  ( 17.50000000000000000, 5.499999999999992895, 61.70309617465829177 ) ) ;
#7836=CARTESIAN_POINT ( 'NONE',  ( -9.474510206698964154, 16.51473224551069663, 60.41557627198102409 ) ) ;
#7838=CARTESIAN_POINT ( 'NONE',  ( -4.379528057220086978, -16.55341960407618274, 24.79275706135235779 ) ) ;
#7840=CARTESIAN_POINT ( 'NONE',  ( -5.049401038298153566, 19.05341960407611168, 50.20724293864770260 ) ) ;
#7841=CARTESIAN_POINT ( 'NONE',  ( -5.823673210054116645, -21.52544592524344225, 107.2905762719810525 ) ) ;
#7842=CARTESIAN_POINT ( 'NONE',  ( 8.314922557960818139, 14.29746914071049879, 49.58224293864769550 ) ) ;
#7843=CARTESIAN_POINT ( 'NONE',  ( 5.153800228976335163, 19.02544592524342804, 54.79057627198103120 ) ) ;
#7844=CARTESIAN_POINT ( 'NONE',  ( -15.72974639402176322, -15.80617190586768395, 79.37609039468567573 ) ) ;
#7845=CARTESIAN_POINT ( 'NONE',  ( -19.03943276465977164, -0.05219959533935918106, 113.7510903946856757 ) ) ;
#7846=CARTESIAN_POINT ( 'NONE',  ( -5.153800228976607833, 19.02544592524334988, 27.70942372801899722 ) ) ;
#7847=CARTESIAN_POINT ( 'NONE',  ( -12.06949235617756955, 12.14591786802309770, 25.62390960531435624 ) ) ;
#7848=CARTESIAN_POINT ( 'NONE',  ( 18.62759615963255655, 10.81492255796105972, 41.66775706135235424 ) ) ;
#7849=CARTESIAN_POINT ( 'NONE',  ( 5.823673210054444382, -21.52544592524334988, 20.20942372801900788 ) ) ;
#7850=CARTESIAN_POINT ( 'NONE',  ( 18.62759615963271287, -10.81492255796078972, 58.33224293864768839 ) ) ;
#7851=CARTESIAN_POINT ( 'NONE',  ( 19.05341960407617918, -5.049401038297876454, 96.04275706135231871 ) ) ;
#7852=CARTESIAN_POINT ( 'NONE',  ( -9.474510206698720793, -16.51473224551083518, 69.58442372801901854 ) ) ;
#7853=CARTESIAN_POINT ( 'NONE',  ( -18.67979575497193778, 10.72451020669871902, 78.33442372801901854 ) ) ;
#7854=CARTESIAN_POINT ( 'NONE',  ( -16.46253265017146816, -9.564922557961047289, 59.16775706135233293 ) ) ;
#7855=CARTESIAN_POINT ( 'NONE',  ( -16.51473224551069308, -9.474510206698971260, 21.66557627198102765 ) ) ;
#7856=CARTESIAN_POINT ( 'NONE',  ( 10.72451020669898902, -18.67979575497178502, 62.91557627198102409 ) ) ;
#7857=CARTESIAN_POINT ( 'NONE',  ( -8.224510206698948167, 14.34966873604960824, 50.41557627198103120 ) ) ;
#7858=CARTESIAN_POINT ( 'NONE',  ( -17.50000000000001421, -5.499999999999956479, 26.28230962303566542 ) ) ;
#7859=CARTESIAN_POINT ( 'NONE',  ( 16.51473224551083163, -9.474510206698727899, 20.83442372801899722 ) ) ;
#7860=CARTESIAN_POINT ( 'NONE',  ( -4.379528057220086978, -16.55341960407618274, 79.79275706135236135 ) ) ;
#7861=CARTESIAN_POINT ( 'NONE',  ( 16.55341960407611168, 4.379528057220329451, 43.95724293864769550 ) ) ;
#7862=CARTESIAN_POINT ( 'NONE',  ( -10.81492255796105439, 18.62759615963255655, 72.91775706135234714 ) ) ;
#7863=CARTESIAN_POINT ( 'NONE',  ( 15.80617190586769283, -15.72974639402175789, 75.62609039468567573 ) ) ;
#7864=CARTESIAN_POINT ( 'NONE',  ( -5.823673210054116645, -21.52544592524344225, 87.29057627198103830 ) ) ;
#7866=CARTESIAN_POINT ( 'NONE',  ( 5.153800228976335163, 19.02544592524342804, 34.79057627198102409 ) ) ;
#7867=CARTESIAN_POINT ( 'NONE',  ( 10.72451020669871369, 18.67979575497193778, 62.08442372801901143 ) ) ;
#7868=CARTESIAN_POINT ( 'NONE',  ( -16.51473224551069308, -9.474510206698971260, 31.66557627198102054 ) ) ;
#7869=CARTESIAN_POINT ( 'NONE',  ( 19.02544592524343514, -5.153800228976328945, 58.54057627198102409 ) ) ;
#7870=CARTESIAN_POINT ( 'NONE',  ( 16.53943276465976808, -0.05219959533910856209, 93.74890960531436690 ) ) ;
#7871=CARTESIAN_POINT ( 'NONE',  ( 13.97604488694527802, 13.89961937509977652, 99.37390960531436690 ) ) ;
#7872=CARTESIAN_POINT ( 'NONE',  ( 16.52544592524342804, -4.483927247898539470, 43.54057627198103830 ) ) ;
#7873=CARTESIAN_POINT ( 'NONE',  ( 16.53943276465976808, -0.05219959533910856209, 108.7489096053143669 ) ) ;
#7874=CARTESIAN_POINT ( 'NONE',  ( 15.72974639402199770, -15.80617190586745480, 83.12390960531436690 ) ) ;
#7875=CARTESIAN_POINT ( 'NONE',  ( -15.80617190586768217, 15.72974639402176855, 28.12609039468568284 ) ) ;
#7877=CARTESIAN_POINT ( 'NONE',  ( 4.379528057220092307, 16.55341960407617563, 37.29275706135235424 ) ) ;
#7878=CARTESIAN_POINT ( 'NONE',  ( -5.719274019375978568, 21.55341960407610458, 75.20724293864769550 ) ) ;
#7879=VECTOR ( 'NONE', #129440, 1000.000000000000000 ) ;
#7880=CARTESIAN_POINT ( 'NONE',  ( -21.55341960407619339, 5.719274019375674811, 98.54275706135234714 ) ) ;
#7881=CARTESIAN_POINT ( 'NONE',  ( -19.05341960407611168, -5.049401038298163336, 76.45724293864769550 ) ) ;
#7882=CARTESIAN_POINT ( 'NONE',  ( -10.72451020669870658, -18.67979575497194134, 24.58442372801901499 ) ) ;
#7883=CARTESIAN_POINT ( 'NONE',  ( -0.05219959533907301413, -21.53943276465977519, 22.49890960531436335 ) ) ;
#7884=CARTESIAN_POINT ( 'NONE',  ( -16.52544592524335698, -4.483927247898792601, 88.95942372801901854 ) ) ;
#7885=CARTESIAN_POINT ( 'NONE',  ( -21.53943276465977519, -0.05219959533937600094, 73.75109039468567573 ) ) ;
#7886=CARTESIAN_POINT ( 'NONE',  ( -19.02544592524334988, -5.153800228976617603, 23.95942372801900078 ) ) ;
#7887=CARTESIAN_POINT ( 'NONE',  ( 4.483927247898790824, -16.52544592524335698, 80.20942372801901854 ) ) ;
#7888=CARTESIAN_POINT ( 'NONE',  ( -5.823673210054431948, 21.52544592524334988, 27.70942372801901854 ) ) ;
#7890=CARTESIAN_POINT ( 'NONE',  ( -13.97604488694527625, -13.89961937509977652, 26.87390960531434558 ) ) ;
#7891=CARTESIAN_POINT ( 'NONE',  ( -10.72451020669870658, -18.67979575497194134, 89.58442372801901854 ) ) ;
#7892=CARTESIAN_POINT ( 'NONE',  ( -13.97604488694527625, -13.89961937509977652, 101.8739096053143811 ) ) ;
#7893=CARTESIAN_POINT ( 'NONE',  ( 15.80617190586746368, 15.72974639402197994, 104.3739096053143669 ) ) ;
#7894=LINE ( 'NONE', #21076, #90322 ) ;
#7895=CARTESIAN_POINT ( 'NONE',  ( -5.823673210054116645, -21.52544592524344225, 52.29057627198102409 ) ) ;
#7896=CARTESIAN_POINT ( 'NONE',  ( 19.02544592524343514, -5.153800228976328945, 93.54057627198102409 ) ) ;
#7897=CARTESIAN_POINT ( 'NONE',  ( -8.314922557960811034, -14.29746914071050412, 52.08224293864768839 ) ) ;
#7899=CARTESIAN_POINT ( 'NONE',  ( -19.02544592524334988, -5.153800228976617603, 73.95942372801900433 ) ) ;
#7901=CARTESIAN_POINT ( 'NONE',  ( -17.13100169013301155, 6.664070546373146442, 105.7678983569985007 ) ) ;
#7902=CARTESIAN_POINT ( 'NONE',  ( 16.51473224551083163, -9.474510206698727899, 110.8344237280190043 ) ) ;
#7903=CARTESIAN_POINT ( 'NONE',  ( -10.72451020669898014, 18.67979575497178502, 85.41557627198102409 ) ) ;
#7904=CARTESIAN_POINT ( 'NONE',  ( -14.34966873604960291, -8.224510206698953496, 61.66557627198103120 ) ) ;
#7905=CARTESIAN_POINT ( 'NONE',  ( -19.03943276465977164, 0.05219959533909376836, 101.2489096053143669 ) ) ;
#7906=CARTESIAN_POINT ( 'NONE',  ( 8.314922557961029526, -14.29746914071037800, 40.41775706135234714 ) ) ;
#7907=CARTESIAN_POINT ( 'NONE',  ( 5.153800228976335163, 19.02544592524342804, 59.79057627198100988 ) ) ;
#7908=CARTESIAN_POINT ( 'NONE',  ( 10.72451020669871369, 18.67979575497193778, 27.08442372801901854 ) ) ;
#7909=CARTESIAN_POINT ( 'NONE',  ( -19.02544592524334988, -5.153800228976617603, 98.95942372801900433 ) ) ;
#7910=CARTESIAN_POINT ( 'NONE',  ( -13.89961937509977652, 13.97604488694528158, 100.6239096053143669 ) ) ;
#7911=CARTESIAN_POINT ( 'NONE',  ( 9.474510206698971260, -16.51473224551069308, 82.91557627198103830 ) ) ;
#7912=CARTESIAN_POINT ( 'NONE',  ( -21.55341960407610458, -5.719274019375992779, 96.45724293864770971 ) ) ;
#7913=CARTESIAN_POINT ( 'NONE',  ( -16.46253265017160317, 9.564922557960807481, 45.83224293864769550 ) ) ;
#7914=CARTESIAN_POINT ( 'NONE',  ( -17.49999999999999645, -5.622605283950893096, 61.31207310596114723 ) ) ;
#7915=CARTESIAN_POINT ( 'NONE',  ( 16.53943276465976808, -0.05219959533910856209, 73.74890960531433848 ) ) ;
#7916=CARTESIAN_POINT ( 'NONE',  ( -13.97604488694527625, -13.89961937509977652, 101.8739096053143811 ) ) ;
#7918=CARTESIAN_POINT ( 'NONE',  ( 0.05219959533936267826, -19.03943276465977164, 60.00109039468566863 ) ) ;
#7919=CARTESIAN_POINT ( 'NONE',  ( -15.80617190586745835, -15.72974639402198527, 91.87390960531436690 ) ) ;
#7920=CARTESIAN_POINT ( 'NONE',  ( -9.474510206698720793, -16.51473224551083518, 54.58442372801899722 ) ) ;
#7921=CARTESIAN_POINT ( 'NONE',  ( 5.049401038298161559, -19.05341960407611168, 97.70724293864766707 ) ) ;
#7922=FILL_AREA_STYLE ('',( #81751 ) ) ;
#7923=CARTESIAN_POINT ( 'NONE',  ( -5.719274019375978568, 21.55341960407610458, 45.20724293864769550 ) ) ;
#7924=CARTESIAN_POINT ( 'NONE',  ( 16.51473224551069308, 9.474510206698969483, 89.16557627198103830 ) ) ;
#7925=CARTESIAN_POINT ( 'NONE',  ( 5.719274019375673035, 21.55341960407619339, 67.29275706135234714 ) ) ;
#7927=CARTESIAN_POINT ( 'NONE',  ( -0.05219959533909027116, -19.03943276465977164, 42.49890960531435269 ) ) ;
#7928=CARTESIAN_POINT ( 'NONE',  ( 8.224510206698953496, -14.34966873604960469, 77.91557627198102409 ) ) ;
#7929=CARTESIAN_POINT ( 'NONE',  ( -16.52544592524335698, -4.483927247898792601, 23.95942372801901143 ) ) ;
#7930=CARTESIAN_POINT ( 'NONE',  ( -18.62759615963255300, -10.81492255796106328, 59.16775706135234714 ) ) ;
#7931=EDGE_LOOP ( 'NONE', ( #62477, #72857 ) ) ;
#7932=CARTESIAN_POINT ( 'NONE',  ( -13.89961937509977652, 13.97604488694528158, 115.6239096053143669 ) ) ;
#7933=CARTESIAN_POINT ( 'NONE',  ( 13.89961937509957401, 13.97604488694547697, 66.87609039468567573 ) ) ;
#7936=CARTESIAN_POINT ( 'NONE',  ( -15.80617190586768217, 15.72974639402176855, 28.12609039468568284 ) ) ;
#7937=CARTESIAN_POINT ( 'NONE',  ( 19.02544592524343514, -5.153800228976328945, 58.54057627198102409 ) ) ;
#7939=CARTESIAN_POINT ( 'NONE',  ( 21.53943276465977519, 0.05219959533937863772, 111.2510903946856899 ) ) ;
#7940=CARTESIAN_POINT ( 'NONE',  ( 0.05219959533909260263, 19.03943276465977164, 49.99890960531435979 ) ) ;
#7941=CARTESIAN_POINT ( 'NONE',  ( 9.474510206698729675, 16.51473224551082808, 22.08442372801899722 ) ) ;
#7942=CARTESIAN_POINT ( 'NONE',  ( -16.53943276465976808, -0.05219959533934237506, 108.7510903946857042 ) ) ;
#7943=CARTESIAN_POINT ( 'NONE',  ( -16.46253265017160317, 9.564922557960807481, 100.8322429386477097 ) ) ;
#7944=CARTESIAN_POINT ( 'NONE',  ( -18.67979575497193778, 10.72451020669871902, 73.33442372801901854 ) ) ;
#7946=CARTESIAN_POINT ( 'NONE',  ( 9.564922557960805705, 16.46253265017160317, 114.5822429386476955 ) ) ;
#7947=CARTESIAN_POINT ( 'NONE',  ( 18.09867054820431420, 5.499999999999960032, 96.48393025253585620 ) ) ;
#7948=CARTESIAN_POINT ( 'NONE',  ( 8.314922557961029526, -14.29746914071037800, 65.41775706135234714 ) ) ;
#7949=CARTESIAN_POINT ( 'NONE',  ( 10.81492255796106328, -18.62759615963255655, 65.41775706135234714 ) ) ;
#7950=CARTESIAN_POINT ( 'NONE',  ( 18.62759615963255655, 10.81492255796105972, 101.6677570613523613 ) ) ;
#7952=CARTESIAN_POINT ( 'NONE',  ( 19.02544592524343514, -5.153800228976328945, 83.54057627198100988 ) ) ;
#7953=CARTESIAN_POINT ( 'NONE',  ( -9.564922557960796823, -16.46253265017161027, 112.0822429386476955 ) ) ;
#7954=EDGE_LOOP ( 'NONE', ( #143380, #17846, #35752, #95480 ) ) ;
#7956=CARTESIAN_POINT ( 'NONE',  ( 9.564922557960805705, 16.46253265017160317, 34.58224293864770260 ) ) ;
#7957=CARTESIAN_POINT ( 'NONE',  ( 5.719274019375991003, -21.55341960407610458, 42.70724293864770260 ) ) ;
#7958=CARTESIAN_POINT ( 'NONE',  ( 16.53943276465976808, 0.05219959533934440121, 106.2510903946856757 ) ) ;
#7959=CARTESIAN_POINT ( 'NONE',  ( -14.29746914071049879, 8.314922557960819915, 95.83224293864770971 ) ) ;
#7960=CARTESIAN_POINT ( 'NONE',  ( -5.153800228976328057, -19.02544592524343514, 77.29057627198099567 ) ) ;
#7961=CARTESIAN_POINT ( 'NONE',  ( -5.719274019375665041, -21.55341960407619695, 104.7927570613523898 ) ) ;
#7962=CARTESIAN_POINT ( 'NONE',  ( 0.05219959533909260263, 19.03943276465977164, 34.99890960531435979 ) ) ;
#7963=CARTESIAN_POINT ( 'NONE',  ( -16.55341960407611168, -4.379528057220339221, 86.45724293864770971 ) ) ;
#7964=CARTESIAN_POINT ( 'NONE',  ( 15.80617190586769283, -15.72974639402175789, 45.62609039468567573 ) ) ;
#7965=CARTESIAN_POINT ( 'NONE',  ( 10.72451020669898902, -18.67979575497178502, 82.91557627198103830 ) ) ;
#7966=CARTESIAN_POINT ( 'NONE',  ( 5.153800228976615827, -19.02544592524334988, 45.20942372801901143 ) ) ;
#7967=CARTESIAN_POINT ( 'NONE',  ( 9.564922557960805705, 16.46253265017160317, 44.58224293864769550 ) ) ;
#7968=CARTESIAN_POINT ( 'NONE',  ( 0.05219959533909260263, 19.03943276465977164, 89.99890960531436690 ) ) ;
#7969=CARTESIAN_POINT ( 'NONE',  ( 12.14591786802309770, 12.06949235617756955, 59.37390960531436690 ) ) ;
#7970=CARTESIAN_POINT ( 'NONE',  ( -4.483927247898539470, -16.52544592524342804, 52.29057627198102409 ) ) ;
#7971=CARTESIAN_POINT ( 'NONE',  ( -5.153800228976607833, 19.02544592524334988, 77.70942372801900433 ) ) ;
#7972=CARTESIAN_POINT ( 'NONE',  ( -19.36337904590693526, 5.499999999999953815, 85.41494137495625694 ) ) ;
#7973=CARTESIAN_POINT ( 'NONE',  ( -15.80617190586745835, -15.72974639402198527, 41.87390960531435979 ) ) ;
#7974=CARTESIAN_POINT ( 'NONE',  ( 12.14591786802309770, 12.06949235617756955, 94.37390960531436690 ) ) ;
#7976=CARTESIAN_POINT ( 'NONE',  ( -13.97604488694527625, -13.89961937509977652, 46.87390960531435979 ) ) ;
#7977=CARTESIAN_POINT ( 'NONE',  ( 5.823673210054125526, 21.52544592524343514, 49.79057627198102409 ) ) ;
#7978=CARTESIAN_POINT ( 'NONE',  ( -16.51473224551069308, -9.474510206698971260, 31.66557627198102054 ) ) ;
#7979=CARTESIAN_POINT ( 'NONE',  ( 12.14591786802327356, -12.06949235617739191, 75.62609039468567573 ) ) ;
#7980=CARTESIAN_POINT ( 'NONE',  ( -16.46253265017160317, 9.564922557960807481, 65.83224293864769550 ) ) ;
#7981=CARTESIAN_POINT ( 'NONE',  ( -16.46253265017146816, -9.564922557961047289, 39.16775706135234003 ) ) ;
#7983=CARTESIAN_POINT ( 'NONE',  ( -15.72974639402176322, -15.80617190586768395, 74.37609039468568994 ) ) ;
#7984=CARTESIAN_POINT ( 'NONE',  ( 15.80617190586746368, 15.72974639402197994, 49.37390960531436690 ) ) ;
#7985=CARTESIAN_POINT ( 'NONE',  ( 8.224510206698953496, -14.34966873604960469, 112.9155762719810383 ) ) ;
#7986=CARTESIAN_POINT ( 'NONE',  ( -9.474510206698720793, -16.51473224551083518, 89.58442372801900433 ) ) ;
#7989=CARTESIAN_POINT ( 'NONE',  ( 18.67979575497178502, 10.72451020669898547, 44.16557627198103120 ) ) ;
#7990=CARTESIAN_POINT ( 'NONE',  ( 16.31925111598459210, -7.325300261831447557, 67.66424538967254421 ) ) ;
#7991=CARTESIAN_POINT ( 'NONE',  ( 5.719274019375673035, 21.55341960407619339, 77.29275706135234714 ) ) ;
#7992=CARTESIAN_POINT ( 'NONE',  ( -0.05219959533910754901, -16.53943276465976808, 52.49890960531435979 ) ) ;
#7993=CARTESIAN_POINT ( 'NONE',  ( -16.52544592524342804, 4.483927247898546575, 56.04057627198102409 ) ) ;
#7994=CARTESIAN_POINT ( 'NONE',  ( -21.52544592524343514, 5.823673210054127303, 86.04057627198102409 ) ) ;
#7995=CARTESIAN_POINT ( 'NONE',  ( -10.72451020669898014, 18.67979575497178502, 75.41557627198102409 ) ) ;
#7997=CARTESIAN_POINT ( 'NONE',  ( 5.823673210054125526, 21.52544592524343514, 34.79057627198103120 ) ) ;
#7998=CARTESIAN_POINT ( 'NONE',  ( -8.224510206698735004, -14.34966873604973081, 59.58442372801901854 ) ) ;
#7999=CARTESIAN_POINT ( 'NONE',  ( -14.34966873604960291, -8.224510206698953496, 76.66557627198103830 ) ) ;
#8000=CARTESIAN_POINT ( 'NONE',  ( -13.97604488694527625, -13.89961937509977652, 61.87390960531435979 ) ) ;
#8001=CARTESIAN_POINT ( 'NONE',  ( -13.97604488694527625, -13.89961937509977652, 36.87390960531436690 ) ) ;
#8003=AXIS2_PLACEMENT_3D ( 'NONE', #45886, #186406, #129656 ) ;
#8004=CARTESIAN_POINT ( 'NONE',  ( 0.05219959533934541429, -16.53943276465976808, 85.00109039468568994 ) ) ;
#8005=CARTESIAN_POINT ( 'NONE',  ( -10.81492255796105439, 18.62759615963255655, 22.91775706135235069 ) ) ;
#8006=CARTESIAN_POINT ( 'NONE',  ( 19.02544592524343514, -5.153800228976328945, 63.54057627198103830 ) ) ;
#8007=CARTESIAN_POINT ( 'NONE',  ( -5.719274019375665041, -21.55341960407619695, 54.79275706135235424 ) ) ;
#8008=CARTESIAN_POINT ( 'NONE',  ( -13.97604488694527625, -13.89961937509977652, 111.8739096053143243 ) ) ;
#8011=CARTESIAN_POINT ( 'NONE',  ( 21.55341960407619695, -5.719274019375665929, 46.04275706135234714 ) ) ;
#8012=CARTESIAN_POINT ( 'NONE',  ( -19.03943276465977164, 0.05219959533909376836, 116.2489096053143669 ) ) ;
#8013=CARTESIAN_POINT ( 'NONE',  ( -13.97604488694527625, -13.89961937509977652, 106.8739096053143669 ) ) ;
#8014=CARTESIAN_POINT ( 'NONE',  ( 0.05219959533936267826, -19.03943276465977164, 60.00109039468566863 ) ) ;
#8015=CARTESIAN_POINT ( 'NONE',  ( 18.62759615963271287, -10.81492255796078972, 108.3322429386477097 ) ) ;
#8016=CARTESIAN_POINT ( 'NONE',  ( 9.564922557961047289, -16.46253265017146816, 40.41775706135234003 ) ) ;
#8017=CARTESIAN_POINT ( 'NONE',  ( -4.379528057220086978, -16.55341960407618274, 94.79275706135234714 ) ) ;
#8018=CARTESIAN_POINT ( 'NONE',  ( -9.564922557961040184, 16.46253265017147172, 67.91775706135233293 ) ) ;
#8019=CARTESIAN_POINT ( 'NONE',  ( -4.483927247898782831, 16.52544592524335698, 102.7094237280190185 ) ) ;
#8021=ORIENTED_EDGE ( 'NONE', *, *, #60920, .F. ) ;
#8022=CARTESIAN_POINT ( 'NONE',  ( -19.05341960407611168, -5.049401038298163336, 86.45724293864769550 ) ) ;
#8024=CARTESIAN_POINT ( 'NONE',  ( -5.823673210054431948, 21.52544592524334988, 87.70942372801901854 ) ) ;
#8025=CARTESIAN_POINT ( 'NONE',  ( -0.05219959533937732626, 21.53943276465977519, 97.50109039468567573 ) ) ;
#8027=CARTESIAN_POINT ( 'NONE',  ( 19.02544592524343514, -5.153800228976328945, 98.54057627198100988 ) ) ;
#8028=CARTESIAN_POINT ( 'NONE',  ( 10.81492255796106328, -18.62759615963255655, 80.41775706135234714 ) ) ;
#8029=CARTESIAN_POINT ( 'NONE',  ( -16.53943276465976808, -0.05219959533934237506, 23.75109039468567929 ) ) ;
#8031=CARTESIAN_POINT ( 'NONE',  ( -16.46253265017160317, 9.564922557960807481, 75.83224293864769550 ) ) ;
#8032=CARTESIAN_POINT ( 'NONE',  ( -18.62759615963270932, 10.81492255796079327, 30.83224293864770260 ) ) ;
#8033=CARTESIAN_POINT ( 'NONE',  ( -19.05341960407611168, -5.049401038298163336, 91.45724293864766707 ) ) ;
#8034=CARTESIAN_POINT ( 'NONE',  ( -17.48847506799968698, -5.747544572773761296, 89.17302562156721990 ) ) ;
#8035=CARTESIAN_POINT ( 'NONE',  ( 13.89961937509977652, -13.97604488694527269, 83.12390960531436690 ) ) ;
#8036=CARTESIAN_POINT ( 'NONE',  ( 5.153800228976335163, 19.02544592524342804, 64.79057627198100988 ) ) ;
#8037=CARTESIAN_POINT ( 'NONE',  ( -12.06949235617739369, -12.14591786802326823, 99.37609039468568994 ) ) ;
#8038=CARTESIAN_POINT ( 'NONE',  ( -19.19724070472090816, -5.500000000000166978, 41.06193348274383226 ) ) ;
#8040=CARTESIAN_POINT ( 'NONE',  ( 13.97604488694548053, -13.89961937509957401, 60.62609039468564731 ) ) ;
#8041=CARTESIAN_POINT ( 'NONE',  ( 19.05341960407611168, 5.049401038298154454, 88.95724293864769550 ) ) ;
#8042=CARTESIAN_POINT ( 'NONE',  ( 16.52544592524342804, -4.483927247898539470, 88.54057627198103830 ) ) ;
#8044=CARTESIAN_POINT ( 'NONE',  ( -21.55341960407610458, -5.719274019375992779, 26.45724293864768839 ) ) ;
#8046=CARTESIAN_POINT ( 'NONE',  ( -0.05219959533909027116, -19.03943276465977164, 112.4989096053143669 ) ) ;
#8047=CARTESIAN_POINT ( 'NONE',  ( 12.14591786802309770, 12.06949235617756955, 89.37390960531435269 ) ) ;
#8049=CARTESIAN_POINT ( 'NONE',  ( -19.05341960407617563, 5.049401038297882671, 48.54275706135233293 ) ) ;
#8050=CARTESIAN_POINT ( 'NONE',  ( 12.14591786802327356, -12.06949235617739191, 105.6260903946856899 ) ) ;
#8051=CARTESIAN_POINT ( 'NONE',  ( 16.46253265017160672, -9.564922557960803928, 88.33224293864769550 ) ) ;
#8052=CARTESIAN_POINT ( 'NONE',  ( 18.62759615963255655, 10.81492255796105972, 71.66775706135234714 ) ) ;
#8053=CARTESIAN_POINT ( 'NONE',  ( -18.67979575497178146, -10.72451020669898902, 51.66557627198102409 ) ) ;
#8054=CARTESIAN_POINT ( 'NONE',  ( -5.719274019375665041, -21.55341960407619695, 29.79275706135234358 ) ) ;
#8056=CARTESIAN_POINT ( 'NONE',  ( -15.80617190586745835, -15.72974639402198527, 86.87390960531438111 ) ) ;
#8057=CARTESIAN_POINT ( 'NONE',  ( -21.55341960407619339, 5.719274019375674811, 38.54275706135234714 ) ) ;
#8058=CARTESIAN_POINT ( 'NONE',  ( 16.53943276465976808, -0.05219959533910856209, 103.7489096053143669 ) ) ;
#8059=CARTESIAN_POINT ( 'NONE',  ( -16.51473224551082808, 9.474510206698731452, 68.33442372801900433 ) ) ;
#8060=CARTESIAN_POINT ( 'NONE',  ( -5.153800228976328057, -19.02544592524343514, 47.29057627198102409 ) ) ;
#8061=CARTESIAN_POINT ( 'NONE',  ( -9.564922557960796823, -16.46253265017161027, 102.0822429386477097 ) ) ;
#8062=CARTESIAN_POINT ( 'NONE',  ( 16.51473224551069308, 9.474510206698969483, 94.16557627198103830 ) ) ;
#8063=CARTESIAN_POINT ( 'NONE',  ( 19.05341960407611168, 5.049401038298154454, 23.95724293864769194 ) ) ;
#8064=CARTESIAN_POINT ( 'NONE',  ( -4.379528057220328563, 16.55341960407611168, 35.20724293864768839 ) ) ;
#8065=CARTESIAN_POINT ( 'NONE',  ( -8.314922557961024197, 14.29746914071037800, 42.91775706135235424 ) ) ;
#8066=CARTESIAN_POINT ( 'NONE',  ( -14.29746914071049879, 8.314922557960819915, 115.8322429386477097 ) ) ;
#8067=CARTESIAN_POINT ( 'NONE',  ( -5.153800228976607833, 19.02544592524334988, 27.70942372801899722 ) ) ;
#8070=CARTESIAN_POINT ( 'NONE',  ( 4.483927247898545687, 16.52544592524342804, 24.79057627198103120 ) ) ;
#8071=CARTESIAN_POINT ( 'NONE',  ( 0.05219959533937995610, -21.53943276465977519, 30.00109039468568284 ) ) ;
#8072=CARTESIAN_POINT ( 'NONE',  ( -5.049401038298153566, 19.05341960407611168, 105.2072429386476671 ) ) ;
#8073=CARTESIAN_POINT ( 'NONE',  ( -16.52544592524335698, -4.483927247898792601, 43.95942372801902565 ) ) ;
#8074=CARTESIAN_POINT ( 'NONE',  ( -12.06949235617739369, -12.14591786802326823, 109.3760903946857042 ) ) ;
#8075=CARTESIAN_POINT ( 'NONE',  ( 4.379528057220092307, 16.55341960407617563, 87.29275706135236135 ) ) ;
#8076=CARTESIAN_POINT ( 'NONE',  ( 12.06949235617739724, 12.14591786802326823, 31.87609039468567929 ) ) ;
#8077=CARTESIAN_POINT ( 'NONE',  ( -5.049401038298153566, 19.05341960407611168, 45.20724293864769550 ) ) ;
#8078=CARTESIAN_POINT ( 'NONE',  ( 14.34966873604960469, 8.224510206698951720, 104.1655762719810241 ) ) ;
#8079=CARTESIAN_POINT ( 'NONE',  ( 5.719274019375673035, 21.55341960407619339, 22.29275706135235069 ) ) ;
#8080=CARTESIAN_POINT ( 'NONE',  ( 13.89961937509977652, -13.97604488694527269, 33.12390960531434558 ) ) ;
#8081=CARTESIAN_POINT ( 'NONE',  ( 9.564922557960805705, 16.46253265017160317, 99.58224293864770971 ) ) ;
#8082=CARTESIAN_POINT ( 'NONE',  ( -5.153800228976328057, -19.02544592524343514, 37.29057627198102409 ) ) ;
#8083=CARTESIAN_POINT ( 'NONE',  ( 19.02544592524343514, -5.153800228976328945, 98.54057627198100988 ) ) ;
#8085=CARTESIAN_POINT ( 'NONE',  ( 5.049401038298161559, -19.05341960407611168, 97.70724293864766707 ) ) ;
#8086=CARTESIAN_POINT ( 'NONE',  ( 18.67979575497194134, -10.72451020669871369, 50.83442372801901143 ) ) ;
#8087=CARTESIAN_POINT ( 'NONE',  ( -8.224510206698948167, 14.34966873604960824, 85.41557627198102409 ) ) ;
#8088=CARTESIAN_POINT ( 'NONE',  ( -13.97604488694527625, -13.89961937509977652, 111.8739096053143243 ) ) ;
#8090=CARTESIAN_POINT ( 'NONE',  ( 4.379528057220092307, 16.55341960407617563, 67.29275706135234714 ) ) ;
#8091=CARTESIAN_POINT ( 'NONE',  ( 5.719274019375673035, 21.55341960407619339, 77.29275706135234714 ) ) ;
#8092=CARTESIAN_POINT ( 'NONE',  ( -12.06949235617739369, -12.14591786802326823, 34.37609039468568284 ) ) ;
#8093=CARTESIAN_POINT ( 'NONE',  ( -13.89961937509977652, 13.97604488694528158, 80.62390960531436690 ) ) ;
#8094=CARTESIAN_POINT ( 'NONE',  ( 19.03943276465977164, 0.05219959533936151252, 106.2510903946856615 ) ) ;
#8095=CARTESIAN_POINT ( 'NONE',  ( 16.53943276465976808, 0.05219959533934440121, 76.25109039468568994 ) ) ;
#8096=CARTESIAN_POINT ( 'NONE',  ( 0.05219959533936267826, -19.03943276465977164, 90.00109039468567573 ) ) ;
#8097=CARTESIAN_POINT ( 'NONE',  ( 0.05219959533909260263, 19.03943276465977164, 64.99890960531436690 ) ) ;
#8098=CARTESIAN_POINT ( 'NONE',  ( 10.72451020669898902, -18.67979575497178502, 92.91557627198103830 ) ) ;
#8099=CARTESIAN_POINT ( 'NONE',  ( -0.05219959533910754901, -16.53943276465976808, 92.49890960531436690 ) ) ;
#8100=CARTESIAN_POINT ( 'NONE',  ( -19.03943276465977164, -0.05219959533935918106, 93.75109039468566152 ) ) ;
#8101=CARTESIAN_POINT ( 'NONE',  ( 16.53943276465976808, 0.05219959533934440121, 61.25109039468567573 ) ) ;
#8102=CARTESIAN_POINT ( 'NONE',  ( -18.39635199886971151, 5.499999999999982236, 81.01967076360003261 ) ) ;
#8103=CARTESIAN_POINT ( 'NONE',  ( -16.51473224551082808, 9.474510206698731452, 68.33442372801900433 ) ) ;
#8104=CARTESIAN_POINT ( 'NONE',  ( -16.55341960407611168, -4.379528057220339221, 26.45724293864768839 ) ) ;
#8105=CARTESIAN_POINT ( 'NONE',  ( 16.52544592524342804, -4.483927247898539470, 83.54057627198102409 ) ) ;
#8106=CARTESIAN_POINT ( 'NONE',  ( 19.05341960407617918, -5.049401038297876454, 26.04275706135233293 ) ) ;
#8107=CARTESIAN_POINT ( 'NONE',  ( -17.12812012977050458, 6.668231424565584042, 38.64051240676854349 ) ) ;
#8108=CARTESIAN_POINT ( 'NONE',  ( 21.53943276465977519, 0.05219959533937863772, 21.25109039468567218 ) ) ;
#8110=CARTESIAN_POINT ( 'NONE',  ( 9.564922557960805705, 16.46253265017160317, 79.58224293864769550 ) ) ;
#8111=CARTESIAN_POINT ( 'NONE',  ( -21.53943276465977519, -0.05219959533937600094, 93.75109039468567573 ) ) ;
#8112=CARTESIAN_POINT ( 'NONE',  ( -13.89961937509977652, 13.97604488694528158, 80.62390960531436690 ) ) ;
#8113=CARTESIAN_POINT ( 'NONE',  ( -18.67979575497178146, -10.72451020669898902, 41.66557627198103120 ) ) ;
#8115=CARTESIAN_POINT ( 'NONE',  ( 16.53943276465976808, -0.05219959533910856209, 83.74890960531435269 ) ) ;
#8116=CARTESIAN_POINT ( 'NONE',  ( -16.51473224551069308, -9.474510206698971260, 56.66557627198103120 ) ) ;
#8117=CARTESIAN_POINT ( 'NONE',  ( -14.29746914071049879, 8.314922557960819915, 105.8322429386476955 ) ) ;
#8118=CARTESIAN_POINT ( 'NONE',  ( 0.05219959533937995610, -21.53943276465977519, 30.00109039468568284 ) ) ;
#8119=CARTESIAN_POINT ( 'NONE',  ( 21.53943276465977519, 0.05219959533937863772, 56.25109039468568284 ) ) ;
#8120=CARTESIAN_POINT ( 'NONE',  ( 13.97604488694527802, 13.89961937509977652, 49.37390960531434558 ) ) ;
#8121=CARTESIAN_POINT ( 'NONE',  ( 4.379528057220092307, 16.55341960407617563, 72.29275706135236135 ) ) ;
#8122=CARTESIAN_POINT ( 'NONE',  ( 0.05219959533907565091, 21.53943276465977519, 114.9989096053143669 ) ) ;
#8123=CARTESIAN_POINT ( 'NONE',  ( -5.719274019375665041, -21.55341960407619695, 19.79275706135235069 ) ) ;
#8124=CARTESIAN_POINT ( 'NONE',  ( 0.05219959533936267826, -19.03943276465977164, 35.00109039468566863 ) ) ;
#8125=CARTESIAN_POINT ( 'NONE',  ( 19.02544592524343514, -5.153800228976328945, 63.54057627198103830 ) ) ;
#8126=CARTESIAN_POINT ( 'NONE',  ( 9.474510206698729675, 16.51473224551082808, 32.08442372801900433 ) ) ;
#8127=CARTESIAN_POINT ( 'NONE',  ( -0.05219959533937732626, 21.53943276465977519, 72.50109039468568994 ) ) ;
#8129=CARTESIAN_POINT ( 'NONE',  ( 10.72451020669898902, -18.67979575497178502, 72.91557627198103830 ) ) ;
#8130=CARTESIAN_POINT ( 'NONE',  ( -12.06949235617756955, 12.14591786802309770, 35.62390960531437401 ) ) ;
#8131=CARTESIAN_POINT ( 'NONE',  ( -5.823673210054431948, 21.52544592524334988, 87.70942372801901854 ) ) ;
#8132=CARTESIAN_POINT ( 'NONE',  ( -18.67979575497193778, 10.72451020669871902, 108.3344237280190185 ) ) ;
#8133=CARTESIAN_POINT ( 'NONE',  ( 8.314922557960818139, 14.29746914071049879, 59.58224293864770260 ) ) ;
#8134=CARTESIAN_POINT ( 'NONE',  ( 4.379528057220339221, -16.55341960407611168, 102.7072429386476955 ) ) ;
#8135=CARTESIAN_POINT ( 'NONE',  ( 9.474510206698729675, 16.51473224551082808, 57.08442372801900433 ) ) ;
#8136=CARTESIAN_POINT ( 'NONE',  ( -14.29746914071049879, 8.314922557960819915, 25.83224293864769194 ) ) ;
#8137=CARTESIAN_POINT ( 'NONE',  ( 5.719274019375673035, 21.55341960407619339, 67.29275706135234714 ) ) ;
#8139=CARTESIAN_POINT ( 'NONE',  ( -16.46253265017160317, 9.564922557960807481, 75.83224293864769550 ) ) ;
#8140=CARTESIAN_POINT ( 'NONE',  ( -19.03943276465977164, -0.05219959533935918106, 48.75109039468566863 ) ) ;
#8141=CARTESIAN_POINT ( 'NONE',  ( 5.823673210054125526, 21.52544592524343514, 49.79057627198102409 ) ) ;
#8142=CARTESIAN_POINT ( 'NONE',  ( -5.823673210054431948, 21.52544592524334988, 42.70942372801901854 ) ) ;
#8143=CARTESIAN_POINT ( 'NONE',  ( 21.55341960407610458, 5.719274019375980345, 103.9572429386476813 ) ) ;
#8144=CARTESIAN_POINT ( 'NONE',  ( 9.564922557961047289, -16.46253265017146816, 100.4177570613523329 ) ) ;
#8145=CARTESIAN_POINT ( 'NONE',  ( -12.14591786802326823, 12.06949235617739902, 63.12609039468568994 ) ) ;
#8147=CARTESIAN_POINT ( 'NONE',  ( -21.55341960407610458, -5.719274019375992779, 96.45724293864770971 ) ) ;
#8148=CARTESIAN_POINT ( 'NONE',  ( -16.53943276465976808, 0.05219959533911058130, 91.24890960531436690 ) ) ;
#8150=CARTESIAN_POINT ( 'NONE',  ( 14.34966873604972726, -8.224510206698740333, 20.83442372801901143 ) ) ;
#8151=CARTESIAN_POINT ( 'NONE',  ( -0.05219959533907301413, -21.53943276465977519, 52.49890960531435979 ) ) ;
#8152=CARTESIAN_POINT ( 'NONE',  ( 16.55341960407618274, -4.379528057220086978, 96.04275706135236135 ) ) ;
#8155=CARTESIAN_POINT ( 'NONE',  ( -8.314922557961024197, 14.29746914071037800, 47.91775706135234714 ) ) ;
#8156=CARTESIAN_POINT ( 'NONE',  ( 18.67979575497194134, -10.72451020669871369, 30.83442372801902209 ) ) ;
#8157=CARTESIAN_POINT ( 'NONE',  ( 10.81492255796078972, 18.62759615963270932, 39.58224293864769550 ) ) ;
#8158=CARTESIAN_POINT ( 'NONE',  ( 4.379528057220092307, 16.55341960407617563, 87.29275706135236135 ) ) ;
#8159=CARTESIAN_POINT ( 'NONE',  ( 0.05219959533909260263, 19.03943276465977164, 94.99890960531436690 ) ) ;
#8160=CARTESIAN_POINT ( 'NONE',  ( -21.52544592524334988, -5.823673210054445271, 68.95942372801901854 ) ) ;
#8161=CARTESIAN_POINT ( 'NONE',  ( -21.53943276465977519, 0.05219959533907696930, 41.24890960531435269 ) ) ;
#8162=CARTESIAN_POINT ( 'NONE',  ( 18.67979575497178502, 10.72451020669898547, 34.16557627198102409 ) ) ;
#8164=CARTESIAN_POINT ( 'NONE',  ( -5.049401038297874678, -19.05341960407617918, 54.79275706135234003 ) ) ;
#8165=CARTESIAN_POINT ( 'NONE',  ( -14.34966873604972548, 8.224510206698743886, 63.33442372801900433 ) ) ;
#8166=CARTESIAN_POINT ( 'NONE',  ( 18.62759615963271287, -10.81492255796078972, 28.33224293864769550 ) ) ;
#8168=CARTESIAN_POINT ( 'NONE',  ( -16.51473224551069308, -9.474510206698971260, 81.66557627198103830 ) ) ;
#8169=CARTESIAN_POINT ( 'NONE',  ( 12.14591786802327356, -12.06949235617739191, 110.6260903946857042 ) ) ;
#8171=CARTESIAN_POINT ( 'NONE',  ( -8.224510206698948167, 14.34966873604960824, 105.4155762719810383 ) ) ;
#8172=CARTESIAN_POINT ( 'NONE',  ( 18.62759615963271287, -10.81492255796078972, 43.33224293864769550 ) ) ;
#8173=CARTESIAN_POINT ( 'NONE',  ( -13.97604488694527625, -13.89961937509977652, 51.87390960531436690 ) ) ;
#8174=CARTESIAN_POINT ( 'NONE',  ( -16.55341960407617563, 4.379528057220093196, 73.54275706135234714 ) ) ;
#8175=CARTESIAN_POINT ( 'NONE',  ( -0.05219959533937732626, 21.53943276465977519, 37.50109039468568284 ) ) ;
#8176=CARTESIAN_POINT ( 'NONE',  ( -16.51473224551082808, 9.474510206698731452, 93.33442372801900433 ) ) ;
#8177=CARTESIAN_POINT ( 'NONE',  ( -16.55341960407611168, -4.379528057220339221, 91.45724293864769550 ) ) ;
#8178=CARTESIAN_POINT ( 'NONE',  ( 19.05341960407611168, 5.049401038298154454, 48.95724293864768129 ) ) ;
#8180=CARTESIAN_POINT ( 'NONE',  ( 19.05341960407611168, 5.049401038298154454, 23.95724293864769194 ) ) ;
#8181=CARTESIAN_POINT ( 'NONE',  ( 5.719274019375673035, 21.55341960407619339, 107.2927570613523471 ) ) ;
#8182=CARTESIAN_POINT ( 'NONE',  ( -19.03943276465977164, 0.05219959533909376836, 81.24890960531436690 ) ) ;
#8183=CARTESIAN_POINT ( 'NONE',  ( -4.379528057220086978, -16.55341960407618274, 59.79275706135234714 ) ) ;
#8184=CARTESIAN_POINT ( 'NONE',  ( 5.823673210054444382, -21.52544592524334988, 95.20942372801903275 ) ) ;
#8185=CARTESIAN_POINT ( 'NONE',  ( 5.719274019375991003, -21.55341960407610458, 47.70724293864770260 ) ) ;
#8186=CARTESIAN_POINT ( 'NONE',  ( 4.379528057220092307, 16.55341960407617563, 77.29275706135234714 ) ) ;
#8187=CARTESIAN_POINT ( 'NONE',  ( 19.05341960407617918, -5.049401038297876454, 46.04275706135233293 ) ) ;
#8189=CARTESIAN_POINT ( 'NONE',  ( 5.049401038297881783, 19.05341960407617563, 72.29275706135234714 ) ) ;
#8190=ORIENTED_EDGE ( 'NONE', *, *, #124207, .T. ) ;
#8191=CARTESIAN_POINT ( 'NONE',  ( -21.52544592524334988, -5.823673210054445271, 68.95942372801901854 ) ) ;
#8192=CARTESIAN_POINT ( 'NONE',  ( 5.049401038298161559, -19.05341960407611168, 67.70724293864769550 ) ) ;
#8193=CARTESIAN_POINT ( 'NONE',  ( -16.46253265017160317, 9.564922557960807481, 25.83224293864769194 ) ) ;
#8194=CARTESIAN_POINT ( 'NONE',  ( -9.564922557961040184, 16.46253265017147172, 52.91775706135233293 ) ) ;
#8195=CARTESIAN_POINT ( 'NONE',  ( -13.97604488694527625, -13.89961937509977652, 106.8739096053143669 ) ) ;
#8196=CARTESIAN_POINT ( 'NONE',  ( 19.03943276465977164, -0.05219959533909143690, 93.74890960531435269 ) ) ;
#8197=CARTESIAN_POINT ( 'NONE',  ( -16.52544592524342804, 4.483927247898546575, 51.04057627198103120 ) ) ;
#8198=CARTESIAN_POINT ( 'NONE',  ( 10.72451020669898902, -18.67979575497178502, 47.91557627198102409 ) ) ;
#8199=DIRECTION ( 'NONE',  ( 1.000000000000000000, -0.000000000000000000, -0.000000000000000000 ) ) ;
#8200=CARTESIAN_POINT ( 'NONE',  ( 19.03943276465977164, 0.05219959533936151252, 21.25109039468565797 ) ) ;
#8201=CARTESIAN_POINT ( 'NONE',  ( 18.22780087662126647, 5.499999999999818812, 46.48236817873107185 ) ) ;
#8202=CARTESIAN_POINT ( 'NONE',  ( 19.05341960407611168, 5.049401038298154454, 48.95724293864768129 ) ) ;
#8203=CARTESIAN_POINT ( 'NONE',  ( 13.97604488694527802, 13.89961937509977830, 84.37390960531435269 ) ) ;
#8206=CARTESIAN_POINT ( 'NONE',  ( 14.29746914071037800, 8.314922557961029526, 66.66775706135234714 ) ) ;
#8207=CARTESIAN_POINT ( 'NONE',  ( 5.719274019375991003, -21.55341960407610458, 82.70724293864770971 ) ) ;
#8208=CARTESIAN_POINT ( 'NONE',  ( 14.29746914071049879, -8.314922557960816363, 58.33224293864768839 ) ) ;
#8209=CARTESIAN_POINT ( 'NONE',  ( 0.05219959533909260263, 19.03943276465977164, 39.99890960531436690 ) ) ;
#8211=CARTESIAN_POINT ( 'NONE',  ( -18.62759615963255300, -10.81492255796106328, 34.16775706135234714 ) ) ;
#8212=CARTESIAN_POINT ( 'NONE',  ( -16.46253265017146816, -9.564922557961047289, 54.16775706135234003 ) ) ;
#8213=CARTESIAN_POINT ( 'NONE',  ( -16.51473224551069308, -9.474510206698971260, 36.66557627198102409 ) ) ;
#8214=CARTESIAN_POINT ( 'NONE',  ( 18.67979575497194134, -10.72451020669871369, 100.8344237280190185 ) ) ;
#8215=CARTESIAN_POINT ( 'NONE',  ( 17.40805194822032931, 6.112264579159340627, 96.66628727489391792 ) ) ;
#8217=CARTESIAN_POINT ( 'NONE',  ( -16.55341960407611168, -4.379528057220339221, 36.45724293864768839 ) ) ;
#8219=CARTESIAN_POINT ( 'NONE',  ( -5.719274019375978568, 21.55341960407610458, 40.20724293864769550 ) ) ;
#8221=CARTESIAN_POINT ( 'NONE',  ( -16.51473224551069308, -9.474510206698971260, 86.66557627198102409 ) ) ;
#8222=CARTESIAN_POINT ( 'NONE',  ( 12.06949235617757843, -12.14591786802309237, 83.12390960531436690 ) ) ;
#8223=CARTESIAN_POINT ( 'NONE',  ( 14.34966873604972726, -8.224510206698740333, 20.83442372801901143 ) ) ;
#8224=CARTESIAN_POINT ( 'NONE',  ( 4.379528057220339221, -16.55341960407611168, 22.70724293864769194 ) ) ;
#8225=ORIENTED_EDGE ( 'NONE', *, *, #128791, .T. ) ;
#8226=CARTESIAN_POINT ( 'NONE',  ( -0.05219959533909027116, -19.03943276465977164, 42.49890960531435269 ) ) ;
#8227=CARTESIAN_POINT ( 'NONE',  ( -5.049401038298153566, 19.05341960407611168, 85.20724293864766707 ) ) ;
#8228=CARTESIAN_POINT ( 'NONE',  ( 15.80617190586746368, 15.72974639402197994, 84.37390960531438111 ) ) ;
#8229=CARTESIAN_POINT ( 'NONE',  ( 4.379528057220339221, -16.55341960407611168, 27.70724293864769905 ) ) ;
#8230=CARTESIAN_POINT ( 'NONE',  ( -13.89961937509977652, 13.97604488694528158, 100.6239096053143669 ) ) ;
#8231=CARTESIAN_POINT ( 'NONE',  ( -19.05341960407617563, 5.049401038297882671, 83.54275706135233293 ) ) ;
#8232=CARTESIAN_POINT ( 'NONE',  ( -21.55341960407619339, 5.719274019375674811, 108.5427570613523756 ) ) ;
#8233=CARTESIAN_POINT ( 'NONE',  ( -21.53943276465977519, 0.05219959533907696930, 86.24890960531436690 ) ) ;
#8234=CARTESIAN_POINT ( 'NONE',  ( -10.72451020669898014, 18.67979575497178502, 40.41557627198103120 ) ) ;
#8235=CARTESIAN_POINT ( 'NONE',  ( -5.049401038298153566, 19.05341960407611168, 70.20724293864769550 ) ) ;
#8236=CARTESIAN_POINT ( 'NONE',  ( -12.14591786802309592, -12.06949235617757132, 36.87390960531435979 ) ) ;
#8237=CARTESIAN_POINT ( 'NONE',  ( 5.153800228976335163, 19.02544592524342804, 74.79057627198103830 ) ) ;
#8239=CARTESIAN_POINT ( 'NONE',  ( 18.22780087662122739, 5.500000000000000888, 76.48236817873106475 ) ) ;
#8240=CARTESIAN_POINT ( 'NONE',  ( 19.02544592524334988, 5.153800228976608722, 26.45942372801899722 ) ) ;
#8241=CARTESIAN_POINT ( 'NONE',  ( -14.34966873604960291, -8.224510206698953496, 81.66557627198103830 ) ) ;
#8242=CARTESIAN_POINT ( 'NONE',  ( -21.53943276465977519, -0.05219959533937600094, 23.75109039468567929 ) ) ;
#8244=CARTESIAN_POINT ( 'NONE',  ( -5.823673210054116645, -21.52544592524344225, 72.29057627198102409 ) ) ;
#8245=CARTESIAN_POINT ( 'NONE',  ( -8.224510206698735004, -14.34966873604973081, 99.58442372801900433 ) ) ;
#8246=CARTESIAN_POINT ( 'NONE',  ( 19.05341960407611168, 5.049401038298154454, 28.95724293864769550 ) ) ;
#8247=CARTESIAN_POINT ( 'NONE',  ( -9.564922557960796823, -16.46253265017161027, 67.08224293864769550 ) ) ;
#8249=CARTESIAN_POINT ( 'NONE',  ( 4.379528057220339221, -16.55341960407611168, 32.70724293864770260 ) ) ;
#8250=CARTESIAN_POINT ( 'NONE',  ( 5.823673210054444382, -21.52544592524334988, 65.20942372801901854 ) ) ;
#8252=CARTESIAN_POINT ( 'NONE',  ( 10.72451020669871369, 18.67979575497193778, 97.08442372801904696 ) ) ;
#8253=CARTESIAN_POINT ( 'NONE',  ( 19.05341960407611168, 5.049401038298154454, 48.95724293864768129 ) ) ;
#8254=CARTESIAN_POINT ( 'NONE',  ( -19.03943276465977164, 0.05219959533909376836, 51.24890960531436690 ) ) ;
#8256=CARTESIAN_POINT ( 'NONE',  ( -21.53943276465977519, -0.05219959533937600094, 98.75109039468568994 ) ) ;
#8257=CARTESIAN_POINT ( 'NONE',  ( -0.05219959533934338120, 16.53943276465976808, 57.50109039468568994 ) ) ;
#8258=CARTESIAN_POINT ( 'NONE',  ( 10.81492255796106328, -18.62759615963255655, 80.41775706135234714 ) ) ;
#8259=CARTESIAN_POINT ( 'NONE',  ( 0.05219959533907565091, 21.53943276465977519, 24.99890960531435624 ) ) ;
#8260=CARTESIAN_POINT ( 'NONE',  ( -16.51473224551082808, 9.474510206698731452, 93.33442372801900433 ) ) ;
#8261=CARTESIAN_POINT ( 'NONE',  ( 10.81492255796106328, -18.62759615963255655, 50.41775706135235424 ) ) ;
#8262=CARTESIAN_POINT ( 'NONE',  ( -16.55341960407617563, 4.379528057220093196, 38.54275706135234714 ) ) ;
#8264=CARTESIAN_POINT ( 'NONE',  ( -0.05219959533907301413, -21.53943276465977519, 87.49890960531436690 ) ) ;
#8265=CARTESIAN_POINT ( 'NONE',  ( 9.474510206698729675, 16.51473224551082808, 92.08442372801900433 ) ) ;
#8266=CARTESIAN_POINT ( 'NONE',  ( 16.46253265017160672, -9.564922557960803928, 68.33224293864770971 ) ) ;
#8267=CARTESIAN_POINT ( 'NONE',  ( 5.153800228976615827, -19.02544592524334988, 100.2094237280190043 ) ) ;
#8268=CARTESIAN_POINT ( 'NONE',  ( -5.153800228976607833, 19.02544592524334988, 107.7094237280189759 ) ) ;
#8269=CARTESIAN_POINT ( 'NONE',  ( -8.314922557960811034, -14.29746914071050412, 52.08224293864768839 ) ) ;
#8270=CARTESIAN_POINT ( 'NONE',  ( 9.564922557961047289, -16.46253265017146816, 80.41775706135234714 ) ) ;
#8272=CARTESIAN_POINT ( 'NONE',  ( -4.483927247898782831, 16.52544592524335698, 57.70942372801901143 ) ) ;
#8273=CARTESIAN_POINT ( 'NONE',  ( -9.564922557961040184, 16.46253265017147172, 37.91775706135233293 ) ) ;
#8274=CARTESIAN_POINT ( 'NONE',  ( -16.51473224551069308, -9.474510206698971260, 36.66557627198102409 ) ) ;
#8275=CARTESIAN_POINT ( 'NONE',  ( 13.89961937509977652, -13.97604488694527269, 53.12390960531434558 ) ) ;
#8276=CARTESIAN_POINT ( 'NONE',  ( -12.06949235617739369, -12.14591786802326823, 54.37609039468568994 ) ) ;
#8279=CARTESIAN_POINT ( 'NONE',  ( -19.05341960407611168, -5.049401038298163336, 106.4572429386476955 ) ) ;
#8280=CARTESIAN_POINT ( 'NONE',  ( 19.03943276465977164, -0.05219959533909143690, 28.74890960531435624 ) ) ;
#8282=CARTESIAN_POINT ( 'NONE',  ( 13.89961937509957401, 13.97604488694547697, 101.8760903946856331 ) ) ;
#8283=CARTESIAN_POINT ( 'NONE',  ( -21.52544592524343514, 5.823673210054127303, 36.04057627198102409 ) ) ;
#8284=CARTESIAN_POINT ( 'NONE',  ( -0.05219959533936034679, 19.03943276465977164, 27.50109039468566507 ) ) ;
#8285=CARTESIAN_POINT ( 'NONE',  ( 12.14591786802327356, -12.06949235617739191, 20.62609039468568639 ) ) ;
#8286=CARTESIAN_POINT ( 'NONE',  ( -9.474510206698964154, 16.51473224551069663, 30.41557627198102054 ) ) ;
#8287=CARTESIAN_POINT ( 'NONE',  ( -19.02544592524342804, 5.153800228976336051, 46.04057627198101699 ) ) ;
#8288=CARTESIAN_POINT ( 'NONE',  ( 0.05219959533907565091, 21.53943276465977519, 69.99890960531435269 ) ) ;
#8289=CARTESIAN_POINT ( 'NONE',  ( 16.46253265017160672, -9.564922557960803928, 103.3322429386476955 ) ) ;
#8290=CARTESIAN_POINT ( 'NONE',  ( 9.564922557960805705, 16.46253265017160317, 34.58224293864770260 ) ) ;
#8292=CARTESIAN_POINT ( 'NONE',  ( 13.89961937509957401, 13.97604488694547697, 86.87609039468567573 ) ) ;
#8293=CARTESIAN_POINT ( 'NONE',  ( -0.05219959533910754901, -16.53943276465976808, 72.49890960531435269 ) ) ;
#8294=CARTESIAN_POINT ( 'NONE',  ( 15.80617190586746368, 15.72974639402197994, 44.37390960531435979 ) ) ;
#8295=CARTESIAN_POINT ( 'NONE',  ( 21.55341960407619695, -5.719274019375665929, 111.0427570613523613 ) ) ;
#8296=CARTESIAN_POINT ( 'NONE',  ( 10.72451020669898902, -18.67979575497178502, 97.91557627198103830 ) ) ;
#8297=CARTESIAN_POINT ( 'NONE',  ( 15.72974639402176855, 15.80617190586768217, 66.87609039468568994 ) ) ;
#8298=CARTESIAN_POINT ( 'NONE',  ( 10.81492255796106328, -18.62759615963255655, 80.41775706135234714 ) ) ;
#8300=CARTESIAN_POINT ( 'NONE',  ( -19.03943276465977164, 0.05219959533909376836, 111.2489096053143669 ) ) ;
#8301=CARTESIAN_POINT ( 'NONE',  ( -8.314922557961024197, 14.29746914071037800, 102.9177570613523756 ) ) ;
#8302=CARTESIAN_POINT ( 'NONE',  ( 21.55341960407619695, -5.719274019375665929, 76.04275706135237556 ) ) ;
#8303=CARTESIAN_POINT ( 'NONE',  ( 9.474510206698971260, -16.51473224551069308, 67.91557627198102409 ) ) ;
#8304=CARTESIAN_POINT ( 'NONE',  ( -16.46253265017146816, -9.564922557961047289, 34.16775706135233293 ) ) ;
#8305=CARTESIAN_POINT ( 'NONE',  ( 21.52544592524334988, 5.823673210054432836, 31.45942372801901854 ) ) ;
#8306=CARTESIAN_POINT ( 'NONE',  ( -16.51473224551069308, -9.474510206698971260, 61.66557627198103120 ) ) ;
#8307=CARTESIAN_POINT ( 'NONE',  ( 12.14591786802309770, 12.06949235617756955, 79.37390960531436690 ) ) ;
#8308=CARTESIAN_POINT ( 'NONE',  ( 14.29746914071049879, -8.314922557960816363, 53.33224293864769550 ) ) ;
#8309=CARTESIAN_POINT ( 'NONE',  ( -5.823673210054116645, -21.52544592524344225, 52.29057627198102409 ) ) ;
#8311=CARTESIAN_POINT ( 'NONE',  ( 13.97604488694527802, 13.89961937509977652, 59.37390960531434558 ) ) ;
#8312=CARTESIAN_POINT ( 'NONE',  ( -5.719274019375978568, 21.55341960407610458, 70.20724293864769550 ) ) ;
#8313=CARTESIAN_POINT ( 'NONE',  ( 13.89961937509957401, 13.97604488694547697, 61.87609039468566863 ) ) ;
#8314=CARTESIAN_POINT ( 'NONE',  ( -19.02544592524335343, -5.153800228976618492, 23.95942372801900078 ) ) ;
#8315=CARTESIAN_POINT ( 'NONE',  ( 16.53943276465976808, -0.05219959533910856209, 63.74890960531435979 ) ) ;
#8316=CARTESIAN_POINT ( 'NONE',  ( 15.80617190586746368, 15.72974639402197994, 39.37390960531436690 ) ) ;
#8318=CARTESIAN_POINT ( 'NONE',  ( 16.19135201231366850, 7.376712067591939537, 102.6868085405203459 ) ) ;
#8319=CARTESIAN_POINT ( 'NONE',  ( 4.483927247898790824, -16.52544592524335698, 85.20942372801901854 ) ) ;
#8321=CARTESIAN_POINT ( 'NONE',  ( -0.05219959533936034679, 19.03943276465977164, 82.50109039468567573 ) ) ;
#8322=CARTESIAN_POINT ( 'NONE',  ( 0.05219959533910956823, 16.53943276465976808, 54.99890960531435269 ) ) ;
#8324=CARTESIAN_POINT ( 'NONE',  ( 19.02544592524343514, -5.153800228976328945, 48.54057627198103120 ) ) ;
#8325=CARTESIAN_POINT ( 'NONE',  ( -16.52544592524342804, 4.483927247898546575, 46.04057627198103830 ) ) ;
#8326=CARTESIAN_POINT ( 'NONE',  ( 5.049401038298161559, -19.05341960407611168, 87.70724293864769550 ) ) ;
#8327=CARTESIAN_POINT ( 'NONE',  ( 19.05341960407611168, 5.049401038298154454, 58.95724293864768129 ) ) ;
#8328=CARTESIAN_POINT ( 'NONE',  ( 21.55341960407619695, -5.719274019375665929, 66.04275706135236135 ) ) ;
#8329=CARTESIAN_POINT ( 'NONE',  ( 9.564922557960805705, 16.46253265017160317, 74.58224293864769550 ) ) ;
#8330=CARTESIAN_POINT ( 'NONE',  ( 13.89961937509977652, -13.97604488694527269, 33.12390960531434558 ) ) ;
#8331=CARTESIAN_POINT ( 'NONE',  ( 19.05341960407611168, 5.049401038298154454, 73.95724293864768129 ) ) ;
#8332=CARTESIAN_POINT ( 'NONE',  ( 21.53943276465977519, -0.05219959533907433946, 48.74890960531435979 ) ) ;
#8333=CARTESIAN_POINT ( 'NONE',  ( 0.05219959533909260263, 19.03943276465977164, 54.99890960531435979 ) ) ;
#8334=CARTESIAN_POINT ( 'NONE',  ( 18.67979575497178502, 10.72451020669898547, 54.16557627198103120 ) ) ;
#8336=CARTESIAN_POINT ( 'NONE',  ( 16.51473224551083163, -9.474510206698727899, 80.83442372801899012 ) ) ;
#8337=CARTESIAN_POINT ( 'NONE',  ( -4.483927247898782831, 16.52544592524335698, 102.7094237280190185 ) ) ;
#8338=CARTESIAN_POINT ( 'NONE',  ( -19.02544592524334988, -5.153800228976617603, 38.95942372801900433 ) ) ;
#8339=CARTESIAN_POINT ( 'NONE',  ( -8.224510206698735004, -14.34966873604973081, 64.58442372801900433 ) ) ;
#8340=CARTESIAN_POINT ( 'NONE',  ( 4.379528057220092307, 16.55341960407617563, 82.29275706135234714 ) ) ;
#8342=CARTESIAN_POINT ( 'NONE',  ( 14.34966873604972726, -8.224510206698740333, 65.83442372801900433 ) ) ;
#8343=CARTESIAN_POINT ( 'NONE',  ( -18.67979575497178146, -10.72451020669898902, 26.66557627198103475 ) ) ;
#8344=CARTESIAN_POINT ( 'NONE',  ( 19.03943276465977164, -0.05219959533909143690, 28.74890960531435624 ) ) ;
#8345=CARTESIAN_POINT ( 'NONE',  ( -14.34966873604972548, 8.224510206698743886, 43.33442372801901143 ) ) ;
#8346=CARTESIAN_POINT ( 'NONE',  ( -5.049401038298153566, 19.05341960407611168, 50.20724293864770260 ) ) ;
#8347=CARTESIAN_POINT ( 'NONE',  ( 21.52544592524334988, 5.823673210054432836, 41.45942372801901143 ) ) ;
#8348=CARTESIAN_POINT ( 'NONE',  ( -8.224510206698735004, -14.34966873604973081, 29.58442372801901854 ) ) ;
#8349=CARTESIAN_POINT ( 'NONE',  ( -12.14591786802326823, 12.06949235617739902, 103.1260903946856757 ) ) ;
#8350=CARTESIAN_POINT ( 'NONE',  ( -17.60779699588842462, -5.499999999999949374, 71.34981316670105400 ) ) ;
#8351=CARTESIAN_POINT ( 'NONE',  ( 21.52544592524334988, 5.823673210054432836, 111.4594237280190328 ) ) ;
#8352=CARTESIAN_POINT ( 'NONE',  ( 19.05341960407617918, -5.049401038297876454, 111.0427570613523329 ) ) ;
#8353=CARTESIAN_POINT ( 'NONE',  ( 5.153800228976615827, -19.02544592524334988, 65.20942372801900433 ) ) ;
#8354=CARTESIAN_POINT ( 'NONE',  ( -16.53943276465976808, 0.05219959533911058130, 76.24890960531435269 ) ) ;
#8355=CARTESIAN_POINT ( 'NONE',  ( -9.474510206698964154, 16.51473224551069663, 35.41557627198102409 ) ) ;
#8356=CARTESIAN_POINT ( 'NONE',  ( -16.51473224551082808, 9.474510206698731452, 63.33442372801900433 ) ) ;
#8357=CARTESIAN_POINT ( 'NONE',  ( 17.31747979337949062, 6.344076630961017926, 78.87944868065184778 ) ) ;
#8358=CARTESIAN_POINT ( 'NONE',  ( -21.52544592524334988, -5.823673210054445271, 58.95942372801902565 ) ) ;
#8359=CARTESIAN_POINT ( 'NONE',  ( 12.06949235617739724, 12.14591786802326823, 36.87609039468568994 ) ) ;
#8361=CARTESIAN_POINT ( 'NONE',  ( -10.81492255796078084, -18.62759615963271287, 22.08224293864769194 ) ) ;
#8362=CARTESIAN_POINT ( 'NONE',  ( -5.049401038297874678, -19.05341960407617918, 104.7927570613523471 ) ) ;
#8363=CARTESIAN_POINT ( 'NONE',  ( -19.05341960407611168, -5.049401038298163336, 111.4572429386476671 ) ) ;
#8365=CARTESIAN_POINT ( 'NONE',  ( 9.474510206698971260, -16.51473224551069308, 27.91557627198103120 ) ) ;
#8366=CARTESIAN_POINT ( 'NONE',  ( 15.72974639402176855, 15.80617190586768217, 111.8760903946856615 ) ) ;
#8367=CARTESIAN_POINT ( 'NONE',  ( 5.153800228976335163, 19.02544592524342804, 59.79057627198100988 ) ) ;
#8369=CARTESIAN_POINT ( 'NONE',  ( 18.67979575497194134, -10.72451020669871369, 60.83442372801901854 ) ) ;
#8370=CARTESIAN_POINT ( 'NONE',  ( 10.72451020669871369, 18.67979575497193778, 97.08442372801904696 ) ) ;
#8371=CARTESIAN_POINT ( 'NONE',  ( 4.483927247898545687, 16.52544592524342804, 24.79057627198103120 ) ) ;
#8372=CARTESIAN_POINT ( 'NONE',  ( 16.46253265017160672, -9.564922557960803928, 33.33224293864770260 ) ) ;
#8373=CARTESIAN_POINT ( 'NONE',  ( -13.97604488694527625, -13.89961937509977652, 96.87390960531433848 ) ) ;
#8374=CARTESIAN_POINT ( 'NONE',  ( -5.823673210054431948, 21.52544592524334988, 57.70942372801901143 ) ) ;
#8375=CARTESIAN_POINT ( 'NONE',  ( 19.03943276465977164, -0.05219959533909143690, 38.74890960531436690 ) ) ;
#8376=CARTESIAN_POINT ( 'NONE',  ( -21.53943276465977519, -0.05219959533937600094, 53.75109039468568994 ) ) ;
#8377=CARTESIAN_POINT ( 'NONE',  ( -19.03943276465977164, -0.05219959533935918106, 83.75109039468567573 ) ) ;
#8378=CARTESIAN_POINT ( 'NONE',  ( 13.97604488694527802, 13.89961937509977652, 99.37390960531436690 ) ) ;
#8379=CARTESIAN_POINT ( 'NONE',  ( 16.53943276465976808, -0.05219959533910856209, 113.7489096053143527 ) ) ;
#8380=CARTESIAN_POINT ( 'NONE',  ( -15.80617190586745835, -15.72974639402198527, 111.8739096053143669 ) ) ;
#8381=CARTESIAN_POINT ( 'NONE',  ( 9.474510206698729675, 16.51473224551082808, 37.08442372801899722 ) ) ;
#8382=CARTESIAN_POINT ( 'NONE',  ( 16.52544592524342804, -4.483927247898539470, 93.54057627198103830 ) ) ;
#8383=CARTESIAN_POINT ( 'NONE',  ( -16.46253265017160317, 9.564922557960807481, 55.83224293864769550 ) ) ;
#8384=CARTESIAN_POINT ( 'NONE',  ( -13.89961937509957401, -13.97604488694547875, 104.3760903946856757 ) ) ;
#8385=CARTESIAN_POINT ( 'NONE',  ( 16.53943276465976808, -0.05219959533910856209, 58.74890960531436690 ) ) ;
#8386=CARTESIAN_POINT ( 'NONE',  ( -5.719274019375665041, -21.55341960407619695, 104.7927570613523898 ) ) ;
#8387=CARTESIAN_POINT ( 'NONE',  ( -16.46253265017160317, 9.564922557960807481, 100.8322429386477097 ) ) ;
#8388=CARTESIAN_POINT ( 'NONE',  ( -16.46253265017146816, -9.564922557961047289, 94.16775706135233293 ) ) ;
#8389=CARTESIAN_POINT ( 'NONE',  ( -18.62759615963270932, 10.81492255796079327, 90.83224293864769550 ) ) ;
#8390=CARTESIAN_POINT ( 'NONE',  ( -21.53943276465977519, -0.05219959533937600094, 43.75109039468568284 ) ) ;
#8391=CARTESIAN_POINT ( 'NONE',  ( 14.29746914071037800, 8.314922557961029526, 46.66775706135234714 ) ) ;
#8392=CARTESIAN_POINT ( 'NONE',  ( -16.55341960407617563, 4.379528057220093196, 108.5427570613523756 ) ) ;
#8393=CARTESIAN_POINT ( 'NONE',  ( 16.52544592524335698, 4.483927247898782831, 46.45942372801901854 ) ) ;
#8394=CARTESIAN_POINT ( 'NONE',  ( 5.823673210054444382, -21.52544592524334988, 45.20942372801901854 ) ) ;
#8395=CARTESIAN_POINT ( 'NONE',  ( -21.53943276465977519, 0.05219959533907696930, 41.24890960531435269 ) ) ;
#8396=CARTESIAN_POINT ( 'NONE',  ( 0.05219959533909260263, 19.03943276465977164, 34.99890960531435979 ) ) ;
#8398=CARTESIAN_POINT ( 'NONE',  ( 4.483927247898790824, -16.52544592524335698, 65.20942372801901854 ) ) ;
#8399=CARTESIAN_POINT ( 'NONE',  ( 21.52544592524344225, -5.823673210054117533, 83.54057627198102409 ) ) ;
#8400=CARTESIAN_POINT ( 'NONE',  ( -16.52544592524342804, 4.483927247898546575, 41.04057627198103120 ) ) ;
#8401=CARTESIAN_POINT ( 'NONE',  ( -14.29746914071037622, -8.314922557961029526, 59.16775706135234714 ) ) ;
#8402=CARTESIAN_POINT ( 'NONE',  ( -13.97604488694527625, -13.89961937509977652, 56.87390960531434558 ) ) ;
#8403=CARTESIAN_POINT ( 'NONE',  ( 16.51473224551083163, -9.474510206698727899, 95.83442372801900433 ) ) ;
#8404=CARTESIAN_POINT ( 'NONE',  ( 0.05219959533907565091, 21.53943276465977519, 79.99890960531435269 ) ) ;
#8405=CARTESIAN_POINT ( 'NONE',  ( -12.14591786802309592, -12.06949235617757132, 31.87390960531435979 ) ) ;
#8407=CARTESIAN_POINT ( 'NONE',  ( 14.29746914071037800, 8.314922557961029526, 76.66775706135234714 ) ) ;
#8409=CARTESIAN_POINT ( 'NONE',  ( -5.823673210054116645, -21.52544592524344225, 77.29057627198102409 ) ) ;
#8411=CARTESIAN_POINT ( 'NONE',  ( 16.53943276465976808, 0.05219959533934440121, 111.2510903946856899 ) ) ;
#8413=DIRECTION ( 'NONE',  ( -1.000000000000000000, 0.000000000000000000, 0.000000000000000000 ) ) ;
#8414=CARTESIAN_POINT ( 'NONE',  ( 10.81492255796078972, 18.62759615963270932, 94.58224293864769550 ) ) ;
#8415=CIRCLE ( 'NONE', #73099, 2.500000000000002220 ) ;
#8416=CARTESIAN_POINT ( 'NONE',  ( 5.719274019375991003, -21.55341960407610458, 107.7072429386476955 ) ) ;
#8417=CARTESIAN_POINT ( 'NONE',  ( -8.224510206698948167, 14.34966873604960824, 30.41557627198101699 ) ) ;
#8418=CARTESIAN_POINT ( 'NONE',  ( -16.53943276465976808, -0.05219959533934237506, 28.75109039468567929 ) ) ;
#8419=CARTESIAN_POINT ( 'NONE',  ( -16.46253265017160317, 9.564922557960807481, 30.83224293864769550 ) ) ;
#8420=CARTESIAN_POINT ( 'NONE',  ( -19.02544592524342804, 5.153800228976336051, 71.04057627198099567 ) ) ;
#8422=CARTESIAN_POINT ( 'NONE',  ( 5.719274019375991003, -21.55341960407610458, 22.70724293864769194 ) ) ;
#8423=CARTESIAN_POINT ( 'NONE',  ( 18.22780087662121673, 5.500000000000056843, 63.98459894673894155 ) ) ;
#8424=CARTESIAN_POINT ( 'NONE',  ( 5.153800228976615827, -19.02544592524334988, 105.2094237280190185 ) ) ;
#8425=CARTESIAN_POINT ( 'NONE',  ( 9.564922557961047289, -16.46253265017146816, 40.41775706135234003 ) ) ;
#8426=CARTESIAN_POINT ( 'NONE',  ( 21.52544592524344225, -5.823673210054117533, 88.54057627198103830 ) ) ;
#8427=CARTESIAN_POINT ( 'NONE',  ( 14.29746914071037800, 8.314922557961029526, 111.6677570613523613 ) ) ;
#8428=CARTESIAN_POINT ( 'NONE',  ( -21.55341960407610458, -5.719274019375992779, 46.45724293864769550 ) ) ;
#8429=CARTESIAN_POINT ( 'NONE',  ( -5.823673210054116645, -21.52544592524344225, 87.29057627198103830 ) ) ;
#8430=CARTESIAN_POINT ( 'NONE',  ( -5.049401038297874678, -19.05341960407617918, 104.7927570613523471 ) ) ;
#8431=CARTESIAN_POINT ( 'NONE',  ( -16.51473224551069308, -9.474510206698971260, 106.6655762719810383 ) ) ;
#8432=CARTESIAN_POINT ( 'NONE',  ( 18.62759615963255655, 10.81492255796105972, 81.66775706135236135 ) ) ;
#8433=CARTESIAN_POINT ( 'NONE',  ( 5.153800228976335163, 19.02544592524342804, 69.79057627198103830 ) ) ;
#8434=CARTESIAN_POINT ( 'NONE',  ( -14.34966873604960291, -8.224510206698953496, 101.6655762719810383 ) ) ;
#8436=CARTESIAN_POINT ( 'NONE',  ( -0.05219959533909027116, -19.03943276465977164, 72.49890960531435269 ) ) ;
#8437=CARTESIAN_POINT ( 'NONE',  ( -0.05219959533910754901, -16.53943276465976808, 87.49890960531436690 ) ) ;
#8439=CARTESIAN_POINT ( 'NONE',  ( -13.97604488694547697, 13.89961937509957934, 103.1260903946856473 ) ) ;
#8440=CARTESIAN_POINT ( 'NONE',  ( 19.05341960407611168, 5.049401038298154454, 53.95724293864770260 ) ) ;
#8441=CARTESIAN_POINT ( 'NONE',  ( 15.80617190586769283, -15.72974639402175789, 85.62609039468568994 ) ) ;
#8442=CARTESIAN_POINT ( 'NONE',  ( -16.51473224551069308, -9.474510206698971260, 96.66557627198102409 ) ) ;
#8443=CARTESIAN_POINT ( 'NONE',  ( -14.34966873604972548, 8.224510206698743886, 78.33442372801901854 ) ) ;
#8445=CARTESIAN_POINT ( 'NONE',  ( -16.51473224551082808, 9.474510206698731452, 58.33442372801900433 ) ) ;
#8446=CARTESIAN_POINT ( 'NONE',  ( -10.81492255796105439, 18.62759615963255655, 102.9177570613523756 ) ) ;
#8449=CARTESIAN_POINT ( 'NONE',  ( 8.314922557960818139, 14.29746914071049879, 24.58224293864768839 ) ) ;
#8451=CARTESIAN_POINT ( 'NONE',  ( 14.29746914071037800, 8.314922557961029526, 96.66775706135234714 ) ) ;
#8453=CARTESIAN_POINT ( 'NONE',  ( -8.314922557961024197, 14.29746914071037800, 67.91775706135234714 ) ) ;
#8455=CARTESIAN_POINT ( 'NONE',  ( 15.80617190586769283, -15.72974639402175789, 85.62609039468568994 ) ) ;
#8456=CARTESIAN_POINT ( 'NONE',  ( 13.89961937509957401, 13.97604488694547697, 86.87609039468567573 ) ) ;
#8457=CARTESIAN_POINT ( 'NONE',  ( 16.46253265017146816, 9.564922557961045513, 36.66775706135233293 ) ) ;
#8458=CARTESIAN_POINT ( 'NONE',  ( 16.51473224551069308, 9.474510206698969483, 69.16557627198102409 ) ) ;
#8459=CARTESIAN_POINT ( 'NONE',  ( 13.89961937509977652, -13.97604488694527269, 58.12390960531436690 ) ) ;
#8461=CARTESIAN_POINT ( 'NONE',  ( -21.55341960407610458, -5.719274019375992779, 76.45724293864769550 ) ) ;
#8462=CARTESIAN_POINT ( 'NONE',  ( 10.72451020669898902, -18.67979575497178502, 32.91557627198102409 ) ) ;
#8463=CARTESIAN_POINT ( 'NONE',  ( 9.474510206698971260, -16.51473224551069308, 37.91557627198102409 ) ) ;
#8464=CARTESIAN_POINT ( 'NONE',  ( 4.379528057220092307, 16.55341960407617563, 67.29275706135234714 ) ) ;
#8465=EDGE_LOOP ( 'NONE', ( #183152, #145287 ) ) ;
#8466=CARTESIAN_POINT ( 'NONE',  ( -0.05219959533937732626, 21.53943276465977519, 27.50109039468567929 ) ) ;
#8467=CARTESIAN_POINT ( 'NONE',  ( 4.483927247898545687, 16.52544592524342804, 69.79057627198102409 ) ) ;
#8469=CARTESIAN_POINT ( 'NONE',  ( 0.05219959533934541429, -16.53943276465976808, 25.00109039468567218 ) ) ;
#8470=CARTESIAN_POINT ( 'NONE',  ( 19.05341960407617918, -5.049401038297876454, 56.04275706135234714 ) ) ;
#8471=CARTESIAN_POINT ( 'NONE',  ( 8.314922557960818139, 14.29746914071049879, 59.58224293864770260 ) ) ;
#8472=CARTESIAN_POINT ( 'NONE',  ( -21.52544592524334988, -5.823673210054445271, 28.95942372801902209 ) ) ;
#8474=CARTESIAN_POINT ( 'NONE',  ( -18.67979575497178146, -10.72451020669898902, 71.66557627198100988 ) ) ;
#8475=CARTESIAN_POINT ( 'NONE',  ( -19.03943276465977164, 0.05219959533909376836, 101.2489096053143669 ) ) ;
#8476=CARTESIAN_POINT ( 'NONE',  ( -4.483927247898539470, -16.52544592524342804, 72.29057627198102409 ) ) ;
#8478=CARTESIAN_POINT ( 'NONE',  ( 17.60779699588838199, 5.500000000000005329, 43.84981316670103979 ) ) ;
#8479=CARTESIAN_POINT ( 'NONE',  ( 19.05341960407617918, -5.049401038297876454, 66.04275706135233293 ) ) ;
#8480=CARTESIAN_POINT ( 'NONE',  ( -18.62759615963255300, -10.81492255796106328, 29.16775706135234003 ) ) ;
#8481=CARTESIAN_POINT ( 'NONE',  ( 16.46253265017160672, -9.564922557960803928, 63.33224293864769550 ) ) ;
#8482=CARTESIAN_POINT ( 'NONE',  ( -13.97604488694547697, 13.89961937509957934, 43.12609039468566152 ) ) ;
#8483=CARTESIAN_POINT ( 'NONE',  ( 13.89961937509977652, -13.97604488694527269, 28.12390960531435624 ) ) ;
#8484=CARTESIAN_POINT ( 'NONE',  ( -18.62759615963255300, -10.81492255796106328, 64.16775706135234714 ) ) ;
#8486=CARTESIAN_POINT ( 'NONE',  ( 0.05219959533910956823, 16.53943276465976808, 39.99890960531436690 ) ) ;
#8487=CARTESIAN_POINT ( 'NONE',  ( 19.03943276465977164, -0.05219959533909143690, 68.74890960531436690 ) ) ;
#8488=CARTESIAN_POINT ( 'NONE',  ( -18.62759615963270932, 10.81492255796079327, 85.83224293864768129 ) ) ;
#8489=CARTESIAN_POINT ( 'NONE',  ( -0.05219959533909027116, -19.03943276465977164, 62.49890960531435979 ) ) ;
#8490=ORIENTED_EDGE ( 'NONE', *, *, #15491, .T. ) ;
#8491=CARTESIAN_POINT ( 'NONE',  ( -21.55341960407610458, -5.719274019375992779, 61.45724293864770260 ) ) ;
#8492=CARTESIAN_POINT ( 'NONE',  ( -10.72451020669870658, -18.67979575497194134, 104.5844237280190185 ) ) ;
#8494=CARTESIAN_POINT ( 'NONE',  ( 14.29746914071037800, 8.314922557961029526, 91.66775706135234714 ) ) ;
#8495=CARTESIAN_POINT ( 'NONE',  ( -4.483927247898539470, -16.52544592524342804, 77.29057627198102409 ) ) ;
#8496=CARTESIAN_POINT ( 'NONE',  ( 16.46253265017146816, 9.564922557961045513, 91.66775706135234714 ) ) ;
#8498=CARTESIAN_POINT ( 'NONE',  ( -10.72451020669898014, 18.67979575497178502, 110.4155762719810383 ) ) ;
#8499=CARTESIAN_POINT ( 'NONE',  ( -9.474510206698720793, -16.51473224551083518, 34.58442372801899722 ) ) ;
#8500=CARTESIAN_POINT ( 'NONE',  ( 8.224510206698742110, 14.34966873604972548, 102.0844237280190185 ) ) ;
#8501=CARTESIAN_POINT ( 'NONE',  ( -16.46253265017146816, -9.564922557961047289, 34.16775706135233293 ) ) ;
#8502=CARTESIAN_POINT ( 'NONE',  ( -16.46253265017160317, 9.564922557960807481, 85.83224293864769550 ) ) ;
#8503=CARTESIAN_POINT ( 'NONE',  ( 21.53943276465977519, -0.05219959533907433946, 63.74890960531435979 ) ) ;
#8504=CARTESIAN_POINT ( 'NONE',  ( 4.379528057220339221, -16.55341960407611168, 112.7072429386476955 ) ) ;
#8505=CARTESIAN_POINT ( 'NONE',  ( 18.62759615963255655, 10.81492255796105972, 111.6677570613523613 ) ) ;
#8506=CARTESIAN_POINT ( 'NONE',  ( 8.314922557961029526, -14.29746914071037800, 80.41775706135234714 ) ) ;
#8507=CARTESIAN_POINT ( 'NONE',  ( 5.823673210054444382, -21.52544592524334988, 30.20942372801902565 ) ) ;
#8508=CARTESIAN_POINT ( 'NONE',  ( -4.379528057220086978, -16.55341960407618274, 34.79275706135235424 ) ) ;
#8509=CARTESIAN_POINT ( 'NONE',  ( 9.564922557960805705, 16.46253265017160317, 99.58224293864770971 ) ) ;
#8510=CARTESIAN_POINT ( 'NONE',  ( -16.46253265017160317, 9.564922557960807481, 40.83224293864769550 ) ) ;
#8511=CARTESIAN_POINT ( 'NONE',  ( -16.51473224551069308, -9.474510206698971260, 61.66557627198103120 ) ) ;
#8513=CARTESIAN_POINT ( 'NONE',  ( -12.06949235617739369, -12.14591786802326823, 44.37609039468567573 ) ) ;
#8514=CARTESIAN_POINT ( 'NONE',  ( -14.34966873604960291, -8.224510206698953496, 96.66557627198102409 ) ) ;
#8515=CARTESIAN_POINT ( 'NONE',  ( -14.34966873604972548, 8.224510206698743886, 103.3344237280190043 ) ) ;
#8516=CARTESIAN_POINT ( 'NONE',  ( 21.53943276465977519, 0.05219959533937863772, 46.25109039468567573 ) ) ;
#8517=CARTESIAN_POINT ( 'NONE',  ( 19.03943276465977164, -0.05219959533909143690, 78.74890960531436690 ) ) ;
#8518=CARTESIAN_POINT ( 'NONE',  ( 5.153800228976335163, 19.02544592524342804, 69.79057627198103830 ) ) ;
#8519=CARTESIAN_POINT ( 'NONE',  ( -5.153800228976328057, -19.02544592524343514, 102.2905762719810383 ) ) ;
#8520=CARTESIAN_POINT ( 'NONE',  ( 14.34966873604960469, 8.224510206698951720, 34.16557627198102409 ) ) ;
#8521=CARTESIAN_POINT ( 'NONE',  ( -4.483927247898782831, 16.52544592524335698, 92.70942372801901854 ) ) ;
#8523=CARTESIAN_POINT ( 'NONE',  ( 16.51473224551083163, -9.474510206698727899, 40.83442372801900433 ) ) ;
#8524=CARTESIAN_POINT ( 'NONE',  ( -16.51473224551069308, -9.474510206698971260, 111.6655762719810383 ) ) ;
#8525=CARTESIAN_POINT ( 'NONE',  ( 16.51473224551069308, 9.474510206698969483, 64.16557627198102409 ) ) ;
#8526=CARTESIAN_POINT ( 'NONE',  ( -19.03943276465977164, -0.05219959533935918106, 38.75109039468566152 ) ) ;
#8528=CARTESIAN_POINT ( 'NONE',  ( 19.53037848336980886, -5.499999999999890754, 72.35532783611448338 ) ) ;
#8529=CARTESIAN_POINT ( 'NONE',  ( 4.483927247898790824, -16.52544592524335698, 55.20942372801902565 ) ) ;
#8530=CARTESIAN_POINT ( 'NONE',  ( 5.153800228976615827, -19.02544592524334988, 65.20942372801900433 ) ) ;
#8531=CARTESIAN_POINT ( 'NONE',  ( -4.379528057220086978, -16.55341960407618274, 54.79275706135235424 ) ) ;
#8532=CARTESIAN_POINT ( 'NONE',  ( -19.05341960407611168, -5.049401038298163336, 91.45724293864766707 ) ) ;
#8533=CARTESIAN_POINT ( 'NONE',  ( -21.55341960407610458, -5.719274019375992779, 111.4572429386476813 ) ) ;
#8534=CARTESIAN_POINT ( 'NONE',  ( 5.049401038297881783, 19.05341960407617563, 77.29275706135231871 ) ) ;
#8535=CARTESIAN_POINT ( 'NONE',  ( -19.05341960407611168, -5.049401038298163336, 106.4572429386476955 ) ) ;
#8536=CARTESIAN_POINT ( 'NONE',  ( 19.02544592524343514, -5.153800228976328945, 28.54057627198102409 ) ) ;
#8538=CARTESIAN_POINT ( 'NONE',  ( 9.474510206698971260, -16.51473224551069308, 82.91557627198103830 ) ) ;
#8539=CARTESIAN_POINT ( 'NONE',  ( -12.06949235617756955, 12.14591786802309770, 50.62390960531435979 ) ) ;
#8540=CARTESIAN_POINT ( 'NONE',  ( -19.05341960407611168, -5.049401038298163336, 36.45724293864766707 ) ) ;
#8541=CARTESIAN_POINT ( 'NONE',  ( 19.02544592524334988, 5.153800228976608722, 56.45942372801898301 ) ) ;
#8542=CARTESIAN_POINT ( 'NONE',  ( 16.55341960407611168, 4.379528057220329451, 88.95724293864769550 ) ) ;
#8543=CARTESIAN_POINT ( 'NONE',  ( 10.72451020669871369, 18.67979575497193778, 107.0844237280190043 ) ) ;
#8544=CARTESIAN_POINT ( 'NONE',  ( 16.51473224551069308, 9.474510206698969483, 49.16557627198102409 ) ) ;
#8545=EDGE_CURVE ( 'NONE', #129803, #55277, #158519, .T. ) ;
#8546=CARTESIAN_POINT ( 'NONE',  ( 5.823673210054125526, 21.52544592524343514, 54.79057627198104541 ) ) ;
#8547=CARTESIAN_POINT ( 'NONE',  ( -0.05219959533910754901, -16.53943276465976808, 47.49890960531435979 ) ) ;
#8548=CARTESIAN_POINT ( 'NONE',  ( -9.474510206698720793, -16.51473224551083518, 19.58442372801899722 ) ) ;
#8549=CARTESIAN_POINT ( 'NONE',  ( -13.97604488694527625, -13.89961937509977652, 101.8739096053143811 ) ) ;
#8551=CARTESIAN_POINT ( 'NONE',  ( 9.564922557960805705, 16.46253265017160317, 114.5822429386476955 ) ) ;
#8552=CARTESIAN_POINT ( 'NONE',  ( 19.03943276465977164, -0.05219959533909143690, 43.74890960531435979 ) ) ;
#8553=CARTESIAN_POINT ( 'NONE',  ( -16.51473224551069308, -9.474510206698971260, 31.66557627198102054 ) ) ;
#8554=CARTESIAN_POINT ( 'NONE',  ( 0.05219959533910956823, 16.53943276465976808, 84.99890960531436690 ) ) ;
#8555=CARTESIAN_POINT ( 'NONE',  ( -5.823673210054116645, -21.52544592524344225, 102.2905762719810383 ) ) ;
#8556=CARTESIAN_POINT ( 'NONE',  ( -0.05219959533909027116, -19.03943276465977164, 97.49890960531436690 ) ) ;
#8557=CARTESIAN_POINT ( 'NONE',  ( -5.823673210054116645, -21.52544592524344225, 107.2905762719810525 ) ) ;
#8558=CARTESIAN_POINT ( 'NONE',  ( 9.564922557960805705, 16.46253265017160317, 99.58224293864770971 ) ) ;
#8560=CARTESIAN_POINT ( 'NONE',  ( 0.05219959533910956823, 16.53943276465976808, 99.99890960531436690 ) ) ;
#8562=CARTESIAN_POINT ( 'NONE',  ( 0.05219959533909260263, 19.03943276465977164, 69.99890960531435269 ) ) ;
#8563=CARTESIAN_POINT ( 'NONE',  ( 21.52544592524344225, -5.823673210054117533, 78.54057627198103830 ) ) ;
#8566=CARTESIAN_POINT ( 'NONE',  ( -21.53943276465977519, 0.05219959533907696930, 26.24890960531435624 ) ) ;
#8567=LINE ( 'NONE', #134920, #185577 ) ;
#8568=CARTESIAN_POINT ( 'NONE',  ( 4.483927247898790824, -16.52544592524335698, 30.20942372801902565 ) ) ;
#8569=CARTESIAN_POINT ( 'NONE',  ( 14.29746914071049879, -8.314922557960816363, 108.3322429386477097 ) ) ;
#8571=CARTESIAN_POINT ( 'NONE',  ( 5.153800228976335163, 19.02544592524342804, 64.79057627198100988 ) ) ;
#8572=CARTESIAN_POINT ( 'NONE',  ( -8.314922557960811034, -14.29746914071050412, 77.08224293864769550 ) ) ;
#8573=CARTESIAN_POINT ( 'NONE',  ( -0.05219959533907301413, -21.53943276465977519, 27.49890960531435269 ) ) ;
#8574=CARTESIAN_POINT ( 'NONE',  ( 4.379528057220339221, -16.55341960407611168, 62.70724293864769550 ) ) ;
#8575=CARTESIAN_POINT ( 'NONE',  ( -19.03943276465977164, -0.05219959533935918106, 113.7510903946856757 ) ) ;
#8576=CARTESIAN_POINT ( 'NONE',  ( -10.72451020669870658, -18.67979575497194134, 74.58442372801901854 ) ) ;
#8577=CARTESIAN_POINT ( 'NONE',  ( 17.44279575226823198, -5.990770900252457842, 78.33557567514317554 ) ) ;
#8578=CARTESIAN_POINT ( 'NONE',  ( -18.67979575497178146, -10.72451020669898902, 21.66557627198102409 ) ) ;
#8579=CARTESIAN_POINT ( 'NONE',  ( 16.55341960407618274, -4.379528057220086978, 81.04275706135236135 ) ) ;
#8581=CARTESIAN_POINT ( 'NONE',  ( 13.97604488694527802, 13.89961937509977652, 39.37390960531435269 ) ) ;
#8582=CARTESIAN_POINT ( 'NONE',  ( 19.02544592524343514, -5.153800228976328945, 88.54057627198102409 ) ) ;
#8583=CARTESIAN_POINT ( 'NONE',  ( -15.72974639402197994, 15.80617190586746368, 90.62390960531436690 ) ) ;
#8584=CARTESIAN_POINT ( 'NONE',  ( -8.224510206698735004, -14.34966873604973081, 19.58442372801901143 ) ) ;
#8585=CARTESIAN_POINT ( 'NONE',  ( -4.483927247898539470, -16.52544592524342804, 52.29057627198102409 ) ) ;
#8586=CARTESIAN_POINT ( 'NONE',  ( 5.719274019375673035, 21.55341960407619339, 77.29275706135234714 ) ) ;
#8587=CARTESIAN_POINT ( 'NONE',  ( -8.314922557961024197, 14.29746914071037800, 102.9177570613523756 ) ) ;
#8590=CARTESIAN_POINT ( 'NONE',  ( -14.34966873604960291, -8.224510206698953496, 31.66557627198102054 ) ) ;
#8591=CARTESIAN_POINT ( 'NONE',  ( 4.483927247898790824, -16.52544592524335698, 55.20942372801902565 ) ) ;
#8592=CARTESIAN_POINT ( 'NONE',  ( 19.02544592524343514, -5.153800228976328945, 78.54057627198099567 ) ) ;
#8594=CARTESIAN_POINT ( 'NONE',  ( 5.049401038298161559, -19.05341960407611168, 82.70724293864770971 ) ) ;
#8595=CARTESIAN_POINT ( 'NONE',  ( 21.52544592524334988, 5.823673210054432836, 66.45942372801903275 ) ) ;
#8596=CARTESIAN_POINT ( 'NONE',  ( 8.314922557961029526, -14.29746914071037800, 70.41775706135236135 ) ) ;
#8597=CARTESIAN_POINT ( 'NONE',  ( 16.52544592524342804, -4.483927247898539470, 53.54057627198103120 ) ) ;
#8598=CARTESIAN_POINT ( 'NONE',  ( 19.02544592524343514, -5.153800228976328945, 68.54057627198103830 ) ) ;
#8600=( BOUNDED_CURVE ( )  B_SPLINE_CURVE ( 2, ( #149282, #26952, #69432, #162438, #54270, #115943, #99760, #72442, #178626, #194792, #23939, #164459, #134118 ),
 .UNSPECIFIED., .F., .F. ) 
 B_SPLINE_CURVE_WITH_KNOTS ( ( 3, 2, 2, 2, 2, 2, 3 ),
 ( 0.1866866425649248151, 0.1885964912280701788, 0.1929824561403508665, 0.1973684210526315819, 0.2017543859649122695, 0.2061403508771929849, 0.2080958793624286540 ),
 .UNSPECIFIED. ) 
 CURVE ( )  GEOMETRIC_REPRESENTATION_ITEM ( )  RATIONAL_B_SPLINE_CURVE ( ( 0.9832469066685285419, 0.9851625545550100060, 1.000000000000000000, 0.9659258262890683122, 1.000000000000000000, 0.9659258262890683122, 1.000000000000000000, 0.9659258262890683122, 1.000000000000000000, 0.9659258262890683122, 1.000000000000000000, 0.9848076720550082985, 0.9831626618144004848 ) ) 
 REPRESENTATION_ITEM ( '' )  );
#8601=CARTESIAN_POINT ( 'NONE',  ( 19.05341960407617918, -5.049401038297876454, 106.0427570613523471 ) ) ;
#8602=CARTESIAN_POINT ( 'NONE',  ( -14.29746914071049879, 8.314922557960819915, 115.8322429386477097 ) ) ;
#8603=CARTESIAN_POINT ( 'NONE',  ( 13.97604488694527802, 13.89961937509977652, 84.37390960531433848 ) ) ;
#8604=CARTESIAN_POINT ( 'NONE',  ( -12.14591786802326823, 12.06949235617739902, 23.12609039468567573 ) ) ;
#8606=CARTESIAN_POINT ( 'NONE',  ( -10.72451020669870658, -18.67979575497194134, 109.5844237280190328 ) ) ;
#8607=CARTESIAN_POINT ( 'NONE',  ( -8.224510206698735004, -14.34966873604973081, 84.58442372801903275 ) ) ;
#8608=CARTESIAN_POINT ( 'NONE',  ( -5.049401038297874678, -19.05341960407617918, 94.79275706135230450 ) ) ;
#8609=CARTESIAN_POINT ( 'NONE',  ( 0.05219959533910956823, 16.53943276465976808, 114.9989096053143669 ) ) ;
#8610=CARTESIAN_POINT ( 'NONE',  ( 16.52544592524335698, 4.483927247898782831, 61.45942372801901854 ) ) ;
#8612=CARTESIAN_POINT ( 'NONE',  ( 5.049401038297881783, 19.05341960407617563, 52.29275706135234003 ) ) ;
#8613=CARTESIAN_POINT ( 'NONE',  ( -18.62759615963255300, -10.81492255796106328, 94.16775706135237556 ) ) ;
#8614=CARTESIAN_POINT ( 'NONE',  ( 16.46253265017160672, -9.564922557960803928, 33.33224293864770260 ) ) ;
#8615=CARTESIAN_POINT ( 'NONE',  ( 19.03943276465977164, -0.05219959533909143690, 73.74890960531435269 ) ) ;
#8616=CARTESIAN_POINT ( 'NONE',  ( 0.05219959533910956823, 16.53943276465976808, 69.99890960531435269 ) ) ;
#8617=B_SPLINE_CURVE_WITH_KNOTS ( 'NONE', 3,
 ( #36357, #98009, #144536, #6022, #129359, #191054 ),
 .UNSPECIFIED., .F., .F.,
 ( 4, 2, 4 ),
 ( 0.003989672132298169478, 0.004372778065220577978, 0.004755883998142986478 ),
 .UNSPECIFIED. ) ;
#8618=CARTESIAN_POINT ( 'NONE',  ( -10.72451020669870658, -18.67979575497194134, 84.58442372801903275 ) ) ;
#8619=CARTESIAN_POINT ( 'NONE',  ( 19.03943276465977164, 0.05219959533936151252, 46.25109039468566863 ) ) ;
#8620=CARTESIAN_POINT ( 'NONE',  ( -9.564922557961040184, 16.46253265017147172, 47.91775706135233293 ) ) ;
#8621=CARTESIAN_POINT ( 'NONE',  ( -21.55341960407610458, -5.719274019375992779, 36.45724293864768839 ) ) ;
#8622=CARTESIAN_POINT ( 'NONE',  ( -21.52544592524334988, -5.823673210054445271, 98.95942372801903275 ) ) ;
#8623=CARTESIAN_POINT ( 'NONE',  ( -16.51473224551069308, -9.474510206698971260, 81.66557627198103830 ) ) ;
#8624=CARTESIAN_POINT ( 'NONE',  ( 15.80617190586769283, -15.72974639402175789, 90.62609039468567573 ) ) ;
#8625=CARTESIAN_POINT ( 'NONE',  ( 21.55341960407610458, 5.719274019375980345, 43.95724293864769550 ) ) ;
#8626=CARTESIAN_POINT ( 'NONE',  ( 9.564922557960805705, 16.46253265017160317, 89.58224293864769550 ) ) ;
#8627=CARTESIAN_POINT ( 'NONE',  ( -19.02544592524334988, -5.153800228976617603, 73.95942372801900433 ) ) ;
#8628=CARTESIAN_POINT ( 'NONE',  ( 9.564922557960805705, 16.46253265017160317, 94.58224293864769550 ) ) ;
#8629=CARTESIAN_POINT ( 'NONE',  ( 16.46253265017146816, 9.564922557961045513, 91.66775706135234714 ) ) ;
#8630=CARTESIAN_POINT ( 'NONE',  ( 14.29746914071037800, 8.314922557961029526, 36.66775706135234714 ) ) ;
#8631=CARTESIAN_POINT ( 'NONE',  ( -8.224510206698948167, 14.34966873604960824, 105.4155762719810383 ) ) ;
#8632=CARTESIAN_POINT ( 'NONE',  ( -9.564922557960796823, -16.46253265017161027, 72.08224293864770971 ) ) ;
#8633=CARTESIAN_POINT ( 'NONE',  ( 15.80617190586746368, 15.72974639402197994, 69.37390960531436690 ) ) ;
#8634=CARTESIAN_POINT ( 'NONE',  ( 14.34966873604972726, -8.224510206698740333, 30.83442372801902209 ) ) ;
#8635=CARTESIAN_POINT ( 'NONE',  ( -21.52544592524334988, -5.823673210054445271, 33.95942372801901143 ) ) ;
#8636=CARTESIAN_POINT ( 'NONE',  ( 21.52544592524334988, 5.823673210054432836, 86.45942372801901854 ) ) ;
#8637=CARTESIAN_POINT ( 'NONE',  ( 12.06949235617739724, 12.14591786802326823, 81.87609039468568994 ) ) ;
#8638=CARTESIAN_POINT ( 'NONE',  ( 16.46253265017160672, -9.564922557960803928, 68.33224293864770971 ) ) ;
#8639=CARTESIAN_POINT ( 'NONE',  ( 4.379528057220339221, -16.55341960407611168, 82.70724293864770971 ) ) ;
#8640=CARTESIAN_POINT ( 'NONE',  ( 4.379528057220092307, 16.55341960407617563, 97.29275706135234714 ) ) ;
#8641=CARTESIAN_POINT ( 'NONE',  ( -13.89961937509957401, -13.97604488694547875, 49.37609039468567573 ) ) ;
#8642=CARTESIAN_POINT ( 'NONE',  ( 10.81492255796106328, -18.62759615963255655, 25.41775706135235779 ) ) ;
#8643=CARTESIAN_POINT ( 'NONE',  ( 14.29746914071049879, -8.314922557960816363, 73.33224293864769550 ) ) ;
#8644=CARTESIAN_POINT ( 'NONE',  ( 9.474510206698971260, -16.51473224551069308, 97.91557627198102409 ) ) ;
#8645=CARTESIAN_POINT ( 'NONE',  ( 4.379528057220092307, 16.55341960407617563, 107.2927570613523471 ) ) ;
#8646=CARTESIAN_POINT ( 'NONE',  ( 18.62759615963255655, 10.81492255796105972, 66.66775706135234714 ) ) ;
#8647=CARTESIAN_POINT ( 'NONE',  ( -8.314922557961024197, 14.29746914071037800, 42.91775706135235424 ) ) ;
#8648=CARTESIAN_POINT ( 'NONE',  ( 10.72451020669871369, 18.67979575497193778, 42.08442372801901854 ) ) ;
#8649=CARTESIAN_POINT ( 'NONE',  ( -12.14591786802309592, -12.06949235617757132, 71.87390960531438111 ) ) ;
#8651=CARTESIAN_POINT ( 'NONE',  ( 15.72974639402199770, -15.80617190586745480, 113.1239096053143953 ) ) ;
#8652=CARTESIAN_POINT ( 'NONE',  ( -19.25918095147780207, -5.499999999999583444, 49.45284276293934056 ) ) ;
#8653=CARTESIAN_POINT ( 'NONE',  ( -8.314922557960811034, -14.29746914071050412, 47.08224293864770260 ) ) ;
#8654=DIRECTION ( 'NONE',  ( 0.000000000000000000, 0.000000000000000000, 1.000000000000000000 ) ) ;
#8655=CARTESIAN_POINT ( 'NONE',  ( 10.72451020669898902, -18.67979575497178502, 42.91557627198103120 ) ) ;
#8656=CARTESIAN_POINT ( 'NONE',  ( 4.483927247898545687, 16.52544592524342804, 74.79057627198105251 ) ) ;
#8658=CARTESIAN_POINT ( 'NONE',  ( -5.719274019375978568, 21.55341960407610458, 85.20724293864770971 ) ) ;
#8659=CARTESIAN_POINT ( 'NONE',  ( 19.03943276465977164, -0.05219959533909143690, 73.74890960531435269 ) ) ;
#8660=CARTESIAN_POINT ( 'NONE',  ( 13.89961937509977652, -13.97604488694527269, 43.12390960531434558 ) ) ;
#8661=CARTESIAN_POINT ( 'NONE',  ( -0.05219959533936034679, 19.03943276465977164, 72.50109039468566152 ) ) ;
#8662=CARTESIAN_POINT ( 'NONE',  ( 21.52544592524334988, 5.823673210054432836, 51.45942372801901854 ) ) ;
#8663=CARTESIAN_POINT ( 'NONE',  ( 10.72451020669898902, -18.67979575497178502, 57.91557627198103120 ) ) ;
#8664=CARTESIAN_POINT ( 'NONE',  ( 5.153800228976335163, 19.02544592524342804, 39.79057627198100988 ) ) ;
#8665=CARTESIAN_POINT ( 'NONE',  ( -9.474510206698964154, 16.51473224551069663, 75.41557627198103830 ) ) ;
#8667=CARTESIAN_POINT ( 'NONE',  ( 0.05219959533934541429, -16.53943276465976808, 50.00109039468568994 ) ) ;
#8668=CARTESIAN_POINT ( 'NONE',  ( -10.81492255796105439, 18.62759615963255655, 32.91775706135234714 ) ) ;
#8669=CARTESIAN_POINT ( 'NONE',  ( -5.719274019375665041, -21.55341960407619695, 59.79275706135234714 ) ) ;
#8670=CARTESIAN_POINT ( 'NONE',  ( -19.02544592524342804, 5.153800228976336051, 106.0405762719810241 ) ) ;
#8671=CARTESIAN_POINT ( 'NONE',  ( 10.72451020669898902, -18.67979575497178502, 82.91557627198103830 ) ) ;
#8672=CARTESIAN_POINT ( 'NONE',  ( 10.81492255796106328, -18.62759615963255655, 25.41775706135235779 ) ) ;
#8673=CARTESIAN_POINT ( 'NONE',  ( 8.314922557961029526, -14.29746914071037800, 45.41775706135234003 ) ) ;
#8675=CARTESIAN_POINT ( 'NONE',  ( -10.72451020669898014, 18.67979575497178502, 45.41557627198103830 ) ) ;
#8676=CARTESIAN_POINT ( 'NONE',  ( 19.03943276465977164, 0.05219959533936151252, 26.25109039468566507 ) ) ;
#8677=CARTESIAN_POINT ( 'NONE',  ( -9.474510206698964154, 16.51473224551069663, 50.41557627198102409 ) ) ;
#8678=CARTESIAN_POINT ( 'NONE',  ( 5.153800228976335163, 19.02544592524342804, 109.7905762719810099 ) ) ;
#8679=CARTESIAN_POINT ( 'NONE',  ( -13.97604488694527625, -13.89961937509977652, 91.87390960531432427 ) ) ;
#8680=CARTESIAN_POINT ( 'NONE',  ( -18.22780087662122028, 5.500000000000031086, 53.51540105326106556 ) ) ;
#8682=CARTESIAN_POINT ( 'NONE',  ( 9.474510206698729675, 16.51473224551082808, 72.08442372801900433 ) ) ;
#8683=CARTESIAN_POINT ( 'NONE',  ( -15.72974639402197994, 15.80617190586746368, 50.62390960531435979 ) ) ;
#8684=CARTESIAN_POINT ( 'NONE',  ( -12.06949235617756955, 12.14591786802309770, 30.62390960531436335 ) ) ;
#8685=CARTESIAN_POINT ( 'NONE',  ( 5.049401038297881783, 19.05341960407617563, 92.29275706135234714 ) ) ;
#8686=EDGE_CURVE ( 'NONE', #132603, #17083, #89459, .T. ) ;
#8688=CARTESIAN_POINT ( 'NONE',  ( 9.474510206698729675, 16.51473224551082808, 27.08442372801900433 ) ) ;
#8689=CARTESIAN_POINT ( 'NONE',  ( 13.89961937509957401, 13.97604488694547697, 91.87609039468567573 ) ) ;
#8690=CARTESIAN_POINT ( 'NONE',  ( 5.153800228976615827, -19.02544592524334988, 40.20942372801898301 ) ) ;
#8692=CARTESIAN_POINT ( 'NONE',  ( -19.02544592524342804, 5.153800228976336051, 56.04057627198100988 ) ) ;
#8693=CARTESIAN_POINT ( 'NONE',  ( 16.52544592524342804, -4.483927247898539470, 58.54057627198103120 ) ) ;
#8694=CARTESIAN_POINT ( 'NONE',  ( 5.153800228976335163, 19.02544592524342804, 29.79057627198102409 ) ) ;
#8695=CARTESIAN_POINT ( 'NONE',  ( 4.483927247898545687, 16.52544592524342804, 34.79057627198103120 ) ) ;
#8696=CARTESIAN_POINT ( 'NONE',  ( 17.50000000000000000, -5.499999999999992895, 56.21769037696436300 ) ) ;
#8697=CARTESIAN_POINT ( 'NONE',  ( 8.314922557961029526, -14.29746914071037800, 105.4177570613523613 ) ) ;
#8698=CARTESIAN_POINT ( 'NONE',  ( 5.049401038298161559, -19.05341960407611168, 57.70724293864769550 ) ) ;
#8699=CARTESIAN_POINT ( 'NONE',  ( 19.03943276465977164, 0.05219959533936151252, 26.25109039468566507 ) ) ;
#8700=CARTESIAN_POINT ( 'NONE',  ( -8.314922557961024197, 14.29746914071037800, 27.91775706135234358 ) ) ;
#8701=CARTESIAN_POINT ( 'NONE',  ( -21.53943276465977519, 0.05219959533907696930, 51.24890960531436690 ) ) ;
#8702=CARTESIAN_POINT ( 'NONE',  ( -5.823673210054431948, 21.52544592524334988, 107.7094237280190328 ) ) ;
#8704=CARTESIAN_POINT ( 'NONE',  ( 16.51473224551069308, 9.474510206698969483, 64.16557627198102409 ) ) ;
#8705=CARTESIAN_POINT ( 'NONE',  ( 0.05219959533909260263, 19.03943276465977164, 104.9989096053143669 ) ) ;
#8706=CARTESIAN_POINT ( 'NONE',  ( 19.03943276465977164, -0.05219959533909143690, 98.74890960531436690 ) ) ;
#8708=CARTESIAN_POINT ( 'NONE',  ( -15.80617190586768217, 15.72974639402176855, 23.12609039468567573 ) ) ;
#8709=AXIS2_PLACEMENT_3D ( 'NONE', #11039, #179908, #106016 ) ;
#8710=CARTESIAN_POINT ( 'NONE',  ( -14.29746914071049879, 8.314922557960819915, 95.83224293864770971 ) ) ;
#8711=CARTESIAN_POINT ( 'NONE',  ( -21.52544592524343514, 5.823673210054127303, 86.04057627198102409 ) ) ;
#8712=CARTESIAN_POINT ( 'NONE',  ( -0.05219959533909027116, -19.03943276465977164, 62.49890960531435979 ) ) ;
#8713=CARTESIAN_POINT ( 'NONE',  ( -13.89961937509977652, 13.97604488694528158, 70.62390960531432427 ) ) ;
#8714=CARTESIAN_POINT ( 'NONE',  ( -5.719274019375978568, 21.55341960407610458, 110.2072429386477239 ) ) ;
#8715=ORIENTED_EDGE ( 'NONE', *, *, #22998, .F. ) ;
#8716=CARTESIAN_POINT ( 'NONE',  ( 19.03943276465977164, -0.05219959533909143690, 73.74890960531435269 ) ) ;
#8717=CARTESIAN_POINT ( 'NONE',  ( 19.02130022317637525, -5.499999999999793943, 98.28188669246577547 ) ) ;
#8718=CARTESIAN_POINT ( 'NONE',  ( -16.52544592524342804, 4.483927247898546575, 111.0405762719810525 ) ) ;
#8720=CARTESIAN_POINT ( 'NONE',  ( 5.153800228976335163, 19.02544592524342804, 69.79057627198103830 ) ) ;
#8721=CARTESIAN_POINT ( 'NONE',  ( 5.049401038297881783, 19.05341960407617563, 92.29275706135234714 ) ) ;
#8722=CARTESIAN_POINT ( 'NONE',  ( -8.224510206698948167, 14.34966873604960824, 100.4155762719810241 ) ) ;
#8723=CARTESIAN_POINT ( 'NONE',  ( -18.62759615963255300, -10.81492255796106328, 69.16775706135234714 ) ) ;
#8724=CARTESIAN_POINT ( 'NONE',  ( 19.05341960407611168, 5.049401038298154454, 43.95724293864769550 ) ) ;
#8725=CARTESIAN_POINT ( 'NONE',  ( -5.823673210054431948, 21.52544592524334988, 27.70942372801901854 ) ) ;
#8726=CARTESIAN_POINT ( 'NONE',  ( -21.52544592524343514, 5.823673210054127303, 111.0405762719810525 ) ) ;
#8728=CARTESIAN_POINT ( 'NONE',  ( 13.89961937509977652, -13.97604488694527269, 73.12390960531436690 ) ) ;
#8730=CARTESIAN_POINT ( 'NONE',  ( -9.474510206698720793, -16.51473224551083518, 104.5844237280190043 ) ) ;
#8731=CARTESIAN_POINT ( 'NONE',  ( 18.67979575497178502, 10.72451020669898547, 34.16557627198102409 ) ) ;
#8732=CARTESIAN_POINT ( 'NONE',  ( -10.72451020669870658, -18.67979575497194134, 69.58442372801900433 ) ) ;
#8733=CARTESIAN_POINT ( 'NONE',  ( -19.05341960407611168, -5.049401038298163336, 91.45724293864766707 ) ) ;
#8734=CARTESIAN_POINT ( 'NONE',  ( -16.51473224551082808, 9.474510206698731452, 78.33442372801900433 ) ) ;
#8735=CARTESIAN_POINT ( 'NONE',  ( 9.474510206698971260, -16.51473224551069308, 42.91557627198103120 ) ) ;
#8736=CARTESIAN_POINT ( 'NONE',  ( 16.46253265017160672, -9.564922557960803928, 68.33224293864770971 ) ) ;
#8737=CARTESIAN_POINT ( 'NONE',  ( 14.29746914071049879, -8.314922557960816363, 98.33224293864769550 ) ) ;
#8738=CARTESIAN_POINT ( 'NONE',  ( 9.564922557960805705, 16.46253265017160317, 104.5822429386476955 ) ) ;
#8739=CARTESIAN_POINT ( 'NONE',  ( -8.314922557960811034, -14.29746914071050412, 87.08224293864769550 ) ) ;
#8740=CARTESIAN_POINT ( 'NONE',  ( 16.51473224551069308, 9.474510206698969483, 94.16557627198103830 ) ) ;
#8741=CARTESIAN_POINT ( 'NONE',  ( 8.224510206698953496, -14.34966873604960469, 37.91557627198102409 ) ) ;
#8742=CARTESIAN_POINT ( 'NONE',  ( -5.049401038298153566, 19.05341960407611168, 25.20724293864768484 ) ) ;
#8743=VERTEX_POINT ( 'NONE', #105828 ) ;
#8744=CARTESIAN_POINT ( 'NONE',  ( -15.72974639402176322, -15.80617190586768395, 64.37609039468568994 ) ) ;
#8745=CARTESIAN_POINT ( 'NONE',  ( 16.51473224551083163, -9.474510206698727899, 80.83442372801899012 ) ) ;
#8746=CARTESIAN_POINT ( 'NONE',  ( 4.483927247898545687, 16.52544592524342804, 44.79057627198103120 ) ) ;
#8747=CARTESIAN_POINT ( 'NONE',  ( -5.719274019375978568, 21.55341960407610458, 95.20724293864769550 ) ) ;
#8748=CARTESIAN_POINT ( 'NONE',  ( 15.72974639402199770, -15.80617190586745480, 28.12390960531435979 ) ) ;
#8749=CARTESIAN_POINT ( 'NONE',  ( -4.483927247898539470, -16.52544592524342804, 77.29057627198102409 ) ) ;
#8750=CARTESIAN_POINT ( 'NONE',  ( 5.049401038298161559, -19.05341960407611168, 57.70724293864769550 ) ) ;
#8751=CARTESIAN_POINT ( 'NONE',  ( -0.05219959533910754901, -16.53943276465976808, 22.49890960531436335 ) ) ;
#8752=CARTESIAN_POINT ( 'NONE',  ( -16.55341960407617563, 4.379528057220093196, 98.54275706135234714 ) ) ;
#8753=CARTESIAN_POINT ( 'NONE',  ( 14.29746914071037800, 8.314922557961029526, 71.66775706135234714 ) ) ;
#8754=CARTESIAN_POINT ( 'NONE',  ( 16.46253265017146816, 9.564922557961045513, 31.66775706135232937 ) ) ;
#8755=CARTESIAN_POINT ( 'NONE',  ( 13.89961937509977652, -13.97604488694527269, 103.1239096053143527 ) ) ;
#8756=CARTESIAN_POINT ( 'NONE',  ( -5.049401038298153566, 19.05341960407611168, 80.20724293864769550 ) ) ;
#8757=CARTESIAN_POINT ( 'NONE',  ( -19.05341960407611168, -5.049401038298163336, 31.45724293864769550 ) ) ;
#8758=ADVANCED_FACE ( 'NONE', ( #117005 ), #40162, .F. ) ;
#8759=CARTESIAN_POINT ( 'NONE',  ( -12.06949235617756955, 12.14591786802309770, 50.62390960531435979 ) ) ;
#8761=CARTESIAN_POINT ( 'NONE',  ( -13.89961937509977652, 13.97604488694528158, 105.6239096053143527 ) ) ;
#8762=CARTESIAN_POINT ( 'NONE',  ( 15.80617190586746368, 15.72974639402197994, 39.37390960531436690 ) ) ;
#8763=CARTESIAN_POINT ( 'NONE',  ( 14.34966873604960469, 8.224510206698951720, 79.16557627198103830 ) ) ;
#8764=CARTESIAN_POINT ( 'NONE',  ( 12.14591786802327356, -12.06949235617739191, 25.62609039468567929 ) ) ;
#8765=CARTESIAN_POINT ( 'NONE',  ( 12.06949235617757843, -12.14591786802309237, 68.12390960531436690 ) ) ;
#8767=CARTESIAN_POINT ( 'NONE',  ( -13.89961937509957401, -13.97604488694547875, 59.37609039468566863 ) ) ;
#8768=CARTESIAN_POINT ( 'NONE',  ( -19.02544592524342804, 5.153800228976336051, 106.0405762719810241 ) ) ;
#8769=CARTESIAN_POINT ( 'NONE',  ( -5.049401038297874678, -19.05341960407617918, 79.79275706135233293 ) ) ;
#8771=CARTESIAN_POINT ( 'NONE',  ( 0.05219959533936267826, -19.03943276465977164, 110.0010903946856757 ) ) ;
#8772=CARTESIAN_POINT ( 'NONE',  ( 12.06949235617739724, 12.14591786802326823, 106.8760903946856899 ) ) ;
#8773=CARTESIAN_POINT ( 'NONE',  ( 16.46253265017160672, -9.564922557960803928, 38.33224293864768839 ) ) ;
#8774=CARTESIAN_POINT ( 'NONE',  ( -21.55341960407610458, -5.719274019375992779, 36.45724293864768839 ) ) ;
#8775=CARTESIAN_POINT ( 'NONE',  ( 0.05219959533937995610, -21.53943276465977519, 55.00109039468568284 ) ) ;
#8777=CARTESIAN_POINT ( 'NONE',  ( 14.34966873604972726, -8.224510206698740333, 25.83442372801901499 ) ) ;
#8779=CARTESIAN_POINT ( 'NONE',  ( -9.474510206698964154, 16.51473224551069663, 75.41557627198103830 ) ) ;
#8781=CARTESIAN_POINT ( 'NONE',  ( 8.314922557960818139, 14.29746914071049879, 89.58224293864768129 ) ) ;
#8782=CARTESIAN_POINT ( 'NONE',  ( -5.153800228976328057, -19.02544592524343514, 72.29057627198102409 ) ) ;
#8783=CARTESIAN_POINT ( 'NONE',  ( -16.51473224551069308, -9.474510206698971260, 91.66557627198103830 ) ) ;
#8784=ORIENTED_EDGE ( 'NONE', *, *, #41117, .T. ) ;
#8785=CARTESIAN_POINT ( 'NONE',  ( -5.049401038297874678, -19.05341960407617918, 89.79275706135230450 ) ) ;
#8786=CARTESIAN_POINT ( 'NONE',  ( 0.05219959533907565091, 21.53943276465977519, 79.99890960531435269 ) ) ;
#8787=CARTESIAN_POINT ( 'NONE',  ( 5.153800228976335163, 19.02544592524342804, 34.79057627198102409 ) ) ;
#8788=CARTESIAN_POINT ( 'NONE',  ( -16.46253265017146816, -9.564922557961047289, 54.16775706135234003 ) ) ;
#8789=CARTESIAN_POINT ( 'NONE',  ( -5.153800228976328057, -19.02544592524343514, 52.29057627198100988 ) ) ;
#8790=CARTESIAN_POINT ( 'NONE',  ( -0.05219959533909027116, -19.03943276465977164, 92.49890960531436690 ) ) ;
#8792=CARTESIAN_POINT ( 'NONE',  ( 18.67979575497178502, 10.72451020669898547, 99.16557627198100988 ) ) ;
#8793=CARTESIAN_POINT ( 'NONE',  ( -8.224510206698948167, 14.34966873604960824, 95.41557627198102409 ) ) ;
#8794=CARTESIAN_POINT ( 'NONE',  ( 19.03943276465977164, -0.05219959533909143690, 83.74890960531436690 ) ) ;
#8795=CARTESIAN_POINT ( 'NONE',  ( 13.97604488694548053, -13.89961937509957401, 60.62609039468564731 ) ) ;
#8796=CARTESIAN_POINT ( 'NONE',  ( 5.823673210054125526, 21.52544592524343514, 84.79057627198102409 ) ) ;
#8797=CARTESIAN_POINT ( 'NONE',  ( 21.52544592524344225, -5.823673210054117533, 73.54057627198102409 ) ) ;
#8798=CARTESIAN_POINT ( 'NONE',  ( -4.483927247898539470, -16.52544592524342804, 32.29057627198102409 ) ) ;
#8799=CARTESIAN_POINT ( 'NONE',  ( -18.67979575497193778, 10.72451020669871902, 98.33442372801901854 ) ) ;
#8800=CARTESIAN_POINT ( 'NONE',  ( -14.34966873604972548, 8.224510206698743886, 63.33442372801900433 ) ) ;
#8801=CARTESIAN_POINT ( 'NONE',  ( 0.05219959533909260263, 19.03943276465977164, 84.99890960531436690 ) ) ;
#8802=CARTESIAN_POINT ( 'NONE',  ( 16.51473224551069308, 9.474510206698969483, 29.16557627198103475 ) ) ;
#8804=CARTESIAN_POINT ( 'NONE',  ( -18.62759615963255300, -10.81492255796106328, 34.16775706135234714 ) ) ;
#8805=CARTESIAN_POINT ( 'NONE',  ( -21.55341960407619339, 5.719274019375674811, 53.54275706135234714 ) ) ;
#8806=CARTESIAN_POINT ( 'NONE',  ( 16.51473224551069308, 9.474510206698969483, 49.16557627198102409 ) ) ;
#8807=CARTESIAN_POINT ( 'NONE',  ( 21.52544592524334988, 5.823673210054432836, 21.45942372801901499 ) ) ;
#8808=CARTESIAN_POINT ( 'NONE',  ( 16.51473224551083163, -9.474510206698727899, 70.83442372801900433 ) ) ;
#8809=CARTESIAN_POINT ( 'NONE',  ( -13.97604488694547697, 13.89961937509957934, 78.12609039468567573 ) ) ;
#8810=CARTESIAN_POINT ( 'NONE',  ( -16.51473224551069308, -9.474510206698971260, 31.66557627198102054 ) ) ;
#8811=CARTESIAN_POINT ( 'NONE',  ( -14.34966873604972548, 8.224510206698743886, 68.33442372801900433 ) ) ;
#8812=CARTESIAN_POINT ( 'NONE',  ( -9.564922557960796823, -16.46253265017161027, 57.08224293864769550 ) ) ;
#8813=CARTESIAN_POINT ( 'NONE',  ( -5.153800228976328057, -19.02544592524343514, 97.29057627198099567 ) ) ;
#8814=CARTESIAN_POINT ( 'NONE',  ( 0.05219959533909260263, 19.03943276465977164, 39.99890960531436690 ) ) ;
#8815=CARTESIAN_POINT ( 'NONE',  ( -5.719274019375978568, 21.55341960407610458, 75.20724293864769550 ) ) ;
#8816=CARTESIAN_POINT ( 'NONE',  ( -16.53943276465976808, -0.05219959533934237506, 58.75109039468568994 ) ) ;
#8818=CARTESIAN_POINT ( 'NONE',  ( 10.81492255796106328, -18.62759615963255655, 110.4177570613523756 ) ) ;
#8819=CARTESIAN_POINT ( 'NONE',  ( -19.05341960407611168, -5.049401038298163336, 56.45724293864768129 ) ) ;
#8820=CARTESIAN_POINT ( 'NONE',  ( 12.14591786802309770, 12.06949235617756955, 39.37390960531436690 ) ) ;
#8821=CARTESIAN_POINT ( 'NONE',  ( -4.483927247898539470, -16.52544592524342804, 72.29057627198102409 ) ) ;
#8822=CARTESIAN_POINT ( 'NONE',  ( -13.97604488694527625, -13.89961937509977652, 76.87390960531433848 ) ) ;
#8823=CARTESIAN_POINT ( 'NONE',  ( 15.72974639402176855, 15.80617190586768217, 36.87609039468568994 ) ) ;
#8824=CARTESIAN_POINT ( 'NONE',  ( 9.474510206698971260, -16.51473224551069308, 87.91557627198102409 ) ) ;
#8825=CARTESIAN_POINT ( 'NONE',  ( -15.80617190586768217, 15.72974639402176855, 103.1260903946856757 ) ) ;
#8826=CARTESIAN_POINT ( 'NONE',  ( 4.379528057220092307, 16.55341960407617563, 72.29275706135236135 ) ) ;
#8827=CARTESIAN_POINT ( 'NONE',  ( 19.02544592524343514, -5.153800228976328945, 108.5405762719810383 ) ) ;
#8829=CARTESIAN_POINT ( 'NONE',  ( 18.62759615963271287, -10.81492255796078972, 88.33224293864769550 ) ) ;
#8830=CARTESIAN_POINT ( 'NONE',  ( 4.483927247898545687, 16.52544592524342804, 49.79057627198102409 ) ) ;
#8831=CARTESIAN_POINT ( 'NONE',  ( 9.564922557960805705, 16.46253265017160317, 44.58224293864769550 ) ) ;
#8832=CARTESIAN_POINT ( 'NONE',  ( 16.52544592524335698, 4.483927247898782831, 56.45942372801902565 ) ) ;
#8833=CARTESIAN_POINT ( 'NONE',  ( 4.483927247898545687, 16.52544592524342804, 69.79057627198102409 ) ) ;
#8834=CARTESIAN_POINT ( 'NONE',  ( -0.05219959533909027116, -19.03943276465977164, 112.4989096053143669 ) ) ;
#8835=CARTESIAN_POINT ( 'NONE',  ( 21.53943276465977519, -0.05219959533907433946, 33.74890960531436690 ) ) ;
#8836=CARTESIAN_POINT ( 'NONE',  ( 9.564922557961047289, -16.46253265017146816, 35.41775706135233293 ) ) ;
#8837=CARTESIAN_POINT ( 'NONE',  ( 4.483927247898545687, 16.52544592524342804, 104.7905762719810241 ) ) ;
#8838=CARTESIAN_POINT ( 'NONE',  ( 5.153800228976335163, 19.02544592524342804, 114.7905762719810241 ) ) ;
#8840=CARTESIAN_POINT ( 'NONE',  ( 14.34966873604972726, -8.224510206698740333, 55.83442372801901854 ) ) ;
#8841=CARTESIAN_POINT ( 'NONE',  ( -16.51473224551069308, -9.474510206698971260, 61.66557627198103120 ) ) ;
#8842=CARTESIAN_POINT ( 'NONE',  ( -16.68133157960667035, -6.285544323925044807, 20.58868060224343211 ) ) ;
#8843=CARTESIAN_POINT ( 'NONE',  ( -16.46253265017146816, -9.564922557961047289, 54.16775706135234003 ) ) ;
#8844=CARTESIAN_POINT ( 'NONE',  ( -8.224510206698735004, -14.34966873604973081, 99.58442372801900433 ) ) ;
#8845=CARTESIAN_POINT ( 'NONE',  ( 13.89961937509957401, 13.97604488694547697, 96.87609039468566152 ) ) ;
#8846=CARTESIAN_POINT ( 'NONE',  ( -5.823673210054431948, 21.52544592524334988, 72.70942372801901854 ) ) ;
#8847=CARTESIAN_POINT ( 'NONE',  ( -19.02544592524342804, 5.153800228976336051, 71.04057627198099567 ) ) ;
#8848=CARTESIAN_POINT ( 'NONE',  ( -21.55341960407610458, -5.719274019375992779, 96.45724293864770971 ) ) ;
#8849=CARTESIAN_POINT ( 'NONE',  ( -16.52544592524342804, 4.483927247898546575, 111.0405762719810525 ) ) ;
#8851=CARTESIAN_POINT ( 'NONE',  ( -19.03943276465977164, -0.05219959533935918106, 83.75109039468567573 ) ) ;
#8852=CARTESIAN_POINT ( 'NONE',  ( 15.80617190586746368, 15.72974639402197994, 74.37390960531436690 ) ) ;
#8853=CARTESIAN_POINT ( 'NONE',  ( -9.474510206698720793, -16.51473224551083518, 39.58442372801899722 ) ) ;
#8854=FACE_BOUND ( 'NONE', #86092, .T. ) ;
#8855=CARTESIAN_POINT ( 'NONE',  ( 5.719274019375991003, -21.55341960407610458, 87.70724293864769550 ) ) ;
#8856=CARTESIAN_POINT ( 'NONE',  ( -18.56197773271732387, 5.499999999999902300, 53.55066217314453780 ) ) ;
#8857=CARTESIAN_POINT ( 'NONE',  ( -0.05219959533909027116, -19.03943276465977164, 67.49890960531436690 ) ) ;
#8859=CARTESIAN_POINT ( 'NONE',  ( -16.52544592524335698, -4.483927247898792601, 18.95942372801901143 ) ) ;
#8861=CARTESIAN_POINT ( 'NONE',  ( 5.153800228976335163, 19.02544592524342804, 49.79057627198100988 ) ) ;
#8862=CARTESIAN_POINT ( 'NONE',  ( -16.51473224551069308, -9.474510206698971260, 111.6655762719810383 ) ) ;
#8863=CARTESIAN_POINT ( 'NONE',  ( 5.719274019375991003, -21.55341960407610458, 102.7072429386476955 ) ) ;
#8864=CARTESIAN_POINT ( 'NONE',  ( -14.29746914071049879, 8.314922557960819915, 45.83224293864769550 ) ) ;
#8865=CARTESIAN_POINT ( 'NONE',  ( 18.62759615963255655, 10.81492255796105972, 76.66775706135234714 ) ) ;
#8866=CARTESIAN_POINT ( 'NONE',  ( -16.53943276465976808, -0.05219959533934237506, 28.75109039468567929 ) ) ;
#8867=CARTESIAN_POINT ( 'NONE',  ( -0.05219959533936034679, 19.03943276465977164, 27.50109039468566507 ) ) ;
#8868=CARTESIAN_POINT ( 'NONE',  ( -8.224510206698948167, 14.34966873604960824, 30.41557627198101699 ) ) ;
#8869=CARTESIAN_POINT ( 'NONE',  ( -15.80617190586768217, 15.72974639402176855, 33.12609039468569705 ) ) ;
#8870=CARTESIAN_POINT ( 'NONE',  ( 18.62759615963271287, -10.81492255796078972, 113.3322429386476955 ) ) ;
#8871=CARTESIAN_POINT ( 'NONE',  ( 14.29746914071049879, -8.314922557960816363, 43.33224293864769550 ) ) ;
#8872=CARTESIAN_POINT ( 'NONE',  ( 13.89961937509957401, 13.97604488694547697, 101.8760903946856331 ) ) ;
#8873=CARTESIAN_POINT ( 'NONE',  ( -19.02544592524334988, -5.153800228976617603, 73.95942372801900433 ) ) ;
#8874=CARTESIAN_POINT ( 'NONE',  ( -21.52544592524334988, -5.823673210054445271, 73.95942372801901854 ) ) ;
#8875=CARTESIAN_POINT ( 'NONE',  ( 16.51473224551083163, -9.474510206698727899, 55.83442372801899722 ) ) ;
#8876=CARTESIAN_POINT ( 'NONE',  ( 19.03943276465977164, -0.05219959533909143690, 28.74890960531435624 ) ) ;
#8877=CARTESIAN_POINT ( 'NONE',  ( 21.52544592524344225, -5.823673210054117533, 48.54057627198103120 ) ) ;
#8878=CARTESIAN_POINT ( 'NONE',  ( -16.52544592524342804, 4.483927247898546575, 56.04057627198102409 ) ) ;
#8879=CARTESIAN_POINT ( 'NONE',  ( 17.50000000000002487, -5.499999999999880984, 53.29690382534172244 ) ) ;
#8880=CARTESIAN_POINT ( 'NONE',  ( 10.81492255796106328, -18.62759615963255655, 110.4177570613523756 ) ) ;
#8881=CARTESIAN_POINT ( 'NONE',  ( 12.06949235617739724, 12.14591786802326823, 81.87609039468568994 ) ) ;
#8882=CARTESIAN_POINT ( 'NONE',  ( -14.29746914071049879, 8.314922557960819915, 35.83224293864768839 ) ) ;
#8883=CARTESIAN_POINT ( 'NONE',  ( -10.72451020669870658, -18.67979575497194134, 69.58442372801900433 ) ) ;
#8884=CARTESIAN_POINT ( 'NONE',  ( 5.719274019375673035, 21.55341960407619339, 87.29275706135236135 ) ) ;
#8885=CARTESIAN_POINT ( 'NONE',  ( 10.81492255796078972, 18.62759615963270932, 79.58224293864769550 ) ) ;
#8886=CARTESIAN_POINT ( 'NONE',  ( -13.97604488694527625, -13.89961937509977652, 31.87390960531435979 ) ) ;
#8887=CARTESIAN_POINT ( 'NONE',  ( -15.80617190586768217, 15.72974639402176855, 63.12609039468568994 ) ) ;
#8888=CARTESIAN_POINT ( 'NONE',  ( -16.51473224551069308, -9.474510206698971260, 36.66557627198102409 ) ) ;
#8889=CARTESIAN_POINT ( 'NONE',  ( 16.46253265017160672, -9.564922557960803928, 53.33224293864768839 ) ) ;
#8890=CARTESIAN_POINT ( 'NONE',  ( -14.34966873604960291, -8.224510206698953496, 86.66557627198102409 ) ) ;
#8891=CARTESIAN_POINT ( 'NONE',  ( 5.153800228976335163, 19.02544592524342804, 94.79057627198103830 ) ) ;
#8892=CARTESIAN_POINT ( 'NONE',  ( 16.53943276465976808, -0.05219959533910856209, 43.74890960531435979 ) ) ;
#8893=CARTESIAN_POINT ( 'NONE',  ( -4.379528057220328563, 16.55341960407611168, 115.2072429386476955 ) ) ;
#8894=CARTESIAN_POINT ( 'NONE',  ( -21.52544592524343514, 5.823673210054127303, 86.04057627198102409 ) ) ;
#8895=CARTESIAN_POINT ( 'NONE',  ( -18.62759615963270932, 10.81492255796079327, 115.8322429386477097 ) ) ;
#8897=CARTESIAN_POINT ( 'NONE',  ( -9.474510206698964154, 16.51473224551069663, 80.41557627198103830 ) ) ;
#8898=CARTESIAN_POINT ( 'NONE',  ( 16.55341960407618274, -4.379528057220086978, 21.04275706135234714 ) ) ;
#8899=CARTESIAN_POINT ( 'NONE',  ( -21.53943276465977519, 0.05219959533907696930, 76.24890960531435269 ) ) ;
#8900=CARTESIAN_POINT ( 'NONE',  ( -10.72451020669870658, -18.67979575497194134, 99.58442372801900433 ) ) ;
#8901=CARTESIAN_POINT ( 'NONE',  ( -5.153800228976328057, -19.02544592524343514, 77.29057627198099567 ) ) ;
#8902=CARTESIAN_POINT ( 'NONE',  ( 10.72451020669871369, 18.67979575497193778, 37.08442372801901143 ) ) ;
#8903=CARTESIAN_POINT ( 'NONE',  ( 5.049401038298161559, -19.05341960407611168, 107.7072429386476955 ) ) ;
#8904=CARTESIAN_POINT ( 'NONE',  ( 12.06949235617739724, 12.14591786802326823, 96.87609039468568994 ) ) ;
#8905=CARTESIAN_POINT ( 'NONE',  ( -18.62759615963255300, -10.81492255796106328, 74.16775706135231871 ) ) ;
#8906=CARTESIAN_POINT ( 'NONE',  ( -15.72974639402176322, -15.80617190586768395, 109.3760903946857042 ) ) ;
#8907=CARTESIAN_POINT ( 'NONE',  ( 14.34966873604972726, -8.224510206698740333, 75.83442372801900433 ) ) ;
#8908=CARTESIAN_POINT ( 'NONE',  ( 0.05219959533937995610, -21.53943276465977519, 25.00109039468567218 ) ) ;
#8909=CARTESIAN_POINT ( 'NONE',  ( -5.049401038298153566, 19.05341960407611168, 25.20724293864768484 ) ) ;
#8910=CARTESIAN_POINT ( 'NONE',  ( 18.62759615963255655, 10.81492255796105972, 86.66775706135234714 ) ) ;
#8911=CARTESIAN_POINT ( 'NONE',  ( -13.89961937509977652, 13.97604488694528158, 90.62390960531432427 ) ) ;
#8912=CARTESIAN_POINT ( 'NONE',  ( 10.81492255796078972, 18.62759615963270932, 89.58224293864768129 ) ) ;
#8913=CARTESIAN_POINT ( 'NONE',  ( 13.89961937509957401, 13.97604488694547697, 61.87609039468566863 ) ) ;
#8915=CARTESIAN_POINT ( 'NONE',  ( -5.719274019375978568, 21.55341960407610458, 55.20724293864770260 ) ) ;
#8916=CARTESIAN_POINT ( 'NONE',  ( 0.05219959533909260263, 19.03943276465977164, 89.99890960531436690 ) ) ;
#8917=CARTESIAN_POINT ( 'NONE',  ( -16.55341960407611168, -4.379528057220339221, 56.45724293864768839 ) ) ;
#8919=CARTESIAN_POINT ( 'NONE',  ( -19.03943276465977164, -0.05219959533935918106, 83.75109039468567573 ) ) ;
#8920=CARTESIAN_POINT ( 'NONE',  ( -17.49999999999999645, 5.499999999999997335, 105.7969038253417153 ) ) ;
#8922=CARTESIAN_POINT ( 'NONE',  ( -5.153800228976607833, 19.02544592524334988, 112.7094237280190043 ) ) ;
#8923=CARTESIAN_POINT ( 'NONE',  ( -18.62759615963270932, 10.81492255796079327, 80.83224293864769550 ) ) ;
#8924=CARTESIAN_POINT ( 'NONE',  ( -12.06949235617756955, 12.14591786802309770, 65.62390960531436690 ) ) ;
#8925=CARTESIAN_POINT ( 'NONE',  ( -19.02544592524342804, 5.153800228976336051, 101.0405762719810241 ) ) ;
#8926=CARTESIAN_POINT ( 'NONE',  ( -0.05219959533934338120, 16.53943276465976808, 47.50109039468568994 ) ) ;
#8927=CARTESIAN_POINT ( 'NONE',  ( -9.474510206698964154, 16.51473224551069663, 60.41557627198102409 ) ) ;
#8928=CARTESIAN_POINT ( 'NONE',  ( 21.52544592524344225, -5.823673210054117533, 113.5405762719810383 ) ) ;
#8929=CARTESIAN_POINT ( 'NONE',  ( -16.51473224551082808, 9.474510206698731452, 103.3344237280190043 ) ) ;
#8930=CARTESIAN_POINT ( 'NONE',  ( 9.564922557960805705, 16.46253265017160317, 99.58224293864770971 ) ) ;
#8931=CARTESIAN_POINT ( 'NONE',  ( 13.89961937509977652, -13.97604488694527269, 73.12390960531436690 ) ) ;
#8932=CARTESIAN_POINT ( 'NONE',  ( -10.81492255796078084, -18.62759615963271287, 72.08224293864769550 ) ) ;
#8933=CARTESIAN_POINT ( 'NONE',  ( 5.153800228976335163, 19.02544592524342804, 39.79057627198100988 ) ) ;
#8935=CARTESIAN_POINT ( 'NONE',  ( -4.483927247898539470, -16.52544592524342804, 57.29057627198103120 ) ) ;
#8936=CARTESIAN_POINT ( 'NONE',  ( -5.153800228976328057, -19.02544592524343514, 97.29057627198099567 ) ) ;
#8937=CARTESIAN_POINT ( 'NONE',  ( 17.50000000000000000, 5.499999999999992895, 38.78230962303566542 ) ) ;
#8938=CARTESIAN_POINT ( 'NONE',  ( -19.02544592524334988, -5.153800228976617603, 58.95942372801900433 ) ) ;
#8939=CARTESIAN_POINT ( 'NONE',  ( -10.81492255796078084, -18.62759615963271287, 97.08224293864770971 ) ) ;
#8940=CARTESIAN_POINT ( 'NONE',  ( -9.474510206698720793, -16.51473224551083518, 49.58442372801899722 ) ) ;
#8941=CARTESIAN_POINT ( 'NONE',  ( 0.05219959533909260263, 19.03943276465977164, 94.99890960531436690 ) ) ;
#8943=CARTESIAN_POINT ( 'NONE',  ( 15.72974639402199770, -15.80617190586745480, 48.12390960531436690 ) ) ;
#8945=CARTESIAN_POINT ( 'NONE',  ( 16.51473224551069308, 9.474510206698969483, 79.16557627198103830 ) ) ;
#8946=CARTESIAN_POINT ( 'NONE',  ( -21.52544592524334988, -5.823673210054445271, 58.95942372801902565 ) ) ;
#8947=CARTESIAN_POINT ( 'NONE',  ( -13.97604488694527625, -13.89961937509977652, 36.87390960531436690 ) ) ;
#8949=CARTESIAN_POINT ( 'NONE',  ( -14.29746914071049879, 8.314922557960819915, 75.83224293864769550 ) ) ;
#8951=CARTESIAN_POINT ( 'NONE',  ( -12.06949235617739369, -12.14591786802326823, 24.37609039468567573 ) ) ;
#8952=CARTESIAN_POINT ( 'NONE',  ( 10.72451020669871369, 18.67979575497193778, 52.08442372801901854 ) ) ;
#8953=EDGE_LOOP ( 'NONE', ( #122779, #89234, #12743, #137387 ) ) ;
#8954=CARTESIAN_POINT ( 'NONE',  ( 19.02544592524343514, -5.153800228976328945, 108.5405762719810383 ) ) ;
#8955=CARTESIAN_POINT ( 'NONE',  ( -9.564922557961040184, 16.46253265017147172, 62.91775706135233293 ) ) ;
#8957=CARTESIAN_POINT ( 'NONE',  ( -18.67979575497193778, 10.72451020669871902, 23.33442372801901499 ) ) ;
#8958=CARTESIAN_POINT ( 'NONE',  ( 13.89961937509977652, -13.97604488694527269, 58.12390960531436690 ) ) ;
#8960=CARTESIAN_POINT ( 'NONE',  ( -18.67979575497193778, 10.72451020669871902, 108.3344237280190185 ) ) ;
#8961=CARTESIAN_POINT ( 'NONE',  ( 16.51473224551069308, 9.474510206698969483, 44.16557627198103120 ) ) ;
#8962=CARTESIAN_POINT ( 'NONE',  ( -19.03943276465977164, -0.05219959533935918106, 18.75109039468567218 ) ) ;
#8963=CARTESIAN_POINT ( 'NONE',  ( -0.05219959533934338120, 16.53943276465976808, 87.50109039468568994 ) ) ;
#8964=CARTESIAN_POINT ( 'NONE',  ( 19.05341960407611168, 5.049401038298154454, 103.9572429386476671 ) ) ;
#8965=CARTESIAN_POINT ( 'NONE',  ( -21.52544592524334988, -5.823673210054445271, 68.95942372801901854 ) ) ;
#8967=CARTESIAN_POINT ( 'NONE',  ( -16.51473224551069308, -9.474510206698971260, 106.6655762719810383 ) ) ;
#8969=CARTESIAN_POINT ( 'NONE',  ( 0.05219959533934541429, -16.53943276465976808, 70.00109039468568994 ) ) ;
#8970=CARTESIAN_POINT ( 'NONE',  ( -15.72974639402176322, -15.80617190586768395, 69.37609039468567573 ) ) ;
#8971=CARTESIAN_POINT ( 'NONE',  ( 18.67979575497194134, -10.72451020669871369, 105.8344237280190328 ) ) ;
#8973=CARTESIAN_POINT ( 'NONE',  ( 16.55341960407618274, -4.379528057220086978, 41.04275706135236135 ) ) ;
#8974=CARTESIAN_POINT ( 'NONE',  ( -0.05219959533909027116, -19.03943276465977164, 87.49890960531436690 ) ) ;
#8975=CARTESIAN_POINT ( 'NONE',  ( -19.03943276465977164, 0.05219959533909376836, 111.2489096053143669 ) ) ;
#8978=CARTESIAN_POINT ( 'NONE',  ( 16.61371651742603461, 7.165104196376041124, 43.64584930007006136 ) ) ;
#8979=CARTESIAN_POINT ( 'NONE',  ( 0.05219959533909260263, 19.03943276465977164, 34.99890960531435979 ) ) ;
#8980=CARTESIAN_POINT ( 'NONE',  ( -18.67979575497178146, -10.72451020669898902, 46.66557627198102409 ) ) ;
#8981=CARTESIAN_POINT ( 'NONE',  ( -14.29746914071037622, -8.314922557961029526, 104.1677570613523471 ) ) ;
#8982=CARTESIAN_POINT ( 'NONE',  ( 12.06949235617757843, -12.14591786802309237, 88.12390960531436690 ) ) ;
#8983=CARTESIAN_POINT ( 'NONE',  ( 9.474510206698971260, -16.51473224551069308, 77.91557627198103830 ) ) ;
#8984=CARTESIAN_POINT ( 'NONE',  ( 15.80617190586769283, -15.72974639402175789, 100.6260903946857184 ) ) ;
#8985=CARTESIAN_POINT ( 'NONE',  ( -0.05219959533934338120, 16.53943276465976808, 22.50109039468567573 ) ) ;
#8986=CARTESIAN_POINT ( 'NONE',  ( -14.34966873604960291, -8.224510206698953496, 86.66557627198102409 ) ) ;
#8987=CARTESIAN_POINT ( 'NONE',  ( 15.80617190586769283, -15.72974639402175789, 35.62609039468568994 ) ) ;
#8988=CARTESIAN_POINT ( 'NONE',  ( 10.72451020669898902, -18.67979575497178502, 87.91557627198103830 ) ) ;
#8989=CARTESIAN_POINT ( 'NONE',  ( 13.89961937509957401, 13.97604488694547697, 46.87609039468565442 ) ) ;
#8991=CARTESIAN_POINT ( 'NONE',  ( -19.05341960407611168, -5.049401038298163336, 101.4572429386476955 ) ) ;
#8992=CARTESIAN_POINT ( 'NONE',  ( 8.224510206698953496, -14.34966873604960469, 62.91557627198102409 ) ) ;
#8993=CARTESIAN_POINT ( 'NONE',  ( -4.379528057220328563, 16.55341960407611168, 45.20724293864769550 ) ) ;
#8994=CARTESIAN_POINT ( 'NONE',  ( -16.52544592524335698, -4.483927247898792601, 103.9594237280190185 ) ) ;
#8995=CARTESIAN_POINT ( 'NONE',  ( -19.05341960407617563, 5.049401038297882671, 63.54275706135234003 ) ) ;
#8997=CARTESIAN_POINT ( 'NONE',  ( 16.46253265017160672, -9.564922557960803928, 113.3322429386476955 ) ) ;
#8998=EDGE_CURVE ( 'NONE', #133171, #50923, #118019, .T. ) ;
#8999=CARTESIAN_POINT ( 'NONE',  ( -4.483927247898539470, -16.52544592524342804, 87.29057627198103830 ) ) ;
#9001=CARTESIAN_POINT ( 'NONE',  ( -5.153800228976328057, -19.02544592524343514, 52.29057627198100988 ) ) ;
#9002=CARTESIAN_POINT ( 'NONE',  ( -10.72451020669898014, 18.67979575497178502, 45.41557627198103830 ) ) ;
#9003=CARTESIAN_POINT ( 'NONE',  ( -19.02544592524342804, 5.153800228976336051, 26.04057627198103120 ) ) ;
#9004=CARTESIAN_POINT ( 'NONE',  ( -8.224510206698735004, -14.34966873604973081, 84.58442372801903275 ) ) ;
#9005=CARTESIAN_POINT ( 'NONE',  ( -13.89961937509977652, 13.97604488694528158, 60.62390960531436690 ) ) ;
#9006=CARTESIAN_POINT ( 'NONE',  ( -5.153800228976607833, 19.02544592524334988, 42.70942372801901143 ) ) ;
#9007=CARTESIAN_POINT ( 'NONE',  ( 18.62759615963255655, 10.81492255796105972, 51.66775706135234714 ) ) ;
#9008=CARTESIAN_POINT ( 'NONE',  ( 5.719274019375991003, -21.55341960407610458, 32.70724293864770260 ) ) ;
#9009=CARTESIAN_POINT ( 'NONE',  ( -8.314922557960811034, -14.29746914071050412, 102.0822429386476955 ) ) ;
#9010=CARTESIAN_POINT ( 'NONE',  ( 16.46253265017146816, 9.564922557961045513, 86.66775706135233293 ) ) ;
#9013=CARTESIAN_POINT ( 'NONE',  ( 10.72451020669898902, -18.67979575497178502, 52.91557627198103830 ) ) ;
#9014=CARTESIAN_POINT ( 'NONE',  ( 13.89961937509977652, -13.97604488694527269, 23.12390960531436335 ) ) ;
#9015=CARTESIAN_POINT ( 'NONE',  ( -5.719274019375665041, -21.55341960407619695, 89.79275706135236135 ) ) ;
#9016=CARTESIAN_POINT ( 'NONE',  ( 4.379528057220339221, -16.55341960407611168, 52.70724293864769550 ) ) ;
#9017=CARTESIAN_POINT ( 'NONE',  ( 8.314922557961029526, -14.29746914071037800, 60.41775706135235424 ) ) ;
#9018=CARTESIAN_POINT ( 'NONE',  ( 14.29746914071049879, -8.314922557960816363, 58.33224293864768839 ) ) ;
#9019=CARTESIAN_POINT ( 'NONE',  ( -0.05219959533907301413, -21.53943276465977519, 77.49890960531433848 ) ) ;
#9020=CARTESIAN_POINT ( 'NONE',  ( -15.72974639402197994, 15.80617190586746368, 70.62390960531436690 ) ) ;
#9022=CARTESIAN_POINT ( 'NONE',  ( 10.72451020669898902, -18.67979575497178502, 22.91557627198102765 ) ) ;
#9023=CARTESIAN_POINT ( 'NONE',  ( -16.46253265017160317, 9.564922557960807481, 65.83224293864769550 ) ) ;
#9024=CARTESIAN_POINT ( 'NONE',  ( 5.153800228976335163, 19.02544592524342804, 29.79057627198102409 ) ) ;
#9025=CARTESIAN_POINT ( 'NONE',  ( -18.09805431107249873, 5.499999999999980460, 76.01606229291883210 ) ) ;
#9026=CARTESIAN_POINT ( 'NONE',  ( 8.224510206698742110, 14.34966873604972548, 82.08442372801901854 ) ) ;
#9027=CARTESIAN_POINT ( 'NONE',  ( 0.05219959533937995610, -21.53943276465977519, 20.00109039468568639 ) ) ;
#9028=CARTESIAN_POINT ( 'NONE',  ( -13.89961937509977652, 13.97604488694528158, 65.62390960531436690 ) ) ;
#9029=CARTESIAN_POINT ( 'NONE',  ( 18.67979575497194134, -10.72451020669871369, 55.83442372801901854 ) ) ;
#9030=CARTESIAN_POINT ( 'NONE',  ( -16.46253265017160317, 9.564922557960807481, 100.8322429386477097 ) ) ;
#9033=CARTESIAN_POINT ( 'NONE',  ( -18.62759615963255300, -10.81492255796106328, 44.16775706135234714 ) ) ;
#9034=CARTESIAN_POINT ( 'NONE',  ( -0.05219959533909027116, -19.03943276465977164, 27.49890960531435624 ) ) ;
#9035=CARTESIAN_POINT ( 'NONE',  ( -5.049401038298153566, 19.05341960407611168, 100.2072429386476955 ) ) ;
#9036=CARTESIAN_POINT ( 'NONE',  ( -13.89961937509957401, -13.97604488694547875, 49.37609039468567573 ) ) ;
#9037=CARTESIAN_POINT ( 'NONE',  ( -15.80617190586745835, -15.72974639402198527, 111.8739096053143669 ) ) ;
#9038=CARTESIAN_POINT ( 'NONE',  ( -19.03943276465977164, -0.05219959533935918106, 48.75109039468566863 ) ) ;
#9039=CARTESIAN_POINT ( 'NONE',  ( 13.89961937509957401, 13.97604488694547697, 46.87609039468565442 ) ) ;
#9040=CARTESIAN_POINT ( 'NONE',  ( -14.29746914071037622, -8.314922557961029526, 104.1677570613523471 ) ) ;
#9042=CARTESIAN_POINT ( 'NONE',  ( 19.03943276465977164, -0.05219959533909143690, 78.74890960531436690 ) ) ;
#9043=CARTESIAN_POINT ( 'NONE',  ( -10.72451020669870658, -18.67979575497194134, 84.58442372801903275 ) ) ;
#9044=CARTESIAN_POINT ( 'NONE',  ( 10.81492255796106328, -18.62759615963255655, 100.4177570613523471 ) ) ;
#9046=CARTESIAN_POINT ( 'NONE',  ( -13.97604488694527625, -13.89961937509977652, 96.87390960531433848 ) ) ;
#9047=CARTESIAN_POINT ( 'NONE',  ( 15.72974639402176855, 15.80617190586768217, 81.87609039468568994 ) ) ;
#9048=CARTESIAN_POINT ( 'NONE',  ( 16.46253265017146816, 9.564922557961045513, 111.6677570613523329 ) ) ;
#9049=CARTESIAN_POINT ( 'NONE',  ( -19.05341960407611168, -5.049401038298163336, 76.45724293864769550 ) ) ;
#9050=CARTESIAN_POINT ( 'NONE',  ( -13.97604488694527625, -13.89961937509977652, 111.8739096053143243 ) ) ;
#9051=CARTESIAN_POINT ( 'NONE',  ( 5.049401038298161559, -19.05341960407611168, 97.70724293864766707 ) ) ;
#9052=CARTESIAN_POINT ( 'NONE',  ( 16.46253265017146816, 9.564922557961045513, 86.66775706135233293 ) ) ;
#9053=CARTESIAN_POINT ( 'NONE',  ( 9.474510206698971260, -16.51473224551069308, 77.91557627198103830 ) ) ;
#9054=CARTESIAN_POINT ( 'NONE',  ( -16.46253265017160317, 9.564922557960807481, 60.83224293864769550 ) ) ;
#9055=CARTESIAN_POINT ( 'NONE',  ( -5.823673210054116645, -21.52544592524344225, 107.2905762719810525 ) ) ;
#9056=CARTESIAN_POINT ( 'NONE',  ( 4.483927247898790824, -16.52544592524335698, 105.2094237280190328 ) ) ;
#9058=CARTESIAN_POINT ( 'NONE',  ( -9.474510206698720793, -16.51473224551083518, 64.58442372801900433 ) ) ;
#9060=CARTESIAN_POINT ( 'NONE',  ( 13.89961937509977652, -13.97604488694527269, 93.12390960531436690 ) ) ;
#9061=CARTESIAN_POINT ( 'NONE',  ( -8.224510206698948167, 14.34966873604960824, 90.41557627198103830 ) ) ;
#9062=CARTESIAN_POINT ( 'NONE',  ( -0.05219959533909027116, -19.03943276465977164, 27.49890960531435624 ) ) ;
#9063=CARTESIAN_POINT ( 'NONE',  ( 10.72451020669898902, -18.67979575497178502, 32.91557627198102409 ) ) ;
#9064=CARTESIAN_POINT ( 'NONE',  ( 10.81492255796078972, 18.62759615963270932, 24.58224293864768839 ) ) ;
#9065=CARTESIAN_POINT ( 'NONE',  ( -16.55341960407611168, -4.379528057220339221, 86.45724293864770971 ) ) ;
#9067=CARTESIAN_POINT ( 'NONE',  ( -5.049401038297874678, -19.05341960407617918, 44.79275706135232582 ) ) ;
#9068=CARTESIAN_POINT ( 'NONE',  ( -0.05219959533934338120, 16.53943276465976808, 102.5010903946856899 ) ) ;
#9069=CARTESIAN_POINT ( 'NONE',  ( -19.02544592524342804, 5.153800228976336051, 91.04057627198100988 ) ) ;
#9070=CARTESIAN_POINT ( 'NONE',  ( 10.81492255796106328, -18.62759615963255655, 70.41775706135236135 ) ) ;
#9071=CARTESIAN_POINT ( 'NONE',  ( -21.55341960407610458, -5.719274019375992779, 41.45724293864769550 ) ) ;
#9072=CARTESIAN_POINT ( 'NONE',  ( 5.823673210054444382, -21.52544592524334988, 35.20942372801901854 ) ) ;
#9073=CARTESIAN_POINT ( 'NONE',  ( -10.72451020669898014, 18.67979575497178502, 80.41557627198103830 ) ) ;
#9074=CARTESIAN_POINT ( 'NONE',  ( -14.29746914071049879, 8.314922557960819915, 105.8322429386476955 ) ) ;
#9075=CARTESIAN_POINT ( 'NONE',  ( 0.05219959533936267826, -19.03943276465977164, 75.00109039468566152 ) ) ;
#9076=CARTESIAN_POINT ( 'NONE',  ( -13.89961937509977652, 13.97604488694528158, 45.62390960531433848 ) ) ;
#9077=CARTESIAN_POINT ( 'NONE',  ( 19.03943276465977164, -0.05219959533909143690, 98.74890960531436690 ) ) ;
#9078=CARTESIAN_POINT ( 'NONE',  ( -9.564922557960796823, -16.46253265017161027, 97.08224293864769550 ) ) ;
#9079=CARTESIAN_POINT ( 'NONE',  ( 9.474510206698971260, -16.51473224551069308, 22.91557627198102765 ) ) ;
#9080=CARTESIAN_POINT ( 'NONE',  ( -8.224510206698948167, 14.34966873604960824, 45.41557627198103830 ) ) ;
#9081=CARTESIAN_POINT ( 'NONE',  ( -8.314922557961024197, 14.29746914071037800, 37.91775706135235424 ) ) ;
#9082=CARTESIAN_POINT ( 'NONE',  ( 15.80617190586769283, -15.72974639402175789, 105.6260903946856899 ) ) ;
#9084=CARTESIAN_POINT ( 'NONE',  ( 18.22780087662123805, -5.499999999999976019, 73.51763182126894947 ) ) ;
#9085=CARTESIAN_POINT ( 'NONE',  ( -4.483927247898539470, -16.52544592524342804, 22.29057627198102765 ) ) ;
#9087=CARTESIAN_POINT ( 'NONE',  ( -18.67979575497193778, 10.72451020669871902, 38.33442372801900433 ) ) ;
#9088=CARTESIAN_POINT ( 'NONE',  ( -16.51473224551069308, -9.474510206698971260, 106.6655762719810383 ) ) ;
#9089=CARTESIAN_POINT ( 'NONE',  ( 8.314922557961029526, -14.29746914071037800, 105.4177570613523613 ) ) ;
#9090=CARTESIAN_POINT ( 'NONE',  ( 12.06949235617739724, 12.14591786802326823, 96.87609039468568994 ) ) ;
#9091=CARTESIAN_POINT ( 'NONE',  ( 16.52544592524335698, 4.483927247898782831, 31.45942372801901854 ) ) ;
#9093=CARTESIAN_POINT ( 'NONE',  ( 19.03943276465977164, -0.05219959533909143690, 48.74890960531435979 ) ) ;
#9094=CARTESIAN_POINT ( 'NONE',  ( -12.06949235617756955, 12.14591786802309770, 110.6239096053143669 ) ) ;
#9095=CARTESIAN_POINT ( 'NONE',  ( -15.72974639402176322, -15.80617190586768395, 19.37609039468568639 ) ) ;
#9096=CARTESIAN_POINT ( 'NONE',  ( -16.51473224551069308, -9.474510206698971260, 26.66557627198103120 ) ) ;
#9097=CARTESIAN_POINT ( 'NONE',  ( -19.03943276465977164, 0.05219959533909376836, 111.2489096053143669 ) ) ;
#9098=CARTESIAN_POINT ( 'NONE',  ( 0.05219959533937995610, -21.53943276465977519, 30.00109039468568284 ) ) ;
#9099=CARTESIAN_POINT ( 'NONE',  ( 19.05341960407611168, 5.049401038298154454, 28.95724293864769550 ) ) ;
#9100=CARTESIAN_POINT ( 'NONE',  ( -5.153800228976328057, -19.02544592524343514, 107.2905762719810383 ) ) ;
#9101=CARTESIAN_POINT ( 'NONE',  ( -17.05587630539787725, -6.762274262135647973, 34.25819690962688213 ) ) ;
#9102=CARTESIAN_POINT ( 'NONE',  ( -19.05341960407611168, -5.049401038298163336, 101.4572429386476955 ) ) ;
#9103=CARTESIAN_POINT ( 'NONE',  ( 21.53943276465977519, 0.05219959533937863772, 41.25109039468568284 ) ) ;
#9104=CARTESIAN_POINT ( 'NONE',  ( -4.379528057220328563, 16.55341960407611168, 90.20724293864770971 ) ) ;
#9105=CARTESIAN_POINT ( 'NONE',  ( 5.153800228976335163, 19.02544592524342804, 94.79057627198103830 ) ) ;
#9107=CARTESIAN_POINT ( 'NONE',  ( 14.34966873604972726, -8.224510206698740333, 70.83442372801901854 ) ) ;
#9108=CARTESIAN_POINT ( 'NONE',  ( 0.05219959533937995610, -21.53943276465977519, 85.00109039468568994 ) ) ;
#9110=CARTESIAN_POINT ( 'NONE',  ( -8.314922557961024197, 14.29746914071037800, 37.91775706135235424 ) ) ;
#9111=CARTESIAN_POINT ( 'NONE',  ( -9.564922557960796823, -16.46253265017161027, 82.08224293864768129 ) ) ;
#9112=CARTESIAN_POINT ( 'NONE',  ( -13.89961937509957401, -13.97604488694547875, 109.3760903946856331 ) ) ;
#9113=CARTESIAN_POINT ( 'NONE',  ( -8.314922557961024197, 14.29746914071037800, 67.91775706135234714 ) ) ;
#9114=CARTESIAN_POINT ( 'NONE',  ( 19.05341960407617918, -5.049401038297876454, 96.04275706135231871 ) ) ;
#9115=CARTESIAN_POINT ( 'NONE',  ( -5.049401038298153566, 19.05341960407611168, 70.20724293864769550 ) ) ;
#9116=CARTESIAN_POINT ( 'NONE',  ( -10.81492255796078084, -18.62759615963271287, 87.08224293864769550 ) ) ;
#9117=CARTESIAN_POINT ( 'NONE',  ( -16.55341960407611168, -4.379528057220339221, 96.45724293864770971 ) ) ;
#9118=CARTESIAN_POINT ( 'NONE',  ( 13.97604488694548053, -13.89961937509957401, 85.62609039468568994 ) ) ;
#9119=CARTESIAN_POINT ( 'NONE',  ( -16.52544592524335698, -4.483927247898792601, 53.95942372801900433 ) ) ;
#9122=CARTESIAN_POINT ( 'NONE',  ( -9.564922557961040184, 16.46253265017147172, 62.91775706135233293 ) ) ;
#9123=CARTESIAN_POINT ( 'NONE',  ( 4.483927247898545687, 16.52544592524342804, 29.79057627198102409 ) ) ;
#9124=CARTESIAN_POINT ( 'NONE',  ( -8.224510206698948167, 14.34966873604960824, 75.41557627198102409 ) ) ;
#9125=CARTESIAN_POINT ( 'NONE',  ( -9.474510206698720793, -16.51473224551083518, 19.58442372801899722 ) ) ;
#9126=CARTESIAN_POINT ( 'NONE',  ( -16.36317988757094710, 7.306389748694859243, 39.09789608363175972 ) ) ;
#9127=CARTESIAN_POINT ( 'NONE',  ( -18.67979575497193778, 10.72451020669871902, 23.33442372801901499 ) ) ;
#9128=CARTESIAN_POINT ( 'NONE',  ( -19.03943276465977164, 0.05219959533909376836, 111.2489096053143669 ) ) ;
#9129=CARTESIAN_POINT ( 'NONE',  ( -0.05219959533909027116, -19.03943276465977164, 77.49890960531435269 ) ) ;
#9130=CARTESIAN_POINT ( 'NONE',  ( -21.52544592524334988, -5.823673210054445271, 93.95942372801903275 ) ) ;
#9131=CARTESIAN_POINT ( 'NONE',  ( -5.049401038298153566, 19.05341960407611168, 80.20724293864769550 ) ) ;
#9132=CARTESIAN_POINT ( 'NONE',  ( -15.72974639402197994, 15.80617190586746368, 45.62390960531436690 ) ) ;
#9133=CARTESIAN_POINT ( 'NONE',  ( -16.55341960407611168, -4.379528057220339221, 76.45724293864769550 ) ) ;
#9134=CARTESIAN_POINT ( 'NONE',  ( 13.97604488694527802, 13.89961937509977652, 59.37390960531434558 ) ) ;
#9135=CARTESIAN_POINT ( 'NONE',  ( -16.52544592524342804, 4.483927247898546575, 111.0405762719810525 ) ) ;
#9136=CARTESIAN_POINT ( 'NONE',  ( 21.55341960407619695, -5.719274019375665929, 21.04275706135234714 ) ) ;
#9137=CARTESIAN_POINT ( 'NONE',  ( -5.823673210054431948, 21.52544592524334988, 62.70942372801902565 ) ) ;
#9138=CARTESIAN_POINT ( 'NONE',  ( 9.474510206698971260, -16.51473224551069308, 37.91557627198102409 ) ) ;
#9139=CARTESIAN_POINT ( 'NONE',  ( -16.52544592524335698, -4.483927247898792601, 63.95942372801901854 ) ) ;
#9140=CARTESIAN_POINT ( 'NONE',  ( 15.80617190586746368, 15.72974639402197994, 109.3739096053143811 ) ) ;
#9141=CARTESIAN_POINT ( 'NONE',  ( 18.67979575497178502, 10.72451020669898547, 109.1655762719810383 ) ) ;
#9142=CARTESIAN_POINT ( 'NONE',  ( -19.02544592524334988, -5.153800228976617603, 38.95942372801900433 ) ) ;
#9143=CARTESIAN_POINT ( 'NONE',  ( -5.049401038298153566, 19.05341960407611168, 65.20724293864765286 ) ) ;
#9145=CARTESIAN_POINT ( 'NONE',  ( -21.52544592524334988, -5.823673210054445271, 73.95942372801901854 ) ) ;
#9146=CARTESIAN_POINT ( 'NONE',  ( 21.52544592524344225, -5.823673210054117533, 53.54057627198103120 ) ) ;
#9147=CARTESIAN_POINT ( 'NONE',  ( -16.53943276465976808, 0.05219959533911058130, 36.24890960531435979 ) ) ;
#9148=CARTESIAN_POINT ( 'NONE',  ( 18.62759615963255655, 10.81492255796105972, 76.66775706135234714 ) ) ;
#9149=CARTESIAN_POINT ( 'NONE',  ( 21.55341960407619695, -5.719274019375665929, 111.0427570613523613 ) ) ;
#9150=CARTESIAN_POINT ( 'NONE',  ( 16.53943276465976808, -0.05219959533910856209, 53.74890960531437401 ) ) ;
#9151=CARTESIAN_POINT ( 'NONE',  ( 16.53943276465976808, -0.05219959533910856209, 103.7489096053143669 ) ) ;
#9153=CARTESIAN_POINT ( 'NONE',  ( 13.89961937509957401, 13.97604488694547697, 56.87609039468564731 ) ) ;
#9154=CARTESIAN_POINT ( 'NONE',  ( 12.06949235617739724, 12.14591786802326823, 111.8760903946856615 ) ) ;
#9155=CARTESIAN_POINT ( 'NONE',  ( 15.72974639402176855, 15.80617190586768217, 61.87609039468568284 ) ) ;
#9156=CARTESIAN_POINT ( 'NONE',  ( -9.564922557960796823, -16.46253265017161027, 72.08224293864770971 ) ) ;
#9157=CARTESIAN_POINT ( 'NONE',  ( 5.049401038297881783, 19.05341960407617563, 32.29275706135233293 ) ) ;
#9158=CARTESIAN_POINT ( 'NONE',  ( 18.67979575497178502, 10.72451020669898547, 44.16557627198103120 ) ) ;
#9159=CARTESIAN_POINT ( 'NONE',  ( 5.719274019375673035, 21.55341960407619339, 27.29275706135234358 ) ) ;
#9160=CARTESIAN_POINT ( 'NONE',  ( 15.80617190586746368, 15.72974639402197994, 94.37390960531436690 ) ) ;
#9161=CARTESIAN_POINT ( 'NONE',  ( -13.97604488694547697, 13.89961937509957934, 98.12609039468566152 ) ) ;
#9162=CARTESIAN_POINT ( 'NONE',  ( -4.483927247898782831, 16.52544592524335698, 47.70942372801902565 ) ) ;
#9164=CARTESIAN_POINT ( 'NONE',  ( -18.67979575497178146, -10.72451020669898902, 96.66557627198102409 ) ) ;
#9165=CARTESIAN_POINT ( 'NONE',  ( 0.05219959533910956823, 16.53943276465976808, 94.99890960531436690 ) ) ;
#9167=CARTESIAN_POINT ( 'NONE',  ( 8.224510206698742110, 14.34966873604972548, 22.08442372801901143 ) ) ;
#9168=CARTESIAN_POINT ( 'NONE',  ( 10.81492255796078972, 18.62759615963270932, 54.58224293864769550 ) ) ;
#9169=CARTESIAN_POINT ( 'NONE',  ( -8.224510206698735004, -14.34966873604973081, 89.58442372801901854 ) ) ;
#9170=DIRECTION ( 'NONE',  ( -0.000000000000000000, 1.000000000000000000, -0.000000000000000000 ) ) ;
#9171=CARTESIAN_POINT ( 'NONE',  ( 16.53943276465976808, 0.05219959533934440121, 56.25109039468568284 ) ) ;
#9172=CARTESIAN_POINT ( 'NONE',  ( 21.53943276465977519, 0.05219959533937863772, 31.25109039468568639 ) ) ;
#9173=CARTESIAN_POINT ( 'NONE',  ( -15.72974639402197994, 15.80617190586746368, 50.62390960531435979 ) ) ;
#9174=CARTESIAN_POINT ( 'NONE',  ( -8.224510206698735004, -14.34966873604973081, 89.58442372801901854 ) ) ;
#9175=CARTESIAN_POINT ( 'NONE',  ( -16.46253265017160317, 9.564922557960807481, 100.8322429386477097 ) ) ;
#9176=CARTESIAN_POINT ( 'NONE',  ( -21.53943276465977519, -0.05219959533937600094, 63.75109039468568284 ) ) ;
#9177=CARTESIAN_POINT ( 'NONE',  ( 18.62759615963271287, -10.81492255796078972, 33.33224293864769550 ) ) ;
#9178=CARTESIAN_POINT ( 'NONE',  ( -5.049401038298153566, 19.05341960407611168, 115.2072429386477097 ) ) ;
#9179=VERTEX_POINT ( 'NONE', #194864 ) ;
#9180=CARTESIAN_POINT ( 'NONE',  ( -9.474510206698720793, -16.51473224551083518, 54.58442372801899722 ) ) ;
#9181=CARTESIAN_POINT ( 'NONE',  ( 16.52544592524335698, 4.483927247898782831, 61.45942372801901854 ) ) ;
#9182=CARTESIAN_POINT ( 'NONE',  ( 18.62759615963271287, -10.81492255796078972, 23.33224293864769194 ) ) ;
#9183=ORIENTED_EDGE ( 'NONE', *, *, #11833, .F. ) ;
#9185=CARTESIAN_POINT ( 'NONE',  ( -5.153800228976328057, -19.02544592524343514, 92.29057627198099567 ) ) ;
#9186=CARTESIAN_POINT ( 'NONE',  ( 16.53943276465976808, 0.05219959533934440121, 106.2510903946856757 ) ) ;
#9188=CARTESIAN_POINT ( 'NONE',  ( -16.55341960407611168, -4.379528057220339221, 91.45724293864769550 ) ) ;
#9189=CARTESIAN_POINT ( 'NONE',  ( 5.719274019375991003, -21.55341960407610458, 47.70724293864770260 ) ) ;
#9190=CARTESIAN_POINT ( 'NONE',  ( -5.049401038298153566, 19.05341960407611168, 35.20724293864768839 ) ) ;
#9191=CARTESIAN_POINT ( 'NONE',  ( 8.224510206698742110, 14.34966873604972548, 72.08442372801899012 ) ) ;
#9192=CARTESIAN_POINT ( 'NONE',  ( -5.823673210054431948, 21.52544592524334988, 37.70942372801900433 ) ) ;
#9193=CARTESIAN_POINT ( 'NONE',  ( 0.05219959533936267826, -19.03943276465977164, 90.00109039468567573 ) ) ;
#9194=CARTESIAN_POINT ( 'NONE',  ( 16.53943276465976808, -0.05219959533910856209, 93.74890960531436690 ) ) ;
#9195=CARTESIAN_POINT ( 'NONE',  ( 9.474510206698971260, -16.51473224551069308, 52.91557627198102409 ) ) ;
#9196=CARTESIAN_POINT ( 'NONE',  ( 19.03943276465977164, -0.05219959533909143690, 23.74890960531435269 ) ) ;
#9197=CARTESIAN_POINT ( 'NONE',  ( 18.62759615963255655, 10.81492255796105972, 106.6677570613523756 ) ) ;
#9198=CARTESIAN_POINT ( 'NONE',  ( 13.89961937509977652, -13.97604488694527269, 78.12390960531433848 ) ) ;
#9200=CARTESIAN_POINT ( 'NONE',  ( 12.14591786802327356, -12.06949235617739191, 60.62609039468567573 ) ) ;
#9201=CARTESIAN_POINT ( 'NONE',  ( 15.72974639402176855, 15.80617190586768217, 96.87609039468568994 ) ) ;
#9202=CARTESIAN_POINT ( 'NONE',  ( 0.05219959533934541429, -16.53943276465976808, 80.00109039468568994 ) ) ;
#9203=CARTESIAN_POINT ( 'NONE',  ( -5.153800228976607833, 19.02544592524334988, 57.70942372801899012 ) ) ;
#9204=CARTESIAN_POINT ( 'NONE',  ( 5.153800228976615827, -19.02544592524334988, 65.20942372801900433 ) ) ;
#9205=CARTESIAN_POINT ( 'NONE',  ( 0.05219959533937995610, -21.53943276465977519, 60.00109039468568284 ) ) ;
#9206=CARTESIAN_POINT ( 'NONE',  ( 5.153800228976335163, 19.02544592524342804, 64.79057627198100988 ) ) ;
#9207=CARTESIAN_POINT ( 'NONE',  ( 13.97604488694548053, -13.89961937509957401, 60.62609039468564731 ) ) ;
#9208=CARTESIAN_POINT ( 'NONE',  ( -16.51473224551069308, -9.474510206698971260, 111.6655762719810383 ) ) ;
#9209=CARTESIAN_POINT ( 'NONE',  ( 5.049401038298161559, -19.05341960407611168, 82.70724293864770971 ) ) ;
#9210=CARTESIAN_POINT ( 'NONE',  ( -16.55341960407611168, -4.379528057220339221, 36.45724293864768839 ) ) ;
#9211=CARTESIAN_POINT ( 'NONE',  ( 15.72974639402199770, -15.80617190586745480, 48.12390960531436690 ) ) ;
#9213=CARTESIAN_POINT ( 'NONE',  ( 15.80617190586769283, -15.72974639402175789, 105.6260903946856899 ) ) ;
#9214=CARTESIAN_POINT ( 'NONE',  ( -16.19135201231366850, -7.376712067591933319, 80.18680854052030327 ) ) ;
#9215=CARTESIAN_POINT ( 'NONE',  ( -9.564922557960796823, -16.46253265017161027, 37.08224293864768839 ) ) ;
#9216=CARTESIAN_POINT ( 'NONE',  ( -9.474510206698964154, 16.51473224551069663, 25.41557627198103120 ) ) ;
#9218=CARTESIAN_POINT ( 'NONE',  ( -0.05219959533937732626, 21.53943276465977519, 62.50109039468568284 ) ) ;
#9220=CARTESIAN_POINT ( 'NONE',  ( 12.06949235617739724, 12.14591786802326823, 56.87609039468568994 ) ) ;
#9221=CARTESIAN_POINT ( 'NONE',  ( 21.53943276465977519, -0.05219959533907433946, 88.74890960531436690 ) ) ;
#9222=CARTESIAN_POINT ( 'NONE',  ( 8.224510206698953496, -14.34966873604960469, 57.91557627198103120 ) ) ;
#9223=CARTESIAN_POINT ( 'NONE',  ( 13.97604488694527802, 13.89961937509977652, 24.37390960531435624 ) ) ;
#9225=CARTESIAN_POINT ( 'NONE',  ( 18.67979575497194134, -10.72451020669871369, 40.83442372801901854 ) ) ;
#9226=CARTESIAN_POINT ( 'NONE',  ( 9.564922557961047289, -16.46253265017146816, 45.41775706135232582 ) ) ;
#9227=CARTESIAN_POINT ( 'NONE',  ( -13.97604488694527625, -13.89961937509977652, 31.87390960531435979 ) ) ;
#9228=CARTESIAN_POINT ( 'NONE',  ( 15.80617190586769283, -15.72974639402175789, 85.62609039468568994 ) ) ;
#9230=CARTESIAN_POINT ( 'NONE',  ( 4.483927247898545687, 16.52544592524342804, 39.79057627198103830 ) ) ;
#9232=CARTESIAN_POINT ( 'NONE',  ( 10.81492255796078972, 18.62759615963270932, 39.58224293864769550 ) ) ;
#9234=CARTESIAN_POINT ( 'NONE',  ( 19.02544592524343514, -5.153800228976328945, 83.54057627198100988 ) ) ;
#9235=CARTESIAN_POINT ( 'NONE',  ( -12.06949235617756955, 12.14591786802309770, 90.62390960531436690 ) ) ;
#9236=CARTESIAN_POINT ( 'NONE',  ( -12.06949235617739369, -12.14591786802326823, 29.37609039468568284 ) ) ;
#9237=CARTESIAN_POINT ( 'NONE',  ( 21.52544592524344225, -5.823673210054117533, 68.54057627198103830 ) ) ;
#9238=VERTEX_POINT ( 'NONE', #13818 ) ;
#9239=CARTESIAN_POINT ( 'NONE',  ( -5.153800228976328057, -19.02544592524343514, 32.29057627198102409 ) ) ;
#9240=CARTESIAN_POINT ( 'NONE',  ( 5.153800228976335163, 19.02544592524342804, 79.79057627198102409 ) ) ;
#9241=CARTESIAN_POINT ( 'NONE',  ( 21.53943276465977519, -0.05219959533907433946, 88.74890960531436690 ) ) ;
#9242=CARTESIAN_POINT ( 'NONE',  ( 8.224510206698742110, 14.34966873604972548, 112.0844237280190185 ) ) ;
#9243=CARTESIAN_POINT ( 'NONE',  ( -19.05341960407611168, -5.049401038298163336, 96.45724293864769550 ) ) ;
#9244=CARTESIAN_POINT ( 'NONE',  ( -13.97604488694547697, 13.89961937509957934, 83.12609039468564731 ) ) ;
#9245=CARTESIAN_POINT ( 'NONE',  ( -19.02544592524334988, -5.153800228976617603, 18.95942372801899722 ) ) ;
#9246=CARTESIAN_POINT ( 'NONE',  ( 10.72451020669898902, -18.67979575497178502, 77.91557627198102409 ) ) ;
#9247=CARTESIAN_POINT ( 'NONE',  ( -18.67979575497178146, -10.72451020669898902, 41.66557627198103120 ) ) ;
#9248=CARTESIAN_POINT ( 'NONE',  ( -9.474510206698964154, 16.51473224551069663, 55.41557627198103120 ) ) ;
#9249=CARTESIAN_POINT ( 'NONE',  ( 16.52544592524342804, -4.483927247898539470, 23.54057627198102765 ) ) ;
#9250=CARTESIAN_POINT ( 'NONE',  ( 19.05341960407611168, 5.049401038298154454, 78.95724293864769550 ) ) ;
#9253=CARTESIAN_POINT ( 'NONE',  ( -5.049401038297874678, -19.05341960407617918, 29.79275706135232227 ) ) ;
#9254=CARTESIAN_POINT ( 'NONE',  ( -12.14591786802309592, -12.06949235617757132, 91.87390960531436690 ) ) ;
#9255=CARTESIAN_POINT ( 'NONE',  ( -10.81492255796105439, 18.62759615963255655, 27.91775706135234358 ) ) ;
#9256=VECTOR ( 'NONE', #68426, 1000.000000000000000 ) ;
#9258=CARTESIAN_POINT ( 'NONE',  ( 15.80617190586746368, 15.72974639402197994, 54.37390960531435979 ) ) ;
#9259=CARTESIAN_POINT ( 'NONE',  ( -4.483927247898782831, 16.52544592524335698, 87.70942372801901854 ) ) ;
#9260=CARTESIAN_POINT ( 'NONE',  ( 13.89961937509977652, -13.97604488694527269, 28.12390960531435624 ) ) ;
#9261=CARTESIAN_POINT ( 'NONE',  ( -19.02544592524342804, 5.153800228976336051, 71.04057627198099567 ) ) ;
#9263=CARTESIAN_POINT ( 'NONE',  ( 14.34966873604960469, 8.224510206698951720, 34.16557627198102409 ) ) ;
#9264=CARTESIAN_POINT ( 'NONE',  ( -15.72974639402176322, -15.80617190586768395, 64.37609039468568994 ) ) ;
#9265=CARTESIAN_POINT ( 'NONE',  ( 5.153800228976335163, 19.02544592524342804, 114.7905762719810241 ) ) ;
#9266=CARTESIAN_POINT ( 'NONE',  ( -15.80617190586768217, 15.72974639402176855, 98.12609039468570415 ) ) ;
#9267=CARTESIAN_POINT ( 'NONE',  ( -5.153800228976328057, -19.02544592524343514, 42.29057627198101699 ) ) ;
#9268=CARTESIAN_POINT ( 'NONE',  ( 5.049401038298161559, -19.05341960407611168, 47.70724293864770260 ) ) ;
#9269=EDGE_LOOP ( 'NONE', ( #41358, #12246, #83229, #108482, #56522, #89351, #151534, #41754 ) ) ;
#9270=CARTESIAN_POINT ( 'NONE',  ( 21.53943276465977519, 0.05219959533937863772, 96.25109039468568994 ) ) ;
#9271=CARTESIAN_POINT ( 'NONE',  ( -14.34966873604972548, 8.224510206698743886, 63.33442372801900433 ) ) ;
#9272=CARTESIAN_POINT ( 'NONE',  ( 21.55341960407619695, -5.719274019375665929, 91.04275706135236135 ) ) ;
#9273=CARTESIAN_POINT ( 'NONE',  ( -18.67979575497178146, -10.72451020669898902, 26.66557627198103475 ) ) ;
#9274=CARTESIAN_POINT ( 'NONE',  ( 13.89961937509957401, 13.97604488694547697, 91.87609039468567573 ) ) ;
#9275=CARTESIAN_POINT ( 'NONE',  ( -15.72974639402176322, -15.80617190586768395, 49.37609039468569705 ) ) ;
#9276=CARTESIAN_POINT ( 'NONE',  ( 14.29746914071037800, 8.314922557961029526, 36.66775706135234714 ) ) ;
#9277=CARTESIAN_POINT ( 'NONE',  ( -5.823673210054116645, -21.52544592524344225, 82.29057627198103830 ) ) ;
#9278=CARTESIAN_POINT ( 'NONE',  ( 16.46253265017146816, 9.564922557961045513, 91.66775706135234714 ) ) ;
#9279=CARTESIAN_POINT ( 'NONE',  ( 9.564922557960805705, 16.46253265017160317, 64.58224293864769550 ) ) ;
#9280=CARTESIAN_POINT ( 'NONE',  ( -0.05219959533936034679, 19.03943276465977164, 102.5010903946856757 ) ) ;
#9281=CARTESIAN_POINT ( 'NONE',  ( -19.02544592524334988, -5.153800228976617603, 88.95942372801897591 ) ) ;
#9282=CARTESIAN_POINT ( 'NONE',  ( 8.224510206698953496, -14.34966873604960469, 57.91557627198103120 ) ) ;
#9283=CARTESIAN_POINT ( 'NONE',  ( 9.474510206698729675, 16.51473224551082808, 77.08442372801900433 ) ) ;
#9284=CARTESIAN_POINT ( 'NONE',  ( 8.314922557961029526, -14.29746914071037800, 55.41775706135234714 ) ) ;
#9285=CARTESIAN_POINT ( 'NONE',  ( 16.51473224551083163, -9.474510206698727899, 30.83442372801900433 ) ) ;
#9286=CARTESIAN_POINT ( 'NONE',  ( -13.97604488694527625, -13.89961937509977652, 36.87390960531436690 ) ) ;
#9287=CARTESIAN_POINT ( 'NONE',  ( -19.02544592524342804, 5.153800228976336051, 46.04057627198101699 ) ) ;
#9288=CARTESIAN_POINT ( 'NONE',  ( -14.34966873604972548, 8.224510206698743886, 58.33442372801901143 ) ) ;
#9291=CARTESIAN_POINT ( 'NONE',  ( 9.474510206698971260, -16.51473224551069308, 102.9155762719810241 ) ) ;
#9292=EDGE_CURVE ( 'NONE', #142736, #40368, #163061, .T. ) ;
#9293=DIRECTION ( 'NONE',  ( 0.000000000000000000, 0.000000000000000000, -1.000000000000000000 ) ) ;
#9295=CARTESIAN_POINT ( 'NONE',  ( -5.049401038297874678, -19.05341960407617918, 99.79275706135234714 ) ) ;
#9296=CARTESIAN_POINT ( 'NONE',  ( -0.05219959533907301413, -21.53943276465977519, 37.49890960531436690 ) ) ;
#9297=CARTESIAN_POINT ( 'NONE',  ( 19.03943276465977164, 0.05219959533936151252, 36.25109039468567573 ) ) ;
#9298=CARTESIAN_POINT ( 'NONE',  ( 14.29746914071037800, 8.314922557961029526, 21.66775706135235069 ) ) ;
#9299=CARTESIAN_POINT ( 'NONE',  ( 9.474510206698971260, -16.51473224551069308, 32.91557627198102409 ) ) ;
#9300=CARTESIAN_POINT ( 'NONE',  ( -13.89961937509977652, 13.97604488694528158, 50.62390960531435979 ) ) ;
#9301=CARTESIAN_POINT ( 'NONE',  ( 18.62759615963271287, -10.81492255796078972, 78.33224293864770971 ) ) ;
#9302=CARTESIAN_POINT ( 'NONE',  ( 13.89961937509977652, -13.97604488694527269, 103.1239096053143527 ) ) ;
#9303=CARTESIAN_POINT ( 'NONE',  ( 5.049401038298161559, -19.05341960407611168, 32.70724293864768129 ) ) ;
#9305=CARTESIAN_POINT ( 'NONE',  ( -16.51473224551082808, 9.474510206698731452, 88.33442372801900433 ) ) ;
#9306=CARTESIAN_POINT ( 'NONE',  ( 16.53943276465976808, -0.05219959533910856209, 53.74890960531437401 ) ) ;
#9307=CARTESIAN_POINT ( 'NONE',  ( -18.62759615963270932, 10.81492255796079327, 30.83224293864770260 ) ) ;
#9308=CARTESIAN_POINT ( 'NONE',  ( -18.67979575497193778, 10.72451020669871902, 103.3344237280190043 ) ) ;
#9309=EDGE_CURVE ( 'NONE', #119772, #30365, #17109, .T. ) ;
#9310=CARTESIAN_POINT ( 'NONE',  ( -21.55341960407610458, -5.719274019375992779, 101.4572429386476955 ) ) ;
#9311=CARTESIAN_POINT ( 'NONE',  ( -21.53943276465977519, -0.05219959533937600094, 73.75109039468567573 ) ) ;
#9312=CARTESIAN_POINT ( 'NONE',  ( 5.719274019375673035, 21.55341960407619339, 72.29275706135236135 ) ) ;
#9313=CARTESIAN_POINT ( 'NONE',  ( 16.46253265017160672, -9.564922557960803928, 108.3322429386476955 ) ) ;
#9314=CARTESIAN_POINT ( 'NONE',  ( -16.52544592524335698, -4.483927247898792601, 103.9594237280190185 ) ) ;
#9315=CARTESIAN_POINT ( 'NONE',  ( 18.62759615963255655, 10.81492255796105972, 66.66775706135234714 ) ) ;
#9316=CARTESIAN_POINT ( 'NONE',  ( 16.51473224551069308, 9.474510206698969483, 59.16557627198102409 ) ) ;
#9317=CARTESIAN_POINT ( 'NONE',  ( -5.049401038297874678, -19.05341960407617918, 39.79275706135232582 ) ) ;
#9318=CARTESIAN_POINT ( 'NONE',  ( 21.53943276465977519, 0.05219959533937863772, 26.25109039468567573 ) ) ;
#9319=CARTESIAN_POINT ( 'NONE',  ( -13.97604488694527625, -13.89961937509977652, 61.87390960531435979 ) ) ;
#9320=CARTESIAN_POINT ( 'NONE',  ( 16.53943276465976808, -0.05219959533910856209, 78.74890960531436690 ) ) ;
#9321=CARTESIAN_POINT ( 'NONE',  ( 14.29746914071049879, -8.314922557960816363, 43.33224293864769550 ) ) ;
#9322=CARTESIAN_POINT ( 'NONE',  ( -15.72974639402197994, 15.80617190586746368, 50.62390960531435979 ) ) ;
#9323=CARTESIAN_POINT ( 'NONE',  ( 19.02544592524343514, -5.153800228976328945, 63.54057627198103830 ) ) ;
#9324=CARTESIAN_POINT ( 'NONE',  ( -15.72974639402197994, 15.80617190586746368, 70.62390960531436690 ) ) ;
#9325=CARTESIAN_POINT ( 'NONE',  ( 9.564922557961047289, -16.46253265017146816, 45.41775706135232582 ) ) ;
#9326=CARTESIAN_POINT ( 'NONE',  ( 16.51473224551083163, -9.474510206698727899, 20.83442372801899722 ) ) ;
#9327=CARTESIAN_POINT ( 'NONE',  ( -4.379528057220328563, 16.55341960407611168, 65.20724293864768129 ) ) ;
#9328=CARTESIAN_POINT ( 'NONE',  ( 5.719274019375991003, -21.55341960407610458, 37.70724293864769550 ) ) ;
#9331=CARTESIAN_POINT ( 'NONE',  ( 16.53943276465976808, 0.05219959533934440121, 81.25109039468568994 ) ) ;
#9333=CARTESIAN_POINT ( 'NONE',  ( 0.05219959533936267826, -19.03943276465977164, 90.00109039468567573 ) ) ;
#9334=CARTESIAN_POINT ( 'NONE',  ( -16.55341960407611168, -4.379528057220339221, 51.45724293864770260 ) ) ;
#9336=CARTESIAN_POINT ( 'NONE',  ( 5.049401038298161559, -19.05341960407611168, 52.70724293864767418 ) ) ;
#9337=CARTESIAN_POINT ( 'NONE',  ( -16.55341960407611168, -4.379528057220339221, 36.45724293864768839 ) ) ;
#9339=CARTESIAN_POINT ( 'NONE',  ( -5.049401038298153566, 19.05341960407611168, 85.20724293864766707 ) ) ;
#9340=CARTESIAN_POINT ( 'NONE',  ( -19.03943276465977164, 0.05219959533909376836, 51.24890960531436690 ) ) ;
#9341=CARTESIAN_POINT ( 'NONE',  ( 21.52544592524334988, 5.823673210054432836, 56.45942372801902565 ) ) ;
#9342=CARTESIAN_POINT ( 'NONE',  ( 9.474510206698971260, -16.51473224551069308, 72.91557627198102409 ) ) ;
#9343=CARTESIAN_POINT ( 'NONE',  ( 19.02544592524343514, -5.153800228976328945, 28.54057627198102409 ) ) ;
#9344=CARTESIAN_POINT ( 'NONE',  ( -16.51473224551069308, -9.474510206698971260, 76.66557627198103830 ) ) ;
#9345=CARTESIAN_POINT ( 'NONE',  ( -5.823673210054116645, -21.52544592524344225, 52.29057627198102409 ) ) ;
#9346=CARTESIAN_POINT ( 'NONE',  ( -9.564922557960796823, -16.46253265017161027, 32.08224293864769550 ) ) ;
#9347=CARTESIAN_POINT ( 'NONE',  ( 15.72974639402199770, -15.80617190586745480, 38.12390960531436690 ) ) ;
#9348=CARTESIAN_POINT ( 'NONE',  ( 4.483927247898790824, -16.52544592524335698, 110.2094237280190185 ) ) ;
#9349=CARTESIAN_POINT ( 'NONE',  ( 16.46253265017146816, 9.564922557961045513, 21.66775706135233648 ) ) ;
#9350=CARTESIAN_POINT ( 'NONE',  ( -14.29746914071037622, -8.314922557961029526, 49.16775706135234003 ) ) ;
#9351=CARTESIAN_POINT ( 'NONE',  ( 16.52544592524335698, 4.483927247898782831, 86.45942372801901854 ) ) ;
#9352=FACE_OUTER_BOUND ( 'NONE', #59736, .T. ) ;
#9353=CARTESIAN_POINT ( 'NONE',  ( 16.55341960407618274, -4.379528057220086978, 71.04275706135234714 ) ) ;
#9354=CARTESIAN_POINT ( 'NONE',  ( -0.05219959533907301413, -21.53943276465977519, 32.49890960531435979 ) ) ;
#9355=CARTESIAN_POINT ( 'NONE',  ( 19.05341960407611168, 5.049401038298154454, 33.95724293864769550 ) ) ;
#9356=CARTESIAN_POINT ( 'NONE',  ( -8.224510206698735004, -14.34966873604973081, 39.58442372801901143 ) ) ;
#9357=CARTESIAN_POINT ( 'NONE',  ( -19.03943276465977164, 0.05219959533909376836, 51.24890960531436690 ) ) ;
#9358=CARTESIAN_POINT ( 'NONE',  ( 0.05219959533937995610, -21.53943276465977519, 45.00109039468568284 ) ) ;
#9359=CARTESIAN_POINT ( 'NONE',  ( -16.53943276465976808, -0.05219959533934237506, 33.75109039468568284 ) ) ;
#9360=CARTESIAN_POINT ( 'NONE',  ( 8.314922557961029526, -14.29746914071037800, 95.41775706135234714 ) ) ;
#9361=CARTESIAN_POINT ( 'NONE',  ( -18.22780087662123094, -5.499999999999984901, 71.48459894673891313 ) ) ;
#9362=CARTESIAN_POINT ( 'NONE',  ( 5.823673210054444382, -21.52544592524334988, 105.2094237280190328 ) ) ;
#9363=CARTESIAN_POINT ( 'NONE',  ( 0.05219959533936267826, -19.03943276465977164, 100.0010903946856757 ) ) ;
#9364=CARTESIAN_POINT ( 'NONE',  ( 19.03943276465977164, 0.05219959533936151252, 51.25109039468567573 ) ) ;
#9365=CARTESIAN_POINT ( 'NONE',  ( -14.34966873604960291, -8.224510206698953496, 76.66557627198103830 ) ) ;
#9366=CARTESIAN_POINT ( 'NONE',  ( -16.46253265017160317, 9.564922557960807481, 25.83224293864769194 ) ) ;
#9367=CARTESIAN_POINT ( 'NONE',  ( 16.51473224551083163, -9.474510206698727899, 55.83442372801899722 ) ) ;
#9369=CARTESIAN_POINT ( 'NONE',  ( 15.72974639402176855, 15.80617190586768217, 66.87609039468568994 ) ) ;
#9370=CARTESIAN_POINT ( 'NONE',  ( -12.06949235617739369, -12.14591786802326823, 24.37609039468567573 ) ) ;
#9371=CARTESIAN_POINT ( 'NONE',  ( 17.48853670773242541, 5.747243402303173987, 38.83328700250009291 ) ) ;
#9372=CARTESIAN_POINT ( 'NONE',  ( -21.53943276465977519, 0.05219959533907696930, 21.24890960531436690 ) ) ;
#9373=CARTESIAN_POINT ( 'NONE',  ( -5.153800228976607833, 19.02544592524334988, 102.7094237280189759 ) ) ;
#9374=CARTESIAN_POINT ( 'NONE',  ( -19.03943276465977164, 0.05219959533909376836, 111.2489096053143669 ) ) ;
#9376=CARTESIAN_POINT ( 'NONE',  ( -8.224510206698948167, 14.34966873604960824, 115.4155762719810241 ) ) ;
#9377=CARTESIAN_POINT ( 'NONE',  ( -21.55341960407619339, 5.719274019375674811, 103.5427570613523613 ) ) ;
#9378=CARTESIAN_POINT ( 'NONE',  ( 9.564922557960805705, 16.46253265017160317, 54.58224293864769550 ) ) ;
#9379=CARTESIAN_POINT ( 'NONE',  ( 21.53943276465977519, 0.05219959533937863772, 61.25109039468567573 ) ) ;
#9380=CARTESIAN_POINT ( 'NONE',  ( -10.72451020669870658, -18.67979575497194134, 104.5844237280190185 ) ) ;
#9381=CARTESIAN_POINT ( 'NONE',  ( -12.14591786802326823, 12.06949235617739902, 113.1260903946856899 ) ) ;
#9382=CARTESIAN_POINT ( 'NONE',  ( -9.474510206698964154, 16.51473224551069663, 75.41557627198103830 ) ) ;
#9383=CARTESIAN_POINT ( 'NONE',  ( -15.72974639402176322, -15.80617190586768395, 54.37609039468568994 ) ) ;
#9384=CARTESIAN_POINT ( 'NONE',  ( -15.80617190586768217, 15.72974639402176855, 48.12609039468568284 ) ) ;
#9385=CARTESIAN_POINT ( 'NONE',  ( 9.564922557961047289, -16.46253265017146816, 75.41775706135234714 ) ) ;
#9386=CARTESIAN_POINT ( 'NONE',  ( -13.97604488694527625, -13.89961937509977652, 106.8739096053143669 ) ) ;
#9387=CARTESIAN_POINT ( 'NONE',  ( -19.03943276465977164, 0.05219959533909376836, 26.24890960531435624 ) ) ;
#9388=CARTESIAN_POINT ( 'NONE',  ( -21.53943276465977519, 0.05219959533907696930, 96.24890960531435269 ) ) ;
#9389=CARTESIAN_POINT ( 'NONE',  ( -13.89961937509957401, -13.97604488694547875, 19.37609039468566507 ) ) ;
#9390=CARTESIAN_POINT ( 'NONE',  ( 12.14591786802309770, 12.06949235617756955, 99.37390960531436690 ) ) ;
#9391=CARTESIAN_POINT ( 'NONE',  ( -19.03943276465977164, 0.05219959533909376836, 56.24890960531435979 ) ) ;
#9392=CARTESIAN_POINT ( 'NONE',  ( -13.89961937509957401, -13.97604488694547875, 99.37609039468567573 ) ) ;
#9393=CARTESIAN_POINT ( 'NONE',  ( 8.224510206698953496, -14.34966873604960469, 67.91557627198102409 ) ) ;
#9394=CARTESIAN_POINT ( 'NONE',  ( -19.02544592524334988, -5.153800228976617603, 18.95942372801899722 ) ) ;
#9395=CARTESIAN_POINT ( 'NONE',  ( 16.51473224551069308, 9.474510206698969483, 99.16557627198102409 ) ) ;
#9396=CARTESIAN_POINT ( 'NONE',  ( 13.97604488694548053, -13.89961937509957401, 80.62609039468567573 ) ) ;
#9397=CARTESIAN_POINT ( 'NONE',  ( -10.81492255796078084, -18.62759615963271287, 82.08224293864768129 ) ) ;
#9398=CARTESIAN_POINT ( 'NONE',  ( -15.80617190586768217, 15.72974639402176855, 43.12609039468568284 ) ) ;
#9399=CARTESIAN_POINT ( 'NONE',  ( -16.55341960407617563, 4.379528057220093196, 48.54275706135234714 ) ) ;
#9400=CARTESIAN_POINT ( 'NONE',  ( -14.34966873604972548, 8.224510206698743886, 98.33442372801901854 ) ) ;
#9401=CARTESIAN_POINT ( 'NONE',  ( 12.14591786802327356, -12.06949235617739191, 40.62609039468567573 ) ) ;
#9402=CARTESIAN_POINT ( 'NONE',  ( 18.67979575497194134, -10.72451020669871369, 35.83442372801901143 ) ) ;
#9403=CARTESIAN_POINT ( 'NONE',  ( 15.72974639402199770, -15.80617190586745480, 43.12390960531435269 ) ) ;
#9404=CARTESIAN_POINT ( 'NONE',  ( 19.03943276465977164, -0.05219959533909143690, 38.74890960531436690 ) ) ;
#9406=CARTESIAN_POINT ( 'NONE',  ( -4.483927247898782831, 16.52544592524335698, 57.70942372801901143 ) ) ;
#9407=CARTESIAN_POINT ( 'NONE',  ( -15.80617190586745835, -15.72974639402198527, 86.87390960531438111 ) ) ;
#9408=CARTESIAN_POINT ( 'NONE',  ( 4.379528057220339221, -16.55341960407611168, 37.70724293864769550 ) ) ;
#9409=CARTESIAN_POINT ( 'NONE',  ( 16.55341960407618274, -4.379528057220086978, 51.04275706135234714 ) ) ;
#9410=CARTESIAN_POINT ( 'NONE',  ( 19.05341960407611168, 5.049401038298154454, 58.95724293864768129 ) ) ;
#9411=CARTESIAN_POINT ( 'NONE',  ( -5.153800228976607833, 19.02544592524334988, 92.70942372801901854 ) ) ;
#9412=CARTESIAN_POINT ( 'NONE',  ( 21.53943276465977519, -0.05219959533907433946, 78.74890960531436690 ) ) ;
#9413=CARTESIAN_POINT ( 'NONE',  ( 0.05219959533910956823, 16.53943276465976808, 34.99890960531435979 ) ) ;
#9414=ORIENTED_EDGE ( 'NONE', *, *, #119720, .T. ) ;
#9415=CARTESIAN_POINT ( 'NONE',  ( 19.46398650005389541, -5.500000000000039968, 92.68269651486369298 ) ) ;
#9416=CARTESIAN_POINT ( 'NONE',  ( 5.719274019375991003, -21.55341960407610458, 62.70724293864769550 ) ) ;
#9418=CARTESIAN_POINT ( 'NONE',  ( 0.05219959533934541429, -16.53943276465976808, 110.0010903946856757 ) ) ;
#9420=CARTESIAN_POINT ( 'NONE',  ( 19.53091890409951858, 5.500000000000029310, 87.56097431831419442 ) ) ;
#9421=CARTESIAN_POINT ( 'NONE',  ( -21.55341960407610458, -5.719274019375992779, 91.45724293864769550 ) ) ;
#9422=CARTESIAN_POINT ( 'NONE',  ( -4.483927247898539470, -16.52544592524342804, 27.29057627198103120 ) ) ;
#9423=CARTESIAN_POINT ( 'NONE',  ( -14.29746914071037622, -8.314922557961029526, 29.16775706135234003 ) ) ;
#9424=CARTESIAN_POINT ( 'NONE',  ( -9.474510206698964154, 16.51473224551069663, 35.41557627198102409 ) ) ;
#9425=CARTESIAN_POINT ( 'NONE',  ( 19.02544592524343514, -5.153800228976328945, 68.54057627198103830 ) ) ;
#9427=CARTESIAN_POINT ( 'NONE',  ( -13.97604488694527625, -13.89961937509977652, 111.8739096053143243 ) ) ;
#9429=CARTESIAN_POINT ( 'NONE',  ( -12.06949235617739369, -12.14591786802326823, 104.3760903946856899 ) ) ;
#9430=CARTESIAN_POINT ( 'NONE',  ( 13.89961937509957401, 13.97604488694547697, 106.8760903946856757 ) ) ;
#9431=CARTESIAN_POINT ( 'NONE',  ( -5.153800228976607833, 19.02544592524334988, 32.70942372801899722 ) ) ;
#9432=CARTESIAN_POINT ( 'NONE',  ( -0.05219959533907301413, -21.53943276465977519, 82.49890960531436690 ) ) ;
#9433=CARTESIAN_POINT ( 'NONE',  ( 14.34966873604960469, 8.224510206698951720, 24.16557627198103120 ) ) ;
#9434=CARTESIAN_POINT ( 'NONE',  ( -5.823673210054116645, -21.52544592524344225, 47.29057627198103120 ) ) ;
#9435=CARTESIAN_POINT ( 'NONE',  ( -15.80617190586745835, -15.72974639402198527, 76.87390960531439532 ) ) ;
#9436=CARTESIAN_POINT ( 'NONE',  ( 16.46253265017146816, 9.564922557961045513, 106.6677570613523471 ) ) ;
#9437=CARTESIAN_POINT ( 'NONE',  ( 16.51473224551069308, 9.474510206698969483, 109.1655762719810383 ) ) ;
#9438=CARTESIAN_POINT ( 'NONE',  ( 0.05219959533937995610, -21.53943276465977519, 75.00109039468568994 ) ) ;
#9439=CARTESIAN_POINT ( 'NONE',  ( -16.46253265017160317, 9.564922557960807481, 65.83224293864769550 ) ) ;
#9441=CARTESIAN_POINT ( 'NONE',  ( 0.05219959533910956823, 16.53943276465976808, 99.99890960531436690 ) ) ;
#9443=CARTESIAN_POINT ( 'NONE',  ( -19.03943276465977164, 0.05219959533909376836, 71.24890960531435269 ) ) ;
#9444=CARTESIAN_POINT ( 'NONE',  ( -16.53943276465976808, 0.05219959533911058130, 91.24890960531436690 ) ) ;
#9446=CARTESIAN_POINT ( 'NONE',  ( -9.474510206698720793, -16.51473224551083518, 89.58442372801900433 ) ) ;
#9448=CARTESIAN_POINT ( 'NONE',  ( -19.03943276465977164, 0.05219959533909376836, 56.24890960531435979 ) ) ;
#9450=CARTESIAN_POINT ( 'NONE',  ( 18.67979575497194134, -10.72451020669871369, 85.83442372801901854 ) ) ;
#9451=CARTESIAN_POINT ( 'NONE',  ( 0.05219959533909260263, 19.03943276465977164, 94.99890960531436690 ) ) ;
#9452=CARTESIAN_POINT ( 'NONE',  ( -14.34966873604972548, 8.224510206698743886, 73.33442372801901854 ) ) ;
#9453=CARTESIAN_POINT ( 'NONE',  ( -17.50000000000000355, -5.622605283950894872, 51.31207310596111171 ) ) ;
#9455=CARTESIAN_POINT ( 'NONE',  ( -16.46253265017146816, -9.564922557961047289, 44.16775706135232582 ) ) ;
#9456=CARTESIAN_POINT ( 'NONE',  ( 18.67979575497194134, -10.72451020669871369, 105.8344237280190328 ) ) ;
#9457=CARTESIAN_POINT ( 'NONE',  ( 17.47620519128089711, 5.664886850699101473, 21.69135819420533196 ) ) ;
#9459=CARTESIAN_POINT ( 'NONE',  ( -16.52544592524335698, -4.483927247898792601, 108.9594237280190185 ) ) ;
#9460=EDGE_CURVE ( 'NONE', #69916, #73939, #5270, .T. ) ;
#9461=CARTESIAN_POINT ( 'NONE',  ( -9.474510206698720793, -16.51473224551083518, 74.58442372801900433 ) ) ;
#9462=CARTESIAN_POINT ( 'NONE',  ( 12.06949235617739724, 12.14591786802326823, 86.87609039468568994 ) ) ;
#9463=CARTESIAN_POINT ( 'NONE',  ( 16.61371651742599909, 7.165104196376162804, 68.64584930007004004 ) ) ;
#9464=CARTESIAN_POINT ( 'NONE',  ( 0.05219959533934541429, -16.53943276465976808, 65.00109039468568994 ) ) ;
#9466=CARTESIAN_POINT ( 'NONE',  ( 10.72451020669871369, 18.67979575497193778, 87.08442372801901854 ) ) ;
#9467=CARTESIAN_POINT ( 'NONE',  ( -0.05219959533936034679, 19.03943276465977164, 92.50109039468566152 ) ) ;
#9468=CARTESIAN_POINT ( 'NONE',  ( -16.46253265017146816, -9.564922557961047289, 29.16775706135232937 ) ) ;
#9469=CARTESIAN_POINT ( 'NONE',  ( 5.049401038298161559, -19.05341960407611168, 67.70724293864769550 ) ) ;
#9470=CARTESIAN_POINT ( 'NONE',  ( 5.049401038298161559, -19.05341960407611168, 52.70724293864767418 ) ) ;
#9472=CARTESIAN_POINT ( 'NONE',  ( -5.719274019375978568, 21.55341960407610458, 85.20724293864770971 ) ) ;
#9473=CARTESIAN_POINT ( 'NONE',  ( -18.67979575497178146, -10.72451020669898902, 31.66557627198102054 ) ) ;
#9474=CARTESIAN_POINT ( 'NONE',  ( 16.51473224551069308, 9.474510206698969483, 29.16557627198103475 ) ) ;
#9475=CARTESIAN_POINT ( 'NONE',  ( -4.379528057220086978, -16.55341960407618274, 69.79275706135234714 ) ) ;
#9477=CARTESIAN_POINT ( 'NONE',  ( -10.81492255796105439, 18.62759615963255655, 27.91775706135234358 ) ) ;
#9478=CARTESIAN_POINT ( 'NONE',  ( -8.314922557960811034, -14.29746914071050412, 67.08224293864770971 ) ) ;
#9480=CARTESIAN_POINT ( 'NONE',  ( -4.379528057220086978, -16.55341960407618274, 24.79275706135235779 ) ) ;
#9481=CARTESIAN_POINT ( 'NONE',  ( -5.049401038297874678, -19.05341960407617918, 54.79275706135234003 ) ) ;
#9482=CARTESIAN_POINT ( 'NONE',  ( -4.379528057220328563, 16.55341960407611168, 60.20724293864768839 ) ) ;
#9483=CARTESIAN_POINT ( 'NONE',  ( -10.72451020669870658, -18.67979575497194134, 19.58442372801901143 ) ) ;
#9485=CARTESIAN_POINT ( 'NONE',  ( 10.81492255796078972, 18.62759615963270932, 74.58224293864768129 ) ) ;
#9486=CARTESIAN_POINT ( 'NONE',  ( 19.03943276465977164, -0.05219959533909143690, 108.7489096053143527 ) ) ;
#9487=CARTESIAN_POINT ( 'NONE',  ( 8.224510206698953496, -14.34966873604960469, 57.91557627198103120 ) ) ;
#9491=CARTESIAN_POINT ( 'NONE',  ( 13.89961937509957401, 13.97604488694547697, 61.87609039468566863 ) ) ;
#9492=CARTESIAN_POINT ( 'NONE',  ( -0.05219959533907301413, -21.53943276465977519, 102.4989096053143811 ) ) ;
#9493=CARTESIAN_POINT ( 'NONE',  ( 5.153800228976335163, 19.02544592524342804, 59.79057627198100988 ) ) ;
#9494=CARTESIAN_POINT ( 'NONE',  ( -5.049401038297874678, -19.05341960407617918, 39.79275706135232582 ) ) ;
#9495=CARTESIAN_POINT ( 'NONE',  ( -13.97604488694527625, -13.89961937509977652, 26.87390960531434558 ) ) ;
#9496=CARTESIAN_POINT ( 'NONE',  ( 5.719274019375673035, 21.55341960407619339, 67.29275706135234714 ) ) ;
#9497=CARTESIAN_POINT ( 'NONE',  ( -16.18388926212239554, -7.379444403734528812, 70.43953151366159204 ) ) ;
#9498=CARTESIAN_POINT ( 'NONE',  ( 8.224510206698953496, -14.34966873604960469, 37.91557627198102409 ) ) ;
#9499=CARTESIAN_POINT ( 'NONE',  ( 5.153800228976335163, 19.02544592524342804, 64.79057627198100988 ) ) ;
#9500=CARTESIAN_POINT ( 'NONE',  ( 21.53943276465977519, -0.05219959533907433946, 68.74890960531435269 ) ) ;
#9501=CARTESIAN_POINT ( 'NONE',  ( -9.564922557960796823, -16.46253265017161027, 62.08224293864769550 ) ) ;
#9502=CARTESIAN_POINT ( 'NONE',  ( 21.53943276465977519, -0.05219959533907433946, 68.74890960531435269 ) ) ;
#9503=CARTESIAN_POINT ( 'NONE',  ( -21.53943276465977519, -0.05219959533937600094, 98.75109039468568994 ) ) ;
#9505=CARTESIAN_POINT ( 'NONE',  ( 16.53943276465976808, 0.05219959533934440121, 101.2510903946856757 ) ) ;
#9506=CARTESIAN_POINT ( 'NONE',  ( -14.29746914071049879, 8.314922557960819915, 85.83224293864768129 ) ) ;
#9507=CARTESIAN_POINT ( 'NONE',  ( 0.05219959533936267826, -19.03943276465977164, 90.00109039468567573 ) ) ;
#9509=CARTESIAN_POINT ( 'NONE',  ( 19.05341960407617918, -5.049401038297876454, 41.04275706135233293 ) ) ;
#9510=CARTESIAN_POINT ( 'NONE',  ( 16.53943276465976808, 0.05219959533934440121, 101.2510903946856757 ) ) ;
#9511=CARTESIAN_POINT ( 'NONE',  ( 5.153800228976615827, -19.02544592524334988, 35.20942372801899722 ) ) ;
#9512=CARTESIAN_POINT ( 'NONE',  ( -19.05341960407611168, -5.049401038298163336, 91.45724293864766707 ) ) ;
#9513=CARTESIAN_POINT ( 'NONE',  ( -10.81492255796078084, -18.62759615963271287, 57.08224293864769550 ) ) ;
#9515=CARTESIAN_POINT ( 'NONE',  ( 9.474510206698971260, -16.51473224551069308, 22.91557627198102765 ) ) ;
#9516=CARTESIAN_POINT ( 'NONE',  ( 15.80617190586769283, -15.72974639402175789, 100.6260903946857184 ) ) ;
#9517=CARTESIAN_POINT ( 'NONE',  ( -16.55341960407617563, 4.379528057220093196, 78.54275706135236135 ) ) ;
#9518=CARTESIAN_POINT ( 'NONE',  ( 5.823673210054444382, -21.52544592524334988, 25.20942372801901854 ) ) ;
#9519=CARTESIAN_POINT ( 'NONE',  ( 14.34966873604972726, -8.224510206698740333, 35.83442372801901143 ) ) ;
#9520=CARTESIAN_POINT ( 'NONE',  ( 0.05219959533909260263, 19.03943276465977164, 109.9989096053143669 ) ) ;
#9521=CARTESIAN_POINT ( 'NONE',  ( 5.153800228976335163, 19.02544592524342804, 34.79057627198102409 ) ) ;
#9522=CARTESIAN_POINT ( 'NONE',  ( 13.97604488694527802, 13.89961937509977652, 49.37390960531434558 ) ) ;
#9523=CARTESIAN_POINT ( 'NONE',  ( -8.314922557961024197, 14.29746914071037800, 52.91775706135235424 ) ) ;
#9524=CARTESIAN_POINT ( 'NONE',  ( 4.483927247898545687, 16.52544592524342804, 94.79057627198105251 ) ) ;
#9525=CARTESIAN_POINT ( 'NONE',  ( -12.06949235617739369, -12.14591786802326823, 99.37609039468568994 ) ) ;
#9526=CARTESIAN_POINT ( 'NONE',  ( 18.62759615963255655, 10.81492255796105972, 41.66775706135235424 ) ) ;
#9527=CARTESIAN_POINT ( 'NONE',  ( -16.46253265017160317, 9.564922557960807481, 80.83224293864769550 ) ) ;
#9528=CARTESIAN_POINT ( 'NONE',  ( 5.049401038298161559, -19.05341960407611168, 67.70724293864769550 ) ) ;
#9529=CARTESIAN_POINT ( 'NONE',  ( 19.03943276465977164, -0.05219959533909143690, 83.74890960531436690 ) ) ;
#9530=CARTESIAN_POINT ( 'NONE',  ( 8.224510206698953496, -14.34966873604960469, 27.91557627198103830 ) ) ;
#9531=CARTESIAN_POINT ( 'NONE',  ( 8.224510206698742110, 14.34966873604972548, 102.0844237280190185 ) ) ;
#9532=VERTEX_POINT ( 'NONE', #109796 ) ;
#9533=CARTESIAN_POINT ( 'NONE',  ( 19.03943276465977164, 0.05219959533936151252, 41.25109039468566152 ) ) ;
#9534=CARTESIAN_POINT ( 'NONE',  ( 13.97604488694527802, 13.89961937509977652, 109.3739096053143669 ) ) ;
#9535=CARTESIAN_POINT ( 'NONE',  ( 16.51473224551069308, 9.474510206698969483, 69.16557627198102409 ) ) ;
#9536=CARTESIAN_POINT ( 'NONE',  ( -5.049401038297874678, -19.05341960407617918, 39.79275706135232582 ) ) ;
#9538=CARTESIAN_POINT ( 'NONE',  ( 16.52544592524335698, 4.483927247898782831, 41.45942372801901143 ) ) ;
#9539=CARTESIAN_POINT ( 'NONE',  ( -16.51473224551082808, 9.474510206698731452, 68.33442372801900433 ) ) ;
#9540=CARTESIAN_POINT ( 'NONE',  ( 8.224510206698742110, 14.34966873604972548, 57.08442372801901854 ) ) ;
#9543=CARTESIAN_POINT ( 'NONE',  ( 19.02544592524343514, -5.153800228976328945, 88.54057627198102409 ) ) ;
#9544=CARTESIAN_POINT ( 'NONE',  ( 5.719274019375991003, -21.55341960407610458, 107.7072429386476955 ) ) ;
#9545=CARTESIAN_POINT ( 'NONE',  ( -19.03943276465977164, -0.05219959533935918106, 78.75109039468567573 ) ) ;
#9546=CARTESIAN_POINT ( 'NONE',  ( 5.049401038298161559, -19.05341960407611168, 107.7072429386476955 ) ) ;
#9547=CARTESIAN_POINT ( 'NONE',  ( 13.97604488694527802, 13.89961937509977652, 34.37390960531436690 ) ) ;
#9548=CARTESIAN_POINT ( 'NONE',  ( -0.05219959533909027116, -19.03943276465977164, 77.49890960531435269 ) ) ;
#9549=CARTESIAN_POINT ( 'NONE',  ( -8.314922557960811034, -14.29746914071050412, 32.08224293864769550 ) ) ;
#9550=CARTESIAN_POINT ( 'NONE',  ( -19.03943276465977164, 0.05219959533909376836, 31.24890960531435979 ) ) ;
#9551=CARTESIAN_POINT ( 'NONE',  ( 13.97604488694548053, -13.89961937509957401, 50.62609039468566152 ) ) ;
#9552=CARTESIAN_POINT ( 'NONE',  ( -4.483927247898539470, -16.52544592524342804, 87.29057627198103830 ) ) ;
#9553=CARTESIAN_POINT ( 'NONE',  ( 0.05219959533936267826, -19.03943276465977164, 20.00109039468567218 ) ) ;
#9554=CARTESIAN_POINT ( 'NONE',  ( 19.03943276465977164, -0.05219959533909143690, 48.74890960531435979 ) ) ;
#9555=CARTESIAN_POINT ( 'NONE',  ( 15.80617190586746368, 15.72974639402197994, 49.37390960531436690 ) ) ;
#9556=CARTESIAN_POINT ( 'NONE',  ( 8.314922557960818139, 14.29746914071049879, 54.58224293864769550 ) ) ;
#9557=CARTESIAN_POINT ( 'NONE',  ( -10.72451020669870658, -18.67979575497194134, 109.5844237280190328 ) ) ;
#9558=CARTESIAN_POINT ( 'NONE',  ( 0.05219959533909260263, 19.03943276465977164, 104.9989096053143669 ) ) ;
#9559=CARTESIAN_POINT ( 'NONE',  ( 0.05219959533909260263, 19.03943276465977164, 104.9989096053143669 ) ) ;
#9560=CARTESIAN_POINT ( 'NONE',  ( -0.05219959533909027116, -19.03943276465977164, 42.49890960531435269 ) ) ;
#9561=CARTESIAN_POINT ( 'NONE',  ( 16.46253265017160672, -9.564922557960803928, 28.33224293864769550 ) ) ;
#9562=CARTESIAN_POINT ( 'NONE',  ( 16.52544592524342804, -4.483927247898539470, 83.54057627198102409 ) ) ;
#9563=CARTESIAN_POINT ( 'NONE',  ( 5.823673210054125526, 21.52544592524343514, 99.79057627198103830 ) ) ;
#9564=CARTESIAN_POINT ( 'NONE',  ( 13.89961937509977652, -13.97604488694527269, 103.1239096053143527 ) ) ;
#9565=CARTESIAN_POINT ( 'NONE',  ( 18.62759615963271287, -10.81492255796078972, 113.3322429386476955 ) ) ;
#9566=CARTESIAN_POINT ( 'NONE',  ( -19.05341960407611168, -5.049401038298163336, 86.45724293864769550 ) ) ;
#9568=CARTESIAN_POINT ( 'NONE',  ( 16.52544592524342804, -4.483927247898539470, 108.5405762719810241 ) ) ;
#9569=CARTESIAN_POINT ( 'NONE',  ( -16.51473224551069308, -9.474510206698971260, 71.66557627198102409 ) ) ;
#9570=CARTESIAN_POINT ( 'NONE',  ( -18.62759615963270932, 10.81492255796079327, 75.83224293864769550 ) ) ;
#9573=CARTESIAN_POINT ( 'NONE',  ( 18.62759615963271287, -10.81492255796078972, 28.33224293864769550 ) ) ;
#9575=CARTESIAN_POINT ( 'NONE',  ( -14.34966873604972548, 8.224510206698743886, 28.33442372801902209 ) ) ;
#9576=CARTESIAN_POINT ( 'NONE',  ( -14.29746914071049879, 8.314922557960819915, 95.83224293864770971 ) ) ;
#9577=CARTESIAN_POINT ( 'NONE',  ( -17.49999999999999645, -5.500000000000000888, 109.2030961746582847 ) ) ;
#9578=CARTESIAN_POINT ( 'NONE',  ( -5.153800228976328057, -19.02544592524343514, 82.29057627198103830 ) ) ;
#9579=CARTESIAN_POINT ( 'NONE',  ( -5.049401038298153566, 19.05341960407611168, 65.20724293864765286 ) ) ;
#9580=CARTESIAN_POINT ( 'NONE',  ( -8.314922557960811034, -14.29746914071050412, 87.08224293864769550 ) ) ;
#9581=CARTESIAN_POINT ( 'NONE',  ( -21.52544592524343514, 5.823673210054127303, 31.04057627198102409 ) ) ;
#9582=CARTESIAN_POINT ( 'NONE',  ( -14.34966873604960291, -8.224510206698953496, 51.66557627198102409 ) ) ;
#9583=CARTESIAN_POINT ( 'NONE',  ( 12.14591786802327356, -12.06949235617739191, 20.62609039468568639 ) ) ;
#9584=CARTESIAN_POINT ( 'NONE',  ( -10.72451020669870658, -18.67979575497194134, 69.58442372801900433 ) ) ;
#9586=CARTESIAN_POINT ( 'NONE',  ( 19.05341960407611168, 5.049401038298154454, 113.9572429386477097 ) ) ;
#9587=CARTESIAN_POINT ( 'NONE',  ( -8.224510206698735004, -14.34966873604973081, 84.58442372801903275 ) ) ;
#9588=B_SPLINE_CURVE_WITH_KNOTS ( 'NONE', 3,
 ( #76078, #152918, #108409, #153920, #186269, #168098 ),
 .UNSPECIFIED., .F., .F.,
 ( 4, 2, 4 ),
 ( 0.000000000000000000, 0.0003837532665635193284, 0.0007675065331270386568 ),
 .UNSPECIFIED. ) ;
#9589=CARTESIAN_POINT ( 'NONE',  ( 5.049401038298161559, -19.05341960407611168, 27.70724293864769550 ) ) ;
#9590=CARTESIAN_POINT ( 'NONE',  ( -16.46253265017160317, 9.564922557960807481, 80.83224293864769550 ) ) ;
#9591=CARTESIAN_POINT ( 'NONE',  ( 15.72974639402199770, -15.80617190586745480, 98.12390960531436690 ) ) ;
#9592=CARTESIAN_POINT ( 'NONE',  ( -0.05219959533934338120, 16.53943276465976808, 27.50109039468567929 ) ) ;
#9593=CARTESIAN_POINT ( 'NONE',  ( 14.29746914071049879, -8.314922557960816363, 48.33224293864770260 ) ) ;
#9594=CARTESIAN_POINT ( 'NONE',  ( -0.05219959533937732626, 21.53943276465977519, 77.50109039468567573 ) ) ;
#9595=CARTESIAN_POINT ( 'NONE',  ( -0.05219959533934338120, 16.53943276465976808, 92.50109039468567573 ) ) ;
#9596=CARTESIAN_POINT ( 'NONE',  ( 19.03943276465977164, -0.05219959533909143690, 113.7489096053143669 ) ) ;
#9597=CARTESIAN_POINT ( 'NONE',  ( 17.40861289039004234, 6.110651285853276882, 28.87232470827434128 ) ) ;
#9599=CARTESIAN_POINT ( 'NONE',  ( -8.314922557961024197, 14.29746914071037800, 112.9177570613523329 ) ) ;
#9600=CARTESIAN_POINT ( 'NONE',  ( 4.483927247898790824, -16.52544592524335698, 65.20942372801901854 ) ) ;
#9601=CARTESIAN_POINT ( 'NONE',  ( -9.474510206698964154, 16.51473224551069663, 70.41557627198102409 ) ) ;
#9602=CARTESIAN_POINT ( 'NONE',  ( 5.153800228976335163, 19.02544592524342804, 84.79057627198099567 ) ) ;
#9603=CARTESIAN_POINT ( 'NONE',  ( -21.52544592524334988, -5.823673210054445271, 78.95942372801901854 ) ) ;
#9604=CARTESIAN_POINT ( 'NONE',  ( -14.29746914071037622, -8.314922557961029526, 79.16775706135234714 ) ) ;
#9605=CARTESIAN_POINT ( 'NONE',  ( 16.53943276465976808, -0.05219959533910856209, 43.74890960531435979 ) ) ;
#9606=CARTESIAN_POINT ( 'NONE',  ( -19.05341960407611168, -5.049401038298163336, 51.45724293864770260 ) ) ;
#9607=CARTESIAN_POINT ( 'NONE',  ( -19.02544592524342804, 5.153800228976336051, 46.04057627198101699 ) ) ;
#9608=ORIENTED_EDGE ( 'NONE', *, *, #10239, .F. ) ;
#9609=CARTESIAN_POINT ( 'NONE',  ( 13.89961937509957401, 13.97604488694547697, 106.8760903946856757 ) ) ;
#9610=CARTESIAN_POINT ( 'NONE',  ( -16.53943276465976808, 0.05219959533911058130, 116.2489096053143669 ) ) ;
#9611=CARTESIAN_POINT ( 'NONE',  ( -9.474510206698964154, 16.51473224551069663, 65.41557627198102409 ) ) ;
#9612=CARTESIAN_POINT ( 'NONE',  ( 5.153800228976615827, -19.02544592524334988, 95.20942372801897591 ) ) ;
#9614=CARTESIAN_POINT ( 'NONE',  ( 10.81492255796106328, -18.62759615963255655, 100.4177570613523471 ) ) ;
#9615=CARTESIAN_POINT ( 'NONE',  ( 4.379528057220092307, 16.55341960407617563, 62.29275706135236845 ) ) ;
#9616=CARTESIAN_POINT ( 'NONE',  ( 19.03943276465977164, 0.05219959533936151252, 91.25109039468566152 ) ) ;
#9617=CARTESIAN_POINT ( 'NONE',  ( -15.72974639402197994, 15.80617190586746368, 65.62390960531436690 ) ) ;
#9618=CARTESIAN_POINT ( 'NONE',  ( -14.29746914071037622, -8.314922557961029526, 49.16775706135234003 ) ) ;
#9620=CARTESIAN_POINT ( 'NONE',  ( 16.46253265017146816, 9.564922557961045513, 61.66775706135234003 ) ) ;
#9621=CARTESIAN_POINT ( 'NONE',  ( 5.719274019375673035, 21.55341960407619339, 97.29275706135234714 ) ) ;
#9622=CARTESIAN_POINT ( 'NONE',  ( -14.29746914071049879, 8.314922557960819915, 115.8322429386477097 ) ) ;
#9623=CARTESIAN_POINT ( 'NONE',  ( -16.46253265017160317, 9.564922557960807481, 65.83224293864769550 ) ) ;
#9624=CARTESIAN_POINT ( 'NONE',  ( -0.05219959533910754901, -16.53943276465976808, 62.49890960531436690 ) ) ;
#9625=CARTESIAN_POINT ( 'NONE',  ( 21.55341960407619695, -5.719274019375665929, 86.04275706135236135 ) ) ;
#9626=CARTESIAN_POINT ( 'NONE',  ( -5.153800228976607833, 19.02544592524334988, 42.70942372801901143 ) ) ;
#9627=CARTESIAN_POINT ( 'NONE',  ( 19.02544592524334988, 5.153800228976608722, 31.45942372801900433 ) ) ;
#9628=CARTESIAN_POINT ( 'NONE',  ( -21.55341960407610458, -5.719274019375992779, 26.45724293864768839 ) ) ;
#9629=CARTESIAN_POINT ( 'NONE',  ( -10.81492255796105439, 18.62759615963255655, 102.9177570613523756 ) ) ;
#9630=CARTESIAN_POINT ( 'NONE',  ( -16.51473224551069308, -9.474510206698971260, 76.66557627198103830 ) ) ;
#9631=CARTESIAN_POINT ( 'NONE',  ( -21.55341960407619339, 5.719274019375674811, 93.54275706135234714 ) ) ;
#9632=CARTESIAN_POINT ( 'NONE',  ( 5.823673210054125526, 21.52544592524343514, 49.79057627198102409 ) ) ;
#9633=CARTESIAN_POINT ( 'NONE',  ( 9.564922557960805705, 16.46253265017160317, 79.58224293864769550 ) ) ;
#9634=CARTESIAN_POINT ( 'NONE',  ( 19.02544592524334988, 5.153800228976608722, 76.45942372801897591 ) ) ;
#9635=CARTESIAN_POINT ( 'NONE',  ( -9.474510206698964154, 16.51473224551069663, 45.41557627198103120 ) ) ;
#9636=CARTESIAN_POINT ( 'NONE',  ( 19.05341960407611168, 5.049401038298154454, 83.95724293864766707 ) ) ;
#9637=CARTESIAN_POINT ( 'NONE',  ( -19.02544592524334988, -5.153800228976617603, 88.95942372801897591 ) ) ;
#9638=CARTESIAN_POINT ( 'NONE',  ( 0.05219959533934541429, -16.53943276465976808, 40.00109039468567573 ) ) ;
#9639=CARTESIAN_POINT ( 'NONE',  ( 16.52544592524342804, -4.483927247898539470, 103.5405762719810383 ) ) ;
#9640=CARTESIAN_POINT ( 'NONE',  ( 5.049401038298161559, -19.05341960407611168, 72.70724293864768129 ) ) ;
#9641=CARTESIAN_POINT ( 'NONE',  ( -18.67979575497178146, -10.72451020669898902, 46.66557627198102409 ) ) ;
#9643=CARTESIAN_POINT ( 'NONE',  ( 12.14591786802327356, -12.06949235617739191, 35.62609039468568994 ) ) ;
#9644=CARTESIAN_POINT ( 'NONE',  ( 10.81492255796106328, -18.62759615963255655, 35.41775706135234003 ) ) ;
#9645=CARTESIAN_POINT ( 'NONE',  ( 18.62759615963255655, 10.81492255796105972, 86.66775706135234714 ) ) ;
#9646=CARTESIAN_POINT ( 'NONE',  ( -16.53943276465976808, -0.05219959533934237506, 83.75109039468568994 ) ) ;
#9647=CARTESIAN_POINT ( 'NONE',  ( -16.46253265017160317, 9.564922557960807481, 75.83224293864769550 ) ) ;
#9648=CARTESIAN_POINT ( 'NONE',  ( 4.379528057220092307, 16.55341960407617563, 102.2927570613523613 ) ) ;
#9649=CARTESIAN_POINT ( 'NONE',  ( -13.97604488694547697, 13.89961937509957934, 53.12609039468565442 ) ) ;
#9650=CARTESIAN_POINT ( 'NONE',  ( 10.81492255796106328, -18.62759615963255655, 35.41775706135234003 ) ) ;
#9651=CARTESIAN_POINT ( 'NONE',  ( -16.53943276465976808, 0.05219959533911058130, 81.24890960531436690 ) ) ;
#9652=CARTESIAN_POINT ( 'NONE',  ( 13.97604488694527802, 13.89961937509977652, 94.37390960531436690 ) ) ;
#9653=CARTESIAN_POINT ( 'NONE',  ( 0.05219959533934541429, -16.53943276465976808, 105.0010903946856757 ) ) ;
#9654=CARTESIAN_POINT ( 'NONE',  ( 10.81492255796106328, -18.62759615963255655, 70.41775706135236135 ) ) ;
#9655=CARTESIAN_POINT ( 'NONE',  ( 8.314922557961029526, -14.29746914071037800, 30.41775706135234358 ) ) ;
#9656=CARTESIAN_POINT ( 'NONE',  ( 5.823673210054444382, -21.52544592524334988, 25.20942372801901854 ) ) ;
#9657=CARTESIAN_POINT ( 'NONE',  ( -16.55341960407611168, -4.379528057220339221, 66.45724293864768129 ) ) ;
#9659=CARTESIAN_POINT ( 'NONE',  ( -15.80617190586768217, 15.72974639402176855, 23.12609039468567573 ) ) ;
#9660=CARTESIAN_POINT ( 'NONE',  ( 12.14591786802309770, 12.06949235617756955, 59.37390960531436690 ) ) ;
#9661=CARTESIAN_POINT ( 'NONE',  ( 9.564922557960805705, 16.46253265017160317, 29.58224293864769550 ) ) ;
#9662=CARTESIAN_POINT ( 'NONE',  ( -10.72451020669898014, 18.67979575497178502, 25.41557627198103120 ) ) ;
#9663=CARTESIAN_POINT ( 'NONE',  ( 21.52544592524334988, 5.823673210054432836, 46.45942372801901854 ) ) ;
#9664=CARTESIAN_POINT ( 'NONE',  ( 14.34966873604960469, 8.224510206698951720, 64.16557627198102409 ) ) ;
#9666=CARTESIAN_POINT ( 'NONE',  ( 21.55341960407610458, 5.719274019375980345, 73.95724293864769550 ) ) ;
#9667=CARTESIAN_POINT ( 'NONE',  ( -16.46253265017160317, 9.564922557960807481, 70.83224293864770971 ) ) ;
#9669=CARTESIAN_POINT ( 'NONE',  ( 13.97604488694527802, 13.89961937509977652, 24.37390960531435624 ) ) ;
#9670=CARTESIAN_POINT ( 'NONE',  ( -19.03943276465977164, -0.05219959533935918106, 73.75109039468566152 ) ) ;
#9671=CARTESIAN_POINT ( 'NONE',  ( -10.81492255796105439, 18.62759615963255655, 52.91775706135235424 ) ) ;
#9672=CARTESIAN_POINT ( 'NONE',  ( 21.55341960407610458, 5.719274019375980345, 63.95724293864770260 ) ) ;
#9673=CARTESIAN_POINT ( 'NONE',  ( -19.03943276465977164, 0.05219959533909376836, 41.24890960531435269 ) ) ;
#9674=CARTESIAN_POINT ( 'NONE',  ( -19.02544592524342804, 5.153800228976336051, 66.04057627198103830 ) ) ;
#9676=CARTESIAN_POINT ( 'NONE',  ( 12.14591786802327356, -12.06949235617739191, 45.62609039468567573 ) ) ;
#9677=CARTESIAN_POINT ( 'NONE',  ( -21.55341960407619339, 5.719274019375674811, 33.54275706135234714 ) ) ;
#9678=CARTESIAN_POINT ( 'NONE',  ( 0.05219959533937995610, -21.53943276465977519, 55.00109039468568284 ) ) ;
#9679=CARTESIAN_POINT ( 'NONE',  ( 0.05219959533909260263, 19.03943276465977164, 99.99890960531436690 ) ) ;
#9680=CARTESIAN_POINT ( 'NONE',  ( -15.80617190586745835, -15.72974639402198527, 86.87390960531438111 ) ) ;
#9681=CARTESIAN_POINT ( 'NONE',  ( -21.52544592524334988, -5.823673210054445271, 28.95942372801902209 ) ) ;
#9682=CARTESIAN_POINT ( 'NONE',  ( -12.06949235617739369, -12.14591786802326823, 49.37609039468569705 ) ) ;
#9683=CARTESIAN_POINT ( 'NONE',  ( 21.53943276465977519, -0.05219959533907433946, 43.74890960531435979 ) ) ;
#9684=CARTESIAN_POINT ( 'NONE',  ( 19.05341960407617918, -5.049401038297876454, 26.04275706135233293 ) ) ;
#9685=CARTESIAN_POINT ( 'NONE',  ( 19.03943276465977164, -0.05219959533909143690, 53.74890960531436690 ) ) ;
#9686=CARTESIAN_POINT ( 'NONE',  ( 16.46253265017160672, -9.564922557960803928, 113.3322429386476955 ) ) ;
#9687=CARTESIAN_POINT ( 'NONE',  ( -16.51473224551069308, -9.474510206698971260, 91.66557627198103830 ) ) ;
#9688=CARTESIAN_POINT ( 'NONE',  ( 16.61371651742640410, -7.165104196375910561, 86.35415069992971837 ) ) ;
#9689=CARTESIAN_POINT ( 'NONE',  ( 19.05341960407617918, -5.049401038297876454, 71.04275706135234714 ) ) ;
#9690=CARTESIAN_POINT ( 'NONE',  ( -21.52544592524343514, 5.823673210054127303, 51.04057627198103120 ) ) ;
#9691=CARTESIAN_POINT ( 'NONE',  ( -16.53943276465976808, 0.05219959533911058130, 26.24890960531435624 ) ) ;
#9692=CARTESIAN_POINT ( 'NONE',  ( 5.153800228976615827, -19.02544592524334988, 85.20942372801900433 ) ) ;
#9694=CARTESIAN_POINT ( 'NONE',  ( -19.02544592524334988, -5.153800228976617603, 23.95942372801900078 ) ) ;
#9695=CARTESIAN_POINT ( 'NONE',  ( 0.05219959533936267826, -19.03943276465977164, 85.00109039468567573 ) ) ;
#9696=CARTESIAN_POINT ( 'NONE',  ( -19.05341960407617563, 5.049401038297882671, 38.54275706135233293 ) ) ;
#9697=CARTESIAN_POINT ( 'NONE',  ( 17.97058386085786097, 5.500000000000047073, 71.50390968646219392 ) ) ;
#9698=CARTESIAN_POINT ( 'NONE',  ( -19.03943276465977164, 0.05219959533909376836, 61.24890960531436690 ) ) ;
#9699=CARTESIAN_POINT ( 'NONE',  ( -12.06949235617756955, 12.14591786802309770, 50.62390960531435979 ) ) ;
#9701=CARTESIAN_POINT ( 'NONE',  ( 16.51473224551069308, 9.474510206698969483, 39.16557627198103120 ) ) ;
#9702=CARTESIAN_POINT ( 'NONE',  ( 12.06949235617757843, -12.14591786802309237, 43.12390960531435269 ) ) ;
#9703=DIRECTION ( 'NONE',  ( -0.000000000000000000, 1.000000000000000000, 0.000000000000000000 ) ) ;
#9704=CARTESIAN_POINT ( 'NONE',  ( -4.483927247898782831, 16.52544592524335698, 112.7094237280190328 ) ) ;
#9705=CARTESIAN_POINT ( 'NONE',  ( 13.89961937509977652, -13.97604488694527269, 63.12390960531435979 ) ) ;
#9706=CARTESIAN_POINT ( 'NONE',  ( -13.89961937509957401, -13.97604488694547875, 19.37609039468566507 ) ) ;
#9707=CARTESIAN_POINT ( 'NONE',  ( -14.29746914071037622, -8.314922557961029526, 34.16775706135234714 ) ) ;
#9708=CARTESIAN_POINT ( 'NONE',  ( 18.62759615963271287, -10.81492255796078972, 43.33224293864769550 ) ) ;
#9709=CARTESIAN_POINT ( 'NONE',  ( 15.72974639402176855, 15.80617190586768217, 86.87609039468568994 ) ) ;
#9711=CARTESIAN_POINT ( 'NONE',  ( 9.474510206698971260, -16.51473224551069308, 67.91557627198102409 ) ) ;
#9712=CARTESIAN_POINT ( 'NONE',  ( -19.05341960407611168, -5.049401038298163336, 111.4572429386476671 ) ) ;
#9713=CARTESIAN_POINT ( 'NONE',  ( 9.474510206698971260, -16.51473224551069308, 97.91557627198102409 ) ) ;
#9715=CARTESIAN_POINT ( 'NONE',  ( 10.72451020669871369, 18.67979575497193778, 22.08442372801901143 ) ) ;
#9716=CARTESIAN_POINT ( 'NONE',  ( 16.53943276465976808, -0.05219959533910856209, 83.74890960531435269 ) ) ;
#9717=CARTESIAN_POINT ( 'NONE',  ( -21.53943276465977519, 0.05219959533907696930, 76.24890960531435269 ) ) ;
#9718=CARTESIAN_POINT ( 'NONE',  ( -0.05219959533909027116, -19.03943276465977164, 72.49890960531435269 ) ) ;
#9719=CARTESIAN_POINT ( 'NONE',  ( -19.02544592524342804, 5.153800228976336051, 71.04057627198099567 ) ) ;
#9720=CARTESIAN_POINT ( 'NONE',  ( -21.52544592524343514, 5.823673210054127303, 116.0405762719810383 ) ) ;
#9722=CARTESIAN_POINT ( 'NONE',  ( 16.46253265017160672, -9.564922557960803928, 73.33224293864769550 ) ) ;
#9723=CARTESIAN_POINT ( 'NONE',  ( -14.34966873604960291, -8.224510206698953496, 106.6655762719810383 ) ) ;
#9725=CARTESIAN_POINT ( 'NONE',  ( -13.89961937509977652, 13.97604488694528158, 60.62390960531436690 ) ) ;
#9726=CARTESIAN_POINT ( 'NONE',  ( -5.153800228976607833, 19.02544592524334988, 92.70942372801901854 ) ) ;
#9727=CARTESIAN_POINT ( 'NONE',  ( -14.29746914071049879, 8.314922557960819915, 95.83224293864770971 ) ) ;
#9728=CARTESIAN_POINT ( 'NONE',  ( 0.05219959533937995610, -21.53943276465977519, 75.00109039468568994 ) ) ;
#9729=CARTESIAN_POINT ( 'NONE',  ( -19.05341960407611168, -5.049401038298163336, 46.45724293864768129 ) ) ;
#9730=CARTESIAN_POINT ( 'NONE',  ( 21.52544592524334988, 5.823673210054432836, 21.45942372801901499 ) ) ;
#9731=CARTESIAN_POINT ( 'NONE',  ( -14.34966873604960291, -8.224510206698953496, 96.66557627198102409 ) ) ;
#9733=CARTESIAN_POINT ( 'NONE',  ( -5.153800228976328057, -19.02544592524343514, 77.29057627198099567 ) ) ;
#9734=CARTESIAN_POINT ( 'NONE',  ( 16.31925111598457789, 7.325300261831532822, 112.3357546103274132 ) ) ;
#9735=CARTESIAN_POINT ( 'NONE',  ( 16.46253265017146816, 9.564922557961045513, 101.6677570613523329 ) ) ;
#9736=CARTESIAN_POINT ( 'NONE',  ( -18.62759615963270932, 10.81492255796079327, 30.83224293864770260 ) ) ;
#9737=CARTESIAN_POINT ( 'NONE',  ( -21.53943276465977519, -0.05219959533937600094, 53.75109039468568994 ) ) ;
#9738=CARTESIAN_POINT ( 'NONE',  ( 13.89961937509977652, -13.97604488694527269, 98.12390960531433848 ) ) ;
#9739=CARTESIAN_POINT ( 'NONE',  ( -5.153800228976607833, 19.02544592524334988, 77.70942372801900433 ) ) ;
#9740=CARTESIAN_POINT ( 'NONE',  ( -0.05219959533909027116, -19.03943276465977164, 77.49890960531435269 ) ) ;
#9741=CARTESIAN_POINT ( 'NONE',  ( 16.55341960407611168, 4.379528057220329451, 83.95724293864770971 ) ) ;
#9742=CARTESIAN_POINT ( 'NONE',  ( 13.97604488694527802, 13.89961937509977652, 109.3739096053143669 ) ) ;
#9743=CARTESIAN_POINT ( 'NONE',  ( -16.52544592524342804, 4.483927247898546575, 91.04057627198103830 ) ) ;
#9744=CARTESIAN_POINT ( 'NONE',  ( -16.46253265017160317, 9.564922557960807481, 100.8322429386477097 ) ) ;
#9745=CARTESIAN_POINT ( 'NONE',  ( 4.379528057220339221, -16.55341960407611168, 42.70724293864770260 ) ) ;
#9746=CARTESIAN_POINT ( 'NONE',  ( -16.51473224551069308, -9.474510206698971260, 21.66557627198102765 ) ) ;
#9748=CARTESIAN_POINT ( 'NONE',  ( -15.80617190586768217, 15.72974639402176855, 53.12609039468568284 ) ) ;
#9749=CARTESIAN_POINT ( 'NONE',  ( -5.153800228976607833, 19.02544592524334988, 77.70942372801900433 ) ) ;
#9750=CARTESIAN_POINT ( 'NONE',  ( -14.29746914071049879, 8.314922557960819915, 45.83224293864769550 ) ) ;
#9751=CARTESIAN_POINT ( 'NONE',  ( -15.72974639402197994, 15.80617190586746368, 105.6239096053143669 ) ) ;
#9752=CARTESIAN_POINT ( 'NONE',  ( 0.05219959533907565091, 21.53943276465977519, 34.99890960531435979 ) ) ;
#9753=CARTESIAN_POINT ( 'NONE',  ( 16.55341960407611168, 4.379528057220329451, 83.95724293864770971 ) ) ;
#9754=CARTESIAN_POINT ( 'NONE',  ( 19.05341960407611168, 5.049401038298154454, 58.95724293864768129 ) ) ;
#9755=CARTESIAN_POINT ( 'NONE',  ( 8.314922557960818139, 14.29746914071049879, 24.58224293864768839 ) ) ;
#9756=CARTESIAN_POINT ( 'NONE',  ( -16.52544592524335698, -4.483927247898792601, 93.95942372801903275 ) ) ;
#9757=CARTESIAN_POINT ( 'NONE',  ( 16.52544592524335698, 4.483927247898782831, 66.45942372801903275 ) ) ;
#9758=CARTESIAN_POINT ( 'NONE',  ( -5.049401038297874678, -19.05341960407617918, 19.79275706135233293 ) ) ;
#9759=CARTESIAN_POINT ( 'NONE',  ( -5.153800228976328057, -19.02544592524343514, 92.29057627198099567 ) ) ;
#9760=CARTESIAN_POINT ( 'NONE',  ( 0.05219959533909260263, 19.03943276465977164, 84.99890960531436690 ) ) ;
#9761=CARTESIAN_POINT ( 'NONE',  ( 8.224510206698742110, 14.34966873604972548, 82.08442372801901854 ) ) ;
#9762=CARTESIAN_POINT ( 'NONE',  ( 19.03943276465977164, -0.05219959533909143690, 43.74890960531435979 ) ) ;
#9763=CARTESIAN_POINT ( 'NONE',  ( -4.483927247898539470, -16.52544592524342804, 52.29057627198102409 ) ) ;
#9764=CARTESIAN_POINT ( 'NONE',  ( 0.05219959533909260263, 19.03943276465977164, 114.9989096053143669 ) ) ;
#9765=CARTESIAN_POINT ( 'NONE',  ( 19.05341960407611168, 5.049401038298154454, 103.9572429386476671 ) ) ;
#9766=CARTESIAN_POINT ( 'NONE',  ( -18.62759615963270932, 10.81492255796079327, 35.83224293864768839 ) ) ;
#9767=CARTESIAN_POINT ( 'NONE',  ( 12.06949235617757843, -12.14591786802309237, 78.12390960531436690 ) ) ;
#9768=CARTESIAN_POINT ( 'NONE',  ( -4.379528057220086978, -16.55341960407618274, 19.79275706135235069 ) ) ;
#9770=CARTESIAN_POINT ( 'NONE',  ( 16.52544592524342804, -4.483927247898539470, 68.54057627198103830 ) ) ;
#9772=CARTESIAN_POINT ( 'NONE',  ( -16.51473224551082808, 9.474510206698731452, 58.33442372801900433 ) ) ;
#9773=CARTESIAN_POINT ( 'NONE',  ( 5.153800228976335163, 19.02544592524342804, 99.79057627198102409 ) ) ;
#9774=CARTESIAN_POINT ( 'NONE',  ( -16.51473224551082808, 9.474510206698731452, 83.33442372801899012 ) ) ;
#9777=CARTESIAN_POINT ( 'NONE',  ( -5.153800228976607833, 19.02544592524334988, 107.7094237280189759 ) ) ;
#9778=CARTESIAN_POINT ( 'NONE',  ( -14.29746914071037622, -8.314922557961029526, 99.16775706135234714 ) ) ;
#9779=CARTESIAN_POINT ( 'NONE',  ( -9.474510206698964154, 16.51473224551069663, 35.41557627198102409 ) ) ;
#9780=CARTESIAN_POINT ( 'NONE',  ( 10.81492255796078972, 18.62759615963270932, 29.58224293864769905 ) ) ;
#9781=CARTESIAN_POINT ( 'NONE',  ( -10.72451020669870658, -18.67979575497194134, 59.58442372801901854 ) ) ;
#9782=CARTESIAN_POINT ( 'NONE',  ( 4.379528057220092307, 16.55341960407617563, 27.29275706135234358 ) ) ;
#9783=CARTESIAN_POINT ( 'NONE',  ( 17.49999999999999289, 3.401555454158704084, 22.96163022339541726 ) ) ;
#9784=CARTESIAN_POINT ( 'NONE',  ( 5.153800228976335163, 19.02544592524342804, 79.79057627198102409 ) ) ;
#9786=CARTESIAN_POINT ( 'NONE',  ( 16.55341960407611168, 4.379528057220329451, 88.95724293864769550 ) ) ;
#9787=CARTESIAN_POINT ( 'NONE',  ( -0.05219959533909027116, -19.03943276465977164, 77.49890960531435269 ) ) ;
#9788=CARTESIAN_POINT ( 'NONE',  ( 19.05341960407611168, 5.049401038298154454, 88.95724293864769550 ) ) ;
#9790=CARTESIAN_POINT ( 'NONE',  ( -9.474510206698720793, -16.51473224551083518, 89.58442372801900433 ) ) ;
#9791=CARTESIAN_POINT ( 'NONE',  ( 10.81492255796078972, 18.62759615963270932, 59.58224293864770260 ) ) ;
#9792=CARTESIAN_POINT ( 'NONE',  ( -19.05341960407611168, -5.049401038298163336, 36.45724293864766707 ) ) ;
#9793=CARTESIAN_POINT ( 'NONE',  ( 5.153800228976615827, -19.02544592524334988, 50.20942372801897591 ) ) ;
#9794=CARTESIAN_POINT ( 'NONE',  ( -19.03943276465977164, 0.05219959533909376836, 56.24890960531435979 ) ) ;
#9795=CARTESIAN_POINT ( 'NONE',  ( -13.97604488694527625, -13.89961937509977652, 86.87390960531436690 ) ) ;
#9797=CARTESIAN_POINT ( 'NONE',  ( 18.67979575497178502, 10.72451020669898547, 94.16557627198103830 ) ) ;
#9798=CARTESIAN_POINT ( 'NONE',  ( 16.52544592524342804, -4.483927247898539470, 88.54057627198103830 ) ) ;
#9799=CARTESIAN_POINT ( 'NONE',  ( -19.05341960407617563, 5.049401038297882671, 48.54275706135233293 ) ) ;
#9800=CARTESIAN_POINT ( 'NONE',  ( 15.72974639402199770, -15.80617190586745480, 88.12390960531436690 ) ) ;
#9801=CARTESIAN_POINT ( 'NONE',  ( 0.05219959533907565091, 21.53943276465977519, 79.99890960531435269 ) ) ;
#9802=CARTESIAN_POINT ( 'NONE',  ( -4.379528057220328563, 16.55341960407611168, 35.20724293864768839 ) ) ;
#9803=CARTESIAN_POINT ( 'NONE',  ( 21.53943276465977519, 0.05219959533937863772, 101.2510903946856757 ) ) ;
#9804=CARTESIAN_POINT ( 'NONE',  ( 4.483927247898790824, -16.52544592524335698, 50.20942372801901854 ) ) ;
#9805=CARTESIAN_POINT ( 'NONE',  ( -5.049401038298153566, 19.05341960407611168, 85.20724293864766707 ) ) ;
#9806=CARTESIAN_POINT ( 'NONE',  ( -13.97604488694527625, -13.89961937509977652, 26.87390960531434558 ) ) ;
#9808=CARTESIAN_POINT ( 'NONE',  ( -18.67979575497193778, 10.72451020669871902, 38.33442372801900433 ) ) ;
#9809=CARTESIAN_POINT ( 'NONE',  ( -21.53943276465977519, -0.05219959533937600094, 53.75109039468568994 ) ) ;
#9810=CARTESIAN_POINT ( 'NONE',  ( -5.153800228976328057, -19.02544592524343514, 52.29057627198100988 ) ) ;
#9811=CARTESIAN_POINT ( 'NONE',  ( 10.81492255796106328, -18.62759615963255655, 20.41775706135234714 ) ) ;
#9812=CARTESIAN_POINT ( 'NONE',  ( 19.02544592524334988, 5.153800228976608722, 66.45942372801899012 ) ) ;
#9813=CARTESIAN_POINT ( 'NONE',  ( -19.05341960407617563, 5.049401038297882671, 68.54275706135230450 ) ) ;
#9814=CARTESIAN_POINT ( 'NONE',  ( -16.55341960407617563, 4.379528057220093196, 28.54275706135234358 ) ) ;
#9815=CARTESIAN_POINT ( 'NONE',  ( 16.51473224551069308, 9.474510206698969483, 24.16557627198102765 ) ) ;
#9816=CARTESIAN_POINT ( 'NONE',  ( 8.224510206698742110, 14.34966873604972548, 67.08442372801901854 ) ) ;
#9817=CARTESIAN_POINT ( 'NONE',  ( -0.05219959533909027116, -19.03943276465977164, 42.49890960531435269 ) ) ;
#9819=CARTESIAN_POINT ( 'NONE',  ( -13.89961937509977652, 13.97604488694528158, 95.62390960531436690 ) ) ;
#9820=CARTESIAN_POINT ( 'NONE',  ( 14.34966873604960469, 8.224510206698951720, 114.1655762719810383 ) ) ;
#9821=CARTESIAN_POINT ( 'NONE',  ( 21.53943276465977519, -0.05219959533907433946, 78.74890960531436690 ) ) ;
#9822=CARTESIAN_POINT ( 'NONE',  ( -8.224510206698735004, -14.34966873604973081, 59.58442372801901854 ) ) ;
#9823=CARTESIAN_POINT ( 'NONE',  ( -19.03943276465977164, -0.05219959533935918106, 18.75109039468567218 ) ) ;
#9824=CARTESIAN_POINT ( 'NONE',  ( 5.153800228976335163, 19.02544592524342804, 44.79057627198103830 ) ) ;
#9825=CARTESIAN_POINT ( 'NONE',  ( 0.05219959533910956823, 16.53943276465976808, 34.99890960531435979 ) ) ;
#9827=CARTESIAN_POINT ( 'NONE',  ( 12.06949235617757843, -12.14591786802309237, 63.12390960531435979 ) ) ;
#9828=CARTESIAN_POINT ( 'NONE',  ( 5.153800228976335163, 19.02544592524342804, 69.79057627198103830 ) ) ;
#9829=CARTESIAN_POINT ( 'NONE',  ( -10.81492255796105439, 18.62759615963255655, 37.91775706135235424 ) ) ;
#9830=CARTESIAN_POINT ( 'NONE',  ( 16.46253265017160672, -9.564922557960803928, 78.33224293864769550 ) ) ;
#9831=CARTESIAN_POINT ( 'NONE',  ( -18.67979575497193778, 10.72451020669871902, 83.33442372801903275 ) ) ;
#9832=CARTESIAN_POINT ( 'NONE',  ( -12.06949235617739369, -12.14591786802326823, 64.37609039468568994 ) ) ;
#9834=CARTESIAN_POINT ( 'NONE',  ( 5.153800228976335163, 19.02544592524342804, 104.7905762719809957 ) ) ;
#9835=CARTESIAN_POINT ( 'NONE',  ( -16.52544592524342804, 4.483927247898546575, 51.04057627198103120 ) ) ;
#9836=CARTESIAN_POINT ( 'NONE',  ( -13.97604488694527625, -13.89961937509977652, 31.87390960531435979 ) ) ;
#9837=CARTESIAN_POINT ( 'NONE',  ( -0.05219959533934338120, 16.53943276465976808, 57.50109039468568994 ) ) ;
#9838=CARTESIAN_POINT ( 'NONE',  ( -8.224510206698948167, 14.34966873604960824, 50.41557627198103120 ) ) ;
#9839=CARTESIAN_POINT ( 'NONE',  ( -19.05341960407611168, -5.049401038298163336, 106.4572429386476955 ) ) ;
#9840=CARTESIAN_POINT ( 'NONE',  ( -18.67979575497178146, -10.72451020669898902, 31.66557627198102054 ) ) ;
#9841=CARTESIAN_POINT ( 'NONE',  ( 9.564922557961047289, -16.46253265017146816, 20.41775706135233293 ) ) ;
#9842=CARTESIAN_POINT ( 'NONE',  ( -4.483927247898539470, -16.52544592524342804, 92.29057627198103830 ) ) ;
#9843=CARTESIAN_POINT ( 'NONE',  ( 9.474510206698971260, -16.51473224551069308, 92.91557627198103830 ) ) ;
#9845=CARTESIAN_POINT ( 'NONE',  ( -12.14591786802326823, 12.06949235617739902, 58.12609039468568994 ) ) ;
#9846=CARTESIAN_POINT ( 'NONE',  ( -19.03943276465977164, 0.05219959533909376836, 51.24890960531436690 ) ) ;
#9848=CARTESIAN_POINT ( 'NONE',  ( -5.153800228976607833, 19.02544592524334988, 42.70942372801901143 ) ) ;
#9849=CARTESIAN_POINT ( 'NONE',  ( 8.224510206698742110, 14.34966873604972548, 82.08442372801901854 ) ) ;
#9850=CARTESIAN_POINT ( 'NONE',  ( 5.153800228976615827, -19.02544592524334988, 100.2094237280190043 ) ) ;
#9851=CARTESIAN_POINT ( 'NONE',  ( 5.823673210054444382, -21.52544592524334988, 60.20942372801902565 ) ) ;
#9852=CARTESIAN_POINT ( 'NONE',  ( -19.02544592524342804, 5.153800228976336051, 76.04057627198102409 ) ) ;
#9853=CARTESIAN_POINT ( 'NONE',  ( -10.81492255796078084, -18.62759615963271287, 97.08224293864770971 ) ) ;
#9854=CARTESIAN_POINT ( 'NONE',  ( -8.224510206698948167, 14.34966873604960824, 100.4155762719810241 ) ) ;
#9855=CARTESIAN_POINT ( 'NONE',  ( -19.02544592524334988, -5.153800228976617603, 73.95942372801900433 ) ) ;
#9856=CARTESIAN_POINT ( 'NONE',  ( -18.62759615963270932, 10.81492255796079327, 60.83224293864769550 ) ) ;
#9857=CARTESIAN_POINT ( 'NONE',  ( 9.474510206698729675, 16.51473224551082808, 37.08442372801899722 ) ) ;
#9858=FACE_BOUND ( 'NONE', #6770, .T. ) ;
#9859=CARTESIAN_POINT ( 'NONE',  ( -21.52544592524343514, 5.823673210054127303, 86.04057627198102409 ) ) ;
#9860=CARTESIAN_POINT ( 'NONE',  ( -19.48894818550243357, 5.500000000000114575, 55.10307310435241135 ) ) ;
#9861=CARTESIAN_POINT ( 'NONE',  ( -9.564922557960796823, -16.46253265017161027, 67.08224293864769550 ) ) ;
#9862=CARTESIAN_POINT ( 'NONE',  ( 16.46253265017160672, -9.564922557960803928, 93.33224293864769550 ) ) ;
#9863=CARTESIAN_POINT ( 'NONE',  ( 9.474510206698729675, 16.51473224551082808, 112.0844237280190043 ) ) ;
#9864=CARTESIAN_POINT ( 'NONE',  ( -19.46398650005389896, 5.499999999999949374, 60.18269651486372851 ) ) ;
#9865=CARTESIAN_POINT ( 'NONE',  ( -16.46253265017160317, 9.564922557960807481, 50.83224293864770260 ) ) ;
#9866=CARTESIAN_POINT ( 'NONE',  ( -0.05219959533909027116, -19.03943276465977164, 107.4989096053143527 ) ) ;
#9867=CARTESIAN_POINT ( 'NONE',  ( -0.05219959533907301413, -21.53943276465977519, 87.49890960531436690 ) ) ;
#9868=CARTESIAN_POINT ( 'NONE',  ( -12.06949235617756955, 12.14591786802309770, 55.62390960531436690 ) ) ;
#9869=CARTESIAN_POINT ( 'NONE',  ( 10.81492255796106328, -18.62759615963255655, 70.41775706135236135 ) ) ;
#9870=CARTESIAN_POINT ( 'NONE',  ( -16.52544592524335698, -4.483927247898792601, 28.95942372801902209 ) ) ;
#9871=CARTESIAN_POINT ( 'NONE',  ( 16.51473224551083163, -9.474510206698727899, 30.83442372801900433 ) ) ;
#9872=CARTESIAN_POINT ( 'NONE',  ( 12.14591786802309770, 12.06949235617756955, 29.37390960531435269 ) ) ;
#9873=CARTESIAN_POINT ( 'NONE',  ( 18.67979575497178502, 10.72451020669898547, 109.1655762719810383 ) ) ;
#9874=CARTESIAN_POINT ( 'NONE',  ( 0.05219959533910956823, 16.53943276465976808, 54.99890960531435269 ) ) ;
#9875=CARTESIAN_POINT ( 'NONE',  ( -13.89961937509957401, -13.97604488694547875, 89.37609039468563310 ) ) ;
#9876=CARTESIAN_POINT ( 'NONE',  ( 13.97604488694548053, -13.89961937509957401, 65.62609039468567573 ) ) ;
#9877=CARTESIAN_POINT ( 'NONE',  ( -21.52544592524334988, -5.823673210054445271, 68.95942372801901854 ) ) ;
#9878=CARTESIAN_POINT ( 'NONE',  ( -16.51473224551082808, 9.474510206698731452, 53.33442372801900433 ) ) ;
#9879=CARTESIAN_POINT ( 'NONE',  ( 4.379528057220339221, -16.55341960407611168, 112.7072429386476955 ) ) ;
#9880=CARTESIAN_POINT ( 'NONE',  ( 15.80617190586746368, 15.72974639402197994, 49.37390960531436690 ) ) ;
#9881=CARTESIAN_POINT ( 'NONE',  ( -14.29746914071049879, 8.314922557960819915, 50.83224293864770971 ) ) ;
#9882=CARTESIAN_POINT ( 'NONE',  ( -17.31747979337953680, -6.344076630960945096, 26.37944868065185133 ) ) ;
#9883=CARTESIAN_POINT ( 'NONE',  ( 5.719274019375673035, 21.55341960407619339, 112.2927570613523471 ) ) ;
#9884=CARTESIAN_POINT ( 'NONE',  ( -4.483927247898782831, 16.52544592524335698, 87.70942372801901854 ) ) ;
#9885=CARTESIAN_POINT ( 'NONE',  ( 14.29746914071049879, -8.314922557960816363, 38.33224293864768839 ) ) ;
#9886=CARTESIAN_POINT ( 'NONE',  ( 10.81492255796106328, -18.62759615963255655, 75.41775706135233293 ) ) ;
#9887=CARTESIAN_POINT ( 'NONE',  ( 0.05219959533937995610, -21.53943276465977519, 65.00109039468568994 ) ) ;
#9888=CARTESIAN_POINT ( 'NONE',  ( 15.72974639402199770, -15.80617190586745480, 78.12390960531436690 ) ) ;
#9889=CARTESIAN_POINT ( 'NONE',  ( 9.474510206698971260, -16.51473224551069308, 42.91557627198103120 ) ) ;
#9890=CARTESIAN_POINT ( 'NONE',  ( -18.67979575497193778, 10.72451020669871902, 53.33442372801901854 ) ) ;
#9891=CARTESIAN_POINT ( 'NONE',  ( 9.564922557960805705, 16.46253265017160317, 34.58224293864770260 ) ) ;
#9892=CARTESIAN_POINT ( 'NONE',  ( 19.05341960407611168, 5.049401038298154454, 58.95724293864768129 ) ) ;
#9893=CARTESIAN_POINT ( 'NONE',  ( 4.483927247898545687, 16.52544592524342804, 94.79057627198105251 ) ) ;
#9894=CARTESIAN_POINT ( 'NONE',  ( -16.51473224551069308, -9.474510206698971260, 91.66557627198103830 ) ) ;
#9895=CARTESIAN_POINT ( 'NONE',  ( -14.34966873604960291, -8.224510206698953496, 41.66557627198103120 ) ) ;
#9896=CARTESIAN_POINT ( 'NONE',  ( -14.34966873604960291, -8.224510206698953496, 101.6655762719810383 ) ) ;
#9897=CARTESIAN_POINT ( 'NONE',  ( -15.80617190586745835, -15.72974639402198527, 66.87390960531436690 ) ) ;
#9898=CARTESIAN_POINT ( 'NONE',  ( -21.52544592524343514, 5.823673210054127303, 116.0405762719810383 ) ) ;
#9899=CARTESIAN_POINT ( 'NONE',  ( -9.474510206698964154, 16.51473224551069663, 115.4155762719810241 ) ) ;
#9901=CARTESIAN_POINT ( 'NONE',  ( -16.51473224551069308, -9.474510206698971260, 76.66557627198103830 ) ) ;
#9902=CARTESIAN_POINT ( 'NONE',  ( -5.153800228976607833, 19.02544592524334988, 112.7094237280190043 ) ) ;
#9903=CARTESIAN_POINT ( 'NONE',  ( -5.823673210054116645, -21.52544592524344225, 77.29057627198102409 ) ) ;
#9904=CARTESIAN_POINT ( 'NONE',  ( 15.80617190586769283, -15.72974639402175789, 100.6260903946857184 ) ) ;
#9905=CARTESIAN_POINT ( 'NONE',  ( 16.51473224551069308, 9.474510206698969483, 74.16557627198103830 ) ) ;
#9906=CARTESIAN_POINT ( 'NONE',  ( -15.72974639402197994, 15.80617190586746368, 115.6239096053143669 ) ) ;
#9907=CARTESIAN_POINT ( 'NONE',  ( -19.02544592524342804, 5.153800228976336051, 116.0405762719810383 ) ) ;
#9908=CARTESIAN_POINT ( 'NONE',  ( -8.314922557961024197, 14.29746914071037800, 87.91775706135234714 ) ) ;
#9909=CARTESIAN_POINT ( 'NONE',  ( -10.81492255796105439, 18.62759615963255655, 72.91775706135234714 ) ) ;
#9910=CARTESIAN_POINT ( 'NONE',  ( -5.719274019375665041, -21.55341960407619695, 99.79275706135234714 ) ) ;
#9911=CARTESIAN_POINT ( 'NONE',  ( 14.29746914071037800, 8.314922557961029526, 56.66775706135235424 ) ) ;
#9912=CARTESIAN_POINT ( 'NONE',  ( 10.72451020669871369, 18.67979575497193778, 22.08442372801901143 ) ) ;
#9913=CARTESIAN_POINT ( 'NONE',  ( -19.02544592524342804, 5.153800228976336051, 26.04057627198103120 ) ) ;
#9914=CARTESIAN_POINT ( 'NONE',  ( -10.72451020669870658, -18.67979575497194134, 94.58442372801901854 ) ) ;
#9915=CARTESIAN_POINT ( 'NONE',  ( 19.02544592524343514, -5.153800228976328945, 98.54057627198100988 ) ) ;
#9916=CARTESIAN_POINT ( 'NONE',  ( -5.719274019375978568, 21.55341960407610458, 90.20724293864770971 ) ) ;
#9917=CARTESIAN_POINT ( 'NONE',  ( 9.564922557961047289, -16.46253265017146816, 55.41775706135234003 ) ) ;
#9919=CARTESIAN_POINT ( 'NONE',  ( -10.81492255796078084, -18.62759615963271287, 52.08224293864768839 ) ) ;
#9920=CARTESIAN_POINT ( 'NONE',  ( 19.03943276465977164, -0.05219959533909143690, 88.74890960531436690 ) ) ;
#9921=CARTESIAN_POINT ( 'NONE',  ( -12.06949235617756955, 12.14591786802309770, 35.62390960531437401 ) ) ;
#9923=CARTESIAN_POINT ( 'NONE',  ( 13.89961937509957401, 13.97604488694547697, 71.87609039468567573 ) ) ;
#9925=CARTESIAN_POINT ( 'NONE',  ( -19.02544592524334988, -5.153800228976617603, 108.9594237280189759 ) ) ;
#9926=CARTESIAN_POINT ( 'NONE',  ( 5.719274019375991003, -21.55341960407610458, 82.70724293864770971 ) ) ;
#9927=CARTESIAN_POINT ( 'NONE',  ( -16.55341960407611168, -4.379528057220339221, 71.45724293864769550 ) ) ;
#9928=CARTESIAN_POINT ( 'NONE',  ( -13.89961937509977652, 13.97604488694528158, 95.62390960531436690 ) ) ;
#9929=CARTESIAN_POINT ( 'NONE',  ( 16.55341960407618274, -4.379528057220086978, 36.04275706135234714 ) ) ;
#9930=CARTESIAN_POINT ( 'NONE',  ( -19.03943276465977164, 0.05219959533909376836, 56.24890960531435979 ) ) ;
#9931=CARTESIAN_POINT ( 'NONE',  ( -5.719274019375978568, 21.55341960407610458, 115.2072429386476955 ) ) ;
#9932=CARTESIAN_POINT ( 'NONE',  ( -16.46253265017146816, -9.564922557961047289, 79.16775706135234714 ) ) ;
#9933=CARTESIAN_POINT ( 'NONE',  ( 9.474510206698971260, -16.51473224551069308, 97.91557627198102409 ) ) ;
#9934=CARTESIAN_POINT ( 'NONE',  ( 5.049401038298161559, -19.05341960407611168, 72.70724293864768129 ) ) ;
#9935=CARTESIAN_POINT ( 'NONE',  ( -18.67979575497178146, -10.72451020669898902, 76.66557627198103830 ) ) ;
#9936=CARTESIAN_POINT ( 'NONE',  ( 13.89961937509977652, -13.97604488694527269, 43.12390960531434558 ) ) ;
#9938=CARTESIAN_POINT ( 'NONE',  ( -4.379528057220328563, 16.55341960407611168, 50.20724293864769550 ) ) ;
#9939=CARTESIAN_POINT ( 'NONE',  ( -19.05341960407611168, -5.049401038298163336, 106.4572429386476955 ) ) ;
#9941=CARTESIAN_POINT ( 'NONE',  ( 19.03943276465977164, 0.05219959533936151252, 66.25109039468567573 ) ) ;
#9942=CARTESIAN_POINT ( 'NONE',  ( -21.52544592524343514, 5.823673210054127303, 76.04057627198102409 ) ) ;
#9943=CARTESIAN_POINT ( 'NONE',  ( 19.03943276465977164, 0.05219959533936151252, 51.25109039468567573 ) ) ;
#9944=CARTESIAN_POINT ( 'NONE',  ( -13.97604488694527625, -13.89961937509977652, 106.8739096053143669 ) ) ;
#9946=CARTESIAN_POINT ( 'NONE',  ( 10.81492255796078972, 18.62759615963270932, 44.58224293864769550 ) ) ;
#9947=CARTESIAN_POINT ( 'NONE',  ( 5.049401038298161559, -19.05341960407611168, 67.70724293864769550 ) ) ;
#9948=CARTESIAN_POINT ( 'NONE',  ( 18.67979575497194134, -10.72451020669871369, 70.83442372801901854 ) ) ;
#9949=CARTESIAN_POINT ( 'NONE',  ( -13.97604488694527625, -13.89961937509977652, 41.87390960531435979 ) ) ;
#9950=CARTESIAN_POINT ( 'NONE',  ( -21.52544592524334988, -5.823673210054445271, 18.95942372801901143 ) ) ;
#9952=CARTESIAN_POINT ( 'NONE',  ( 21.52544592524334988, 5.823673210054432836, 51.45942372801901854 ) ) ;
#9954=CARTESIAN_POINT ( 'NONE',  ( 9.474510206698971260, -16.51473224551069308, 107.9155762719810383 ) ) ;
#9955=CARTESIAN_POINT ( 'NONE',  ( 19.03943276465977164, 0.05219959533936151252, 71.25109039468566152 ) ) ;
#9957=CARTESIAN_POINT ( 'NONE',  ( -15.72974639402176322, -15.80617190586768395, 24.37609039468567573 ) ) ;
#9958=CARTESIAN_POINT ( 'NONE',  ( 0.05219959533909260263, 19.03943276465977164, 59.99890960531436690 ) ) ;
#9959=CARTESIAN_POINT ( 'NONE',  ( -8.314922557961024197, 14.29746914071037800, 42.91775706135235424 ) ) ;
#9961=CARTESIAN_POINT ( 'NONE',  ( -19.03943276465977164, -0.05219959533935918106, 18.75109039468567218 ) ) ;
#9962=CARTESIAN_POINT ( 'NONE',  ( 5.049401038298161559, -19.05341960407611168, 37.70724293864768839 ) ) ;
#9963=CARTESIAN_POINT ( 'NONE',  ( -13.97604488694547697, 13.89961937509957934, 23.12609039468565442 ) ) ;
#9964=CARTESIAN_POINT ( 'NONE',  ( 14.29746914071037800, 8.314922557961029526, 86.66775706135234714 ) ) ;
#9965=CARTESIAN_POINT ( 'NONE',  ( 16.46253265017160672, -9.564922557960803928, 88.33224293864769550 ) ) ;
#9966=CARTESIAN_POINT ( 'NONE',  ( 15.72974639402176855, 15.80617190586768217, 56.87609039468568994 ) ) ;
#9969=CARTESIAN_POINT ( 'NONE',  ( -17.49999999999999645, 5.499999999999992006, 28.71769037696435234 ) ) ;
#9970=CARTESIAN_POINT ( 'NONE',  ( -16.52544592524335698, -4.483927247898792601, 48.95942372801902565 ) ) ;
#9971=CARTESIAN_POINT ( 'NONE',  ( 21.53943276465977519, 0.05219959533937863772, 71.25109039468568994 ) ) ;
#9972=CARTESIAN_POINT ( 'NONE',  ( -18.62759615963255300, -10.81492255796106328, 104.1677570613523471 ) ) ;
#9974=CARTESIAN_POINT ( 'NONE',  ( 14.29746914071037800, 8.314922557961029526, 26.66775706135235424 ) ) ;
#9975=CARTESIAN_POINT ( 'NONE',  ( -19.03943276465977164, 0.05219959533909376836, 91.24890960531436690 ) ) ;
#9976=CARTESIAN_POINT ( 'NONE',  ( -5.153800228976328057, -19.02544592524343514, 112.2905762719810099 ) ) ;
#9978=CARTESIAN_POINT ( 'NONE',  ( 16.19135201231368981, 7.376712067591806310, 42.68680854052031748 ) ) ;
#9979=CARTESIAN_POINT ( 'NONE',  ( -14.29746914071049879, 8.314922557960819915, 115.8322429386477097 ) ) ;
#9980=CARTESIAN_POINT ( 'NONE',  ( -10.81492255796078084, -18.62759615963271287, 42.08224293864769550 ) ) ;
#9981=CARTESIAN_POINT ( 'NONE',  ( 14.29746914071037800, 8.314922557961029526, 101.6677570613523613 ) ) ;
#9982=CARTESIAN_POINT ( 'NONE',  ( 0.05219959533910956823, 16.53943276465976808, 79.99890960531435269 ) ) ;
#9983=CARTESIAN_POINT ( 'NONE',  ( 5.049401038298161559, -19.05341960407611168, 67.70724293864769550 ) ) ;
#9984=CARTESIAN_POINT ( 'NONE',  ( 18.62759615963255655, 10.81492255796105972, 86.66775706135234714 ) ) ;
#9985=CARTESIAN_POINT ( 'NONE',  ( -14.29746914071037622, -8.314922557961029526, 19.16775706135234714 ) ) ;
#9986=CARTESIAN_POINT ( 'NONE',  ( -12.06949235617756955, 12.14591786802309770, 95.62390960531436690 ) ) ;
#9987=CARTESIAN_POINT ( 'NONE',  ( 0.05219959533937995610, -21.53943276465977519, 40.00109039468567573 ) ) ;
#9988=CARTESIAN_POINT ( 'NONE',  ( 5.719274019375991003, -21.55341960407610458, 77.70724293864770971 ) ) ;
#9989=CARTESIAN_POINT ( 'NONE',  ( 5.049401038297881783, 19.05341960407617563, 32.29275706135233293 ) ) ;
#9991=CARTESIAN_POINT ( 'NONE',  ( -0.05219959533909027116, -19.03943276465977164, 102.4989096053143669 ) ) ;
#9992=CARTESIAN_POINT ( 'NONE',  ( 8.314922557960818139, 14.29746914071049879, 64.58224293864769550 ) ) ;
#9993=CARTESIAN_POINT ( 'NONE',  ( 14.34966873604960469, 8.224510206698951720, 44.16557627198103120 ) ) ;
#9994=CARTESIAN_POINT ( 'NONE',  ( 14.29746914071049879, -8.314922557960816363, 23.33224293864769194 ) ) ;
#9995=CARTESIAN_POINT ( 'NONE',  ( 19.03943276465977164, 0.05219959533936151252, 66.25109039468567573 ) ) ;
#9996=CARTESIAN_POINT ( 'NONE',  ( 19.49671883438228903, 5.499999999999973355, 52.39279849105685116 ) ) ;
#9997=CARTESIAN_POINT ( 'NONE',  ( 16.51473224551069308, 9.474510206698969483, 114.1655762719810241 ) ) ;
#9998=CARTESIAN_POINT ( 'NONE',  ( 16.55341960407611168, 4.379528057220329451, 88.95724293864769550 ) ) ;
#10000=CARTESIAN_POINT ( 'NONE',  ( -16.51473224551069308, -9.474510206698971260, 46.66557627198102409 ) ) ;
#10001=CARTESIAN_POINT ( 'NONE',  ( -15.72974639402197994, 15.80617190586746368, 50.62390960531435979 ) ) ;
#10002=CARTESIAN_POINT ( 'NONE',  ( -0.05219959533907301413, -21.53943276465977519, 82.49890960531436690 ) ) ;
#10003=CARTESIAN_POINT ( 'NONE',  ( 0.05219959533910956823, 16.53943276465976808, 114.9989096053143669 ) ) ;
#10004=CARTESIAN_POINT ( 'NONE',  ( 16.55341960407618274, -4.379528057220086978, 66.04275706135236135 ) ) ;
#10005=CARTESIAN_POINT ( 'NONE',  ( 5.049401038298161559, -19.05341960407611168, 42.70724293864767418 ) ) ;
#10006=CARTESIAN_POINT ( 'NONE',  ( 19.05341960407617918, -5.049401038297876454, 46.04275706135233293 ) ) ;
#10007=CARTESIAN_POINT ( 'NONE',  ( 18.67979575497194134, -10.72451020669871369, 60.83442372801901854 ) ) ;
#10008=CARTESIAN_POINT ( 'NONE',  ( 4.379528057220339221, -16.55341960407611168, 102.7072429386476955 ) ) ;
#10009=CARTESIAN_POINT ( 'NONE',  ( -16.51473224551082808, 9.474510206698731452, 88.33442372801900433 ) ) ;
#10012=CARTESIAN_POINT ( 'NONE',  ( 10.72451020669898902, -18.67979575497178502, 47.91557627198102409 ) ) ;
#10013=CARTESIAN_POINT ( 'NONE',  ( 13.89961937509977652, -13.97604488694527269, 28.12390960531435624 ) ) ;
#10014=CARTESIAN_POINT ( 'NONE',  ( -5.823673210054431948, 21.52544592524334988, 82.70942372801900433 ) ) ;
#10015=ORIENTED_EDGE ( 'NONE', *, *, #45882, .T. ) ;
#10016=CARTESIAN_POINT ( 'NONE',  ( -12.14591786802309592, -12.06949235617757132, 36.87390960531435979 ) ) ;
#10017=CARTESIAN_POINT ( 'NONE',  ( 8.314922557961029526, -14.29746914071037800, 55.41775706135234714 ) ) ;
#10018=CARTESIAN_POINT ( 'NONE',  ( 12.06949235617757843, -12.14591786802309237, 43.12390960531435269 ) ) ;
#10019=CARTESIAN_POINT ( 'NONE',  ( -15.72974639402197994, 15.80617190586746368, 75.62390960531439532 ) ) ;
#10020=CARTESIAN_POINT ( 'NONE',  ( 0.05219959533907565091, 21.53943276465977519, 79.99890960531435269 ) ) ;
#10021=DIRECTION ( 'NONE',  ( -1.000000000000000000, -0.000000000000000000, -0.000000000000000000 ) ) ;
#10022=CARTESIAN_POINT ( 'NONE',  ( 0.05219959533936267826, -19.03943276465977164, 90.00109039468567573 ) ) ;
#10023=CARTESIAN_POINT ( 'NONE',  ( 13.97604488694527802, 13.89961937509977652, 114.3739096053143669 ) ) ;
#10024=CARTESIAN_POINT ( 'NONE',  ( -16.51473224551069308, -9.474510206698971260, 46.66557627198102409 ) ) ;
#10025=CARTESIAN_POINT ( 'NONE',  ( -19.03943276465977164, 0.05219959533909376836, 36.24890960531436690 ) ) ;
#10027=VERTEX_POINT ( 'NONE', #136917 ) ;
#10028=CARTESIAN_POINT ( 'NONE',  ( 14.34966873604972726, -8.224510206698740333, 80.83442372801901854 ) ) ;
#10029=CARTESIAN_POINT ( 'NONE',  ( 10.81492255796078972, 18.62759615963270932, 109.5822429386476955 ) ) ;
#10030=CARTESIAN_POINT ( 'NONE',  ( -19.03943276465977164, 0.05219959533909376836, 76.24890960531435269 ) ) ;
#10031=CARTESIAN_POINT ( 'NONE',  ( 10.72451020669871369, 18.67979575497193778, 37.08442372801901143 ) ) ;
#10032=CARTESIAN_POINT ( 'NONE',  ( -9.564922557960796823, -16.46253265017161027, 102.0822429386477097 ) ) ;
#10035=CARTESIAN_POINT ( 'NONE',  ( -0.05219959533937732626, 21.53943276465977519, 32.50109039468568284 ) ) ;
#10036=CARTESIAN_POINT ( 'NONE',  ( 0.05219959533909260263, 19.03943276465977164, 114.9989096053143669 ) ) ;
#10037=CARTESIAN_POINT ( 'NONE',  ( -13.89961937509977652, 13.97604488694528158, 105.6239096053143527 ) ) ;
#10038=CARTESIAN_POINT ( 'NONE',  ( 9.474510206698729675, 16.51473224551082808, 37.08442372801899722 ) ) ;
#10039=CARTESIAN_POINT ( 'NONE',  ( 21.52544592524334988, 5.823673210054432836, 21.45942372801901499 ) ) ;
#10040=CARTESIAN_POINT ( 'NONE',  ( -5.049401038297874678, -19.05341960407617918, 44.79275706135232582 ) ) ;
#10041=CARTESIAN_POINT ( 'NONE',  ( -19.05341960407617563, 5.049401038297882671, 43.54275706135232582 ) ) ;
#10042=CARTESIAN_POINT ( 'NONE',  ( 16.55341960407618274, -4.379528057220086978, 96.04275706135236135 ) ) ;
#10043=CARTESIAN_POINT ( 'NONE',  ( 9.564922557960805705, 16.46253265017160317, 114.5822429386476955 ) ) ;
#10044=CARTESIAN_POINT ( 'NONE',  ( 19.02544592524343514, -5.153800228976328945, 78.54057627198099567 ) ) ;
#10045=CARTESIAN_POINT ( 'NONE',  ( 18.67979575497194134, -10.72451020669871369, 80.83442372801901854 ) ) ;
#10046=CARTESIAN_POINT ( 'NONE',  ( -21.52544592524334988, -5.823673210054445271, 98.95942372801903275 ) ) ;
#10048=CARTESIAN_POINT ( 'NONE',  ( 19.03943276465977164, -0.05219959533909143690, 83.74890960531436690 ) ) ;
#10049=CARTESIAN_POINT ( 'NONE',  ( -21.52544592524334988, -5.823673210054445271, 63.95942372801901854 ) ) ;
#10050=CARTESIAN_POINT ( 'NONE',  ( -5.153800228976607833, 19.02544592524334988, 107.7094237280189759 ) ) ;
#10051=CARTESIAN_POINT ( 'NONE',  ( 16.46253265017160672, -9.564922557960803928, 63.33224293864769550 ) ) ;
#10052=CARTESIAN_POINT ( 'NONE',  ( 21.52544592524344225, -5.823673210054117533, 23.54057627198102765 ) ) ;
#10053=CARTESIAN_POINT ( 'NONE',  ( 19.05341960407611168, 5.049401038298154454, 83.95724293864766707 ) ) ;
#10055=CARTESIAN_POINT ( 'NONE',  ( -13.97604488694527625, -13.89961937509977652, 61.87390960531435979 ) ) ;
#10056=CARTESIAN_POINT ( 'NONE',  ( -9.474510206698964154, 16.51473224551069663, 50.41557627198102409 ) ) ;
#10057=CARTESIAN_POINT ( 'NONE',  ( 10.81492255796078972, 18.62759615963270932, 109.5822429386476955 ) ) ;
#10058=CARTESIAN_POINT ( 'NONE',  ( 14.34966873604972726, -8.224510206698740333, 100.8344237280190185 ) ) ;
#10060=CARTESIAN_POINT ( 'NONE',  ( 9.564922557961047289, -16.46253265017146816, 60.41775706135233293 ) ) ;
#10061=CARTESIAN_POINT ( 'NONE',  ( 5.153800228976335163, 19.02544592524342804, 89.79057627198102409 ) ) ;
#10062=CARTESIAN_POINT ( 'NONE',  ( 16.53943276465976808, -0.05219959533910856209, 73.74890960531433848 ) ) ;
#10063=CARTESIAN_POINT ( 'NONE',  ( 14.29746914071049879, -8.314922557960816363, 113.3322429386476955 ) ) ;
#10064=CARTESIAN_POINT ( 'NONE',  ( 15.80617190586746368, 15.72974639402197994, 39.37390960531436690 ) ) ;
#10065=CARTESIAN_POINT ( 'NONE',  ( 19.03943276465977164, -0.05219959533909143690, 113.7489096053143669 ) ) ;
#10066=CARTESIAN_POINT ( 'NONE',  ( 14.29746914071049879, -8.314922557960816363, 93.33224293864769550 ) ) ;
#10068=CARTESIAN_POINT ( 'NONE',  ( -19.02544592524334988, -5.153800228976617603, 28.95942372801900433 ) ) ;
#10069=CARTESIAN_POINT ( 'NONE',  ( -8.314922557961024197, 14.29746914071037800, 107.9177570613523471 ) ) ;
#10070=CARTESIAN_POINT ( 'NONE',  ( -19.03943276465977164, 0.05219959533909376836, 91.24890960531436690 ) ) ;
#10072=CARTESIAN_POINT ( 'NONE',  ( -21.55341960407619339, 5.719274019375674811, 48.54275706135234714 ) ) ;
#10073=CARTESIAN_POINT ( 'NONE',  ( 18.62759615963271287, -10.81492255796078972, 43.33224293864769550 ) ) ;
#10074=CARTESIAN_POINT ( 'NONE',  ( -18.62759615963255300, -10.81492255796106328, 29.16775706135234003 ) ) ;
#10076=CARTESIAN_POINT ( 'NONE',  ( 18.67979575497178502, 10.72451020669898547, 79.16557627198103830 ) ) ;
#10077=CARTESIAN_POINT ( 'NONE',  ( -8.314922557960811034, -14.29746914071050412, 97.08224293864770971 ) ) ;
#10078=CARTESIAN_POINT ( 'NONE',  ( 19.05341960407617918, -5.049401038297876454, 56.04275706135234714 ) ) ;
#10079=CARTESIAN_POINT ( 'NONE',  ( -13.89961937509977652, 13.97604488694528158, 50.62390960531435979 ) ) ;
#10080=CARTESIAN_POINT ( 'NONE',  ( 19.03943276465977164, -0.05219959533909143690, 93.74890960531435269 ) ) ;
#10081=CARTESIAN_POINT ( 'NONE',  ( -19.05341960407611168, -5.049401038298163336, 96.45724293864769550 ) ) ;
#10082=CARTESIAN_POINT ( 'NONE',  ( -12.14591786802309592, -12.06949235617757132, 111.8739096053143669 ) ) ;
#10083=CARTESIAN_POINT ( 'NONE',  ( -16.53943276465976808, 0.05219959533911058130, 46.24890960531435979 ) ) ;
#10084=CARTESIAN_POINT ( 'NONE',  ( 8.224510206698742110, 14.34966873604972548, 37.08442372801901143 ) ) ;
#10085=CARTESIAN_POINT ( 'NONE',  ( -5.719274019375665041, -21.55341960407619695, 104.7927570613523898 ) ) ;
#10086=CARTESIAN_POINT ( 'NONE',  ( 5.049401038298161559, -19.05341960407611168, 112.7072429386476813 ) ) ;
#10087=CARTESIAN_POINT ( 'NONE',  ( 16.52544592524335698, 4.483927247898782831, 111.4594237280190328 ) ) ;
#10088=CARTESIAN_POINT ( 'NONE',  ( -21.52544592524334988, -5.823673210054445271, 38.95942372801901854 ) ) ;
#10089=CARTESIAN_POINT ( 'NONE',  ( 19.02544592524343514, -5.153800228976328945, 103.5405762719809957 ) ) ;
#10090=CARTESIAN_POINT ( 'NONE',  ( 14.29746914071037800, 8.314922557961029526, 51.66775706135234714 ) ) ;
#10091=CARTESIAN_POINT ( 'NONE',  ( -8.314922557961024197, 14.29746914071037800, 112.9177570613523329 ) ) ;
#10092=CARTESIAN_POINT ( 'NONE',  ( 16.52544592524335698, 4.483927247898782831, 96.45942372801901854 ) ) ;
#10093=CARTESIAN_POINT ( 'NONE',  ( 14.29746914071037800, 8.314922557961029526, 21.66775706135235069 ) ) ;
#10094=CARTESIAN_POINT ( 'NONE',  ( 16.46253265017160672, -9.564922557960803928, 43.33224293864769550 ) ) ;
#10095=CARTESIAN_POINT ( 'NONE',  ( 8.314922557960818139, 14.29746914071049879, 114.5822429386477097 ) ) ;
#10096=CARTESIAN_POINT ( 'NONE',  ( 10.72451020669898902, -18.67979575497178502, 112.9155762719810383 ) ) ;
#10097=CARTESIAN_POINT ( 'NONE',  ( 19.03943276465977164, -0.05219959533909143690, 33.74890960531435979 ) ) ;
#10098=CARTESIAN_POINT ( 'NONE',  ( -13.89961937509977652, 13.97604488694528158, 105.6239096053143527 ) ) ;
#10099=CARTESIAN_POINT ( 'NONE',  ( 18.67979575497194134, -10.72451020669871369, 30.83442372801902209 ) ) ;
#10101=CARTESIAN_POINT ( 'NONE',  ( -16.51473224551069308, -9.474510206698971260, 106.6655762719810383 ) ) ;
#10102=CARTESIAN_POINT ( 'NONE',  ( 17.40805194822032220, -6.112264579159320199, 113.3337127251061389 ) ) ;
#10103=CARTESIAN_POINT ( 'NONE',  ( 16.51473224551069308, 9.474510206698969483, 94.16557627198103830 ) ) ;
#10104=CARTESIAN_POINT ( 'NONE',  ( 21.53943276465977519, 0.05219959533937863772, 51.25109039468568994 ) ) ;
#10105=CARTESIAN_POINT ( 'NONE',  ( -8.224510206698948167, 14.34966873604960824, 95.41557627198102409 ) ) ;
#10106=CARTESIAN_POINT ( 'NONE',  ( 16.46253265017160672, -9.564922557960803928, 98.33224293864769550 ) ) ;
#10108=CARTESIAN_POINT ( 'NONE',  ( -4.483927247898782831, 16.52544592524335698, 62.70942372801902565 ) ) ;
#10109=CARTESIAN_POINT ( 'NONE',  ( -5.719274019375665041, -21.55341960407619695, 79.79275706135236135 ) ) ;
#10110=CARTESIAN_POINT ( 'NONE',  ( -16.53943276465976808, -0.05219959533934237506, 43.75109039468568284 ) ) ;
#10111=CARTESIAN_POINT ( 'NONE',  ( 9.564922557960805705, 16.46253265017160317, 79.58224293864769550 ) ) ;
#10112=CARTESIAN_POINT ( 'NONE',  ( 19.05341960407617918, -5.049401038297876454, 111.0427570613523329 ) ) ;
#10113=CARTESIAN_POINT ( 'NONE',  ( 12.06949235617739724, 12.14591786802326823, 66.87609039468568994 ) ) ;
#10114=CARTESIAN_POINT ( 'NONE',  ( -10.72451020669870658, -18.67979575497194134, 104.5844237280190185 ) ) ;
#10115=CARTESIAN_POINT ( 'NONE',  ( 9.564922557961047289, -16.46253265017146816, 95.41775706135233293 ) ) ;
#10116=CARTESIAN_POINT ( 'NONE',  ( -16.46253265017160317, 9.564922557960807481, 65.83224293864769550 ) ) ;
#10117=CARTESIAN_POINT ( 'NONE',  ( -21.53943276465977519, 0.05219959533907696930, 86.24890960531436690 ) ) ;
#10118=CARTESIAN_POINT ( 'NONE',  ( -16.52544592524342804, 4.483927247898546575, 96.04057627198102409 ) ) ;
#10119=CARTESIAN_POINT ( 'NONE',  ( 16.46253265017146816, 9.564922557961045513, 96.66775706135233293 ) ) ;
#10120=CARTESIAN_POINT ( 'NONE',  ( 16.55341960407618274, -4.379528057220086978, 66.04275706135236135 ) ) ;
#10122=CARTESIAN_POINT ( 'NONE',  ( 16.51473224551083163, -9.474510206698727899, 55.83442372801899722 ) ) ;
#10123=CARTESIAN_POINT ( 'NONE',  ( 16.55341960407611168, 4.379528057220329451, 28.95724293864769905 ) ) ;
#10124=CARTESIAN_POINT ( 'NONE',  ( 16.55341960407611168, 4.379528057220329451, 83.95724293864770971 ) ) ;
#10125=CARTESIAN_POINT ( 'NONE',  ( 9.474510206698729675, 16.51473224551082808, 22.08442372801899722 ) ) ;
#10126=CARTESIAN_POINT ( 'NONE',  ( -17.50000000001356781, 5.500000000000039968, 40.79690382535057580 ) ) ;
#10127=CARTESIAN_POINT ( 'NONE',  ( 18.62759615963255655, 10.81492255796105972, 26.66775706135235424 ) ) ;
#10128=CARTESIAN_POINT ( 'NONE',  ( -5.049401038298153566, 19.05341960407611168, 105.2072429386476671 ) ) ;
#10129=CARTESIAN_POINT ( 'NONE',  ( 5.049401038298161559, -19.05341960407611168, 82.70724293864770971 ) ) ;
#10130=CARTESIAN_POINT ( 'NONE',  ( 21.53943276465977519, 0.05219959533937863772, 101.2510903946856757 ) ) ;
#10131=CARTESIAN_POINT ( 'NONE',  ( -9.474510206698964154, 16.51473224551069663, 75.41557627198103830 ) ) ;
#10132=CARTESIAN_POINT ( 'NONE',  ( -10.72451020669898014, 18.67979575497178502, 45.41557627198103830 ) ) ;
#10133=CARTESIAN_POINT ( 'NONE',  ( 14.34966873604960469, 8.224510206698951720, 84.16557627198103830 ) ) ;
#10134=CARTESIAN_POINT ( 'NONE',  ( -16.51473224551069308, -9.474510206698971260, 61.66557627198103120 ) ) ;
#10135=CARTESIAN_POINT ( 'NONE',  ( 12.14591786802309770, 12.06949235617756955, 94.37390960531436690 ) ) ;
#10136=CARTESIAN_POINT ( 'NONE',  ( 10.72451020669898902, -18.67979575497178502, 107.9155762719810241 ) ) ;
#10137=CARTESIAN_POINT ( 'NONE',  ( -18.67979575497193778, 10.72451020669871902, 63.33442372801900433 ) ) ;
#10138=CARTESIAN_POINT ( 'NONE',  ( -13.89961937509977652, 13.97604488694528158, 30.62390960531435269 ) ) ;
#10140=CARTESIAN_POINT ( 'NONE',  ( -16.55341960407617563, 4.379528057220093196, 68.54275706135234714 ) ) ;
#10141=CARTESIAN_POINT ( 'NONE',  ( 21.55341960407619695, -5.719274019375665929, 21.04275706135234714 ) ) ;
#10142=CARTESIAN_POINT ( 'NONE',  ( 10.81492255796078972, 18.62759615963270932, 109.5822429386476955 ) ) ;
#10143=CARTESIAN_POINT ( 'NONE',  ( 0.05219959533936267826, -19.03943276465977164, 45.00109039468566863 ) ) ;
#10144=CARTESIAN_POINT ( 'NONE',  ( 16.51473224551069308, 9.474510206698969483, 49.16557627198102409 ) ) ;
#10146=CARTESIAN_POINT ( 'NONE',  ( 18.67979575497194134, -10.72451020669871369, 65.83442372801900433 ) ) ;
#10147=CARTESIAN_POINT ( 'NONE',  ( 18.67979575497178502, 10.72451020669898547, 54.16557627198103120 ) ) ;
#10148=CARTESIAN_POINT ( 'NONE',  ( 16.55341960407611168, 4.379528057220329451, 33.95724293864769550 ) ) ;
#10149=CARTESIAN_POINT ( 'NONE',  ( 21.55341960407619695, -5.719274019375665929, 81.04275706135236135 ) ) ;
#10150=CARTESIAN_POINT ( 'NONE',  ( 5.823673210054444382, -21.52544592524334988, 105.2094237280190328 ) ) ;
#10151=CARTESIAN_POINT ( 'NONE',  ( -4.483927247898539470, -16.52544592524342804, 62.29057627198102409 ) ) ;
#10152=CARTESIAN_POINT ( 'NONE',  ( 4.483927247898545687, 16.52544592524342804, 109.7905762719810383 ) ) ;
#10153=CARTESIAN_POINT ( 'NONE',  ( -0.05219959533936034679, 19.03943276465977164, 47.50109039468566863 ) ) ;
#10154=CARTESIAN_POINT ( 'NONE',  ( -12.06949235617739369, -12.14591786802326823, 109.3760903946857042 ) ) ;
#10155=CARTESIAN_POINT ( 'NONE',  ( 5.823673210054444382, -21.52544592524334988, 70.20942372801904696 ) ) ;
#10156=CARTESIAN_POINT ( 'NONE',  ( -16.51473224551069308, -9.474510206698971260, 56.66557627198103120 ) ) ;
#10157=CARTESIAN_POINT ( 'NONE',  ( -19.02544592524334988, -5.153800228976617603, 33.95942372801897591 ) ) ;
#10158=CARTESIAN_POINT ( 'NONE',  ( -10.81492255796078084, -18.62759615963271287, 32.08224293864769550 ) ) ;
#10159=CARTESIAN_POINT ( 'NONE',  ( -5.823673210054431948, 21.52544592524334988, 32.70942372801900433 ) ) ;
#10160=CARTESIAN_POINT ( 'NONE',  ( 10.72451020669898902, -18.67979575497178502, 87.91557627198103830 ) ) ;
#10161=CARTESIAN_POINT ( 'NONE',  ( 19.02544592524334988, 5.153800228976608722, 86.45942372801900433 ) ) ;
#10162=CARTESIAN_POINT ( 'NONE',  ( -14.29746914071037622, -8.314922557961029526, 59.16775706135234714 ) ) ;
#10164=CARTESIAN_POINT ( 'NONE',  ( 5.719274019375991003, -21.55341960407610458, 87.70724293864769550 ) ) ;
#10165=CARTESIAN_POINT ( 'NONE',  ( -14.29746914071049879, 8.314922557960819915, 90.83224293864769550 ) ) ;
#10167=CARTESIAN_POINT ( 'NONE',  ( -8.224510206698735004, -14.34966873604973081, 19.58442372801901143 ) ) ;
#10168=CARTESIAN_POINT ( 'NONE',  ( -21.52544592524343514, 5.823673210054127303, 46.04057627198103830 ) ) ;
#10169=CARTESIAN_POINT ( 'NONE',  ( -4.379528057220086978, -16.55341960407618274, 79.79275706135236135 ) ) ;
#10170=LINE ( 'NONE', #71830, #164109 ) ;
#10171=CARTESIAN_POINT ( 'NONE',  ( -14.34966873604972548, 8.224510206698743886, 53.33442372801901854 ) ) ;
#10172=CARTESIAN_POINT ( 'NONE',  ( 0.05219959533937995610, -21.53943276465977519, 30.00109039468568284 ) ) ;
#10173=CARTESIAN_POINT ( 'NONE',  ( 21.52544592524344225, -5.823673210054117533, 48.54057627198103120 ) ) ;
#10174=CARTESIAN_POINT ( 'NONE',  ( 4.379528057220092307, 16.55341960407617563, 72.29275706135236135 ) ) ;
#10175=CARTESIAN_POINT ( 'NONE',  ( 19.05341960407611168, 5.049401038298154454, 93.95724293864769550 ) ) ;
#10176=CARTESIAN_POINT ( 'NONE',  ( 0.05219959533937995610, -21.53943276465977519, 60.00109039468568284 ) ) ;
#10177=CARTESIAN_POINT ( 'NONE',  ( -5.153800228976328057, -19.02544592524343514, 22.29057627198102765 ) ) ;
#10178=CARTESIAN_POINT ( 'NONE',  ( -0.05219959533907301413, -21.53943276465977519, 37.49890960531436690 ) ) ;
#10179=CARTESIAN_POINT ( 'NONE',  ( 21.52544592524344225, -5.823673210054117533, 23.54057627198102765 ) ) ;
#10181=CARTESIAN_POINT ( 'NONE',  ( 19.03943276465977164, 0.05219959533936151252, 41.25109039468566152 ) ) ;
#10182=CARTESIAN_POINT ( 'NONE',  ( -8.314922557961024197, 14.29746914071037800, 47.91775706135234714 ) ) ;
#10183=CARTESIAN_POINT ( 'NONE',  ( 16.46253265017160672, -9.564922557960803928, 113.3322429386476955 ) ) ;
#10184=VERTEX_POINT ( 'NONE', #31732 ) ;
#10185=CARTESIAN_POINT ( 'NONE',  ( 19.03943276465977164, -0.05219959533909143690, 83.74890960531436690 ) ) ;
#10186=CARTESIAN_POINT ( 'NONE',  ( 16.55341960407618274, -4.379528057220086978, 96.04275706135236135 ) ) ;
#10188=CARTESIAN_POINT ( 'NONE',  ( -14.29746914071049879, 8.314922557960819915, 90.83224293864769550 ) ) ;
#10189=CARTESIAN_POINT ( 'NONE',  ( 0.05219959533907565091, 21.53943276465977519, 54.99890960531435269 ) ) ;
#10190=CARTESIAN_POINT ( 'NONE',  ( -16.51473224551069308, -9.474510206698971260, 31.66557627198102054 ) ) ;
#10191=CARTESIAN_POINT ( 'NONE',  ( 16.55341960407618274, -4.379528057220086978, 71.04275706135234714 ) ) ;
#10192=CARTESIAN_POINT ( 'NONE',  ( -15.72974639402176322, -15.80617190586768395, 29.37609039468568284 ) ) ;
#10193=CARTESIAN_POINT ( 'NONE',  ( 13.89961937509957401, 13.97604488694547697, 86.87609039468567573 ) ) ;
#10194=CARTESIAN_POINT ( 'NONE',  ( -19.03943276465977164, 0.05219959533909376836, 36.24890960531436690 ) ) ;
#10195=CARTESIAN_POINT ( 'NONE',  ( -0.05219959533909027116, -19.03943276465977164, 107.4989096053143527 ) ) ;
#10196=CARTESIAN_POINT ( 'NONE',  ( -10.72451020669870658, -18.67979575497194134, 109.5844237280190328 ) ) ;
#10197=CARTESIAN_POINT ( 'NONE',  ( 13.97604488694527802, 13.89961937509977652, 84.37390960531433848 ) ) ;
#10198=CARTESIAN_POINT ( 'NONE',  ( -16.53943276465976808, -0.05219959533934237506, 68.75109039468568994 ) ) ;
#10199=CARTESIAN_POINT ( 'NONE',  ( -5.823673210054431948, 21.52544592524334988, 92.70942372801901854 ) ) ;
#10200=CARTESIAN_POINT ( 'NONE',  ( 0.05219959533936267826, -19.03943276465977164, 50.00109039468566863 ) ) ;
#10201=CARTESIAN_POINT ( 'NONE',  ( 13.89961937509957401, 13.97604488694547697, 66.87609039468567573 ) ) ;
#10203=CARTESIAN_POINT ( 'NONE',  ( 15.72974639402176855, 15.80617190586768217, 66.87609039468568994 ) ) ;
#10204=CARTESIAN_POINT ( 'NONE',  ( 16.46253265017160672, -9.564922557960803928, 63.33224293864769550 ) ) ;
#10205=CARTESIAN_POINT ( 'NONE',  ( -16.51473224551069308, -9.474510206698971260, 26.66557627198103120 ) ) ;
#10206=CARTESIAN_POINT ( 'NONE',  ( 5.049401038297881783, 19.05341960407617563, 57.29275706135231871 ) ) ;
#10207=CARTESIAN_POINT ( 'NONE',  ( 9.474510206698971260, -16.51473224551069308, 112.9155762719810383 ) ) ;
#10208=CARTESIAN_POINT ( 'NONE',  ( 5.153800228976335163, 19.02544592524342804, 84.79057627198099567 ) ) ;
#10209=CARTESIAN_POINT ( 'NONE',  ( 14.29746914071049879, -8.314922557960816363, 33.33224293864769550 ) ) ;
#10210=CARTESIAN_POINT ( 'NONE',  ( -21.53943276465977519, 0.05219959533907696930, 31.24890960531435979 ) ) ;
#10211=CARTESIAN_POINT ( 'NONE',  ( -17.72662750342726667, -5.499999999999959144, 96.40179492283743912 ) ) ;
#10212=CARTESIAN_POINT ( 'NONE',  ( -0.05219959533936034679, 19.03943276465977164, 22.50109039468566152 ) ) ;
#10214=CARTESIAN_POINT ( 'NONE',  ( 19.03943276465977164, -0.05219959533909143690, 43.74890960531435979 ) ) ;
#10215=CARTESIAN_POINT ( 'NONE',  ( -16.46253265017160317, 9.564922557960807481, 85.83224293864769550 ) ) ;
#10217=CARTESIAN_POINT ( 'NONE',  ( -15.80617190586768217, 15.72974639402176855, 68.12609039468567573 ) ) ;
#10219=CARTESIAN_POINT ( 'NONE',  ( -16.53943276465976808, -0.05219959533934237506, 58.75109039468568994 ) ) ;
#10220=CARTESIAN_POINT ( 'NONE',  ( 5.823673210054125526, 21.52544592524343514, 79.79057627198102409 ) ) ;
#10221=CARTESIAN_POINT ( 'NONE',  ( -4.379528057220328563, 16.55341960407611168, 50.20724293864769550 ) ) ;
#10222=CARTESIAN_POINT ( 'NONE',  ( 19.03943276465977164, -0.05219959533909143690, 33.74890960531435979 ) ) ;
#10223=CARTESIAN_POINT ( 'NONE',  ( 19.02544592524343514, -5.153800228976328945, 113.5405762719810241 ) ) ;
#10224=CARTESIAN_POINT ( 'NONE',  ( 21.55341960407619695, -5.719274019375665929, 26.04275706135235779 ) ) ;
#10225=CARTESIAN_POINT ( 'NONE',  ( -16.51473224551082808, 9.474510206698731452, 43.33442372801900433 ) ) ;
#10226=CARTESIAN_POINT ( 'NONE',  ( -19.03943276465977164, 0.05219959533909376836, 31.24890960531435979 ) ) ;
#10227=CARTESIAN_POINT ( 'NONE',  ( 5.823673210054444382, -21.52544592524334988, 80.20942372801901854 ) ) ;
#10228=CARTESIAN_POINT ( 'NONE',  ( 16.31925111598458855, -7.325300261831445781, 32.66424538967252289 ) ) ;
#10229=CARTESIAN_POINT ( 'NONE',  ( 4.483927247898545687, 16.52544592524342804, 24.79057627198103120 ) ) ;
#10231=CARTESIAN_POINT ( 'NONE',  ( 10.81492255796078972, 18.62759615963270932, 44.58224293864769550 ) ) ;
#10233=CARTESIAN_POINT ( 'NONE',  ( -13.89961937509977652, 13.97604488694528158, 95.62390960531436690 ) ) ;
#10234=CARTESIAN_POINT ( 'NONE',  ( 16.52544592524342804, -4.483927247898539470, 93.54057627198103830 ) ) ;
#10235=CARTESIAN_POINT ( 'NONE',  ( 9.474510206698729675, 16.51473224551082808, 112.0844237280190043 ) ) ;
#10236=CARTESIAN_POINT ( 'NONE',  ( -10.81492255796078084, -18.62759615963271287, 67.08224293864770971 ) ) ;
#10238=CARTESIAN_POINT ( 'NONE',  ( 0.05219959533909260263, 19.03943276465977164, 29.99890960531435979 ) ) ;
#10239=EDGE_CURVE ( 'NONE', #176032, #199255, #155066, .T. ) ;
#10240=CARTESIAN_POINT ( 'NONE',  ( 5.049401038298161559, -19.05341960407611168, 82.70724293864770971 ) ) ;
#10241=CARTESIAN_POINT ( 'NONE',  ( -21.55341960407610458, -5.719274019375992779, 86.45724293864770971 ) ) ;
#10242=CARTESIAN_POINT ( 'NONE',  ( 14.29746914071037800, 8.314922557961029526, 111.6677570613523613 ) ) ;
#10243=CARTESIAN_POINT ( 'NONE',  ( -19.02544592524342804, 5.153800228976336051, 106.0405762719810241 ) ) ;
#10244=CARTESIAN_POINT ( 'NONE',  ( 5.049401038297881783, 19.05341960407617563, 77.29275706135231871 ) ) ;
#10245=CARTESIAN_POINT ( 'NONE',  ( -10.81492255796105439, 18.62759615963255655, 92.91775706135236135 ) ) ;
#10246=CARTESIAN_POINT ( 'NONE',  ( -18.62759615963270932, 10.81492255796079327, 80.83224293864769550 ) ) ;
#10247=CARTESIAN_POINT ( 'NONE',  ( 0.05219959533907565091, 21.53943276465977519, 39.99890960531436690 ) ) ;
#10248=CARTESIAN_POINT ( 'NONE',  ( -13.89961937509977652, 13.97604488694528158, 50.62390960531435979 ) ) ;
#10249=CARTESIAN_POINT ( 'NONE',  ( 4.483927247898545687, 16.52544592524342804, 24.79057627198103120 ) ) ;
#10250=CARTESIAN_POINT ( 'NONE',  ( 13.97604488694527802, 13.89961937509977652, 69.37390960531436690 ) ) ;
#10253=CARTESIAN_POINT ( 'NONE',  ( 0.05219959533936267826, -19.03943276465977164, 25.00109039468566152 ) ) ;
#10254=CARTESIAN_POINT ( 'NONE',  ( 16.53943276465976808, -0.05219959533910856209, 78.74890960531436690 ) ) ;
#10255=CARTESIAN_POINT ( 'NONE',  ( 5.823673210054444382, -21.52544592524334988, 30.20942372801902565 ) ) ;
#10257=CARTESIAN_POINT ( 'NONE',  ( -18.62759615963270932, 10.81492255796079327, 60.83224293864769550 ) ) ;
#10258=CARTESIAN_POINT ( 'NONE',  ( 0.05219959533934541429, -16.53943276465976808, 100.0010903946857042 ) ) ;
#10259=CARTESIAN_POINT ( 'NONE',  ( -12.06949235617756955, 12.14591786802309770, 110.6239096053143669 ) ) ;
#10260=CARTESIAN_POINT ( 'NONE',  ( 19.03943276465977164, -0.05219959533909143690, 68.74890960531436690 ) ) ;
#10263=CARTESIAN_POINT ( 'NONE',  ( 16.52544592524342804, -4.483927247898539470, 33.54057627198102409 ) ) ;
#10264=CARTESIAN_POINT ( 'NONE',  ( 5.823673210054444382, -21.52544592524334988, 45.20942372801901854 ) ) ;
#10265=CARTESIAN_POINT ( 'NONE',  ( 16.51473224551069308, 9.474510206698969483, 109.1655762719810383 ) ) ;
#10266=CARTESIAN_POINT ( 'NONE',  ( 15.80617190586769283, -15.72974639402175789, 80.62609039468567573 ) ) ;
#10267=CARTESIAN_POINT ( 'NONE',  ( 9.474510206698971260, -16.51473224551069308, 32.91557627198102409 ) ) ;
#10268=CARTESIAN_POINT ( 'NONE',  ( 5.049401038298161559, -19.05341960407611168, 42.70724293864767418 ) ) ;
#10270=CARTESIAN_POINT ( 'NONE',  ( -5.719274019375665041, -21.55341960407619695, 99.79275706135234714 ) ) ;
#10271=CARTESIAN_POINT ( 'NONE',  ( 0.05219959533934541429, -16.53943276465976808, 50.00109039468568994 ) ) ;
#10272=CARTESIAN_POINT ( 'NONE',  ( 15.80617190586769283, -15.72974639402175789, 80.62609039468567573 ) ) ;
#10273=CARTESIAN_POINT ( 'NONE',  ( 16.46253265017160672, -9.564922557960803928, 108.3322429386476955 ) ) ;
#10274=CARTESIAN_POINT ( 'NONE',  ( -16.51473224551082808, 9.474510206698731452, 88.33442372801900433 ) ) ;
#10275=CARTESIAN_POINT ( 'NONE',  ( 18.67979575497194134, -10.72451020669871369, 55.83442372801901854 ) ) ;
#10276=CARTESIAN_POINT ( 'NONE',  ( 12.14591786802327356, -12.06949235617739191, 25.62609039468567929 ) ) ;
#10277=CARTESIAN_POINT ( 'NONE',  ( -13.97604488694547697, 13.89961937509957934, 88.12609039468563310 ) ) ;
#10278=CARTESIAN_POINT ( 'NONE',  ( -16.51473224551069308, -9.474510206698971260, 46.66557627198102409 ) ) ;
#10279=CARTESIAN_POINT ( 'NONE',  ( -0.05219959533936034679, 19.03943276465977164, 92.50109039468566152 ) ) ;
#10281=CARTESIAN_POINT ( 'NONE',  ( -12.06949235617756955, 12.14591786802309770, 25.62390960531435624 ) ) ;
#10282=CARTESIAN_POINT ( 'NONE',  ( 5.049401038297881783, 19.05341960407617563, 87.29275706135234714 ) ) ;
#10283=CARTESIAN_POINT ( 'NONE',  ( 8.224510206698953496, -14.34966873604960469, 47.91557627198102409 ) ) ;
#10284=CARTESIAN_POINT ( 'NONE',  ( 9.564922557961047289, -16.46253265017146816, 65.41775706135233293 ) ) ;
#10285=CARTESIAN_POINT ( 'NONE',  ( 14.29746914071037800, 8.314922557961029526, 66.66775706135234714 ) ) ;
#10286=CARTESIAN_POINT ( 'NONE',  ( -16.46253265017146816, -9.564922557961047289, 19.16775706135233293 ) ) ;
#10287=CARTESIAN_POINT ( 'NONE',  ( -12.06949235617756955, 12.14591786802309770, 115.6239096053143669 ) ) ;
#10288=CARTESIAN_POINT ( 'NONE',  ( -19.03943276465977164, 0.05219959533909376836, 36.24890960531436690 ) ) ;
#10289=CARTESIAN_POINT ( 'NONE',  ( 16.52544592524335698, 4.483927247898782831, 56.45942372801902565 ) ) ;
#10293=CARTESIAN_POINT ( 'NONE',  ( 16.46253265017160672, -9.564922557960803928, 108.3322429386476955 ) ) ;
#10296=CARTESIAN_POINT ( 'NONE',  ( 16.51473224551083163, -9.474510206698727899, 95.83442372801900433 ) ) ;
#10297=CARTESIAN_POINT ( 'NONE',  ( 5.823673210054125526, 21.52544592524343514, 39.79057627198103830 ) ) ;
#10298=CARTESIAN_POINT ( 'NONE',  ( 19.02544592524334988, 5.153800228976608722, 26.45942372801899722 ) ) ;
#10299=CARTESIAN_POINT ( 'NONE',  ( -19.03943276465977164, -0.05219959533935918106, 113.7510903946856757 ) ) ;
#10300=CARTESIAN_POINT ( 'NONE',  ( 8.314922557960818139, 14.29746914071049879, 109.5822429386476955 ) ) ;
#10301=CARTESIAN_POINT ( 'NONE',  ( -19.02544592524342804, 5.153800228976336051, 36.04057627198100988 ) ) ;
#10302=CARTESIAN_POINT ( 'NONE',  ( -0.05219959533907301413, -21.53943276465977519, 72.49890960531435269 ) ) ;
#10303=CARTESIAN_POINT ( 'NONE',  ( -16.46253265017160317, 9.564922557960807481, 30.83224293864769550 ) ) ;
#10305=CARTESIAN_POINT ( 'NONE',  ( 19.02544592524334988, 5.153800228976608722, 81.45942372801897591 ) ) ;
#10306=CARTESIAN_POINT ( 'NONE',  ( 4.483927247898545687, 16.52544592524342804, 54.79057627198104541 ) ) ;
#10307=CARTESIAN_POINT ( 'NONE',  ( -18.67979575497178146, -10.72451020669898902, 31.66557627198102054 ) ) ;
#10308=CARTESIAN_POINT ( 'NONE',  ( -10.81492255796105439, 18.62759615963255655, 97.91775706135236135 ) ) ;
#10309=CARTESIAN_POINT ( 'NONE',  ( 5.719274019375991003, -21.55341960407610458, 87.70724293864769550 ) ) ;
#10310=CARTESIAN_POINT ( 'NONE',  ( -10.72451020669870658, -18.67979575497194134, 74.58442372801901854 ) ) ;
#10311=CARTESIAN_POINT ( 'NONE',  ( 5.823673210054444382, -21.52544592524334988, 60.20942372801902565 ) ) ;
#10312=CARTESIAN_POINT ( 'NONE',  ( 13.97604488694527802, 13.89961937509977652, 104.3739096053143385 ) ) ;
#10313=CARTESIAN_POINT ( 'NONE',  ( 8.314922557961029526, -14.29746914071037800, 100.4177570613523471 ) ) ;
#10314=CARTESIAN_POINT ( 'NONE',  ( -5.823673210054431948, 21.52544592524334988, 67.70942372801901854 ) ) ;
#10315=CARTESIAN_POINT ( 'NONE',  ( 5.153800228976335163, 19.02544592524342804, 54.79057627198103120 ) ) ;
#10316=CARTESIAN_POINT ( 'NONE',  ( -9.474510206698720793, -16.51473224551083518, 39.58442372801899722 ) ) ;
#10317=CARTESIAN_POINT ( 'NONE',  ( -21.53943276465977519, -0.05219959533937600094, 23.75109039468567929 ) ) ;
#10318=CARTESIAN_POINT ( 'NONE',  ( 13.97604488694527802, 13.89961937509977652, 64.37390960531436690 ) ) ;
#10319=CARTESIAN_POINT ( 'NONE',  ( -16.53943276465976808, 0.05219959533911058130, 81.24890960531436690 ) ) ;
#10320=CARTESIAN_POINT ( 'NONE',  ( -16.55341960407611168, -4.379528057220339221, 46.45724293864769550 ) ) ;
#10321=CARTESIAN_POINT ( 'NONE',  ( 21.55341960407610458, 5.719274019375980345, 58.95724293864770971 ) ) ;
#10322=CARTESIAN_POINT ( 'NONE',  ( -13.89961937509977652, 13.97604488694528158, 45.62390960531433848 ) ) ;
#10323=CARTESIAN_POINT ( 'NONE',  ( 10.72451020669898902, -18.67979575497178502, 72.91557627198103830 ) ) ;
#10324=CARTESIAN_POINT ( 'NONE',  ( 19.05341960407617918, -5.049401038297876454, 56.04275706135234714 ) ) ;
#10325=CARTESIAN_POINT ( 'NONE',  ( -16.51473224551082808, 9.474510206698731452, 23.33442372801900078 ) ) ;
#10326=CARTESIAN_POINT ( 'NONE',  ( 16.53943276465976808, -0.05219959533910856209, 68.74890960531435269 ) ) ;
#10327=CARTESIAN_POINT ( 'NONE',  ( -15.72974639402197994, 15.80617190586746368, 40.62390960531435269 ) ) ;
#10329=CARTESIAN_POINT ( 'NONE',  ( 16.36317988757058473, 7.306389748694926745, 103.4021039163677642 ) ) ;
#10330=CARTESIAN_POINT ( 'NONE',  ( -0.05219959533934338120, 16.53943276465976808, 82.50109039468568994 ) ) ;
#10332=CARTESIAN_POINT ( 'NONE',  ( -0.05219959533936034679, 19.03943276465977164, 87.50109039468567573 ) ) ;
#10333=EDGE_CURVE ( 'NONE', #90405, #14227, #118471, .T. ) ;
#10334=CARTESIAN_POINT ( 'NONE',  ( 16.53943276465976808, -0.05219959533910856209, 48.74890960531435979 ) ) ;
#10335=CARTESIAN_POINT ( 'NONE',  ( -19.35543954521081744, -5.499999999999585221, 59.58901960356450900 ) ) ;
#10336=CARTESIAN_POINT ( 'NONE',  ( -9.474510206698964154, 16.51473224551069663, 50.41557627198102409 ) ) ;
#10337=CARTESIAN_POINT ( 'NONE',  ( -4.379528057220328563, 16.55341960407611168, 45.20724293864769550 ) ) ;
#10338=CARTESIAN_POINT ( 'NONE',  ( 9.474510206698971260, -16.51473224551069308, 92.91557627198103830 ) ) ;
#10339=CARTESIAN_POINT ( 'NONE',  ( 13.97604488694527802, 13.89961937509977652, 49.37390960531434558 ) ) ;
#10340=CARTESIAN_POINT ( 'NONE',  ( -21.55341960407619339, 5.719274019375674811, 58.54275706135235424 ) ) ;
#10341=CARTESIAN_POINT ( 'NONE',  ( 13.97604488694527802, 13.89961937509977652, 69.37390960531436690 ) ) ;
#10342=CARTESIAN_POINT ( 'NONE',  ( -16.46253265017160317, 9.564922557960807481, 25.83224293864769194 ) ) ;
#10343=CARTESIAN_POINT ( 'NONE',  ( 5.153800228976335163, 19.02544592524342804, 59.79057627198100988 ) ) ;
#10344=CARTESIAN_POINT ( 'NONE',  ( 18.67979575497178502, 10.72451020669898547, 49.16557627198102409 ) ) ;
#10345=CARTESIAN_POINT ( 'NONE',  ( -16.51473224551069308, -9.474510206698971260, 41.66557627198103120 ) ) ;
#10346=CARTESIAN_POINT ( 'NONE',  ( -18.62759615963270932, 10.81492255796079327, 40.83224293864769550 ) ) ;
#10347=CARTESIAN_POINT ( 'NONE',  ( 12.14591786802327356, -12.06949235617739191, 105.6260903946856899 ) ) ;
#10348=CARTESIAN_POINT ( 'NONE',  ( -13.97604488694547697, 13.89961937509957934, 23.12609039468565442 ) ) ;
#10349=CARTESIAN_POINT ( 'NONE',  ( -4.379528057220086978, -16.55341960407618274, 49.79275706135234714 ) ) ;
#10350=CARTESIAN_POINT ( 'NONE',  ( -14.34966873604972548, 8.224510206698743886, 83.33442372801903275 ) ) ;
#10352=CARTESIAN_POINT ( 'NONE',  ( 16.52544592524335698, 4.483927247898782831, 61.45942372801901854 ) ) ;
#10353=CARTESIAN_POINT ( 'NONE',  ( 8.224510206698742110, 14.34966873604972548, 47.08442372801901854 ) ) ;
#10354=CARTESIAN_POINT ( 'NONE',  ( 16.46253265017160672, -9.564922557960803928, 108.3322429386476955 ) ) ;
#10355=CARTESIAN_POINT ( 'NONE',  ( -13.89961937509977652, 13.97604488694528158, 35.62390960531435269 ) ) ;
#10356=CARTESIAN_POINT ( 'NONE',  ( -12.14591786802326823, 12.06949235617739902, 33.12609039468569705 ) ) ;
#10357=CARTESIAN_POINT ( 'NONE',  ( -16.46253265017160317, 9.564922557960807481, 45.83224293864769550 ) ) ;
#10358=CARTESIAN_POINT ( 'NONE',  ( -15.80617190586768217, 15.72974639402176855, 28.12609039468568284 ) ) ;
#10359=CARTESIAN_POINT ( 'NONE',  ( -12.06949235617739369, -12.14591786802326823, 39.37609039468567573 ) ) ;
#10360=CARTESIAN_POINT ( 'NONE',  ( -12.14591786802326823, 12.06949235617739902, 93.12609039468568994 ) ) ;
#10362=CARTESIAN_POINT ( 'NONE',  ( -21.55341960407619339, 5.719274019375674811, 103.5427570613523613 ) ) ;
#10363=CARTESIAN_POINT ( 'NONE',  ( 13.97604488694548053, -13.89961937509957401, 100.6260903946856615 ) ) ;
#10364=CARTESIAN_POINT ( 'NONE',  ( 0.05219959533936267826, -19.03943276465977164, 60.00109039468566863 ) ) ;
#10365=CARTESIAN_POINT ( 'NONE',  ( 14.29746914071049879, -8.314922557960816363, 53.33224293864769550 ) ) ;
#10366=CARTESIAN_POINT ( 'NONE',  ( -19.05341960407611168, -5.049401038298163336, 31.45724293864769550 ) ) ;
#10367=CARTESIAN_POINT ( 'NONE',  ( -5.049401038297874678, -19.05341960407617918, 64.79275706135233293 ) ) ;
#10368=CARTESIAN_POINT ( 'NONE',  ( 16.61371651742601685, 7.165104196376161916, 78.64584930007005426 ) ) ;
#10369=CARTESIAN_POINT ( 'NONE',  ( -15.80617190586768217, 15.72974639402176855, 68.12609039468567573 ) ) ;
#10370=CARTESIAN_POINT ( 'NONE',  ( 4.379528057220092307, 16.55341960407617563, 32.29275706135235424 ) ) ;
#10371=CARTESIAN_POINT ( 'NONE',  ( 17.31728774477273092, 6.344390552232407110, 81.68093348310684121 ) ) ;
#10372=CARTESIAN_POINT ( 'NONE',  ( -13.89961937509977652, 13.97604488694528158, 115.6239096053143669 ) ) ;
#10373=CARTESIAN_POINT ( 'NONE',  ( 13.97604488694548053, -13.89961937509957401, 110.6260903946856615 ) ) ;
#10374=CARTESIAN_POINT ( 'NONE',  ( 5.153800228976335163, 19.02544592524342804, 109.7905762719810099 ) ) ;
#10376=CARTESIAN_POINT ( 'NONE',  ( -5.153800228976328057, -19.02544592524343514, 27.29057627198103120 ) ) ;
#10377=CARTESIAN_POINT ( 'NONE',  ( 21.52544592524334988, 5.823673210054432836, 111.4594237280190328 ) ) ;
#10378=CARTESIAN_POINT ( 'NONE',  ( 0.05219959533909260263, 19.03943276465977164, 44.99890960531435979 ) ) ;
#10379=CARTESIAN_POINT ( 'NONE',  ( -10.72451020669870658, -18.67979575497194134, 64.58442372801900433 ) ) ;
#10380=CARTESIAN_POINT ( 'NONE',  ( -21.53943276465977519, -0.05219959533937600094, 103.7510903946857042 ) ) ;
#10381=CARTESIAN_POINT ( 'NONE',  ( 4.379528057220092307, 16.55341960407617563, 107.2927570613523471 ) ) ;
#10382=CARTESIAN_POINT ( 'NONE',  ( 9.474510206698971260, -16.51473224551069308, 82.91557627198103830 ) ) ;
#10383=CARTESIAN_POINT ( 'NONE',  ( 21.55341960407619695, -5.719274019375665929, 51.04275706135234714 ) ) ;
#10384=CARTESIAN_POINT ( 'NONE',  ( -21.53943276465977519, -0.05219959533937600094, 58.75109039468568994 ) ) ;
#10385=CARTESIAN_POINT ( 'NONE',  ( -16.51473224551082808, 9.474510206698731452, 73.33442372801900433 ) ) ;
#10386=CARTESIAN_POINT ( 'NONE',  ( -5.153800228976328057, -19.02544592524343514, 102.2905762719810383 ) ) ;
#10387=CARTESIAN_POINT ( 'NONE',  ( 14.29746914071049879, -8.314922557960816363, 113.3322429386476955 ) ) ;
#10388=CARTESIAN_POINT ( 'NONE',  ( -15.72974639402197994, 15.80617190586746368, 95.62390960531436690 ) ) ;
#10389=CARTESIAN_POINT ( 'NONE',  ( -13.97604488694547697, 13.89961937509957934, 28.12609039468565797 ) ) ;
#10390=CARTESIAN_POINT ( 'NONE',  ( -14.34966873604960291, -8.224510206698953496, 96.66557627198102409 ) ) ;
#10391=CARTESIAN_POINT ( 'NONE',  ( -16.46253265017160317, 9.564922557960807481, 50.83224293864770260 ) ) ;
#10392=CARTESIAN_POINT ( 'NONE',  ( -0.05219959533936034679, 19.03943276465977164, 82.50109039468567573 ) ) ;
#10393=CARTESIAN_POINT ( 'NONE',  ( -8.224510206698948167, 14.34966873604960824, 60.41557627198102409 ) ) ;
#10394=CARTESIAN_POINT ( 'NONE',  ( -18.67979575497193778, 10.72451020669871902, 103.3344237280190043 ) ) ;
#10395=CARTESIAN_POINT ( 'NONE',  ( 5.153800228976335163, 19.02544592524342804, 109.7905762719810099 ) ) ;
#10396=CARTESIAN_POINT ( 'NONE',  ( 13.97604488694548053, -13.89961937509957401, 70.62609039468567573 ) ) ;
#10397=CARTESIAN_POINT ( 'NONE',  ( -15.72974639402197994, 15.80617190586746368, 75.62390960531439532 ) ) ;
#10398=CARTESIAN_POINT ( 'NONE',  ( -21.55341960407619339, 5.719274019375674811, 28.54275706135234358 ) ) ;
#10399=CARTESIAN_POINT ( 'NONE',  ( 4.483927247898790824, -16.52544592524335698, 35.20942372801901854 ) ) ;
#10400=CARTESIAN_POINT ( 'NONE',  ( -14.29746914071037622, -8.314922557961029526, 89.16775706135236135 ) ) ;
#10401=CARTESIAN_POINT ( 'NONE',  ( -8.314922557961024197, 14.29746914071037800, 47.91775706135234714 ) ) ;
#10402=CARTESIAN_POINT ( 'NONE',  ( 18.62759615963255655, 10.81492255796105972, 36.66775706135234714 ) ) ;
#10403=CARTESIAN_POINT ( 'NONE',  ( 21.52544592524344225, -5.823673210054117533, 43.54057627198103830 ) ) ;
#10404=CARTESIAN_POINT ( 'NONE',  ( -19.03943276465977164, 0.05219959533909376836, 41.24890960531435269 ) ) ;
#10406=CARTESIAN_POINT ( 'NONE',  ( 8.314922557961029526, -14.29746914071037800, 60.41775706135235424 ) ) ;
#10407=CARTESIAN_POINT ( 'NONE',  ( -15.80617190586745835, -15.72974639402198527, 91.87390960531436690 ) ) ;
#10408=CARTESIAN_POINT ( 'NONE',  ( -14.29746914071049879, 8.314922557960819915, 35.83224293864768839 ) ) ;
#10409=CARTESIAN_POINT ( 'NONE',  ( -0.05219959533934338120, 16.53943276465976808, 47.50109039468568994 ) ) ;
#10410=CARTESIAN_POINT ( 'NONE',  ( 0.05219959533909260263, 19.03943276465977164, 59.99890960531436690 ) ) ;
#10411=CARTESIAN_POINT ( 'NONE',  ( -8.224510206698735004, -14.34966873604973081, 89.58442372801901854 ) ) ;
#10412=CARTESIAN_POINT ( 'NONE',  ( -0.05219959533936034679, 19.03943276465977164, 87.50109039468567573 ) ) ;
#10413=CARTESIAN_POINT ( 'NONE',  ( 15.80617190586746368, 15.72974639402197994, 89.37390960531435269 ) ) ;
#10414=CARTESIAN_POINT ( 'NONE',  ( -0.05219959533910754901, -16.53943276465976808, 27.49890960531435269 ) ) ;
#10415=ORIENTED_EDGE ( 'NONE', *, *, #114658, .T. ) ;
#10417=CARTESIAN_POINT ( 'NONE',  ( -21.55341960407610458, -5.719274019375992779, 56.45724293864768839 ) ) ;
#10418=VERTEX_POINT ( 'NONE', #141872 ) ;
#10419=CARTESIAN_POINT ( 'NONE',  ( -8.224510206698735004, -14.34966873604973081, 99.58442372801900433 ) ) ;
#10421=CARTESIAN_POINT ( 'NONE',  ( -5.719274019375978568, 21.55341960407610458, 25.20724293864769550 ) ) ;
#10422=CARTESIAN_POINT ( 'NONE',  ( 17.50000000000000000, -3.270424329311308220, 102.5422648494460987 ) ) ;
#10423=CARTESIAN_POINT ( 'NONE',  ( -10.81492255796078084, -18.62759615963271287, 82.08224293864768129 ) ) ;
#10424=CARTESIAN_POINT ( 'NONE',  ( 8.224510206698742110, 14.34966873604972548, 112.0844237280190185 ) ) ;
#10425=CARTESIAN_POINT ( 'NONE',  ( -8.314922557961024197, 14.29746914071037800, 37.91775706135235424 ) ) ;
#10426=CARTESIAN_POINT ( 'NONE',  ( -5.049401038298153566, 19.05341960407611168, 35.20724293864768839 ) ) ;
#10427=CARTESIAN_POINT ( 'NONE',  ( 4.379528057220092307, 16.55341960407617563, 32.29275706135235424 ) ) ;
#10428=CARTESIAN_POINT ( 'NONE',  ( 13.89961937509977652, -13.97604488694527269, 48.12390960531435979 ) ) ;
#10430=CARTESIAN_POINT ( 'NONE',  ( 0.05219959533907565091, 21.53943276465977519, 24.99890960531435624 ) ) ;
#10431=CARTESIAN_POINT ( 'NONE',  ( 16.51473224551069308, 9.474510206698969483, 114.1655762719810241 ) ) ;
#10432=CARTESIAN_POINT ( 'NONE',  ( 16.52544592524335698, 4.483927247898782831, 106.4594237280190328 ) ) ;
#10433=CARTESIAN_POINT ( 'NONE',  ( -5.153800228976607833, 19.02544592524334988, 87.70942372801897591 ) ) ;
#10434=CARTESIAN_POINT ( 'NONE',  ( -9.564922557961040184, 16.46253265017147172, 42.91775706135234003 ) ) ;
#10435=CARTESIAN_POINT ( 'NONE',  ( -18.67979575497178146, -10.72451020669898902, 91.66557627198103830 ) ) ;
#10436=CARTESIAN_POINT ( 'NONE',  ( -8.224510206698735004, -14.34966873604973081, 109.5844237280190328 ) ) ;
#10437=CARTESIAN_POINT ( 'NONE',  ( -0.05219959533907301413, -21.53943276465977519, 37.49890960531436690 ) ) ;
#10438=CARTESIAN_POINT ( 'NONE',  ( -16.51473224551082808, 9.474510206698731452, 103.3344237280190043 ) ) ;
#10439=CARTESIAN_POINT ( 'NONE',  ( 19.05341960407611168, 5.049401038298154454, 103.9572429386476671 ) ) ;
#10440=CARTESIAN_POINT ( 'NONE',  ( -5.719274019375665041, -21.55341960407619695, 59.79275706135234714 ) ) ;
#10441=CARTESIAN_POINT ( 'NONE',  ( -13.97604488694527625, -13.89961937509977652, 66.87390960531436690 ) ) ;
#10442=CARTESIAN_POINT ( 'NONE',  ( -12.06949235617756955, 12.14591786802309770, 100.6239096053143811 ) ) ;
#10444=CARTESIAN_POINT ( 'NONE',  ( -8.314922557960811034, -14.29746914071050412, 72.08224293864769550 ) ) ;
#10445=EDGE_LOOP ( 'NONE', ( #100057, #148167, #197663, #25841, #94026, #51172, #193489, #48491 ) ) ;
#10446=CARTESIAN_POINT ( 'NONE',  ( 19.03943276465977164, 0.05219959533936151252, 91.25109039468566152 ) ) ;
#10447=CARTESIAN_POINT ( 'NONE',  ( 16.88567814943162659, -6.947325034625689177, 81.20998877347412304 ) ) ;
#10448=CARTESIAN_POINT ( 'NONE',  ( -13.97604488694527625, -13.89961937509977652, 66.87390960531436690 ) ) ;
#10450=CARTESIAN_POINT ( 'NONE',  ( -9.474510206698964154, 16.51473224551069663, 80.41557627198103830 ) ) ;
#10451=CARTESIAN_POINT ( 'NONE',  ( 9.474510206698971260, -16.51473224551069308, 102.9155762719810241 ) ) ;
#10452=CARTESIAN_POINT ( 'NONE',  ( 12.14591786802327356, -12.06949235617739191, 70.62609039468567573 ) ) ;
#10454=CARTESIAN_POINT ( 'NONE',  ( 13.97604488694548053, -13.89961937509957401, 40.62609039468564731 ) ) ;
#10455=CARTESIAN_POINT ( 'NONE',  ( -15.72974639402176322, -15.80617190586768395, 99.37609039468568994 ) ) ;
#10456=CARTESIAN_POINT ( 'NONE',  ( 16.62544781628812274, 7.153289815129877383, 22.00000000000000000 ) ) ;
#10457=CARTESIAN_POINT ( 'NONE',  ( 5.049401038298161559, -19.05341960407611168, 107.7072429386476955 ) ) ;
#10458=CARTESIAN_POINT ( 'NONE',  ( 4.483927247898790824, -16.52544592524335698, 105.2094237280190328 ) ) ;
#10460=CARTESIAN_POINT ( 'NONE',  ( 4.379528057220092307, 16.55341960407617563, 92.29275706135236135 ) ) ;
#10461=CARTESIAN_POINT ( 'NONE',  ( 15.50000000000000178, -7.500000000000000888, 22.00000000000000711 ) ) ;
#10462=CARTESIAN_POINT ( 'NONE',  ( 8.224510206698742110, 14.34966873604972548, 72.08442372801899012 ) ) ;
#10464=CARTESIAN_POINT ( 'NONE',  ( 0.05219959533937995610, -21.53943276465977519, 80.00109039468568994 ) ) ;
#10465=CARTESIAN_POINT ( 'NONE',  ( -19.02544592524334988, -5.153800228976617603, 93.95942372801900433 ) ) ;
#10466=CARTESIAN_POINT ( 'NONE',  ( 13.89961937509957401, 13.97604488694547697, 21.87609039468566152 ) ) ;
#10467=CARTESIAN_POINT ( 'NONE',  ( 13.89961937509977652, -13.97604488694527269, 68.12390960531436690 ) ) ;
#10468=CARTESIAN_POINT ( 'NONE',  ( -16.51473224551069308, -9.474510206698971260, 46.66557627198102409 ) ) ;
#10469=CARTESIAN_POINT ( 'NONE',  ( 17.43550251053431666, -6.020693471854104750, 23.33574881071265139 ) ) ;
#10470=CARTESIAN_POINT ( 'NONE',  ( 15.72974639402199770, -15.80617190586745480, 78.12390960531436690 ) ) ;
#10471=CARTESIAN_POINT ( 'NONE',  ( 10.81492255796078972, 18.62759615963270932, 34.58224293864770260 ) ) ;
#10472=CARTESIAN_POINT ( 'NONE',  ( 9.474510206698971260, -16.51473224551069308, 32.91557627198102409 ) ) ;
#10473=CARTESIAN_POINT ( 'NONE',  ( -8.314922557961024197, 14.29746914071037800, 52.91775706135235424 ) ) ;
#10476=CARTESIAN_POINT ( 'NONE',  ( 21.55341960407619695, -5.719274019375665929, 36.04275706135234714 ) ) ;
#10477=CARTESIAN_POINT ( 'NONE',  ( 4.379528057220339221, -16.55341960407611168, 57.70724293864770260 ) ) ;
#10479=CARTESIAN_POINT ( 'NONE',  ( -16.52544592524335698, -4.483927247898792601, 18.95942372801901143 ) ) ;
#10480=CARTESIAN_POINT ( 'NONE',  ( 5.153800228976615827, -19.02544592524334988, 35.20942372801899722 ) ) ;
#10481=CARTESIAN_POINT ( 'NONE',  ( -16.53943276465976808, 0.05219959533911058130, 51.24890960531436690 ) ) ;
#10482=CARTESIAN_POINT ( 'NONE',  ( 18.62759615963255655, 10.81492255796105972, 21.66775706135235069 ) ) ;
#10484=CARTESIAN_POINT ( 'NONE',  ( -5.823673210054116645, -21.52544592524344225, 77.29057627198102409 ) ) ;
#10485=CARTESIAN_POINT ( 'NONE',  ( 19.03943276465977164, -0.05219959533909143690, 83.74890960531436690 ) ) ;
#10486=CARTESIAN_POINT ( 'NONE',  ( 4.379528057220339221, -16.55341960407611168, 67.70724293864769550 ) ) ;
#10487=FACE_OUTER_BOUND ( 'NONE', #49407, .T. ) ;
#10488=CARTESIAN_POINT ( 'NONE',  ( -17.49999999999999645, 5.499999999999997335, 120.0000000000000142 ) ) ;
#10489=CARTESIAN_POINT ( 'NONE',  ( -19.05341960407617563, 5.049401038297882671, 63.54275706135234003 ) ) ;
#10490=CARTESIAN_POINT ( 'NONE',  ( -18.67979575497178146, -10.72451020669898902, 101.6655762719810383 ) ) ;
#10491=CARTESIAN_POINT ( 'NONE',  ( -19.05341960407611168, -5.049401038298163336, 61.45724293864769550 ) ) ;
#10492=CARTESIAN_POINT ( 'NONE',  ( 16.51473224551083163, -9.474510206698727899, 45.83442372801900433 ) ) ;
#10493=CARTESIAN_POINT ( 'NONE',  ( -5.049401038298153566, 19.05341960407611168, 25.20724293864768484 ) ) ;
#10494=CARTESIAN_POINT ( 'NONE',  ( 15.80617190586769283, -15.72974639402175789, 60.62609039468567573 ) ) ;
#10495=CARTESIAN_POINT ( 'NONE',  ( -16.36317988757060249, -7.306389748694935626, 70.90210391636776421 ) ) ;
#10496=CARTESIAN_POINT ( 'NONE',  ( -12.06949235617756955, 12.14591786802309770, 40.62390960531435269 ) ) ;
#10497=CARTESIAN_POINT ( 'NONE',  ( -0.05219959533909027116, -19.03943276465977164, 57.49890960531435979 ) ) ;
#10498=CARTESIAN_POINT ( 'NONE',  ( -15.72974639402197994, 15.80617190586746368, 80.62390960531438111 ) ) ;
#10500=CARTESIAN_POINT ( 'NONE',  ( -19.03943276465977164, 0.05219959533909376836, 56.24890960531435979 ) ) ;
#10501=CARTESIAN_POINT ( 'NONE',  ( 21.52544592524344225, -5.823673210054117533, 68.54057627198103830 ) ) ;
#10503=CARTESIAN_POINT ( 'NONE',  ( 21.55341960407619695, -5.719274019375665929, 106.0427570613523471 ) ) ;
#10505=CARTESIAN_POINT ( 'NONE',  ( 12.06949235617739724, 12.14591786802326823, 101.8760903946857042 ) ) ;
#10506=CARTESIAN_POINT ( 'NONE',  ( -14.29746914071049879, 8.314922557960819915, 80.83224293864769550 ) ) ;
#10507=CARTESIAN_POINT ( 'NONE',  ( -9.474510206698964154, 16.51473224551069663, 65.41557627198102409 ) ) ;
#10509=CARTESIAN_POINT ( 'NONE',  ( 19.05341960407617918, -5.049401038297876454, 36.04275706135234003 ) ) ;
#10510=CARTESIAN_POINT ( 'NONE',  ( -14.34966873604972548, 8.224510206698743886, 93.33442372801901854 ) ) ;
#10511=CARTESIAN_POINT ( 'NONE',  ( -9.564922557961040184, 16.46253265017147172, 32.91775706135233293 ) ) ;
#10512=CARTESIAN_POINT ( 'NONE',  ( 5.049401038298161559, -19.05341960407611168, 82.70724293864770971 ) ) ;
#10513=CARTESIAN_POINT ( 'NONE',  ( 5.719274019375991003, -21.55341960407610458, 57.70724293864770260 ) ) ;
#10514=DIRECTION ( 'NONE',  ( 0.000000000000000000, 0.000000000000000000, -1.000000000000000000 ) ) ;
#10515=CARTESIAN_POINT ( 'NONE',  ( -16.55341960407611168, -4.379528057220339221, 111.4572429386476813 ) ) ;
#10516=CARTESIAN_POINT ( 'NONE',  ( 15.72974639402176855, 15.80617190586768217, 101.8760903946857042 ) ) ;
#10517=CARTESIAN_POINT ( 'NONE',  ( 8.224510206698742110, 14.34966873604972548, 62.08442372801901143 ) ) ;
#10518=CARTESIAN_POINT ( 'NONE',  ( 18.62759615963255655, 10.81492255796105972, 31.66775706135234358 ) ) ;
#10519=CARTESIAN_POINT ( 'NONE',  ( -12.06949235617739369, -12.14591786802326823, 24.37609039468567573 ) ) ;
#10520=CARTESIAN_POINT ( 'NONE',  ( -16.46253265017160317, 9.564922557960807481, 95.83224293864769550 ) ) ;
#10521=CARTESIAN_POINT ( 'NONE',  ( 13.89961937509977652, -13.97604488694527269, 43.12390960531434558 ) ) ;
#10522=CARTESIAN_POINT ( 'NONE',  ( 19.05341960407611168, 5.049401038298154454, 53.95724293864770260 ) ) ;
#10523=CARTESIAN_POINT ( 'NONE',  ( -8.224510206698735004, -14.34966873604973081, 39.58442372801901143 ) ) ;
#10524=CARTESIAN_POINT ( 'NONE',  ( 16.55341960407611168, 4.379528057220329451, 98.95724293864770971 ) ) ;
#10525=CARTESIAN_POINT ( 'NONE',  ( 16.52544592524335698, 4.483927247898782831, 96.45942372801901854 ) ) ;
#10526=CARTESIAN_POINT ( 'NONE',  ( -5.719274019375665041, -21.55341960407619695, 44.79275706135234714 ) ) ;
#10527=CARTESIAN_POINT ( 'NONE',  ( -13.97604488694527625, -13.89961937509977652, 81.87390960531436690 ) ) ;
#10528=CARTESIAN_POINT ( 'NONE',  ( 0.05219959533909260263, 19.03943276465977164, 54.99890960531435979 ) ) ;
#10529=CARTESIAN_POINT ( 'NONE',  ( 9.564922557960805705, 16.46253265017160317, 79.58224293864769550 ) ) ;
#10530=CARTESIAN_POINT ( 'NONE',  ( 16.52544592524342804, -4.483927247898539470, 33.54057627198102409 ) ) ;
#10531=CARTESIAN_POINT ( 'NONE',  ( -8.314922557961024197, 14.29746914071037800, 97.91775706135236135 ) ) ;
#10533=CARTESIAN_POINT ( 'NONE',  ( -0.05219959533936034679, 19.03943276465977164, 47.50109039468566863 ) ) ;
#10534=CARTESIAN_POINT ( 'NONE',  ( -19.03943276465977164, 0.05219959533909376836, 116.2489096053143669 ) ) ;
#10535=CARTESIAN_POINT ( 'NONE',  ( 5.049401038298161559, -19.05341960407611168, 52.70724293864767418 ) ) ;
#10536=CARTESIAN_POINT ( 'NONE',  ( -5.049401038297874678, -19.05341960407617918, 19.79275706135233293 ) ) ;
#10538=CARTESIAN_POINT ( 'NONE',  ( -4.483927247898782831, 16.52544592524335698, 37.70942372801900433 ) ) ;
#10539=CARTESIAN_POINT ( 'NONE',  ( 5.049401038297881783, 19.05341960407617563, 77.29275706135231871 ) ) ;
#10540=CARTESIAN_POINT ( 'NONE',  ( -16.55341960407617563, 4.379528057220093196, 58.54275706135235424 ) ) ;
#10542=CARTESIAN_POINT ( 'NONE',  ( 9.474510206698971260, -16.51473224551069308, 77.91557627198103830 ) ) ;
#10543=CARTESIAN_POINT ( 'NONE',  ( 21.53943276465977519, 0.05219959533937863772, 21.25109039468567218 ) ) ;
#10544=CARTESIAN_POINT ( 'NONE',  ( 9.474510206698729675, 16.51473224551082808, 72.08442372801900433 ) ) ;
#10545=CARTESIAN_POINT ( 'NONE',  ( -5.153800228976328057, -19.02544592524343514, 107.2905762719810383 ) ) ;
#10546=CARTESIAN_POINT ( 'NONE',  ( -5.153800228976328057, -19.02544592524343514, 32.29057627198102409 ) ) ;
#10547=CARTESIAN_POINT ( 'NONE',  ( 19.05341960407611168, 5.049401038298154454, 78.95724293864769550 ) ) ;
#10548=CARTESIAN_POINT ( 'NONE',  ( 4.483927247898545687, 16.52544592524342804, 39.79057627198103830 ) ) ;
#10549=CARTESIAN_POINT ( 'NONE',  ( -19.05341960407611168, -5.049401038298163336, 41.45724293864769550 ) ) ;
#10550=CARTESIAN_POINT ( 'NONE',  ( -5.153800228976607833, 19.02544592524334988, 47.70942372801900433 ) ) ;
#10551=CARTESIAN_POINT ( 'NONE',  ( -12.06949235617756955, 12.14591786802309770, 80.62390960531438111 ) ) ;
#10552=CARTESIAN_POINT ( 'NONE',  ( -19.02544592524334988, -5.153800228976617603, 18.95942372801899722 ) ) ;
#10553=CARTESIAN_POINT ( 'NONE',  ( -13.89961937509977652, 13.97604488694528158, 55.62390960531434558 ) ) ;
#10554=CARTESIAN_POINT ( 'NONE',  ( 5.719274019375991003, -21.55341960407610458, 47.70724293864770260 ) ) ;
#10555=CARTESIAN_POINT ( 'NONE',  ( 12.06949235617757843, -12.14591786802309237, 53.12390960531436690 ) ) ;
#10556=CARTESIAN_POINT ( 'NONE',  ( -15.80617190586768217, 15.72974639402176855, 108.1260903946856757 ) ) ;
#10557=CARTESIAN_POINT ( 'NONE',  ( 19.02544592524343514, -5.153800228976328945, 93.54057627198102409 ) ) ;
#10558=CARTESIAN_POINT ( 'NONE',  ( -9.564922557960796823, -16.46253265017161027, 112.0822429386476955 ) ) ;
#10559=CARTESIAN_POINT ( 'NONE',  ( 16.46253265017160672, -9.564922557960803928, 43.33224293864769550 ) ) ;
#10560=CARTESIAN_POINT ( 'NONE',  ( -13.97604488694527625, -13.89961937509977652, 21.87390960531435979 ) ) ;
#10561=CARTESIAN_POINT ( 'NONE',  ( -4.379528057220328563, 16.55341960407611168, 90.20724293864770971 ) ) ;
#10562=CARTESIAN_POINT ( 'NONE',  ( 21.52544592524344225, -5.823673210054117533, 103.5405762719810383 ) ) ;
#10563=CARTESIAN_POINT ( 'NONE',  ( 19.02544592524343514, -5.153800228976328945, 88.54057627198102409 ) ) ;
#10564=CARTESIAN_POINT ( 'NONE',  ( 21.52544592524344225, -5.823673210054117533, 113.5405762719810383 ) ) ;
#10565=CARTESIAN_POINT ( 'NONE',  ( -9.474510206698964154, 16.51473224551069663, 95.41557627198102409 ) ) ;
#10567=CARTESIAN_POINT ( 'NONE',  ( -4.483927247898539470, -16.52544592524342804, 107.2905762719810525 ) ) ;
#10568=CARTESIAN_POINT ( 'NONE',  ( 19.03943276465977164, -0.05219959533909143690, 68.74890960531436690 ) ) ;
#10569=CARTESIAN_POINT ( 'NONE',  ( 0.05219959533907565091, 21.53943276465977519, 74.99890960531435269 ) ) ;
#10572=CARTESIAN_POINT ( 'NONE',  ( 15.80617190586746368, 15.72974639402197994, 29.37390960531435269 ) ) ;
#10574=CARTESIAN_POINT ( 'NONE',  ( -14.29746914071037622, -8.314922557961029526, 34.16775706135234714 ) ) ;
#10576=CARTESIAN_POINT ( 'NONE',  ( 12.06949235617757843, -12.14591786802309237, 88.12390960531436690 ) ) ;
#10578=CARTESIAN_POINT ( 'NONE',  ( -17.50000000000002132, -5.499999999999948486, 91.28230962303565832 ) ) ;
#10579=CARTESIAN_POINT ( 'NONE',  ( -13.89961937509977652, 13.97604488694528158, 90.62390960531432427 ) ) ;
#10580=CARTESIAN_POINT ( 'NONE',  ( 5.153800228976335163, 19.02544592524342804, 44.79057627198103830 ) ) ;
#10581=CARTESIAN_POINT ( 'NONE',  ( 14.34966873604960469, 8.224510206698951720, 74.16557627198102409 ) ) ;
#10582=CARTESIAN_POINT ( 'NONE',  ( -5.823673210054116645, -21.52544592524344225, 32.29057627198102409 ) ) ;
#10583=CARTESIAN_POINT ( 'NONE',  ( -4.379528057220328563, 16.55341960407611168, 55.20724293864770260 ) ) ;
#10584=CARTESIAN_POINT ( 'NONE',  ( 9.564922557961047289, -16.46253265017146816, 100.4177570613523329 ) ) ;
#10585=CARTESIAN_POINT ( 'NONE',  ( -5.823673210054431948, 21.52544592524334988, 72.70942372801901854 ) ) ;
#10587=CARTESIAN_POINT ( 'NONE',  ( 19.02544592524343514, -5.153800228976328945, 113.5405762719810241 ) ) ;
#10588=CARTESIAN_POINT ( 'NONE',  ( 14.34966873604972726, -8.224510206698740333, 90.83442372801901854 ) ) ;
#10589=CARTESIAN_POINT ( 'NONE',  ( -17.48847506799949159, 5.747544572775296956, 95.82697437843293642 ) ) ;
#10590=CARTESIAN_POINT ( 'NONE',  ( 19.05341960407611168, 5.049401038298154454, 73.95724293864768129 ) ) ;
#10591=CARTESIAN_POINT ( 'NONE',  ( -10.81492255796078084, -18.62759615963271287, 82.08224293864768129 ) ) ;
#10592=CARTESIAN_POINT ( 'NONE',  ( -14.34966873604972548, 8.224510206698743886, 28.33442372801902209 ) ) ;
#10593=CARTESIAN_POINT ( 'NONE',  ( 4.379528057220339221, -16.55341960407611168, 52.70724293864769550 ) ) ;
#10594=CARTESIAN_POINT ( 'NONE',  ( -21.52544592524334988, -5.823673210054445271, 78.95942372801901854 ) ) ;
#10595=CARTESIAN_POINT ( 'NONE',  ( 0.05219959533934541429, -16.53943276465976808, 85.00109039468568994 ) ) ;
#10596=CARTESIAN_POINT ( 'NONE',  ( -21.55341960407610458, -5.719274019375992779, 26.45724293864768839 ) ) ;
#10599=CARTESIAN_POINT ( 'NONE',  ( -4.379528057220086978, -16.55341960407618274, 104.7927570613523898 ) ) ;
#10600=CARTESIAN_POINT ( 'NONE',  ( 12.14591786802327356, -12.06949235617739191, 55.62609039468568284 ) ) ;
#10601=CARTESIAN_POINT ( 'NONE',  ( -19.05341960407611168, -5.049401038298163336, 71.45724293864766707 ) ) ;
#10602=CARTESIAN_POINT ( 'NONE',  ( -9.474510206698964154, 16.51473224551069663, 90.41557627198103830 ) ) ;
#10603=CARTESIAN_POINT ( 'NONE',  ( -10.81492255796105439, 18.62759615963255655, 77.91775706135231871 ) ) ;
#10605=CARTESIAN_POINT ( 'NONE',  ( 12.06949235617739724, 12.14591786802326823, 76.87609039468567573 ) ) ;
#10606=CARTESIAN_POINT ( 'NONE',  ( 12.14591786802309770, 12.06949235617756955, 44.37390960531435979 ) ) ;
#10607=CARTESIAN_POINT ( 'NONE',  ( -5.153800228976328057, -19.02544592524343514, 57.29057627198103120 ) ) ;
#10608=CARTESIAN_POINT ( 'NONE',  ( -9.564922557960796823, -16.46253265017161027, 42.08224293864769550 ) ) ;
#10610=CARTESIAN_POINT ( 'NONE',  ( 16.46253265017146816, 9.564922557961045513, 96.66775706135233293 ) ) ;
#10611=CARTESIAN_POINT ( 'NONE',  ( 16.53943276465976808, -0.05219959533910856209, 93.74890960531436690 ) ) ;
#10612=CARTESIAN_POINT ( 'NONE',  ( 9.564922557960805705, 16.46253265017160317, 59.58224293864769550 ) ) ;
#10613=CARTESIAN_POINT ( 'NONE',  ( -13.97604488694547697, 13.89961937509957934, 98.12609039468566152 ) ) ;
#10615=CARTESIAN_POINT ( 'NONE',  ( -15.72974639402176322, -15.80617190586768395, 109.3760903946857042 ) ) ;
#10616=CARTESIAN_POINT ( 'NONE',  ( -12.14591786802326823, 12.06949235617739902, 68.12609039468567573 ) ) ;
#10617=CARTESIAN_POINT ( 'NONE',  ( 16.46253265017146816, 9.564922557961045513, 91.66775706135234714 ) ) ;
#10618=CARTESIAN_POINT ( 'NONE',  ( 10.81492255796078972, 18.62759615963270932, 59.58224293864770260 ) ) ;
#10619=CARTESIAN_POINT ( 'NONE',  ( 12.14591786802327356, -12.06949235617739191, 55.62609039468568284 ) ) ;
#10621=CARTESIAN_POINT ( 'NONE',  ( -19.05341960407617563, 5.049401038297882671, 53.54275706135231871 ) ) ;
#10622=CARTESIAN_POINT ( 'NONE',  ( 10.81492255796106328, -18.62759615963255655, 100.4177570613523471 ) ) ;
#10623=CARTESIAN_POINT ( 'NONE',  ( -16.55341960407611168, -4.379528057220339221, 111.4572429386476813 ) ) ;
#10624=CARTESIAN_POINT ( 'NONE',  ( -19.02544592524342804, 5.153800228976336051, 71.04057627198099567 ) ) ;
#10625=CARTESIAN_POINT ( 'NONE',  ( -16.53943276465976808, 0.05219959533911058130, 56.24890960531436690 ) ) ;
#10626=CARTESIAN_POINT ( 'NONE',  ( -10.81492255796105439, 18.62759615963255655, 92.91775706135236135 ) ) ;
#10627=CARTESIAN_POINT ( 'NONE',  ( 13.97604488694548053, -13.89961937509957401, 50.62609039468566152 ) ) ;
#10628=CARTESIAN_POINT ( 'NONE',  ( 16.46253265017146816, 9.564922557961045513, 26.66775706135234003 ) ) ;
#10629=CARTESIAN_POINT ( 'NONE',  ( 5.719274019375991003, -21.55341960407610458, 27.70724293864769905 ) ) ;
#10630=CARTESIAN_POINT ( 'NONE',  ( 15.80617190586769283, -15.72974639402175789, 90.62609039468567573 ) ) ;
#10631=CARTESIAN_POINT ( 'NONE',  ( -19.02544592524342804, 5.153800228976336051, 81.04057627198103830 ) ) ;
#10633=CARTESIAN_POINT ( 'NONE',  ( 18.62759615963255655, 10.81492255796105972, 91.66775706135234714 ) ) ;
#10634=CARTESIAN_POINT ( 'NONE',  ( -18.67979575497178146, -10.72451020669898902, 46.66557627198102409 ) ) ;
#10635=CARTESIAN_POINT ( 'NONE',  ( 16.46253265017160672, -9.564922557960803928, 83.33224293864768129 ) ) ;
#10636=CARTESIAN_POINT ( 'NONE',  ( 16.51473224551083163, -9.474510206698727899, 60.83442372801900433 ) ) ;
#10637=CARTESIAN_POINT ( 'NONE',  ( -5.153800228976328057, -19.02544592524343514, 42.29057627198101699 ) ) ;
#10638=CARTESIAN_POINT ( 'NONE',  ( -5.049401038298153566, 19.05341960407611168, 90.20724293864766707 ) ) ;
#10639=CARTESIAN_POINT ( 'NONE',  ( -9.474510206698720793, -16.51473224551083518, 84.58442372801900433 ) ) ;
#10640=CARTESIAN_POINT ( 'NONE',  ( 14.29746914071037800, 8.314922557961029526, 46.66775706135234714 ) ) ;
#10641=CARTESIAN_POINT ( 'NONE',  ( 8.224510206698953496, -14.34966873604960469, 102.9155762719810383 ) ) ;
#10642=CARTESIAN_POINT ( 'NONE',  ( -9.564922557960796823, -16.46253265017161027, 77.08224293864769550 ) ) ;
#10643=CARTESIAN_POINT ( 'NONE',  ( -21.53943276465977519, 0.05219959533907696930, 56.24890960531436690 ) ) ;
#10644=CARTESIAN_POINT ( 'NONE',  ( 13.97604488694548053, -13.89961937509957401, 110.6260903946856615 ) ) ;
#10645=CARTESIAN_POINT ( 'NONE',  ( 5.823673210054444382, -21.52544592524334988, 20.20942372801900788 ) ) ;
#10646=CARTESIAN_POINT ( 'NONE',  ( -10.81492255796105439, 18.62759615963255655, 72.91775706135234714 ) ) ;
#10647=CARTESIAN_POINT ( 'NONE',  ( -12.14591786802326823, 12.06949235617739902, 78.12609039468570415 ) ) ;
#10648=CARTESIAN_POINT ( 'NONE',  ( 13.97604488694527802, 13.89961937509977652, 74.37390960531436690 ) ) ;
#10649=CARTESIAN_POINT ( 'NONE',  ( 16.52544592524335698, 4.483927247898782831, 101.4594237280190185 ) ) ;
#10650=CARTESIAN_POINT ( 'NONE',  ( 0.05219959533936267826, -19.03943276465977164, 60.00109039468566863 ) ) ;
#10651=CARTESIAN_POINT ( 'NONE',  ( -5.823673210054431948, 21.52544592524334988, 37.70942372801900433 ) ) ;
#10652=CARTESIAN_POINT ( 'NONE',  ( 8.224510206698953496, -14.34966873604960469, 82.91557627198103830 ) ) ;
#10653=CARTESIAN_POINT ( 'NONE',  ( -9.474510206698964154, 16.51473224551069663, 105.4155762719810383 ) ) ;
#10654=CARTESIAN_POINT ( 'NONE',  ( -16.53943276465976808, -0.05219959533934237506, 83.75109039468568994 ) ) ;
#10655=CARTESIAN_POINT ( 'NONE',  ( 15.80617190586769283, -15.72974639402175789, 70.62609039468567573 ) ) ;
#10656=CARTESIAN_POINT ( 'NONE',  ( 0.05219959533934541429, -16.53943276465976808, 35.00109039468568284 ) ) ;
#10657=CARTESIAN_POINT ( 'NONE',  ( 0.05219959533937995610, -21.53943276465977519, 30.00109039468568284 ) ) ;
#10658=CARTESIAN_POINT ( 'NONE',  ( 4.483927247898545687, 16.52544592524342804, 74.79057627198105251 ) ) ;
#10659=ORIENTED_EDGE ( 'NONE', *, *, #166522, .F. ) ;
#10660=CARTESIAN_POINT ( 'NONE',  ( -5.719274019375978568, 21.55341960407610458, 100.2072429386476955 ) ) ;
#10661=CARTESIAN_POINT ( 'NONE',  ( 16.53943276465976808, -0.05219959533910856209, 58.74890960531436690 ) ) ;
#10663=CARTESIAN_POINT ( 'NONE',  ( 19.02544592524343514, -5.153800228976328945, 28.54057627198102409 ) ) ;
#10664=CARTESIAN_POINT ( 'NONE',  ( -21.53943276465977519, 0.05219959533907696930, 31.24890960531435979 ) ) ;
#10665=CARTESIAN_POINT ( 'NONE',  ( 21.53943276465977519, 0.05219959533937863772, 36.25109039468567573 ) ) ;
#10666=CARTESIAN_POINT ( 'NONE',  ( -12.06949235617756955, 12.14591786802309770, 65.62390960531436690 ) ) ;
#10667=CARTESIAN_POINT ( 'NONE',  ( 21.53943276465977519, -0.05219959533907433946, 63.74890960531435979 ) ) ;
#10668=CARTESIAN_POINT ( 'NONE',  ( -5.049401038298153566, 19.05341960407611168, 70.20724293864769550 ) ) ;
#10669=CARTESIAN_POINT ( 'NONE',  ( -9.564922557960796823, -16.46253265017161027, 27.08224293864769550 ) ) ;
#10670=CARTESIAN_POINT ( 'NONE',  ( -5.049401038297874678, -19.05341960407617918, 84.79275706135233293 ) ) ;
#10671=CARTESIAN_POINT ( 'NONE',  ( 15.72974639402199770, -15.80617190586745480, 58.12390960531435979 ) ) ;
#10672=CARTESIAN_POINT ( 'NONE',  ( -9.474510206698964154, 16.51473224551069663, 45.41557627198103120 ) ) ;
#10673=CARTESIAN_POINT ( 'NONE',  ( -9.474510206698964154, 16.51473224551069663, 65.41557627198102409 ) ) ;
#10675=CARTESIAN_POINT ( 'NONE',  ( 14.34966873604972726, -8.224510206698740333, 55.83442372801901854 ) ) ;
#10676=CARTESIAN_POINT ( 'NONE',  ( -10.81492255796105439, 18.62759615963255655, 27.91775706135234358 ) ) ;
#10677=CARTESIAN_POINT ( 'NONE',  ( -21.53943276465977519, -0.05219959533937600094, 53.75109039468568994 ) ) ;
#10678=CARTESIAN_POINT ( 'NONE',  ( -13.97604488694527625, -13.89961937509977652, 106.8739096053143669 ) ) ;
#10679=CARTESIAN_POINT ( 'NONE',  ( -21.53943276465977519, 0.05219959533907696930, 71.24890960531435269 ) ) ;
#10680=CARTESIAN_POINT ( 'NONE',  ( 5.823673210054125526, 21.52544592524343514, 114.7905762719810383 ) ) ;
#10681=CARTESIAN_POINT ( 'NONE',  ( 16.53943276465976808, 0.05219959533934440121, 51.25109039468568994 ) ) ;
#10683=CARTESIAN_POINT ( 'NONE',  ( -10.72451020669898014, 18.67979575497178502, 50.41557627198103120 ) ) ;
#10684=CARTESIAN_POINT ( 'NONE',  ( -5.823673210054431948, 21.52544592524334988, 107.7094237280190328 ) ) ;
#10685=CARTESIAN_POINT ( 'NONE',  ( -16.46253265017160317, 9.564922557960807481, 60.83224293864769550 ) ) ;
#10686=CARTESIAN_POINT ( 'NONE',  ( 0.05219959533909260263, 19.03943276465977164, 104.9989096053143669 ) ) ;
#10687=CARTESIAN_POINT ( 'NONE',  ( -19.05341960407611168, -5.049401038298163336, 76.45724293864769550 ) ) ;
#10689=CARTESIAN_POINT ( 'NONE',  ( 5.153800228976615827, -19.02544592524334988, 70.20942372801899012 ) ) ;
#10690=CARTESIAN_POINT ( 'NONE',  ( 5.823673210054444382, -21.52544592524334988, 110.2094237280190185 ) ) ;
#10691=CARTESIAN_POINT ( 'NONE',  ( 18.62759615963271287, -10.81492255796078972, 43.33224293864769550 ) ) ;
#10692=CARTESIAN_POINT ( 'NONE',  ( -4.483927247898782831, 16.52544592524335698, 102.7094237280190185 ) ) ;
#10693=EDGE_CURVE ( 'NONE', #84229, #1850, #127695, .T. ) ;
#10694=CARTESIAN_POINT ( 'NONE',  ( -5.153800228976607833, 19.02544592524334988, 92.70942372801901854 ) ) ;
#10695=CARTESIAN_POINT ( 'NONE',  ( -17.26172910966779028, 6.454744622555848466, 60.80646908649224258 ) ) ;
#10696=CARTESIAN_POINT ( 'NONE',  ( -18.67979575497193778, 10.72451020669871902, 113.3344237280190328 ) ) ;
#10697=CARTESIAN_POINT ( 'NONE',  ( 16.46253265017146816, 9.564922557961045513, 86.66775706135233293 ) ) ;
#10698=CARTESIAN_POINT ( 'NONE',  ( 9.474510206698729675, 16.51473224551082808, 47.08442372801900433 ) ) ;
#10699=CARTESIAN_POINT ( 'NONE',  ( 17.50000000000000000, 5.499999999999995559, 108.7823096230356867 ) ) ;
#10700=CARTESIAN_POINT ( 'NONE',  ( 0.05219959533909260263, 19.03943276465977164, 39.99890960531436690 ) ) ;
#10701=CARTESIAN_POINT ( 'NONE',  ( 4.379528057220339221, -16.55341960407611168, 52.70724293864769550 ) ) ;
#10702=CARTESIAN_POINT ( 'NONE',  ( 5.049401038298161559, -19.05341960407611168, 37.70724293864768839 ) ) ;
#10703=CARTESIAN_POINT ( 'NONE',  ( 16.53943276465976808, -0.05219959533910856209, 38.74890960531435979 ) ) ;
#10705=CARTESIAN_POINT ( 'NONE',  ( 8.314922557961029526, -14.29746914071037800, 110.4177570613523756 ) ) ;
#10706=CARTESIAN_POINT ( 'NONE',  ( -19.05341960407611168, -5.049401038298163336, 56.45724293864768129 ) ) ;
#10707=CARTESIAN_POINT ( 'NONE',  ( 0.05219959533936267826, -19.03943276465977164, 30.00109039468566863 ) ) ;
#10708=CARTESIAN_POINT ( 'NONE',  ( 16.53943276465976808, 0.05219959533934440121, 36.25109039468567573 ) ) ;
#10709=CARTESIAN_POINT ( 'NONE',  ( -18.62759615963270932, 10.81492255796079327, 40.83224293864769550 ) ) ;
#10710=CARTESIAN_POINT ( 'NONE',  ( -0.05219959533937732626, 21.53943276465977519, 97.50109039468567573 ) ) ;
#10712=CARTESIAN_POINT ( 'NONE',  ( -13.97604488694527625, -13.89961937509977652, 106.8739096053143669 ) ) ;
#10713=CARTESIAN_POINT ( 'NONE',  ( -9.564922557960796823, -16.46253265017161027, 92.08224293864769550 ) ) ;
#10715=CARTESIAN_POINT ( 'NONE',  ( -18.62759615963255300, -10.81492255796106328, 19.16775706135234714 ) ) ;
#10716=CARTESIAN_POINT ( 'NONE',  ( 16.53943276465976808, -0.05219959533910856209, 73.74890960531433848 ) ) ;
#10717=CARTESIAN_POINT ( 'NONE',  ( 0.05219959533907565091, 21.53943276465977519, 74.99890960531435269 ) ) ;
#10718=CARTESIAN_POINT ( 'NONE',  ( -0.05219959533909027116, -19.03943276465977164, 67.49890960531436690 ) ) ;
#10719=CARTESIAN_POINT ( 'NONE',  ( -16.51473224551069308, -9.474510206698971260, 76.66557627198103830 ) ) ;
#10720=CARTESIAN_POINT ( 'NONE',  ( -21.53943276465977519, -0.05219959533937600094, 18.75109039468568639 ) ) ;
#10722=CARTESIAN_POINT ( 'NONE',  ( 19.02544592524343514, -5.153800228976328945, 58.54057627198102409 ) ) ;
#10723=CARTESIAN_POINT ( 'NONE',  ( -14.34966873604960291, -8.224510206698953496, 111.6655762719810525 ) ) ;
#10725=CARTESIAN_POINT ( 'NONE',  ( 13.97604488694527802, 13.89961937509977652, 59.37390960531434558 ) ) ;
#10726=CARTESIAN_POINT ( 'NONE',  ( -9.474510206698720793, -16.51473224551083518, 94.58442372801900433 ) ) ;
#10727=CARTESIAN_POINT ( 'NONE',  ( 16.55341960407611168, 4.379528057220329451, 98.95724293864770971 ) ) ;
#10728=CARTESIAN_POINT ( 'NONE',  ( -21.55341960407619339, 5.719274019375674811, 53.54275706135234714 ) ) ;
#10729=CARTESIAN_POINT ( 'NONE',  ( 13.97604488694527802, 13.89961937509977652, 54.37390960531435979 ) ) ;
#10730=CARTESIAN_POINT ( 'NONE',  ( -5.719274019375978568, 21.55341960407610458, 115.2072429386476955 ) ) ;
#10731=CARTESIAN_POINT ( 'NONE',  ( -12.06949235617756955, 12.14591786802309770, 95.62390960531436690 ) ) ;
#10733=CARTESIAN_POINT ( 'NONE',  ( 19.05341960407611168, 5.049401038298154454, 78.95724293864769550 ) ) ;
#10734=CARTESIAN_POINT ( 'NONE',  ( 17.13100169013301155, 6.664070546373125126, 111.7321016430014993 ) ) ;
#10735=CARTESIAN_POINT ( 'NONE',  ( -13.97604488694547697, 13.89961937509957934, 108.1260903946856331 ) ) ;
#10736=CARTESIAN_POINT ( 'NONE',  ( -21.55341960407610458, -5.719274019375992779, 26.45724293864768839 ) ) ;
#10737=CARTESIAN_POINT ( 'NONE',  ( 18.67979575497194134, -10.72451020669871369, 55.83442372801901854 ) ) ;
#10738=CARTESIAN_POINT ( 'NONE',  ( -9.474510206698964154, 16.51473224551069663, 95.41557627198102409 ) ) ;
#10739=CARTESIAN_POINT ( 'NONE',  ( 9.564922557961047289, -16.46253265017146816, 85.41775706135233293 ) ) ;
#10740=CARTESIAN_POINT ( 'NONE',  ( -19.05341960407611168, -5.049401038298163336, 71.45724293864766707 ) ) ;
#10741=CARTESIAN_POINT ( 'NONE',  ( -12.14591786802309592, -12.06949235617757132, 86.87390960531438111 ) ) ;
#10742=CARTESIAN_POINT ( 'NONE',  ( 5.049401038298161559, -19.05341960407611168, 107.7072429386476955 ) ) ;
#10743=CARTESIAN_POINT ( 'NONE',  ( 8.314922557960818139, 14.29746914071049879, 74.58224293864768129 ) ) ;
#10744=CARTESIAN_POINT ( 'NONE',  ( 19.05341960407611168, 5.049401038298154454, 103.9572429386476671 ) ) ;
#10745=CARTESIAN_POINT ( 'NONE',  ( 9.474510206698729675, 16.51473224551082808, 42.08442372801900433 ) ) ;
#10746=CARTESIAN_POINT ( 'NONE',  ( 13.97604488694527802, 13.89961937509977652, 49.37390960531434558 ) ) ;
#10747=CARTESIAN_POINT ( 'NONE',  ( -4.379528057220328563, 16.55341960407611168, 40.20724293864769550 ) ) ;
#10748=CARTESIAN_POINT ( 'NONE',  ( 5.049401038298161559, -19.05341960407611168, 27.70724293864769550 ) ) ;
#10750=CARTESIAN_POINT ( 'NONE',  ( 10.81492255796106328, -18.62759615963255655, 40.41775706135234714 ) ) ;
#10751=CARTESIAN_POINT ( 'NONE',  ( 9.474510206698729675, 16.51473224551082808, 82.08442372801899012 ) ) ;
#10752=CARTESIAN_POINT ( 'NONE',  ( -14.34966873604960291, -8.224510206698953496, 51.66557627198102409 ) ) ;
#10753=CARTESIAN_POINT ( 'NONE',  ( 21.52544592524344225, -5.823673210054117533, 103.5405762719810383 ) ) ;
#10754=CARTESIAN_POINT ( 'NONE',  ( 5.719274019375991003, -21.55341960407610458, 27.70724293864769905 ) ) ;
#10755=CARTESIAN_POINT ( 'NONE',  ( 0.05219959533910956823, 16.53943276465976808, 89.99890960531438111 ) ) ;
#10756=CARTESIAN_POINT ( 'NONE',  ( 9.474510206698971260, -16.51473224551069308, 37.91557627198102409 ) ) ;
#10757=CARTESIAN_POINT ( 'NONE',  ( -16.55341960407611168, -4.379528057220339221, 21.45724293864769550 ) ) ;
#10758=CARTESIAN_POINT ( 'NONE',  ( 16.53943276465976808, 0.05219959533934440121, 86.25109039468568994 ) ) ;
#10759=CARTESIAN_POINT ( 'NONE',  ( 8.314922557961029526, -14.29746914071037800, 65.41775706135234714 ) ) ;
#10760=CARTESIAN_POINT ( 'NONE',  ( 19.05341960407617918, -5.049401038297876454, 31.04275706135232227 ) ) ;
#10761=CARTESIAN_POINT ( 'NONE',  ( 9.474510206698971260, -16.51473224551069308, 97.91557627198102409 ) ) ;
#10762=CARTESIAN_POINT ( 'NONE',  ( 13.89961937509977652, -13.97604488694527269, 83.12390960531436690 ) ) ;
#10763=CARTESIAN_POINT ( 'NONE',  ( -16.55341960407617563, 4.379528057220093196, 73.54275706135234714 ) ) ;
#10764=CARTESIAN_POINT ( 'NONE',  ( 9.474510206698971260, -16.51473224551069308, 37.91557627198102409 ) ) ;
#10765=CARTESIAN_POINT ( 'NONE',  ( -8.314922557960811034, -14.29746914071050412, 52.08224293864768839 ) ) ;
#10766=FACE_OUTER_BOUND ( 'NONE', #100934, .T. ) ;
#10767=CARTESIAN_POINT ( 'NONE',  ( 13.89961937509977652, -13.97604488694527269, 103.1239096053143527 ) ) ;
#10768=CARTESIAN_POINT ( 'NONE',  ( 15.72974639402199770, -15.80617190586745480, 33.12390960531435979 ) ) ;
#10769=CARTESIAN_POINT ( 'NONE',  ( -16.53943276465976808, 0.05219959533911058130, 66.24890960531436690 ) ) ;
#10772=CARTESIAN_POINT ( 'NONE',  ( -14.34966873604960291, -8.224510206698953496, 61.66557627198103120 ) ) ;
#10774=CARTESIAN_POINT ( 'NONE',  ( -16.51473224551082808, 9.474510206698731452, 68.33442372801900433 ) ) ;
#10775=CARTESIAN_POINT ( 'NONE',  ( 19.03943276465977164, -0.05219959533909143690, 93.74890960531435269 ) ) ;
#10776=CARTESIAN_POINT ( 'NONE',  ( 19.05341960407617918, -5.049401038297876454, 76.04275706135230450 ) ) ;
#10777=CARTESIAN_POINT ( 'NONE',  ( -0.05219959533936034679, 19.03943276465977164, 107.5010903946856615 ) ) ;
#10778=CARTESIAN_POINT ( 'NONE',  ( 14.29746914071037800, 8.314922557961029526, 96.66775706135234714 ) ) ;
#10779=CARTESIAN_POINT ( 'NONE',  ( -19.05341960407611168, -5.049401038298163336, 41.45724293864769550 ) ) ;
#10780=CARTESIAN_POINT ( 'NONE',  ( -10.72451020669898014, 18.67979575497178502, 40.41557627198103120 ) ) ;
#10781=CARTESIAN_POINT ( 'NONE',  ( -15.72974639402176322, -15.80617190586768395, 49.37609039468569705 ) ) ;
#10782=CARTESIAN_POINT ( 'NONE',  ( 0.05219959533934541429, -16.53943276465976808, 25.00109039468567218 ) ) ;
#10784=CARTESIAN_POINT ( 'NONE',  ( -0.05219959533909027116, -19.03943276465977164, 77.49890960531435269 ) ) ;
#10786=CARTESIAN_POINT ( 'NONE',  ( -0.05219959533910754901, -16.53943276465976808, 77.49890960531433848 ) ) ;
#10787=CARTESIAN_POINT ( 'NONE',  ( 0.05219959533909260263, 19.03943276465977164, 74.99890960531435269 ) ) ;
#10788=CARTESIAN_POINT ( 'NONE',  ( 19.02544592524343514, -5.153800228976328945, 68.54057627198103830 ) ) ;
#10790=CARTESIAN_POINT ( 'NONE',  ( -19.02544592524334988, -5.153800228976617603, 93.95942372801900433 ) ) ;
#10791=CARTESIAN_POINT ( 'NONE',  ( 10.72451020669898902, -18.67979575497178502, 57.91557627198103120 ) ) ;
#10792=CARTESIAN_POINT ( 'NONE',  ( 19.05341960407611168, 5.049401038298154454, 33.95724293864769550 ) ) ;
#10793=CARTESIAN_POINT ( 'NONE',  ( 5.049401038297881783, 19.05341960407617563, 62.29275706135234003 ) ) ;
#10794=CARTESIAN_POINT ( 'NONE',  ( 5.153800228976335163, 19.02544592524342804, 54.79057627198103120 ) ) ;
#10795=CARTESIAN_POINT ( 'NONE',  ( 16.51473224551069308, 9.474510206698969483, 94.16557627198103830 ) ) ;
#10797=CARTESIAN_POINT ( 'NONE',  ( -5.823673210054116645, -21.52544592524344225, 87.29057627198103830 ) ) ;
#10798=CARTESIAN_POINT ( 'NONE',  ( -12.14591786802309592, -12.06949235617757132, 96.87390960531436690 ) ) ;
#10799=CARTESIAN_POINT ( 'NONE',  ( 19.03943276465977164, 0.05219959533936151252, 46.25109039468566863 ) ) ;
#10800=CARTESIAN_POINT ( 'NONE',  ( -10.81492255796078084, -18.62759615963271287, 87.08224293864769550 ) ) ;
#10801=CARTESIAN_POINT ( 'NONE',  ( 5.823673210054125526, 21.52544592524343514, 74.79057627198105251 ) ) ;
#10802=CARTESIAN_POINT ( 'NONE',  ( -16.55341960407611168, -4.379528057220339221, 31.45724293864769550 ) ) ;
#10803=CARTESIAN_POINT ( 'NONE',  ( 0.05219959533937995610, -21.53943276465977519, 110.0010903946856757 ) ) ;
#10804=CARTESIAN_POINT ( 'NONE',  ( -5.049401038298153566, 19.05341960407611168, 80.20724293864769550 ) ) ;
#10805=CARTESIAN_POINT ( 'NONE',  ( -0.05219959533909027116, -19.03943276465977164, 32.49890960531435979 ) ) ;
#10806=CARTESIAN_POINT ( 'NONE',  ( -21.52544592524334988, -5.823673210054445271, 38.95942372801901854 ) ) ;
#10807=CARTESIAN_POINT ( 'NONE',  ( 21.55341960407619695, -5.719274019375665929, 51.04275706135234714 ) ) ;
#10808=CARTESIAN_POINT ( 'NONE',  ( 13.89961937509977652, -13.97604488694527269, 43.12390960531434558 ) ) ;
#10809=CARTESIAN_POINT ( 'NONE',  ( 18.62759615963271287, -10.81492255796078972, 113.3322429386476955 ) ) ;
#10810=CARTESIAN_POINT ( 'NONE',  ( -13.97604488694547697, 13.89961937509957934, 58.12609039468566863 ) ) ;
#10811=CARTESIAN_POINT ( 'NONE',  ( -5.049401038298153566, 19.05341960407611168, 35.20724293864768839 ) ) ;
#10812=CARTESIAN_POINT ( 'NONE',  ( -16.53943276465976808, -0.05219959533934237506, 23.75109039468567929 ) ) ;
#10813=CARTESIAN_POINT ( 'NONE',  ( 5.049401038298161559, -19.05341960407611168, 32.70724293864768129 ) ) ;
#10814=CARTESIAN_POINT ( 'NONE',  ( -8.224510206698735004, -14.34966873604973081, 74.58442372801901854 ) ) ;
#10815=CARTESIAN_POINT ( 'NONE',  ( 19.05341960407611168, 5.049401038298154454, 43.95724293864769550 ) ) ;
#10817=CARTESIAN_POINT ( 'NONE',  ( -16.51473224551069308, -9.474510206698971260, 81.66557627198103830 ) ) ;
#10818=CARTESIAN_POINT ( 'NONE',  ( 16.51473224551069308, 9.474510206698969483, 29.16557627198103475 ) ) ;
#10819=CARTESIAN_POINT ( 'NONE',  ( -15.80617190586745835, -15.72974639402198527, 71.87390960531438111 ) ) ;
#10820=CARTESIAN_POINT ( 'NONE',  ( 16.53943276465976808, 0.05219959533934440121, 41.25109039468568284 ) ) ;
#10821=CARTESIAN_POINT ( 'NONE',  ( -13.89961937509957401, -13.97604488694547875, 24.37609039468565442 ) ) ;
#10822=CARTESIAN_POINT ( 'NONE',  ( 19.03943276465977164, -0.05219959533909143690, 33.74890960531435979 ) ) ;
#10823=CARTESIAN_POINT ( 'NONE',  ( 8.224510206698953496, -14.34966873604960469, 32.91557627198102409 ) ) ;
#10824=CARTESIAN_POINT ( 'NONE',  ( 12.14591786802309770, 12.06949235617756955, 69.37390960531436690 ) ) ;
#10825=CARTESIAN_POINT ( 'NONE',  ( 9.564922557960805705, 16.46253265017160317, 64.58224293864769550 ) ) ;
#10826=CARTESIAN_POINT ( 'NONE',  ( 18.67979575497194134, -10.72451020669871369, 110.8344237280190043 ) ) ;
#10827=CARTESIAN_POINT ( 'NONE',  ( -10.72451020669898014, 18.67979575497178502, 115.4155762719810241 ) ) ;
#10828=CARTESIAN_POINT ( 'NONE',  ( 13.89961937509977652, -13.97604488694527269, 78.12390960531433848 ) ) ;
#10830=CARTESIAN_POINT ( 'NONE',  ( -18.62759615963255300, -10.81492255796106328, 84.16775706135234714 ) ) ;
#10831=CARTESIAN_POINT ( 'NONE',  ( -0.05219959533934338120, 16.53943276465976808, 62.50109039468568284 ) ) ;
#10832=CARTESIAN_POINT ( 'NONE',  ( -0.05219959533910754901, -16.53943276465976808, 87.49890960531436690 ) ) ;
#10833=CARTESIAN_POINT ( 'NONE',  ( -16.51473224551069308, -9.474510206698971260, 106.6655762719810383 ) ) ;
#10834=CARTESIAN_POINT ( 'NONE',  ( 0.05219959533910956823, 16.53943276465976808, 29.99890960531435979 ) ) ;
#10835=CARTESIAN_POINT ( 'NONE',  ( -19.05341960407611168, -5.049401038298163336, 26.45724293864769550 ) ) ;
#10836=CARTESIAN_POINT ( 'NONE',  ( 12.06949235617739724, 12.14591786802326823, 56.87609039468568994 ) ) ;
#10837=CARTESIAN_POINT ( 'NONE',  ( -4.379528057220328563, 16.55341960407611168, 50.20724293864769550 ) ) ;
#10838=CARTESIAN_POINT ( 'NONE',  ( 16.53943276465976808, 0.05219959533934440121, 106.2510903946856757 ) ) ;
#10839=CARTESIAN_POINT ( 'NONE',  ( -0.05219959533907301413, -21.53943276465977519, 22.49890960531436335 ) ) ;
#10840=CARTESIAN_POINT ( 'NONE',  ( -21.52544592524343514, 5.823673210054127303, 36.04057627198102409 ) ) ;
#10841=CARTESIAN_POINT ( 'NONE',  ( 21.53943276465977519, 0.05219959533937863772, 106.2510903946856757 ) ) ;
#10843=CARTESIAN_POINT ( 'NONE',  ( 14.34966873604960469, 8.224510206698951720, 84.16557627198103830 ) ) ;
#10844=CARTESIAN_POINT ( 'NONE',  ( -19.05341960407611168, -5.049401038298163336, 91.45724293864766707 ) ) ;
#10846=CARTESIAN_POINT ( 'NONE',  ( 4.379528057220092307, 16.55341960407617563, 42.29275706135235424 ) ) ;
#10847=CARTESIAN_POINT ( 'NONE',  ( 9.564922557960805705, 16.46253265017160317, 54.58224293864769550 ) ) ;
#10849=CARTESIAN_POINT ( 'NONE',  ( -13.89961937509957401, -13.97604488694547875, 44.37609039468566863 ) ) ;
#10850=CARTESIAN_POINT ( 'NONE',  ( -19.05341960407611168, -5.049401038298163336, 51.45724293864770260 ) ) ;
#10851=CARTESIAN_POINT ( 'NONE',  ( 16.52544592524335698, 4.483927247898782831, 76.45942372801901854 ) ) ;
#10852=CARTESIAN_POINT ( 'NONE',  ( -0.05219959533936034679, 19.03943276465977164, 97.50109039468567573 ) ) ;
#10853=CARTESIAN_POINT ( 'NONE',  ( -19.05341960407611168, -5.049401038298163336, 56.45724293864768129 ) ) ;
#10854=CARTESIAN_POINT ( 'NONE',  ( 18.67979575497178502, 10.72451020669898547, 94.16557627198103830 ) ) ;
#10855=CARTESIAN_POINT ( 'NONE',  ( 16.53943276465976808, -0.05219959533910856209, 103.7489096053143669 ) ) ;
#10856=CARTESIAN_POINT ( 'NONE',  ( -9.474510206698720793, -16.51473224551083518, 64.58442372801900433 ) ) ;
#10857=CARTESIAN_POINT ( 'NONE',  ( 18.67979575497178502, 10.72451020669898547, 59.16557627198103120 ) ) ;
#10858=CARTESIAN_POINT ( 'NONE',  ( -19.02544592524334988, -5.153800228976617603, 43.95942372801899012 ) ) ;
#10859=CARTESIAN_POINT ( 'NONE',  ( 0.05219959533909260263, 19.03943276465977164, 114.9989096053143669 ) ) ;
#10860=CARTESIAN_POINT ( 'NONE',  ( 18.67979575497178502, 10.72451020669898547, 94.16557627198103830 ) ) ;
#10861=CARTESIAN_POINT ( 'NONE',  ( -18.87075004821571511, 5.499999999999904077, 53.67408112101048800 ) ) ;
#10862=CARTESIAN_POINT ( 'NONE',  ( 19.05341960407617918, -5.049401038297876454, 106.0427570613523471 ) ) ;
#10863=CARTESIAN_POINT ( 'NONE',  ( -19.26498983726237313, 5.499999999999599432, 60.55319577422002908 ) ) ;
#10864=CARTESIAN_POINT ( 'NONE',  ( -0.05219959533934338120, 16.53943276465976808, 32.50109039468568284 ) ) ;
#10865=CARTESIAN_POINT ( 'NONE',  ( -13.89961937509977652, 13.97604488694528158, 50.62390960531435979 ) ) ;
#10866=CARTESIAN_POINT ( 'NONE',  ( 5.153800228976335163, 19.02544592524342804, 114.7905762719810241 ) ) ;
#10867=CARTESIAN_POINT ( 'NONE',  ( 18.67979575497178502, 10.72451020669898547, 84.16557627198103830 ) ) ;
#10868=CARTESIAN_POINT ( 'NONE',  ( 5.719274019375673035, 21.55341960407619339, 57.29275706135234714 ) ) ;
#10869=CARTESIAN_POINT ( 'NONE',  ( 16.55341960407618274, -4.379528057220086978, 31.04275706135234714 ) ) ;
#10870=CARTESIAN_POINT ( 'NONE',  ( -16.46253265017146816, -9.564922557961047289, 29.16775706135232937 ) ) ;
#10871=CARTESIAN_POINT ( 'NONE',  ( -16.52544592524342804, 4.483927247898546575, 36.04057627198102409 ) ) ;
#10872=CARTESIAN_POINT ( 'NONE',  ( 0.05219959533937995610, -21.53943276465977519, 20.00109039468568639 ) ) ;
#10873=CARTESIAN_POINT ( 'NONE',  ( -0.05219959533910754901, -16.53943276465976808, 52.49890960531435979 ) ) ;
#10874=CARTESIAN_POINT ( 'NONE',  ( -9.564922557961040184, 16.46253265017147172, 97.91775706135233293 ) ) ;
#10875=CARTESIAN_POINT ( 'NONE',  ( 9.564922557961047289, -16.46253265017146816, 60.41775706135233293 ) ) ;
#10876=CARTESIAN_POINT ( 'NONE',  ( 21.55341960407619695, -5.719274019375665929, 76.04275706135237556 ) ) ;
#10877=CARTESIAN_POINT ( 'NONE',  ( -0.05219959533936034679, 19.03943276465977164, 42.50109039468566152 ) ) ;
#10878=CARTESIAN_POINT ( 'NONE',  ( 5.049401038298161559, -19.05341960407611168, 22.70724293864769194 ) ) ;
#10879=CARTESIAN_POINT ( 'NONE',  ( 0.05219959533907565091, 21.53943276465977519, 49.99890960531437401 ) ) ;
#10880=CARTESIAN_POINT ( 'NONE',  ( -16.53943276465976808, 0.05219959533911058130, 31.24890960531435979 ) ) ;
#10881=CARTESIAN_POINT ( 'NONE',  ( 21.53943276465977519, 0.05219959533937863772, 111.2510903946856899 ) ) ;
#10882=CARTESIAN_POINT ( 'NONE',  ( 16.52544592524335698, 4.483927247898782831, 71.45942372801901854 ) ) ;
#10883=CARTESIAN_POINT ( 'NONE',  ( 16.52544592524342804, -4.483927247898539470, 43.54057627198103830 ) ) ;
#10884=CARTESIAN_POINT ( 'NONE',  ( -0.05219959533937732626, 21.53943276465977519, 72.50109039468568994 ) ) ;
#10885=CARTESIAN_POINT ( 'NONE',  ( 10.72451020669871369, 18.67979575497193778, 62.08442372801901143 ) ) ;
#10886=CARTESIAN_POINT ( 'NONE',  ( -15.80617190586745835, -15.72974639402198527, 66.87390960531436690 ) ) ;
#10887=CARTESIAN_POINT ( 'NONE',  ( 5.049401038298161559, -19.05341960407611168, 42.70724293864767418 ) ) ;
#10888=CARTESIAN_POINT ( 'NONE',  ( 15.72974639402176855, 15.80617190586768217, 46.87609039468568994 ) ) ;
#10889=CARTESIAN_POINT ( 'NONE',  ( 5.049401038298161559, -19.05341960407611168, 27.70724293864769550 ) ) ;
#10890=CARTESIAN_POINT ( 'NONE',  ( -19.05341960407611168, -5.049401038298163336, 41.45724293864769550 ) ) ;
#10891=CARTESIAN_POINT ( 'NONE',  ( 8.314922557960818139, 14.29746914071049879, 94.58224293864769550 ) ) ;
#10892=CARTESIAN_POINT ( 'NONE',  ( -13.89961937509977652, 13.97604488694528158, 80.62390960531436690 ) ) ;
#10893=CARTESIAN_POINT ( 'NONE',  ( 4.483927247898545687, 16.52544592524342804, 34.79057627198103120 ) ) ;
#10894=CARTESIAN_POINT ( 'NONE',  ( -4.379528057220328563, 16.55341960407611168, 95.20724293864769550 ) ) ;
#10895=CARTESIAN_POINT ( 'NONE',  ( 18.67979575497178502, 10.72451020669898547, 64.16557627198102409 ) ) ;
#10896=CARTESIAN_POINT ( 'NONE',  ( -10.81492255796078084, -18.62759615963271287, 112.0822429386477097 ) ) ;
#10898=CARTESIAN_POINT ( 'NONE',  ( -19.03943276465977164, 0.05219959533909376836, 61.24890960531436690 ) ) ;
#10899=CARTESIAN_POINT ( 'NONE',  ( -8.224510206698735004, -14.34966873604973081, 29.58442372801901854 ) ) ;
#10900=CARTESIAN_POINT ( 'NONE',  ( -0.05219959533907301413, -21.53943276465977519, 52.49890960531435979 ) ) ;
#10901=CARTESIAN_POINT ( 'NONE',  ( -21.52544592524334988, -5.823673210054445271, 93.95942372801903275 ) ) ;
#10902=CARTESIAN_POINT ( 'NONE',  ( 19.05341960407611168, 5.049401038298154454, 83.95724293864766707 ) ) ;
#10903=CARTESIAN_POINT ( 'NONE',  ( -18.62759615963255300, -10.81492255796106328, 19.16775706135234714 ) ) ;
#10905=CARTESIAN_POINT ( 'NONE',  ( 9.564922557960805705, 16.46253265017160317, 114.5822429386476955 ) ) ;
#10906=CARTESIAN_POINT ( 'NONE',  ( 12.06949235617739724, 12.14591786802326823, 91.87609039468568994 ) ) ;
#10907=CARTESIAN_POINT ( 'NONE',  ( -15.80617190586768217, 15.72974639402176855, 68.12609039468567573 ) ) ;
#10908=CARTESIAN_POINT ( 'NONE',  ( -21.53943276465977519, -0.05219959533937600094, 98.75109039468568994 ) ) ;
#10909=CARTESIAN_POINT ( 'NONE',  ( 4.483927247898790824, -16.52544592524335698, 65.20942372801901854 ) ) ;
#10910=CARTESIAN_POINT ( 'NONE',  ( -18.67979575497193778, 10.72451020669871902, 28.33442372801902209 ) ) ;
#10911=CARTESIAN_POINT ( 'NONE',  ( 19.03943276465977164, -0.05219959533909143690, 23.74890960531435269 ) ) ;
#10912=CARTESIAN_POINT ( 'NONE',  ( -21.52544592524334988, -5.823673210054445271, 88.95942372801901854 ) ) ;
#10913=CARTESIAN_POINT ( 'NONE',  ( -19.03943276465977164, 0.05219959533909376836, 96.24890960531436690 ) ) ;
#10914=CARTESIAN_POINT ( 'NONE',  ( -18.62759615963270932, 10.81492255796079327, 85.83224293864768129 ) ) ;
#10915=CARTESIAN_POINT ( 'NONE',  ( -13.97604488694547697, 13.89961937509957934, 63.12609039468566152 ) ) ;
#10916=CARTESIAN_POINT ( 'NONE',  ( 18.67979575497178502, 10.72451020669898547, 49.16557627198102409 ) ) ;
#10917=CARTESIAN_POINT ( 'NONE',  ( 9.474510206698971260, -16.51473224551069308, 92.91557627198103830 ) ) ;
#10918=CARTESIAN_POINT ( 'NONE',  ( -8.224510206698948167, 14.34966873604960824, 40.41557627198103120 ) ) ;
#10920=CARTESIAN_POINT ( 'NONE',  ( -0.05219959533936034679, 19.03943276465977164, 62.50109039468566863 ) ) ;
#10921=CARTESIAN_POINT ( 'NONE',  ( -19.19724070472094013, -5.500000000000079936, 81.06193348274383936 ) ) ;
#10922=CARTESIAN_POINT ( 'NONE',  ( 13.97604488694548053, -13.89961937509957401, 105.6260903946856757 ) ) ;
#10923=CARTESIAN_POINT ( 'NONE',  ( 21.52544592524344225, -5.823673210054117533, 78.54057627198103830 ) ) ;
#10924=CARTESIAN_POINT ( 'NONE',  ( -14.34966873604960291, -8.224510206698953496, 46.66557627198102409 ) ) ;
#10925=CARTESIAN_POINT ( 'NONE',  ( 14.34966873604972726, -8.224510206698740333, 25.83442372801901499 ) ) ;
#10926=CARTESIAN_POINT ( 'NONE',  ( -16.46253265017160317, 9.564922557960807481, 50.83224293864770260 ) ) ;
#10927=CARTESIAN_POINT ( 'NONE',  ( -10.81492255796105439, 18.62759615963255655, 22.91775706135235069 ) ) ;
#10928=CARTESIAN_POINT ( 'NONE',  ( 13.97604488694548053, -13.89961937509957401, 80.62609039468567573 ) ) ;
#10929=CARTESIAN_POINT ( 'NONE',  ( -5.049401038298153566, 19.05341960407611168, 90.20724293864766707 ) ) ;
#10930=CARTESIAN_POINT ( 'NONE',  ( 19.05341960407611168, 5.049401038298154454, 73.95724293864768129 ) ) ;
#10931=CARTESIAN_POINT ( 'NONE',  ( -21.55341960407610458, -5.719274019375992779, 81.45724293864769550 ) ) ;
#10932=CARTESIAN_POINT ( 'NONE',  ( -5.049401038298153566, 19.05341960407611168, 50.20724293864770260 ) ) ;
#10934=CARTESIAN_POINT ( 'NONE',  ( -8.314922557960811034, -14.29746914071050412, 52.08224293864768839 ) ) ;
#10935=CARTESIAN_POINT ( 'NONE',  ( 19.03943276465977164, -0.05219959533909143690, 93.74890960531435269 ) ) ;
#10937=CARTESIAN_POINT ( 'NONE',  ( 19.02544592524334988, 5.153800228976608722, 71.45942372801900433 ) ) ;
#10938=CARTESIAN_POINT ( 'NONE',  ( -5.823673210054116645, -21.52544592524344225, 72.29057627198102409 ) ) ;
#10939=CARTESIAN_POINT ( 'NONE',  ( 5.049401038297881783, 19.05341960407617563, 37.29275706135232582 ) ) ;
#10940=CARTESIAN_POINT ( 'NONE',  ( 5.153800228976335163, 19.02544592524342804, 99.79057627198102409 ) ) ;
#10941=CARTESIAN_POINT ( 'NONE',  ( -17.49999999999999645, 3.565345528327948710, 114.4249448680647276 ) ) ;
#10942=CARTESIAN_POINT ( 'NONE',  ( 10.72451020669898902, -18.67979575497178502, 42.91557627198103120 ) ) ;
#10943=CARTESIAN_POINT ( 'NONE',  ( 19.02544592524343514, -5.153800228976328945, 78.54057627198099567 ) ) ;
#10944=CARTESIAN_POINT ( 'NONE',  ( 18.67979575497194134, -10.72451020669871369, 60.83442372801901854 ) ) ;
#10945=CARTESIAN_POINT ( 'NONE',  ( 13.89961937509977652, -13.97604488694527269, 23.12390960531436335 ) ) ;
#10946=CARTESIAN_POINT ( 'NONE',  ( -10.81492255796105439, 18.62759615963255655, 22.91775706135235069 ) ) ;
#10947=EDGE_LOOP ( 'NONE', ( #98390, #76097, #93621, #165339 ) ) ;
#10948=CARTESIAN_POINT ( 'NONE',  ( -10.72451020669870658, -18.67979575497194134, 49.58442372801901143 ) ) ;
#10950=CARTESIAN_POINT ( 'NONE',  ( -16.46253265017160317, 9.564922557960807481, 115.8322429386477097 ) ) ;
#10951=CARTESIAN_POINT ( 'NONE',  ( 16.46253265017146816, 9.564922557961045513, 61.66775706135234003 ) ) ;
#10953=CARTESIAN_POINT ( 'NONE',  ( 21.53943276465977519, -0.05219959533907433946, 103.7489096053143669 ) ) ;
#10954=CARTESIAN_POINT ( 'NONE',  ( -13.89961937509977652, 13.97604488694528158, 60.62390960531436690 ) ) ;
#10955=CARTESIAN_POINT ( 'NONE',  ( -8.224510206698735004, -14.34966873604973081, 39.58442372801901143 ) ) ;
#10957=CARTESIAN_POINT ( 'NONE',  ( -18.67979575497193778, 10.72451020669871902, 103.3344237280190043 ) ) ;
#10958=CARTESIAN_POINT ( 'NONE',  ( 19.05341960407611168, 5.049401038298154454, 48.95724293864768129 ) ) ;
#10959=CARTESIAN_POINT ( 'NONE',  ( 18.67979575497194134, -10.72451020669871369, 95.83442372801903275 ) ) ;
#10960=CARTESIAN_POINT ( 'NONE',  ( 13.89961937509977652, -13.97604488694527269, 83.12390960531436690 ) ) ;
#10961=CARTESIAN_POINT ( 'NONE',  ( 18.62759615963255655, 10.81492255796105972, 56.66775706135235424 ) ) ;
#10963=CARTESIAN_POINT ( 'NONE',  ( 0.05219959533909260263, 19.03943276465977164, 114.9989096053143669 ) ) ;
#10965=CARTESIAN_POINT ( 'NONE',  ( -16.53943276465976808, -0.05219959533934237506, 58.75109039468568994 ) ) ;
#10966=CARTESIAN_POINT ( 'NONE',  ( -21.55341960407619339, 5.719274019375674811, 68.54275706135234714 ) ) ;
#10967=CARTESIAN_POINT ( 'NONE',  ( 0.05219959533937995610, -21.53943276465977519, 95.00109039468568994 ) ) ;
#10970=CARTESIAN_POINT ( 'NONE',  ( -14.29746914071037622, -8.314922557961029526, 24.16775706135235424 ) ) ;
#10971=CARTESIAN_POINT ( 'NONE',  ( 5.049401038298161559, -19.05341960407611168, 87.70724293864769550 ) ) ;
#10972=CARTESIAN_POINT ( 'NONE',  ( -16.46253265017160317, 9.564922557960807481, 115.8322429386477097 ) ) ;
#10974=CARTESIAN_POINT ( 'NONE',  ( -17.49999999999999645, -5.500000000000000000, 111.2823096230356725 ) ) ;
#10975=CARTESIAN_POINT ( 'NONE',  ( 4.483927247898545687, 16.52544592524342804, 114.7905762719810383 ) ) ;
#10976=CARTESIAN_POINT ( 'NONE',  ( -15.72974639402197994, 15.80617190586746368, 45.62390960531436690 ) ) ;
#10977=CARTESIAN_POINT ( 'NONE',  ( -16.52544592524335698, -4.483927247898792601, 93.95942372801903275 ) ) ;
#10978=CARTESIAN_POINT ( 'NONE',  ( -4.483927247898539470, -16.52544592524342804, 82.29057627198103830 ) ) ;
#10979=CARTESIAN_POINT ( 'NONE',  ( -16.46253265017160317, 9.564922557960807481, 65.83224293864769550 ) ) ;
#10980=CARTESIAN_POINT ( 'NONE',  ( 5.719274019375673035, 21.55341960407619339, 87.29275706135236135 ) ) ;
#10982=CARTESIAN_POINT ( 'NONE',  ( -19.03943276465977164, -0.05219959533935918106, 113.7510903946856757 ) ) ;
#10983=CARTESIAN_POINT ( 'NONE',  ( -4.379528057220328563, 16.55341960407611168, 85.20724293864770971 ) ) ;
#10984=CARTESIAN_POINT ( 'NONE',  ( 21.55341960407619695, -5.719274019375665929, 41.04275706135236135 ) ) ;
#10985=CARTESIAN_POINT ( 'NONE',  ( -0.05219959533907301413, -21.53943276465977519, 72.49890960531435269 ) ) ;
#10986=CARTESIAN_POINT ( 'NONE',  ( 16.51473224551083163, -9.474510206698727899, 35.83442372801899722 ) ) ;
#10988=CARTESIAN_POINT ( 'NONE',  ( -16.51473224551069308, -9.474510206698971260, 81.66557627198103830 ) ) ;
#10989=CARTESIAN_POINT ( 'NONE',  ( 14.34966873604960469, 8.224510206698951720, 69.16557627198102409 ) ) ;
#10991=CARTESIAN_POINT ( 'NONE',  ( -14.34966873604960291, -8.224510206698953496, 36.66557627198103120 ) ) ;
#10992=CARTESIAN_POINT ( 'NONE',  ( -4.483927247898782831, 16.52544592524335698, 107.7094237280190328 ) ) ;
#10993=CARTESIAN_POINT ( 'NONE',  ( -13.89961937509957401, -13.97604488694547875, 59.37609039468566863 ) ) ;
#10994=CARTESIAN_POINT ( 'NONE',  ( 19.49190055781009434, 5.500000000000042633, 53.06116087098784817 ) ) ;
#10995=CARTESIAN_POINT ( 'NONE',  ( -10.72451020669898014, 18.67979575497178502, 25.41557627198103120 ) ) ;
#10996=CARTESIAN_POINT ( 'NONE',  ( 12.06949235617757843, -12.14591786802309237, 88.12390960531436690 ) ) ;
#10998=CARTESIAN_POINT ( 'NONE',  ( -0.05219959533909027116, -19.03943276465977164, 47.49890960531435979 ) ) ;
#10999=CARTESIAN_POINT ( 'NONE',  ( -21.55341960407610458, -5.719274019375992779, 46.45724293864769550 ) ) ;
#11000=CARTESIAN_POINT ( 'NONE',  ( -10.81492255796078084, -18.62759615963271287, 67.08224293864770971 ) ) ;
#11001=CARTESIAN_POINT ( 'NONE',  ( 4.379528057220339221, -16.55341960407611168, 112.7072429386476955 ) ) ;
#11002=CARTESIAN_POINT ( 'NONE',  ( -8.224510206698735004, -14.34966873604973081, 69.58442372801900433 ) ) ;
#11003=CARTESIAN_POINT ( 'NONE',  ( 0.05219959533909260263, 19.03943276465977164, 49.99890960531435979 ) ) ;
#11004=CARTESIAN_POINT ( 'NONE',  ( 10.72451020669871369, 18.67979575497193778, 57.08442372801901854 ) ) ;
#11005=CARTESIAN_POINT ( 'NONE',  ( -16.53943276465976808, 0.05219959533911058130, 111.2489096053143669 ) ) ;
#11006=CARTESIAN_POINT ( 'NONE',  ( -13.97604488694547697, 13.89961937509957934, 93.12609039468566152 ) ) ;
#11008=CARTESIAN_POINT ( 'NONE',  ( 17.49999999999999645, 5.099703775204536882, 36.76678814087944147 ) ) ;
#11009=CARTESIAN_POINT ( 'NONE',  ( -21.55341960407610458, -5.719274019375992779, 51.45724293864770260 ) ) ;
#11010=CARTESIAN_POINT ( 'NONE',  ( 0.05219959533909260263, 19.03943276465977164, 24.99890960531435269 ) ) ;
#11011=CARTESIAN_POINT ( 'NONE',  ( 5.719274019375673035, 21.55341960407619339, 82.29275706135234714 ) ) ;
#11012=CARTESIAN_POINT ( 'NONE',  ( -8.224510206698948167, 14.34966873604960824, 30.41557627198101699 ) ) ;
#11013=CARTESIAN_POINT ( 'NONE',  ( -16.55341960407617563, 4.379528057220093196, 58.54275706135235424 ) ) ;
#11014=CARTESIAN_POINT ( 'NONE',  ( -8.314922557960811034, -14.29746914071050412, 37.08224293864768129 ) ) ;
#11015=CARTESIAN_POINT ( 'NONE',  ( 21.52544592524344225, -5.823673210054117533, 68.54057627198103830 ) ) ;
#11016=CARTESIAN_POINT ( 'NONE',  ( -21.52544592524343514, 5.823673210054127303, 76.04057627198102409 ) ) ;
#11018=CARTESIAN_POINT ( 'NONE',  ( 19.02544592524334988, 5.153800228976608722, 86.45942372801900433 ) ) ;
#11019=CARTESIAN_POINT ( 'NONE',  ( 5.049401038298161559, -19.05341960407611168, 112.7072429386476813 ) ) ;
#11020=CARTESIAN_POINT ( 'NONE',  ( 13.89961937509977652, -13.97604488694527269, 53.12390960531434558 ) ) ;
#11021=CARTESIAN_POINT ( 'NONE',  ( 0.05219959533910956823, 16.53943276465976808, 114.9989096053143669 ) ) ;
#11023=ORIENTED_EDGE ( 'NONE', *, *, #97826, .T. ) ;
#11024=CARTESIAN_POINT ( 'NONE',  ( 4.379528057220092307, 16.55341960407617563, 87.29275706135236135 ) ) ;
#11025=CARTESIAN_POINT ( 'NONE',  ( -15.80617190586745835, -15.72974639402198527, 106.8739096053143811 ) ) ;
#11026=CARTESIAN_POINT ( 'NONE',  ( -9.474510206698964154, 16.51473224551069663, 65.41557627198102409 ) ) ;
#11027=CARTESIAN_POINT ( 'NONE',  ( -21.53943276465977519, -0.05219959533937600094, 43.75109039468568284 ) ) ;
#11028=CARTESIAN_POINT ( 'NONE',  ( -16.51473224551069308, -9.474510206698971260, 91.66557627198103830 ) ) ;
#11030=ORIENTED_EDGE ( 'NONE', *, *, #121212, .F. ) ;
#11031=CARTESIAN_POINT ( 'NONE',  ( 21.53943276465977519, 0.05219959533937863772, 26.25109039468567573 ) ) ;
#11032=CARTESIAN_POINT ( 'NONE',  ( 19.02544592524343514, -5.153800228976328945, 23.54057627198102054 ) ) ;
#11033=CARTESIAN_POINT ( 'NONE',  ( -16.51473224551082808, 9.474510206698731452, 93.33442372801900433 ) ) ;
#11034=CARTESIAN_POINT ( 'NONE',  ( -19.03943276465977164, -0.05219959533935918106, 43.75109039468566863 ) ) ;
#11035=CARTESIAN_POINT ( 'NONE',  ( 10.72451020669871369, 18.67979575497193778, 22.08442372801901143 ) ) ;
#11036=CARTESIAN_POINT ( 'NONE',  ( 0.05219959533936267826, -19.03943276465977164, 30.00109039468566863 ) ) ;
#11037=CARTESIAN_POINT ( 'NONE',  ( -19.03943276465977164, -0.05219959533935918106, 53.75109039468566863 ) ) ;
#11038=CARTESIAN_POINT ( 'NONE',  ( 14.34966873604972726, -8.224510206698740333, 90.83442372801901854 ) ) ;
#11039=CARTESIAN_POINT ( 'NONE',  ( 30.00000000000000000, 5.499999999999992895, 102.5000000000000142 ) ) ;
#11041=CARTESIAN_POINT ( 'NONE',  ( -0.05219959533909027116, -19.03943276465977164, 72.49890960531435269 ) ) ;
#11042=CARTESIAN_POINT ( 'NONE',  ( 5.823673210054444382, -21.52544592524334988, 80.20942372801901854 ) ) ;
#11043=CARTESIAN_POINT ( 'NONE',  ( 18.67979575497194134, -10.72451020669871369, 100.8344237280190185 ) ) ;
#11045=CARTESIAN_POINT ( 'NONE',  ( -19.03943276465977164, 0.05219959533909376836, 86.24890960531436690 ) ) ;
#11046=CARTESIAN_POINT ( 'NONE',  ( 21.53943276465977519, 0.05219959533937863772, 61.25109039468567573 ) ) ;
#11047=CARTESIAN_POINT ( 'NONE',  ( 5.153800228976615827, -19.02544592524334988, 95.20942372801897591 ) ) ;
#11048=CARTESIAN_POINT ( 'NONE',  ( -5.153800228976328057, -19.02544592524343514, 62.29057627198100988 ) ) ;
#11049=CARTESIAN_POINT ( 'NONE',  ( -5.823673210054116645, -21.52544592524344225, 22.29057627198102765 ) ) ;
#11051=CARTESIAN_POINT ( 'NONE',  ( 0.05219959533909260263, 19.03943276465977164, 74.99890960531435269 ) ) ;
#11052=CARTESIAN_POINT ( 'NONE',  ( -17.50000000000001066, -5.622605283950841581, 91.31207310596107618 ) ) ;
#11053=CARTESIAN_POINT ( 'NONE',  ( 19.03943276465977164, -0.05219959533909143690, 58.74890960531435979 ) ) ;
#11054=CARTESIAN_POINT ( 'NONE',  ( -19.02544592524342804, 5.153800228976336051, 56.04057627198100988 ) ) ;
#11055=CARTESIAN_POINT ( 'NONE',  ( -10.72451020669870658, -18.67979575497194134, 19.58442372801901143 ) ) ;
#11056=CARTESIAN_POINT ( 'NONE',  ( 14.29746914071037800, 8.314922557961029526, 96.66775706135234714 ) ) ;
#11059=CARTESIAN_POINT ( 'NONE',  ( 5.049401038297881783, 19.05341960407617563, 52.29275706135234003 ) ) ;
#11060=CARTESIAN_POINT ( 'NONE',  ( -0.05219959533909027116, -19.03943276465977164, 77.49890960531435269 ) ) ;
#11061=CARTESIAN_POINT ( 'NONE',  ( -14.34966873604960291, -8.224510206698953496, 76.66557627198103830 ) ) ;
#11062=CARTESIAN_POINT ( 'NONE',  ( -14.29746914071049879, 8.314922557960819915, 105.8322429386476955 ) ) ;
#11063=CARTESIAN_POINT ( 'NONE',  ( 15.80617190586746368, 15.72974639402197994, 34.37390960531435979 ) ) ;
#11064=CARTESIAN_POINT ( 'NONE',  ( -19.03943276465977164, 0.05219959533909376836, 111.2489096053143669 ) ) ;
#11065=CARTESIAN_POINT ( 'NONE',  ( 0.05219959533910956823, 16.53943276465976808, 94.99890960531436690 ) ) ;
#11066=CARTESIAN_POINT ( 'NONE',  ( 9.474510206698971260, -16.51473224551069308, 82.91557627198103830 ) ) ;
#11067=CARTESIAN_POINT ( 'NONE',  ( -0.05219959533936034679, 19.03943276465977164, 27.50109039468566507 ) ) ;
#11068=CARTESIAN_POINT ( 'NONE',  ( 8.314922557961029526, -14.29746914071037800, 105.4177570613523613 ) ) ;
#11069=CARTESIAN_POINT ( 'NONE',  ( -9.564922557960796823, -16.46253265017161027, 87.08224293864769550 ) ) ;
#11070=CARTESIAN_POINT ( 'NONE',  ( -15.80617190586768217, 15.72974639402176855, 53.12609039468568284 ) ) ;
#11071=CARTESIAN_POINT ( 'NONE',  ( -18.67979575497178146, -10.72451020669898902, 41.66557627198103120 ) ) ;
#11072=CARTESIAN_POINT ( 'NONE',  ( -0.05219959533907301413, -21.53943276465977519, 112.4989096053143669 ) ) ;
#11073=CARTESIAN_POINT ( 'NONE',  ( 10.81492255796078972, 18.62759615963270932, 74.58224293864768129 ) ) ;
#11074=CARTESIAN_POINT ( 'NONE',  ( -12.14591786802309592, -12.06949235617757132, 91.87390960531436690 ) ) ;
#11075=CARTESIAN_POINT ( 'NONE',  ( -0.05219959533936034679, 19.03943276465977164, 57.50109039468566863 ) ) ;
#11076=EDGE_CURVE ( 'NONE', #82999, #84229, #111277, .T. ) ;
#11078=CARTESIAN_POINT ( 'NONE',  ( -13.97604488694527625, -13.89961937509977652, 31.87390960531435979 ) ) ;
#11079=CARTESIAN_POINT ( 'NONE',  ( -16.46253265017160317, 9.564922557960807481, 95.83224293864769550 ) ) ;
#11080=CARTESIAN_POINT ( 'NONE',  ( 16.46253265017160672, -9.564922557960803928, 98.33224293864769550 ) ) ;
#11081=CARTESIAN_POINT ( 'NONE',  ( 14.34966873604960469, 8.224510206698951720, 109.1655762719810383 ) ) ;
#11082=CARTESIAN_POINT ( 'NONE',  ( -14.34966873604960291, -8.224510206698953496, 26.66557627198103475 ) ) ;
#11083=CARTESIAN_POINT ( 'NONE',  ( 16.55341960407618274, -4.379528057220086978, 46.04275706135234714 ) ) ;
#11084=CARTESIAN_POINT ( 'NONE',  ( -21.52544592524334988, -5.823673210054445271, 103.9594237280190185 ) ) ;
#11085=CARTESIAN_POINT ( 'NONE',  ( -9.474510206698964154, 16.51473224551069663, 105.4155762719810383 ) ) ;
#11086=CARTESIAN_POINT ( 'NONE',  ( 14.29746914071049879, -8.314922557960816363, 28.33224293864769550 ) ) ;
#11087=CARTESIAN_POINT ( 'NONE',  ( -18.62759615963255300, -10.81492255796106328, 29.16775706135234003 ) ) ;
#11088=CARTESIAN_POINT ( 'NONE',  ( 5.153800228976335163, 19.02544592524342804, 39.79057627198100988 ) ) ;
#11089=CARTESIAN_POINT ( 'NONE',  ( -0.05219959533934338120, 16.53943276465976808, 47.50109039468568994 ) ) ;
#11090=CARTESIAN_POINT ( 'NONE',  ( 14.34966873604972726, -8.224510206698740333, 110.8344237280190043 ) ) ;
#11091=CARTESIAN_POINT ( 'NONE',  ( -14.34966873604972548, 8.224510206698743886, 98.33442372801901854 ) ) ;
#11093=CARTESIAN_POINT ( 'NONE',  ( 0.05219959533936267826, -19.03943276465977164, 105.0010903946856615 ) ) ;
#11094=CARTESIAN_POINT ( 'NONE',  ( 16.51473224551069308, 9.474510206698969483, 29.16557627198103475 ) ) ;
#11095=CARTESIAN_POINT ( 'NONE',  ( 14.34966873604960469, 8.224510206698951720, 94.16557627198103830 ) ) ;
#11096=CARTESIAN_POINT ( 'NONE',  ( -15.80617190586745835, -15.72974639402198527, 106.8739096053143811 ) ) ;
#11097=CARTESIAN_POINT ( 'NONE',  ( -9.564922557960796823, -16.46253265017161027, 32.08224293864769550 ) ) ;
#11098=CARTESIAN_POINT ( 'NONE',  ( -5.153800228976328057, -19.02544592524343514, 102.2905762719810383 ) ) ;
#11099=CARTESIAN_POINT ( 'NONE',  ( -5.823673210054431948, 21.52544592524334988, 27.70942372801901854 ) ) ;
#11101=CARTESIAN_POINT ( 'NONE',  ( 19.02544592524343514, -5.153800228976328945, 103.5405762719809957 ) ) ;
#11103=CARTESIAN_POINT ( 'NONE',  ( 17.50000000000000355, -5.624438216177584771, 113.3167034491464307 ) ) ;
#11104=CARTESIAN_POINT ( 'NONE',  ( 13.97604488694527802, 13.89961937509977652, 79.37390960531435269 ) ) ;
#11105=CARTESIAN_POINT ( 'NONE',  ( 5.719274019375673035, 21.55341960407619339, 37.29275706135235424 ) ) ;
#11106=CARTESIAN_POINT ( 'NONE',  ( -16.53943276465976808, 0.05219959533911058130, 96.24890960531435269 ) ) ;
#11107=CARTESIAN_POINT ( 'NONE',  ( -16.46253265017160317, 9.564922557960807481, 95.83224293864769550 ) ) ;
#11108=CARTESIAN_POINT ( 'NONE',  ( -19.03943276465977164, -0.05219959533935918106, 28.75109039468566507 ) ) ;
#11109=CARTESIAN_POINT ( 'NONE',  ( -8.224510206698735004, -14.34966873604973081, 59.58442372801901854 ) ) ;
#11110=CARTESIAN_POINT ( 'NONE',  ( 18.62759615963255655, 10.81492255796105972, 76.66775706135234714 ) ) ;
#11111=CARTESIAN_POINT ( 'NONE',  ( 14.29746914071037800, 8.314922557961029526, 36.66775706135234714 ) ) ;
#11112=CARTESIAN_POINT ( 'NONE',  ( -9.564922557960796823, -16.46253265017161027, 77.08224293864769550 ) ) ;
#11113=CARTESIAN_POINT ( 'NONE',  ( -13.89961937509957401, -13.97604488694547875, 89.37609039468563310 ) ) ;
#11114=CARTESIAN_POINT ( 'NONE',  ( -12.14591786802326823, 12.06949235617739902, 63.12609039468568994 ) ) ;
#11115=CARTESIAN_POINT ( 'NONE',  ( 5.719274019375673035, 21.55341960407619339, 107.2927570613523471 ) ) ;
#11116=CARTESIAN_POINT ( 'NONE',  ( -13.97604488694547697, 13.89961937509957934, 98.12609039468566152 ) ) ;
#11117=CARTESIAN_POINT ( 'NONE',  ( -19.05341960407611168, -5.049401038298163336, 66.45724293864769550 ) ) ;
#11118=CARTESIAN_POINT ( 'NONE',  ( -18.67979575497178146, -10.72451020669898902, 86.66557627198102409 ) ) ;
#11119=CARTESIAN_POINT ( 'NONE',  ( 4.379528057220339221, -16.55341960407611168, 92.70724293864770971 ) ) ;
#11120=CARTESIAN_POINT ( 'NONE',  ( -9.564922557961040184, 16.46253265017147172, 92.91775706135233293 ) ) ;
#11121=CARTESIAN_POINT ( 'NONE',  ( 16.52544592524335698, 4.483927247898782831, 61.45942372801901854 ) ) ;
#11123=CARTESIAN_POINT ( 'NONE',  ( 19.02544592524334988, 5.153800228976608722, 61.45942372801900433 ) ) ;
#11124=CARTESIAN_POINT ( 'NONE',  ( -12.14591786802326823, 12.06949235617739902, 108.1260903946856757 ) ) ;
#11125=CARTESIAN_POINT ( 'NONE',  ( 8.224510206698953496, -14.34966873604960469, 77.91557627198102409 ) ) ;
#11126=CARTESIAN_POINT ( 'NONE',  ( 13.89961937509957401, 13.97604488694547697, 26.87609039468566507 ) ) ;
#11127=CARTESIAN_POINT ( 'NONE',  ( -19.52837319214027900, 5.499999999999900524, 89.60471352585535953 ) ) ;
#11128=CARTESIAN_POINT ( 'NONE',  ( 5.719274019375673035, 21.55341960407619339, 22.29275706135235069 ) ) ;
#11129=CARTESIAN_POINT ( 'NONE',  ( 5.049401038298161559, -19.05341960407611168, 107.7072429386476955 ) ) ;
#11130=CARTESIAN_POINT ( 'NONE',  ( 5.153800228976335163, 19.02544592524342804, 84.79057627198099567 ) ) ;
#11131=CARTESIAN_POINT ( 'NONE',  ( 5.719274019375673035, 21.55341960407619339, 82.29275706135234714 ) ) ;
#11132=CARTESIAN_POINT ( 'NONE',  ( 16.51473224551069308, 9.474510206698969483, 59.16557627198102409 ) ) ;
#11134=CARTESIAN_POINT ( 'NONE',  ( 15.72974639402199770, -15.80617190586745480, 33.12390960531435979 ) ) ;
#11135=CARTESIAN_POINT ( 'NONE',  ( -16.53943276465976808, 0.05219959533911058130, 76.24890960531435269 ) ) ;
#11136=CARTESIAN_POINT ( 'NONE',  ( 0.05219959533909260263, 19.03943276465977164, 39.99890960531436690 ) ) ;
#11137=CARTESIAN_POINT ( 'NONE',  ( -8.314922557960811034, -14.29746914071050412, 102.0822429386476955 ) ) ;
#11139=CARTESIAN_POINT ( 'NONE',  ( 0.05219959533907565091, 21.53943276465977519, 104.9989096053143669 ) ) ;
#11140=CARTESIAN_POINT ( 'NONE',  ( 21.53943276465977519, 0.05219959533937863772, 66.25109039468567573 ) ) ;
#11141=CARTESIAN_POINT ( 'NONE',  ( 19.05341960407611168, 5.049401038298154454, 33.95724293864769550 ) ) ;
#11142=CARTESIAN_POINT ( 'NONE',  ( -14.34966873604972548, 8.224510206698743886, 68.33442372801900433 ) ) ;
#11143=CARTESIAN_POINT ( 'NONE',  ( 21.53943276465977519, -0.05219959533907433946, 103.7489096053143669 ) ) ;
#11144=CARTESIAN_POINT ( 'NONE',  ( -21.53943276465977519, -0.05219959533937600094, 18.75109039468568639 ) ) ;
#11145=CARTESIAN_POINT ( 'NONE',  ( 16.51473224551083163, -9.474510206698727899, 40.83442372801900433 ) ) ;
#11146=CARTESIAN_POINT ( 'NONE',  ( -5.153800228976328057, -19.02544592524343514, 57.29057627198103120 ) ) ;
#11147=CARTESIAN_POINT ( 'NONE',  ( -17.60769864724389677, 5.499999999999980460, 83.65024842019165874 ) ) ;
#11148=CARTESIAN_POINT ( 'NONE',  ( -15.72974639402176322, -15.80617190586768395, 59.37609039468568284 ) ) ;
#11149=CARTESIAN_POINT ( 'NONE',  ( 15.80617190586746368, 15.72974639402197994, 59.37390960531436690 ) ) ;
#11150=CARTESIAN_POINT ( 'NONE',  ( 8.224510206698953496, -14.34966873604960469, 32.91557627198102409 ) ) ;
#11151=CARTESIAN_POINT ( 'NONE',  ( -15.80617190586768217, 15.72974639402176855, 83.12609039468568994 ) ) ;
#11152=CARTESIAN_POINT ( 'NONE',  ( -21.53943276465977519, -0.05219959533937600094, 113.7510903946856757 ) ) ;
#11153=CARTESIAN_POINT ( 'NONE',  ( -16.52544592524342804, 4.483927247898546575, 56.04057627198102409 ) ) ;
#11154=CARTESIAN_POINT ( 'NONE',  ( 14.29746914071049879, -8.314922557960816363, 108.3322429386477097 ) ) ;
#11155=CARTESIAN_POINT ( 'NONE',  ( 0.05219959533936267826, -19.03943276465977164, 50.00109039468566863 ) ) ;
#11156=CARTESIAN_POINT ( 'NONE',  ( -4.379528057220086978, -16.55341960407618274, 104.7927570613523898 ) ) ;
#11157=CARTESIAN_POINT ( 'NONE',  ( 18.67979575497194134, -10.72451020669871369, 65.83442372801900433 ) ) ;
#11158=CARTESIAN_POINT ( 'NONE',  ( 19.05341960407611168, 5.049401038298154454, 63.95724293864769550 ) ) ;
#11159=CARTESIAN_POINT ( 'NONE',  ( 9.474510206698729675, 16.51473224551082808, 37.08442372801899722 ) ) ;
#11160=CARTESIAN_POINT ( 'NONE',  ( -0.05219959533907301413, -21.53943276465977519, 32.49890960531435979 ) ) ;
#11161=CARTESIAN_POINT ( 'NONE',  ( -18.62759615963255300, -10.81492255796106328, 29.16775706135234003 ) ) ;
#11162=CARTESIAN_POINT ( 'NONE',  ( -0.05219959533907301413, -21.53943276465977519, 82.49890960531436690 ) ) ;
#11163=CARTESIAN_POINT ( 'NONE',  ( -19.05341960407617563, 5.049401038297882671, 83.54275706135233293 ) ) ;
#11164=CARTESIAN_POINT ( 'NONE',  ( -12.14591786802326823, 12.06949235617739902, 53.12609039468568284 ) ) ;
#11165=CARTESIAN_POINT ( 'NONE',  ( 17.50000000000002132, -3.734851586428651782, 36.81917961330525202 ) ) ;
#11166=CARTESIAN_POINT ( 'NONE',  ( 21.53943276465977519, -0.05219959533907433946, 88.74890960531436690 ) ) ;
#11167=CARTESIAN_POINT ( 'NONE',  ( -8.224510206698948167, 14.34966873604960824, 75.41557627198102409 ) ) ;
#11168=CARTESIAN_POINT ( 'NONE',  ( -17.05116617787824396, -6.768360034955821725, 101.3432444674080415 ) ) ;
#11169=CARTESIAN_POINT ( 'NONE',  ( 19.05341960407617918, -5.049401038297876454, 111.0427570613523329 ) ) ;
#11170=CARTESIAN_POINT ( 'NONE',  ( 18.67979575497178502, 10.72451020669898547, 39.16557627198102409 ) ) ;
#11171=CARTESIAN_POINT ( 'NONE',  ( -4.483927247898782831, 16.52544592524335698, 82.70942372801900433 ) ) ;
#11172=CARTESIAN_POINT ( 'NONE',  ( -17.49999999999999645, 7.499999999999998224, 118.0000000000000142 ) ) ;
#11173=CARTESIAN_POINT ( 'NONE',  ( 16.55341960407618274, -4.379528057220086978, 56.04275706135235424 ) ) ;
#11174=CARTESIAN_POINT ( 'NONE',  ( -21.55341960407619339, 5.719274019375674811, 33.54275706135234714 ) ) ;
#11175=CARTESIAN_POINT ( 'NONE',  ( 18.62759615963271287, -10.81492255796078972, 43.33224293864769550 ) ) ;
#11176=CARTESIAN_POINT ( 'NONE',  ( 4.379528057220092307, 16.55341960407617563, 67.29275706135234714 ) ) ;
#11177=CARTESIAN_POINT ( 'NONE',  ( 9.564922557960805705, 16.46253265017160317, 89.58224293864769550 ) ) ;
#11178=CARTESIAN_POINT ( 'NONE',  ( -15.72974639402176322, -15.80617190586768395, 59.37609039468568284 ) ) ;
#11179=CARTESIAN_POINT ( 'NONE',  ( 19.05341960407611168, 5.049401038298154454, 28.95724293864769550 ) ) ;
#11180=CARTESIAN_POINT ( 'NONE',  ( -15.80617190586745835, -15.72974639402198527, 36.87390960531435979 ) ) ;
#11181=CARTESIAN_POINT ( 'NONE',  ( -19.03943276465977164, 0.05219959533909376836, 111.2489096053143669 ) ) ;
#11183=CARTESIAN_POINT ( 'NONE',  ( -19.02544592524334988, -5.153800228976617603, 43.95942372801899012 ) ) ;
#11184=CARTESIAN_POINT ( 'NONE',  ( 16.52544592524335698, 4.483927247898782831, 51.45942372801901854 ) ) ;
#11185=CARTESIAN_POINT ( 'NONE',  ( 16.46253265017160672, -9.564922557960803928, 108.3322429386476955 ) ) ;
#11187=CARTESIAN_POINT ( 'NONE',  ( 13.89961937509977652, -13.97604488694527269, 83.12390960531436690 ) ) ;
#11188=CARTESIAN_POINT ( 'NONE',  ( -8.224510206698735004, -14.34966873604973081, 94.58442372801901854 ) ) ;
#11190=CARTESIAN_POINT ( 'NONE',  ( 16.53943276465976808, -0.05219959533910856209, 88.74890960531436690 ) ) ;
#11191=CARTESIAN_POINT ( 'NONE',  ( 21.52544592524344225, -5.823673210054117533, 33.54057627198102409 ) ) ;
#11192=CARTESIAN_POINT ( 'NONE',  ( -19.02544592524342804, 5.153800228976336051, 36.04057627198100988 ) ) ;
#11193=CARTESIAN_POINT ( 'NONE',  ( 12.14591786802327356, -12.06949235617739191, 80.62609039468567573 ) ) ;
#11194=CARTESIAN_POINT ( 'NONE',  ( 21.53943276465977519, -0.05219959533907433946, 113.7489096053143527 ) ) ;
#11195=CARTESIAN_POINT ( 'NONE',  ( 5.153800228976615827, -19.02544592524334988, 75.20942372801896170 ) ) ;
#11196=CARTESIAN_POINT ( 'NONE',  ( 19.03943276465977164, -0.05219959533909143690, 43.74890960531435979 ) ) ;
#11197=CARTESIAN_POINT ( 'NONE',  ( 19.05341960407611168, 5.049401038298154454, 113.9572429386477097 ) ) ;
#11198=CARTESIAN_POINT ( 'NONE',  ( -10.81492255796105439, 18.62759615963255655, 107.9177570613523471 ) ) ;
#11199=CARTESIAN_POINT ( 'NONE',  ( -16.51473224551069308, -9.474510206698971260, 66.66557627198102409 ) ) ;
#11200=CARTESIAN_POINT ( 'NONE',  ( -4.483927247898782831, 16.52544592524335698, 42.70942372801901854 ) ) ;
#11201=CARTESIAN_POINT ( 'NONE',  ( -0.05219959533937732626, 21.53943276465977519, 87.50109039468568994 ) ) ;
#11202=CARTESIAN_POINT ( 'NONE',  ( 13.89961937509957401, 13.97604488694547697, 51.87609039468566863 ) ) ;
#11204=CARTESIAN_POINT ( 'NONE',  ( 16.46253265017146816, 9.564922557961045513, 51.66775706135233293 ) ) ;
#11206=CARTESIAN_POINT ( 'NONE',  ( 10.72451020669871369, 18.67979575497193778, 47.08442372801901854 ) ) ;
#11207=CARTESIAN_POINT ( 'NONE',  ( -16.51473224551069308, -9.474510206698971260, 56.66557627198103120 ) ) ;
#11208=CARTESIAN_POINT ( 'NONE',  ( -0.05219959533936034679, 19.03943276465977164, 42.50109039468566152 ) ) ;
#11209=CARTESIAN_POINT ( 'NONE',  ( 0.05219959533909260263, 19.03943276465977164, 104.9989096053143669 ) ) ;
#11210=CARTESIAN_POINT ( 'NONE',  ( -16.51473224551069308, -9.474510206698971260, 81.66557627198103830 ) ) ;
#11211=CARTESIAN_POINT ( 'NONE',  ( 4.483927247898545687, 16.52544592524342804, 34.79057627198103120 ) ) ;
#11212=CARTESIAN_POINT ( 'NONE',  ( -5.719274019375978568, 21.55341960407610458, 35.20724293864768839 ) ) ;
#11215=CARTESIAN_POINT ( 'NONE',  ( -19.02544592524334988, -5.153800228976617603, 18.95942372801899722 ) ) ;
#11217=CARTESIAN_POINT ( 'NONE',  ( -19.03943276465977164, 0.05219959533909376836, 31.24890960531435979 ) ) ;
#11218=CARTESIAN_POINT ( 'NONE',  ( -9.564922557960796823, -16.46253265017161027, 27.08224293864769550 ) ) ;
#11222=CARTESIAN_POINT ( 'NONE',  ( 16.53943276465976808, 0.05219959533934440121, 66.25109039468567573 ) ) ;
#11223=CARTESIAN_POINT ( 'NONE',  ( -5.719274019375978568, 21.55341960407610458, 80.20724293864769550 ) ) ;
#11225=CARTESIAN_POINT ( 'NONE',  ( 8.314922557960818139, 14.29746914071049879, 54.58224293864769550 ) ) ;
#11226=CARTESIAN_POINT ( 'NONE',  ( 5.153800228976335163, 19.02544592524342804, 34.79057627198102409 ) ) ;
#11227=CARTESIAN_POINT ( 'NONE',  ( -19.05341960407611168, -5.049401038298163336, 101.4572429386476955 ) ) ;
#11228=CARTESIAN_POINT ( 'NONE',  ( -18.67979575497193778, 10.72451020669871902, 33.33442372801900433 ) ) ;
#11229=CARTESIAN_POINT ( 'NONE',  ( 16.46253265017146816, 9.564922557961045513, 36.66775706135233293 ) ) ;
#11230=CARTESIAN_POINT ( 'NONE',  ( 5.153800228976335163, 19.02544592524342804, 39.79057627198100988 ) ) ;
#11231=CARTESIAN_POINT ( 'NONE',  ( -18.67979575497193778, 10.72451020669871902, 78.33442372801901854 ) ) ;
#11232=CARTESIAN_POINT ( 'NONE',  ( 17.31728774477274158, -6.344390552232386682, 33.31906651689320142 ) ) ;
#11233=CARTESIAN_POINT ( 'NONE',  ( -16.52544592524342804, 4.483927247898546575, 26.04057627198103475 ) ) ;
#11234=CARTESIAN_POINT ( 'NONE',  ( 17.50000000000000355, 3.471454075611732915, 113.0166741885564505 ) ) ;
#11235=CARTESIAN_POINT ( 'NONE',  ( -21.55341960407610458, -5.719274019375992779, 41.45724293864769550 ) ) ;
#11236=CARTESIAN_POINT ( 'NONE',  ( -4.483927247898539470, -16.52544592524342804, 102.2905762719810383 ) ) ;
#11238=CARTESIAN_POINT ( 'NONE',  ( -9.564922557960796823, -16.46253265017161027, 92.08224293864769550 ) ) ;
#11239=CARTESIAN_POINT ( 'NONE',  ( -0.05219959533910754901, -16.53943276465976808, 72.49890960531435269 ) ) ;
#11240=CARTESIAN_POINT ( 'NONE',  ( 19.02544592524334988, 5.153800228976608722, 106.4594237280190185 ) ) ;
#11241=CARTESIAN_POINT ( 'NONE',  ( 15.72974639402199770, -15.80617190586745480, 58.12390960531435979 ) ) ;
#11243=CARTESIAN_POINT ( 'NONE',  ( -19.03943276465977164, 0.05219959533909376836, 31.24890960531435979 ) ) ;
#11245=CARTESIAN_POINT ( 'NONE',  ( 9.564922557960805705, 16.46253265017160317, 84.58224293864769550 ) ) ;
#11246=CARTESIAN_POINT ( 'NONE',  ( -21.53943276465977519, 0.05219959533907696930, 91.24890960531436690 ) ) ;
#11247=CARTESIAN_POINT ( 'NONE',  ( 12.14591786802327356, -12.06949235617739191, 105.6260903946856899 ) ) ;
#11248=CARTESIAN_POINT ( 'NONE',  ( -16.46253265017160317, 9.564922557960807481, 90.83224293864769550 ) ) ;
#11249=CARTESIAN_POINT ( 'NONE',  ( -16.51473224551082808, 9.474510206698731452, 78.33442372801900433 ) ) ;
#11250=CARTESIAN_POINT ( 'NONE',  ( 5.823673210054444382, -21.52544592524334988, 95.20942372801903275 ) ) ;
#11251=CARTESIAN_POINT ( 'NONE',  ( -10.72451020669898014, 18.67979575497178502, 75.41557627198102409 ) ) ;
#11252=CARTESIAN_POINT ( 'NONE',  ( 18.67979575497178502, 10.72451020669898547, 39.16557627198102409 ) ) ;
#11254=CARTESIAN_POINT ( 'NONE',  ( -16.51473224551069308, -9.474510206698971260, 51.66557627198102409 ) ) ;
#11255=CARTESIAN_POINT ( 'NONE',  ( -8.314922557961024197, 14.29746914071037800, 112.9177570613523329 ) ) ;
#11256=CARTESIAN_POINT ( 'NONE',  ( -16.51473224551069308, -9.474510206698971260, 61.66557627198103120 ) ) ;
#11258=CARTESIAN_POINT ( 'NONE',  ( -9.564922557961040184, 16.46253265017147172, 27.91775706135232582 ) ) ;
#11259=CARTESIAN_POINT ( 'NONE',  ( 12.14591786802309770, 12.06949235617756955, 79.37390960531436690 ) ) ;
#11261=CARTESIAN_POINT ( 'NONE',  ( -21.52544592524343514, 5.823673210054127303, 106.0405762719810525 ) ) ;
#11263=CARTESIAN_POINT ( 'NONE',  ( 21.52544592524344225, -5.823673210054117533, 58.54057627198103120 ) ) ;
#11264=CARTESIAN_POINT ( 'NONE',  ( -16.52544592524335698, -4.483927247898792601, 98.95942372801903275 ) ) ;
#11265=CARTESIAN_POINT ( 'NONE',  ( -14.29746914071049879, 8.314922557960819915, 105.8322429386476955 ) ) ;
#11266=CARTESIAN_POINT ( 'NONE',  ( 16.51473224551069308, 9.474510206698969483, 59.16557627198102409 ) ) ;
#11267=CARTESIAN_POINT ( 'NONE',  ( -14.34966873604960291, -8.224510206698953496, 26.66557627198103475 ) ) ;
#11268=CARTESIAN_POINT ( 'NONE',  ( -10.72451020669870658, -18.67979575497194134, 49.58442372801901143 ) ) ;
#11269=CARTESIAN_POINT ( 'NONE',  ( -19.02544592524342804, 5.153800228976336051, 116.0405762719810383 ) ) ;
#11270=CARTESIAN_POINT ( 'NONE',  ( 18.62759615963255655, 10.81492255796105972, 86.66775706135234714 ) ) ;
#11271=CARTESIAN_POINT ( 'NONE',  ( 9.474510206698971260, -16.51473224551069308, 27.91557627198103120 ) ) ;
#11272=CARTESIAN_POINT ( 'NONE',  ( 19.05341960407611168, 5.049401038298154454, 43.95724293864769550 ) ) ;
#11273=ORIENTED_EDGE ( 'NONE', *, *, #120239, .F. ) ;
#11274=CARTESIAN_POINT ( 'NONE',  ( 10.81492255796106328, -18.62759615963255655, 100.4177570613523471 ) ) ;
#11275=CARTESIAN_POINT ( 'NONE',  ( 14.34966873604972726, -8.224510206698740333, 50.83442372801901143 ) ) ;
#11276=CARTESIAN_POINT ( 'NONE',  ( 15.72974639402176855, 15.80617190586768217, 71.87609039468568994 ) ) ;
#11277=CARTESIAN_POINT ( 'NONE',  ( -9.564922557960796823, -16.46253265017161027, 97.08224293864769550 ) ) ;
#11278=CARTESIAN_POINT ( 'NONE',  ( -5.153800228976607833, 19.02544592524334988, 77.70942372801900433 ) ) ;
#11279=CARTESIAN_POINT ( 'NONE',  ( -5.823673210054431948, 21.52544592524334988, 52.70942372801902565 ) ) ;
#11280=CARTESIAN_POINT ( 'NONE',  ( 16.52544592524335698, 4.483927247898782831, 21.45942372801901499 ) ) ;
#11281=CARTESIAN_POINT ( 'NONE',  ( 5.049401038297881783, 19.05341960407617563, 92.29275706135234714 ) ) ;
#11282=CARTESIAN_POINT ( 'NONE',  ( -13.97604488694527625, -13.89961937509977652, 56.87390960531434558 ) ) ;
#11283=CARTESIAN_POINT ( 'NONE',  ( 19.02544592524334988, 5.153800228976608722, 86.45942372801900433 ) ) ;
#11285=CARTESIAN_POINT ( 'NONE',  ( 16.55341960407611168, 4.379528057220329451, 23.95724293864769550 ) ) ;
#11286=CARTESIAN_POINT ( 'NONE',  ( 5.049401038297881783, 19.05341960407617563, 92.29275706135234714 ) ) ;
#11287=CARTESIAN_POINT ( 'NONE',  ( 12.06949235617757843, -12.14591786802309237, 43.12390960531435269 ) ) ;
#11288=CARTESIAN_POINT ( 'NONE',  ( -19.03943276465977164, -0.05219959533935918106, 68.75109039468566152 ) ) ;
#11289=CARTESIAN_POINT ( 'NONE',  ( -12.14591786802326823, 12.06949235617739902, 48.12609039468568284 ) ) ;
#11290=CARTESIAN_POINT ( 'NONE',  ( -13.97604488694547697, 13.89961937509957934, 28.12609039468565797 ) ) ;
#11292=CARTESIAN_POINT ( 'NONE',  ( -5.153800228976328057, -19.02544592524343514, 22.29057627198102765 ) ) ;
#11293=CARTESIAN_POINT ( 'NONE',  ( 16.51473224551069308, 9.474510206698969483, 44.16557627198103120 ) ) ;
#11294=CARTESIAN_POINT ( 'NONE',  ( 8.224510206698742110, 14.34966873604972548, 47.08442372801901854 ) ) ;
#11298=CARTESIAN_POINT ( 'NONE',  ( -19.05341960407611168, -5.049401038298163336, 86.45724293864769550 ) ) ;
#11299=CARTESIAN_POINT ( 'NONE',  ( 17.76566638676866461, -1.079584607091855997, 102.5000000000000284 ) ) ;
#11301=CARTESIAN_POINT ( 'NONE',  ( 19.02544592524334988, 5.153800228976608722, 96.45942372801897591 ) ) ;
#11302=EDGE_CURVE ( 'NONE', #192686, #15160, #43709, .T. ) ;
#11303=CARTESIAN_POINT ( 'NONE',  ( 5.823673210054125526, 21.52544592524343514, 24.79057627198103120 ) ) ;
#11304=CARTESIAN_POINT ( 'NONE',  ( -5.153800228976607833, 19.02544592524334988, 27.70942372801899722 ) ) ;
#11305=CARTESIAN_POINT ( 'NONE',  ( -13.97604488694547697, 13.89961937509957934, 113.1260903946856757 ) ) ;
#11306=CARTESIAN_POINT ( 'NONE',  ( -0.05219959533909027116, -19.03943276465977164, 22.49890960531436690 ) ) ;
#11307=CARTESIAN_POINT ( 'NONE',  ( 19.05341960407611168, 5.049401038298154454, 33.95724293864769550 ) ) ;
#11308=CARTESIAN_POINT ( 'NONE',  ( 21.55341960407610458, 5.719274019375980345, 73.95724293864769550 ) ) ;
#11309=CARTESIAN_POINT ( 'NONE',  ( -9.474510206698964154, 16.51473224551069663, 40.41557627198103120 ) ) ;
#11310=CARTESIAN_POINT ( 'NONE',  ( -18.22780087662114212, 5.499999999999995559, 48.51540105326107266 ) ) ;
#11311=CARTESIAN_POINT ( 'NONE',  ( -13.89961937509957401, -13.97604488694547875, 74.37609039468566152 ) ) ;
#11312=CARTESIAN_POINT ( 'NONE',  ( 8.224510206698953496, -14.34966873604960469, 52.91557627198103830 ) ) ;
#11313=CARTESIAN_POINT ( 'NONE',  ( -5.719274019375978568, 21.55341960407610458, 35.20724293864768839 ) ) ;
#11314=CARTESIAN_POINT ( 'NONE',  ( -15.80617190586768217, 15.72974639402176855, 93.12609039468568994 ) ) ;
#11315=CARTESIAN_POINT ( 'NONE',  ( -5.719274019375978568, 21.55341960407610458, 85.20724293864770971 ) ) ;
#11316=CARTESIAN_POINT ( 'NONE',  ( -21.53943276465977519, -0.05219959533937600094, 68.75109039468568994 ) ) ;
#11317=CARTESIAN_POINT ( 'NONE',  ( -21.55341960407619339, 5.719274019375674811, 63.54275706135234003 ) ) ;
#11318=CARTESIAN_POINT ( 'NONE',  ( 5.153800228976335163, 19.02544592524342804, 94.79057627198103830 ) ) ;
#11319=CARTESIAN_POINT ( 'NONE',  ( -14.29746914071037622, -8.314922557961029526, 94.16775706135237556 ) ) ;
#11320=CARTESIAN_POINT ( 'NONE',  ( 21.55341960407619695, -5.719274019375665929, 66.04275706135236135 ) ) ;
#11321=CARTESIAN_POINT ( 'NONE',  ( -16.46253265017160317, 9.564922557960807481, 50.83224293864770260 ) ) ;
#11322=CARTESIAN_POINT ( 'NONE',  ( -5.719274019375665041, -21.55341960407619695, 29.79275706135234358 ) ) ;
#11323=CARTESIAN_POINT ( 'NONE',  ( -16.51473224551069308, -9.474510206698971260, 71.66557627198102409 ) ) ;
#11324=CARTESIAN_POINT ( 'NONE',  ( -4.379528057220328563, 16.55341960407611168, 65.20724293864768129 ) ) ;
#11325=CARTESIAN_POINT ( 'NONE',  ( 12.14591786802309770, 12.06949235617756955, 44.37390960531435979 ) ) ;
#11326=CARTESIAN_POINT ( 'NONE',  ( 0.05219959533907565091, 21.53943276465977519, 39.99890960531436690 ) ) ;
#11327=CARTESIAN_POINT ( 'NONE',  ( 19.02544592524343514, -5.153800228976328945, 48.54057627198103120 ) ) ;
#11328=CARTESIAN_POINT ( 'NONE',  ( 18.67979575497178502, 10.72451020669898547, 59.16557627198103120 ) ) ;
#11329=CARTESIAN_POINT ( 'NONE',  ( -0.05219959533936034679, 19.03943276465977164, 52.50109039468566863 ) ) ;
#11330=CARTESIAN_POINT ( 'NONE',  ( -9.474510206698720793, -16.51473224551083518, 19.58442372801899722 ) ) ;
#11331=CARTESIAN_POINT ( 'NONE',  ( -4.483927247898539470, -16.52544592524342804, 57.29057627198103120 ) ) ;
#11332=CARTESIAN_POINT ( 'NONE',  ( 21.53943276465977519, -0.05219959533907433946, 33.74890960531436690 ) ) ;
#11333=ORIENTED_EDGE ( 'NONE', *, *, #58394, .F. ) ;
#11334=CARTESIAN_POINT ( 'NONE',  ( 15.50000000000000178, -5.500000000000000888, 22.00000000000000000 ) ) ;
#11335=CARTESIAN_POINT ( 'NONE',  ( 8.314922557961029526, -14.29746914071037800, 80.41775706135234714 ) ) ;
#11336=CARTESIAN_POINT ( 'NONE',  ( -16.46253265017146816, -9.564922557961047289, 89.16775706135234714 ) ) ;
#11337=CARTESIAN_POINT ( 'NONE',  ( 12.06949235617757843, -12.14591786802309237, 53.12390960531436690 ) ) ;
#11339=CARTESIAN_POINT ( 'NONE',  ( 19.02544592524343514, -5.153800228976328945, 43.54057627198103120 ) ) ;
#11340=CARTESIAN_POINT ( 'NONE',  ( -8.224510206698948167, 14.34966873604960824, 40.41557627198103120 ) ) ;
#11341=CARTESIAN_POINT ( 'NONE',  ( -13.89961937509977652, 13.97604488694528158, 55.62390960531434558 ) ) ;
#11342=CARTESIAN_POINT ( 'NONE',  ( -19.03943276465977164, 0.05219959533909376836, 71.24890960531435269 ) ) ;
#11343=CARTESIAN_POINT ( 'NONE',  ( 16.51473224551069308, 9.474510206698969483, 54.16557627198103120 ) ) ;
#11344=CARTESIAN_POINT ( 'NONE',  ( 18.67979575497194134, -10.72451020669871369, 50.83442372801901143 ) ) ;
#11345=CARTESIAN_POINT ( 'NONE',  ( 9.564922557960805705, 16.46253265017160317, 69.58224293864770971 ) ) ;
#11346=CARTESIAN_POINT ( 'NONE',  ( 9.474510206698971260, -16.51473224551069308, 27.91557627198103120 ) ) ;
#11347=CARTESIAN_POINT ( 'NONE',  ( 0.05219959533909260263, 19.03943276465977164, 54.99890960531435979 ) ) ;
#11348=CARTESIAN_POINT ( 'NONE',  ( -10.81492255796078084, -18.62759615963271287, 52.08224293864768839 ) ) ;
#11349=CARTESIAN_POINT ( 'NONE',  ( 9.564922557960805705, 16.46253265017160317, 34.58224293864770260 ) ) ;
#11350=CARTESIAN_POINT ( 'NONE',  ( 10.72451020669898902, -18.67979575497178502, 37.91557627198102409 ) ) ;
#11351=CARTESIAN_POINT ( 'NONE',  ( -4.379528057220086978, -16.55341960407618274, 99.79275706135234714 ) ) ;
#11352=CARTESIAN_POINT ( 'NONE',  ( 0.05219959533936267826, -19.03943276465977164, 30.00109039468566863 ) ) ;
#11353=CARTESIAN_POINT ( 'NONE',  ( 4.483927247898790824, -16.52544592524335698, 40.20942372801901854 ) ) ;
#11354=CARTESIAN_POINT ( 'NONE',  ( 0.05219959533934541429, -16.53943276465976808, 75.00109039468568994 ) ) ;
#11356=CARTESIAN_POINT ( 'NONE',  ( -14.34966873604972548, 8.224510206698743886, 73.33442372801901854 ) ) ;
#11357=CARTESIAN_POINT ( 'NONE',  ( -12.14591786802326823, 12.06949235617739902, 53.12609039468568284 ) ) ;
#11358=CARTESIAN_POINT ( 'NONE',  ( -19.03943276465977164, 0.05219959533909376836, 106.2489096053143669 ) ) ;
#11360=CARTESIAN_POINT ( 'NONE',  ( 14.29746914071037800, 8.314922557961029526, 36.66775706135234714 ) ) ;
#11361=CARTESIAN_POINT ( 'NONE',  ( 19.05341960407611168, 5.049401038298154454, 33.95724293864769550 ) ) ;
#11362=CARTESIAN_POINT ( 'NONE',  ( 21.52544592524334988, 5.823673210054432836, 26.45942372801901854 ) ) ;
#11363=CARTESIAN_POINT ( 'NONE',  ( -12.06949235617739369, -12.14591786802326823, 34.37609039468568284 ) ) ;
#11364=CARTESIAN_POINT ( 'NONE',  ( 4.379528057220092307, 16.55341960407617563, 102.2927570613523613 ) ) ;
#11366=CARTESIAN_POINT ( 'NONE',  ( 5.719274019375673035, 21.55341960407619339, 102.2927570613523613 ) ) ;
#11367=CARTESIAN_POINT ( 'NONE',  ( 5.153800228976615827, -19.02544592524334988, 95.20942372801897591 ) ) ;
#11368=CARTESIAN_POINT ( 'NONE',  ( -12.06949235617756955, 12.14591786802309770, 50.62390960531435979 ) ) ;
#11369=CARTESIAN_POINT ( 'NONE',  ( -9.474510206698964154, 16.51473224551069663, 25.41557627198103120 ) ) ;
#11370=CARTESIAN_POINT ( 'NONE',  ( -19.03943276465977164, -0.05219959533935918106, 63.75109039468566863 ) ) ;
#11372=CARTESIAN_POINT ( 'NONE',  ( -5.719274019375665041, -21.55341960407619695, 64.79275706135234714 ) ) ;
#11373=CARTESIAN_POINT ( 'NONE',  ( 4.483927247898790824, -16.52544592524335698, 30.20942372801902565 ) ) ;
#11375=CARTESIAN_POINT ( 'NONE',  ( -18.62759615963270932, 10.81492255796079327, 25.83224293864769194 ) ) ;
#11376=CARTESIAN_POINT ( 'NONE',  ( -13.97604488694547697, 13.89961937509957934, 108.1260903946856331 ) ) ;
#11377=FACE_OUTER_BOUND ( 'NONE', #154733, .T. ) ;
#11379=CARTESIAN_POINT ( 'NONE',  ( 19.03943276465977164, -0.05219959533909143690, 28.74890960531435624 ) ) ;
#11380=CARTESIAN_POINT ( 'NONE',  ( -5.719274019375665041, -21.55341960407619695, 109.7927570613523613 ) ) ;
#11381=CARTESIAN_POINT ( 'NONE',  ( -13.89961937509977652, 13.97604488694528158, 45.62390960531433848 ) ) ;
#11383=CARTESIAN_POINT ( 'NONE',  ( 18.67979575497194134, -10.72451020669871369, 45.83442372801901854 ) ) ;
#11384=CARTESIAN_POINT ( 'NONE',  ( -21.52544592524334988, -5.823673210054445271, 103.9594237280190185 ) ) ;
#11385=CARTESIAN_POINT ( 'NONE',  ( -8.314922557961024197, 14.29746914071037800, 107.9177570613523471 ) ) ;
#11386=CARTESIAN_POINT ( 'NONE',  ( 16.46253265017160672, -9.564922557960803928, 78.33224293864769550 ) ) ;
#11387=CARTESIAN_POINT ( 'NONE',  ( -15.72974639402176322, -15.80617190586768395, 44.37609039468567573 ) ) ;
#11388=CARTESIAN_POINT ( 'NONE',  ( 21.52544592524334988, 5.823673210054432836, 56.45942372801902565 ) ) ;
#11389=CARTESIAN_POINT ( 'NONE',  ( -19.03943276465977164, -0.05219959533935918106, 73.75109039468566152 ) ) ;
#11390=CARTESIAN_POINT ( 'NONE',  ( -19.02544592524342804, 5.153800228976336051, 91.04057627198100988 ) ) ;
#11391=CARTESIAN_POINT ( 'NONE',  ( 4.483927247898545687, 16.52544592524342804, 109.7905762719810383 ) ) ;
#11392=CARTESIAN_POINT ( 'NONE',  ( 15.72974639402199770, -15.80617190586745480, 98.12390960531436690 ) ) ;
#11393=CARTESIAN_POINT ( 'NONE',  ( 19.02544592524334988, 5.153800228976608722, 21.45942372801899012 ) ) ;
#11394=CARTESIAN_POINT ( 'NONE',  ( 14.29746914071049879, -8.314922557960816363, 103.3322429386476955 ) ) ;
#11395=CARTESIAN_POINT ( 'NONE',  ( -19.03943276465977164, 0.05219959533909376836, 51.24890960531436690 ) ) ;
#11396=CARTESIAN_POINT ( 'NONE',  ( -9.474510206698720793, -16.51473224551083518, 89.58442372801900433 ) ) ;
#11397=VECTOR ( 'NONE', #120005, 1000.000000000000000 ) ;
#11398=CARTESIAN_POINT ( 'NONE',  ( 16.55341960407611168, 4.379528057220329451, 43.95724293864769550 ) ) ;
#11399=CARTESIAN_POINT ( 'NONE',  ( 5.719274019375673035, 21.55341960407619339, 102.2927570613523613 ) ) ;
#11400=CARTESIAN_POINT ( 'NONE',  ( -13.89961937509977652, 13.97604488694528158, 110.6239096053143243 ) ) ;
#11401=CARTESIAN_POINT ( 'NONE',  ( -19.05341960407617563, 5.049401038297882671, 78.54275706135233293 ) ) ;
#11402=CARTESIAN_POINT ( 'NONE',  ( -5.823673210054116645, -21.52544592524344225, 72.29057627198102409 ) ) ;
#11403=CARTESIAN_POINT ( 'NONE',  ( -18.67979575497193778, 10.72451020669871902, 28.33442372801902209 ) ) ;
#11404=CARTESIAN_POINT ( 'NONE',  ( -8.224510206698735004, -14.34966873604973081, 34.58442372801900433 ) ) ;
#11405=CARTESIAN_POINT ( 'NONE',  ( 14.34966873604972726, -8.224510206698740333, 90.83442372801901854 ) ) ;
#11406=CARTESIAN_POINT ( 'NONE',  ( 9.564922557960805705, 16.46253265017160317, 29.58224293864769550 ) ) ;
#11407=CARTESIAN_POINT ( 'NONE',  ( 5.719274019375673035, 21.55341960407619339, 32.29275706135235424 ) ) ;
#11408=CARTESIAN_POINT ( 'NONE',  ( -21.52544592524343514, 5.823673210054127303, 46.04057627198103830 ) ) ;
#11409=CARTESIAN_POINT ( 'NONE',  ( -14.34966873604960291, -8.224510206698953496, 111.6655762719810525 ) ) ;
#11411=CARTESIAN_POINT ( 'NONE',  ( -16.55341960407617563, 4.379528057220093196, 68.54275706135234714 ) ) ;
#11412=CARTESIAN_POINT ( 'NONE',  ( -4.483927247898539470, -16.52544592524342804, 92.29057627198103830 ) ) ;
#11413=CARTESIAN_POINT ( 'NONE',  ( -5.823673210054116645, -21.52544592524344225, 82.29057627198103830 ) ) ;
#11414=CARTESIAN_POINT ( 'NONE',  ( -8.314922557960811034, -14.29746914071050412, 32.08224293864769550 ) ) ;
#11415=CARTESIAN_POINT ( 'NONE',  ( 4.483927247898790824, -16.52544592524335698, 45.20942372801901854 ) ) ;
#11416=CARTESIAN_POINT ( 'NONE',  ( 19.02544592524343514, -5.153800228976328945, 58.54057627198102409 ) ) ;
#11417=CARTESIAN_POINT ( 'NONE',  ( 4.379528057220092307, 16.55341960407617563, 87.29275706135236135 ) ) ;
#11418=CARTESIAN_POINT ( 'NONE',  ( -13.97604488694547697, 13.89961937509957934, 93.12609039468566152 ) ) ;
#11419=CARTESIAN_POINT ( 'NONE',  ( 0.05219959533907565091, 21.53943276465977519, 89.99890960531438111 ) ) ;
#11420=CARTESIAN_POINT ( 'NONE',  ( -16.52544592524335698, -4.483927247898792601, 108.9594237280190185 ) ) ;
#11422=CARTESIAN_POINT ( 'NONE',  ( 13.97604488694527802, 13.89961937509977652, 114.3739096053143669 ) ) ;
#11423=CARTESIAN_POINT ( 'NONE',  ( -21.52544592524343514, 5.823673210054127303, 66.04057627198103830 ) ) ;
#11424=CARTESIAN_POINT ( 'NONE',  ( 0.05219959533934541429, -16.53943276465976808, 90.00109039468567573 ) ) ;
#11426=CARTESIAN_POINT ( 'NONE',  ( -18.62759615963270932, 10.81492255796079327, 35.83224293864768839 ) ) ;
#11427=CARTESIAN_POINT ( 'NONE',  ( -19.52217212775661181, 5.499999999999918288, 74.93993709005260939 ) ) ;
#11428=CARTESIAN_POINT ( 'NONE',  ( -21.55341960407610458, -5.719274019375992779, 86.45724293864770971 ) ) ;
#11429=CARTESIAN_POINT ( 'NONE',  ( 14.34966873604960469, 8.224510206698951720, 29.16557627198103120 ) ) ;
#11431=CARTESIAN_POINT ( 'NONE',  ( -4.379528057220086978, -16.55341960407618274, 34.79275706135235424 ) ) ;
#11432=CARTESIAN_POINT ( 'NONE',  ( 13.89961937509977652, -13.97604488694527269, 28.12390960531435624 ) ) ;
#11433=CARTESIAN_POINT ( 'NONE',  ( 8.314922557961029526, -14.29746914071037800, 25.41775706135235779 ) ) ;
#11434=CARTESIAN_POINT ( 'NONE',  ( 19.05341960407611168, 5.049401038298154454, 53.95724293864770260 ) ) ;
#11436=CARTESIAN_POINT ( 'NONE',  ( -19.03943276465977164, 0.05219959533909376836, 106.2489096053143669 ) ) ;
#11438=CARTESIAN_POINT ( 'NONE',  ( -4.483927247898782831, 16.52544592524335698, 102.7094237280190185 ) ) ;
#11439=CARTESIAN_POINT ( 'NONE',  ( 13.97604488694548053, -13.89961937509957401, 90.62609039468567573 ) ) ;
#11440=CARTESIAN_POINT ( 'NONE',  ( 9.474510206698729675, 16.51473224551082808, 37.08442372801899722 ) ) ;
#11441=CARTESIAN_POINT ( 'NONE',  ( -15.80617190586745835, -15.72974639402198527, 81.87390960531435269 ) ) ;
#11442=CARTESIAN_POINT ( 'NONE',  ( -16.53943276465976808, -0.05219959533934237506, 103.7510903946857042 ) ) ;
#11443=CARTESIAN_POINT ( 'NONE',  ( 18.67979575497178502, 10.72451020669898547, 29.16557627198103120 ) ) ;
#11444=CARTESIAN_POINT ( 'NONE',  ( 19.02544592524334988, 5.153800228976608722, 96.45942372801897591 ) ) ;
#11445=CARTESIAN_POINT ( 'NONE',  ( 19.03943276465977164, -0.05219959533909143690, 53.74890960531436690 ) ) ;
#11446=CARTESIAN_POINT ( 'NONE',  ( -0.05219959533909027116, -19.03943276465977164, 102.4989096053143669 ) ) ;
#11447=CARTESIAN_POINT ( 'NONE',  ( -21.53943276465977519, -0.05219959533937600094, 63.75109039468568284 ) ) ;
#11448=CARTESIAN_POINT ( 'NONE',  ( 13.97604488694527802, 13.89961937509977652, 64.37390960531436690 ) ) ;
#11449=CARTESIAN_POINT ( 'NONE',  ( 14.34966873604960469, 8.224510206698951720, 94.16557627198103830 ) ) ;
#11451=CARTESIAN_POINT ( 'NONE',  ( -16.55341960407611168, -4.379528057220339221, 71.45724293864769550 ) ) ;
#11452=CARTESIAN_POINT ( 'NONE',  ( 18.67979575497178502, 10.72451020669898547, 69.16557627198102409 ) ) ;
#11454=CARTESIAN_POINT ( 'NONE',  ( -16.46253265017146816, -9.564922557961047289, 89.16775706135234714 ) ) ;
#11456=CARTESIAN_POINT ( 'NONE',  ( 19.02544592524343514, -5.153800228976328945, 58.54057627198102409 ) ) ;
#11457=CARTESIAN_POINT ( 'NONE',  ( 17.50000000000000000, -5.499999999999992895, 71.21769037696435589 ) ) ;
#11458=CARTESIAN_POINT ( 'NONE',  ( 5.049401038298161559, -19.05341960407611168, 72.70724293864768129 ) ) ;
#11459=CARTESIAN_POINT ( 'NONE',  ( -0.05219959533909027116, -19.03943276465977164, 87.49890960531436690 ) ) ;
#11460=EDGE_CURVE ( 'NONE', #121091, #179892, #256, .T. ) ;
#11461=CARTESIAN_POINT ( 'NONE',  ( -8.314922557961024197, 14.29746914071037800, 67.91775706135234714 ) ) ;
#11462=CARTESIAN_POINT ( 'NONE',  ( -17.48847506799968343, -5.747544572773812810, 49.17302562156721280 ) ) ;
#11463=CARTESIAN_POINT ( 'NONE',  ( 9.474510206698729675, 16.51473224551082808, 42.08442372801900433 ) ) ;
#11464=CARTESIAN_POINT ( 'NONE',  ( 17.37248965764951336, 6.147170618106522433, 21.68035186998432451 ) ) ;
#11465=CARTESIAN_POINT ( 'NONE',  ( -13.89961937509977652, 13.97604488694528158, 105.6239096053143527 ) ) ;
#11466=CARTESIAN_POINT ( 'NONE',  ( -16.53943276465976808, -0.05219959533934237506, 98.75109039468568994 ) ) ;
#11468=CARTESIAN_POINT ( 'NONE',  ( -8.224510206698735004, -14.34966873604973081, 99.58442372801900433 ) ) ;
#11469=CARTESIAN_POINT ( 'NONE',  ( -17.48853670773243607, 5.747243402303161552, 28.66671299749991775 ) ) ;
#11470=CARTESIAN_POINT ( 'NONE',  ( -12.06949235617739369, -12.14591786802326823, 74.37609039468568994 ) ) ;
#11472=CARTESIAN_POINT ( 'NONE',  ( -21.52544592524334988, -5.823673210054445271, 73.95942372801901854 ) ) ;
#11473=CARTESIAN_POINT ( 'NONE',  ( 5.049401038297881783, 19.05341960407617563, 77.29275706135231871 ) ) ;
#11474=CARTESIAN_POINT ( 'NONE',  ( 16.51473224551083163, -9.474510206698727899, 25.83442372801900078 ) ) ;
#11475=CARTESIAN_POINT ( 'NONE',  ( 9.564922557960805705, 16.46253265017160317, 64.58224293864769550 ) ) ;
#11476=CARTESIAN_POINT ( 'NONE',  ( 19.03943276465977164, -0.05219959533909143690, 43.74890960531435979 ) ) ;
#11478=CARTESIAN_POINT ( 'NONE',  ( 15.72974639402199770, -15.80617190586745480, 83.12390960531436690 ) ) ;
#11479=CARTESIAN_POINT ( 'NONE',  ( 10.72451020669898902, -18.67979575497178502, 37.91557627198102409 ) ) ;
#11480=CARTESIAN_POINT ( 'NONE',  ( -19.02544592524342804, 5.153800228976336051, 31.04057627198102409 ) ) ;
#11481=CARTESIAN_POINT ( 'NONE',  ( -12.14591786802326823, 12.06949235617739902, 53.12609039468568284 ) ) ;
#11484=CARTESIAN_POINT ( 'NONE',  ( -21.52544592524334988, -5.823673210054445271, 33.95942372801901143 ) ) ;
#11485=CARTESIAN_POINT ( 'NONE',  ( -16.52544592524342804, 4.483927247898546575, 51.04057627198103120 ) ) ;
#11487=CARTESIAN_POINT ( 'NONE',  ( 16.52544592524335698, 4.483927247898782831, 26.45942372801901854 ) ) ;
#11488=CARTESIAN_POINT ( 'NONE',  ( -16.46253265017146816, -9.564922557961047289, 39.16775706135234003 ) ) ;
#11489=CARTESIAN_POINT ( 'NONE',  ( -0.05219959533910754901, -16.53943276465976808, 62.49890960531436690 ) ) ;
#11490=CARTESIAN_POINT ( 'NONE',  ( -21.52544592524343514, 5.823673210054127303, 111.0405762719810525 ) ) ;
#11492=CARTESIAN_POINT ( 'NONE',  ( 15.80617190586746368, 15.72974639402197994, 79.37390960531436690 ) ) ;
#11493=CARTESIAN_POINT ( 'NONE',  ( -16.51473224551069308, -9.474510206698971260, 91.66557627198103830 ) ) ;
#11494=CARTESIAN_POINT ( 'NONE',  ( -4.483927247898539470, -16.52544592524342804, 67.29057627198103830 ) ) ;
#11495=CARTESIAN_POINT ( 'NONE',  ( -16.51473224551069308, -9.474510206698971260, 101.6655762719810241 ) ) ;
#11497=CARTESIAN_POINT ( 'NONE',  ( -9.564922557961040184, 16.46253265017147172, 67.91775706135233293 ) ) ;
#11498=CARTESIAN_POINT ( 'NONE',  ( 5.719274019375991003, -21.55341960407610458, 102.7072429386476955 ) ) ;
#11499=CARTESIAN_POINT ( 'NONE',  ( -9.474510206698964154, 16.51473224551069663, 60.41557627198102409 ) ) ;
#11500=CARTESIAN_POINT ( 'NONE',  ( 19.05341960407617918, -5.049401038297876454, 46.04275706135233293 ) ) ;
#11501=CARTESIAN_POINT ( 'NONE',  ( -12.06949235617756955, 12.14591786802309770, 115.6239096053143669 ) ) ;
#11502=CARTESIAN_POINT ( 'NONE',  ( -5.823673210054431948, 21.52544592524334988, 62.70942372801902565 ) ) ;
#11503=CARTESIAN_POINT ( 'NONE',  ( -16.88567814943164436, -6.947325034625695395, 71.29001122652586275 ) ) ;
#11504=CARTESIAN_POINT ( 'NONE',  ( 4.483927247898545687, 16.52544592524342804, 39.79057627198103830 ) ) ;
#11505=CARTESIAN_POINT ( 'NONE',  ( 13.97604488694527802, 13.89961937509977652, 54.37390960531435979 ) ) ;
#11506=CARTESIAN_POINT ( 'NONE',  ( -9.474510206698964154, 16.51473224551069663, 115.4155762719810241 ) ) ;
#11507=CARTESIAN_POINT ( 'NONE',  ( 18.67979575497178502, 10.72451020669898547, 74.16557627198102409 ) ) ;
#11509=CARTESIAN_POINT ( 'NONE',  ( -16.46253265017160317, 9.564922557960807481, 40.83224293864769550 ) ) ;
#11511=CARTESIAN_POINT ( 'NONE',  ( -10.72451020669898014, 18.67979575497178502, 60.41557627198102409 ) ) ;
#11513=CARTESIAN_POINT ( 'NONE',  ( 21.55341960407619695, -5.719274019375665929, 81.04275706135236135 ) ) ;
#11515=CARTESIAN_POINT ( 'NONE',  ( 8.314922557961029526, -14.29746914071037800, 100.4177570613523471 ) ) ;
#11516=CARTESIAN_POINT ( 'NONE',  ( -8.314922557960811034, -14.29746914071050412, 77.08224293864769550 ) ) ;
#11517=CARTESIAN_POINT ( 'NONE',  ( 16.51473224551069308, 9.474510206698969483, 74.16557627198103830 ) ) ;
#11519=CARTESIAN_POINT ( 'NONE',  ( -19.02544592524334988, -5.153800228976617603, 43.95942372801899012 ) ) ;
#11520=CARTESIAN_POINT ( 'NONE',  ( -8.314922557961024197, 14.29746914071037800, 92.91775706135236135 ) ) ;
#11521=CARTESIAN_POINT ( 'NONE',  ( -0.05219959533936034679, 19.03943276465977164, 22.50109039468566152 ) ) ;
#11522=CARTESIAN_POINT ( 'NONE',  ( 16.51473224551069308, 9.474510206698969483, 84.16557627198102409 ) ) ;
#11523=CARTESIAN_POINT ( 'NONE',  ( 21.55341960407610458, 5.719274019375980345, 43.95724293864769550 ) ) ;
#11525=CARTESIAN_POINT ( 'NONE',  ( 21.52544592524334988, 5.823673210054432836, 101.4594237280190185 ) ) ;
#11526=CARTESIAN_POINT ( 'NONE',  ( -16.55341960407617563, 4.379528057220093196, 58.54275706135235424 ) ) ;
#11527=CARTESIAN_POINT ( 'NONE',  ( 10.81492255796078972, 18.62759615963270932, 109.5822429386476955 ) ) ;
#11528=CARTESIAN_POINT ( 'NONE',  ( 16.52544592524335698, 4.483927247898782831, 31.45942372801901854 ) ) ;
#11529=CARTESIAN_POINT ( 'NONE',  ( 9.564922557960805705, 16.46253265017160317, 89.58224293864769550 ) ) ;
#11530=CARTESIAN_POINT ( 'NONE',  ( 5.049401038298161559, -19.05341960407611168, 42.70724293864767418 ) ) ;
#11531=CARTESIAN_POINT ( 'NONE',  ( 19.05341960407611168, 5.049401038298154454, 48.95724293864768129 ) ) ;
#11533=CARTESIAN_POINT ( 'NONE',  ( -16.53943276465976808, -0.05219959533934237506, 28.75109039468567929 ) ) ;
#11534=CARTESIAN_POINT ( 'NONE',  ( 16.55341960407611168, 4.379528057220329451, 73.95724293864769550 ) ) ;
#11535=CARTESIAN_POINT ( 'NONE',  ( -16.55341960407617563, 4.379528057220093196, 88.54275706135236135 ) ) ;
#11537=CARTESIAN_POINT ( 'NONE',  ( 5.719274019375673035, 21.55341960407619339, 42.29275706135235424 ) ) ;
#11538=CARTESIAN_POINT ( 'NONE',  ( -0.05219959533909027116, -19.03943276465977164, 67.49890960531436690 ) ) ;
#11539=CARTESIAN_POINT ( 'NONE',  ( 19.02544592524343514, -5.153800228976328945, 48.54057627198103120 ) ) ;
#11540=CARTESIAN_POINT ( 'NONE',  ( -19.05341960407611168, -5.049401038298163336, 76.45724293864769550 ) ) ;
#11541=CARTESIAN_POINT ( 'NONE',  ( -14.34966873604960291, -8.224510206698953496, 31.66557627198102054 ) ) ;
#11542=CARTESIAN_POINT ( 'NONE',  ( 8.224510206698742110, 14.34966873604972548, 82.08442372801901854 ) ) ;
#11544=CARTESIAN_POINT ( 'NONE',  ( 13.97604488694548053, -13.89961937509957401, 25.62609039468566507 ) ) ;
#11545=CARTESIAN_POINT ( 'NONE',  ( -9.564922557960796823, -16.46253265017161027, 97.08224293864769550 ) ) ;
#11546=CARTESIAN_POINT ( 'NONE',  ( -16.51473224551069308, -9.474510206698971260, 46.66557627198102409 ) ) ;
#11547=CARTESIAN_POINT ( 'NONE',  ( 0.05219959533936267826, -19.03943276465977164, 20.00109039468567218 ) ) ;
#11549=CARTESIAN_POINT ( 'NONE',  ( -4.379528057220086978, -16.55341960407618274, 44.79275706135234714 ) ) ;
#11551=CARTESIAN_POINT ( 'NONE',  ( 9.564922557961047289, -16.46253265017146816, 75.41775706135234714 ) ) ;
#11552=CARTESIAN_POINT ( 'NONE',  ( -12.06949235617739369, -12.14591786802326823, 49.37609039468569705 ) ) ;
#11553=CARTESIAN_POINT ( 'NONE',  ( -13.89961937509977652, 13.97604488694528158, 115.6239096053143669 ) ) ;
#11554=CARTESIAN_POINT ( 'NONE',  ( 5.049401038298161559, -19.05341960407611168, 72.70724293864768129 ) ) ;
#11555=CARTESIAN_POINT ( 'NONE',  ( 10.81492255796078972, 18.62759615963270932, 109.5822429386476955 ) ) ;
#11556=CARTESIAN_POINT ( 'NONE',  ( -0.05219959533936034679, 19.03943276465977164, 67.50109039468566152 ) ) ;
#11557=CARTESIAN_POINT ( 'NONE',  ( 0.05219959533909260263, 19.03943276465977164, 109.9989096053143669 ) ) ;
#11558=CARTESIAN_POINT ( 'NONE',  ( -16.46253265017160317, 9.564922557960807481, 40.83224293864769550 ) ) ;
#11559=CARTESIAN_POINT ( 'NONE',  ( -0.05219959533909027116, -19.03943276465977164, 82.49890960531436690 ) ) ;
#11560=CARTESIAN_POINT ( 'NONE',  ( -8.314922557960811034, -14.29746914071050412, 37.08224293864768129 ) ) ;
#11561=CARTESIAN_POINT ( 'NONE',  ( -18.22780087662123805, 5.499999999999981348, 71.01763182126894947 ) ) ;
#11562=CARTESIAN_POINT ( 'NONE',  ( -5.153800228976607833, 19.02544592524334988, 32.70942372801899722 ) ) ;
#11563=CARTESIAN_POINT ( 'NONE',  ( 8.314922557960818139, 14.29746914071049879, 79.58224293864769550 ) ) ;
#11564=CARTESIAN_POINT ( 'NONE',  ( 10.81492255796106328, -18.62759615963255655, 110.4177570613523756 ) ) ;
#11565=CARTESIAN_POINT ( 'NONE',  ( -16.51473224551069308, -9.474510206698971260, 56.66557627198103120 ) ) ;
#11566=CARTESIAN_POINT ( 'NONE',  ( 14.29746914071049879, -8.314922557960816363, 38.33224293864768839 ) ) ;
#11567=CARTESIAN_POINT ( 'NONE',  ( 0.05219959533937995610, -21.53943276465977519, 105.0010903946856757 ) ) ;
#11568=CARTESIAN_POINT ( 'NONE',  ( -19.03943276465977164, 0.05219959533909376836, 91.24890960531436690 ) ) ;
#11569=CARTESIAN_POINT ( 'NONE',  ( -19.02544592524342804, 5.153800228976336051, 111.0405762719810099 ) ) ;
#11570=CARTESIAN_POINT ( 'NONE',  ( 13.97604488694527802, 13.89961937509977652, 44.37390960531435269 ) ) ;
#11571=CARTESIAN_POINT ( 'NONE',  ( 0.05219959533910956823, 16.53943276465976808, 114.9989096053143669 ) ) ;
#11572=CARTESIAN_POINT ( 'NONE',  ( 12.06949235617757843, -12.14591786802309237, 83.12390960531436690 ) ) ;
#11573=CARTESIAN_POINT ( 'NONE',  ( 21.52544592524344225, -5.823673210054117533, 93.54057627198103830 ) ) ;
#11574=CARTESIAN_POINT ( 'NONE',  ( 9.564922557960805705, 16.46253265017160317, 89.58224293864769550 ) ) ;
#11575=CARTESIAN_POINT ( 'NONE',  ( 21.55341960407610458, 5.719274019375980345, 93.95724293864770971 ) ) ;
#11576=CARTESIAN_POINT ( 'NONE',  ( -9.474510206698964154, 16.51473224551069663, 85.41557627198102409 ) ) ;
#11577=PLANE ( 'NONE',  #52581 ) ;
#11578=CARTESIAN_POINT ( 'NONE',  ( 16.52544592524342804, -4.483927247898539470, 103.5405762719810383 ) ) ;
#11579=CARTESIAN_POINT ( 'NONE',  ( -5.153800228976328057, -19.02544592524343514, 67.29057627198102409 ) ) ;
#11580=CARTESIAN_POINT ( 'NONE',  ( 21.52544592524344225, -5.823673210054117533, 73.54057627198102409 ) ) ;
#11582=CARTESIAN_POINT ( 'NONE',  ( 10.72451020669898902, -18.67979575497178502, 22.91557627198102765 ) ) ;
#11584=CARTESIAN_POINT ( 'NONE',  ( -14.29746914071037622, -8.314922557961029526, 29.16775706135234003 ) ) ;
#11585=CARTESIAN_POINT ( 'NONE',  ( 8.224510206698953496, -14.34966873604960469, 97.91557627198103830 ) ) ;
#11586=CARTESIAN_POINT ( 'NONE',  ( 19.02130022317635749, -5.499999999999802824, 53.28188669246574705 ) ) ;
#11587=CARTESIAN_POINT ( 'NONE',  ( -5.153800228976328057, -19.02544592524343514, 87.29057627198103830 ) ) ;
#11588=CARTESIAN_POINT ( 'NONE',  ( -19.05341960407611168, -5.049401038298163336, 46.45724293864768129 ) ) ;
#11589=CARTESIAN_POINT ( 'NONE',  ( 8.224510206698953496, -14.34966873604960469, 77.91557627198102409 ) ) ;
#11590=CARTESIAN_POINT ( 'NONE',  ( 0.05219959533907565091, 21.53943276465977519, 29.99890960531435979 ) ) ;
#11591=CARTESIAN_POINT ( 'NONE',  ( -14.29746914071049879, 8.314922557960819915, 55.83224293864770260 ) ) ;
#11592=CARTESIAN_POINT ( 'NONE',  ( 19.02544592524334988, 5.153800228976608722, 96.45942372801897591 ) ) ;
#11593=CARTESIAN_POINT ( 'NONE',  ( -18.67979575497193778, 10.72451020669871902, 63.33442372801900433 ) ) ;
#11595=CARTESIAN_POINT ( 'NONE',  ( -5.153800228976328057, -19.02544592524343514, 102.2905762719810383 ) ) ;
#11596=CARTESIAN_POINT ( 'NONE',  ( 4.379528057220092307, 16.55341960407617563, 82.29275706135234714 ) ) ;
#11597=CARTESIAN_POINT ( 'NONE',  ( 13.89961937509977652, -13.97604488694527269, 28.12390960531435624 ) ) ;
#11598=CARTESIAN_POINT ( 'NONE',  ( 9.564922557960805705, 16.46253265017160317, 79.58224293864769550 ) ) ;
#11599=CARTESIAN_POINT ( 'NONE',  ( 0.05219959533907565091, 21.53943276465977519, 79.99890960531435269 ) ) ;
#11600=CARTESIAN_POINT ( 'NONE',  ( 5.049401038297881783, 19.05341960407617563, 107.2927570613523187 ) ) ;
#11601=CARTESIAN_POINT ( 'NONE',  ( 16.53943276465976808, -0.05219959533910856209, 48.74890960531435979 ) ) ;
#11602=CARTESIAN_POINT ( 'NONE',  ( 5.823673210054444382, -21.52544592524334988, 60.20942372801902565 ) ) ;
#11603=CARTESIAN_POINT ( 'NONE',  ( -4.483927247898782831, 16.52544592524335698, 82.70942372801900433 ) ) ;
#11604=CARTESIAN_POINT ( 'NONE',  ( -5.719274019375978568, 21.55341960407610458, 30.20724293864769550 ) ) ;
#11607=CARTESIAN_POINT ( 'NONE',  ( 12.06949235617739724, 12.14591786802326823, 111.8760903946856615 ) ) ;
#11608=CARTESIAN_POINT ( 'NONE',  ( 16.53943276465976808, 0.05219959533934440121, 61.25109039468567573 ) ) ;
#11609=CARTESIAN_POINT ( 'NONE',  ( 5.153800228976335163, 19.02544592524342804, 69.79057627198103830 ) ) ;
#11610=CARTESIAN_POINT ( 'NONE',  ( 19.05341960407611168, 5.049401038298154454, 83.95724293864766707 ) ) ;
#11611=CARTESIAN_POINT ( 'NONE',  ( -15.80617190586768217, 15.72974639402176855, 68.12609039468567573 ) ) ;
#11612=CARTESIAN_POINT ( 'NONE',  ( -16.53943276465976808, -0.05219959533934237506, 73.75109039468567573 ) ) ;
#11613=CARTESIAN_POINT ( 'NONE',  ( -0.05219959533910754901, -16.53943276465976808, 42.49890960531435979 ) ) ;
#11614=CARTESIAN_POINT ( 'NONE',  ( -19.05341960407611168, -5.049401038298163336, 56.45724293864768129 ) ) ;
#11615=CARTESIAN_POINT ( 'NONE',  ( -13.89961937509977652, 13.97604488694528158, 50.62390960531435979 ) ) ;
#11616=CARTESIAN_POINT ( 'NONE',  ( -12.14591786802326823, 12.06949235617739902, 43.12609039468568284 ) ) ;
#11618=CARTESIAN_POINT ( 'NONE',  ( 5.153800228976615827, -19.02544592524334988, 100.2094237280190043 ) ) ;
#11619=CARTESIAN_POINT ( 'NONE',  ( -8.224510206698948167, 14.34966873604960824, 100.4155762719810241 ) ) ;
#11620=CARTESIAN_POINT ( 'NONE',  ( -16.46253265017160317, 9.564922557960807481, 60.83224293864769550 ) ) ;
#11621=CARTESIAN_POINT ( 'NONE',  ( 16.51473224551083163, -9.474510206698727899, 95.83442372801900433 ) ) ;
#11623=CARTESIAN_POINT ( 'NONE',  ( -15.72974639402176322, -15.80617190586768395, 104.3760903946856899 ) ) ;
#11624=CARTESIAN_POINT ( 'NONE',  ( -0.05219959533934338120, 16.53943276465976808, 62.50109039468568284 ) ) ;
#11626=CARTESIAN_POINT ( 'NONE',  ( 18.62759615963271287, -10.81492255796078972, 68.33224293864769550 ) ) ;
#11627=CARTESIAN_POINT ( 'NONE',  ( -0.05219959533934338120, 16.53943276465976808, 47.50109039468568994 ) ) ;
#11629=CARTESIAN_POINT ( 'NONE',  ( 16.51473224551083163, -9.474510206698727899, 40.83442372801900433 ) ) ;
#11631=CARTESIAN_POINT ( 'NONE',  ( 13.97604488694527802, 13.89961937509977652, 84.37390960531433848 ) ) ;
#11632=CARTESIAN_POINT ( 'NONE',  ( -19.05341960407611168, -5.049401038298163336, 26.45724293864769550 ) ) ;
#11633=CARTESIAN_POINT ( 'NONE',  ( 19.05341960407611168, 5.049401038298154454, 58.95724293864768129 ) ) ;
#11634=CARTESIAN_POINT ( 'NONE',  ( 4.379528057220339221, -16.55341960407611168, 57.70724293864770260 ) ) ;
#11635=CARTESIAN_POINT ( 'NONE',  ( 0.05219959533937995610, -21.53943276465977519, 80.00109039468568994 ) ) ;
#11636=CARTESIAN_POINT ( 'NONE',  ( 13.89961937509957401, 13.97604488694547697, 46.87609039468565442 ) ) ;
#11637=CARTESIAN_POINT ( 'NONE',  ( -13.89961937509957401, -13.97604488694547875, 29.37609039468565797 ) ) ;
#11638=CARTESIAN_POINT ( 'NONE',  ( -19.05341960407611168, -5.049401038298163336, 51.45724293864770260 ) ) ;
#11639=CARTESIAN_POINT ( 'NONE',  ( -0.05219959533907301413, -21.53943276465977519, 22.49890960531436335 ) ) ;
#11640=CARTESIAN_POINT ( 'NONE',  ( 18.67979575497194134, -10.72451020669871369, 100.8344237280190185 ) ) ;
#11641=CARTESIAN_POINT ( 'NONE',  ( -9.474510206698964154, 16.51473224551069663, 65.41557627198102409 ) ) ;
#11642=EDGE_CURVE ( 'NONE', #78253, #165007, #123449, .T. ) ;
#11643=CARTESIAN_POINT ( 'NONE',  ( 21.52544592524334988, 5.823673210054432836, 91.45942372801901854 ) ) ;
#11644=CARTESIAN_POINT ( 'NONE',  ( -10.72451020669898014, 18.67979575497178502, 35.41557627198102409 ) ) ;
#11645=CARTESIAN_POINT ( 'NONE',  ( 13.89961937509977652, -13.97604488694527269, 88.12390960531438111 ) ) ;
#11646=CARTESIAN_POINT ( 'NONE',  ( -13.97604488694547697, 13.89961937509957934, 68.12609039468563310 ) ) ;
#11647=CARTESIAN_POINT ( 'NONE',  ( 9.474510206698971260, -16.51473224551069308, 42.91557627198103120 ) ) ;
#11648=CARTESIAN_POINT ( 'NONE',  ( -0.05219959533909027116, -19.03943276465977164, 87.49890960531436690 ) ) ;
#11649=CARTESIAN_POINT ( 'NONE',  ( 16.52544592524335698, 4.483927247898782831, 31.45942372801901854 ) ) ;
#11650=CARTESIAN_POINT ( 'NONE',  ( 14.29746914071049879, -8.314922557960816363, 88.33224293864769550 ) ) ;
#11651=CARTESIAN_POINT ( 'NONE',  ( 13.89961937509977652, -13.97604488694527269, 68.12390960531436690 ) ) ;
#11652=CARTESIAN_POINT ( 'NONE',  ( 0.05219959533907565091, 21.53943276465977519, 54.99890960531435269 ) ) ;
#11653=CARTESIAN_POINT ( 'NONE',  ( -19.03943276465977164, -0.05219959533935918106, 113.7510903946856757 ) ) ;
#11654=CARTESIAN_POINT ( 'NONE',  ( 10.81492255796078972, 18.62759615963270932, 114.5822429386477097 ) ) ;
#11655=CARTESIAN_POINT ( 'NONE',  ( 5.719274019375673035, 21.55341960407619339, 67.29275706135234714 ) ) ;
#11656=CARTESIAN_POINT ( 'NONE',  ( -14.34966873604972548, 8.224510206698743886, 68.33442372801900433 ) ) ;
#11657=CARTESIAN_POINT ( 'NONE',  ( 16.55341960407618274, -4.379528057220086978, 66.04275706135236135 ) ) ;
#11658=CARTESIAN_POINT ( 'NONE',  ( -5.049401038298153566, 19.05341960407611168, 60.20724293864768129 ) ) ;
#11659=CARTESIAN_POINT ( 'NONE',  ( -12.14591786802326823, 12.06949235617739902, 108.1260903946856757 ) ) ;
#11660=CARTESIAN_POINT ( 'NONE',  ( 5.049401038297881783, 19.05341960407617563, 42.29275706135234003 ) ) ;
#11661=CARTESIAN_POINT ( 'NONE',  ( -15.72974639402176322, -15.80617190586768395, 34.37609039468568284 ) ) ;
#11662=CARTESIAN_POINT ( 'NONE',  ( 16.53943276465976808, -0.05219959533910856209, 63.74890960531435979 ) ) ;
#11663=CARTESIAN_POINT ( 'NONE',  ( 0.05219959533909260263, 19.03943276465977164, 104.9989096053143669 ) ) ;
#11664=CARTESIAN_POINT ( 'NONE',  ( -8.224510206698735004, -14.34966873604973081, 94.58442372801901854 ) ) ;
#11665=CARTESIAN_POINT ( 'NONE',  ( -21.55341960407619339, 5.719274019375674811, 73.54275706135234714 ) ) ;
#11666=CARTESIAN_POINT ( 'NONE',  ( 16.52544592524335698, 4.483927247898782831, 26.45942372801901854 ) ) ;
#11667=CARTESIAN_POINT ( 'NONE',  ( -21.55341960407619339, 5.719274019375674811, 23.54275706135235424 ) ) ;
#11668=CARTESIAN_POINT ( 'NONE',  ( -14.34966873604960291, -8.224510206698953496, 56.66557627198103830 ) ) ;
#11669=VERTEX_POINT ( 'NONE', #170990 ) ;
#11670=CARTESIAN_POINT ( 'NONE',  ( -5.823673210054116645, -21.52544592524344225, 102.2905762719810383 ) ) ;
#11671=CARTESIAN_POINT ( 'NONE',  ( 16.53943276465976808, -0.05219959533910856209, 43.74890960531435979 ) ) ;
#11672=VERTEX_POINT ( 'NONE', #2133 ) ;
#11673=CARTESIAN_POINT ( 'NONE',  ( -19.02544592524342804, 5.153800228976336051, 26.04057627198103120 ) ) ;
#11674=CARTESIAN_POINT ( 'NONE',  ( -18.62759615963270932, 10.81492255796079327, 30.83224293864770260 ) ) ;
#11675=CARTESIAN_POINT ( 'NONE',  ( -10.81492255796105439, 18.62759615963255655, 32.91775706135234714 ) ) ;
#11676=CARTESIAN_POINT ( 'NONE',  ( 14.29746914071049879, -8.314922557960816363, 63.33224293864770260 ) ) ;
#11678=CARTESIAN_POINT ( 'NONE',  ( 5.823673210054125526, 21.52544592524343514, 69.79057627198102409 ) ) ;
#11679=CARTESIAN_POINT ( 'NONE',  ( -13.97604488694527625, -13.89961937509977652, 71.87390960531433848 ) ) ;
#11680=CARTESIAN_POINT ( 'NONE',  ( 0.05219959533909260263, 19.03943276465977164, 24.99890960531435269 ) ) ;
#11681=CARTESIAN_POINT ( 'NONE',  ( -13.97604488694547697, 13.89961937509957934, 83.12609039468564731 ) ) ;
#11682=CARTESIAN_POINT ( 'NONE',  ( -10.72451020669898014, 18.67979575497178502, 45.41557627198103830 ) ) ;
#11683=CARTESIAN_POINT ( 'NONE',  ( 0.05219959533909260263, 19.03943276465977164, 39.99890960531436690 ) ) ;
#11684=CARTESIAN_POINT ( 'NONE',  ( -19.03943276465977164, 0.05219959533909376836, 71.24890960531435269 ) ) ;
#11686=CARTESIAN_POINT ( 'NONE',  ( -8.314922557961024197, 14.29746914071037800, 37.91775706135235424 ) ) ;
#11687=CARTESIAN_POINT ( 'NONE',  ( 15.72974639402176855, 15.80617190586768217, 21.87609039468567573 ) ) ;
#11688=CARTESIAN_POINT ( 'NONE',  ( 8.314922557960818139, 14.29746914071049879, 44.58224293864769550 ) ) ;
#11689=CARTESIAN_POINT ( 'NONE',  ( 13.89961937509977652, -13.97604488694527269, 108.1239096053143669 ) ) ;
#11690=CARTESIAN_POINT ( 'NONE',  ( -0.05219959533907301413, -21.53943276465977519, 77.49890960531433848 ) ) ;
#11691=CARTESIAN_POINT ( 'NONE',  ( 15.80617190586746368, 15.72974639402197994, 104.3739096053143669 ) ) ;
#11692=CARTESIAN_POINT ( 'NONE',  ( 16.52544592524335698, 4.483927247898782831, 46.45942372801901854 ) ) ;
#11693=CARTESIAN_POINT ( 'NONE',  ( -0.05219959533907301413, -21.53943276465977519, 47.49890960531435979 ) ) ;
#11694=CARTESIAN_POINT ( 'NONE',  ( -21.52544592524334988, -5.823673210054445271, 98.95942372801903275 ) ) ;
#11695=CARTESIAN_POINT ( 'NONE',  ( 9.564922557960805705, 16.46253265017160317, 49.58224293864770260 ) ) ;
#11696=CARTESIAN_POINT ( 'NONE',  ( 9.564922557960805705, 16.46253265017160317, 94.58224293864769550 ) ) ;
#11697=CARTESIAN_POINT ( 'NONE',  ( -5.049401038298153566, 19.05341960407611168, 70.20724293864769550 ) ) ;
#11699=CARTESIAN_POINT ( 'NONE',  ( 9.564922557961047289, -16.46253265017146816, 55.41775706135234003 ) ) ;
#11700=CARTESIAN_POINT ( 'NONE',  ( -21.53943276465977519, -0.05219959533937600094, 113.7510903946856757 ) ) ;
#11701=CARTESIAN_POINT ( 'NONE',  ( 15.80617190586746368, 15.72974639402197994, 29.37390960531435269 ) ) ;
#11702=CARTESIAN_POINT ( 'NONE',  ( -16.52544592524335698, -4.483927247898792601, 108.9594237280190185 ) ) ;
#11703=CARTESIAN_POINT ( 'NONE',  ( 13.89961937509957401, 13.97604488694547697, 91.87609039468567573 ) ) ;
#11704=CARTESIAN_POINT ( 'NONE',  ( -16.20579543436675962, 7.371946100355235565, 59.43479165828123456 ) ) ;
#11705=CARTESIAN_POINT ( 'NONE',  ( -13.97604488694547697, 13.89961937509957934, 23.12609039468565442 ) ) ;
#11706=CARTESIAN_POINT ( 'NONE',  ( -13.89961937509957401, -13.97604488694547875, 84.37609039468567573 ) ) ;
#11707=CARTESIAN_POINT ( 'NONE',  ( -16.46253265017146816, -9.564922557961047289, 44.16775706135232582 ) ) ;
#11708=DIRECTION ( 'NONE',  ( 0.000000000000000000, 0.000000000000000000, 1.000000000000000000 ) ) ;
#11709=CARTESIAN_POINT ( 'NONE',  ( -5.153800228976328057, -19.02544592524343514, 47.29057627198102409 ) ) ;
#11710=CARTESIAN_POINT ( 'NONE',  ( -14.29746914071049879, 8.314922557960819915, 55.83224293864770260 ) ) ;
#11711=CARTESIAN_POINT ( 'NONE',  ( 9.474510206698971260, -16.51473224551069308, 27.91557627198103120 ) ) ;
#11712=CARTESIAN_POINT ( 'NONE',  ( -16.53943276465976808, 0.05219959533911058130, 36.24890960531435979 ) ) ;
#11714=CARTESIAN_POINT ( 'NONE',  ( 14.34966873604972726, -8.224510206698740333, 105.8344237280190328 ) ) ;
#11715=CARTESIAN_POINT ( 'NONE',  ( -19.03943276465977164, 0.05219959533909376836, 51.24890960531436690 ) ) ;
#11716=CARTESIAN_POINT ( 'NONE',  ( -5.823673210054431948, 21.52544592524334988, 107.7094237280190328 ) ) ;
#11717=CARTESIAN_POINT ( 'NONE',  ( 4.483927247898790824, -16.52544592524335698, 35.20942372801901854 ) ) ;
#11718=CARTESIAN_POINT ( 'NONE',  ( 15.72974639402199770, -15.80617190586745480, 38.12390960531436690 ) ) ;
#11719=CARTESIAN_POINT ( 'NONE',  ( 5.719274019375673035, 21.55341960407619339, 92.29275706135236135 ) ) ;
#11720=CARTESIAN_POINT ( 'NONE',  ( 0.05219959533909260263, 19.03943276465977164, 99.99890960531436690 ) ) ;
#11721=CARTESIAN_POINT ( 'NONE',  ( 5.153800228976335163, 19.02544592524342804, 89.79057627198102409 ) ) ;
#11723=CARTESIAN_POINT ( 'NONE',  ( 18.62759615963271287, -10.81492255796078972, 108.3322429386477097 ) ) ;
#11725=CARTESIAN_POINT ( 'NONE',  ( -8.224510206698948167, 14.34966873604960824, 85.41557627198102409 ) ) ;
#11726=CARTESIAN_POINT ( 'NONE',  ( 15.80617190586746368, 15.72974639402197994, 79.37390960531436690 ) ) ;
#11727=CARTESIAN_POINT ( 'NONE',  ( 16.46253265017160672, -9.564922557960803928, 73.33224293864769550 ) ) ;
#11728=CARTESIAN_POINT ( 'NONE',  ( 10.72451020669898902, -18.67979575497178502, 102.9155762719810383 ) ) ;
#11730=VERTEX_POINT ( 'NONE', #138653 ) ;
#11731=CARTESIAN_POINT ( 'NONE',  ( 5.153800228976335163, 19.02544592524342804, 54.79057627198103120 ) ) ;
#11732=CARTESIAN_POINT ( 'NONE',  ( -8.314922557960811034, -14.29746914071050412, 92.08224293864769550 ) ) ;
#11733=CARTESIAN_POINT ( 'NONE',  ( 16.51473224551069308, 9.474510206698969483, 24.16557627198102765 ) ) ;
#11734=CARTESIAN_POINT ( 'NONE',  ( 5.049401038298161559, -19.05341960407611168, 67.70724293864769550 ) ) ;
#11735=CARTESIAN_POINT ( 'NONE',  ( -5.049401038297874678, -19.05341960407617918, 74.79275706135231871 ) ) ;
#11736=CARTESIAN_POINT ( 'NONE',  ( -16.52544592524342804, 4.483927247898546575, 101.0405762719810383 ) ) ;
#11737=CARTESIAN_POINT ( 'NONE',  ( -21.52544592524334988, -5.823673210054445271, 58.95942372801902565 ) ) ;
#11738=CARTESIAN_POINT ( 'NONE',  ( -13.97604488694527625, -13.89961937509977652, 46.87390960531435979 ) ) ;
#11739=CARTESIAN_POINT ( 'NONE',  ( -21.55341960407619339, 5.719274019375674811, 23.54275706135235424 ) ) ;
#11740=CARTESIAN_POINT ( 'NONE',  ( 8.224510206698953496, -14.34966873604960469, 107.9155762719810241 ) ) ;
#11741=CYLINDRICAL_SURFACE ( 'NONE', #185239, 2.000000000000001776 ) ;
#11742=CARTESIAN_POINT ( 'NONE',  ( 19.05341960407611168, 5.049401038298154454, 53.95724293864770260 ) ) ;
#11744=CARTESIAN_POINT ( 'NONE',  ( 19.05341960407617918, -5.049401038297876454, 106.0427570613523471 ) ) ;
#11745=CARTESIAN_POINT ( 'NONE',  ( -5.153800228976328057, -19.02544592524343514, 112.2905762719810099 ) ) ;
#11746=CARTESIAN_POINT ( 'NONE',  ( -21.55341960407619339, 5.719274019375674811, 43.54275706135235424 ) ) ;
#11747=CARTESIAN_POINT ( 'NONE',  ( -9.564922557960796823, -16.46253265017161027, 97.08224293864769550 ) ) ;
#11748=CARTESIAN_POINT ( 'NONE',  ( -5.049401038297874678, -19.05341960407617918, 84.79275706135233293 ) ) ;
#11749=CARTESIAN_POINT ( 'NONE',  ( 13.89961937509977652, -13.97604488694527269, 63.12390960531435979 ) ) ;
#11750=CARTESIAN_POINT ( 'NONE',  ( 14.34966873604960469, 8.224510206698951720, 79.16557627198103830 ) ) ;
#11751=CARTESIAN_POINT ( 'NONE',  ( 5.049401038298161559, -19.05341960407611168, 87.70724293864769550 ) ) ;
#11752=CARTESIAN_POINT ( 'NONE',  ( -16.53943276465976808, 0.05219959533911058130, 76.24890960531435269 ) ) ;
#11753=CARTESIAN_POINT ( 'NONE',  ( -19.02544592524342804, 5.153800228976336051, 81.04057627198103830 ) ) ;
#11754=CARTESIAN_POINT ( 'NONE',  ( 19.05341960407617918, -5.049401038297876454, 31.04275706135232227 ) ) ;
#11755=CARTESIAN_POINT ( 'NONE',  ( 19.05341960407611168, 5.049401038298154454, 43.95724293864769550 ) ) ;
#11756=CARTESIAN_POINT ( 'NONE',  ( 12.14591786802309770, 12.06949235617756955, 49.37390960531436690 ) ) ;
#11757=CARTESIAN_POINT ( 'NONE',  ( 19.02544592524343514, -5.153800228976328945, 23.54057627198102054 ) ) ;
#11759=CARTESIAN_POINT ( 'NONE',  ( 21.52544592524334988, 5.823673210054432836, 46.45942372801901854 ) ) ;
#11760=CARTESIAN_POINT ( 'NONE',  ( 19.05341960407617918, -5.049401038297876454, 76.04275706135230450 ) ) ;
#11761=CARTESIAN_POINT ( 'NONE',  ( -4.379528057220328563, 16.55341960407611168, 30.20724293864769550 ) ) ;
#11762=CARTESIAN_POINT ( 'NONE',  ( 10.72451020669898902, -18.67979575497178502, 97.91557627198103830 ) ) ;
#11763=CARTESIAN_POINT ( 'NONE',  ( -18.67979575497178146, -10.72451020669898902, 36.66557627198103120 ) ) ;
#11765=CARTESIAN_POINT ( 'NONE',  ( -8.224510206698948167, 14.34966873604960824, 75.41557627198102409 ) ) ;
#11766=CARTESIAN_POINT ( 'NONE',  ( 0.05219959533909260263, 19.03943276465977164, 44.99890960531435979 ) ) ;
#11767=CARTESIAN_POINT ( 'NONE',  ( -16.55341960407617563, 4.379528057220093196, 108.5427570613523756 ) ) ;
#11769=CARTESIAN_POINT ( 'NONE',  ( 4.379528057220092307, 16.55341960407617563, 67.29275706135234714 ) ) ;
#11770=CARTESIAN_POINT ( 'NONE',  ( -13.97604488694547697, 13.89961937509957934, 23.12609039468565442 ) ) ;
#11771=CARTESIAN_POINT ( 'NONE',  ( -9.564922557960796823, -16.46253265017161027, 92.08224293864769550 ) ) ;
#11772=CARTESIAN_POINT ( 'NONE',  ( 5.049401038298161559, -19.05341960407611168, 77.70724293864765286 ) ) ;
#11774=CARTESIAN_POINT ( 'NONE',  ( -14.34966873604972548, 8.224510206698743886, 78.33442372801901854 ) ) ;
#11775=CARTESIAN_POINT ( 'NONE',  ( -5.153800228976328057, -19.02544592524343514, 42.29057627198101699 ) ) ;
#11776=CARTESIAN_POINT ( 'NONE',  ( 16.53943276465976808, -0.05219959533910856209, 48.74890960531435979 ) ) ;
#11777=CARTESIAN_POINT ( 'NONE',  ( -19.03943276465977164, 0.05219959533909376836, 101.2489096053143669 ) ) ;
#11778=CARTESIAN_POINT ( 'NONE',  ( -5.153800228976328057, -19.02544592524343514, 87.29057627198103830 ) ) ;
#11779=CARTESIAN_POINT ( 'NONE',  ( 10.72451020669898902, -18.67979575497178502, 22.91557627198102765 ) ) ;
#11780=CARTESIAN_POINT ( 'NONE',  ( -8.224510206698948167, 14.34966873604960824, 75.41557627198102409 ) ) ;
#11781=CARTESIAN_POINT ( 'NONE',  ( 16.52544592524342804, -4.483927247898539470, 63.54057627198103830 ) ) ;
#11782=CARTESIAN_POINT ( 'NONE',  ( 8.224510206698742110, 14.34966873604972548, 47.08442372801901854 ) ) ;
#11783=CARTESIAN_POINT ( 'NONE',  ( 17.49999999999999289, -3.345213924137297123, 32.08768623094358219 ) ) ;
#11784=CARTESIAN_POINT ( 'NONE',  ( -5.153800228976607833, 19.02544592524334988, 62.70942372801899722 ) ) ;
#11785=CARTESIAN_POINT ( 'NONE',  ( -9.564922557960796823, -16.46253265017161027, 87.08224293864769550 ) ) ;
#11786=CARTESIAN_POINT ( 'NONE',  ( 16.51473224551083163, -9.474510206698727899, 60.83442372801900433 ) ) ;
#11788=CARTESIAN_POINT ( 'NONE',  ( -8.224510206698735004, -14.34966873604973081, 19.58442372801901143 ) ) ;
#11789=CARTESIAN_POINT ( 'NONE',  ( -4.379528057220086978, -16.55341960407618274, 94.79275706135234714 ) ) ;
#11790=CARTESIAN_POINT ( 'NONE',  ( 5.049401038298161559, -19.05341960407611168, 37.70724293864768839 ) ) ;
#11791=CARTESIAN_POINT ( 'NONE',  ( -21.52544592524343514, 5.823673210054127303, 26.04057627198103475 ) ) ;
#11792=CARTESIAN_POINT ( 'NONE',  ( 5.823673210054444382, -21.52544592524334988, 50.20942372801901854 ) ) ;
#11793=CARTESIAN_POINT ( 'NONE',  ( 19.05341960407617918, -5.049401038297876454, 106.0427570613523471 ) ) ;
#11795=CARTESIAN_POINT ( 'NONE',  ( 16.46253265017160672, -9.564922557960803928, 73.33224293864769550 ) ) ;
#11797=CARTESIAN_POINT ( 'NONE',  ( -16.55341960407611168, -4.379528057220339221, 76.45724293864769550 ) ) ;
#11798=CARTESIAN_POINT ( 'NONE',  ( -13.89961937509977652, 13.97604488694528158, 75.62390960531438111 ) ) ;
#11800=CARTESIAN_POINT ( 'NONE',  ( 5.153800228976335163, 19.02544592524342804, 74.79057627198103830 ) ) ;
#11801=CARTESIAN_POINT ( 'NONE',  ( -0.05219959533936034679, 19.03943276465977164, 82.50109039468567573 ) ) ;
#11802=CARTESIAN_POINT ( 'NONE',  ( -5.719274019375978568, 21.55341960407610458, 65.20724293864768129 ) ) ;
#11803=CARTESIAN_POINT ( 'NONE',  ( 19.03943276465977164, -0.05219959533909143690, 28.74890960531435624 ) ) ;
#11804=CARTESIAN_POINT ( 'NONE',  ( 13.89961937509957401, 13.97604488694547697, 61.87609039468566863 ) ) ;
#11805=CARTESIAN_POINT ( 'NONE',  ( 16.46253265017160672, -9.564922557960803928, 58.33224293864769550 ) ) ;
#11806=CARTESIAN_POINT ( 'NONE',  ( 19.03943276465977164, -0.05219959533909143690, 93.74890960531435269 ) ) ;
#11808=CARTESIAN_POINT ( 'NONE',  ( -21.55341960407610458, -5.719274019375992779, 86.45724293864770971 ) ) ;
#11809=CARTESIAN_POINT ( 'NONE',  ( -8.224510206698948167, 14.34966873604960824, 90.41557627198103830 ) ) ;
#11810=CARTESIAN_POINT ( 'NONE',  ( 5.049401038297881783, 19.05341960407617563, 42.29275706135234003 ) ) ;
#11811=CARTESIAN_POINT ( 'NONE',  ( 15.80617190586746368, 15.72974639402197994, 79.37390960531436690 ) ) ;
#11812=CARTESIAN_POINT ( 'NONE',  ( 10.72451020669898902, -18.67979575497178502, 57.91557627198103120 ) ) ;
#11813=CARTESIAN_POINT ( 'NONE',  ( 16.53943276465976808, -0.05219959533910856209, 28.74890960531435624 ) ) ;
#11814=CARTESIAN_POINT ( 'NONE',  ( -18.67979575497193778, 10.72451020669871902, 103.3344237280190043 ) ) ;
#11815=CARTESIAN_POINT ( 'NONE',  ( 5.049401038298161559, -19.05341960407611168, 77.70724293864765286 ) ) ;
#11816=CARTESIAN_POINT ( 'NONE',  ( -5.153800228976328057, -19.02544592524343514, 32.29057627198102409 ) ) ;
#11817=CARTESIAN_POINT ( 'NONE',  ( -10.72451020669870658, -18.67979575497194134, 34.58442372801900433 ) ) ;
#11818=CARTESIAN_POINT ( 'NONE',  ( 18.62759615963255655, 10.81492255796105972, 46.66775706135234714 ) ) ;
#11819=CARTESIAN_POINT ( 'NONE',  ( 13.97604488694527802, 13.89961937509977652, 54.37390960531435979 ) ) ;
#11820=CARTESIAN_POINT ( 'NONE',  ( -10.72451020669870658, -18.67979575497194134, 24.58442372801901499 ) ) ;
#11821=CARTESIAN_POINT ( 'NONE',  ( -0.05219959533936034679, 19.03943276465977164, 57.50109039468566863 ) ) ;
#11822=CARTESIAN_POINT ( 'NONE',  ( -19.03943276465977164, 0.05219959533909376836, 31.24890960531435979 ) ) ;
#11823=CARTESIAN_POINT ( 'NONE',  ( 12.06949235617739724, 12.14591786802326823, 21.87609039468567573 ) ) ;
#11824=CARTESIAN_POINT ( 'NONE',  ( 16.51473224551069308, 9.474510206698969483, 29.16557627198103475 ) ) ;
#11825=CARTESIAN_POINT ( 'NONE',  ( 14.34966873604972726, -8.224510206698740333, 75.83442372801900433 ) ) ;
#11826=CARTESIAN_POINT ( 'NONE',  ( -19.02544592524342804, 5.153800228976336051, 46.04057627198101699 ) ) ;
#11828=CARTESIAN_POINT ( 'NONE',  ( -19.02544592524342804, 5.153800228976336051, 81.04057627198103830 ) ) ;
#11829=CARTESIAN_POINT ( 'NONE',  ( 19.05341960407611168, 5.049401038298154454, 28.95724293864769550 ) ) ;
#11830=CARTESIAN_POINT ( 'NONE',  ( -0.05219959533907301413, -21.53943276465977519, 77.49890960531433848 ) ) ;
#11831=CARTESIAN_POINT ( 'NONE',  ( 16.53943276465976808, 0.05219959533934440121, 46.25109039468567573 ) ) ;
#11832=CARTESIAN_POINT ( 'NONE',  ( -21.53943276465977519, -0.05219959533937600094, 98.75109039468568994 ) ) ;
#11833=EDGE_CURVE ( 'NONE', #198671, #10418, #185165, .T. ) ;
#11834=CARTESIAN_POINT ( 'NONE',  ( 16.51473224551069308, 9.474510206698969483, 44.16557627198103120 ) ) ;
#11835=CARTESIAN_POINT ( 'NONE',  ( 14.29746914071049879, -8.314922557960816363, 28.33224293864769550 ) ) ;
#11836=CARTESIAN_POINT ( 'NONE',  ( 16.55341960407611168, 4.379528057220329451, 68.95724293864769550 ) ) ;
#11837=CARTESIAN_POINT ( 'NONE',  ( -13.97604488694527625, -13.89961937509977652, 71.87390960531433848 ) ) ;
#11838=CARTESIAN_POINT ( 'NONE',  ( 10.72451020669871369, 18.67979575497193778, 112.0844237280190185 ) ) ;
#11839=CARTESIAN_POINT ( 'NONE',  ( -21.55341960407619339, 5.719274019375674811, 28.54275706135234358 ) ) ;
#11840=CARTESIAN_POINT ( 'NONE',  ( -0.05219959533909027116, -19.03943276465977164, 77.49890960531435269 ) ) ;
#11841=CARTESIAN_POINT ( 'NONE',  ( -10.72451020669870658, -18.67979575497194134, 79.58442372801903275 ) ) ;
#11842=CARTESIAN_POINT ( 'NONE',  ( 12.14591786802327356, -12.06949235617739191, 70.62609039468567573 ) ) ;
#11843=CARTESIAN_POINT ( 'NONE',  ( 12.14591786802327356, -12.06949235617739191, 35.62609039468568994 ) ) ;
#11844=CARTESIAN_POINT ( 'NONE',  ( -4.483927247898539470, -16.52544592524342804, 92.29057627198103830 ) ) ;
#11845=CARTESIAN_POINT ( 'NONE',  ( -18.62759615963255300, -10.81492255796106328, 104.1677570613523471 ) ) ;
#11847=CARTESIAN_POINT ( 'NONE',  ( -8.314922557960811034, -14.29746914071050412, 37.08224293864768129 ) ) ;
#11848=CARTESIAN_POINT ( 'NONE',  ( 5.153800228976335163, 19.02544592524342804, 24.79057627198102765 ) ) ;
#11849=CARTESIAN_POINT ( 'NONE',  ( 16.52544592524335698, 4.483927247898782831, 46.45942372801901854 ) ) ;
#11850=CARTESIAN_POINT ( 'NONE',  ( 4.483927247898545687, 16.52544592524342804, 49.79057627198102409 ) ) ;
#11851=CARTESIAN_POINT ( 'NONE',  ( -12.14591786802326823, 12.06949235617739902, 103.1260903946856757 ) ) ;
#11852=CARTESIAN_POINT ( 'NONE',  ( 13.89961937509977652, -13.97604488694527269, 113.1239096053143527 ) ) ;
#11853=CARTESIAN_POINT ( 'NONE',  ( 15.72974639402199770, -15.80617190586745480, 33.12390960531435979 ) ) ;
#11854=CARTESIAN_POINT ( 'NONE',  ( -16.46253265017146816, -9.564922557961047289, 19.16775706135233293 ) ) ;
#11855=CARTESIAN_POINT ( 'NONE',  ( 8.314922557960818139, 14.29746914071049879, 84.58224293864769550 ) ) ;
#11856=CARTESIAN_POINT ( 'NONE',  ( -19.02544592524342804, 5.153800228976336051, 91.04057627198100988 ) ) ;
#11857=VERTEX_POINT ( 'NONE', #95134 ) ;
#11858=CARTESIAN_POINT ( 'NONE',  ( -14.34966873604972548, 8.224510206698743886, 43.33442372801901143 ) ) ;
#11859=CARTESIAN_POINT ( 'NONE',  ( -19.05341960407611168, -5.049401038298163336, 36.45724293864766707 ) ) ;
#11860=CARTESIAN_POINT ( 'NONE',  ( -12.06949235617739369, -12.14591786802326823, 49.37609039468569705 ) ) ;
#11862=CARTESIAN_POINT ( 'NONE',  ( -19.02544592524334988, -5.153800228976617603, 48.95942372801900433 ) ) ;
#11863=CARTESIAN_POINT ( 'NONE',  ( -5.049401038298153566, 19.05341960407611168, 40.20724293864768839 ) ) ;
#11864=CARTESIAN_POINT ( 'NONE',  ( 4.483927247898790824, -16.52544592524335698, 80.20942372801901854 ) ) ;
#11865=CARTESIAN_POINT ( 'NONE',  ( 19.02544592524334988, 5.153800228976608722, 101.4594237280189759 ) ) ;
#11866=CARTESIAN_POINT ( 'NONE',  ( -0.05219959533936034679, 19.03943276465977164, 27.50109039468566507 ) ) ;
#11867=CARTESIAN_POINT ( 'NONE',  ( -9.474510206698964154, 16.51473224551069663, 60.41557627198102409 ) ) ;
#11868=CARTESIAN_POINT ( 'NONE',  ( 0.05219959533910956823, 16.53943276465976808, 94.99890960531436690 ) ) ;
#11870=CARTESIAN_POINT ( 'NONE',  ( 5.153800228976615827, -19.02544592524334988, 70.20942372801899012 ) ) ;
#11871=CARTESIAN_POINT ( 'NONE',  ( -18.62759615963270932, 10.81492255796079327, 65.83224293864769550 ) ) ;
#11872=CARTESIAN_POINT ( 'NONE',  ( 5.153800228976615827, -19.02544592524334988, 35.20942372801899722 ) ) ;
#11873=CARTESIAN_POINT ( 'NONE',  ( -19.03943276465977164, 0.05219959533909376836, 101.2489096053143669 ) ) ;
#11874=EDGE_CURVE ( 'NONE', #11672, #142306, #113785, .T. ) ;
#11875=CARTESIAN_POINT ( 'NONE',  ( 10.72451020669898902, -18.67979575497178502, 92.91557627198103830 ) ) ;
#11877=CARTESIAN_POINT ( 'NONE',  ( 5.153800228976615827, -19.02544592524334988, 105.2094237280190185 ) ) ;
#11879=CARTESIAN_POINT ( 'NONE',  ( -16.52544592524335698, -4.483927247898792601, 23.95942372801901143 ) ) ;
#11880=CARTESIAN_POINT ( 'NONE',  ( 9.474510206698971260, -16.51473224551069308, 52.91557627198102409 ) ) ;
#11881=CARTESIAN_POINT ( 'NONE',  ( -9.564922557960796823, -16.46253265017161027, 112.0822429386476955 ) ) ;
#11882=CARTESIAN_POINT ( 'NONE',  ( -21.55341960407610458, -5.719274019375992779, 96.45724293864770971 ) ) ;
#11883=CARTESIAN_POINT ( 'NONE',  ( 21.52544592524334988, 5.823673210054432836, 56.45942372801902565 ) ) ;
#11884=CARTESIAN_POINT ( 'NONE',  ( -19.05341960407617563, 5.049401038297882671, 108.5427570613523187 ) ) ;
#11885=CARTESIAN_POINT ( 'NONE',  ( -5.719274019375665041, -21.55341960407619695, 104.7927570613523898 ) ) ;
#11886=CARTESIAN_POINT ( 'NONE',  ( 4.483927247898790824, -16.52544592524335698, 110.2094237280190185 ) ) ;
#11887=CARTESIAN_POINT ( 'NONE',  ( -15.80617190586745835, -15.72974639402198527, 101.8739096053143811 ) ) ;
#11888=CARTESIAN_POINT ( 'NONE',  ( 16.53943276465976808, -0.05219959533910856209, 53.74890960531437401 ) ) ;
#11889=CARTESIAN_POINT ( 'NONE',  ( 9.564922557961047289, -16.46253265017146816, 80.41775706135234714 ) ) ;
#11890=CARTESIAN_POINT ( 'NONE',  ( -9.474510206698720793, -16.51473224551083518, 59.58442372801900433 ) ) ;
#11891=CARTESIAN_POINT ( 'NONE',  ( 5.823673210054444382, -21.52544592524334988, 75.20942372801901854 ) ) ;
#11892=CARTESIAN_POINT ( 'NONE',  ( -5.049401038297874678, -19.05341960407617918, 34.79275706135233293 ) ) ;
#11893=CARTESIAN_POINT ( 'NONE',  ( -13.97604488694527625, -13.89961937509977652, 26.87390960531434558 ) ) ;
#11894=CARTESIAN_POINT ( 'NONE',  ( -21.55341960407610458, -5.719274019375992779, 41.45724293864769550 ) ) ;
#11895=CARTESIAN_POINT ( 'NONE',  ( 14.34966873604960469, 8.224510206698951720, 39.16557627198102409 ) ) ;
#11896=CARTESIAN_POINT ( 'NONE',  ( -21.53943276465977519, -0.05219959533937600094, 108.7510903946857042 ) ) ;
#11897=CARTESIAN_POINT ( 'NONE',  ( -4.379528057220086978, -16.55341960407618274, 74.79275706135234714 ) ) ;
#11898=CARTESIAN_POINT ( 'NONE',  ( -14.29746914071049879, 8.314922557960819915, 45.83224293864769550 ) ) ;
#11899=CARTESIAN_POINT ( 'NONE',  ( 15.80617190586769283, -15.72974639402175789, 65.62609039468568994 ) ) ;
#11900=CARTESIAN_POINT ( 'NONE',  ( 15.80617190586769283, -15.72974639402175789, 70.62609039468567573 ) ) ;
#11901=CARTESIAN_POINT ( 'NONE',  ( -10.72451020669898014, 18.67979575497178502, 70.41557627198102409 ) ) ;
#11902=CARTESIAN_POINT ( 'NONE',  ( -19.03943276465977164, 0.05219959533909376836, 26.24890960531435624 ) ) ;
#11903=CARTESIAN_POINT ( 'NONE',  ( 15.72974639402176855, 15.80617190586768217, 36.87609039468568994 ) ) ;
#11904=CARTESIAN_POINT ( 'NONE',  ( 4.379528057220339221, -16.55341960407611168, 112.7072429386476955 ) ) ;
#11905=CARTESIAN_POINT ( 'NONE',  ( -0.05219959533909027116, -19.03943276465977164, 32.49890960531435979 ) ) ;
#11906=CARTESIAN_POINT ( 'NONE',  ( -14.34966873604960291, -8.224510206698953496, 91.66557627198103830 ) ) ;
#11907=CARTESIAN_POINT ( 'NONE',  ( 16.51473224551069308, 9.474510206698969483, 89.16557627198103830 ) ) ;
#11908=CARTESIAN_POINT ( 'NONE',  ( -4.379528057220328563, 16.55341960407611168, 30.20724293864769550 ) ) ;
#11909=CARTESIAN_POINT ( 'NONE',  ( -4.379528057220328563, 16.55341960407611168, 105.2072429386477097 ) ) ;
#11910=CARTESIAN_POINT ( 'NONE',  ( -18.67979575497178146, -10.72451020669898902, 71.66557627198100988 ) ) ;
#11912=CARTESIAN_POINT ( 'NONE',  ( 5.719274019375991003, -21.55341960407610458, 102.7072429386476955 ) ) ;
#11913=CARTESIAN_POINT ( 'NONE',  ( 19.05341960407611168, 5.049401038298154454, 108.9572429386477097 ) ) ;
#11914=CARTESIAN_POINT ( 'NONE',  ( 19.03943276465977164, -0.05219959533909143690, 58.74890960531435979 ) ) ;
#11915=CARTESIAN_POINT ( 'NONE',  ( -8.224510206698735004, -14.34966873604973081, 24.58442372801901499 ) ) ;
#11916=CARTESIAN_POINT ( 'NONE',  ( -18.62759615963270932, 10.81492255796079327, 60.83224293864769550 ) ) ;
#11917=CARTESIAN_POINT ( 'NONE',  ( -5.719274019375665041, -21.55341960407619695, 84.79275706135234714 ) ) ;
#11918=CARTESIAN_POINT ( 'NONE',  ( -5.049401038298153566, 19.05341960407611168, 80.20724293864769550 ) ) ;
#11919=CARTESIAN_POINT ( 'NONE',  ( 5.719274019375991003, -21.55341960407610458, 22.70724293864769194 ) ) ;
#11920=CARTESIAN_POINT ( 'NONE',  ( -16.55341960407617563, 4.379528057220093196, 73.54275706135234714 ) ) ;
#11921=CARTESIAN_POINT ( 'NONE',  ( -21.55341960407619339, 5.719274019375674811, 73.54275706135234714 ) ) ;
#11922=CARTESIAN_POINT ( 'NONE',  ( -0.05219959533937732626, 21.53943276465977519, 97.50109039468567573 ) ) ;
#11923=CARTESIAN_POINT ( 'NONE',  ( 16.53943276465976808, 0.05219959533934440121, 66.25109039468567573 ) ) ;
#11924=CARTESIAN_POINT ( 'NONE',  ( 15.80617190586746368, 15.72974639402197994, 109.3739096053143811 ) ) ;
#11925=CARTESIAN_POINT ( 'NONE',  ( -16.51473224551069308, -9.474510206698971260, 21.66557627198102765 ) ) ;
#11926=CARTESIAN_POINT ( 'NONE',  ( -5.719274019375978568, 21.55341960407610458, 95.20724293864769550 ) ) ;
#11927=CARTESIAN_POINT ( 'NONE',  ( -19.03943276465977164, -0.05219959533935918106, 43.75109039468566863 ) ) ;
#11928=CARTESIAN_POINT ( 'NONE',  ( -0.05219959533907301413, -21.53943276465977519, 57.49890960531435979 ) ) ;
#11929=CARTESIAN_POINT ( 'NONE',  ( -19.02544592524342804, 5.153800228976336051, 91.04057627198100988 ) ) ;
#11930=CARTESIAN_POINT ( 'NONE',  ( 4.379528057220339221, -16.55341960407611168, 42.70724293864770260 ) ) ;
#11933=CARTESIAN_POINT ( 'NONE',  ( -18.22780087662122028, 5.500000000000031086, 73.51540105326107266 ) ) ;
#11934=CARTESIAN_POINT ( 'NONE',  ( 13.89961937509957401, 13.97604488694547697, 111.8760903946856757 ) ) ;
#11935=CARTESIAN_POINT ( 'NONE',  ( 5.823673210054125526, 21.52544592524343514, 89.79057627198103830 ) ) ;
#11936=CARTESIAN_POINT ( 'NONE',  ( -16.55341960407611168, -4.379528057220339221, 46.45724293864769550 ) ) ;
#11937=CARTESIAN_POINT ( 'NONE',  ( 12.14591786802327356, -12.06949235617739191, 30.62609039468567929 ) ) ;
#11938=CARTESIAN_POINT ( 'NONE',  ( -5.049401038298153566, 19.05341960407611168, 50.20724293864770260 ) ) ;
#11939=CARTESIAN_POINT ( 'NONE',  ( -10.81492255796078084, -18.62759615963271287, 112.0822429386477097 ) ) ;
#11940=CARTESIAN_POINT ( 'NONE',  ( -19.03943276465977164, -0.05219959533935918106, 83.75109039468567573 ) ) ;
#11941=CARTESIAN_POINT ( 'NONE',  ( 5.049401038298161559, -19.05341960407611168, 87.70724293864769550 ) ) ;
#11942=CARTESIAN_POINT ( 'NONE',  ( -16.51473224551069308, -9.474510206698971260, 71.66557627198102409 ) ) ;
#11943=CARTESIAN_POINT ( 'NONE',  ( -5.719274019375978568, 21.55341960407610458, 75.20724293864769550 ) ) ;
#11944=CARTESIAN_POINT ( 'NONE',  ( 5.153800228976335163, 19.02544592524342804, 34.79057627198102409 ) ) ;
#11946=CARTESIAN_POINT ( 'NONE',  ( 8.314922557960818139, 14.29746914071049879, 59.58224293864770260 ) ) ;
#11947=CARTESIAN_POINT ( 'NONE',  ( -16.51473224551069308, -9.474510206698971260, 96.66557627198102409 ) ) ;
#11949=CARTESIAN_POINT ( 'NONE',  ( -19.05341960407617563, 5.049401038297882671, 63.54275706135234003 ) ) ;
#11950=CARTESIAN_POINT ( 'NONE',  ( -18.62759615963270932, 10.81492255796079327, 80.83224293864769550 ) ) ;
#11951=CARTESIAN_POINT ( 'NONE',  ( 13.97604488694548053, -13.89961937509957401, 30.62609039468566863 ) ) ;
#11952=CARTESIAN_POINT ( 'NONE',  ( 19.05341960407611168, 5.049401038298154454, 93.95724293864769550 ) ) ;
#11954=CARTESIAN_POINT ( 'NONE',  ( 18.62759615963271287, -10.81492255796078972, 28.33224293864769550 ) ) ;
#11955=CARTESIAN_POINT ( 'NONE',  ( 9.474510206698971260, -16.51473224551069308, 77.91557627198103830 ) ) ;
#11956=CARTESIAN_POINT ( 'NONE',  ( 15.72974639402176855, 15.80617190586768217, 56.87609039468568994 ) ) ;
#11957=CARTESIAN_POINT ( 'NONE',  ( 5.153800228976335163, 19.02544592524342804, 24.79057627198102765 ) ) ;
#11958=CARTESIAN_POINT ( 'NONE',  ( 21.53943276465977519, 0.05219959533937863772, 21.25109039468567218 ) ) ;
#11959=ORIENTED_EDGE ( 'NONE', *, *, #131511, .F. ) ;
#11960=CARTESIAN_POINT ( 'NONE',  ( -5.719274019375665041, -21.55341960407619695, 44.79275706135234714 ) ) ;
#11962=CARTESIAN_POINT ( 'NONE',  ( -9.474510206698964154, 16.51473224551069663, 95.41557627198102409 ) ) ;
#11964=CARTESIAN_POINT ( 'NONE',  ( 21.52544592524344225, -5.823673210054117533, 108.5405762719810241 ) ) ;
#11965=CARTESIAN_POINT ( 'NONE',  ( 19.02544592524343514, -5.153800228976328945, 63.54057627198103830 ) ) ;
#11966=CARTESIAN_POINT ( 'NONE',  ( -4.379528057220086978, -16.55341960407618274, 19.79275706135235069 ) ) ;
#11968=CARTESIAN_POINT ( 'NONE',  ( -5.823673210054431948, 21.52544592524334988, 107.7094237280190328 ) ) ;
#11969=CARTESIAN_POINT ( 'NONE',  ( -9.474510206698964154, 16.51473224551069663, 40.41557627198103120 ) ) ;
#11970=CARTESIAN_POINT ( 'NONE',  ( -10.81492255796105439, 18.62759615963255655, 97.91775706135236135 ) ) ;
#11971=CARTESIAN_POINT ( 'NONE',  ( 19.05341960407611168, 5.049401038298154454, 83.95724293864766707 ) ) ;
#11972=CARTESIAN_POINT ( 'NONE',  ( -10.81492255796105439, 18.62759615963255655, 57.91775706135234714 ) ) ;
#11974=CARTESIAN_POINT ( 'NONE',  ( -9.564922557960796823, -16.46253265017161027, 107.0822429386476955 ) ) ;
#11976=CARTESIAN_POINT ( 'NONE',  ( 4.379528057220092307, 16.55341960407617563, 57.29275706135234714 ) ) ;
#11977=CARTESIAN_POINT ( 'NONE',  ( -14.29746914071037622, -8.314922557961029526, 64.16775706135234714 ) ) ;
#11978=CARTESIAN_POINT ( 'NONE',  ( -5.719274019375665041, -21.55341960407619695, 64.79275706135234714 ) ) ;
#11979=CARTESIAN_POINT ( 'NONE',  ( -21.55341960407619339, 5.719274019375674811, 93.54275706135234714 ) ) ;
#11981=CARTESIAN_POINT ( 'NONE',  ( 14.34966873604972726, -8.224510206698740333, 25.83442372801901499 ) ) ;
#11982=CARTESIAN_POINT ( 'NONE',  ( 19.05341960407611168, 5.049401038298154454, 68.95724293864769550 ) ) ;
#11983=CARTESIAN_POINT ( 'NONE',  ( 13.97604488694527802, 13.89961937509977652, 114.3739096053143669 ) ) ;
#11984=CARTESIAN_POINT ( 'NONE',  ( -15.49999999999999822, -5.500000000000000888, 22.00000000000000000 ) ) ;
#11985=B_SPLINE_CURVE_WITH_KNOTS ( 'NONE', 3,
 ( #86516, #72358, #26868, #133022, #121824, #134032, #10695, #195725, #181540, #136021, #194712, #59161, #165374, #167358, #25872, #44011, #11704, #198688, #24867, #60155, #152178, #197695, #13662, #88511, #73371, #183518, #120829, #56181, #182529, #117864, #179555, #119856 ),
 .UNSPECIFIED., .F., .F.,
 ( 4, 2, 2, 2, 2, 2, 2, 2, 2, 2, 2, 2, 2, 2, 2, 4 ),
 ( 2.539163526713095107E-17, 0.0003712461730037033662, 0.0007424923460073813621, 0.001113738519011059358, 0.001484984692014737354, 0.002227477038022093563, 0.002598723211025767872, 0.002969969384029442182, 0.003341215557033117359, 0.003712461730036790801, 0.004083707903040465111, 0.004454954076044138553, 0.004826200249047812862, 0.005197446422051487172, 0.005568692595055160614, 0.005939938768058834924 ),
 .UNSPECIFIED. ) ;
#11986=CARTESIAN_POINT ( 'NONE',  ( -9.474510206698964154, 16.51473224551069663, 30.41557627198102054 ) ) ;
#11987=CARTESIAN_POINT ( 'NONE',  ( 15.80617190586746368, 15.72974639402197994, 49.37390960531436690 ) ) ;
#11989=CARTESIAN_POINT ( 'NONE',  ( -8.224510206698735004, -14.34966873604973081, 89.58442372801901854 ) ) ;
#11990=CARTESIAN_POINT ( 'NONE',  ( -4.483927247898539470, -16.52544592524342804, 87.29057627198103830 ) ) ;
#11991=CARTESIAN_POINT ( 'NONE',  ( -19.05341960407611168, -5.049401038298163336, 61.45724293864769550 ) ) ;
#11992=CARTESIAN_POINT ( 'NONE',  ( 21.55341960407619695, -5.719274019375665929, 86.04275706135236135 ) ) ;
#11994=CARTESIAN_POINT ( 'NONE',  ( -4.483927247898782831, 16.52544592524335698, 22.70942372801901499 ) ) ;
#11995=CARTESIAN_POINT ( 'NONE',  ( 8.224510206698953496, -14.34966873604960469, 72.91557627198103830 ) ) ;
#11996=CARTESIAN_POINT ( 'NONE',  ( 18.67979575497194134, -10.72451020669871369, 35.83442372801901143 ) ) ;
#11997=CARTESIAN_POINT ( 'NONE',  ( -21.52544592524343514, 5.823673210054127303, 71.04057627198103830 ) ) ;
#11998=CARTESIAN_POINT ( 'NONE',  ( -9.564922557961040184, 16.46253265017147172, 32.91775706135233293 ) ) ;
#11999=CARTESIAN_POINT ( 'NONE',  ( 0.05219959533909260263, 19.03943276465977164, 44.99890960531435979 ) ) ;
#12000=CARTESIAN_POINT ( 'NONE',  ( -13.97604488694527625, -13.89961937509977652, 76.87390960531433848 ) ) ;
#12001=CARTESIAN_POINT ( 'NONE',  ( -0.05219959533910754901, -16.53943276465976808, 47.49890960531435979 ) ) ;
#12002=EDGE_CURVE ( 'NONE', #189322, #192521, #104153, .T. ) ;
#12004=CARTESIAN_POINT ( 'NONE',  ( -16.55341960407611168, -4.379528057220339221, 31.45724293864769550 ) ) ;
#12005=CARTESIAN_POINT ( 'NONE',  ( -16.55341960407617563, 4.379528057220093196, 108.5427570613523756 ) ) ;
#12006=CARTESIAN_POINT ( 'NONE',  ( -13.97604488694547697, 13.89961937509957934, 63.12609039468566152 ) ) ;
#12007=CARTESIAN_POINT ( 'NONE',  ( 16.81555441253550143, 7.025013491695497159, 46.86314554665745646 ) ) ;
#12008=CARTESIAN_POINT ( 'NONE',  ( 21.52544592524344225, -5.823673210054117533, 23.54057627198102765 ) ) ;
#12009=CARTESIAN_POINT ( 'NONE',  ( 16.52544592524342804, -4.483927247898539470, 88.54057627198103830 ) ) ;
#12011=CARTESIAN_POINT ( 'NONE',  ( 9.564922557960805705, 16.46253265017160317, 39.58224293864768839 ) ) ;
#12012=CARTESIAN_POINT ( 'NONE',  ( -18.67979575497178146, -10.72451020669898902, 31.66557627198102054 ) ) ;
#12013=CARTESIAN_POINT ( 'NONE',  ( 18.62759615963271287, -10.81492255796078972, 68.33224293864769550 ) ) ;
#12014=CARTESIAN_POINT ( 'NONE',  ( 16.55341960407611168, 4.379528057220329451, 113.9572429386477239 ) ) ;
#12015=CARTESIAN_POINT ( 'NONE',  ( -12.14591786802326823, 12.06949235617739902, 68.12609039468567573 ) ) ;
#12016=CARTESIAN_POINT ( 'NONE',  ( 13.89961937509977652, -13.97604488694527269, 53.12390960531434558 ) ) ;
#12017=CARTESIAN_POINT ( 'NONE',  ( -10.72451020669870658, -18.67979575497194134, 54.58442372801901143 ) ) ;
#12019=CARTESIAN_POINT ( 'NONE',  ( 14.29746914071049879, -8.314922557960816363, 103.3322429386476955 ) ) ;
#12020=CARTESIAN_POINT ( 'NONE',  ( -9.474510206698720793, -16.51473224551083518, 94.58442372801900433 ) ) ;
#12022=CARTESIAN_POINT ( 'NONE',  ( -18.10062525802553779, 5.500000000000031974, 38.51383468041921532 ) ) ;
#12023=CARTESIAN_POINT ( 'NONE',  ( 18.67979575497178502, 10.72451020669898547, 34.16557627198102409 ) ) ;
#12025=CARTESIAN_POINT ( 'NONE',  ( 21.55341960407619695, -5.719274019375665929, 71.04275706135234714 ) ) ;
#12026=CARTESIAN_POINT ( 'NONE',  ( 8.314922557961029526, -14.29746914071037800, 50.41775706135235424 ) ) ;
#12027=CARTESIAN_POINT ( 'NONE',  ( -14.34966873604960291, -8.224510206698953496, 46.66557627198102409 ) ) ;
#12028=CARTESIAN_POINT ( 'NONE',  ( -21.53943276465977519, 0.05219959533907696930, 66.24890960531436690 ) ) ;
#12029=CARTESIAN_POINT ( 'NONE',  ( -0.05219959533907301413, -21.53943276465977519, 62.49890960531436690 ) ) ;
#12031=CARTESIAN_POINT ( 'NONE',  ( 5.049401038297881783, 19.05341960407617563, 87.29275706135234714 ) ) ;
#12032=CARTESIAN_POINT ( 'NONE',  ( -21.53943276465977519, 0.05219959533907696930, 21.24890960531436690 ) ) ;
#12033=CARTESIAN_POINT ( 'NONE',  ( -13.97604488694527625, -13.89961937509977652, 51.87390960531436690 ) ) ;
#12034=CARTESIAN_POINT ( 'NONE',  ( 8.224510206698953496, -14.34966873604960469, 112.9155762719810383 ) ) ;
#12037=CARTESIAN_POINT ( 'NONE',  ( -16.53943276465976808, -0.05219959533934237506, 73.75109039468567573 ) ) ;
#12038=CARTESIAN_POINT ( 'NONE',  ( 21.55341960407610458, 5.719274019375980345, 108.9572429386476955 ) ) ;
#12039=CARTESIAN_POINT ( 'NONE',  ( 0.05219959533909260263, 19.03943276465977164, 69.99890960531435269 ) ) ;
#12040=CARTESIAN_POINT ( 'NONE',  ( 0.05219959533937995610, -21.53943276465977519, 45.00109039468568284 ) ) ;
#12041=CARTESIAN_POINT ( 'NONE',  ( -9.474510206698964154, 16.51473224551069663, 95.41557627198102409 ) ) ;
#12044=CARTESIAN_POINT ( 'NONE',  ( -21.55341960407619339, 5.719274019375674811, 38.54275706135234714 ) ) ;
#12045=CARTESIAN_POINT ( 'NONE',  ( -13.97604488694527625, -13.89961937509977652, 26.87390960531434558 ) ) ;
#12046=CARTESIAN_POINT ( 'NONE',  ( 9.474510206698729675, 16.51473224551082808, 87.08442372801900433 ) ) ;
#12047=CARTESIAN_POINT ( 'NONE',  ( 13.89961937509957401, 13.97604488694547697, 41.87609039468566152 ) ) ;
#12048=CARTESIAN_POINT ( 'NONE',  ( 15.72974639402199770, -15.80617190586745480, 113.1239096053143953 ) ) ;
#12049=CARTESIAN_POINT ( 'NONE',  ( -19.03943276465977164, -0.05219959533935918106, 33.75109039468566863 ) ) ;
#12050=CARTESIAN_POINT ( 'NONE',  ( 16.46253265017146816, 9.564922557961045513, 46.66775706135233293 ) ) ;
#12051=CARTESIAN_POINT ( 'NONE',  ( 12.14591786802327356, -12.06949235617739191, 90.62609039468567573 ) ) ;
#12052=CARTESIAN_POINT ( 'NONE',  ( -19.02544592524342804, 5.153800228976336051, 116.0405762719810383 ) ) ;
#12054=CARTESIAN_POINT ( 'NONE',  ( 19.03943276465977164, -0.05219959533909143690, 68.74890960531436690 ) ) ;
#12056=CARTESIAN_POINT ( 'NONE',  ( -18.67979575497193778, 10.72451020669871902, 83.33442372801903275 ) ) ;
#12057=CARTESIAN_POINT ( 'NONE',  ( 5.823673210054444382, -21.52544592524334988, 95.20942372801903275 ) ) ;
#12059=CARTESIAN_POINT ( 'NONE',  ( 0.05219959533909260263, 19.03943276465977164, 89.99890960531436690 ) ) ;
#12060=CARTESIAN_POINT ( 'NONE',  ( 10.81492255796106328, -18.62759615963255655, 65.41775706135234714 ) ) ;
#12061=CARTESIAN_POINT ( 'NONE',  ( -9.474510206698720793, -16.51473224551083518, 99.58442372801900433 ) ) ;
#12062=CARTESIAN_POINT ( 'NONE',  ( -5.049401038298153566, 19.05341960407611168, 65.20724293864765286 ) ) ;
#12063=CARTESIAN_POINT ( 'NONE',  ( -19.02544592524342804, 5.153800228976336051, 111.0405762719810099 ) ) ;
#12064=CARTESIAN_POINT ( 'NONE',  ( -9.474510206698964154, 16.51473224551069663, 85.41557627198102409 ) ) ;
#12065=CARTESIAN_POINT ( 'NONE',  ( 17.49999999999997513, -3.267433481402603146, 22.16880360417568241 ) ) ;
#12066=CARTESIAN_POINT ( 'NONE',  ( -13.89961937509977652, 13.97604488694528158, 65.62390960531436690 ) ) ;
#12067=CARTESIAN_POINT ( 'NONE',  ( -19.05341960407611168, -5.049401038298163336, 46.45724293864768129 ) ) ;
#12068=CARTESIAN_POINT ( 'NONE',  ( -5.719274019375978568, 21.55341960407610458, 115.2072429386476955 ) ) ;
#12069=CARTESIAN_POINT ( 'NONE',  ( -4.379528057220086978, -16.55341960407618274, 84.79275706135234714 ) ) ;
#12071=CARTESIAN_POINT ( 'NONE',  ( 19.05341960407617918, -5.049401038297876454, 61.04275706135232582 ) ) ;
#12072=CARTESIAN_POINT ( 'NONE',  ( -5.049401038298153566, 19.05341960407611168, 80.20724293864769550 ) ) ;
#12073=CARTESIAN_POINT ( 'NONE',  ( -4.379528057220328563, 16.55341960407611168, 75.20724293864769550 ) ) ;
#12074=CARTESIAN_POINT ( 'NONE',  ( -12.06949235617756955, 12.14591786802309770, 110.6239096053143669 ) ) ;
#12075=CARTESIAN_POINT ( 'NONE',  ( -0.05219959533909027116, -19.03943276465977164, 112.4989096053143669 ) ) ;
#12076=CARTESIAN_POINT ( 'NONE',  ( -13.97604488694527625, -13.89961937509977652, 106.8739096053143669 ) ) ;
#12077=CARTESIAN_POINT ( 'NONE',  ( -4.379528057220328563, 16.55341960407611168, 80.20724293864769550 ) ) ;
#12079=CARTESIAN_POINT ( 'NONE',  ( 9.474510206698729675, 16.51473224551082808, 37.08442372801899722 ) ) ;
#12080=CARTESIAN_POINT ( 'NONE',  ( -14.34966873604972548, 8.224510206698743886, 103.3344237280190043 ) ) ;
#12081=CARTESIAN_POINT ( 'NONE',  ( 19.05341960407611168, 5.049401038298154454, 83.95724293864766707 ) ) ;
#12082=CARTESIAN_POINT ( 'NONE',  ( -18.67979575497193778, 10.72451020669871902, 53.33442372801901854 ) ) ;
#12083=CARTESIAN_POINT ( 'NONE',  ( -18.62759615963270932, 10.81492255796079327, 50.83224293864770971 ) ) ;
#12084=CARTESIAN_POINT ( 'NONE',  ( 10.72451020669898902, -18.67979575497178502, 112.9155762719810383 ) ) ;
#12085=CARTESIAN_POINT ( 'NONE',  ( 21.53943276465977519, -0.05219959533907433946, 63.74890960531435979 ) ) ;
#12086=CARTESIAN_POINT ( 'NONE',  ( -8.314922557960811034, -14.29746914071050412, 92.08224293864769550 ) ) ;
#12087=CARTESIAN_POINT ( 'NONE',  ( 19.05341960407617918, -5.049401038297876454, 51.04275706135231871 ) ) ;
#12088=CARTESIAN_POINT ( 'NONE',  ( -16.46253265017160317, 9.564922557960807481, 25.83224293864769194 ) ) ;
#12089=CARTESIAN_POINT ( 'NONE',  ( -16.46253265017160317, 9.564922557960807481, 80.83224293864769550 ) ) ;
#12090=CARTESIAN_POINT ( 'NONE',  ( 16.46253265017160672, -9.564922557960803928, 78.33224293864769550 ) ) ;
#12091=CARTESIAN_POINT ( 'NONE',  ( -8.314922557960811034, -14.29746914071050412, 102.0822429386476955 ) ) ;
#12092=VERTEX_POINT ( 'NONE', #101105 ) ;
#12093=CARTESIAN_POINT ( 'NONE',  ( -16.53943276465976808, 0.05219959533911058130, 26.24890960531435624 ) ) ;
#12094=CARTESIAN_POINT ( 'NONE',  ( -16.53943276465976808, -0.05219959533934237506, 38.75109039468567573 ) ) ;
#12095=CARTESIAN_POINT ( 'NONE',  ( 18.67979575497194134, -10.72451020669871369, 105.8344237280190328 ) ) ;
#12096=CARTESIAN_POINT ( 'NONE',  ( -19.03943276465977164, 0.05219959533909376836, 96.24890960531436690 ) ) ;
#12097=CARTESIAN_POINT ( 'NONE',  ( -21.53943276465977519, -0.05219959533937600094, 38.75109039468567573 ) ) ;
#12098=CARTESIAN_POINT ( 'NONE',  ( 16.46253265017160672, -9.564922557960803928, 38.33224293864768839 ) ) ;
#12099=CARTESIAN_POINT ( 'NONE',  ( 4.483927247898790824, -16.52544592524335698, 40.20942372801901854 ) ) ;
#12100=CARTESIAN_POINT ( 'NONE',  ( 13.97604488694548053, -13.89961937509957401, 105.6260903946856757 ) ) ;
#12101=CARTESIAN_POINT ( 'NONE',  ( 16.46253265017160672, -9.564922557960803928, 38.33224293864768839 ) ) ;
#12102=CARTESIAN_POINT ( 'NONE',  ( -14.34966873604960291, -8.224510206698953496, 91.66557627198103830 ) ) ;
#12103=CARTESIAN_POINT ( 'NONE',  ( 18.67979575497178502, 10.72451020669898547, 109.1655762719810383 ) ) ;
#12104=CARTESIAN_POINT ( 'NONE',  ( -5.153800228976607833, 19.02544592524334988, 87.70942372801897591 ) ) ;
#12105=CARTESIAN_POINT ( 'NONE',  ( 13.89961937509977652, -13.97604488694527269, 28.12390960531435624 ) ) ;
#12106=CARTESIAN_POINT ( 'NONE',  ( 19.02544592524343514, -5.153800228976328945, 93.54057627198102409 ) ) ;
#12107=CARTESIAN_POINT ( 'NONE',  ( 15.72974639402176855, 15.80617190586768217, 36.87609039468568994 ) ) ;
#12109=CARTESIAN_POINT ( 'NONE',  ( 9.474510206698971260, -16.51473224551069308, 97.91557627198102409 ) ) ;
#12110=CARTESIAN_POINT ( 'NONE',  ( 16.36317988757056696, -7.306389748694960495, 111.5978960836323068 ) ) ;
#12111=CARTESIAN_POINT ( 'NONE',  ( 13.89961937509977652, -13.97604488694527269, 88.12390960531438111 ) ) ;
#12112=CARTESIAN_POINT ( 'NONE',  ( -0.05219959533937732626, 21.53943276465977519, 32.50109039468568284 ) ) ;
#12113=CARTESIAN_POINT ( 'NONE',  ( -16.52544592524342804, 4.483927247898546575, 91.04057627198103830 ) ) ;
#12114=CARTESIAN_POINT ( 'NONE',  ( 5.153800228976335163, 19.02544592524342804, 99.79057627198102409 ) ) ;
#12115=CARTESIAN_POINT ( 'NONE',  ( -21.53943276465977519, -0.05219959533937600094, 113.7510903946856757 ) ) ;
#12116=CARTESIAN_POINT ( 'NONE',  ( -0.05219959533934338120, 16.53943276465976808, 52.50109039468567573 ) ) ;
#12117=CARTESIAN_POINT ( 'NONE',  ( 15.72974639402176855, 15.80617190586768217, 76.87609039468567573 ) ) ;
#12118=CARTESIAN_POINT ( 'NONE',  ( 12.06949235617739724, 12.14591786802326823, 31.87609039468567929 ) ) ;
#12119=CARTESIAN_POINT ( 'NONE',  ( 13.89961937509977652, -13.97604488694527269, 73.12390960531436690 ) ) ;
#12120=CARTESIAN_POINT ( 'NONE',  ( -19.05341960407617563, 5.049401038297882671, 93.54275706135234714 ) ) ;
#12121=CARTESIAN_POINT ( 'NONE',  ( -12.06949235617739369, -12.14591786802326823, 69.37609039468567573 ) ) ;
#12122=CARTESIAN_POINT ( 'NONE',  ( -19.03943276465977164, -0.05219959533935918106, 18.75109039468567218 ) ) ;
#12123=CARTESIAN_POINT ( 'NONE',  ( 13.89961937509957401, 13.97604488694547697, 81.87609039468564731 ) ) ;
#12124=CARTESIAN_POINT ( 'NONE',  ( -16.46253265017160317, 9.564922557960807481, 60.83224293864769550 ) ) ;
#12125=CARTESIAN_POINT ( 'NONE',  ( 18.62759615963271287, -10.81492255796078972, 88.33224293864769550 ) ) ;
#12126=CARTESIAN_POINT ( 'NONE',  ( -14.34966873604960291, -8.224510206698953496, 76.66557627198103830 ) ) ;
#12127=CARTESIAN_POINT ( 'NONE',  ( 9.474510206698729675, 16.51473224551082808, 77.08442372801900433 ) ) ;
#12128=CARTESIAN_POINT ( 'NONE',  ( -18.56197773271725993, 5.500000000000081712, 78.55066217314451649 ) ) ;
#12129=CARTESIAN_POINT ( 'NONE',  ( -13.97604488694547697, 13.89961937509957934, 58.12609039468566863 ) ) ;
#12130=CARTESIAN_POINT ( 'NONE',  ( 4.379528057220339221, -16.55341960407611168, 22.70724293864769194 ) ) ;
#12131=CARTESIAN_POINT ( 'NONE',  ( -16.55341960407611168, -4.379528057220339221, 81.45724293864769550 ) ) ;
#12132=CARTESIAN_POINT ( 'NONE',  ( -5.049401038297874678, -19.05341960407617918, 19.79275706135233293 ) ) ;
#12134=CARTESIAN_POINT ( 'NONE',  ( -10.81492255796078084, -18.62759615963271287, 112.0822429386477097 ) ) ;
#12135=CARTESIAN_POINT ( 'NONE',  ( 16.51473224551069308, 9.474510206698969483, 104.1655762719810241 ) ) ;
#12136=CARTESIAN_POINT ( 'NONE',  ( 13.89961937509977652, -13.97604488694527269, 73.12390960531436690 ) ) ;
#12137=CARTESIAN_POINT ( 'NONE',  ( 5.823673210054444382, -21.52544592524334988, 80.20942372801901854 ) ) ;
#12138=CARTESIAN_POINT ( 'NONE',  ( -0.05219959533909027116, -19.03943276465977164, 57.49890960531435979 ) ) ;
#12140=CARTESIAN_POINT ( 'NONE',  ( -16.51473224551069308, -9.474510206698971260, 36.66557627198102409 ) ) ;
#12141=CARTESIAN_POINT ( 'NONE',  ( 5.719274019375991003, -21.55341960407610458, 27.70724293864769905 ) ) ;
#12142=CARTESIAN_POINT ( 'NONE',  ( -12.14591786802309592, -12.06949235617757132, 81.87390960531435269 ) ) ;
#12143=CARTESIAN_POINT ( 'NONE',  ( -16.46253265017160317, 9.564922557960807481, 45.83224293864769550 ) ) ;
#12144=CARTESIAN_POINT ( 'NONE',  ( -16.52544592524342804, 4.483927247898546575, 96.04057627198102409 ) ) ;
#12146=CARTESIAN_POINT ( 'NONE',  ( -15.80617190586745835, -15.72974639402198527, 106.8739096053143811 ) ) ;
#12147=CARTESIAN_POINT ( 'NONE',  ( 0.05219959533937995610, -21.53943276465977519, 45.00109039468568284 ) ) ;
#12148=CARTESIAN_POINT ( 'NONE',  ( -9.564922557960796823, -16.46253265017161027, 32.08224293864769550 ) ) ;
#12149=CARTESIAN_POINT ( 'NONE',  ( 16.52544592524335698, 4.483927247898782831, 66.45942372801903275 ) ) ;
#12150=CARTESIAN_POINT ( 'NONE',  ( -0.05219959533907301413, -21.53943276465977519, 97.49890960531436690 ) ) ;
#12151=CARTESIAN_POINT ( 'NONE',  ( 0.05219959533907565091, 21.53943276465977519, 99.99890960531436690 ) ) ;
#12152=CARTESIAN_POINT ( 'NONE',  ( -9.474510206698720793, -16.51473224551083518, 39.58442372801899722 ) ) ;
#12153=CARTESIAN_POINT ( 'NONE',  ( -16.51473224551069308, -9.474510206698971260, 46.66557627198102409 ) ) ;
#12154=CARTESIAN_POINT ( 'NONE',  ( -13.89961937509977652, 13.97604488694528158, 115.6239096053143669 ) ) ;
#12155=CARTESIAN_POINT ( 'NONE',  ( -10.81492255796105439, 18.62759615963255655, 57.91775706135234714 ) ) ;
#12156=CARTESIAN_POINT ( 'NONE',  ( -21.53943276465977519, 0.05219959533907696930, 61.24890960531435979 ) ) ;
#12157=CARTESIAN_POINT ( 'NONE',  ( 12.06949235617757843, -12.14591786802309237, 38.12390960531436690 ) ) ;
#12158=CARTESIAN_POINT ( 'NONE',  ( 5.823673210054444382, -21.52544592524334988, 75.20942372801901854 ) ) ;
#12159=CARTESIAN_POINT ( 'NONE',  ( 13.97604488694548053, -13.89961937509957401, 20.62609039468567573 ) ) ;
#12160=CARTESIAN_POINT ( 'NONE',  ( 16.51473224551083163, -9.474510206698727899, 40.83442372801900433 ) ) ;
#12161=CARTESIAN_POINT ( 'NONE',  ( 14.34966873604972726, -8.224510206698740333, 100.8344237280190185 ) ) ;
#12162=CARTESIAN_POINT ( 'NONE',  ( -21.53943276465977519, -0.05219959533937600094, 58.75109039468568994 ) ) ;
#12163=CARTESIAN_POINT ( 'NONE',  ( -16.46253265017160317, 9.564922557960807481, 65.83224293864769550 ) ) ;
#12164=CARTESIAN_POINT ( 'NONE',  ( -5.049401038297874678, -19.05341960407617918, 39.79275706135232582 ) ) ;
#12165=CARTESIAN_POINT ( 'NONE',  ( 21.55341960407610458, 5.719274019375980345, 43.95724293864769550 ) ) ;
#12166=CARTESIAN_POINT ( 'NONE',  ( -15.80617190586768217, 15.72974639402176855, 28.12609039468568284 ) ) ;
#12167=CARTESIAN_POINT ( 'NONE',  ( 5.719274019375991003, -21.55341960407610458, 87.70724293864769550 ) ) ;
#12168=CARTESIAN_POINT ( 'NONE',  ( 16.46253265017146816, 9.564922557961045513, 86.66775706135233293 ) ) ;
#12169=CARTESIAN_POINT ( 'NONE',  ( -16.55341960407617563, 4.379528057220093196, 58.54275706135235424 ) ) ;
#12170=CARTESIAN_POINT ( 'NONE',  ( 17.49999999999998934, -5.047551163040834510, 36.33463913479419460 ) ) ;
#12171=CARTESIAN_POINT ( 'NONE',  ( 0.05219959533907565091, 21.53943276465977519, 89.99890960531438111 ) ) ;
#12172=CARTESIAN_POINT ( 'NONE',  ( 16.55341960407618274, -4.379528057220086978, 76.04275706135237556 ) ) ;
#12173=CARTESIAN_POINT ( 'NONE',  ( -14.34966873604960291, -8.224510206698953496, 76.66557627198103830 ) ) ;
#12174=CARTESIAN_POINT ( 'NONE',  ( -16.36317988757058117, -7.306389748694932962, 100.9021039163677500 ) ) ;
#12175=CARTESIAN_POINT ( 'NONE',  ( -0.05219959533936034679, 19.03943276465977164, 102.5010903946856757 ) ) ;
#12176=CARTESIAN_POINT ( 'NONE',  ( -15.80617190586745835, -15.72974639402198527, 41.87390960531435979 ) ) ;
#12179=CARTESIAN_POINT ( 'NONE',  ( 12.14591786802327356, -12.06949235617739191, 55.62609039468568284 ) ) ;
#12180=CARTESIAN_POINT ( 'NONE',  ( 10.81492255796106328, -18.62759615963255655, 25.41775706135235779 ) ) ;
#12181=CARTESIAN_POINT ( 'NONE',  ( -18.62759615963270932, 10.81492255796079327, 50.83224293864770971 ) ) ;
#12182=CARTESIAN_POINT ( 'NONE',  ( 12.06949235617739724, 12.14591786802326823, 66.87609039468568994 ) ) ;
#12183=CARTESIAN_POINT ( 'NONE',  ( -16.46253265017160317, 9.564922557960807481, 90.83224293864769550 ) ) ;
#12184=CARTESIAN_POINT ( 'NONE',  ( -21.52544592524334988, -5.823673210054445271, 53.95942372801900433 ) ) ;
#12185=CARTESIAN_POINT ( 'NONE',  ( 16.46253265017160672, -9.564922557960803928, 28.33224293864769550 ) ) ;
#12186=CARTESIAN_POINT ( 'NONE',  ( 15.80617190586746368, 15.72974639402197994, 29.37390960531435269 ) ) ;
#12188=CARTESIAN_POINT ( 'NONE',  ( -13.89961937509957401, -13.97604488694547875, 44.37609039468566863 ) ) ;
#12189=CARTESIAN_POINT ( 'NONE',  ( 8.224510206698742110, 14.34966873604972548, 47.08442372801901854 ) ) ;
#12190=CARTESIAN_POINT ( 'NONE',  ( -10.81492255796078084, -18.62759615963271287, 22.08224293864769194 ) ) ;
#12192=CARTESIAN_POINT ( 'NONE',  ( 19.05341960407611168, 5.049401038298154454, 78.95724293864769550 ) ) ;
#12193=CARTESIAN_POINT ( 'NONE',  ( 0.05219959533934541429, -16.53943276465976808, 105.0010903946856757 ) ) ;
#12195=CARTESIAN_POINT ( 'NONE',  ( 16.55341960407611168, 4.379528057220329451, 98.95724293864770971 ) ) ;
#12196=CARTESIAN_POINT ( 'NONE',  ( 15.72974639402199770, -15.80617190586745480, 38.12390960531436690 ) ) ;
#12197=CARTESIAN_POINT ( 'NONE',  ( -13.89961937509977652, 13.97604488694528158, 30.62390960531435269 ) ) ;
#12198=CARTESIAN_POINT ( 'NONE',  ( 0.05219959533934541429, -16.53943276465976808, 75.00109039468568994 ) ) ;
#12199=CARTESIAN_POINT ( 'NONE',  ( 10.81492255796106328, -18.62759615963255655, 20.41775706135234714 ) ) ;
#12200=CARTESIAN_POINT ( 'NONE',  ( 19.02544592524334988, 5.153800228976608722, 81.45942372801897591 ) ) ;
#12201=CARTESIAN_POINT ( 'NONE',  ( -9.474510206698964154, 16.51473224551069663, 45.41557627198103120 ) ) ;
#12203=CARTESIAN_POINT ( 'NONE',  ( 5.153800228976335163, 19.02544592524342804, 114.7905762719810241 ) ) ;
#12204=EDGE_CURVE ( 'NONE', #184582, #66658, #133796, .T. ) ;
#12205=CARTESIAN_POINT ( 'NONE',  ( -5.719274019375665041, -21.55341960407619695, 109.7927570613523613 ) ) ;
#12206=CARTESIAN_POINT ( 'NONE',  ( 19.05341960407611168, 5.049401038298154454, 58.95724293864768129 ) ) ;
#12207=CARTESIAN_POINT ( 'NONE',  ( 8.224510206698742110, 14.34966873604972548, 52.08442372801901854 ) ) ;
#12208=CARTESIAN_POINT ( 'NONE',  ( 10.72451020669871369, 18.67979575497193778, 92.08442372801901854 ) ) ;
#12209=CARTESIAN_POINT ( 'NONE',  ( 13.89961937509957401, 13.97604488694547697, 36.87609039468565442 ) ) ;
#12210=CARTESIAN_POINT ( 'NONE',  ( 19.05341960407617918, -5.049401038297876454, 56.04275706135234714 ) ) ;
#12212=CARTESIAN_POINT ( 'NONE',  ( -18.62759615963255300, -10.81492255796106328, 44.16775706135234714 ) ) ;
#12213=CARTESIAN_POINT ( 'NONE',  ( -16.46253265017160317, 9.564922557960807481, 55.83224293864769550 ) ) ;
#12214=CARTESIAN_POINT ( 'NONE',  ( -5.153800228976607833, 19.02544592524334988, 42.70942372801901143 ) ) ;
#12215=CARTESIAN_POINT ( 'NONE',  ( 13.89961937509977652, -13.97604488694527269, 103.1239096053143527 ) ) ;
#12216=CARTESIAN_POINT ( 'NONE',  ( 9.474510206698971260, -16.51473224551069308, 77.91557627198103830 ) ) ;
#12217=CARTESIAN_POINT ( 'NONE',  ( 14.29746914071049879, -8.314922557960816363, 43.33224293864769550 ) ) ;
#12218=CARTESIAN_POINT ( 'NONE',  ( 21.55341960407610458, 5.719274019375980345, 33.95724293864769550 ) ) ;
#12221=CARTESIAN_POINT ( 'NONE',  ( -18.62759615963255300, -10.81492255796106328, 104.1677570613523471 ) ) ;
#12223=CARTESIAN_POINT ( 'NONE',  ( 19.05341960407611168, 5.049401038298154454, 43.95724293864769550 ) ) ;
#12224=CARTESIAN_POINT ( 'NONE',  ( 19.03943276465977164, -0.05219959533909143690, 108.7489096053143527 ) ) ;
#12226=CARTESIAN_POINT ( 'NONE',  ( -14.34966873604972548, 8.224510206698743886, 58.33442372801901143 ) ) ;
#12227=CARTESIAN_POINT ( 'NONE',  ( 0.05219959533907565091, 21.53943276465977519, 79.99890960531435269 ) ) ;
#12228=EDGE_CURVE ( 'NONE', #83853, #179366, #186155, .T. ) ;
#12229=CARTESIAN_POINT ( 'NONE',  ( -16.55341960407611168, -4.379528057220339221, 36.45724293864768839 ) ) ;
#12230=CARTESIAN_POINT ( 'NONE',  ( -19.05341960407611168, -5.049401038298163336, 31.45724293864769550 ) ) ;
#12231=CARTESIAN_POINT ( 'NONE',  ( -19.02544592524342804, 5.153800228976336051, 106.0405762719810241 ) ) ;
#12232=CARTESIAN_POINT ( 'NONE',  ( -5.823673210054431948, 21.52544592524334988, 32.70942372801900433 ) ) ;
#12233=CARTESIAN_POINT ( 'NONE',  ( -19.03943276465977164, -0.05219959533935918106, 33.75109039468566863 ) ) ;
#12234=CARTESIAN_POINT ( 'NONE',  ( 0.05219959533909260263, 19.03943276465977164, 34.99890960531435979 ) ) ;
#12235=CARTESIAN_POINT ( 'NONE',  ( -21.52544592524334988, -5.823673210054445271, 83.95942372801900433 ) ) ;
#12236=CARTESIAN_POINT ( 'NONE',  ( 16.19135201231363297, -7.376712067592066546, 32.31319145947969673 ) ) ;
#12237=CARTESIAN_POINT ( 'NONE',  ( 14.34966873604960469, 8.224510206698951720, 29.16557627198103120 ) ) ;
#12239=CARTESIAN_POINT ( 'NONE',  ( -10.72451020669898014, 18.67979575497178502, 30.41557627198101699 ) ) ;
#12240=CARTESIAN_POINT ( 'NONE',  ( -4.379528057220328563, 16.55341960407611168, 105.2072429386477097 ) ) ;
#12242=CARTESIAN_POINT ( 'NONE',  ( -13.97604488694527625, -13.89961937509977652, 86.87390960531436690 ) ) ;
#12243=CARTESIAN_POINT ( 'NONE',  ( 16.55341960407611168, 4.379528057220329451, 73.95724293864769550 ) ) ;
#12244=CARTESIAN_POINT ( 'NONE',  ( -9.474510206698720793, -16.51473224551083518, 104.5844237280190043 ) ) ;
#12245=CARTESIAN_POINT ( 'NONE',  ( 5.719274019375991003, -21.55341960407610458, 62.70724293864769550 ) ) ;
#12246=ORIENTED_EDGE ( 'NONE', *, *, #194452, .T. ) ;
#12247=CARTESIAN_POINT ( 'NONE',  ( 13.89961937509977652, -13.97604488694527269, 28.12390960531435624 ) ) ;
#12248=CARTESIAN_POINT ( 'NONE',  ( -13.89961937509977652, 13.97604488694528158, 80.62390960531436690 ) ) ;
#12249=CARTESIAN_POINT ( 'NONE',  ( -0.05219959533907301413, -21.53943276465977519, 87.49890960531436690 ) ) ;
#12250=CARTESIAN_POINT ( 'NONE',  ( 14.34966873604972726, -8.224510206698740333, 110.8344237280190043 ) ) ;
#12251=CARTESIAN_POINT ( 'NONE',  ( -5.049401038298153566, 19.05341960407611168, 85.20724293864766707 ) ) ;
#12252=CARTESIAN_POINT ( 'NONE',  ( 0.05219959533936267826, -19.03943276465977164, 70.00109039468566152 ) ) ;
#12253=CARTESIAN_POINT ( 'NONE',  ( -10.72451020669870658, -18.67979575497194134, 89.58442372801901854 ) ) ;
#12254=CARTESIAN_POINT ( 'NONE',  ( -15.80617190586745835, -15.72974639402198527, 71.87390960531438111 ) ) ;
#12255=CARTESIAN_POINT ( 'NONE',  ( -21.55341960407610458, -5.719274019375992779, 41.45724293864769550 ) ) ;
#12256=CARTESIAN_POINT ( 'NONE',  ( 16.46253265017160672, -9.564922557960803928, 53.33224293864768839 ) ) ;
#12257=CARTESIAN_POINT ( 'NONE',  ( 14.29746914071037800, 8.314922557961029526, 111.6677570613523613 ) ) ;
#12258=CARTESIAN_POINT ( 'NONE',  ( -13.89961937509977652, 13.97604488694528158, 65.62390960531436690 ) ) ;
#12259=CARTESIAN_POINT ( 'NONE',  ( 21.53943276465977519, 0.05219959533937863772, 106.2510903946856757 ) ) ;
#12260=CARTESIAN_POINT ( 'NONE',  ( -0.05219959533910754901, -16.53943276465976808, 77.49890960531433848 ) ) ;
#12261=CARTESIAN_POINT ( 'NONE',  ( -21.53943276465977519, 0.05219959533907696930, 111.2489096053143669 ) ) ;
#12262=CARTESIAN_POINT ( 'NONE',  ( -21.53943276465977519, 0.05219959533907696930, 101.2489096053143669 ) ) ;
#12264=CARTESIAN_POINT ( 'NONE',  ( -21.53943276465977519, 0.05219959533907696930, 56.24890960531436690 ) ) ;
#12265=CARTESIAN_POINT ( 'NONE',  ( -4.379528057220086978, -16.55341960407618274, 89.79275706135236135 ) ) ;
#12266=CARTESIAN_POINT ( 'NONE',  ( 12.14591786802309770, 12.06949235617756955, 104.3739096053143669 ) ) ;
#12267=CARTESIAN_POINT ( 'NONE',  ( -9.564922557960796823, -16.46253265017161027, 57.08224293864769550 ) ) ;
#12268=CARTESIAN_POINT ( 'NONE',  ( 16.55341960407618274, -4.379528057220086978, 111.0427570613523613 ) ) ;
#12269=CARTESIAN_POINT ( 'NONE',  ( 15.80617190586769283, -15.72974639402175789, 40.62609039468567573 ) ) ;
#12270=CARTESIAN_POINT ( 'NONE',  ( 19.02544592524343514, -5.153800228976328945, 103.5405762719809957 ) ) ;
#12271=CARTESIAN_POINT ( 'NONE',  ( 5.719274019375673035, 21.55341960407619339, 82.29275706135234714 ) ) ;
#12272=CARTESIAN_POINT ( 'NONE',  ( -19.02544592524342804, 5.153800228976336051, 36.04057627198100988 ) ) ;
#12273=CARTESIAN_POINT ( 'NONE',  ( 19.02544592524343514, -5.153800228976328945, 43.54057627198103120 ) ) ;
#12275=CARTESIAN_POINT ( 'NONE',  ( 21.52544592524334988, 5.823673210054432836, 86.45942372801901854 ) ) ;
#12276=CARTESIAN_POINT ( 'NONE',  ( -0.05219959533937732626, 21.53943276465977519, 67.50109039468568994 ) ) ;
#12277=CARTESIAN_POINT ( 'NONE',  ( 5.153800228976335163, 19.02544592524342804, 109.7905762719810099 ) ) ;
#12278=CARTESIAN_POINT ( 'NONE',  ( -16.46253265017146816, -9.564922557961047289, 74.16775706135234714 ) ) ;
#12279=CARTESIAN_POINT ( 'NONE',  ( 15.72974639402176855, 15.80617190586768217, 61.87609039468568284 ) ) ;
#12280=CARTESIAN_POINT ( 'NONE',  ( 8.224510206698742110, 14.34966873604972548, 22.08442372801901143 ) ) ;
#12281=CARTESIAN_POINT ( 'NONE',  ( -5.153800228976607833, 19.02544592524334988, 77.70942372801900433 ) ) ;
#12282=CARTESIAN_POINT ( 'NONE',  ( -16.46253265017160317, 9.564922557960807481, 50.83224293864770260 ) ) ;
#12283=CARTESIAN_POINT ( 'NONE',  ( -19.03943276465977164, -0.05219959533935918106, 88.75109039468567573 ) ) ;
#12285=CARTESIAN_POINT ( 'NONE',  ( 16.52544592524342804, -4.483927247898539470, 23.54057627198102765 ) ) ;
#12286=CARTESIAN_POINT ( 'NONE',  ( -19.02544592524334988, -5.153800228976617603, 93.95942372801900433 ) ) ;
#12287=CARTESIAN_POINT ( 'NONE',  ( 12.14591786802309770, 12.06949235617756955, 44.37390960531435979 ) ) ;
#12288=CARTESIAN_POINT ( 'NONE',  ( -13.89961937509957401, -13.97604488694547875, 59.37609039468566863 ) ) ;
#12289=CARTESIAN_POINT ( 'NONE',  ( -16.53943276465976808, -0.05219959533934237506, 43.75109039468568284 ) ) ;
#12290=CARTESIAN_POINT ( 'NONE',  ( -19.05341960407617563, 5.049401038297882671, 23.54275706135233648 ) ) ;
#12291=CARTESIAN_POINT ( 'NONE',  ( -5.049401038298153566, 19.05341960407611168, 40.20724293864768839 ) ) ;
#12292=CARTESIAN_POINT ( 'NONE',  ( -16.21995358207306026, -7.366697692864124569, 65.06448998487844904 ) ) ;
#12293=CARTESIAN_POINT ( 'NONE',  ( 16.53943276465976808, 0.05219959533934440121, 41.25109039468568284 ) ) ;
#12296=CARTESIAN_POINT ( 'NONE',  ( 5.049401038298161559, -19.05341960407611168, 97.70724293864766707 ) ) ;
#12298=CARTESIAN_POINT ( 'NONE',  ( 5.153800228976615827, -19.02544592524334988, 95.20942372801897591 ) ) ;
#12299=CARTESIAN_POINT ( 'NONE',  ( -0.05219959533907301413, -21.53943276465977519, 22.49890960531436335 ) ) ;
#12300=CARTESIAN_POINT ( 'NONE',  ( -9.564922557961040184, 16.46253265017147172, 22.91775706135233648 ) ) ;
#12301=CARTESIAN_POINT ( 'NONE',  ( 9.474510206698729675, 16.51473224551082808, 112.0844237280190043 ) ) ;
#12302=CARTESIAN_POINT ( 'NONE',  ( -4.483927247898539470, -16.52544592524342804, 112.2905762719810241 ) ) ;
#12303=CARTESIAN_POINT ( 'NONE',  ( -16.51473224551069308, -9.474510206698971260, 31.66557627198102054 ) ) ;
#12304=CARTESIAN_POINT ( 'NONE',  ( -5.823673210054116645, -21.52544592524344225, 57.29057627198103120 ) ) ;
#12305=CARTESIAN_POINT ( 'NONE',  ( 19.02544592524343514, -5.153800228976328945, 43.54057627198103120 ) ) ;
#12306=CARTESIAN_POINT ( 'NONE',  ( 9.474510206698729675, 16.51473224551082808, 47.08442372801900433 ) ) ;
#12307=CARTESIAN_POINT ( 'NONE',  ( 19.02544592524334988, 5.153800228976608722, 71.45942372801900433 ) ) ;
#12308=CARTESIAN_POINT ( 'NONE',  ( -8.314922557960811034, -14.29746914071050412, 52.08224293864768839 ) ) ;
#12310=CARTESIAN_POINT ( 'NONE',  ( 10.72451020669898902, -18.67979575497178502, 32.91557627198102409 ) ) ;
#12311=CARTESIAN_POINT ( 'NONE',  ( 18.67979575497194134, -10.72451020669871369, 95.83442372801903275 ) ) ;
#12312=CARTESIAN_POINT ( 'NONE',  ( 10.81492255796078972, 18.62759615963270932, 84.58224293864769550 ) ) ;
#12313=CARTESIAN_POINT ( 'NONE',  ( -18.67979575497193778, 10.72451020669871902, 63.33442372801900433 ) ) ;
#12314=CARTESIAN_POINT ( 'NONE',  ( -21.55341960407619339, 5.719274019375674811, 68.54275706135234714 ) ) ;
#12315=CARTESIAN_POINT ( 'NONE',  ( 19.03943276465977164, -0.05219959533909143690, 93.74890960531435269 ) ) ;
#12316=CARTESIAN_POINT ( 'NONE',  ( -8.224510206698735004, -14.34966873604973081, 89.58442372801901854 ) ) ;
#12317=CARTESIAN_POINT ( 'NONE',  ( -21.52544592524334988, -5.823673210054445271, 68.95942372801901854 ) ) ;
#12318=CARTESIAN_POINT ( 'NONE',  ( -9.474510206698964154, 16.51473224551069663, 55.41557627198103120 ) ) ;
#12319=CARTESIAN_POINT ( 'NONE',  ( 19.03943276465977164, -0.05219959533909143690, 23.74890960531435269 ) ) ;
#12320=CARTESIAN_POINT ( 'NONE',  ( -19.03943276465977164, 0.05219959533909376836, 51.24890960531436690 ) ) ;
#12321=CARTESIAN_POINT ( 'NONE',  ( 4.379528057220339221, -16.55341960407611168, 62.70724293864769550 ) ) ;
#12322=CARTESIAN_POINT ( 'NONE',  ( -4.379528057220328563, 16.55341960407611168, 35.20724293864768839 ) ) ;
#12323=CARTESIAN_POINT ( 'NONE',  ( -5.719274019375978568, 21.55341960407610458, 45.20724293864769550 ) ) ;
#12324=CARTESIAN_POINT ( 'NONE',  ( 9.474510206698971260, -16.51473224551069308, 47.91557627198102409 ) ) ;
#12325=CARTESIAN_POINT ( 'NONE',  ( -5.823673210054116645, -21.52544592524344225, 52.29057627198102409 ) ) ;
#12326=CARTESIAN_POINT ( 'NONE',  ( -19.02544592524334988, -5.153800228976617603, 48.95942372801900433 ) ) ;
#12328=CARTESIAN_POINT ( 'NONE',  ( 16.53943276465976808, -0.05219959533910856209, 48.74890960531435979 ) ) ;
#12329=CARTESIAN_POINT ( 'NONE',  ( -18.62759615963270932, 10.81492255796079327, 25.83224293864769194 ) ) ;
#12331=ORIENTED_EDGE ( 'NONE', *, *, #190442, .T. ) ;
#12333=CARTESIAN_POINT ( 'NONE',  ( -12.14591786802326823, 12.06949235617739902, 88.12609039468570415 ) ) ;
#12334=CARTESIAN_POINT ( 'NONE',  ( -5.049401038297874678, -19.05341960407617918, 74.79275706135231871 ) ) ;
#12335=CARTESIAN_POINT ( 'NONE',  ( 8.314922557960818139, 14.29746914071049879, 54.58224293864769550 ) ) ;
#12336=CARTESIAN_POINT ( 'NONE',  ( -18.22780087662126647, -5.499999999999827693, 58.98236817873108606 ) ) ;
#12337=CARTESIAN_POINT ( 'NONE',  ( -14.34966873604960291, -8.224510206698953496, 46.66557627198102409 ) ) ;
#12338=CARTESIAN_POINT ( 'NONE',  ( -5.153800228976328057, -19.02544592524343514, 57.29057627198103120 ) ) ;
#12339=CARTESIAN_POINT ( 'NONE',  ( 16.46253265017160672, -9.564922557960803928, 68.33224293864770971 ) ) ;
#12340=CARTESIAN_POINT ( 'NONE',  ( -13.89961937509977652, 13.97604488694528158, 35.62390960531435269 ) ) ;
#12341=CARTESIAN_POINT ( 'NONE',  ( 0.05219959533937995610, -21.53943276465977519, 40.00109039468567573 ) ) ;
#12342=CARTESIAN_POINT ( 'NONE',  ( 13.97604488694527802, 13.89961937509977652, 74.37390960531436690 ) ) ;
#12343=CARTESIAN_POINT ( 'NONE',  ( -9.564922557960796823, -16.46253265017161027, 22.08224293864768839 ) ) ;
#12344=CARTESIAN_POINT ( 'NONE',  ( -5.049401038298153566, 19.05341960407611168, 60.20724293864768129 ) ) ;
#12345=CARTESIAN_POINT ( 'NONE',  ( 18.62759615963271287, -10.81492255796078972, 53.33224293864769550 ) ) ;
#12346=CARTESIAN_POINT ( 'NONE',  ( -5.049401038298153566, 19.05341960407611168, 35.20724293864768839 ) ) ;
#12347=CARTESIAN_POINT ( 'NONE',  ( -21.55341960407610458, -5.719274019375992779, 46.45724293864769550 ) ) ;
#12348=CARTESIAN_POINT ( 'NONE',  ( 16.53943276465976808, 0.05219959533934440121, 96.25109039468568994 ) ) ;
#12350=CARTESIAN_POINT ( 'NONE',  ( -16.51473224551082808, 9.474510206698731452, 28.33442372801900433 ) ) ;
#12351=CARTESIAN_POINT ( 'NONE',  ( 16.55341960407618274, -4.379528057220086978, 51.04275706135234714 ) ) ;
#12352=CARTESIAN_POINT ( 'NONE',  ( -14.34966873604972548, 8.224510206698743886, 78.33442372801901854 ) ) ;
#12353=CARTESIAN_POINT ( 'NONE',  ( -18.22780087662123805, 5.499999999999981348, 101.0176318212689495 ) ) ;
#12354=CARTESIAN_POINT ( 'NONE',  ( 8.224510206698742110, 14.34966873604972548, 72.08442372801899012 ) ) ;
#12355=CARTESIAN_POINT ( 'NONE',  ( -16.53943276465976808, -0.05219959533934237506, 38.75109039468567573 ) ) ;
#12356=CARTESIAN_POINT ( 'NONE',  ( -13.97604488694527625, -13.89961937509977652, 111.8739096053143243 ) ) ;
#12357=CARTESIAN_POINT ( 'NONE',  ( -8.224510206698735004, -14.34966873604973081, 24.58442372801901499 ) ) ;
#12358=CARTESIAN_POINT ( 'NONE',  ( 9.564922557960805705, 16.46253265017160317, 29.58224293864769550 ) ) ;
#12359=CARTESIAN_POINT ( 'NONE',  ( 21.52544592524334988, 5.823673210054432836, 21.45942372801901499 ) ) ;
#12360=CARTESIAN_POINT ( 'NONE',  ( 14.34966873604972726, -8.224510206698740333, 40.83442372801901854 ) ) ;
#12361=CARTESIAN_POINT ( 'NONE',  ( 12.06949235617739724, 12.14591786802326823, 96.87609039468568994 ) ) ;
#12363=CARTESIAN_POINT ( 'NONE',  ( -18.67979575497193778, 10.72451020669871902, 98.33442372801901854 ) ) ;
#12364=CARTESIAN_POINT ( 'NONE',  ( 9.564922557961047289, -16.46253265017146816, 95.41775706135233293 ) ) ;
#12365=CARTESIAN_POINT ( 'NONE',  ( -12.06949235617756955, 12.14591786802309770, 55.62390960531436690 ) ) ;
#12366=CARTESIAN_POINT ( 'NONE',  ( -5.049401038298153566, 19.05341960407611168, 25.20724293864768484 ) ) ;
#12367=CARTESIAN_POINT ( 'NONE',  ( 13.97604488694548053, -13.89961937509957401, 55.62609039468566863 ) ) ;
#12368=CARTESIAN_POINT ( 'NONE',  ( 17.12812012977029141, 6.668231424565949972, 78.85948759323146362 ) ) ;
#12369=CARTESIAN_POINT ( 'NONE',  ( 15.72974639402176855, 15.80617190586768217, 56.87609039468568994 ) ) ;
#12370=CARTESIAN_POINT ( 'NONE',  ( 12.06949235617739724, 12.14591786802326823, 31.87609039468567929 ) ) ;
#12371=CARTESIAN_POINT ( 'NONE',  ( 16.31925111598459210, 7.325300261831483972, 82.33575461032749843 ) ) ;
#12372=CARTESIAN_POINT ( 'NONE',  ( 21.55341960407610458, 5.719274019375980345, 28.95724293864769905 ) ) ;
#12373=CARTESIAN_POINT ( 'NONE',  ( 5.823673210054125526, 21.52544592524343514, 69.79057627198102409 ) ) ;
#12374=CARTESIAN_POINT ( 'NONE',  ( 13.89961937509957401, 13.97604488694547697, 106.8760903946856757 ) ) ;
#12375=CARTESIAN_POINT ( 'NONE',  ( 5.049401038298161559, -19.05341960407611168, 102.7072429386476955 ) ) ;
#12378=CARTESIAN_POINT ( 'NONE',  ( 16.55341960407611168, 4.379528057220329451, 113.9572429386477239 ) ) ;
#12379=CARTESIAN_POINT ( 'NONE',  ( 18.62759615963255655, 10.81492255796105972, 96.66775706135234714 ) ) ;
#12380=CARTESIAN_POINT ( 'NONE',  ( -19.05341960407611168, -5.049401038298163336, 36.45724293864766707 ) ) ;
#12381=CARTESIAN_POINT ( 'NONE',  ( 10.81492255796106328, -18.62759615963255655, 50.41775706135235424 ) ) ;
#12382=CARTESIAN_POINT ( 'NONE',  ( -10.72451020669870658, -18.67979575497194134, 94.58442372801901854 ) ) ;
#12383=CARTESIAN_POINT ( 'NONE',  ( 4.483927247898790824, -16.52544592524335698, 110.2094237280190185 ) ) ;
#12384=CARTESIAN_POINT ( 'NONE',  ( 13.97604488694527802, 13.89961937509977652, 84.37390960531433848 ) ) ;
#12385=CARTESIAN_POINT ( 'NONE',  ( 0.05219959533937995610, -21.53943276465977519, 40.00109039468567573 ) ) ;
#12386=CARTESIAN_POINT ( 'NONE',  ( -21.55341960407619339, 5.719274019375674811, 43.54275706135235424 ) ) ;
#12387=CARTESIAN_POINT ( 'NONE',  ( 19.03943276465977164, 0.05219959533936151252, 76.25109039468566152 ) ) ;
#12388=CARTESIAN_POINT ( 'NONE',  ( 5.049401038298161559, -19.05341960407611168, 92.70724293864769550 ) ) ;
#12389=CARTESIAN_POINT ( 'NONE',  ( 14.29746914071049879, -8.314922557960816363, 103.3322429386476955 ) ) ;
#12390=CARTESIAN_POINT ( 'NONE',  ( 18.67979575497178502, 10.72451020669898547, 99.16557627198100988 ) ) ;
#12391=CARTESIAN_POINT ( 'NONE',  ( -8.314922557960811034, -14.29746914071050412, 82.08224293864768129 ) ) ;
#12392=CARTESIAN_POINT ( 'NONE',  ( -13.89961937509957401, -13.97604488694547875, 24.37609039468565442 ) ) ;
#12393=CARTESIAN_POINT ( 'NONE',  ( 4.379528057220339221, -16.55341960407611168, 97.70724293864772392 ) ) ;
#12394=CARTESIAN_POINT ( 'NONE',  ( 13.97604488694527802, 13.89961937509977652, 44.37390960531435269 ) ) ;
#12395=CARTESIAN_POINT ( 'NONE',  ( -19.05341960407617563, 5.049401038297882671, 88.54275706135230450 ) ) ;
#12396=CARTESIAN_POINT ( 'NONE',  ( -4.483927247898539470, -16.52544592524342804, 47.29057627198103120 ) ) ;
#12397=CARTESIAN_POINT ( 'NONE',  ( -16.46253265017146816, -9.564922557961047289, 19.16775706135233293 ) ) ;
#12398=CARTESIAN_POINT ( 'NONE',  ( -19.02544592524342804, 5.153800228976336051, 106.0405762719810241 ) ) ;
#12399=CARTESIAN_POINT ( 'NONE',  ( 5.153800228976615827, -19.02544592524334988, 80.20942372801901854 ) ) ;
#12400=CARTESIAN_POINT ( 'NONE',  ( 5.719274019375991003, -21.55341960407610458, 77.70724293864770971 ) ) ;
#12401=CARTESIAN_POINT ( 'NONE',  ( 15.80617190586769283, -15.72974639402175789, 25.62609039468567929 ) ) ;
#12402=CARTESIAN_POINT ( 'NONE',  ( -12.14591786802326823, 12.06949235617739902, 23.12609039468567573 ) ) ;
#12403=CARTESIAN_POINT ( 'NONE',  ( -0.05219959533934338120, 16.53943276465976808, 92.50109039468567573 ) ) ;
#12404=CARTESIAN_POINT ( 'NONE',  ( -19.03943276465977164, 0.05219959533909376836, 21.24890960531436335 ) ) ;
#12405=CARTESIAN_POINT ( 'NONE',  ( -15.72974639402176322, -15.80617190586768395, 29.37609039468568284 ) ) ;
#12406=CARTESIAN_POINT ( 'NONE',  ( 0.05219959533910956823, 16.53943276465976808, 109.9989096053143527 ) ) ;
#12408=CARTESIAN_POINT ( 'NONE',  ( -16.55341960407617563, 4.379528057220093196, 53.54275706135234714 ) ) ;
#12409=CARTESIAN_POINT ( 'NONE',  ( 4.379528057220339221, -16.55341960407611168, 82.70724293864770971 ) ) ;
#12410=CARTESIAN_POINT ( 'NONE',  ( 18.62759615963271287, -10.81492255796078972, 78.33224293864770971 ) ) ;
#12411=CARTESIAN_POINT ( 'NONE',  ( 0.05219959533910956823, 16.53943276465976808, 24.99890960531435624 ) ) ;
#12412=CARTESIAN_POINT ( 'NONE',  ( 12.14591786802327356, -12.06949235617739191, 50.62609039468568994 ) ) ;
#12413=CARTESIAN_POINT ( 'NONE',  ( -9.474510206698964154, 16.51473224551069663, 50.41557627198102409 ) ) ;
#12414=CARTESIAN_POINT ( 'NONE',  ( 4.483927247898790824, -16.52544592524335698, 95.20942372801903275 ) ) ;
#12415=CARTESIAN_POINT ( 'NONE',  ( 9.474510206698729675, 16.51473224551082808, 87.08442372801900433 ) ) ;
#12416=CARTESIAN_POINT ( 'NONE',  ( -10.81492255796078084, -18.62759615963271287, 82.08224293864768129 ) ) ;
#12417=CARTESIAN_POINT ( 'NONE',  ( 8.314922557961029526, -14.29746914071037800, 110.4177570613523756 ) ) ;
#12420=CARTESIAN_POINT ( 'NONE',  ( -21.52544592524343514, 5.823673210054127303, 56.04057627198102409 ) ) ;
#12422=CARTESIAN_POINT ( 'NONE',  ( -12.14591786802326823, 12.06949235617739902, 98.12609039468570415 ) ) ;
#12423=ORIENTED_EDGE ( 'NONE', *, *, #65499, .F. ) ;
#12424=CARTESIAN_POINT ( 'NONE',  ( 18.67979575497178502, 10.72451020669898547, 34.16557627198102409 ) ) ;
#12425=CARTESIAN_POINT ( 'NONE',  ( 17.50000000000147793, 3.202012800152216787, 107.5717758397274508 ) ) ;
#12426=CARTESIAN_POINT ( 'NONE',  ( 18.67979575497178502, 10.72451020669898547, 74.16557627198102409 ) ) ;
#12427=CARTESIAN_POINT ( 'NONE',  ( -16.53943276465976808, 0.05219959533911058130, 31.24890960531435979 ) ) ;
#12428=CARTESIAN_POINT ( 'NONE',  ( -19.03943276465977164, -0.05219959533935918106, 113.7510903946856757 ) ) ;
#12429=CARTESIAN_POINT ( 'NONE',  ( -5.049401038298153566, 19.05341960407611168, 40.20724293864768839 ) ) ;
#12430=CARTESIAN_POINT ( 'NONE',  ( -4.483927247898782831, 16.52544592524335698, 32.70942372801900433 ) ) ;
#12431=CARTESIAN_POINT ( 'NONE',  ( 9.564922557960805705, 16.46253265017160317, 49.58224293864770260 ) ) ;
#12434=CARTESIAN_POINT ( 'NONE',  ( -19.05341960407611168, -5.049401038298163336, 106.4572429386476955 ) ) ;
#12435=CARTESIAN_POINT ( 'NONE',  ( 5.049401038298161559, -19.05341960407611168, 102.7072429386476955 ) ) ;
#12436=CARTESIAN_POINT ( 'NONE',  ( 14.34966873604972726, -8.224510206698740333, 90.83442372801901854 ) ) ;
#12437=CARTESIAN_POINT ( 'NONE',  ( -5.153800228976607833, 19.02544592524334988, 92.70942372801901854 ) ) ;
#12438=CARTESIAN_POINT ( 'NONE',  ( 19.05341960407617918, -5.049401038297876454, 36.04275706135234003 ) ) ;
#12439=CARTESIAN_POINT ( 'NONE',  ( -21.53943276465977519, 0.05219959533907696930, 76.24890960531435269 ) ) ;
#12440=CARTESIAN_POINT ( 'NONE',  ( 14.29746914071037800, 8.314922557961029526, 101.6677570613523613 ) ) ;
#12441=CARTESIAN_POINT ( 'NONE',  ( -21.53943276465977519, 0.05219959533907696930, 36.24890960531435979 ) ) ;
#12442=CARTESIAN_POINT ( 'NONE',  ( 9.474510206698729675, 16.51473224551082808, 97.08442372801900433 ) ) ;
#12443=CARTESIAN_POINT ( 'NONE',  ( 13.97604488694527802, 13.89961937509977652, 49.37390960531434558 ) ) ;
#12444=CARTESIAN_POINT ( 'NONE',  ( 9.564922557960805705, 16.46253265017160317, 94.58224293864769550 ) ) ;
#12445=CARTESIAN_POINT ( 'NONE',  ( 21.53943276465977519, 0.05219959533937863772, 66.25109039468567573 ) ) ;
#12446=CARTESIAN_POINT ( 'NONE',  ( -13.89961937509977652, 13.97604488694528158, 55.62390960531434558 ) ) ;
#12447=CARTESIAN_POINT ( 'NONE',  ( 16.55341960407611168, 4.379528057220329451, 103.9572429386476813 ) ) ;
#12449=CARTESIAN_POINT ( 'NONE',  ( -8.224510206698948167, 14.34966873604960824, 75.41557627198102409 ) ) ;
#12450=CARTESIAN_POINT ( 'NONE',  ( -0.05219959533907301413, -21.53943276465977519, 67.49890960531436690 ) ) ;
#12451=CARTESIAN_POINT ( 'NONE',  ( 16.46253265017146816, 9.564922557961045513, 91.66775706135234714 ) ) ;
#12452=CARTESIAN_POINT ( 'NONE',  ( 18.56399227203342406, 5.499999999999960032, 91.47830131249901342 ) ) ;
#12453=CARTESIAN_POINT ( 'NONE',  ( 13.97604488694527802, 13.89961937509977652, 59.37390960531434558 ) ) ;
#12456=CARTESIAN_POINT ( 'NONE',  ( 19.05341960407611168, 5.049401038298154454, 78.95724293864769550 ) ) ;
#12457=CARTESIAN_POINT ( 'NONE',  ( -19.02544592524342804, 5.153800228976336051, 81.04057627198103830 ) ) ;
#12458=CARTESIAN_POINT ( 'NONE',  ( 0.05219959533934541429, -16.53943276465976808, 70.00109039468568994 ) ) ;
#12460=CARTESIAN_POINT ( 'NONE',  ( -19.05341960407617563, 5.049401038297882671, 38.54275706135233293 ) ) ;
#12462=CARTESIAN_POINT ( 'NONE',  ( -19.02544592524342804, 5.153800228976336051, 116.0405762719810383 ) ) ;
#12463=CARTESIAN_POINT ( 'NONE',  ( 8.224510206698742110, 14.34966873604972548, 97.08442372801904696 ) ) ;
#12465=CARTESIAN_POINT ( 'NONE',  ( 14.29746914071037800, 8.314922557961029526, 81.66775706135236135 ) ) ;
#12466=CARTESIAN_POINT ( 'NONE',  ( -12.06949235617739369, -12.14591786802326823, 49.37609039468569705 ) ) ;
#12468=CARTESIAN_POINT ( 'NONE',  ( 10.72451020669871369, 18.67979575497193778, 62.08442372801901143 ) ) ;
#12469=CARTESIAN_POINT ( 'NONE',  ( 16.51473224551083163, -9.474510206698727899, 70.83442372801900433 ) ) ;
#12470=CARTESIAN_POINT ( 'NONE',  ( -16.51473224551082808, 9.474510206698731452, 23.33442372801900078 ) ) ;
#12471=CARTESIAN_POINT ( 'NONE',  ( 19.03943276465977164, -0.05219959533909143690, 48.74890960531435979 ) ) ;
#12472=CARTESIAN_POINT ( 'NONE',  ( 9.474510206698971260, -16.51473224551069308, 42.91557627198103120 ) ) ;
#12474=CARTESIAN_POINT ( 'NONE',  ( 18.67979575497178502, 10.72451020669898547, 74.16557627198102409 ) ) ;
#12475=CARTESIAN_POINT ( 'NONE',  ( -21.55341960407610458, -5.719274019375992779, 31.45724293864769550 ) ) ;
#12476=CARTESIAN_POINT ( 'NONE',  ( -16.46253265017160317, 9.564922557960807481, 25.83224293864769194 ) ) ;
#12477=CARTESIAN_POINT ( 'NONE',  ( 16.52544592524335698, 4.483927247898782831, 51.45942372801901854 ) ) ;
#12479=CARTESIAN_POINT ( 'NONE',  ( 21.53943276465977519, 0.05219959533937863772, 36.25109039468567573 ) ) ;
#12480=CARTESIAN_POINT ( 'NONE',  ( 12.14591786802309770, 12.06949235617756955, 54.37390960531435979 ) ) ;
#12482=CARTESIAN_POINT ( 'NONE',  ( -12.06949235617739369, -12.14591786802326823, 24.37609039468567573 ) ) ;
#12483=CARTESIAN_POINT ( 'NONE',  ( 19.03943276465977164, 0.05219959533936151252, 36.25109039468567573 ) ) ;
#12484=CARTESIAN_POINT ( 'NONE',  ( -16.53943276465976808, 0.05219959533911058130, 46.24890960531435979 ) ) ;
#12485=CARTESIAN_POINT ( 'NONE',  ( 5.823673210054125526, 21.52544592524343514, 114.7905762719810383 ) ) ;
#12487=CARTESIAN_POINT ( 'NONE',  ( -0.05219959533907301413, -21.53943276465977519, 82.49890960531436690 ) ) ;
#12488=CARTESIAN_POINT ( 'NONE',  ( -19.03943276465977164, 0.05219959533909376836, 91.24890960531436690 ) ) ;
#12489=CARTESIAN_POINT ( 'NONE',  ( 14.29746914071049879, -8.314922557960816363, 58.33224293864768839 ) ) ;
#12490=CARTESIAN_POINT ( 'NONE',  ( -19.05341960407611168, -5.049401038298163336, 106.4572429386476955 ) ) ;
#12492=CARTESIAN_POINT ( 'NONE',  ( -5.049401038297874678, -19.05341960407617918, 64.79275706135233293 ) ) ;
#12493=CARTESIAN_POINT ( 'NONE',  ( 0.05219959533907565091, 21.53943276465977519, 109.9989096053143527 ) ) ;
#12494=CARTESIAN_POINT ( 'NONE',  ( 16.46253265017160672, -9.564922557960803928, 58.33224293864769550 ) ) ;
#12495=CARTESIAN_POINT ( 'NONE',  ( -16.52544592524342804, 4.483927247898546575, 111.0405762719810525 ) ) ;
#12496=CARTESIAN_POINT ( 'NONE',  ( 21.53943276465977519, 0.05219959533937863772, 51.25109039468568994 ) ) ;
#12498=CARTESIAN_POINT ( 'NONE',  ( -4.483927247898539470, -16.52544592524342804, 37.29057627198102409 ) ) ;
#12499=CARTESIAN_POINT ( 'NONE',  ( 19.03943276465977164, -0.05219959533909143690, 43.74890960531435979 ) ) ;
#12500=CARTESIAN_POINT ( 'NONE',  ( -19.05341960407611168, -5.049401038298163336, 96.45724293864769550 ) ) ;
#12501=CARTESIAN_POINT ( 'NONE',  ( 5.719274019375991003, -21.55341960407610458, 67.70724293864769550 ) ) ;
#12503=CARTESIAN_POINT ( 'NONE',  ( 19.05341960407611168, 5.049401038298154454, 43.95724293864769550 ) ) ;
#12504=CARTESIAN_POINT ( 'NONE',  ( 5.823673210054125526, 21.52544592524343514, 59.79057627198103120 ) ) ;
#12505=CARTESIAN_POINT ( 'NONE',  ( -10.72451020669870658, -18.67979575497194134, 89.58442372801901854 ) ) ;
#12507=CARTESIAN_POINT ( 'NONE',  ( 8.224510206698742110, 14.34966873604972548, 82.08442372801901854 ) ) ;
#12508=CARTESIAN_POINT ( 'NONE',  ( -4.483927247898539470, -16.52544592524342804, 82.29057627198103830 ) ) ;
#12509=CARTESIAN_POINT ( 'NONE',  ( -13.97604488694527625, -13.89961937509977652, 71.87390960531433848 ) ) ;
#12510=ORIENTED_EDGE ( 'NONE', *, *, #158809, .T. ) ;
#12511=CARTESIAN_POINT ( 'NONE',  ( 5.049401038297881783, 19.05341960407617563, 32.29275706135233293 ) ) ;
#12512=CARTESIAN_POINT ( 'NONE',  ( 4.483927247898790824, -16.52544592524335698, 85.20942372801901854 ) ) ;
#12513=CARTESIAN_POINT ( 'NONE',  ( 21.52544592524334988, 5.823673210054432836, 106.4594237280190328 ) ) ;
#12514=CARTESIAN_POINT ( 'NONE',  ( -19.02544592524342804, 5.153800228976336051, 91.04057627198100988 ) ) ;
#12515=CARTESIAN_POINT ( 'NONE',  ( -21.52544592524343514, 5.823673210054127303, 46.04057627198103830 ) ) ;
#12516=CARTESIAN_POINT ( 'NONE',  ( -0.05219959533937732626, 21.53943276465977519, 92.50109039468567573 ) ) ;
#12517=CARTESIAN_POINT ( 'NONE',  ( -4.483927247898782831, 16.52544592524335698, 57.70942372801901143 ) ) ;
#12518=CARTESIAN_POINT ( 'NONE',  ( -18.62759615963270932, 10.81492255796079327, 115.8322429386477097 ) ) ;
#12519=CARTESIAN_POINT ( 'NONE',  ( 12.14591786802327356, -12.06949235617739191, 20.62609039468568639 ) ) ;
#12520=CARTESIAN_POINT ( 'NONE',  ( 16.51473224551069308, 9.474510206698969483, 89.16557627198103830 ) ) ;
#12521=CARTESIAN_POINT ( 'NONE',  ( -14.34966873604972548, 8.224510206698743886, 28.33442372801902209 ) ) ;
#12522=CARTESIAN_POINT ( 'NONE',  ( 9.474510206698971260, -16.51473224551069308, 57.91557627198103120 ) ) ;
#12523=CARTESIAN_POINT ( 'NONE',  ( 0.05219959533934541429, -16.53943276465976808, 40.00109039468567573 ) ) ;
#12524=CARTESIAN_POINT ( 'NONE',  ( -4.483927247898539470, -16.52544592524342804, 77.29057627198102409 ) ) ;
#12525=CARTESIAN_POINT ( 'NONE',  ( 14.34966873604972726, -8.224510206698740333, 90.83442372801901854 ) ) ;
#12526=CARTESIAN_POINT ( 'NONE',  ( -15.80617190586768217, 15.72974639402176855, 48.12609039468568284 ) ) ;
#12527=CARTESIAN_POINT ( 'NONE',  ( -16.51473224551069308, -9.474510206698971260, 61.66557627198103120 ) ) ;
#12528=CARTESIAN_POINT ( 'NONE',  ( 13.97604488694527802, 13.89961937509977652, 79.37390960531435269 ) ) ;
#12529=CARTESIAN_POINT ( 'NONE',  ( -14.29746914071037622, -8.314922557961029526, 84.16775706135234714 ) ) ;
#12532=CARTESIAN_POINT ( 'NONE',  ( -19.03943276465977164, -0.05219959533935918106, 33.75109039468566863 ) ) ;
#12533=CARTESIAN_POINT ( 'NONE',  ( 19.05341960407611168, 5.049401038298154454, 93.95724293864769550 ) ) ;
#12534=CARTESIAN_POINT ( 'NONE',  ( -13.89961937509977652, 13.97604488694528158, 55.62390960531434558 ) ) ;
#12535=CARTESIAN_POINT ( 'NONE',  ( -9.564922557960796823, -16.46253265017161027, 112.0822429386476955 ) ) ;
#12536=CARTESIAN_POINT ( 'NONE',  ( -16.53943276465976808, -0.05219959533934237506, 38.75109039468567573 ) ) ;
#12537=CARTESIAN_POINT ( 'NONE',  ( -5.049401038297874678, -19.05341960407617918, 59.79275706135231871 ) ) ;
#12538=CARTESIAN_POINT ( 'NONE',  ( -8.224510206698735004, -14.34966873604973081, 59.58442372801901854 ) ) ;
#12540=CARTESIAN_POINT ( 'NONE',  ( -16.51473224551069308, -9.474510206698971260, 71.66557627198102409 ) ) ;
#12541=CARTESIAN_POINT ( 'NONE',  ( 21.52544592524344225, -5.823673210054117533, 108.5405762719810241 ) ) ;
#12542=CARTESIAN_POINT ( 'NONE',  ( 9.474510206698729675, 16.51473224551082808, 62.08442372801899722 ) ) ;
#12543=CARTESIAN_POINT ( 'NONE',  ( 19.02544592524343514, -5.153800228976328945, 103.5405762719809957 ) ) ;
#12544=CARTESIAN_POINT ( 'NONE',  ( -16.46253265017160317, 9.564922557960807481, 25.83224293864769194 ) ) ;
#12545=CARTESIAN_POINT ( 'NONE',  ( -13.89961937509977652, 13.97604488694528158, 70.62390960531432427 ) ) ;
#12546=CARTESIAN_POINT ( 'NONE',  ( -16.52544592524342804, 4.483927247898546575, 31.04057627198102409 ) ) ;
#12547=CARTESIAN_POINT ( 'NONE',  ( -9.474510206698964154, 16.51473224551069663, 25.41557627198103120 ) ) ;
#12548=CARTESIAN_POINT ( 'NONE',  ( 19.02544592524334988, 5.153800228976608722, 31.45942372801900433 ) ) ;
#12549=CARTESIAN_POINT ( 'NONE',  ( -14.34966873604960291, -8.224510206698953496, 71.66557627198100988 ) ) ;
#12550=CARTESIAN_POINT ( 'NONE',  ( 21.53943276465977519, 0.05219959533937863772, 101.2510903946856757 ) ) ;
#12551=CARTESIAN_POINT ( 'NONE',  ( 5.153800228976335163, 19.02544592524342804, 39.79057627198100988 ) ) ;
#12552=CARTESIAN_POINT ( 'NONE',  ( -14.34966873604960291, -8.224510206698953496, 46.66557627198102409 ) ) ;
#12553=CARTESIAN_POINT ( 'NONE',  ( 5.823673210054444382, -21.52544592524334988, 100.2094237280190043 ) ) ;
#12554=CARTESIAN_POINT ( 'NONE',  ( 19.02544592524343514, -5.153800228976328945, 98.54057627198100988 ) ) ;
#12555=CARTESIAN_POINT ( 'NONE',  ( -19.05341960407611168, -5.049401038298163336, 91.45724293864766707 ) ) ;
#12556=CARTESIAN_POINT ( 'NONE',  ( 5.153800228976335163, 19.02544592524342804, 44.79057627198103830 ) ) ;
#12557=CARTESIAN_POINT ( 'NONE',  ( -4.379528057220328563, 16.55341960407611168, 105.2072429386477097 ) ) ;
#12558=CARTESIAN_POINT ( 'NONE',  ( -8.224510206698948167, 14.34966873604960824, 75.41557627198102409 ) ) ;
#12559=CARTESIAN_POINT ( 'NONE',  ( -0.05219959533907301413, -21.53943276465977519, 87.49890960531436690 ) ) ;
#12560=CARTESIAN_POINT ( 'NONE',  ( -19.02544592524342804, 5.153800228976336051, 91.04057627198100988 ) ) ;
#12561=CARTESIAN_POINT ( 'NONE',  ( -21.53943276465977519, 0.05219959533907696930, 96.24890960531435269 ) ) ;
#12562=CARTESIAN_POINT ( 'NONE',  ( 19.05341960407611168, 5.049401038298154454, 93.95724293864769550 ) ) ;
#12563=CARTESIAN_POINT ( 'NONE',  ( -19.19724070472098276, -5.499999999999896083, 91.06193348274382515 ) ) ;
#12564=CARTESIAN_POINT ( 'NONE',  ( -14.29746914071049879, 8.314922557960819915, 100.8322429386477097 ) ) ;
#12565=CARTESIAN_POINT ( 'NONE',  ( 5.049401038298161559, -19.05341960407611168, 77.70724293864765286 ) ) ;
#12566=CARTESIAN_POINT ( 'NONE',  ( -18.62759615963270932, 10.81492255796079327, 85.83224293864768129 ) ) ;
#12568=CARTESIAN_POINT ( 'NONE',  ( -21.52544592524343514, 5.823673210054127303, 26.04057627198103475 ) ) ;
#12570=CARTESIAN_POINT ( 'NONE',  ( 14.34966873604972726, -8.224510206698740333, 25.83442372801901499 ) ) ;
#12571=CARTESIAN_POINT ( 'NONE',  ( -8.314922557960811034, -14.29746914071050412, 97.08224293864770971 ) ) ;
#12572=CARTESIAN_POINT ( 'NONE',  ( -16.36317988757060604, -7.306389748694945396, 95.90210391636779264 ) ) ;
#12573=CARTESIAN_POINT ( 'NONE',  ( -16.51473224551069308, -9.474510206698971260, 91.66557627198103830 ) ) ;
#12574=CARTESIAN_POINT ( 'NONE',  ( -16.46253265017160317, 9.564922557960807481, 45.83224293864769550 ) ) ;
#12575=CARTESIAN_POINT ( 'NONE',  ( 12.14591786802309770, 12.06949235617756955, 84.37390960531438111 ) ) ;
#12576=B_SPLINE_CURVE_WITH_KNOTS ( 'NONE', 3,
 ( #163542, #134209, #103862, #151369, #121002, #167531, #12860, #29026, #197865, #90666, #152348, #148369, #9864, #26037, #10863, #118036, #57371, #180726, #42202, #165543 ),
 .UNSPECIFIED., .F., .F.,
 ( 4, 2, 2, 2, 2, 2, 2, 2, 2, 4 ),
 ( 0.004000878361811900999, 0.004499404418915920432, 0.004997930476019939866, 0.005496456533123958432, 0.005994982590227977866, 0.006244245618779977608, 0.006493508647331976483, 0.006992034704435960354, 0.007490560761539944226, 0.007989086818643928098 ),
 .UNSPECIFIED. ) ;
#12577=CARTESIAN_POINT ( 'NONE',  ( 13.97604488694527802, 13.89961937509977652, 114.3739096053143669 ) ) ;
#12578=CARTESIAN_POINT ( 'NONE',  ( -4.483927247898539470, -16.52544592524342804, 57.29057627198103120 ) ) ;
#12579=CARTESIAN_POINT ( 'NONE',  ( -9.474510206698720793, -16.51473224551083518, 104.5844237280190043 ) ) ;
#12580=CARTESIAN_POINT ( 'NONE',  ( 10.81492255796106328, -18.62759615963255655, 55.41775706135234714 ) ) ;
#12582=CARTESIAN_POINT ( 'NONE',  ( -9.474510206698964154, 16.51473224551069663, 105.4155762719810383 ) ) ;
#12583=CARTESIAN_POINT ( 'NONE',  ( 15.80617190586746368, 15.72974639402197994, 89.37390960531435269 ) ) ;
#12584=CARTESIAN_POINT ( 'NONE',  ( 14.29746914071037800, 8.314922557961029526, 86.66775706135234714 ) ) ;
#12585=CARTESIAN_POINT ( 'NONE',  ( -9.564922557960796823, -16.46253265017161027, 22.08224293864768839 ) ) ;
#12586=CARTESIAN_POINT ( 'NONE',  ( 5.153800228976335163, 19.02544592524342804, 79.79057627198102409 ) ) ;
#12587=CARTESIAN_POINT ( 'NONE',  ( -18.62759615963270932, 10.81492255796079327, 80.83224293864769550 ) ) ;
#12588=CARTESIAN_POINT ( 'NONE',  ( 0.05219959533936267826, -19.03943276465977164, 110.0010903946856757 ) ) ;
#12589=CARTESIAN_POINT ( 'NONE',  ( -12.06949235617756955, 12.14591786802309770, 50.62390960531435979 ) ) ;
#12590=CARTESIAN_POINT ( 'NONE',  ( -10.72451020669870658, -18.67979575497194134, 54.58442372801901143 ) ) ;
#12592=CARTESIAN_POINT ( 'NONE',  ( -4.379528057220086978, -16.55341960407618274, 84.79275706135234714 ) ) ;
#12593=CARTESIAN_POINT ( 'NONE',  ( 10.81492255796078972, 18.62759615963270932, 29.58224293864769905 ) ) ;
#12594=CARTESIAN_POINT ( 'NONE',  ( 13.97604488694527802, 13.89961937509977830, 109.3739096053143385 ) ) ;
#12596=CARTESIAN_POINT ( 'NONE',  ( 8.224510206698742110, 14.34966873604972548, 107.0844237280190043 ) ) ;
#12597=CARTESIAN_POINT ( 'NONE',  ( 0.05219959533934541429, -16.53943276465976808, 65.00109039468568994 ) ) ;
#12598=CARTESIAN_POINT ( 'NONE',  ( -19.05341960407611168, -5.049401038298163336, 76.45724293864769550 ) ) ;
#12599=CARTESIAN_POINT ( 'NONE',  ( -13.97604488694527625, -13.89961937509977652, 76.87390960531433848 ) ) ;
#12600=CARTESIAN_POINT ( 'NONE',  ( -8.314922557961024197, 14.29746914071037800, 77.91775706135231871 ) ) ;
#12601=CARTESIAN_POINT ( 'NONE',  ( 16.55341960407611168, 4.379528057220329451, 43.95724293864769550 ) ) ;
#12602=CARTESIAN_POINT ( 'NONE',  ( -19.03943276465977164, 0.05219959533909376836, 51.24890960531436690 ) ) ;
#12603=CARTESIAN_POINT ( 'NONE',  ( -19.03943276465977164, 0.05219959533909376836, 51.24890960531436690 ) ) ;
#12604=CARTESIAN_POINT ( 'NONE',  ( -8.314922557961024197, 14.29746914071037800, 42.91775706135235424 ) ) ;
#12605=ORIENTED_EDGE ( 'NONE', *, *, #121376, .F. ) ;
#12606=CARTESIAN_POINT ( 'NONE',  ( -19.02544592524334988, -5.153800228976617603, 98.95942372801900433 ) ) ;
#12607=CARTESIAN_POINT ( 'NONE',  ( 0.05219959533910956823, 16.53943276465976808, 94.99890960531436690 ) ) ;
#12608=CARTESIAN_POINT ( 'NONE',  ( 16.51473224551069308, 9.474510206698969483, 64.16557627198102409 ) ) ;
#12609=CARTESIAN_POINT ( 'NONE',  ( 5.049401038297881783, 19.05341960407617563, 102.2927570613523045 ) ) ;
#12611=CARTESIAN_POINT ( 'NONE',  ( -0.05219959533937732626, 21.53943276465977519, 107.5010903946856899 ) ) ;
#12612=CARTESIAN_POINT ( 'NONE',  ( 12.14591786802327356, -12.06949235617739191, 70.62609039468567573 ) ) ;
#12614=CARTESIAN_POINT ( 'NONE',  ( -18.67979575497178146, -10.72451020669898902, 66.66557627198102409 ) ) ;
#12615=CARTESIAN_POINT ( 'NONE',  ( 4.379528057220092307, 16.55341960407617563, 52.29275706135236135 ) ) ;
#12616=CARTESIAN_POINT ( 'NONE',  ( -13.97604488694527625, -13.89961937509977830, 31.87390960531435979 ) ) ;
#12617=CARTESIAN_POINT ( 'NONE',  ( -19.03943276465977164, -0.05219959533935918106, 38.75109039468566152 ) ) ;
#12618=CARTESIAN_POINT ( 'NONE',  ( -5.049401038298153566, 19.05341960407611168, 95.20724293864770971 ) ) ;
#12619=CARTESIAN_POINT ( 'NONE',  ( -12.06949235617756955, 12.14591786802309770, 115.6239096053143669 ) ) ;
#12620=CARTESIAN_POINT ( 'NONE',  ( 5.049401038298161559, -19.05341960407611168, 67.70724293864769550 ) ) ;
#12621=CARTESIAN_POINT ( 'NONE',  ( 21.55341960407619695, -5.719274019375665929, 81.04275706135236135 ) ) ;
#12622=CARTESIAN_POINT ( 'NONE',  ( 16.46253265017146816, 9.564922557961045513, 51.66775706135233293 ) ) ;
#12623=CARTESIAN_POINT ( 'NONE',  ( 19.03943276465977164, 0.05219959533936151252, 26.25109039468566507 ) ) ;
#12624=CARTESIAN_POINT ( 'NONE',  ( -9.564922557960796823, -16.46253265017161027, 57.08224293864769550 ) ) ;
#12625=CARTESIAN_POINT ( 'NONE',  ( -21.52544592524343514, 5.823673210054127303, 26.04057627198103475 ) ) ;
#12626=CARTESIAN_POINT ( 'NONE',  ( -5.719274019375665041, -21.55341960407619695, 84.79275706135234714 ) ) ;
#12627=CARTESIAN_POINT ( 'NONE',  ( -9.564922557960796823, -16.46253265017161027, 62.08224293864769550 ) ) ;
#12628=CARTESIAN_POINT ( 'NONE',  ( -5.823673210054431948, 21.52544592524334988, 97.70942372801904696 ) ) ;
#12629=CARTESIAN_POINT ( 'NONE',  ( -5.823673210054116645, -21.52544592524344225, 32.29057627198102409 ) ) ;
#12630=CARTESIAN_POINT ( 'NONE',  ( -9.564922557960796823, -16.46253265017161027, 82.08224293864768129 ) ) ;
#12631=CARTESIAN_POINT ( 'NONE',  ( -10.81492255796105439, 18.62759615963255655, 37.91775706135235424 ) ) ;
#12632=CARTESIAN_POINT ( 'NONE',  ( 9.474510206698729675, 16.51473224551082808, 62.08442372801899722 ) ) ;
#12633=CARTESIAN_POINT ( 'NONE',  ( 16.46253265017160672, -9.564922557960803928, 38.33224293864768839 ) ) ;
#12634=CARTESIAN_POINT ( 'NONE',  ( -19.02544592524342804, 5.153800228976336051, 86.04057627198103830 ) ) ;
#12635=CARTESIAN_POINT ( 'NONE',  ( -14.29746914071037622, -8.314922557961029526, 24.16775706135235424 ) ) ;
#12636=CARTESIAN_POINT ( 'NONE',  ( 14.29746914071049879, -8.314922557960816363, 83.33224293864769550 ) ) ;
#12637=CARTESIAN_POINT ( 'NONE',  ( -16.46253265017160317, 9.564922557960807481, 70.83224293864770971 ) ) ;
#12638=CARTESIAN_POINT ( 'NONE',  ( -0.05219959533907301413, -21.53943276465977519, 52.49890960531435979 ) ) ;
#12639=CARTESIAN_POINT ( 'NONE',  ( -12.14591786802326823, 12.06949235617739902, 23.12609039468567573 ) ) ;
#12640=CARTESIAN_POINT ( 'NONE',  ( 21.55341960407619695, -5.719274019375665929, 21.04275706135234714 ) ) ;
#12641=CARTESIAN_POINT ( 'NONE',  ( 0.05219959533937995610, -21.53943276465977519, 70.00109039468568994 ) ) ;
#12642=CARTESIAN_POINT ( 'NONE',  ( -12.06949235617739369, -12.14591786802326823, 74.37609039468568994 ) ) ;
#12643=CARTESIAN_POINT ( 'NONE',  ( -0.05219959533934338120, 16.53943276465976808, 62.50109039468568284 ) ) ;
#12644=CARTESIAN_POINT ( 'NONE',  ( -13.89961937509977652, 13.97604488694528158, 65.62390960531436690 ) ) ;
#12645=CARTESIAN_POINT ( 'NONE',  ( -8.224510206698735004, -14.34966873604973081, 99.58442372801900433 ) ) ;
#12646=CARTESIAN_POINT ( 'NONE',  ( 9.564922557961047289, -16.46253265017146816, 45.41775706135232582 ) ) ;
#12647=CARTESIAN_POINT ( 'NONE',  ( 21.55341960407619695, -5.719274019375665929, 21.04275706135234714 ) ) ;
#12648=CARTESIAN_POINT ( 'NONE',  ( -12.06949235617756955, 12.14591786802309770, 60.62390960531437401 ) ) ;
#12649=CARTESIAN_POINT ( 'NONE',  ( 19.05341960407611168, 5.049401038298154454, 88.95724293864769550 ) ) ;
#12650=CARTESIAN_POINT ( 'NONE',  ( 12.14591786802327356, -12.06949235617739191, 90.62609039468567573 ) ) ;
#12651=CARTESIAN_POINT ( 'NONE',  ( -10.81492255796105439, 18.62759615963255655, 57.91775706135234714 ) ) ;
#12652=CARTESIAN_POINT ( 'NONE',  ( 14.29746914071037800, 8.314922557961029526, 31.66775706135234358 ) ) ;
#12653=CARTESIAN_POINT ( 'NONE',  ( 21.55341960407619695, -5.719274019375665929, 21.04275706135234714 ) ) ;
#12654=CARTESIAN_POINT ( 'NONE',  ( 14.29746914071049879, -8.314922557960816363, 63.33224293864770260 ) ) ;
#12656=CARTESIAN_POINT ( 'NONE',  ( 10.72451020669898902, -18.67979575497178502, 97.91557627198103830 ) ) ;
#12657=CARTESIAN_POINT ( 'NONE',  ( 12.06949235617757843, -12.14591786802309237, 33.12390960531435979 ) ) ;
#12658=ORIENTED_EDGE ( 'NONE', *, *, #135901, .T. ) ;
#12660=CARTESIAN_POINT ( 'NONE',  ( -21.53943276465977519, 0.05219959533907696930, 36.24890960531435979 ) ) ;
#12661=CARTESIAN_POINT ( 'NONE',  ( 21.52544592524334988, 5.823673210054432836, 41.45942372801901143 ) ) ;
#12662=CARTESIAN_POINT ( 'NONE',  ( -16.55341960407611168, -4.379528057220339221, 61.45724293864770260 ) ) ;
#12663=CARTESIAN_POINT ( 'NONE',  ( 5.823673210054125526, 21.52544592524343514, 64.79057627198103830 ) ) ;
#12664=CARTESIAN_POINT ( 'NONE',  ( -19.02544592524342804, 5.153800228976336051, 81.04057627198103830 ) ) ;
#12665=CARTESIAN_POINT ( 'NONE',  ( 19.03943276465977164, -0.05219959533909143690, 28.74890960531435624 ) ) ;
#12666=CARTESIAN_POINT ( 'NONE',  ( -16.46253265017146816, -9.564922557961047289, 59.16775706135233293 ) ) ;
#12667=EDGE_CURVE ( 'NONE', #59885, #155722, #67574, .T. ) ;
#12668=CARTESIAN_POINT ( 'NONE',  ( -10.81492255796078084, -18.62759615963271287, 52.08224293864768839 ) ) ;
#12669=CARTESIAN_POINT ( 'NONE',  ( -16.51473224551069308, -9.474510206698971260, 56.66557627198103120 ) ) ;
#12670=CARTESIAN_POINT ( 'NONE',  ( -4.379528057220086978, -16.55341960407618274, 39.79275706135235424 ) ) ;
#12671=CARTESIAN_POINT ( 'NONE',  ( -21.52544592524334988, -5.823673210054445271, 18.95942372801901143 ) ) ;
#12672=CARTESIAN_POINT ( 'NONE',  ( -8.314922557960811034, -14.29746914071050412, 52.08224293864768839 ) ) ;
#12673=CARTESIAN_POINT ( 'NONE',  ( -9.474510206698964154, 16.51473224551069663, 105.4155762719810383 ) ) ;
#12674=CARTESIAN_POINT ( 'NONE',  ( 15.72974639402199770, -15.80617190586745480, 73.12390960531436690 ) ) ;
#12675=CARTESIAN_POINT ( 'NONE',  ( 18.67979575497178502, 10.72451020669898547, 109.1655762719810383 ) ) ;
#12676=CARTESIAN_POINT ( 'NONE',  ( -16.53943276465976808, -0.05219959533934237506, 43.75109039468568284 ) ) ;
#12677=CARTESIAN_POINT ( 'NONE',  ( 0.05219959533907565091, 21.53943276465977519, 29.99890960531435979 ) ) ;
#12678=CARTESIAN_POINT ( 'NONE',  ( 21.53943276465977519, 0.05219959533937863772, 96.25109039468568994 ) ) ;
#12680=CARTESIAN_POINT ( 'NONE',  ( -5.049401038298153566, 19.05341960407611168, 35.20724293864768839 ) ) ;
#12681=CARTESIAN_POINT ( 'NONE',  ( 16.51473224551069308, 9.474510206698969483, 94.16557627198103830 ) ) ;
#12682=CARTESIAN_POINT ( 'NONE',  ( -0.05219959533909027116, -19.03943276465977164, 77.49890960531435269 ) ) ;
#12684=CARTESIAN_POINT ( 'NONE',  ( -19.05341960407617563, 5.049401038297882671, 53.54275706135231871 ) ) ;
#12685=CARTESIAN_POINT ( 'NONE',  ( 15.80617190586769283, -15.72974639402175789, 110.6260903946857042 ) ) ;
#12686=CARTESIAN_POINT ( 'NONE',  ( -21.52544592524343514, 5.823673210054127303, 26.04057627198103475 ) ) ;
#12687=CARTESIAN_POINT ( 'NONE',  ( 8.314922557961029526, -14.29746914071037800, 105.4177570613523613 ) ) ;
#12688=CARTESIAN_POINT ( 'NONE',  ( 19.05341960407617918, -5.049401038297876454, 91.04275706135234714 ) ) ;
#12690=CARTESIAN_POINT ( 'NONE',  ( 9.474510206698729675, 16.51473224551082808, 87.08442372801900433 ) ) ;
#12691=CARTESIAN_POINT ( 'NONE',  ( -5.049401038297874678, -19.05341960407617918, 39.79275706135232582 ) ) ;
#12692=CARTESIAN_POINT ( 'NONE',  ( -22.00000000000000000, -1.163414459189985801E-14, 95.00000000000000000 ) ) ;
#12693=CARTESIAN_POINT ( 'NONE',  ( 5.153800228976335163, 19.02544592524342804, 44.79057627198103830 ) ) ;
#12694=CARTESIAN_POINT ( 'NONE',  ( -14.34966873604960291, -8.224510206698953496, 51.66557627198102409 ) ) ;
#12695=CARTESIAN_POINT ( 'NONE',  ( -16.51473224551069308, -9.474510206698971260, 26.66557627198103120 ) ) ;
#12696=CARTESIAN_POINT ( 'NONE',  ( 16.55341960407611168, 4.379528057220329451, 23.95724293864769550 ) ) ;
#12698=CARTESIAN_POINT ( 'NONE',  ( 4.483927247898790824, -16.52544592524335698, 95.20942372801903275 ) ) ;
#12699=CARTESIAN_POINT ( 'NONE',  ( 5.153800228976335163, 19.02544592524342804, 49.79057627198100988 ) ) ;
#12700=CARTESIAN_POINT ( 'NONE',  ( -21.55341960407619339, 5.719274019375674811, 103.5427570613523613 ) ) ;
#12701=CARTESIAN_POINT ( 'NONE',  ( -0.05219959533934338120, 16.53943276465976808, 22.50109039468567573 ) ) ;
#12702=CARTESIAN_POINT ( 'NONE',  ( -10.81492255796078084, -18.62759615963271287, 42.08224293864769550 ) ) ;
#12703=CARTESIAN_POINT ( 'NONE',  ( 10.81492255796106328, -18.62759615963255655, 85.41775706135236135 ) ) ;
#12705=CARTESIAN_POINT ( 'NONE',  ( 13.97604488694527802, 13.89961937509977652, 104.3739096053143385 ) ) ;
#12706=CARTESIAN_POINT ( 'NONE',  ( 13.97604488694527802, 13.89961937509977652, 79.37390960531435269 ) ) ;
#12708=CARTESIAN_POINT ( 'NONE',  ( 18.67979575497178502, 10.72451020669898547, 104.1655762719810241 ) ) ;
#12709=CARTESIAN_POINT ( 'NONE',  ( -4.483927247898539470, -16.52544592524342804, 82.29057627198103830 ) ) ;
#12710=CARTESIAN_POINT ( 'NONE',  ( 15.72974639402199770, -15.80617190586745480, 68.12390960531436690 ) ) ;
#12711=CARTESIAN_POINT ( 'NONE',  ( 19.05341960407611168, 5.049401038298154454, 63.95724293864769550 ) ) ;
#12712=CARTESIAN_POINT ( 'NONE',  ( -21.53943276465977519, 0.05219959533907696930, 101.2489096053143669 ) ) ;
#12713=ORIENTED_EDGE ( 'NONE', *, *, #122412, .T. ) ;
#12714=CARTESIAN_POINT ( 'NONE',  ( 5.153800228976335163, 19.02544592524342804, 59.79057627198100988 ) ) ;
#12715=CARTESIAN_POINT ( 'NONE',  ( 16.53943276465976808, -0.05219959533910856209, 88.74890960531436690 ) ) ;
#12717=CARTESIAN_POINT ( 'NONE',  ( 5.153800228976335163, 19.02544592524342804, 64.79057627198100988 ) ) ;
#12718=CARTESIAN_POINT ( 'NONE',  ( -19.03943276465977164, -0.05219959533935918106, 73.75109039468566152 ) ) ;
#12719=CARTESIAN_POINT ( 'NONE',  ( -16.52544592524342804, 4.483927247898546575, 91.04057627198103830 ) ) ;
#12720=CARTESIAN_POINT ( 'NONE',  ( 18.62759615963255655, 10.81492255796105972, 61.66775706135235424 ) ) ;
#12721=CARTESIAN_POINT ( 'NONE',  ( 13.97604488694527802, 13.89961937509977652, 44.37390960531435269 ) ) ;
#12722=CARTESIAN_POINT ( 'NONE',  ( 15.80617190586746368, 15.72974639402197994, 114.3739096053143527 ) ) ;
#12723=CARTESIAN_POINT ( 'NONE',  ( -16.52544592524342804, 4.483927247898546575, 106.0405762719810525 ) ) ;
#12725=CARTESIAN_POINT ( 'NONE',  ( 0.05219959533909260263, 19.03943276465977164, 64.99890960531436690 ) ) ;
#12726=CARTESIAN_POINT ( 'NONE',  ( 16.36317988757057051, 7.306389748694948949, 113.4021039163677500 ) ) ;
#12727=CARTESIAN_POINT ( 'NONE',  ( 5.049401038297881783, 19.05341960407617563, 112.2927570613523471 ) ) ;
#12728=CARTESIAN_POINT ( 'NONE',  ( -9.564922557960796823, -16.46253265017161027, 107.0822429386476955 ) ) ;
#12729=CARTESIAN_POINT ( 'NONE',  ( -21.52544592524334988, -5.823673210054445271, 48.95942372801902565 ) ) ;
#12730=CARTESIAN_POINT ( 'NONE',  ( 9.474510206698971260, -16.51473224551069308, 92.91557627198103830 ) ) ;
#12731=CARTESIAN_POINT ( 'NONE',  ( 19.03943276465977164, 0.05219959533936151252, 81.25109039468567573 ) ) ;
#12732=CARTESIAN_POINT ( 'NONE',  ( 19.05341960407611168, 5.049401038298154454, 63.95724293864769550 ) ) ;
#12733=CARTESIAN_POINT ( 'NONE',  ( -14.34966873604960291, -8.224510206698953496, 76.66557627198103830 ) ) ;
#12734=CARTESIAN_POINT ( 'NONE',  ( -0.05219959533910754901, -16.53943276465976808, 77.49890960531433848 ) ) ;
#12735=CARTESIAN_POINT ( 'NONE',  ( 19.03943276465977164, -0.05219959533909143690, 93.74890960531435269 ) ) ;
#12736=CARTESIAN_POINT ( 'NONE',  ( 16.53943276465976808, -0.05219959533910856209, 73.74890960531433848 ) ) ;
#12737=CARTESIAN_POINT ( 'NONE',  ( 13.89961937509977652, -13.97604488694527269, 83.12390960531436690 ) ) ;
#12738=CARTESIAN_POINT ( 'NONE',  ( 19.03943276465977164, 0.05219959533936151252, 36.25109039468567573 ) ) ;
#12739=CARTESIAN_POINT ( 'NONE',  ( -19.03943276465977164, 0.05219959533909376836, 56.24890960531435979 ) ) ;
#12740=CARTESIAN_POINT ( 'NONE',  ( 0.05219959533910956823, 16.53943276465976808, 24.99890960531435624 ) ) ;
#12741=( BOUNDED_CURVE ( )  B_SPLINE_CURVE ( 2, ( #52063, #127897, #174426, #113720, #54070, #188607, #100559, #5550, #82381, #34906, #69230, #84383, #67229 ),
 .UNSPECIFIED., .F., .T. ) 
 B_SPLINE_CURVE_WITH_KNOTS ( ( 3, 2, 2, 2, 2, 2, 3 ),
 ( 0.6603251732691504117, 0.6622807017543859143, 0.6666666666666666297, 0.6710526315789473450, 0.6754385964912280604, 0.6798245614035087758, 0.6817344100666542506 ),
 .UNSPECIFIED. ) 
 CURVE ( )  GEOMETRIC_REPRESENTATION_ITEM ( )  RATIONAL_B_SPLINE_CURVE ( ( 0.9831626618144004848, 0.9848076720550091867, 1.000000000000000000, 0.9659258262890683122, 1.000000000000000000, 0.9659258262890683122, 1.000000000000000000, 0.9659258262890683122, 1.000000000000000000, 0.9659258262890683122, 1.000000000000000000, 0.9851625545550091179, 0.9832469066685282089 ) ) 
 REPRESENTATION_ITEM ( '' )  );
#12742=CARTESIAN_POINT ( 'NONE',  ( -5.049401038298153566, 19.05341960407611168, 30.20724293864768839 ) ) ;
#12743=ORIENTED_EDGE ( 'NONE', *, *, #108640, .T. ) ;
#12744=CARTESIAN_POINT ( 'NONE',  ( -15.72974639402176322, -15.80617190586768395, 49.37609039468569705 ) ) ;
#12745=CARTESIAN_POINT ( 'NONE',  ( 5.049401038297881783, 19.05341960407617563, 77.29275706135231871 ) ) ;
#12746=CARTESIAN_POINT ( 'NONE',  ( -16.53943276465976808, 0.05219959533911058130, 36.24890960531435979 ) ) ;
#12747=CARTESIAN_POINT ( 'NONE',  ( -15.80617190586745835, -15.72974639402198527, 91.87390960531436690 ) ) ;
#12748=CARTESIAN_POINT ( 'NONE',  ( 21.52544592524344225, -5.823673210054117533, 28.54057627198103120 ) ) ;
#12749=CARTESIAN_POINT ( 'NONE',  ( 0.05219959533910956823, 16.53943276465976808, 74.99890960531435269 ) ) ;
#12750=CARTESIAN_POINT ( 'NONE',  ( 9.474510206698971260, -16.51473224551069308, 42.91557627198103120 ) ) ;
#12751=CARTESIAN_POINT ( 'NONE',  ( -12.14591786802326823, 12.06949235617739902, 98.12609039468570415 ) ) ;
#12752=CARTESIAN_POINT ( 'NONE',  ( 0.05219959533934541429, -16.53943276465976808, 75.00109039468568994 ) ) ;
#12753=CARTESIAN_POINT ( 'NONE',  ( 21.53943276465977519, -0.05219959533907433946, 38.74890960531435979 ) ) ;
#12754=CARTESIAN_POINT ( 'NONE',  ( 19.05341960407617918, -5.049401038297876454, 26.04275706135233293 ) ) ;
#12755=CARTESIAN_POINT ( 'NONE',  ( -5.049401038298153566, 19.05341960407611168, 95.20724293864770971 ) ) ;
#12756=CARTESIAN_POINT ( 'NONE',  ( -14.34966873604972548, 8.224510206698743886, 68.33442372801900433 ) ) ;
#12757=CARTESIAN_POINT ( 'NONE',  ( -19.03943276465977164, 0.05219959533909376836, 21.24890960531436335 ) ) ;
#12758=CARTESIAN_POINT ( 'NONE',  ( 16.55341960407611168, 4.379528057220329451, 38.95724293864768839 ) ) ;
#12759=CARTESIAN_POINT ( 'NONE',  ( -16.46253265017160317, 9.564922557960807481, 105.8322429386476955 ) ) ;
#12760=CARTESIAN_POINT ( 'NONE',  ( 16.46253265017160672, -9.564922557960803928, 88.33224293864769550 ) ) ;
#12761=CARTESIAN_POINT ( 'NONE',  ( -21.53943276465977519, 0.05219959533907696930, 21.24890960531436690 ) ) ;
#12762=CARTESIAN_POINT ( 'NONE',  ( 4.483927247898545687, 16.52544592524342804, 74.79057627198105251 ) ) ;
#12764=CARTESIAN_POINT ( 'NONE',  ( 16.53943276465976808, -0.05219959533910856209, 58.74890960531436690 ) ) ;
#12765=CARTESIAN_POINT ( 'NONE',  ( -16.52544592524335698, -4.483927247898792601, 58.95942372801902565 ) ) ;
#12766=CARTESIAN_POINT ( 'NONE',  ( -17.97214573761829826, -5.500000000000085265, 56.46970049038657180 ) ) ;
#12767=CARTESIAN_POINT ( 'NONE',  ( 19.03943276465977164, 0.05219959533936151252, 51.25109039468567573 ) ) ;
#12768=CARTESIAN_POINT ( 'NONE',  ( 16.46253265017160672, -9.564922557960803928, 93.33224293864769550 ) ) ;
#12769=CARTESIAN_POINT ( 'NONE',  ( -16.51473224551082808, 9.474510206698731452, 63.33442372801900433 ) ) ;
#12771=CARTESIAN_POINT ( 'NONE',  ( 9.474510206698729675, 16.51473224551082808, 57.08442372801900433 ) ) ;
#12772=CARTESIAN_POINT ( 'NONE',  ( 8.314922557961029526, -14.29746914071037800, 20.41775706135234714 ) ) ;
#12773=CARTESIAN_POINT ( 'NONE',  ( 8.314922557961029526, -14.29746914071037800, 90.41775706135236135 ) ) ;
#12774=CARTESIAN_POINT ( 'NONE',  ( 19.03943276465977164, -0.05219959533909143690, 43.74890960531435979 ) ) ;
#12775=CARTESIAN_POINT ( 'NONE',  ( 9.474510206698971260, -16.51473224551069308, 112.9155762719810383 ) ) ;
#12776=CARTESIAN_POINT ( 'NONE',  ( -5.719274019375665041, -21.55341960407619695, 59.79275706135234714 ) ) ;
#12777=CARTESIAN_POINT ( 'NONE',  ( -13.97604488694547697, 13.89961937509957934, 98.12609039468566152 ) ) ;
#12778=CARTESIAN_POINT ( 'NONE',  ( 0.05219959533936267826, -19.03943276465977164, 55.00109039468566863 ) ) ;
#12779=CARTESIAN_POINT ( 'NONE',  ( -16.51473224551069308, -9.474510206698971260, 56.66557627198103120 ) ) ;
#12780=CARTESIAN_POINT ( 'NONE',  ( -19.03943276465977164, 0.05219959533909376836, 111.2489096053143669 ) ) ;
#12781=CARTESIAN_POINT ( 'NONE',  ( -14.29746914071049879, 8.314922557960819915, 75.83224293864769550 ) ) ;
#12782=CARTESIAN_POINT ( 'NONE',  ( -13.97604488694527625, -13.89961937509977652, 66.87390960531436690 ) ) ;
#12784=CARTESIAN_POINT ( 'NONE',  ( -0.05219959533909027116, -19.03943276465977164, 72.49890960531435269 ) ) ;
#12785=CARTESIAN_POINT ( 'NONE',  ( 5.049401038297881783, 19.05341960407617563, 72.29275706135234714 ) ) ;
#12786=CARTESIAN_POINT ( 'NONE',  ( -0.05219959533907301413, -21.53943276465977519, 62.49890960531436690 ) ) ;
#12787=CARTESIAN_POINT ( 'NONE',  ( -8.224510206698948167, 14.34966873604960824, 110.4155762719810383 ) ) ;
#12788=CARTESIAN_POINT ( 'NONE',  ( 5.049401038297881783, 19.05341960407617563, 52.29275706135234003 ) ) ;
#12789=CARTESIAN_POINT ( 'NONE',  ( 19.03943276465977164, -0.05219959533909143690, 53.74890960531436690 ) ) ;
#12790=CARTESIAN_POINT ( 'NONE',  ( 9.474510206698971260, -16.51473224551069308, 92.91557627198103830 ) ) ;
#12791=CARTESIAN_POINT ( 'NONE',  ( 21.52544592524344225, -5.823673210054117533, 93.54057627198103830 ) ) ;
#12792=CARTESIAN_POINT ( 'NONE',  ( 16.55341960407611168, 4.379528057220329451, 83.95724293864770971 ) ) ;
#12793=CARTESIAN_POINT ( 'NONE',  ( -19.03943276465977164, -0.05219959533935918106, 43.75109039468566863 ) ) ;
#12794=CARTESIAN_POINT ( 'NONE',  ( 18.67979575497178502, 10.72451020669898547, 74.16557627198102409 ) ) ;
#12795=CARTESIAN_POINT ( 'NONE',  ( 5.719274019375991003, -21.55341960407610458, 57.70724293864770260 ) ) ;
#12796=CARTESIAN_POINT ( 'NONE',  ( -0.05219959533910754901, -16.53943276465976808, 37.49890960531436690 ) ) ;
#12797=CARTESIAN_POINT ( 'NONE',  ( 5.719274019375673035, 21.55341960407619339, 92.29275706135236135 ) ) ;
#12798=CARTESIAN_POINT ( 'NONE',  ( -19.03943276465977164, 0.05219959533909376836, 86.24890960531436690 ) ) ;
#12799=CARTESIAN_POINT ( 'NONE',  ( 14.34966873604960469, 8.224510206698951720, 114.1655762719810383 ) ) ;
#12800=CARTESIAN_POINT ( 'NONE',  ( 21.55341960407619695, -5.719274019375665929, 31.04275706135234714 ) ) ;
#12801=CARTESIAN_POINT ( 'NONE',  ( 10.81492255796106328, -18.62759615963255655, 35.41775706135234003 ) ) ;
#12802=CARTESIAN_POINT ( 'NONE',  ( 16.46253265017160672, -9.564922557960803928, 43.33224293864769550 ) ) ;
#12803=CARTESIAN_POINT ( 'NONE',  ( -15.72974639402197994, 15.80617190586746368, 115.6239096053143669 ) ) ;
#12804=CARTESIAN_POINT ( 'NONE',  ( 13.89961937509957401, 13.97604488694547697, 61.87609039468566863 ) ) ;
#12805=CARTESIAN_POINT ( 'NONE',  ( 5.049401038298161559, -19.05341960407611168, 37.70724293864768839 ) ) ;
#12806=CARTESIAN_POINT ( 'NONE',  ( 16.55341960407618274, -4.379528057220086978, 26.04275706135235779 ) ) ;
#12808=CARTESIAN_POINT ( 'NONE',  ( -16.53943276465976808, -0.05219959533934237506, 68.75109039468568994 ) ) ;
#12809=CARTESIAN_POINT ( 'NONE',  ( -9.474510206698964154, 16.51473224551069663, 45.41557627198103120 ) ) ;
#12811=CARTESIAN_POINT ( 'NONE',  ( 5.153800228976335163, 19.02544592524342804, 89.79057627198102409 ) ) ;
#12812=CARTESIAN_POINT ( 'NONE',  ( 13.89961937509977652, -13.97604488694527269, 23.12390960531436335 ) ) ;
#12813=CARTESIAN_POINT ( 'NONE',  ( 21.53943276465977519, -0.05219959533907433946, 63.74890960531435979 ) ) ;
#12814=CARTESIAN_POINT ( 'NONE',  ( -14.29746914071037622, -8.314922557961029526, 44.16775706135234714 ) ) ;
#12815=CARTESIAN_POINT ( 'NONE',  ( 21.53943276465977519, 0.05219959533937863772, 106.2510903946856757 ) ) ;
#12816=CARTESIAN_POINT ( 'NONE',  ( -5.049401038298153566, 19.05341960407611168, 35.20724293864768839 ) ) ;
#12817=CARTESIAN_POINT ( 'NONE',  ( -12.06949235617756955, 12.14591786802309770, 35.62390960531437401 ) ) ;
#12818=CARTESIAN_POINT ( 'NONE',  ( 8.314922557960818139, 14.29746914071049879, 64.58224293864769550 ) ) ;
#12819=VECTOR ( 'NONE', #47624, 1000.000000000000000 ) ;
#12820=CARTESIAN_POINT ( 'NONE',  ( 9.564922557960805705, 16.46253265017160317, 59.58224293864769550 ) ) ;
#12821=CARTESIAN_POINT ( 'NONE',  ( 5.719274019375673035, 21.55341960407619339, 107.2927570613523471 ) ) ;
#12822=CARTESIAN_POINT ( 'NONE',  ( 5.823673210054444382, -21.52544592524334988, 20.20942372801900788 ) ) ;
#12823=CARTESIAN_POINT ( 'NONE',  ( -19.03943276465977164, 0.05219959533909376836, 76.24890960531435269 ) ) ;
#12824=CARTESIAN_POINT ( 'NONE',  ( -5.823673210054431948, 21.52544592524334988, 92.70942372801901854 ) ) ;
#12825=CARTESIAN_POINT ( 'NONE',  ( 0.05219959533934541429, -16.53943276465976808, 50.00109039468568994 ) ) ;
#12826=CARTESIAN_POINT ( 'NONE',  ( 12.14591786802327356, -12.06949235617739191, 30.62609039468567929 ) ) ;
#12827=CARTESIAN_POINT ( 'NONE',  ( -12.14591786802309592, -12.06949235617757132, 91.87390960531436690 ) ) ;
#12828=CARTESIAN_POINT ( 'NONE',  ( 18.67979575497194134, -10.72451020669871369, 95.83442372801903275 ) ) ;
#12829=CARTESIAN_POINT ( 'NONE',  ( 0.05219959533910956823, 16.53943276465976808, 34.99890960531435979 ) ) ;
#12830=CARTESIAN_POINT ( 'NONE',  ( -16.51473224551069308, -9.474510206698971260, 26.66557627198103120 ) ) ;
#12831=CARTESIAN_POINT ( 'NONE',  ( -8.314922557961024197, 14.29746914071037800, 52.91775706135235424 ) ) ;
#12832=CARTESIAN_POINT ( 'NONE',  ( -12.06949235617756955, 12.14591786802309770, 55.62390960531436690 ) ) ;
#12833=CARTESIAN_POINT ( 'NONE',  ( 4.483927247898790824, -16.52544592524335698, 95.20942372801903275 ) ) ;
#12834=CARTESIAN_POINT ( 'NONE',  ( -19.03943276465977164, 0.05219959533909376836, 111.2489096053143669 ) ) ;
#12835=CARTESIAN_POINT ( 'NONE',  ( -5.049401038298153566, 19.05341960407611168, 115.2072429386477097 ) ) ;
#12836=CARTESIAN_POINT ( 'NONE',  ( -15.80617190586768217, 15.72974639402176855, 113.1260903946856899 ) ) ;
#12837=CARTESIAN_POINT ( 'NONE',  ( -16.53943276465976808, 0.05219959533911058130, 91.24890960531436690 ) ) ;
#12838=CARTESIAN_POINT ( 'NONE',  ( -13.97604488694527625, -13.89961937509977652, 96.87390960531433848 ) ) ;
#12840=CARTESIAN_POINT ( 'NONE',  ( 14.34966873604972726, -8.224510206698740333, 45.83442372801901854 ) ) ;
#12841=CARTESIAN_POINT ( 'NONE',  ( -5.153800228976328057, -19.02544592524343514, 37.29057627198102409 ) ) ;
#12842=CARTESIAN_POINT ( 'NONE',  ( -4.483927247898782831, 16.52544592524335698, 42.70942372801901854 ) ) ;
#12844=CARTESIAN_POINT ( 'NONE',  ( 16.46253265017146816, 9.564922557961045513, 46.66775706135233293 ) ) ;
#12845=CARTESIAN_POINT ( 'NONE',  ( 13.89961937509977652, -13.97604488694527269, 43.12390960531434558 ) ) ;
#12846=CARTESIAN_POINT ( 'NONE',  ( 12.14591786802327356, -12.06949235617739191, 80.62609039468567573 ) ) ;
#12847=CARTESIAN_POINT ( 'NONE',  ( -16.51473224551082808, 9.474510206698731452, 83.33442372801899012 ) ) ;
#12848=CARTESIAN_POINT ( 'NONE',  ( 19.03943276465977164, 0.05219959533936151252, 31.25109039468566863 ) ) ;
#12849=CARTESIAN_POINT ( 'NONE',  ( -9.474510206698964154, 16.51473224551069663, 55.41557627198103120 ) ) ;
#12850=CARTESIAN_POINT ( 'NONE',  ( 14.34966873604960469, 8.224510206698951720, 94.16557627198103830 ) ) ;
#12853=CARTESIAN_POINT ( 'NONE',  ( -0.05219959533936034679, 19.03943276465977164, 72.50109039468566152 ) ) ;
#12854=CARTESIAN_POINT ( 'NONE',  ( -21.53943276465977519, 0.05219959533907696930, 66.24890960531436690 ) ) ;
#12855=CARTESIAN_POINT ( 'NONE',  ( -5.049401038297874678, -19.05341960407617918, 29.79275706135232227 ) ) ;
#12856=CARTESIAN_POINT ( 'NONE',  ( -16.46253265017160317, 9.564922557960807481, 110.8322429386476955 ) ) ;
#12857=CARTESIAN_POINT ( 'NONE',  ( 10.72451020669898902, -18.67979575497178502, 77.91557627198102409 ) ) ;
#12858=CARTESIAN_POINT ( 'NONE',  ( -16.20579543436679160, 7.371946100355091680, 84.43479165828125588 ) ) ;
#12859=CARTESIAN_POINT ( 'NONE',  ( -19.05341960407617563, 5.049401038297882671, 103.5427570613523329 ) ) ;
#12860=CARTESIAN_POINT ( 'NONE',  ( -19.35633801406906684, 5.499999999999783284, 59.13373818172765084 ) ) ;
#12861=CARTESIAN_POINT ( 'NONE',  ( -4.379528057220086978, -16.55341960407618274, 29.79275706135234358 ) ) ;
#12862=CARTESIAN_POINT ( 'NONE',  ( -16.46253265017160317, 9.564922557960807481, 30.83224293864769550 ) ) ;
#12863=CARTESIAN_POINT ( 'NONE',  ( -0.05219959533909027116, -19.03943276465977164, 112.4989096053143669 ) ) ;
#12864=CARTESIAN_POINT ( 'NONE',  ( -21.52544592524343514, 5.823673210054127303, 96.04057627198102409 ) ) ;
#12865=CARTESIAN_POINT ( 'NONE',  ( 15.80617190586769283, -15.72974639402175789, 65.62609039468568994 ) ) ;
#12866=CARTESIAN_POINT ( 'NONE',  ( -0.05219959533936034679, 19.03943276465977164, 107.5010903946856615 ) ) ;
#12867=CARTESIAN_POINT ( 'NONE',  ( 0.05219959533937995610, -21.53943276465977519, 105.0010903946856757 ) ) ;
#12868=CARTESIAN_POINT ( 'NONE',  ( 16.53943276465976808, 0.05219959533934440121, 106.2510903946856757 ) ) ;
#12869=CARTESIAN_POINT ( 'NONE',  ( 0.05219959533907565091, 21.53943276465977519, 104.9989096053143669 ) ) ;
#12870=CARTESIAN_POINT ( 'NONE',  ( 16.52544592524342804, -4.483927247898539470, 43.54057627198103830 ) ) ;
#12871=CARTESIAN_POINT ( 'NONE',  ( -5.049401038297874678, -19.05341960407617918, 84.79275706135233293 ) ) ;
#12872=CARTESIAN_POINT ( 'NONE',  ( 19.02544592524334988, 5.153800228976608722, 56.45942372801898301 ) ) ;
#12873=CARTESIAN_POINT ( 'NONE',  ( 0.05219959533937995610, -21.53943276465977519, 60.00109039468568284 ) ) ;
#12874=CARTESIAN_POINT ( 'NONE',  ( -19.02544592524334988, -5.153800228976617603, 38.95942372801900433 ) ) ;
#12875=CARTESIAN_POINT ( 'NONE',  ( -14.29746914071049879, 8.314922557960819915, 100.8322429386477097 ) ) ;
#12876=CARTESIAN_POINT ( 'NONE',  ( 21.55341960407610458, 5.719274019375980345, 48.95724293864770971 ) ) ;
#12877=CARTESIAN_POINT ( 'NONE',  ( -16.52544592524342804, 4.483927247898546575, 41.04057627198103120 ) ) ;
#12878=CARTESIAN_POINT ( 'NONE',  ( 15.72974639402176855, 15.80617190586768217, 101.8760903946857042 ) ) ;
#12879=CARTESIAN_POINT ( 'NONE',  ( -14.34966873604972548, 8.224510206698743886, 78.33442372801901854 ) ) ;
#12880=CARTESIAN_POINT ( 'NONE',  ( 12.06949235617757843, -12.14591786802309237, 28.12390960531435979 ) ) ;
#12881=CARTESIAN_POINT ( 'NONE',  ( 15.72974639402176855, 15.80617190586768217, 56.87609039468568994 ) ) ;
#12882=CARTESIAN_POINT ( 'NONE',  ( -15.80617190586768217, 15.72974639402176855, 63.12609039468568994 ) ) ;
#12883=CARTESIAN_POINT ( 'NONE',  ( 18.67979575497178502, 10.72451020669898547, 64.16557627198102409 ) ) ;
#12885=CARTESIAN_POINT ( 'NONE',  ( -5.153800228976328057, -19.02544592524343514, 22.29057627198102765 ) ) ;
#12886=CARTESIAN_POINT ( 'NONE',  ( 0.05219959533937995610, -21.53943276465977519, 50.00109039468568994 ) ) ;
#12887=CARTESIAN_POINT ( 'NONE',  ( -14.29746914071049879, 8.314922557960819915, 115.8322429386477097 ) ) ;
#12888=CARTESIAN_POINT ( 'NONE',  ( 19.03943276465977164, -0.05219959533909143690, 43.74890960531435979 ) ) ;
#12889=CARTESIAN_POINT ( 'NONE',  ( 12.06949235617757843, -12.14591786802309237, 73.12390960531436690 ) ) ;
#12890=CARTESIAN_POINT ( 'NONE',  ( -19.02544592524342804, 5.153800228976336051, 91.04057627198100988 ) ) ;
#12891=CARTESIAN_POINT ( 'NONE',  ( -16.53943276465976808, -0.05219959533934237506, 113.7510903946856757 ) ) ;
#12892=CARTESIAN_POINT ( 'NONE',  ( -8.314922557960811034, -14.29746914071050412, 97.08224293864770971 ) ) ;
#12893=CARTESIAN_POINT ( 'NONE',  ( 0.05219959533907565091, 21.53943276465977519, 74.99890960531435269 ) ) ;
#12894=CARTESIAN_POINT ( 'NONE',  ( 0.05219959533907565091, 21.53943276465977519, 109.9989096053143527 ) ) ;
#12895=CARTESIAN_POINT ( 'NONE',  ( -19.05341960407611168, -5.049401038298163336, 66.45724293864769550 ) ) ;
#12896=CARTESIAN_POINT ( 'NONE',  ( -14.29746914071037622, -8.314922557961029526, 19.16775706135234714 ) ) ;
#12897=CARTESIAN_POINT ( 'NONE',  ( -21.53943276465977519, 0.05219959533907696930, 51.24890960531436690 ) ) ;
#12898=CARTESIAN_POINT ( 'NONE',  ( 15.72974639402176855, 15.80617190586768217, 76.87609039468567573 ) ) ;
#12899=CARTESIAN_POINT ( 'NONE',  ( -16.51473224551069308, -9.474510206698971260, 61.66557627198103120 ) ) ;
#12900=CARTESIAN_POINT ( 'NONE',  ( 19.03943276465977164, -0.05219959533909143690, 103.7489096053143669 ) ) ;
#12901=CARTESIAN_POINT ( 'NONE',  ( -14.29746914071037622, -8.314922557961029526, 79.16775706135234714 ) ) ;
#12902=CARTESIAN_POINT ( 'NONE',  ( 21.53943276465977519, 0.05219959533937863772, 51.25109039468568994 ) ) ;
#12903=CARTESIAN_POINT ( 'NONE',  ( 5.823673210054444382, -21.52544592524334988, 95.20942372801903275 ) ) ;
#12904=CARTESIAN_POINT ( 'NONE',  ( 21.52544592524344225, -5.823673210054117533, 113.5405762719810383 ) ) ;
#12905=CARTESIAN_POINT ( 'NONE',  ( 5.823673210054125526, 21.52544592524343514, 89.79057627198103830 ) ) ;
#12906=CARTESIAN_POINT ( 'NONE',  ( 13.89961937509957401, 13.97604488694547697, 41.87609039468566152 ) ) ;
#12907=CARTESIAN_POINT ( 'NONE',  ( -18.67979575497178146, -10.72451020669898902, 36.66557627198103120 ) ) ;
#12908=CARTESIAN_POINT ( 'NONE',  ( -9.474510206698964154, 16.51473224551069663, 75.41557627198103830 ) ) ;
#12909=CARTESIAN_POINT ( 'NONE',  ( -16.53943276465976808, 0.05219959533911058130, 31.24890960531435979 ) ) ;
#12910=CARTESIAN_POINT ( 'NONE',  ( -16.38665767535054840, 7.295008042176032603, 65.26400864214548392 ) ) ;
#12912=CARTESIAN_POINT ( 'NONE',  ( -16.46253265017146816, -9.564922557961047289, 99.16775706135233293 ) ) ;
#12913=CARTESIAN_POINT ( 'NONE',  ( -18.67979575497178146, -10.72451020669898902, 66.66557627198102409 ) ) ;
#12914=CARTESIAN_POINT ( 'NONE',  ( -14.29746914071049879, 8.314922557960819915, 50.83224293864770971 ) ) ;
#12915=CARTESIAN_POINT ( 'NONE',  ( 4.379528057220092307, 16.55341960407617563, 37.29275706135235424 ) ) ;
#12916=CARTESIAN_POINT ( 'NONE',  ( 16.46253265017160672, -9.564922557960803928, 48.33224293864769550 ) ) ;
#12917=CARTESIAN_POINT ( 'NONE',  ( -18.62759615963270932, 10.81492255796079327, 110.8322429386476955 ) ) ;
#12918=CARTESIAN_POINT ( 'NONE',  ( -0.05219959533936034679, 19.03943276465977164, 87.50109039468567573 ) ) ;
#12919=CARTESIAN_POINT ( 'NONE',  ( -16.46253265017160317, 9.564922557960807481, 75.83224293864769550 ) ) ;
#12920=CARTESIAN_POINT ( 'NONE',  ( -12.14591786802309592, -12.06949235617757132, 91.87390960531436690 ) ) ;
#12921=CARTESIAN_POINT ( 'NONE',  ( 9.474510206698971260, -16.51473224551069308, 67.91557627198102409 ) ) ;
#12922=CARTESIAN_POINT ( 'NONE',  ( -21.52544592524343514, 5.823673210054127303, 81.04057627198102409 ) ) ;
#12923=CARTESIAN_POINT ( 'NONE',  ( 19.05341960407611168, 5.049401038298154454, 28.95724293864769550 ) ) ;
#12925=CARTESIAN_POINT ( 'NONE',  ( -14.29746914071049879, 8.314922557960819915, 55.83224293864770260 ) ) ;
#12926=CARTESIAN_POINT ( 'NONE',  ( -5.049401038298153566, 19.05341960407611168, 95.20724293864770971 ) ) ;
#12928=CARTESIAN_POINT ( 'NONE',  ( -0.05219959533936034679, 19.03943276465977164, 52.50109039468566863 ) ) ;
#12929=CARTESIAN_POINT ( 'NONE',  ( 0.05219959533934541429, -16.53943276465976808, 65.00109039468568994 ) ) ;
#12930=CARTESIAN_POINT ( 'NONE',  ( -5.719274019375978568, 21.55341960407610458, 80.20724293864769550 ) ) ;
#12931=CARTESIAN_POINT ( 'NONE',  ( 16.46253265017146816, 9.564922557961045513, 41.66775706135234003 ) ) ;
#12932=CARTESIAN_POINT ( 'NONE',  ( 9.474510206698971260, -16.51473224551069308, 87.91557627198102409 ) ) ;
#12934=CARTESIAN_POINT ( 'NONE',  ( 18.62759615963271287, -10.81492255796078972, 23.33224293864769194 ) ) ;
#12935=CARTESIAN_POINT ( 'NONE',  ( 5.049401038298161559, -19.05341960407611168, 72.70724293864768129 ) ) ;
#12936=CARTESIAN_POINT ( 'NONE',  ( 10.81492255796106328, -18.62759615963255655, 55.41775706135234714 ) ) ;
#12937=CARTESIAN_POINT ( 'NONE',  ( -16.51473224551069308, -9.474510206698971260, 21.66557627198102765 ) ) ;
#12938=CARTESIAN_POINT ( 'NONE',  ( 18.67979575497178502, 10.72451020669898547, 114.1655762719810383 ) ) ;
#12939=CARTESIAN_POINT ( 'NONE',  ( -19.05341960407611168, -5.049401038298163336, 91.45724293864766707 ) ) ;
#12940=ORIENTED_EDGE ( 'NONE', *, *, #141236, .F. ) ;
#12941=CARTESIAN_POINT ( 'NONE',  ( 21.55341960407619695, -5.719274019375665929, 46.04275706135234714 ) ) ;
#12943=CARTESIAN_POINT ( 'NONE',  ( 9.474510206698971260, -16.51473224551069308, 102.9155762719810241 ) ) ;
#12944=B_SPLINE_CURVE_WITH_KNOTS ( 'NONE', 3,
 ( #12991, #133326, #167659, #26173, #74654, #195017, #164679, #87814 ),
 .UNSPECIFIED., .F., .F.,
 ( 4, 2, 2, 4 ),
 ( 0.000000000000000000, 0.0004423531491111659989, 0.0008847062982223319978, 0.001769412596444684812 ),
 .UNSPECIFIED. ) ;
#12946=CARTESIAN_POINT ( 'NONE',  ( -18.62759615963270932, 10.81492255796079327, 105.8322429386476955 ) ) ;
#12947=CARTESIAN_POINT ( 'NONE',  ( 9.564922557960805705, 16.46253265017160317, 49.58224293864770260 ) ) ;
#12948=CARTESIAN_POINT ( 'NONE',  ( -16.52544592524335698, -4.483927247898792601, 28.95942372801902209 ) ) ;
#12950=CARTESIAN_POINT ( 'NONE',  ( -0.05219959533937732626, 21.53943276465977519, 107.5010903946856899 ) ) ;
#12951=CARTESIAN_POINT ( 'NONE',  ( -9.474510206698964154, 16.51473224551069663, 45.41557627198103120 ) ) ;
#12952=CARTESIAN_POINT ( 'NONE',  ( -15.80617190586768217, 15.72974639402176855, 93.12609039468568994 ) ) ;
#12953=CARTESIAN_POINT ( 'NONE',  ( 19.05341960407611168, 5.049401038298154454, 88.95724293864769550 ) ) ;
#12954=CARTESIAN_POINT ( 'NONE',  ( 18.67979575497194134, -10.72451020669871369, 55.83442372801901854 ) ) ;
#12957=CARTESIAN_POINT ( 'NONE',  ( 19.05341960407611168, 5.049401038298154454, 98.95724293864766707 ) ) ;
#12958=CARTESIAN_POINT ( 'NONE',  ( -17.49999999999998224, 3.805241302050397678, 30.37352472782594504 ) ) ;
#12959=CARTESIAN_POINT ( 'NONE',  ( -8.314922557961024197, 14.29746914071037800, 52.91775706135235424 ) ) ;
#12960=CARTESIAN_POINT ( 'NONE',  ( -8.314922557961024197, 14.29746914071037800, 62.91775706135236135 ) ) ;
#12961=CARTESIAN_POINT ( 'NONE',  ( 18.67979575497194134, -10.72451020669871369, 55.83442372801901854 ) ) ;
#12962=CARTESIAN_POINT ( 'NONE',  ( -21.55341960407619339, 5.719274019375674811, 83.54275706135234714 ) ) ;
#12964=CARTESIAN_POINT ( 'NONE',  ( 0.05219959533934541429, -16.53943276465976808, 30.00109039468568284 ) ) ;
#12965=CARTESIAN_POINT ( 'NONE',  ( -16.46253265017160317, 9.564922557960807481, 75.83224293864769550 ) ) ;
#12966=CARTESIAN_POINT ( 'NONE',  ( -5.153800228976328057, -19.02544592524343514, 102.2905762719810383 ) ) ;
#12968=CARTESIAN_POINT ( 'NONE',  ( -16.46253265017160317, 9.564922557960807481, 115.8322429386477097 ) ) ;
#12969=CARTESIAN_POINT ( 'NONE',  ( 19.02544592524343514, -5.153800228976328945, 23.54057627198102054 ) ) ;
#12970=CARTESIAN_POINT ( 'NONE',  ( 15.80617190586746368, 15.72974639402197994, 29.37390960531435269 ) ) ;
#12971=CARTESIAN_POINT ( 'NONE',  ( 12.06949235617739724, 12.14591786802326823, 86.87609039468568994 ) ) ;
#12972=CARTESIAN_POINT ( 'NONE',  ( -14.34966873604960291, -8.224510206698953496, 86.66557627198102409 ) ) ;
#12973=CARTESIAN_POINT ( 'NONE',  ( -5.153800228976328057, -19.02544592524343514, 62.29057627198100988 ) ) ;
#12974=CARTESIAN_POINT ( 'NONE',  ( 15.72974639402176855, 15.80617190586768217, 86.87609039468568994 ) ) ;
#12976=CARTESIAN_POINT ( 'NONE',  ( -0.05219959533934338120, 16.53943276465976808, 27.50109039468567929 ) ) ;
#12977=CARTESIAN_POINT ( 'NONE',  ( 16.55341960407611168, 4.379528057220329451, 73.95724293864769550 ) ) ;
#12978=CARTESIAN_POINT ( 'NONE',  ( -18.62759615963255300, -10.81492255796106328, 24.16775706135235424 ) ) ;
#12979=CARTESIAN_POINT ( 'NONE',  ( -15.72974639402197994, 15.80617190586746368, 75.62390960531439532 ) ) ;
#12980=CARTESIAN_POINT ( 'NONE',  ( -0.05219959533936034679, 19.03943276465977164, 42.50109039468566152 ) ) ;
#12982=CARTESIAN_POINT ( 'NONE',  ( 16.46253265017160672, -9.564922557960803928, 83.33224293864768129 ) ) ;
#12983=CARTESIAN_POINT ( 'NONE',  ( 12.06949235617757843, -12.14591786802309237, 53.12390960531436690 ) ) ;
#12985=CARTESIAN_POINT ( 'NONE',  ( -4.379528057220328563, 16.55341960407611168, 40.20724293864769550 ) ) ;
#12986=CARTESIAN_POINT ( 'NONE',  ( -16.55341960407611168, -4.379528057220339221, 21.45724293864769550 ) ) ;
#12987=CARTESIAN_POINT ( 'NONE',  ( -5.049401038297874678, -19.05341960407617918, 64.79275706135233293 ) ) ;
#12988=CARTESIAN_POINT ( 'NONE',  ( 18.89770734986053569, 5.499999999999910294, 51.60214472496640781 ) ) ;
#12989=CARTESIAN_POINT ( 'NONE',  ( -19.03943276465977164, 0.05219959533909376836, 101.2489096053143669 ) ) ;
#12990=CARTESIAN_POINT ( 'NONE',  ( 12.14591786802309770, 12.06949235617756955, 69.37390960531436690 ) ) ;
#12991=CARTESIAN_POINT ( 'NONE',  ( 19.50973618000807619, -5.499999999999992895, 37.50000000000000000 ) ) ;
#12992=CARTESIAN_POINT ( 'NONE',  ( -0.05219959533909027116, -19.03943276465977164, 27.49890960531435624 ) ) ;
#12993=CARTESIAN_POINT ( 'NONE',  ( -5.823673210054116645, -21.52544592524344225, 42.29057627198103120 ) ) ;
#12994=CARTESIAN_POINT ( 'NONE',  ( 15.72974639402199770, -15.80617190586745480, 73.12390960531436690 ) ) ;
#12995=CARTESIAN_POINT ( 'NONE',  ( -4.379528057220328563, 16.55341960407611168, 110.2072429386477239 ) ) ;
#12996=CARTESIAN_POINT ( 'NONE',  ( 8.314922557961029526, -14.29746914071037800, 65.41775706135234714 ) ) ;
#12997=CARTESIAN_POINT ( 'NONE',  ( 19.03943276465977164, -0.05219959533909143690, 43.74890960531435979 ) ) ;
#12999=CARTESIAN_POINT ( 'NONE',  ( -21.53943276465977519, -0.05219959533937600094, 53.75109039468568994 ) ) ;
#13000=CARTESIAN_POINT ( 'NONE',  ( -14.29746914071049879, 8.314922557960819915, 110.8322429386476955 ) ) ;
#13001=CARTESIAN_POINT ( 'NONE',  ( 16.29526858892872454, -7.335722546920260712, 36.70329402199793378 ) ) ;
#13003=CARTESIAN_POINT ( 'NONE',  ( 5.823673210054125526, 21.52544592524343514, 34.79057627198103120 ) ) ;
#13005=CARTESIAN_POINT ( 'NONE',  ( 5.719274019375673035, 21.55341960407619339, 72.29275706135236135 ) ) ;
#13006=CARTESIAN_POINT ( 'NONE',  ( 4.379528057220092307, 16.55341960407617563, 62.29275706135236845 ) ) ;
#13007=CARTESIAN_POINT ( 'NONE',  ( 14.34966873604960469, 8.224510206698951720, 39.16557627198102409 ) ) ;
#13008=CARTESIAN_POINT ( 'NONE',  ( 5.823673210054125526, 21.52544592524343514, 69.79057627198102409 ) ) ;
#13009=CARTESIAN_POINT ( 'NONE',  ( -15.72974639402197994, 15.80617190586746368, 65.62390960531436690 ) ) ;
#13010=CARTESIAN_POINT ( 'NONE',  ( 30.00000000000000000, 5.499999999999992895, 102.5000000000000142 ) ) ;
#13011=CARTESIAN_POINT ( 'NONE',  ( -16.46253265017146816, -9.564922557961047289, 79.16775706135234714 ) ) ;
#13012=CARTESIAN_POINT ( 'NONE',  ( -15.72974639402197994, 15.80617190586746368, 25.62390960531435624 ) ) ;
#13013=CARTESIAN_POINT ( 'NONE',  ( -5.049401038298153566, 19.05341960407611168, 55.20724293864769550 ) ) ;
#13014=CARTESIAN_POINT ( 'NONE',  ( 5.153800228976335163, 19.02544592524342804, 24.79057627198102765 ) ) ;
#13015=CARTESIAN_POINT ( 'NONE',  ( 9.474510206698971260, -16.51473224551069308, 107.9155762719810383 ) ) ;
#13017=CARTESIAN_POINT ( 'NONE',  ( 8.224510206698742110, 14.34966873604972548, 72.08442372801899012 ) ) ;
#13018=CARTESIAN_POINT ( 'NONE',  ( 18.62759615963271287, -10.81492255796078972, 108.3322429386477097 ) ) ;
#13019=CARTESIAN_POINT ( 'NONE',  ( -16.46253265017160317, 9.564922557960807481, 55.83224293864769550 ) ) ;
#13020=CARTESIAN_POINT ( 'NONE',  ( -18.67979575497193778, 10.72451020669871902, 38.33442372801900433 ) ) ;
#13021=CARTESIAN_POINT ( 'NONE',  ( 19.02544592524343514, -5.153800228976328945, 93.54057627198102409 ) ) ;
#13024=CARTESIAN_POINT ( 'NONE',  ( 10.72451020669871369, 18.67979575497193778, 32.08442372801901854 ) ) ;
#13025=CARTESIAN_POINT ( 'NONE',  ( 13.89961937509977652, -13.97604488694527269, 108.1239096053143669 ) ) ;
#13026=CARTESIAN_POINT ( 'NONE',  ( 19.02544592524334988, 5.153800228976608722, 86.45942372801900433 ) ) ;
#13027=CARTESIAN_POINT ( 'NONE',  ( 19.02544592524334988, 5.153800228976608722, 41.45942372801900433 ) ) ;
#13028=CARTESIAN_POINT ( 'NONE',  ( 5.823673210054125526, 21.52544592524343514, 104.7905762719810241 ) ) ;
#13029=CARTESIAN_POINT ( 'NONE',  ( -16.51473224551082808, 9.474510206698731452, 28.33442372801900433 ) ) ;
#13030=CARTESIAN_POINT ( 'NONE',  ( 0.05219959533936267826, -19.03943276465977164, 55.00109039468566863 ) ) ;
#13031=CARTESIAN_POINT ( 'NONE',  ( 8.224510206698742110, 14.34966873604972548, 92.08442372801901854 ) ) ;
#13034=CARTESIAN_POINT ( 'NONE',  ( -16.51473224551069308, -9.474510206698971260, 66.66557627198102409 ) ) ;
#13035=CARTESIAN_POINT ( 'NONE',  ( 0.05219959533937995610, -21.53943276465977519, 85.00109039468568994 ) ) ;
#13036=CARTESIAN_POINT ( 'NONE',  ( 15.80617190586769283, -15.72974639402175789, 75.62609039468567573 ) ) ;
#13038=CARTESIAN_POINT ( 'NONE',  ( 13.89961937509977652, -13.97604488694527269, 88.12390960531438111 ) ) ;
#13039=CARTESIAN_POINT ( 'NONE',  ( 18.67979575497194134, -10.72451020669871369, 55.83442372801901854 ) ) ;
#13040=CARTESIAN_POINT ( 'NONE',  ( -0.05219959533936034679, 19.03943276465977164, 102.5010903946856757 ) ) ;
#13041=CARTESIAN_POINT ( 'NONE',  ( -0.05219959533909027116, -19.03943276465977164, 67.49890960531436690 ) ) ;
#13042=CARTESIAN_POINT ( 'NONE',  ( -9.564922557960796823, -16.46253265017161027, 107.0822429386476955 ) ) ;
#13043=CARTESIAN_POINT ( 'NONE',  ( -19.05341960407611168, -5.049401038298163336, 76.45724293864769550 ) ) ;
#13044=CARTESIAN_POINT ( 'NONE',  ( 17.50000000000000711, -3.404445912590670087, 22.03715329543141621 ) ) ;
#13045=CARTESIAN_POINT ( 'NONE',  ( -19.05341960407611168, -5.049401038298163336, 71.45724293864766707 ) ) ;
#13046=CARTESIAN_POINT ( 'NONE',  ( 5.049401038298161559, -19.05341960407611168, 57.70724293864769550 ) ) ;
#13047=CARTESIAN_POINT ( 'NONE',  ( -15.72974639402197994, 15.80617190586746368, 95.62390960531436690 ) ) ;
#13048=CARTESIAN_POINT ( 'NONE',  ( 16.55341960407618274, -4.379528057220086978, 81.04275706135236135 ) ) ;
#13050=CARTESIAN_POINT ( 'NONE',  ( -5.049401038297874678, -19.05341960407617918, 44.79275706135232582 ) ) ;
#13051=CARTESIAN_POINT ( 'NONE',  ( -5.153800228976328057, -19.02544592524343514, 77.29057627198099567 ) ) ;
#13052=CARTESIAN_POINT ( 'NONE',  ( -8.314922557960811034, -14.29746914071050412, 77.08224293864769550 ) ) ;
#13053=CARTESIAN_POINT ( 'NONE',  ( -4.379528057220328563, 16.55341960407611168, 105.2072429386477097 ) ) ;
#13054=CARTESIAN_POINT ( 'NONE',  ( -18.62759615963270932, 10.81492255796079327, 25.83224293864769194 ) ) ;
#13055=CARTESIAN_POINT ( 'NONE',  ( 13.97604488694527802, 13.89961937509977652, 104.3739096053143385 ) ) ;
#13056=CARTESIAN_POINT ( 'NONE',  ( 4.483927247898545687, 16.52544592524342804, 74.79057627198105251 ) ) ;
#13058=CARTESIAN_POINT ( 'NONE',  ( 19.05341960407617918, -5.049401038297876454, 26.04275706135233293 ) ) ;
#13059=CARTESIAN_POINT ( 'NONE',  ( -12.06949235617739369, -12.14591786802326823, 94.37609039468568994 ) ) ;
#13060=CARTESIAN_POINT ( 'NONE',  ( -0.05219959533909027116, -19.03943276465977164, 72.49890960531435269 ) ) ;
#13061=CARTESIAN_POINT ( 'NONE',  ( 21.55341960407619695, -5.719274019375665929, 51.04275706135234714 ) ) ;
#13062=CARTESIAN_POINT ( 'NONE',  ( -21.53943276465977519, 0.05219959533907696930, 41.24890960531435269 ) ) ;
#13063=CARTESIAN_POINT ( 'NONE',  ( 5.823673210054125526, 21.52544592524343514, 109.7905762719810383 ) ) ;
#13064=CARTESIAN_POINT ( 'NONE',  ( 5.823673210054125526, 21.52544592524343514, 69.79057627198102409 ) ) ;
#13065=CARTESIAN_POINT ( 'NONE',  ( 16.55341960407611168, 4.379528057220329451, 93.95724293864770971 ) ) ;
#13066=CARTESIAN_POINT ( 'NONE',  ( 5.049401038297881783, 19.05341960407617563, 52.29275706135234003 ) ) ;
#13067=CARTESIAN_POINT ( 'NONE',  ( -0.05219959533909027116, -19.03943276465977164, 32.49890960531435979 ) ) ;
#13068=CARTESIAN_POINT ( 'NONE',  ( -13.89961937509977652, 13.97604488694528158, 80.62390960531436690 ) ) ;
#13069=CARTESIAN_POINT ( 'NONE',  ( 0.05219959533909260263, 19.03943276465977164, 84.99890960531436690 ) ) ;
#13070=CARTESIAN_POINT ( 'NONE',  ( -14.34966873604960291, -8.224510206698953496, 101.6655762719810383 ) ) ;
#13071=CARTESIAN_POINT ( 'NONE',  ( -16.53943276465976808, 0.05219959533911058130, 31.24890960531435979 ) ) ;
#13072=CARTESIAN_POINT ( 'NONE',  ( -4.379528057220086978, -16.55341960407618274, 29.79275706135234358 ) ) ;
#13073=CARTESIAN_POINT ( 'NONE',  ( 10.81492255796106328, -18.62759615963255655, 90.41775706135236135 ) ) ;
#13074=CARTESIAN_POINT ( 'NONE',  ( 13.89961937509977652, -13.97604488694527269, 103.1239096053143527 ) ) ;
#13075=CARTESIAN_POINT ( 'NONE',  ( 21.53943276465977519, 0.05219959533937863772, 26.25109039468567573 ) ) ;
#13076=CARTESIAN_POINT ( 'NONE',  ( -16.46253265017160317, 9.564922557960807481, 45.83224293864769550 ) ) ;
#13077=CARTESIAN_POINT ( 'NONE',  ( -12.06949235617739369, -12.14591786802326823, 44.37609039468567573 ) ) ;
#13080=CARTESIAN_POINT ( 'NONE',  ( -5.153800228976607833, 19.02544592524334988, 102.7094237280189759 ) ) ;
#13081=CARTESIAN_POINT ( 'NONE',  ( -13.89961937509977652, 13.97604488694528158, 40.62390960531435979 ) ) ;
#13082=CARTESIAN_POINT ( 'NONE',  ( -14.29746914071049879, 8.314922557960819915, 100.8322429386477097 ) ) ;
#13083=CARTESIAN_POINT ( 'NONE',  ( 10.81492255796078972, 18.62759615963270932, 109.5822429386476955 ) ) ;
#13084=CARTESIAN_POINT ( 'NONE',  ( -9.564922557961040184, 16.46253265017147172, 77.91775706135234714 ) ) ;
#13085=CARTESIAN_POINT ( 'NONE',  ( 13.89961937509977652, -13.97604488694527269, 23.12390960531436335 ) ) ;
#13086=CARTESIAN_POINT ( 'NONE',  ( -16.51473224551069308, -9.474510206698971260, 86.66557627198102409 ) ) ;
#13087=CARTESIAN_POINT ( 'NONE',  ( 10.72451020669898902, -18.67979575497178502, 112.9155762719810383 ) ) ;
#13088=CARTESIAN_POINT ( 'NONE',  ( -13.97604488694527625, -13.89961937509977652, 21.87390960531435979 ) ) ;
#13089=CARTESIAN_POINT ( 'NONE',  ( -13.97604488694527625, -13.89961937509977652, 86.87390960531436690 ) ) ;
#13091=CARTESIAN_POINT ( 'NONE',  ( -13.97604488694527625, -13.89961937509977652, 81.87390960531436690 ) ) ;
#13092=CARTESIAN_POINT ( 'NONE',  ( -10.81492255796105439, 18.62759615963255655, 27.91775706135234358 ) ) ;
#13093=CARTESIAN_POINT ( 'NONE',  ( 4.379528057220339221, -16.55341960407611168, 77.70724293864770971 ) ) ;
#13094=CARTESIAN_POINT ( 'NONE',  ( 0.05219959533909260263, 19.03943276465977164, 94.99890960531436690 ) ) ;
#13095=CARTESIAN_POINT ( 'NONE',  ( 9.474510206698729675, 16.51473224551082808, 22.08442372801899722 ) ) ;
#13096=CARTESIAN_POINT ( 'NONE',  ( 4.483927247898790824, -16.52544592524335698, 45.20942372801901854 ) ) ;
#13097=( BOUNDED_SURFACE ( )  B_SPLINE_SURFACE ( 3, 2, ( 
 ( #84572, #146250, #42102, #148272, #102763, #176620, #9764, #116922, #178615, #7736, #72430, #69422, #71428, #118944, #131089, #103766, #68414, #192777, #115932, #177622, #39090, #40078, #153227, #184575, #121896, #77385, #137071, #92546, #107711, #139053, #183589, #198761, #108721, #59231, #45074, #46056, #120900, #28926, #90566, #170398, #91539, #89583, #73441, #43088, #169390, #154235, #14731, #533, #196788, #199749, #12759, #76392, #152248, #166445, #104755, #27941, #30899, #123869, #60227, #15725, #138068, #62205, #122887, #167430, #106732, #168406, #61215, #185567, #47061, #88582, #135112, #150280, #11777, #105743, #151269, #74424, #136090, #197765, #29901, #119925, #58256, #182600, #181610, #44085, #13733, #75400, #113676, #48060, #3521, #186588, #51029, #127852, #142033, #81338, #124889, #65197, #189557, #31889, #171399, #159184, #33874, #190543, #4499, #64214, #111705, #80360, #188562, #16717, #109716, #32886, #67187, #50041, #143021, #140041, #96516, #157220, #18713, #78367, #174382, #1530, #158206, #66190, #17718, #173391, #93543, #19696, #112690, #34861, #35852, #97498, #20679, #82334, #126856, #144024, #5505, #128844, #52017, #155228, #63209, #94536, #156218, #2533, #79376, #141047, #125880, #172383, #95533, #187580, #49048, #110703, #160198, #129831, #71193, #179391, #39843, #164211, #83341, #86352, #99514, #178379, #115698, #53007, #191530, #114686, #132857, #10527, #147033, #102528, #163199, #25708, #9527, #54025, #193546, #131862, #101509, #40854, #148038, #87353, #21688, #57029, #8517, #145018, #6499, #133864, #38858, #194545, #24703, #56016, #68179, #146017, #117694, #161195, #130850, #69184, #149039, #177387, #192542, #176381, #72190, #37855, #22691, #7500, #195555, #84338, #100515, #162194, #175370, #23692, #85340, #70195, #36838, #55019, #98503, #116689, #73206, #119695, #104521, #166202, #90327, #150031, #103530, #134877, #296, #106489, #107473, #136835, #118702, #196554, #152012, #58025, #137827, #14486, #28691, #168167, #11538, #13498, #76148, #180393, #181378, #45822, #120666, #77145, #91296, #151037, #198518, #167194, #75163, #165205, #42856, #27703, #153991, #59989, #29664, #26700, #183351, #43842, #105507, #88340, #60976, #89346, #44834, #152987, #12527, #121657, #41864, #199510, #122652, #184340, #169150, #30654, #92308, #15488, #138815, #74192, #135861, #197532, #59000, #182364, #156975, #110461, #82085, #32640, #95291, #157966, #94294, #2288, #63970, #143778, #64956, #62961, #46817, #16478, #19458, #65944, #126615, #50792, #170155, #173146, #186337, #188317, #125640, #139796, #78128, #1285, #81105, #97257, #33629, #189315, #49795, #112451, #96280, #140799, #80122, #18472, #111461, #127615, #34621, #174140, #108477, #61964, #141791, #31648, #93297, #20434, #187337, #142783, #4264, #35612, #172142, #154983, #124642, #123631, #48807, #17470, #158945, #3285, #185327, #47819, #109468, #171152, #155973, #79126, #66942, #100273, #25471, #147801, #190297, #23448, #145775, #99267, #115454, #128604, #83100, #86110, #7256, #84096, #131617, #177144, #37604, #51774, #191289, #159952, #179147, #52765, #116450, #163974, #38615, #85095, #114434, #87111, #98250, #69952, #68941, #40615, #161952, #67940, #22447, #36594, #101264, #178139, #146781, #9286, #8274, #113434, #21440, #39605, #176135, #130605, #5259, #24460, #162954, #70951, #193301, #54776, #192300, #132621, #194308, #55775, #160953, #53779, #117448, #102285, #175127, #144776, #6260, #129593, #31168, #107985, #26460, #186863, #183856, #139327, #45343, #169672, #78645, #124151, #125164, #185850, #91812, #153504, #56790, #171667, #118462, #15001, #180154, #170673, #41623, #103287, #164967, #184846, #806, #32161, #62479, #93818, #140320, #16000, #33156, #92818, #200020, #1810, #76661, #106995, #149788, #46330, #122166, #47337, #88103, #154504, #63488, #71945, #108992, #11292, #77658, #16991, #148797, #30168, #133616 ),
 ( #48332, #155498, #109987, #10287, #138340, #61488, #72964, #195309, #134633, #123158, #196318, #57787, #168668, #126151, #64484, #128125, #144291, #175643, #5781, #37117, #83612, #159457, #176655, #112960, #143289, #145290, #35134, #50320, #95807, #189827, #65466, #190812, #187847, #51299, #6773, #17995, #52287, #49316, #174653, #160470, #94815, #173667, #4775, #141317, #110976, #53283, #96786, #111975, #130106, #36118, #97770, #34148, #158475, #3789, #19963, #20953, #156493, #82610, #114962, #98776, #79648, #67455, #81605, #188835, #66463, #2806, #172661, #21961, #129113, #113944, #68452, #191802, #127129, #157493, #80632, #18986, #142309, #85617, #149304, #196819, #71460, #117970, #147304, #119955, #131124, #102795, #101790, #73473, #194815, #100778, #55286, #69457, #134140, #10798, #179661, #118977, #56288, #99785, #54294, #72467, #8793, #40112, #38132, #57300, #195829, #180660, #164481, #133125, #178649, #41131, #25975, #88616, #193821, #24975, #87618, #115966, #42136, #70463, #163478, #161471, #103797, #165477, #26973, #150313, #11809, #86621, #135146, #58286, #22960, #116958, #148304, #84608, #146287, #9798, #7774, #192812, #177654, #39123, #162461, #23962, #132128, #13765, #169426, #75433, #199782, #108752, #154267, #155259, #15758, #121930, #183625, #89614, #1564, #151303, #45107, #12792, #564, #74457, #136123, #197799, #14764, #30931, #62235, #92579, #123903, #170428, #46090, #63239, #61250, #29935, #31920, #106764, #137107, #182633, #76425, #152281, #77417, #59265, #138101, #93574, #104788, #139089, #120934, #122921, #47091, #181641, #60259, #91574, #27975, #44117, #140073, #168439, #198793, #16749, #184609, #107745, #105776, #153263, #90599, #185602, #78397, #43120, #166476, #167463, #28958, #109744, #143049, #65225, #18742, #34890, #48088, #2562, #5535, #126885, #3547, #51056, #96546, #157248, #171428, #110735, #79406, #98534, #172416, #35880, #83371, #158233, #4528, #33904, #6529, #17750, #189584, #188591, #160227, #81365, #187609, #142061, #156248, #20709, #97527, #66220, #67214, #50072, #144053, #127880, #112718, #32915, #95561, #174411, #49078, #80389, #111733, #159214, #173420, #19724, #94570, #128872, #141077, #82365, #190572, #64244, #125911, #52048, #113704, #175401, #36869, #21718, #145048, #124919, #186616, #57057, #86381, #150061, #84368, #39872, #22720, #87382, #164241, #178408, #117723, #161226, #101539, #25736, #68209, #7529, #195585, #70224, #26728, #40883, #100544, #148065, #116719, #24731, #53038, #146045, #69214, #103559, #9556, #179418, #176410, #132885, #193576, #55048, #114718, #10555, #37886, #194574, #102556, #54055, #71222, #129861, #56044, #149067, #72219, #133894, #118732, #180420, #41893, #163231, #165234, #88367, #191559, #99544, #130882, #192571, #115729, #177416, #38887, #162223, #23722, #85371, #8547, #131892, #147064, #14515, #12552, #196580, #166229, #107501, #15515, #76176, #322, #119721, #122678, #135886, #137856, #152040, #89372, #27729, #151061, #169177, #46844, #183381, #31677, #106518, #29693, #136862, #90355, #91324, #168196, #199536, #77172, #184367, #123656, #58050, #93326, #44863, #181404, #42882, #170183, #75191, #45848, #92334, #61990, #61006, #11566, #153016, #60018, #185353, #13525, #167220, #74218, #30683, #182391, #154020, #104547, #138842, #108504, #134903, #73232, #197558, #59025, #120692, #43869, #198548, #121685, #105534, #28718, #113460, #95314, #110485, #190324, #34646, #157991, #94321, #156999, #63995, #18497, #173170, #16507, #49821, #175154, #97284, #139823, #96305, #80145, #48832, #64982, #78155, #32668, #35638, #141816, #33653, #81128, #126640, #187363, #1312, #140824, #109498, #128630, #2313, #65970, #36621, #188342, #19483, #125665, #155011, #47845, #142809, #3309, #51801, #111485, #17496, #172168, #186366, #50818, #112475, #4289, #189340, #127640, #62991, #171180, #174168, #158971, #20463, #124669, #82113, #143804 ),
 ( #155999, #79153, #5287, #66970, #176161, #133644, #130632, #86137, #192326, #116477, #25496, #70979, #71970, #132647, #38643, #100300, #6286, #118489, #67965, #161978, #129619, #117475, #191314, #52791, #114459, #131646, #147828, #179173, #37631, #99294, #56815, #23474, #40641, #101291, #162981, #83127, #68968, #24486, #22474, #53807, #115482, #194335, #177170, #85123, #160980, #102310, #144803, #9314, #146807, #84122, #145801, #7284, #8301, #69978, #193328, #54802, #178166, #180180, #55803, #87139, #39631, #98278, #164000, #148823, #10313, #195335, #159979, #21465, #91092, #134658, #74958, #199299, #123422, #181166, #168936, #43630, #84, #14271, #73981, #121447, #90118, #198301, #26487, #196344, #57812, #76933, #59778, #152780, #149813, #106276, #166981, #28484, #88129, #184130, #11319, #167961, #75940, #27488, #183139, #41649, #29460, #137615, #44623, #122438, #107265, #60766, #45613, #136620, #30443, #151802, #92089, #153778, #15273, #138602, #13293, #61754, #12316, #103313, #164993, #135650, #182146, #105293, #72989, #119484, #42643, #104305, #165988, #89131, #150819, #197321, #58784, #120453, #64756, #124431, #18267, #78916, #139590, #77923, #1076, #49587, #65739, #48604, #189116, #110256, #95085, #2083, #17263, #156773, #171937, #79920, #34420, #126418, #142582, #108266, #50589, #33426, #154774, #141593, #111250, #185115, #62751, #80905, #63763, #46605, #172941, #140593, #3080, #188115, #96079, #93090, #186128, #47607, #169945, #157768, #19259, #109261, #4061, #127407, #31436, #170940, #16271, #125436, #32432, #94086, #155765, #187132, #165644, #153440, #91745, #122102, #46265, #31103, #30105, #61422, #198961, #154439, #13933, #169605, #184779, #15933, #60428, #75600, #185782, #136290, #183792, #123093, #197966, #105944, #167629, #47269, #168605, #166644, #150482, #120120, #107920, #92751, #14938, #77592, #73642, #76598, #89786, #138274, #29126, #43289, #181811, #104958, #139263, #739, #137279, #27142, #45279, #106932, #90764, #44286, #199957, #62411, #124081, #88789, #11977, #135313, #196986, #58452, #28146, #151471, #12960, #74624, #152447, #59436, #121109, #182803, #48385, #80686, #5834, #83666, #79702, #66517, #143342, #64538, #22014, #19039, #174706, #142362, #4829, #113997, #159511, #160523, #21007, #127181, #188891, #94869, #6826, #156550, #50372, #18049, #67510, #141373, #2860, #126204, #20016, #36170, #129167, #97822, #190864, #175695, #173721, #33210, #52341, #187900, #113013, #82662, #172717, #128179, #186914, #144346, #37170, #189878, #98829, #145344, #51353, #68504, #81659, #110042, #35189, #171721, #49367, #111031, #34200, #96843, #95862, #157545, #3842, #65521, #112032, #158528, #134954, #14567, #135938, #131179, #115016, #84662, #28767, #136912, #197608, #121735, #38184, #43920, #57110, #59074, #73284, #7828, #146340, #69513, #90404, #168245, #104597, #153065, #27781, #151112, #58101, #11616, #12604, #89423, #120741, #198599, #105582, #44911, #176710, #130159, #166284, #99840, #161524, #91374, #196632, #152089, #182440, #191856, #53337, #167268, #119771, #118784, #88421, #26779, #13574, #181455, #150115, #23016, #60067, #195637, #75241, #42933, #180472, #41944, #103610, #165286, #74268, #183427, #106568, #29741, #158041, #64046, #65033, #94370, #76225, #92382, #47894, #30735, #95366, #172219, #186417, #125716, #169226, #109547, #33703, #137904, #15563, #3358, #78203, #34697, #48883, #108554, #156049, #124719, #32718, #61054, #154068, #77221, #111536, #17546, #187415, #184416, #140876, #1362, #157051, #107550, #138890, #45897, #171229, #110538, #18548, #80195, #141867, #126689, #2365, #199586, #79207, #188393, #49870, #16556, #31726, #370, #173221, #46894, #96354, #62041, #122726, #123705, #185403, #170233, #93374, #155061, #139873, #63041, #98330, #129667, #66022, #35687, #178215, #160030, #175206, #54853, #99346, #22523, #159021, #21517, #128680, #83178, #37681 ),
 ( #52841, #115533, #190377, #144852, #6335, #101341, #84170, #20514, #4338, #174219, #177221, #23525, #145850, #8352, #127690, #130682, #143858, #7332, #68015, #97335, #82162, #5337, #38694, #116527, #191363, #39679, #114510, #161029, #176212, #69016, #192376, #53859, #100350, #85171, #162029, #131696, #189390, #19532, #146859, #50867, #112525, #81177, #70027, #193377, #142859, #67021, #51852, #113511, #36671, #87191, #118539, #56864, #197369, #41698, #180228, #132695, #167026, #147877, #89178, #103363, #117525, #164048, #148872, #10363, #134709, #194384, #9363, #179223, #44669, #150870, #196392, #165041, #42692, #166037, #13337, #26534, #73037, #88178, #24536, #149862, #182192, #59823, #55851, #104353, #119533, #40689, #198349, #195386, #12364, #11367, #181216, #90164, #135697, #136667, #58834, #57860, #27537, #71028, #183187, #102358, #74027, #25547, #43677, #72020, #133693, #120501, #105339, #28528, #151847, #75002, #121493, #163030, #86187, #188160, #124476, #154818, #95129, #46650, #61798, #107308, #139633, #76977, #2127, #137659, #1121, #156819, #29504, #63809, #199346, #62795, #171983, #106322, #185160, #16316, #152827, #122484, #64801, #108310, #123468, #141636, #186173, #109306, #45657, #169990, #15318, #31481, #47655, #168008, #170985, #126462, #48649, #91137, #32478, #93133, #129, #77966, #14321, #184175, #187178, #94131, #155810, #17308, #78963, #138648, #75986, #92136, #60811, #79967, #153823, #140638, #168980, #125482, #110301, #33471, #30485, #18311, #3126, #113276, #84930, #6099, #112291, #66779, #80949, #145615, #7094, #21280, #83934, #160795, #111296, #65782, #68775, #20273, #51612, #131449, #130433, #192132, #53613, #114270, #36432, #96122, #115289, #157810, #175974, #22283, #35449, #67779, #49633, #37443, #99103, #129436, #176982, #38452, #100107, #161791, #82937, #23286, #98087, #146610, #8103, #69781, #144615, #159785, #172985, #81919, #191134, #34463, #143612, #190137, #174968, #19301, #52608, #50630, #142624, #4103, #127451, #189157, #173981, #97101, #158785, #5096, #128440, #196153, #133452, #70788, #9122, #132456, #150633, #28297, #164802, #13110, #87938, #11123, #118297, #71782, #72798, #149625, #119293, #197134, #104116, #105110, #177973, #74775, #26297, #101101, #162787, #151618, #56623, #12129, #57625, #193136, #54609, #165798, #179988, #117285, #148632, #86948, #27295, #195142, #10122, #24295, #58601, #39441, #180976, #41456, #147633, #194147, #178979, #40446, #134468, #85944, #55611, #102119, #116283, #42452, #181959, #88942, #163804, #25306, #73793, #103121, #135465, #120267, #43441, #166796, #89937, #169754, #93901, #18078, #75748, #63573, #138419, #94899, #109075, #168747, #16081, #184927, #92899, #121259, #90905, #29274, #171752, #154585, #185934, #44436, #887, #61567, #107076, #31249, #32243, #30251, #76744, #200099, #136437, #139405, #137425, #182953, #152591, #155579, #140404, #62562, #125247, #106090, #47419, #60572, #123236, #198118, #77739, #199105, #153585, #167776, #17074, #78728, #108070, #170754, #1892, #59585, #14082, #186945, #91894, #46411, #122248, #48416, #110072, #33241, #124238, #156583, #183938, #45423, #15083, #130191, #35218, #189908, #158555, #141402, #173750, #98861, #176741, #172749, #159542, #36199, #157575, #115049, #112062, #67540, #96871, #97853, #6857, #52372, #53371, #114029, #20045, #81688, #187929, #99870, #49398, #143370, #111061, #160556, #34230, #95892, #19068, #113044, #129198, #22046, #190896, #83697, #68536, #144377, #161554, #21040, #128211, #191887, #4862, #66547, #80715, #174736, #50402, #175726, #142393, #82693, #38214, #2890, #37205, #3872, #5864, #145375, #79733, #51383, #64569, #126234, #65551, #127210, #188924, #178736, #58371, #102878, #26057, #162546, #163561, #132215, #25061, #41217, #84692, #118057, #43206, #165561, #7859, #164563, #86704, #117041, #133209, #146372, #100864, #103881, #87700, #179747, #149385 ),
 ( #23047, #134229, #148389, #147392, #40199, #101879, #57389, #9883, #71543, #192901, #27058, #69546, #10881, #194900, #177739, #24050, #8880, #70548, #56374, #54378, #131210, #39208, #104873, #72551, #11896, #195914, #116050, #85706, #119062, #193907, #42220, #180744, #88704, #150400, #55371, #73559, #135232, #196904, #120038, #181725, #168526, #125013, #139177, #198879, #46179, #14854, #123009, #151388, #121021, #59352, #1658, #184695, #15847, #74543, #31016, #91662, #153352, #12878, #108840, #136208, #92666, #653, #152366, #107832, #166562, #154354, #77506, #169516, #47181, #32010, #62323, #123993, #199874, #155352, #76515, #170521, #185691, #16842, #61338, #138191, #186709, #137193, #93667, #78492, #60346, #106851, #30024, #48180, #140165, #167549, #197883, #182718, #63336, #28061, #89702, #44203, #105862, #29044, #90684, #13851, #75518, #122020, #183711, #45197, #67306, #145141, #81456, #129954, #4622, #127974, #34985, #188686, #142156, #189677, #36966, #82457, #83464, #144145, #50166, #111824, #17842, #191654, #79500, #173512, #141169, #128965, #2658, #64335, #126004, #143142, #159307, #190665, #20802, #52141, #98627, #174503, #109836, #51149, #158326, #160321, #96638, #65318, #110829, #66313, #80482, #5629, #187700, #112810, #21812, #33008, #113798, #49170, #35970, #175493, #171519, #19815, #97617, #156342, #172513, #68303, #6624, #126977, #94663, #33998, #95654, #157342, #18837, #3640, #55143, #71320, #114812, #148163, #73331, #195685, #37981, #132983, #193672, #147158, #163332, #176504, #130974, #133994, #116814, #131987, #179517, #24828, #85469, #99638, #38981, #7624, #26827, #100637, #164339, #11665, #86478, #194674, #162318, #135003, #146138, #56143, #178505, #53133, #117824, #115821, #70320, #84460, #149165, #10655, #9654, #87478, #25834, #161321, #69308, #72318, #23819, #39971, #22814, #57156, #118835, #180518, #40986, #102654, #101641, #41991, #103657, #165335, #8646, #88468, #150165, #192665, #54148, #177511, #93421, #89472, #76274, #153113, #74318, #31773, #28816, #184465, #45944, #77267, #107599, #138936, #185452, #61102, #78249, #14617, #44962, #46942, #136961, #152140, #197656, #29790, #167320, #92430, #27831, #91426, #108602, #119818, #154117, #151163, #137952, #62090, #196681, #75290, #106620, #42981, #12651, #155108, #198650, #13623, #16602, #199635, #122775, #135985, #60116, #105631, #121784, #169277, #58150, #30783, #181503, #416, #104646, #15610, #183478, #90456, #168294, #166333, #59122, #123753, #170279, #120788, #182488, #43969, #175006, #186467, #128479, #97139, #116320, #190174, #53652, #101137, #176012, #22320, #51650, #24332, #35489, #83971, #67818, #139922, #145651, #5134, #159824, #174018, #38489, #100146, #114310, #177020, #115329, #1411, #158822, #161827, #113314, #144653, #63090, #23322, #84966, #146648, #7132, #37481, #82977, #68815, #130474, #193173, #98127, #52646, #21319, #124769, #36470, #8142, #39476, #20310, #192171, #99143, #81958, #178009, #6135, #69819, #129473, #160832, #131486, #54645, #162823, #50668, #191172, #112328, #143650, #66816, #194183, #149663, #55648, #105146, #117320, #179016, #40484, #119330, #133487, #57663, #102156, #70825, #163842, #167810, #73831, #74810, #104154, #85982, #25343, #181016, #86984, #166832, #181996, #196191, #135501, #148671, #42490, #43479, #147671, #10159, #13147, #87975, #44472, #58637, #118333, #165835, #134505, #27332, #132494, #71819, #195179, #121296, #88978, #197172, #56660, #150668, #11161, #72835, #180026, #28333, #41495, #12166, #120303, #103158, #89972, #9159, #151652, #136472, #198152, #59622, #182988, #106127, #164839, #26335, #18113, #77772, #33274, #48450, #79768, #124273, #139439, #49434, #200132, #62595, #125283, #61601, #169789, #31282, #111095, #32279, #30285, #14117, #183971, #186980, #94933, #93935, #141438, #137462, #140438, #153622, #110108, #91930, #123270, #199142, #107112, #171786, #64603 ),
 ( #156618, #155614, #185969, #92933, #109109, #17110, #2925, #184961, #921, #108105, #90940, #46445, #126267, #187964, #122283, #170788, #47453, #168783, #29310, #154621, #78761, #16114, #1928, #152627, #63607, #75784, #60608, #45458, #15118, #76780, #138451, #54410, #190929, #21075, #161586, #113076, #128244, #173786, #5898, #143409, #68568, #3907, #67575, #23080, #95925, #130225, #65587, #129232, #38246, #172785, #51416, #82731, #19101, #188960, #131244, #174768, #189941, #7893, #52406, #175763, #112096, #36234, #81724, #97886, #114065, #34266, #37239, #192933, #115082, #157610, #98895, #159578, #66579, #144412, #80750, #50437, #53404, #160589, #22078, #83729, #145408, #4897, #142428, #158590, #127247, #146403, #20079, #6890, #35253, #191921, #176774, #99901, #96906, #84725, #69578, #41249, #197911, #195948, #178769, #133241, #147425, #11926, #73590, #87733, #150431, #27091, #177770, #132249, #135263, #86736, #118090, #116082, #196934, #58402, #120068, #180776, #149418, #56409, #57421, #119094, #166593, #71575, #26089, #194933, #39239, #9916, #181756, #12905, #8912, #42251, #72587, #193940, #151418, #148421, #103913, #179780, #134261, #43238, #88737, #89732, #104905, #102911, #164595, #24083, #136237, #85738, #10914, #70580, #28093, #55403, #117073, #40235, #165593, #74569, #100895, #101911, #162579, #163593, #25094, #155380, #169546, #108870, #152393, #92694, #16869, #141197, #198907, #186737, #61366, #17873, #32040, #91691, #139207, #107861, #15877, #44233, #13879, #75546, #94691, #77535, #170550, #167577, #124023, #184723, #46207, #105890, #1687, #29071, #185721, #93697, #45225, #682, #59381, #47211, #78520, #62353, #140194, #125041, #63364, #48208, #154382, #109862, #31045, #171547, #33036, #156369, #79527, #121054, #182749, #30050, #90710, #137221, #153382, #199902, #123037, #60375, #122047, #183738, #106879, #168552, #14883, #76544, #138220, #191682, #110857, #113826, #127007, #83493, #3669, #35013, #172542, #80512, #160351, #38011, #174532, #22842, #97646, #20832, #128005, #81485, #82488, #159335, #128996, #6654, #175521, #114841, #187728, #84489, #35999, #34027, #95685, #161351, #66343, #21841, #5658, #2686, #64363, #36996, #189707, #188715, #158356, #96668, #98657, #143172, #19844, #157372, #68332, #49199, #190694, #4652, #18866, #65347, #50198, #111854, #144172, #142185, #173544, #51180, #126032, #52169, #53163, #67334, #112840, #145170, #129982, #176535, #99667, #164366, #27859, #162346, #117852, #100664, #165363, #42019, #56171, #195713, #39009, #179545, #103684, #146167, #85497, #73360, #148189, #104675, #118862, #178531, #25861, #194702, #102681, #131002, #23847, #147185, #181529, #87505, #57186, #54177, #10683, #71348, #133012, #192694, #88499, #115850, #72347, #180545, #132014, #149193, #7652, #134021, #26857, #150195, #11693, #135032, #196707, #58177, #41015, #119844, #43008, #166362, #69336, #177540, #8675, #70347, #193701, #116841, #55171, #39998, #101670, #86505, #9683, #163360, #24856, #90484, #74344, #43997, #185482, #93451, #154147, #78279, #197682, #445, #13649, #170309, #152166, #121811, #59147, #167346, #46972, #124799, #61130, #109625, #184493, #107626, #14644, #168321, #169304, #45972, #15639, #155139, #62120, #1442, #136010, #171309, #122803, #120817, #182517, #47973, #153142, #108631, #92459, #89500, #151189, #123783, #76304, #75316, #44989, #183506, #31802, #29818, #106649, #105659, #16632, #28843, #77297, #91454, #136987, #198676, #60143, #137982, #30810, #199665, #139952, #63120, #138967, #186497, #12677, #94448, #48958, #67097, #3431, #34773, #114592, #51928, #128756, #113588, #97409, #66099, #173299, #112601, #35763, #83253, #188469, #142932, #111614, #156128, #126765, #175282, #129743, #125790, #174293, #189465, #110612, #68090, #65107, #20590, #49950, #50943, #160107, #36747, #96430, #172294, #159096, #64125, #17627, #187492, #32796, #82242, #21595 ),
 ( #33783, #144928, #158116, #191440, #5414, #19608, #143933, #81250, #190453, #79286, #95443, #157127, #52916, #98411, #6409, #140956, #2443, #4413, #127765, #18623, #80270, #141940, #102435, #148949, #162107, #194456, #176289, #164122, #25620, #132769, #56941, #41773, #40766, #72099, #9437, #165118, #24613, #180305, #195466, #26610, #71102, #86261, #196469, #146941, #55927, #133771, #8431, #116603, #178291, #57939, #179302, #177298, #161105, #130760, #118615, #103438, #87264, #88253, #84247, #10439, #100426, #149939, #38769, #70103, #145927, #53934, #11446, #73118, #193454, #101417, #147951, #134787, #39755, #7410, #37761, #69093, #163110, #192452, #99423, #115609, #23604, #85250, #117601, #22600, #131772, #54930, #209, #108395, #184255, #1201, #137740, #168084, #170072, #59903, #75078, #120581, #152903, #90242, #15400, #150950, #14399, #31563, #42771, #77057, #12444, #76065, #185242, #119610, #198429, #29581, #166116, #135776, #78044, #121571, #136745, #154899, #199424, #122565, #58913, #183266, #28604, #44746, #60889, #181293, #45737, #139713, #61878, #104433, #107389, #106402, #13414, #91212, #27619, #197447, #123548, #169062, #30568, #92219, #153905, #151925, #89258, #105420, #74106, #93214, #167103, #138729, #182274, #46733, #16398, #43756, #144695, #155889, #142704, #188237, #62877, #4183, #125559, #80043, #94210, #158866, #20355, #34542, #97180, #174064, #124558, #79042, #82003, #33548, #64877, #186255, #143696, #5179, #66860, #127533, #96201, #3203, #65862, #189236, #113359, #18392, #173065, #141712, #47733, #156896, #128523, #159871, #17387, #50714, #19379, #140717, #98170, #95209, #112372, #126538, #81028, #190217, #109386, #2207, #51696, #49712, #21363, #35532, #111376, #175051, #157890, #36515, #171066, #63888, #187256, #83021, #32556, #48725, #110378, #172061, #23369, #85014, #191216, #55694, #52690, #101183, #147718, #7179, #116367, #6181, #24380, #86031, #178055, #117367, #179064, #162872, #132540, #193220, #163893, #8192, #40533, #194228, #25389, #54694, #69867, #71864, #53701, #39523, #102204, #115378, #161875, #146695, #67861, #9206, #68863, #114354, #160877, #87031, #148716, #70872, #10204, #176058, #129516, #177066, #37526, #38537, #131536, #145697, #100193, #99189, #22368, #84019, #130522, #192218, #101172, #97170, #51686, #69854, #6170, #37514, #117357, #54681, #131522, #116355, #100181, #68851, #176046, #115365, #38525, #86018, #191205, #145686, #114343, #158855, #129505, #178044, #132529, #128512, #177055, #192206, #113348, #70860, #67850, #23357, #52680, #53688, #162860, #99176, #160866, #7168, #9195, #22356, #143685, #55683, #5166, #84008, #66849, #39512, #190207, #175040, #36505, #130510, #85002, #24367, #146683, #147707, #194218, #161863, #35522, #8178, #98159, #20343, #159859, #81992, #193208, #21352, #83010, #144685, #195215, #150703, #133523, #198185, #74842, #89012, #28367, #71854, #12201, #136505, #60642, #118369, #106161, #181050, #137495, #151688, #11196, #58669, #27366, #135535, #163880, #56695, #180062, #14150, #197206, #90005, #87020, #43513, #104188, #165870, #25378, #121329, #148706, #105179, #13179, #164875, #120335, #179053, #166865, #59655, #182030, #183021, #44505, #167843, #29344, #73866, #90973, #152660, #75817, #199175, #40521, #102192, #10194, #41531, #149698, #103194, #26370, #72871, #119366, #42525, #88010, #134540, #196228, #57698, #76812, #18144, #126295, #187011, #111124, #30319, #33304, #46479, #2954, #123302, #154653, #91962, #200164, #79797, #157640, #93966, #140472, #153655, #124305, #139472, #952, #1960, #78793, #48481, #187992, #94963, #34294, #107145, #3935, #155646, #15150, #138483, #80779, #186003, #141470, #125315, #122316, #184007, #156648, #47484, #108139, #77803, #16148, #64633, #62628, #109141, #61634, #49462, #168815, #110137, #170820, #184995, #172814, #32312, #169823, #171816, #17141, #63639, #31314, #95955, #92967 ) ),
 .UNSPECIFIED., .T., .F., .F. ) 
 B_SPLINE_SURFACE_WITH_KNOTS ( ( 4, 3, 4 ),
 ( 3, 2, 2, 2, 2, 2, 2, 2, 2, 2, 2, 2, 2, 2, 2, 2, 2, 2, 2, 2, 2, 2, 2, 2, 2, 2, 2, 2, 2, 2, 2, 2, 2, 2, 2, 2, 2, 2, 2, 2, 2, 2, 2, 2, 2, 2, 2, 2, 2, 2, 2, 2, 2, 2, 2, 2, 2, 2, 2, 2, 2, 2, 2, 2, 2, 2, 2, 2, 2, 2, 2, 2, 2, 2, 2, 2, 2, 2, 2, 2, 2, 2, 2, 2, 2, 2, 2, 2, 2, 2, 2, 2, 2, 2, 2, 2, 2, 2, 2, 2, 2, 2, 2, 2, 2, 2, 2, 2, 2, 2, 2, 2, 2, 2, 2, 2, 2, 2, 2, 2, 2, 2, 2, 2, 2, 2, 2, 2, 2, 2, 2, 2, 2, 2, 2, 2, 2, 2, 2, 2, 2, 2, 2, 2, 2, 2, 2, 2, 2, 2, 2, 2, 2, 2, 2, 2, 2, 2, 2, 2, 2, 2, 2, 2, 2, 2, 2, 2, 2, 2, 2, 2, 2, 2, 2, 2, 2, 2, 2, 2, 2, 2, 2, 2, 2, 2, 2, 2, 2, 2, 2, 2, 2, 2, 2, 2, 2, 2, 2, 2, 2, 2, 2, 2, 2, 2, 2, 2, 2, 2, 2, 2, 2, 2, 2, 2, 2, 2, 2, 2, 2, 2, 2, 2, 2, 2, 2, 2, 3 ),
 ( 0.000000000000000000, 0.5000000000000000000, 1.000000000000000000 ),
 ( 0.000000000000000000, 0.004385964912280701511, 0.008771929824561403022, 0.01315789473684210453, 0.01754385964912280604, 0.02192982456140350755, 0.02631578947368420907, 0.03070175438596491058, 0.03508771929824561209, 0.03947368421052631360, 0.04385964912280701511, 0.04824561403508771662, 0.05263157894736841813, 0.05701754385964911964, 0.06140350877192982115, 0.06578947368421052266, 0.07017543859649122417, 0.07456140350877192569, 0.07894736842105262720, 0.08333333333333332871, 0.08771929824561403022, 0.09210526315789473173, 0.09649122807017543324, 0.1008771929824561348, 0.1052631578947368363, 0.1096491228070175378, 0.1140350877192982393, 0.1184210526315789408, 0.1228070175438596423, 0.1271929824561403577, 0.1315789473684210453, 0.1359649122807017607, 0.1403508771929824483, 0.1447368421052631637, 0.1491228070175438514, 0.1535087719298245668, 0.1578947368421052544, 0.1622807017543859698, 0.1666666666666666574, 0.1710526315789473728, 0.1754385964912280604, 0.1798245614035087758, 0.1842105263157894635, 0.1885964912280701788, 0.1929824561403508665, 0.1973684210526315819, 0.2017543859649122695, 0.2061403508771929849, 0.2105263157894736725, 0.2149122807017543879, 0.2192982456140350755, 0.2236842105263157909, 0.2280701754385964786, 0.2324561403508771940, 0.2368421052631578816, 0.2412280701754385970, 0.2456140350877192846, 0.2500000000000000000, 0.2543859649122807154, 0.2587719298245614308, 0.2631578947368420907, 0.2675438596491228060, 0.2719298245614035214, 0.2763157894736842368, 0.2807017543859648967, 0.2850877192982456121, 0.2894736842105263275, 0.2938596491228070429, 0.2982456140350877027, 0.3026315789473684181, 0.3070175438596491335, 0.3114035087719298489, 0.3157894736842105088, 0.3201754385964912242, 0.3245614035087719396, 0.3289473684210526550, 0.3333333333333333148, 0.3377192982456140302, 0.3421052631578947456, 0.3464912280701754610, 0.3508771929824561209, 0.3552631578947368363, 0.3596491228070175517, 0.3640350877192982670, 0.3684210526315789269, 0.3728070175438596423, 0.3771929824561403577, 0.3815789473684210731, 0.3859649122807017330, 0.3903508771929824483, 0.3947368421052631637, 0.3991228070175438791, 0.4035087719298245390, 0.4078947368421052544, 0.4122807017543859698, 0.4166666666666666852, 0.4210526315789473450, 0.4254385964912280604, 0.4298245614035087758, 0.4342105263157894912, 0.4385964912280701511, 0.4429824561403508665, 0.4473684210526315819, 0.4517543859649122973, 0.4561403508771929571, 0.4605263157894736725, 0.4649122807017543879, 0.4692982456140351033, 0.4736842105263157632, 0.4780701754385964786, 0.4824561403508771940, 0.4868421052631579093, 0.4912280701754385692, 0.4956140350877192846, 0.5000000000000000000, 0.5043859649122807154, 0.5087719298245614308, 0.5131578947368421462, 0.5175438596491228616, 0.5219298245614034659, 0.5263157894736841813, 0.5307017543859648967, 0.5350877192982456121, 0.5394736842105263275, 0.5438596491228070429, 0.5482456140350877583, 0.5526315789473684736, 0.5570175438596490780, 0.5614035087719297934, 0.5657894736842105088, 0.5701754385964912242, 0.5745614035087719396, 0.5789473684210526550, 0.5833333333333333703, 0.5877192982456140857, 0.5921052631578946901, 0.5964912280701754055, 0.6008771929824561209, 0.6052631578947368363, 0.6096491228070175517, 0.6140350877192982670, 0.6184210526315789824, 0.6228070175438596978, 0.6271929824561403022, 0.6315789473684210176, 0.6359649122807017330, 0.6403508771929824483, 0.6447368421052631637, 0.6491228070175438791, 0.6535087719298245945, 0.6578947368421053099, 0.6622807017543859143, 0.6666666666666666297, 0.6710526315789473450, 0.6754385964912280604, 0.6798245614035087758, 0.6842105263157894912, 0.6885964912280702066, 0.6929824561403509220, 0.6973684210526315264, 0.7017543859649122417, 0.7061403508771929571, 0.7105263157894736725, 0.7149122807017543879, 0.7192982456140351033, 0.7236842105263158187, 0.7280701754385965341, 0.7324561403508771384, 0.7368421052631578538, 0.7412280701754385692, 0.7456140350877192846, 0.7500000000000000000, 0.7543859649122807154, 0.7587719298245614308, 0.7631578947368421462, 0.7675438596491228616, 0.7719298245614034659, 0.7763157894736841813, 0.7807017543859648967, 0.7850877192982456121, 0.7894736842105263275, 0.7938596491228070429, 0.7982456140350877583, 0.8026315789473684736, 0.8070175438596490780, 0.8114035087719297934, 0.8157894736842105088, 0.8201754385964912242, 0.8245614035087719396, 0.8289473684210526550, 0.8333333333333333703, 0.8377192982456140857, 0.8421052631578946901, 0.8464912280701754055, 0.8508771929824561209, 0.8552631578947368363, 0.8596491228070175517, 0.8640350877192982670, 0.8684210526315789824, 0.8728070175438596978, 0.8771929824561403022, 0.8815789473684210176, 0.8859649122807017330, 0.8903508771929824483, 0.8947368421052631637, 0.8991228070175438791, 0.9035087719298245945, 0.9078947368421053099, 0.9122807017543859143, 0.9166666666666666297, 0.9210526315789473450, 0.9254385964912280604, 0.9298245614035087758, 0.9342105263157894912, 0.9385964912280702066, 0.9429824561403509220, 0.9473684210526315264, 0.9517543859649122417, 0.9561403508771929571, 0.9605263157894736725, 0.9649122807017543879, 0.9692982456140351033, 0.9736842105263158187, 0.9780701754385965341, 0.9824561403508771384, 0.9868421052631578538, 0.9912280701754385692, 0.9956140350877192846, 1.000000000000000000 ),
 .UNSPECIFIED. ) 
 GEOMETRIC_REPRESENTATION_ITEM ( )  RATIONAL_B_SPLINE_SURFACE ( (
 ( 1.000000000000000000, 0.9659258262890683122, 1.000000000000000000, 0.9659258262890683122, 1.000000000000000000, 0.9659258262890683122, 1.000000000000000000, 0.9659258262890683122, 1.000000000000000000, 0.9659258262890683122, 1.000000000000000000, 0.9659258262890683122, 1.000000000000000000, 0.9659258262890683122, 1.000000000000000000, 0.9659258262890683122, 1.000000000000000000, 0.9659258262890683122, 1.000000000000000000, 0.9659258262890683122, 1.000000000000000000, 0.9659258262890683122, 1.000000000000000000, 0.9659258262890683122, 1.000000000000000000, 0.9659258262890683122, 1.000000000000000000, 0.9659258262890683122, 1.000000000000000000, 0.9659258262890683122, 1.000000000000000000, 0.9659258262890683122, 1.000000000000000000, 0.9659258262890683122, 1.000000000000000000, 0.9659258262890683122, 1.000000000000000000, 0.9659258262890683122, 1.000000000000000000, 0.9659258262890683122, 1.000000000000000000, 0.9659258262890683122, 1.000000000000000000, 0.9659258262890683122, 1.000000000000000000, 0.9659258262890683122, 1.000000000000000000, 0.9659258262890683122, 1.000000000000000000, 0.9659258262890683122, 1.000000000000000000, 0.9659258262890683122, 1.000000000000000000, 0.9659258262890683122, 1.000000000000000000, 0.9659258262890683122, 1.000000000000000000, 0.9659258262890683122, 1.000000000000000000, 0.9659258262890683122, 1.000000000000000000, 0.9659258262890683122, 1.000000000000000000, 0.9659258262890683122, 1.000000000000000000, 0.9659258262890683122, 1.000000000000000000, 0.9659258262890683122, 1.000000000000000000, 0.9659258262890683122, 1.000000000000000000, 0.9659258262890683122, 1.000000000000000000, 0.9659258262890683122, 1.000000000000000000, 0.9659258262890683122, 1.000000000000000000, 0.9659258262890683122, 1.000000000000000000, 0.9659258262890683122, 1.000000000000000000, 0.9659258262890683122, 1.000000000000000000, 0.9659258262890683122, 1.000000000000000000, 0.9659258262890683122, 1.000000000000000000, 0.9659258262890683122, 1.000000000000000000, 0.9659258262890683122, 1.000000000000000000, 0.9659258262890683122, 1.000000000000000000, 0.9659258262890683122, 1.000000000000000000, 0.9659258262890683122, 1.000000000000000000, 0.9659258262890683122, 1.000000000000000000, 0.9659258262890683122, 1.000000000000000000, 0.9659258262890683122, 1.000000000000000000, 0.9659258262890683122, 1.000000000000000000, 0.9659258262890683122, 1.000000000000000000, 0.9659258262890683122, 1.000000000000000000, 0.9659258262890683122, 1.000000000000000000, 0.9659258262890683122, 1.000000000000000000, 0.9659258262890683122, 1.000000000000000000, 0.9659258262890683122, 1.000000000000000000, 0.9659258262890683122, 1.000000000000000000, 0.9659258262890683122, 1.000000000000000000, 0.9659258262890683122, 1.000000000000000000, 0.9659258262890683122, 1.000000000000000000, 0.9659258262890683122, 1.000000000000000000, 0.9659258262890683122, 1.000000000000000000, 0.9659258262890683122, 1.000000000000000000, 0.9659258262890683122, 1.000000000000000000, 0.9659258262890683122, 1.000000000000000000, 0.9659258262890683122, 1.000000000000000000, 0.9659258262890683122, 1.000000000000000000, 0.9659258262890683122, 1.000000000000000000, 0.9659258262890683122, 1.000000000000000000, 0.9659258262890683122, 1.000000000000000000, 0.9659258262890683122, 1.000000000000000000, 0.9659258262890683122, 1.000000000000000000, 0.9659258262890683122, 1.000000000000000000, 0.9659258262890683122, 1.000000000000000000, 0.9659258262890683122, 1.000000000000000000, 0.9659258262890683122, 1.000000000000000000, 0.9659258262890683122, 1.000000000000000000, 0.9659258262890683122, 1.000000000000000000, 0.9659258262890683122, 1.000000000000000000, 0.9659258262890683122, 1.000000000000000000, 0.9659258262890683122, 1.000000000000000000, 0.9659258262890683122, 1.000000000000000000, 0.9659258262890683122, 1.000000000000000000, 0.9659258262890683122, 1.000000000000000000, 0.9659258262890683122, 1.000000000000000000, 0.9659258262890683122, 1.000000000000000000, 0.9659258262890683122, 1.000000000000000000, 0.9659258262890683122, 1.000000000000000000, 0.9659258262890683122, 1.000000000000000000, 0.9659258262890683122, 1.000000000000000000, 0.9659258262890683122, 1.000000000000000000, 0.9659258262890683122, 1.000000000000000000, 0.9659258262890683122, 1.000000000000000000, 0.9659258262890683122, 1.000000000000000000, 0.9659258262890683122, 1.000000000000000000, 0.9659258262890683122, 1.000000000000000000, 0.9659258262890683122, 1.000000000000000000, 0.9659258262890683122, 1.000000000000000000, 0.9659258262890683122, 1.000000000000000000, 0.9659258262890683122, 1.000000000000000000, 0.9659258262890683122, 1.000000000000000000, 0.9659258262890683122, 1.000000000000000000, 0.9659258262890683122, 1.000000000000000000, 0.9659258262890683122, 1.000000000000000000, 0.9659258262890683122, 1.000000000000000000, 0.9659258262890683122, 1.000000000000000000, 0.9659258262890683122, 1.000000000000000000, 0.9659258262890683122, 1.000000000000000000, 0.9659258262890683122, 1.000000000000000000, 0.9659258262890683122, 1.000000000000000000, 0.9659258262890683122, 1.000000000000000000, 0.9659258262890683122, 1.000000000000000000, 0.9659258262890683122, 1.000000000000000000, 0.9659258262890683122, 1.000000000000000000, 0.9659258262890683122, 1.000000000000000000, 0.9659258262890683122, 1.000000000000000000, 0.9659258262890683122, 1.000000000000000000, 0.9659258262890683122, 1.000000000000000000, 0.9659258262890683122, 1.000000000000000000, 0.9659258262890683122, 1.000000000000000000, 0.9659258262890683122, 1.000000000000000000, 0.9659258262890683122, 1.000000000000000000, 0.9659258262890683122, 1.000000000000000000, 0.9659258262890683122, 1.000000000000000000, 0.9659258262890683122, 1.000000000000000000, 0.9659258262890683122, 1.000000000000000000, 0.9659258262890683122, 1.000000000000000000, 0.9659258262890683122, 1.000000000000000000, 0.9659258262890683122, 1.000000000000000000, 0.9659258262890683122, 1.000000000000000000, 0.9659258262890683122, 1.000000000000000000, 0.9659258262890683122, 1.000000000000000000, 0.9659258262890683122, 1.000000000000000000, 0.9659258262890683122, 1.000000000000000000, 0.9659258262890683122, 1.000000000000000000, 0.9659258262890683122, 1.000000000000000000, 0.9659258262890683122, 1.000000000000000000, 0.9659258262890683122, 1.000000000000000000, 0.9659258262890683122, 1.000000000000000000, 0.9659258262890683122, 1.000000000000000000, 0.9659258262890683122, 1.000000000000000000, 0.9659258262890683122, 1.000000000000000000, 0.9659258262890683122, 1.000000000000000000, 0.9659258262890683122, 1.000000000000000000, 0.9659258262890683122, 1.000000000000000000, 0.9659258262890683122, 1.000000000000000000, 0.9659258262890683122, 1.000000000000000000, 0.9659258262890683122, 1.000000000000000000, 0.9659258262890683122, 1.000000000000000000, 0.9659258262890683122, 1.000000000000000000, 0.9659258262890683122, 1.000000000000000000, 0.9659258262890683122, 1.000000000000000000, 0.9659258262890683122, 1.000000000000000000, 0.9659258262890683122, 1.000000000000000000, 0.9659258262890683122, 1.000000000000000000, 0.9659258262890683122, 1.000000000000000000, 0.9659258262890683122, 1.000000000000000000, 0.9659258262890683122, 1.000000000000000000, 0.9659258262890683122, 1.000000000000000000, 0.9659258262890683122, 1.000000000000000000, 0.9659258262890683122, 1.000000000000000000, 0.9659258262890683122, 1.000000000000000000, 0.9659258262890683122, 1.000000000000000000, 0.9659258262890683122, 1.000000000000000000, 0.9659258262890683122, 1.000000000000000000, 0.9659258262890683122, 1.000000000000000000, 0.9659258262890683122, 1.000000000000000000, 0.9659258262890683122, 1.000000000000000000, 0.9659258262890683122, 1.000000000000000000, 0.9659258262890683122, 1.000000000000000000, 0.9659258262890683122, 1.000000000000000000, 0.9659258262890683122, 1.000000000000000000, 0.9659258262890683122, 1.000000000000000000, 0.9659258262890683122, 1.000000000000000000, 0.9659258262890683122, 1.000000000000000000, 0.9659258262890683122, 1.000000000000000000, 0.9659258262890683122, 1.000000000000000000, 0.9659258262890683122, 1.000000000000000000, 0.9659258262890683122, 1.000000000000000000, 0.9659258262890683122, 1.000000000000000000, 0.9659258262890683122, 1.000000000000000000, 0.9659258262890683122, 1.000000000000000000, 0.9659258262890683122, 1.000000000000000000, 0.9659258262890683122, 1.000000000000000000, 0.9659258262890683122, 1.000000000000000000, 0.9659258262890683122, 1.000000000000000000, 0.9659258262890683122, 1.000000000000000000, 0.9659258262890683122, 1.000000000000000000, 0.9659258262890683122, 1.000000000000000000, 0.9659258262890683122, 1.000000000000000000, 0.9659258262890683122, 1.000000000000000000, 0.9659258262890683122, 1.000000000000000000, 0.9659258262890683122, 1.000000000000000000, 0.9659258262890683122, 1.000000000000000000, 0.9659258262890683122, 1.000000000000000000, 0.9659258262890683122, 1.000000000000000000, 0.9659258262890683122, 1.000000000000000000, 0.9659258262890683122, 1.000000000000000000, 0.9659258262890683122, 1.000000000000000000, 0.9659258262890683122, 1.000000000000000000, 0.9659258262890683122, 1.000000000000000000, 0.9659258262890683122, 1.000000000000000000, 0.9659258262890683122, 1.000000000000000000, 0.9659258262890683122, 1.000000000000000000, 0.9659258262890683122, 1.000000000000000000, 0.9659258262890683122, 1.000000000000000000, 0.9659258262890683122, 1.000000000000000000, 0.9659258262890683122, 1.000000000000000000, 0.9659258262890683122, 1.000000000000000000, 0.9659258262890683122, 1.000000000000000000, 0.9659258262890683122, 1.000000000000000000, 0.9659258262890683122, 1.000000000000000000, 0.9659258262890683122, 1.000000000000000000, 0.9659258262890683122, 1.000000000000000000, 0.9659258262890683122, 1.000000000000000000, 0.9659258262890683122, 1.000000000000000000, 0.9659258262890683122, 1.000000000000000000, 0.9659258262890683122, 1.000000000000000000, 0.9659258262890683122, 1.000000000000000000, 0.9659258262890683122, 1.000000000000000000, 0.9659258262890683122, 1.000000000000000000, 0.9659258262890683122, 1.000000000000000000, 0.9659258262890683122, 1.000000000000000000, 0.9659258262890683122, 1.000000000000000000, 0.9659258262890683122, 1.000000000000000000, 0.9659258262890683122, 1.000000000000000000),
 ( 0.3333333333333333703, 0.3219752754296894559, 0.3333333333333333703, 0.3219752754296894559, 0.3333333333333333703, 0.3219752754296894559, 0.3333333333333333703, 0.3219752754296894559, 0.3333333333333333703, 0.3219752754296894559, 0.3333333333333333703, 0.3219752754296894559, 0.3333333333333333703, 0.3219752754296894559, 0.3333333333333333703, 0.3219752754296894559, 0.3333333333333333703, 0.3219752754296894559, 0.3333333333333333703, 0.3219752754296894559, 0.3333333333333333703, 0.3219752754296894559, 0.3333333333333333703, 0.3219752754296894559, 0.3333333333333333703, 0.3219752754296894559, 0.3333333333333333703, 0.3219752754296894559, 0.3333333333333333703, 0.3219752754296894559, 0.3333333333333333703, 0.3219752754296894559, 0.3333333333333333703, 0.3219752754296894559, 0.3333333333333333703, 0.3219752754296894559, 0.3333333333333333703, 0.3219752754296894559, 0.3333333333333333703, 0.3219752754296894559, 0.3333333333333333703, 0.3219752754296894559, 0.3333333333333333703, 0.3219752754296894559, 0.3333333333333333703, 0.3219752754296894559, 0.3333333333333333703, 0.3219752754296894559, 0.3333333333333333703, 0.3219752754296894559, 0.3333333333333333703, 0.3219752754296894559, 0.3333333333333333703, 0.3219752754296894559, 0.3333333333333333703, 0.3219752754296894559, 0.3333333333333333703, 0.3219752754296894559, 0.3333333333333333703, 0.3219752754296894559, 0.3333333333333333703, 0.3219752754296894559, 0.3333333333333333703, 0.3219752754296894559, 0.3333333333333333703, 0.3219752754296894559, 0.3333333333333333703, 0.3219752754296894559, 0.3333333333333333703, 0.3219752754296894559, 0.3333333333333333703, 0.3219752754296894559, 0.3333333333333333703, 0.3219752754296894559, 0.3333333333333333703, 0.3219752754296894559, 0.3333333333333333703, 0.3219752754296894559, 0.3333333333333333703, 0.3219752754296894559, 0.3333333333333333703, 0.3219752754296894559, 0.3333333333333333703, 0.3219752754296894559, 0.3333333333333333703, 0.3219752754296894559, 0.3333333333333333703, 0.3219752754296894559, 0.3333333333333333703, 0.3219752754296894559, 0.3333333333333333703, 0.3219752754296894559, 0.3333333333333333703, 0.3219752754296894559, 0.3333333333333333703, 0.3219752754296894559, 0.3333333333333333703, 0.3219752754296894559, 0.3333333333333333703, 0.3219752754296894559, 0.3333333333333333703, 0.3219752754296894559, 0.3333333333333333703, 0.3219752754296894559, 0.3333333333333333703, 0.3219752754296894559, 0.3333333333333333703, 0.3219752754296894559, 0.3333333333333333703, 0.3219752754296894559, 0.3333333333333333703, 0.3219752754296894559, 0.3333333333333333703, 0.3219752754296894559, 0.3333333333333333703, 0.3219752754296894559, 0.3333333333333333703, 0.3219752754296894559, 0.3333333333333333703, 0.3219752754296894559, 0.3333333333333333703, 0.3219752754296894559, 0.3333333333333333703, 0.3219752754296894559, 0.3333333333333333703, 0.3219752754296894559, 0.3333333333333333703, 0.3219752754296894559, 0.3333333333333333703, 0.3219752754296894559, 0.3333333333333333703, 0.3219752754296894559, 0.3333333333333333703, 0.3219752754296894559, 0.3333333333333333703, 0.3219752754296894559, 0.3333333333333333703, 0.3219752754296894559, 0.3333333333333333703, 0.3219752754296894559, 0.3333333333333333703, 0.3219752754296894559, 0.3333333333333333703, 0.3219752754296894559, 0.3333333333333333703, 0.3219752754296894559, 0.3333333333333333703, 0.3219752754296894559, 0.3333333333333333703, 0.3219752754296894559, 0.3333333333333333703, 0.3219752754296894559, 0.3333333333333333703, 0.3219752754296894559, 0.3333333333333333703, 0.3219752754296894559, 0.3333333333333333703, 0.3219752754296894559, 0.3333333333333333703, 0.3219752754296894559, 0.3333333333333333703, 0.3219752754296894559, 0.3333333333333333703, 0.3219752754296894559, 0.3333333333333333703, 0.3219752754296894559, 0.3333333333333333703, 0.3219752754296894559, 0.3333333333333333703, 0.3219752754296894559, 0.3333333333333333703, 0.3219752754296894559, 0.3333333333333333703, 0.3219752754296894559, 0.3333333333333333703, 0.3219752754296894559, 0.3333333333333333703, 0.3219752754296894559, 0.3333333333333333703, 0.3219752754296894559, 0.3333333333333333703, 0.3219752754296894559, 0.3333333333333333703, 0.3219752754296894559, 0.3333333333333333703, 0.3219752754296894559, 0.3333333333333333703, 0.3219752754296894559, 0.3333333333333333703, 0.3219752754296894559, 0.3333333333333333703, 0.3219752754296894559, 0.3333333333333333703, 0.3219752754296894559, 0.3333333333333333703, 0.3219752754296894559, 0.3333333333333333703, 0.3219752754296894559, 0.3333333333333333703, 0.3219752754296894559, 0.3333333333333333703, 0.3219752754296894559, 0.3333333333333333703, 0.3219752754296894559, 0.3333333333333333703, 0.3219752754296894559, 0.3333333333333333703, 0.3219752754296894559, 0.3333333333333333703, 0.3219752754296894559, 0.3333333333333333703, 0.3219752754296894559, 0.3333333333333333703, 0.3219752754296894559, 0.3333333333333333703, 0.3219752754296894559, 0.3333333333333333703, 0.3219752754296894559, 0.3333333333333333703, 0.3219752754296894559, 0.3333333333333333703, 0.3219752754296894559, 0.3333333333333333703, 0.3219752754296894559, 0.3333333333333333703, 0.3219752754296894559, 0.3333333333333333703, 0.3219752754296894559, 0.3333333333333333703, 0.3219752754296894559, 0.3333333333333333703, 0.3219752754296894559, 0.3333333333333333703, 0.3219752754296894559, 0.3333333333333333703, 0.3219752754296894559, 0.3333333333333333703, 0.3219752754296894559, 0.3333333333333333703, 0.3219752754296894559, 0.3333333333333333703, 0.3219752754296894559, 0.3333333333333333703, 0.3219752754296894559, 0.3333333333333333703, 0.3219752754296894559, 0.3333333333333333703, 0.3219752754296894559, 0.3333333333333333703, 0.3219752754296894559, 0.3333333333333333703, 0.3219752754296894559, 0.3333333333333333703, 0.3219752754296894559, 0.3333333333333333703, 0.3219752754296894559, 0.3333333333333333703, 0.3219752754296894559, 0.3333333333333333703, 0.3219752754296894559, 0.3333333333333333703, 0.3219752754296894559, 0.3333333333333333703, 0.3219752754296894559, 0.3333333333333333703, 0.3219752754296894559, 0.3333333333333333703, 0.3219752754296894559, 0.3333333333333333703, 0.3219752754296894559, 0.3333333333333333703, 0.3219752754296894559, 0.3333333333333333703, 0.3219752754296894559, 0.3333333333333333703, 0.3219752754296894559, 0.3333333333333333703, 0.3219752754296894559, 0.3333333333333333703, 0.3219752754296894559, 0.3333333333333333703, 0.3219752754296894559, 0.3333333333333333703, 0.3219752754296894559, 0.3333333333333333703, 0.3219752754296894559, 0.3333333333333333703, 0.3219752754296894559, 0.3333333333333333703, 0.3219752754296894559, 0.3333333333333333703, 0.3219752754296894559, 0.3333333333333333703, 0.3219752754296894559, 0.3333333333333333703, 0.3219752754296894559, 0.3333333333333333703, 0.3219752754296894559, 0.3333333333333333703, 0.3219752754296894559, 0.3333333333333333703, 0.3219752754296894559, 0.3333333333333333703, 0.3219752754296894559, 0.3333333333333333703, 0.3219752754296894559, 0.3333333333333333703, 0.3219752754296894559, 0.3333333333333333703, 0.3219752754296894559, 0.3333333333333333703, 0.3219752754296894559, 0.3333333333333333703, 0.3219752754296894559, 0.3333333333333333703, 0.3219752754296894559, 0.3333333333333333703, 0.3219752754296894559, 0.3333333333333333703, 0.3219752754296894559, 0.3333333333333333703, 0.3219752754296894559, 0.3333333333333333703, 0.3219752754296894559, 0.3333333333333333703, 0.3219752754296894559, 0.3333333333333333703, 0.3219752754296894559, 0.3333333333333333703, 0.3219752754296894559, 0.3333333333333333703, 0.3219752754296894559, 0.3333333333333333703, 0.3219752754296894559, 0.3333333333333333703, 0.3219752754296894559, 0.3333333333333333703, 0.3219752754296894559, 0.3333333333333333703, 0.3219752754296894559, 0.3333333333333333703, 0.3219752754296894559, 0.3333333333333333703, 0.3219752754296894559, 0.3333333333333333703, 0.3219752754296894559, 0.3333333333333333703, 0.3219752754296894559, 0.3333333333333333703, 0.3219752754296894559, 0.3333333333333333703, 0.3219752754296894559, 0.3333333333333333703, 0.3219752754296894559, 0.3333333333333333703, 0.3219752754296894559, 0.3333333333333333703, 0.3219752754296894559, 0.3333333333333333703, 0.3219752754296894559, 0.3333333333333333703, 0.3219752754296894559, 0.3333333333333333703, 0.3219752754296894559, 0.3333333333333333703, 0.3219752754296894559, 0.3333333333333333703, 0.3219752754296894559, 0.3333333333333333703, 0.3219752754296894559, 0.3333333333333333703, 0.3219752754296894559, 0.3333333333333333703, 0.3219752754296894559, 0.3333333333333333703, 0.3219752754296894559, 0.3333333333333333703, 0.3219752754296894559, 0.3333333333333333703, 0.3219752754296894559, 0.3333333333333333703, 0.3219752754296894559, 0.3333333333333333703, 0.3219752754296894559, 0.3333333333333333703, 0.3219752754296894559, 0.3333333333333333703, 0.3219752754296894559, 0.3333333333333333703, 0.3219752754296894559, 0.3333333333333333703, 0.3219752754296894559, 0.3333333333333333703, 0.3219752754296894559, 0.3333333333333333703, 0.3219752754296894559, 0.3333333333333333703, 0.3219752754296894559, 0.3333333333333333703, 0.3219752754296894559, 0.3333333333333333703, 0.3219752754296894559, 0.3333333333333333703, 0.3219752754296894559, 0.3333333333333333703, 0.3219752754296894559, 0.3333333333333333703, 0.3219752754296894559, 0.3333333333333333703, 0.3219752754296894559, 0.3333333333333333703, 0.3219752754296894559, 0.3333333333333333703, 0.3219752754296894559, 0.3333333333333333703, 0.3219752754296894559, 0.3333333333333333703, 0.3219752754296894559, 0.3333333333333333703, 0.3219752754296894559, 0.3333333333333333703, 0.3219752754296894559, 0.3333333333333333703, 0.3219752754296894559, 0.3333333333333333703, 0.3219752754296894559, 0.3333333333333333703, 0.3219752754296894559, 0.3333333333333333703, 0.3219752754296894559, 0.3333333333333333703, 0.3219752754296894559, 0.3333333333333333703, 0.3219752754296894559, 0.3333333333333333703, 0.3219752754296894559, 0.3333333333333333703, 0.3219752754296894559, 0.3333333333333333703, 0.3219752754296894559, 0.3333333333333333703, 0.3219752754296894559, 0.3333333333333333703, 0.3219752754296894559, 0.3333333333333333703, 0.3219752754296894559, 0.3333333333333333703, 0.3219752754296894559, 0.3333333333333333703, 0.3219752754296894559, 0.3333333333333333703, 0.3219752754296894559, 0.3333333333333333703, 0.3219752754296894559, 0.3333333333333333703, 0.3219752754296894559, 0.3333333333333333703),
 ( 0.3333333333333333703, 0.3219752754296894559, 0.3333333333333333703, 0.3219752754296894559, 0.3333333333333333703, 0.3219752754296894559, 0.3333333333333333703, 0.3219752754296894559, 0.3333333333333333703, 0.3219752754296894559, 0.3333333333333333703, 0.3219752754296894559, 0.3333333333333333703, 0.3219752754296894559, 0.3333333333333333703, 0.3219752754296894559, 0.3333333333333333703, 0.3219752754296894559, 0.3333333333333333703, 0.3219752754296894559, 0.3333333333333333703, 0.3219752754296894559, 0.3333333333333333703, 0.3219752754296894559, 0.3333333333333333703, 0.3219752754296894559, 0.3333333333333333703, 0.3219752754296894559, 0.3333333333333333703, 0.3219752754296894559, 0.3333333333333333703, 0.3219752754296894559, 0.3333333333333333703, 0.3219752754296894559, 0.3333333333333333703, 0.3219752754296894559, 0.3333333333333333703, 0.3219752754296894559, 0.3333333333333333703, 0.3219752754296894559, 0.3333333333333333703, 0.3219752754296894559, 0.3333333333333333703, 0.3219752754296894559, 0.3333333333333333703, 0.3219752754296894559, 0.3333333333333333703, 0.3219752754296894559, 0.3333333333333333703, 0.3219752754296894559, 0.3333333333333333703, 0.3219752754296894559, 0.3333333333333333703, 0.3219752754296894559, 0.3333333333333333703, 0.3219752754296894559, 0.3333333333333333703, 0.3219752754296894559, 0.3333333333333333703, 0.3219752754296894559, 0.3333333333333333703, 0.3219752754296894559, 0.3333333333333333703, 0.3219752754296894559, 0.3333333333333333703, 0.3219752754296894559, 0.3333333333333333703, 0.3219752754296894559, 0.3333333333333333703, 0.3219752754296894559, 0.3333333333333333703, 0.3219752754296894559, 0.3333333333333333703, 0.3219752754296894559, 0.3333333333333333703, 0.3219752754296894559, 0.3333333333333333703, 0.3219752754296894559, 0.3333333333333333703, 0.3219752754296894559, 0.3333333333333333703, 0.3219752754296894559, 0.3333333333333333703, 0.3219752754296894559, 0.3333333333333333703, 0.3219752754296894559, 0.3333333333333333703, 0.3219752754296894559, 0.3333333333333333703, 0.3219752754296894559, 0.3333333333333333703, 0.3219752754296894559, 0.3333333333333333703, 0.3219752754296894559, 0.3333333333333333703, 0.3219752754296894559, 0.3333333333333333703, 0.3219752754296894559, 0.3333333333333333703, 0.3219752754296894559, 0.3333333333333333703, 0.3219752754296894559, 0.3333333333333333703, 0.3219752754296894559, 0.3333333333333333703, 0.3219752754296894559, 0.3333333333333333703, 0.3219752754296894559, 0.3333333333333333703, 0.3219752754296894559, 0.3333333333333333703, 0.3219752754296894559, 0.3333333333333333703, 0.3219752754296894559, 0.3333333333333333703, 0.3219752754296894559, 0.3333333333333333703, 0.3219752754296894559, 0.3333333333333333703, 0.3219752754296894559, 0.3333333333333333703, 0.3219752754296894559, 0.3333333333333333703, 0.3219752754296894559, 0.3333333333333333703, 0.3219752754296894559, 0.3333333333333333703, 0.3219752754296894559, 0.3333333333333333703, 0.3219752754296894559, 0.3333333333333333703, 0.3219752754296894559, 0.3333333333333333703, 0.3219752754296894559, 0.3333333333333333703, 0.3219752754296894559, 0.3333333333333333703, 0.3219752754296894559, 0.3333333333333333703, 0.3219752754296894559, 0.3333333333333333703, 0.3219752754296894559, 0.3333333333333333703, 0.3219752754296894559, 0.3333333333333333703, 0.3219752754296894559, 0.3333333333333333703, 0.3219752754296894559, 0.3333333333333333703, 0.3219752754296894559, 0.3333333333333333703, 0.3219752754296894559, 0.3333333333333333703, 0.3219752754296894559, 0.3333333333333333703, 0.3219752754296894559, 0.3333333333333333703, 0.3219752754296894559, 0.3333333333333333703, 0.3219752754296894559, 0.3333333333333333703, 0.3219752754296894559, 0.3333333333333333703, 0.3219752754296894559, 0.3333333333333333703, 0.3219752754296894559, 0.3333333333333333703, 0.3219752754296894559, 0.3333333333333333703, 0.3219752754296894559, 0.3333333333333333703, 0.3219752754296894559, 0.3333333333333333703, 0.3219752754296894559, 0.3333333333333333703, 0.3219752754296894559, 0.3333333333333333703, 0.3219752754296894559, 0.3333333333333333703, 0.3219752754296894559, 0.3333333333333333703, 0.3219752754296894559, 0.3333333333333333703, 0.3219752754296894559, 0.3333333333333333703, 0.3219752754296894559, 0.3333333333333333703, 0.3219752754296894559, 0.3333333333333333703, 0.3219752754296894559, 0.3333333333333333703, 0.3219752754296894559, 0.3333333333333333703, 0.3219752754296894559, 0.3333333333333333703, 0.3219752754296894559, 0.3333333333333333703, 0.3219752754296894559, 0.3333333333333333703, 0.3219752754296894559, 0.3333333333333333703, 0.3219752754296894559, 0.3333333333333333703, 0.3219752754296894559, 0.3333333333333333703, 0.3219752754296894559, 0.3333333333333333703, 0.3219752754296894559, 0.3333333333333333703, 0.3219752754296894559, 0.3333333333333333703, 0.3219752754296894559, 0.3333333333333333703, 0.3219752754296894559, 0.3333333333333333703, 0.3219752754296894559, 0.3333333333333333703, 0.3219752754296894559, 0.3333333333333333703, 0.3219752754296894559, 0.3333333333333333703, 0.3219752754296894559, 0.3333333333333333703, 0.3219752754296894559, 0.3333333333333333703, 0.3219752754296894559, 0.3333333333333333703, 0.3219752754296894559, 0.3333333333333333703, 0.3219752754296894559, 0.3333333333333333703, 0.3219752754296894559, 0.3333333333333333703, 0.3219752754296894559, 0.3333333333333333703, 0.3219752754296894559, 0.3333333333333333703, 0.3219752754296894559, 0.3333333333333333703, 0.3219752754296894559, 0.3333333333333333703, 0.3219752754296894559, 0.3333333333333333703, 0.3219752754296894559, 0.3333333333333333703, 0.3219752754296894559, 0.3333333333333333703, 0.3219752754296894559, 0.3333333333333333703, 0.3219752754296894559, 0.3333333333333333703, 0.3219752754296894559, 0.3333333333333333703, 0.3219752754296894559, 0.3333333333333333703, 0.3219752754296894559, 0.3333333333333333703, 0.3219752754296894559, 0.3333333333333333703, 0.3219752754296894559, 0.3333333333333333703, 0.3219752754296894559, 0.3333333333333333703, 0.3219752754296894559, 0.3333333333333333703, 0.3219752754296894559, 0.3333333333333333703, 0.3219752754296894559, 0.3333333333333333703, 0.3219752754296894559, 0.3333333333333333703, 0.3219752754296894559, 0.3333333333333333703, 0.3219752754296894559, 0.3333333333333333703, 0.3219752754296894559, 0.3333333333333333703, 0.3219752754296894559, 0.3333333333333333703, 0.3219752754296894559, 0.3333333333333333703, 0.3219752754296894559, 0.3333333333333333703, 0.3219752754296894559, 0.3333333333333333703, 0.3219752754296894559, 0.3333333333333333703, 0.3219752754296894559, 0.3333333333333333703, 0.3219752754296894559, 0.3333333333333333703, 0.3219752754296894559, 0.3333333333333333703, 0.3219752754296894559, 0.3333333333333333703, 0.3219752754296894559, 0.3333333333333333703, 0.3219752754296894559, 0.3333333333333333703, 0.3219752754296894559, 0.3333333333333333703, 0.3219752754296894559, 0.3333333333333333703, 0.3219752754296894559, 0.3333333333333333703, 0.3219752754296894559, 0.3333333333333333703, 0.3219752754296894559, 0.3333333333333333703, 0.3219752754296894559, 0.3333333333333333703, 0.3219752754296894559, 0.3333333333333333703, 0.3219752754296894559, 0.3333333333333333703, 0.3219752754296894559, 0.3333333333333333703, 0.3219752754296894559, 0.3333333333333333703, 0.3219752754296894559, 0.3333333333333333703, 0.3219752754296894559, 0.3333333333333333703, 0.3219752754296894559, 0.3333333333333333703, 0.3219752754296894559, 0.3333333333333333703, 0.3219752754296894559, 0.3333333333333333703, 0.3219752754296894559, 0.3333333333333333703, 0.3219752754296894559, 0.3333333333333333703, 0.3219752754296894559, 0.3333333333333333703, 0.3219752754296894559, 0.3333333333333333703, 0.3219752754296894559, 0.3333333333333333703, 0.3219752754296894559, 0.3333333333333333703, 0.3219752754296894559, 0.3333333333333333703, 0.3219752754296894559, 0.3333333333333333703, 0.3219752754296894559, 0.3333333333333333703, 0.3219752754296894559, 0.3333333333333333703, 0.3219752754296894559, 0.3333333333333333703, 0.3219752754296894559, 0.3333333333333333703, 0.3219752754296894559, 0.3333333333333333703, 0.3219752754296894559, 0.3333333333333333703, 0.3219752754296894559, 0.3333333333333333703, 0.3219752754296894559, 0.3333333333333333703, 0.3219752754296894559, 0.3333333333333333703, 0.3219752754296894559, 0.3333333333333333703, 0.3219752754296894559, 0.3333333333333333703, 0.3219752754296894559, 0.3333333333333333703, 0.3219752754296894559, 0.3333333333333333703, 0.3219752754296894559, 0.3333333333333333703, 0.3219752754296894559, 0.3333333333333333703, 0.3219752754296894559, 0.3333333333333333703, 0.3219752754296894559, 0.3333333333333333703, 0.3219752754296894559, 0.3333333333333333703, 0.3219752754296894559, 0.3333333333333333703, 0.3219752754296894559, 0.3333333333333333703, 0.3219752754296894559, 0.3333333333333333703, 0.3219752754296894559, 0.3333333333333333703, 0.3219752754296894559, 0.3333333333333333703, 0.3219752754296894559, 0.3333333333333333703, 0.3219752754296894559, 0.3333333333333333703, 0.3219752754296894559, 0.3333333333333333703, 0.3219752754296894559, 0.3333333333333333703, 0.3219752754296894559, 0.3333333333333333703, 0.3219752754296894559, 0.3333333333333333703, 0.3219752754296894559, 0.3333333333333333703, 0.3219752754296894559, 0.3333333333333333703, 0.3219752754296894559, 0.3333333333333333703, 0.3219752754296894559, 0.3333333333333333703, 0.3219752754296894559, 0.3333333333333333703, 0.3219752754296894559, 0.3333333333333333703, 0.3219752754296894559, 0.3333333333333333703, 0.3219752754296894559, 0.3333333333333333703, 0.3219752754296894559, 0.3333333333333333703, 0.3219752754296894559, 0.3333333333333333703, 0.3219752754296894559, 0.3333333333333333703, 0.3219752754296894559, 0.3333333333333333703, 0.3219752754296894559, 0.3333333333333333703, 0.3219752754296894559, 0.3333333333333333703, 0.3219752754296894559, 0.3333333333333333703, 0.3219752754296894559, 0.3333333333333333703, 0.3219752754296894559, 0.3333333333333333703, 0.3219752754296894559, 0.3333333333333333703, 0.3219752754296894559, 0.3333333333333333703, 0.3219752754296894559, 0.3333333333333333703, 0.3219752754296894559, 0.3333333333333333703, 0.3219752754296894559, 0.3333333333333333703, 0.3219752754296894559, 0.3333333333333333703, 0.3219752754296894559, 0.3333333333333333703, 0.3219752754296894559, 0.3333333333333333703, 0.3219752754296894559, 0.3333333333333333703, 0.3219752754296894559, 0.3333333333333333703),
 ( 1.000000000000000000, 0.9659258262890683122, 1.000000000000000000, 0.9659258262890683122, 1.000000000000000000, 0.9659258262890683122, 1.000000000000000000, 0.9659258262890683122, 1.000000000000000000, 0.9659258262890683122, 1.000000000000000000, 0.9659258262890683122, 1.000000000000000000, 0.9659258262890683122, 1.000000000000000000, 0.9659258262890683122, 1.000000000000000000, 0.9659258262890683122, 1.000000000000000000, 0.9659258262890683122, 1.000000000000000000, 0.9659258262890683122, 1.000000000000000000, 0.9659258262890683122, 1.000000000000000000, 0.9659258262890683122, 1.000000000000000000, 0.9659258262890683122, 1.000000000000000000, 0.9659258262890683122, 1.000000000000000000, 0.9659258262890683122, 1.000000000000000000, 0.9659258262890683122, 1.000000000000000000, 0.9659258262890683122, 1.000000000000000000, 0.9659258262890683122, 1.000000000000000000, 0.9659258262890683122, 1.000000000000000000, 0.9659258262890683122, 1.000000000000000000, 0.9659258262890683122, 1.000000000000000000, 0.9659258262890683122, 1.000000000000000000, 0.9659258262890683122, 1.000000000000000000, 0.9659258262890683122, 1.000000000000000000, 0.9659258262890683122, 1.000000000000000000, 0.9659258262890683122, 1.000000000000000000, 0.9659258262890683122, 1.000000000000000000, 0.9659258262890683122, 1.000000000000000000, 0.9659258262890683122, 1.000000000000000000, 0.9659258262890683122, 1.000000000000000000, 0.9659258262890683122, 1.000000000000000000, 0.9659258262890683122, 1.000000000000000000, 0.9659258262890683122, 1.000000000000000000, 0.9659258262890683122, 1.000000000000000000, 0.9659258262890683122, 1.000000000000000000, 0.9659258262890683122, 1.000000000000000000, 0.9659258262890683122, 1.000000000000000000, 0.9659258262890683122, 1.000000000000000000, 0.9659258262890683122, 1.000000000000000000, 0.9659258262890683122, 1.000000000000000000, 0.9659258262890683122, 1.000000000000000000, 0.9659258262890683122, 1.000000000000000000, 0.9659258262890683122, 1.000000000000000000, 0.9659258262890683122, 1.000000000000000000, 0.9659258262890683122, 1.000000000000000000, 0.9659258262890683122, 1.000000000000000000, 0.9659258262890683122, 1.000000000000000000, 0.9659258262890683122, 1.000000000000000000, 0.9659258262890683122, 1.000000000000000000, 0.9659258262890683122, 1.000000000000000000, 0.9659258262890683122, 1.000000000000000000, 0.9659258262890683122, 1.000000000000000000, 0.9659258262890683122, 1.000000000000000000, 0.9659258262890683122, 1.000000000000000000, 0.9659258262890683122, 1.000000000000000000, 0.9659258262890683122, 1.000000000000000000, 0.9659258262890683122, 1.000000000000000000, 0.9659258262890683122, 1.000000000000000000, 0.9659258262890683122, 1.000000000000000000, 0.9659258262890683122, 1.000000000000000000, 0.9659258262890683122, 1.000000000000000000, 0.9659258262890683122, 1.000000000000000000, 0.9659258262890683122, 1.000000000000000000, 0.9659258262890683122, 1.000000000000000000, 0.9659258262890683122, 1.000000000000000000, 0.9659258262890683122, 1.000000000000000000, 0.9659258262890683122, 1.000000000000000000, 0.9659258262890683122, 1.000000000000000000, 0.9659258262890683122, 1.000000000000000000, 0.9659258262890683122, 1.000000000000000000, 0.9659258262890683122, 1.000000000000000000, 0.9659258262890683122, 1.000000000000000000, 0.9659258262890683122, 1.000000000000000000, 0.9659258262890683122, 1.000000000000000000, 0.9659258262890683122, 1.000000000000000000, 0.9659258262890683122, 1.000000000000000000, 0.9659258262890683122, 1.000000000000000000, 0.9659258262890683122, 1.000000000000000000, 0.9659258262890683122, 1.000000000000000000, 0.9659258262890683122, 1.000000000000000000, 0.9659258262890683122, 1.000000000000000000, 0.9659258262890683122, 1.000000000000000000, 0.9659258262890683122, 1.000000000000000000, 0.9659258262890683122, 1.000000000000000000, 0.9659258262890683122, 1.000000000000000000, 0.9659258262890683122, 1.000000000000000000, 0.9659258262890683122, 1.000000000000000000, 0.9659258262890683122, 1.000000000000000000, 0.9659258262890683122, 1.000000000000000000, 0.9659258262890683122, 1.000000000000000000, 0.9659258262890683122, 1.000000000000000000, 0.9659258262890683122, 1.000000000000000000, 0.9659258262890683122, 1.000000000000000000, 0.9659258262890683122, 1.000000000000000000, 0.9659258262890683122, 1.000000000000000000, 0.9659258262890683122, 1.000000000000000000, 0.9659258262890683122, 1.000000000000000000, 0.9659258262890683122, 1.000000000000000000, 0.9659258262890683122, 1.000000000000000000, 0.9659258262890683122, 1.000000000000000000, 0.9659258262890683122, 1.000000000000000000, 0.9659258262890683122, 1.000000000000000000, 0.9659258262890683122, 1.000000000000000000, 0.9659258262890683122, 1.000000000000000000, 0.9659258262890683122, 1.000000000000000000, 0.9659258262890683122, 1.000000000000000000, 0.9659258262890683122, 1.000000000000000000, 0.9659258262890683122, 1.000000000000000000, 0.9659258262890683122, 1.000000000000000000, 0.9659258262890683122, 1.000000000000000000, 0.9659258262890683122, 1.000000000000000000, 0.9659258262890683122, 1.000000000000000000, 0.9659258262890683122, 1.000000000000000000, 0.9659258262890683122, 1.000000000000000000, 0.9659258262890683122, 1.000000000000000000, 0.9659258262890683122, 1.000000000000000000, 0.9659258262890683122, 1.000000000000000000, 0.9659258262890683122, 1.000000000000000000, 0.9659258262890683122, 1.000000000000000000, 0.9659258262890683122, 1.000000000000000000, 0.9659258262890683122, 1.000000000000000000, 0.9659258262890683122, 1.000000000000000000, 0.9659258262890683122, 1.000000000000000000, 0.9659258262890683122, 1.000000000000000000, 0.9659258262890683122, 1.000000000000000000, 0.9659258262890683122, 1.000000000000000000, 0.9659258262890683122, 1.000000000000000000, 0.9659258262890683122, 1.000000000000000000, 0.9659258262890683122, 1.000000000000000000, 0.9659258262890683122, 1.000000000000000000, 0.9659258262890683122, 1.000000000000000000, 0.9659258262890683122, 1.000000000000000000, 0.9659258262890683122, 1.000000000000000000, 0.9659258262890683122, 1.000000000000000000, 0.9659258262890683122, 1.000000000000000000, 0.9659258262890683122, 1.000000000000000000, 0.9659258262890683122, 1.000000000000000000, 0.9659258262890683122, 1.000000000000000000, 0.9659258262890683122, 1.000000000000000000, 0.9659258262890683122, 1.000000000000000000, 0.9659258262890683122, 1.000000000000000000, 0.9659258262890683122, 1.000000000000000000, 0.9659258262890683122, 1.000000000000000000, 0.9659258262890683122, 1.000000000000000000, 0.9659258262890683122, 1.000000000000000000, 0.9659258262890683122, 1.000000000000000000, 0.9659258262890683122, 1.000000000000000000, 0.9659258262890683122, 1.000000000000000000, 0.9659258262890683122, 1.000000000000000000, 0.9659258262890683122, 1.000000000000000000, 0.9659258262890683122, 1.000000000000000000, 0.9659258262890683122, 1.000000000000000000, 0.9659258262890683122, 1.000000000000000000, 0.9659258262890683122, 1.000000000000000000, 0.9659258262890683122, 1.000000000000000000, 0.9659258262890683122, 1.000000000000000000, 0.9659258262890683122, 1.000000000000000000, 0.9659258262890683122, 1.000000000000000000, 0.9659258262890683122, 1.000000000000000000, 0.9659258262890683122, 1.000000000000000000, 0.9659258262890683122, 1.000000000000000000, 0.9659258262890683122, 1.000000000000000000, 0.9659258262890683122, 1.000000000000000000, 0.9659258262890683122, 1.000000000000000000, 0.9659258262890683122, 1.000000000000000000, 0.9659258262890683122, 1.000000000000000000, 0.9659258262890683122, 1.000000000000000000, 0.9659258262890683122, 1.000000000000000000, 0.9659258262890683122, 1.000000000000000000, 0.9659258262890683122, 1.000000000000000000, 0.9659258262890683122, 1.000000000000000000, 0.9659258262890683122, 1.000000000000000000, 0.9659258262890683122, 1.000000000000000000, 0.9659258262890683122, 1.000000000000000000, 0.9659258262890683122, 1.000000000000000000, 0.9659258262890683122, 1.000000000000000000, 0.9659258262890683122, 1.000000000000000000, 0.9659258262890683122, 1.000000000000000000, 0.9659258262890683122, 1.000000000000000000, 0.9659258262890683122, 1.000000000000000000, 0.9659258262890683122, 1.000000000000000000, 0.9659258262890683122, 1.000000000000000000, 0.9659258262890683122, 1.000000000000000000, 0.9659258262890683122, 1.000000000000000000, 0.9659258262890683122, 1.000000000000000000, 0.9659258262890683122, 1.000000000000000000, 0.9659258262890683122, 1.000000000000000000, 0.9659258262890683122, 1.000000000000000000, 0.9659258262890683122, 1.000000000000000000, 0.9659258262890683122, 1.000000000000000000, 0.9659258262890683122, 1.000000000000000000, 0.9659258262890683122, 1.000000000000000000, 0.9659258262890683122, 1.000000000000000000, 0.9659258262890683122, 1.000000000000000000, 0.9659258262890683122, 1.000000000000000000, 0.9659258262890683122, 1.000000000000000000, 0.9659258262890683122, 1.000000000000000000, 0.9659258262890683122, 1.000000000000000000, 0.9659258262890683122, 1.000000000000000000, 0.9659258262890683122, 1.000000000000000000, 0.9659258262890683122, 1.000000000000000000, 0.9659258262890683122, 1.000000000000000000, 0.9659258262890683122, 1.000000000000000000, 0.9659258262890683122, 1.000000000000000000, 0.9659258262890683122, 1.000000000000000000, 0.9659258262890683122, 1.000000000000000000, 0.9659258262890683122, 1.000000000000000000, 0.9659258262890683122, 1.000000000000000000, 0.9659258262890683122, 1.000000000000000000, 0.9659258262890683122, 1.000000000000000000, 0.9659258262890683122, 1.000000000000000000, 0.9659258262890683122, 1.000000000000000000, 0.9659258262890683122, 1.000000000000000000, 0.9659258262890683122, 1.000000000000000000, 0.9659258262890683122, 1.000000000000000000, 0.9659258262890683122, 1.000000000000000000, 0.9659258262890683122, 1.000000000000000000, 0.9659258262890683122, 1.000000000000000000, 0.9659258262890683122, 1.000000000000000000, 0.9659258262890683122, 1.000000000000000000, 0.9659258262890683122, 1.000000000000000000, 0.9659258262890683122, 1.000000000000000000, 0.9659258262890683122, 1.000000000000000000, 0.9659258262890683122, 1.000000000000000000, 0.9659258262890683122, 1.000000000000000000, 0.9659258262890683122, 1.000000000000000000, 0.9659258262890683122, 1.000000000000000000),
 ( 0.3333333333333333703, 0.3219752754296894559, 0.3333333333333333703, 0.3219752754296894559, 0.3333333333333333703, 0.3219752754296894559, 0.3333333333333333703, 0.3219752754296894559, 0.3333333333333333703, 0.3219752754296894559, 0.3333333333333333703, 0.3219752754296894559, 0.3333333333333333703, 0.3219752754296894559, 0.3333333333333333703, 0.3219752754296894559, 0.3333333333333333703, 0.3219752754296894559, 0.3333333333333333703, 0.3219752754296894559, 0.3333333333333333703, 0.3219752754296894559, 0.3333333333333333703, 0.3219752754296894559, 0.3333333333333333703, 0.3219752754296894559, 0.3333333333333333703, 0.3219752754296894559, 0.3333333333333333703, 0.3219752754296894559, 0.3333333333333333703, 0.3219752754296894559, 0.3333333333333333703, 0.3219752754296894559, 0.3333333333333333703, 0.3219752754296894559, 0.3333333333333333703, 0.3219752754296894559, 0.3333333333333333703, 0.3219752754296894559, 0.3333333333333333703, 0.3219752754296894559, 0.3333333333333333703, 0.3219752754296894559, 0.3333333333333333703, 0.3219752754296894559, 0.3333333333333333703, 0.3219752754296894559, 0.3333333333333333703, 0.3219752754296894559, 0.3333333333333333703, 0.3219752754296894559, 0.3333333333333333703, 0.3219752754296894559, 0.3333333333333333703, 0.3219752754296894559, 0.3333333333333333703, 0.3219752754296894559, 0.3333333333333333703, 0.3219752754296894559, 0.3333333333333333703, 0.3219752754296894559, 0.3333333333333333703, 0.3219752754296894559, 0.3333333333333333703, 0.3219752754296894559, 0.3333333333333333703, 0.3219752754296894559, 0.3333333333333333703, 0.3219752754296894559, 0.3333333333333333703, 0.3219752754296894559, 0.3333333333333333703, 0.3219752754296894559, 0.3333333333333333703, 0.3219752754296894559, 0.3333333333333333703, 0.3219752754296894559, 0.3333333333333333703, 0.3219752754296894559, 0.3333333333333333703, 0.3219752754296894559, 0.3333333333333333703, 0.3219752754296894559, 0.3333333333333333703, 0.3219752754296894559, 0.3333333333333333703, 0.3219752754296894559, 0.3333333333333333703, 0.3219752754296894559, 0.3333333333333333703, 0.3219752754296894559, 0.3333333333333333703, 0.3219752754296894559, 0.3333333333333333703, 0.3219752754296894559, 0.3333333333333333703, 0.3219752754296894559, 0.3333333333333333703, 0.3219752754296894559, 0.3333333333333333703, 0.3219752754296894559, 0.3333333333333333703, 0.3219752754296894559, 0.3333333333333333703, 0.3219752754296894559, 0.3333333333333333703, 0.3219752754296894559, 0.3333333333333333703, 0.3219752754296894559, 0.3333333333333333703, 0.3219752754296894559, 0.3333333333333333703, 0.3219752754296894559, 0.3333333333333333703, 0.3219752754296894559, 0.3333333333333333703, 0.3219752754296894559, 0.3333333333333333703, 0.3219752754296894559, 0.3333333333333333703, 0.3219752754296894559, 0.3333333333333333703, 0.3219752754296894559, 0.3333333333333333703, 0.3219752754296894559, 0.3333333333333333703, 0.3219752754296894559, 0.3333333333333333703, 0.3219752754296894559, 0.3333333333333333703, 0.3219752754296894559, 0.3333333333333333703, 0.3219752754296894559, 0.3333333333333333703, 0.3219752754296894559, 0.3333333333333333703, 0.3219752754296894559, 0.3333333333333333703, 0.3219752754296894559, 0.3333333333333333703, 0.3219752754296894559, 0.3333333333333333703, 0.3219752754296894559, 0.3333333333333333703, 0.3219752754296894559, 0.3333333333333333703, 0.3219752754296894559, 0.3333333333333333703, 0.3219752754296894559, 0.3333333333333333703, 0.3219752754296894559, 0.3333333333333333703, 0.3219752754296894559, 0.3333333333333333703, 0.3219752754296894559, 0.3333333333333333703, 0.3219752754296894559, 0.3333333333333333703, 0.3219752754296894559, 0.3333333333333333703, 0.3219752754296894559, 0.3333333333333333703, 0.3219752754296894559, 0.3333333333333333703, 0.3219752754296894559, 0.3333333333333333703, 0.3219752754296894559, 0.3333333333333333703, 0.3219752754296894559, 0.3333333333333333703, 0.3219752754296894559, 0.3333333333333333703, 0.3219752754296894559, 0.3333333333333333703, 0.3219752754296894559, 0.3333333333333333703, 0.3219752754296894559, 0.3333333333333333703, 0.3219752754296894559, 0.3333333333333333703, 0.3219752754296894559, 0.3333333333333333703, 0.3219752754296894559, 0.3333333333333333703, 0.3219752754296894559, 0.3333333333333333703, 0.3219752754296894559, 0.3333333333333333703, 0.3219752754296894559, 0.3333333333333333703, 0.3219752754296894559, 0.3333333333333333703, 0.3219752754296894559, 0.3333333333333333703, 0.3219752754296894559, 0.3333333333333333703, 0.3219752754296894559, 0.3333333333333333703, 0.3219752754296894559, 0.3333333333333333703, 0.3219752754296894559, 0.3333333333333333703, 0.3219752754296894559, 0.3333333333333333703, 0.3219752754296894559, 0.3333333333333333703, 0.3219752754296894559, 0.3333333333333333703, 0.3219752754296894559, 0.3333333333333333703, 0.3219752754296894559, 0.3333333333333333703, 0.3219752754296894559, 0.3333333333333333703, 0.3219752754296894559, 0.3333333333333333703, 0.3219752754296894559, 0.3333333333333333703, 0.3219752754296894559, 0.3333333333333333703, 0.3219752754296894559, 0.3333333333333333703, 0.3219752754296894559, 0.3333333333333333703, 0.3219752754296894559, 0.3333333333333333703, 0.3219752754296894559, 0.3333333333333333703, 0.3219752754296894559, 0.3333333333333333703, 0.3219752754296894559, 0.3333333333333333703, 0.3219752754296894559, 0.3333333333333333703, 0.3219752754296894559, 0.3333333333333333703, 0.3219752754296894559, 0.3333333333333333703, 0.3219752754296894559, 0.3333333333333333703, 0.3219752754296894559, 0.3333333333333333703, 0.3219752754296894559, 0.3333333333333333703, 0.3219752754296894559, 0.3333333333333333703, 0.3219752754296894559, 0.3333333333333333703, 0.3219752754296894559, 0.3333333333333333703, 0.3219752754296894559, 0.3333333333333333703, 0.3219752754296894559, 0.3333333333333333703, 0.3219752754296894559, 0.3333333333333333703, 0.3219752754296894559, 0.3333333333333333703, 0.3219752754296894559, 0.3333333333333333703, 0.3219752754296894559, 0.3333333333333333703, 0.3219752754296894559, 0.3333333333333333703, 0.3219752754296894559, 0.3333333333333333703, 0.3219752754296894559, 0.3333333333333333703, 0.3219752754296894559, 0.3333333333333333703, 0.3219752754296894559, 0.3333333333333333703, 0.3219752754296894559, 0.3333333333333333703, 0.3219752754296894559, 0.3333333333333333703, 0.3219752754296894559, 0.3333333333333333703, 0.3219752754296894559, 0.3333333333333333703, 0.3219752754296894559, 0.3333333333333333703, 0.3219752754296894559, 0.3333333333333333703, 0.3219752754296894559, 0.3333333333333333703, 0.3219752754296894559, 0.3333333333333333703, 0.3219752754296894559, 0.3333333333333333703, 0.3219752754296894559, 0.3333333333333333703, 0.3219752754296894559, 0.3333333333333333703, 0.3219752754296894559, 0.3333333333333333703, 0.3219752754296894559, 0.3333333333333333703, 0.3219752754296894559, 0.3333333333333333703, 0.3219752754296894559, 0.3333333333333333703, 0.3219752754296894559, 0.3333333333333333703, 0.3219752754296894559, 0.3333333333333333703, 0.3219752754296894559, 0.3333333333333333703, 0.3219752754296894559, 0.3333333333333333703, 0.3219752754296894559, 0.3333333333333333703, 0.3219752754296894559, 0.3333333333333333703, 0.3219752754296894559, 0.3333333333333333703, 0.3219752754296894559, 0.3333333333333333703, 0.3219752754296894559, 0.3333333333333333703, 0.3219752754296894559, 0.3333333333333333703, 0.3219752754296894559, 0.3333333333333333703, 0.3219752754296894559, 0.3333333333333333703, 0.3219752754296894559, 0.3333333333333333703, 0.3219752754296894559, 0.3333333333333333703, 0.3219752754296894559, 0.3333333333333333703, 0.3219752754296894559, 0.3333333333333333703, 0.3219752754296894559, 0.3333333333333333703, 0.3219752754296894559, 0.3333333333333333703, 0.3219752754296894559, 0.3333333333333333703, 0.3219752754296894559, 0.3333333333333333703, 0.3219752754296894559, 0.3333333333333333703, 0.3219752754296894559, 0.3333333333333333703, 0.3219752754296894559, 0.3333333333333333703, 0.3219752754296894559, 0.3333333333333333703, 0.3219752754296894559, 0.3333333333333333703, 0.3219752754296894559, 0.3333333333333333703, 0.3219752754296894559, 0.3333333333333333703, 0.3219752754296894559, 0.3333333333333333703, 0.3219752754296894559, 0.3333333333333333703, 0.3219752754296894559, 0.3333333333333333703, 0.3219752754296894559, 0.3333333333333333703, 0.3219752754296894559, 0.3333333333333333703, 0.3219752754296894559, 0.3333333333333333703, 0.3219752754296894559, 0.3333333333333333703, 0.3219752754296894559, 0.3333333333333333703, 0.3219752754296894559, 0.3333333333333333703, 0.3219752754296894559, 0.3333333333333333703, 0.3219752754296894559, 0.3333333333333333703, 0.3219752754296894559, 0.3333333333333333703, 0.3219752754296894559, 0.3333333333333333703, 0.3219752754296894559, 0.3333333333333333703, 0.3219752754296894559, 0.3333333333333333703, 0.3219752754296894559, 0.3333333333333333703, 0.3219752754296894559, 0.3333333333333333703, 0.3219752754296894559, 0.3333333333333333703, 0.3219752754296894559, 0.3333333333333333703, 0.3219752754296894559, 0.3333333333333333703, 0.3219752754296894559, 0.3333333333333333703, 0.3219752754296894559, 0.3333333333333333703, 0.3219752754296894559, 0.3333333333333333703, 0.3219752754296894559, 0.3333333333333333703, 0.3219752754296894559, 0.3333333333333333703, 0.3219752754296894559, 0.3333333333333333703, 0.3219752754296894559, 0.3333333333333333703, 0.3219752754296894559, 0.3333333333333333703, 0.3219752754296894559, 0.3333333333333333703, 0.3219752754296894559, 0.3333333333333333703, 0.3219752754296894559, 0.3333333333333333703, 0.3219752754296894559, 0.3333333333333333703, 0.3219752754296894559, 0.3333333333333333703, 0.3219752754296894559, 0.3333333333333333703, 0.3219752754296894559, 0.3333333333333333703, 0.3219752754296894559, 0.3333333333333333703, 0.3219752754296894559, 0.3333333333333333703, 0.3219752754296894559, 0.3333333333333333703, 0.3219752754296894559, 0.3333333333333333703, 0.3219752754296894559, 0.3333333333333333703, 0.3219752754296894559, 0.3333333333333333703, 0.3219752754296894559, 0.3333333333333333703, 0.3219752754296894559, 0.3333333333333333703, 0.3219752754296894559, 0.3333333333333333703, 0.3219752754296894559, 0.3333333333333333703, 0.3219752754296894559, 0.3333333333333333703, 0.3219752754296894559, 0.3333333333333333703, 0.3219752754296894559, 0.3333333333333333703, 0.3219752754296894559, 0.3333333333333333703, 0.3219752754296894559, 0.3333333333333333703),
 ( 0.3333333333333333703, 0.3219752754296894559, 0.3333333333333333703, 0.3219752754296894559, 0.3333333333333333703, 0.3219752754296894559, 0.3333333333333333703, 0.3219752754296894559, 0.3333333333333333703, 0.3219752754296894559, 0.3333333333333333703, 0.3219752754296894559, 0.3333333333333333703, 0.3219752754296894559, 0.3333333333333333703, 0.3219752754296894559, 0.3333333333333333703, 0.3219752754296894559, 0.3333333333333333703, 0.3219752754296894559, 0.3333333333333333703, 0.3219752754296894559, 0.3333333333333333703, 0.3219752754296894559, 0.3333333333333333703, 0.3219752754296894559, 0.3333333333333333703, 0.3219752754296894559, 0.3333333333333333703, 0.3219752754296894559, 0.3333333333333333703, 0.3219752754296894559, 0.3333333333333333703, 0.3219752754296894559, 0.3333333333333333703, 0.3219752754296894559, 0.3333333333333333703, 0.3219752754296894559, 0.3333333333333333703, 0.3219752754296894559, 0.3333333333333333703, 0.3219752754296894559, 0.3333333333333333703, 0.3219752754296894559, 0.3333333333333333703, 0.3219752754296894559, 0.3333333333333333703, 0.3219752754296894559, 0.3333333333333333703, 0.3219752754296894559, 0.3333333333333333703, 0.3219752754296894559, 0.3333333333333333703, 0.3219752754296894559, 0.3333333333333333703, 0.3219752754296894559, 0.3333333333333333703, 0.3219752754296894559, 0.3333333333333333703, 0.3219752754296894559, 0.3333333333333333703, 0.3219752754296894559, 0.3333333333333333703, 0.3219752754296894559, 0.3333333333333333703, 0.3219752754296894559, 0.3333333333333333703, 0.3219752754296894559, 0.3333333333333333703, 0.3219752754296894559, 0.3333333333333333703, 0.3219752754296894559, 0.3333333333333333703, 0.3219752754296894559, 0.3333333333333333703, 0.3219752754296894559, 0.3333333333333333703, 0.3219752754296894559, 0.3333333333333333703, 0.3219752754296894559, 0.3333333333333333703, 0.3219752754296894559, 0.3333333333333333703, 0.3219752754296894559, 0.3333333333333333703, 0.3219752754296894559, 0.3333333333333333703, 0.3219752754296894559, 0.3333333333333333703, 0.3219752754296894559, 0.3333333333333333703, 0.3219752754296894559, 0.3333333333333333703, 0.3219752754296894559, 0.3333333333333333703, 0.3219752754296894559, 0.3333333333333333703, 0.3219752754296894559, 0.3333333333333333703, 0.3219752754296894559, 0.3333333333333333703, 0.3219752754296894559, 0.3333333333333333703, 0.3219752754296894559, 0.3333333333333333703, 0.3219752754296894559, 0.3333333333333333703, 0.3219752754296894559, 0.3333333333333333703, 0.3219752754296894559, 0.3333333333333333703, 0.3219752754296894559, 0.3333333333333333703, 0.3219752754296894559, 0.3333333333333333703, 0.3219752754296894559, 0.3333333333333333703, 0.3219752754296894559, 0.3333333333333333703, 0.3219752754296894559, 0.3333333333333333703, 0.3219752754296894559, 0.3333333333333333703, 0.3219752754296894559, 0.3333333333333333703, 0.3219752754296894559, 0.3333333333333333703, 0.3219752754296894559, 0.3333333333333333703, 0.3219752754296894559, 0.3333333333333333703, 0.3219752754296894559, 0.3333333333333333703, 0.3219752754296894559, 0.3333333333333333703, 0.3219752754296894559, 0.3333333333333333703, 0.3219752754296894559, 0.3333333333333333703, 0.3219752754296894559, 0.3333333333333333703, 0.3219752754296894559, 0.3333333333333333703, 0.3219752754296894559, 0.3333333333333333703, 0.3219752754296894559, 0.3333333333333333703, 0.3219752754296894559, 0.3333333333333333703, 0.3219752754296894559, 0.3333333333333333703, 0.3219752754296894559, 0.3333333333333333703, 0.3219752754296894559, 0.3333333333333333703, 0.3219752754296894559, 0.3333333333333333703, 0.3219752754296894559, 0.3333333333333333703, 0.3219752754296894559, 0.3333333333333333703, 0.3219752754296894559, 0.3333333333333333703, 0.3219752754296894559, 0.3333333333333333703, 0.3219752754296894559, 0.3333333333333333703, 0.3219752754296894559, 0.3333333333333333703, 0.3219752754296894559, 0.3333333333333333703, 0.3219752754296894559, 0.3333333333333333703, 0.3219752754296894559, 0.3333333333333333703, 0.3219752754296894559, 0.3333333333333333703, 0.3219752754296894559, 0.3333333333333333703, 0.3219752754296894559, 0.3333333333333333703, 0.3219752754296894559, 0.3333333333333333703, 0.3219752754296894559, 0.3333333333333333703, 0.3219752754296894559, 0.3333333333333333703, 0.3219752754296894559, 0.3333333333333333703, 0.3219752754296894559, 0.3333333333333333703, 0.3219752754296894559, 0.3333333333333333703, 0.3219752754296894559, 0.3333333333333333703, 0.3219752754296894559, 0.3333333333333333703, 0.3219752754296894559, 0.3333333333333333703, 0.3219752754296894559, 0.3333333333333333703, 0.3219752754296894559, 0.3333333333333333703, 0.3219752754296894559, 0.3333333333333333703, 0.3219752754296894559, 0.3333333333333333703, 0.3219752754296894559, 0.3333333333333333703, 0.3219752754296894559, 0.3333333333333333703, 0.3219752754296894559, 0.3333333333333333703, 0.3219752754296894559, 0.3333333333333333703, 0.3219752754296894559, 0.3333333333333333703, 0.3219752754296894559, 0.3333333333333333703, 0.3219752754296894559, 0.3333333333333333703, 0.3219752754296894559, 0.3333333333333333703, 0.3219752754296894559, 0.3333333333333333703, 0.3219752754296894559, 0.3333333333333333703, 0.3219752754296894559, 0.3333333333333333703, 0.3219752754296894559, 0.3333333333333333703, 0.3219752754296894559, 0.3333333333333333703, 0.3219752754296894559, 0.3333333333333333703, 0.3219752754296894559, 0.3333333333333333703, 0.3219752754296894559, 0.3333333333333333703, 0.3219752754296894559, 0.3333333333333333703, 0.3219752754296894559, 0.3333333333333333703, 0.3219752754296894559, 0.3333333333333333703, 0.3219752754296894559, 0.3333333333333333703, 0.3219752754296894559, 0.3333333333333333703, 0.3219752754296894559, 0.3333333333333333703, 0.3219752754296894559, 0.3333333333333333703, 0.3219752754296894559, 0.3333333333333333703, 0.3219752754296894559, 0.3333333333333333703, 0.3219752754296894559, 0.3333333333333333703, 0.3219752754296894559, 0.3333333333333333703, 0.3219752754296894559, 0.3333333333333333703, 0.3219752754296894559, 0.3333333333333333703, 0.3219752754296894559, 0.3333333333333333703, 0.3219752754296894559, 0.3333333333333333703, 0.3219752754296894559, 0.3333333333333333703, 0.3219752754296894559, 0.3333333333333333703, 0.3219752754296894559, 0.3333333333333333703, 0.3219752754296894559, 0.3333333333333333703, 0.3219752754296894559, 0.3333333333333333703, 0.3219752754296894559, 0.3333333333333333703, 0.3219752754296894559, 0.3333333333333333703, 0.3219752754296894559, 0.3333333333333333703, 0.3219752754296894559, 0.3333333333333333703, 0.3219752754296894559, 0.3333333333333333703, 0.3219752754296894559, 0.3333333333333333703, 0.3219752754296894559, 0.3333333333333333703, 0.3219752754296894559, 0.3333333333333333703, 0.3219752754296894559, 0.3333333333333333703, 0.3219752754296894559, 0.3333333333333333703, 0.3219752754296894559, 0.3333333333333333703, 0.3219752754296894559, 0.3333333333333333703, 0.3219752754296894559, 0.3333333333333333703, 0.3219752754296894559, 0.3333333333333333703, 0.3219752754296894559, 0.3333333333333333703, 0.3219752754296894559, 0.3333333333333333703, 0.3219752754296894559, 0.3333333333333333703, 0.3219752754296894559, 0.3333333333333333703, 0.3219752754296894559, 0.3333333333333333703, 0.3219752754296894559, 0.3333333333333333703, 0.3219752754296894559, 0.3333333333333333703, 0.3219752754296894559, 0.3333333333333333703, 0.3219752754296894559, 0.3333333333333333703, 0.3219752754296894559, 0.3333333333333333703, 0.3219752754296894559, 0.3333333333333333703, 0.3219752754296894559, 0.3333333333333333703, 0.3219752754296894559, 0.3333333333333333703, 0.3219752754296894559, 0.3333333333333333703, 0.3219752754296894559, 0.3333333333333333703, 0.3219752754296894559, 0.3333333333333333703, 0.3219752754296894559, 0.3333333333333333703, 0.3219752754296894559, 0.3333333333333333703, 0.3219752754296894559, 0.3333333333333333703, 0.3219752754296894559, 0.3333333333333333703, 0.3219752754296894559, 0.3333333333333333703, 0.3219752754296894559, 0.3333333333333333703, 0.3219752754296894559, 0.3333333333333333703, 0.3219752754296894559, 0.3333333333333333703, 0.3219752754296894559, 0.3333333333333333703, 0.3219752754296894559, 0.3333333333333333703, 0.3219752754296894559, 0.3333333333333333703, 0.3219752754296894559, 0.3333333333333333703, 0.3219752754296894559, 0.3333333333333333703, 0.3219752754296894559, 0.3333333333333333703, 0.3219752754296894559, 0.3333333333333333703, 0.3219752754296894559, 0.3333333333333333703, 0.3219752754296894559, 0.3333333333333333703, 0.3219752754296894559, 0.3333333333333333703, 0.3219752754296894559, 0.3333333333333333703, 0.3219752754296894559, 0.3333333333333333703, 0.3219752754296894559, 0.3333333333333333703, 0.3219752754296894559, 0.3333333333333333703, 0.3219752754296894559, 0.3333333333333333703, 0.3219752754296894559, 0.3333333333333333703, 0.3219752754296894559, 0.3333333333333333703, 0.3219752754296894559, 0.3333333333333333703, 0.3219752754296894559, 0.3333333333333333703, 0.3219752754296894559, 0.3333333333333333703, 0.3219752754296894559, 0.3333333333333333703, 0.3219752754296894559, 0.3333333333333333703, 0.3219752754296894559, 0.3333333333333333703, 0.3219752754296894559, 0.3333333333333333703, 0.3219752754296894559, 0.3333333333333333703, 0.3219752754296894559, 0.3333333333333333703, 0.3219752754296894559, 0.3333333333333333703, 0.3219752754296894559, 0.3333333333333333703, 0.3219752754296894559, 0.3333333333333333703, 0.3219752754296894559, 0.3333333333333333703, 0.3219752754296894559, 0.3333333333333333703, 0.3219752754296894559, 0.3333333333333333703, 0.3219752754296894559, 0.3333333333333333703, 0.3219752754296894559, 0.3333333333333333703, 0.3219752754296894559, 0.3333333333333333703, 0.3219752754296894559, 0.3333333333333333703, 0.3219752754296894559, 0.3333333333333333703, 0.3219752754296894559, 0.3333333333333333703, 0.3219752754296894559, 0.3333333333333333703, 0.3219752754296894559, 0.3333333333333333703, 0.3219752754296894559, 0.3333333333333333703, 0.3219752754296894559, 0.3333333333333333703, 0.3219752754296894559, 0.3333333333333333703, 0.3219752754296894559, 0.3333333333333333703, 0.3219752754296894559, 0.3333333333333333703, 0.3219752754296894559, 0.3333333333333333703, 0.3219752754296894559, 0.3333333333333333703, 0.3219752754296894559, 0.3333333333333333703, 0.3219752754296894559, 0.3333333333333333703, 0.3219752754296894559, 0.3333333333333333703, 0.3219752754296894559, 0.3333333333333333703),
 ( 1.000000000000000000, 0.9659258262890683122, 1.000000000000000000, 0.9659258262890683122, 1.000000000000000000, 0.9659258262890683122, 1.000000000000000000, 0.9659258262890683122, 1.000000000000000000, 0.9659258262890683122, 1.000000000000000000, 0.9659258262890683122, 1.000000000000000000, 0.9659258262890683122, 1.000000000000000000, 0.9659258262890683122, 1.000000000000000000, 0.9659258262890683122, 1.000000000000000000, 0.9659258262890683122, 1.000000000000000000, 0.9659258262890683122, 1.000000000000000000, 0.9659258262890683122, 1.000000000000000000, 0.9659258262890683122, 1.000000000000000000, 0.9659258262890683122, 1.000000000000000000, 0.9659258262890683122, 1.000000000000000000, 0.9659258262890683122, 1.000000000000000000, 0.9659258262890683122, 1.000000000000000000, 0.9659258262890683122, 1.000000000000000000, 0.9659258262890683122, 1.000000000000000000, 0.9659258262890683122, 1.000000000000000000, 0.9659258262890683122, 1.000000000000000000, 0.9659258262890683122, 1.000000000000000000, 0.9659258262890683122, 1.000000000000000000, 0.9659258262890683122, 1.000000000000000000, 0.9659258262890683122, 1.000000000000000000, 0.9659258262890683122, 1.000000000000000000, 0.9659258262890683122, 1.000000000000000000, 0.9659258262890683122, 1.000000000000000000, 0.9659258262890683122, 1.000000000000000000, 0.9659258262890683122, 1.000000000000000000, 0.9659258262890683122, 1.000000000000000000, 0.9659258262890683122, 1.000000000000000000, 0.9659258262890683122, 1.000000000000000000, 0.9659258262890683122, 1.000000000000000000, 0.9659258262890683122, 1.000000000000000000, 0.9659258262890683122, 1.000000000000000000, 0.9659258262890683122, 1.000000000000000000, 0.9659258262890683122, 1.000000000000000000, 0.9659258262890683122, 1.000000000000000000, 0.9659258262890683122, 1.000000000000000000, 0.9659258262890683122, 1.000000000000000000, 0.9659258262890683122, 1.000000000000000000, 0.9659258262890683122, 1.000000000000000000, 0.9659258262890683122, 1.000000000000000000, 0.9659258262890683122, 1.000000000000000000, 0.9659258262890683122, 1.000000000000000000, 0.9659258262890683122, 1.000000000000000000, 0.9659258262890683122, 1.000000000000000000, 0.9659258262890683122, 1.000000000000000000, 0.9659258262890683122, 1.000000000000000000, 0.9659258262890683122, 1.000000000000000000, 0.9659258262890683122, 1.000000000000000000, 0.9659258262890683122, 1.000000000000000000, 0.9659258262890683122, 1.000000000000000000, 0.9659258262890683122, 1.000000000000000000, 0.9659258262890683122, 1.000000000000000000, 0.9659258262890683122, 1.000000000000000000, 0.9659258262890683122, 1.000000000000000000, 0.9659258262890683122, 1.000000000000000000, 0.9659258262890683122, 1.000000000000000000, 0.9659258262890683122, 1.000000000000000000, 0.9659258262890683122, 1.000000000000000000, 0.9659258262890683122, 1.000000000000000000, 0.9659258262890683122, 1.000000000000000000, 0.9659258262890683122, 1.000000000000000000, 0.9659258262890683122, 1.000000000000000000, 0.9659258262890683122, 1.000000000000000000, 0.9659258262890683122, 1.000000000000000000, 0.9659258262890683122, 1.000000000000000000, 0.9659258262890683122, 1.000000000000000000, 0.9659258262890683122, 1.000000000000000000, 0.9659258262890683122, 1.000000000000000000, 0.9659258262890683122, 1.000000000000000000, 0.9659258262890683122, 1.000000000000000000, 0.9659258262890683122, 1.000000000000000000, 0.9659258262890683122, 1.000000000000000000, 0.9659258262890683122, 1.000000000000000000, 0.9659258262890683122, 1.000000000000000000, 0.9659258262890683122, 1.000000000000000000, 0.9659258262890683122, 1.000000000000000000, 0.9659258262890683122, 1.000000000000000000, 0.9659258262890683122, 1.000000000000000000, 0.9659258262890683122, 1.000000000000000000, 0.9659258262890683122, 1.000000000000000000, 0.9659258262890683122, 1.000000000000000000, 0.9659258262890683122, 1.000000000000000000, 0.9659258262890683122, 1.000000000000000000, 0.9659258262890683122, 1.000000000000000000, 0.9659258262890683122, 1.000000000000000000, 0.9659258262890683122, 1.000000000000000000, 0.9659258262890683122, 1.000000000000000000, 0.9659258262890683122, 1.000000000000000000, 0.9659258262890683122, 1.000000000000000000, 0.9659258262890683122, 1.000000000000000000, 0.9659258262890683122, 1.000000000000000000, 0.9659258262890683122, 1.000000000000000000, 0.9659258262890683122, 1.000000000000000000, 0.9659258262890683122, 1.000000000000000000, 0.9659258262890683122, 1.000000000000000000, 0.9659258262890683122, 1.000000000000000000, 0.9659258262890683122, 1.000000000000000000, 0.9659258262890683122, 1.000000000000000000, 0.9659258262890683122, 1.000000000000000000, 0.9659258262890683122, 1.000000000000000000, 0.9659258262890683122, 1.000000000000000000, 0.9659258262890683122, 1.000000000000000000, 0.9659258262890683122, 1.000000000000000000, 0.9659258262890683122, 1.000000000000000000, 0.9659258262890683122, 1.000000000000000000, 0.9659258262890683122, 1.000000000000000000, 0.9659258262890683122, 1.000000000000000000, 0.9659258262890683122, 1.000000000000000000, 0.9659258262890683122, 1.000000000000000000, 0.9659258262890683122, 1.000000000000000000, 0.9659258262890683122, 1.000000000000000000, 0.9659258262890683122, 1.000000000000000000, 0.9659258262890683122, 1.000000000000000000, 0.9659258262890683122, 1.000000000000000000, 0.9659258262890683122, 1.000000000000000000, 0.9659258262890683122, 1.000000000000000000, 0.9659258262890683122, 1.000000000000000000, 0.9659258262890683122, 1.000000000000000000, 0.9659258262890683122, 1.000000000000000000, 0.9659258262890683122, 1.000000000000000000, 0.9659258262890683122, 1.000000000000000000, 0.9659258262890683122, 1.000000000000000000, 0.9659258262890683122, 1.000000000000000000, 0.9659258262890683122, 1.000000000000000000, 0.9659258262890683122, 1.000000000000000000, 0.9659258262890683122, 1.000000000000000000, 0.9659258262890683122, 1.000000000000000000, 0.9659258262890683122, 1.000000000000000000, 0.9659258262890683122, 1.000000000000000000, 0.9659258262890683122, 1.000000000000000000, 0.9659258262890683122, 1.000000000000000000, 0.9659258262890683122, 1.000000000000000000, 0.9659258262890683122, 1.000000000000000000, 0.9659258262890683122, 1.000000000000000000, 0.9659258262890683122, 1.000000000000000000, 0.9659258262890683122, 1.000000000000000000, 0.9659258262890683122, 1.000000000000000000, 0.9659258262890683122, 1.000000000000000000, 0.9659258262890683122, 1.000000000000000000, 0.9659258262890683122, 1.000000000000000000, 0.9659258262890683122, 1.000000000000000000, 0.9659258262890683122, 1.000000000000000000, 0.9659258262890683122, 1.000000000000000000, 0.9659258262890683122, 1.000000000000000000, 0.9659258262890683122, 1.000000000000000000, 0.9659258262890683122, 1.000000000000000000, 0.9659258262890683122, 1.000000000000000000, 0.9659258262890683122, 1.000000000000000000, 0.9659258262890683122, 1.000000000000000000, 0.9659258262890683122, 1.000000000000000000, 0.9659258262890683122, 1.000000000000000000, 0.9659258262890683122, 1.000000000000000000, 0.9659258262890683122, 1.000000000000000000, 0.9659258262890683122, 1.000000000000000000, 0.9659258262890683122, 1.000000000000000000, 0.9659258262890683122, 1.000000000000000000, 0.9659258262890683122, 1.000000000000000000, 0.9659258262890683122, 1.000000000000000000, 0.9659258262890683122, 1.000000000000000000, 0.9659258262890683122, 1.000000000000000000, 0.9659258262890683122, 1.000000000000000000, 0.9659258262890683122, 1.000000000000000000, 0.9659258262890683122, 1.000000000000000000, 0.9659258262890683122, 1.000000000000000000, 0.9659258262890683122, 1.000000000000000000, 0.9659258262890683122, 1.000000000000000000, 0.9659258262890683122, 1.000000000000000000, 0.9659258262890683122, 1.000000000000000000, 0.9659258262890683122, 1.000000000000000000, 0.9659258262890683122, 1.000000000000000000, 0.9659258262890683122, 1.000000000000000000, 0.9659258262890683122, 1.000000000000000000, 0.9659258262890683122, 1.000000000000000000, 0.9659258262890683122, 1.000000000000000000, 0.9659258262890683122, 1.000000000000000000, 0.9659258262890683122, 1.000000000000000000, 0.9659258262890683122, 1.000000000000000000, 0.9659258262890683122, 1.000000000000000000, 0.9659258262890683122, 1.000000000000000000, 0.9659258262890683122, 1.000000000000000000, 0.9659258262890683122, 1.000000000000000000, 0.9659258262890683122, 1.000000000000000000, 0.9659258262890683122, 1.000000000000000000, 0.9659258262890683122, 1.000000000000000000, 0.9659258262890683122, 1.000000000000000000, 0.9659258262890683122, 1.000000000000000000, 0.9659258262890683122, 1.000000000000000000, 0.9659258262890683122, 1.000000000000000000, 0.9659258262890683122, 1.000000000000000000, 0.9659258262890683122, 1.000000000000000000, 0.9659258262890683122, 1.000000000000000000, 0.9659258262890683122, 1.000000000000000000, 0.9659258262890683122, 1.000000000000000000, 0.9659258262890683122, 1.000000000000000000, 0.9659258262890683122, 1.000000000000000000, 0.9659258262890683122, 1.000000000000000000, 0.9659258262890683122, 1.000000000000000000, 0.9659258262890683122, 1.000000000000000000, 0.9659258262890683122, 1.000000000000000000, 0.9659258262890683122, 1.000000000000000000, 0.9659258262890683122, 1.000000000000000000, 0.9659258262890683122, 1.000000000000000000, 0.9659258262890683122, 1.000000000000000000, 0.9659258262890683122, 1.000000000000000000, 0.9659258262890683122, 1.000000000000000000, 0.9659258262890683122, 1.000000000000000000, 0.9659258262890683122, 1.000000000000000000, 0.9659258262890683122, 1.000000000000000000, 0.9659258262890683122, 1.000000000000000000, 0.9659258262890683122, 1.000000000000000000, 0.9659258262890683122, 1.000000000000000000, 0.9659258262890683122, 1.000000000000000000, 0.9659258262890683122, 1.000000000000000000, 0.9659258262890683122, 1.000000000000000000, 0.9659258262890683122, 1.000000000000000000, 0.9659258262890683122, 1.000000000000000000, 0.9659258262890683122, 1.000000000000000000, 0.9659258262890683122, 1.000000000000000000, 0.9659258262890683122, 1.000000000000000000, 0.9659258262890683122, 1.000000000000000000, 0.9659258262890683122, 1.000000000000000000, 0.9659258262890683122, 1.000000000000000000, 0.9659258262890683122, 1.000000000000000000, 0.9659258262890683122, 1.000000000000000000) ) ) 
 REPRESENTATION_ITEM ( '' )  SURFACE ( )  );
#13098=CARTESIAN_POINT ( 'NONE',  ( -5.719274019375665041, -21.55341960407619695, 64.79275706135234714 ) ) ;
#13099=CARTESIAN_POINT ( 'NONE',  ( -16.53943276465976808, -0.05219959533934237506, 28.75109039468567929 ) ) ;
#13100=CARTESIAN_POINT ( 'NONE',  ( 5.049401038298161559, -19.05341960407611168, 72.70724293864768129 ) ) ;
#13101=CARTESIAN_POINT ( 'NONE',  ( 5.153800228976615827, -19.02544592524334988, 90.20942372801900433 ) ) ;
#13102=CARTESIAN_POINT ( 'NONE',  ( 8.224510206698742110, 14.34966873604972548, 72.08442372801899012 ) ) ;
#13103=CARTESIAN_POINT ( 'NONE',  ( 18.62759615963255655, 10.81492255796105972, 106.6677570613523756 ) ) ;
#13104=CARTESIAN_POINT ( 'NONE',  ( -19.02544592524334988, -5.153800228976617603, 73.95942372801900433 ) ) ;
#13105=CARTESIAN_POINT ( 'NONE',  ( 19.02544592524343514, -5.153800228976328945, 53.54057627198102409 ) ) ;
#13106=CARTESIAN_POINT ( 'NONE',  ( -18.62759615963270932, 10.81492255796079327, 85.83224293864768129 ) ) ;
#13107=CARTESIAN_POINT ( 'NONE',  ( -16.53943276465976808, 0.05219959533911058130, 76.24890960531435269 ) ) ;
#13108=CARTESIAN_POINT ( 'NONE',  ( 19.03943276465977164, 0.05219959533936151252, 76.25109039468566152 ) ) ;
#13110=CARTESIAN_POINT ( 'NONE',  ( 13.89961937509957401, 13.97604488694547697, 61.87609039468566863 ) ) ;
#13112=CARTESIAN_POINT ( 'NONE',  ( 8.224510206698742110, 14.34966873604972548, 107.0844237280190043 ) ) ;
#13113=CARTESIAN_POINT ( 'NONE',  ( -16.53943276465976808, 0.05219959533911058130, 66.24890960531436690 ) ) ;
#13114=CARTESIAN_POINT ( 'NONE',  ( 18.62759615963255655, 10.81492255796105972, 106.6677570613523756 ) ) ;
#13116=CARTESIAN_POINT ( 'NONE',  ( -10.72451020669898014, 18.67979575497178502, 105.4155762719810383 ) ) ;
#13117=CARTESIAN_POINT ( 'NONE',  ( -5.153800228976328057, -19.02544592524343514, 62.29057627198100988 ) ) ;
#13118=CARTESIAN_POINT ( 'NONE',  ( -15.80617190586768217, 15.72974639402176855, 78.12609039468570415 ) ) ;
#13119=CARTESIAN_POINT ( 'NONE',  ( 9.564922557960805705, 16.46253265017160317, 59.58224293864769550 ) ) ;
#13121=CARTESIAN_POINT ( 'NONE',  ( 13.97604488694527802, 13.89961937509977652, 29.37390960531435979 ) ) ;
#13122=CARTESIAN_POINT ( 'NONE',  ( 21.53943276465977519, -0.05219959533907433946, 23.74890960531435269 ) ) ;
#13123=CARTESIAN_POINT ( 'NONE',  ( 14.29746914071049879, -8.314922557960816363, 68.33224293864769550 ) ) ;
#13124=CARTESIAN_POINT ( 'NONE',  ( -13.89961937509977652, 13.97604488694528158, 40.62390960531435979 ) ) ;
#13125=CARTESIAN_POINT ( 'NONE',  ( 12.14591786802309770, 12.06949235617756955, 99.37390960531436690 ) ) ;
#13126=CARTESIAN_POINT ( 'NONE',  ( 21.55341960407610458, 5.719274019375980345, 108.9572429386476955 ) ) ;
#13128=CARTESIAN_POINT ( 'NONE',  ( -21.52544592524334988, -5.823673210054445271, 48.95942372801902565 ) ) ;
#13129=CARTESIAN_POINT ( 'NONE',  ( 19.03943276465977164, -0.05219959533909143690, 28.74890960531435624 ) ) ;
#13130=CARTESIAN_POINT ( 'NONE',  ( 4.483927247898790824, -16.52544592524335698, 60.20942372801902565 ) ) ;
#13131=CARTESIAN_POINT ( 'NONE',  ( -21.55341960407610458, -5.719274019375992779, 96.45724293864770971 ) ) ;
#13132=CARTESIAN_POINT ( 'NONE',  ( -15.80617190586745835, -15.72974639402198527, 91.87390960531436690 ) ) ;
#13133=CARTESIAN_POINT ( 'NONE',  ( 19.03943276465977164, 0.05219959533936151252, 31.25109039468566863 ) ) ;
#13134=CARTESIAN_POINT ( 'NONE',  ( -16.46253265017160317, 9.564922557960807481, 50.83224293864770260 ) ) ;
#13136=CARTESIAN_POINT ( 'NONE',  ( -15.80617190586768217, 15.72974639402176855, 63.12609039468568994 ) ) ;
#13137=CARTESIAN_POINT ( 'NONE',  ( 15.72974639402199770, -15.80617190586745480, 63.12390960531435979 ) ) ;
#13138=CARTESIAN_POINT ( 'NONE',  ( 16.52544592524342804, -4.483927247898539470, 23.54057627198102765 ) ) ;
#13139=CARTESIAN_POINT ( 'NONE',  ( -5.823673210054431948, 21.52544592524334988, 82.70942372801900433 ) ) ;
#13140=CARTESIAN_POINT ( 'NONE',  ( -21.55341960407619339, 5.719274019375674811, 98.54275706135234714 ) ) ;
#13141=CARTESIAN_POINT ( 'NONE',  ( 13.97604488694548053, -13.89961937509957401, 40.62609039468564731 ) ) ;
#13142=CARTESIAN_POINT ( 'NONE',  ( -0.05219959533934338120, 16.53943276465976808, 97.50109039468567573 ) ) ;
#13143=CARTESIAN_POINT ( 'NONE',  ( 10.81492255796106328, -18.62759615963255655, 50.41775706135235424 ) ) ;
#13144=CARTESIAN_POINT ( 'NONE',  ( 13.89961937509977652, -13.97604488694527269, 53.12390960531434558 ) ) ;
#13145=CARTESIAN_POINT ( 'NONE',  ( -16.46253265017146816, -9.564922557961047289, 39.16775706135234003 ) ) ;
#13146=CARTESIAN_POINT ( 'NONE',  ( 15.80617190586746368, 15.72974639402197994, 34.37390960531435979 ) ) ;
#13147=CARTESIAN_POINT ( 'NONE',  ( -0.05219959533937732626, 21.53943276465977519, 32.50109039468568284 ) ) ;
#13148=CARTESIAN_POINT ( 'NONE',  ( -21.53943276465977519, 0.05219959533907696930, 91.24890960531436690 ) ) ;
#13149=CARTESIAN_POINT ( 'NONE',  ( 16.51473224551083163, -9.474510206698727899, 85.83442372801900433 ) ) ;
#13150=CARTESIAN_POINT ( 'NONE',  ( 14.34966873604972726, -8.224510206698740333, 55.83442372801901854 ) ) ;
#13151=CARTESIAN_POINT ( 'NONE',  ( 17.50000000000001776, -3.242565516147306592, 37.50000000000000000 ) ) ;
#13152=CARTESIAN_POINT ( 'NONE',  ( -18.62759615963270932, 10.81492255796079327, 85.83224293864768129 ) ) ;
#13153=CARTESIAN_POINT ( 'NONE',  ( -8.314922557961024197, 14.29746914071037800, 77.91775706135231871 ) ) ;
#13154=CARTESIAN_POINT ( 'NONE',  ( 14.34966873604960469, 8.224510206698951720, 74.16557627198102409 ) ) ;
#13156=CARTESIAN_POINT ( 'NONE',  ( -16.51473224551082808, 9.474510206698731452, 98.33442372801900433 ) ) ;
#13157=CARTESIAN_POINT ( 'NONE',  ( 15.80617190586746368, 15.72974639402197994, 29.37390960531435269 ) ) ;
#13159=CARTESIAN_POINT ( 'NONE',  ( -0.05219959533934338120, 16.53943276465976808, 37.50109039468568284 ) ) ;
#13160=CARTESIAN_POINT ( 'NONE',  ( -21.52544592524343514, 5.823673210054127303, 111.0405762719810525 ) ) ;
#13161=CARTESIAN_POINT ( 'NONE',  ( 15.80617190586746368, 15.72974639402197994, 29.37390960531435269 ) ) ;
#13162=CARTESIAN_POINT ( 'NONE',  ( 16.53943276465976808, 0.05219959533934440121, 66.25109039468567573 ) ) ;
#13163=CARTESIAN_POINT ( 'NONE',  ( 19.05341960407611168, 5.049401038298154454, 83.95724293864766707 ) ) ;
#13164=CARTESIAN_POINT ( 'NONE',  ( 21.52544592524334988, 5.823673210054432836, 51.45942372801901854 ) ) ;
#13165=CARTESIAN_POINT ( 'NONE',  ( 0.05219959533909260263, 19.03943276465977164, 29.99890960531435979 ) ) ;
#13166=CARTESIAN_POINT ( 'NONE',  ( -10.81492255796078084, -18.62759615963271287, 22.08224293864769194 ) ) ;
#13168=CARTESIAN_POINT ( 'NONE',  ( 13.89961937509957401, 13.97604488694547697, 41.87609039468566152 ) ) ;
#13169=CARTESIAN_POINT ( 'NONE',  ( 12.14591786802327356, -12.06949235617739191, 55.62609039468568284 ) ) ;
#13170=CARTESIAN_POINT ( 'NONE',  ( 10.81492255796078972, 18.62759615963270932, 24.58224293864768839 ) ) ;
#13171=CARTESIAN_POINT ( 'NONE',  ( -13.97604488694527625, -13.89961937509977652, 76.87390960531433848 ) ) ;
#13172=CARTESIAN_POINT ( 'NONE',  ( -16.55341960407617563, 4.379528057220093196, 98.54275706135234714 ) ) ;
#13173=CARTESIAN_POINT ( 'NONE',  ( 4.483927247898545687, 16.52544592524342804, 94.79057627198105251 ) ) ;
#13174=CARTESIAN_POINT ( 'NONE',  ( -18.67979575497178146, -10.72451020669898902, 36.66557627198103120 ) ) ;
#13175=CARTESIAN_POINT ( 'NONE',  ( -16.46253265017160317, 9.564922557960807481, 30.83224293864769550 ) ) ;
#13176=CARTESIAN_POINT ( 'NONE',  ( -16.52544592524335698, -4.483927247898792601, 63.95942372801901854 ) ) ;
#13177=CARTESIAN_POINT ( 'NONE',  ( 10.81492255796106328, -18.62759615963255655, 25.41775706135235779 ) ) ;
#13178=CARTESIAN_POINT ( 'NONE',  ( 13.89961937509957401, 13.97604488694547697, 76.87609039468566152 ) ) ;
#13179=CARTESIAN_POINT ( 'NONE',  ( 0.05219959533909260263, 19.03943276465977164, 39.99890960531436690 ) ) ;
#13180=CARTESIAN_POINT ( 'NONE',  ( 15.72974639402199770, -15.80617190586745480, 68.12390960531436690 ) ) ;
#13181=CARTESIAN_POINT ( 'NONE',  ( -5.049401038298153566, 19.05341960407611168, 110.2072429386476671 ) ) ;
#13182=CARTESIAN_POINT ( 'NONE',  ( -0.05219959533937732626, 21.53943276465977519, 97.50109039468567573 ) ) ;
#13183=CARTESIAN_POINT ( 'NONE',  ( -19.03943276465977164, 0.05219959533909376836, 66.24890960531436690 ) ) ;
#13184=CARTESIAN_POINT ( 'NONE',  ( 8.224510206698742110, 14.34966873604972548, 47.08442372801901854 ) ) ;
#13185=CARTESIAN_POINT ( 'NONE',  ( -13.89961937509977652, 13.97604488694528158, 65.62390960531436690 ) ) ;
#13186=CARTESIAN_POINT ( 'NONE',  ( -18.62759615963255300, -10.81492255796106328, 84.16775706135234714 ) ) ;
#13187=CARTESIAN_POINT ( 'NONE',  ( -9.474510206698720793, -16.51473224551083518, 44.58442372801900433 ) ) ;
#13188=CARTESIAN_POINT ( 'NONE',  ( -9.564922557961040184, 16.46253265017147172, 52.91775706135233293 ) ) ;
#13190=CARTESIAN_POINT ( 'NONE',  ( -0.05219959533937732626, 21.53943276465977519, 47.50109039468568994 ) ) ;
#13193=CARTESIAN_POINT ( 'NONE',  ( -13.89961937509957401, -13.97604488694547875, 44.37609039468566863 ) ) ;
#13194=CARTESIAN_POINT ( 'NONE',  ( -9.474510206698964154, 16.51473224551069663, 105.4155762719810383 ) ) ;
#13195=CARTESIAN_POINT ( 'NONE',  ( -19.03943276465977164, 0.05219959533909376836, 76.24890960531435269 ) ) ;
#13196=CARTESIAN_POINT ( 'NONE',  ( -8.314922557960811034, -14.29746914071050412, 37.08224293864768129 ) ) ;
#13197=CARTESIAN_POINT ( 'NONE',  ( 21.53943276465977519, -0.05219959533907433946, 38.74890960531435979 ) ) ;
#13200=CARTESIAN_POINT ( 'NONE',  ( 18.62759615963255655, 10.81492255796105972, 101.6677570613523613 ) ) ;
#13202=CARTESIAN_POINT ( 'NONE',  ( 16.46253265017160672, -9.564922557960803928, 33.33224293864770260 ) ) ;
#13203=CARTESIAN_POINT ( 'NONE',  ( 13.89961937509977652, -13.97604488694527269, 113.1239096053143527 ) ) ;
#13205=CARTESIAN_POINT ( 'NONE',  ( 8.314922557961029526, -14.29746914071037800, 50.41775706135235424 ) ) ;
#13206=CARTESIAN_POINT ( 'NONE',  ( -5.823673210054116645, -21.52544592524344225, 72.29057627198102409 ) ) ;
#13207=CARTESIAN_POINT ( 'NONE',  ( -8.224510206698948167, 14.34966873604960824, 35.41557627198102409 ) ) ;
#13208=CARTESIAN_POINT ( 'NONE',  ( 0.05219959533909260263, 19.03943276465977164, 29.99890960531435979 ) ) ;
#13209=CARTESIAN_POINT ( 'NONE',  ( 16.51473224551069308, 9.474510206698969483, 114.1655762719810241 ) ) ;
#13210=CARTESIAN_POINT ( 'NONE',  ( -15.80617190586768217, 15.72974639402176855, 28.12609039468568284 ) ) ;
#13211=CARTESIAN_POINT ( 'NONE',  ( 16.51473224551083163, -9.474510206698727899, 40.83442372801900433 ) ) ;
#13212=CARTESIAN_POINT ( 'NONE',  ( 16.55341960407611168, 4.379528057220329451, 113.9572429386477239 ) ) ;
#13213=CARTESIAN_POINT ( 'NONE',  ( 15.80617190586769283, -15.72974639402175789, 75.62609039468567573 ) ) ;
#13214=CARTESIAN_POINT ( 'NONE',  ( 16.81555441253552985, -7.025013491695479395, 33.13685445334258617 ) ) ;
#13215=CARTESIAN_POINT ( 'NONE',  ( 12.06949235617757843, -12.14591786802309237, 28.12390960531435979 ) ) ;
#13217=CARTESIAN_POINT ( 'NONE',  ( 5.823673210054125526, 21.52544592524343514, 29.79057627198102409 ) ) ;
#13218=CARTESIAN_POINT ( 'NONE',  ( -14.29746914071049879, 8.314922557960819915, 95.83224293864770971 ) ) ;
#13220=CARTESIAN_POINT ( 'NONE',  ( -13.97604488694527625, -13.89961937509977652, 76.87390960531433848 ) ) ;
#13221=CARTESIAN_POINT ( 'NONE',  ( -4.379528057220328563, 16.55341960407611168, 80.20724293864769550 ) ) ;
#13222=CARTESIAN_POINT ( 'NONE',  ( -5.153800228976607833, 19.02544592524334988, 102.7094237280189759 ) ) ;
#13223=CARTESIAN_POINT ( 'NONE',  ( -10.72451020669898014, 18.67979575497178502, 65.41557627198102409 ) ) ;
#13224=ORIENTED_EDGE ( 'NONE', *, *, #63994, .F. ) ;
#13225=CARTESIAN_POINT ( 'NONE',  ( 9.564922557960805705, 16.46253265017160317, 29.58224293864769550 ) ) ;
#13226=CARTESIAN_POINT ( 'NONE',  ( -16.46253265017160317, 9.564922557960807481, 70.83224293864770971 ) ) ;
#13227=CARTESIAN_POINT ( 'NONE',  ( -18.62759615963270932, 10.81492255796079327, 80.83224293864769550 ) ) ;
#13228=CARTESIAN_POINT ( 'NONE',  ( -8.224510206698735004, -14.34966873604973081, 109.5844237280190328 ) ) ;
#13229=CARTESIAN_POINT ( 'NONE',  ( -19.05341960407611168, -5.049401038298163336, 86.45724293864769550 ) ) ;
#13230=CARTESIAN_POINT ( 'NONE',  ( 13.97604488694548053, -13.89961937509957401, 65.62609039468567573 ) ) ;
#13231=CARTESIAN_POINT ( 'NONE',  ( -10.72451020669870658, -18.67979575497194134, 99.58442372801900433 ) ) ;
#13232=CARTESIAN_POINT ( 'NONE',  ( -5.823673210054116645, -21.52544592524344225, 77.29057627198102409 ) ) ;
#13233=CARTESIAN_POINT ( 'NONE',  ( -5.719274019375978568, 21.55341960407610458, 30.20724293864769550 ) ) ;
#13234=CARTESIAN_POINT ( 'NONE',  ( -0.05219959533909027116, -19.03943276465977164, 52.49890960531436690 ) ) ;
#13235=CARTESIAN_POINT ( 'NONE',  ( 4.483927247898790824, -16.52544592524335698, 95.20942372801903275 ) ) ;
#13236=CARTESIAN_POINT ( 'NONE',  ( 5.153800228976335163, 19.02544592524342804, 64.79057627198100988 ) ) ;
#13238=CARTESIAN_POINT ( 'NONE',  ( -21.53943276465977519, -0.05219959533937600094, 103.7510903946857042 ) ) ;
#13239=CARTESIAN_POINT ( 'NONE',  ( 14.29746914071049879, -8.314922557960816363, 68.33224293864769550 ) ) ;
#13240=CARTESIAN_POINT ( 'NONE',  ( -5.823673210054116645, -21.52544592524344225, 112.2905762719810241 ) ) ;
#13241=CARTESIAN_POINT ( 'NONE',  ( 10.72451020669898902, -18.67979575497178502, 107.9155762719810241 ) ) ;
#13243=CARTESIAN_POINT ( 'NONE',  ( 5.823673210054125526, 21.52544592524343514, 54.79057627198104541 ) ) ;
#13244=CARTESIAN_POINT ( 'NONE',  ( 16.53943276465976808, 0.05219959533934440121, 86.25109039468568994 ) ) ;
#13245=CARTESIAN_POINT ( 'NONE',  ( 8.314922557960818139, 14.29746914071049879, 104.5822429386477097 ) ) ;
#13246=CARTESIAN_POINT ( 'NONE',  ( 13.89961937509977652, -13.97604488694527269, 63.12390960531435979 ) ) ;
#13248=CARTESIAN_POINT ( 'NONE',  ( -12.14591786802309592, -12.06949235617757132, 21.87390960531436690 ) ) ;
#13249=CARTESIAN_POINT ( 'NONE',  ( 21.53943276465977519, 0.05219959533937863772, 51.25109039468568994 ) ) ;
#13250=CARTESIAN_POINT ( 'NONE',  ( 13.97604488694527802, 13.89961937509977652, 99.37390960531436690 ) ) ;
#13251=CARTESIAN_POINT ( 'NONE',  ( 21.52544592524334988, 5.823673210054432836, 81.45942372801900433 ) ) ;
#13252=CARTESIAN_POINT ( 'NONE',  ( -19.05341960407611168, -5.049401038298163336, 26.45724293864769550 ) ) ;
#13253=CARTESIAN_POINT ( 'NONE',  ( 5.153800228976335163, 19.02544592524342804, 34.79057627198102409 ) ) ;
#13255=CARTESIAN_POINT ( 'NONE',  ( 10.72451020669871369, 18.67979575497193778, 77.08442372801901854 ) ) ;
#13256=CARTESIAN_POINT ( 'NONE',  ( 19.03943276465977164, -0.05219959533909143690, 108.7489096053143527 ) ) ;
#13257=CARTESIAN_POINT ( 'NONE',  ( 5.153800228976615827, -19.02544592524334988, 75.20942372801896170 ) ) ;
#13258=CARTESIAN_POINT ( 'NONE',  ( 15.80617190586769283, -15.72974639402175789, 45.62609039468567573 ) ) ;
#13259=CARTESIAN_POINT ( 'NONE',  ( -14.29746914071037622, -8.314922557961029526, 19.16775706135234714 ) ) ;
#13260=CARTESIAN_POINT ( 'NONE',  ( 0.05219959533936267826, -19.03943276465977164, 70.00109039468566152 ) ) ;
#13261=CARTESIAN_POINT ( 'NONE',  ( 13.89961937509977652, -13.97604488694527269, 53.12390960531434558 ) ) ;
#13262=CARTESIAN_POINT ( 'NONE',  ( 9.564922557961047289, -16.46253265017146816, 80.41775706135234714 ) ) ;
#13263=CARTESIAN_POINT ( 'NONE',  ( -14.34966873604960291, -8.224510206698953496, 26.66557627198103475 ) ) ;
#13264=CARTESIAN_POINT ( 'NONE',  ( 13.89961937509957401, 13.97604488694547697, 91.87609039468567573 ) ) ;
#13265=CARTESIAN_POINT ( 'NONE',  ( 14.29746914071049879, -8.314922557960816363, 43.33224293864769550 ) ) ;
#13266=CARTESIAN_POINT ( 'NONE',  ( 5.153800228976615827, -19.02544592524334988, 65.20942372801900433 ) ) ;
#13267=CARTESIAN_POINT ( 'NONE',  ( -14.34966873604972548, 8.224510206698743886, 53.33442372801901854 ) ) ;
#13268=CARTESIAN_POINT ( 'NONE',  ( 19.03943276465977164, 0.05219959533936151252, 26.25109039468566507 ) ) ;
#13269=CARTESIAN_POINT ( 'NONE',  ( 19.03943276465977164, -0.05219959533909143690, 48.74890960531435979 ) ) ;
#13271=CARTESIAN_POINT ( 'NONE',  ( 16.52544592524335698, 4.483927247898782831, 46.45942372801901854 ) ) ;
#13274=CARTESIAN_POINT ( 'NONE',  ( -9.474510206698964154, 16.51473224551069663, 95.41557627198102409 ) ) ;
#13275=CARTESIAN_POINT ( 'NONE',  ( -9.474510206698720793, -16.51473224551083518, 84.58442372801900433 ) ) ;
#13276=CARTESIAN_POINT ( 'NONE',  ( -0.05219959533936034679, 19.03943276465977164, 82.50109039468567573 ) ) ;
#13277=CARTESIAN_POINT ( 'NONE',  ( 10.72451020669898902, -18.67979575497178502, 27.91557627198103830 ) ) ;
#13278=CARTESIAN_POINT ( 'NONE',  ( -0.05219959533936034679, 19.03943276465977164, 22.50109039468566152 ) ) ;
#13279=CARTESIAN_POINT ( 'NONE',  ( -0.05219959533936034679, 19.03943276465977164, 97.50109039468567573 ) ) ;
#13280=CARTESIAN_POINT ( 'NONE',  ( -8.224510206698948167, 14.34966873604960824, 115.4155762719810241 ) ) ;
#13281=CARTESIAN_POINT ( 'NONE',  ( 19.02544592524343514, -5.153800228976328945, 38.54057627198103120 ) ) ;
#13282=CARTESIAN_POINT ( 'NONE',  ( -15.80617190586745835, -15.72974639402198527, 61.87390960531436690 ) ) ;
#13283=CARTESIAN_POINT ( 'NONE',  ( -16.52544592524342804, 4.483927247898546575, 116.0405762719810383 ) ) ;
#13285=CARTESIAN_POINT ( 'NONE',  ( 5.153800228976615827, -19.02544592524334988, 70.20942372801899012 ) ) ;
#13286=CARTESIAN_POINT ( 'NONE',  ( -8.224510206698948167, 14.34966873604960824, 35.41557627198102409 ) ) ;
#13287=CARTESIAN_POINT ( 'NONE',  ( -5.823673210054116645, -21.52544592524344225, 37.29057627198102409 ) ) ;
#13288=CARTESIAN_POINT ( 'NONE',  ( 18.62759615963255655, 10.81492255796105972, 91.66775706135234714 ) ) ;
#13289=CARTESIAN_POINT ( 'NONE',  ( -21.53943276465977519, 0.05219959533907696930, 86.24890960531436690 ) ) ;
#13290=CARTESIAN_POINT ( 'NONE',  ( -10.81492255796105439, 18.62759615963255655, 52.91775706135235424 ) ) ;
#13291=CARTESIAN_POINT ( 'NONE',  ( 5.823673210054444382, -21.52544592524334988, 65.20942372801901854 ) ) ;
#13292=CARTESIAN_POINT ( 'NONE',  ( 19.05341960407611168, 5.049401038298154454, 93.95724293864769550 ) ) ;
#13293=CARTESIAN_POINT ( 'NONE',  ( 0.05219959533934541429, -16.53943276465976808, 90.00109039468567573 ) ) ;
#13294=CARTESIAN_POINT ( 'NONE',  ( 18.62759615963255655, 10.81492255796105972, 46.66775706135234714 ) ) ;
#13295=CARTESIAN_POINT ( 'NONE',  ( 8.314922557960818139, 14.29746914071049879, 114.5822429386477097 ) ) ;
#13296=CARTESIAN_POINT ( 'NONE',  ( -12.14591786802309592, -12.06949235617757132, 71.87390960531438111 ) ) ;
#13297=CARTESIAN_POINT ( 'NONE',  ( -14.29746914071049879, 8.314922557960819915, 30.83224293864770260 ) ) ;
#13298=CARTESIAN_POINT ( 'NONE',  ( -18.62759615963270932, 10.81492255796079327, 45.83224293864769550 ) ) ;
#13299=CARTESIAN_POINT ( 'NONE',  ( -19.05341960407611168, -5.049401038298163336, 51.45724293864770260 ) ) ;
#13300=CARTESIAN_POINT ( 'NONE',  ( 5.823673210054125526, 21.52544592524343514, 64.79057627198103830 ) ) ;
#13301=CARTESIAN_POINT ( 'NONE',  ( -13.89961937509957401, -13.97604488694547875, 49.37609039468567573 ) ) ;
#13302=CARTESIAN_POINT ( 'NONE',  ( -16.38665767535053774, -7.295008042176053031, 39.73599135785456582 ) ) ;
#13303=CARTESIAN_POINT ( 'NONE',  ( 0.05219959533910956823, 16.53943276465976808, 54.99890960531435269 ) ) ;
#13304=CARTESIAN_POINT ( 'NONE',  ( 5.719274019375991003, -21.55341960407610458, 22.70724293864769194 ) ) ;
#13307=CARTESIAN_POINT ( 'NONE',  ( -4.379528057220086978, -16.55341960407618274, 69.79275706135234714 ) ) ;
#13308=CARTESIAN_POINT ( 'NONE',  ( -13.97604488694547697, 13.89961937509957934, 78.12609039468567573 ) ) ;
#13309=CARTESIAN_POINT ( 'NONE',  ( -12.14591786802309592, -12.06949235617757132, 36.87390960531435979 ) ) ;
#13310=LINE ( 'NONE', #106295, #99949 ) ;
#13311=CARTESIAN_POINT ( 'NONE',  ( 4.483927247898545687, 16.52544592524342804, 24.79057627198103120 ) ) ;
#13312=CARTESIAN_POINT ( 'NONE',  ( -0.05219959533909027116, -19.03943276465977164, 57.49890960531435979 ) ) ;
#13313=CARTESIAN_POINT ( 'NONE',  ( 16.51473224551069308, 9.474510206698969483, 74.16557627198103830 ) ) ;
#13314=CARTESIAN_POINT ( 'NONE',  ( 16.46253265017160672, -9.564922557960803928, 43.33224293864769550 ) ) ;
#13315=CARTESIAN_POINT ( 'NONE',  ( -10.72451020669870658, -18.67979575497194134, 49.58442372801901143 ) ) ;
#13316=CARTESIAN_POINT ( 'NONE',  ( 16.51473224551069308, 9.474510206698969483, 64.16557627198102409 ) ) ;
#13318=CARTESIAN_POINT ( 'NONE',  ( -19.02544592524342804, 5.153800228976336051, 61.04057627198103120 ) ) ;
#13319=CARTESIAN_POINT ( 'NONE',  ( -21.52544592524343514, 5.823673210054127303, 41.04057627198103120 ) ) ;
#13321=CARTESIAN_POINT ( 'NONE',  ( -5.049401038298153566, 19.05341960407611168, 40.20724293864768839 ) ) ;
#13322=CARTESIAN_POINT ( 'NONE',  ( -21.53943276465977519, 0.05219959533907696930, 36.24890960531435979 ) ) ;
#13323=CARTESIAN_POINT ( 'NONE',  ( 12.06949235617739724, 12.14591786802326823, 91.87609039468568994 ) ) ;
#13324=CARTESIAN_POINT ( 'NONE',  ( -19.03943276465977164, -0.05219959533935918106, 28.75109039468566507 ) ) ;
#13325=CARTESIAN_POINT ( 'NONE',  ( 14.29746914071037800, 8.314922557961029526, 71.66775706135234714 ) ) ;
#13326=CARTESIAN_POINT ( 'NONE',  ( -0.05219959533909027116, -19.03943276465977164, 102.4989096053143669 ) ) ;
#13327=CARTESIAN_POINT ( 'NONE',  ( -14.34966873604972548, 8.224510206698743886, 53.33442372801901854 ) ) ;
#13328=CARTESIAN_POINT ( 'NONE',  ( 4.379528057220092307, 16.55341960407617563, 37.29275706135235424 ) ) ;
#13329=CARTESIAN_POINT ( 'NONE',  ( 13.89961937509977652, -13.97604488694527269, 103.1239096053143527 ) ) ;
#13330=CARTESIAN_POINT ( 'NONE',  ( 16.53943276465976808, 0.05219959533934440121, 31.25109039468568639 ) ) ;
#13331=CARTESIAN_POINT ( 'NONE',  ( -19.05341960407611168, -5.049401038298163336, 31.45724293864769550 ) ) ;
#13332=CARTESIAN_POINT ( 'NONE',  ( -0.05219959533937732626, 21.53943276465977519, 27.50109039468567929 ) ) ;
#13333=CARTESIAN_POINT ( 'NONE',  ( -12.14591786802326823, 12.06949235617739902, 23.12609039468567573 ) ) ;
#13334=CARTESIAN_POINT ( 'NONE',  ( -0.05219959533934338120, 16.53943276465976808, 92.50109039468567573 ) ) ;
#13336=CARTESIAN_POINT ( 'NONE',  ( -21.53943276465977519, -0.05219959533937600094, 98.75109039468568994 ) ) ;
#13337=CARTESIAN_POINT ( 'NONE',  ( -16.51473224551082808, 9.474510206698731452, 98.33442372801900433 ) ) ;
#13339=CARTESIAN_POINT ( 'NONE',  ( -12.14591786802309592, -12.06949235617757132, 51.87390960531437401 ) ) ;
#13340=CARTESIAN_POINT ( 'NONE',  ( 19.05341960407611168, 5.049401038298154454, 23.95724293864769194 ) ) ;
#13341=CARTESIAN_POINT ( 'NONE',  ( 16.51473224551083163, -9.474510206698727899, 45.83442372801900433 ) ) ;
#13343=CARTESIAN_POINT ( 'NONE',  ( -5.823673210054431948, 21.52544592524334988, 52.70942372801902565 ) ) ;
#13344=CARTESIAN_POINT ( 'NONE',  ( 4.379528057220092307, 16.55341960407617563, 22.29275706135235069 ) ) ;
#13345=CARTESIAN_POINT ( 'NONE',  ( 17.26172910966779028, 6.454744622555872446, 81.69353091350777163 ) ) ;
#13346=CARTESIAN_POINT ( 'NONE',  ( -19.05341960407611168, -5.049401038298163336, 106.4572429386476955 ) ) ;
#13347=CARTESIAN_POINT ( 'NONE',  ( 18.62759615963271287, -10.81492255796078972, 73.33224293864769550 ) ) ;
#13348=CARTESIAN_POINT ( 'NONE',  ( 19.05341960407617918, -5.049401038297876454, 96.04275706135231871 ) ) ;
#13349=CARTESIAN_POINT ( 'NONE',  ( -5.153800228976328057, -19.02544592524343514, 97.29057627198099567 ) ) ;
#13351=CARTESIAN_POINT ( 'NONE',  ( 8.314922557960818139, 14.29746914071049879, 104.5822429386477097 ) ) ;
#13352=CARTESIAN_POINT ( 'NONE',  ( -21.52544592524334988, -5.823673210054445271, 98.95942372801903275 ) ) ;
#13353=CARTESIAN_POINT ( 'NONE',  ( 5.049401038298161559, -19.05341960407611168, 47.70724293864770260 ) ) ;
#13354=CARTESIAN_POINT ( 'NONE',  ( 15.80617190586769283, -15.72974639402175789, 55.62609039468568284 ) ) ;
#13355=CARTESIAN_POINT ( 'NONE',  ( 18.62759615963255655, 10.81492255796105972, 86.66775706135234714 ) ) ;
#13356=CARTESIAN_POINT ( 'NONE',  ( -4.379528057220086978, -16.55341960407618274, 104.7927570613523898 ) ) ;
#13357=CARTESIAN_POINT ( 'NONE',  ( 9.564922557960805705, 16.46253265017160317, 69.58224293864770971 ) ) ;
#13358=CARTESIAN_POINT ( 'NONE',  ( 18.62759615963255655, 10.81492255796105972, 46.66775706135234714 ) ) ;
#13359=CARTESIAN_POINT ( 'NONE',  ( -15.80617190586768217, 15.72974639402176855, 43.12609039468568284 ) ) ;
#13360=CARTESIAN_POINT ( 'NONE',  ( -0.05219959533936034679, 19.03943276465977164, 72.50109039468566152 ) ) ;
#13361=CARTESIAN_POINT ( 'NONE',  ( -0.05219959533909027116, -19.03943276465977164, 92.49890960531436690 ) ) ;
#13362=CARTESIAN_POINT ( 'NONE',  ( 14.34966873604960469, 8.224510206698951720, 99.16557627198100988 ) ) ;
#13363=CARTESIAN_POINT ( 'NONE',  ( 0.05219959533907565091, 21.53943276465977519, 99.99890960531436690 ) ) ;
#13364=CARTESIAN_POINT ( 'NONE',  ( 14.34966873604960469, 8.224510206698951720, 59.16557627198103120 ) ) ;
#13365=CARTESIAN_POINT ( 'NONE',  ( -10.81492255796105439, 18.62759615963255655, 112.9177570613523329 ) ) ;
#13366=CARTESIAN_POINT ( 'NONE',  ( 0.05219959533910956823, 16.53943276465976808, 84.99890960531436690 ) ) ;
#13367=CARTESIAN_POINT ( 'NONE',  ( -9.564922557960796823, -16.46253265017161027, 32.08224293864769550 ) ) ;
#13368=CARTESIAN_POINT ( 'NONE',  ( -5.153800228976607833, 19.02544592524334988, 82.70942372801897591 ) ) ;
#13369=CARTESIAN_POINT ( 'NONE',  ( -16.52544592524342804, 4.483927247898546575, 51.04057627198103120 ) ) ;
#13370=CARTESIAN_POINT ( 'NONE',  ( 21.53943276465977519, 0.05219959533937863772, 96.25109039468568994 ) ) ;
#13371=CARTESIAN_POINT ( 'NONE',  ( 16.51473224551069308, 9.474510206698969483, 94.16557627198103830 ) ) ;
#13372=CARTESIAN_POINT ( 'NONE',  ( 19.05341960407617918, -5.049401038297876454, 71.04275706135234714 ) ) ;
#13373=CARTESIAN_POINT ( 'NONE',  ( 15.80617190586746368, 15.72974639402197994, 79.37390960531436690 ) ) ;
#13374=CARTESIAN_POINT ( 'NONE',  ( -21.52544592524334988, -5.823673210054445271, 33.95942372801901143 ) ) ;
#13375=CARTESIAN_POINT ( 'NONE',  ( -4.379528057220086978, -16.55341960407618274, 24.79275706135235779 ) ) ;
#13376=CARTESIAN_POINT ( 'NONE',  ( -4.483927247898782831, 16.52544592524335698, 97.70942372801904696 ) ) ;
#13377=CARTESIAN_POINT ( 'NONE',  ( -5.049401038298153566, 19.05341960407611168, 25.20724293864768484 ) ) ;
#13378=CARTESIAN_POINT ( 'NONE',  ( -5.823673210054431948, 21.52544592524334988, 32.70942372801900433 ) ) ;
#13379=CARTESIAN_POINT ( 'NONE',  ( -5.153800228976328057, -19.02544592524343514, 22.29057627198102765 ) ) ;
#13381=CARTESIAN_POINT ( 'NONE',  ( 16.53943276465976808, 0.05219959533934440121, 46.25109039468567573 ) ) ;
#13382=CARTESIAN_POINT ( 'NONE',  ( 0.05219959533910956823, 16.53943276465976808, 74.99890960531435269 ) ) ;
#13383=CARTESIAN_POINT ( 'NONE',  ( 15.80617190586746368, 15.72974639402197994, 69.37390960531436690 ) ) ;
#13384=CARTESIAN_POINT ( 'NONE',  ( 16.55341960407611168, 4.379528057220329451, 23.95724293864769550 ) ) ;
#13385=CARTESIAN_POINT ( 'NONE',  ( -8.314922557961024197, 14.29746914071037800, 47.91775706135234714 ) ) ;
#13386=CARTESIAN_POINT ( 'NONE',  ( -19.02544592524342804, 5.153800228976336051, 51.04057627198103120 ) ) ;
#13387=CARTESIAN_POINT ( 'NONE',  ( -14.34966873604972548, 8.224510206698743886, 88.33442372801901854 ) ) ;
#13388=CARTESIAN_POINT ( 'NONE',  ( 19.05341960407617918, -5.049401038297876454, 81.04275706135231871 ) ) ;
#13389=CARTESIAN_POINT ( 'NONE',  ( 21.53943276465977519, -0.05219959533907433946, 68.74890960531435269 ) ) ;
#13390=CARTESIAN_POINT ( 'NONE',  ( 16.53943276465976808, -0.05219959533910856209, 23.74890960531435269 ) ) ;
#13391=VERTEX_POINT ( 'NONE', #163977 ) ;
#13392=CARTESIAN_POINT ( 'NONE',  ( -0.05219959533909027116, -19.03943276465977164, 112.4989096053143669 ) ) ;
#13393=CARTESIAN_POINT ( 'NONE',  ( 10.72451020669898902, -18.67979575497178502, 62.91557627198102409 ) ) ;
#13395=CARTESIAN_POINT ( 'NONE',  ( -16.52544592524335698, -4.483927247898792601, 88.95942372801901854 ) ) ;
#13396=ORIENTED_EDGE ( 'NONE', *, *, #43196, .T. ) ;
#13397=CARTESIAN_POINT ( 'NONE',  ( 9.474510206698971260, -16.51473224551069308, 107.9155762719810383 ) ) ;
#13399=CARTESIAN_POINT ( 'NONE',  ( -5.719274019375978568, 21.55341960407610458, 70.20724293864769550 ) ) ;
#13400=CARTESIAN_POINT ( 'NONE',  ( -12.14591786802326823, 12.06949235617739902, 108.1260903946856757 ) ) ;
#13401=CARTESIAN_POINT ( 'NONE',  ( 4.483927247898790824, -16.52544592524335698, 20.20942372801900788 ) ) ;
#13402=CARTESIAN_POINT ( 'NONE',  ( 5.049401038298161559, -19.05341960407611168, 22.70724293864769194 ) ) ;
#13403=CARTESIAN_POINT ( 'NONE',  ( 4.379528057220092307, 16.55341960407617563, 27.29275706135234358 ) ) ;
#13404=CARTESIAN_POINT ( 'NONE',  ( 0.05219959533909260263, 19.03943276465977164, 49.99890960531435979 ) ) ;
#13406=CARTESIAN_POINT ( 'NONE',  ( 5.153800228976335163, 19.02544592524342804, 99.79057627198102409 ) ) ;
#13407=CARTESIAN_POINT ( 'NONE',  ( 12.14591786802327356, -12.06949235617739191, 95.62609039468568994 ) ) ;
#13408=CARTESIAN_POINT ( 'NONE',  ( -16.51473224551082808, 9.474510206698731452, 88.33442372801900433 ) ) ;
#13409=CARTESIAN_POINT ( 'NONE',  ( 5.153800228976615827, -19.02544592524334988, 20.20942372801899722 ) ) ;
#13410=CARTESIAN_POINT ( 'NONE',  ( 0.05219959533907565091, 21.53943276465977519, 69.99890960531435269 ) ) ;
#13411=CARTESIAN_POINT ( 'NONE',  ( -8.224510206698735004, -14.34966873604973081, 94.58442372801901854 ) ) ;
#13412=CARTESIAN_POINT ( 'NONE',  ( 16.46253265017146816, 9.564922557961045513, 91.66775706135234714 ) ) ;
#13413=CARTESIAN_POINT ( 'NONE',  ( 19.03943276465977164, -0.05219959533909143690, 43.74890960531435979 ) ) ;
#13414=CARTESIAN_POINT ( 'NONE',  ( 16.51473224551069308, 9.474510206698969483, 89.16557627198103830 ) ) ;
#13415=CARTESIAN_POINT ( 'NONE',  ( 18.62759615963255655, 10.81492255796105972, 56.66775706135235424 ) ) ;
#13416=CARTESIAN_POINT ( 'NONE',  ( 9.564922557960805705, 16.46253265017160317, 59.58224293864769550 ) ) ;
#13417=CARTESIAN_POINT ( 'NONE',  ( -4.483927247898539470, -16.52544592524342804, 87.29057627198103830 ) ) ;
#13419=CARTESIAN_POINT ( 'NONE',  ( -4.379528057220328563, 16.55341960407611168, 75.20724293864769550 ) ) ;
#13420=CARTESIAN_POINT ( 'NONE',  ( 10.81492255796078972, 18.62759615963270932, 79.58224293864769550 ) ) ;
#13421=CARTESIAN_POINT ( 'NONE',  ( 13.97604488694548053, -13.89961937509957401, 95.62609039468563310 ) ) ;
#13422=CARTESIAN_POINT ( 'NONE',  ( 19.39720447994794483, 5.500000000000019540, 92.16317477297178584 ) ) ;
#13423=CARTESIAN_POINT ( 'NONE',  ( -16.46253265017146816, -9.564922557961047289, 39.16775706135234003 ) ) ;
#13424=CARTESIAN_POINT ( 'NONE',  ( 17.40805194821986035, -6.112264579160785694, 73.33371272510611050 ) ) ;
#13425=CARTESIAN_POINT ( 'NONE',  ( 0.05219959533909260263, 19.03943276465977164, 74.99890960531435269 ) ) ;
#13426=CARTESIAN_POINT ( 'NONE',  ( -16.51473224551069308, -9.474510206698971260, 81.66557627198103830 ) ) ;
#13427=CARTESIAN_POINT ( 'NONE',  ( 4.379528057220092307, 16.55341960407617563, 67.29275706135234714 ) ) ;
#13429=CARTESIAN_POINT ( 'NONE',  ( 19.03943276465977164, 0.05219959533936151252, 46.25109039468566863 ) ) ;
#13430=CARTESIAN_POINT ( 'NONE',  ( 17.45411292087690569, 5.827443620977868832, 21.68149470724943129 ) ) ;
#13431=CARTESIAN_POINT ( 'NONE',  ( -13.89961937509977652, 13.97604488694528158, 110.6239096053143243 ) ) ;
#13432=CARTESIAN_POINT ( 'NONE',  ( 0.05219959533934541429, -16.53943276465976808, 95.00109039468568994 ) ) ;
#13434=CARTESIAN_POINT ( 'NONE',  ( -12.06949235617739369, -12.14591786802326823, 74.37609039468568994 ) ) ;
#13435=DIRECTION ( 'NONE',  ( 0.000000000000000000, 0.000000000000000000, -1.000000000000000000 ) ) ;
#13436=CARTESIAN_POINT ( 'NONE',  ( 8.224510206698742110, 14.34966873604972548, 52.08442372801901854 ) ) ;
#13438=CARTESIAN_POINT ( 'NONE',  ( -10.72451020669870658, -18.67979575497194134, 64.58442372801900433 ) ) ;
#13439=CARTESIAN_POINT ( 'NONE',  ( -13.89961937509957401, -13.97604488694547875, 69.37609039468564731 ) ) ;
#13440=CARTESIAN_POINT ( 'NONE',  ( 0.05219959533936267826, -19.03943276465977164, 25.00109039468566152 ) ) ;
#13441=CARTESIAN_POINT ( 'NONE',  ( 0.05219959533909260263, 19.03943276465977164, 54.99890960531435979 ) ) ;
#13442=CARTESIAN_POINT ( 'NONE',  ( -16.46253265017160317, 9.564922557960807481, 40.83224293864769550 ) ) ;
#13444=CARTESIAN_POINT ( 'NONE',  ( 21.53943276465977519, -0.05219959533907433946, 63.74890960531435979 ) ) ;
#13445=CARTESIAN_POINT ( 'NONE',  ( -9.474510206698964154, 16.51473224551069663, 115.4155762719810241 ) ) ;
#13446=CARTESIAN_POINT ( 'NONE',  ( 13.89961937509977652, -13.97604488694527269, 23.12390960531436335 ) ) ;
#13447=CARTESIAN_POINT ( 'NONE',  ( 12.14591786802327356, -12.06949235617739191, 45.62609039468567573 ) ) ;
#13449=CARTESIAN_POINT ( 'NONE',  ( 18.62759615963271287, -10.81492255796078972, 113.3322429386476955 ) ) ;
#13450=CARTESIAN_POINT ( 'NONE',  ( 16.52544592524342804, -4.483927247898539470, 58.54057627198103120 ) ) ;
#13452=CARTESIAN_POINT ( 'NONE',  ( 5.153800228976615827, -19.02544592524334988, 110.2094237280189901 ) ) ;
#13453=CARTESIAN_POINT ( 'NONE',  ( -5.153800228976607833, 19.02544592524334988, 42.70942372801901143 ) ) ;
#13454=CARTESIAN_POINT ( 'NONE',  ( -4.379528057220328563, 16.55341960407611168, 40.20724293864769550 ) ) ;
#13455=CARTESIAN_POINT ( 'NONE',  ( -0.05219959533907301413, -21.53943276465977519, 112.4989096053143669 ) ) ;
#13456=CARTESIAN_POINT ( 'NONE',  ( 16.29526858892879204, 7.335722546919996034, 33.29670597800208043 ) ) ;
#13457=CARTESIAN_POINT ( 'NONE',  ( 18.62759615963271287, -10.81492255796078972, 58.33224293864768839 ) ) ;
#13458=CARTESIAN_POINT ( 'NONE',  ( -9.564922557960796823, -16.46253265017161027, 87.08224293864769550 ) ) ;
#13459=CARTESIAN_POINT ( 'NONE',  ( 12.06949235617757843, -12.14591786802309237, 58.12390960531435979 ) ) ;
#13460=CARTESIAN_POINT ( 'NONE',  ( 13.97604488694527802, 13.89961937509977652, 104.3739096053143385 ) ) ;
#13462=CARTESIAN_POINT ( 'NONE',  ( -16.46253265017146816, -9.564922557961047289, 49.16775706135233293 ) ) ;
#13463=CARTESIAN_POINT ( 'NONE',  ( 15.72974639402199770, -15.80617190586745480, 103.1239096053143811 ) ) ;
#13464=CARTESIAN_POINT ( 'NONE',  ( -0.05219959533909027116, -19.03943276465977164, 47.49890960531435979 ) ) ;
#13465=CARTESIAN_POINT ( 'NONE',  ( 13.97604488694527802, 13.89961937509977652, 24.37390960531435624 ) ) ;
#13467=CARTESIAN_POINT ( 'NONE',  ( 10.81492255796106328, -18.62759615963255655, 55.41775706135234714 ) ) ;
#13469=CARTESIAN_POINT ( 'NONE',  ( -16.53943276465976808, 0.05219959533911058130, 31.24890960531435979 ) ) ;
#13470=CARTESIAN_POINT ( 'NONE',  ( -19.02544592524342804, 5.153800228976336051, 46.04057627198101699 ) ) ;
#13471=CARTESIAN_POINT ( 'NONE',  ( -9.474510206698964154, 16.51473224551069663, 105.4155762719810383 ) ) ;
#13472=CARTESIAN_POINT ( 'NONE',  ( 5.823673210054125526, 21.52544592524343514, 74.79057627198105251 ) ) ;
#13474=CARTESIAN_POINT ( 'NONE',  ( -16.51473224551069308, -9.474510206698971260, 41.66557627198103120 ) ) ;
#13475=CARTESIAN_POINT ( 'NONE',  ( 21.53943276465977519, -0.05219959533907433946, 58.74890960531436690 ) ) ;
#13476=CARTESIAN_POINT ( 'NONE',  ( 21.53943276465977519, 0.05219959533937863772, 91.25109039468568994 ) ) ;
#13477=CARTESIAN_POINT ( 'NONE',  ( -16.55341960407617563, 4.379528057220093196, 83.54275706135234714 ) ) ;
#13478=CARTESIAN_POINT ( 'NONE',  ( 4.483927247898545687, 16.52544592524342804, 74.79057627198105251 ) ) ;
#13479=CARTESIAN_POINT ( 'NONE',  ( 19.02544592524343514, -5.153800228976328945, 68.54057627198103830 ) ) ;
#13481=CARTESIAN_POINT ( 'NONE',  ( -0.05219959533936034679, 19.03943276465977164, 32.50109039468566863 ) ) ;
#13482=CARTESIAN_POINT ( 'NONE',  ( -4.379528057220086978, -16.55341960407618274, 94.79275706135234714 ) ) ;
#13483=CARTESIAN_POINT ( 'NONE',  ( -10.81492255796105439, 18.62759615963255655, 112.9177570613523329 ) ) ;
#13484=CARTESIAN_POINT ( 'NONE',  ( 16.46253265017160672, -9.564922557960803928, 73.33224293864769550 ) ) ;
#13485=CARTESIAN_POINT ( 'NONE',  ( -18.67979575497178146, -10.72451020669898902, 46.66557627198102409 ) ) ;
#13486=CARTESIAN_POINT ( 'NONE',  ( -16.53943276465976808, -0.05219959533934237506, 18.75109039468568639 ) ) ;
#13487=CARTESIAN_POINT ( 'NONE',  ( -21.55341960407619339, 5.719274019375674811, 93.54275706135234714 ) ) ;
#13488=CARTESIAN_POINT ( 'NONE',  ( 8.224510206698742110, 14.34966873604972548, 67.08442372801901854 ) ) ;
#13489=CARTESIAN_POINT ( 'NONE',  ( -0.05219959533907301413, -21.53943276465977519, 112.4989096053143669 ) ) ;
#13490=CARTESIAN_POINT ( 'NONE',  ( -9.564922557961040184, 16.46253265017147172, 112.9177570613523329 ) ) ;
#13491=CARTESIAN_POINT ( 'NONE',  ( -19.03943276465977164, 0.05219959533909376836, 91.24890960531436690 ) ) ;
#13492=CARTESIAN_POINT ( 'NONE',  ( 8.224510206698742110, 14.34966873604972548, 22.08442372801901143 ) ) ;
#13493=CARTESIAN_POINT ( 'NONE',  ( 16.46253265017160672, -9.564922557960803928, 48.33224293864769550 ) ) ;
#13494=CARTESIAN_POINT ( 'NONE',  ( -0.05219959533934338120, 16.53943276465976808, 37.50109039468568284 ) ) ;
#13495=CARTESIAN_POINT ( 'NONE',  ( -12.06949235617756955, 12.14591786802309770, 80.62390960531438111 ) ) ;
#13496=CARTESIAN_POINT ( 'NONE',  ( -4.483927247898782831, 16.52544592524335698, 92.70942372801901854 ) ) ;
#13497=CARTESIAN_POINT ( 'NONE',  ( 15.80617190586769283, -15.72974639402175789, 25.62609039468567929 ) ) ;
#13498=CARTESIAN_POINT ( 'NONE',  ( -5.153800228976328057, -19.02544592524343514, 67.29057627198102409 ) ) ;
#13499=CARTESIAN_POINT ( 'NONE',  ( -0.05219959533909027116, -19.03943276465977164, 77.49890960531435269 ) ) ;
#13500=CARTESIAN_POINT ( 'NONE',  ( -12.14591786802326823, 12.06949235617739902, 88.12609039468570415 ) ) ;
#13503=ORIENTED_EDGE ( 'NONE', *, *, #26464, .T. ) ;
#13504=CARTESIAN_POINT ( 'NONE',  ( 19.05341960407617918, -5.049401038297876454, 31.04275706135232227 ) ) ;
#13505=CARTESIAN_POINT ( 'NONE',  ( -16.46253265017160317, 9.564922557960807481, 95.83224293864769550 ) ) ;
#13506=CARTESIAN_POINT ( 'NONE',  ( 19.05341960407611168, 5.049401038298154454, 53.95724293864770260 ) ) ;
#13508=CARTESIAN_POINT ( 'NONE',  ( 16.55341960407618274, -4.379528057220086978, 36.04275706135234714 ) ) ;
#13509=CARTESIAN_POINT ( 'NONE',  ( 13.97604488694548053, -13.89961937509957401, 55.62609039468566863 ) ) ;
#13510=CARTESIAN_POINT ( 'NONE',  ( 14.34966873604972726, -8.224510206698740333, 40.83442372801901854 ) ) ;
#13511=CARTESIAN_POINT ( 'NONE',  ( 13.97604488694527802, 13.89961937509977652, 109.3739096053143669 ) ) ;
#13512=CARTESIAN_POINT ( 'NONE',  ( 13.97604488694527802, 13.89961937509977652, 74.37390960531436690 ) ) ;
#13513=CARTESIAN_POINT ( 'NONE',  ( -21.55341960407610458, -5.719274019375992779, 96.45724293864770971 ) ) ;
#13514=CARTESIAN_POINT ( 'NONE',  ( 16.46253265017146816, 9.564922557961045513, 61.66775706135234003 ) ) ;
#13515=CARTESIAN_POINT ( 'NONE',  ( -5.049401038298153566, 19.05341960407611168, 95.20724293864770971 ) ) ;
#13516=CARTESIAN_POINT ( 'NONE',  ( 17.47739027167831694, -4.111523782424557183, 21.69296162454243770 ) ) ;
#13517=CARTESIAN_POINT ( 'NONE',  ( 5.049401038298161559, -19.05341960407611168, 62.70724293864769550 ) ) ;
#13518=CARTESIAN_POINT ( 'NONE',  ( -14.29746914071049879, 8.314922557960819915, 35.83224293864768839 ) ) ;
#13519=CARTESIAN_POINT ( 'NONE',  ( -9.564922557960796823, -16.46253265017161027, 27.08224293864769550 ) ) ;
#13520=CARTESIAN_POINT ( 'NONE',  ( -9.564922557961040184, 16.46253265017147172, 37.91775706135233293 ) ) ;
#13521=CARTESIAN_POINT ( 'NONE',  ( -14.29746914071049879, 8.314922557960819915, 75.83224293864769550 ) ) ;
#13522=CARTESIAN_POINT ( 'NONE',  ( 18.62759615963255655, 10.81492255796105972, 96.66775706135234714 ) ) ;
#13523=CARTESIAN_POINT ( 'NONE',  ( 19.03943276465977164, -0.05219959533909143690, 33.74890960531435979 ) ) ;
#13524=CARTESIAN_POINT ( 'NONE',  ( -8.314922557961024197, 14.29746914071037800, 47.91775706135234714 ) ) ;
#13525=CARTESIAN_POINT ( 'NONE',  ( -0.05219959533910754901, -16.53943276465976808, 37.49890960531436690 ) ) ;
#13526=CARTESIAN_POINT ( 'NONE',  ( -21.52544592524334988, -5.823673210054445271, 108.9594237280190185 ) ) ;
#13527=CARTESIAN_POINT ( 'NONE',  ( 19.03943276465977164, -0.05219959533909143690, 98.74890960531436690 ) ) ;
#13528=CARTESIAN_POINT ( 'NONE',  ( 16.46253265017160672, -9.564922557960803928, 88.33224293864769550 ) ) ;
#13529=CARTESIAN_POINT ( 'NONE',  ( 19.02544592524343514, -5.153800228976328945, 28.54057627198102409 ) ) ;
#13530=CARTESIAN_POINT ( 'NONE',  ( -12.06949235617756955, 12.14591786802309770, 105.6239096053143669 ) ) ;
#13531=CARTESIAN_POINT ( 'NONE',  ( -0.05219959533910754901, -16.53943276465976808, 77.49890960531433848 ) ) ;
#13532=CARTESIAN_POINT ( 'NONE',  ( -0.05219959533907301413, -21.53943276465977519, 82.49890960531436690 ) ) ;
#13533=CARTESIAN_POINT ( 'NONE',  ( -9.474510206698964154, 16.51473224551069663, 90.41557627198103830 ) ) ;
#13534=CARTESIAN_POINT ( 'NONE',  ( 10.81492255796078972, 18.62759615963270932, 94.58224293864769550 ) ) ;
#13535=CARTESIAN_POINT ( 'NONE',  ( 0.05219959533909260263, 19.03943276465977164, 94.99890960531436690 ) ) ;
#13536=CARTESIAN_POINT ( 'NONE',  ( 18.39443945427639093, -5.500000000000022204, 46.01745347608652281 ) ) ;
#13537=CARTESIAN_POINT ( 'NONE',  ( -0.05219959533910754901, -16.53943276465976808, 87.49890960531436690 ) ) ;
#13538=CARTESIAN_POINT ( 'NONE',  ( 19.05341960407611168, 5.049401038298154454, 58.95724293864768129 ) ) ;
#13539=CARTESIAN_POINT ( 'NONE',  ( 10.72451020669898902, -18.67979575497178502, 72.91557627198103830 ) ) ;
#13540=EDGE_CURVE ( 'NONE', #155869, #53672, #71948, .T. ) ;
#13542=CARTESIAN_POINT ( 'NONE',  ( 12.14591786802327356, -12.06949235617739191, 110.6260903946857042 ) ) ;
#13543=CARTESIAN_POINT ( 'NONE',  ( -14.29746914071037622, -8.314922557961029526, 24.16775706135235424 ) ) ;
#13544=CARTESIAN_POINT ( 'NONE',  ( -16.53943276465976808, 0.05219959533911058130, 86.24890960531436690 ) ) ;
#13545=CARTESIAN_POINT ( 'NONE',  ( -17.49999999999999645, -5.624438216177593652, 94.18329655085352670 ) ) ;
#13546=CARTESIAN_POINT ( 'NONE',  ( 16.46253265017160672, -9.564922557960803928, 78.33224293864769550 ) ) ;
#13547=CARTESIAN_POINT ( 'NONE',  ( -19.03943276465977164, 0.05219959533909376836, 51.24890960531436690 ) ) ;
#13548=CARTESIAN_POINT ( 'NONE',  ( 12.06949235617757843, -12.14591786802309237, 68.12390960531436690 ) ) ;
#13549=CARTESIAN_POINT ( 'NONE',  ( 0.05219959533909260263, 19.03943276465977164, 114.9989096053143669 ) ) ;
#13550=CARTESIAN_POINT ( 'NONE',  ( 5.153800228976615827, -19.02544592524334988, 100.2094237280190043 ) ) ;
#13551=CARTESIAN_POINT ( 'NONE',  ( -5.823673210054431948, 21.52544592524334988, 57.70942372801901143 ) ) ;
#13552=CARTESIAN_POINT ( 'NONE',  ( 19.03943276465977164, -0.05219959533909143690, 103.7489096053143669 ) ) ;
#13553=CARTESIAN_POINT ( 'NONE',  ( -5.823673210054116645, -21.52544592524344225, 82.29057627198103830 ) ) ;
#13554=CARTESIAN_POINT ( 'NONE',  ( -16.52544592524335698, -4.483927247898792601, 68.95942372801901854 ) ) ;
#13555=CARTESIAN_POINT ( 'NONE',  ( -17.44279575226785894, 5.990770900253882481, 95.83557567514318976 ) ) ;
#13556=CARTESIAN_POINT ( 'NONE',  ( 9.474510206698971260, -16.51473224551069308, 72.91557627198102409 ) ) ;
#13557=CARTESIAN_POINT ( 'NONE',  ( 21.55341960407610458, 5.719274019375980345, 83.95724293864770971 ) ) ;
#13558=CARTESIAN_POINT ( 'NONE',  ( -9.564922557961040184, 16.46253265017147172, 102.9177570613523329 ) ) ;
#13559=CARTESIAN_POINT ( 'NONE',  ( -12.14591786802309592, -12.06949235617757132, 41.87390960531435979 ) ) ;
#13560=CARTESIAN_POINT ( 'NONE',  ( -21.53943276465977519, -0.05219959533937600094, 53.75109039468568994 ) ) ;
#13561=CARTESIAN_POINT ( 'NONE',  ( -14.29746914071037622, -8.314922557961029526, 84.16775706135234714 ) ) ;
#13562=CARTESIAN_POINT ( 'NONE',  ( 5.049401038298161559, -19.05341960407611168, 102.7072429386476955 ) ) ;
#13563=CARTESIAN_POINT ( 'NONE',  ( -13.97604488694527625, -13.89961937509977830, 101.8739096053143669 ) ) ;
#13565=CARTESIAN_POINT ( 'NONE',  ( -4.483927247898782831, 16.52544592524335698, 97.70942372801904696 ) ) ;
#13566=CARTESIAN_POINT ( 'NONE',  ( 4.379528057220092307, 16.55341960407617563, 52.29275706135236135 ) ) ;
#13567=CARTESIAN_POINT ( 'NONE',  ( 13.89961937509977652, -13.97604488694527269, 58.12390960531436690 ) ) ;
#13568=CARTESIAN_POINT ( 'NONE',  ( -0.05219959533909027116, -19.03943276465977164, 67.49890960531436690 ) ) ;
#13569=CARTESIAN_POINT ( 'NONE',  ( 5.719274019375673035, 21.55341960407619339, 62.29275706135236845 ) ) ;
#13570=CARTESIAN_POINT ( 'NONE',  ( -8.314922557961024197, 14.29746914071037800, 67.91775706135234714 ) ) ;
#13571=CARTESIAN_POINT ( 'NONE',  ( -16.55341960407611168, -4.379528057220339221, 51.45724293864770260 ) ) ;
#13572=CARTESIAN_POINT ( 'NONE',  ( 9.474510206698971260, -16.51473224551069308, 47.91557627198102409 ) ) ;
#13573=CARTESIAN_POINT ( 'NONE',  ( 13.89961937509977652, -13.97604488694527269, 53.12390960531434558 ) ) ;
#13574=CARTESIAN_POINT ( 'NONE',  ( -14.34966873604972548, 8.224510206698743886, 38.33442372801900433 ) ) ;
#13575=CARTESIAN_POINT ( 'NONE',  ( -5.049401038297874678, -19.05341960407617918, 89.79275706135230450 ) ) ;
#13576=CARTESIAN_POINT ( 'NONE',  ( 12.14591786802309770, 12.06949235617756955, 94.37390960531436690 ) ) ;
#13577=CARTESIAN_POINT ( 'NONE',  ( 16.51473224551069308, 9.474510206698969483, 69.16557627198102409 ) ) ;
#13578=CARTESIAN_POINT ( 'NONE',  ( -0.05219959533936034679, 19.03943276465977164, 102.5010903946856757 ) ) ;
#13580=CARTESIAN_POINT ( 'NONE',  ( 10.81492255796106328, -18.62759615963255655, 90.41775706135236135 ) ) ;
#13581=CARTESIAN_POINT ( 'NONE',  ( 16.53943276465976808, 0.05219959533934440121, 61.25109039468567573 ) ) ;
#13583=CARTESIAN_POINT ( 'NONE',  ( 15.72974639402199770, -15.80617190586745480, 58.12390960531435979 ) ) ;
#13584=CARTESIAN_POINT ( 'NONE',  ( -12.14591786802326823, 12.06949235617739902, 53.12609039468568284 ) ) ;
#13585=CARTESIAN_POINT ( 'NONE',  ( -9.564922557960796823, -16.46253265017161027, 37.08224293864768839 ) ) ;
#13586=CARTESIAN_POINT ( 'NONE',  ( -16.46253265017146816, -9.564922557961047289, 49.16775706135233293 ) ) ;
#13587=CARTESIAN_POINT ( 'NONE',  ( -19.05341960407611168, -5.049401038298163336, 86.45724293864769550 ) ) ;
#13588=CARTESIAN_POINT ( 'NONE',  ( 19.02544592524343514, -5.153800228976328945, 23.54057627198102054 ) ) ;
#13589=CARTESIAN_POINT ( 'NONE',  ( -5.049401038298153566, 19.05341960407611168, 70.20724293864769550 ) ) ;
#13591=CARTESIAN_POINT ( 'NONE',  ( -15.80617190586768217, 15.72974639402176855, 83.12609039468568994 ) ) ;
#13592=CARTESIAN_POINT ( 'NONE',  ( -18.22780087662121673, -5.500000000000063061, 56.48459894673892734 ) ) ;
#13593=CARTESIAN_POINT ( 'NONE',  ( -13.89961937509957401, -13.97604488694547875, 39.37609039468566152 ) ) ;
#13594=CARTESIAN_POINT ( 'NONE',  ( -5.049401038297874678, -19.05341960407617918, 24.79275706135233648 ) ) ;
#13595=CARTESIAN_POINT ( 'NONE',  ( 4.379528057220339221, -16.55341960407611168, 52.70724293864769550 ) ) ;
#13596=CARTESIAN_POINT ( 'NONE',  ( 0.05219959533909260263, 19.03943276465977164, 54.99890960531435979 ) ) ;
#13597=CARTESIAN_POINT ( 'NONE',  ( 18.67979575497178502, 10.72451020669898547, 24.16557627198103120 ) ) ;
#13598=CARTESIAN_POINT ( 'NONE',  ( -5.823673210054431948, 21.52544592524334988, 77.70942372801900433 ) ) ;
#13599=CARTESIAN_POINT ( 'NONE',  ( -16.51473224551069308, -9.474510206698971260, 61.66557627198103120 ) ) ;
#13600=CARTESIAN_POINT ( 'NONE',  ( -18.67979575497193778, 10.72451020669871902, 78.33442372801901854 ) ) ;
#13601=CARTESIAN_POINT ( 'NONE',  ( -21.52544592524343514, 5.823673210054127303, 31.04057627198102409 ) ) ;
#13602=CARTESIAN_POINT ( 'NONE',  ( -10.81492255796105439, 18.62759615963255655, 42.91775706135235424 ) ) ;
#13603=CARTESIAN_POINT ( 'NONE',  ( 5.153800228976615827, -19.02544592524334988, 55.20942372801899722 ) ) ;
#13604=CARTESIAN_POINT ( 'NONE',  ( -16.46253265017160317, 9.564922557960807481, 45.83224293864769550 ) ) ;
#13605=CARTESIAN_POINT ( 'NONE',  ( 13.97604488694527802, 13.89961937509977652, 74.37390960531436690 ) ) ;
#13606=CARTESIAN_POINT ( 'NONE',  ( -8.314922557961024197, 14.29746914071037800, 32.91775706135234714 ) ) ;
#13607=CARTESIAN_POINT ( 'NONE',  ( -8.224510206698948167, 14.34966873604960824, 95.41557627198102409 ) ) ;
#13608=CARTESIAN_POINT ( 'NONE',  ( -19.02544592524342804, 5.153800228976336051, 56.04057627198100988 ) ) ;
#13609=CARTESIAN_POINT ( 'NONE',  ( 0.05219959533907565091, 21.53943276465977519, 44.99890960531435979 ) ) ;
#13610=CARTESIAN_POINT ( 'NONE',  ( 0.05219959533934541429, -16.53943276465976808, 25.00109039468567218 ) ) ;
#13611=CARTESIAN_POINT ( 'NONE',  ( -10.72451020669870658, -18.67979575497194134, 24.58442372801901499 ) ) ;
#13612=CARTESIAN_POINT ( 'NONE',  ( -10.72451020669870658, -18.67979575497194134, 74.58442372801901854 ) ) ;
#13614=CARTESIAN_POINT ( 'NONE',  ( -8.314922557961024197, 14.29746914071037800, 67.91775706135234714 ) ) ;
#13615=CARTESIAN_POINT ( 'NONE',  ( -8.314922557961024197, 14.29746914071037800, 67.91775706135234714 ) ) ;
#13616=CARTESIAN_POINT ( 'NONE',  ( -19.03943276465977164, 0.05219959533909376836, 66.24890960531436690 ) ) ;
#13617=CARTESIAN_POINT ( 'NONE',  ( 14.34966873604972726, -8.224510206698740333, 90.83442372801901854 ) ) ;
#13618=CARTESIAN_POINT ( 'NONE',  ( -9.564922557961040184, 16.46253265017147172, 37.91775706135233293 ) ) ;
#13619=CARTESIAN_POINT ( 'NONE',  ( 21.55341960407610458, 5.719274019375980345, 108.9572429386476955 ) ) ;
#13620=CARTESIAN_POINT ( 'NONE',  ( 4.483927247898545687, 16.52544592524342804, 64.79057627198103830 ) ) ;
#13621=CARTESIAN_POINT ( 'NONE',  ( 13.89961937509977652, -13.97604488694527269, 88.12390960531438111 ) ) ;
#13622=CARTESIAN_POINT ( 'NONE',  ( -14.29746914071037622, -8.314922557961029526, 94.16775706135237556 ) ) ;
#13623=CARTESIAN_POINT ( 'NONE',  ( 5.719274019375673035, 21.55341960407619339, 57.29275706135234714 ) ) ;
#13624=CARTESIAN_POINT ( 'NONE',  ( 8.314922557961029526, -14.29746914071037800, 35.41775706135234003 ) ) ;
#13625=CARTESIAN_POINT ( 'NONE',  ( -15.72974639402176322, -15.80617190586768395, 29.37609039468568284 ) ) ;
#13626=CARTESIAN_POINT ( 'NONE',  ( 14.34966873604960469, 8.224510206698951720, 59.16557627198103120 ) ) ;
#13628=CARTESIAN_POINT ( 'NONE',  ( -18.62759615963270932, 10.81492255796079327, 95.83224293864770971 ) ) ;
#13629=CARTESIAN_POINT ( 'NONE',  ( -4.379528057220328563, 16.55341960407611168, 45.20724293864769550 ) ) ;
#13632=CARTESIAN_POINT ( 'NONE',  ( -5.823673210054116645, -21.52544592524344225, 22.29057627198102765 ) ) ;
#13633=CARTESIAN_POINT ( 'NONE',  ( -10.81492255796105439, 18.62759615963255655, 42.91775706135235424 ) ) ;
#13634=CARTESIAN_POINT ( 'NONE',  ( -14.29746914071049879, 8.314922557960819915, 65.83224293864769550 ) ) ;
#13635=CARTESIAN_POINT ( 'NONE',  ( 9.474510206698971260, -16.51473224551069308, 57.91557627198103120 ) ) ;
#13636=CARTESIAN_POINT ( 'NONE',  ( -19.03943276465977164, 0.05219959533909376836, 21.24890960531436335 ) ) ;
#13637=CARTESIAN_POINT ( 'NONE',  ( -5.049401038297874678, -19.05341960407617918, 64.79275706135233293 ) ) ;
#13638=CARTESIAN_POINT ( 'NONE',  ( 10.81492255796078972, 18.62759615963270932, 54.58224293864769550 ) ) ;
#13640=CARTESIAN_POINT ( 'NONE',  ( -19.05341960407611168, -5.049401038298163336, 61.45724293864769550 ) ) ;
#13641=CARTESIAN_POINT ( 'NONE',  ( 8.224510206698742110, 14.34966873604972548, 37.08442372801901143 ) ) ;
#13642=CARTESIAN_POINT ( 'NONE',  ( -18.62759615963270932, 10.81492255796079327, 110.8322429386476955 ) ) ;
#13643=CARTESIAN_POINT ( 'NONE',  ( -12.14591786802309592, -12.06949235617757132, 41.87390960531435979 ) ) ;
#13644=EDGE_LOOP ( 'NONE', ( #185573, #160143, #79077, #16374 ) ) ;
#13645=CARTESIAN_POINT ( 'NONE',  ( 19.05341960407611168, 5.049401038298154454, 88.95724293864769550 ) ) ;
#13646=CARTESIAN_POINT ( 'NONE',  ( 21.55341960407610458, 5.719274019375980345, 78.95724293864769550 ) ) ;
#13647=CARTESIAN_POINT ( 'NONE',  ( -10.81492255796078084, -18.62759615963271287, 112.0822429386477097 ) ) ;
#13648=CARTESIAN_POINT ( 'NONE',  ( -8.314922557961024197, 14.29746914071037800, 42.91775706135235424 ) ) ;
#13649=CARTESIAN_POINT ( 'NONE',  ( -21.53943276465977519, 0.05219959533907696930, 41.24890960531435269 ) ) ;
#13650=CARTESIAN_POINT ( 'NONE',  ( -10.81492255796105439, 18.62759615963255655, 102.9177570613523756 ) ) ;
#13651=CARTESIAN_POINT ( 'NONE',  ( 13.89961937509977652, -13.97604488694527269, 103.1239096053143527 ) ) ;
#13652=CARTESIAN_POINT ( 'NONE',  ( -9.564922557960796823, -16.46253265017161027, 47.08224293864769550 ) ) ;
#13653=CARTESIAN_POINT ( 'NONE',  ( 9.474510206698971260, -16.51473224551069308, 92.91557627198103830 ) ) ;
#13654=CARTESIAN_POINT ( 'NONE',  ( 16.46253265017160672, -9.564922557960803928, 73.33224293864769550 ) ) ;
#13655=CARTESIAN_POINT ( 'NONE',  ( 16.21995358207279381, -7.366697692864220492, 87.43551001512066989 ) ) ;
#13656=CARTESIAN_POINT ( 'NONE',  ( 19.05341960407617918, -5.049401038297876454, 51.04275706135231871 ) ) ;
#13657=CARTESIAN_POINT ( 'NONE',  ( 10.81492255796106328, -18.62759615963255655, 105.4177570613523613 ) ) ;
#13658=CARTESIAN_POINT ( 'NONE',  ( -5.719274019375978568, 21.55341960407610458, 25.20724293864769550 ) ) ;
#13660=CARTESIAN_POINT ( 'NONE',  ( -8.314922557961024197, 14.29746914071037800, 102.9177570613523756 ) ) ;
#13661=CARTESIAN_POINT ( 'NONE',  ( -9.474510206698720793, -16.51473224551083518, 74.58442372801900433 ) ) ;
#13662=CARTESIAN_POINT ( 'NONE',  ( -16.88567814943164080, 6.947325034625569273, 58.70998877347415856 ) ) ;
#13663=CARTESIAN_POINT ( 'NONE',  ( 13.97604488694548053, -13.89961937509957401, 85.62609039468568994 ) ) ;
#13664=CARTESIAN_POINT ( 'NONE',  ( 16.46253265017146816, 9.564922557961045513, 36.66775706135233293 ) ) ;
#13665=CARTESIAN_POINT ( 'NONE',  ( 17.40861289039002102, 6.110651285853324843, 108.8723247082743342 ) ) ;
#13666=CARTESIAN_POINT ( 'NONE',  ( -16.51473224551069308, -9.474510206698971260, 41.66557627198103120 ) ) ;
#13667=CARTESIAN_POINT ( 'NONE',  ( 8.314922557960818139, 14.29746914071049879, 44.58224293864769550 ) ) ;
#13668=CARTESIAN_POINT ( 'NONE',  ( -5.153800228976328057, -19.02544592524343514, 22.29057627198102765 ) ) ;
#13669=CARTESIAN_POINT ( 'NONE',  ( -8.314922557960811034, -14.29746914071050412, 22.08224293864769194 ) ) ;
#13671=CARTESIAN_POINT ( 'NONE',  ( -16.55341960407617563, 4.379528057220093196, 88.54275706135236135 ) ) ;
#13672=CARTESIAN_POINT ( 'NONE',  ( 13.97604488694527802, 13.89961937509977652, 54.37390960531435979 ) ) ;
#13673=CARTESIAN_POINT ( 'NONE',  ( -15.72974639402176322, -15.80617190586768395, 109.3760903946857042 ) ) ;
#13674=CARTESIAN_POINT ( 'NONE',  ( 5.153800228976615827, -19.02544592524334988, 110.2094237280189901 ) ) ;
#13675=CARTESIAN_POINT ( 'NONE',  ( 5.823673210054444382, -21.52544592524334988, 95.20942372801903275 ) ) ;
#13677=CARTESIAN_POINT ( 'NONE',  ( -19.05341960407611168, -5.049401038298163336, 91.45724293864766707 ) ) ;
#13678=CARTESIAN_POINT ( 'NONE',  ( -5.153800228976328057, -19.02544592524343514, 77.29057627198099567 ) ) ;
#13680=CARTESIAN_POINT ( 'NONE',  ( 10.72451020669898902, -18.67979575497178502, 107.9155762719810241 ) ) ;
#13681=CARTESIAN_POINT ( 'NONE',  ( 12.06949235617757843, -12.14591786802309237, 83.12390960531436690 ) ) ;
#13682=CARTESIAN_POINT ( 'NONE',  ( 18.67979575497178502, 10.72451020669898547, 74.16557627198102409 ) ) ;
#13683=CARTESIAN_POINT ( 'NONE',  ( -16.51473224551069308, -9.474510206698971260, 61.66557627198103120 ) ) ;
#13684=CARTESIAN_POINT ( 'NONE',  ( -15.72974639402197994, 15.80617190586746368, 100.6239096053143811 ) ) ;
#13685=CARTESIAN_POINT ( 'NONE',  ( 14.29746914071037800, 8.314922557961029526, 91.66775706135234714 ) ) ;
#13687=CARTESIAN_POINT ( 'NONE',  ( 5.049401038298161559, -19.05341960407611168, 62.70724293864769550 ) ) ;
#13688=CARTESIAN_POINT ( 'NONE',  ( -14.29746914071049879, 8.314922557960819915, 90.83224293864769550 ) ) ;
#13690=CARTESIAN_POINT ( 'NONE',  ( 9.564922557960805705, 16.46253265017160317, 54.58224293864769550 ) ) ;
#13691=CARTESIAN_POINT ( 'NONE',  ( 5.049401038297881783, 19.05341960407617563, 82.29275706135229029 ) ) ;
#13692=CARTESIAN_POINT ( 'NONE',  ( -8.224510206698948167, 14.34966873604960824, 80.41557627198103830 ) ) ;
#13693=CARTESIAN_POINT ( 'NONE',  ( 21.53943276465977519, 0.05219959533937863772, 61.25109039468567573 ) ) ;
#13694=CARTESIAN_POINT ( 'NONE',  ( 5.153800228976335163, 19.02544592524342804, 34.79057627198102409 ) ) ;
#13695=CARTESIAN_POINT ( 'NONE',  ( -10.81492255796078084, -18.62759615963271287, 112.0822429386477097 ) ) ;
#13696=CARTESIAN_POINT ( 'NONE',  ( 0.05219959533910956823, 16.53943276465976808, 99.99890960531436690 ) ) ;
#13698=CARTESIAN_POINT ( 'NONE',  ( 9.474510206698971260, -16.51473224551069308, 52.91557627198102409 ) ) ;
#13700=CARTESIAN_POINT ( 'NONE',  ( -19.05341960407617563, 5.049401038297882671, 88.54275706135230450 ) ) ;
#13701=CARTESIAN_POINT ( 'NONE',  ( 0.05219959533909260263, 19.03943276465977164, 114.9989096053143669 ) ) ;
#13702=CARTESIAN_POINT ( 'NONE',  ( -5.719274019375665041, -21.55341960407619695, 49.79275706135234714 ) ) ;
#13703=CARTESIAN_POINT ( 'NONE',  ( 0.05219959533909260263, 19.03943276465977164, 84.99890960531436690 ) ) ;
#13704=CARTESIAN_POINT ( 'NONE',  ( -19.05341960407617563, 5.049401038297882671, 73.54275706135233293 ) ) ;
#13705=CARTESIAN_POINT ( 'NONE',  ( 19.03943276465977164, -0.05219959533909143690, 63.74890960531435979 ) ) ;
#13707=CARTESIAN_POINT ( 'NONE',  ( 16.55341960407611168, 4.379528057220329451, 73.95724293864769550 ) ) ;
#13708=CARTESIAN_POINT ( 'NONE',  ( 16.53943276465976808, -0.05219959533910856209, 83.74890960531435269 ) ) ;
#13709=CARTESIAN_POINT ( 'NONE',  ( -16.46253265017160317, 9.564922557960807481, 85.83224293864769550 ) ) ;
#13710=CARTESIAN_POINT ( 'NONE',  ( -8.224510206698948167, 14.34966873604960824, 75.41557627198102409 ) ) ;
#13711=CARTESIAN_POINT ( 'NONE',  ( -19.05341960407611168, -5.049401038298163336, 91.45724293864766707 ) ) ;
#13712=CARTESIAN_POINT ( 'NONE',  ( 5.049401038297881783, 19.05341960407617563, 32.29275706135233293 ) ) ;
#13713=CARTESIAN_POINT ( 'NONE',  ( 19.02544592524343514, -5.153800228976328945, 48.54057627198103120 ) ) ;
#13714=CARTESIAN_POINT ( 'NONE',  ( 16.53943276465976808, -0.05219959533910856209, 23.74890960531435269 ) ) ;
#13715=CARTESIAN_POINT ( 'NONE',  ( -12.14591786802309592, -12.06949235617757132, 106.8739096053143811 ) ) ;
#13717=CARTESIAN_POINT ( 'NONE',  ( 10.81492255796106328, -18.62759615963255655, 45.41775706135234003 ) ) ;
#13718=CARTESIAN_POINT ( 'NONE',  ( -9.564922557961040184, 16.46253265017147172, 62.91775706135233293 ) ) ;
#13719=CARTESIAN_POINT ( 'NONE',  ( 8.224510206698953496, -14.34966873604960469, 32.91557627198102409 ) ) ;
#13720=CARTESIAN_POINT ( 'NONE',  ( -10.72451020669898014, 18.67979575497178502, 80.41557627198103830 ) ) ;
#13721=CARTESIAN_POINT ( 'NONE',  ( 15.72974639402199770, -15.80617190586745480, 23.12390960531436335 ) ) ;
#13722=CARTESIAN_POINT ( 'NONE',  ( -12.14591786802309592, -12.06949235617757132, 66.87390960531436690 ) ) ;
#13723=CARTESIAN_POINT ( 'NONE',  ( 13.97604488694527802, 13.89961937509977652, 49.37390960531434558 ) ) ;
#13724=CARTESIAN_POINT ( 'NONE',  ( 19.02544592524334988, 5.153800228976608722, 41.45942372801900433 ) ) ;
#13725=CARTESIAN_POINT ( 'NONE',  ( 4.379528057220092307, 16.55341960407617563, 102.2927570613523613 ) ) ;
#13726=CARTESIAN_POINT ( 'NONE',  ( 16.52544592524335698, 4.483927247898782831, 51.45942372801901854 ) ) ;
#13727=CARTESIAN_POINT ( 'NONE',  ( 21.52544592524344225, -5.823673210054117533, 38.54057627198103120 ) ) ;
#13728=CARTESIAN_POINT ( 'NONE',  ( -0.05219959533937732626, 21.53943276465977519, 102.5010903946856899 ) ) ;
#13729=CARTESIAN_POINT ( 'NONE',  ( -16.51473224551069308, -9.474510206698971260, 96.66557627198102409 ) ) ;
#13730=CARTESIAN_POINT ( 'NONE',  ( 0.05219959533934541429, -16.53943276465976808, 75.00109039468568994 ) ) ;
#13731=CARTESIAN_POINT ( 'NONE',  ( -19.03943276465977164, 0.05219959533909376836, 26.24890960531435624 ) ) ;
#13732=CARTESIAN_POINT ( 'NONE',  ( 8.224510206698953496, -14.34966873604960469, 37.91557627198102409 ) ) ;
#13733=CARTESIAN_POINT ( 'NONE',  ( 19.03943276465977164, -0.05219959533909143690, 98.74890960531436690 ) ) ;
#13734=CARTESIAN_POINT ( 'NONE',  ( -9.474510206698964154, 16.51473224551069663, 95.41557627198102409 ) ) ;
#13735=CARTESIAN_POINT ( 'NONE',  ( -21.52544592524343514, 5.823673210054127303, 26.04057627198103475 ) ) ;
#13736=CARTESIAN_POINT ( 'NONE',  ( -14.34966873604960291, -8.224510206698953496, 66.66557627198102409 ) ) ;
#13737=CARTESIAN_POINT ( 'NONE',  ( 14.34966873604960469, 8.224510206698951720, 49.16557627198102409 ) ) ;
#13739=CARTESIAN_POINT ( 'NONE',  ( 4.379528057220092307, 16.55341960407617563, 57.29275706135234714 ) ) ;
#13740=DIRECTION ( 'NONE',  ( -0.000000000000000000, 1.000000000000000000, 0.000000000000000000 ) ) ;
#13741=CARTESIAN_POINT ( 'NONE',  ( 13.97604488694548053, -13.89961937509957401, 50.62609039468566152 ) ) ;
#13742=CARTESIAN_POINT ( 'NONE',  ( 13.97604488694527802, 13.89961937509977652, 89.37390960531436690 ) ) ;
#13743=CARTESIAN_POINT ( 'NONE',  ( 13.89961937509957401, 13.97604488694547697, 61.87609039468566863 ) ) ;
#13745=CARTESIAN_POINT ( 'NONE',  ( 19.05341960407617918, -5.049401038297876454, 51.04275706135231871 ) ) ;
#13746=CARTESIAN_POINT ( 'NONE',  ( -19.02544592524334988, -5.153800228976617603, 98.95942372801900433 ) ) ;
#13747=CARTESIAN_POINT ( 'NONE',  ( 14.29746914071037800, 8.314922557961029526, 101.6677570613523613 ) ) ;
#13749=CARTESIAN_POINT ( 'NONE',  ( -9.564922557960796823, -16.46253265017161027, 22.08224293864768839 ) ) ;
#13750=CARTESIAN_POINT ( 'NONE',  ( -0.05219959533907301413, -21.53943276465977519, 22.49890960531436335 ) ) ;
#13751=CARTESIAN_POINT ( 'NONE',  ( 21.53943276465977519, 0.05219959533937863772, 46.25109039468567573 ) ) ;
#13752=CARTESIAN_POINT ( 'NONE',  ( 16.51473224551083163, -9.474510206698727899, 105.8344237280190043 ) ) ;
#13754=CARTESIAN_POINT ( 'NONE',  ( -0.05219959533909027116, -19.03943276465977164, 62.49890960531435979 ) ) ;
#13756=CARTESIAN_POINT ( 'NONE',  ( -12.06949235617756955, 12.14591786802309770, 70.62390960531436690 ) ) ;
#13757=CARTESIAN_POINT ( 'NONE',  ( 13.97604488694527802, 13.89961937509977652, 69.37390960531436690 ) ) ;
#13758=CARTESIAN_POINT ( 'NONE',  ( -16.46253265017160317, 9.564922557960807481, 80.83224293864769550 ) ) ;
#13759=CARTESIAN_POINT ( 'NONE',  ( 9.564922557961047289, -16.46253265017146816, 80.41775706135234714 ) ) ;
#13760=CARTESIAN_POINT ( 'NONE',  ( -21.53943276465977519, 0.05219959533907696930, 51.24890960531436690 ) ) ;
#13761=CARTESIAN_POINT ( 'NONE',  ( 14.29746914071049879, -8.314922557960816363, 108.3322429386477097 ) ) ;
#13762=CARTESIAN_POINT ( 'NONE',  ( -5.049401038297874678, -19.05341960407617918, 39.79275706135232582 ) ) ;
#13763=CARTESIAN_POINT ( 'NONE',  ( 16.46253265017160672, -9.564922557960803928, 73.33224293864769550 ) ) ;
#13764=CARTESIAN_POINT ( 'NONE',  ( 15.80617190586746368, 15.72974639402197994, 84.37390960531438111 ) ) ;
#13765=CARTESIAN_POINT ( 'NONE',  ( -12.14591786802309592, -12.06949235617757132, 86.87390960531438111 ) ) ;
#13766=CARTESIAN_POINT ( 'NONE',  ( 16.51473224551083163, -9.474510206698727899, 50.83442372801899722 ) ) ;
#13767=CARTESIAN_POINT ( 'NONE',  ( 21.53943276465977519, -0.05219959533907433946, 78.74890960531436690 ) ) ;
#13768=CARTESIAN_POINT ( 'NONE',  ( 21.52544592524344225, -5.823673210054117533, 58.54057627198103120 ) ) ;
#13769=CARTESIAN_POINT ( 'NONE',  ( 15.72974639402199770, -15.80617190586745480, 38.12390960531436690 ) ) ;
#13770=CARTESIAN_POINT ( 'NONE',  ( 21.52544592524334988, 5.823673210054432836, 91.45942372801901854 ) ) ;
#13771=CARTESIAN_POINT ( 'NONE',  ( -16.46253265017160317, 9.564922557960807481, 65.83224293864769550 ) ) ;
#13772=CARTESIAN_POINT ( 'NONE',  ( -8.224510206698948167, 14.34966873604960824, 110.4155762719810383 ) ) ;
#13773=CARTESIAN_POINT ( 'NONE',  ( 10.72451020669871369, 18.67979575497193778, 22.08442372801901143 ) ) ;
#13774=CARTESIAN_POINT ( 'NONE',  ( -15.72974639402176322, -15.80617190586768395, 44.37609039468567573 ) ) ;
#13775=CARTESIAN_POINT ( 'NONE',  ( -16.46253265017160317, 9.564922557960807481, 30.83224293864769550 ) ) ;
#13776=CARTESIAN_POINT ( 'NONE',  ( 21.53943276465977519, -0.05219959533907433946, 103.7489096053143669 ) ) ;
#13778=CARTESIAN_POINT ( 'NONE',  ( 19.03943276465977164, 0.05219959533936151252, 56.25109039468566863 ) ) ;
#13779=CARTESIAN_POINT ( 'NONE',  ( 5.153800228976335163, 19.02544592524342804, 34.79057627198102409 ) ) ;
#13780=CARTESIAN_POINT ( 'NONE',  ( -8.314922557961024197, 14.29746914071037800, 27.91775706135234358 ) ) ;
#13781=CARTESIAN_POINT ( 'NONE',  ( 16.44184284207323543, -7.208923782155263638, 21.54787411603375702 ) ) ;
#13782=CARTESIAN_POINT ( 'NONE',  ( 12.06949235617739724, 12.14591786802326823, 61.87609039468568284 ) ) ;
#13783=CARTESIAN_POINT ( 'NONE',  ( -16.46253265017160317, 9.564922557960807481, 35.83224293864768839 ) ) ;
#13785=CARTESIAN_POINT ( 'NONE',  ( 16.51473224551069308, 9.474510206698969483, 84.16557627198102409 ) ) ;
#13786=CARTESIAN_POINT ( 'NONE',  ( -16.52544592524342804, 4.483927247898546575, 116.0405762719810383 ) ) ;
#13787=CARTESIAN_POINT ( 'NONE',  ( -21.55341960407610458, -5.719274019375992779, 56.45724293864768839 ) ) ;
#13789=CARTESIAN_POINT ( 'NONE',  ( 14.29746914071037800, 8.314922557961029526, 46.66775706135234714 ) ) ;
#13790=CARTESIAN_POINT ( 'NONE',  ( 5.719274019375673035, 21.55341960407619339, 102.2927570613523613 ) ) ;
#13791=CARTESIAN_POINT ( 'NONE',  ( -13.97604488694527625, -13.89961937509977652, 41.87390960531435979 ) ) ;
#13793=CARTESIAN_POINT ( 'NONE',  ( 16.55341960407618274, -4.379528057220086978, 106.0427570613523471 ) ) ;
#13794=CARTESIAN_POINT ( 'NONE',  ( -14.34966873604960291, -8.224510206698953496, 56.66557627198103830 ) ) ;
#13795=CARTESIAN_POINT ( 'NONE',  ( -13.89961937509977652, 13.97604488694528158, 70.62390960531432427 ) ) ;
#13796=CARTESIAN_POINT ( 'NONE',  ( 18.62759615963255655, 10.81492255796105972, 106.6677570613523756 ) ) ;
#13797=CARTESIAN_POINT ( 'NONE',  ( -18.67979575497193778, 10.72451020669871902, 28.33442372801902209 ) ) ;
#13798=CARTESIAN_POINT ( 'NONE',  ( 15.72974639402176855, 15.80617190586768217, 86.87609039468568994 ) ) ;
#13799=CARTESIAN_POINT ( 'NONE',  ( 14.29746914071037800, 8.314922557961029526, 46.66775706135234714 ) ) ;
#13800=CARTESIAN_POINT ( 'NONE',  ( 12.14591786802327356, -12.06949235617739191, 25.62609039468567929 ) ) ;
#13801=CARTESIAN_POINT ( 'NONE',  ( -4.379528057220328563, 16.55341960407611168, 75.20724293864769550 ) ) ;
#13802=CARTESIAN_POINT ( 'NONE',  ( -15.72974639402176322, -15.80617190586768395, 94.37609039468568994 ) ) ;
#13803=CARTESIAN_POINT ( 'NONE',  ( -12.06949235617756955, 12.14591786802309770, 30.62390960531436335 ) ) ;
#13804=CARTESIAN_POINT ( 'NONE',  ( 0.05219959533909260263, 19.03943276465977164, 29.99890960531435979 ) ) ;
#13805=CARTESIAN_POINT ( 'NONE',  ( -12.14591786802326823, 12.06949235617739902, 43.12609039468568284 ) ) ;
#13806=CARTESIAN_POINT ( 'NONE',  ( 14.34966873604960469, 8.224510206698951720, 59.16557627198103120 ) ) ;
#13807=CARTESIAN_POINT ( 'NONE',  ( 14.34966873604972726, -8.224510206698740333, 85.83442372801901854 ) ) ;
#13808=CARTESIAN_POINT ( 'NONE',  ( 19.03943276465977164, -0.05219959533909143690, 93.74890960531435269 ) ) ;
#13809=CARTESIAN_POINT ( 'NONE',  ( 13.89961937509977652, -13.97604488694527269, 108.1239096053143669 ) ) ;
#13810=CARTESIAN_POINT ( 'NONE',  ( -10.81492255796105439, 18.62759615963255655, 107.9177570613523471 ) ) ;
#13811=CARTESIAN_POINT ( 'NONE',  ( 12.06949235617757843, -12.14591786802309237, 83.12390960531436690 ) ) ;
#13812=CARTESIAN_POINT ( 'NONE',  ( 13.97604488694527802, 13.89961937509977652, 94.37390960531436690 ) ) ;
#13814=CARTESIAN_POINT ( 'NONE',  ( 12.06949235617739724, 12.14591786802326823, 46.87609039468568994 ) ) ;
#13815=CARTESIAN_POINT ( 'NONE',  ( 19.05341960407611168, 5.049401038298154454, 38.95724293864767418 ) ) ;
#13816=CARTESIAN_POINT ( 'NONE',  ( -9.474510206698964154, 16.51473224551069663, 105.4155762719810383 ) ) ;
#13817=CARTESIAN_POINT ( 'NONE',  ( 16.55341960407618274, -4.379528057220086978, 41.04275706135236135 ) ) ;
#13818=CARTESIAN_POINT ( 'NONE',  ( -30.00000000000000000, -1.132798289211302014E-14, 92.50000000000000000 ) ) ;
#13819=CARTESIAN_POINT ( 'NONE',  ( -19.03943276465977164, -0.05219959533935918106, 38.75109039468566152 ) ) ;
#13820=CARTESIAN_POINT ( 'NONE',  ( -5.153800228976328057, -19.02544592524343514, 47.29057627198102409 ) ) ;
#13821=CARTESIAN_POINT ( 'NONE',  ( -16.52544592524335698, -4.483927247898792601, 83.95942372801900433 ) ) ;
#13822=CARTESIAN_POINT ( 'NONE',  ( 16.46253265017146816, 9.564922557961045513, 81.66775706135233293 ) ) ;
#13823=CARTESIAN_POINT ( 'NONE',  ( -19.05341960407617563, 5.049401038297882671, 23.54275706135233648 ) ) ;
#13824=CARTESIAN_POINT ( 'NONE',  ( 19.02544592524343514, -5.153800228976328945, 58.54057627198102409 ) ) ;
#13825=CARTESIAN_POINT ( 'NONE',  ( -0.05219959533910754901, -16.53943276465976808, 102.4989096053143811 ) ) ;
#13826=CARTESIAN_POINT ( 'NONE',  ( 9.564922557961047289, -16.46253265017146816, 65.41775706135233293 ) ) ;
#13827=CARTESIAN_POINT ( 'NONE',  ( 18.62759615963271287, -10.81492255796078972, 63.33224293864770260 ) ) ;
#13828=CARTESIAN_POINT ( 'NONE',  ( 5.049401038297881783, 19.05341960407617563, 22.29275706135233648 ) ) ;
#13829=CARTESIAN_POINT ( 'NONE',  ( 9.564922557960805705, 16.46253265017160317, 109.5822429386476955 ) ) ;
#13830=CARTESIAN_POINT ( 'NONE',  ( 21.52544592524344225, -5.823673210054117533, 78.54057627198103830 ) ) ;
#13831=CARTESIAN_POINT ( 'NONE',  ( -0.05219959533909027116, -19.03943276465977164, 107.4989096053143527 ) ) ;
#13832=CARTESIAN_POINT ( 'NONE',  ( 13.97604488694548053, -13.89961937509957401, 100.6260903946856615 ) ) ;
#13833=CARTESIAN_POINT ( 'NONE',  ( -30.00000000000000000, -1.163414459189985801E-14, 95.00000000000000000 ) ) ;
#13834=CARTESIAN_POINT ( 'NONE',  ( -12.14591786802326823, 12.06949235617739902, 28.12609039468568284 ) ) ;
#13835=CARTESIAN_POINT ( 'NONE',  ( -19.02544592524342804, 5.153800228976336051, 36.04057627198100988 ) ) ;
#13836=CARTESIAN_POINT ( 'NONE',  ( 13.97604488694527802, 13.89961937509977652, 94.37390960531436690 ) ) ;
#13837=CARTESIAN_POINT ( 'NONE',  ( -5.823673210054116645, -21.52544592524344225, 87.29057627198103830 ) ) ;
#13838=CARTESIAN_POINT ( 'NONE',  ( -10.81492255796105439, 18.62759615963255655, 62.91775706135236135 ) ) ;
#13839=CARTESIAN_POINT ( 'NONE',  ( 19.03943276465977164, 0.05219959533936151252, 106.2510903946856615 ) ) ;
#13840=CARTESIAN_POINT ( 'NONE',  ( 13.89961937509957401, 13.97604488694547697, 21.87609039468566152 ) ) ;
#13841=CARTESIAN_POINT ( 'NONE',  ( 16.52544592524335698, 4.483927247898782831, 111.4594237280190328 ) ) ;
#13842=CARTESIAN_POINT ( 'NONE',  ( -21.53943276465977519, 0.05219959533907696930, 96.24890960531435269 ) ) ;
#13843=CARTESIAN_POINT ( 'NONE',  ( -4.379528057220328563, 16.55341960407611168, 40.20724293864769550 ) ) ;
#13844=CARTESIAN_POINT ( 'NONE',  ( -19.02544592524334988, -5.153800228976617603, 88.95942372801897591 ) ) ;
#13845=CARTESIAN_POINT ( 'NONE',  ( 0.05219959533936267826, -19.03943276465977164, 55.00109039468566863 ) ) ;
#13846=CARTESIAN_POINT ( 'NONE',  ( 0.05219959533937995610, -21.53943276465977519, 55.00109039468568284 ) ) ;
#13847=CARTESIAN_POINT ( 'NONE',  ( -13.97604488694547697, 13.89961937509957934, 38.12609039468566152 ) ) ;
#13848=CARTESIAN_POINT ( 'NONE',  ( 16.55341960407611168, 4.379528057220329451, 108.9572429386476955 ) ) ;
#13849=CARTESIAN_POINT ( 'NONE',  ( 5.823673210054125526, 21.52544592524343514, 29.79057627198102409 ) ) ;
#13850=CARTESIAN_POINT ( 'NONE',  ( -14.34966873604960291, -8.224510206698953496, 41.66557627198103120 ) ) ;
#13851=CARTESIAN_POINT ( 'NONE',  ( -15.80617190586768217, 15.72974639402176855, 93.12609039468568994 ) ) ;
#13852=CARTESIAN_POINT ( 'NONE',  ( -4.379528057220086978, -16.55341960407618274, 69.79275706135234714 ) ) ;
#13853=CARTESIAN_POINT ( 'NONE',  ( 8.314922557960818139, 14.29746914071049879, 29.58224293864769905 ) ) ;
#13854=CARTESIAN_POINT ( 'NONE',  ( 10.72451020669871369, 18.67979575497193778, 67.08442372801901854 ) ) ;
#13855=CARTESIAN_POINT ( 'NONE',  ( -21.53943276465977519, -0.05219959533937600094, 73.75109039468567573 ) ) ;
#13856=CARTESIAN_POINT ( 'NONE',  ( 10.81492255796078972, 18.62759615963270932, 74.58224293864768129 ) ) ;
#13858=CARTESIAN_POINT ( 'NONE',  ( -13.97604488694527625, -13.89961937509977652, 21.87390960531435979 ) ) ;
#13859=CARTESIAN_POINT ( 'NONE',  ( -18.67979575497193778, 10.72451020669871902, 43.33442372801901143 ) ) ;
#13860=CARTESIAN_POINT ( 'NONE',  ( 19.02544592524343514, -5.153800228976328945, 23.54057627198102054 ) ) ;
#13861=CARTESIAN_POINT ( 'NONE',  ( -19.02544592524342804, 5.153800228976336051, 36.04057627198100988 ) ) ;
#13862=CARTESIAN_POINT ( 'NONE',  ( 8.224510206698953496, -14.34966873604960469, 72.91557627198103830 ) ) ;
#13863=CARTESIAN_POINT ( 'NONE',  ( -13.97604488694527625, -13.89961937509977652, 81.87390960531436690 ) ) ;
#13864=CARTESIAN_POINT ( 'NONE',  ( 14.29746914071049879, -8.314922557960816363, 33.33224293864769550 ) ) ;
#13865=CARTESIAN_POINT ( 'NONE',  ( -0.05219959533907301413, -21.53943276465977519, 72.49890960531435269 ) ) ;
#13866=CARTESIAN_POINT ( 'NONE',  ( 10.72451020669898902, -18.67979575497178502, 107.9155762719810241 ) ) ;
#13867=FACE_OUTER_BOUND ( 'NONE', #37797, .T. ) ;
#13868=CARTESIAN_POINT ( 'NONE',  ( -19.03943276465977164, 0.05219959533909376836, 66.24890960531436690 ) ) ;
#13869=CARTESIAN_POINT ( 'NONE',  ( -19.03943276465977164, -0.05219959533935918106, 108.7510903946856615 ) ) ;
#13870=CARTESIAN_POINT ( 'NONE',  ( -15.80617190586745835, -15.72974639402198527, 61.87390960531436690 ) ) ;
#13871=CARTESIAN_POINT ( 'NONE',  ( -10.81492255796105439, 18.62759615963255655, 77.91775706135231871 ) ) ;
#13872=CARTESIAN_POINT ( 'NONE',  ( -19.02544592524342804, 5.153800228976336051, 61.04057627198103120 ) ) ;
#13874=CARTESIAN_POINT ( 'NONE',  ( 13.89961937509977652, -13.97604488694527269, 93.12390960531436690 ) ) ;
#13875=CARTESIAN_POINT ( 'NONE',  ( 14.34966873604972726, -8.224510206698740333, 70.83442372801901854 ) ) ;
#13876=CARTESIAN_POINT ( 'NONE',  ( 21.53943276465977519, 0.05219959533937863772, 61.25109039468567573 ) ) ;
#13877=CARTESIAN_POINT ( 'NONE',  ( -15.72974639402176322, -15.80617190586768395, 84.37609039468570415 ) ) ;
#13878=CARTESIAN_POINT ( 'NONE',  ( -0.05219959533907301413, -21.53943276465977519, 112.4989096053143669 ) ) ;
#13879=CARTESIAN_POINT ( 'NONE',  ( 10.81492255796078972, 18.62759615963270932, 79.58224293864769550 ) ) ;
#13880=CARTESIAN_POINT ( 'NONE',  ( 19.03943276465977164, 0.05219959533936151252, 41.25109039468566152 ) ) ;
#13881=CARTESIAN_POINT ( 'NONE',  ( -21.52544592524343514, 5.823673210054127303, 41.04057627198103120 ) ) ;
#13882=CARTESIAN_POINT ( 'NONE',  ( 5.049401038298161559, -19.05341960407611168, 87.70724293864769550 ) ) ;
#13883=CARTESIAN_POINT ( 'NONE',  ( -12.06949235617756955, 12.14591786802309770, 30.62390960531436335 ) ) ;
#13884=LINE ( 'NONE', #197916, #17547 ) ;
#13887=CARTESIAN_POINT ( 'NONE',  ( -5.153800228976607833, 19.02544592524334988, 92.70942372801901854 ) ) ;
#13888=CARTESIAN_POINT ( 'NONE',  ( 15.80617190586746368, 15.72974639402197994, 69.37390960531436690 ) ) ;
#13889=CARTESIAN_POINT ( 'NONE',  ( -16.55341960407611168, -4.379528057220339221, 56.45724293864768839 ) ) ;
#13890=CARTESIAN_POINT ( 'NONE',  ( 4.483927247898790824, -16.52544592524335698, 30.20942372801902565 ) ) ;
#13891=CARTESIAN_POINT ( 'NONE',  ( 9.474510206698971260, -16.51473224551069308, 42.91557627198103120 ) ) ;
#13892=CARTESIAN_POINT ( 'NONE',  ( 21.55341960407610458, 5.719274019375980345, 103.9572429386476813 ) ) ;
#13893=CARTESIAN_POINT ( 'NONE',  ( 19.03943276465977164, 0.05219959533936151252, 66.25109039468567573 ) ) ;
#13894=CARTESIAN_POINT ( 'NONE',  ( -0.05219959533909027116, -19.03943276465977164, 87.49890960531436690 ) ) ;
#13895=CARTESIAN_POINT ( 'NONE',  ( 4.483927247898545687, 16.52544592524342804, 84.79057627198102409 ) ) ;
#13896=( BOUNDED_SURFACE ( )  B_SPLINE_SURFACE ( 3, 2, ( 
 ( #146460, #53463, #10972, #101973, #24147, #177830, #72645, #117135, #42310, #11983, #163654, #25156, #38303, #147485, #192991, #54469, #88795, #87791, #196006, #9976, #7953, #57479, #86798, #41308, #8975, #70644, #116139, #115139, #56470, #119151, #27148, #85799, #148485, #71636, #133303, #132310, #130282, #194993, #23137, #194002, #55465, #118148, #176831, #179838, #149476, #134320, #180833, #26149, #69636, #150488, #165650, #161643, #84782, #131302, #39299, #100956, #76604, #90770, #77598, #47275, #151476, #61428, #108932, #105950, #74630, #91751, #107926, #12966, #199963, #169611, #31109, #137285, #197972, #104964, #135319, #106938, #183798, #46271, #154445, #167635, #166651, #92757, #45285, #139269, #30111, #184785, #15939, #745, #62417, #58458, #182809, #28152, #138281, #168611, #89792, #170612, #153446, #136296, #60434, #29132, #59442, #124089, #120126, #185788, #44292, #32102, #198967, #121115, #123099, #152454, #13939, #93759, #155440, #75606, #122108, #14944, #73648, #196992, #181817, #43296, #35072, #64422, #4715, #174595, #140257, #19904, #81546, #65407, #127068, #156433, #33096, #3730, #1749, #95746, #188776, #189768, #144235, #67397, #96727, #190754, #51240, #36060, #112901, #82553, #97709, #187787, #2745, #18925, #126091, #50259, #111915, #159400, #125102, #49257, #157431, #109926, #173603, #158415, #143232, #186800, #20895, #66404, #5719, #142245, #128066, #52228, #129053, #78583, #113884, #175582, #63427, #48271, #110915, #80570, #37059, #98718, #17933, #94752, #16930, #171608, #79587, #141256, #172601, #34087, #132073, #24917, #9740, #41073, #146225, #192753, #117912, #130042, #131064, #180602, #102736, #39065, #164425, #85559, #40055, #6712, #68390, #118918, #84547, #7712, #191741, #87562, #83551, #177597, #86563, #69396, #176595, #163420, #99725, #54236, #133068, #10740, #53225, #115907, #38069, #161409, #21901, #194758, #162403, #178592, #100722, #148246, #179601, #145230, #71404, #56230, #8736, #70405, #22901, #23905, #147244, #114901, #193762, #55230, #25918, #149249, #72404, #101732, #134081, #195770, #57244, #42076, #160412, #116899, #74398, #89557, #105716, #12732, #13705, #137042, #138041, #11749, #136063, #182573, #196763, #198733, #60199, #121869, #73416, #199722, #168379, #46028, #28899, #90539, #139024, #45047, #165420, #29874, #504, #26914, #135087, #197738, #167403, #123840, #152221, #43062, #119899, #75372, #88556, #61188, #76364, #58230, #122860, #183561, #91511, #153198, #184548, #151243, #59204, #107684, #181584, #120873, #185538, #169361, #44056, #30871, #106705, #14702, #150255, #104728, #62176, #27914, #92517, #166420, #154207, #15696, #77357, #103740, #32854, #157185, #112657, #3486, #158171, #189523, #127818, #81304, #31859, #156186, #78337, #111670, #18679, #140011, #143990, #126822, #48028, #33839, #141013, #109685, #35818, #93512, #174348, #17685, #50996, #172350, #95499, #80325, #82299, #188528, #108689, #173358, #5471, #170367, #16687, #79343, #110670, #67153, #49015, #186556, #63177, #141998, #155198, #142988, #19663, #1499, #4466, #65163, #34828, #96483, #97464, #94504, #2500, #66155, #124856, #64181, #128811, #159150, #125847, #20646, #50005, #47031, #171366, #187548, #149004, #114648, #37818, #98469, #117660, #113642, #7464, #54986, #176346, #100481, #55983, #146996, #101474, #132824, #71158, #24667, #175337, #99479, #21654, #116655, #162160, #83307, #87320, #70158, #191493, #177353, #84303, #52971, #179357, #36804, #40820, #161160, #194510, #115663, #6464, #193509, #129796, #22656, #163164, #102490, #144984, #145982, #68145, #69148, #51984, #86317, #192506, #8483, #130815, #178346, #148005, #160163, #39808, #9495, #38823, #23656, #53990, #85304, #131828, #164177, #25675, #10493, #72153, #190510, #184307, #13465, #107440, #106454, #91261, #29629, #199475, #168133, #104486, #119662, #135828, #42823, #43809, #167158, #152952, #41827, #166170 ),
 ( #151004, #137791, #169112, #11501, #121622, #30619, #27671, #134842, #151977, #14451, #73172, #59955, #76114, #60942, #197498, #57991, #165172, #195520, #28658, #105472, #122617, #45788, #89311, #26665, #92272, #12495, #75129, #88307, #90293, #136798, #198483, #153956, #74157, #120633, #44799, #15452, #183317, #133829, #118667, #56993, #182330, #180358, #149995, #103494, #196521, #181344, #58965, #96247, #34590, #158914, #18440, #77110, #138780, #33596, #3251, #171117, #154949, #80091, #141759, #174111, #64924, #126584, #16445, #173114, #97227, #124608, #261, #65911, #123598, #46784, #157935, #93263, #61929, #19426, #125605, #32607, #186303, #81073, #63936, #189284, #185292, #187303, #48774, #108443, #94260, #139763, #1249, #35581, #142752, #4232, #156943, #78094, #127584, #110429, #188286, #155940, #17436, #62928, #170119, #49761, #50762, #31613, #79092, #172110, #95260, #111428, #109435, #47783, #112419, #140765, #2254, #22416, #84066, #143748, #52735, #178105, #101232, #9254, #69919, #98219, #179116, #86077, #37573, #40584, #116415, #54743, #145745, #144743, #51744, #82053, #53750, #130571, #193269, #162920, #114402, #113405, #39573, #191260, #100240, #175096, #192268, #115424, #177113, #24429, #99236, #7226, #131585, #147768, #38584, #102254, #5227, #161922, #68911, #66909, #36564, #70921, #23416, #128572, #67909, #132588, #194277, #20405, #85064, #190267, #159922, #146746, #8241, #176103, #21411, #55744, #117418, #83068, #6230, #129562, #160923, #59720, #184069, #11259, #45552, #152721, #10254, #133585, #44566, #180123, #87080, #106221, #12260, #57756, #72932, #167905, #150763, #75880, #163942, #73923, #135593, #71913, #181110, #26430, #88070, #122380, #121391, #29405, #43574, #41591, #91035, #197265, #74902, #42584, #104247, #149756, #25439, #90064, #14212, #60704, #119426, #58727, #120396, #182090, #196287, #148765, #105238, #56758, #165930, #27427, #89072, #195275, #166926, #183083, #137556, #199239, #13239, #103255, #118430, #164937, #28427, #134601, #151746, #136565, #198246, #110198, #124372, #111189, #80846, #185058, #95024, #142523, #139533, #108207, #125378, #141533, #46546, #33366, #18206, #3022, #63703, #65680, #92028, #17202, #155707, #168877, #61696, #79864, #78856, #30382, #154718, #126360, #64698, #189056, #48544, #107207, #153719, #187075, #156714, #1016, #169887, #171877, #188056, #4001, #49526, #172880, #31380, #34360, #127343, #16211, #15215, #96021, #76874, #138544, #157707, #123365, #22, #19197, #140536, #62690, #77866, #93030, #94027, #186067, #47550, #2024, #109203, #170883, #32374, #113173, #174862, #9016, #7992, #116179, #130321, #66676, #177870, #22174, #161682, #129330, #67672, #36329, #112191, #176872, #39338, #147528, #144508, #98993, #6986, #68666, #82827, #132350, #192018, #143505, #5993, #52500, #114160, #173880, #191025, #69675, #131342, #100997, #99997, #128338, #70684, #162682, #175862, #50529, #37335, #193030, #35350, #53502, #160682, #54507, #24188, #190037, #38341, #85838, #83824, #51511, #115179, #84822, #97982, #23179, #146501, #97001, #145505, #159676, #81818, #158683, #20172, #4991, #21172, #77389, #26189, #25197, #169396, #164694, #76396, #86840, #106736, #29905, #91543, #30903, #75404, #183594, #133342, #10016, #45078, #178871, #137076, #168411, #92550, #123874, #47065, #138072, #170402, #154239, #15729, #139058, #62209, #537, #87829, #179879, #198765, #185572, #60231, #108725, #153232, #149515, #41347, #31893, #14735, #93547, #78371, #199753, #61220, #102013, #11012, #56510, #118188, #155232, #16722, #194042, #122891, #71675, #55506, #184579, #107715, #121900, #46061, #103010, #117176, #40338, #163695, #148525, #195033, #188566, #96520, #158210, #172388, #21692, #19700, #32890, #33878, #142037, #3525, #63213, #95537, #97502, #20683, #128848, #189561, #17722, #98507, #5510, #157225, #160202, #126860, #82338, #140045, #143026, #18717 ),
 ( #171403, #4503, #50046, #94541, #36842, #81342, #141051, #111709, #80364, #2537, #190548, #186592, #67191, #49052, #144028, #65201, #156222, #66194, #79381, #187584, #112695, #52021, #64218, #125884, #110707, #173395, #1536, #174386, #34866, #127857, #51033, #35856, #159188, #124893, #113680, #175374, #48064, #109720, #149043, #100519, #41868, #70199, #164215, #103534, #86356, #162198, #87357, #57033, #161200, #71197, #118706, #115702, #84342, #101513, #117698, #22695, #9531, #179395, #40858, #147037, #7504, #114690, #145022, #116694, #193550, #56020, #25712, #177391, #176385, #102532, #54029, #163203, #37859, #55023, #178383, #39847, #10531, #23696, #131866, #194550, #72195, #24707, #165209, #68183, #148042, #132861, #6503, #99518, #133868, #195559, #129835, #130854, #180397, #83346, #191534, #53011, #146021, #69188, #192546, #38863, #85344, #8521, #29666, #168169, #123633, #14488, #76150, #104524, #122654, #46819, #74194, #108479, #15490, #73210, #134881, #61966, #107475, #90329, #169153, #75165, #120668, #135863, #30656, #13500, #138818, #26704, #136837, #198520, #196557, #43844, #89349, #151039, #185329, #184342, #92310, #106492, #42859, #153993, #59991, #137829, #105510, #167196, #12529, #88344, #152989, #77147, #150036, #182366, #121659, #183354, #44836, #59002, #11542, #91298, #119698, #28693, #152014, #199512, #58028, #60979, #45824, #298, #181381, #166205, #27707, #197534, #95293, #156977, #5262, #111463, #31650, #96282, #66944, #93299, #139798, #140801, #33631, #190299, #172145, #109470, #186339, #141793, #154985, #65946, #142785, #1287, #4266, #3287, #34623, #19461, #50794, #155975, #2290, #127618, #62963, #63972, #51776, #112453, #48809, #174142, #18474, #49798, #16481, #78130, #128606, #94297, #17472, #124644, #97259, #47821, #187339, #157968, #79128, #80124, #35614, #126617, #81107, #158947, #20436, #189317, #171154, #125642, #32642, #82087, #64958, #110463, #170157, #173148, #188319, #143780, #7258, #114436, #102287, #159954, #40617, #22449, #194311, #38618, #129595, #116453, #52767, #160956, #86112, #163976, #6262, #99269, #191291, #176137, #175129, #147803, #115456, #131619, #84098, #101266, #70953, #36596, #178141, #39607, #161954, #23450, #37606, #145777, #100275, #98252, #192302, #85097, #9288, #25473, #87113, #193303, #148799, #132623, #55777, #117450, #179149, #10289, #68943, #130607, #177146, #146783, #162956, #71947, #133618, #21442, #53781, #8276, #67942, #69954, #54778, #24462, #83103, #195311, #113436, #144779, #60741, #30417, #134635, #44599, #92065, #89107, #57789, #74934, #91068, #196320, #183116, #152754, #14244, #120429, #181143, #88105, #118464, #90096, #166958, #29436, #137590, #150797, #149790, #75916, #27465, #136597, #11294, #28460, #151778, #13271, #199273, #135626, #43606, #167937, #122415, #198277, #15248, #41625, #59754, #105271, #180156, #72966, #184105, #121424, #103289, #104281, #45587, #107240, #138578, #106254, #56792, #164969, #168911, #153753, #12293, #119459, #76907, #26462, #42617, #165963, #73958, #197297, #58760, #182120, #47583, #20206, #189092, #46580, #108241, #35384, #80881, #63737, #142558, #48579, #94062, #109235, #4036, #187109, #112225, #81852, #110232, #171913, #169921, #17238, #62724, #124408, #158716, #157743, #65714, #79897, #16248, #127380, #33402, #111226, #78890, #140569, #186101, #61731, #126394, #50565, #97035, #155741, #95060, #156750, #18244, #32407, #58, #141567, #93064, #2059, #125412, #3056, #123399, #64733, #19232, #173915, #185091, #49562, #77900, #31413, #154751, #188091, #139567, #172918, #1051, #170914, #34397, #96055, #145541, #82866, #159710, #115215, #5028, #39374, #116215, #113210, #177906, #176908, #8029, #193066, #24224, #129366, #175899, #101033, #174898, #114195, #163733, #85874, #22211, #147563, #68702, #23216, #190070, #51546, #102049, #67708, #191062, #36364, #70718, #66713, #160719, #69711, #52534 ),
 ( #40375, #84859, #144544, #130357, #37371, #6029, #132386, #98016, #194079, #99029, #9048, #192056, #21209, #146536, #83860, #7020, #162718, #55542, #53538, #38379, #100035, #161721, #128374, #117214, #131378, #54542, #178907, #25234, #143541, #10050, #89868, #151550, #135396, #197066, #26224, #103048, #73723, #71710, #165725, #58534, #59513, #14012, #137357, #166724, #60506, #121190, #44366, #182883, #152524, #106023, #57553, #72723, #88869, #150562, #13040, #45358, #167710, #195068, #119222, #27221, #179916, #181890, #43368, #105040, #56548, #29206, #74706, #90840, #12061, #120200, #122181, #28228, #148559, #136370, #183873, #133378, #118225, #180907, #198047, #107010, #41382, #75678, #168683, #164730, #87864, #42382, #199036, #86875, #149552, #11047, #134396, #196082, #104045, #126165, #2820, #200035, #64498, #1823, #94829, #79662, #110990, #16014, #62493, #187860, #61503, #819, #50333, #172675, #109007, #34160, #155511, #110000, #76677, #138353, #188849, #154517, #77671, #123172, #157506, #153519, #47352, #156507, #139340, #140333, #95821, #186876, #141332, #18999, #80646, #49329, #15016, #124164, #184860, #18008, #63504, #46343, #127142, #171680, #31181, #17006, #185865, #92832, #142322, #107999, #3802, #170686, #65480, #78658, #169686, #33170, #32175, #93831, #111990, #30183, #125180, #48346, #91826, #51313, #35147, #7789, #175657, #191818, #20966, #161486, #131139, #96801, #176670, #38146, #21975, #83627, #112974, #189840, #160485, #158489, #52300, #145304, #146301, #100792, #23977, #53298, #147319, #69473, #192827, #54308, #39137, #115980, #144305, #159471, #37131, #98791, #99800, #132143, #177669, #81619, #5795, #113958, #66478, #68466, #130120, #114977, #143302, #162475, #22974, #85632, #6787, #84622, #8808, #70477, #4788, #193836, #55300, #174666, #173680, #67468, #36132, #19976, #128140, #97783, #82623, #129127, #190825, #133138, #119967, #56302, #164494, #89627, #167475, #9812, #102809, #194829, #117984, #178663, #151315, #118989, #135158, #25987, #104801, #74470, #40126, #181653, #43132, #165489, #26985, #179674, #41145, #103809, #101804, #195841, #88630, #12804, #44130, #28970, #196831, #90612, #136136, #197811, #59277, #182646, #120947, #87630, #149316, #180673, #42149, #166490, #75445, #105789, #24990, #10810, #57314, #71473, #11821, #73486, #58300, #86634, #152293, #27988, #13778, #150326, #137120, #198806, #116972, #163491, #148317, #72480, #134153, #29948, #30944, #123915, #80403, #62246, #199796, #76438, #31932, #121944, #156260, #32927, #91587, #94582, #93586, #124932, #109756, #141089, #46102, #92591, #17763, #153277, #154280, #142075, #2576, #139101, #64256, #185614, #140085, #106777, #168452, #18756, #184620, #107757, #14778, #187621, #183637, #77430, #186629, #169441, #170441, #125923, #16761, #171440, #49091, #110748, #79419, #45119, #15770, #138115, #48100, #155272, #78409, #1577, #172429, #575, #47104, #33918, #95575, #63252, #60271, #61263, #157261, #108764, #122933, #34904, #86140, #146810, #65239, #66235, #70982, #9317, #10316, #116480, #3561, #126899, #178169, #147831, #100303, #143063, #162984, #24489, #188605, #132650, #194338, #4541, #55806, #50086, #177173, #111746, #148826, #158247, #19737, #173434, #25499, #54805, #87143, #39634, #8304, #161981, #96559, #117478, #81378, #127895, #179176, #40644, #38646, #102313, #69981, #131649, #192329, #53810, #115485, #23477, #101295, #85126, #193331, #164003, #62898, #1220, #46755, #45757, #113132, #114119, #83785, #78063, #32577, #143464, #4949, #16416, #68625, #66634, #77079, #139731, #186274, #47753, #107409, #124578, #144468, #67629, #175821, #36287, #61898, #145464, #52461, #109407, #6946, #171086, #129289, #184274, #189996, #94230, #190984, #160643, #123568, #174822, #22135, #155911, #185263, #128297, #21131, #108414, #97943, #82786, #5952, #20133, #170089, #15420, #169082, #81778, #51471, #159635, #37294 ),
 ( #30588, #98953, #92240, #153926, #138748, #230, #31583, #154918, #93233, #150706, #26372, #192208, #161865, #27368, #24370, #179055, #87022, #148708, #162862, #12205, #10196, #23359, #86021, #132531, #194220, #53690, #147710, #88012, #11198, #119369, #180065, #8181, #89015, #196231, #9197, #130512, #117359, #72874, #115368, #133525, #70863, #134542, #104190, #69857, #118371, #55685, #195217, #40524, #41533, #57700, #164877, #177057, #39514, #85004, #56698, #102195, #146685, #38527, #71856, #131525, #163883, #25380, #193210, #181052, #100183, #42527, #101174, #165872, #103197, #54684, #149700, #116357, #178046, #46482, #124308, #166869, #59658, #151692, #13182, #135538, #108142, #75820, #91965, #121332, #61637, #31318, #197209, #76815, #138486, #122319, #184011, #74845, #90008, #60645, #58672, #152663, #45493, #169826, #956, #186006, #153658, #47488, #92970, #154656, #16152, #139475, #77806, #44508, #183025, #137498, #199179, #200168, #32316, #62632, #182033, #106164, #14153, #28370, #168818, #30323, #15154, #109144, #120338, #170823, #167847, #93969, #107148, #136508, #123305, #198188, #29347, #155649, #73868, #90976, #184998, #43516, #105182, #78797, #51447, #19132, #35283, #64636, #4928, #174798, #140475, #20110, #81754, #65618, #127278, #156651, #33307, #3938, #1963, #95959, #188991, #189972, #144444, #67605, #96939, #190960, #113108, #36264, #97918, #82763, #159610, #187995, #2957, #80783, #142460, #143442, #175797, #21108, #125318, #49465, #157643, #110140, #112127, #173818, #158620, #187014, #5929, #66611, #129266, #50467, #128275, #52437, #114095, #63643, #37270, #98928, #48485, #171819, #111128, #17144, #94967, #126298, #18147, #79801, #141473, #172817, #34297, #133273, #130256, #194964, #132281, #25128, #9948, #41280, #146435, #192963, #118122, #191952, #131275, #180805, #102942, #39271, #164626, #85770, #40271, #6922, #68600, #119124, #84757, #7925, #53437, #87763, #83760, #177802, #86770, #69610, #70614, #24117, #163625, #193973, #71607, #26120, #56443, #145440, #54443, #115112, #148453, #55435, #176806, #57452, #101944, #161618, #147457, #116113, #23112, #22110, #100928, #179810, #149448, #42284, #10944, #160619, #38278, #117106, #72618, #162612, #99932, #134293, #195979, #8946, #178801, #153418, #181786, #199936, #124058, #151449, #185758, #92728, #150461, #11956, #139241, #184757, #167607, #46242, #152424, #197943, #12936, #107896, #90741, #15911, #103942, #13912, #75578, #73621, #121087, #166622, #28124, #62388, #61399, #169583, #183771, #120098, #31081, #137255, #14916, #182781, #44264, #165622, #123071, #27121, #135291, #716, #59412, #198940, #60407, #122080, #136268, #88768, #45257, #196963, #105922, #29102, #106911, #58431, #168584, #154417, #77569, #43267, #76577, #104936, #89764, #74601, #30082, #91723, #138253, #128037, #67368, #50232, #64396, #51212, #20867, #125074, #35045, #126064, #96699, #173576, #2719, #81517, #186771, #158388, #143204, #4685, #110889, #171580, #78553, #108904, #80544, #157405, #19877, #189739, #79560, #140228, #66377, #17905, #127040, #1721, #18898, #142218, #3701, #112873, #187761, #34060, #174565, #36032, #65380, #5692, #32074, #188747, #95718, #170583, #63397, #97681, #111886, #159370, #16902, #141228, #129027, #82524, #49231, #144206, #172574, #47246, #93730, #155412, #48241, #33068, #94723, #109896, #156401, #113859, #7684, #55203, #176568, #100695, #54210, #193735, #162376, #101701, #71379, #24888, #175555, #99699, #21875, #116872, #23878, #83525, #87537, #70378, #191714, #177571, #84521, #53198, #179576, #37030, #117885, #161383, #133043, #115881, #6686, #178563, #130015, #38043, #163391, #41046, #145203, #22874, #68364, #114873, #52201, #86537, #192726, #8708, #146198, #40028, #148221, #98691, #9715, #194733, #39038, #85529, #69368, #131037, #147217, #160385, #132046, #56203, #102711, #164400, #25892, #149224, #10715, #72378, #190728 ),
 ( #26888, #28873, #90514, #152196, #103715, #168353, #198706, #76337, #59179, #120848, #169335, #75347, #195744, #60173, #30843, #57218, #165395, #104704, #197714, #154179, #119875, #92490, #29849, #45020, #118892, #91486, #106680, #88531, #153173, #105690, #121842, #183536, #14675, #181560, #166393, #150227, #138013, #44029, #11723, #15670, #13680, #135063, #182547, #27889, #196739, #122834, #180577, #61162, #43038, #199697, #167377, #73391, #137016, #58206, #89531, #184523, #46003, #151219, #12708, #74374, #136039, #42051, #107658, #134052, #98185, #127553, #67876, #37539, #476, #83036, #144711, #128538, #190233, #19396, #93483, #66876, #62150, #158882, #51711, #52704, #7193, #130536, #159889, #53715, #114367, #99203, #176072, #145711, #160891, #50730, #65879, #82019, #143715, #6196, #38551, #22383, #185512, #112388, #20371, #170340, #175065, #36531, #21377, #47003, #84033, #129530, #68877, #5194, #113374, #115392, #191230, #138997, #192234, #177080, #123814, #108662, #174080, #100208, #161888, #189254, #77329, #31833, #155170, #81045, #142721, #4201, #35549, #97196, #195240, #88035, #72898, #104214, #9221, #55711, #181076, #193236, #194244, #43539, #165895, #102220, #27392, #148732, #103220, #69882, #131551, #182056, #147734, #70888, #54709, #150728, #146710, #40551, #149723, #132556, #133550, #87047, #26396, #56724, #134566, #89038, #57723, #8207, #117383, #119393, #116381, #179080, #163909, #178071, #118395, #180089, #41557, #39538, #42551, #11223, #12227, #10220, #71880, #58693, #164902, #85030, #196254, #120363, #101196, #162887, #25405, #73890, #105205, #135560, #23383, #197232, #24396, #86045, #62656, #139498, #136531, #980, #138510, #31344, #16176, #47513, #152687, #199204, #124335, #198212, #137522, #187040, #109169, #45517, #170848, #91990, #46510, #13206, #74869, #125342, #91001, #14176, #59684, #93992, #90030, #184035, #92995, #75846, #76839, #30348, #169850, #159881, #77831, #32339, #186031, #151713, #60671, #121355, #154681, #61661, #183048, #63668, #108169, #167870, #153684, #122346, #29370, #155673, #44532, #17168, #107172, #78821, #15180, #106187, #140500, #168843, #123329, #1989, #48510, #185023, #166892, #28392, #188020, #171843, #144471, #112154, #128300, #157670, #97946, #67632, #33331, #113136, #174826, #158644, #20136, #49492, #126323, #96964, #94991, #189017, #81781, #82789, #37297, #160646, #189999, #83788, #5955, #129292, #190988, #175824, #52464, #80807, #95985, #173844, #35310, #36290, #68629, #143468, #21134, #50491, #127306, #130285, #114122, #156676, #141498, #6949, #3964, #4952, #66637, #51474, #142486, #191979, #159638, #2982, #65644, #98956, #22138, #18171, #145467, #110164, #79828, #64661, #111154, #172843, #34323, #19159, #70648, #11987, #40302, #134323, #73651, #56473, #132314, #57484, #27151, #131306, #41313, #194006, #102973, #179842, #8980, #87795, #192996, #164658, #149480, #10976, #117139, #177834, #84786, #115143, #86803, #163658, #26153, #196009, #85803, #146465, #72649, #24152, #133307, #7957, #25161, #148489, #9980, #119154, #55469, #101978, #180836, #42313, #71640, #135323, #38307, #194996, #118152, #176836, #69640, #103974, #165653, #99962, #100960, #88798, #150491, #53466, #161646, #23141, #54473, #116143, #39302, #147489, #162645, #178833, #138284, #93762, #184787, #46273, #74634, #92760, #16933, #44295, #78586, #185791, #43299, #104967, #32105, #77601, #60436, #139272, #45287, #90772, #105954, #748, #183800, #108935, #196995, #106940, #168613, #166654, #13942, #59445, #121118, #155443, #154449, #62420, #76606, #12970, #124092, #30113, #91754, #169615, #47279, #29135, #28155, #31112, #167638, #199965, #89796, #153448, #14946, #61430, #15942, #75608, #123101, #107929, #170616, #58462, #120129, #181820, #151479, #136300, #197975, #182812, #152456, #137287, #198969, #122111, #159403, #97712, #21905, #81549, #140260, #1752, #96730, #66407, #34090 ),
 ( #126094, #142248, #3733, #128069, #98722, #174598, #48274, #172604, #18929, #33099, #35076, #158419, #19907, #109929, #36064, #4718, #82556, #65410, #127071, #175587, #143235, #63430, #189771, #37063, #125106, #171611, #110918, #188779, #160416, #187791, #186804, #20898, #51244, #94755, #144238, #112904, #156436, #5722, #111918, #67400, #129056, #190757, #49260, #95749, #52232, #17936, #157434, #79590, #113889, #80574, #141259, #50262, #2749, #64425, #173606, #42080, #7716, #131068, #191746, #10744, #6716, #100726, #148250, #69401, #193766, #147249, #86567, #55234, #194762, #164429, #117916, #68394, #192757, #114905, #9744, #116903, #176599, #180607, #53229, #162407, #146229, #54240, #103744, #41077, #149253, #163424, #99729, #72408, #178596, #56234, #23909, #85563, #165424, #179605, #145234, #38073, #83555, #177601, #132077, #40059, #101736, #115911, #130046, #24922, #161413, #39069, #8740, #70409, #22905, #71408, #102741, #25922, #134085, #133072, #84551, #87566, #195775, #57248, #118922, #13711, #107689, #47037, #29879, #44061, #30876, #509, #104732, #14708, #105721, #76369, #153203, #182578, #61193, #166424, #138046, #122865, #184553, #90544, #151248, #58235, #88560, #60204, #137047, #199727, #169367, #59209, #119903, #46034, #152226, #196767, #120878, #167408, #43066, #91517, #27919, #74403, #92522, #77362, #181588, #12737, #89562, #136069, #150259, #154212, #28904, #45052, #197743, #15701, #139030, #11753, #62181, #123845, #75377, #198739, #121874, #183567, #106710, #73420, #168384, #185543, #108694, #26918, #135091, #50011, #143995, #142993, #127823, #66161, #35824, #4471, #141019, #156191, #172355, #33844, #96488, #128816, #189529, #78342, #2506, #49020, #63182, #65168, #126827, #188533, #140016, #111676, #173363, #64186, #51989, #34833, #124862, #125852, #95504, #157190, #93517, #187553, #51001, #112662, #159155, #19668, #48033, #190515, #97470, #110675, #170372, #18684, #174354, #31864, #158178, #80331, #20651, #5476, #109690, #81309, #142003, #82305, #67159, #3491, #155203, #171371, #16692, #1504, #186561, #32859, #94509, #17690, #79348, #147003, #23663, #86324, #194516, #145988, #144989, #148011, #69155, #36809, #68151, #164183, #8489, #70165, #9501, #192512, #100487, #24674, #71165, #131834, #72161, #98476, #85312, #162166, #175342, #129802, #132830, #193516, #160169, #161166, #55990, #117667, #195527, #54992, #113648, #21659, #116661, #39815, #7471, #191501, #178352, #101481, #10500, #163170, #179363, #52977, #40826, #133836, #22662, #83312, #102498, #6470, #114655, #149011, #25681, #177359, #87326, #176352, #130821, #84309, #37825, #99485, #53996, #115670, #38829, #43817, #165179, #74165, #119670, #181352, #15462, #14459, #122625, #136807, #73180, #184315, #28666, #168141, #135837, #197506, #77118, #152961, #118675, #88315, #153964, #151012, #105480, #58973, #138788, #167167, #137800, #57000, #59964, #120641, #60950, #30627, #134851, #44807, #182339, #106462, #183326, #12503, #91270, #196529, #29637, #76122, #199484, #90301, #42831, #150003, #180366, #151986, #13474, #45796, #107448, #89319, #11509, #169122, #75138, #41834, #58000, #92280, #198491, #121630, #103502, #26674, #104496, #166178, #27679, #156950, #158921, #185301, #110437, #48783, #61937, #154957, #173122, #172118, #123606, #47792, #19433, #157942, #82061, #141766, #269, #46792, #18447, #126591, #94269, #78102, #3258, #64932, #97234, #188293, #49770, #139771, #96255, #20411, #109443, #108451, #189291, #170127, #31622, #35588, #81080, #63945, #142759, #33604, #155947, #171126, #4239, #187312, #112427, #93272, #95267, #80098, #16453, #17444, #62936, #124616, #1259, #65919, #127592, #111435, #186311, #50768, #34597, #174117, #79100, #140773, #32615, #2262, #125613, #175102, #40591, #37580, #192274, #100248, #161929, #176110, #25447, #23424, #36570, #99243, #145751, #7233, #66916, #160931, #101240, #24436, #132595 ) ),
 .UNSPECIFIED., .T., .F., .T. ) 
 B_SPLINE_SURFACE_WITH_KNOTS ( ( 4, 3, 4 ),
 ( 3, 2, 2, 2, 2, 2, 2, 2, 2, 2, 2, 2, 2, 2, 2, 2, 2, 2, 2, 2, 2, 2, 2, 2, 2, 2, 2, 2, 2, 2, 2, 2, 2, 2, 2, 2, 2, 2, 2, 2, 2, 2, 2, 2, 2, 2, 2, 2, 2, 2, 2, 2, 2, 2, 2, 2, 2, 2, 2, 2, 2, 2, 2, 2, 2, 2, 2, 2, 2, 2, 2, 2, 2, 2, 2, 2, 2, 2, 2, 2, 2, 2, 2, 2, 2, 2, 2, 2, 2, 2, 2, 2, 2, 2, 2, 2, 2, 2, 2, 2, 2, 2, 2, 2, 2, 2, 2, 2, 2, 2, 2, 2, 2, 2, 2, 2, 2, 2, 2, 2, 2, 2, 2, 2, 2, 2, 2, 2, 2, 2, 2, 2, 2, 2, 2, 2, 2, 2, 2, 2, 2, 2, 2, 2, 2, 2, 2, 2, 2, 2, 2, 2, 2, 2, 2, 2, 2, 2, 2, 2, 2, 2, 2, 2, 2, 2, 2, 2, 2, 2, 2, 2, 2, 2, 2, 2, 2, 2, 2, 2, 2, 2, 2, 2, 2, 2, 2, 2, 2, 2, 2, 2, 2, 2, 2, 2, 2, 2, 2, 2, 2, 2, 2, 2, 2, 2, 2, 2, 2, 2, 2, 2, 2, 2, 2, 2, 2, 2, 2, 2, 2, 2, 2, 2, 2, 2, 2, 2, 3 ),
 ( 0.000000000000000000, 0.5000000000000000000, 1.000000000000000000 ),
 ( 0.000000000000000000, 0.004385964912280701511, 0.008771929824561403022, 0.01315789473684210453, 0.01754385964912280604, 0.02192982456140350755, 0.02631578947368420907, 0.03070175438596491058, 0.03508771929824561209, 0.03947368421052631360, 0.04385964912280701511, 0.04824561403508771662, 0.05263157894736841813, 0.05701754385964911964, 0.06140350877192982115, 0.06578947368421052266, 0.07017543859649122417, 0.07456140350877192569, 0.07894736842105262720, 0.08333333333333332871, 0.08771929824561403022, 0.09210526315789473173, 0.09649122807017543324, 0.1008771929824561348, 0.1052631578947368363, 0.1096491228070175378, 0.1140350877192982393, 0.1184210526315789408, 0.1228070175438596423, 0.1271929824561403577, 0.1315789473684210453, 0.1359649122807017607, 0.1403508771929824483, 0.1447368421052631637, 0.1491228070175438514, 0.1535087719298245668, 0.1578947368421052544, 0.1622807017543859698, 0.1666666666666666574, 0.1710526315789473728, 0.1754385964912280604, 0.1798245614035087758, 0.1842105263157894635, 0.1885964912280701788, 0.1929824561403508665, 0.1973684210526315819, 0.2017543859649122695, 0.2061403508771929849, 0.2105263157894736725, 0.2149122807017543879, 0.2192982456140350755, 0.2236842105263157909, 0.2280701754385964786, 0.2324561403508771940, 0.2368421052631578816, 0.2412280701754385970, 0.2456140350877192846, 0.2500000000000000000, 0.2543859649122807154, 0.2587719298245614308, 0.2631578947368420907, 0.2675438596491228060, 0.2719298245614035214, 0.2763157894736842368, 0.2807017543859648967, 0.2850877192982456121, 0.2894736842105263275, 0.2938596491228070429, 0.2982456140350877027, 0.3026315789473684181, 0.3070175438596491335, 0.3114035087719298489, 0.3157894736842105088, 0.3201754385964912242, 0.3245614035087719396, 0.3289473684210526550, 0.3333333333333333148, 0.3377192982456140302, 0.3421052631578947456, 0.3464912280701754610, 0.3508771929824561209, 0.3552631578947368363, 0.3596491228070175517, 0.3640350877192982670, 0.3684210526315789269, 0.3728070175438596423, 0.3771929824561403577, 0.3815789473684210731, 0.3859649122807017330, 0.3903508771929824483, 0.3947368421052631637, 0.3991228070175438791, 0.4035087719298245390, 0.4078947368421052544, 0.4122807017543859698, 0.4166666666666666852, 0.4210526315789473450, 0.4254385964912280604, 0.4298245614035087758, 0.4342105263157894912, 0.4385964912280701511, 0.4429824561403508665, 0.4473684210526315819, 0.4517543859649122973, 0.4561403508771929571, 0.4605263157894736725, 0.4649122807017543879, 0.4692982456140351033, 0.4736842105263157632, 0.4780701754385964786, 0.4824561403508771940, 0.4868421052631579093, 0.4912280701754385692, 0.4956140350877192846, 0.5000000000000000000, 0.5043859649122807154, 0.5087719298245614308, 0.5131578947368421462, 0.5175438596491228616, 0.5219298245614034659, 0.5263157894736841813, 0.5307017543859648967, 0.5350877192982456121, 0.5394736842105263275, 0.5438596491228070429, 0.5482456140350877583, 0.5526315789473684736, 0.5570175438596490780, 0.5614035087719297934, 0.5657894736842105088, 0.5701754385964912242, 0.5745614035087719396, 0.5789473684210526550, 0.5833333333333333703, 0.5877192982456140857, 0.5921052631578946901, 0.5964912280701754055, 0.6008771929824561209, 0.6052631578947368363, 0.6096491228070175517, 0.6140350877192982670, 0.6184210526315789824, 0.6228070175438596978, 0.6271929824561403022, 0.6315789473684210176, 0.6359649122807017330, 0.6403508771929824483, 0.6447368421052631637, 0.6491228070175438791, 0.6535087719298245945, 0.6578947368421053099, 0.6622807017543859143, 0.6666666666666666297, 0.6710526315789473450, 0.6754385964912280604, 0.6798245614035087758, 0.6842105263157894912, 0.6885964912280702066, 0.6929824561403509220, 0.6973684210526315264, 0.7017543859649122417, 0.7061403508771929571, 0.7105263157894736725, 0.7149122807017543879, 0.7192982456140351033, 0.7236842105263158187, 0.7280701754385965341, 0.7324561403508771384, 0.7368421052631578538, 0.7412280701754385692, 0.7456140350877192846, 0.7500000000000000000, 0.7543859649122807154, 0.7587719298245614308, 0.7631578947368421462, 0.7675438596491228616, 0.7719298245614034659, 0.7763157894736841813, 0.7807017543859648967, 0.7850877192982456121, 0.7894736842105263275, 0.7938596491228070429, 0.7982456140350877583, 0.8026315789473684736, 0.8070175438596490780, 0.8114035087719297934, 0.8157894736842105088, 0.8201754385964912242, 0.8245614035087719396, 0.8289473684210526550, 0.8333333333333333703, 0.8377192982456140857, 0.8421052631578946901, 0.8464912280701754055, 0.8508771929824561209, 0.8552631578947368363, 0.8596491228070175517, 0.8640350877192982670, 0.8684210526315789824, 0.8728070175438596978, 0.8771929824561403022, 0.8815789473684210176, 0.8859649122807017330, 0.8903508771929824483, 0.8947368421052631637, 0.8991228070175438791, 0.9035087719298245945, 0.9078947368421053099, 0.9122807017543859143, 0.9166666666666666297, 0.9210526315789473450, 0.9254385964912280604, 0.9298245614035087758, 0.9342105263157894912, 0.9385964912280702066, 0.9429824561403509220, 0.9473684210526315264, 0.9517543859649122417, 0.9561403508771929571, 0.9605263157894736725, 0.9649122807017543879, 0.9692982456140351033, 0.9736842105263158187, 0.9780701754385965341, 0.9824561403508771384, 0.9868421052631578538, 0.9912280701754385692, 0.9956140350877192846, 1.000000000000000000 ),
 .UNSPECIFIED. ) 
 GEOMETRIC_REPRESENTATION_ITEM ( )  RATIONAL_B_SPLINE_SURFACE ( (
 ( 1.000000000000000000, 0.9659258262890683122, 1.000000000000000000, 0.9659258262890683122, 1.000000000000000000, 0.9659258262890683122, 1.000000000000000000, 0.9659258262890683122, 1.000000000000000000, 0.9659258262890683122, 1.000000000000000000, 0.9659258262890683122, 1.000000000000000000, 0.9659258262890683122, 1.000000000000000000, 0.9659258262890683122, 1.000000000000000000, 0.9659258262890683122, 1.000000000000000000, 0.9659258262890683122, 1.000000000000000000, 0.9659258262890683122, 1.000000000000000000, 0.9659258262890683122, 1.000000000000000000, 0.9659258262890683122, 1.000000000000000000, 0.9659258262890683122, 1.000000000000000000, 0.9659258262890683122, 1.000000000000000000, 0.9659258262890683122, 1.000000000000000000, 0.9659258262890683122, 1.000000000000000000, 0.9659258262890683122, 1.000000000000000000, 0.9659258262890683122, 1.000000000000000000, 0.9659258262890683122, 1.000000000000000000, 0.9659258262890683122, 1.000000000000000000, 0.9659258262890683122, 1.000000000000000000, 0.9659258262890683122, 1.000000000000000000, 0.9659258262890683122, 1.000000000000000000, 0.9659258262890683122, 1.000000000000000000, 0.9659258262890683122, 1.000000000000000000, 0.9659258262890683122, 1.000000000000000000, 0.9659258262890683122, 1.000000000000000000, 0.9659258262890683122, 1.000000000000000000, 0.9659258262890683122, 1.000000000000000000, 0.9659258262890683122, 1.000000000000000000, 0.9659258262890683122, 1.000000000000000000, 0.9659258262890683122, 1.000000000000000000, 0.9659258262890683122, 1.000000000000000000, 0.9659258262890683122, 1.000000000000000000, 0.9659258262890683122, 1.000000000000000000, 0.9659258262890683122, 1.000000000000000000, 0.9659258262890683122, 1.000000000000000000, 0.9659258262890683122, 1.000000000000000000, 0.9659258262890683122, 1.000000000000000000, 0.9659258262890683122, 1.000000000000000000, 0.9659258262890683122, 1.000000000000000000, 0.9659258262890683122, 1.000000000000000000, 0.9659258262890683122, 1.000000000000000000, 0.9659258262890683122, 1.000000000000000000, 0.9659258262890683122, 1.000000000000000000, 0.9659258262890683122, 1.000000000000000000, 0.9659258262890683122, 1.000000000000000000, 0.9659258262890683122, 1.000000000000000000, 0.9659258262890683122, 1.000000000000000000, 0.9659258262890683122, 1.000000000000000000, 0.9659258262890683122, 1.000000000000000000, 0.9659258262890683122, 1.000000000000000000, 0.9659258262890683122, 1.000000000000000000, 0.9659258262890683122, 1.000000000000000000, 0.9659258262890683122, 1.000000000000000000, 0.9659258262890683122, 1.000000000000000000, 0.9659258262890683122, 1.000000000000000000, 0.9659258262890683122, 1.000000000000000000, 0.9659258262890683122, 1.000000000000000000, 0.9659258262890683122, 1.000000000000000000, 0.9659258262890683122, 1.000000000000000000, 0.9659258262890683122, 1.000000000000000000, 0.9659258262890683122, 1.000000000000000000, 0.9659258262890683122, 1.000000000000000000, 0.9659258262890683122, 1.000000000000000000, 0.9659258262890683122, 1.000000000000000000, 0.9659258262890683122, 1.000000000000000000, 0.9659258262890683122, 1.000000000000000000, 0.9659258262890683122, 1.000000000000000000, 0.9659258262890683122, 1.000000000000000000, 0.9659258262890683122, 1.000000000000000000, 0.9659258262890683122, 1.000000000000000000, 0.9659258262890683122, 1.000000000000000000, 0.9659258262890683122, 1.000000000000000000, 0.9659258262890683122, 1.000000000000000000, 0.9659258262890683122, 1.000000000000000000, 0.9659258262890683122, 1.000000000000000000, 0.9659258262890683122, 1.000000000000000000, 0.9659258262890683122, 1.000000000000000000, 0.9659258262890683122, 1.000000000000000000, 0.9659258262890683122, 1.000000000000000000, 0.9659258262890683122, 1.000000000000000000, 0.9659258262890683122, 1.000000000000000000, 0.9659258262890683122, 1.000000000000000000, 0.9659258262890683122, 1.000000000000000000, 0.9659258262890683122, 1.000000000000000000, 0.9659258262890683122, 1.000000000000000000, 0.9659258262890683122, 1.000000000000000000, 0.9659258262890683122, 1.000000000000000000, 0.9659258262890683122, 1.000000000000000000, 0.9659258262890683122, 1.000000000000000000, 0.9659258262890683122, 1.000000000000000000, 0.9659258262890683122, 1.000000000000000000, 0.9659258262890683122, 1.000000000000000000, 0.9659258262890683122, 1.000000000000000000, 0.9659258262890683122, 1.000000000000000000, 0.9659258262890683122, 1.000000000000000000, 0.9659258262890683122, 1.000000000000000000, 0.9659258262890683122, 1.000000000000000000, 0.9659258262890683122, 1.000000000000000000, 0.9659258262890683122, 1.000000000000000000, 0.9659258262890683122, 1.000000000000000000, 0.9659258262890683122, 1.000000000000000000, 0.9659258262890683122, 1.000000000000000000, 0.9659258262890683122, 1.000000000000000000, 0.9659258262890683122, 1.000000000000000000, 0.9659258262890683122, 1.000000000000000000, 0.9659258262890683122, 1.000000000000000000, 0.9659258262890683122, 1.000000000000000000, 0.9659258262890683122, 1.000000000000000000, 0.9659258262890683122, 1.000000000000000000, 0.9659258262890683122, 1.000000000000000000, 0.9659258262890683122, 1.000000000000000000, 0.9659258262890683122, 1.000000000000000000, 0.9659258262890683122, 1.000000000000000000, 0.9659258262890683122, 1.000000000000000000, 0.9659258262890683122, 1.000000000000000000, 0.9659258262890683122, 1.000000000000000000, 0.9659258262890683122, 1.000000000000000000, 0.9659258262890683122, 1.000000000000000000, 0.9659258262890683122, 1.000000000000000000, 0.9659258262890683122, 1.000000000000000000, 0.9659258262890683122, 1.000000000000000000, 0.9659258262890683122, 1.000000000000000000, 0.9659258262890683122, 1.000000000000000000, 0.9659258262890683122, 1.000000000000000000, 0.9659258262890683122, 1.000000000000000000, 0.9659258262890683122, 1.000000000000000000, 0.9659258262890683122, 1.000000000000000000, 0.9659258262890683122, 1.000000000000000000, 0.9659258262890683122, 1.000000000000000000, 0.9659258262890683122, 1.000000000000000000, 0.9659258262890683122, 1.000000000000000000, 0.9659258262890683122, 1.000000000000000000, 0.9659258262890683122, 1.000000000000000000, 0.9659258262890683122, 1.000000000000000000, 0.9659258262890683122, 1.000000000000000000, 0.9659258262890683122, 1.000000000000000000, 0.9659258262890683122, 1.000000000000000000, 0.9659258262890683122, 1.000000000000000000, 0.9659258262890683122, 1.000000000000000000, 0.9659258262890683122, 1.000000000000000000, 0.9659258262890683122, 1.000000000000000000, 0.9659258262890683122, 1.000000000000000000, 0.9659258262890683122, 1.000000000000000000, 0.9659258262890683122, 1.000000000000000000, 0.9659258262890683122, 1.000000000000000000, 0.9659258262890683122, 1.000000000000000000, 0.9659258262890683122, 1.000000000000000000, 0.9659258262890683122, 1.000000000000000000, 0.9659258262890683122, 1.000000000000000000, 0.9659258262890683122, 1.000000000000000000, 0.9659258262890683122, 1.000000000000000000, 0.9659258262890683122, 1.000000000000000000, 0.9659258262890683122, 1.000000000000000000, 0.9659258262890683122, 1.000000000000000000, 0.9659258262890683122, 1.000000000000000000, 0.9659258262890683122, 1.000000000000000000, 0.9659258262890683122, 1.000000000000000000, 0.9659258262890683122, 1.000000000000000000, 0.9659258262890683122, 1.000000000000000000, 0.9659258262890683122, 1.000000000000000000, 0.9659258262890683122, 1.000000000000000000, 0.9659258262890683122, 1.000000000000000000, 0.9659258262890683122, 1.000000000000000000, 0.9659258262890683122, 1.000000000000000000, 0.9659258262890683122, 1.000000000000000000, 0.9659258262890683122, 1.000000000000000000, 0.9659258262890683122, 1.000000000000000000, 0.9659258262890683122, 1.000000000000000000, 0.9659258262890683122, 1.000000000000000000, 0.9659258262890683122, 1.000000000000000000, 0.9659258262890683122, 1.000000000000000000, 0.9659258262890683122, 1.000000000000000000, 0.9659258262890683122, 1.000000000000000000, 0.9659258262890683122, 1.000000000000000000, 0.9659258262890683122, 1.000000000000000000, 0.9659258262890683122, 1.000000000000000000, 0.9659258262890683122, 1.000000000000000000, 0.9659258262890683122, 1.000000000000000000, 0.9659258262890683122, 1.000000000000000000, 0.9659258262890683122, 1.000000000000000000, 0.9659258262890683122, 1.000000000000000000, 0.9659258262890683122, 1.000000000000000000, 0.9659258262890683122, 1.000000000000000000, 0.9659258262890683122, 1.000000000000000000, 0.9659258262890683122, 1.000000000000000000, 0.9659258262890683122, 1.000000000000000000, 0.9659258262890683122, 1.000000000000000000, 0.9659258262890683122, 1.000000000000000000, 0.9659258262890683122, 1.000000000000000000, 0.9659258262890683122, 1.000000000000000000, 0.9659258262890683122, 1.000000000000000000, 0.9659258262890683122, 1.000000000000000000, 0.9659258262890683122, 1.000000000000000000, 0.9659258262890683122, 1.000000000000000000, 0.9659258262890683122, 1.000000000000000000, 0.9659258262890683122, 1.000000000000000000, 0.9659258262890683122, 1.000000000000000000, 0.9659258262890683122, 1.000000000000000000, 0.9659258262890683122, 1.000000000000000000, 0.9659258262890683122, 1.000000000000000000, 0.9659258262890683122, 1.000000000000000000, 0.9659258262890683122, 1.000000000000000000, 0.9659258262890683122, 1.000000000000000000, 0.9659258262890683122, 1.000000000000000000, 0.9659258262890683122, 1.000000000000000000, 0.9659258262890683122, 1.000000000000000000, 0.9659258262890683122, 1.000000000000000000, 0.9659258262890683122, 1.000000000000000000, 0.9659258262890683122, 1.000000000000000000, 0.9659258262890683122, 1.000000000000000000, 0.9659258262890683122, 1.000000000000000000, 0.9659258262890683122, 1.000000000000000000, 0.9659258262890683122, 1.000000000000000000, 0.9659258262890683122, 1.000000000000000000, 0.9659258262890683122, 1.000000000000000000, 0.9659258262890683122, 1.000000000000000000, 0.9659258262890683122, 1.000000000000000000, 0.9659258262890683122, 1.000000000000000000, 0.9659258262890683122, 1.000000000000000000, 0.9659258262890683122, 1.000000000000000000, 0.9659258262890683122, 1.000000000000000000, 0.9659258262890683122, 1.000000000000000000, 0.9659258262890683122, 1.000000000000000000, 0.9659258262890683122, 1.000000000000000000, 0.9659258262890683122, 1.000000000000000000),
 ( 0.3333333333333333703, 0.3219752754296894559, 0.3333333333333333703, 0.3219752754296894559, 0.3333333333333333703, 0.3219752754296894559, 0.3333333333333333703, 0.3219752754296894559, 0.3333333333333333703, 0.3219752754296894559, 0.3333333333333333703, 0.3219752754296894559, 0.3333333333333333703, 0.3219752754296894559, 0.3333333333333333703, 0.3219752754296894559, 0.3333333333333333703, 0.3219752754296894559, 0.3333333333333333703, 0.3219752754296894559, 0.3333333333333333703, 0.3219752754296894559, 0.3333333333333333703, 0.3219752754296894559, 0.3333333333333333703, 0.3219752754296894559, 0.3333333333333333703, 0.3219752754296894559, 0.3333333333333333703, 0.3219752754296894559, 0.3333333333333333703, 0.3219752754296894559, 0.3333333333333333703, 0.3219752754296894559, 0.3333333333333333703, 0.3219752754296894559, 0.3333333333333333703, 0.3219752754296894559, 0.3333333333333333703, 0.3219752754296894559, 0.3333333333333333703, 0.3219752754296894559, 0.3333333333333333703, 0.3219752754296894559, 0.3333333333333333703, 0.3219752754296894559, 0.3333333333333333703, 0.3219752754296894559, 0.3333333333333333703, 0.3219752754296894559, 0.3333333333333333703, 0.3219752754296894559, 0.3333333333333333703, 0.3219752754296894559, 0.3333333333333333703, 0.3219752754296894559, 0.3333333333333333703, 0.3219752754296894559, 0.3333333333333333703, 0.3219752754296894559, 0.3333333333333333703, 0.3219752754296894559, 0.3333333333333333703, 0.3219752754296894559, 0.3333333333333333703, 0.3219752754296894559, 0.3333333333333333703, 0.3219752754296894559, 0.3333333333333333703, 0.3219752754296894559, 0.3333333333333333703, 0.3219752754296894559, 0.3333333333333333703, 0.3219752754296894559, 0.3333333333333333703, 0.3219752754296894559, 0.3333333333333333703, 0.3219752754296894559, 0.3333333333333333703, 0.3219752754296894559, 0.3333333333333333703, 0.3219752754296894559, 0.3333333333333333703, 0.3219752754296894559, 0.3333333333333333703, 0.3219752754296894559, 0.3333333333333333703, 0.3219752754296894559, 0.3333333333333333703, 0.3219752754296894559, 0.3333333333333333703, 0.3219752754296894559, 0.3333333333333333703, 0.3219752754296894559, 0.3333333333333333703, 0.3219752754296894559, 0.3333333333333333703, 0.3219752754296894559, 0.3333333333333333703, 0.3219752754296894559, 0.3333333333333333703, 0.3219752754296894559, 0.3333333333333333703, 0.3219752754296894559, 0.3333333333333333703, 0.3219752754296894559, 0.3333333333333333703, 0.3219752754296894559, 0.3333333333333333703, 0.3219752754296894559, 0.3333333333333333703, 0.3219752754296894559, 0.3333333333333333703, 0.3219752754296894559, 0.3333333333333333703, 0.3219752754296894559, 0.3333333333333333703, 0.3219752754296894559, 0.3333333333333333703, 0.3219752754296894559, 0.3333333333333333703, 0.3219752754296894559, 0.3333333333333333703, 0.3219752754296894559, 0.3333333333333333703, 0.3219752754296894559, 0.3333333333333333703, 0.3219752754296894559, 0.3333333333333333703, 0.3219752754296894559, 0.3333333333333333703, 0.3219752754296894559, 0.3333333333333333703, 0.3219752754296894559, 0.3333333333333333703, 0.3219752754296894559, 0.3333333333333333703, 0.3219752754296894559, 0.3333333333333333703, 0.3219752754296894559, 0.3333333333333333703, 0.3219752754296894559, 0.3333333333333333703, 0.3219752754296894559, 0.3333333333333333703, 0.3219752754296894559, 0.3333333333333333703, 0.3219752754296894559, 0.3333333333333333703, 0.3219752754296894559, 0.3333333333333333703, 0.3219752754296894559, 0.3333333333333333703, 0.3219752754296894559, 0.3333333333333333703, 0.3219752754296894559, 0.3333333333333333703, 0.3219752754296894559, 0.3333333333333333703, 0.3219752754296894559, 0.3333333333333333703, 0.3219752754296894559, 0.3333333333333333703, 0.3219752754296894559, 0.3333333333333333703, 0.3219752754296894559, 0.3333333333333333703, 0.3219752754296894559, 0.3333333333333333703, 0.3219752754296894559, 0.3333333333333333703, 0.3219752754296894559, 0.3333333333333333703, 0.3219752754296894559, 0.3333333333333333703, 0.3219752754296894559, 0.3333333333333333703, 0.3219752754296894559, 0.3333333333333333703, 0.3219752754296894559, 0.3333333333333333703, 0.3219752754296894559, 0.3333333333333333703, 0.3219752754296894559, 0.3333333333333333703, 0.3219752754296894559, 0.3333333333333333703, 0.3219752754296894559, 0.3333333333333333703, 0.3219752754296894559, 0.3333333333333333703, 0.3219752754296894559, 0.3333333333333333703, 0.3219752754296894559, 0.3333333333333333703, 0.3219752754296894559, 0.3333333333333333703, 0.3219752754296894559, 0.3333333333333333703, 0.3219752754296894559, 0.3333333333333333703, 0.3219752754296894559, 0.3333333333333333703, 0.3219752754296894559, 0.3333333333333333703, 0.3219752754296894559, 0.3333333333333333703, 0.3219752754296894559, 0.3333333333333333703, 0.3219752754296894559, 0.3333333333333333703, 0.3219752754296894559, 0.3333333333333333703, 0.3219752754296894559, 0.3333333333333333703, 0.3219752754296894559, 0.3333333333333333703, 0.3219752754296894559, 0.3333333333333333703, 0.3219752754296894559, 0.3333333333333333703, 0.3219752754296894559, 0.3333333333333333703, 0.3219752754296894559, 0.3333333333333333703, 0.3219752754296894559, 0.3333333333333333703, 0.3219752754296894559, 0.3333333333333333703, 0.3219752754296894559, 0.3333333333333333703, 0.3219752754296894559, 0.3333333333333333703, 0.3219752754296894559, 0.3333333333333333703, 0.3219752754296894559, 0.3333333333333333703, 0.3219752754296894559, 0.3333333333333333703, 0.3219752754296894559, 0.3333333333333333703, 0.3219752754296894559, 0.3333333333333333703, 0.3219752754296894559, 0.3333333333333333703, 0.3219752754296894559, 0.3333333333333333703, 0.3219752754296894559, 0.3333333333333333703, 0.3219752754296894559, 0.3333333333333333703, 0.3219752754296894559, 0.3333333333333333703, 0.3219752754296894559, 0.3333333333333333703, 0.3219752754296894559, 0.3333333333333333703, 0.3219752754296894559, 0.3333333333333333703, 0.3219752754296894559, 0.3333333333333333703, 0.3219752754296894559, 0.3333333333333333703, 0.3219752754296894559, 0.3333333333333333703, 0.3219752754296894559, 0.3333333333333333703, 0.3219752754296894559, 0.3333333333333333703, 0.3219752754296894559, 0.3333333333333333703, 0.3219752754296894559, 0.3333333333333333703, 0.3219752754296894559, 0.3333333333333333703, 0.3219752754296894559, 0.3333333333333333703, 0.3219752754296894559, 0.3333333333333333703, 0.3219752754296894559, 0.3333333333333333703, 0.3219752754296894559, 0.3333333333333333703, 0.3219752754296894559, 0.3333333333333333703, 0.3219752754296894559, 0.3333333333333333703, 0.3219752754296894559, 0.3333333333333333703, 0.3219752754296894559, 0.3333333333333333703, 0.3219752754296894559, 0.3333333333333333703, 0.3219752754296894559, 0.3333333333333333703, 0.3219752754296894559, 0.3333333333333333703, 0.3219752754296894559, 0.3333333333333333703, 0.3219752754296894559, 0.3333333333333333703, 0.3219752754296894559, 0.3333333333333333703, 0.3219752754296894559, 0.3333333333333333703, 0.3219752754296894559, 0.3333333333333333703, 0.3219752754296894559, 0.3333333333333333703, 0.3219752754296894559, 0.3333333333333333703, 0.3219752754296894559, 0.3333333333333333703, 0.3219752754296894559, 0.3333333333333333703, 0.3219752754296894559, 0.3333333333333333703, 0.3219752754296894559, 0.3333333333333333703, 0.3219752754296894559, 0.3333333333333333703, 0.3219752754296894559, 0.3333333333333333703, 0.3219752754296894559, 0.3333333333333333703, 0.3219752754296894559, 0.3333333333333333703, 0.3219752754296894559, 0.3333333333333333703, 0.3219752754296894559, 0.3333333333333333703, 0.3219752754296894559, 0.3333333333333333703, 0.3219752754296894559, 0.3333333333333333703, 0.3219752754296894559, 0.3333333333333333703, 0.3219752754296894559, 0.3333333333333333703, 0.3219752754296894559, 0.3333333333333333703, 0.3219752754296894559, 0.3333333333333333703, 0.3219752754296894559, 0.3333333333333333703, 0.3219752754296894559, 0.3333333333333333703, 0.3219752754296894559, 0.3333333333333333703, 0.3219752754296894559, 0.3333333333333333703, 0.3219752754296894559, 0.3333333333333333703, 0.3219752754296894559, 0.3333333333333333703, 0.3219752754296894559, 0.3333333333333333703, 0.3219752754296894559, 0.3333333333333333703, 0.3219752754296894559, 0.3333333333333333703, 0.3219752754296894559, 0.3333333333333333703, 0.3219752754296894559, 0.3333333333333333703, 0.3219752754296894559, 0.3333333333333333703, 0.3219752754296894559, 0.3333333333333333703, 0.3219752754296894559, 0.3333333333333333703, 0.3219752754296894559, 0.3333333333333333703, 0.3219752754296894559, 0.3333333333333333703, 0.3219752754296894559, 0.3333333333333333703, 0.3219752754296894559, 0.3333333333333333703, 0.3219752754296894559, 0.3333333333333333703, 0.3219752754296894559, 0.3333333333333333703, 0.3219752754296894559, 0.3333333333333333703, 0.3219752754296894559, 0.3333333333333333703, 0.3219752754296894559, 0.3333333333333333703, 0.3219752754296894559, 0.3333333333333333703, 0.3219752754296894559, 0.3333333333333333703, 0.3219752754296894559, 0.3333333333333333703, 0.3219752754296894559, 0.3333333333333333703, 0.3219752754296894559, 0.3333333333333333703, 0.3219752754296894559, 0.3333333333333333703, 0.3219752754296894559, 0.3333333333333333703, 0.3219752754296894559, 0.3333333333333333703, 0.3219752754296894559, 0.3333333333333333703, 0.3219752754296894559, 0.3333333333333333703, 0.3219752754296894559, 0.3333333333333333703, 0.3219752754296894559, 0.3333333333333333703, 0.3219752754296894559, 0.3333333333333333703, 0.3219752754296894559, 0.3333333333333333703, 0.3219752754296894559, 0.3333333333333333703, 0.3219752754296894559, 0.3333333333333333703, 0.3219752754296894559, 0.3333333333333333703, 0.3219752754296894559, 0.3333333333333333703, 0.3219752754296894559, 0.3333333333333333703, 0.3219752754296894559, 0.3333333333333333703, 0.3219752754296894559, 0.3333333333333333703, 0.3219752754296894559, 0.3333333333333333703, 0.3219752754296894559, 0.3333333333333333703, 0.3219752754296894559, 0.3333333333333333703, 0.3219752754296894559, 0.3333333333333333703, 0.3219752754296894559, 0.3333333333333333703, 0.3219752754296894559, 0.3333333333333333703, 0.3219752754296894559, 0.3333333333333333703, 0.3219752754296894559, 0.3333333333333333703, 0.3219752754296894559, 0.3333333333333333703, 0.3219752754296894559, 0.3333333333333333703, 0.3219752754296894559, 0.3333333333333333703, 0.3219752754296894559, 0.3333333333333333703, 0.3219752754296894559, 0.3333333333333333703),
 ( 0.3333333333333333703, 0.3219752754296894559, 0.3333333333333333703, 0.3219752754296894559, 0.3333333333333333703, 0.3219752754296894559, 0.3333333333333333703, 0.3219752754296894559, 0.3333333333333333703, 0.3219752754296894559, 0.3333333333333333703, 0.3219752754296894559, 0.3333333333333333703, 0.3219752754296894559, 0.3333333333333333703, 0.3219752754296894559, 0.3333333333333333703, 0.3219752754296894559, 0.3333333333333333703, 0.3219752754296894559, 0.3333333333333333703, 0.3219752754296894559, 0.3333333333333333703, 0.3219752754296894559, 0.3333333333333333703, 0.3219752754296894559, 0.3333333333333333703, 0.3219752754296894559, 0.3333333333333333703, 0.3219752754296894559, 0.3333333333333333703, 0.3219752754296894559, 0.3333333333333333703, 0.3219752754296894559, 0.3333333333333333703, 0.3219752754296894559, 0.3333333333333333703, 0.3219752754296894559, 0.3333333333333333703, 0.3219752754296894559, 0.3333333333333333703, 0.3219752754296894559, 0.3333333333333333703, 0.3219752754296894559, 0.3333333333333333703, 0.3219752754296894559, 0.3333333333333333703, 0.3219752754296894559, 0.3333333333333333703, 0.3219752754296894559, 0.3333333333333333703, 0.3219752754296894559, 0.3333333333333333703, 0.3219752754296894559, 0.3333333333333333703, 0.3219752754296894559, 0.3333333333333333703, 0.3219752754296894559, 0.3333333333333333703, 0.3219752754296894559, 0.3333333333333333703, 0.3219752754296894559, 0.3333333333333333703, 0.3219752754296894559, 0.3333333333333333703, 0.3219752754296894559, 0.3333333333333333703, 0.3219752754296894559, 0.3333333333333333703, 0.3219752754296894559, 0.3333333333333333703, 0.3219752754296894559, 0.3333333333333333703, 0.3219752754296894559, 0.3333333333333333703, 0.3219752754296894559, 0.3333333333333333703, 0.3219752754296894559, 0.3333333333333333703, 0.3219752754296894559, 0.3333333333333333703, 0.3219752754296894559, 0.3333333333333333703, 0.3219752754296894559, 0.3333333333333333703, 0.3219752754296894559, 0.3333333333333333703, 0.3219752754296894559, 0.3333333333333333703, 0.3219752754296894559, 0.3333333333333333703, 0.3219752754296894559, 0.3333333333333333703, 0.3219752754296894559, 0.3333333333333333703, 0.3219752754296894559, 0.3333333333333333703, 0.3219752754296894559, 0.3333333333333333703, 0.3219752754296894559, 0.3333333333333333703, 0.3219752754296894559, 0.3333333333333333703, 0.3219752754296894559, 0.3333333333333333703, 0.3219752754296894559, 0.3333333333333333703, 0.3219752754296894559, 0.3333333333333333703, 0.3219752754296894559, 0.3333333333333333703, 0.3219752754296894559, 0.3333333333333333703, 0.3219752754296894559, 0.3333333333333333703, 0.3219752754296894559, 0.3333333333333333703, 0.3219752754296894559, 0.3333333333333333703, 0.3219752754296894559, 0.3333333333333333703, 0.3219752754296894559, 0.3333333333333333703, 0.3219752754296894559, 0.3333333333333333703, 0.3219752754296894559, 0.3333333333333333703, 0.3219752754296894559, 0.3333333333333333703, 0.3219752754296894559, 0.3333333333333333703, 0.3219752754296894559, 0.3333333333333333703, 0.3219752754296894559, 0.3333333333333333703, 0.3219752754296894559, 0.3333333333333333703, 0.3219752754296894559, 0.3333333333333333703, 0.3219752754296894559, 0.3333333333333333703, 0.3219752754296894559, 0.3333333333333333703, 0.3219752754296894559, 0.3333333333333333703, 0.3219752754296894559, 0.3333333333333333703, 0.3219752754296894559, 0.3333333333333333703, 0.3219752754296894559, 0.3333333333333333703, 0.3219752754296894559, 0.3333333333333333703, 0.3219752754296894559, 0.3333333333333333703, 0.3219752754296894559, 0.3333333333333333703, 0.3219752754296894559, 0.3333333333333333703, 0.3219752754296894559, 0.3333333333333333703, 0.3219752754296894559, 0.3333333333333333703, 0.3219752754296894559, 0.3333333333333333703, 0.3219752754296894559, 0.3333333333333333703, 0.3219752754296894559, 0.3333333333333333703, 0.3219752754296894559, 0.3333333333333333703, 0.3219752754296894559, 0.3333333333333333703, 0.3219752754296894559, 0.3333333333333333703, 0.3219752754296894559, 0.3333333333333333703, 0.3219752754296894559, 0.3333333333333333703, 0.3219752754296894559, 0.3333333333333333703, 0.3219752754296894559, 0.3333333333333333703, 0.3219752754296894559, 0.3333333333333333703, 0.3219752754296894559, 0.3333333333333333703, 0.3219752754296894559, 0.3333333333333333703, 0.3219752754296894559, 0.3333333333333333703, 0.3219752754296894559, 0.3333333333333333703, 0.3219752754296894559, 0.3333333333333333703, 0.3219752754296894559, 0.3333333333333333703, 0.3219752754296894559, 0.3333333333333333703, 0.3219752754296894559, 0.3333333333333333703, 0.3219752754296894559, 0.3333333333333333703, 0.3219752754296894559, 0.3333333333333333703, 0.3219752754296894559, 0.3333333333333333703, 0.3219752754296894559, 0.3333333333333333703, 0.3219752754296894559, 0.3333333333333333703, 0.3219752754296894559, 0.3333333333333333703, 0.3219752754296894559, 0.3333333333333333703, 0.3219752754296894559, 0.3333333333333333703, 0.3219752754296894559, 0.3333333333333333703, 0.3219752754296894559, 0.3333333333333333703, 0.3219752754296894559, 0.3333333333333333703, 0.3219752754296894559, 0.3333333333333333703, 0.3219752754296894559, 0.3333333333333333703, 0.3219752754296894559, 0.3333333333333333703, 0.3219752754296894559, 0.3333333333333333703, 0.3219752754296894559, 0.3333333333333333703, 0.3219752754296894559, 0.3333333333333333703, 0.3219752754296894559, 0.3333333333333333703, 0.3219752754296894559, 0.3333333333333333703, 0.3219752754296894559, 0.3333333333333333703, 0.3219752754296894559, 0.3333333333333333703, 0.3219752754296894559, 0.3333333333333333703, 0.3219752754296894559, 0.3333333333333333703, 0.3219752754296894559, 0.3333333333333333703, 0.3219752754296894559, 0.3333333333333333703, 0.3219752754296894559, 0.3333333333333333703, 0.3219752754296894559, 0.3333333333333333703, 0.3219752754296894559, 0.3333333333333333703, 0.3219752754296894559, 0.3333333333333333703, 0.3219752754296894559, 0.3333333333333333703, 0.3219752754296894559, 0.3333333333333333703, 0.3219752754296894559, 0.3333333333333333703, 0.3219752754296894559, 0.3333333333333333703, 0.3219752754296894559, 0.3333333333333333703, 0.3219752754296894559, 0.3333333333333333703, 0.3219752754296894559, 0.3333333333333333703, 0.3219752754296894559, 0.3333333333333333703, 0.3219752754296894559, 0.3333333333333333703, 0.3219752754296894559, 0.3333333333333333703, 0.3219752754296894559, 0.3333333333333333703, 0.3219752754296894559, 0.3333333333333333703, 0.3219752754296894559, 0.3333333333333333703, 0.3219752754296894559, 0.3333333333333333703, 0.3219752754296894559, 0.3333333333333333703, 0.3219752754296894559, 0.3333333333333333703, 0.3219752754296894559, 0.3333333333333333703, 0.3219752754296894559, 0.3333333333333333703, 0.3219752754296894559, 0.3333333333333333703, 0.3219752754296894559, 0.3333333333333333703, 0.3219752754296894559, 0.3333333333333333703, 0.3219752754296894559, 0.3333333333333333703, 0.3219752754296894559, 0.3333333333333333703, 0.3219752754296894559, 0.3333333333333333703, 0.3219752754296894559, 0.3333333333333333703, 0.3219752754296894559, 0.3333333333333333703, 0.3219752754296894559, 0.3333333333333333703, 0.3219752754296894559, 0.3333333333333333703, 0.3219752754296894559, 0.3333333333333333703, 0.3219752754296894559, 0.3333333333333333703, 0.3219752754296894559, 0.3333333333333333703, 0.3219752754296894559, 0.3333333333333333703, 0.3219752754296894559, 0.3333333333333333703, 0.3219752754296894559, 0.3333333333333333703, 0.3219752754296894559, 0.3333333333333333703, 0.3219752754296894559, 0.3333333333333333703, 0.3219752754296894559, 0.3333333333333333703, 0.3219752754296894559, 0.3333333333333333703, 0.3219752754296894559, 0.3333333333333333703, 0.3219752754296894559, 0.3333333333333333703, 0.3219752754296894559, 0.3333333333333333703, 0.3219752754296894559, 0.3333333333333333703, 0.3219752754296894559, 0.3333333333333333703, 0.3219752754296894559, 0.3333333333333333703, 0.3219752754296894559, 0.3333333333333333703, 0.3219752754296894559, 0.3333333333333333703, 0.3219752754296894559, 0.3333333333333333703, 0.3219752754296894559, 0.3333333333333333703, 0.3219752754296894559, 0.3333333333333333703, 0.3219752754296894559, 0.3333333333333333703, 0.3219752754296894559, 0.3333333333333333703, 0.3219752754296894559, 0.3333333333333333703, 0.3219752754296894559, 0.3333333333333333703, 0.3219752754296894559, 0.3333333333333333703, 0.3219752754296894559, 0.3333333333333333703, 0.3219752754296894559, 0.3333333333333333703, 0.3219752754296894559, 0.3333333333333333703, 0.3219752754296894559, 0.3333333333333333703, 0.3219752754296894559, 0.3333333333333333703, 0.3219752754296894559, 0.3333333333333333703, 0.3219752754296894559, 0.3333333333333333703, 0.3219752754296894559, 0.3333333333333333703, 0.3219752754296894559, 0.3333333333333333703, 0.3219752754296894559, 0.3333333333333333703, 0.3219752754296894559, 0.3333333333333333703, 0.3219752754296894559, 0.3333333333333333703, 0.3219752754296894559, 0.3333333333333333703, 0.3219752754296894559, 0.3333333333333333703, 0.3219752754296894559, 0.3333333333333333703, 0.3219752754296894559, 0.3333333333333333703, 0.3219752754296894559, 0.3333333333333333703, 0.3219752754296894559, 0.3333333333333333703, 0.3219752754296894559, 0.3333333333333333703, 0.3219752754296894559, 0.3333333333333333703, 0.3219752754296894559, 0.3333333333333333703, 0.3219752754296894559, 0.3333333333333333703, 0.3219752754296894559, 0.3333333333333333703, 0.3219752754296894559, 0.3333333333333333703, 0.3219752754296894559, 0.3333333333333333703, 0.3219752754296894559, 0.3333333333333333703, 0.3219752754296894559, 0.3333333333333333703, 0.3219752754296894559, 0.3333333333333333703, 0.3219752754296894559, 0.3333333333333333703, 0.3219752754296894559, 0.3333333333333333703, 0.3219752754296894559, 0.3333333333333333703, 0.3219752754296894559, 0.3333333333333333703, 0.3219752754296894559, 0.3333333333333333703, 0.3219752754296894559, 0.3333333333333333703, 0.3219752754296894559, 0.3333333333333333703, 0.3219752754296894559, 0.3333333333333333703, 0.3219752754296894559, 0.3333333333333333703, 0.3219752754296894559, 0.3333333333333333703, 0.3219752754296894559, 0.3333333333333333703, 0.3219752754296894559, 0.3333333333333333703, 0.3219752754296894559, 0.3333333333333333703, 0.3219752754296894559, 0.3333333333333333703, 0.3219752754296894559, 0.3333333333333333703, 0.3219752754296894559, 0.3333333333333333703, 0.3219752754296894559, 0.3333333333333333703),
 ( 1.000000000000000000, 0.9659258262890683122, 1.000000000000000000, 0.9659258262890683122, 1.000000000000000000, 0.9659258262890683122, 1.000000000000000000, 0.9659258262890683122, 1.000000000000000000, 0.9659258262890683122, 1.000000000000000000, 0.9659258262890683122, 1.000000000000000000, 0.9659258262890683122, 1.000000000000000000, 0.9659258262890683122, 1.000000000000000000, 0.9659258262890683122, 1.000000000000000000, 0.9659258262890683122, 1.000000000000000000, 0.9659258262890683122, 1.000000000000000000, 0.9659258262890683122, 1.000000000000000000, 0.9659258262890683122, 1.000000000000000000, 0.9659258262890683122, 1.000000000000000000, 0.9659258262890683122, 1.000000000000000000, 0.9659258262890683122, 1.000000000000000000, 0.9659258262890683122, 1.000000000000000000, 0.9659258262890683122, 1.000000000000000000, 0.9659258262890683122, 1.000000000000000000, 0.9659258262890683122, 1.000000000000000000, 0.9659258262890683122, 1.000000000000000000, 0.9659258262890683122, 1.000000000000000000, 0.9659258262890683122, 1.000000000000000000, 0.9659258262890683122, 1.000000000000000000, 0.9659258262890683122, 1.000000000000000000, 0.9659258262890683122, 1.000000000000000000, 0.9659258262890683122, 1.000000000000000000, 0.9659258262890683122, 1.000000000000000000, 0.9659258262890683122, 1.000000000000000000, 0.9659258262890683122, 1.000000000000000000, 0.9659258262890683122, 1.000000000000000000, 0.9659258262890683122, 1.000000000000000000, 0.9659258262890683122, 1.000000000000000000, 0.9659258262890683122, 1.000000000000000000, 0.9659258262890683122, 1.000000000000000000, 0.9659258262890683122, 1.000000000000000000, 0.9659258262890683122, 1.000000000000000000, 0.9659258262890683122, 1.000000000000000000, 0.9659258262890683122, 1.000000000000000000, 0.9659258262890683122, 1.000000000000000000, 0.9659258262890683122, 1.000000000000000000, 0.9659258262890683122, 1.000000000000000000, 0.9659258262890683122, 1.000000000000000000, 0.9659258262890683122, 1.000000000000000000, 0.9659258262890683122, 1.000000000000000000, 0.9659258262890683122, 1.000000000000000000, 0.9659258262890683122, 1.000000000000000000, 0.9659258262890683122, 1.000000000000000000, 0.9659258262890683122, 1.000000000000000000, 0.9659258262890683122, 1.000000000000000000, 0.9659258262890683122, 1.000000000000000000, 0.9659258262890683122, 1.000000000000000000, 0.9659258262890683122, 1.000000000000000000, 0.9659258262890683122, 1.000000000000000000, 0.9659258262890683122, 1.000000000000000000, 0.9659258262890683122, 1.000000000000000000, 0.9659258262890683122, 1.000000000000000000, 0.9659258262890683122, 1.000000000000000000, 0.9659258262890683122, 1.000000000000000000, 0.9659258262890683122, 1.000000000000000000, 0.9659258262890683122, 1.000000000000000000, 0.9659258262890683122, 1.000000000000000000, 0.9659258262890683122, 1.000000000000000000, 0.9659258262890683122, 1.000000000000000000, 0.9659258262890683122, 1.000000000000000000, 0.9659258262890683122, 1.000000000000000000, 0.9659258262890683122, 1.000000000000000000, 0.9659258262890683122, 1.000000000000000000, 0.9659258262890683122, 1.000000000000000000, 0.9659258262890683122, 1.000000000000000000, 0.9659258262890683122, 1.000000000000000000, 0.9659258262890683122, 1.000000000000000000, 0.9659258262890683122, 1.000000000000000000, 0.9659258262890683122, 1.000000000000000000, 0.9659258262890683122, 1.000000000000000000, 0.9659258262890683122, 1.000000000000000000, 0.9659258262890683122, 1.000000000000000000, 0.9659258262890683122, 1.000000000000000000, 0.9659258262890683122, 1.000000000000000000, 0.9659258262890683122, 1.000000000000000000, 0.9659258262890683122, 1.000000000000000000, 0.9659258262890683122, 1.000000000000000000, 0.9659258262890683122, 1.000000000000000000, 0.9659258262890683122, 1.000000000000000000, 0.9659258262890683122, 1.000000000000000000, 0.9659258262890683122, 1.000000000000000000, 0.9659258262890683122, 1.000000000000000000, 0.9659258262890683122, 1.000000000000000000, 0.9659258262890683122, 1.000000000000000000, 0.9659258262890683122, 1.000000000000000000, 0.9659258262890683122, 1.000000000000000000, 0.9659258262890683122, 1.000000000000000000, 0.9659258262890683122, 1.000000000000000000, 0.9659258262890683122, 1.000000000000000000, 0.9659258262890683122, 1.000000000000000000, 0.9659258262890683122, 1.000000000000000000, 0.9659258262890683122, 1.000000000000000000, 0.9659258262890683122, 1.000000000000000000, 0.9659258262890683122, 1.000000000000000000, 0.9659258262890683122, 1.000000000000000000, 0.9659258262890683122, 1.000000000000000000, 0.9659258262890683122, 1.000000000000000000, 0.9659258262890683122, 1.000000000000000000, 0.9659258262890683122, 1.000000000000000000, 0.9659258262890683122, 1.000000000000000000, 0.9659258262890683122, 1.000000000000000000, 0.9659258262890683122, 1.000000000000000000, 0.9659258262890683122, 1.000000000000000000, 0.9659258262890683122, 1.000000000000000000, 0.9659258262890683122, 1.000000000000000000, 0.9659258262890683122, 1.000000000000000000, 0.9659258262890683122, 1.000000000000000000, 0.9659258262890683122, 1.000000000000000000, 0.9659258262890683122, 1.000000000000000000, 0.9659258262890683122, 1.000000000000000000, 0.9659258262890683122, 1.000000000000000000, 0.9659258262890683122, 1.000000000000000000, 0.9659258262890683122, 1.000000000000000000, 0.9659258262890683122, 1.000000000000000000, 0.9659258262890683122, 1.000000000000000000, 0.9659258262890683122, 1.000000000000000000, 0.9659258262890683122, 1.000000000000000000, 0.9659258262890683122, 1.000000000000000000, 0.9659258262890683122, 1.000000000000000000, 0.9659258262890683122, 1.000000000000000000, 0.9659258262890683122, 1.000000000000000000, 0.9659258262890683122, 1.000000000000000000, 0.9659258262890683122, 1.000000000000000000, 0.9659258262890683122, 1.000000000000000000, 0.9659258262890683122, 1.000000000000000000, 0.9659258262890683122, 1.000000000000000000, 0.9659258262890683122, 1.000000000000000000, 0.9659258262890683122, 1.000000000000000000, 0.9659258262890683122, 1.000000000000000000, 0.9659258262890683122, 1.000000000000000000, 0.9659258262890683122, 1.000000000000000000, 0.9659258262890683122, 1.000000000000000000, 0.9659258262890683122, 1.000000000000000000, 0.9659258262890683122, 1.000000000000000000, 0.9659258262890683122, 1.000000000000000000, 0.9659258262890683122, 1.000000000000000000, 0.9659258262890683122, 1.000000000000000000, 0.9659258262890683122, 1.000000000000000000, 0.9659258262890683122, 1.000000000000000000, 0.9659258262890683122, 1.000000000000000000, 0.9659258262890683122, 1.000000000000000000, 0.9659258262890683122, 1.000000000000000000, 0.9659258262890683122, 1.000000000000000000, 0.9659258262890683122, 1.000000000000000000, 0.9659258262890683122, 1.000000000000000000, 0.9659258262890683122, 1.000000000000000000, 0.9659258262890683122, 1.000000000000000000, 0.9659258262890683122, 1.000000000000000000, 0.9659258262890683122, 1.000000000000000000, 0.9659258262890683122, 1.000000000000000000, 0.9659258262890683122, 1.000000000000000000, 0.9659258262890683122, 1.000000000000000000, 0.9659258262890683122, 1.000000000000000000, 0.9659258262890683122, 1.000000000000000000, 0.9659258262890683122, 1.000000000000000000, 0.9659258262890683122, 1.000000000000000000, 0.9659258262890683122, 1.000000000000000000, 0.9659258262890683122, 1.000000000000000000, 0.9659258262890683122, 1.000000000000000000, 0.9659258262890683122, 1.000000000000000000, 0.9659258262890683122, 1.000000000000000000, 0.9659258262890683122, 1.000000000000000000, 0.9659258262890683122, 1.000000000000000000, 0.9659258262890683122, 1.000000000000000000, 0.9659258262890683122, 1.000000000000000000, 0.9659258262890683122, 1.000000000000000000, 0.9659258262890683122, 1.000000000000000000, 0.9659258262890683122, 1.000000000000000000, 0.9659258262890683122, 1.000000000000000000, 0.9659258262890683122, 1.000000000000000000, 0.9659258262890683122, 1.000000000000000000, 0.9659258262890683122, 1.000000000000000000, 0.9659258262890683122, 1.000000000000000000, 0.9659258262890683122, 1.000000000000000000, 0.9659258262890683122, 1.000000000000000000, 0.9659258262890683122, 1.000000000000000000, 0.9659258262890683122, 1.000000000000000000, 0.9659258262890683122, 1.000000000000000000, 0.9659258262890683122, 1.000000000000000000, 0.9659258262890683122, 1.000000000000000000, 0.9659258262890683122, 1.000000000000000000, 0.9659258262890683122, 1.000000000000000000, 0.9659258262890683122, 1.000000000000000000, 0.9659258262890683122, 1.000000000000000000, 0.9659258262890683122, 1.000000000000000000, 0.9659258262890683122, 1.000000000000000000, 0.9659258262890683122, 1.000000000000000000, 0.9659258262890683122, 1.000000000000000000, 0.9659258262890683122, 1.000000000000000000, 0.9659258262890683122, 1.000000000000000000, 0.9659258262890683122, 1.000000000000000000, 0.9659258262890683122, 1.000000000000000000, 0.9659258262890683122, 1.000000000000000000, 0.9659258262890683122, 1.000000000000000000, 0.9659258262890683122, 1.000000000000000000, 0.9659258262890683122, 1.000000000000000000, 0.9659258262890683122, 1.000000000000000000, 0.9659258262890683122, 1.000000000000000000, 0.9659258262890683122, 1.000000000000000000, 0.9659258262890683122, 1.000000000000000000, 0.9659258262890683122, 1.000000000000000000, 0.9659258262890683122, 1.000000000000000000, 0.9659258262890683122, 1.000000000000000000, 0.9659258262890683122, 1.000000000000000000, 0.9659258262890683122, 1.000000000000000000, 0.9659258262890683122, 1.000000000000000000, 0.9659258262890683122, 1.000000000000000000, 0.9659258262890683122, 1.000000000000000000, 0.9659258262890683122, 1.000000000000000000, 0.9659258262890683122, 1.000000000000000000, 0.9659258262890683122, 1.000000000000000000, 0.9659258262890683122, 1.000000000000000000, 0.9659258262890683122, 1.000000000000000000, 0.9659258262890683122, 1.000000000000000000, 0.9659258262890683122, 1.000000000000000000, 0.9659258262890683122, 1.000000000000000000, 0.9659258262890683122, 1.000000000000000000, 0.9659258262890683122, 1.000000000000000000, 0.9659258262890683122, 1.000000000000000000, 0.9659258262890683122, 1.000000000000000000, 0.9659258262890683122, 1.000000000000000000, 0.9659258262890683122, 1.000000000000000000, 0.9659258262890683122, 1.000000000000000000),
 ( 0.3333333333333333703, 0.3219752754296894559, 0.3333333333333333703, 0.3219752754296894559, 0.3333333333333333703, 0.3219752754296894559, 0.3333333333333333703, 0.3219752754296894559, 0.3333333333333333703, 0.3219752754296894559, 0.3333333333333333703, 0.3219752754296894559, 0.3333333333333333703, 0.3219752754296894559, 0.3333333333333333703, 0.3219752754296894559, 0.3333333333333333703, 0.3219752754296894559, 0.3333333333333333703, 0.3219752754296894559, 0.3333333333333333703, 0.3219752754296894559, 0.3333333333333333703, 0.3219752754296894559, 0.3333333333333333703, 0.3219752754296894559, 0.3333333333333333703, 0.3219752754296894559, 0.3333333333333333703, 0.3219752754296894559, 0.3333333333333333703, 0.3219752754296894559, 0.3333333333333333703, 0.3219752754296894559, 0.3333333333333333703, 0.3219752754296894559, 0.3333333333333333703, 0.3219752754296894559, 0.3333333333333333703, 0.3219752754296894559, 0.3333333333333333703, 0.3219752754296894559, 0.3333333333333333703, 0.3219752754296894559, 0.3333333333333333703, 0.3219752754296894559, 0.3333333333333333703, 0.3219752754296894559, 0.3333333333333333703, 0.3219752754296894559, 0.3333333333333333703, 0.3219752754296894559, 0.3333333333333333703, 0.3219752754296894559, 0.3333333333333333703, 0.3219752754296894559, 0.3333333333333333703, 0.3219752754296894559, 0.3333333333333333703, 0.3219752754296894559, 0.3333333333333333703, 0.3219752754296894559, 0.3333333333333333703, 0.3219752754296894559, 0.3333333333333333703, 0.3219752754296894559, 0.3333333333333333703, 0.3219752754296894559, 0.3333333333333333703, 0.3219752754296894559, 0.3333333333333333703, 0.3219752754296894559, 0.3333333333333333703, 0.3219752754296894559, 0.3333333333333333703, 0.3219752754296894559, 0.3333333333333333703, 0.3219752754296894559, 0.3333333333333333703, 0.3219752754296894559, 0.3333333333333333703, 0.3219752754296894559, 0.3333333333333333703, 0.3219752754296894559, 0.3333333333333333703, 0.3219752754296894559, 0.3333333333333333703, 0.3219752754296894559, 0.3333333333333333703, 0.3219752754296894559, 0.3333333333333333703, 0.3219752754296894559, 0.3333333333333333703, 0.3219752754296894559, 0.3333333333333333703, 0.3219752754296894559, 0.3333333333333333703, 0.3219752754296894559, 0.3333333333333333703, 0.3219752754296894559, 0.3333333333333333703, 0.3219752754296894559, 0.3333333333333333703, 0.3219752754296894559, 0.3333333333333333703, 0.3219752754296894559, 0.3333333333333333703, 0.3219752754296894559, 0.3333333333333333703, 0.3219752754296894559, 0.3333333333333333703, 0.3219752754296894559, 0.3333333333333333703, 0.3219752754296894559, 0.3333333333333333703, 0.3219752754296894559, 0.3333333333333333703, 0.3219752754296894559, 0.3333333333333333703, 0.3219752754296894559, 0.3333333333333333703, 0.3219752754296894559, 0.3333333333333333703, 0.3219752754296894559, 0.3333333333333333703, 0.3219752754296894559, 0.3333333333333333703, 0.3219752754296894559, 0.3333333333333333703, 0.3219752754296894559, 0.3333333333333333703, 0.3219752754296894559, 0.3333333333333333703, 0.3219752754296894559, 0.3333333333333333703, 0.3219752754296894559, 0.3333333333333333703, 0.3219752754296894559, 0.3333333333333333703, 0.3219752754296894559, 0.3333333333333333703, 0.3219752754296894559, 0.3333333333333333703, 0.3219752754296894559, 0.3333333333333333703, 0.3219752754296894559, 0.3333333333333333703, 0.3219752754296894559, 0.3333333333333333703, 0.3219752754296894559, 0.3333333333333333703, 0.3219752754296894559, 0.3333333333333333703, 0.3219752754296894559, 0.3333333333333333703, 0.3219752754296894559, 0.3333333333333333703, 0.3219752754296894559, 0.3333333333333333703, 0.3219752754296894559, 0.3333333333333333703, 0.3219752754296894559, 0.3333333333333333703, 0.3219752754296894559, 0.3333333333333333703, 0.3219752754296894559, 0.3333333333333333703, 0.3219752754296894559, 0.3333333333333333703, 0.3219752754296894559, 0.3333333333333333703, 0.3219752754296894559, 0.3333333333333333703, 0.3219752754296894559, 0.3333333333333333703, 0.3219752754296894559, 0.3333333333333333703, 0.3219752754296894559, 0.3333333333333333703, 0.3219752754296894559, 0.3333333333333333703, 0.3219752754296894559, 0.3333333333333333703, 0.3219752754296894559, 0.3333333333333333703, 0.3219752754296894559, 0.3333333333333333703, 0.3219752754296894559, 0.3333333333333333703, 0.3219752754296894559, 0.3333333333333333703, 0.3219752754296894559, 0.3333333333333333703, 0.3219752754296894559, 0.3333333333333333703, 0.3219752754296894559, 0.3333333333333333703, 0.3219752754296894559, 0.3333333333333333703, 0.3219752754296894559, 0.3333333333333333703, 0.3219752754296894559, 0.3333333333333333703, 0.3219752754296894559, 0.3333333333333333703, 0.3219752754296894559, 0.3333333333333333703, 0.3219752754296894559, 0.3333333333333333703, 0.3219752754296894559, 0.3333333333333333703, 0.3219752754296894559, 0.3333333333333333703, 0.3219752754296894559, 0.3333333333333333703, 0.3219752754296894559, 0.3333333333333333703, 0.3219752754296894559, 0.3333333333333333703, 0.3219752754296894559, 0.3333333333333333703, 0.3219752754296894559, 0.3333333333333333703, 0.3219752754296894559, 0.3333333333333333703, 0.3219752754296894559, 0.3333333333333333703, 0.3219752754296894559, 0.3333333333333333703, 0.3219752754296894559, 0.3333333333333333703, 0.3219752754296894559, 0.3333333333333333703, 0.3219752754296894559, 0.3333333333333333703, 0.3219752754296894559, 0.3333333333333333703, 0.3219752754296894559, 0.3333333333333333703, 0.3219752754296894559, 0.3333333333333333703, 0.3219752754296894559, 0.3333333333333333703, 0.3219752754296894559, 0.3333333333333333703, 0.3219752754296894559, 0.3333333333333333703, 0.3219752754296894559, 0.3333333333333333703, 0.3219752754296894559, 0.3333333333333333703, 0.3219752754296894559, 0.3333333333333333703, 0.3219752754296894559, 0.3333333333333333703, 0.3219752754296894559, 0.3333333333333333703, 0.3219752754296894559, 0.3333333333333333703, 0.3219752754296894559, 0.3333333333333333703, 0.3219752754296894559, 0.3333333333333333703, 0.3219752754296894559, 0.3333333333333333703, 0.3219752754296894559, 0.3333333333333333703, 0.3219752754296894559, 0.3333333333333333703, 0.3219752754296894559, 0.3333333333333333703, 0.3219752754296894559, 0.3333333333333333703, 0.3219752754296894559, 0.3333333333333333703, 0.3219752754296894559, 0.3333333333333333703, 0.3219752754296894559, 0.3333333333333333703, 0.3219752754296894559, 0.3333333333333333703, 0.3219752754296894559, 0.3333333333333333703, 0.3219752754296894559, 0.3333333333333333703, 0.3219752754296894559, 0.3333333333333333703, 0.3219752754296894559, 0.3333333333333333703, 0.3219752754296894559, 0.3333333333333333703, 0.3219752754296894559, 0.3333333333333333703, 0.3219752754296894559, 0.3333333333333333703, 0.3219752754296894559, 0.3333333333333333703, 0.3219752754296894559, 0.3333333333333333703, 0.3219752754296894559, 0.3333333333333333703, 0.3219752754296894559, 0.3333333333333333703, 0.3219752754296894559, 0.3333333333333333703, 0.3219752754296894559, 0.3333333333333333703, 0.3219752754296894559, 0.3333333333333333703, 0.3219752754296894559, 0.3333333333333333703, 0.3219752754296894559, 0.3333333333333333703, 0.3219752754296894559, 0.3333333333333333703, 0.3219752754296894559, 0.3333333333333333703, 0.3219752754296894559, 0.3333333333333333703, 0.3219752754296894559, 0.3333333333333333703, 0.3219752754296894559, 0.3333333333333333703, 0.3219752754296894559, 0.3333333333333333703, 0.3219752754296894559, 0.3333333333333333703, 0.3219752754296894559, 0.3333333333333333703, 0.3219752754296894559, 0.3333333333333333703, 0.3219752754296894559, 0.3333333333333333703, 0.3219752754296894559, 0.3333333333333333703, 0.3219752754296894559, 0.3333333333333333703, 0.3219752754296894559, 0.3333333333333333703, 0.3219752754296894559, 0.3333333333333333703, 0.3219752754296894559, 0.3333333333333333703, 0.3219752754296894559, 0.3333333333333333703, 0.3219752754296894559, 0.3333333333333333703, 0.3219752754296894559, 0.3333333333333333703, 0.3219752754296894559, 0.3333333333333333703, 0.3219752754296894559, 0.3333333333333333703, 0.3219752754296894559, 0.3333333333333333703, 0.3219752754296894559, 0.3333333333333333703, 0.3219752754296894559, 0.3333333333333333703, 0.3219752754296894559, 0.3333333333333333703, 0.3219752754296894559, 0.3333333333333333703, 0.3219752754296894559, 0.3333333333333333703, 0.3219752754296894559, 0.3333333333333333703, 0.3219752754296894559, 0.3333333333333333703, 0.3219752754296894559, 0.3333333333333333703, 0.3219752754296894559, 0.3333333333333333703, 0.3219752754296894559, 0.3333333333333333703, 0.3219752754296894559, 0.3333333333333333703, 0.3219752754296894559, 0.3333333333333333703, 0.3219752754296894559, 0.3333333333333333703, 0.3219752754296894559, 0.3333333333333333703, 0.3219752754296894559, 0.3333333333333333703, 0.3219752754296894559, 0.3333333333333333703, 0.3219752754296894559, 0.3333333333333333703, 0.3219752754296894559, 0.3333333333333333703, 0.3219752754296894559, 0.3333333333333333703, 0.3219752754296894559, 0.3333333333333333703, 0.3219752754296894559, 0.3333333333333333703, 0.3219752754296894559, 0.3333333333333333703, 0.3219752754296894559, 0.3333333333333333703, 0.3219752754296894559, 0.3333333333333333703, 0.3219752754296894559, 0.3333333333333333703, 0.3219752754296894559, 0.3333333333333333703, 0.3219752754296894559, 0.3333333333333333703, 0.3219752754296894559, 0.3333333333333333703, 0.3219752754296894559, 0.3333333333333333703, 0.3219752754296894559, 0.3333333333333333703, 0.3219752754296894559, 0.3333333333333333703, 0.3219752754296894559, 0.3333333333333333703, 0.3219752754296894559, 0.3333333333333333703, 0.3219752754296894559, 0.3333333333333333703, 0.3219752754296894559, 0.3333333333333333703, 0.3219752754296894559, 0.3333333333333333703, 0.3219752754296894559, 0.3333333333333333703, 0.3219752754296894559, 0.3333333333333333703, 0.3219752754296894559, 0.3333333333333333703, 0.3219752754296894559, 0.3333333333333333703, 0.3219752754296894559, 0.3333333333333333703, 0.3219752754296894559, 0.3333333333333333703, 0.3219752754296894559, 0.3333333333333333703, 0.3219752754296894559, 0.3333333333333333703, 0.3219752754296894559, 0.3333333333333333703, 0.3219752754296894559, 0.3333333333333333703, 0.3219752754296894559, 0.3333333333333333703, 0.3219752754296894559, 0.3333333333333333703, 0.3219752754296894559, 0.3333333333333333703, 0.3219752754296894559, 0.3333333333333333703, 0.3219752754296894559, 0.3333333333333333703),
 ( 0.3333333333333333703, 0.3219752754296894559, 0.3333333333333333703, 0.3219752754296894559, 0.3333333333333333703, 0.3219752754296894559, 0.3333333333333333703, 0.3219752754296894559, 0.3333333333333333703, 0.3219752754296894559, 0.3333333333333333703, 0.3219752754296894559, 0.3333333333333333703, 0.3219752754296894559, 0.3333333333333333703, 0.3219752754296894559, 0.3333333333333333703, 0.3219752754296894559, 0.3333333333333333703, 0.3219752754296894559, 0.3333333333333333703, 0.3219752754296894559, 0.3333333333333333703, 0.3219752754296894559, 0.3333333333333333703, 0.3219752754296894559, 0.3333333333333333703, 0.3219752754296894559, 0.3333333333333333703, 0.3219752754296894559, 0.3333333333333333703, 0.3219752754296894559, 0.3333333333333333703, 0.3219752754296894559, 0.3333333333333333703, 0.3219752754296894559, 0.3333333333333333703, 0.3219752754296894559, 0.3333333333333333703, 0.3219752754296894559, 0.3333333333333333703, 0.3219752754296894559, 0.3333333333333333703, 0.3219752754296894559, 0.3333333333333333703, 0.3219752754296894559, 0.3333333333333333703, 0.3219752754296894559, 0.3333333333333333703, 0.3219752754296894559, 0.3333333333333333703, 0.3219752754296894559, 0.3333333333333333703, 0.3219752754296894559, 0.3333333333333333703, 0.3219752754296894559, 0.3333333333333333703, 0.3219752754296894559, 0.3333333333333333703, 0.3219752754296894559, 0.3333333333333333703, 0.3219752754296894559, 0.3333333333333333703, 0.3219752754296894559, 0.3333333333333333703, 0.3219752754296894559, 0.3333333333333333703, 0.3219752754296894559, 0.3333333333333333703, 0.3219752754296894559, 0.3333333333333333703, 0.3219752754296894559, 0.3333333333333333703, 0.3219752754296894559, 0.3333333333333333703, 0.3219752754296894559, 0.3333333333333333703, 0.3219752754296894559, 0.3333333333333333703, 0.3219752754296894559, 0.3333333333333333703, 0.3219752754296894559, 0.3333333333333333703, 0.3219752754296894559, 0.3333333333333333703, 0.3219752754296894559, 0.3333333333333333703, 0.3219752754296894559, 0.3333333333333333703, 0.3219752754296894559, 0.3333333333333333703, 0.3219752754296894559, 0.3333333333333333703, 0.3219752754296894559, 0.3333333333333333703, 0.3219752754296894559, 0.3333333333333333703, 0.3219752754296894559, 0.3333333333333333703, 0.3219752754296894559, 0.3333333333333333703, 0.3219752754296894559, 0.3333333333333333703, 0.3219752754296894559, 0.3333333333333333703, 0.3219752754296894559, 0.3333333333333333703, 0.3219752754296894559, 0.3333333333333333703, 0.3219752754296894559, 0.3333333333333333703, 0.3219752754296894559, 0.3333333333333333703, 0.3219752754296894559, 0.3333333333333333703, 0.3219752754296894559, 0.3333333333333333703, 0.3219752754296894559, 0.3333333333333333703, 0.3219752754296894559, 0.3333333333333333703, 0.3219752754296894559, 0.3333333333333333703, 0.3219752754296894559, 0.3333333333333333703, 0.3219752754296894559, 0.3333333333333333703, 0.3219752754296894559, 0.3333333333333333703, 0.3219752754296894559, 0.3333333333333333703, 0.3219752754296894559, 0.3333333333333333703, 0.3219752754296894559, 0.3333333333333333703, 0.3219752754296894559, 0.3333333333333333703, 0.3219752754296894559, 0.3333333333333333703, 0.3219752754296894559, 0.3333333333333333703, 0.3219752754296894559, 0.3333333333333333703, 0.3219752754296894559, 0.3333333333333333703, 0.3219752754296894559, 0.3333333333333333703, 0.3219752754296894559, 0.3333333333333333703, 0.3219752754296894559, 0.3333333333333333703, 0.3219752754296894559, 0.3333333333333333703, 0.3219752754296894559, 0.3333333333333333703, 0.3219752754296894559, 0.3333333333333333703, 0.3219752754296894559, 0.3333333333333333703, 0.3219752754296894559, 0.3333333333333333703, 0.3219752754296894559, 0.3333333333333333703, 0.3219752754296894559, 0.3333333333333333703, 0.3219752754296894559, 0.3333333333333333703, 0.3219752754296894559, 0.3333333333333333703, 0.3219752754296894559, 0.3333333333333333703, 0.3219752754296894559, 0.3333333333333333703, 0.3219752754296894559, 0.3333333333333333703, 0.3219752754296894559, 0.3333333333333333703, 0.3219752754296894559, 0.3333333333333333703, 0.3219752754296894559, 0.3333333333333333703, 0.3219752754296894559, 0.3333333333333333703, 0.3219752754296894559, 0.3333333333333333703, 0.3219752754296894559, 0.3333333333333333703, 0.3219752754296894559, 0.3333333333333333703, 0.3219752754296894559, 0.3333333333333333703, 0.3219752754296894559, 0.3333333333333333703, 0.3219752754296894559, 0.3333333333333333703, 0.3219752754296894559, 0.3333333333333333703, 0.3219752754296894559, 0.3333333333333333703, 0.3219752754296894559, 0.3333333333333333703, 0.3219752754296894559, 0.3333333333333333703, 0.3219752754296894559, 0.3333333333333333703, 0.3219752754296894559, 0.3333333333333333703, 0.3219752754296894559, 0.3333333333333333703, 0.3219752754296894559, 0.3333333333333333703, 0.3219752754296894559, 0.3333333333333333703, 0.3219752754296894559, 0.3333333333333333703, 0.3219752754296894559, 0.3333333333333333703, 0.3219752754296894559, 0.3333333333333333703, 0.3219752754296894559, 0.3333333333333333703, 0.3219752754296894559, 0.3333333333333333703, 0.3219752754296894559, 0.3333333333333333703, 0.3219752754296894559, 0.3333333333333333703, 0.3219752754296894559, 0.3333333333333333703, 0.3219752754296894559, 0.3333333333333333703, 0.3219752754296894559, 0.3333333333333333703, 0.3219752754296894559, 0.3333333333333333703, 0.3219752754296894559, 0.3333333333333333703, 0.3219752754296894559, 0.3333333333333333703, 0.3219752754296894559, 0.3333333333333333703, 0.3219752754296894559, 0.3333333333333333703, 0.3219752754296894559, 0.3333333333333333703, 0.3219752754296894559, 0.3333333333333333703, 0.3219752754296894559, 0.3333333333333333703, 0.3219752754296894559, 0.3333333333333333703, 0.3219752754296894559, 0.3333333333333333703, 0.3219752754296894559, 0.3333333333333333703, 0.3219752754296894559, 0.3333333333333333703, 0.3219752754296894559, 0.3333333333333333703, 0.3219752754296894559, 0.3333333333333333703, 0.3219752754296894559, 0.3333333333333333703, 0.3219752754296894559, 0.3333333333333333703, 0.3219752754296894559, 0.3333333333333333703, 0.3219752754296894559, 0.3333333333333333703, 0.3219752754296894559, 0.3333333333333333703, 0.3219752754296894559, 0.3333333333333333703, 0.3219752754296894559, 0.3333333333333333703, 0.3219752754296894559, 0.3333333333333333703, 0.3219752754296894559, 0.3333333333333333703, 0.3219752754296894559, 0.3333333333333333703, 0.3219752754296894559, 0.3333333333333333703, 0.3219752754296894559, 0.3333333333333333703, 0.3219752754296894559, 0.3333333333333333703, 0.3219752754296894559, 0.3333333333333333703, 0.3219752754296894559, 0.3333333333333333703, 0.3219752754296894559, 0.3333333333333333703, 0.3219752754296894559, 0.3333333333333333703, 0.3219752754296894559, 0.3333333333333333703, 0.3219752754296894559, 0.3333333333333333703, 0.3219752754296894559, 0.3333333333333333703, 0.3219752754296894559, 0.3333333333333333703, 0.3219752754296894559, 0.3333333333333333703, 0.3219752754296894559, 0.3333333333333333703, 0.3219752754296894559, 0.3333333333333333703, 0.3219752754296894559, 0.3333333333333333703, 0.3219752754296894559, 0.3333333333333333703, 0.3219752754296894559, 0.3333333333333333703, 0.3219752754296894559, 0.3333333333333333703, 0.3219752754296894559, 0.3333333333333333703, 0.3219752754296894559, 0.3333333333333333703, 0.3219752754296894559, 0.3333333333333333703, 0.3219752754296894559, 0.3333333333333333703, 0.3219752754296894559, 0.3333333333333333703, 0.3219752754296894559, 0.3333333333333333703, 0.3219752754296894559, 0.3333333333333333703, 0.3219752754296894559, 0.3333333333333333703, 0.3219752754296894559, 0.3333333333333333703, 0.3219752754296894559, 0.3333333333333333703, 0.3219752754296894559, 0.3333333333333333703, 0.3219752754296894559, 0.3333333333333333703, 0.3219752754296894559, 0.3333333333333333703, 0.3219752754296894559, 0.3333333333333333703, 0.3219752754296894559, 0.3333333333333333703, 0.3219752754296894559, 0.3333333333333333703, 0.3219752754296894559, 0.3333333333333333703, 0.3219752754296894559, 0.3333333333333333703, 0.3219752754296894559, 0.3333333333333333703, 0.3219752754296894559, 0.3333333333333333703, 0.3219752754296894559, 0.3333333333333333703, 0.3219752754296894559, 0.3333333333333333703, 0.3219752754296894559, 0.3333333333333333703, 0.3219752754296894559, 0.3333333333333333703, 0.3219752754296894559, 0.3333333333333333703, 0.3219752754296894559, 0.3333333333333333703, 0.3219752754296894559, 0.3333333333333333703, 0.3219752754296894559, 0.3333333333333333703, 0.3219752754296894559, 0.3333333333333333703, 0.3219752754296894559, 0.3333333333333333703, 0.3219752754296894559, 0.3333333333333333703, 0.3219752754296894559, 0.3333333333333333703, 0.3219752754296894559, 0.3333333333333333703, 0.3219752754296894559, 0.3333333333333333703, 0.3219752754296894559, 0.3333333333333333703, 0.3219752754296894559, 0.3333333333333333703, 0.3219752754296894559, 0.3333333333333333703, 0.3219752754296894559, 0.3333333333333333703, 0.3219752754296894559, 0.3333333333333333703, 0.3219752754296894559, 0.3333333333333333703, 0.3219752754296894559, 0.3333333333333333703, 0.3219752754296894559, 0.3333333333333333703, 0.3219752754296894559, 0.3333333333333333703, 0.3219752754296894559, 0.3333333333333333703, 0.3219752754296894559, 0.3333333333333333703, 0.3219752754296894559, 0.3333333333333333703, 0.3219752754296894559, 0.3333333333333333703, 0.3219752754296894559, 0.3333333333333333703, 0.3219752754296894559, 0.3333333333333333703, 0.3219752754296894559, 0.3333333333333333703, 0.3219752754296894559, 0.3333333333333333703, 0.3219752754296894559, 0.3333333333333333703, 0.3219752754296894559, 0.3333333333333333703, 0.3219752754296894559, 0.3333333333333333703, 0.3219752754296894559, 0.3333333333333333703, 0.3219752754296894559, 0.3333333333333333703, 0.3219752754296894559, 0.3333333333333333703, 0.3219752754296894559, 0.3333333333333333703, 0.3219752754296894559, 0.3333333333333333703, 0.3219752754296894559, 0.3333333333333333703, 0.3219752754296894559, 0.3333333333333333703, 0.3219752754296894559, 0.3333333333333333703, 0.3219752754296894559, 0.3333333333333333703, 0.3219752754296894559, 0.3333333333333333703, 0.3219752754296894559, 0.3333333333333333703, 0.3219752754296894559, 0.3333333333333333703, 0.3219752754296894559, 0.3333333333333333703, 0.3219752754296894559, 0.3333333333333333703, 0.3219752754296894559, 0.3333333333333333703, 0.3219752754296894559, 0.3333333333333333703),
 ( 1.000000000000000000, 0.9659258262890683122, 1.000000000000000000, 0.9659258262890683122, 1.000000000000000000, 0.9659258262890683122, 1.000000000000000000, 0.9659258262890683122, 1.000000000000000000, 0.9659258262890683122, 1.000000000000000000, 0.9659258262890683122, 1.000000000000000000, 0.9659258262890683122, 1.000000000000000000, 0.9659258262890683122, 1.000000000000000000, 0.9659258262890683122, 1.000000000000000000, 0.9659258262890683122, 1.000000000000000000, 0.9659258262890683122, 1.000000000000000000, 0.9659258262890683122, 1.000000000000000000, 0.9659258262890683122, 1.000000000000000000, 0.9659258262890683122, 1.000000000000000000, 0.9659258262890683122, 1.000000000000000000, 0.9659258262890683122, 1.000000000000000000, 0.9659258262890683122, 1.000000000000000000, 0.9659258262890683122, 1.000000000000000000, 0.9659258262890683122, 1.000000000000000000, 0.9659258262890683122, 1.000000000000000000, 0.9659258262890683122, 1.000000000000000000, 0.9659258262890683122, 1.000000000000000000, 0.9659258262890683122, 1.000000000000000000, 0.9659258262890683122, 1.000000000000000000, 0.9659258262890683122, 1.000000000000000000, 0.9659258262890683122, 1.000000000000000000, 0.9659258262890683122, 1.000000000000000000, 0.9659258262890683122, 1.000000000000000000, 0.9659258262890683122, 1.000000000000000000, 0.9659258262890683122, 1.000000000000000000, 0.9659258262890683122, 1.000000000000000000, 0.9659258262890683122, 1.000000000000000000, 0.9659258262890683122, 1.000000000000000000, 0.9659258262890683122, 1.000000000000000000, 0.9659258262890683122, 1.000000000000000000, 0.9659258262890683122, 1.000000000000000000, 0.9659258262890683122, 1.000000000000000000, 0.9659258262890683122, 1.000000000000000000, 0.9659258262890683122, 1.000000000000000000, 0.9659258262890683122, 1.000000000000000000, 0.9659258262890683122, 1.000000000000000000, 0.9659258262890683122, 1.000000000000000000, 0.9659258262890683122, 1.000000000000000000, 0.9659258262890683122, 1.000000000000000000, 0.9659258262890683122, 1.000000000000000000, 0.9659258262890683122, 1.000000000000000000, 0.9659258262890683122, 1.000000000000000000, 0.9659258262890683122, 1.000000000000000000, 0.9659258262890683122, 1.000000000000000000, 0.9659258262890683122, 1.000000000000000000, 0.9659258262890683122, 1.000000000000000000, 0.9659258262890683122, 1.000000000000000000, 0.9659258262890683122, 1.000000000000000000, 0.9659258262890683122, 1.000000000000000000, 0.9659258262890683122, 1.000000000000000000, 0.9659258262890683122, 1.000000000000000000, 0.9659258262890683122, 1.000000000000000000, 0.9659258262890683122, 1.000000000000000000, 0.9659258262890683122, 1.000000000000000000, 0.9659258262890683122, 1.000000000000000000, 0.9659258262890683122, 1.000000000000000000, 0.9659258262890683122, 1.000000000000000000, 0.9659258262890683122, 1.000000000000000000, 0.9659258262890683122, 1.000000000000000000, 0.9659258262890683122, 1.000000000000000000, 0.9659258262890683122, 1.000000000000000000, 0.9659258262890683122, 1.000000000000000000, 0.9659258262890683122, 1.000000000000000000, 0.9659258262890683122, 1.000000000000000000, 0.9659258262890683122, 1.000000000000000000, 0.9659258262890683122, 1.000000000000000000, 0.9659258262890683122, 1.000000000000000000, 0.9659258262890683122, 1.000000000000000000, 0.9659258262890683122, 1.000000000000000000, 0.9659258262890683122, 1.000000000000000000, 0.9659258262890683122, 1.000000000000000000, 0.9659258262890683122, 1.000000000000000000, 0.9659258262890683122, 1.000000000000000000, 0.9659258262890683122, 1.000000000000000000, 0.9659258262890683122, 1.000000000000000000, 0.9659258262890683122, 1.000000000000000000, 0.9659258262890683122, 1.000000000000000000, 0.9659258262890683122, 1.000000000000000000, 0.9659258262890683122, 1.000000000000000000, 0.9659258262890683122, 1.000000000000000000, 0.9659258262890683122, 1.000000000000000000, 0.9659258262890683122, 1.000000000000000000, 0.9659258262890683122, 1.000000000000000000, 0.9659258262890683122, 1.000000000000000000, 0.9659258262890683122, 1.000000000000000000, 0.9659258262890683122, 1.000000000000000000, 0.9659258262890683122, 1.000000000000000000, 0.9659258262890683122, 1.000000000000000000, 0.9659258262890683122, 1.000000000000000000, 0.9659258262890683122, 1.000000000000000000, 0.9659258262890683122, 1.000000000000000000, 0.9659258262890683122, 1.000000000000000000, 0.9659258262890683122, 1.000000000000000000, 0.9659258262890683122, 1.000000000000000000, 0.9659258262890683122, 1.000000000000000000, 0.9659258262890683122, 1.000000000000000000, 0.9659258262890683122, 1.000000000000000000, 0.9659258262890683122, 1.000000000000000000, 0.9659258262890683122, 1.000000000000000000, 0.9659258262890683122, 1.000000000000000000, 0.9659258262890683122, 1.000000000000000000, 0.9659258262890683122, 1.000000000000000000, 0.9659258262890683122, 1.000000000000000000, 0.9659258262890683122, 1.000000000000000000, 0.9659258262890683122, 1.000000000000000000, 0.9659258262890683122, 1.000000000000000000, 0.9659258262890683122, 1.000000000000000000, 0.9659258262890683122, 1.000000000000000000, 0.9659258262890683122, 1.000000000000000000, 0.9659258262890683122, 1.000000000000000000, 0.9659258262890683122, 1.000000000000000000, 0.9659258262890683122, 1.000000000000000000, 0.9659258262890683122, 1.000000000000000000, 0.9659258262890683122, 1.000000000000000000, 0.9659258262890683122, 1.000000000000000000, 0.9659258262890683122, 1.000000000000000000, 0.9659258262890683122, 1.000000000000000000, 0.9659258262890683122, 1.000000000000000000, 0.9659258262890683122, 1.000000000000000000, 0.9659258262890683122, 1.000000000000000000, 0.9659258262890683122, 1.000000000000000000, 0.9659258262890683122, 1.000000000000000000, 0.9659258262890683122, 1.000000000000000000, 0.9659258262890683122, 1.000000000000000000, 0.9659258262890683122, 1.000000000000000000, 0.9659258262890683122, 1.000000000000000000, 0.9659258262890683122, 1.000000000000000000, 0.9659258262890683122, 1.000000000000000000, 0.9659258262890683122, 1.000000000000000000, 0.9659258262890683122, 1.000000000000000000, 0.9659258262890683122, 1.000000000000000000, 0.9659258262890683122, 1.000000000000000000, 0.9659258262890683122, 1.000000000000000000, 0.9659258262890683122, 1.000000000000000000, 0.9659258262890683122, 1.000000000000000000, 0.9659258262890683122, 1.000000000000000000, 0.9659258262890683122, 1.000000000000000000, 0.9659258262890683122, 1.000000000000000000, 0.9659258262890683122, 1.000000000000000000, 0.9659258262890683122, 1.000000000000000000, 0.9659258262890683122, 1.000000000000000000, 0.9659258262890683122, 1.000000000000000000, 0.9659258262890683122, 1.000000000000000000, 0.9659258262890683122, 1.000000000000000000, 0.9659258262890683122, 1.000000000000000000, 0.9659258262890683122, 1.000000000000000000, 0.9659258262890683122, 1.000000000000000000, 0.9659258262890683122, 1.000000000000000000, 0.9659258262890683122, 1.000000000000000000, 0.9659258262890683122, 1.000000000000000000, 0.9659258262890683122, 1.000000000000000000, 0.9659258262890683122, 1.000000000000000000, 0.9659258262890683122, 1.000000000000000000, 0.9659258262890683122, 1.000000000000000000, 0.9659258262890683122, 1.000000000000000000, 0.9659258262890683122, 1.000000000000000000, 0.9659258262890683122, 1.000000000000000000, 0.9659258262890683122, 1.000000000000000000, 0.9659258262890683122, 1.000000000000000000, 0.9659258262890683122, 1.000000000000000000, 0.9659258262890683122, 1.000000000000000000, 0.9659258262890683122, 1.000000000000000000, 0.9659258262890683122, 1.000000000000000000, 0.9659258262890683122, 1.000000000000000000, 0.9659258262890683122, 1.000000000000000000, 0.9659258262890683122, 1.000000000000000000, 0.9659258262890683122, 1.000000000000000000, 0.9659258262890683122, 1.000000000000000000, 0.9659258262890683122, 1.000000000000000000, 0.9659258262890683122, 1.000000000000000000, 0.9659258262890683122, 1.000000000000000000, 0.9659258262890683122, 1.000000000000000000, 0.9659258262890683122, 1.000000000000000000, 0.9659258262890683122, 1.000000000000000000, 0.9659258262890683122, 1.000000000000000000, 0.9659258262890683122, 1.000000000000000000, 0.9659258262890683122, 1.000000000000000000, 0.9659258262890683122, 1.000000000000000000, 0.9659258262890683122, 1.000000000000000000, 0.9659258262890683122, 1.000000000000000000, 0.9659258262890683122, 1.000000000000000000, 0.9659258262890683122, 1.000000000000000000, 0.9659258262890683122, 1.000000000000000000, 0.9659258262890683122, 1.000000000000000000, 0.9659258262890683122, 1.000000000000000000, 0.9659258262890683122, 1.000000000000000000, 0.9659258262890683122, 1.000000000000000000, 0.9659258262890683122, 1.000000000000000000, 0.9659258262890683122, 1.000000000000000000, 0.9659258262890683122, 1.000000000000000000, 0.9659258262890683122, 1.000000000000000000, 0.9659258262890683122, 1.000000000000000000, 0.9659258262890683122, 1.000000000000000000, 0.9659258262890683122, 1.000000000000000000, 0.9659258262890683122, 1.000000000000000000, 0.9659258262890683122, 1.000000000000000000, 0.9659258262890683122, 1.000000000000000000, 0.9659258262890683122, 1.000000000000000000, 0.9659258262890683122, 1.000000000000000000, 0.9659258262890683122, 1.000000000000000000, 0.9659258262890683122, 1.000000000000000000, 0.9659258262890683122, 1.000000000000000000, 0.9659258262890683122, 1.000000000000000000, 0.9659258262890683122, 1.000000000000000000, 0.9659258262890683122, 1.000000000000000000, 0.9659258262890683122, 1.000000000000000000, 0.9659258262890683122, 1.000000000000000000, 0.9659258262890683122, 1.000000000000000000, 0.9659258262890683122, 1.000000000000000000, 0.9659258262890683122, 1.000000000000000000, 0.9659258262890683122, 1.000000000000000000, 0.9659258262890683122, 1.000000000000000000, 0.9659258262890683122, 1.000000000000000000, 0.9659258262890683122, 1.000000000000000000, 0.9659258262890683122, 1.000000000000000000, 0.9659258262890683122, 1.000000000000000000, 0.9659258262890683122, 1.000000000000000000, 0.9659258262890683122, 1.000000000000000000, 0.9659258262890683122, 1.000000000000000000, 0.9659258262890683122, 1.000000000000000000, 0.9659258262890683122, 1.000000000000000000, 0.9659258262890683122, 1.000000000000000000, 0.9659258262890683122, 1.000000000000000000) ) ) 
 REPRESENTATION_ITEM ( '' )  SURFACE ( )  );
#13897=CARTESIAN_POINT ( 'NONE',  ( -19.05341960407611168, -5.049401038298163336, 66.45724293864769550 ) ) ;
#13898=CARTESIAN_POINT ( 'NONE',  ( -14.29746914071049879, 8.314922557960819915, 70.83224293864770971 ) ) ;
#13899=CARTESIAN_POINT ( 'NONE',  ( -9.474510206698964154, 16.51473224551069663, 30.41557627198102054 ) ) ;
#13900=CARTESIAN_POINT ( 'NONE',  ( -17.19557940625944070, -5.324144293544740947, 20.93786341900914394 ) ) ;
#13901=CARTESIAN_POINT ( 'NONE',  ( -4.379528057220328563, 16.55341960407611168, 45.20724293864769550 ) ) ;
#13902=CARTESIAN_POINT ( 'NONE',  ( -13.97604488694527625, -13.89961937509977652, 86.87390960531436690 ) ) ;
#13904=CARTESIAN_POINT ( 'NONE',  ( 16.46253265017146816, 9.564922557961045513, 51.66775706135233293 ) ) ;
#13905=CARTESIAN_POINT ( 'NONE',  ( -14.29746914071037622, -8.314922557961029526, 64.16775706135234714 ) ) ;
#13906=CARTESIAN_POINT ( 'NONE',  ( -21.53943276465977519, 0.05219959533907696930, 81.24890960531436690 ) ) ;
#13907=CARTESIAN_POINT ( 'NONE',  ( -13.97604488694547697, 13.89961937509957934, 33.12609039468566863 ) ) ;
#13908=CARTESIAN_POINT ( 'NONE',  ( 13.89961937509977652, -13.97604488694527269, 88.12390960531438111 ) ) ;
#13910=CARTESIAN_POINT ( 'NONE',  ( 5.719274019375991003, -21.55341960407610458, 22.70724293864769194 ) ) ;
#13911=CARTESIAN_POINT ( 'NONE',  ( 0.05219959533909260263, 19.03943276465977164, 64.99890960531436690 ) ) ;
#13912=CARTESIAN_POINT ( 'NONE',  ( -15.72974639402176322, -15.80617190586768395, 54.37609039468568994 ) ) ;
#13913=CARTESIAN_POINT ( 'NONE',  ( 19.02544592524343514, -5.153800228976328945, 28.54057627198102409 ) ) ;
#13914=CARTESIAN_POINT ( 'NONE',  ( -18.62759615963270932, 10.81492255796079327, 115.8322429386477097 ) ) ;
#13915=CARTESIAN_POINT ( 'NONE',  ( -13.97604488694527625, -13.89961937509977652, 91.87390960531432427 ) ) ;
#13916=VERTEX_POINT ( 'NONE', #88106 ) ;
#13917=CARTESIAN_POINT ( 'NONE',  ( -18.67979575497193778, 10.72451020669871902, 43.33442372801901143 ) ) ;
#13919=CARTESIAN_POINT ( 'NONE',  ( 5.049401038298161559, -19.05341960407611168, 97.70724293864766707 ) ) ;
#13920=CARTESIAN_POINT ( 'NONE',  ( 21.55341960407610458, 5.719274019375980345, 113.9572429386477239 ) ) ;
#13921=CARTESIAN_POINT ( 'NONE',  ( 13.89961937509977652, -13.97604488694527269, 43.12390960531434558 ) ) ;
#13922=CARTESIAN_POINT ( 'NONE',  ( 12.14591786802327356, -12.06949235617739191, 25.62609039468567929 ) ) ;
#13924=CARTESIAN_POINT ( 'NONE',  ( 18.67979575497194134, -10.72451020669871369, 105.8344237280190328 ) ) ;
#13925=CARTESIAN_POINT ( 'NONE',  ( 13.89961937509977652, -13.97604488694527269, 33.12390960531434558 ) ) ;
#13926=CARTESIAN_POINT ( 'NONE',  ( 21.53943276465977519, 0.05219959533937863772, 96.25109039468568994 ) ) ;
#13927=CARTESIAN_POINT ( 'NONE',  ( 5.153800228976335163, 19.02544592524342804, 94.79057627198103830 ) ) ;
#13928=CARTESIAN_POINT ( 'NONE',  ( 5.823673210054444382, -21.52544592524334988, 55.20942372801902565 ) ) ;
#13930=CARTESIAN_POINT ( 'NONE',  ( 5.153800228976335163, 19.02544592524342804, 94.79057627198103830 ) ) ;
#13932=CARTESIAN_POINT ( 'NONE',  ( 0.05219959533934541429, -16.53943276465976808, 40.00109039468567573 ) ) ;
#13933=CARTESIAN_POINT ( 'NONE',  ( -8.314922557961024197, 14.29746914071037800, 72.91775706135234714 ) ) ;
#13934=CARTESIAN_POINT ( 'NONE',  ( 21.52544592524334988, 5.823673210054432836, 56.45942372801902565 ) ) ;
#13935=CARTESIAN_POINT ( 'NONE',  ( -18.67979575497193778, 10.72451020669871902, 83.33442372801903275 ) ) ;
#13936=CARTESIAN_POINT ( 'NONE',  ( 18.22780087662123805, -5.499999999999989342, 53.51763182126895657 ) ) ;
#13937=CARTESIAN_POINT ( 'NONE',  ( 16.55341960407618274, -4.379528057220086978, 31.04275706135234714 ) ) ;
#13938=CARTESIAN_POINT ( 'NONE',  ( -16.46253265017160317, 9.564922557960807481, 70.83224293864770971 ) ) ;
#13939=CARTESIAN_POINT ( 'NONE',  ( 16.46253265017160672, -9.564922557960803928, 93.33224293864769550 ) ) ;
#13941=CARTESIAN_POINT ( 'NONE',  ( -16.52544592524342804, 4.483927247898546575, 116.0405762719810383 ) ) ;
#13942=CARTESIAN_POINT ( 'NONE',  ( -18.62759615963270932, 10.81492255796079327, 30.83224293864770260 ) ) ;
#13943=CARTESIAN_POINT ( 'NONE',  ( -16.55341960407617563, 4.379528057220093196, 98.54275706135234714 ) ) ;
#13944=CARTESIAN_POINT ( 'NONE',  ( -0.05219959533910754901, -16.53943276465976808, 67.49890960531436690 ) ) ;
#13945=CARTESIAN_POINT ( 'NONE',  ( -5.049401038298153566, 19.05341960407611168, 65.20724293864765286 ) ) ;
#13946=CARTESIAN_POINT ( 'NONE',  ( -10.72451020669870658, -18.67979575497194134, 94.58442372801901854 ) ) ;
#13948=CARTESIAN_POINT ( 'NONE',  ( -5.049401038297874678, -19.05341960407617918, 104.7927570613523471 ) ) ;
#13949=CARTESIAN_POINT ( 'NONE',  ( -4.379528057220328563, 16.55341960407611168, 80.20724293864769550 ) ) ;
#13950=CARTESIAN_POINT ( 'NONE',  ( -0.05219959533937732626, 21.53943276465977519, 22.50109039468567573 ) ) ;
#13951=CARTESIAN_POINT ( 'NONE',  ( -21.53943276465977519, 0.05219959533907696930, 61.24890960531435979 ) ) ;
#13952=CARTESIAN_POINT ( 'NONE',  ( 0.05219959533936267826, -19.03943276465977164, 40.00109039468566152 ) ) ;
#13954=CARTESIAN_POINT ( 'NONE',  ( -19.03943276465977164, 0.05219959533909376836, 86.24890960531436690 ) ) ;
#13955=CARTESIAN_POINT ( 'NONE',  ( -4.379528057220328563, 16.55341960407611168, 55.20724293864770260 ) ) ;
#13956=CARTESIAN_POINT ( 'NONE',  ( -8.314922557960811034, -14.29746914071050412, 37.08224293864768129 ) ) ;
#13957=CARTESIAN_POINT ( 'NONE',  ( -16.53943276465976808, -0.05219959533934237506, 103.7510903946857042 ) ) ;
#13958=CARTESIAN_POINT ( 'NONE',  ( 16.51473224551083163, -9.474510206698727899, 55.83442372801899722 ) ) ;
#13960=CARTESIAN_POINT ( 'NONE',  ( -5.049401038298153566, 19.05341960407611168, 100.2072429386476955 ) ) ;
#13962=CARTESIAN_POINT ( 'NONE',  ( -16.53943276465976808, 0.05219959533911058130, 81.24890960531436690 ) ) ;
#13963=CARTESIAN_POINT ( 'NONE',  ( -5.049401038297874678, -19.05341960407617918, 49.79275706135231871 ) ) ;
#13964=CARTESIAN_POINT ( 'NONE',  ( 16.46253265017160672, -9.564922557960803928, 33.33224293864770260 ) ) ;
#13965=CARTESIAN_POINT ( 'NONE',  ( 0.05219959533907565091, 21.53943276465977519, 39.99890960531436690 ) ) ;
#13966=CARTESIAN_POINT ( 'NONE',  ( 21.53943276465977519, -0.05219959533907433946, 63.74890960531435979 ) ) ;
#13967=CARTESIAN_POINT ( 'NONE',  ( -4.379528057220328563, 16.55341960407611168, 115.2072429386476955 ) ) ;
#13968=CARTESIAN_POINT ( 'NONE',  ( -14.34966873604972548, 8.224510206698743886, 48.33442372801902565 ) ) ;
#13969=CARTESIAN_POINT ( 'NONE',  ( 19.03943276465977164, -0.05219959533909143690, 48.74890960531435979 ) ) ;
#13970=CARTESIAN_POINT ( 'NONE',  ( -5.823673210054431948, 21.52544592524334988, 42.70942372801901854 ) ) ;
#13971=CARTESIAN_POINT ( 'NONE',  ( -16.53943276465976808, 0.05219959533911058130, 86.24890960531436690 ) ) ;
#13974=CARTESIAN_POINT ( 'NONE',  ( -5.823673210054116645, -21.52544592524344225, 32.29057627198102409 ) ) ;
#13977=CARTESIAN_POINT ( 'NONE',  ( -16.55341960407617563, 4.379528057220093196, 38.54275706135234714 ) ) ;
#13978=CARTESIAN_POINT ( 'NONE',  ( 14.34966873604960469, 8.224510206698951720, 44.16557627198103120 ) ) ;
#13979=CARTESIAN_POINT ( 'NONE',  ( -10.72451020669898014, 18.67979575497178502, 70.41557627198102409 ) ) ;
#13981=CARTESIAN_POINT ( 'NONE',  ( 5.719274019375991003, -21.55341960407610458, 57.70724293864770260 ) ) ;
#13983=CARTESIAN_POINT ( 'NONE',  ( 19.02544592524343514, -5.153800228976328945, 43.54057627198103120 ) ) ;
#13984=CARTESIAN_POINT ( 'NONE',  ( -16.51473224551069308, -9.474510206698971260, 101.6655762719810241 ) ) ;
#13985=CARTESIAN_POINT ( 'NONE',  ( -19.03943276465977164, 0.05219959533909376836, 51.24890960531436690 ) ) ;
#13986=CARTESIAN_POINT ( 'NONE',  ( -0.05219959533910754901, -16.53943276465976808, 112.4989096053143669 ) ) ;
#13988=CARTESIAN_POINT ( 'NONE',  ( -13.89961937509977652, 13.97604488694528158, 115.6239096053143669 ) ) ;
#13990=CARTESIAN_POINT ( 'NONE',  ( 4.379528057220092307, 16.55341960407617563, 72.29275706135236135 ) ) ;
#13991=CARTESIAN_POINT ( 'NONE',  ( -10.72451020669898014, 18.67979575497178502, 110.4155762719810383 ) ) ;
#13992=CARTESIAN_POINT ( 'NONE',  ( -9.564922557960796823, -16.46253265017161027, 62.08224293864769550 ) ) ;
#13993=CARTESIAN_POINT ( 'NONE',  ( 5.823673210054444382, -21.52544592524334988, 45.20942372801901854 ) ) ;
#13994=CARTESIAN_POINT ( 'NONE',  ( -16.46253265017160317, 9.564922557960807481, 80.83224293864769550 ) ) ;
#13995=CARTESIAN_POINT ( 'NONE',  ( -16.46253265017160317, 9.564922557960807481, 115.8322429386477097 ) ) ;
#13997=CARTESIAN_POINT ( 'NONE',  ( -18.67979575497193778, 10.72451020669871902, 28.33442372801902209 ) ) ;
#13998=CARTESIAN_POINT ( 'NONE',  ( 13.97604488694527802, 13.89961937509977652, 109.3739096053143669 ) ) ;
#13999=CARTESIAN_POINT ( 'NONE',  ( -5.153800228976607833, 19.02544592524334988, 87.70942372801897591 ) ) ;
#14000=CARTESIAN_POINT ( 'NONE',  ( 19.02544592524334988, 5.153800228976608722, 46.45942372801899012 ) ) ;
#14001=CARTESIAN_POINT ( 'NONE',  ( -21.55341960407610458, -5.719274019375992779, 101.4572429386476955 ) ) ;
#14002=CARTESIAN_POINT ( 'NONE',  ( -19.02544592524334988, -5.153800228976617603, 28.95942372801900433 ) ) ;
#14003=CARTESIAN_POINT ( 'NONE',  ( -0.05219959533936034679, 19.03943276465977164, 32.50109039468566863 ) ) ;
#14004=CARTESIAN_POINT ( 'NONE',  ( -14.34966873604972548, 8.224510206698743886, 93.33442372801901854 ) ) ;
#14006=CARTESIAN_POINT ( 'NONE',  ( 16.46253265017160672, -9.564922557960803928, 58.33224293864769550 ) ) ;
#14007=CARTESIAN_POINT ( 'NONE',  ( 21.55341960407619695, -5.719274019375665929, 66.04275706135236135 ) ) ;
#14008=CARTESIAN_POINT ( 'NONE',  ( 10.72451020669871369, 18.67979575497193778, 77.08442372801901854 ) ) ;
#14010=CARTESIAN_POINT ( 'NONE',  ( -9.564922557960796823, -16.46253265017161027, 82.08224293864768129 ) ) ;
#14011=CARTESIAN_POINT ( 'NONE',  ( 18.62759615963255655, 10.81492255796105972, 61.66775706135235424 ) ) ;
#14012=CARTESIAN_POINT ( 'NONE',  ( 5.153800228976615827, -19.02544592524334988, 105.2094237280190185 ) ) ;
#14013=CARTESIAN_POINT ( 'NONE',  ( 19.03943276465977164, -0.05219959533909143690, 63.74890960531435979 ) ) ;
#14014=CARTESIAN_POINT ( 'NONE',  ( -5.049401038298153566, 19.05341960407611168, 95.20724293864770971 ) ) ;
#14015=CARTESIAN_POINT ( 'NONE',  ( -13.89961937509977652, 13.97604488694528158, 85.62390960531433848 ) ) ;
#14017=CARTESIAN_POINT ( 'NONE',  ( -9.474510206698964154, 16.51473224551069663, 70.41557627198102409 ) ) ;
#14018=CARTESIAN_POINT ( 'NONE',  ( 18.67979575497178502, 10.72451020669898547, 94.16557627198103830 ) ) ;
#14019=CARTESIAN_POINT ( 'NONE',  ( -12.06949235617739369, -12.14591786802326823, 89.37609039468568994 ) ) ;
#14021=CARTESIAN_POINT ( 'NONE',  ( -19.03943276465977164, -0.05219959533935918106, 38.75109039468566152 ) ) ;
#14022=CARTESIAN_POINT ( 'NONE',  ( 9.474510206698971260, -16.51473224551069308, 77.91557627198103830 ) ) ;
#14023=CARTESIAN_POINT ( 'NONE',  ( 8.224510206698953496, -14.34966873604960469, 77.91557627198102409 ) ) ;
#14024=CARTESIAN_POINT ( 'NONE',  ( -8.224510206698948167, 14.34966873604960824, 110.4155762719810383 ) ) ;
#14025=CARTESIAN_POINT ( 'NONE',  ( -19.03943276465977164, 0.05219959533909376836, 116.2489096053143669 ) ) ;
#14026=VERTEX_POINT ( 'NONE', #106255 ) ;
#14027=CARTESIAN_POINT ( 'NONE',  ( -9.474510206698964154, 16.51473224551069663, 105.4155762719810383 ) ) ;
#14028=CARTESIAN_POINT ( 'NONE',  ( -18.22780087662123094, -5.499999999999984901, 81.48459894673892734 ) ) ;
#14029=CARTESIAN_POINT ( 'NONE',  ( 16.51473224551083163, -9.474510206698727899, 25.83442372801900078 ) ) ;
#14030=CARTESIAN_POINT ( 'NONE',  ( -12.06949235617739369, -12.14591786802326823, 89.37609039468568994 ) ) ;
#14031=CARTESIAN_POINT ( 'NONE',  ( 19.05341960407611168, 5.049401038298154454, 78.95724293864769550 ) ) ;
#14032=CARTESIAN_POINT ( 'NONE',  ( -10.81492255796105439, 18.62759615963255655, 57.91775706135234714 ) ) ;
#14033=CARTESIAN_POINT ( 'NONE',  ( 10.81492255796078972, 18.62759615963270932, 34.58224293864770260 ) ) ;
#14034=CARTESIAN_POINT ( 'NONE',  ( -10.72451020669870658, -18.67979575497194134, 24.58442372801901499 ) ) ;
#14035=CARTESIAN_POINT ( 'NONE',  ( -10.81492255796078084, -18.62759615963271287, 72.08224293864769550 ) ) ;
#14036=CARTESIAN_POINT ( 'NONE',  ( -0.05219959533910754901, -16.53943276465976808, 97.49890960531436690 ) ) ;
#14037=CARTESIAN_POINT ( 'NONE',  ( 19.03943276465977164, 0.05219959533936151252, 61.25109039468566863 ) ) ;
#14038=CARTESIAN_POINT ( 'NONE',  ( 19.02544592524343514, -5.153800228976328945, 33.54057627198102409 ) ) ;
#14039=CARTESIAN_POINT ( 'NONE',  ( 19.02544592524343514, -5.153800228976328945, 78.54057627198099567 ) ) ;
#14040=CARTESIAN_POINT ( 'NONE',  ( 19.05341960407611168, 5.049401038298154454, 78.95724293864769550 ) ) ;
#14042=CARTESIAN_POINT ( 'NONE',  ( -0.05219959533910754901, -16.53943276465976808, 107.4989096053143669 ) ) ;
#14044=CARTESIAN_POINT ( 'NONE',  ( 16.52544592524342804, -4.483927247898539470, 33.54057627198102409 ) ) ;
#14045=CARTESIAN_POINT ( 'NONE',  ( -16.52544592524335698, -4.483927247898792601, 28.95942372801902209 ) ) ;
#14046=CARTESIAN_POINT ( 'NONE',  ( -5.719274019375665041, -21.55341960407619695, 94.79275706135234714 ) ) ;
#14047=CARTESIAN_POINT ( 'NONE',  ( -16.51473224551069308, -9.474510206698971260, 106.6655762719810383 ) ) ;
#14048=CARTESIAN_POINT ( 'NONE',  ( -10.72451020669870658, -18.67979575497194134, 19.58442372801901143 ) ) ;
#14049=CARTESIAN_POINT ( 'NONE',  ( 9.474510206698971260, -16.51473224551069308, 37.91557627198102409 ) ) ;
#14050=CARTESIAN_POINT ( 'NONE',  ( 8.314922557961029526, -14.29746914071037800, 40.41775706135234714 ) ) ;
#14051=CARTESIAN_POINT ( 'NONE',  ( 9.564922557961047289, -16.46253265017146816, 105.4177570613523471 ) ) ;
#14052=CARTESIAN_POINT ( 'NONE',  ( -13.97604488694527625, -13.89961937509977652, 31.87390960531435979 ) ) ;
#14054=CARTESIAN_POINT ( 'NONE',  ( -16.52544592524342804, 4.483927247898546575, 101.0405762719810383 ) ) ;
#14055=CARTESIAN_POINT ( 'NONE',  ( 5.823673210054125526, 21.52544592524343514, 99.79057627198103830 ) ) ;
#14056=CARTESIAN_POINT ( 'NONE',  ( -16.51473224551082808, 9.474510206698731452, 68.33442372801900433 ) ) ;
#14057=CARTESIAN_POINT ( 'NONE',  ( -18.09867054820433907, -5.499999999999827693, 63.98393025253586330 ) ) ;
#14058=CARTESIAN_POINT ( 'NONE',  ( -10.81492255796078084, -18.62759615963271287, 112.0822429386477097 ) ) ;
#14060=CARTESIAN_POINT ( 'NONE',  ( 16.51473224551069308, 9.474510206698969483, 94.16557627198103830 ) ) ;
#14061=CARTESIAN_POINT ( 'NONE',  ( 17.50000000000000000, -5.500000000000000888, 120.0000000000000142 ) ) ;
#14063=CARTESIAN_POINT ( 'NONE',  ( -9.474510206698964154, 16.51473224551069663, 80.41557627198103830 ) ) ;
#14064=CARTESIAN_POINT ( 'NONE',  ( -10.81492255796105439, 18.62759615963255655, 37.91775706135235424 ) ) ;
#14065=CARTESIAN_POINT ( 'NONE',  ( 0.05219959533910956823, 16.53943276465976808, 74.99890960531435269 ) ) ;
#14066=CARTESIAN_POINT ( 'NONE',  ( -16.51473224551069308, -9.474510206698971260, 76.66557627198103830 ) ) ;
#14067=CARTESIAN_POINT ( 'NONE',  ( -8.314922557961024197, 14.29746914071037800, 52.91775706135235424 ) ) ;
#14068=CARTESIAN_POINT ( 'NONE',  ( -5.153800228976607833, 19.02544592524334988, 57.70942372801899012 ) ) ;
#14069=CARTESIAN_POINT ( 'NONE',  ( 21.52544592524334988, 5.823673210054432836, 61.45942372801901854 ) ) ;
#14070=CARTESIAN_POINT ( 'NONE',  ( -8.314922557961024197, 14.29746914071037800, 27.91775706135234358 ) ) ;
#14071=CARTESIAN_POINT ( 'NONE',  ( 16.46253265017160672, -9.564922557960803928, 73.33224293864769550 ) ) ;
#14072=CARTESIAN_POINT ( 'NONE',  ( -19.03943276465977164, -0.05219959533935918106, 93.75109039468566152 ) ) ;
#14073=CARTESIAN_POINT ( 'NONE',  ( 12.06949235617739724, 12.14591786802326823, 61.87609039468568284 ) ) ;
#14074=CARTESIAN_POINT ( 'NONE',  ( -10.72451020669870658, -18.67979575497194134, 99.58442372801900433 ) ) ;
#14076=CARTESIAN_POINT ( 'NONE',  ( -19.02544592524334988, -5.153800228976617603, 83.95942372801901854 ) ) ;
#14077=CARTESIAN_POINT ( 'NONE',  ( 13.89961937509977652, -13.97604488694527269, 48.12390960531435979 ) ) ;
#14078=CARTESIAN_POINT ( 'NONE',  ( -5.719274019375978568, 21.55341960407610458, 70.20724293864769550 ) ) ;
#14079=CARTESIAN_POINT ( 'NONE',  ( -4.483927247898539470, -16.52544592524342804, 72.29057627198102409 ) ) ;
#14080=CARTESIAN_POINT ( 'NONE',  ( -19.05341960407617563, 5.049401038297882671, 78.54275706135233293 ) ) ;
#14081=CARTESIAN_POINT ( 'NONE',  ( 17.05116617787822975, -6.768360034955865245, 61.15675553259200115 ) ) ;
#14082=CARTESIAN_POINT ( 'NONE',  ( -9.474510206698720793, -16.51473224551083518, 39.58442372801899722 ) ) ;
#14083=CARTESIAN_POINT ( 'NONE',  ( 14.29746914071037800, 8.314922557961029526, 106.6677570613523756 ) ) ;
#14084=CARTESIAN_POINT ( 'NONE',  ( -12.14591786802309592, -12.06949235617757132, 61.87390960531436690 ) ) ;
#14085=CARTESIAN_POINT ( 'NONE',  ( 15.72974639402176855, 15.80617190586768217, 96.87609039468568994 ) ) ;
#14087=CARTESIAN_POINT ( 'NONE',  ( -18.62759615963270932, 10.81492255796079327, 110.8322429386476955 ) ) ;
#14088=CARTESIAN_POINT ( 'NONE',  ( 5.153800228976335163, 19.02544592524342804, 69.79057627198103830 ) ) ;
#14089=CARTESIAN_POINT ( 'NONE',  ( 21.52544592524334988, 5.823673210054432836, 86.45942372801901854 ) ) ;
#14090=CARTESIAN_POINT ( 'NONE',  ( -16.51473224551069308, -9.474510206698971260, 61.66557627198103120 ) ) ;
#14091=CARTESIAN_POINT ( 'NONE',  ( -19.05341960407611168, -5.049401038298163336, 26.45724293864769550 ) ) ;
#14092=CARTESIAN_POINT ( 'NONE',  ( 0.05219959533907565091, 21.53943276465977519, 34.99890960531435979 ) ) ;
#14093=CARTESIAN_POINT ( 'NONE',  ( 14.29746914071049879, -8.314922557960816363, 73.33224293864769550 ) ) ;
#14094=CARTESIAN_POINT ( 'NONE',  ( 13.89961937509977652, -13.97604488694527269, 43.12390960531434558 ) ) ;
#14095=CARTESIAN_POINT ( 'NONE',  ( -14.29746914071049879, 8.314922557960819915, 100.8322429386477097 ) ) ;
#14096=CARTESIAN_POINT ( 'NONE',  ( -21.53943276465977519, 0.05219959533907696930, 106.2489096053143811 ) ) ;
#14097=CARTESIAN_POINT ( 'NONE',  ( 18.67979575497194134, -10.72451020669871369, 50.83442372801901143 ) ) ;
#14098=CARTESIAN_POINT ( 'NONE',  ( -16.46253265017160317, 9.564922557960807481, 35.83224293864768839 ) ) ;
#14099=CARTESIAN_POINT ( 'NONE',  ( 12.14591786802327356, -12.06949235617739191, 50.62609039468568994 ) ) ;
#14100=CARTESIAN_POINT ( 'NONE',  ( -5.719274019375978568, 21.55341960407610458, 105.2072429386477097 ) ) ;
#14101=CARTESIAN_POINT ( 'NONE',  ( -18.62759615963270932, 10.81492255796079327, 100.8322429386477097 ) ) ;
#14102=CARTESIAN_POINT ( 'NONE',  ( 13.89961937509957401, 13.97604488694547697, 21.87609039468566152 ) ) ;
#14103=CARTESIAN_POINT ( 'NONE',  ( -5.049401038298153566, 19.05341960407611168, 50.20724293864770260 ) ) ;
#14104=CARTESIAN_POINT ( 'NONE',  ( -9.564922557960796823, -16.46253265017161027, 112.0822429386476955 ) ) ;
#14105=CARTESIAN_POINT ( 'NONE',  ( -15.80617190586768217, 15.72974639402176855, 58.12609039468568994 ) ) ;
#14107=CARTESIAN_POINT ( 'NONE',  ( 0.05219959533907565091, 21.53943276465977519, 39.99890960531436690 ) ) ;
#14108=CARTESIAN_POINT ( 'NONE',  ( 4.483927247898545687, 16.52544592524342804, 24.79057627198103120 ) ) ;
#14109=CARTESIAN_POINT ( 'NONE',  ( 10.72451020669871369, 18.67979575497193778, 62.08442372801901143 ) ) ;
#14110=CARTESIAN_POINT ( 'NONE',  ( 10.72451020669871369, 18.67979575497193778, 97.08442372801904696 ) ) ;
#14111=CARTESIAN_POINT ( 'NONE',  ( 9.564922557961047289, -16.46253265017146816, 45.41775706135232582 ) ) ;
#14112=CARTESIAN_POINT ( 'NONE',  ( 8.314922557961029526, -14.29746914071037800, 105.4177570613523613 ) ) ;
#14113=CARTESIAN_POINT ( 'NONE',  ( -18.62759615963255300, -10.81492255796106328, 54.16775706135235424 ) ) ;
#14114=CARTESIAN_POINT ( 'NONE',  ( 9.474510206698971260, -16.51473224551069308, 62.91557627198102409 ) ) ;
#14115=CARTESIAN_POINT ( 'NONE',  ( 5.823673210054444382, -21.52544592524334988, 110.2094237280190185 ) ) ;
#14116=CARTESIAN_POINT ( 'NONE',  ( -9.474510206698964154, 16.51473224551069663, 115.4155762719810241 ) ) ;
#14117=CARTESIAN_POINT ( 'NONE',  ( 15.72974639402176855, 15.80617190586768217, 21.87609039468567573 ) ) ;
#14118=CARTESIAN_POINT ( 'NONE',  ( 21.52544592524344225, -5.823673210054117533, 73.54057627198102409 ) ) ;
#14119=CARTESIAN_POINT ( 'NONE',  ( -12.06949235617739369, -12.14591786802326823, 44.37609039468567573 ) ) ;
#14121=CARTESIAN_POINT ( 'NONE',  ( -15.72974639402197994, 15.80617190586746368, 80.62390960531438111 ) ) ;
#14122=CARTESIAN_POINT ( 'NONE',  ( -16.55341960407617563, 4.379528057220093196, 68.54275706135234714 ) ) ;
#14123=CARTESIAN_POINT ( 'NONE',  ( 12.06949235617757843, -12.14591786802309237, 78.12390960531436690 ) ) ;
#14125=CARTESIAN_POINT ( 'NONE',  ( -19.02544592524334988, -5.153800228976617603, 103.9594237280190043 ) ) ;
#14126=CARTESIAN_POINT ( 'NONE',  ( -21.53943276465977519, 0.05219959533907696930, 41.24890960531435269 ) ) ;
#14127=CARTESIAN_POINT ( 'NONE',  ( -9.474510206698964154, 16.51473224551069663, 95.41557627198102409 ) ) ;
#14128=CARTESIAN_POINT ( 'NONE',  ( 14.34966873604972726, -8.224510206698740333, 35.83442372801901143 ) ) ;
#14129=CARTESIAN_POINT ( 'NONE',  ( 15.80617190586746368, 15.72974639402197994, 109.3739096053143811 ) ) ;
#14130=CARTESIAN_POINT ( 'NONE',  ( 18.67979575497178502, 10.72451020669898547, 29.16557627198103120 ) ) ;
#14131=CARTESIAN_POINT ( 'NONE',  ( 16.55341960407618274, -4.379528057220086978, 71.04275706135234714 ) ) ;
#14132=CARTESIAN_POINT ( 'NONE',  ( -19.05341960407611168, -5.049401038298163336, 91.45724293864766707 ) ) ;
#14133=CARTESIAN_POINT ( 'NONE',  ( 5.719274019375673035, 21.55341960407619339, 52.29275706135236135 ) ) ;
#14134=CARTESIAN_POINT ( 'NONE',  ( 19.03943276465977164, -0.05219959533909143690, 33.74890960531435979 ) ) ;
#14135=CARTESIAN_POINT ( 'NONE',  ( -18.62759615963270932, 10.81492255796079327, 30.83224293864770260 ) ) ;
#14137=CARTESIAN_POINT ( 'NONE',  ( -5.153800228976607833, 19.02544592524334988, 42.70942372801901143 ) ) ;
#14138=CARTESIAN_POINT ( 'NONE',  ( 0.05219959533934541429, -16.53943276465976808, 55.00109039468568284 ) ) ;
#14139=CARTESIAN_POINT ( 'NONE',  ( 19.05341960407611168, 5.049401038298154454, 103.9572429386476671 ) ) ;
#14140=CARTESIAN_POINT ( 'NONE',  ( -5.823673210054116645, -21.52544592524344225, 102.2905762719810383 ) ) ;
#14141=CARTESIAN_POINT ( 'NONE',  ( 9.564922557960805705, 16.46253265017160317, 69.58224293864770971 ) ) ;
#14144=CARTESIAN_POINT ( 'NONE',  ( -12.06949235617756955, 12.14591786802309770, 75.62390960531439532 ) ) ;
#14145=CARTESIAN_POINT ( 'NONE',  ( 21.52544592524344225, -5.823673210054117533, 38.54057627198103120 ) ) ;
#14146=CARTESIAN_POINT ( 'NONE',  ( -17.13100169013300444, 6.664070546373152659, 35.76789835699850784 ) ) ;
#14147=CARTESIAN_POINT ( 'NONE',  ( 16.55341960407618274, -4.379528057220086978, 66.04275706135236135 ) ) ;
#14148=CARTESIAN_POINT ( 'NONE',  ( 15.80617190586769283, -15.72974639402175789, 25.62609039468567929 ) ) ;
#14149=CARTESIAN_POINT ( 'NONE',  ( 19.02544592524334988, 5.153800228976608722, 76.45942372801897591 ) ) ;
#14150=CARTESIAN_POINT ( 'NONE',  ( -5.153800228976328057, -19.02544592524343514, 42.29057627198101699 ) ) ;
#14151=CARTESIAN_POINT ( 'NONE',  ( 18.62759615963271287, -10.81492255796078972, 73.33224293864769550 ) ) ;
#14152=CARTESIAN_POINT ( 'NONE',  ( 19.02544592524343514, -5.153800228976328945, 113.5405762719810241 ) ) ;
#14153=CARTESIAN_POINT ( 'NONE',  ( -10.72451020669870658, -18.67979575497194134, 89.58442372801901854 ) ) ;
#14154=CARTESIAN_POINT ( 'NONE',  ( 19.05341960407611168, 5.049401038298154454, 68.95724293864769550 ) ) ;
#14155=CARTESIAN_POINT ( 'NONE',  ( -12.06949235617739369, -12.14591786802326823, 44.37609039468567573 ) ) ;
#14156=CARTESIAN_POINT ( 'NONE',  ( 19.02544592524343514, -5.153800228976328945, 58.54057627198102409 ) ) ;
#14157=CARTESIAN_POINT ( 'NONE',  ( 18.67979575497194134, -10.72451020669871369, 75.83442372801900433 ) ) ;
#14158=CARTESIAN_POINT ( 'NONE',  ( -16.46253265017146816, -9.564922557961047289, 34.16775706135233293 ) ) ;
#14159=CARTESIAN_POINT ( 'NONE',  ( -0.05219959533936034679, 19.03943276465977164, 52.50109039468566863 ) ) ;
#14160=CARTESIAN_POINT ( 'NONE',  ( 21.55341960407619695, -5.719274019375665929, 56.04275706135235424 ) ) ;
#14161=CARTESIAN_POINT ( 'NONE',  ( -18.39639308325437383, -5.500000000000040856, 46.48252246182197922 ) ) ;
#14162=CARTESIAN_POINT ( 'NONE',  ( 19.03943276465977164, 0.05219959533936151252, 41.25109039468566152 ) ) ;
#14163=CARTESIAN_POINT ( 'NONE',  ( -13.89961937509977652, 13.97604488694528158, 105.6239096053143527 ) ) ;
#14164=CARTESIAN_POINT ( 'NONE',  ( 16.46253265017160672, -9.564922557960803928, 68.33224293864770971 ) ) ;
#14165=CARTESIAN_POINT ( 'NONE',  ( -12.06949235617756955, 12.14591786802309770, 30.62390960531436335 ) ) ;
#14166=CARTESIAN_POINT ( 'NONE',  ( 21.55341960407610458, 5.719274019375980345, 28.95724293864769905 ) ) ;
#14167=CARTESIAN_POINT ( 'NONE',  ( -21.55341960407619339, 5.719274019375674811, 103.5427570613523613 ) ) ;
#14169=CARTESIAN_POINT ( 'NONE',  ( 16.19135201231368981, 7.376712067591808086, 57.68680854052030327 ) ) ;
#14170=CARTESIAN_POINT ( 'NONE',  ( -15.72974639402176322, -15.80617190586768395, 104.3760903946856899 ) ) ;
#14172=CARTESIAN_POINT ( 'NONE',  ( 16.46253265017160672, -9.564922557960803928, 23.33224293864769194 ) ) ;
#14173=CARTESIAN_POINT ( 'NONE',  ( 0.05219959533909260263, 19.03943276465977164, 114.9989096053143669 ) ) ;
#14175=CARTESIAN_POINT ( 'NONE',  ( 8.224510206698742110, 14.34966873604972548, 52.08442372801901854 ) ) ;
#14176=CARTESIAN_POINT ( 'NONE',  ( -21.55341960407610458, -5.719274019375992779, 71.45724293864769550 ) ) ;
#14177=CARTESIAN_POINT ( 'NONE',  ( 16.52544592524342804, -4.483927247898539470, 43.54057627198103830 ) ) ;
#14178=CARTESIAN_POINT ( 'NONE',  ( 14.29746914071049879, -8.314922557960816363, 113.3322429386476955 ) ) ;
#14179=CARTESIAN_POINT ( 'NONE',  ( 9.474510206698971260, -16.51473224551069308, 107.9155762719810383 ) ) ;
#14180=CARTESIAN_POINT ( 'NONE',  ( -18.62759615963255300, -10.81492255796106328, 29.16775706135234003 ) ) ;
#14181=CARTESIAN_POINT ( 'NONE',  ( 19.05341960407617918, -5.049401038297876454, 36.04275706135234003 ) ) ;
#14182=CARTESIAN_POINT ( 'NONE',  ( -14.29746914071049879, 8.314922557960819915, 110.8322429386476955 ) ) ;
#14183=CARTESIAN_POINT ( 'NONE',  ( 15.72974639402176855, 15.80617190586768217, 71.87609039468568994 ) ) ;
#14184=CARTESIAN_POINT ( 'NONE',  ( 17.50000000000000711, -5.499999999999992895, 31.21769037696435589 ) ) ;
#14185=CARTESIAN_POINT ( 'NONE',  ( 16.55341960407611168, 4.379528057220329451, 28.95724293864769905 ) ) ;
#14187=CARTESIAN_POINT ( 'NONE',  ( 21.53943276465977519, -0.05219959533907433946, 33.74890960531436690 ) ) ;
#14188=CARTESIAN_POINT ( 'NONE',  ( 14.34966873604960469, 8.224510206698951720, 84.16557627198103830 ) ) ;
#14190=CARTESIAN_POINT ( 'NONE',  ( -0.05219959533909027116, -19.03943276465977164, 77.49890960531435269 ) ) ;
#14191=CARTESIAN_POINT ( 'NONE',  ( 4.483927247898545687, 16.52544592524342804, 79.79057627198102409 ) ) ;
#14192=CARTESIAN_POINT ( 'NONE',  ( 0.05219959533936267826, -19.03943276465977164, 110.0010903946856757 ) ) ;
#14193=CARTESIAN_POINT ( 'NONE',  ( 5.823673210054125526, 21.52544592524343514, 44.79057627198103120 ) ) ;
#14196=CARTESIAN_POINT ( 'NONE',  ( -16.46253265017160317, 9.564922557960807481, 25.83224293864769194 ) ) ;
#14197=CARTESIAN_POINT ( 'NONE',  ( -9.564922557960796823, -16.46253265017161027, 77.08224293864769550 ) ) ;
#14198=CARTESIAN_POINT ( 'NONE',  ( 21.52544592524344225, -5.823673210054117533, 78.54057627198103830 ) ) ;
#14200=CARTESIAN_POINT ( 'NONE',  ( -16.53943276465976808, -0.05219959533934237506, 103.7510903946857042 ) ) ;
#14201=CARTESIAN_POINT ( 'NONE',  ( 19.02544592524343514, -5.153800228976328945, 83.54057627198100988 ) ) ;
#14202=CARTESIAN_POINT ( 'NONE',  ( -13.89961937509957401, -13.97604488694547875, 69.37609039468564731 ) ) ;
#14203=CARTESIAN_POINT ( 'NONE',  ( 15.72974639402176855, 15.80617190586768217, 91.87609039468568994 ) ) ;
#14204=CARTESIAN_POINT ( 'NONE',  ( 15.72974639402199770, -15.80617190586745480, 63.12390960531435979 ) ) ;
#14205=CARTESIAN_POINT ( 'NONE',  ( 18.67979575497178502, 10.72451020669898547, 29.16557627198103120 ) ) ;
#14206=CARTESIAN_POINT ( 'NONE',  ( -9.474510206698964154, 16.51473224551069663, 30.41557627198102054 ) ) ;
#14207=CARTESIAN_POINT ( 'NONE',  ( -4.483927247898782831, 16.52544592524335698, 97.70942372801904696 ) ) ;
#14208=CARTESIAN_POINT ( 'NONE',  ( -5.049401038298153566, 19.05341960407611168, 60.20724293864768129 ) ) ;
#14209=CARTESIAN_POINT ( 'NONE',  ( 4.483927247898790824, -16.52544592524335698, 25.20942372801901854 ) ) ;
#14210=CARTESIAN_POINT ( 'NONE',  ( 16.29526858892879915, 7.335722546920000475, 53.29670597800210174 ) ) ;
#14211=CARTESIAN_POINT ( 'NONE',  ( -10.72451020669870658, -18.67979575497194134, 109.5844237280190328 ) ) ;
#14212=CARTESIAN_POINT ( 'NONE',  ( -8.314922557960811034, -14.29746914071050412, 72.08224293864769550 ) ) ;
#14213=CARTESIAN_POINT ( 'NONE',  ( 15.72974639402199770, -15.80617190586745480, 103.1239096053143811 ) ) ;
#14214=CARTESIAN_POINT ( 'NONE',  ( -21.55341960407610458, -5.719274019375992779, 96.45724293864770971 ) ) ;
#14216=CARTESIAN_POINT ( 'NONE',  ( -10.72451020669898014, 18.67979575497178502, 40.41557627198103120 ) ) ;
#14217=CARTESIAN_POINT ( 'NONE',  ( -16.52544592524335698, -4.483927247898792601, 83.95942372801900433 ) ) ;
#14218=CARTESIAN_POINT ( 'NONE',  ( -8.224510206698948167, 14.34966873604960824, 100.4155762719810241 ) ) ;
#14219=CARTESIAN_POINT ( 'NONE',  ( 5.049401038298161559, -19.05341960407611168, 57.70724293864769550 ) ) ;
#14221=CARTESIAN_POINT ( 'NONE',  ( 14.29746914071049879, -8.314922557960816363, 23.33224293864769194 ) ) ;
#14222=CARTESIAN_POINT ( 'NONE',  ( 10.72451020669871369, 18.67979575497193778, 42.08442372801901854 ) ) ;
#14223=CARTESIAN_POINT ( 'NONE',  ( 19.03943276465977164, -0.05219959533909143690, 98.74890960531436690 ) ) ;
#14224=CARTESIAN_POINT ( 'NONE',  ( -18.67979575497193778, 10.72451020669871902, 83.33442372801903275 ) ) ;
#14225=CARTESIAN_POINT ( 'NONE',  ( 19.03943276465977164, -0.05219959533909143690, 28.74890960531435624 ) ) ;
#14226=CARTESIAN_POINT ( 'NONE',  ( 5.153800228976335163, 19.02544592524342804, 39.79057627198100988 ) ) ;
#14227=VERTEX_POINT ( 'NONE', #177554 ) ;
#14228=CARTESIAN_POINT ( 'NONE',  ( 10.81492255796106328, -18.62759615963255655, 75.41775706135233293 ) ) ;
#14229=CARTESIAN_POINT ( 'NONE',  ( 19.05341960407611168, 5.049401038298154454, 103.9572429386476671 ) ) ;
#14230=CARTESIAN_POINT ( 'NONE',  ( -9.474510206698720793, -16.51473224551083518, 74.58442372801900433 ) ) ;
#14231=CARTESIAN_POINT ( 'NONE',  ( 10.72451020669871369, 18.67979575497193778, 37.08442372801901143 ) ) ;
#14232=CARTESIAN_POINT ( 'NONE',  ( -16.53943276465976808, -0.05219959533934237506, 28.75109039468567929 ) ) ;
#14233=CARTESIAN_POINT ( 'NONE',  ( 16.46253265017146816, 9.564922557961045513, 66.66775706135233293 ) ) ;
#14234=CARTESIAN_POINT ( 'NONE',  ( 19.02544592524343514, -5.153800228976328945, 48.54057627198103120 ) ) ;
#14235=CARTESIAN_POINT ( 'NONE',  ( -9.474510206698720793, -16.51473224551083518, 89.58442372801900433 ) ) ;
#14236=CARTESIAN_POINT ( 'NONE',  ( -8.314922557960811034, -14.29746914071050412, 32.08224293864769550 ) ) ;
#14237=CARTESIAN_POINT ( 'NONE',  ( -0.05219959533936034679, 19.03943276465977164, 82.50109039468567573 ) ) ;
#14238=CARTESIAN_POINT ( 'NONE',  ( 4.483927247898545687, 16.52544592524342804, 34.79057627198103120 ) ) ;
#14239=CARTESIAN_POINT ( 'NONE',  ( 16.46253265017146816, 9.564922557961045513, 66.66775706135233293 ) ) ;
#14240=CARTESIAN_POINT ( 'NONE',  ( 16.52544592524335698, 4.483927247898782831, 41.45942372801901143 ) ) ;
#14241=CARTESIAN_POINT ( 'NONE',  ( 15.72974639402176855, 15.80617190586768217, 111.8760903946856615 ) ) ;
#14242=CARTESIAN_POINT ( 'NONE',  ( 5.153800228976335163, 19.02544592524342804, 29.79057627198102409 ) ) ;
#14243=CARTESIAN_POINT ( 'NONE',  ( -16.52216118717208460, -7.221426719304528064, 66.07599021046993926 ) ) ;
#14244=CARTESIAN_POINT ( 'NONE',  ( 0.05219959533934541429, -16.53943276465976808, 50.00109039468568994 ) ) ;
#14247=CARTESIAN_POINT ( 'NONE',  ( 13.89961937509977652, -13.97604488694527269, 88.12390960531438111 ) ) ;
#14251=CARTESIAN_POINT ( 'NONE',  ( -9.564922557961040184, 16.46253265017147172, 87.91775706135233293 ) ) ;
#14252=CARTESIAN_POINT ( 'NONE',  ( -19.02544592524342804, 5.153800228976336051, 116.0405762719810383 ) ) ;
#14253=CARTESIAN_POINT ( 'NONE',  ( 15.72974639402176855, 15.80617190586768217, 111.8760903946856615 ) ) ;
#14254=CARTESIAN_POINT ( 'NONE',  ( -9.474510206698720793, -16.51473224551083518, 99.58442372801900433 ) ) ;
#14255=CARTESIAN_POINT ( 'NONE',  ( 16.53943276465976808, -0.05219959533910856209, 113.7489096053143527 ) ) ;
#14256=CARTESIAN_POINT ( 'NONE',  ( -5.049401038298153566, 19.05341960407611168, 40.20724293864768839 ) ) ;
#14257=CARTESIAN_POINT ( 'NONE',  ( 10.72451020669898902, -18.67979575497178502, 52.91557627198103830 ) ) ;
#14260=CARTESIAN_POINT ( 'NONE',  ( 0.05219959533907565091, 21.53943276465977519, 54.99890960531435269 ) ) ;
#14261=CARTESIAN_POINT ( 'NONE',  ( -16.51473224551069308, -9.474510206698971260, 26.66557627198103120 ) ) ;
#14263=CARTESIAN_POINT ( 'NONE',  ( -9.474510206698720793, -16.51473224551083518, 69.58442372801901854 ) ) ;
#14264=CARTESIAN_POINT ( 'NONE',  ( -12.14591786802309592, -12.06949235617757132, 36.87390960531435979 ) ) ;
#14265=CARTESIAN_POINT ( 'NONE',  ( -5.823673210054116645, -21.52544592524344225, 22.29057627198102765 ) ) ;
#14266=CARTESIAN_POINT ( 'NONE',  ( -15.72974639402176322, -15.80617190586768395, 99.37609039468568994 ) ) ;
#14267=CARTESIAN_POINT ( 'NONE',  ( 5.823673210054125526, 21.52544592524343514, 79.79057627198102409 ) ) ;
#14268=CARTESIAN_POINT ( 'NONE',  ( -5.823673210054431948, 21.52544592524334988, 62.70942372801902565 ) ) ;
#14269=CARTESIAN_POINT ( 'NONE',  ( 10.81492255796106328, -18.62759615963255655, 70.41775706135236135 ) ) ;
#14270=CARTESIAN_POINT ( 'NONE',  ( -19.02544592524342804, 5.153800228976336051, 91.04057627198100988 ) ) ;
#14271=CARTESIAN_POINT ( 'NONE',  ( -4.483927247898782831, 16.52544592524335698, 97.70942372801904696 ) ) ;
#14272=CARTESIAN_POINT ( 'NONE',  ( 21.55341960407619695, -5.719274019375665929, 46.04275706135234714 ) ) ;
#14273=CARTESIAN_POINT ( 'NONE',  ( -19.05341960407611168, -5.049401038298163336, 26.45724293864769550 ) ) ;
#14275=CARTESIAN_POINT ( 'NONE',  ( -8.224510206698948167, 14.34966873604960824, 70.41557627198102409 ) ) ;
#14276=CARTESIAN_POINT ( 'NONE',  ( -4.379528057220328563, 16.55341960407611168, 30.20724293864769550 ) ) ;
#14277=CARTESIAN_POINT ( 'NONE',  ( -5.719274019375978568, 21.55341960407610458, 40.20724293864769550 ) ) ;
#14278=CARTESIAN_POINT ( 'NONE',  ( 9.564922557960805705, 16.46253265017160317, 69.58224293864770971 ) ) ;
#14279=CARTESIAN_POINT ( 'NONE',  ( 5.153800228976335163, 19.02544592524342804, 44.79057627198103830 ) ) ;
#14280=CARTESIAN_POINT ( 'NONE',  ( 21.52544592524344225, -5.823673210054117533, 58.54057627198103120 ) ) ;
#14281=CARTESIAN_POINT ( 'NONE',  ( -16.46253265017146816, -9.564922557961047289, 39.16775706135234003 ) ) ;
#14284=CARTESIAN_POINT ( 'NONE',  ( -8.224510206698948167, 14.34966873604960824, 50.41557627198103120 ) ) ;
#14285=CARTESIAN_POINT ( 'NONE',  ( -16.46253265017160317, 9.564922557960807481, 115.8322429386477097 ) ) ;
#14287=CARTESIAN_POINT ( 'NONE',  ( 17.59632111031587343, 2.707012485675212243, 37.50000000000002842 ) ) ;
#14288=CARTESIAN_POINT ( 'NONE',  ( 16.52544592524335698, 4.483927247898782831, 66.45942372801903275 ) ) ;
#14289=CARTESIAN_POINT ( 'NONE',  ( -19.02544592524334988, -5.153800228976617603, 73.95942372801900433 ) ) ;
#14290=CARTESIAN_POINT ( 'NONE',  ( 4.483927247898545687, 16.52544592524342804, 34.79057627198103120 ) ) ;
#14293=CARTESIAN_POINT ( 'NONE',  ( -16.53943276465976808, -0.05219959533934237506, 113.7510903946856757 ) ) ;
#14294=CARTESIAN_POINT ( 'NONE',  ( 5.153800228976335163, 19.02544592524342804, 54.79057627198103120 ) ) ;
#14295=CARTESIAN_POINT ( 'NONE',  ( -13.89961937509977652, 13.97604488694528158, 75.62390960531438111 ) ) ;
#14296=CARTESIAN_POINT ( 'NONE',  ( -19.05341960407611168, -5.049401038298163336, 36.45724293864766707 ) ) ;
#14297=CARTESIAN_POINT ( 'NONE',  ( -5.719274019375665041, -21.55341960407619695, 44.79275706135234714 ) ) ;
#14298=CARTESIAN_POINT ( 'NONE',  ( 0.05219959533909260263, 19.03943276465977164, 64.99890960531436690 ) ) ;
#14300=CARTESIAN_POINT ( 'NONE',  ( 16.46253265017160672, -9.564922557960803928, 63.33224293864769550 ) ) ;
#14302=CARTESIAN_POINT ( 'NONE',  ( -5.823673210054116645, -21.52544592524344225, 37.29057627198102409 ) ) ;
#14303=CARTESIAN_POINT ( 'NONE',  ( -19.03943276465977164, 0.05219959533909376836, 26.24890960531435624 ) ) ;
#14304=CARTESIAN_POINT ( 'NONE',  ( 15.80617190586746368, 15.72974639402197994, 29.37390960531435269 ) ) ;
#14305=CARTESIAN_POINT ( 'NONE',  ( 4.483927247898790824, -16.52544592524335698, 85.20942372801901854 ) ) ;
#14306=CARTESIAN_POINT ( 'NONE',  ( -5.719274019375665041, -21.55341960407619695, 104.7927570613523898 ) ) ;
#14307=CARTESIAN_POINT ( 'NONE',  ( 12.06949235617739724, 12.14591786802326823, 61.87609039468568284 ) ) ;
#14308=CARTESIAN_POINT ( 'NONE',  ( 13.89961937509977652, -13.97604488694527269, 113.1239096053143527 ) ) ;
#14310=CARTESIAN_POINT ( 'NONE',  ( 14.34966873604972726, -8.224510206698740333, 55.83442372801901854 ) ) ;
#14311=CARTESIAN_POINT ( 'NONE',  ( -14.34966873604972548, 8.224510206698743886, 43.33442372801901143 ) ) ;
#14312=CARTESIAN_POINT ( 'NONE',  ( 19.02544592524343514, -5.153800228976328945, 108.5405762719810383 ) ) ;
#14314=CARTESIAN_POINT ( 'NONE',  ( -14.29746914071037622, -8.314922557961029526, 24.16775706135235424 ) ) ;
#14315=CARTESIAN_POINT ( 'NONE',  ( 16.51473224551069308, 9.474510206698969483, 39.16557627198103120 ) ) ;
#14316=CARTESIAN_POINT ( 'NONE',  ( 5.823673210054444382, -21.52544592524334988, 30.20942372801902565 ) ) ;
#14317=CARTESIAN_POINT ( 'NONE',  ( 16.52544592524335698, 4.483927247898782831, 21.45942372801901499 ) ) ;
#14318=CARTESIAN_POINT ( 'NONE',  ( -0.05219959533934338120, 16.53943276465976808, 87.50109039468568994 ) ) ;
#14319=CARTESIAN_POINT ( 'NONE',  ( -17.49999999999999289, 5.624438216177559013, 45.81670344914643778 ) ) ;
#14320=CARTESIAN_POINT ( 'NONE',  ( -15.80617190586768217, 15.72974639402176855, 93.12609039468568994 ) ) ;
#14321=CARTESIAN_POINT ( 'NONE',  ( 19.03943276465977164, 0.05219959533936151252, 81.25109039468567573 ) ) ;
#14322=CARTESIAN_POINT ( 'NONE',  ( -16.52544592524342804, 4.483927247898546575, 61.04057627198103120 ) ) ;
#14323=CARTESIAN_POINT ( 'NONE',  ( -0.05219959533910754901, -16.53943276465976808, 112.4989096053143669 ) ) ;
#14324=CARTESIAN_POINT ( 'NONE',  ( -13.89961937509957401, -13.97604488694547875, 44.37609039468566863 ) ) ;
#14325=CARTESIAN_POINT ( 'NONE',  ( 17.05116617787849620, -6.768360034955525073, 56.15675553259194430 ) ) ;
#14326=CARTESIAN_POINT ( 'NONE',  ( 15.72974639402176855, 15.80617190586768217, 46.87609039468568994 ) ) ;
#14327=CARTESIAN_POINT ( 'NONE',  ( -0.05219959533936034679, 19.03943276465977164, 112.5010903946856757 ) ) ;
#14329=CARTESIAN_POINT ( 'NONE',  ( 16.51473224551069308, 9.474510206698969483, 109.1655762719810383 ) ) ;
#14330=CARTESIAN_POINT ( 'NONE',  ( 15.80617190586746368, 15.72974639402197994, 74.37390960531436690 ) ) ;
#14331=CARTESIAN_POINT ( 'NONE',  ( -19.05341960407617563, 5.049401038297882671, 93.54275706135234714 ) ) ;
#14332=CARTESIAN_POINT ( 'NONE',  ( 0.05219959533909260263, 19.03943276465977164, 104.9989096053143669 ) ) ;
#14333=CARTESIAN_POINT ( 'NONE',  ( -16.46253265017146816, -9.564922557961047289, 49.16775706135233293 ) ) ;
#14334=CARTESIAN_POINT ( 'NONE',  ( -16.52544592524342804, 4.483927247898546575, 101.0405762719810383 ) ) ;
#14335=CARTESIAN_POINT ( 'NONE',  ( 5.823673210054444382, -21.52544592524334988, 90.20942372801903275 ) ) ;
#14336=CARTESIAN_POINT ( 'NONE',  ( -9.474510206698964154, 16.51473224551069663, 45.41557627198103120 ) ) ;
#14337=CARTESIAN_POINT ( 'NONE',  ( 10.72451020669871369, 18.67979575497193778, 52.08442372801901854 ) ) ;
#14338=CARTESIAN_POINT ( 'NONE',  ( -21.52544592524334988, -5.823673210054445271, 93.95942372801903275 ) ) ;
#14339=CARTESIAN_POINT ( 'NONE',  ( -14.29746914071037622, -8.314922557961029526, 94.16775706135237556 ) ) ;
#14340=CARTESIAN_POINT ( 'NONE',  ( -18.62759615963255300, -10.81492255796106328, 44.16775706135234714 ) ) ;
#14341=CARTESIAN_POINT ( 'NONE',  ( -21.55341960407619339, 5.719274019375674811, 33.54275706135234714 ) ) ;
#14342=CARTESIAN_POINT ( 'NONE',  ( 19.05341960407617918, -5.049401038297876454, 61.04275706135232582 ) ) ;
#14343=CARTESIAN_POINT ( 'NONE',  ( 13.97604488694527802, 13.89961937509977652, 89.37390960531436690 ) ) ;
#14344=CARTESIAN_POINT ( 'NONE',  ( -4.483927247898539470, -16.52544592524342804, 107.2905762719810525 ) ) ;
#14346=CARTESIAN_POINT ( 'NONE',  ( 10.72451020669898902, -18.67979575497178502, 82.91557627198103830 ) ) ;
#14347=CARTESIAN_POINT ( 'NONE',  ( 16.52544592524342804, -4.483927247898539470, 58.54057627198103120 ) ) ;
#14348=CARTESIAN_POINT ( 'NONE',  ( -21.55341960407619339, 5.719274019375674811, 103.5427570613523613 ) ) ;
#14349=CARTESIAN_POINT ( 'NONE',  ( 16.53943276465976808, -0.05219959533910856209, 78.74890960531436690 ) ) ;
#14350=CARTESIAN_POINT ( 'NONE',  ( -9.564922557960796823, -16.46253265017161027, 42.08224293864769550 ) ) ;
#14351=CARTESIAN_POINT ( 'NONE',  ( -9.474510206698720793, -16.51473224551083518, 84.58442372801900433 ) ) ;
#14352=CARTESIAN_POINT ( 'NONE',  ( 12.14591786802309770, 12.06949235617756955, 49.37390960531436690 ) ) ;
#14353=CARTESIAN_POINT ( 'NONE',  ( 15.72974639402176855, 15.80617190586768217, 96.87609039468568994 ) ) ;
#14354=CARTESIAN_POINT ( 'NONE',  ( -19.05341960407611168, -5.049401038298163336, 86.45724293864769550 ) ) ;
#14355=CARTESIAN_POINT ( 'NONE',  ( 5.153800228976615827, -19.02544592524334988, 60.20942372801899012 ) ) ;
#14356=CARTESIAN_POINT ( 'NONE',  ( 18.62759615963271287, -10.81492255796078972, 63.33224293864770260 ) ) ;
#14357=CARTESIAN_POINT ( 'NONE',  ( -15.72974639402176322, -15.80617190586768395, 24.37609039468567573 ) ) ;
#14358=CARTESIAN_POINT ( 'NONE',  ( -14.29746914071037622, -8.314922557961029526, 29.16775706135234003 ) ) ;
#14359=CARTESIAN_POINT ( 'NONE',  ( -8.224510206698735004, -14.34966873604973081, 74.58442372801901854 ) ) ;
#14360=CARTESIAN_POINT ( 'NONE',  ( 19.03943276465977164, -0.05219959533909143690, 23.74890960531435269 ) ) ;
#14361=CARTESIAN_POINT ( 'NONE',  ( 15.80617190586746368, 15.72974639402197994, 114.3739096053143527 ) ) ;
#14362=CARTESIAN_POINT ( 'NONE',  ( -0.05219959533910754901, -16.53943276465976808, 112.4989096053143669 ) ) ;
#14364=CARTESIAN_POINT ( 'NONE',  ( -0.05219959533934338120, 16.53943276465976808, 42.50109039468567573 ) ) ;
#14365=CARTESIAN_POINT ( 'NONE',  ( 12.06949235617757843, -12.14591786802309237, 83.12390960531436690 ) ) ;
#14366=CARTESIAN_POINT ( 'NONE',  ( -5.719274019375978568, 21.55341960407610458, 80.20724293864769550 ) ) ;
#14367=CARTESIAN_POINT ( 'NONE',  ( -0.05219959533910754901, -16.53943276465976808, 22.49890960531436335 ) ) ;
#14368=CARTESIAN_POINT ( 'NONE',  ( 4.483927247898790824, -16.52544592524335698, 35.20942372801901854 ) ) ;
#14369=CARTESIAN_POINT ( 'NONE',  ( -13.97604488694527625, -13.89961937509977652, 51.87390960531436690 ) ) ;
#14370=CARTESIAN_POINT ( 'NONE',  ( -12.06949235617739369, -12.14591786802326823, 84.37609039468570415 ) ) ;
#14371=CARTESIAN_POINT ( 'NONE',  ( -13.97604488694547697, 13.89961937509957934, 73.12609039468568994 ) ) ;
#14372=CARTESIAN_POINT ( 'NONE',  ( -21.55341960407610458, -5.719274019375992779, 66.45724293864768129 ) ) ;
#14373=CARTESIAN_POINT ( 'NONE',  ( -8.224510206698735004, -14.34966873604973081, 109.5844237280190328 ) ) ;
#14374=ORIENTED_EDGE ( 'NONE', *, *, #48933, .T. ) ;
#14376=CARTESIAN_POINT ( 'NONE',  ( 5.823673210054125526, 21.52544592524343514, 49.79057627198102409 ) ) ;
#14378=CARTESIAN_POINT ( 'NONE',  ( -4.379528057220086978, -16.55341960407618274, 89.79275706135236135 ) ) ;
#14380=CARTESIAN_POINT ( 'NONE',  ( -16.46253265017160317, 9.564922557960807481, 115.8322429386477097 ) ) ;
#14381=CARTESIAN_POINT ( 'NONE',  ( 17.50000000000000000, 5.499999999999997335, 106.7030961746582847 ) ) ;
#14382=CARTESIAN_POINT ( 'NONE',  ( -21.52544592524343514, 5.823673210054127303, 76.04057627198102409 ) ) ;
#14383=CARTESIAN_POINT ( 'NONE',  ( -16.52544592524335698, -4.483927247898792601, 108.9594237280190185 ) ) ;
#14384=CARTESIAN_POINT ( 'NONE',  ( -5.823673210054431948, 21.52544592524334988, 62.70942372801902565 ) ) ;
#14385=CARTESIAN_POINT ( 'NONE',  ( 4.483927247898790824, -16.52544592524335698, 25.20942372801901854 ) ) ;
#14386=CARTESIAN_POINT ( 'NONE',  ( 5.153800228976335163, 19.02544592524342804, 24.79057627198102765 ) ) ;
#14387=CARTESIAN_POINT ( 'NONE',  ( -16.52544592524335698, -4.483927247898792601, 23.95942372801901143 ) ) ;
#14388=CARTESIAN_POINT ( 'NONE',  ( 13.89961937509977652, -13.97604488694527269, 58.12390960531436690 ) ) ;
#14390=CARTESIAN_POINT ( 'NONE',  ( 5.153800228976335163, 19.02544592524342804, 109.7905762719810099 ) ) ;
#14392=CARTESIAN_POINT ( 'NONE',  ( -12.06949235617739369, -12.14591786802326823, 94.37609039468568994 ) ) ;
#14393=CARTESIAN_POINT ( 'NONE',  ( -13.89961937509957401, -13.97604488694547875, 94.37609039468566152 ) ) ;
#14394=CARTESIAN_POINT ( 'NONE',  ( 5.153800228976615827, -19.02544592524334988, 25.20942372801900433 ) ) ;
#14395=CARTESIAN_POINT ( 'NONE',  ( -10.72451020669898014, 18.67979575497178502, 70.41557627198102409 ) ) ;
#14396=CARTESIAN_POINT ( 'NONE',  ( -16.55341960407617563, 4.379528057220093196, 98.54275706135234714 ) ) ;
#14397=CARTESIAN_POINT ( 'NONE',  ( -0.05219959533936034679, 19.03943276465977164, 92.50109039468566152 ) ) ;
#14398=CARTESIAN_POINT ( 'NONE',  ( -19.03943276465977164, 0.05219959533909376836, 56.24890960531435979 ) ) ;
#14399=CARTESIAN_POINT ( 'NONE',  ( -9.474510206698964154, 16.51473224551069663, 95.41557627198102409 ) ) ;
#14401=CARTESIAN_POINT ( 'NONE',  ( -15.80617190586768217, 15.72974639402176855, 68.12609039468567573 ) ) ;
#14402=CARTESIAN_POINT ( 'NONE',  ( 16.46253265017160672, -9.564922557960803928, 48.33224293864769550 ) ) ;
#14404=CARTESIAN_POINT ( 'NONE',  ( 16.52544592524342804, -4.483927247898539470, 73.54057627198102409 ) ) ;
#14405=CARTESIAN_POINT ( 'NONE',  ( -18.67979575497178146, -10.72451020669898902, 71.66557627198100988 ) ) ;
#14407=CARTESIAN_POINT ( 'NONE',  ( 9.474510206698729675, 16.51473224551082808, 37.08442372801899722 ) ) ;
#14409=CARTESIAN_POINT ( 'NONE',  ( 13.89961937509977652, -13.97604488694527269, 83.12390960531436690 ) ) ;
#14410=CARTESIAN_POINT ( 'NONE',  ( -19.02544592524342804, 5.153800228976336051, 91.04057627198100988 ) ) ;
#14411=CARTESIAN_POINT ( 'NONE',  ( 8.314922557961029526, -14.29746914071037800, 50.41775706135235424 ) ) ;
#14413=CARTESIAN_POINT ( 'NONE',  ( -5.049401038297874678, -19.05341960407617918, 24.79275706135233648 ) ) ;
#14415=CARTESIAN_POINT ( 'NONE',  ( -8.314922557961024197, 14.29746914071037800, 82.91775706135234714 ) ) ;
#14417=CARTESIAN_POINT ( 'NONE',  ( -4.379528057220086978, -16.55341960407618274, 79.79275706135236135 ) ) ;
#14418=CARTESIAN_POINT ( 'NONE',  ( -14.34966873604972548, 8.224510206698743886, 53.33442372801901854 ) ) ;
#14419=CARTESIAN_POINT ( 'NONE',  ( -19.05341960407611168, -5.049401038298163336, 51.45724293864770260 ) ) ;
#14421=CARTESIAN_POINT ( 'NONE',  ( -21.55341960407619339, 5.719274019375674811, 63.54275706135234003 ) ) ;
#14422=CARTESIAN_POINT ( 'NONE',  ( 9.564922557961047289, -16.46253265017146816, 75.41775706135234714 ) ) ;
#14423=CARTESIAN_POINT ( 'NONE',  ( 15.72974639402176855, 15.80617190586768217, 101.8760903946857042 ) ) ;
#14424=CARTESIAN_POINT ( 'NONE',  ( 19.03943276465977164, -0.05219959533909143690, 58.74890960531435979 ) ) ;
#14425=CARTESIAN_POINT ( 'NONE',  ( 5.049401038298161559, -19.05341960407611168, 37.70724293864768839 ) ) ;
#14426=CARTESIAN_POINT ( 'NONE',  ( 16.35915291253759207, 7.306589564586257524, 22.28015278803768595 ) ) ;
#14427=CARTESIAN_POINT ( 'NONE',  ( 18.62759615963271287, -10.81492255796078972, 63.33224293864770260 ) ) ;
#14430=CARTESIAN_POINT ( 'NONE',  ( 9.564922557960805705, 16.46253265017160317, 114.5822429386476955 ) ) ;
#14431=CARTESIAN_POINT ( 'NONE',  ( 19.05341960407611168, 5.049401038298154454, 23.95724293864769194 ) ) ;
#14432=CARTESIAN_POINT ( 'NONE',  ( 12.06949235617739724, 12.14591786802326823, 56.87609039468568994 ) ) ;
#14433=CARTESIAN_POINT ( 'NONE',  ( -14.34966873604960291, -8.224510206698953496, 26.66557627198103475 ) ) ;
#14435=CARTESIAN_POINT ( 'NONE',  ( -5.823673210054431948, 21.52544592524334988, 22.70942372801901499 ) ) ;
#14436=CARTESIAN_POINT ( 'NONE',  ( 4.483927247898545687, 16.52544592524342804, 54.79057627198104541 ) ) ;
#14438=CARTESIAN_POINT ( 'NONE',  ( -9.474510206698720793, -16.51473224551083518, 104.5844237280190043 ) ) ;
#14439=CARTESIAN_POINT ( 'NONE',  ( -9.474510206698720793, -16.51473224551083518, 44.58442372801900433 ) ) ;
#14440=CARTESIAN_POINT ( 'NONE',  ( -16.52544592524342804, 4.483927247898546575, 51.04057627198103120 ) ) ;
#14441=CARTESIAN_POINT ( 'NONE',  ( 21.52544592524344225, -5.823673210054117533, 98.54057627198105251 ) ) ;
#14443=CARTESIAN_POINT ( 'NONE',  ( 21.53943276465977519, -0.05219959533907433946, 58.74890960531436690 ) ) ;
#14444=CARTESIAN_POINT ( 'NONE',  ( -13.89961937509977652, 13.97604488694528158, 95.62390960531436690 ) ) ;
#14445=CARTESIAN_POINT ( 'NONE',  ( 12.14591786802309770, 12.06949235617756955, 49.37390960531436690 ) ) ;
#14446=CARTESIAN_POINT ( 'NONE',  ( -13.97604488694527625, -13.89961937509977652, 106.8739096053143669 ) ) ;
#14448=CARTESIAN_POINT ( 'NONE',  ( 13.89961937509957401, 13.97604488694547697, 56.87609039468564731 ) ) ;
#14449=CARTESIAN_POINT ( 'NONE',  ( -21.52544592524343514, 5.823673210054127303, 96.04057627198102409 ) ) ;
#14450=CARTESIAN_POINT ( 'NONE',  ( -9.564922557960796823, -16.46253265017161027, 37.08224293864768839 ) ) ;
#14451=CARTESIAN_POINT ( 'NONE',  ( 12.14591786802309770, 12.06949235617756955, 114.3739096053143527 ) ) ;
#14452=CARTESIAN_POINT ( 'NONE',  ( 15.72974639402176855, 15.80617190586768217, 56.87609039468568994 ) ) ;
#14454=CARTESIAN_POINT ( 'NONE',  ( -14.34966873604960291, -8.224510206698953496, 21.66557627198102409 ) ) ;
#14455=CARTESIAN_POINT ( 'NONE',  ( 16.46253265017160672, -9.564922557960803928, 48.33224293864769550 ) ) ;
#14456=CARTESIAN_POINT ( 'NONE',  ( 19.02544592524343514, -5.153800228976328945, 98.54057627198100988 ) ) ;
#14457=CARTESIAN_POINT ( 'NONE',  ( 15.80617190586746368, 15.72974639402197994, 64.37390960531435269 ) ) ;
#14459=CARTESIAN_POINT ( 'NONE',  ( -5.049401038298153566, 19.05341960407611168, 50.20724293864770260 ) ) ;
#14460=CARTESIAN_POINT ( 'NONE',  ( 5.719274019375991003, -21.55341960407610458, 52.70724293864769550 ) ) ;
#14462=CARTESIAN_POINT ( 'NONE',  ( 18.67979575497194134, -10.72451020669871369, 90.83442372801901854 ) ) ;
#14464=CARTESIAN_POINT ( 'NONE',  ( 14.29746914071037800, 8.314922557961029526, 86.66775706135234714 ) ) ;
#14465=CARTESIAN_POINT ( 'NONE',  ( 16.52544592524342804, -4.483927247898539470, 73.54057627198102409 ) ) ;
#14466=CARTESIAN_POINT ( 'NONE',  ( 16.55341960407618274, -4.379528057220086978, 86.04275706135236135 ) ) ;
#14467=CARTESIAN_POINT ( 'NONE',  ( 9.474510206698971260, -16.51473224551069308, 72.91557627198102409 ) ) ;
#14469=CARTESIAN_POINT ( 'NONE',  ( -13.97604488694547697, 13.89961937509957934, 33.12609039468566863 ) ) ;
#14470=CARTESIAN_POINT ( 'NONE',  ( -8.314922557961024197, 14.29746914071037800, 87.91775706135234714 ) ) ;
#14471=CARTESIAN_POINT ( 'NONE',  ( -21.52544592524334988, -5.823673210054445271, 108.9594237280190185 ) ) ;
#14472=CARTESIAN_POINT ( 'NONE',  ( -19.05341960407611168, -5.049401038298163336, 76.45724293864769550 ) ) ;
#14473=CARTESIAN_POINT ( 'NONE',  ( 21.52544592524344225, -5.823673210054117533, 43.54057627198103830 ) ) ;
#14474=CARTESIAN_POINT ( 'NONE',  ( -8.314922557961024197, 14.29746914071037800, 22.91775706135235069 ) ) ;
#14475=CARTESIAN_POINT ( 'NONE',  ( -5.823673210054431948, 21.52544592524334988, 82.70942372801900433 ) ) ;
#14476=CARTESIAN_POINT ( 'NONE',  ( 12.06949235617739724, 12.14591786802326823, 61.87609039468568284 ) ) ;
#14477=CARTESIAN_POINT ( 'NONE',  ( 18.67979575497178502, 10.72451020669898547, 114.1655762719810383 ) ) ;
#14478=CARTESIAN_POINT ( 'NONE',  ( -14.34966873604972548, 8.224510206698743886, 23.33442372801901499 ) ) ;
#14479=CARTESIAN_POINT ( 'NONE',  ( -13.97604488694527625, -13.89961937509977652, 91.87390960531432427 ) ) ;
#14480=CARTESIAN_POINT ( 'NONE',  ( 14.29746914071037800, 8.314922557961029526, 21.66775706135235069 ) ) ;
#14481=CARTESIAN_POINT ( 'NONE',  ( 19.03943276465977164, -0.05219959533909143690, 38.74890960531436690 ) ) ;
#14482=CARTESIAN_POINT ( 'NONE',  ( 14.34966873604972726, -8.224510206698740333, 35.83442372801901143 ) ) ;
#14483=CARTESIAN_POINT ( 'NONE',  ( -4.379528057220328563, 16.55341960407611168, 85.20724293864770971 ) ) ;
#14484=CARTESIAN_POINT ( 'NONE',  ( -12.06949235617739369, -12.14591786802326823, 89.37609039468568994 ) ) ;
#14485=CARTESIAN_POINT ( 'NONE',  ( -21.53943276465977519, -0.05219959533937600094, 23.75109039468567929 ) ) ;
#14486=CARTESIAN_POINT ( 'NONE',  ( 13.89961937509977652, -13.97604488694527269, 68.12390960531436690 ) ) ;
#14487=CARTESIAN_POINT ( 'NONE',  ( -5.153800228976328057, -19.02544592524343514, 72.29057627198102409 ) ) ;
#14488=CARTESIAN_POINT ( 'NONE',  ( 12.06949235617739724, 12.14591786802326823, 91.87609039468568994 ) ) ;
#14490=CARTESIAN_POINT ( 'NONE',  ( -17.60779699588842107, -5.499999999999944933, 81.34981316670108242 ) ) ;
#14493=CARTESIAN_POINT ( 'NONE',  ( -13.97604488694547697, 13.89961937509957934, 28.12609039468565797 ) ) ;
#14494=CARTESIAN_POINT ( 'NONE',  ( 19.02544592524343514, -5.153800228976328945, 48.54057627198103120 ) ) ;
#14495=CARTESIAN_POINT ( 'NONE',  ( -13.89961937509977652, 13.97604488694528158, 115.6239096053143669 ) ) ;
#14497=CARTESIAN_POINT ( 'NONE',  ( -14.34966873604972548, 8.224510206698743886, 23.33442372801901499 ) ) ;
#14498=CARTESIAN_POINT ( 'NONE',  ( 9.564922557961047289, -16.46253265017146816, 55.41775706135234003 ) ) ;
#14499=CARTESIAN_POINT ( 'NONE',  ( -16.52544592524335698, -4.483927247898792601, 43.95942372801902565 ) ) ;
#14500=CARTESIAN_POINT ( 'NONE',  ( -5.049401038298153566, 19.05341960407611168, 100.2072429386476955 ) ) ;
#14501=CARTESIAN_POINT ( 'NONE',  ( -16.46253265017160317, 9.564922557960807481, 75.83224293864769550 ) ) ;
#14502=CARTESIAN_POINT ( 'NONE',  ( -18.67979575497178146, -10.72451020669898902, 101.6655762719810383 ) ) ;
#14503=CARTESIAN_POINT ( 'NONE',  ( -16.46253265017146816, -9.564922557961047289, 59.16775706135233293 ) ) ;
#14504=CARTESIAN_POINT ( 'NONE',  ( -19.03943276465977164, 0.05219959533909376836, 86.24890960531436690 ) ) ;
#14505=CARTESIAN_POINT ( 'NONE',  ( 17.49281420622803651, -3.774461901019551924, 21.82614614838133349 ) ) ;
#14506=CARTESIAN_POINT ( 'NONE',  ( 5.049401038298161559, -19.05341960407611168, 57.70724293864769550 ) ) ;
#14507=CARTESIAN_POINT ( 'NONE',  ( -8.314922557961024197, 14.29746914071037800, 107.9177570613523471 ) ) ;
#14508=CARTESIAN_POINT ( 'NONE',  ( -13.97604488694527625, -13.89961937509977652, 26.87390960531434558 ) ) ;
#14509=CARTESIAN_POINT ( 'NONE',  ( 16.46253265017146816, 9.564922557961045513, 41.66775706135234003 ) ) ;
#14511=CARTESIAN_POINT ( 'NONE',  ( 16.52544592524342804, -4.483927247898539470, 78.54057627198103830 ) ) ;
#14512=CARTESIAN_POINT ( 'NONE',  ( 0.05219959533937995610, -21.53943276465977519, 100.0010903946857042 ) ) ;
#14513=CARTESIAN_POINT ( 'NONE',  ( 9.564922557960805705, 16.46253265017160317, 44.58224293864769550 ) ) ;
#14514=CARTESIAN_POINT ( 'NONE',  ( -16.52544592524335698, -4.483927247898792601, 48.95942372801902565 ) ) ;
#14515=CARTESIAN_POINT ( 'NONE',  ( -12.14591786802309592, -12.06949235617757132, 46.87390960531435979 ) ) ;
#14516=CARTESIAN_POINT ( 'NONE',  ( -10.81492255796105439, 18.62759615963255655, 92.91775706135236135 ) ) ;
#14517=CARTESIAN_POINT ( 'NONE',  ( 9.564922557960805705, 16.46253265017160317, 99.58224293864770971 ) ) ;
#14518=CARTESIAN_POINT ( 'NONE',  ( 13.97604488694527802, 13.89961937509977652, 99.37390960531436690 ) ) ;
#14519=CARTESIAN_POINT ( 'NONE',  ( 16.52544592524342804, -4.483927247898539470, 113.5405762719810383 ) ) ;
#14520=CARTESIAN_POINT ( 'NONE',  ( 12.14591786802309770, 12.06949235617756955, 69.37390960531436690 ) ) ;
#14521=CARTESIAN_POINT ( 'NONE',  ( -15.80617190586745835, -15.72974639402198527, 81.87390960531435269 ) ) ;
#14522=CARTESIAN_POINT ( 'NONE',  ( -13.97604488694527625, -13.89961937509977652, 86.87390960531436690 ) ) ;
#14523=CARTESIAN_POINT ( 'NONE',  ( 10.72451020669898902, -18.67979575497178502, 97.91557627198103830 ) ) ;
#14525=CARTESIAN_POINT ( 'NONE',  ( -5.153800228976607833, 19.02544592524334988, 72.70942372801900433 ) ) ;
#14526=CARTESIAN_POINT ( 'NONE',  ( -19.25176906914648356, -5.499999999999852562, 90.99927264242278113 ) ) ;
#14527=CARTESIAN_POINT ( 'NONE',  ( -14.29746914071049879, 8.314922557960819915, 90.83224293864769550 ) ) ;
#14528=CARTESIAN_POINT ( 'NONE',  ( 19.02544592524343514, -5.153800228976328945, 63.54057627198103830 ) ) ;
#14529=CARTESIAN_POINT ( 'NONE',  ( -21.52544592524343514, 5.823673210054127303, 71.04057627198103830 ) ) ;
#14531=CARTESIAN_POINT ( 'NONE',  ( -0.05219959533934338120, 16.53943276465976808, 112.5010903946857042 ) ) ;
#14533=CARTESIAN_POINT ( 'NONE',  ( 12.14591786802327356, -12.06949235617739191, 20.62609039468568639 ) ) ;
#14534=CARTESIAN_POINT ( 'NONE',  ( -12.06949235617756955, 12.14591786802309770, 80.62390960531438111 ) ) ;
#14535=CARTESIAN_POINT ( 'NONE',  ( -16.79531203550650531, -7.028104445595562133, 96.25244988220441655 ) ) ;
#14536=CARTESIAN_POINT ( 'NONE',  ( -9.474510206698964154, 16.51473224551069663, 70.41557627198102409 ) ) ;
#14537=CARTESIAN_POINT ( 'NONE',  ( 19.02544592524343514, -5.153800228976328945, 33.54057627198102409 ) ) ;
#14538=CARTESIAN_POINT ( 'NONE',  ( 8.224510206698953496, -14.34966873604960469, 67.91557627198102409 ) ) ;
#14539=CARTESIAN_POINT ( 'NONE',  ( 9.474510206698971260, -16.51473224551069308, 112.9155762719810383 ) ) ;
#14540=CARTESIAN_POINT ( 'NONE',  ( -9.474510206698720793, -16.51473224551083518, 99.58442372801900433 ) ) ;
#14542=CARTESIAN_POINT ( 'NONE',  ( 19.02544592524343514, -5.153800228976328945, 103.5405762719809957 ) ) ;
#14543=CARTESIAN_POINT ( 'NONE',  ( -10.81492255796078084, -18.62759615963271287, 82.08224293864768129 ) ) ;
#14544=CARTESIAN_POINT ( 'NONE',  ( 4.483927247898790824, -16.52544592524335698, 70.20942372801904696 ) ) ;
#14546=CARTESIAN_POINT ( 'NONE',  ( -16.51473224551082808, 9.474510206698731452, 113.3344237280190043 ) ) ;
#14547=CARTESIAN_POINT ( 'NONE',  ( 5.153800228976335163, 19.02544592524342804, 64.79057627198100988 ) ) ;
#14548=CARTESIAN_POINT ( 'NONE',  ( 21.52544592524344225, -5.823673210054117533, 83.54057627198102409 ) ) ;
#14549=CARTESIAN_POINT ( 'NONE',  ( -21.53943276465977519, 0.05219959533907696930, 26.24890960531435624 ) ) ;
#14550=CARTESIAN_POINT ( 'NONE',  ( 16.46253265017146816, 9.564922557961045513, 106.6677570613523471 ) ) ;
#14551=CARTESIAN_POINT ( 'NONE',  ( 0.05219959533910956823, 16.53943276465976808, 39.99890960531436690 ) ) ;
#14552=CARTESIAN_POINT ( 'NONE',  ( -10.81492255796105439, 18.62759615963255655, 52.91775706135235424 ) ) ;
#14553=CARTESIAN_POINT ( 'NONE',  ( 18.22780087662121673, 5.500000000000056843, 83.98459894673892734 ) ) ;
#14554=CARTESIAN_POINT ( 'NONE',  ( 16.52544592524335698, 4.483927247898782831, 71.45942372801901854 ) ) ;
#14555=CARTESIAN_POINT ( 'NONE',  ( -19.02544592524342804, 5.153800228976336051, 101.0405762719810241 ) ) ;
#14556=CARTESIAN_POINT ( 'NONE',  ( 13.89961937509978007, -13.97604488694527269, 103.1239096053143385 ) ) ;
#14558=CARTESIAN_POINT ( 'NONE',  ( -8.224510206698735004, -14.34966873604973081, 99.58442372801900433 ) ) ;
#14559=CARTESIAN_POINT ( 'NONE',  ( -14.29746914071037622, -8.314922557961029526, 44.16775706135234714 ) ) ;
#14560=CARTESIAN_POINT ( 'NONE',  ( 19.05341960407611168, 5.049401038298154454, 53.95724293864770260 ) ) ;
#14561=CARTESIAN_POINT ( 'NONE',  ( -19.02544592524342804, 5.153800228976336051, 76.04057627198102409 ) ) ;
#14562=CARTESIAN_POINT ( 'NONE',  ( -21.53943276465977519, -0.05219959533937600094, 68.75109039468568994 ) ) ;
#14563=CARTESIAN_POINT ( 'NONE',  ( 14.29746914071037800, 8.314922557961029526, 61.66775706135235424 ) ) ;
#14564=CARTESIAN_POINT ( 'NONE',  ( 4.379528057220339221, -16.55341960407611168, 32.70724293864770260 ) ) ;
#14565=CARTESIAN_POINT ( 'NONE',  ( -5.049401038298153566, 19.05341960407611168, 40.20724293864768839 ) ) ;
#14566=CARTESIAN_POINT ( 'NONE',  ( 9.564922557960805705, 16.46253265017160317, 34.58224293864770260 ) ) ;
#14567=CARTESIAN_POINT ( 'NONE',  ( -12.14591786802326823, 12.06949235617739902, 48.12609039468568284 ) ) ;
#14568=CARTESIAN_POINT ( 'NONE',  ( 16.46253265017146816, 9.564922557961045513, 91.66775706135234714 ) ) ;
#14569=CARTESIAN_POINT ( 'NONE',  ( -12.14591786802309592, -12.06949235617757132, 96.87390960531436690 ) ) ;
#14570=CARTESIAN_POINT ( 'NONE',  ( -9.474510206698964154, 16.51473224551069663, 50.41557627198102409 ) ) ;
#14571=CARTESIAN_POINT ( 'NONE',  ( -19.02544592524334988, -5.153800228976617603, 83.95942372801901854 ) ) ;
#14573=CARTESIAN_POINT ( 'NONE',  ( -18.62759615963255300, -10.81492255796106328, 89.16775706135236135 ) ) ;
#14574=CARTESIAN_POINT ( 'NONE',  ( 16.52544592524335698, 4.483927247898782831, 51.45942372801901854 ) ) ;
#14576=CARTESIAN_POINT ( 'NONE',  ( 21.53943276465977519, -0.05219959533907433946, 53.74890960531437401 ) ) ;
#14577=CARTESIAN_POINT ( 'NONE',  ( -4.379528057220086978, -16.55341960407618274, 39.79275706135235424 ) ) ;
#14578=CARTESIAN_POINT ( 'NONE',  ( -19.46398650005391318, 5.499999999999952038, 70.18269651486372140 ) ) ;
#14579=CARTESIAN_POINT ( 'NONE',  ( 13.97604488694548053, -13.89961937509957401, 40.62609039468564731 ) ) ;
#14580=CARTESIAN_POINT ( 'NONE',  ( 9.564922557960805705, 16.46253265017160317, 84.58224293864769550 ) ) ;
#14581=CARTESIAN_POINT ( 'NONE',  ( -14.29746914071049879, 8.314922557960819915, 105.8322429386476955 ) ) ;
#14582=CARTESIAN_POINT ( 'NONE',  ( -19.03943276465977164, 0.05219959533909376836, 51.24890960531436690 ) ) ;
#14583=CIRCLE ( 'NONE', #1571, 2.000000000000001776 ) ;
#14585=CARTESIAN_POINT ( 'NONE',  ( 21.55341960407619695, -5.719274019375665929, 76.04275706135237556 ) ) ;
#14586=CARTESIAN_POINT ( 'NONE',  ( 30.00000000000000000, -1.132798289211302014E-14, 97.50000000000000000 ) ) ;
#14588=CARTESIAN_POINT ( 'NONE',  ( -0.05219959533936034679, 19.03943276465977164, 27.50109039468566507 ) ) ;
#14589=CARTESIAN_POINT ( 'NONE',  ( 10.81492255796106328, -18.62759615963255655, 110.4177570613523756 ) ) ;
#14590=CARTESIAN_POINT ( 'NONE',  ( -0.05219959533910754901, -16.53943276465976808, 47.49890960531435979 ) ) ;
#14591=CARTESIAN_POINT ( 'NONE',  ( 13.89961937509977652, -13.97604488694527269, 63.12390960531435979 ) ) ;
#14592=CARTESIAN_POINT ( 'NONE',  ( -16.46253265017160317, 9.564922557960807481, 110.8322429386476955 ) ) ;
#14593=CARTESIAN_POINT ( 'NONE',  ( -18.62759615963255300, -10.81492255796106328, 89.16775706135236135 ) ) ;
#14594=CARTESIAN_POINT ( 'NONE',  ( 19.03943276465977164, -0.05219959533909143690, 58.74890960531435979 ) ) ;
#14595=CARTESIAN_POINT ( 'NONE',  ( 5.719274019375673035, 21.55341960407619339, 77.29275706135234714 ) ) ;
#14596=CARTESIAN_POINT ( 'NONE',  ( -21.53943276465977519, 0.05219959533907696930, 41.24890960531435269 ) ) ;
#14597=CARTESIAN_POINT ( 'NONE',  ( -18.62759615963255300, -10.81492255796106328, 34.16775706135234714 ) ) ;
#14598=CARTESIAN_POINT ( 'NONE',  ( 5.049401038297881783, 19.05341960407617563, 62.29275706135234003 ) ) ;
#14599=CARTESIAN_POINT ( 'NONE',  ( 13.89961937509977652, -13.97604488694527269, 33.12390960531434558 ) ) ;
#14600=CARTESIAN_POINT ( 'NONE',  ( -19.02544592524342804, 5.153800228976336051, 71.04057627198099567 ) ) ;
#14601=CARTESIAN_POINT ( 'NONE',  ( -16.53943276465976808, -0.05219959533934237506, 23.75109039468567929 ) ) ;
#14602=CARTESIAN_POINT ( 'NONE',  ( 8.224510206698953496, -14.34966873604960469, 92.91557627198103830 ) ) ;
#14603=CARTESIAN_POINT ( 'NONE',  ( -9.564922557960796823, -16.46253265017161027, 57.08224293864769550 ) ) ;
#14604=CARTESIAN_POINT ( 'NONE',  ( 5.719274019375991003, -21.55341960407610458, 42.70724293864770260 ) ) ;
#14605=CARTESIAN_POINT ( 'NONE',  ( -16.51473224551082808, 9.474510206698731452, 98.33442372801900433 ) ) ;
#14606=CARTESIAN_POINT ( 'NONE',  ( -15.72974639402197994, 15.80617190586746368, 115.6239096053143669 ) ) ;
#14607=CARTESIAN_POINT ( 'NONE',  ( 5.823673210054444382, -21.52544592524334988, 65.20942372801901854 ) ) ;
#14608=CARTESIAN_POINT ( 'NONE',  ( 16.55341960407618274, -4.379528057220086978, 71.04275706135234714 ) ) ;
#14609=CARTESIAN_POINT ( 'NONE',  ( -16.52544592524335698, -4.483927247898792601, 68.95942372801901854 ) ) ;
#14610=CARTESIAN_POINT ( 'NONE',  ( 16.46253265017160672, -9.564922557960803928, 58.33224293864769550 ) ) ;
#14611=CARTESIAN_POINT ( 'NONE',  ( 4.483927247898790824, -16.52544592524335698, 90.20942372801903275 ) ) ;
#14612=CARTESIAN_POINT ( 'NONE',  ( 5.153800228976615827, -19.02544592524334988, 40.20942372801898301 ) ) ;
#14613=CARTESIAN_POINT ( 'NONE',  ( -5.823673210054116645, -21.52544592524344225, 112.2905762719810241 ) ) ;
#14614=CARTESIAN_POINT ( 'NONE',  ( -16.55341960407611168, -4.379528057220339221, 66.45724293864768129 ) ) ;
#14615=CARTESIAN_POINT ( 'NONE',  ( 19.02544592524343514, -5.153800228976328945, 88.54057627198102409 ) ) ;
#14616=CARTESIAN_POINT ( 'NONE',  ( 16.53943276465976808, 0.05219959533934440121, 86.25109039468568994 ) ) ;
#14617=CARTESIAN_POINT ( 'NONE',  ( 5.719274019375673035, 21.55341960407619339, 62.29275706135236845 ) ) ;
#14618=CARTESIAN_POINT ( 'NONE',  ( -12.06949235617739369, -12.14591786802326823, 19.37609039468568639 ) ) ;
#14619=CARTESIAN_POINT ( 'NONE',  ( 18.67979575497194134, -10.72451020669871369, 20.83442372801901143 ) ) ;
#14620=CARTESIAN_POINT ( 'NONE',  ( 0.05219959533910956823, 16.53943276465976808, 59.99890960531436690 ) ) ;
#14621=VERTEX_POINT ( 'NONE', #69351 ) ;
#14622=CARTESIAN_POINT ( 'NONE',  ( 21.55341960407610458, 5.719274019375980345, 83.95724293864770971 ) ) ;
#14623=CARTESIAN_POINT ( 'NONE',  ( 14.34966873604960469, 8.224510206698951720, 44.16557627198103120 ) ) ;
#14626=CARTESIAN_POINT ( 'NONE',  ( 0.05219959533907565091, 21.53943276465977519, 109.9989096053143527 ) ) ;
#14627=CARTESIAN_POINT ( 'NONE',  ( -16.46253265017160317, 9.564922557960807481, 105.8322429386476955 ) ) ;
#14628=CARTESIAN_POINT ( 'NONE',  ( 18.67979575497194134, -10.72451020669871369, 35.83442372801901143 ) ) ;
#14629=CARTESIAN_POINT ( 'NONE',  ( 8.314922557960818139, 14.29746914071049879, 54.58224293864769550 ) ) ;
#14630=CARTESIAN_POINT ( 'NONE',  ( -9.564922557960796823, -16.46253265017161027, 57.08224293864769550 ) ) ;
#14631=CARTESIAN_POINT ( 'NONE',  ( -9.474510206698720793, -16.51473224551083518, 64.58442372801900433 ) ) ;
#14632=CARTESIAN_POINT ( 'NONE',  ( -9.474510206698964154, 16.51473224551069663, 90.41557627198103830 ) ) ;
#14633=CARTESIAN_POINT ( 'NONE',  ( -0.05219959533907301413, -21.53943276465977519, 52.49890960531435979 ) ) ;
#14635=CARTESIAN_POINT ( 'NONE',  ( 19.05341960407611168, 5.049401038298154454, 58.95724293864768129 ) ) ;
#14636=CARTESIAN_POINT ( 'NONE',  ( -12.06949235617739369, -12.14591786802326823, 34.37609039468568284 ) ) ;
#14637=CARTESIAN_POINT ( 'NONE',  ( -13.89961937509957401, -13.97604488694547875, 59.37609039468566863 ) ) ;
#14638=CARTESIAN_POINT ( 'NONE',  ( 15.80617190586746368, 15.72974639402197994, 114.3739096053143527 ) ) ;
#14639=CARTESIAN_POINT ( 'NONE',  ( 4.379528057220339221, -16.55341960407611168, 52.70724293864769550 ) ) ;
#14640=CARTESIAN_POINT ( 'NONE',  ( -5.049401038298153566, 19.05341960407611168, 85.20724293864766707 ) ) ;
#14641=CARTESIAN_POINT ( 'NONE',  ( 5.823673210054125526, 21.52544592524343514, 74.79057627198105251 ) ) ;
#14642=CARTESIAN_POINT ( 'NONE',  ( -21.52544592524343514, 5.823673210054127303, 106.0405762719810525 ) ) ;
#14643=CARTESIAN_POINT ( 'NONE',  ( 12.06949235617739724, 12.14591786802326823, 41.87609039468568284 ) ) ;
#14644=CARTESIAN_POINT ( 'NONE',  ( 21.53943276465977519, -0.05219959533907433946, 38.74890960531435979 ) ) ;
#14645=CARTESIAN_POINT ( 'NONE',  ( -5.823673210054431948, 21.52544592524334988, 102.7094237280190185 ) ) ;
#14646=CARTESIAN_POINT ( 'NONE',  ( 16.46253265017160672, -9.564922557960803928, 93.33224293864769550 ) ) ;
#14647=CARTESIAN_POINT ( 'NONE',  ( 19.05341960407611168, 5.049401038298154454, 43.95724293864769550 ) ) ;
#14648=CARTESIAN_POINT ( 'NONE',  ( 19.03943276465977164, -0.05219959533909143690, 103.7489096053143669 ) ) ;
#14649=CARTESIAN_POINT ( 'NONE',  ( 19.02544592524343514, -5.153800228976328945, 78.54057627198099567 ) ) ;
#14650=CARTESIAN_POINT ( 'NONE',  ( 8.314922557961029526, -14.29746914071037800, 25.41775706135235779 ) ) ;
#14652=CARTESIAN_POINT ( 'NONE',  ( -13.89961937509957401, -13.97604488694547875, 54.37609039468565442 ) ) ;
#14653=CARTESIAN_POINT ( 'NONE',  ( -18.67979575497193778, 10.72451020669871902, 113.3344237280190328 ) ) ;
#14654=CARTESIAN_POINT ( 'NONE',  ( 15.72974639402199770, -15.80617190586745480, 38.12390960531436690 ) ) ;
#14655=CARTESIAN_POINT ( 'NONE',  ( 16.55341960407618274, -4.379528057220086978, 106.0427570613523471 ) ) ;
#14657=CARTESIAN_POINT ( 'NONE',  ( 13.89961937509957401, 13.97604488694547697, 76.87609039468566152 ) ) ;
#14658=CARTESIAN_POINT ( 'NONE',  ( 5.153800228976615827, -19.02544592524334988, 35.20942372801899722 ) ) ;
#14660=CARTESIAN_POINT ( 'NONE',  ( -19.05341960407611168, -5.049401038298163336, 46.45724293864768129 ) ) ;
#14661=CARTESIAN_POINT ( 'NONE',  ( 14.29746914071049879, -8.314922557960816363, 33.33224293864769550 ) ) ;
#14662=CARTESIAN_POINT ( 'NONE',  ( -16.19135201231367915, -7.376712067591919997, 110.1868085405203459 ) ) ;
#14663=CARTESIAN_POINT ( 'NONE',  ( 4.379528057220339221, -16.55341960407611168, 32.70724293864770260 ) ) ;
#14665=CARTESIAN_POINT ( 'NONE',  ( -12.14591786802326823, 12.06949235617739902, 93.12609039468568994 ) ) ;
#14666=CARTESIAN_POINT ( 'NONE',  ( 16.46253265017160672, -9.564922557960803928, 38.33224293864768839 ) ) ;
#14667=CARTESIAN_POINT ( 'NONE',  ( -0.05219959533937732626, 21.53943276465977519, 107.5010903946856899 ) ) ;
#14668=CARTESIAN_POINT ( 'NONE',  ( 8.314922557961029526, -14.29746914071037800, 20.41775706135234714 ) ) ;
#14669=CARTESIAN_POINT ( 'NONE',  ( -0.05219959533937732626, 21.53943276465977519, 82.50109039468568994 ) ) ;
#14671=CARTESIAN_POINT ( 'NONE',  ( -19.02544592524334988, -5.153800228976617603, 63.95942372801899012 ) ) ;
#14672=CARTESIAN_POINT ( 'NONE',  ( -9.564922557960796823, -16.46253265017161027, 97.08224293864769550 ) ) ;
#14673=CARTESIAN_POINT ( 'NONE',  ( 9.564922557960805705, 16.46253265017160317, 89.58224293864769550 ) ) ;
#14675=CARTESIAN_POINT ( 'NONE',  ( 10.81492255796078972, 18.62759615963270932, 109.5822429386476955 ) ) ;
#14677=CARTESIAN_POINT ( 'NONE',  ( -8.314922557960811034, -14.29746914071050412, 67.08224293864770971 ) ) ;
#14678=CARTESIAN_POINT ( 'NONE',  ( -10.72451020669898014, 18.67979575497178502, 60.41557627198102409 ) ) ;
#14679=CARTESIAN_POINT ( 'NONE',  ( 16.51473224551069308, 9.474510206698969483, 59.16557627198102409 ) ) ;
#14680=CARTESIAN_POINT ( 'NONE',  ( -21.52544592524343514, 5.823673210054127303, 101.0405762719810383 ) ) ;
#14681=CARTESIAN_POINT ( 'NONE',  ( -14.34966873604972548, 8.224510206698743886, 88.33442372801901854 ) ) ;
#14683=CARTESIAN_POINT ( 'NONE',  ( 16.51473224551069308, 9.474510206698969483, 59.16557627198102409 ) ) ;
#14684=CARTESIAN_POINT ( 'NONE',  ( 12.06949235617757843, -12.14591786802309237, 93.12390960531436690 ) ) ;
#14686=CARTESIAN_POINT ( 'NONE',  ( 19.05341960407611168, 5.049401038298154454, 48.95724293864768129 ) ) ;
#14687=CARTESIAN_POINT ( 'NONE',  ( 5.153800228976615827, -19.02544592524334988, 75.20942372801896170 ) ) ;
#14688=CARTESIAN_POINT ( 'NONE',  ( -0.05219959533910754901, -16.53943276465976808, 82.49890960531436690 ) ) ;
#14689=CARTESIAN_POINT ( 'NONE',  ( -10.81492255796105439, 18.62759615963255655, 57.91775706135234714 ) ) ;
#14690=CARTESIAN_POINT ( 'NONE',  ( 16.51473224551069308, 9.474510206698969483, 34.16557627198102409 ) ) ;
#14691=CARTESIAN_POINT ( 'NONE',  ( 10.72451020669898902, -18.67979575497178502, 107.9155762719810241 ) ) ;
#14692=CARTESIAN_POINT ( 'NONE',  ( -0.05219959533910754901, -16.53943276465976808, 87.49890960531436690 ) ) ;
#14694=CARTESIAN_POINT ( 'NONE',  ( -16.46253265017160317, 9.564922557960807481, 55.83224293864769550 ) ) ;
#14696=FACE_OUTER_BOUND ( 'NONE', #81979, .T. ) ;
#14697=CARTESIAN_POINT ( 'NONE',  ( -13.89961937509957401, -13.97604488694547875, 89.37609039468563310 ) ) ;
#14698=CARTESIAN_POINT ( 'NONE',  ( -10.81492255796078084, -18.62759615963271287, 22.08224293864769194 ) ) ;
#14699=CARTESIAN_POINT ( 'NONE',  ( -10.81492255796105439, 18.62759615963255655, 42.91775706135235424 ) ) ;
#14700=CARTESIAN_POINT ( 'NONE',  ( 16.51473224551069308, 9.474510206698969483, 79.16557627198103830 ) ) ;
#14701=CARTESIAN_POINT ( 'NONE',  ( -5.049401038297874678, -19.05341960407617918, 74.79275706135231871 ) ) ;
#14702=CARTESIAN_POINT ( 'NONE',  ( 19.02544592524343514, -5.153800228976328945, 53.54057627198102409 ) ) ;
#14704=CARTESIAN_POINT ( 'NONE',  ( -4.379528057220328563, 16.55341960407611168, 75.20724293864769550 ) ) ;
#14705=CARTESIAN_POINT ( 'NONE',  ( 8.224510206698953496, -14.34966873604960469, 67.91557627198102409 ) ) ;
#14706=CARTESIAN_POINT ( 'NONE',  ( -9.474510206698964154, 16.51473224551069663, 90.41557627198103830 ) ) ;
#14707=CARTESIAN_POINT ( 'NONE',  ( 14.29746914071049879, -8.314922557960816363, 73.33224293864769550 ) ) ;
#14708=CARTESIAN_POINT ( 'NONE',  ( 5.153800228976335163, 19.02544592524342804, 89.79057627198102409 ) ) ;
#14710=CARTESIAN_POINT ( 'NONE',  ( 19.05341960407617918, -5.049401038297876454, 36.04275706135234003 ) ) ;
#14711=CARTESIAN_POINT ( 'NONE',  ( -0.05219959533909027116, -19.03943276465977164, 42.49890960531435269 ) ) ;
#14712=CARTESIAN_POINT ( 'NONE',  ( -16.52544592524342804, 4.483927247898546575, 31.04057627198102409 ) ) ;
#14713=CARTESIAN_POINT ( 'NONE',  ( 14.29746914071049879, -8.314922557960816363, 108.3322429386477097 ) ) ;
#14714=ORIENTED_EDGE ( 'NONE', *, *, #107363, .T. ) ;
#14715=CARTESIAN_POINT ( 'NONE',  ( -18.67979575497193778, 10.72451020669871902, 38.33442372801900433 ) ) ;
#14716=CARTESIAN_POINT ( 'NONE',  ( 13.97604488694548053, -13.89961937509957401, 60.62609039468564731 ) ) ;
#14717=CARTESIAN_POINT ( 'NONE',  ( 4.379528057220339221, -16.55341960407611168, 32.70724293864770260 ) ) ;
#14718=CARTESIAN_POINT ( 'NONE',  ( 21.52544592524344225, -5.823673210054117533, 88.54057627198103830 ) ) ;
#14719=CARTESIAN_POINT ( 'NONE',  ( -9.474510206698964154, 16.51473224551069663, 115.4155762719810241 ) ) ;
#14720=CARTESIAN_POINT ( 'NONE',  ( 12.06949235617757843, -12.14591786802309237, 68.12390960531436690 ) ) ;
#14721=CARTESIAN_POINT ( 'NONE',  ( -5.049401038298153566, 19.05341960407611168, 45.20724293864769550 ) ) ;
#14722=CARTESIAN_POINT ( 'NONE',  ( 19.05341960407617918, -5.049401038297876454, 26.04275706135233293 ) ) ;
#14723=CARTESIAN_POINT ( 'NONE',  ( 8.224510206698742110, 14.34966873604972548, 97.08442372801904696 ) ) ;
#14724=CARTESIAN_POINT ( 'NONE',  ( 8.224510206698742110, 14.34966873604972548, 57.08442372801901854 ) ) ;
#14725=CARTESIAN_POINT ( 'NONE',  ( 15.80617190586746368, 15.72974639402197994, 34.37390960531435979 ) ) ;
#14726=CARTESIAN_POINT ( 'NONE',  ( 21.55341960407619695, -5.719274019375665929, 111.0427570613523613 ) ) ;
#14727=CARTESIAN_POINT ( 'NONE',  ( -5.153800228976328057, -19.02544592524343514, 82.29057627198103830 ) ) ;
#14728=CARTESIAN_POINT ( 'NONE',  ( -4.483927247898782831, 16.52544592524335698, 67.70942372801901854 ) ) ;
#14729=CARTESIAN_POINT ( 'NONE',  ( 13.97604488694527802, 13.89961937509977652, 24.37390960531435624 ) ) ;
#14730=CARTESIAN_POINT ( 'NONE',  ( -8.224510206698948167, 14.34966873604960824, 35.41557627198102409 ) ) ;
#14731=CARTESIAN_POINT ( 'NONE',  ( -16.51473224551069308, -9.474510206698971260, 106.6655762719810383 ) ) ;
#14732=CARTESIAN_POINT ( 'NONE',  ( -9.474510206698964154, 16.51473224551069663, 90.41557627198103830 ) ) ;
#14733=CARTESIAN_POINT ( 'NONE',  ( -5.823673210054116645, -21.52544592524344225, 27.29057627198103120 ) ) ;
#14734=CARTESIAN_POINT ( 'NONE',  ( -14.34966873604960291, -8.224510206698953496, 56.66557627198103830 ) ) ;
#14735=CARTESIAN_POINT ( 'NONE',  ( -14.34966873604960291, -8.224510206698953496, 31.66557627198102054 ) ) ;
#14736=EDGE_LOOP ( 'NONE', ( #183241, #96003 ) ) ;
#14737=CARTESIAN_POINT ( 'NONE',  ( -0.05219959533910754901, -16.53943276465976808, 52.49890960531435979 ) ) ;
#14738=CARTESIAN_POINT ( 'NONE',  ( 14.29746914071037800, 8.314922557961029526, 41.66775706135235424 ) ) ;
#14740=CARTESIAN_POINT ( 'NONE',  ( 16.46253265017146816, 9.564922557961045513, 46.66775706135233293 ) ) ;
#14741=CARTESIAN_POINT ( 'NONE',  ( 5.049401038298161559, -19.05341960407611168, 92.70724293864769550 ) ) ;
#14742=CARTESIAN_POINT ( 'NONE',  ( 16.46253265017146816, 9.564922557961045513, 61.66775706135234003 ) ) ;
#14744=CARTESIAN_POINT ( 'NONE',  ( 0.05219959533936267826, -19.03943276465977164, 50.00109039468566863 ) ) ;
#14745=CARTESIAN_POINT ( 'NONE',  ( -0.05219959533936034679, 19.03943276465977164, 97.50109039468567573 ) ) ;
#14746=CARTESIAN_POINT ( 'NONE',  ( 16.52544592524335698, 4.483927247898782831, 76.45942372801901854 ) ) ;
#14748=CARTESIAN_POINT ( 'NONE',  ( 0.05219959533909260263, 19.03943276465977164, 24.99890960531435269 ) ) ;
#14749=CARTESIAN_POINT ( 'NONE',  ( 5.153800228976335163, 19.02544592524342804, 114.7905762719810241 ) ) ;
#14750=CARTESIAN_POINT ( 'NONE',  ( -15.80617190586768217, 15.72974639402176855, 38.12609039468567573 ) ) ;
#14751=CARTESIAN_POINT ( 'NONE',  ( 5.153800228976615827, -19.02544592524334988, 100.2094237280190043 ) ) ;
#14752=CARTESIAN_POINT ( 'NONE',  ( 17.50000000000000000, -3.850315288878792153, 106.7662913060345034 ) ) ;
#14753=CARTESIAN_POINT ( 'NONE',  ( 5.153800228976335163, 19.02544592524342804, 59.79057627198100988 ) ) ;
#14754=CARTESIAN_POINT ( 'NONE',  ( 13.89961937509977652, -13.97604488694527269, 103.1239096053143527 ) ) ;
#14755=CARTESIAN_POINT ( 'NONE',  ( -0.05219959533910754901, -16.53943276465976808, 57.49890960531435979 ) ) ;
#14756=CARTESIAN_POINT ( 'NONE',  ( 0.05219959533909260263, 19.03943276465977164, 69.99890960531435269 ) ) ;
#14757=CARTESIAN_POINT ( 'NONE',  ( -0.05219959533909027116, -19.03943276465977164, 77.49890960531435269 ) ) ;
#14758=CARTESIAN_POINT ( 'NONE',  ( 19.02544592524334988, 5.153800228976608722, 76.45942372801897591 ) ) ;
#14759=CARTESIAN_POINT ( 'NONE',  ( 21.53943276465977519, -0.05219959533907433946, 48.74890960531435979 ) ) ;
#14760=CARTESIAN_POINT ( 'NONE',  ( 4.379528057220339221, -16.55341960407611168, 107.7072429386476955 ) ) ;
#14761=CARTESIAN_POINT ( 'NONE',  ( -5.153800228976607833, 19.02544592524334988, 47.70942372801900433 ) ) ;
#14762=CARTESIAN_POINT ( 'NONE',  ( -16.46253265017160317, 9.564922557960807481, 85.83224293864769550 ) ) ;
#14763=CARTESIAN_POINT ( 'NONE',  ( 18.67979575497178502, 10.72451020669898547, 79.16557627198103830 ) ) ;
#14764=CARTESIAN_POINT ( 'NONE',  ( 8.224510206698953496, -14.34966873604960469, 82.91557627198103830 ) ) ;
#14765=CARTESIAN_POINT ( 'NONE',  ( -13.97604488694547697, 13.89961937509957934, 38.12609039468566152 ) ) ;
#14766=CARTESIAN_POINT ( 'NONE',  ( -15.80617190586745835, -15.72974639402198527, 81.87390960531435269 ) ) ;
#14767=CARTESIAN_POINT ( 'NONE',  ( -10.81492255796078084, -18.62759615963271287, 62.08224293864769550 ) ) ;
#14768=AXIS2_PLACEMENT_3D ( 'NONE', #93141, #154826, #155818 ) ;
#14769=CARTESIAN_POINT ( 'NONE',  ( 15.80617190586746368, 15.72974639402197994, 44.37390960531435979 ) ) ;
#14770=CARTESIAN_POINT ( 'NONE',  ( 21.55341960407619695, -5.719274019375665929, 86.04275706135236135 ) ) ;
#14771=CARTESIAN_POINT ( 'NONE',  ( -13.97604488694527625, -13.89961937509977652, 71.87390960531433848 ) ) ;
#14772=CARTESIAN_POINT ( 'NONE',  ( -8.224510206698948167, 14.34966873604960824, 115.4155762719810241 ) ) ;
#14773=CARTESIAN_POINT ( 'NONE',  ( 15.72974639402176855, 15.80617190586768217, 31.87609039468567929 ) ) ;
#14775=CARTESIAN_POINT ( 'NONE',  ( -18.67979575497193778, 10.72451020669871902, 38.33442372801900433 ) ) ;
#14776=CARTESIAN_POINT ( 'NONE',  ( -5.049401038298153566, 19.05341960407611168, 30.20724293864768839 ) ) ;
#14777=CARTESIAN_POINT ( 'NONE',  ( 15.80617190586746368, 15.72974639402197994, 104.3739096053143669 ) ) ;
#14778=CARTESIAN_POINT ( 'NONE',  ( -0.05219959533936034679, 19.03943276465977164, 47.50109039468566863 ) ) ;
#14779=CARTESIAN_POINT ( 'NONE',  ( -13.89961937509977652, 13.97604488694528158, 40.62390960531435979 ) ) ;
#14782=CARTESIAN_POINT ( 'NONE',  ( 12.14591786802327356, -12.06949235617739191, 65.62609039468568994 ) ) ;
#14783=CARTESIAN_POINT ( 'NONE',  ( -19.02544592524342804, 5.153800228976336051, 31.04057627198102409 ) ) ;
#14785=CARTESIAN_POINT ( 'NONE',  ( 13.97604488694527802, 13.89961937509977652, 79.37390960531435269 ) ) ;
#14786=CARTESIAN_POINT ( 'NONE',  ( -16.55341960407611168, -4.379528057220339221, 106.4572429386477097 ) ) ;
#14787=CARTESIAN_POINT ( 'NONE',  ( 15.72974639402199770, -15.80617190586745480, 53.12390960531436690 ) ) ;
#14788=CARTESIAN_POINT ( 'NONE',  ( -16.52544592524335698, -4.483927247898792601, 48.95942372801902565 ) ) ;
#14789=CARTESIAN_POINT ( 'NONE',  ( -10.81492255796105439, 18.62759615963255655, 102.9177570613523756 ) ) ;
#14790=CARTESIAN_POINT ( 'NONE',  ( -5.049401038298153566, 19.05341960407611168, 25.20724293864768484 ) ) ;
#14791=CARTESIAN_POINT ( 'NONE',  ( 8.224510206698742110, 14.34966873604972548, 112.0844237280190185 ) ) ;
#14792=CARTESIAN_POINT ( 'NONE',  ( -16.52544592524342804, 4.483927247898546575, 51.04057627198103120 ) ) ;
#14793=CARTESIAN_POINT ( 'NONE',  ( -16.51473224551069308, -9.474510206698971260, 56.66557627198103120 ) ) ;
#14794=CARTESIAN_POINT ( 'NONE',  ( 21.53943276465977519, 0.05219959533937863772, 106.2510903946856757 ) ) ;
#14795=CARTESIAN_POINT ( 'NONE',  ( 21.52544592524334988, 5.823673210054432836, 21.45942372801901499 ) ) ;
#14796=CARTESIAN_POINT ( 'NONE',  ( -18.62759615963255300, -10.81492255796106328, 79.16775706135234714 ) ) ;
#14797=CARTESIAN_POINT ( 'NONE',  ( -4.379528057220086978, -16.55341960407618274, 49.79275706135234714 ) ) ;
#14798=CARTESIAN_POINT ( 'NONE',  ( 12.06949235617739724, 12.14591786802326823, 31.87609039468567929 ) ) ;
#14799=CARTESIAN_POINT ( 'NONE',  ( 4.379528057220339221, -16.55341960407611168, 72.70724293864769550 ) ) ;
#14800=CARTESIAN_POINT ( 'NONE',  ( -21.52544592524334988, -5.823673210054445271, 93.95942372801903275 ) ) ;
#14801=CARTESIAN_POINT ( 'NONE',  ( -4.483927247898539470, -16.52544592524342804, 37.29057627198102409 ) ) ;
#14802=CARTESIAN_POINT ( 'NONE',  ( -17.48853670773244673, 5.747243402303102044, 113.6667129974999710 ) ) ;
#14803=CARTESIAN_POINT ( 'NONE',  ( 8.314922557961029526, -14.29746914071037800, 40.41775706135234714 ) ) ;
#14804=CARTESIAN_POINT ( 'NONE',  ( -8.224510206698948167, 14.34966873604960824, 40.41557627198103120 ) ) ;
#14805=CARTESIAN_POINT ( 'NONE',  ( 4.483927247898790824, -16.52544592524335698, 85.20942372801901854 ) ) ;
#14806=CARTESIAN_POINT ( 'NONE',  ( -0.05219959533909027116, -19.03943276465977164, 92.49890960531436690 ) ) ;
#14807=CARTESIAN_POINT ( 'NONE',  ( -19.02544592524342804, 5.153800228976336051, 111.0405762719810099 ) ) ;
#14808=CARTESIAN_POINT ( 'NONE',  ( 21.52544592524334988, 5.823673210054432836, 101.4594237280190185 ) ) ;
#14809=CARTESIAN_POINT ( 'NONE',  ( 16.53943276465976808, 0.05219959533934440121, 101.2510903946856757 ) ) ;
#14810=CARTESIAN_POINT ( 'NONE',  ( 16.55341960407611168, 4.379528057220329451, 73.95724293864769550 ) ) ;
#14811=CARTESIAN_POINT ( 'NONE',  ( 9.564922557960805705, 16.46253265017160317, 84.58224293864769550 ) ) ;
#14813=CARTESIAN_POINT ( 'NONE',  ( -16.55341960407617563, 4.379528057220093196, 38.54275706135234714 ) ) ;
#14814=CARTESIAN_POINT ( 'NONE',  ( -19.03943276465977164, 0.05219959533909376836, 46.24890960531435979 ) ) ;
#14815=CARTESIAN_POINT ( 'NONE',  ( -19.03943276465977164, 0.05219959533909376836, 91.24890960531436690 ) ) ;
#14816=CARTESIAN_POINT ( 'NONE',  ( 8.224510206698742110, 14.34966873604972548, 37.08442372801901143 ) ) ;
#14818=CARTESIAN_POINT ( 'NONE',  ( 16.51473224551083163, -9.474510206698727899, 35.83442372801899722 ) ) ;
#14819=CARTESIAN_POINT ( 'NONE',  ( 16.53943276465976808, 0.05219959533934440121, 111.2510903946856899 ) ) ;
#14820=CARTESIAN_POINT ( 'NONE',  ( -9.474510206698964154, 16.51473224551069663, 30.41557627198102054 ) ) ;
#14821=CARTESIAN_POINT ( 'NONE',  ( 16.52544592524335698, 4.483927247898782831, 76.45942372801901854 ) ) ;
#14822=CARTESIAN_POINT ( 'NONE',  ( 4.379528057220092307, 16.55341960407617563, 67.29275706135234714 ) ) ;
#14823=CARTESIAN_POINT ( 'NONE',  ( 13.97604488694548053, -13.89961937509957401, 80.62609039468567573 ) ) ;
#14824=CARTESIAN_POINT ( 'NONE',  ( 5.153800228976615827, -19.02544592524334988, 30.20942372801900433 ) ) ;
#14825=CARTESIAN_POINT ( 'NONE',  ( 9.564922557960805705, 16.46253265017160317, 59.58224293864769550 ) ) ;
#14826=CARTESIAN_POINT ( 'NONE',  ( -12.06949235617756955, 12.14591786802309770, 90.62390960531436690 ) ) ;
#14827=CARTESIAN_POINT ( 'NONE',  ( 19.03943276465977164, 0.05219959533936151252, 61.25109039468566863 ) ) ;
#14828=CARTESIAN_POINT ( 'NONE',  ( 10.72451020669898902, -18.67979575497178502, 52.91557627198103830 ) ) ;
#14829=CARTESIAN_POINT ( 'NONE',  ( 9.474510206698729675, 16.51473224551082808, 22.08442372801899722 ) ) ;
#14830=CARTESIAN_POINT ( 'NONE',  ( -13.97604488694527625, -13.89961937509977652, 106.8739096053143669 ) ) ;
#14831=CARTESIAN_POINT ( 'NONE',  ( 5.823673210054125526, 21.52544592524343514, 79.79057627198102409 ) ) ;
#14832=CARTESIAN_POINT ( 'NONE',  ( 13.97604488694527802, 13.89961937509977652, 104.3739096053143385 ) ) ;
#14833=CARTESIAN_POINT ( 'NONE',  ( 9.564922557961047289, -16.46253265017146816, 95.41775706135233293 ) ) ;
#14834=CARTESIAN_POINT ( 'NONE',  ( 5.049401038298161559, -19.05341960407611168, 112.7072429386476813 ) ) ;
#14835=CARTESIAN_POINT ( 'NONE',  ( -16.52544592524335698, -4.483927247898792601, 33.95942372801901143 ) ) ;
#14836=CARTESIAN_POINT ( 'NONE',  ( -5.153800228976328057, -19.02544592524343514, 32.29057627198102409 ) ) ;
#14837=CARTESIAN_POINT ( 'NONE',  ( -9.564922557960796823, -16.46253265017161027, 97.08224293864769550 ) ) ;
#14838=CARTESIAN_POINT ( 'NONE',  ( 10.81492255796078972, 18.62759615963270932, 74.58224293864768129 ) ) ;
#14839=CARTESIAN_POINT ( 'NONE',  ( 0.05219959533934541429, -16.53943276465976808, 55.00109039468568284 ) ) ;
#14840=CARTESIAN_POINT ( 'NONE',  ( -18.62759615963255300, -10.81492255796106328, 59.16775706135234714 ) ) ;
#14841=CARTESIAN_POINT ( 'NONE',  ( -5.153800228976607833, 19.02544592524334988, 102.7094237280189759 ) ) ;
#14842=CARTESIAN_POINT ( 'NONE',  ( -19.03943276465977164, -0.05219959533935918106, 18.75109039468567218 ) ) ;
#14843=CARTESIAN_POINT ( 'NONE',  ( 14.34966873604972726, -8.224510206698740333, 110.8344237280190043 ) ) ;
#14844=CARTESIAN_POINT ( 'NONE',  ( 5.823673210054125526, 21.52544592524343514, 99.79057627198103830 ) ) ;
#14845=CARTESIAN_POINT ( 'NONE',  ( 8.314922557960818139, 14.29746914071049879, 34.58224293864770260 ) ) ;
#14846=CARTESIAN_POINT ( 'NONE',  ( -0.05219959533936034679, 19.03943276465977164, 77.50109039468566152 ) ) ;
#14848=CARTESIAN_POINT ( 'NONE',  ( 5.719274019375673035, 21.55341960407619339, 52.29275706135236135 ) ) ;
#14849=CARTESIAN_POINT ( 'NONE',  ( -16.51473224551082808, 9.474510206698731452, 38.33442372801899722 ) ) ;
#14850=CARTESIAN_POINT ( 'NONE',  ( -4.483927247898539470, -16.52544592524342804, 102.2905762719810383 ) ) ;
#14851=CARTESIAN_POINT ( 'NONE',  ( -18.67979575497178146, -10.72451020669898902, 26.66557627198103475 ) ) ;
#14852=CARTESIAN_POINT ( 'NONE',  ( 12.06949235617757843, -12.14591786802309237, 43.12390960531435269 ) ) ;
#14853=EDGE_CURVE ( 'NONE', #9532, #107482, #50757, .T. ) ;
#14854=CARTESIAN_POINT ( 'NONE',  ( -15.72974639402176322, -15.80617190586768395, 104.3760903946856899 ) ) ;
#14855=CARTESIAN_POINT ( 'NONE',  ( 0.05219959533934541429, -16.53943276465976808, 75.00109039468568994 ) ) ;
#14856=CARTESIAN_POINT ( 'NONE',  ( -8.314922557960811034, -14.29746914071050412, 32.08224293864769550 ) ) ;
#14857=CARTESIAN_POINT ( 'NONE',  ( 21.55341960407619695, -5.719274019375665929, 66.04275706135236135 ) ) ;
#14858=CARTESIAN_POINT ( 'NONE',  ( -21.53943276465977519, -0.05219959533937600094, 53.75109039468568994 ) ) ;
#14860=CARTESIAN_POINT ( 'NONE',  ( -19.02544592524342804, 5.153800228976336051, 26.04057627198103120 ) ) ;
#14861=CARTESIAN_POINT ( 'NONE',  ( -21.52544592524334988, -5.823673210054445271, 38.95942372801901854 ) ) ;
#14862=CARTESIAN_POINT ( 'NONE',  ( 0.05219959533909260263, 19.03943276465977164, 24.99890960531435269 ) ) ;
#14863=CARTESIAN_POINT ( 'NONE',  ( 9.564922557960805705, 16.46253265017160317, 39.58224293864768839 ) ) ;
#14864=CARTESIAN_POINT ( 'NONE',  ( 16.55341960407611168, 4.379528057220329451, 83.95724293864770971 ) ) ;
#14865=CARTESIAN_POINT ( 'NONE',  ( 13.97604488694527802, 13.89961937509977652, 74.37390960531436690 ) ) ;
#14866=CARTESIAN_POINT ( 'NONE',  ( -16.55341960407611168, -4.379528057220339221, 31.45724293864769550 ) ) ;
#14867=CARTESIAN_POINT ( 'NONE',  ( 5.823673210054125526, 21.52544592524343514, 54.79057627198104541 ) ) ;
#14868=CARTESIAN_POINT ( 'NONE',  ( -14.29746914071049879, 8.314922557960819915, 90.83224293864769550 ) ) ;
#14870=CARTESIAN_POINT ( 'NONE',  ( -18.67979575497178146, -10.72451020669898902, 101.6655762719810383 ) ) ;
#14871=CARTESIAN_POINT ( 'NONE',  ( -0.05219959533909027116, -19.03943276465977164, 102.4989096053143669 ) ) ;
#14872=CARTESIAN_POINT ( 'NONE',  ( -19.05341960407611168, -5.049401038298163336, 61.45724293864769550 ) ) ;
#14873=CARTESIAN_POINT ( 'NONE',  ( -13.89961937509957401, -13.97604488694547875, 109.3760903946856331 ) ) ;
#14874=CARTESIAN_POINT ( 'NONE',  ( 18.67979575497178502, 10.72451020669898547, 54.16557627198103120 ) ) ;
#14875=CARTESIAN_POINT ( 'NONE',  ( 0.05219959533937995610, -21.53943276465977519, 75.00109039468568994 ) ) ;
#14876=CARTESIAN_POINT ( 'NONE',  ( -16.51473224551069308, -9.474510206698971260, 66.66557627198102409 ) ) ;
#14877=CARTESIAN_POINT ( 'NONE',  ( 19.05341960407611168, 5.049401038298154454, 103.9572429386476671 ) ) ;
#14878=CARTESIAN_POINT ( 'NONE',  ( -8.224510206698735004, -14.34966873604973081, 74.58442372801901854 ) ) ;
#14879=CARTESIAN_POINT ( 'NONE',  ( -18.62759615963255300, -10.81492255796106328, 59.16775706135234714 ) ) ;
#14880=CARTESIAN_POINT ( 'NONE',  ( -21.55341960407619339, 5.719274019375674811, 83.54275706135234714 ) ) ;
#14881=CARTESIAN_POINT ( 'NONE',  ( 10.72451020669898902, -18.67979575497178502, 107.9155762719810241 ) ) ;
#14882=CARTESIAN_POINT ( 'NONE',  ( -14.34966873604972548, 8.224510206698743886, 73.33442372801901854 ) ) ;
#14883=CARTESIAN_POINT ( 'NONE',  ( -10.72451020669898014, 18.67979575497178502, 70.41557627198102409 ) ) ;
#14884=CARTESIAN_POINT ( 'NONE',  ( 19.05341960407617918, -5.049401038297876454, 51.04275706135231871 ) ) ;
#14885=CARTESIAN_POINT ( 'NONE',  ( -15.80617190586745835, -15.72974639402198527, 41.87390960531435979 ) ) ;
#14886=CARTESIAN_POINT ( 'NONE',  ( -19.02544592524342804, 5.153800228976336051, 76.04057627198102409 ) ) ;
#14887=CARTESIAN_POINT ( 'NONE',  ( -12.14591786802309592, -12.06949235617757132, 21.87390960531436690 ) ) ;
#14888=CARTESIAN_POINT ( 'NONE',  ( -16.79531203550650531, 7.028104445595468874, 63.74755011779561897 ) ) ;
#14889=CARTESIAN_POINT ( 'NONE',  ( -9.474510206698964154, 16.51473224551069663, 115.4155762719810241 ) ) ;
#14891=CARTESIAN_POINT ( 'NONE',  ( -0.05219959533936034679, 19.03943276465977164, 92.50109039468566152 ) ) ;
#14892=CARTESIAN_POINT ( 'NONE',  ( -21.55341960407610458, -5.719274019375992779, 76.45724293864769550 ) ) ;
#14893=CARTESIAN_POINT ( 'NONE',  ( -8.314922557960811034, -14.29746914071050412, 52.08224293864768839 ) ) ;
#14894=CARTESIAN_POINT ( 'NONE',  ( 8.224510206698742110, 14.34966873604972548, 22.08442372801901143 ) ) ;
#14895=CARTESIAN_POINT ( 'NONE',  ( 19.05341960407611168, 5.049401038298154454, 48.95724293864768129 ) ) ;
#14896=CARTESIAN_POINT ( 'NONE',  ( -0.05219959533907301413, -21.53943276465977519, 97.49890960531436690 ) ) ;
#14897=CARTESIAN_POINT ( 'NONE',  ( 9.564922557961047289, -16.46253265017146816, 75.41775706135234714 ) ) ;
#14898=CARTESIAN_POINT ( 'NONE',  ( -0.05219959533909027116, -19.03943276465977164, 82.49890960531436690 ) ) ;
#14899=CARTESIAN_POINT ( 'NONE',  ( -8.224510206698948167, 14.34966873604960824, 80.41557627198103830 ) ) ;
#14900=CARTESIAN_POINT ( 'NONE',  ( -13.89961937509977652, 13.97604488694528158, 60.62390960531436690 ) ) ;
#14901=CARTESIAN_POINT ( 'NONE',  ( 14.29746914071049879, -8.314922557960816363, 68.33224293864769550 ) ) ;
#14902=CARTESIAN_POINT ( 'NONE',  ( 19.02544592524343514, -5.153800228976328945, 33.54057627198102409 ) ) ;
#14904=CARTESIAN_POINT ( 'NONE',  ( 14.29746914071049879, -8.314922557960816363, 43.33224293864769550 ) ) ;
#14905=CARTESIAN_POINT ( 'NONE',  ( -19.05341960407611168, -5.049401038298163336, 91.45724293864766707 ) ) ;
#14907=CARTESIAN_POINT ( 'NONE',  ( -16.51473224551082808, 9.474510206698731452, 48.33442372801900433 ) ) ;
#14908=CARTESIAN_POINT ( 'NONE',  ( -14.29746914071037622, -8.314922557961029526, 59.16775706135234714 ) ) ;
#14910=CARTESIAN_POINT ( 'NONE',  ( -15.72974639402197994, 15.80617190586746368, 60.62390960531437401 ) ) ;
#14911=CARTESIAN_POINT ( 'NONE',  ( -19.02544592524334988, -5.153800228976617603, 33.95942372801897591 ) ) ;
#14912=CARTESIAN_POINT ( 'NONE',  ( -5.153800228976328057, -19.02544592524343514, 92.29057627198099567 ) ) ;
#14913=CARTESIAN_POINT ( 'NONE',  ( -18.22780087662124160, -5.499999999999927169, 83.98236817873107896 ) ) ;
#14914=CARTESIAN_POINT ( 'NONE',  ( -18.67979575497178146, -10.72451020669898902, 26.66557627198103475 ) ) ;
#14915=CARTESIAN_POINT ( 'NONE',  ( 5.153800228976335163, 19.02544592524342804, 59.79057627198100988 ) ) ;
#14916=CARTESIAN_POINT ( 'NONE',  ( 18.62759615963255655, 10.81492255796105972, 51.66775706135234714 ) ) ;
#14917=CARTESIAN_POINT ( 'NONE',  ( 16.55341960407611168, 4.379528057220329451, 113.9572429386477239 ) ) ;
#14919=CARTESIAN_POINT ( 'NONE',  ( 21.53943276465977519, -0.05219959533907433946, 98.74890960531438111 ) ) ;
#14920=CARTESIAN_POINT ( 'NONE',  ( -0.05219959533909027116, -19.03943276465977164, 97.49890960531436690 ) ) ;
#14921=ORIENTED_EDGE ( 'NONE', *, *, #169635, .F. ) ;
#14922=CARTESIAN_POINT ( 'NONE',  ( 5.823673210054444382, -21.52544592524334988, 35.20942372801901854 ) ) ;
#14924=CARTESIAN_POINT ( 'NONE',  ( 13.97604488694527802, 13.89961937509977652, 104.3739096053143385 ) ) ;
#14926=CARTESIAN_POINT ( 'NONE',  ( 21.55341960407610458, 5.719274019375980345, 88.95724293864769550 ) ) ;
#14927=CARTESIAN_POINT ( 'NONE',  ( -16.46253265017160317, 9.564922557960807481, 45.83224293864769550 ) ) ;
#14928=CARTESIAN_POINT ( 'NONE',  ( 16.52544592524335698, 4.483927247898782831, 21.45942372801901499 ) ) ;
#14930=CARTESIAN_POINT ( 'NONE',  ( -16.51473224551069308, -9.474510206698971260, 31.66557627198102054 ) ) ;
#14931=CARTESIAN_POINT ( 'NONE',  ( -0.05219959533937732626, 21.53943276465977519, 102.5010903946856899 ) ) ;
#14932=CARTESIAN_POINT ( 'NONE',  ( -16.46253265017160317, 9.564922557960807481, 75.83224293864769550 ) ) ;
#14933=CARTESIAN_POINT ( 'NONE',  ( 18.62759615963255655, 10.81492255796105972, 46.66775706135234714 ) ) ;
#14935=CARTESIAN_POINT ( 'NONE',  ( 16.46253265017160672, -9.564922557960803928, 93.33224293864769550 ) ) ;
#14937=CARTESIAN_POINT ( 'NONE',  ( 8.224510206698742110, 14.34966873604972548, 37.08442372801901143 ) ) ;
#14938=CARTESIAN_POINT ( 'NONE',  ( -16.53943276465976808, -0.05219959533934237506, 68.75109039468568994 ) ) ;
#14939=CARTESIAN_POINT ( 'NONE',  ( -21.55341960407619339, 5.719274019375674811, 53.54275706135234714 ) ) ;
#14940=CARTESIAN_POINT ( 'NONE',  ( 0.05219959533937995610, -21.53943276465977519, 85.00109039468568994 ) ) ;
#14942=CARTESIAN_POINT ( 'NONE',  ( -13.89961937509957401, -13.97604488694547875, 104.3760903946856757 ) ) ;
#14943=CARTESIAN_POINT ( 'NONE',  ( 19.03943276465977164, -0.05219959533909143690, 78.74890960531436690 ) ) ;
#14944=CARTESIAN_POINT ( 'NONE',  ( -5.153800228976328057, -19.02544592524343514, 92.29057627198099567 ) ) ;
#14945=CARTESIAN_POINT ( 'NONE',  ( -12.14591786802309592, -12.06949235617757132, 111.8739096053143669 ) ) ;
#14946=CARTESIAN_POINT ( 'NONE',  ( -18.67979575497178146, -10.72451020669898902, 26.66557627198103475 ) ) ;
#14947=CARTESIAN_POINT ( 'NONE',  ( 8.314922557961029526, -14.29746914071037800, 90.41775706135236135 ) ) ;
#14948=CARTESIAN_POINT ( 'NONE',  ( 4.483927247898545687, 16.52544592524342804, 74.79057627198105251 ) ) ;
#14949=CARTESIAN_POINT ( 'NONE',  ( -9.474510206698964154, 16.51473224551069663, 60.41557627198102409 ) ) ;
#14950=CARTESIAN_POINT ( 'NONE',  ( -21.53943276465977519, -0.05219959533937600094, 78.75109039468568994 ) ) ;
#14952=CARTESIAN_POINT ( 'NONE',  ( 16.51473224551083163, -9.474510206698727899, 100.8344237280190043 ) ) ;
#14953=CARTESIAN_POINT ( 'NONE',  ( 16.52544592524342804, -4.483927247898539470, 78.54057627198103830 ) ) ;
#14954=CARTESIAN_POINT ( 'NONE',  ( -21.55341960407619339, 5.719274019375674811, 33.54275706135234714 ) ) ;
#14955=CARTESIAN_POINT ( 'NONE',  ( -5.719274019375978568, 21.55341960407610458, 65.20724293864768129 ) ) ;
#14956=CARTESIAN_POINT ( 'NONE',  ( -16.62475595723698873, -7.163666690055295660, 104.4728664818953519 ) ) ;
#14958=CARTESIAN_POINT ( 'NONE',  ( 13.97604488694527802, 13.89961937509977652, 79.37390960531435269 ) ) ;
#14959=CARTESIAN_POINT ( 'NONE',  ( -0.05219959533910754901, -16.53943276465976808, 52.49890960531435979 ) ) ;
#14960=CARTESIAN_POINT ( 'NONE',  ( -12.06949235617756955, 12.14591786802309770, 40.62390960531435269 ) ) ;
#14961=CARTESIAN_POINT ( 'NONE',  ( -8.224510206698735004, -14.34966873604973081, 99.58442372801900433 ) ) ;
#14962=CARTESIAN_POINT ( 'NONE',  ( 9.564922557961047289, -16.46253265017146816, 55.41775706135234003 ) ) ;
#14964=CARTESIAN_POINT ( 'NONE',  ( 19.02544592524343514, -5.153800228976328945, 98.54057627198100988 ) ) ;
#14965=CARTESIAN_POINT ( 'NONE',  ( 16.52544592524342804, -4.483927247898539470, 68.54057627198103830 ) ) ;
#14966=CARTESIAN_POINT ( 'NONE',  ( -5.153800228976607833, 19.02544592524334988, 42.70942372801901143 ) ) ;
#14967=CARTESIAN_POINT ( 'NONE',  ( -13.97604488694527625, -13.89961937509977652, 36.87390960531436690 ) ) ;
#14968=CARTESIAN_POINT ( 'NONE',  ( 0.05219959533907565091, 21.53943276465977519, 34.99890960531435979 ) ) ;
#14969=CARTESIAN_POINT ( 'NONE',  ( -21.53943276465977519, 0.05219959533907696930, 61.24890960531435979 ) ) ;
#14970=CARTESIAN_POINT ( 'NONE',  ( -8.224510206698948167, 14.34966873604960824, 95.41557627198102409 ) ) ;
#14971=CARTESIAN_POINT ( 'NONE',  ( -12.06949235617739369, -12.14591786802326823, 49.37609039468569705 ) ) ;
#14972=CARTESIAN_POINT ( 'NONE',  ( 18.62759615963255655, 10.81492255796105972, 36.66775706135234714 ) ) ;
#14973=CARTESIAN_POINT ( 'NONE',  ( 12.06949235617757843, -12.14591786802309237, 93.12390960531436690 ) ) ;
#14974=CARTESIAN_POINT ( 'NONE',  ( 16.62475595723696387, -7.163666690055227271, 38.02713351810466946 ) ) ;
#14975=CARTESIAN_POINT ( 'NONE',  ( -16.79531203550651242, 7.028104445595470651, 48.74755011779559055 ) ) ;
#14976=CARTESIAN_POINT ( 'NONE',  ( 15.72974639402199770, -15.80617190586745480, 33.12390960531435979 ) ) ;
#14979=CARTESIAN_POINT ( 'NONE',  ( -4.483927247898782831, 16.52544592524335698, 37.70942372801900433 ) ) ;
#14980=CARTESIAN_POINT ( 'NONE',  ( 14.34966873604960469, 8.224510206698951720, 29.16557627198103120 ) ) ;
#14981=CARTESIAN_POINT ( 'NONE',  ( 21.55341960407610458, 5.719274019375980345, 73.95724293864769550 ) ) ;
#14982=CARTESIAN_POINT ( 'NONE',  ( -19.05341960407617563, 5.049401038297882671, 83.54275706135233293 ) ) ;
#14983=CARTESIAN_POINT ( 'NONE',  ( -18.62759615963270932, 10.81492255796079327, 65.83224293864769550 ) ) ;
#14985=CARTESIAN_POINT ( 'NONE',  ( -12.06949235617739369, -12.14591786802326823, 49.37609039468569705 ) ) ;
#14986=CARTESIAN_POINT ( 'NONE',  ( 19.03943276465977164, -0.05219959533909143690, 33.74890960531435979 ) ) ;
#14987=CARTESIAN_POINT ( 'NONE',  ( 5.049401038298161559, -19.05341960407611168, 107.7072429386476955 ) ) ;
#14988=CARTESIAN_POINT ( 'NONE',  ( 9.564922557960805705, 16.46253265017160317, 39.58224293864768839 ) ) ;
#14989=CARTESIAN_POINT ( 'NONE',  ( -9.474510206698964154, 16.51473224551069663, 25.41557627198103120 ) ) ;
#14991=CARTESIAN_POINT ( 'NONE',  ( -16.46253265017160317, 9.564922557960807481, 115.8322429386477097 ) ) ;
#14993=CARTESIAN_POINT ( 'NONE',  ( 12.14591786802327356, -12.06949235617739191, 70.62609039468567573 ) ) ;
#14994=CARTESIAN_POINT ( 'NONE',  ( -21.55341960407610458, -5.719274019375992779, 91.45724293864769550 ) ) ;
#14995=CARTESIAN_POINT ( 'NONE',  ( -9.564922557960796823, -16.46253265017161027, 57.08224293864769550 ) ) ;
#14996=CARTESIAN_POINT ( 'NONE',  ( -5.823673210054431948, 21.52544592524334988, 32.70942372801900433 ) ) ;
#14997=CARTESIAN_POINT ( 'NONE',  ( 19.02544592524343514, -5.153800228976328945, 83.54057627198100988 ) ) ;
#14998=CARTESIAN_POINT ( 'NONE',  ( 19.02544592524343514, -5.153800228976328945, 113.5405762719810241 ) ) ;
#14999=ORIENTED_EDGE ( 'NONE', *, *, #143971, .T. ) ;
#15000=CARTESIAN_POINT ( 'NONE',  ( -5.823673210054431948, 21.52544592524334988, 22.70942372801901499 ) ) ;
#15001=CARTESIAN_POINT ( 'NONE',  ( 13.89961937509977652, -13.97604488694527269, 28.12390960531435624 ) ) ;
#15002=CARTESIAN_POINT ( 'NONE',  ( -13.97604488694527625, -13.89961937509977652, 106.8739096053143669 ) ) ;
#15003=CARTESIAN_POINT ( 'NONE',  ( 9.564922557961047289, -16.46253265017146816, 90.41775706135234714 ) ) ;
#15004=CARTESIAN_POINT ( 'NONE',  ( -16.51473224551082808, 9.474510206698731452, 28.33442372801900433 ) ) ;
#15005=CARTESIAN_POINT ( 'NONE',  ( -10.72451020669898014, 18.67979575497178502, 105.4155762719810383 ) ) ;
#15006=CARTESIAN_POINT ( 'NONE',  ( -9.564922557961040184, 16.46253265017147172, 37.91775706135233293 ) ) ;
#15007=CARTESIAN_POINT ( 'NONE',  ( -16.53943276465976808, -0.05219959533934237506, 73.75109039468567573 ) ) ;
#15008=CARTESIAN_POINT ( 'NONE',  ( -9.564922557960796823, -16.46253265017161027, 102.0822429386477097 ) ) ;
#15009=CARTESIAN_POINT ( 'NONE',  ( 13.89961937509977652, -13.97604488694527269, 58.12390960531436690 ) ) ;
#15011=CARTESIAN_POINT ( 'NONE',  ( -0.05219959533937732626, 21.53943276465977519, 62.50109039468568284 ) ) ;
#15012=CARTESIAN_POINT ( 'NONE',  ( 21.53943276465977519, 0.05219959533937863772, 81.25109039468568994 ) ) ;
#15013=CARTESIAN_POINT ( 'NONE',  ( 19.05341960407611168, 5.049401038298154454, 113.9572429386477097 ) ) ;
#15014=CARTESIAN_POINT ( 'NONE',  ( -5.153800228976328057, -19.02544592524343514, 77.29057627198099567 ) ) ;
#15015=CARTESIAN_POINT ( 'NONE',  ( -15.72974639402176322, -15.80617190586768395, 49.37609039468569705 ) ) ;
#15016=CARTESIAN_POINT ( 'NONE',  ( 16.46253265017146816, 9.564922557961045513, 86.66775706135233293 ) ) ;
#15017=CARTESIAN_POINT ( 'NONE',  ( -19.05341960407611168, -5.049401038298163336, 46.45724293864768129 ) ) ;
#15018=CARTESIAN_POINT ( 'NONE',  ( 5.153800228976335163, 19.02544592524342804, 104.7905762719809957 ) ) ;
#15019=CARTESIAN_POINT ( 'NONE',  ( 9.564922557960805705, 16.46253265017160317, 64.58224293864769550 ) ) ;
#15020=CARTESIAN_POINT ( 'NONE',  ( 17.50000000000000000, -3.556245443207693313, 22.75258077879468388 ) ) ;
#15021=CARTESIAN_POINT ( 'NONE',  ( 13.89961937509977652, -13.97604488694527269, 58.12390960531436690 ) ) ;
#15022=CARTESIAN_POINT ( 'NONE',  ( -21.53943276465977519, 0.05219959533907696930, 106.2489096053143811 ) ) ;
#15023=CARTESIAN_POINT ( 'NONE',  ( 16.52544592524335698, 4.483927247898782831, 86.45942372801901854 ) ) ;
#15025=CARTESIAN_POINT ( 'NONE',  ( -13.89961937509957401, -13.97604488694547875, 49.37609039468567573 ) ) ;
#15026=CARTESIAN_POINT ( 'NONE',  ( -16.46253265017160317, 9.564922557960807481, 80.83224293864769550 ) ) ;
#15027=CARTESIAN_POINT ( 'NONE',  ( 12.06949235617757843, -12.14591786802309237, 63.12390960531435979 ) ) ;
#15028=CARTESIAN_POINT ( 'NONE',  ( -8.224510206698948167, 14.34966873604960824, 95.41557627198102409 ) ) ;
#15029=CARTESIAN_POINT ( 'NONE',  ( 5.049401038298161559, -19.05341960407611168, 112.7072429386476813 ) ) ;
#15030=ORIENTED_EDGE ( 'NONE', *, *, #126618, .T. ) ;
#15031=CARTESIAN_POINT ( 'NONE',  ( 9.564922557960805705, 16.46253265017160317, 99.58224293864770971 ) ) ;
#15032=CARTESIAN_POINT ( 'NONE',  ( -19.05341960407611168, -5.049401038298163336, 111.4572429386476671 ) ) ;
#15033=CARTESIAN_POINT ( 'NONE',  ( -9.564922557961040184, 16.46253265017147172, 22.91775706135233648 ) ) ;
#15034=CARTESIAN_POINT ( 'NONE',  ( -4.379528057220086978, -16.55341960407618274, 94.79275706135234714 ) ) ;
#15035=CARTESIAN_POINT ( 'NONE',  ( 0.05219959533909260263, 19.03943276465977164, 74.99890960531435269 ) ) ;
#15036=CARTESIAN_POINT ( 'NONE',  ( 21.55341960407619695, -5.719274019375665929, 36.04275706135234714 ) ) ;
#15037=CARTESIAN_POINT ( 'NONE',  ( 10.72451020669898902, -18.67979575497178502, 32.91557627198102409 ) ) ;
#15038=CARTESIAN_POINT ( 'NONE',  ( -21.52544592524343514, 5.823673210054127303, 111.0405762719810525 ) ) ;
#15039=CARTESIAN_POINT ( 'NONE',  ( 15.72974639402199770, -15.80617190586745480, 73.12390960531436690 ) ) ;
#15040=CARTESIAN_POINT ( 'NONE',  ( 4.379528057220339221, -16.55341960407611168, 82.70724293864770971 ) ) ;
#15041=CARTESIAN_POINT ( 'NONE',  ( -16.51473224551082808, 9.474510206698731452, 43.33442372801900433 ) ) ;
#15042=CARTESIAN_POINT ( 'NONE',  ( -16.46253265017160317, 9.564922557960807481, 35.83224293864768839 ) ) ;
#15043=CARTESIAN_POINT ( 'NONE',  ( 9.474510206698971260, -16.51473224551069308, 77.91557627198103830 ) ) ;
#15044=CARTESIAN_POINT ( 'NONE',  ( -13.97604488694527625, -13.89961937509977652, 76.87390960531433848 ) ) ;
#15046=CARTESIAN_POINT ( 'NONE',  ( -4.379528057220328563, 16.55341960407611168, 95.20724293864769550 ) ) ;
#15048=CARTESIAN_POINT ( 'NONE',  ( -8.224510206698948167, 14.34966873604960824, 25.41557627198103120 ) ) ;
#15049=CARTESIAN_POINT ( 'NONE',  ( -14.29746914071037622, -8.314922557961029526, 24.16775706135235424 ) ) ;
#15050=CARTESIAN_POINT ( 'NONE',  ( 0.05219959533937995610, -21.53943276465977519, 90.00109039468567573 ) ) ;
#15051=CARTESIAN_POINT ( 'NONE',  ( -5.049401038298153566, 19.05341960407611168, 100.2072429386476955 ) ) ;
#15052=CARTESIAN_POINT ( 'NONE',  ( 21.55341960407619695, -5.719274019375665929, 26.04275706135235779 ) ) ;
#15053=CARTESIAN_POINT ( 'NONE',  ( 9.564922557960805705, 16.46253265017160317, 39.58224293864768839 ) ) ;
#15055=CARTESIAN_POINT ( 'NONE',  ( 14.34966873604972726, -8.224510206698740333, 40.83442372801901854 ) ) ;
#15056=CARTESIAN_POINT ( 'NONE',  ( -13.97604488694547697, 13.89961937509957934, 103.1260903946856473 ) ) ;
#15057=CARTESIAN_POINT ( 'NONE',  ( 5.823673210054125526, 21.52544592524343514, 104.7905762719810241 ) ) ;
#15058=CARTESIAN_POINT ( 'NONE',  ( -16.46253265017146816, -9.564922557961047289, 64.16775706135233293 ) ) ;
#15060=CARTESIAN_POINT ( 'NONE',  ( -5.719274019375665041, -21.55341960407619695, 19.79275706135235069 ) ) ;
#15062=CARTESIAN_POINT ( 'NONE',  ( 9.474510206698971260, -16.51473224551069308, 92.91557627198103830 ) ) ;
#15064=CARTESIAN_POINT ( 'NONE',  ( 9.564922557960805705, 16.46253265017160317, 89.58224293864769550 ) ) ;
#15065=CARTESIAN_POINT ( 'NONE',  ( -21.55341960407619339, 5.719274019375674811, 38.54275706135234714 ) ) ;
#15066=CARTESIAN_POINT ( 'NONE',  ( -16.53943276465976808, 0.05219959533911058130, 76.24890960531435269 ) ) ;
#15067=CARTESIAN_POINT ( 'NONE',  ( -19.02544592524342804, 5.153800228976336051, 81.04057627198103830 ) ) ;
#15068=CARTESIAN_POINT ( 'NONE',  ( 16.55341960407618274, -4.379528057220086978, 46.04275706135234714 ) ) ;
#15069=CARTESIAN_POINT ( 'NONE',  ( -13.97604488694547697, 13.89961937509957934, 53.12609039468565442 ) ) ;
#15070=CARTESIAN_POINT ( 'NONE',  ( 15.80617190586769283, -15.72974639402175789, 70.62609039468567573 ) ) ;
#15071=CARTESIAN_POINT ( 'NONE',  ( -14.34966873604972548, 8.224510206698743886, 28.33442372801902209 ) ) ;
#15072=CARTESIAN_POINT ( 'NONE',  ( 16.51473224551069308, 9.474510206698969483, 64.16557627198102409 ) ) ;
#15074=CARTESIAN_POINT ( 'NONE',  ( 9.564922557961047289, -16.46253265017146816, 90.41775706135234714 ) ) ;
#15075=CARTESIAN_POINT ( 'NONE',  ( 16.53943276465976808, 0.05219959533934440121, 51.25109039468568994 ) ) ;
#15076=CARTESIAN_POINT ( 'NONE',  ( 15.72974639402176855, 15.80617190586768217, 96.87609039468568994 ) ) ;
#15077=CARTESIAN_POINT ( 'NONE',  ( -13.97604488694547697, 13.89961937509957934, 83.12609039468564731 ) ) ;
#15078=CARTESIAN_POINT ( 'NONE',  ( 19.05341960407611168, 5.049401038298154454, 43.95724293864769550 ) ) ;
#15079=CARTESIAN_POINT ( 'NONE',  ( -15.72974639402197994, 15.80617190586746368, 75.62390960531439532 ) ) ;
#15080=CARTESIAN_POINT ( 'NONE',  ( 14.29746914071049879, -8.314922557960816363, 73.33224293864769550 ) ) ;
#15081=CARTESIAN_POINT ( 'NONE',  ( -19.02544592524334988, -5.153800228976617603, 78.95942372801900433 ) ) ;
#15082=CARTESIAN_POINT ( 'NONE',  ( 15.50000000000000355, 5.499999999999998224, 118.0000000000000142 ) ) ;
#15083=CARTESIAN_POINT ( 'NONE',  ( 9.474510206698729675, 16.51473224551082808, 37.08442372801899722 ) ) ;
#15084=CARTESIAN_POINT ( 'NONE',  ( -14.34966873604960291, -8.224510206698953496, 21.66557627198102409 ) ) ;
#15085=CARTESIAN_POINT ( 'NONE',  ( -8.224510206698948167, 14.34966873604960824, 60.41557627198102409 ) ) ;
#15086=CARTESIAN_POINT ( 'NONE',  ( -15.80617190586768217, 15.72974639402176855, 103.1260903946856757 ) ) ;
#15088=CARTESIAN_POINT ( 'NONE',  ( 15.80617190586746368, 15.72974639402197994, 114.3739096053143527 ) ) ;
#15090=CARTESIAN_POINT ( 'NONE',  ( 9.564922557960805705, 16.46253265017160317, 69.58224293864770971 ) ) ;
#15091=CARTESIAN_POINT ( 'NONE',  ( -15.72974639402176322, -15.80617190586768395, 84.37609039468570415 ) ) ;
#15092=CARTESIAN_POINT ( 'NONE',  ( -5.049401038298153566, 19.05341960407611168, 60.20724293864768129 ) ) ;
#15094=CARTESIAN_POINT ( 'NONE',  ( 9.564922557960805705, 16.46253265017160317, 29.58224293864769550 ) ) ;
#15095=CARTESIAN_POINT ( 'NONE',  ( -21.53943276465977519, 0.05219959533907696930, 36.24890960531435979 ) ) ;
#15096=CARTESIAN_POINT ( 'NONE',  ( -12.06949235617756955, 12.14591786802309770, 60.62390960531437401 ) ) ;
#15097=CARTESIAN_POINT ( 'NONE',  ( -16.46253265017160317, 9.564922557960807481, 25.83224293864769194 ) ) ;
#15098=CARTESIAN_POINT ( 'NONE',  ( -12.14591786802309592, -12.06949235617757132, 86.87390960531438111 ) ) ;
#15099=CARTESIAN_POINT ( 'NONE',  ( 10.81492255796078972, 18.62759615963270932, 99.58224293864770971 ) ) ;
#15100=CARTESIAN_POINT ( 'NONE',  ( 21.55341960407619695, -5.719274019375665929, 46.04275706135234714 ) ) ;
#15102=CARTESIAN_POINT ( 'NONE',  ( 14.34966873604972726, -8.224510206698740333, 50.83442372801901143 ) ) ;
#15103=CARTESIAN_POINT ( 'NONE',  ( -15.80617190586745835, -15.72974639402198527, 101.8739096053143811 ) ) ;
#15104=CARTESIAN_POINT ( 'NONE',  ( -5.153800228976607833, 19.02544592524334988, 32.70942372801899722 ) ) ;
#15105=CARTESIAN_POINT ( 'NONE',  ( -0.05219959533909027116, -19.03943276465977164, 32.49890960531435979 ) ) ;
#15106=CARTESIAN_POINT ( 'NONE',  ( 13.89961937509977652, -13.97604488694527269, 103.1239096053143527 ) ) ;
#15107=CARTESIAN_POINT ( 'NONE',  ( -21.55341960407619339, 5.719274019375674811, 63.54275706135234003 ) ) ;
#15108=CARTESIAN_POINT ( 'NONE',  ( -21.53943276465977519, 0.05219959533907696930, 41.24890960531435269 ) ) ;
#15109=CARTESIAN_POINT ( 'NONE',  ( -12.14591786802326823, 12.06949235617739902, 113.1260903946856899 ) ) ;
#15110=CARTESIAN_POINT ( 'NONE',  ( 5.823673210054444382, -21.52544592524334988, 70.20942372801904696 ) ) ;
#15111=CARTESIAN_POINT ( 'NONE',  ( 10.72451020669871369, 18.67979575497193778, 92.08442372801901854 ) ) ;
#15112=CARTESIAN_POINT ( 'NONE',  ( -5.049401038297874678, -19.05341960407617918, 34.79275706135233293 ) ) ;
#15113=CARTESIAN_POINT ( 'NONE',  ( -12.06949235617739369, -12.14591786802326823, 89.37609039468568994 ) ) ;
#15114=CARTESIAN_POINT ( 'NONE',  ( 5.823673210054444382, -21.52544592524334988, 55.20942372801902565 ) ) ;
#15115=CARTESIAN_POINT ( 'NONE',  ( 19.05341960407611168, 5.049401038298154454, 43.95724293864769550 ) ) ;
#15116=CARTESIAN_POINT ( 'NONE',  ( 13.97604488694548053, -13.89961937509957401, 25.62609039468566507 ) ) ;
#15117=CARTESIAN_POINT ( 'NONE',  ( 19.05341960407611168, 5.049401038298154454, 113.9572429386477097 ) ) ;
#15118=CARTESIAN_POINT ( 'NONE',  ( -10.72451020669898014, 18.67979575497178502, 110.4155762719810383 ) ) ;
#15119=CARTESIAN_POINT ( 'NONE',  ( 18.67979575497178502, 10.72451020669898547, 69.16557627198102409 ) ) ;
#15120=CARTESIAN_POINT ( 'NONE',  ( 14.29746914071037800, 8.314922557961029526, 41.66775706135235424 ) ) ;
#15122=CARTESIAN_POINT ( 'NONE',  ( -21.53943276465977519, 0.05219959533907696930, 76.24890960531435269 ) ) ;
#15123=CARTESIAN_POINT ( 'NONE',  ( -0.05219959533934338120, 16.53943276465976808, 67.50109039468568994 ) ) ;
#15124=CARTESIAN_POINT ( 'NONE',  ( -14.29746914071049879, 8.314922557960819915, 60.83224293864769550 ) ) ;
#15126=CARTESIAN_POINT ( 'NONE',  ( -9.474510206698720793, -16.51473224551083518, 99.58442372801900433 ) ) ;
#15127=CARTESIAN_POINT ( 'NONE',  ( 15.72974639402199770, -15.80617190586745480, 38.12390960531436690 ) ) ;
#15129=CARTESIAN_POINT ( 'NONE',  ( -16.52544592524335698, -4.483927247898792601, 33.95942372801901143 ) ) ;
#15130=CARTESIAN_POINT ( 'NONE',  ( -0.05219959533907301413, -21.53943276465977519, 112.4989096053143669 ) ) ;
#15131=CARTESIAN_POINT ( 'NONE',  ( 15.72974639402199770, -15.80617190586745480, 38.12390960531436690 ) ) ;
#15132=CARTESIAN_POINT ( 'NONE',  ( -16.53943276465976808, -0.05219959533934237506, 58.75109039468568994 ) ) ;
#15133=CARTESIAN_POINT ( 'NONE',  ( 19.02544592524343514, -5.153800228976328945, 78.54057627198099567 ) ) ;
#15134=CARTESIAN_POINT ( 'NONE',  ( 0.05219959533937995610, -21.53943276465977519, 40.00109039468567573 ) ) ;
#15135=CARTESIAN_POINT ( 'NONE',  ( 5.153800228976615827, -19.02544592524334988, 110.2094237280189901 ) ) ;
#15136=CARTESIAN_POINT ( 'NONE',  ( 5.823673210054125526, 21.52544592524343514, 29.79057627198102409 ) ) ;
#15138=CARTESIAN_POINT ( 'NONE',  ( 9.474510206698729675, 16.51473224551082808, 27.08442372801900433 ) ) ;
#15139=CARTESIAN_POINT ( 'NONE',  ( -4.379528057220086978, -16.55341960407618274, 44.79275706135234714 ) ) ;
#15140=CARTESIAN_POINT ( 'NONE',  ( -19.03943276465977164, 0.05219959533909376836, 96.24890960531436690 ) ) ;
#15141=CARTESIAN_POINT ( 'NONE',  ( 21.55341960407610458, 5.719274019375980345, 98.95724293864770971 ) ) ;
#15142=CARTESIAN_POINT ( 'NONE',  ( 19.02544592524343514, -5.153800228976328945, 78.54057627198099567 ) ) ;
#15144=CARTESIAN_POINT ( 'NONE',  ( 14.29746914071049879, -8.314922557960816363, 83.33224293864769550 ) ) ;
#15145=CARTESIAN_POINT ( 'NONE',  ( 0.05219959533907565091, 21.53943276465977519, 29.99890960531435979 ) ) ;
#15146=CARTESIAN_POINT ( 'NONE',  ( -17.40805194822030799, 6.112264579159341515, 35.83371272510612471 ) ) ;
#15147=CARTESIAN_POINT ( 'NONE',  ( 4.483927247898790824, -16.52544592524335698, 70.20942372801904696 ) ) ;
#15148=CARTESIAN_POINT ( 'NONE',  ( 21.53943276465977519, 0.05219959533937863772, 26.25109039468567573 ) ) ;
#15149=CARTESIAN_POINT ( 'NONE',  ( -16.51473224551082808, 9.474510206698731452, 78.33442372801900433 ) ) ;
#15150=CARTESIAN_POINT ( 'NONE',  ( -0.05219959533909027116, -19.03943276465977164, 27.49890960531435624 ) ) ;
#15151=CARTESIAN_POINT ( 'NONE',  ( -5.719274019375978568, 21.55341960407610458, 70.20724293864769550 ) ) ;
#15153=CARTESIAN_POINT ( 'NONE',  ( -5.049401038298153566, 19.05341960407611168, 105.2072429386476671 ) ) ;
#15154=CARTESIAN_POINT ( 'NONE',  ( -21.53943276465977519, -0.05219959533937600094, 88.75109039468567573 ) ) ;
#15155=CARTESIAN_POINT ( 'NONE',  ( -13.89961937509977652, 13.97604488694528158, 65.62390960531436690 ) ) ;
#15157=CARTESIAN_POINT ( 'NONE',  ( -14.34966873604972548, 8.224510206698743886, 48.33442372801902565 ) ) ;
#15158=CARTESIAN_POINT ( 'NONE',  ( -13.89961937509977652, 13.97604488694528158, 60.62390960531436690 ) ) ;
#15159=CARTESIAN_POINT ( 'NONE',  ( 18.67979575497194134, -10.72451020669871369, 85.83442372801901854 ) ) ;
#15160=VERTEX_POINT ( 'NONE', #179559 ) ;
#15161=CARTESIAN_POINT ( 'NONE',  ( -13.97604488694547697, 13.89961937509957934, 33.12609039468566863 ) ) ;
#15162=CARTESIAN_POINT ( 'NONE',  ( -9.474510206698720793, -16.51473224551083518, 49.58442372801899722 ) ) ;
#15163=CARTESIAN_POINT ( 'NONE',  ( -15.80617190586768217, 15.72974639402176855, 48.12609039468568284 ) ) ;
#15165=CARTESIAN_POINT ( 'NONE',  ( 16.51473224551069308, 9.474510206698969483, 54.16557627198103120 ) ) ;
#15166=CARTESIAN_POINT ( 'NONE',  ( 19.05341960407617918, -5.049401038297876454, 46.04275706135233293 ) ) ;
#15167=CARTESIAN_POINT ( 'NONE',  ( 19.02544592524343514, -5.153800228976328945, 98.54057627198100988 ) ) ;
#15168=CARTESIAN_POINT ( 'NONE',  ( 5.153800228976335163, 19.02544592524342804, 64.79057627198100988 ) ) ;
#15169=CARTESIAN_POINT ( 'NONE',  ( 0.05219959533910956823, 16.53943276465976808, 24.99890960531435624 ) ) ;
#15170=CARTESIAN_POINT ( 'NONE',  ( -21.52544592524343514, 5.823673210054127303, 26.04057627198103475 ) ) ;
#15171=CARTESIAN_POINT ( 'NONE',  ( 10.81492255796106328, -18.62759615963255655, 105.4177570613523613 ) ) ;
#15174=CARTESIAN_POINT ( 'NONE',  ( -5.719274019375665041, -21.55341960407619695, 104.7927570613523898 ) ) ;
#15176=CARTESIAN_POINT ( 'NONE',  ( -13.89961937509977652, 13.97604488694528158, 25.62390960531434558 ) ) ;
#15179=CARTESIAN_POINT ( 'NONE',  ( -0.05219959533934338120, 16.53943276465976808, 47.50109039468568994 ) ) ;
#15180=CARTESIAN_POINT ( 'NONE',  ( 0.05219959533907565091, 21.53943276465977519, 64.99890960531435269 ) ) ;
#15181=CARTESIAN_POINT ( 'NONE',  ( 16.52544592524342804, -4.483927247898539470, 38.54057627198103120 ) ) ;
#15182=CARTESIAN_POINT ( 'NONE',  ( -16.55341960407611168, -4.379528057220339221, 106.4572429386477097 ) ) ;
#15183=CARTESIAN_POINT ( 'NONE',  ( 19.05341960407611168, 5.049401038298154454, 93.95724293864769550 ) ) ;
#15184=CARTESIAN_POINT ( 'NONE',  ( 9.474510206698729675, 16.51473224551082808, 32.08442372801900433 ) ) ;
#15185=CARTESIAN_POINT ( 'NONE',  ( -12.06949235617756955, 12.14591786802309770, 110.6239096053143669 ) ) ;
#15186=CARTESIAN_POINT ( 'NONE',  ( 5.823673210054444382, -21.52544592524334988, 70.20942372801904696 ) ) ;
#15188=CARTESIAN_POINT ( 'NONE',  ( -16.55341960407617563, 4.379528057220093196, 103.5427570613523613 ) ) ;
#15190=CARTESIAN_POINT ( 'NONE',  ( 5.719274019375991003, -21.55341960407610458, 27.70724293864769905 ) ) ;
#15191=CARTESIAN_POINT ( 'NONE',  ( -16.53943276465976808, 0.05219959533911058130, 96.24890960531435269 ) ) ;
#15192=CARTESIAN_POINT ( 'NONE',  ( -16.46253265017146816, -9.564922557961047289, 54.16775706135234003 ) ) ;
#15193=CARTESIAN_POINT ( 'NONE',  ( 16.46253265017160672, -9.564922557960803928, 78.33224293864769550 ) ) ;
#15194=CARTESIAN_POINT ( 'NONE',  ( 16.52544592524342804, -4.483927247898539470, 73.54057627198102409 ) ) ;
#15195=CARTESIAN_POINT ( 'NONE',  ( 19.05341960407617918, -5.049401038297876454, 91.04275706135234714 ) ) ;
#15196=CARTESIAN_POINT ( 'NONE',  ( -15.80617190586745835, -15.72974639402198527, 46.87390960531435979 ) ) ;
#15198=CARTESIAN_POINT ( 'NONE',  ( 12.06949235617757843, -12.14591786802309237, 108.1239096053143811 ) ) ;
#15199=B_SPLINE_CURVE_WITH_KNOTS ( 'NONE', 3,
 ( #40541, #163900, #10211, #87038, #71871, #164894 ),
 .UNSPECIFIED., .F., .F.,
 ( 4, 2, 4 ),
 ( 0.007228050697041583060, 0.007608510107495075961, 0.007988969517948567994 ),
 .UNSPECIFIED. ) ;
#15200=CARTESIAN_POINT ( 'NONE',  ( -17.40861289039004589, -6.110651285853283987, 31.37232470827432707 ) ) ;
#15201=CARTESIAN_POINT ( 'NONE',  ( 19.03943276465977164, -0.05219959533909143690, 68.74890960531436690 ) ) ;
#15202=CARTESIAN_POINT ( 'NONE',  ( -21.52544592524343514, 5.823673210054127303, 76.04057627198102409 ) ) ;
#15203=CARTESIAN_POINT ( 'NONE',  ( 14.34966873604972726, -8.224510206698740333, 90.83442372801901854 ) ) ;
#15204=CARTESIAN_POINT ( 'NONE',  ( 19.03943276465977164, -0.05219959533909143690, 88.74890960531436690 ) ) ;
#15205=CARTESIAN_POINT ( 'NONE',  ( -0.05219959533936034679, 19.03943276465977164, 72.50109039468566152 ) ) ;
#15206=CARTESIAN_POINT ( 'NONE',  ( 21.53943276465977519, 0.05219959533937863772, 76.25109039468568994 ) ) ;
#15207=CARTESIAN_POINT ( 'NONE',  ( -15.72974639402197994, 15.80617190586746368, 60.62390960531437401 ) ) ;
#15208=CARTESIAN_POINT ( 'NONE',  ( -5.823673210054116645, -21.52544592524344225, 27.29057627198103120 ) ) ;
#15209=CARTESIAN_POINT ( 'NONE',  ( 16.46253265017160672, -9.564922557960803928, 33.33224293864770260 ) ) ;
#15210=CARTESIAN_POINT ( 'NONE',  ( -16.52544592524335698, -4.483927247898792601, 98.95942372801903275 ) ) ;
#15211=CARTESIAN_POINT ( 'NONE',  ( -19.03943276465977164, 0.05219959533909376836, 46.24890960531435979 ) ) ;
#15212=CARTESIAN_POINT ( 'NONE',  ( 12.14591786802327356, -12.06949235617739191, 25.62609039468567929 ) ) ;
#15214=CARTESIAN_POINT ( 'NONE',  ( -18.67979575497193778, 10.72451020669871902, 108.3344237280190185 ) ) ;
#15215=CARTESIAN_POINT ( 'NONE',  ( -8.314922557960811034, -14.29746914071050412, 57.08224293864769550 ) ) ;
#15216=CARTESIAN_POINT ( 'NONE',  ( 15.80617190586746368, 15.72974639402197994, 109.3739096053143811 ) ) ;
#15217=CARTESIAN_POINT ( 'NONE',  ( -5.823673210054116645, -21.52544592524344225, 107.2905762719810525 ) ) ;
#15219=CARTESIAN_POINT ( 'NONE',  ( -15.80617190586745835, -15.72974639402198527, 46.87390960531435979 ) ) ;
#15220=CARTESIAN_POINT ( 'NONE',  ( 16.53943276465976808, 0.05219959533934440121, 76.25109039468568994 ) ) ;
#15221=CARTESIAN_POINT ( 'NONE',  ( 14.29746914071049879, -8.314922557960816363, 88.33224293864769550 ) ) ;
#15222=CARTESIAN_POINT ( 'NONE',  ( 19.02544592524343514, -5.153800228976328945, 63.54057627198103830 ) ) ;
#15224=CARTESIAN_POINT ( 'NONE',  ( -4.483927247898539470, -16.52544592524342804, 22.29057627198102765 ) ) ;
#15225=CARTESIAN_POINT ( 'NONE',  ( 10.81492255796106328, -18.62759615963255655, 30.41775706135234358 ) ) ;
#15226=CARTESIAN_POINT ( 'NONE',  ( -5.153800228976328057, -19.02544592524343514, 97.29057627198099567 ) ) ;
#15227=CARTESIAN_POINT ( 'NONE',  ( -18.62759615963255300, -10.81492255796106328, 64.16775706135234714 ) ) ;
#15229=CARTESIAN_POINT ( 'NONE',  ( -19.05341960407611168, -5.049401038298163336, 31.45724293864769550 ) ) ;
#15230=ORIENTED_EDGE ( 'NONE', *, *, #65989, .F. ) ;
#15231=CARTESIAN_POINT ( 'NONE',  ( -15.80617190586768217, 15.72974639402176855, 53.12609039468568284 ) ) ;
#15232=CARTESIAN_POINT ( 'NONE',  ( -19.03943276465977164, 0.05219959533909376836, 46.24890960531435979 ) ) ;
#15233=CARTESIAN_POINT ( 'NONE',  ( -13.89961937509977652, 13.97604488694528158, 95.62390960531436690 ) ) ;
#15234=CARTESIAN_POINT ( 'NONE',  ( -16.51473224551082808, 9.474510206698731452, 78.33442372801900433 ) ) ;
#15235=CARTESIAN_POINT ( 'NONE',  ( 21.53943276465977519, 0.05219959533937863772, 36.25109039468567573 ) ) ;
#15236=CARTESIAN_POINT ( 'NONE',  ( -5.153800228976607833, 19.02544592524334988, 107.7094237280189759 ) ) ;
#15237=CARTESIAN_POINT ( 'NONE',  ( 16.46253265017146816, 9.564922557961045513, 71.66775706135233293 ) ) ;
#15238=CARTESIAN_POINT ( 'NONE',  ( -16.51473224551069308, -9.474510206698971260, 36.66557627198102409 ) ) ;
#15239=CARTESIAN_POINT ( 'NONE',  ( -5.049401038297874678, -19.05341960407617918, 79.79275706135233293 ) ) ;
#15240=CARTESIAN_POINT ( 'NONE',  ( -4.483927247898782831, 16.52544592524335698, 102.7094237280190185 ) ) ;
#15241=CARTESIAN_POINT ( 'NONE',  ( 13.97604488694548053, -13.89961937509957401, 80.62609039468567573 ) ) ;
#15242=CARTESIAN_POINT ( 'NONE',  ( -8.314922557960811034, -14.29746914071050412, 37.08224293864768129 ) ) ;
#15243=CARTESIAN_POINT ( 'NONE',  ( 0.05219959533936267826, -19.03943276465977164, 50.00109039468566863 ) ) ;
#15244=CARTESIAN_POINT ( 'NONE',  ( 15.72974639402176855, 15.80617190586768217, 101.8760903946857042 ) ) ;
#15245=CARTESIAN_POINT ( 'NONE',  ( -13.89961937509957401, -13.97604488694547875, 19.37609039468566507 ) ) ;
#15246=CARTESIAN_POINT ( 'NONE',  ( -13.89961937509977652, 13.97604488694528158, 35.62390960531435269 ) ) ;
#15247=CARTESIAN_POINT ( 'NONE',  ( -15.72974639402176322, -15.80617190586768395, 94.37609039468568994 ) ) ;
#15248=CARTESIAN_POINT ( 'NONE',  ( 0.05219959533934541429, -16.53943276465976808, 45.00109039468568284 ) ) ;
#15249=CARTESIAN_POINT ( 'NONE',  ( 19.02544592524343514, -5.153800228976328945, 88.54057627198102409 ) ) ;
#15252=CARTESIAN_POINT ( 'NONE',  ( 9.564922557960805705, 16.46253265017160317, 84.58224293864769550 ) ) ;
#15253=CARTESIAN_POINT ( 'NONE',  ( 17.59632111031626067, -2.707012485672555702, 102.5000000000000284 ) ) ;
#15254=ORIENTED_EDGE ( 'NONE', *, *, #184219, .F. ) ;
#15255=CARTESIAN_POINT ( 'NONE',  ( -0.05219959533936034679, 19.03943276465977164, 87.50109039468567573 ) ) ;
#15256=CARTESIAN_POINT ( 'NONE',  ( -18.67979575497178146, -10.72451020669898902, 21.66557627198102409 ) ) ;
#15257=CARTESIAN_POINT ( 'NONE',  ( -18.67979575497193778, 10.72451020669871902, 113.3344237280190328 ) ) ;
#15258=CARTESIAN_POINT ( 'NONE',  ( 9.564922557961047289, -16.46253265017146816, 95.41775706135233293 ) ) ;
#15259=CARTESIAN_POINT ( 'NONE',  ( 16.52544592524342804, -4.483927247898539470, 98.54057627198105251 ) ) ;
#15260=CARTESIAN_POINT ( 'NONE',  ( -9.474510206698964154, 16.51473224551069663, 30.41557627198102054 ) ) ;
#15261=CARTESIAN_POINT ( 'NONE',  ( 21.53943276465977519, -0.05219959533907433946, 58.74890960531436690 ) ) ;
#15262=CARTESIAN_POINT ( 'NONE',  ( -21.52544592524343514, 5.823673210054127303, 51.04057627198103120 ) ) ;
#15263=CARTESIAN_POINT ( 'NONE',  ( -19.05341960407611168, -5.049401038298163336, 21.45724293864768839 ) ) ;
#15265=CARTESIAN_POINT ( 'NONE',  ( -5.153800228976607833, 19.02544592524334988, 67.70942372801900433 ) ) ;
#15266=CARTESIAN_POINT ( 'NONE',  ( -12.14591786802309592, -12.06949235617757132, 41.87390960531435979 ) ) ;
#15267=CARTESIAN_POINT ( 'NONE',  ( 13.97604488694527802, 13.89961937509977652, 114.3739096053143669 ) ) ;
#15268=CARTESIAN_POINT ( 'NONE',  ( 10.72451020669871369, 18.67979575497193778, 77.08442372801901854 ) ) ;
#15269=CARTESIAN_POINT ( 'NONE',  ( 0.05219959533907565091, 21.53943276465977519, 69.99890960531435269 ) ) ;
#15270=CARTESIAN_POINT ( 'NONE',  ( -10.72451020669870658, -18.67979575497194134, 64.58442372801900433 ) ) ;
#15271=CARTESIAN_POINT ( 'NONE',  ( -15.80617190586768217, 15.72974639402176855, 53.12609039468568284 ) ) ;
#15272=CARTESIAN_POINT ( 'NONE',  ( -9.564922557960796823, -16.46253265017161027, 102.0822429386477097 ) ) ;
#15273=CARTESIAN_POINT ( 'NONE',  ( 8.314922557961029526, -14.29746914071037800, 90.41775706135236135 ) ) ;
#15274=CARTESIAN_POINT ( 'NONE',  ( -16.51473224551069308, -9.474510206698971260, 26.66557627198103120 ) ) ;
#15276=CARTESIAN_POINT ( 'NONE',  ( 12.06949235617757843, -12.14591786802309237, 73.12390960531436690 ) ) ;
#15277=CARTESIAN_POINT ( 'NONE',  ( 4.483927247898545687, 16.52544592524342804, 39.79057627198103830 ) ) ;
#15278=CARTESIAN_POINT ( 'NONE',  ( -16.46253265017160317, 9.564922557960807481, 60.83224293864769550 ) ) ;
#15279=CARTESIAN_POINT ( 'NONE',  ( 19.05341960407611168, 5.049401038298154454, 38.95724293864767418 ) ) ;
#15280=CARTESIAN_POINT ( 'NONE',  ( 18.67979575497178502, 10.72451020669898547, 44.16557627198103120 ) ) ;
#15281=CARTESIAN_POINT ( 'NONE',  ( 19.05341960407617918, -5.049401038297876454, 36.04275706135234003 ) ) ;
#15284=CARTESIAN_POINT ( 'NONE',  ( 0.05219959533910956823, 16.53943276465976808, 49.99890960531437401 ) ) ;
#15285=CARTESIAN_POINT ( 'NONE',  ( 10.72451020669898902, -18.67979575497178502, 27.91557627198103830 ) ) ;
#15287=CARTESIAN_POINT ( 'NONE',  ( -16.52544592524335698, -4.483927247898792601, 73.95942372801901854 ) ) ;
#15288=CARTESIAN_POINT ( 'NONE',  ( 19.05341960407617918, -5.049401038297876454, 81.04275706135231871 ) ) ;
#15289=CARTESIAN_POINT ( 'NONE',  ( -16.55341960407611168, -4.379528057220339221, 46.45724293864769550 ) ) ;
#15290=CARTESIAN_POINT ( 'NONE',  ( 15.50000000000000178, -7.500000000000000888, 20.00000000000000000 ) ) ;
#15291=CARTESIAN_POINT ( 'NONE',  ( 14.29746914071049879, -8.314922557960816363, 28.33224293864769550 ) ) ;
#15292=CARTESIAN_POINT ( 'NONE',  ( 16.51473224551069308, 9.474510206698969483, 49.16557627198102409 ) ) ;
#15293=CARTESIAN_POINT ( 'NONE',  ( 5.153800228976335163, 19.02544592524342804, 79.79057627198102409 ) ) ;
#15294=CARTESIAN_POINT ( 'NONE',  ( 19.05341960407611168, 5.049401038298154454, 43.95724293864769550 ) ) ;
#15295=CARTESIAN_POINT ( 'NONE',  ( -5.823673210054431948, 21.52544592524334988, 42.70942372801901854 ) ) ;
#15296=CARTESIAN_POINT ( 'NONE',  ( 5.153800228976335163, 19.02544592524342804, 64.79057627198100988 ) ) ;
#15298=CARTESIAN_POINT ( 'NONE',  ( 0.05219959533909260263, 19.03943276465977164, 44.99890960531435979 ) ) ;
#15299=CARTESIAN_POINT ( 'NONE',  ( 5.719274019375991003, -21.55341960407610458, 42.70724293864770260 ) ) ;
#15300=CARTESIAN_POINT ( 'NONE',  ( -0.05219959533937732626, 21.53943276465977519, 67.50109039468568994 ) ) ;
#15301=CARTESIAN_POINT ( 'NONE',  ( 14.34966873604960469, 8.224510206698951720, 114.1655762719810383 ) ) ;
#15302=CARTESIAN_POINT ( 'NONE',  ( 18.67979575497178502, 10.72451020669898547, 24.16557627198103120 ) ) ;
#15303=CARTESIAN_POINT ( 'NONE',  ( -16.52544592524335698, -4.483927247898792601, 88.95942372801901854 ) ) ;
#15304=CARTESIAN_POINT ( 'NONE',  ( -10.72451020669870658, -18.67979575497194134, 99.58442372801900433 ) ) ;
#15306=CARTESIAN_POINT ( 'NONE',  ( 16.52544592524335698, 4.483927247898782831, 66.45942372801903275 ) ) ;
#15307=CARTESIAN_POINT ( 'NONE',  ( 9.564922557960805705, 16.46253265017160317, 109.5822429386476955 ) ) ;
#15308=CARTESIAN_POINT ( 'NONE',  ( 8.224510206698742110, 14.34966873604972548, 57.08442372801901854 ) ) ;
#15309=CARTESIAN_POINT ( 'NONE',  ( -8.224510206698735004, -14.34966873604973081, 44.58442372801901854 ) ) ;
#15310=CARTESIAN_POINT ( 'NONE',  ( 16.52544592524335698, 4.483927247898782831, 101.4594237280190185 ) ) ;
#15311=CARTESIAN_POINT ( 'NONE',  ( -15.72974639402176322, -15.80617190586768395, 49.37609039468569705 ) ) ;
#15312=CARTESIAN_POINT ( 'NONE',  ( 14.29746914071037800, 8.314922557961029526, 21.66775706135235069 ) ) ;
#15313=CARTESIAN_POINT ( 'NONE',  ( -21.53943276465977519, 0.05219959533907696930, 111.2489096053143669 ) ) ;
#15314=CARTESIAN_POINT ( 'NONE',  ( 12.06949235617739724, 12.14591786802326823, 21.87609039468567573 ) ) ;
#15315=CARTESIAN_POINT ( 'NONE',  ( 0.05219959533934541429, -16.53943276465976808, 90.00109039468567573 ) ) ;
#15316=CARTESIAN_POINT ( 'NONE',  ( -16.62475595723610411, 7.163666690055881858, 45.52713351810403708 ) ) ;
#15317=CARTESIAN_POINT ( 'NONE',  ( -18.62759615963255300, -10.81492255796106328, 84.16775706135234714 ) ) ;
#15318=CARTESIAN_POINT ( 'NONE',  ( -19.03943276465977164, -0.05219959533935918106, 83.75109039468567573 ) ) ;
#15319=CARTESIAN_POINT ( 'NONE',  ( 12.14591786802309770, 12.06949235617756955, 59.37390960531436690 ) ) ;
#15320=CARTESIAN_POINT ( 'NONE',  ( 12.14591786802309770, 12.06949235617756955, 44.37390960531435979 ) ) ;
#15321=CARTESIAN_POINT ( 'NONE',  ( -4.483927247898539470, -16.52544592524342804, 112.2905762719810241 ) ) ;
#15322=CARTESIAN_POINT ( 'NONE',  ( -16.51473224551082808, 9.474510206698731452, 53.33442372801900433 ) ) ;
#15324=CARTESIAN_POINT ( 'NONE',  ( -18.62759615963255300, -10.81492255796106328, 49.16775706135234003 ) ) ;
#15325=CARTESIAN_POINT ( 'NONE',  ( -9.564922557961040184, 16.46253265017147172, 107.9177570613523471 ) ) ;
#15327=CARTESIAN_POINT ( 'NONE',  ( -19.05341960407611168, -5.049401038298163336, 101.4572429386476955 ) ) ;
#15328=CARTESIAN_POINT ( 'NONE',  ( -21.53943276465977519, 0.05219959533907696930, 76.24890960531435269 ) ) ;
#15329=CARTESIAN_POINT ( 'NONE',  ( 16.46253265017146816, 9.564922557961045513, 101.6677570613523329 ) ) ;
#15330=ADVANCED_FACE ( 'NONE', ( #168337 ), #24239, .F. ) ;
#15331=CARTESIAN_POINT ( 'NONE',  ( -16.46253265017160317, 9.564922557960807481, 105.8322429386476955 ) ) ;
#15333=CARTESIAN_POINT ( 'NONE',  ( 14.34966873604960469, 8.224510206698951720, 104.1655762719810241 ) ) ;
#15334=CARTESIAN_POINT ( 'NONE',  ( 18.67979575497194134, -10.72451020669871369, 100.8344237280190185 ) ) ;
#15335=CARTESIAN_POINT ( 'NONE',  ( 5.153800228976335163, 19.02544592524342804, 24.79057627198102765 ) ) ;
#15337=CARTESIAN_POINT ( 'NONE',  ( 10.72451020669871369, 18.67979575497193778, 57.08442372801901854 ) ) ;
#15338=CARTESIAN_POINT ( 'NONE',  ( 15.80617190586769283, -15.72974639402175789, 90.62609039468567573 ) ) ;
#15339=CARTESIAN_POINT ( 'NONE',  ( -4.379528057220086978, -16.55341960407618274, 94.79275706135234714 ) ) ;
#15340=EDGE_CURVE ( 'NONE', #67326, #33580, #137405, .T. ) ;
#15341=CARTESIAN_POINT ( 'NONE',  ( 18.62759615963255655, 10.81492255796105972, 41.66775706135235424 ) ) ;
#15342=CARTESIAN_POINT ( 'NONE',  ( 21.53943276465977519, 0.05219959533937863772, 46.25109039468567573 ) ) ;
#15343=CARTESIAN_POINT ( 'NONE',  ( -5.153800228976607833, 19.02544592524334988, 67.70942372801900433 ) ) ;
#15344=CARTESIAN_POINT ( 'NONE',  ( -19.05341960407611168, -5.049401038298163336, 96.45724293864769550 ) ) ;
#15345=CARTESIAN_POINT ( 'NONE',  ( 16.55341960407611168, 4.379528057220329451, 108.9572429386476955 ) ) ;
#15346=CARTESIAN_POINT ( 'NONE',  ( 15.72974639402199770, -15.80617190586745480, 78.12390960531436690 ) ) ;
#15347=CARTESIAN_POINT ( 'NONE',  ( -16.53943276465976808, 0.05219959533911058130, 61.24890960531435979 ) ) ;
#15348=CARTESIAN_POINT ( 'NONE',  ( -5.823673210054431948, 21.52544592524334988, 97.70942372801904696 ) ) ;
#15349=CARTESIAN_POINT ( 'NONE',  ( 16.52544592524342804, -4.483927247898539470, 83.54057627198102409 ) ) ;
#15350=CARTESIAN_POINT ( 'NONE',  ( -19.02544592524342804, 5.153800228976336051, 36.04057627198100988 ) ) ;
#15351=CARTESIAN_POINT ( 'NONE',  ( -19.03943276465977164, -0.05219959533935918106, 73.75109039468566152 ) ) ;
#15352=CARTESIAN_POINT ( 'NONE',  ( 8.314922557960818139, 14.29746914071049879, 44.58224293864769550 ) ) ;
#15353=CARTESIAN_POINT ( 'NONE',  ( 21.53943276465977519, 0.05219959533937863772, 101.2510903946856757 ) ) ;
#15354=CARTESIAN_POINT ( 'NONE',  ( -9.564922557960796823, -16.46253265017161027, 97.08224293864769550 ) ) ;
#15355=CARTESIAN_POINT ( 'NONE',  ( 16.51473224551083163, -9.474510206698727899, 55.83442372801899722 ) ) ;
#15356=CARTESIAN_POINT ( 'NONE',  ( -18.62759615963270932, 10.81492255796079327, 65.83224293864769550 ) ) ;
#15357=CARTESIAN_POINT ( 'NONE',  ( 10.81492255796106328, -18.62759615963255655, 20.41775706135234714 ) ) ;
#15358=CARTESIAN_POINT ( 'NONE',  ( -16.52544592524335698, -4.483927247898792601, 18.95942372801901143 ) ) ;
#15359=CARTESIAN_POINT ( 'NONE',  ( -14.29746914071037622, -8.314922557961029526, 79.16775706135234714 ) ) ;
#15360=CARTESIAN_POINT ( 'NONE',  ( -9.474510206698964154, 16.51473224551069663, 25.41557627198103120 ) ) ;
#15361=CARTESIAN_POINT ( 'NONE',  ( -15.80617190586768217, 15.72974639402176855, 23.12609039468567573 ) ) ;
#15362=CARTESIAN_POINT ( 'NONE',  ( 16.55341960407611168, 4.379528057220329451, 113.9572429386477239 ) ) ;
#15364=CARTESIAN_POINT ( 'NONE',  ( -8.224510206698735004, -14.34966873604973081, 49.58442372801901143 ) ) ;
#15365=CARTESIAN_POINT ( 'NONE',  ( 16.53943276465976808, -0.05219959533910856209, 83.74890960531435269 ) ) ;
#15366=CARTESIAN_POINT ( 'NONE',  ( -15.80617190586745835, -15.72974639402198527, 76.87390960531439532 ) ) ;
#15367=CARTESIAN_POINT ( 'NONE',  ( -14.34966873604972548, 8.224510206698743886, 113.3344237280190328 ) ) ;
#15368=CARTESIAN_POINT ( 'NONE',  ( -16.55341960407617563, 4.379528057220093196, 33.54275706135234714 ) ) ;
#15369=CARTESIAN_POINT ( 'NONE',  ( 16.51473224551069308, 9.474510206698969483, 39.16557627198103120 ) ) ;
#15370=CARTESIAN_POINT ( 'NONE',  ( -14.29746914071037622, -8.314922557961029526, 74.16775706135231871 ) ) ;
#15371=CARTESIAN_POINT ( 'NONE',  ( -13.97604488694547697, 13.89961937509957934, 68.12609039468563310 ) ) ;
#15372=CARTESIAN_POINT ( 'NONE',  ( -18.62759615963270932, 10.81492255796079327, 75.83224293864769550 ) ) ;
#15373=CARTESIAN_POINT ( 'NONE',  ( 14.34966873604960469, 8.224510206698951720, 24.16557627198103120 ) ) ;
#15375=CARTESIAN_POINT ( 'NONE',  ( 18.67979575497194134, -10.72451020669871369, 85.83442372801901854 ) ) ;
#15376=CARTESIAN_POINT ( 'NONE',  ( 15.80617190586746368, 15.72974639402197994, 44.37390960531435979 ) ) ;
#15378=CARTESIAN_POINT ( 'NONE',  ( 8.224510206698742110, 14.34966873604972548, 92.08442372801901854 ) ) ;
#15379=CARTESIAN_POINT ( 'NONE',  ( -21.53943276465977519, 0.05219959533907696930, 51.24890960531436690 ) ) ;
#15381=CARTESIAN_POINT ( 'NONE',  ( -19.03943276465977164, 0.05219959533909376836, 106.2489096053143669 ) ) ;
#15382=CARTESIAN_POINT ( 'NONE',  ( 17.50000000000000000, 3.471454075611686729, 108.0166741885564221 ) ) ;
#15383=CARTESIAN_POINT ( 'NONE',  ( 5.049401038298161559, -19.05341960407611168, 27.70724293864769550 ) ) ;
#15384=CARTESIAN_POINT ( 'NONE',  ( 10.81492255796078972, 18.62759615963270932, 79.58224293864769550 ) ) ;
#15385=CARTESIAN_POINT ( 'NONE',  ( 0.05219959533934541429, -16.53943276465976808, 110.0010903946856757 ) ) ;
#15386=CARTESIAN_POINT ( 'NONE',  ( -10.72451020669870658, -18.67979575497194134, 59.58442372801901854 ) ) ;
#15387=CARTESIAN_POINT ( 'NONE',  ( -12.14591786802326823, 12.06949235617739902, 23.12609039468567573 ) ) ;
#15388=CARTESIAN_POINT ( 'NONE',  ( -9.474510206698964154, 16.51473224551069663, 25.41557627198103120 ) ) ;
#15389=CARTESIAN_POINT ( 'NONE',  ( -9.564922557961040184, 16.46253265017147172, 107.9177570613523471 ) ) ;
#15390=CARTESIAN_POINT ( 'NONE',  ( -19.02544592524342804, 5.153800228976336051, 36.04057627198100988 ) ) ;
#15392=CARTESIAN_POINT ( 'NONE',  ( -16.46253265017160317, 9.564922557960807481, 105.8322429386476955 ) ) ;
#15393=CARTESIAN_POINT ( 'NONE',  ( 12.14591786802327356, -12.06949235617739191, 90.62609039468567573 ) ) ;
#15394=CARTESIAN_POINT ( 'NONE',  ( 9.564922557961047289, -16.46253265017146816, 80.41775706135234714 ) ) ;
#15395=CARTESIAN_POINT ( 'NONE',  ( -5.153800228976607833, 19.02544592524334988, 27.70942372801899722 ) ) ;
#15396=CARTESIAN_POINT ( 'NONE',  ( -5.719274019375978568, 21.55341960407610458, 75.20724293864769550 ) ) ;
#15397=CARTESIAN_POINT ( 'NONE',  ( 14.29746914071037800, 8.314922557961029526, 106.6677570613523756 ) ) ;
#15398=CARTESIAN_POINT ( 'NONE',  ( 19.03943276465977164, 0.05219959533936151252, 91.25109039468566152 ) ) ;
#15399=CARTESIAN_POINT ( 'NONE',  ( 19.02544592524343514, -5.153800228976328945, 48.54057627198103120 ) ) ;
#15400=CARTESIAN_POINT ( 'NONE',  ( -16.46253265017160317, 9.564922557960807481, 95.83224293864769550 ) ) ;
#15401=CARTESIAN_POINT ( 'NONE',  ( 21.53943276465977519, 0.05219959533937863772, 51.25109039468568994 ) ) ;
#15402=CARTESIAN_POINT ( 'NONE',  ( 5.153800228976335163, 19.02544592524342804, 44.79057627198103830 ) ) ;
#15403=CARTESIAN_POINT ( 'NONE',  ( -17.31728774477274868, -6.344390552232371583, 84.18093348310685542 ) ) ;
#15404=CARTESIAN_POINT ( 'NONE',  ( 5.153800228976335163, 19.02544592524342804, 114.7905762719810241 ) ) ;
#15405=CARTESIAN_POINT ( 'NONE',  ( -0.05219959533910754901, -16.53943276465976808, 67.49890960531436690 ) ) ;
#15406=CARTESIAN_POINT ( 'NONE',  ( 5.719274019375991003, -21.55341960407610458, 72.70724293864769550 ) ) ;
#15408=CARTESIAN_POINT ( 'NONE',  ( 16.46253265017146816, 9.564922557961045513, 46.66775706135233293 ) ) ;
#15410=CARTESIAN_POINT ( 'NONE',  ( -5.049401038298153566, 19.05341960407611168, 70.20724293864769550 ) ) ;
#15411=CARTESIAN_POINT ( 'NONE',  ( -5.153800228976328057, -19.02544592524343514, 92.29057627198099567 ) ) ;
#15412=CARTESIAN_POINT ( 'NONE',  ( 16.52544592524335698, 4.483927247898782831, 46.45942372801901854 ) ) ;
#15414=CARTESIAN_POINT ( 'NONE',  ( -13.89961937509957401, -13.97604488694547875, 24.37609039468565442 ) ) ;
#15416=CARTESIAN_POINT ( 'NONE',  ( -14.34966873604972548, 8.224510206698743886, 93.33442372801901854 ) ) ;
#15418=CARTESIAN_POINT ( 'NONE',  ( 8.314922557961029526, -14.29746914071037800, 85.41775706135236135 ) ) ;
#15419=CARTESIAN_POINT ( 'NONE',  ( -0.05219959533934338120, 16.53943276465976808, 52.50109039468567573 ) ) ;
#15420=CARTESIAN_POINT ( 'NONE',  ( -5.049401038297874678, -19.05341960407617918, 19.79275706135233293 ) ) ;
#15421=CARTESIAN_POINT ( 'NONE',  ( -5.153800228976328057, -19.02544592524343514, 52.29057627198100988 ) ) ;
#15423=CARTESIAN_POINT ( 'NONE',  ( 15.72974639402176855, 15.80617190586768217, 66.87609039468568994 ) ) ;
#15424=CARTESIAN_POINT ( 'NONE',  ( 16.51473224551083163, -9.474510206698727899, 80.83442372801899012 ) ) ;
#15425=CARTESIAN_POINT ( 'NONE',  ( -5.049401038297874678, -19.05341960407617918, 19.79275706135233293 ) ) ;
#15426=CARTESIAN_POINT ( 'NONE',  ( 5.153800228976335163, 19.02544592524342804, 34.79057627198102409 ) ) ;
#15428=CARTESIAN_POINT ( 'NONE',  ( 18.62759615963271287, -10.81492255796078972, 73.33224293864769550 ) ) ;
#15430=CARTESIAN_POINT ( 'NONE',  ( 0.05219959533907565091, 21.53943276465977519, 24.99890960531435624 ) ) ;
#15431=CARTESIAN_POINT ( 'NONE',  ( 13.97604488694527802, 13.89961937509977652, 24.37390960531435624 ) ) ;
#15432=CARTESIAN_POINT ( 'NONE',  ( -12.06949235617739369, -12.14591786802326823, 39.37609039468567573 ) ) ;
#15433=CARTESIAN_POINT ( 'NONE',  ( 16.53943276465976808, -0.05219959533910856209, 28.74890960531435624 ) ) ;
#15434=EDGE_LOOP ( 'NONE', ( #117415, #7690, #54758, #129558 ) ) ;
#15435=CARTESIAN_POINT ( 'NONE',  ( -18.62759615963255300, -10.81492255796106328, 24.16775706135235424 ) ) ;
#15436=CARTESIAN_POINT ( 'NONE',  ( 16.53943276465976808, -0.05219959533910856209, 43.74890960531435979 ) ) ;
#15438=CARTESIAN_POINT ( 'NONE',  ( 5.049401038297881783, 19.05341960407617563, 107.2927570613523187 ) ) ;
#15439=CARTESIAN_POINT ( 'NONE',  ( 13.89961937509957401, 13.97604488694547697, 21.87609039468566152 ) ) ;
#15440=CARTESIAN_POINT ( 'NONE',  ( -4.483927247898539470, -16.52544592524342804, 42.29057627198103120 ) ) ;
#15441=CARTESIAN_POINT ( 'NONE',  ( -5.823673210054116645, -21.52544592524344225, 107.2905762719810525 ) ) ;
#15442=EDGE_CURVE ( 'NONE', #193741, #188751, #19240, .T. ) ;
#15443=CARTESIAN_POINT ( 'NONE',  ( 16.62475595723694965, 7.163666690055250363, 31.97286648189535896 ) ) ;
#15444=CARTESIAN_POINT ( 'NONE',  ( 10.81492255796078972, 18.62759615963270932, 69.58224293864769550 ) ) ;
#15445=CARTESIAN_POINT ( 'NONE',  ( 19.02544592524343514, -5.153800228976328945, 73.54057627198103830 ) ) ;
#15446=CARTESIAN_POINT ( 'NONE',  ( 14.29746914071049879, -8.314922557960816363, 43.33224293864769550 ) ) ;
#15447=CARTESIAN_POINT ( 'NONE',  ( 16.51473224551069308, 9.474510206698969483, 94.16557627198103830 ) ) ;
#15448=DIRECTION ( 'NONE',  ( -0.000000000000000000, -0.000000000000000000, 1.000000000000000000 ) ) ;
#15449=CARTESIAN_POINT ( 'NONE',  ( -5.153800228976607833, 19.02544592524334988, 57.70942372801899012 ) ) ;
#15450=CARTESIAN_POINT ( 'NONE',  ( -21.53943276465977519, 0.05219959533907696930, 91.24890960531436690 ) ) ;
#15451=CARTESIAN_POINT ( 'NONE',  ( 16.51473224551069308, 9.474510206698969483, 39.16557627198103120 ) ) ;
#15452=CARTESIAN_POINT ( 'NONE',  ( 16.55341960407611168, 4.379528057220329451, 108.9572429386476955 ) ) ;
#15453=CARTESIAN_POINT ( 'NONE',  ( -21.52544592524334988, -5.823673210054445271, 53.95942372801900433 ) ) ;
#15457=CARTESIAN_POINT ( 'NONE',  ( -12.14591786802309592, -12.06949235617757132, 26.87390960531435979 ) ) ;
#15458=CARTESIAN_POINT ( 'NONE',  ( -19.03943276465977164, 0.05219959533909376836, 46.24890960531435979 ) ) ;
#15459=CARTESIAN_POINT ( 'NONE',  ( -9.564922557960796823, -16.46253265017161027, 97.08224293864769550 ) ) ;
#15460=CARTESIAN_POINT ( 'NONE',  ( 15.72974639402199770, -15.80617190586745480, 58.12390960531435979 ) ) ;
#15461=CARTESIAN_POINT ( 'NONE',  ( -5.153800228976607833, 19.02544592524335343, 92.70942372801900433 ) ) ;
#15462=CARTESIAN_POINT ( 'NONE',  ( -9.474510206698964154, 16.51473224551069663, 50.41557627198102409 ) ) ;
#15463=CARTESIAN_POINT ( 'NONE',  ( 21.53943276465977519, -0.05219959533907433946, 53.74890960531437401 ) ) ;
#15464=CARTESIAN_POINT ( 'NONE',  ( 21.52544592524334988, 5.823673210054432836, 81.45942372801900433 ) ) ;
#15466=CARTESIAN_POINT ( 'NONE',  ( -16.55341960407617563, 4.379528057220093196, 88.54275706135236135 ) ) ;
#15467=CARTESIAN_POINT ( 'NONE',  ( -0.05219959533934338120, 16.53943276465976808, 92.50109039468567573 ) ) ;
#15468=CARTESIAN_POINT ( 'NONE',  ( -19.03943276465977164, 0.05219959533909376836, 61.24890960531436690 ) ) ;
#15469=CARTESIAN_POINT ( 'NONE',  ( 9.474510206698971260, -16.51473224551069308, 62.91557627198102409 ) ) ;
#15471=CARTESIAN_POINT ( 'NONE',  ( 5.153800228976615827, -19.02544592524334988, 30.20942372801900433 ) ) ;
#15472=CARTESIAN_POINT ( 'NONE',  ( -8.314922557961024197, 14.29746914071037800, 72.91775706135234714 ) ) ;
#15473=CARTESIAN_POINT ( 'NONE',  ( -0.05219959533937732626, 21.53943276465977519, 107.5010903946856899 ) ) ;
#15474=CARTESIAN_POINT ( 'NONE',  ( -0.05219959533909027116, -19.03943276465977164, 72.49890960531435269 ) ) ;
#15475=CARTESIAN_POINT ( 'NONE',  ( 15.80617190586746368, 15.72974639402197994, 54.37390960531435979 ) ) ;
#15476=CARTESIAN_POINT ( 'NONE',  ( 12.14591786802327356, -12.06949235617739191, 20.62609039468568639 ) ) ;
#15477=CARTESIAN_POINT ( 'NONE',  ( 18.62759615963255655, 10.81492255796105972, 86.66775706135234714 ) ) ;
#15478=CARTESIAN_POINT ( 'NONE',  ( -12.06949235617739369, -12.14591786802326823, 44.37609039468567573 ) ) ;
#15479=CARTESIAN_POINT ( 'NONE',  ( 21.53943276465977519, -0.05219959533907433946, 113.7489096053143527 ) ) ;
#15480=CARTESIAN_POINT ( 'NONE',  ( -0.05219959533934338120, 16.53943276465976808, 22.50109039468567573 ) ) ;
#15481=CARTESIAN_POINT ( 'NONE',  ( 19.02544592524343514, -5.153800228976328945, 83.54057627198100988 ) ) ;
#15482=CARTESIAN_POINT ( 'NONE',  ( -16.53943276465976808, -0.05219959533934237506, 28.75109039468567929 ) ) ;
#15483=CARTESIAN_POINT ( 'NONE',  ( 9.564922557960805705, 16.46253265017160317, 39.58224293864768839 ) ) ;
#15484=CARTESIAN_POINT ( 'NONE',  ( -8.224510206698735004, -14.34966873604973081, 19.58442372801901143 ) ) ;
#15485=CARTESIAN_POINT ( 'NONE',  ( 8.314922557960818139, 14.29746914071049879, 74.58224293864768129 ) ) ;
#15486=CARTESIAN_POINT ( 'NONE',  ( -4.483927247898782831, 16.52544592524335698, 87.70942372801901854 ) ) ;
#15487=CARTESIAN_POINT ( 'NONE',  ( 15.72974639402176855, 15.80617190586768217, 31.87609039468567929 ) ) ;
#15488=CARTESIAN_POINT ( 'NONE',  ( 5.153800228976335163, 19.02544592524342804, 59.79057627198100988 ) ) ;
#15489=CARTESIAN_POINT ( 'NONE',  ( 13.89961937509977652, -13.97604488694527269, 68.12390960531436690 ) ) ;
#15490=CARTESIAN_POINT ( 'NONE',  ( 8.314922557961029526, -14.29746914071037800, 90.41775706135236135 ) ) ;
#15491=EDGE_CURVE ( 'NONE', #135989, #186347, #126781, .T. ) ;
#15493=ORIENTED_EDGE ( 'NONE', *, *, #160761, .F. ) ;
#15494=VERTEX_POINT ( 'NONE', #47988 ) ;
#15495=CARTESIAN_POINT ( 'NONE',  ( 5.049401038297881783, 19.05341960407617563, 32.29275706135233293 ) ) ;
#15496=CARTESIAN_POINT ( 'NONE',  ( -13.97604488694527625, -13.89961937509977652, 31.87390960531435979 ) ) ;
#15499=CARTESIAN_POINT ( 'NONE',  ( -16.52544592524335698, -4.483927247898792601, 28.95942372801902209 ) ) ;
#15500=CARTESIAN_POINT ( 'NONE',  ( -0.05219959533936034679, 19.03943276465977164, 52.50109039468566863 ) ) ;
#15501=CARTESIAN_POINT ( 'NONE',  ( 16.55341960407618274, -4.379528057220086978, 46.04275706135234714 ) ) ;
#15502=CARTESIAN_POINT ( 'NONE',  ( 9.564922557960805705, 16.46253265017160317, 104.5822429386476955 ) ) ;
#15503=CARTESIAN_POINT ( 'NONE',  ( 19.05341960407611168, 5.049401038298154454, 63.95724293864769550 ) ) ;
#15504=CARTESIAN_POINT ( 'NONE',  ( 15.72974639402199770, -15.80617190586745480, 103.1239096053143811 ) ) ;
#15505=CARTESIAN_POINT ( 'NONE',  ( 5.153800228976335163, 19.02544592524342804, 94.79057627198103830 ) ) ;
#15506=CARTESIAN_POINT ( 'NONE',  ( 17.48933443480910199, -3.858464096052834247, 21.79111074916215784 ) ) ;
#15507=CARTESIAN_POINT ( 'NONE',  ( 16.51473224551069308, 9.474510206698969483, 64.16557627198102409 ) ) ;
#15508=CARTESIAN_POINT ( 'NONE',  ( -4.483927247898539470, -16.52544592524342804, 22.29057627198102765 ) ) ;
#15509=CARTESIAN_POINT ( 'NONE',  ( 5.049401038298161559, -19.05341960407611168, 22.70724293864769194 ) ) ;
#15510=CARTESIAN_POINT ( 'NONE',  ( -16.46253265017146816, -9.564922557961047289, 39.16775706135234003 ) ) ;
#15511=CARTESIAN_POINT ( 'NONE',  ( 4.483927247898545687, 16.52544592524342804, 59.79057627198103120 ) ) ;
#15512=CARTESIAN_POINT ( 'NONE',  ( -5.719274019375665041, -21.55341960407619695, 104.7927570613523898 ) ) ;
#15513=CARTESIAN_POINT ( 'NONE',  ( 19.05341960407611168, 5.049401038298154454, 43.95724293864769550 ) ) ;
#15514=CARTESIAN_POINT ( 'NONE',  ( 4.379528057220092307, 16.55341960407617563, 57.29275706135234714 ) ) ;
#15515=CARTESIAN_POINT ( 'NONE',  ( -14.29746914071049879, 8.314922557960819915, 45.83224293864769550 ) ) ;
#15516=CARTESIAN_POINT ( 'NONE',  ( -18.62759615963255300, -10.81492255796106328, 94.16775706135237556 ) ) ;
#15517=CARTESIAN_POINT ( 'NONE',  ( -13.89961937509977652, 13.97604488694528158, 75.62390960531438111 ) ) ;
#15518=CARTESIAN_POINT ( 'NONE',  ( 5.153800228976335163, 19.02544592524342804, 94.79057627198103830 ) ) ;
#15519=CARTESIAN_POINT ( 'NONE',  ( 8.314922557960818139, 14.29746914071049879, 109.5822429386476955 ) ) ;
#15520=CARTESIAN_POINT ( 'NONE',  ( 16.52544592524342804, -4.483927247898539470, 78.54057627198103830 ) ) ;
#15521=CARTESIAN_POINT ( 'NONE',  ( 21.52544592524344225, -5.823673210054117533, 88.54057627198103830 ) ) ;
#15522=CARTESIAN_POINT ( 'NONE',  ( 19.02544592524343514, -5.153800228976328945, 73.54057627198103830 ) ) ;
#15523=CARTESIAN_POINT ( 'NONE',  ( -10.81492255796078084, -18.62759615963271287, 97.08224293864770971 ) ) ;
#15524=CARTESIAN_POINT ( 'NONE',  ( -19.02544592524334988, -5.153800228976617603, 83.95942372801901854 ) ) ;
#15526=CARTESIAN_POINT ( 'NONE',  ( 8.314922557960818139, 14.29746914071049879, 94.58224293864769550 ) ) ;
#15527=CARTESIAN_POINT ( 'NONE',  ( 13.89961937509977652, -13.97604488694527269, 63.12390960531435979 ) ) ;
#15528=CARTESIAN_POINT ( 'NONE',  ( -5.823673210054116645, -21.52544592524344225, 67.29057627198103830 ) ) ;
#15529=CARTESIAN_POINT ( 'NONE',  ( 17.40805194822030799, -6.112264579159331745, 28.33371272510611760 ) ) ;
#15530=CARTESIAN_POINT ( 'NONE',  ( -12.06949235617739369, -12.14591786802326823, 109.3760903946857042 ) ) ;
#15532=CARTESIAN_POINT ( 'NONE',  ( 0.05219959533936267826, -19.03943276465977164, 110.0010903946856757 ) ) ;
#15533=CARTESIAN_POINT ( 'NONE',  ( 12.06949235617757843, -12.14591786802309237, 78.12390960531436690 ) ) ;
#15534=CARTESIAN_POINT ( 'NONE',  ( -17.97214573761830536, -5.500000000000085265, 46.46970049038654338 ) ) ;
#15535=CARTESIAN_POINT ( 'NONE',  ( 19.03943276465977164, -0.05219959533909143690, 78.74890960531436690 ) ) ;
#15536=CARTESIAN_POINT ( 'NONE',  ( -16.51473224551069308, -9.474510206698971260, 36.66557627198102409 ) ) ;
#15537=CARTESIAN_POINT ( 'NONE',  ( -12.14591786802309592, -12.06949235617757132, 66.87390960531436690 ) ) ;
#15538=CARTESIAN_POINT ( 'NONE',  ( 19.02544592524343514, -5.153800228976328945, 113.5405762719810241 ) ) ;
#15539=CARTESIAN_POINT ( 'NONE',  ( 13.89961937509957401, 13.97604488694547697, 91.87609039468567573 ) ) ;
#15540=CARTESIAN_POINT ( 'NONE',  ( -5.153800228976328057, -19.02544592524343514, 97.29057627198099567 ) ) ;
#15541=CARTESIAN_POINT ( 'NONE',  ( 10.81492255796078972, 18.62759615963270932, 79.58224293864769550 ) ) ;
#15542=CARTESIAN_POINT ( 'NONE',  ( 8.224510206698742110, 14.34966873604972548, 72.08442372801899012 ) ) ;
#15543=CARTESIAN_POINT ( 'NONE',  ( 5.049401038297881783, 19.05341960407617918, 112.2927570613523471 ) ) ;
#15544=CARTESIAN_POINT ( 'NONE',  ( 5.049401038298161559, -19.05341960407611168, 57.70724293864769550 ) ) ;
#15545=CARTESIAN_POINT ( 'NONE',  ( -18.67979575497178146, -10.72451020669898902, 71.66557627198100988 ) ) ;
#15546=CARTESIAN_POINT ( 'NONE',  ( 19.02544592524334988, 5.153800228976608722, 101.4594237280189759 ) ) ;
#15547=CARTESIAN_POINT ( 'NONE',  ( -4.379528057220328563, 16.55341960407611168, 40.20724293864769550 ) ) ;
#15548=CARTESIAN_POINT ( 'NONE',  ( -5.823673210054431948, 21.52544592524334988, 57.70942372801901143 ) ) ;
#15550=CARTESIAN_POINT ( 'NONE',  ( 8.224510206698742110, 14.34966873604972548, 67.08442372801901854 ) ) ;
#15551=CARTESIAN_POINT ( 'NONE',  ( 5.153800228976335163, 19.02544592524342804, 104.7905762719809957 ) ) ;
#15552=CARTESIAN_POINT ( 'NONE',  ( -19.05341960407611168, -5.049401038298164224, 106.4572429386476955 ) ) ;
#15554=CARTESIAN_POINT ( 'NONE',  ( 4.483927247898790824, -16.52544592524335698, 95.20942372801903275 ) ) ;
#15555=CARTESIAN_POINT ( 'NONE',  ( 4.483927247898790824, -16.52544592524335698, 45.20942372801901854 ) ) ;
#15556=CARTESIAN_POINT ( 'NONE',  ( 5.153800228976335163, 19.02544592524342804, 54.79057627198103120 ) ) ;
#15557=CARTESIAN_POINT ( 'NONE',  ( -19.05341960407611168, -5.049401038298163336, 71.45724293864766707 ) ) ;
#15558=CARTESIAN_POINT ( 'NONE',  ( -21.52544592524334988, -5.823673210054445271, 53.95942372801900433 ) ) ;
#15559=CARTESIAN_POINT ( 'NONE',  ( 8.224510206698742110, 14.34966873604972548, 62.08442372801901143 ) ) ;
#15560=CARTESIAN_POINT ( 'NONE',  ( 4.379528057220339221, -16.55341960407611168, 27.70724293864769905 ) ) ;
#15561=CARTESIAN_POINT ( 'NONE',  ( -19.03943276465977164, 0.05219959533909376836, 36.24890960531436690 ) ) ;
#15562=CARTESIAN_POINT ( 'NONE',  ( -19.02544592524342804, 5.153800228976336051, 31.04057627198102409 ) ) ;
#15563=CARTESIAN_POINT ( 'NONE',  ( 14.29746914071037800, 8.314922557961029526, 31.66775706135234358 ) ) ;
#15564=CARTESIAN_POINT ( 'NONE',  ( 0.05219959533936267826, -19.03943276465977164, 80.00109039468567573 ) ) ;
#15565=CARTESIAN_POINT ( 'NONE',  ( 8.224510206698953496, -14.34966873604960469, 77.91557627198102409 ) ) ;
#15566=CARTESIAN_POINT ( 'NONE',  ( -13.97604488694527625, -13.89961937509977652, 46.87390960531435979 ) ) ;
#15567=CARTESIAN_POINT ( 'NONE',  ( 19.05341960407617918, -5.049401038297876454, 81.04275706135231871 ) ) ;
#15569=CARTESIAN_POINT ( 'NONE',  ( 21.53943276465977519, 0.05219959533937863772, 86.25109039468568994 ) ) ;
#15570=CARTESIAN_POINT ( 'NONE',  ( 4.483927247898790824, -16.52544592524335698, 60.20942372801902565 ) ) ;
#15572=CARTESIAN_POINT ( 'NONE',  ( 5.823673210054125526, 21.52544592524343514, 54.79057627198104541 ) ) ;
#15573=CARTESIAN_POINT ( 'NONE',  ( 12.14591786802327356, -12.06949235617739191, 40.62609039468567573 ) ) ;
#15574=CARTESIAN_POINT ( 'NONE',  ( -5.153800228976328057, -19.02544592524343514, 37.29057627198102409 ) ) ;
#15575=CARTESIAN_POINT ( 'NONE',  ( -16.46253265017146816, -9.564922557961047289, 44.16775706135232582 ) ) ;
#15576=CARTESIAN_POINT ( 'NONE',  ( 16.51473224551069308, 9.474510206698969483, 89.16557627198103830 ) ) ;
#15577=CARTESIAN_POINT ( 'NONE',  ( -0.05219959533909027116, -19.03943276465977164, 47.49890960531435979 ) ) ;
#15579=CARTESIAN_POINT ( 'NONE',  ( 10.72451020669871369, 18.67979575497193778, 82.08442372801901854 ) ) ;
#15580=CARTESIAN_POINT ( 'NONE',  ( 5.049401038298163336, -19.05341960407611168, 92.70724293864769550 ) ) ;
#15581=CARTESIAN_POINT ( 'NONE',  ( -16.46253265017146816, -9.564922557961047289, 39.16775706135234003 ) ) ;
#15582=CARTESIAN_POINT ( 'NONE',  ( 18.62759615963255655, 10.81492255796105972, 106.6677570613523756 ) ) ;
#15583=CARTESIAN_POINT ( 'NONE',  ( -8.314922557960811034, -14.29746914071050412, 42.08224293864769550 ) ) ;
#15584=CARTESIAN_POINT ( 'NONE',  ( 5.153800228976335163, 19.02544592524342804, 39.79057627198100988 ) ) ;
#15585=CARTESIAN_POINT ( 'NONE',  ( 0.05219959533909260263, 19.03943276465977164, 99.99890960531436690 ) ) ;
#15586=CARTESIAN_POINT ( 'NONE',  ( 0.05219959533937995610, -21.53943276465977519, 80.00109039468568994 ) ) ;
#15587=CARTESIAN_POINT ( 'NONE',  ( 19.02544592524343514, -5.153800228976328945, 58.54057627198102409 ) ) ;
#15588=CARTESIAN_POINT ( 'NONE',  ( -5.719274019375665041, -21.55341960407619695, 74.79275706135234714 ) ) ;
#15589=CARTESIAN_POINT ( 'NONE',  ( 18.62759615963271287, -10.81492255796078972, 43.33224293864769550 ) ) ;
#15590=CARTESIAN_POINT ( 'NONE',  ( 15.72974639402176855, 15.80617190586768217, 26.87609039468567218 ) ) ;
#15591=CARTESIAN_POINT ( 'NONE',  ( -16.46253265017146816, -9.564922557961047289, 49.16775706135233293 ) ) ;
#15592=CARTESIAN_POINT ( 'NONE',  ( 13.89961937509977652, -13.97604488694527269, 23.12390960531436335 ) ) ;
#15593=CARTESIAN_POINT ( 'NONE',  ( 5.153800228976335163, 19.02544592524342804, 79.79057627198102409 ) ) ;
#15594=CARTESIAN_POINT ( 'NONE',  ( -16.52544592524335698, -4.483927247898792601, 28.95942372801902209 ) ) ;
#15595=CARTESIAN_POINT ( 'NONE',  ( -4.379528057220328563, 16.55341960407611168, 95.20724293864769550 ) ) ;
#15596=CARTESIAN_POINT ( 'NONE',  ( 0.05219959533909260263, 19.03943276465977164, 59.99890960531436690 ) ) ;
#15597=CARTESIAN_POINT ( 'NONE',  ( -15.72974639402197994, 15.80617190586746368, 35.62390960531437401 ) ) ;
#15598=CARTESIAN_POINT ( 'NONE',  ( -19.05341960407617563, 5.049401038297882671, 103.5427570613523329 ) ) ;
#15599=CARTESIAN_POINT ( 'NONE',  ( -18.67979575497178146, -10.72451020669898902, 106.6655762719810383 ) ) ;
#15600=CARTESIAN_POINT ( 'NONE',  ( -18.67979575497193778, 10.72451020669871902, 63.33442372801900433 ) ) ;
#15601=CARTESIAN_POINT ( 'NONE',  ( 14.29746914071037800, 8.314922557961029526, 71.66775706135234714 ) ) ;
#15602=CARTESIAN_POINT ( 'NONE',  ( -8.314922557961024197, 14.29746914071037800, 72.91775706135234714 ) ) ;
#15603=CARTESIAN_POINT ( 'NONE',  ( -9.564922557960796823, -16.46253265017161027, 67.08224293864769550 ) ) ;
#15604=CARTESIAN_POINT ( 'NONE',  ( -14.29746914071037622, -8.314922557961029526, 94.16775706135237556 ) ) ;
#15605=AXIS2_PLACEMENT_3D ( 'NONE', #777, #169645, #122140 ) ;
#15606=CARTESIAN_POINT ( 'NONE',  ( -15.72974639402197994, 15.80617190586746368, 115.6239096053143669 ) ) ;
#15607=CARTESIAN_POINT ( 'NONE',  ( -8.224510206698948167, 14.34966873604960824, 70.41557627198102409 ) ) ;
#15608=CARTESIAN_POINT ( 'NONE',  ( -5.049401038298153566, 19.05341960407611168, 90.20724293864766707 ) ) ;
#15609=CARTESIAN_POINT ( 'NONE',  ( -14.34966873604972548, 8.224510206698743886, 73.33442372801901854 ) ) ;
#15610=CARTESIAN_POINT ( 'NONE',  ( -15.72974639402176322, -15.80617190586768395, 54.37609039468568994 ) ) ;
#15611=CARTESIAN_POINT ( 'NONE',  ( -12.14591786802326823, 12.06949235617739902, 23.12609039468567573 ) ) ;
#15612=CARTESIAN_POINT ( 'NONE',  ( -10.81492255796078084, -18.62759615963271287, 112.0822429386477097 ) ) ;
#15613=CARTESIAN_POINT ( 'NONE',  ( 8.224510206698953496, -14.34966873604960469, 52.91557627198103830 ) ) ;
#15615=ORIENTED_EDGE ( 'NONE', *, *, #157780, .T. ) ;
#15616=CARTESIAN_POINT ( 'NONE',  ( -18.62759615963270932, 10.81492255796079327, 85.83224293864768129 ) ) ;
#15617=CARTESIAN_POINT ( 'NONE',  ( -16.55341960407611168, -4.379528057220339221, 36.45724293864768839 ) ) ;
#15619=LINE ( 'NONE', #155117, #179331 ) ;
#15620=CARTESIAN_POINT ( 'NONE',  ( -21.52544592524334988, -5.823673210054445271, 23.95942372801901143 ) ) ;
#15621=CARTESIAN_POINT ( 'NONE',  ( -9.564922557960796823, -16.46253265017161027, 112.0822429386476955 ) ) ;
#15622=CARTESIAN_POINT ( 'NONE',  ( 5.719274019375673035, 21.55341960407619339, 27.29275706135234358 ) ) ;
#15623=CARTESIAN_POINT ( 'NONE',  ( 0.05219959533910956823, 16.53943276465976808, 54.99890960531435269 ) ) ;
#15624=CARTESIAN_POINT ( 'NONE',  ( -16.53943276465976808, -0.05219959533934237506, 58.75109039468568994 ) ) ;
#15625=CARTESIAN_POINT ( 'NONE',  ( 9.564922557960805705, 16.46253265017160317, 64.58224293864769550 ) ) ;
#15626=CARTESIAN_POINT ( 'NONE',  ( 0.05219959533936267826, -19.03943276465977164, 60.00109039468566863 ) ) ;
#15627=CARTESIAN_POINT ( 'NONE',  ( 5.049401038298161559, -19.05341960407611168, 82.70724293864770971 ) ) ;
#15628=CARTESIAN_POINT ( 'NONE',  ( -21.55341960407610458, -5.719274019375992779, 46.45724293864769550 ) ) ;
#15630=CARTESIAN_POINT ( 'NONE',  ( -9.474510206698964154, 16.51473224551069663, 60.41557627198102409 ) ) ;
#15631=CARTESIAN_POINT ( 'NONE',  ( -4.483927247898782831, 16.52544592524335698, 37.70942372801900433 ) ) ;
#15632=CARTESIAN_POINT ( 'NONE',  ( -13.97604488694547697, 13.89961937509957934, 58.12609039468566863 ) ) ;
#15633=CARTESIAN_POINT ( 'NONE',  ( -15.80617190586768217, 15.72974639402176855, 23.12609039468567573 ) ) ;
#15634=CARTESIAN_POINT ( 'NONE',  ( 8.224510206698953496, -14.34966873604960469, 42.91557627198103120 ) ) ;
#15635=CARTESIAN_POINT ( 'NONE',  ( -13.97604488694527625, -13.89961937509977652, 91.87390960531432427 ) ) ;
#15636=CARTESIAN_POINT ( 'NONE',  ( -15.80617190586745835, -15.72974639402198527, 61.87390960531436690 ) ) ;
#15637=CARTESIAN_POINT ( 'NONE',  ( -5.719274019375978568, 21.55341960407610458, 100.2072429386476955 ) ) ;
#15638=CARTESIAN_POINT ( 'NONE',  ( 12.06949235617739724, 12.14591786802326823, 36.87609039468568994 ) ) ;
#15639=CARTESIAN_POINT ( 'NONE',  ( 10.72451020669898902, -18.67979575497178502, 37.91557627198102409 ) ) ;
#15640=CARTESIAN_POINT ( 'NONE',  ( -5.823673210054431948, 21.52544592524334988, 87.70942372801901854 ) ) ;
#15641=CARTESIAN_POINT ( 'NONE',  ( 19.05341960407611168, 5.049401038298154454, 83.95724293864766707 ) ) ;
#15642=CARTESIAN_POINT ( 'NONE',  ( 5.049401038298161559, -19.05341960407611168, 37.70724293864768839 ) ) ;
#15643=CARTESIAN_POINT ( 'NONE',  ( 19.03943276465977164, -0.05219959533909143690, 98.74890960531436690 ) ) ;
#15644=CARTESIAN_POINT ( 'NONE',  ( -14.29746914071049879, 8.314922557960819915, 110.8322429386476955 ) ) ;
#15645=CARTESIAN_POINT ( 'NONE',  ( 13.97604488694527802, 13.89961937509977652, 69.37390960531436690 ) ) ;
#15646=CARTESIAN_POINT ( 'NONE',  ( -12.06949235617739369, -12.14591786802326823, 29.37609039468568284 ) ) ;
#15647=CARTESIAN_POINT ( 'NONE',  ( 17.50000000000000355, 3.305555262949610995, 32.87482847843406830 ) ) ;
#15648=CARTESIAN_POINT ( 'NONE',  ( 13.97604488694548053, -13.89961937509957401, 60.62609039468564731 ) ) ;
#15649=CARTESIAN_POINT ( 'NONE',  ( 18.67979575497194134, -10.72451020669871369, 100.8344237280190185 ) ) ;
#15650=CARTESIAN_POINT ( 'NONE',  ( -10.72451020669898014, 18.67979575497178502, 30.41557627198101699 ) ) ;
#15651=CARTESIAN_POINT ( 'NONE',  ( 16.53943276465976808, 0.05219959533934440121, 96.25109039468568994 ) ) ;
#15653=CARTESIAN_POINT ( 'NONE',  ( -13.89961937509957401, -13.97604488694547875, 64.37609039468567573 ) ) ;
#15654=CARTESIAN_POINT ( 'NONE',  ( -9.474510206698720793, -16.51473224551083518, 29.58442372801900433 ) ) ;
#15656=CARTESIAN_POINT ( 'NONE',  ( -13.97604488694527625, -13.89961937509977652, 26.87390960531434558 ) ) ;
#15657=CARTESIAN_POINT ( 'NONE',  ( 8.224510206698953496, -14.34966873604960469, 37.91557627198102409 ) ) ;
#15658=CARTESIAN_POINT ( 'NONE',  ( -13.89961937509977652, 13.97604488694528158, 25.62390960531434558 ) ) ;
#15659=CARTESIAN_POINT ( 'NONE',  ( -16.55341960407611168, -4.379528057220339221, 31.45724293864769550 ) ) ;
#15660=CARTESIAN_POINT ( 'NONE',  ( -18.22780087662124160, -5.499999999999927169, 83.98236817873107896 ) ) ;
#15661=CARTESIAN_POINT ( 'NONE',  ( 12.06949235617739724, 12.14591786802326823, 96.87609039468568994 ) ) ;
#15662=CARTESIAN_POINT ( 'NONE',  ( -19.02544592524342804, 5.153800228976336051, 36.04057627198100988 ) ) ;
#15663=CARTESIAN_POINT ( 'NONE',  ( -10.72451020669870658, -18.67979575497194134, 109.5844237280190328 ) ) ;
#15664=CARTESIAN_POINT ( 'NONE',  ( -19.05341960407617563, 5.049401038297882671, 113.5427570613523471 ) ) ;
#15665=CARTESIAN_POINT ( 'NONE',  ( 0.05219959533937995610, -21.53943276465977519, 80.00109039468568994 ) ) ;
#15666=CARTESIAN_POINT ( 'NONE',  ( -0.05219959533936034679, 19.03943276465977164, 57.50109039468566863 ) ) ;
#15667=CARTESIAN_POINT ( 'NONE',  ( 9.474510206698971260, -16.51473224551069308, 97.91557627198102409 ) ) ;
#15668=CARTESIAN_POINT ( 'NONE',  ( 19.03943276465977164, -0.05219959533909143690, 78.74890960531436690 ) ) ;
#15669=CARTESIAN_POINT ( 'NONE',  ( 17.48847506799967988, 5.747544572773810145, 71.67302562156723411 ) ) ;
#15670=CARTESIAN_POINT ( 'NONE',  ( 15.72974639402199770, -15.80617190586745480, 108.1239096053143811 ) ) ;
#15671=CARTESIAN_POINT ( 'NONE',  ( -16.53943276465976808, 0.05219959533911058130, 61.24890960531435979 ) ) ;
#15672=CARTESIAN_POINT ( 'NONE',  ( -21.53943276465977519, 0.05219959533907696930, 61.24890960531435979 ) ) ;
#15673=CARTESIAN_POINT ( 'NONE',  ( -13.89961937509977652, 13.97604488694528158, 55.62390960531434558 ) ) ;
#15674=CARTESIAN_POINT ( 'NONE',  ( 10.72451020669898902, -18.67979575497178502, 92.91557627198103830 ) ) ;
#15675=CARTESIAN_POINT ( 'NONE',  ( 8.224510206698742110, 14.34966873604972548, 92.08442372801901854 ) ) ;
#15677=CARTESIAN_POINT ( 'NONE',  ( 13.89961937509977652, -13.97604488694527269, 53.12390960531434558 ) ) ;
#15678=CARTESIAN_POINT ( 'NONE',  ( 4.483927247898545687, 16.52544592524342804, 89.79057627198103830 ) ) ;
#15680=CARTESIAN_POINT ( 'NONE',  ( -19.03943276465977164, 0.05219959533909376836, 46.24890960531435979 ) ) ;
#15681=CARTESIAN_POINT ( 'NONE',  ( -16.53943276465976808, 0.05219959533911058130, 116.2489096053143669 ) ) ;
#15682=CARTESIAN_POINT ( 'NONE',  ( 19.03943276465977164, 0.05219959533936151252, 76.25109039468566152 ) ) ;
#15683=CARTESIAN_POINT ( 'NONE',  ( -16.53943276465976808, 0.05219959533911058130, 81.24890960531436690 ) ) ;
#15684=CARTESIAN_POINT ( 'NONE',  ( -18.62759615963255300, -10.81492255796106328, 49.16775706135234003 ) ) ;
#15685=CARTESIAN_POINT ( 'NONE',  ( 9.474510206698971260, -16.51473224551069308, 32.91557627198102409 ) ) ;
#15686=CARTESIAN_POINT ( 'NONE',  ( 5.823673210054125526, 21.52544592524343514, 104.7905762719810241 ) ) ;
#15687=CARTESIAN_POINT ( 'NONE',  ( 8.314922557960818139, 14.29746914071049879, 84.58224293864769550 ) ) ;
#15689=CARTESIAN_POINT ( 'NONE',  ( 19.03943276465977164, -0.05219959533909143690, 58.74890960531435979 ) ) ;
#15690=CARTESIAN_POINT ( 'NONE',  ( 17.26058549869091152, 6.457015423128539489, 113.8774583747606925 ) ) ;
#15691=CARTESIAN_POINT ( 'NONE',  ( 9.564922557961047289, -16.46253265017146816, 90.41775706135234714 ) ) ;
#15692=CARTESIAN_POINT ( 'NONE',  ( 16.46253265017160672, -9.564922557960803928, 113.3322429386476955 ) ) ;
#15693=CARTESIAN_POINT ( 'NONE',  ( 10.81492255796106328, -18.62759615963255655, 30.41775706135234358 ) ) ;
#15694=CARTESIAN_POINT ( 'NONE',  ( -5.153800228976328057, -19.02544592524343514, 77.29057627198099567 ) ) ;
#15695=CARTESIAN_POINT ( 'NONE',  ( -5.049401038297874678, -19.05341960407617918, 64.79275706135233293 ) ) ;
#15696=CARTESIAN_POINT ( 'NONE',  ( -13.97604488694527625, -13.89961937509977652, 51.87390960531436690 ) ) ;
#15697=CARTESIAN_POINT ( 'NONE',  ( -12.14591786802309592, -12.06949235617757132, 71.87390960531438111 ) ) ;
#15698=CARTESIAN_POINT ( 'NONE',  ( -12.06949235617756955, 12.14591786802309770, 65.62390960531436690 ) ) ;
#15699=CARTESIAN_POINT ( 'NONE',  ( -13.97604488694527625, -13.89961937509977652, 91.87390960531432427 ) ) ;
#15700=CARTESIAN_POINT ( 'NONE',  ( -5.719274019375978568, 21.55341960407610458, 95.20724293864769550 ) ) ;
#15701=CARTESIAN_POINT ( 'NONE',  ( -19.05341960407611168, -5.049401038298163336, 81.45724293864769550 ) ) ;
#15703=CARTESIAN_POINT ( 'NONE',  ( -5.153800228976607833, 19.02544592524334988, 32.70942372801899722 ) ) ;
#15704=CARTESIAN_POINT ( 'NONE',  ( -19.03943276465977164, 0.05219959533909376836, 31.24890960531435979 ) ) ;
#15705=CARTESIAN_POINT ( 'NONE',  ( 0.05219959533910956823, 16.53943276465976808, 29.99890960531435979 ) ) ;
#15706=CARTESIAN_POINT ( 'NONE',  ( 16.55341960407611168, 4.379528057220329451, 103.9572429386476813 ) ) ;
#15707=VERTEX_POINT ( 'NONE', #16647 ) ;
#15708=CARTESIAN_POINT ( 'NONE',  ( 0.05219959533937995610, -21.53943276465977519, 35.00109039468568284 ) ) ;
#15709=CARTESIAN_POINT ( 'NONE',  ( 5.049401038297881783, 19.05341960407617563, 62.29275706135234003 ) ) ;
#15710=CARTESIAN_POINT ( 'NONE',  ( -4.483927247898539470, -16.52544592524342804, 32.29057627198102409 ) ) ;
#15711=CARTESIAN_POINT ( 'NONE',  ( 21.55341960407610458, 5.719274019375980345, 83.95724293864770971 ) ) ;
#15712=CARTESIAN_POINT ( 'NONE',  ( 10.81492255796078972, 18.62759615963270932, 24.58224293864768839 ) ) ;
#15713=CARTESIAN_POINT ( 'NONE',  ( -12.06949235617756955, 12.14591786802309770, 70.62390960531436690 ) ) ;
#15714=CARTESIAN_POINT ( 'NONE',  ( -19.03943276465977164, 0.05219959533909376836, 31.24890960531435979 ) ) ;
#15715=CARTESIAN_POINT ( 'NONE',  ( -5.153800228976607833, 19.02544592524334988, 32.70942372801899722 ) ) ;
#15716=CARTESIAN_POINT ( 'NONE',  ( 8.224510206698742110, 14.34966873604972548, 102.0844237280190185 ) ) ;
#15717=CARTESIAN_POINT ( 'NONE',  ( -14.34966873604972548, 8.224510206698743886, 58.33442372801901143 ) ) ;
#15718=CARTESIAN_POINT ( 'NONE',  ( 13.89961937509977652, -13.97604488694527269, 113.1239096053143527 ) ) ;
#15719=CARTESIAN_POINT ( 'NONE',  ( -5.823673210054431948, 21.52544592524334988, 107.7094237280190328 ) ) ;
#15720=CARTESIAN_POINT ( 'NONE',  ( 13.97604488694527802, 13.89961937509977652, 79.37390960531435269 ) ) ;
#15721=CARTESIAN_POINT ( 'NONE',  ( 12.14591786802327356, -12.06949235617739191, 60.62609039468567573 ) ) ;
#15722=CARTESIAN_POINT ( 'NONE',  ( -4.379528057220328563, 16.55341960407611168, 115.2072429386476955 ) ) ;
#15723=CARTESIAN_POINT ( 'NONE',  ( -16.55341960407611168, -4.379528057220339221, 36.45724293864768839 ) ) ;
#15725=CARTESIAN_POINT ( 'NONE',  ( 19.05341960407611168, 5.049401038298154454, 103.9572429386476671 ) ) ;
#15726=CARTESIAN_POINT ( 'NONE',  ( -13.97604488694527625, -13.89961937509977652, 96.87390960531433848 ) ) ;
#15727=CARTESIAN_POINT ( 'NONE',  ( 9.474510206698971260, -16.51473224551069308, 112.9155762719810383 ) ) ;
#15728=CARTESIAN_POINT ( 'NONE',  ( 0.05219959533910956823, 16.53943276465976808, 64.99890960531435269 ) ) ;
#15729=CARTESIAN_POINT ( 'NONE',  ( 8.314922557960818139, 14.29746914071049879, 34.58224293864770260 ) ) ;
#15730=CARTESIAN_POINT ( 'NONE',  ( -14.29746914071049879, 8.314922557960819915, 55.83224293864770260 ) ) ;
#15732=CARTESIAN_POINT ( 'NONE',  ( 4.379528057220092307, 16.55341960407617563, 37.29275706135235424 ) ) ;
#15733=CARTESIAN_POINT ( 'NONE',  ( 17.50000000000000711, -5.499999999999992895, 31.21769037696435589 ) ) ;
#15734=CARTESIAN_POINT ( 'NONE',  ( 13.89961937509957401, 13.97604488694547697, 46.87609039468565442 ) ) ;
#15735=CARTESIAN_POINT ( 'NONE',  ( -9.564922557960796823, -16.46253265017161027, 77.08224293864769550 ) ) ;
#15736=CARTESIAN_POINT ( 'NONE',  ( 9.474510206698729675, 16.51473224551082808, 67.08442372801900433 ) ) ;
#15738=CARTESIAN_POINT ( 'NONE',  ( -16.46253265017146816, -9.564922557961047289, 59.16775706135233293 ) ) ;
#15739=CARTESIAN_POINT ( 'NONE',  ( 19.03943276465977164, 0.05219959533936151252, 101.2510903946856757 ) ) ;
#15740=CARTESIAN_POINT ( 'NONE',  ( -12.14591786802326823, 12.06949235617739902, 83.12609039468568994 ) ) ;
#15742=CARTESIAN_POINT ( 'NONE',  ( 5.049401038298161559, -19.05341960407611168, 27.70724293864769550 ) ) ;
#15743=CARTESIAN_POINT ( 'NONE',  ( -19.03943276465977164, 0.05219959533909376836, 106.2489096053143669 ) ) ;
#15744=CARTESIAN_POINT ( 'NONE',  ( -5.719274019375665041, -21.55341960407619695, 44.79275706135234714 ) ) ;
#15745=CARTESIAN_POINT ( 'NONE',  ( 5.153800228976615827, -19.02544592524334988, 105.2094237280190185 ) ) ;
#15746=CARTESIAN_POINT ( 'NONE',  ( 17.49999999999999645, -3.512728167236924826, 107.7280999518112594 ) ) ;
#15747=CARTESIAN_POINT ( 'NONE',  ( 19.02544592524343514, -5.153800228976328945, 58.54057627198102409 ) ) ;
#15748=CARTESIAN_POINT ( 'NONE',  ( -19.02544592524342804, 5.153800228976336051, 101.0405762719810241 ) ) ;
#15749=CARTESIAN_POINT ( 'NONE',  ( -4.379528057220328563, 16.55341960407611168, 65.20724293864768129 ) ) ;
#15750=CARTESIAN_POINT ( 'NONE',  ( 13.89961937509977652, -13.97604488694527269, 68.12390960531436690 ) ) ;
#15751=CARTESIAN_POINT ( 'NONE',  ( 19.03943276465977164, -0.05219959533909143690, 63.74890960531435979 ) ) ;
#15752=CARTESIAN_POINT ( 'NONE',  ( -19.02544592524334988, -5.153800228976617603, 73.95942372801900433 ) ) ;
#15753=CARTESIAN_POINT ( 'NONE',  ( -15.72974639402197994, 15.80617190586746368, 50.62390960531435979 ) ) ;
#15754=CARTESIAN_POINT ( 'NONE',  ( 12.14591786802309770, 12.06949235617756955, 114.3739096053143527 ) ) ;
#15755=CARTESIAN_POINT ( 'NONE',  ( -0.05219959533936034679, 19.03943276465977164, 42.50109039468566152 ) ) ;
#15756=CARTESIAN_POINT ( 'NONE',  ( 5.049401038298161559, -19.05341960407611168, 82.70724293864770971 ) ) ;
#15757=CARTESIAN_POINT ( 'NONE',  ( 21.55341960407610458, 5.719274019375980345, 73.95724293864769550 ) ) ;
#15758=CARTESIAN_POINT ( 'NONE',  ( -8.224510206698948167, 14.34966873604960824, 85.41557627198102409 ) ) ;
#15759=CARTESIAN_POINT ( 'NONE',  ( 13.89961937509957401, 13.97604488694547697, 36.87609039468565442 ) ) ;
#15760=CARTESIAN_POINT ( 'NONE',  ( 0.05219959533907565091, 21.53943276465977519, 59.99890960531436690 ) ) ;
#15761=CARTESIAN_POINT ( 'NONE',  ( 18.62759615963271287, -10.81492255796078972, 38.33224293864768839 ) ) ;
#15762=CARTESIAN_POINT ( 'NONE',  ( -18.67979575497193778, 10.72451020669871902, 88.33442372801901854 ) ) ;
#15763=CARTESIAN_POINT ( 'NONE',  ( -9.474510206698964154, 16.51473224551069663, 60.41557627198102409 ) ) ;
#15764=CARTESIAN_POINT ( 'NONE',  ( -16.55341960407611168, -4.379528057220339221, 111.4572429386476813 ) ) ;
#15765=CARTESIAN_POINT ( 'NONE',  ( 15.72974639402176855, 15.80617190586768217, 21.87609039468567573 ) ) ;
#15766=CARTESIAN_POINT ( 'NONE',  ( -17.72560187377285246, -5.500000000000057732, 49.07814504131319211 ) ) ;
#15767=CARTESIAN_POINT ( 'NONE',  ( 21.52544592524334988, 5.823673210054432836, 36.45942372801901143 ) ) ;
#15768=CARTESIAN_POINT ( 'NONE',  ( -19.05341960407611168, -5.049401038298163336, 36.45724293864766707 ) ) ;
#15769=CARTESIAN_POINT ( 'NONE',  ( 21.55341960407610458, 5.719274019375980345, 103.9572429386476813 ) ) ;
#15770=CARTESIAN_POINT ( 'NONE',  ( -9.474510206698720793, -16.51473224551083518, 44.58442372801900433 ) ) ;
#15774=CARTESIAN_POINT ( 'NONE',  ( 8.314922557961029526, -14.29746914071037800, 65.41775706135234714 ) ) ;
#15775=CARTESIAN_POINT ( 'NONE',  ( 9.564922557960805705, 16.46253265017160317, 29.58224293864769550 ) ) ;
#15777=CARTESIAN_POINT ( 'NONE',  ( -0.05219959533909027116, -19.03943276465977164, 77.49890960531435269 ) ) ;
#15778=CARTESIAN_POINT ( 'NONE',  ( 12.14591786802309770, 12.06949235617756955, 109.3739096053143811 ) ) ;
#15779=CARTESIAN_POINT ( 'NONE',  ( 21.55341960407610458, 5.719274019375980345, 63.95724293864770260 ) ) ;
#15780=CARTESIAN_POINT ( 'NONE',  ( 4.483927247898790824, -16.52544592524335698, 35.20942372801901854 ) ) ;
#15781=CARTESIAN_POINT ( 'NONE',  ( 21.52544592524334988, 5.823673210054432836, 101.4594237280190185 ) ) ;
#15783=CARTESIAN_POINT ( 'NONE',  ( -4.483927247898782831, 16.52544592524335698, 112.7094237280190328 ) ) ;
#15784=CARTESIAN_POINT ( 'NONE',  ( 4.379528057220339221, -16.55341960407611168, 52.70724293864769550 ) ) ;
#15785=CARTESIAN_POINT ( 'NONE',  ( -13.89961937509977652, 13.97604488694528158, 45.62390960531433848 ) ) ;
#15786=CARTESIAN_POINT ( 'NONE',  ( -21.52544592524334988, -5.823673210054445271, 98.95942372801903275 ) ) ;
#15787=CARTESIAN_POINT ( 'NONE',  ( 18.62759615963271287, -10.81492255796078972, 113.3322429386476955 ) ) ;
#15788=CARTESIAN_POINT ( 'NONE',  ( 18.62759615963255655, 10.81492255796105972, 66.66775706135234714 ) ) ;
#15789=CARTESIAN_POINT ( 'NONE',  ( -14.29746914071037622, -8.314922557961029526, 59.16775706135234714 ) ) ;
#15790=CARTESIAN_POINT ( 'NONE',  ( 16.52544592524342804, -4.483927247898539470, 83.54057627198102409 ) ) ;
#15791=CARTESIAN_POINT ( 'NONE',  ( -18.62759615963255300, -10.81492255796106328, 99.16775706135234714 ) ) ;
#15792=CARTESIAN_POINT ( 'NONE',  ( 16.53943276465976808, 0.05219959533934440121, 111.2510903946856899 ) ) ;
#15793=CARTESIAN_POINT ( 'NONE',  ( 18.10062525802556266, -5.499999999999865885, 61.01383468041922953 ) ) ;
#15794=CARTESIAN_POINT ( 'NONE',  ( -8.314922557961024197, 14.29746914071037800, 37.91775706135235424 ) ) ;
#15795=CARTESIAN_POINT ( 'NONE',  ( 0.05219959533910956823, 16.53943276465976808, 39.99890960531436690 ) ) ;
#15796=CARTESIAN_POINT ( 'NONE',  ( -16.53943276465976808, -0.05219959533934237506, 83.75109039468568994 ) ) ;
#15797=CARTESIAN_POINT ( 'NONE',  ( -9.474510206698964154, 16.51473224551069663, 95.41557627198102409 ) ) ;
#15798=CARTESIAN_POINT ( 'NONE',  ( -21.53943276465977519, 0.05219959533907696930, 21.24890960531436690 ) ) ;
#15799=CARTESIAN_POINT ( 'NONE',  ( -0.05219959533937732626, 21.53943276465977519, 92.50109039468567573 ) ) ;
#15800=CARTESIAN_POINT ( 'NONE',  ( 16.53943276465976808, 0.05219959533934440121, 106.2510903946856757 ) ) ;
#15801=CARTESIAN_POINT ( 'NONE',  ( 0.05219959533910956823, 16.53943276465976808, 79.99890960531435269 ) ) ;
#15802=CARTESIAN_POINT ( 'NONE',  ( -5.049401038298153566, 19.05341960407611168, 85.20724293864766707 ) ) ;
#15804=CARTESIAN_POINT ( 'NONE',  ( -16.55341960407617563, 4.379528057220093196, 33.54275706135234714 ) ) ;
#15805=CARTESIAN_POINT ( 'NONE',  ( -9.474510206698964154, 16.51473224551069663, 40.41557627198103120 ) ) ;
#15806=CARTESIAN_POINT ( 'NONE',  ( 19.05341960407611168, 5.049401038298154454, 88.95724293864769550 ) ) ;
#15807=CARTESIAN_POINT ( 'NONE',  ( 0.05219959533934541429, -16.53943276465976808, 30.00109039468568284 ) ) ;
#15809=CARTESIAN_POINT ( 'NONE',  ( 16.51473224551083163, -9.474510206698727899, 40.83442372801900433 ) ) ;
#15810=CARTESIAN_POINT ( 'NONE',  ( -16.53943276465976808, -0.05219959533934237506, 88.75109039468567573 ) ) ;
#15811=CARTESIAN_POINT ( 'NONE',  ( 19.03943276465977164, -0.05219959533909143690, 38.74890960531436690 ) ) ;
#15812=CARTESIAN_POINT ( 'NONE',  ( 16.53943276465976808, 0.05219959533934440121, 76.25109039468568994 ) ) ;
#15813=CARTESIAN_POINT ( 'NONE',  ( 8.224510206698742110, 14.34966873604972548, 72.08442372801899012 ) ) ;
#15814=CARTESIAN_POINT ( 'NONE',  ( 19.05341960407617918, -5.049401038297876454, 86.04275706135233293 ) ) ;
#15815=CARTESIAN_POINT ( 'NONE',  ( -5.049401038297874678, -19.05341960407617918, 34.79275706135233293 ) ) ;
#15816=CARTESIAN_POINT ( 'NONE',  ( -5.049401038298153566, 19.05341960407611168, 45.20724293864769550 ) ) ;
#15817=CARTESIAN_POINT ( 'NONE',  ( -16.55341960407611168, -4.379528057220339221, 91.45724293864769550 ) ) ;
#15818=EDGE_CURVE ( 'NONE', #15160, #142224, #92027, .T. ) ;
#15819=CARTESIAN_POINT ( 'NONE',  ( 13.97604488694548053, -13.89961937509957401, 50.62609039468566152 ) ) ;
#15820=CARTESIAN_POINT ( 'NONE',  ( -15.72974639402197994, 15.80617190586746368, 50.62390960531435979 ) ) ;
#15821=CARTESIAN_POINT ( 'NONE',  ( -13.89961937509957401, -13.97604488694547875, 29.37609039468565797 ) ) ;
#15822=CARTESIAN_POINT ( 'NONE',  ( -0.05219959533909027116, -19.03943276465977164, 107.4989096053143527 ) ) ;
#15823=CARTESIAN_POINT ( 'NONE',  ( -10.72451020669898014, 18.67979575497178502, 80.41557627198103830 ) ) ;
#15824=CARTESIAN_POINT ( 'NONE',  ( -13.89961937509977652, 13.97604488694528158, 115.6239096053143669 ) ) ;
#15825=CARTESIAN_POINT ( 'NONE',  ( -19.03943276465977164, -0.05219959533935918106, 83.75109039468567573 ) ) ;
#15826=CARTESIAN_POINT ( 'NONE',  ( -17.49999999999999645, 3.805241302050257790, 110.3735247278259237 ) ) ;
#15827=CARTESIAN_POINT ( 'NONE',  ( -12.06949235617739369, -12.14591786802326823, 19.37609039468568639 ) ) ;
#15829=CARTESIAN_POINT ( 'NONE',  ( 16.51473224551069308, 9.474510206698969483, 39.16557627198103120 ) ) ;
#15830=CARTESIAN_POINT ( 'NONE',  ( 13.89961937509977652, -13.97604488694527269, 98.12390960531433848 ) ) ;
#15831=CARTESIAN_POINT ( 'NONE',  ( -18.62759615963270932, 10.81492255796079327, 75.83224293864769550 ) ) ;
#15833=CARTESIAN_POINT ( 'NONE',  ( -14.29746914071037622, -8.314922557961029526, 44.16775706135234714 ) ) ;
#15834=CARTESIAN_POINT ( 'NONE',  ( -15.72974639402176322, -15.80617190586768395, 49.37609039468569705 ) ) ;
#15835=CARTESIAN_POINT ( 'NONE',  ( -16.51473224551082808, 9.474510206698731452, 88.33442372801900433 ) ) ;
#15836=CARTESIAN_POINT ( 'NONE',  ( 5.719274019375673035, 21.55341960407619339, 107.2927570613523471 ) ) ;
#15837=CARTESIAN_POINT ( 'NONE',  ( 16.53943276465976808, 0.05219959533934440121, 111.2510903946856899 ) ) ;
#15838=CARTESIAN_POINT ( 'NONE',  ( -19.05341960407611168, -5.049401038298163336, 96.45724293864769550 ) ) ;
#15839=CARTESIAN_POINT ( 'NONE',  ( -4.379528057220328563, 16.55341960407611168, 90.20724293864770971 ) ) ;
#15840=CARTESIAN_POINT ( 'NONE',  ( -14.34966873604960291, -8.224510206698953496, 31.66557627198102054 ) ) ;
#15841=CARTESIAN_POINT ( 'NONE',  ( 0.05219959533936267826, -19.03943276465977164, 85.00109039468567573 ) ) ;
#15842=CARTESIAN_POINT ( 'NONE',  ( -18.62759615963255300, -10.81492255796106328, 64.16775706135234714 ) ) ;
#15843=CARTESIAN_POINT ( 'NONE',  ( 13.89961937509957401, 13.97604488694547697, 26.87609039468566507 ) ) ;
#15844=CARTESIAN_POINT ( 'NONE',  ( -8.224510206698948167, 14.34966873604960824, 105.4155762719810383 ) ) ;
#15845=CARTESIAN_POINT ( 'NONE',  ( -5.823673210054116645, -21.52544592524344225, 27.29057627198103120 ) ) ;
#15846=CARTESIAN_POINT ( 'NONE',  ( -16.55341960407617563, 4.379528057220093196, 113.5427570613523756 ) ) ;
#15847=CARTESIAN_POINT ( 'NONE',  ( -10.81492255796105439, 18.62759615963255655, 102.9177570613523756 ) ) ;
#15848=CARTESIAN_POINT ( 'NONE',  ( -4.379528057220086978, -16.55341960407618274, 64.79275706135234714 ) ) ;
#15849=CARTESIAN_POINT ( 'NONE',  ( 0.05219959533910956823, 16.53943276465976808, 24.99890960531435624 ) ) ;
#15850=CARTESIAN_POINT ( 'NONE',  ( 10.81492255796106328, -18.62759615963255655, 60.41775706135235424 ) ) ;
#15851=CARTESIAN_POINT ( 'NONE',  ( 15.80617190586769283, -15.72974639402175789, 50.62609039468568994 ) ) ;
#15854=CARTESIAN_POINT ( 'NONE',  ( 0.05219959533909260263, 19.03943276465977164, 24.99890960531435269 ) ) ;
#15855=CARTESIAN_POINT ( 'NONE',  ( -15.80617190586768217, 15.72974639402176855, 33.12609039468569705 ) ) ;
#15856=CARTESIAN_POINT ( 'NONE',  ( -16.55341960407611168, -4.379528057220339221, 106.4572429386477097 ) ) ;
#15857=CARTESIAN_POINT ( 'NONE',  ( -19.02544592524342804, 5.153800228976336051, 26.04057627198103120 ) ) ;
#15858=CARTESIAN_POINT ( 'NONE',  ( -8.314922557960811034, -14.29746914071050412, 77.08224293864769550 ) ) ;
#15859=CARTESIAN_POINT ( 'NONE',  ( 19.03943276465977164, -0.05219959533909143690, 68.74890960531436690 ) ) ;
#15860=CARTESIAN_POINT ( 'NONE',  ( 16.52544592524342804, -4.483927247898539470, 23.54057627198102765 ) ) ;
#15861=CARTESIAN_POINT ( 'NONE',  ( 18.62759615963271287, -10.81492255796078972, 53.33224293864769550 ) ) ;
#15862=CARTESIAN_POINT ( 'NONE',  ( -16.52544592524342804, 4.483927247898546575, 96.04057627198102409 ) ) ;
#15863=CARTESIAN_POINT ( 'NONE',  ( 15.72974639402199770, -15.80617190586745480, 93.12390960531436690 ) ) ;
#15864=CARTESIAN_POINT ( 'NONE',  ( 13.97604488694527802, 13.89961937509977652, 104.3739096053143385 ) ) ;
#15865=CARTESIAN_POINT ( 'NONE',  ( -0.05219959533909027116, -19.03943276465977164, 47.49890960531435979 ) ) ;
#15866=CARTESIAN_POINT ( 'NONE',  ( 16.46253265017146816, 9.564922557961045513, 111.6677570613523329 ) ) ;
#15867=CARTESIAN_POINT ( 'NONE',  ( 21.53943276465977519, -0.05219959533907433946, 48.74890960531435979 ) ) ;
#15868=CARTESIAN_POINT ( 'NONE',  ( 18.62759615963255655, 10.81492255796105972, 86.66775706135234714 ) ) ;
#15869=CARTESIAN_POINT ( 'NONE',  ( -19.05341960407611168, -5.049401038298163336, 71.45724293864766707 ) ) ;
#15870=CARTESIAN_POINT ( 'NONE',  ( -13.97604488694527625, -13.89961937509977652, 101.8739096053143811 ) ) ;
#15871=CARTESIAN_POINT ( 'NONE',  ( 4.379528057220092307, 16.55341960407617563, 77.29275706135234714 ) ) ;
#15872=CARTESIAN_POINT ( 'NONE',  ( -21.55341960407619339, 5.719274019375674811, 53.54275706135234714 ) ) ;
#15873=CARTESIAN_POINT ( 'NONE',  ( 10.81492255796106328, -18.62759615963255655, 80.41775706135234714 ) ) ;
#15874=CARTESIAN_POINT ( 'NONE',  ( -21.53943276465977519, 0.05219959533907696930, 106.2489096053143811 ) ) ;
#15875=CARTESIAN_POINT ( 'NONE',  ( -5.719274019375665041, -21.55341960407619695, 39.79275706135235424 ) ) ;
#15876=CARTESIAN_POINT ( 'NONE',  ( -16.53943276465976808, -0.05219959533934237506, 83.75109039468568994 ) ) ;
#15877=CARTESIAN_POINT ( 'NONE',  ( 0.05219959533907565091, 21.53943276465977519, 79.99890960531435269 ) ) ;
#15878=CARTESIAN_POINT ( 'NONE',  ( 13.97604488694548053, -13.89961937509957401, 30.62609039468566863 ) ) ;
#15879=CARTESIAN_POINT ( 'NONE',  ( -18.67979575497178146, -10.72451020669898902, 46.66557627198102409 ) ) ;
#15880=CARTESIAN_POINT ( 'NONE',  ( -19.05341960407611168, -5.049401038298163336, 76.45724293864769550 ) ) ;
#15881=CARTESIAN_POINT ( 'NONE',  ( 16.55341960407618274, -4.379528057220086978, 111.0427570613523613 ) ) ;
#15883=CARTESIAN_POINT ( 'NONE',  ( 5.049401038298161559, -19.05341960407611168, 112.7072429386476813 ) ) ;
#15885=CARTESIAN_POINT ( 'NONE',  ( -16.51473224551082808, 9.474510206698731452, 98.33442372801900433 ) ) ;
#15886=CARTESIAN_POINT ( 'NONE',  ( -10.72451020669898014, 18.67979575497178502, 75.41557627198102409 ) ) ;
#15887=CARTESIAN_POINT ( 'NONE',  ( -0.05219959533910754901, -16.53943276465976808, 37.49890960531436690 ) ) ;
#15888=CARTESIAN_POINT ( 'NONE',  ( -19.05341960407617563, 5.049401038297882671, 108.5427570613523187 ) ) ;
#15889=CARTESIAN_POINT ( 'NONE',  ( 13.89961937509977652, -13.97604488694527269, 33.12390960531434558 ) ) ;
#15890=CARTESIAN_POINT ( 'NONE',  ( -9.564922557961040184, 16.46253265017147172, 112.9177570613523329 ) ) ;
#15891=CARTESIAN_POINT ( 'NONE',  ( -21.55341960407610458, -5.719274019375992779, 106.4572429386477097 ) ) ;
#15892=CARTESIAN_POINT ( 'NONE',  ( 9.564922557961047289, -16.46253265017146816, 65.41775706135233293 ) ) ;
#15893=CARTESIAN_POINT ( 'NONE',  ( 12.06949235617739724, 12.14591786802326823, 81.87609039468568994 ) ) ;
#15894=CARTESIAN_POINT ( 'NONE',  ( -13.89961937509977652, 13.97604488694528158, 85.62390960531433848 ) ) ;
#15895=CARTESIAN_POINT ( 'NONE',  ( -8.224510206698948167, 14.34966873604960824, 75.41557627198102409 ) ) ;
#15896=CARTESIAN_POINT ( 'NONE',  ( -16.46253265017160317, 9.564922557960807481, 55.83224293864769550 ) ) ;
#15897=CARTESIAN_POINT ( 'NONE',  ( 8.224510206698953496, -14.34966873604960469, 62.91557627198102409 ) ) ;
#15898=CARTESIAN_POINT ( 'NONE',  ( -13.97604488694527625, -13.89961937509977652, 31.87390960531435979 ) ) ;
#15900=CARTESIAN_POINT ( 'NONE',  ( 16.52544592524342804, -4.483927247898539470, 43.54057627198103830 ) ) ;
#15901=CARTESIAN_POINT ( 'NONE',  ( 13.89961937509977652, -13.97604488694527269, 83.12390960531436690 ) ) ;
#15903=CARTESIAN_POINT ( 'NONE',  ( 13.89961937509957401, 13.97604488694547697, 46.87609039468565442 ) ) ;
#15904=CARTESIAN_POINT ( 'NONE',  ( 16.53943276465976808, 0.05219959533934440121, 56.25109039468568284 ) ) ;
#15905=CARTESIAN_POINT ( 'NONE',  ( 10.72451020669898902, -18.67979575497178502, 57.91557627198103120 ) ) ;
#15906=CARTESIAN_POINT ( 'NONE',  ( -9.564922557961040184, 16.46253265017147172, 27.91775706135232582 ) ) ;
#15907=CARTESIAN_POINT ( 'NONE',  ( -19.05341960407611168, -5.049401038298163336, 86.45724293864769550 ) ) ;
#15909=CARTESIAN_POINT ( 'NONE',  ( 21.55341960407610458, 5.719274019375980345, 33.95724293864769550 ) ) ;
#15910=CARTESIAN_POINT ( 'NONE',  ( 0.05219959533909260263, 19.03943276465977164, 59.99890960531436690 ) ) ;
#15911=CARTESIAN_POINT ( 'NONE',  ( -5.719274019375665041, -21.55341960407619695, 54.79275706135235424 ) ) ;
#15912=CARTESIAN_POINT ( 'NONE',  ( -14.29746914071049879, 8.314922557960819915, 100.8322429386477097 ) ) ;
#15913=CARTESIAN_POINT ( 'NONE',  ( -18.62759615963270932, 10.81492255796079327, 105.8322429386476955 ) ) ;
#15914=CARTESIAN_POINT ( 'NONE',  ( 13.89961937509977652, -13.97604488694527269, 93.12390960531436690 ) ) ;
#15916=CARTESIAN_POINT ( 'NONE',  ( -15.80617190586768217, 15.72974639402176855, 33.12609039468569705 ) ) ;
#15918=CARTESIAN_POINT ( 'NONE',  ( 13.89961937509977652, -13.97604488694527269, 88.12390960531438111 ) ) ;
#15919=CARTESIAN_POINT ( 'NONE',  ( 18.56453257813363678, -5.500000000000045297, 83.49000423690681316 ) ) ;
#15920=CARTESIAN_POINT ( 'NONE',  ( 21.52544592524344225, -5.823673210054117533, 88.54057627198103830 ) ) ;
#15921=CARTESIAN_POINT ( 'NONE',  ( -19.05341960407611168, -5.049401038298163336, 51.45724293864770260 ) ) ;
#15922=CARTESIAN_POINT ( 'NONE',  ( 16.55341960407618274, -4.379528057220086978, 21.04275706135234714 ) ) ;
#15924=CARTESIAN_POINT ( 'NONE',  ( 19.02544592524343514, -5.153800228976328945, 23.54057627198102054 ) ) ;
#15925=CARTESIAN_POINT ( 'NONE',  ( 10.72451020669871369, 18.67979575497193778, 87.08442372801901854 ) ) ;
#15926=CARTESIAN_POINT ( 'NONE',  ( -9.474510206698964154, 16.51473224551069663, 70.41557627198102409 ) ) ;
#15927=CARTESIAN_POINT ( 'NONE',  ( -15.80617190586768217, 15.72974639402176855, 53.12609039468568284 ) ) ;
#15928=CARTESIAN_POINT ( 'NONE',  ( -10.81492255796105439, 18.62759615963255655, 32.91775706135234714 ) ) ;
#15930=CARTESIAN_POINT ( 'NONE',  ( -13.89961937509977652, 13.97604488694528158, 95.62390960531436690 ) ) ;
#15932=CARTESIAN_POINT ( 'NONE',  ( 16.52544592524335698, 4.483927247898782831, 36.45942372801901143 ) ) ;
#15933=CARTESIAN_POINT ( 'NONE',  ( 4.379528057220092307, 16.55341960407617563, 72.29275706135236135 ) ) ;
#15934=CARTESIAN_POINT ( 'NONE',  ( 15.72974639402176855, 15.80617190586768217, 56.87609039468568994 ) ) ;
#15935=CARTESIAN_POINT ( 'NONE',  ( 0.05219959533937995610, -21.53943276465977519, 75.00109039468568994 ) ) ;
#15937=CARTESIAN_POINT ( 'NONE',  ( -4.379528057220086978, -16.55341960407618274, 19.79275706135235069 ) ) ;
#15938=CARTESIAN_POINT ( 'NONE',  ( -5.153800228976328057, -19.02544592524343514, 72.29057627198102409 ) ) ;
#15939=CARTESIAN_POINT ( 'NONE',  ( 16.46253265017160672, -9.564922557960803928, 98.33224293864769550 ) ) ;
#15940=CARTESIAN_POINT ( 'NONE',  ( 4.379528057220339221, -16.55341960407611168, 102.7072429386476955 ) ) ;
#15941=CARTESIAN_POINT ( 'NONE',  ( 4.379528057220339221, -16.55341960407611168, 102.7072429386476955 ) ) ;
#15942=CARTESIAN_POINT ( 'NONE',  ( -21.53943276465977519, 0.05219959533907696930, 26.24890960531435624 ) ) ;
#15943=CARTESIAN_POINT ( 'NONE',  ( -4.379528057220086978, -16.55341960407618274, 84.79275706135234714 ) ) ;
#15944=CARTESIAN_POINT ( 'NONE',  ( -0.05219959533910754901, -16.53943276465976808, 72.49890960531435269 ) ) ;
#15945=CARTESIAN_POINT ( 'NONE',  ( -5.153800228976328057, -19.02544592524343514, 52.29057627198100988 ) ) ;
#15946=CARTESIAN_POINT ( 'NONE',  ( 15.72974639402176855, 15.80617190586768217, 71.87609039468568994 ) ) ;
#15947=CARTESIAN_POINT ( 'NONE',  ( 5.719274019375673035, 21.55341960407619339, 72.29275706135236135 ) ) ;
#15948=CARTESIAN_POINT ( 'NONE',  ( -9.474510206698720793, -16.51473224551083518, 104.5844237280190043 ) ) ;
#15949=CARTESIAN_POINT ( 'NONE',  ( -0.05219959533910754901, -16.53943276465976808, 72.49890960531435269 ) ) ;
#15950=CARTESIAN_POINT ( 'NONE',  ( 15.72974639402176855, 15.80617190586768217, 26.87609039468567218 ) ) ;
#15951=CARTESIAN_POINT ( 'NONE',  ( -21.55341960407610458, -5.719274019375992779, 56.45724293864768839 ) ) ;
#15952=CARTESIAN_POINT ( 'NONE',  ( -17.26058549869089731, -6.457015423128557252, 106.3774583747607068 ) ) ;
#15954=CARTESIAN_POINT ( 'NONE',  ( -19.02544592524342804, 5.153800228976336051, 71.04057627198099567 ) ) ;
#15955=CARTESIAN_POINT ( 'NONE',  ( 8.224510206698953496, -14.34966873604960469, 52.91557627198103830 ) ) ;
#15956=CARTESIAN_POINT ( 'NONE',  ( -14.34966873604972548, 8.224510206698743886, 113.3344237280190328 ) ) ;
#15957=CARTESIAN_POINT ( 'NONE',  ( 16.55341960407618274, -4.379528057220086978, 96.04275706135236135 ) ) ;
#15958=CARTESIAN_POINT ( 'NONE',  ( -0.05219959533936034679, 19.03943276465977164, 57.50109039468566863 ) ) ;
#15960=CARTESIAN_POINT ( 'NONE',  ( 16.51473224551069308, 9.474510206698969483, 104.1655762719810241 ) ) ;
#15961=CARTESIAN_POINT ( 'NONE',  ( 4.379528057220339221, -16.55341960407611168, 72.70724293864769550 ) ) ;
#15962=CARTESIAN_POINT ( 'NONE',  ( -16.51473224551082808, 9.474510206698731452, 48.33442372801900433 ) ) ;
#15963=CARTESIAN_POINT ( 'NONE',  ( 5.153800228976335163, 19.02544592524342804, 29.79057627198102409 ) ) ;
#15964=CARTESIAN_POINT ( 'NONE',  ( -21.52544592524343514, 5.823673210054127303, 41.04057627198103120 ) ) ;
#15965=CARTESIAN_POINT ( 'NONE',  ( -5.719274019375978568, 21.55341960407610458, 60.20724293864768839 ) ) ;
#15967=CARTESIAN_POINT ( 'NONE',  ( -16.53943276465976808, 0.05219959533911058130, 96.24890960531435269 ) ) ;
#15968=CARTESIAN_POINT ( 'NONE',  ( 16.52544592524335698, 4.483927247898782831, 51.45942372801901854 ) ) ;
#15969=CARTESIAN_POINT ( 'NONE',  ( 16.53943276465976808, -0.05219959533910856209, 88.74890960531436690 ) ) ;
#15970=CARTESIAN_POINT ( 'NONE',  ( 16.18388926212235646, -7.379444403734663815, 37.06046848633847901 ) ) ;
#15972=CARTESIAN_POINT ( 'NONE',  ( 21.53943276465977519, -0.05219959533907433946, 33.74890960531436690 ) ) ;
#15976=CARTESIAN_POINT ( 'NONE',  ( 14.34966873604972726, -8.224510206698740333, 45.83442372801901854 ) ) ;
#15977=CARTESIAN_POINT ( 'NONE',  ( 8.314922557960818139, 14.29746914071049879, 24.58224293864768839 ) ) ;
#15978=CARTESIAN_POINT ( 'NONE',  ( -21.53943276465977519, 0.05219959533907696930, 51.24890960531436690 ) ) ;
#15979=CARTESIAN_POINT ( 'NONE',  ( -13.89961937509957401, -13.97604488694547875, 84.37609039468567573 ) ) ;
#15980=CARTESIAN_POINT ( 'NONE',  ( 18.62759615963271287, -10.81492255796078972, 58.33224293864768839 ) ) ;
#15981=CARTESIAN_POINT ( 'NONE',  ( 21.55341960407619695, -5.719274019375665929, 76.04275706135237556 ) ) ;
#15983=CARTESIAN_POINT ( 'NONE',  ( 4.379528057220092307, 16.55341960407617563, 42.29275706135235424 ) ) ;
#15984=CARTESIAN_POINT ( 'NONE',  ( 13.89961937509977652, -13.97604488694527269, 33.12390960531434558 ) ) ;
#15985=CARTESIAN_POINT ( 'NONE',  ( 5.153800228976335163, 19.02544592524342804, 94.79057627198103830 ) ) ;
#15987=CARTESIAN_POINT ( 'NONE',  ( -19.03943276465977164, 0.05219959533909376836, 36.24890960531436690 ) ) ;
#15988=CARTESIAN_POINT ( 'NONE',  ( -14.29746914071049879, 8.314922557960819915, 95.83224293864770971 ) ) ;
#15990=CARTESIAN_POINT ( 'NONE',  ( -0.05219959533909027116, -19.03943276465977164, 112.4989096053143669 ) ) ;
#15992=CARTESIAN_POINT ( 'NONE',  ( 4.483927247898790824, -16.52544592524335698, 65.20942372801901854 ) ) ;
#15993=CARTESIAN_POINT ( 'NONE',  ( -5.719274019375978568, 21.55341960407610458, 85.20724293864770971 ) ) ;
#15994=CARTESIAN_POINT ( 'NONE',  ( -9.474510206698964154, 16.51473224551069663, 55.41557627198103120 ) ) ;
#15995=CARTESIAN_POINT ( 'NONE',  ( 18.62759615963255655, 10.81492255796105972, 26.66775706135235424 ) ) ;
#15996=CARTESIAN_POINT ( 'NONE',  ( -16.51473224551069308, -9.474510206698971260, 76.66557627198103830 ) ) ;
#15999=CARTESIAN_POINT ( 'NONE',  ( 5.719274019375991003, -21.55341960407610458, 112.7072429386476955 ) ) ;
#16000=CARTESIAN_POINT ( 'NONE',  ( -13.89961937509977652, 13.97604488694528158, 25.62390960531434558 ) ) ;
#16001=CARTESIAN_POINT ( 'NONE',  ( -16.51473224551069308, -9.474510206698971260, 106.6655762719810383 ) ) ;
#16002=CARTESIAN_POINT ( 'NONE',  ( -16.46253265017146816, -9.564922557961047289, 74.16775706135234714 ) ) ;
#16003=CARTESIAN_POINT ( 'NONE',  ( -16.46253265017146816, -9.564922557961047289, 24.16775706135233648 ) ) ;
#16004=CARTESIAN_POINT ( 'NONE',  ( 5.719274019375991003, -21.55341960407610458, 102.7072429386476955 ) ) ;
#16005=CARTESIAN_POINT ( 'NONE',  ( 5.153800228976615827, -19.02544592524334988, 30.20942372801900433 ) ) ;
#16006=CARTESIAN_POINT ( 'NONE',  ( 8.224510206698742110, 14.34966873604972548, 77.08442372801901854 ) ) ;
#16007=CARTESIAN_POINT ( 'NONE',  ( -5.153800228976328057, -19.02544592524343514, 107.2905762719810383 ) ) ;
#16008=CARTESIAN_POINT ( 'NONE',  ( 5.153800228976335163, 19.02544592524342804, 59.79057627198100988 ) ) ;
#16010=CARTESIAN_POINT ( 'NONE',  ( 0.05219959533937995610, -21.53943276465977519, 60.00109039468568284 ) ) ;
#16011=CARTESIAN_POINT ( 'NONE',  ( -5.719274019375665041, -21.55341960407619695, 84.79275706135234714 ) ) ;
#16012=CARTESIAN_POINT ( 'NONE',  ( 9.474510206698971260, -16.51473224551069308, 72.91557627198102409 ) ) ;
#16013=CARTESIAN_POINT ( 'NONE',  ( 21.53943276465977519, 0.05219959533937863772, 46.25109039468567573 ) ) ;
#16014=CARTESIAN_POINT ( 'NONE',  ( -5.153800228976607833, 19.02544592524334988, 92.70942372801901854 ) ) ;
#16015=CARTESIAN_POINT ( 'NONE',  ( 16.46253265017160672, -9.564922557960803928, 58.33224293864769550 ) ) ;
#16016=CARTESIAN_POINT ( 'NONE',  ( -9.564922557960796823, -16.46253265017161027, 102.0822429386477097 ) ) ;
#16017=CARTESIAN_POINT ( 'NONE',  ( 16.46253265017160672, -9.564922557960803928, 63.33224293864769550 ) ) ;
#16018=CARTESIAN_POINT ( 'NONE',  ( -13.89961937509977652, 13.97604488694528158, 115.6239096053143669 ) ) ;
#16019=CARTESIAN_POINT ( 'NONE',  ( -16.46253265017160317, 9.564922557960807481, 45.83224293864769550 ) ) ;
#16020=CARTESIAN_POINT ( 'NONE',  ( -0.05219959533907301413, -21.53943276465977519, 102.4989096053143811 ) ) ;
#16021=CARTESIAN_POINT ( 'NONE',  ( 4.483927247898790824, -16.52544592524335698, 90.20942372801903275 ) ) ;
#16023=CARTESIAN_POINT ( 'NONE',  ( -13.97604488694547697, 13.89961937509957934, 48.12609039468566863 ) ) ;
#16024=CARTESIAN_POINT ( 'NONE',  ( -13.89961937509977652, 13.97604488694528158, 60.62390960531436690 ) ) ;
#16025=CARTESIAN_POINT ( 'NONE',  ( 14.29746914071049879, -8.314922557960816363, 58.33224293864768839 ) ) ;
#16026=CARTESIAN_POINT ( 'NONE',  ( 0.05219959533910956823, 16.53943276465976808, 89.99890960531438111 ) ) ;
#16027=CARTESIAN_POINT ( 'NONE',  ( -21.55341960407610458, -5.719274019375992779, 21.45724293864769550 ) ) ;
#16028=CARTESIAN_POINT ( 'NONE',  ( 9.474510206698971260, -16.51473224551069308, 87.91557627198102409 ) ) ;
#16029=CARTESIAN_POINT ( 'NONE',  ( -19.03943276465977164, 0.05219959533909376836, 106.2489096053143669 ) ) ;
#16030=CARTESIAN_POINT ( 'NONE',  ( 10.72451020669871369, 18.67979575497193778, 112.0844237280190185 ) ) ;
#16031=CARTESIAN_POINT ( 'NONE',  ( -14.34966873604972548, 8.224510206698743886, 88.33442372801901854 ) ) ;
#16032=CARTESIAN_POINT ( 'NONE',  ( -9.474510206698964154, 16.51473224551069663, 80.41557627198103830 ) ) ;
#16033=CARTESIAN_POINT ( 'NONE',  ( 5.719274019375673035, 21.55341960407619339, 42.29275706135235424 ) ) ;
#16034=CARTESIAN_POINT ( 'NONE',  ( 5.823673210054125526, 21.52544592524343514, 24.79057627198103120 ) ) ;
#16035=CARTESIAN_POINT ( 'NONE',  ( -21.55341960407610458, -5.719274019375992779, 106.4572429386477097 ) ) ;
#16036=CARTESIAN_POINT ( 'NONE',  ( -12.14591786802309592, -12.06949235617757132, 61.87390960531436690 ) ) ;
#16037=CARTESIAN_POINT ( 'NONE',  ( 9.564922557960805705, 16.46253265017160317, 59.58224293864769550 ) ) ;
#16038=CARTESIAN_POINT ( 'NONE',  ( -8.224510206698948167, 14.34966873604960824, 80.41557627198103830 ) ) ;
#16039=CARTESIAN_POINT ( 'NONE',  ( -5.153800228976607833, 19.02544592524334988, 42.70942372801901143 ) ) ;
#16040=CARTESIAN_POINT ( 'NONE',  ( -8.314922557960811034, -14.29746914071050412, 112.0822429386477097 ) ) ;
#16041=CARTESIAN_POINT ( 'NONE',  ( -5.049401038298153566, 19.05341960407611168, 85.20724293864766707 ) ) ;
#16042=CARTESIAN_POINT ( 'NONE',  ( -19.02544592524342804, 5.153800228976336051, 81.04057627198103830 ) ) ;
#16044=CARTESIAN_POINT ( 'NONE',  ( 8.314922557960818139, 14.29746914071049879, 94.58224293864769550 ) ) ;
#16046=CARTESIAN_POINT ( 'NONE',  ( 4.379528057220092307, 16.55341960407617563, 112.2927570613523471 ) ) ;
#16047=CARTESIAN_POINT ( 'NONE',  ( -4.379528057220086978, -16.55341960407618274, 24.79275706135235779 ) ) ;
#16048=CARTESIAN_POINT ( 'NONE',  ( -10.72451020669870658, -18.67979575497194134, 99.58442372801900433 ) ) ;
#16049=CARTESIAN_POINT ( 'NONE',  ( -5.153800228976328057, -19.02544592524343514, 87.29057627198103830 ) ) ;
#16050=CARTESIAN_POINT ( 'NONE',  ( -21.53943276465977519, -0.05219959533937600094, 23.75109039468567929 ) ) ;
#16051=CARTESIAN_POINT ( 'NONE',  ( -13.97604488694527625, -13.89961937509977652, 31.87390960531435979 ) ) ;
#16053=CARTESIAN_POINT ( 'NONE',  ( 16.52544592524335698, 4.483927247898782831, 36.45942372801901143 ) ) ;
#16054=CARTESIAN_POINT ( 'NONE',  ( 19.02544592524334988, 5.153800228976608722, 101.4594237280189759 ) ) ;
#16055=CARTESIAN_POINT ( 'NONE',  ( 5.823673210054125526, 21.52544592524343514, 94.79057627198105251 ) ) ;
#16056=CARTESIAN_POINT ( 'NONE',  ( -13.97604488694547697, 13.89961937509957934, 73.12609039468568994 ) ) ;
#16057=CARTESIAN_POINT ( 'NONE',  ( 13.97604488694527802, 13.89961937509977652, 24.37390960531435624 ) ) ;
#16058=CARTESIAN_POINT ( 'NONE',  ( -18.67979575497193778, 10.72451020669871902, 23.33442372801901499 ) ) ;
#16060=CARTESIAN_POINT ( 'NONE',  ( 19.02544592524343514, -5.153800228976328945, 93.54057627198102409 ) ) ;
#16061=CARTESIAN_POINT ( 'NONE',  ( 4.379528057220092307, 16.55341960407617563, 52.29275706135236135 ) ) ;
#16063=CARTESIAN_POINT ( 'NONE',  ( -16.51473224551082808, 9.474510206698731452, 63.33442372801900433 ) ) ;
#16064=CARTESIAN_POINT ( 'NONE',  ( 15.72974639402176855, 15.80617190586768217, 21.87609039468567573 ) ) ;
#16065=CARTESIAN_POINT ( 'NONE',  ( -0.05219959533910754901, -16.53943276465976808, 77.49890960531433848 ) ) ;
#16066=CARTESIAN_POINT ( 'NONE',  ( -13.97604488694527625, -13.89961937509977652, 86.87390960531436690 ) ) ;
#16067=CARTESIAN_POINT ( 'NONE',  ( 8.314922557961029526, -14.29746914071037800, 50.41775706135235424 ) ) ;
#16068=CARTESIAN_POINT ( 'NONE',  ( -19.03943276465977164, -0.05219959533935918106, 58.75109039468566863 ) ) ;
#16069=CARTESIAN_POINT ( 'NONE',  ( -18.67979575497193778, 10.72451020669871902, 63.33442372801900433 ) ) ;
#16070=CARTESIAN_POINT ( 'NONE',  ( -8.224510206698735004, -14.34966873604973081, 29.58442372801901854 ) ) ;
#16071=CARTESIAN_POINT ( 'NONE',  ( -9.564922557960796823, -16.46253265017161027, 72.08224293864770971 ) ) ;
#16072=CARTESIAN_POINT ( 'NONE',  ( 16.46253265017146816, 9.564922557961045513, 81.66775706135233293 ) ) ;
#16073=CARTESIAN_POINT ( 'NONE',  ( -16.52544592524335698, -4.483927247898792601, 53.95942372801900433 ) ) ;
#16074=CARTESIAN_POINT ( 'NONE',  ( -21.52544592524334988, -5.823673210054445271, 93.95942372801903275 ) ) ;
#16075=CARTESIAN_POINT ( 'NONE',  ( 19.03943276465977164, 0.05219959533936151252, 86.25109039468567573 ) ) ;
#16076=CARTESIAN_POINT ( 'NONE',  ( -16.51473224551069308, -9.474510206698971260, 56.66557627198103120 ) ) ;
#16077=CARTESIAN_POINT ( 'NONE',  ( -0.05219959533907301413, -21.53943276465977519, 72.49890960531435269 ) ) ;
#16078=CARTESIAN_POINT ( 'NONE',  ( -12.06949235617756955, 12.14591786802309770, 70.62390960531436690 ) ) ;
#16079=CARTESIAN_POINT ( 'NONE',  ( 19.03943276465977164, 0.05219959533936151252, 81.25109039468567573 ) ) ;
#16081=CARTESIAN_POINT ( 'NONE',  ( -16.51473224551082808, 9.474510206698731452, 48.33442372801900433 ) ) ;
#16082=CARTESIAN_POINT ( 'NONE',  ( 0.05219959533934541429, -16.53943276465976808, 100.0010903946857042 ) ) ;
#16083=CARTESIAN_POINT ( 'NONE',  ( -8.314922557960811034, -14.29746914071050412, 72.08224293864769550 ) ) ;
#16084=CARTESIAN_POINT ( 'NONE',  ( -15.80617190586768217, 15.72974639402176855, 108.1260903946856757 ) ) ;
#16086=CARTESIAN_POINT ( 'NONE',  ( 10.81492255796078972, 18.62759615963270932, 104.5822429386477097 ) ) ;
#16087=CARTESIAN_POINT ( 'NONE',  ( 0.05219959533909260263, 19.03943276465977164, 59.99890960531436690 ) ) ;
#16088=CARTESIAN_POINT ( 'NONE',  ( -10.72451020669870658, -18.67979575497194134, 74.58442372801901854 ) ) ;
#16089=CARTESIAN_POINT ( 'NONE',  ( 19.02544592524343514, -5.153800228976328945, 48.54057627198103120 ) ) ;
#16091=CARTESIAN_POINT ( 'NONE',  ( -0.05219959533909027116, -19.03943276465977164, 27.49890960531435624 ) ) ;
#16092=CARTESIAN_POINT ( 'NONE',  ( -13.89961937509977652, 13.97604488694528158, 110.6239096053143243 ) ) ;
#16093=CARTESIAN_POINT ( 'NONE',  ( -12.14591786802309592, -12.06949235617757132, 66.87390960531436690 ) ) ;
#16094=CARTESIAN_POINT ( 'NONE',  ( 9.564922557960805705, 16.46253265017160317, 24.58224293864769194 ) ) ;
#16095=CARTESIAN_POINT ( 'NONE',  ( 8.314922557960818139, 14.29746914071049879, 79.58224293864769550 ) ) ;
#16096=CARTESIAN_POINT ( 'NONE',  ( 10.81492255796078972, 18.62759615963270932, 94.58224293864769550 ) ) ;
#16097=CARTESIAN_POINT ( 'NONE',  ( 18.67979575497194134, -10.72451020669871369, 45.83442372801901854 ) ) ;
#16099=CARTESIAN_POINT ( 'NONE',  ( 12.06949235617739724, 12.14591786802326823, 51.87609039468568284 ) ) ;
#16100=CARTESIAN_POINT ( 'NONE',  ( -0.05219959533907301413, -21.53943276465977519, 102.4989096053143811 ) ) ;
#16101=CARTESIAN_POINT ( 'NONE',  ( -9.564922557961040184, 16.46253265017147172, 32.91775706135233293 ) ) ;
#16102=CARTESIAN_POINT ( 'NONE',  ( -16.46253265017160317, 9.564922557960807481, 105.8322429386476955 ) ) ;
#16103=CARTESIAN_POINT ( 'NONE',  ( 10.81492255796106328, -18.62759615963255655, 50.41775706135235424 ) ) ;
#16104=CARTESIAN_POINT ( 'NONE',  ( -5.719274019375978568, 21.55341960407610458, 40.20724293864769550 ) ) ;
#16105=CARTESIAN_POINT ( 'NONE',  ( -14.29746914071049879, 8.314922557960819915, 25.83224293864769194 ) ) ;
#16106=CARTESIAN_POINT ( 'NONE',  ( 18.67979575497194134, -10.72451020669871369, 60.83442372801901854 ) ) ;
#16107=CARTESIAN_POINT ( 'NONE',  ( -21.52544592524334988, -5.823673210054445271, 98.95942372801903275 ) ) ;
#16108=CARTESIAN_POINT ( 'NONE',  ( 19.03943276465977164, 0.05219959533936151252, 26.25109039468566507 ) ) ;
#16109=CARTESIAN_POINT ( 'NONE',  ( 8.224510206698742110, 14.34966873604972548, 82.08442372801901854 ) ) ;
#16110=CARTESIAN_POINT ( 'NONE',  ( 21.52544592524334988, 5.823673210054432836, 51.45942372801901854 ) ) ;
#16111=CARTESIAN_POINT ( 'NONE',  ( -9.474510206698964154, 16.51473224551069663, 40.41557627198103120 ) ) ;
#16112=CARTESIAN_POINT ( 'NONE',  ( -19.03943276465977164, -0.05219959533935918106, 18.75109039468567218 ) ) ;
#16113=CARTESIAN_POINT ( 'NONE',  ( -21.52544592524343514, 5.823673210054127303, 26.04057627198103475 ) ) ;
#16114=CARTESIAN_POINT ( 'NONE',  ( -15.80617190586745835, -15.72974639402198527, 111.8739096053143669 ) ) ;
#16116=CARTESIAN_POINT ( 'NONE',  ( 18.62759615963271287, -10.81492255796078972, 78.33224293864770971 ) ) ;
#16117=CARTESIAN_POINT ( 'NONE',  ( 4.379528057220092307, 16.55341960407617563, 42.29275706135235424 ) ) ;
#16119=CARTESIAN_POINT ( 'NONE',  ( -10.81492255796078084, -18.62759615963271287, 82.08224293864768129 ) ) ;
#16120=CARTESIAN_POINT ( 'NONE',  ( 12.06949235617739724, 12.14591786802326823, 66.87609039468568994 ) ) ;
#16121=B_SPLINE_CURVE_WITH_KNOTS ( 'NONE', 3,
 ( #174272, #35740, #186472, #62095, #158093, #185457, #95418, #110588, #18599, #188444, #49923, #34747, #9415, #113565, #160085, #51906, #102414, #20567, #21571, #5391 ),
 .UNSPECIFIED., .F., .F.,
 ( 4, 2, 2, 2, 2, 2, 2, 2, 2, 4 ),
 ( 0.004000878361811972990, 0.004499404418915994158, 0.004997930476020014459, 0.005496456533124034760, 0.005994982590228055928, 0.006244245618780045262, 0.006493508647332034596, 0.006992034704436017600, 0.007490560761540001472, 0.007989086818643985344 ),
 .UNSPECIFIED. ) ;
#16122=CARTESIAN_POINT ( 'NONE',  ( -14.34966873604960291, -8.224510206698953496, 61.66557627198103120 ) ) ;
#16124=CARTESIAN_POINT ( 'NONE',  ( -19.05341960407617563, 5.049401038297882671, 98.54275706135233293 ) ) ;
#16126=CARTESIAN_POINT ( 'NONE',  ( -4.379528057220086978, -16.55341960407618274, 39.79275706135235424 ) ) ;
#16127=CARTESIAN_POINT ( 'NONE',  ( -21.52544592524343514, 5.823673210054127303, 106.0405762719810525 ) ) ;
#16128=CARTESIAN_POINT ( 'NONE',  ( -10.72451020669898014, 18.67979575497178502, 25.41557627198103120 ) ) ;
#16129=CARTESIAN_POINT ( 'NONE',  ( 14.29746914071037800, 8.314922557961029526, 51.66775706135234714 ) ) ;
#16130=CARTESIAN_POINT ( 'NONE',  ( -9.564922557960796823, -16.46253265017161027, 77.08224293864769550 ) ) ;
#16131=CARTESIAN_POINT ( 'NONE',  ( 5.823673210054444382, -21.52544592524334988, 45.20942372801901854 ) ) ;
#16132=CARTESIAN_POINT ( 'NONE',  ( 5.049401038297881783, 19.05341960407617563, 112.2927570613523471 ) ) ;
#16133=CARTESIAN_POINT ( 'NONE',  ( -18.62759615963270932, 10.81492255796079327, 25.83224293864769194 ) ) ;
#16134=VERTEX_POINT ( 'NONE', #178309 ) ;
#16135=CARTESIAN_POINT ( 'NONE',  ( -16.46253265017146816, -9.564922557961047289, 29.16775706135232937 ) ) ;
#16136=CARTESIAN_POINT ( 'NONE',  ( 8.314922557961029526, -14.29746914071037800, 40.41775706135234714 ) ) ;
#16137=CARTESIAN_POINT ( 'NONE',  ( 9.564922557960805705, 16.46253265017160317, 94.58224293864769550 ) ) ;
#16138=CARTESIAN_POINT ( 'NONE',  ( -15.80617190586745835, -15.72974639402198527, 106.8739096053143811 ) ) ;
#16139=CARTESIAN_POINT ( 'NONE',  ( -19.02544592524342804, 5.153800228976336051, 71.04057627198099567 ) ) ;
#16141=CARTESIAN_POINT ( 'NONE',  ( -12.14591786802309592, -12.06949235617757132, 81.87390960531435269 ) ) ;
#16142=CARTESIAN_POINT ( 'NONE',  ( 19.03943276465977164, -0.05219959533909143690, 113.7489096053143669 ) ) ;
#16143=CARTESIAN_POINT ( 'NONE',  ( -17.12812012977024878, 6.668231424566046783, 33.64051240676857191 ) ) ;
#16144=CARTESIAN_POINT ( 'NONE',  ( 8.314922557961029526, -14.29746914071037800, 65.41775706135234714 ) ) ;
#16145=CARTESIAN_POINT ( 'NONE',  ( -18.62759615963270932, 10.81492255796079327, 105.8322429386476955 ) ) ;
#16146=CARTESIAN_POINT ( 'NONE',  ( -9.474510206698720793, -16.51473224551083518, 64.58442372801900433 ) ) ;
#16147=CARTESIAN_POINT ( 'NONE',  ( 5.719274019375991003, -21.55341960407610458, 27.70724293864769905 ) ) ;
#16148=CARTESIAN_POINT ( 'NONE',  ( 0.05219959533909260263, 19.03943276465977164, 24.99890960531435269 ) ) ;
#16149=CARTESIAN_POINT ( 'NONE',  ( -10.81492255796078084, -18.62759615963271287, 67.08224293864770971 ) ) ;
#16151=CARTESIAN_POINT ( 'NONE',  ( 16.46253265017160672, -9.564922557960803928, 93.33224293864769550 ) ) ;
#16152=CARTESIAN_POINT ( 'NONE',  ( 10.72451020669871369, 18.67979575497193778, 92.08442372801901854 ) ) ;
#16153=CARTESIAN_POINT ( 'NONE',  ( -19.03943276465977164, 0.05219959533909376836, 56.24890960531435979 ) ) ;
#16154=CARTESIAN_POINT ( 'NONE',  ( -4.483927247898782831, 16.52544592524335698, 37.70942372801900433 ) ) ;
#16155=CARTESIAN_POINT ( 'NONE',  ( 0.05219959533909260263, 19.03943276465977164, 54.99890960531435979 ) ) ;
#16156=CARTESIAN_POINT ( 'NONE',  ( -5.719274019375665041, -21.55341960407619695, 74.79275706135234714 ) ) ;
#16158=CARTESIAN_POINT ( 'NONE',  ( 16.51473224551083163, -9.474510206698727899, 40.83442372801900433 ) ) ;
#16159=CARTESIAN_POINT ( 'NONE',  ( 19.02544592524334988, 5.153800228976608722, 46.45942372801899012 ) ) ;
#16160=CARTESIAN_POINT ( 'NONE',  ( 0.05219959533937995610, -21.53943276465977519, 35.00109039468568284 ) ) ;
#16162=CARTESIAN_POINT ( 'NONE',  ( -5.049401038297874678, -19.05341960407617918, 29.79275706135232227 ) ) ;
#16163=CARTESIAN_POINT ( 'NONE',  ( -5.153800228976328057, -19.02544592524343514, 87.29057627198103830 ) ) ;
#16164=CARTESIAN_POINT ( 'NONE',  ( -5.049401038298153566, 19.05341960407611168, 65.20724293864765286 ) ) ;
#16165=CARTESIAN_POINT ( 'NONE',  ( 16.55341960407611168, 4.379528057220329451, 28.95724293864769905 ) ) ;
#16166=CARTESIAN_POINT ( 'NONE',  ( 9.474510206698971260, -16.51473224551069308, 112.9155762719810383 ) ) ;
#16167=CARTESIAN_POINT ( 'NONE',  ( -15.72974639402176322, -15.80617190586768395, 84.37609039468570415 ) ) ;
#16169=CARTESIAN_POINT ( 'NONE',  ( 16.38665767535054130, 7.295008042176050367, 57.23599135785458003 ) ) ;
#16170=CARTESIAN_POINT ( 'NONE',  ( 10.72451020669871369, 18.67979575497193778, 97.08442372801904696 ) ) ;
#16171=CARTESIAN_POINT ( 'NONE',  ( 17.48847506799967988, -5.747544572773779947, 43.32697437843280852 ) ) ;
#16172=CARTESIAN_POINT ( 'NONE',  ( -0.05219959533909027116, -19.03943276465977164, 27.49890960531435624 ) ) ;
#16175=CARTESIAN_POINT ( 'NONE',  ( -14.34966873604972548, 8.224510206698743886, 53.33442372801901854 ) ) ;
#16176=CARTESIAN_POINT ( 'NONE',  ( 0.05219959533907565091, 21.53943276465977519, 74.99890960531435269 ) ) ;
#16177=CARTESIAN_POINT ( 'NONE',  ( -4.379528057220328563, 16.55341960407611168, 40.20724293864769550 ) ) ;
#16178=CARTESIAN_POINT ( 'NONE',  ( 12.06949235617757843, -12.14591786802309237, 108.1239096053143811 ) ) ;
#16179=CARTESIAN_POINT ( 'NONE',  ( 16.51473224551069308, 9.474510206698969483, 89.16557627198103830 ) ) ;
#16180=CARTESIAN_POINT ( 'NONE',  ( -19.05341960407617563, 5.049401038297882671, 23.54275706135233648 ) ) ;
#16181=CARTESIAN_POINT ( 'NONE',  ( -19.02544592524342804, 5.153800228976336051, 26.04057627198103120 ) ) ;
#16182=CARTESIAN_POINT ( 'NONE',  ( 15.80617190586769283, -15.72974639402175789, 70.62609039468567573 ) ) ;
#16183=FACE_OUTER_BOUND ( 'NONE', #147162, .T. ) ;
#16184=CARTESIAN_POINT ( 'NONE',  ( -16.55341960407617563, 4.379528057220093196, 113.5427570613523756 ) ) ;
#16185=CARTESIAN_POINT ( 'NONE',  ( -19.05341960407617563, 5.049401038297882671, 58.54275706135234003 ) ) ;
#16187=CARTESIAN_POINT ( 'NONE',  ( -15.72974639402197994, 15.80617190586746368, 25.62390960531435624 ) ) ;
#16188=CARTESIAN_POINT ( 'NONE',  ( -16.55341960407611168, -4.379528057220339221, 96.45724293864770971 ) ) ;
#16189=CARTESIAN_POINT ( 'NONE',  ( 13.89961937509957401, 13.97604488694547697, 51.87609039468566863 ) ) ;
#16190=CARTESIAN_POINT ( 'NONE',  ( -5.049401038298153566, 19.05341960407611168, 70.20724293864769550 ) ) ;
#16191=CARTESIAN_POINT ( 'NONE',  ( 16.52544592524342804, -4.483927247898539470, 68.54057627198103830 ) ) ;
#16192=CARTESIAN_POINT ( 'NONE',  ( -5.049401038297874678, -19.05341960407617918, 89.79275706135230450 ) ) ;
#16193=CARTESIAN_POINT ( 'NONE',  ( -18.67979575497178146, -10.72451020669898902, 51.66557627198102409 ) ) ;
#16194=EDGE_LOOP ( 'NONE', ( #158664, #51672, #151674, #15230 ) ) ;
#16195=CARTESIAN_POINT ( 'NONE',  ( -14.34966873604960291, -8.224510206698953496, 111.6655762719810525 ) ) ;
#16197=CARTESIAN_POINT ( 'NONE',  ( 9.474510206698971260, -16.51473224551069308, 72.91557627198102409 ) ) ;
#16198=CARTESIAN_POINT ( 'NONE',  ( -21.53943276465977519, 0.05219959533907696930, 71.24890960531435269 ) ) ;
#16199=CARTESIAN_POINT ( 'NONE',  ( -16.53943276465976808, -0.05219959533934237506, 93.75109039468567573 ) ) ;
#16200=CARTESIAN_POINT ( 'NONE',  ( 9.564922557960805705, 16.46253265017160317, 74.58224293864769550 ) ) ;
#16201=CARTESIAN_POINT ( 'NONE',  ( -19.03943276465977164, -0.05219959533935918106, 68.75109039468566152 ) ) ;
#16202=CARTESIAN_POINT ( 'NONE',  ( 10.81492255796106328, -18.62759615963255655, 75.41775706135233293 ) ) ;
#16203=CARTESIAN_POINT ( 'NONE',  ( -18.62759615963270932, 10.81492255796079327, 60.83224293864769550 ) ) ;
#16204=CARTESIAN_POINT ( 'NONE',  ( -5.719274019375978568, 21.55341960407610458, 25.20724293864769550 ) ) ;
#16205=CARTESIAN_POINT ( 'NONE',  ( 13.89961937509977652, -13.97604488694527269, 33.12390960531434558 ) ) ;
#16206=CARTESIAN_POINT ( 'NONE',  ( -16.53943276465976808, -0.05219959533934237506, 98.75109039468568994 ) ) ;
#16207=CARTESIAN_POINT ( 'NONE',  ( -5.153800228976328057, -19.02544592524343514, 47.29057627198102409 ) ) ;
#16208=CARTESIAN_POINT ( 'NONE',  ( -14.34966873604972548, 8.224510206698743886, 23.33442372801901499 ) ) ;
#16209=CARTESIAN_POINT ( 'NONE',  ( 5.049401038297881783, 19.05341960407617918, 82.29275706135231871 ) ) ;
#16210=CARTESIAN_POINT ( 'NONE',  ( 19.03943276465977164, 0.05219959533936151252, 21.25109039468565797 ) ) ;
#16211=CARTESIAN_POINT ( 'NONE',  ( -4.483927247898539470, -16.52544592524342804, 57.29057627198103120 ) ) ;
#16212=CARTESIAN_POINT ( 'NONE',  ( -21.53943276465977519, 0.05219959533907696930, 91.24890960531436690 ) ) ;
#16213=CARTESIAN_POINT ( 'NONE',  ( -15.72974639402197994, 15.80617190586746368, 95.62390960531436690 ) ) ;
#16215=CARTESIAN_POINT ( 'NONE',  ( -18.67979575497178146, -10.72451020669898902, 41.66557627198103120 ) ) ;
#16217=CARTESIAN_POINT ( 'NONE',  ( -8.314922557961024197, 14.29746914071037800, 77.91775706135231871 ) ) ;
#16218=CARTESIAN_POINT ( 'NONE',  ( -16.52544592524342804, 4.483927247898546575, 86.04057627198102409 ) ) ;
#16219=B_SPLINE_CURVE_WITH_KNOTS ( 'NONE', 3,
 ( #97040, #128381, #189097, #80886, #67716, #8038, #4042, #65719, #50570, #112230, #35389, #20212, #36371, #98025, #169436, #139097, #46098, #119232, #72732, #164739 ),
 .UNSPECIFIED., .F., .F.,
 ( 4, 2, 2, 2, 2, 2, 2, 2, 2, 4 ),
 ( 0.000000000000000000, 0.0004987090165372827857, 0.0009974180330745655715, 0.001246772541343199809, 0.001496127049611834263, 0.001994836066149079535, 0.002493545082686324590, 0.002742899590954957310, 0.002992254099223589162, 0.003989672132298133049 ),
 .UNSPECIFIED. ) ;
#16220=CARTESIAN_POINT ( 'NONE',  ( -0.05219959533909027116, -19.03943276465977164, 52.49890960531436690 ) ) ;
#16221=SURFACE_STYLE_USAGE ( .BOTH. , #18215 ) ;
#16223=CARTESIAN_POINT ( 'NONE',  ( 8.224510206698742110, 14.34966873604972548, 107.0844237280190043 ) ) ;
#16224=CARTESIAN_POINT ( 'NONE',  ( -21.55341960407619339, 5.719274019375674811, 28.54275706135234358 ) ) ;
#16225=CARTESIAN_POINT ( 'NONE',  ( 0.05219959533909260263, 19.03943276465977164, 99.99890960531436690 ) ) ;
#16226=CARTESIAN_POINT ( 'NONE',  ( 15.80617190586769283, -15.72974639402175789, 70.62609039468567573 ) ) ;
#16227=CARTESIAN_POINT ( 'NONE',  ( -19.03943276465977164, 0.05219959533909376836, 21.24890960531436335 ) ) ;
#16230=CARTESIAN_POINT ( 'NONE',  ( 15.80617190586769283, -15.72974639402175789, 60.62609039468567573 ) ) ;
#16231=CARTESIAN_POINT ( 'NONE',  ( 13.97604488694527802, 13.89961937509977652, 54.37390960531435979 ) ) ;
#16232=CARTESIAN_POINT ( 'NONE',  ( 19.02544592524343514, -5.153800228976328945, 23.54057627198102054 ) ) ;
#16233=CARTESIAN_POINT ( 'NONE',  ( -16.46253265017160317, 9.564922557960807481, 95.83224293864769550 ) ) ;
#16234=CARTESIAN_POINT ( 'NONE',  ( 19.05341960407617918, -5.049401038297876454, 66.04275706135233293 ) ) ;
#16235=CARTESIAN_POINT ( 'NONE',  ( 15.72974639402176855, 15.80617190586768217, 41.87609039468568284 ) ) ;
#16236=CARTESIAN_POINT ( 'NONE',  ( -16.51473224551082808, 9.474510206698731452, 98.33442372801900433 ) ) ;
#16237=CARTESIAN_POINT ( 'NONE',  ( -9.474510206698720793, -16.51473224551083518, 69.58442372801901854 ) ) ;
#16238=CARTESIAN_POINT ( 'NONE',  ( -5.153800228976328057, -19.02544592524343514, 32.29057627198102409 ) ) ;
#16239=CARTESIAN_POINT ( 'NONE',  ( -14.34966873604972548, 8.224510206698743886, 103.3344237280190043 ) ) ;
#16240=CARTESIAN_POINT ( 'NONE',  ( -13.89961937509957401, -13.97604488694547875, 74.37609039468566152 ) ) ;
#16241=CARTESIAN_POINT ( 'NONE',  ( -16.53943276465976808, 0.05219959533911058130, 31.24890960531435979 ) ) ;
#16242=CARTESIAN_POINT ( 'NONE',  ( 19.05341960407617918, -5.049401038297876454, 51.04275706135231871 ) ) ;
#16243=CARTESIAN_POINT ( 'NONE',  ( 10.72451020669871369, 18.67979575497193778, 107.0844237280190043 ) ) ;
#16245=CARTESIAN_POINT ( 'NONE',  ( 0.05219959533936267826, -19.03943276465977164, 25.00109039468566152 ) ) ;
#16246=CARTESIAN_POINT ( 'NONE',  ( 5.049401038298161559, -19.05341960407611168, 22.70724293864769194 ) ) ;
#16247=CARTESIAN_POINT ( 'NONE',  ( -0.05219959533937732626, 21.53943276465977519, 92.50109039468567573 ) ) ;
#16248=CARTESIAN_POINT ( 'NONE',  ( -16.53943276465976808, -0.05219959533934237506, 33.75109039468568284 ) ) ;
#16249=CARTESIAN_POINT ( 'NONE',  ( -19.03943276465977164, 0.05219959533909376836, 96.24890960531436690 ) ) ;
#16251=CARTESIAN_POINT ( 'NONE',  ( -13.89961937509977652, 13.97604488694528158, 80.62390960531436690 ) ) ;
#16252=CARTESIAN_POINT ( 'NONE',  ( -18.09805431107523077, 5.499999999999980460, 96.01606229291888894 ) ) ;
#16253=CARTESIAN_POINT ( 'NONE',  ( -16.46253265017146816, -9.564922557961047289, 79.16775706135234714 ) ) ;
#16255=CARTESIAN_POINT ( 'NONE',  ( 5.153800228976335163, 19.02544592524342804, 109.7905762719810099 ) ) ;
#16256=CARTESIAN_POINT ( 'NONE',  ( -21.55341960407619339, 5.719274019375674811, 108.5427570613523756 ) ) ;
#16257=CARTESIAN_POINT ( 'NONE',  ( 8.224510206698953496, -14.34966873604960469, 92.91557627198103830 ) ) ;
#16259=CARTESIAN_POINT ( 'NONE',  ( -10.81492255796078084, -18.62759615963271287, 62.08224293864769550 ) ) ;
#16260=CARTESIAN_POINT ( 'NONE',  ( 0.05219959533907565091, 21.53943276465977519, 39.99890960531436690 ) ) ;
#16261=CARTESIAN_POINT ( 'NONE',  ( 13.89961937509977652, -13.97604488694527269, 23.12390960531436335 ) ) ;
#16263=CARTESIAN_POINT ( 'NONE',  ( 16.46253265017146816, 9.564922557961045513, 56.66775706135233293 ) ) ;
#16264=CARTESIAN_POINT ( 'NONE',  ( -16.55341960407611168, -4.379528057220339221, 41.45724293864769550 ) ) ;
#16265=CARTESIAN_POINT ( 'NONE',  ( 0.05219959533909260263, 19.03943276465977164, 109.9989096053143669 ) ) ;
#16266=CARTESIAN_POINT ( 'NONE',  ( 18.67979575497194134, -10.72451020669871369, 75.83442372801900433 ) ) ;
#16267=CARTESIAN_POINT ( 'NONE',  ( 18.62759615963271287, -10.81492255796078972, 73.33224293864769550 ) ) ;
#16268=CARTESIAN_POINT ( 'NONE',  ( -21.53943276465977519, -0.05219959533937600094, 58.75109039468568994 ) ) ;
#16269=CARTESIAN_POINT ( 'NONE',  ( 5.719274019375673035, 21.55341960407619339, 47.29275706135234003 ) ) ;
#16270=CARTESIAN_POINT ( 'NONE',  ( 5.153800228976335163, 19.02544592524342804, 84.79057627198099567 ) ) ;
#16271=CARTESIAN_POINT ( 'NONE',  ( 16.53943276465976808, 0.05219959533934440121, 76.25109039468568994 ) ) ;
#16272=CARTESIAN_POINT ( 'NONE',  ( -19.03943276465977164, 0.05219959533909376836, 26.24890960531435624 ) ) ;
#16274=CARTESIAN_POINT ( 'NONE',  ( 8.224510206698953496, -14.34966873604960469, 47.91557627198102409 ) ) ;
#16275=CARTESIAN_POINT ( 'NONE',  ( -16.55341960407617563, 4.379528057220093196, 108.5427570613523756 ) ) ;
#16276=CARTESIAN_POINT ( 'NONE',  ( 19.02544592524343514, -5.153800228976328945, 63.54057627198103830 ) ) ;
#16277=CARTESIAN_POINT ( 'NONE',  ( 13.89961937509977652, -13.97604488694527269, 38.12390960531436690 ) ) ;
#16278=CARTESIAN_POINT ( 'NONE',  ( 5.719274019375991003, -21.55341960407610458, 42.70724293864770260 ) ) ;
#16279=CARTESIAN_POINT ( 'NONE',  ( -19.02544592524334988, -5.153800228976617603, 38.95942372801900433 ) ) ;
#16280=CARTESIAN_POINT ( 'NONE',  ( -17.49999999999998934, -5.624438216177606975, 39.18329655085358354 ) ) ;
#16281=CARTESIAN_POINT ( 'NONE',  ( -4.379528057220328563, 16.55341960407611168, 50.20724293864769550 ) ) ;
#16282=CARTESIAN_POINT ( 'NONE',  ( -5.049401038298153566, 19.05341960407611168, 115.2072429386477097 ) ) ;
#16285=CARTESIAN_POINT ( 'NONE',  ( -4.483927247898782831, 16.52544592524335698, 72.70942372801901854 ) ) ;
#16287=CARTESIAN_POINT ( 'NONE',  ( 0.05219959533936267826, -19.03943276465977164, 70.00109039468566152 ) ) ;
#16288=CARTESIAN_POINT ( 'NONE',  ( 14.34966873604960469, 8.224510206698951720, 39.16557627198102409 ) ) ;
#16290=CARTESIAN_POINT ( 'NONE',  ( 8.314922557960818139, 14.29746914071049879, 24.58224293864768839 ) ) ;
#16291=CARTESIAN_POINT ( 'NONE',  ( -9.564922557960796823, -16.46253265017161027, 42.08224293864769550 ) ) ;
#16292=CARTESIAN_POINT ( 'NONE',  ( -0.05219959533909027116, -19.03943276465977164, 57.49890960531435979 ) ) ;
#16293=CARTESIAN_POINT ( 'NONE',  ( 5.153800228976335163, 19.02544592524342804, 24.79057627198102765 ) ) ;
#16294=CARTESIAN_POINT ( 'NONE',  ( -15.80617190586768217, 15.72974639402176855, 28.12609039468568284 ) ) ;
#16295=CARTESIAN_POINT ( 'NONE',  ( -16.46253265017160317, 9.564922557960807481, 55.83224293864769550 ) ) ;
#16297=CARTESIAN_POINT ( 'NONE',  ( 16.51473224551069308, 9.474510206698969483, 44.16557627198103120 ) ) ;
#16298=CARTESIAN_POINT ( 'NONE',  ( 5.719274019375991003, -21.55341960407610458, 32.70724293864770260 ) ) ;
#16299=CARTESIAN_POINT ( 'NONE',  ( -10.81492255796105439, 18.62759615963255655, 57.91775706135234714 ) ) ;
#16300=CARTESIAN_POINT ( 'NONE',  ( 5.049401038298161559, -19.05341960407611168, 27.70724293864769550 ) ) ;
#16301=CARTESIAN_POINT ( 'NONE',  ( -10.72451020669898014, 18.67979575497178502, 25.41557627198103120 ) ) ;
#16302=CARTESIAN_POINT ( 'NONE',  ( -16.53943276465976808, -0.05219959533934237506, 88.75109039468567573 ) ) ;
#16303=CARTESIAN_POINT ( 'NONE',  ( 5.719274019375673035, 21.55341960407619339, 102.2927570613523613 ) ) ;
#16304=CARTESIAN_POINT ( 'NONE',  ( -8.314922557961024197, 14.29746914071037800, 72.91775706135234714 ) ) ;
#16305=CARTESIAN_POINT ( 'NONE',  ( 16.46253265017160672, -9.564922557960803928, 113.3322429386476955 ) ) ;
#16306=CARTESIAN_POINT ( 'NONE',  ( 12.06949235617739724, 12.14591786802326823, 51.87609039468568284 ) ) ;
#16307=CARTESIAN_POINT ( 'NONE',  ( 4.483927247898790824, -16.52544592524335698, 40.20942372801901854 ) ) ;
#16308=CARTESIAN_POINT ( 'NONE',  ( 16.53943276465976808, 0.05219959533934440121, 91.25109039468568994 ) ) ;
#16309=CARTESIAN_POINT ( 'NONE',  ( -21.55341960407619339, 5.719274019375674811, 58.54275706135235424 ) ) ;
#16310=CARTESIAN_POINT ( 'NONE',  ( 4.483927247898790824, -16.52544592524335698, 25.20942372801901854 ) ) ;
#16311=CARTESIAN_POINT ( 'NONE',  ( 21.53943276465977519, -0.05219959533907433946, 108.7489096053143669 ) ) ;
#16312=CARTESIAN_POINT ( 'NONE',  ( -14.29746914071037622, -8.314922557961029526, 24.16775706135235424 ) ) ;
#16313=CARTESIAN_POINT ( 'NONE',  ( -4.379528057220086978, -16.55341960407618274, 89.79275706135236135 ) ) ;
#16314=CARTESIAN_POINT ( 'NONE',  ( 18.22780087662122384, -5.500000000000022204, 71.01540105326107266 ) ) ;
#16315=CARTESIAN_POINT ( 'NONE',  ( 15.72974639402176855, 15.80617190586768217, 86.87609039468568994 ) ) ;
#16316=CARTESIAN_POINT ( 'NONE',  ( 19.05341960407617918, -5.049401038297876454, 86.04275706135233293 ) ) ;
#16317=CARTESIAN_POINT ( 'NONE',  ( 14.34966873604960469, 8.224510206698951720, 64.16557627198102409 ) ) ;
#16318=CARTESIAN_POINT ( 'NONE',  ( -16.52544592524342804, 4.483927247898546575, 46.04057627198103830 ) ) ;
#16319=CARTESIAN_POINT ( 'NONE',  ( -8.224510206698948167, 14.34966873604960824, 105.4155762719810383 ) ) ;
#16320=CARTESIAN_POINT ( 'NONE',  ( 19.05341960407617918, -5.049401038297876454, 46.04275706135233293 ) ) ;
#16322=CARTESIAN_POINT ( 'NONE',  ( 15.80617190586769283, -15.72974639402175789, 50.62609039468568994 ) ) ;
#16323=CARTESIAN_POINT ( 'NONE',  ( 16.51473224551083163, -9.474510206698727899, 110.8344237280190043 ) ) ;
#16325=CARTESIAN_POINT ( 'NONE',  ( -16.46253265017160317, 9.564922557960807481, 105.8322429386476955 ) ) ;
#16326=CARTESIAN_POINT ( 'NONE',  ( -10.81492255796078084, -18.62759615963271287, 67.08224293864770971 ) ) ;
#16327=CARTESIAN_POINT ( 'NONE',  ( -13.97604488694547697, 13.89961937509957934, 93.12609039468566152 ) ) ;
#16328=CARTESIAN_POINT ( 'NONE',  ( 19.03943276465977164, -0.05219959533909143690, 108.7489096053143527 ) ) ;
#16329=CARTESIAN_POINT ( 'NONE',  ( -5.823673210054116645, -21.52544592524344225, 62.29057627198102409 ) ) ;
#16330=CARTESIAN_POINT ( 'NONE',  ( -14.34966873604960291, -8.224510206698953496, 101.6655762719810383 ) ) ;
#16331=CARTESIAN_POINT ( 'NONE',  ( -0.05219959533909027116, -19.03943276465977164, 67.49890960531436690 ) ) ;
#16332=CARTESIAN_POINT ( 'NONE',  ( -10.72451020669870658, -18.67979575497194134, 89.58442372801901854 ) ) ;
#16333=CARTESIAN_POINT ( 'NONE',  ( -5.153800228976328057, -19.02544592524343514, 32.29057627198102409 ) ) ;
#16334=CARTESIAN_POINT ( 'NONE',  ( 15.72974639402176855, 15.80617190586768217, 41.87609039468568284 ) ) ;
#16335=CARTESIAN_POINT ( 'NONE',  ( 5.719274019375673035, 21.55341960407619339, 87.29275706135236135 ) ) ;
#16336=CARTESIAN_POINT ( 'NONE',  ( 4.379528057220092307, 16.55341960407617563, 87.29275706135236135 ) ) ;
#16337=CARTESIAN_POINT ( 'NONE',  ( 0.05219959533937995610, -21.53943276465977519, 25.00109039468567218 ) ) ;
#16338=CARTESIAN_POINT ( 'NONE',  ( 21.55341960407619695, -5.719274019375665929, 46.04275706135234714 ) ) ;
#16339=CARTESIAN_POINT ( 'NONE',  ( 19.02544592524334988, 5.153800228976608722, 61.45942372801900433 ) ) ;
#16340=CARTESIAN_POINT ( 'NONE',  ( 19.05341960407611168, 5.049401038298154454, 83.95724293864766707 ) ) ;
#16341=CARTESIAN_POINT ( 'NONE',  ( -18.67979575497193778, 10.72451020669871902, 88.33442372801901854 ) ) ;
#16342=CARTESIAN_POINT ( 'NONE',  ( -21.52544592524343514, 5.823673210054127303, 86.04057627198102409 ) ) ;
#16343=CARTESIAN_POINT ( 'NONE',  ( 8.224510206698953496, -14.34966873604960469, 57.91557627198103120 ) ) ;
#16344=CARTESIAN_POINT ( 'NONE',  ( 21.53943276465977519, 0.05219959533937863772, 106.2510903946856757 ) ) ;
#16345=CARTESIAN_POINT ( 'NONE',  ( -14.29746914071049879, 8.314922557960819915, 80.83224293864769550 ) ) ;
#16346=CARTESIAN_POINT ( 'NONE',  ( 13.97604488694527802, 13.89961937509977652, 34.37390960531436690 ) ) ;
#16347=CARTESIAN_POINT ( 'NONE',  ( 19.05341960407617918, -5.049401038297876454, 71.04275706135234714 ) ) ;
#16349=CARTESIAN_POINT ( 'NONE',  ( 16.52544592524342804, -4.483927247898539470, 38.54057627198103120 ) ) ;
#16350=CARTESIAN_POINT ( 'NONE',  ( -18.62759615963255300, -10.81492255796106328, 94.16775706135237556 ) ) ;
#16351=CARTESIAN_POINT ( 'NONE',  ( 9.474510206698971260, -16.51473224551069308, 92.91557627198103830 ) ) ;
#16352=CARTESIAN_POINT ( 'NONE',  ( 0.05219959533936267826, -19.03943276465977164, 65.00109039468567573 ) ) ;
#16353=CARTESIAN_POINT ( 'NONE',  ( 10.72451020669898902, -18.67979575497178502, 62.91557627198102409 ) ) ;
#16354=CARTESIAN_POINT ( 'NONE',  ( -18.62759615963270932, 10.81492255796079327, 115.8322429386477097 ) ) ;
#16355=CARTESIAN_POINT ( 'NONE',  ( 5.049401038297881783, 19.05341960407617563, 107.2927570613523187 ) ) ;
#16356=CARTESIAN_POINT ( 'NONE',  ( 4.379528057220092307, 16.55341960407617563, 77.29275706135234714 ) ) ;
#16358=CARTESIAN_POINT ( 'NONE',  ( 18.62759615963255655, 10.81492255796105972, 21.66775706135235069 ) ) ;
#16359=CARTESIAN_POINT ( 'NONE',  ( -16.55341960407611168, -4.379528057220339221, 106.4572429386477097 ) ) ;
#16361=CARTESIAN_POINT ( 'NONE',  ( 4.379528057220092307, 16.55341960407617563, 47.29275706135234003 ) ) ;
#16362=CARTESIAN_POINT ( 'NONE',  ( 5.719274019375991003, -21.55341960407610458, 57.70724293864770260 ) ) ;
#16363=CARTESIAN_POINT ( 'NONE',  ( 16.53943276465976808, 0.05219959533934440121, 106.2510903946856757 ) ) ;
#16364=CARTESIAN_POINT ( 'NONE',  ( 16.52544592524335698, 4.483927247898782831, 41.45942372801901143 ) ) ;
#16365=CARTESIAN_POINT ( 'NONE',  ( 5.153800228976335163, 19.02544592524342804, 44.79057627198103830 ) ) ;
#16366=CARTESIAN_POINT ( 'NONE',  ( -16.55341960407617563, 4.379528057220093196, 73.54275706135234714 ) ) ;
#16367=CARTESIAN_POINT ( 'NONE',  ( 5.049401038297881783, 19.05341960407617563, 67.29275706135234714 ) ) ;
#16368=CARTESIAN_POINT ( 'NONE',  ( 10.81492255796078972, 18.62759615963270932, 69.58224293864769550 ) ) ;
#16369=CARTESIAN_POINT ( 'NONE',  ( 8.314922557961029526, -14.29746914071037800, 95.41775706135234714 ) ) ;
#16370=CARTESIAN_POINT ( 'NONE',  ( 5.823673210054444382, -21.52544592524334988, 80.20942372801901854 ) ) ;
#16371=CARTESIAN_POINT ( 'NONE',  ( 5.719274019375991003, -21.55341960407610458, 72.70724293864769550 ) ) ;
#16372=CARTESIAN_POINT ( 'NONE',  ( -18.62759615963270932, 10.81492255796079327, 50.83224293864770971 ) ) ;
#16374=ORIENTED_EDGE ( 'NONE', *, *, #190638, .T. ) ;
#16375=CARTESIAN_POINT ( 'NONE',  ( -12.14591786802326823, 12.06949235617739902, 73.12609039468567573 ) ) ;
#16376=CARTESIAN_POINT ( 'NONE',  ( 15.80617190586746368, 15.72974639402197994, 44.37390960531435979 ) ) ;
#16378=CARTESIAN_POINT ( 'NONE',  ( 15.72974639402199770, -15.80617190586745480, 23.12390960531436335 ) ) ;
#16380=CARTESIAN_POINT ( 'NONE',  ( 0.05219959533909260263, 19.03943276465977164, 24.99890960531435269 ) ) ;
#16381=CARTESIAN_POINT ( 'NONE',  ( -15.72974639402197994, 15.80617190586746368, 80.62390960531438111 ) ) ;
#16382=CARTESIAN_POINT ( 'NONE',  ( 4.483927247898790824, -16.52544592524335698, 105.2094237280190328 ) ) ;
#16383=CARTESIAN_POINT ( 'NONE',  ( -15.80617190586768217, 15.72974639402176855, 53.12609039468568284 ) ) ;
#16384=CARTESIAN_POINT ( 'NONE',  ( 16.51473224551083163, -9.474510206698727899, 110.8344237280190043 ) ) ;
#16385=CARTESIAN_POINT ( 'NONE',  ( 19.02544592524343514, -5.153800228976328945, 23.54057627198102054 ) ) ;
#16386=CARTESIAN_POINT ( 'NONE',  ( -8.224510206698735004, -14.34966873604973081, 19.58442372801901143 ) ) ;
#16387=CARTESIAN_POINT ( 'NONE',  ( -0.05219959533909027116, -19.03943276465977164, 42.49890960531435269 ) ) ;
#16389=CARTESIAN_POINT ( 'NONE',  ( -13.89961937509977652, 13.97604488694528158, 85.62390960531433848 ) ) ;
#16390=CARTESIAN_POINT ( 'NONE',  ( 14.34966873604972726, -8.224510206698740333, 95.83442372801903275 ) ) ;
#16391=CARTESIAN_POINT ( 'NONE',  ( 0.05219959533936267826, -19.03943276465977164, 75.00109039468566152 ) ) ;
#16392=CARTESIAN_POINT ( 'NONE',  ( -0.05219959533936034679, 19.03943276465977164, 27.50109039468566507 ) ) ;
#16393=CARTESIAN_POINT ( 'NONE',  ( -10.72451020669898014, 18.67979575497178502, 55.41557627198102409 ) ) ;
#16395=CARTESIAN_POINT ( 'NONE',  ( 12.06949235617739724, 12.14591786802326823, 91.87609039468568994 ) ) ;
#16396=CARTESIAN_POINT ( 'NONE',  ( -19.03943276465977164, -0.05219959533935918106, 83.75109039468567573 ) ) ;
#16397=CARTESIAN_POINT ( 'NONE',  ( -5.049401038298153566, 19.05341960407611168, 40.20724293864768839 ) ) ;
#16398=CARTESIAN_POINT ( 'NONE',  ( -9.474510206698964154, 16.51473224551069663, 85.41557627198102409 ) ) ;
#16399=CARTESIAN_POINT ( 'NONE',  ( 15.72974639402176855, 15.80617190586768217, 46.87609039468568994 ) ) ;
#16400=CARTESIAN_POINT ( 'NONE',  ( -19.02544592524342804, 5.153800228976336051, 51.04057627198103120 ) ) ;
#16402=CARTESIAN_POINT ( 'NONE',  ( -16.46253265017160317, 9.564922557960807481, 110.8322429386476955 ) ) ;
#16403=CARTESIAN_POINT ( 'NONE',  ( 16.52544592524342804, -4.483927247898539470, 63.54057627198103830 ) ) ;
#16404=CARTESIAN_POINT ( 'NONE',  ( -21.55341960407610458, -5.719274019375992779, 61.45724293864770260 ) ) ;
#16406=CARTESIAN_POINT ( 'NONE',  ( -5.153800228976607833, 19.02544592524334988, 42.70942372801901143 ) ) ;
#16407=CARTESIAN_POINT ( 'NONE',  ( 5.153800228976335163, 19.02544592524342804, 59.79057627198100988 ) ) ;
#16408=CARTESIAN_POINT ( 'NONE',  ( 19.02544592524343514, -5.153800228976328945, 73.54057627198103830 ) ) ;
#16409=CARTESIAN_POINT ( 'NONE',  ( 14.29746914071037800, 8.314922557961029526, 56.66775706135235424 ) ) ;
#16410=CARTESIAN_POINT ( 'NONE',  ( 9.564922557961047289, -16.46253265017146816, 80.41775706135234714 ) ) ;
#16412=CARTESIAN_POINT ( 'NONE',  ( 0.05219959533934541429, -16.53943276465976808, 90.00109039468567573 ) ) ;
#16414=CARTESIAN_POINT ( 'NONE',  ( -12.06949235617739369, -12.14591786802326823, 79.37609039468567573 ) ) ;
#16415=CARTESIAN_POINT ( 'NONE',  ( 12.06949235617739724, 12.14591786802326823, 56.87609039468568994 ) ) ;
#16416=CARTESIAN_POINT ( 'NONE',  ( -5.153800228976607833, 19.02544592524334988, 27.70942372801899722 ) ) ;
#16417=CARTESIAN_POINT ( 'NONE',  ( 16.51473224551069308, 9.474510206698969483, 49.16557627198102409 ) ) ;
#16419=CARTESIAN_POINT ( 'NONE',  ( -18.62759615963255300, -10.81492255796106328, 59.16775706135234714 ) ) ;
#16420=CARTESIAN_POINT ( 'NONE',  ( -9.474510206698720793, -16.51473224551083518, 59.58442372801900433 ) ) ;
#16421=CARTESIAN_POINT ( 'NONE',  ( 21.52544592524334988, 5.823673210054432836, 106.4594237280190328 ) ) ;
#16422=CARTESIAN_POINT ( 'NONE',  ( -16.46253265017160317, 9.564922557960807481, 25.83224293864769194 ) ) ;
#16424=CARTESIAN_POINT ( 'NONE',  ( 5.719274019375991003, -21.55341960407610458, 72.70724293864769550 ) ) ;
#16425=CARTESIAN_POINT ( 'NONE',  ( -18.67979575497178146, -10.72451020669898902, 26.66557627198103475 ) ) ;
#16426=CARTESIAN_POINT ( 'NONE',  ( 5.049401038298161559, -19.05341960407611168, 22.70724293864769194 ) ) ;
#16427=CARTESIAN_POINT ( 'NONE',  ( 8.224510206698742110, 14.34966873604972548, 32.08442372801901854 ) ) ;
#16428=CARTESIAN_POINT ( 'NONE',  ( 16.52544592524342804, -4.483927247898539470, 23.54057627198102765 ) ) ;
#16429=ORIENTED_EDGE ( 'NONE', *, *, #13540, .T. ) ;
#16430=CARTESIAN_POINT ( 'NONE',  ( 0.05219959533937995610, -21.53943276465977519, 20.00109039468568639 ) ) ;
#16431=CARTESIAN_POINT ( 'NONE',  ( -12.06949235617756955, 12.14591786802309770, 40.62390960531435269 ) ) ;
#16433=CARTESIAN_POINT ( 'NONE',  ( 13.89961937509957401, 13.97604488694547697, 111.8760903946856757 ) ) ;
#16434=CARTESIAN_POINT ( 'NONE',  ( 16.46253265017146816, 9.564922557961045513, 31.66775706135232937 ) ) ;
#16435=CARTESIAN_POINT ( 'NONE',  ( -0.05219959533910754901, -16.53943276465976808, 47.49890960531435979 ) ) ;
#16436=CARTESIAN_POINT ( 'NONE',  ( -18.62759615963270932, 10.81492255796079327, 105.8322429386476955 ) ) ;
#16437=CARTESIAN_POINT ( 'NONE',  ( 16.61371651742603817, 7.165104196376044676, 33.64584930007004004 ) ) ;
#16438=CARTESIAN_POINT ( 'NONE',  ( -21.55341960407610458, -5.719274019375992779, 66.45724293864768129 ) ) ;
#16439=CARTESIAN_POINT ( 'NONE',  ( -16.46253265017160317, 9.564922557960807481, 70.83224293864770971 ) ) ;
#16440=CARTESIAN_POINT ( 'NONE',  ( -8.224510206698948167, 14.34966873604960824, 45.41557627198103830 ) ) ;
#16441=CARTESIAN_POINT ( 'NONE',  ( 5.153800228976335163, 19.02544592524342804, 89.79057627198102409 ) ) ;
#16443=CARTESIAN_POINT ( 'NONE',  ( 19.03943276465977164, 0.05219959533936151252, 51.25109039468567573 ) ) ;
#16444=CARTESIAN_POINT ( 'NONE',  ( 15.72974639402199770, -15.80617190586745480, 98.12390960531436690 ) ) ;
#16445=CARTESIAN_POINT ( 'NONE',  ( 14.29746914071049879, -8.314922557960816363, 103.3322429386476955 ) ) ;
#16446=CARTESIAN_POINT ( 'NONE',  ( 0.05219959533937995610, -21.53943276465977519, 45.00109039468568284 ) ) ;
#16448=CARTESIAN_POINT ( 'NONE',  ( 16.52544592524342804, -4.483927247898539470, 28.54057627198103120 ) ) ;
#16449=CARTESIAN_POINT ( 'NONE',  ( -5.153800228976328057, -19.02544592524343514, 37.29057627198102409 ) ) ;
#16450=CARTESIAN_POINT ( 'NONE',  ( 13.97604488694527802, 13.89961937509977652, 104.3739096053143385 ) ) ;
#16451=CARTESIAN_POINT ( 'NONE',  ( 10.81492255796078972, 18.62759615963270932, 64.58224293864769550 ) ) ;
#16453=CARTESIAN_POINT ( 'NONE',  ( 16.46253265017160672, -9.564922557960803928, 28.33224293864769550 ) ) ;
#16454=CARTESIAN_POINT ( 'NONE',  ( -5.823673210054116645, -21.52544592524344225, 52.29057627198102409 ) ) ;
#16455=CARTESIAN_POINT ( 'NONE',  ( -5.823673210054431948, 21.52544592524334988, 77.70942372801900433 ) ) ;
#16457=CARTESIAN_POINT ( 'NONE',  ( -16.52544592524335698, -4.483927247898792601, 88.95942372801901854 ) ) ;
#16458=CARTESIAN_POINT ( 'NONE',  ( -13.97604488694527625, -13.89961937509977652, 56.87390960531434558 ) ) ;
#16459=CARTESIAN_POINT ( 'NONE',  ( 16.46253265017160672, -9.564922557960803928, 63.33224293864769550 ) ) ;
#16460=ORIENTED_EDGE ( 'NONE', *, *, #83608, .T. ) ;
#16461=CARTESIAN_POINT ( 'NONE',  ( -0.05219959533936034679, 19.03943276465977164, 22.50109039468566152 ) ) ;
#16462=CARTESIAN_POINT ( 'NONE',  ( -16.52544592524335698, -4.483927247898792601, 73.95942372801901854 ) ) ;
#16463=CARTESIAN_POINT ( 'NONE',  ( 21.52544592524334988, 5.823673210054432836, 96.45942372801901854 ) ) ;
#16464=CARTESIAN_POINT ( 'NONE',  ( -5.049401038298153566, 19.05341960407611168, 80.20724293864769550 ) ) ;
#16465=CARTESIAN_POINT ( 'NONE',  ( -18.62759615963270932, 10.81492255796079327, 30.83224293864770260 ) ) ;
#16466=CARTESIAN_POINT ( 'NONE',  ( -0.05219959533936034679, 19.03943276465977164, 112.5010903946856757 ) ) ;
#16467=CARTESIAN_POINT ( 'NONE',  ( -10.81492255796105439, 18.62759615963255655, 87.91775706135234714 ) ) ;
#16468=CARTESIAN_POINT ( 'NONE',  ( -14.34966873604972548, 8.224510206698743886, 53.33442372801901854 ) ) ;
#16469=CARTESIAN_POINT ( 'NONE',  ( 0.05219959533907565091, 21.53943276465977519, 94.99890960531436690 ) ) ;
#16470=CARTESIAN_POINT ( 'NONE',  ( -8.314922557961024197, 14.29746914071037800, 22.91775706135235069 ) ) ;
#16471=CARTESIAN_POINT ( 'NONE',  ( 5.049401038298161559, -19.05341960407611168, 72.70724293864768129 ) ) ;
#16472=CARTESIAN_POINT ( 'NONE',  ( -4.379528057220086978, -16.55341960407618274, 24.79275706135235779 ) ) ;
#16473=CARTESIAN_POINT ( 'NONE',  ( -19.05341960407611168, -5.049401038298163336, 36.45724293864766707 ) ) ;
#16474=CARTESIAN_POINT ( 'NONE',  ( 0.05219959533936267826, -19.03943276465977164, 110.0010903946856757 ) ) ;
#16475=CARTESIAN_POINT ( 'NONE',  ( 14.29746914071049879, -8.314922557960816363, 68.33224293864769550 ) ) ;
#16476=CARTESIAN_POINT ( 'NONE',  ( 4.483927247898790824, -16.52544592524335698, 80.20942372801901854 ) ) ;
#16477=CARTESIAN_POINT ( 'NONE',  ( -0.05219959533937732626, 21.53943276465977519, 27.50109039468567929 ) ) ;
#16478=CARTESIAN_POINT ( 'NONE',  ( -13.89961937509977652, 13.97604488694528158, 55.62390960531434558 ) ) ;
#16479=CARTESIAN_POINT ( 'NONE',  ( -9.564922557960796823, -16.46253265017161027, 72.08224293864770971 ) ) ;
#16481=CARTESIAN_POINT ( 'NONE',  ( 14.29746914071037800, 8.314922557961029526, 71.66775706135234714 ) ) ;
#16485=CARTESIAN_POINT ( 'NONE',  ( 9.474510206698729675, 16.51473224551082808, 22.08442372801899722 ) ) ;
#16486=CARTESIAN_POINT ( 'NONE',  ( -13.97604488694527625, -13.89961937509977652, 36.87390960531436690 ) ) ;
#16489=CARTESIAN_POINT ( 'NONE',  ( -12.14591786802326823, 12.06949235617739902, 28.12609039468568284 ) ) ;
#16490=CARTESIAN_POINT ( 'NONE',  ( 19.02544592524334988, 5.153800228976608722, 61.45942372801900433 ) ) ;
#16491=CARTESIAN_POINT ( 'NONE',  ( -12.06949235617739369, -12.14591786802326823, 44.37609039468567573 ) ) ;
#16492=CARTESIAN_POINT ( 'NONE',  ( 5.153800228976335163, 19.02544592524342804, 44.79057627198103830 ) ) ;
#16493=CARTESIAN_POINT ( 'NONE',  ( -5.153800228976328057, -19.02544592524343514, 102.2905762719810383 ) ) ;
#16494=CARTESIAN_POINT ( 'NONE',  ( -9.564922557960796823, -16.46253265017161027, 67.08224293864769550 ) ) ;
#16495=CARTESIAN_POINT ( 'NONE',  ( -10.72451020669898014, 18.67979575497178502, 95.41557627198102409 ) ) ;
#16496=CARTESIAN_POINT ( 'NONE',  ( -16.51473224551069308, -9.474510206698971260, 96.66557627198102409 ) ) ;
#16499=CARTESIAN_POINT ( 'NONE',  ( 19.03943276465977164, -0.05219959533909143690, 63.74890960531435979 ) ) ;
#16500=CARTESIAN_POINT ( 'NONE',  ( 12.14591786802309770, 12.06949235617756955, 24.37390960531435979 ) ) ;
#16502=CARTESIAN_POINT ( 'NONE',  ( -19.02544592524334988, -5.153800228976617603, 98.95942372801900433 ) ) ;
#16503=CARTESIAN_POINT ( 'NONE',  ( 19.02544592524334988, 5.153800228976608722, 26.45942372801899722 ) ) ;
#16504=CARTESIAN_POINT ( 'NONE',  ( -0.05219959533910754901, -16.53943276465976808, 67.49890960531436690 ) ) ;
#16505=CARTESIAN_POINT ( 'NONE',  ( 10.72451020669871369, 18.67979575497193778, 102.0844237280190185 ) ) ;
#16506=CARTESIAN_POINT ( 'NONE',  ( 0.05219959533909260263, 19.03943276465977164, 34.99890960531435979 ) ) ;
#16507=CARTESIAN_POINT ( 'NONE',  ( -16.53943276465976808, 0.05219959533911058130, 31.24890960531435979 ) ) ;
#16508=CARTESIAN_POINT ( 'NONE',  ( -10.72451020669870658, -18.67979575497194134, 94.58442372801901854 ) ) ;
#16509=CARTESIAN_POINT ( 'NONE',  ( -13.97604488694527625, -13.89961937509977652, 76.87390960531433848 ) ) ;
#16510=CARTESIAN_POINT ( 'NONE',  ( 9.474510206698971260, -16.51473224551069308, 97.91557627198102409 ) ) ;
#16511=CARTESIAN_POINT ( 'NONE',  ( -4.379528057220328563, 16.55341960407611168, 110.2072429386477239 ) ) ;
#16512=CARTESIAN_POINT ( 'NONE',  ( 16.53943276465976808, -0.05219959533910856209, 78.74890960531436690 ) ) ;
#16513=CARTESIAN_POINT ( 'NONE',  ( -18.67979575497178146, -10.72451020669898902, 86.66557627198102409 ) ) ;
#16514=CARTESIAN_POINT ( 'NONE',  ( -16.46253265017160317, 9.564922557960807481, 80.83224293864769550 ) ) ;
#16515=CARTESIAN_POINT ( 'NONE',  ( -21.52544592524343514, 5.823673210054127303, 81.04057627198102409 ) ) ;
#16516=CARTESIAN_POINT ( 'NONE',  ( 16.51473224551083163, -9.474510206698727899, 75.83442372801900433 ) ) ;
#16518=CARTESIAN_POINT ( 'NONE',  ( -0.05219959533910754901, -16.53943276465976808, 92.49890960531436690 ) ) ;
#16519=CARTESIAN_POINT ( 'NONE',  ( -16.46253265017160317, 9.564922557960807481, 55.83224293864769550 ) ) ;
#16520=CARTESIAN_POINT ( 'NONE',  ( 15.72974639402199770, -15.80617190586745480, 73.12390960531436690 ) ) ;
#16522=CARTESIAN_POINT ( 'NONE',  ( -14.29746914071037622, -8.314922557961029526, 109.1677570613523613 ) ) ;
#16524=CARTESIAN_POINT ( 'NONE',  ( -16.55341960407617563, 4.379528057220093196, 23.54275706135235424 ) ) ;
#16525=CARTESIAN_POINT ( 'NONE',  ( 14.34966873604960469, 8.224510206698951720, 79.16557627198103830 ) ) ;
#16527=CARTESIAN_POINT ( 'NONE',  ( -19.03943276465977164, 0.05219959533909376836, 71.24890960531435269 ) ) ;
#16528=CARTESIAN_POINT ( 'NONE',  ( -5.153800228976328057, -19.02544592524343514, 27.29057627198103120 ) ) ;
#16529=CARTESIAN_POINT ( 'NONE',  ( -4.483927247898539470, -16.52544592524342804, 72.29057627198102409 ) ) ;
#16530=CARTESIAN_POINT ( 'NONE',  ( -19.05341960407611168, -5.049401038298163336, 106.4572429386476955 ) ) ;
#16531=CARTESIAN_POINT ( 'NONE',  ( -16.51473224551082808, 9.474510206698731452, 88.33442372801900433 ) ) ;
#16532=CARTESIAN_POINT ( 'NONE',  ( -9.474510206698964154, 16.51473224551069663, 80.41557627198103830 ) ) ;
#16533=CARTESIAN_POINT ( 'NONE',  ( 13.97604488694527802, 13.89961937509977652, 89.37390960531436690 ) ) ;
#16534=CARTESIAN_POINT ( 'NONE',  ( -21.55341960407610458, -5.719274019375992779, 81.45724293864769550 ) ) ;
#16535=CARTESIAN_POINT ( 'NONE',  ( 16.55341960407618274, -4.379528057220086978, 71.04275706135234714 ) ) ;
#16536=CARTESIAN_POINT ( 'NONE',  ( 19.05341960407618274, -5.049401038297876454, 111.0427570613523329 ) ) ;
#16537=CARTESIAN_POINT ( 'NONE',  ( -16.46253265017160317, 9.564922557960807481, 65.83224293864769550 ) ) ;
#16538=CARTESIAN_POINT ( 'NONE',  ( -18.67979575497178146, -10.72451020669898902, 66.66557627198102409 ) ) ;
#16539=CARTESIAN_POINT ( 'NONE',  ( -13.97604488694547697, 13.89961937509957934, 93.12609039468566152 ) ) ;
#16540=CARTESIAN_POINT ( 'NONE',  ( -0.05219959533910754901, -16.53943276465976808, 32.49890960531435979 ) ) ;
#16541=CARTESIAN_POINT ( 'NONE',  ( 5.823673210054444382, -21.52544592524334988, 40.20942372801901854 ) ) ;
#16543=CARTESIAN_POINT ( 'NONE',  ( -14.29746914071037622, -8.314922557961029526, 79.16775706135234714 ) ) ;
#16544=CARTESIAN_POINT ( 'NONE',  ( -5.049401038298153566, 19.05341960407611168, 105.2072429386476671 ) ) ;
#16546=DIRECTION ( 'NONE',  ( -0.000000000000000000, -0.000000000000000000, 1.000000000000000000 ) ) ;
#16547=CARTESIAN_POINT ( 'NONE',  ( -8.224510206698735004, -14.34966873604973081, 89.58442372801901854 ) ) ;
#16548=CARTESIAN_POINT ( 'NONE',  ( -16.55341960407617563, 4.379528057220093196, 43.54275706135235424 ) ) ;
#16549=CARTESIAN_POINT ( 'NONE',  ( -5.153800228976328057, -19.02544592524343514, 62.29057627198100988 ) ) ;
#16550=CARTESIAN_POINT ( 'NONE',  ( 19.03943276465977164, -0.05219959533909143690, 78.74890960531436690 ) ) ;
#16551=CARTESIAN_POINT ( 'NONE',  ( -5.719274019375665041, -21.55341960407619695, 49.79275706135234714 ) ) ;
#16552=CARTESIAN_POINT ( 'NONE',  ( 12.14591786802327356, -12.06949235617739191, 60.62609039468567573 ) ) ;
#16553=CARTESIAN_POINT ( 'NONE',  ( -16.55341960407611168, -4.379528057220339221, 36.45724293864768839 ) ) ;
#16554=CARTESIAN_POINT ( 'NONE',  ( -5.153800228976328057, -19.02544592524343514, 37.29057627198102409 ) ) ;
#16555=CARTESIAN_POINT ( 'NONE',  ( -13.89961937509977652, 13.97604488694528158, 30.62390960531435269 ) ) ;
#16556=CARTESIAN_POINT ( 'NONE',  ( -4.379528057220086978, -16.55341960407618274, 24.79275706135235779 ) ) ;
#16557=CARTESIAN_POINT ( 'NONE',  ( -5.153800228976607833, 19.02544592524334988, 77.70942372801900433 ) ) ;
#16558=CARTESIAN_POINT ( 'NONE',  ( -8.224510206698948167, 14.34966873604960824, 85.41557627198102409 ) ) ;
#16559=CARTESIAN_POINT ( 'NONE',  ( -5.049401038298153566, 19.05341960407611168, 45.20724293864769550 ) ) ;
#16560=CARTESIAN_POINT ( 'NONE',  ( 5.153800228976615827, -19.02544592524334988, 90.20942372801900433 ) ) ;
#16561=CARTESIAN_POINT ( 'NONE',  ( 15.50000000000000178, 0.000000000000000000, 120.0000000000000142 ) ) ;
#16562=CARTESIAN_POINT ( 'NONE',  ( -5.823673210054431948, 21.52544592524334988, 87.70942372801901854 ) ) ;
#16563=CARTESIAN_POINT ( 'NONE',  ( -8.224510206698735004, -14.34966873604973081, 59.58442372801901854 ) ) ;
#16564=CARTESIAN_POINT ( 'NONE',  ( -17.49999999999998224, 3.237210098469581521, 24.71236987379559835 ) ) ;
#16565=CARTESIAN_POINT ( 'NONE',  ( 10.72451020669898902, -18.67979575497178502, 52.91557627198103830 ) ) ;
#16566=CARTESIAN_POINT ( 'NONE',  ( 16.52544592524335698, 4.483927247898782831, 41.45942372801901143 ) ) ;
#16567=FACE_OUTER_BOUND ( 'NONE', #110708, .T. ) ;
#16568=CARTESIAN_POINT ( 'NONE',  ( -19.05341960407617563, 5.049401038297882671, 33.54275706135231871 ) ) ;
#16569=CARTESIAN_POINT ( 'NONE',  ( -16.51473224551069308, -9.474510206698971260, 76.66557627198103830 ) ) ;
#16570=CARTESIAN_POINT ( 'NONE',  ( -9.474510206698964154, 16.51473224551069663, 45.41557627198103120 ) ) ;
#16572=CARTESIAN_POINT ( 'NONE',  ( 5.153800228976335163, 19.02544592524342804, 74.79057627198103830 ) ) ;
#16573=CARTESIAN_POINT ( 'NONE',  ( -19.35633801406907040, 5.499999999999674927, 99.13373818172765084 ) ) ;
#16574=CARTESIAN_POINT ( 'NONE',  ( -16.46253265017146816, -9.564922557961047289, 34.16775706135233293 ) ) ;
#16575=CARTESIAN_POINT ( 'NONE',  ( -21.52544592524334988, -5.823673210054445271, 103.9594237280190185 ) ) ;
#16576=CARTESIAN_POINT ( 'NONE',  ( -8.224510206698948167, 14.34966873604960824, 40.41557627198103120 ) ) ;
#16577=CARTESIAN_POINT ( 'NONE',  ( -16.51473224551069308, -9.474510206698971260, 36.66557627198102409 ) ) ;
#16578=CARTESIAN_POINT ( 'NONE',  ( 5.153800228976335163, 19.02544592524342804, 109.7905762719810099 ) ) ;
#16579=CARTESIAN_POINT ( 'NONE',  ( -10.81492255796105439, 18.62759615963255655, 87.91775706135234714 ) ) ;
#16580=CARTESIAN_POINT ( 'NONE',  ( -19.02544592524342804, 5.153800228976336051, 56.04057627198100988 ) ) ;
#16581=CARTESIAN_POINT ( 'NONE',  ( 18.67979575497194134, -10.72451020669871369, 75.83442372801900433 ) ) ;
#16582=CARTESIAN_POINT ( 'NONE',  ( 19.02544592524343514, -5.153800228976328945, 113.5405762719810241 ) ) ;
#16583=CARTESIAN_POINT ( 'NONE',  ( -15.80617190586768217, 15.72974639402176855, 28.12609039468568284 ) ) ;
#16584=CARTESIAN_POINT ( 'NONE',  ( -5.153800228976607833, 19.02544592524334988, 47.70942372801900433 ) ) ;
#16585=CARTESIAN_POINT ( 'NONE',  ( -5.049401038298153566, 19.05341960407611168, 35.20724293864768839 ) ) ;
#16586=CARTESIAN_POINT ( 'NONE',  ( -19.02544592524342804, 5.153800228976336051, 76.04057627198102409 ) ) ;
#16587=CARTESIAN_POINT ( 'NONE',  ( 16.46253265017146816, 9.564922557961045513, 111.6677570613523329 ) ) ;
#16588=CARTESIAN_POINT ( 'NONE',  ( 0.05219959533910956823, 16.53943276465976808, 69.99890960531435269 ) ) ;
#16589=CARTESIAN_POINT ( 'NONE',  ( 21.55341960407610458, 5.719274019375980345, 38.95724293864768839 ) ) ;
#16590=CARTESIAN_POINT ( 'NONE',  ( 5.153800228976615827, -19.02544592524334988, 95.20942372801897591 ) ) ;
#16591=CARTESIAN_POINT ( 'NONE',  ( 18.67979575497178502, 10.72451020669898547, 99.16557627198100988 ) ) ;
#16592=CARTESIAN_POINT ( 'NONE',  ( 18.67979575497194134, -10.72451020669871369, 50.83442372801901143 ) ) ;
#16593=CARTESIAN_POINT ( 'NONE',  ( -8.224510206698735004, -14.34966873604973081, 59.58442372801901854 ) ) ;
#16594=CARTESIAN_POINT ( 'NONE',  ( 0.05219959533934541429, -16.53943276465976808, 60.00109039468568284 ) ) ;
#16595=CARTESIAN_POINT ( 'NONE',  ( 13.89961937509977652, -13.97604488694527269, 53.12390960531434558 ) ) ;
#16596=CARTESIAN_POINT ( 'NONE',  ( 4.483927247898790824, -16.52544592524335698, 95.20942372801903275 ) ) ;
#16597=CARTESIAN_POINT ( 'NONE',  ( 21.53943276465977519, -0.05219959533907433946, 113.7489096053143527 ) ) ;
#16598=CARTESIAN_POINT ( 'NONE',  ( 16.53943276465976808, -0.05219959533910856209, 48.74890960531435979 ) ) ;
#16599=CARTESIAN_POINT ( 'NONE',  ( 5.049401038298161559, -19.05341960407611168, 87.70724293864769550 ) ) ;
#16600=CARTESIAN_POINT ( 'NONE',  ( -4.379528057220086978, -16.55341960407618274, 69.79275706135234714 ) ) ;
#16601=B_SPLINE_CURVE_WITH_KNOTS ( 'NONE', 3,
 ( #31144, #167671, #182845, #92792, #47311, #135358 ),
 .UNSPECIFIED., .F., .F.,
 ( 4, 2, 4 ),
 ( 0.000000000000000000, 0.0003837532665635264842, 0.0007675065331270529683 ),
 .UNSPECIFIED. ) ;
#16602=CARTESIAN_POINT ( 'NONE',  ( 10.72451020669871369, 18.67979575497193778, 57.08442372801901854 ) ) ;
#16603=CARTESIAN_POINT ( 'NONE',  ( 14.29746914071037800, 8.314922557961029526, 21.66775706135235069 ) ) ;
#16604=CARTESIAN_POINT ( 'NONE',  ( -15.80617190586745835, -15.72974639402198527, 106.8739096053143811 ) ) ;
#16605=CARTESIAN_POINT ( 'NONE',  ( -12.14591786802309592, -12.06949235617757132, 41.87390960531435979 ) ) ;
#16607=CARTESIAN_POINT ( 'NONE',  ( -17.50000000000000711, 5.622605283950874444, 68.68792689403892382 ) ) ;
#16608=CARTESIAN_POINT ( 'NONE',  ( -21.55341960407610458, -5.719274019375992779, 91.45724293864769550 ) ) ;
#16609=CARTESIAN_POINT ( 'NONE',  ( 4.379528057220339221, -16.55341960407611168, 22.70724293864769194 ) ) ;
#16612=CARTESIAN_POINT ( 'NONE',  ( 21.53943276465977519, -0.05219959533907433946, 113.7489096053143527 ) ) ;
#16613=CARTESIAN_POINT ( 'NONE',  ( 9.564922557960805705, 16.46253265017160317, 114.5822429386476955 ) ) ;
#16614=CARTESIAN_POINT ( 'NONE',  ( -10.81492255796105439, 18.62759615963255655, 22.91775706135235069 ) ) ;
#16615=CARTESIAN_POINT ( 'NONE',  ( 4.379528057220339221, -16.55341960407611168, 52.70724293864769550 ) ) ;
#16616=CARTESIAN_POINT ( 'NONE',  ( 4.379528057220092307, 16.55341960407617563, 67.29275706135234714 ) ) ;
#16617=CARTESIAN_POINT ( 'NONE',  ( 19.03943276465977164, -0.05219959533909143690, 63.74890960531435979 ) ) ;
#16618=CARTESIAN_POINT ( 'NONE',  ( -9.474510206698720793, -16.51473224551083518, 59.58442372801900433 ) ) ;
#16619=CARTESIAN_POINT ( 'NONE',  ( 9.564922557960805705, 16.46253265017160317, 74.58224293864769550 ) ) ;
#16620=CARTESIAN_POINT ( 'NONE',  ( -21.52544592524343514, 5.823673210054127303, 31.04057627198102409 ) ) ;
#16622=CARTESIAN_POINT ( 'NONE',  ( -13.89961937509977652, 13.97604488694528158, 60.62390960531436690 ) ) ;
#16623=CARTESIAN_POINT ( 'NONE',  ( -8.314922557961024197, 14.29746914071037800, 22.91775706135235069 ) ) ;
#16624=CARTESIAN_POINT ( 'NONE',  ( -13.97604488694547697, 13.89961937509957934, 68.12609039468563310 ) ) ;
#16625=CARTESIAN_POINT ( 'NONE',  ( -0.05219959533907301413, -21.53943276465977519, 102.4989096053143811 ) ) ;
#16627=CARTESIAN_POINT ( 'NONE',  ( 12.14591786802309770, 12.06949235617756955, 39.37390960531436690 ) ) ;
#16628=CARTESIAN_POINT ( 'NONE',  ( -13.97604488694527625, -13.89961937509977652, 96.87390960531433848 ) ) ;
#16629=CARTESIAN_POINT ( 'NONE',  ( 18.62759615963271287, -10.81492255796078972, 63.33224293864770260 ) ) ;
#16630=CARTESIAN_POINT ( 'NONE',  ( -5.719274019375978568, 21.55341960407610458, 95.20724293864769550 ) ) ;
#16631=CARTESIAN_POINT ( 'NONE',  ( 4.379528057220092307, 16.55341960407617563, 42.29275706135235424 ) ) ;
#16632=CARTESIAN_POINT ( 'NONE',  ( 10.72451020669898902, -18.67979575497178502, 32.91557627198102409 ) ) ;
#16633=CARTESIAN_POINT ( 'NONE',  ( -21.55341960407619339, 5.719274019375674811, 93.54275706135234714 ) ) ;
#16634=CARTESIAN_POINT ( 'NONE',  ( 5.153800228976335163, 19.02544592524342804, 84.79057627198099567 ) ) ;
#16635=CARTESIAN_POINT ( 'NONE',  ( -13.97604488694527625, -13.89961937509977652, 36.87390960531436690 ) ) ;
#16636=CARTESIAN_POINT ( 'NONE',  ( 9.564922557960805705, 16.46253265017160317, 84.58224293864769550 ) ) ;
#16637=CARTESIAN_POINT ( 'NONE',  ( -8.224510206698948167, 14.34966873604960824, 110.4155762719810383 ) ) ;
#16638=CARTESIAN_POINT ( 'NONE',  ( 13.89961937509977652, -13.97604488694527269, 63.12390960531435979 ) ) ;
#16639=CARTESIAN_POINT ( 'NONE',  ( -8.224510206698735004, -14.34966873604973081, 24.58442372801901499 ) ) ;
#16640=CARTESIAN_POINT ( 'NONE',  ( 17.50000000000001066, -5.622605283950831812, 86.18792689403892382 ) ) ;
#16641=CARTESIAN_POINT ( 'NONE',  ( 10.81492255796106328, -18.62759615963255655, 95.41775706135234714 ) ) ;
#16642=CARTESIAN_POINT ( 'NONE',  ( 13.97604488694527802, 13.89961937509977652, 114.3739096053143669 ) ) ;
#16643=CARTESIAN_POINT ( 'NONE',  ( -14.29746914071037622, -8.314922557961029526, 89.16775706135236135 ) ) ;
#16645=CARTESIAN_POINT ( 'NONE',  ( 19.03943276465977164, 0.05219959533936151252, 76.25109039468566152 ) ) ;
#16646=CARTESIAN_POINT ( 'NONE',  ( -19.02544592524334988, -5.153800228976617603, 28.95942372801900433 ) ) ;
#16647=CARTESIAN_POINT ( 'NONE',  ( 17.50000000000000000, 5.499999999999998224, 118.0000000000000142 ) ) ;
#16648=CARTESIAN_POINT ( 'NONE',  ( 0.05219959533909260263, 19.03943276465977164, 34.99890960531435979 ) ) ;
#16649=CARTESIAN_POINT ( 'NONE',  ( 4.379528057220339221, -16.55341960407611168, 37.70724293864769550 ) ) ;
#16650=CARTESIAN_POINT ( 'NONE',  ( -13.97604488694527625, -13.89961937509977652, 21.87390960531435979 ) ) ;
#16651=CARTESIAN_POINT ( 'NONE',  ( 16.55341960407611168, 4.379528057220329451, 28.95724293864769905 ) ) ;
#16653=CARTESIAN_POINT ( 'NONE',  ( -12.06949235617739369, -12.14591786802326823, 99.37609039468568994 ) ) ;
#16654=CARTESIAN_POINT ( 'NONE',  ( 13.89961937509977652, -13.97604488694527269, 43.12390960531434558 ) ) ;
#16655=CARTESIAN_POINT ( 'NONE',  ( 10.72451020669871369, 18.67979575497193778, 92.08442372801901854 ) ) ;
#16656=CARTESIAN_POINT ( 'NONE',  ( 19.02544592524334988, 5.153800228976608722, 111.4594237280190043 ) ) ;
#16657=CARTESIAN_POINT ( 'NONE',  ( -10.72451020669870658, -18.67979575497194134, 84.58442372801903275 ) ) ;
#16658=CARTESIAN_POINT ( 'NONE',  ( 9.474510206698729675, 16.51473224551082808, 47.08442372801900433 ) ) ;
#16659=CARTESIAN_POINT ( 'NONE',  ( 19.02544592524343514, -5.153800228976328945, 98.54057627198100988 ) ) ;
#16660=CARTESIAN_POINT ( 'NONE',  ( 19.03943276465977164, -0.05219959533909143690, 68.74890960531436690 ) ) ;
#16661=CARTESIAN_POINT ( 'NONE',  ( 17.50000000000000355, 5.622605283950890431, 73.81207310596110460 ) ) ;
#16662=CARTESIAN_POINT ( 'NONE',  ( -8.314922557960811034, -14.29746914071050412, 72.08224293864769550 ) ) ;
#16663=CARTESIAN_POINT ( 'NONE',  ( -18.67979575497178146, -10.72451020669898902, 66.66557627198102409 ) ) ;
#16664=CARTESIAN_POINT ( 'NONE',  ( 0.05219959533909260263, 19.03943276465977164, 64.99890960531436690 ) ) ;
#16665=CARTESIAN_POINT ( 'NONE',  ( 10.81492255796078972, 18.62759615963270932, 79.58224293864769550 ) ) ;
#16666=CARTESIAN_POINT ( 'NONE',  ( 14.34966873604972726, -8.224510206698740333, 75.83442372801900433 ) ) ;
#16668=CARTESIAN_POINT ( 'NONE',  ( -9.474510206698964154, 16.51473224551069663, 50.41557627198102409 ) ) ;
#16669=CARTESIAN_POINT ( 'NONE',  ( 0.05219959533910956823, 16.53943276465976808, 84.99890960531436690 ) ) ;
#16671=CARTESIAN_POINT ( 'NONE',  ( -19.02544592524342804, 5.153800228976336051, 56.04057627198100988 ) ) ;
#16672=CARTESIAN_POINT ( 'NONE',  ( 5.049401038298161559, -19.05341960407611168, 27.70724293864769550 ) ) ;
#16673=CARTESIAN_POINT ( 'NONE',  ( 9.564922557961047289, -16.46253265017146816, 65.41775706135233293 ) ) ;
#16674=CARTESIAN_POINT ( 'NONE',  ( 4.483927247898545687, 16.52544592524342804, 89.79057627198103830 ) ) ;
#16675=CARTESIAN_POINT ( 'NONE',  ( 18.62759615963255655, 10.81492255796105972, 41.66775706135235424 ) ) ;
#16676=CARTESIAN_POINT ( 'NONE',  ( 5.049401038298161559, -19.05341960407611168, 37.70724293864768839 ) ) ;
#16677=CARTESIAN_POINT ( 'NONE',  ( -5.719274019375978568, 21.55341960407610458, 110.2072429386477239 ) ) ;
#16678=CARTESIAN_POINT ( 'NONE',  ( 17.60691670004652565, 5.500000000000029310, 91.63333313366439370 ) ) ;
#16679=CARTESIAN_POINT ( 'NONE',  ( -16.52544592524342804, 4.483927247898546575, 91.04057627198103830 ) ) ;
#16681=CARTESIAN_POINT ( 'NONE',  ( -19.05341960407611168, -5.049401038298163336, 46.45724293864768129 ) ) ;
#16682=CARTESIAN_POINT ( 'NONE',  ( -5.049401038297874678, -19.05341960407617918, 89.79275706135230450 ) ) ;
#16683=CARTESIAN_POINT ( 'NONE',  ( -19.02544592524342804, 5.153800228976336051, 101.0405762719810241 ) ) ;
#16684=CARTESIAN_POINT ( 'NONE',  ( 5.823673210054444382, -21.52544592524334988, 35.20942372801901854 ) ) ;
#16685=CARTESIAN_POINT ( 'NONE',  ( 19.05341960407611168, 5.049401038298154454, 83.95724293864766707 ) ) ;
#16686=CARTESIAN_POINT ( 'NONE',  ( 19.02544592524334988, 5.153800228976608722, 76.45942372801897591 ) ) ;
#16687=CARTESIAN_POINT ( 'NONE',  ( 16.51473224551069308, 9.474510206698969483, 44.16557627198103120 ) ) ;
#16688=CARTESIAN_POINT ( 'NONE',  ( 16.52544592524342804, -4.483927247898539470, 78.54057627198103830 ) ) ;
#16689=CARTESIAN_POINT ( 'NONE',  ( -12.14591786802309592, -12.06949235617757132, 61.87390960531436690 ) ) ;
#16690=CARTESIAN_POINT ( 'NONE',  ( 13.97604488694527802, 13.89961937509977652, 79.37390960531435269 ) ) ;
#16691=CARTESIAN_POINT ( 'NONE',  ( 15.80617190586746368, 15.72974639402197994, 94.37390960531436690 ) ) ;
#16692=CARTESIAN_POINT ( 'NONE',  ( -19.03943276465977164, 0.05219959533909376836, 66.24890960531436690 ) ) ;
#16693=CARTESIAN_POINT ( 'NONE',  ( 21.55341960407619695, -5.719274019375665929, 111.0427570613523613 ) ) ;
#16694=CARTESIAN_POINT ( 'NONE',  ( -9.564922557960796823, -16.46253265017161027, 37.08224293864768839 ) ) ;
#16695=CARTESIAN_POINT ( 'NONE',  ( -16.53943276465976808, 0.05219959533911058130, 36.24890960531435979 ) ) ;
#16696=CARTESIAN_POINT ( 'NONE',  ( 8.224510206698953496, -14.34966873604960469, 107.9155762719810241 ) ) ;
#16697=CARTESIAN_POINT ( 'NONE',  ( -5.049401038297874678, -19.05341960407617918, 104.7927570613523471 ) ) ;
#16699=CARTESIAN_POINT ( 'NONE',  ( 18.62759615963255655, 10.81492255796105972, 26.66775706135235424 ) ) ;
#16700=CARTESIAN_POINT ( 'NONE',  ( 13.97604488694548053, -13.89961937509957401, 65.62609039468567573 ) ) ;
#16701=CARTESIAN_POINT ( 'NONE',  ( -8.224510206698948167, 14.34966873604960824, 25.41557627198103120 ) ) ;
#16702=CARTESIAN_POINT ( 'NONE',  ( 5.719274019375991003, -21.55341960407610458, 87.70724293864769550 ) ) ;
#16703=CARTESIAN_POINT ( 'NONE',  ( -16.46253265017160317, 9.564922557960807481, 115.8322429386477097 ) ) ;
#16704=CARTESIAN_POINT ( 'NONE',  ( -8.314922557960811034, -14.29746914071050412, 57.08224293864769550 ) ) ;
#16705=CARTESIAN_POINT ( 'NONE',  ( -13.89961937509977652, 13.97604488694528158, 30.62390960531435269 ) ) ;
#16706=CARTESIAN_POINT ( 'NONE',  ( 19.03943276465977164, 0.05219959533936151252, 21.25109039468565797 ) ) ;
#16707=CARTESIAN_POINT ( 'NONE',  ( 16.55341960407618274, -4.379528057220086978, 96.04275706135236135 ) ) ;
#16708=CARTESIAN_POINT ( 'NONE',  ( 16.53943276465976808, 0.05219959533934440121, 51.25109039468568994 ) ) ;
#16709=CARTESIAN_POINT ( 'NONE',  ( -19.02544592524342804, 5.153800228976336051, 116.0405762719810383 ) ) ;
#16710=CARTESIAN_POINT ( 'NONE',  ( -15.72974639402176322, -15.80617190586768395, 109.3760903946857042 ) ) ;
#16711=CARTESIAN_POINT ( 'NONE',  ( -0.05219959533909027116, -19.03943276465977164, 82.49890960531436690 ) ) ;
#16712=CARTESIAN_POINT ( 'NONE',  ( 14.29746914071037800, 8.314922557961029526, 61.66775706135235424 ) ) ;
#16713=CARTESIAN_POINT ( 'NONE',  ( -13.97604488694527625, -13.89961937509977652, 26.87390960531434558 ) ) ;
#16714=CARTESIAN_POINT ( 'NONE',  ( 14.29746914071049879, -8.314922557960816363, 38.33224293864768839 ) ) ;
#16716=CARTESIAN_POINT ( 'NONE',  ( -10.72451020669870658, -18.67979575497194134, 74.58442372801901854 ) ) ;
#16717=CARTESIAN_POINT ( 'NONE',  ( 19.05341960407611168, 5.049401038298154454, 93.95724293864769550 ) ) ;
#16718=CARTESIAN_POINT ( 'NONE',  ( 0.05219959533909260263, 19.03943276465977164, 79.99890960531436690 ) ) ;
#16719=CARTESIAN_POINT ( 'NONE',  ( 19.02544592524343514, -5.153800228976328945, 108.5405762719810383 ) ) ;
#16721=CARTESIAN_POINT ( 'NONE',  ( 4.483927247898545687, 16.52544592524342804, 64.79057627198103830 ) ) ;
#16722=CARTESIAN_POINT ( 'NONE',  ( 8.314922557960818139, 14.29746914071049879, 29.58224293864769905 ) ) ;
#16724=CARTESIAN_POINT ( 'NONE',  ( -16.52544592524342804, 4.483927247898546575, 51.04057627198103120 ) ) ;
#16725=CARTESIAN_POINT ( 'NONE',  ( 16.53943276465976808, 0.05219959533934440121, 36.25109039468567573 ) ) ;
#16727=CARTESIAN_POINT ( 'NONE',  ( 5.049401038297881783, 19.05341960407617563, 57.29275706135231871 ) ) ;
#16728=CARTESIAN_POINT ( 'NONE',  ( -16.51473224551069308, -9.474510206698971260, 76.66557627198103830 ) ) ;
#16729=CARTESIAN_POINT ( 'NONE',  ( 16.51473224551083163, -9.474510206698727899, 55.83442372801899722 ) ) ;
#16730=CARTESIAN_POINT ( 'NONE',  ( -13.89961937509957401, -13.97604488694547875, 59.37609039468566863 ) ) ;
#16731=CARTESIAN_POINT ( 'NONE',  ( 13.89961937509957401, 13.97604488694547697, 101.8760903946856331 ) ) ;
#16732=CARTESIAN_POINT ( 'NONE',  ( -14.34966873604972548, 8.224510206698743886, 83.33442372801903275 ) ) ;
#16734=CARTESIAN_POINT ( 'NONE',  ( -13.97604488694527625, -13.89961937509977652, 26.87390960531434558 ) ) ;
#16735=CARTESIAN_POINT ( 'NONE',  ( -16.46253265017160317, 9.564922557960807481, 105.8322429386476955 ) ) ;
#16736=CARTESIAN_POINT ( 'NONE',  ( -21.53943276465977519, -0.05219959533937600094, 38.75109039468567573 ) ) ;
#16737=CARTESIAN_POINT ( 'NONE',  ( -16.46253265017146816, -9.564922557961047289, 94.16775706135233293 ) ) ;
#16738=CARTESIAN_POINT ( 'NONE',  ( -5.049401038298153566, 19.05341960407611168, 60.20724293864768129 ) ) ;
#16739=CARTESIAN_POINT ( 'NONE',  ( 13.97604488694527802, 13.89961937509977652, 99.37390960531436690 ) ) ;
#16740=CARTESIAN_POINT ( 'NONE',  ( 16.53943276465976808, -0.05219959533910856209, 58.74890960531436690 ) ) ;
#16741=CARTESIAN_POINT ( 'NONE',  ( -5.153800228976328057, -19.02544592524343514, 67.29057627198102409 ) ) ;
#16742=CARTESIAN_POINT ( 'NONE',  ( -16.51473224551069308, -9.474510206698971260, 56.66557627198103120 ) ) ;
#16743=CARTESIAN_POINT ( 'NONE',  ( -16.46253265017146816, -9.564922557961047289, 69.16775706135233293 ) ) ;
#16744=CARTESIAN_POINT ( 'NONE',  ( 5.719274019375991003, -21.55341960407610458, 47.70724293864770260 ) ) ;
#16745=CARTESIAN_POINT ( 'NONE',  ( -13.97604488694547697, 13.89961937509957934, 38.12609039468566152 ) ) ;
#16746=CARTESIAN_POINT ( 'NONE',  ( -19.03943276465977164, 0.05219959533909376836, 76.24890960531435269 ) ) ;
#16748=CARTESIAN_POINT ( 'NONE',  ( -15.80617190586745835, -15.72974639402198527, 81.87390960531435269 ) ) ;
#16749=CARTESIAN_POINT ( 'NONE',  ( -16.52544592524342804, 4.483927247898546575, 76.04057627198102409 ) ) ;
#16750=CARTESIAN_POINT ( 'NONE',  ( 13.97604488694548053, -13.89961937509957401, 35.62609039468567573 ) ) ;
#16751=CARTESIAN_POINT ( 'NONE',  ( -18.62759615963270932, 10.81492255796079327, 40.83224293864769550 ) ) ;
#16752=CARTESIAN_POINT ( 'NONE',  ( -15.80617190586745835, -15.72974639402198527, 36.87390960531435979 ) ) ;
#16753=CARTESIAN_POINT ( 'NONE',  ( -9.564922557960796823, -16.46253265017161027, 72.08224293864770971 ) ) ;
#16754=CARTESIAN_POINT ( 'NONE',  ( 9.564922557960805705, 16.46253265017160317, 54.58224293864769550 ) ) ;
#16755=CARTESIAN_POINT ( 'NONE',  ( -12.14591786802309592, -12.06949235617757132, 111.8739096053143669 ) ) ;
#16756=CARTESIAN_POINT ( 'NONE',  ( -15.80617190586768217, 15.72974639402176855, 23.12609039468567573 ) ) ;
#16758=CARTESIAN_POINT ( 'NONE',  ( 15.80617190586769283, -15.72974639402175789, 30.62609039468567929 ) ) ;
#16759=CARTESIAN_POINT ( 'NONE',  ( 5.153800228976335163, 19.02544592524342804, 29.79057627198102409 ) ) ;
#16760=CARTESIAN_POINT ( 'NONE',  ( -15.72974639402197994, 15.80617190586746368, 110.6239096053143669 ) ) ;
#16761=CARTESIAN_POINT ( 'NONE',  ( 16.51473224551083163, -9.474510206698727899, 45.83442372801900433 ) ) ;
#16762=CARTESIAN_POINT ( 'NONE',  ( 16.46253265017160672, -9.564922557960803928, 28.33224293864769550 ) ) ;
#16763=CARTESIAN_POINT ( 'NONE',  ( -9.564922557960796823, -16.46253265017161027, 27.08224293864769550 ) ) ;
#16765=CARTESIAN_POINT ( 'NONE',  ( 16.53943276465976808, 0.05219959533934440121, 66.25109039468567573 ) ) ;
#16766=CARTESIAN_POINT ( 'NONE',  ( -16.51473224551069308, -9.474510206698971260, 26.66557627198103120 ) ) ;
#16768=CARTESIAN_POINT ( 'NONE',  ( -19.03943276465977164, 0.05219959533909376836, 76.24890960531435269 ) ) ;
#16769=CARTESIAN_POINT ( 'NONE',  ( 16.55341960407611168, 4.379528057220329451, 108.9572429386476955 ) ) ;
#16771=CARTESIAN_POINT ( 'NONE',  ( -21.55341960407610458, -5.719274019375992779, 61.45724293864770260 ) ) ;
#16772=CARTESIAN_POINT ( 'NONE',  ( -16.53943276465976808, 0.05219959533911058130, 76.24890960531435269 ) ) ;
#16773=CARTESIAN_POINT ( 'NONE',  ( 8.314922557961029526, -14.29746914071037800, 30.41775706135234358 ) ) ;
#16774=CARTESIAN_POINT ( 'NONE',  ( -0.05219959533937732626, 21.53943276465977519, 87.50109039468568994 ) ) ;
#16775=CARTESIAN_POINT ( 'NONE',  ( 0.05219959533909260263, 19.03943276465977164, 24.99890960531435269 ) ) ;
#16776=CARTESIAN_POINT ( 'NONE',  ( 14.29746914071037800, 8.314922557961029526, 111.6677570613523613 ) ) ;
#16777=CARTESIAN_POINT ( 'NONE',  ( 8.314922557960818139, 14.29746914071049879, 59.58224293864770260 ) ) ;
#16778=CARTESIAN_POINT ( 'NONE',  ( -5.049401038298153566, 19.05341960407611168, 55.20724293864769550 ) ) ;
#16779=CARTESIAN_POINT ( 'NONE',  ( 21.55341960407619695, -5.719274019375665929, 96.04275706135236135 ) ) ;
#16780=CARTESIAN_POINT ( 'NONE',  ( -5.823673210054116645, -21.52544592524344225, 102.2905762719810383 ) ) ;
#16781=CARTESIAN_POINT ( 'NONE',  ( 15.80617190586769283, -15.72974639402175789, 75.62609039468567573 ) ) ;
#16782=CARTESIAN_POINT ( 'NONE',  ( -14.34966873604972548, 8.224510206698743886, 38.33442372801900433 ) ) ;
#16783=CARTESIAN_POINT ( 'NONE',  ( -12.14591786802309592, -12.06949235617757132, 81.87390960531435269 ) ) ;
#16784=CARTESIAN_POINT ( 'NONE',  ( 15.80617190586769283, -15.72974639402175789, 90.62609039468567573 ) ) ;
#16785=CARTESIAN_POINT ( 'NONE',  ( -12.14591786802309592, -12.06949235617757132, 26.87390960531435979 ) ) ;
#16786=CARTESIAN_POINT ( 'NONE',  ( -17.05587630539788435, 6.762274262135666625, 115.7418030903731392 ) ) ;
#16787=CARTESIAN_POINT ( 'NONE',  ( 4.483927247898790824, -16.52544592524335698, 45.20942372801901854 ) ) ;
#16788=CARTESIAN_POINT ( 'NONE',  ( -16.52544592524342804, 4.483927247898546575, 36.04057627198102409 ) ) ;
#16789=CARTESIAN_POINT ( 'NONE',  ( 8.314922557961029526, -14.29746914071037800, 90.41775706135236135 ) ) ;
#16790=CARTESIAN_POINT ( 'NONE',  ( 16.46253265017160672, -9.564922557960803928, 98.33224293864769550 ) ) ;
#16791=CARTESIAN_POINT ( 'NONE',  ( 9.564922557960805705, 16.46253265017160317, 109.5822429386476955 ) ) ;
#16792=CARTESIAN_POINT ( 'NONE',  ( -10.81492255796105439, 18.62759615963255655, 102.9177570613523756 ) ) ;
#16793=CARTESIAN_POINT ( 'NONE',  ( 12.14591786802327356, -12.06949235617739191, 105.6260903946856899 ) ) ;
#16794=CARTESIAN_POINT ( 'NONE',  ( 16.53943276465976808, -0.05219959533910856209, 73.74890960531433848 ) ) ;
#16795=CARTESIAN_POINT ( 'NONE',  ( 0.05219959533909260263, 19.03943276465977164, 79.99890960531436690 ) ) ;
#16797=CARTESIAN_POINT ( 'NONE',  ( -16.53943276465976808, -0.05219959533934237506, 28.75109039468567929 ) ) ;
#16798=CARTESIAN_POINT ( 'NONE',  ( 0.05219959533909260263, 19.03943276465977164, 29.99890960531435979 ) ) ;
#16799=CARTESIAN_POINT ( 'NONE',  ( -16.51473224551069308, -9.474510206698971260, 86.66557627198102409 ) ) ;
#16800=CARTESIAN_POINT ( 'NONE',  ( 16.52544592524335698, 4.483927247898782831, 36.45942372801901143 ) ) ;
#16802=CARTESIAN_POINT ( 'NONE',  ( 19.02544592524334988, 5.153800228976608722, 36.45942372801900433 ) ) ;
#16803=CARTESIAN_POINT ( 'NONE',  ( -16.55341960407617563, 4.379528057220093196, 93.54275706135234714 ) ) ;
#16804=CARTESIAN_POINT ( 'NONE',  ( -16.46253265017146816, -9.564922557961047289, 104.1677570613523329 ) ) ;
#16805=CARTESIAN_POINT ( 'NONE',  ( -13.89961937509977652, 13.97604488694528158, 30.62390960531435269 ) ) ;
#16806=CARTESIAN_POINT ( 'NONE',  ( 4.483927247898790824, -16.52544592524335698, 75.20942372801901854 ) ) ;
#16807=CARTESIAN_POINT ( 'NONE',  ( -14.34966873604972548, 8.224510206698743886, 63.33442372801900433 ) ) ;
#16808=CARTESIAN_POINT ( 'NONE',  ( -9.564922557961040184, 16.46253265017147172, 77.91775706135234714 ) ) ;
#16809=CARTESIAN_POINT ( 'NONE',  ( -5.049401038297874678, -19.05341960407617918, 19.79275706135233293 ) ) ;
#16810=CARTESIAN_POINT ( 'NONE',  ( -13.97604488694527625, -13.89961937509977652, 41.87390960531435979 ) ) ;
#16811=CARTESIAN_POINT ( 'NONE',  ( -5.153800228976328057, -19.02544592524343514, 87.29057627198103830 ) ) ;
#16812=CARTESIAN_POINT ( 'NONE',  ( 0.05219959533910956823, 16.53943276465976808, 89.99890960531438111 ) ) ;
#16813=CARTESIAN_POINT ( 'NONE',  ( 9.474510206698729675, 16.51473224551082808, 52.08442372801900433 ) ) ;
#16814=CARTESIAN_POINT ( 'NONE',  ( 21.55341960407610458, 5.719274019375980345, 43.95724293864769550 ) ) ;
#16815=CARTESIAN_POINT ( 'NONE',  ( 5.153800228976615827, -19.02544592524334988, 30.20942372801900433 ) ) ;
#16816=CARTESIAN_POINT ( 'NONE',  ( 19.02544592524343514, -5.153800228976328945, 93.54057627198102409 ) ) ;
#16817=CARTESIAN_POINT ( 'NONE',  ( 0.05219959533936267826, -19.03943276465977164, 30.00109039468566863 ) ) ;
#16818=CARTESIAN_POINT ( 'NONE',  ( 21.55341960407610458, 5.719274019375980345, 78.95724293864769550 ) ) ;
#16819=CARTESIAN_POINT ( 'NONE',  ( -16.46253265017160317, 9.564922557960807481, 115.8322429386477097 ) ) ;
#16820=CARTESIAN_POINT ( 'NONE',  ( 9.474510206698729675, 16.51473224551082808, 82.08442372801899012 ) ) ;
#16821=CARTESIAN_POINT ( 'NONE',  ( -17.49999999999998934, 3.189878218039177149, 109.8705143742875237 ) ) ;
#16822=EDGE_CURVE ( 'NONE', #168063, #40368, #192932, .T. ) ;
#16823=CARTESIAN_POINT ( 'NONE',  ( 13.97604488694548053, -13.89961937509957401, 105.6260903946856757 ) ) ;
#16824=CARTESIAN_POINT ( 'NONE',  ( 9.564922557960805705, 16.46253265017160317, 39.58224293864768839 ) ) ;
#16825=CARTESIAN_POINT ( 'NONE',  ( -19.05341960407611168, -5.049401038298163336, 91.45724293864766707 ) ) ;
#16826=CARTESIAN_POINT ( 'NONE',  ( 5.823673210054125526, 21.52544592524343514, 74.79057627198105251 ) ) ;
#16827=CARTESIAN_POINT ( 'NONE',  ( 14.29746914071037800, 8.314922557961029526, 46.66775706135234714 ) ) ;
#16828=CARTESIAN_POINT ( 'NONE',  ( 21.55341960407619695, -5.719274019375665929, 46.04275706135234714 ) ) ;
#16829=CARTESIAN_POINT ( 'NONE',  ( 9.474510206698729675, 16.51473224551082808, 87.08442372801900433 ) ) ;
#16830=CARTESIAN_POINT ( 'NONE',  ( -10.72451020669870658, -18.67979575497194134, 99.58442372801900433 ) ) ;
#16831=CARTESIAN_POINT ( 'NONE',  ( 8.224510206698742110, 14.34966873604972548, 92.08442372801901854 ) ) ;
#16832=CARTESIAN_POINT ( 'NONE',  ( -16.46253265017160317, 9.564922557960807481, 95.83224293864769550 ) ) ;
#16833=CARTESIAN_POINT ( 'NONE',  ( 12.06949235617757843, -12.14591786802309237, 93.12390960531436690 ) ) ;
#16834=CARTESIAN_POINT ( 'NONE',  ( 8.224510206698953496, -14.34966873604960469, 32.91557627198102409 ) ) ;
#16835=CARTESIAN_POINT ( 'NONE',  ( -16.51473224551082808, 9.474510206698731452, 68.33442372801900433 ) ) ;
#16836=CARTESIAN_POINT ( 'NONE',  ( 21.52544592524334988, 5.823673210054432836, 56.45942372801902565 ) ) ;
#16837=CARTESIAN_POINT ( 'NONE',  ( -9.564922557961040184, 16.46253265017147172, 27.91775706135232582 ) ) ;
#16839=CARTESIAN_POINT ( 'NONE',  ( 16.52544592524342804, -4.483927247898539470, 108.5405762719810241 ) ) ;
#16840=CARTESIAN_POINT ( 'NONE',  ( 10.81492255796078972, 18.62759615963270932, 29.58224293864769905 ) ) ;
#16841=CARTESIAN_POINT ( 'NONE',  ( -4.483927247898782831, 16.52544592524335698, 112.7094237280190328 ) ) ;
#16842=CARTESIAN_POINT ( 'NONE',  ( -5.823673210054431948, 21.52544592524334988, 97.70942372801904696 ) ) ;
#16843=CARTESIAN_POINT ( 'NONE',  ( 12.14591786802327356, -12.06949235617739191, 60.62609039468567573 ) ) ;
#16844=CARTESIAN_POINT ( 'NONE',  ( -4.483927247898539470, -16.52544592524342804, 22.29057627198102765 ) ) ;
#16845=CARTESIAN_POINT ( 'NONE',  ( -10.81492255796105439, 18.62759615963255655, 52.91775706135235424 ) ) ;
#16846=CARTESIAN_POINT ( 'NONE',  ( -18.62759615963255300, -10.81492255796106328, 49.16775706135234003 ) ) ;
#16847=CARTESIAN_POINT ( 'NONE',  ( -18.67979575497193778, 10.72451020669871902, 28.33442372801902209 ) ) ;
#16848=CARTESIAN_POINT ( 'NONE',  ( 8.314922557960818139, 14.29746914071049879, 99.58224293864770971 ) ) ;
#16849=CARTESIAN_POINT ( 'NONE',  ( 5.049401038298161559, -19.05341960407611168, 27.70724293864769550 ) ) ;
#16850=CARTESIAN_POINT ( 'NONE',  ( 12.14591786802309770, 12.06949235617756955, 74.37390960531436690 ) ) ;
#16851=CARTESIAN_POINT ( 'NONE',  ( -19.05341960407611168, -5.049401038298163336, 66.45724293864769550 ) ) ;
#16852=CARTESIAN_POINT ( 'NONE',  ( 4.379528057220092307, 16.55341960407617563, 112.2927570613523471 ) ) ;
#16853=CARTESIAN_POINT ( 'NONE',  ( 10.72451020669898902, -18.67979575497178502, 57.91557627198103120 ) ) ;
#16854=CARTESIAN_POINT ( 'NONE',  ( -14.34966873604960291, -8.224510206698953496, 86.66557627198102409 ) ) ;
#16855=CARTESIAN_POINT ( 'NONE',  ( 10.81492255796078972, 18.62759615963270932, 99.58224293864770971 ) ) ;
#16856=CARTESIAN_POINT ( 'NONE',  ( 5.049401038298161559, -19.05341960407611168, 97.70724293864766707 ) ) ;
#16857=CARTESIAN_POINT ( 'NONE',  ( 0.05219959533909260263, 19.03943276465977164, 49.99890960531435979 ) ) ;
#16858=CARTESIAN_POINT ( 'NONE',  ( 19.03943276465977164, 0.05219959533936151252, 106.2510903946856615 ) ) ;
#16859=CARTESIAN_POINT ( 'NONE',  ( 18.62759615963271287, -10.81492255796078972, 48.33224293864770260 ) ) ;
#16860=CARTESIAN_POINT ( 'NONE',  ( 10.72451020669871369, 18.67979575497193778, 72.08442372801899012 ) ) ;
#16861=CARTESIAN_POINT ( 'NONE',  ( -9.474510206698964154, 16.51473224551069663, 70.41557627198102409 ) ) ;
#16862=CARTESIAN_POINT ( 'NONE',  ( 19.03943276465977164, -0.05219959533909143690, 93.74890960531435269 ) ) ;
#16863=CARTESIAN_POINT ( 'NONE',  ( 12.14591786802327356, -12.06949235617739191, 65.62609039468568994 ) ) ;
#16864=CARTESIAN_POINT ( 'NONE',  ( 18.67979575497194134, -10.72451020669871369, 55.83442372801901854 ) ) ;
#16865=CARTESIAN_POINT ( 'NONE',  ( -5.823673210054431948, 21.52544592524334988, 87.70942372801901854 ) ) ;
#16866=CARTESIAN_POINT ( 'NONE',  ( 15.72974639402199770, -15.80617190586745480, 93.12390960531436690 ) ) ;
#16867=CARTESIAN_POINT ( 'NONE',  ( 10.81492255796106328, -18.62759615963255655, 35.41775706135234003 ) ) ;
#16868=CARTESIAN_POINT ( 'NONE',  ( 8.224510206698742110, 14.34966873604972548, 72.08442372801899012 ) ) ;
#16869=CARTESIAN_POINT ( 'NONE',  ( -10.81492255796078084, -18.62759615963271287, 82.08224293864768129 ) ) ;
#16870=CARTESIAN_POINT ( 'NONE',  ( 5.153800228976615827, -19.02544592524334988, 30.20942372801900433 ) ) ;
#16871=CARTESIAN_POINT ( 'NONE',  ( 5.049401038298161559, -19.05341960407611168, 82.70724293864770971 ) ) ;
#16872=CARTESIAN_POINT ( 'NONE',  ( -8.314922557960811034, -14.29746914071050412, 22.08224293864769194 ) ) ;
#16874=CARTESIAN_POINT ( 'NONE',  ( 13.89961937509977652, -13.97604488694527269, 103.1239096053143527 ) ) ;
#16875=CARTESIAN_POINT ( 'NONE',  ( 17.72560187377284535, 5.500000000000042633, 81.57814504131323474 ) ) ;
#16876=CARTESIAN_POINT ( 'NONE',  ( 16.51473224551083163, -9.474510206698727899, 90.83442372801900433 ) ) ;
#16877=CARTESIAN_POINT ( 'NONE',  ( 21.52544592524344225, -5.823673210054117533, 58.54057627198103120 ) ) ;
#16878=CARTESIAN_POINT ( 'NONE',  ( 12.14591786802309770, 12.06949235617756955, 34.37390960531435979 ) ) ;
#16879=CARTESIAN_POINT ( 'NONE',  ( -16.55341960407617563, 4.379528057220093196, 23.54275706135235424 ) ) ;
#16880=CARTESIAN_POINT ( 'NONE',  ( 13.89961937509977652, -13.97604488694527269, 38.12390960531436690 ) ) ;
#16881=CARTESIAN_POINT ( 'NONE',  ( -5.049401038297874678, -19.05341960407617918, 109.7927570613523187 ) ) ;
#16882=CARTESIAN_POINT ( 'NONE',  ( 0.05219959533907565091, 21.53943276465977519, 104.9989096053143669 ) ) ;
#16883=CARTESIAN_POINT ( 'NONE',  ( 9.474510206698729675, 16.51473224551082808, 77.08442372801900433 ) ) ;
#16884=CARTESIAN_POINT ( 'NONE',  ( 4.483927247898790824, -16.52544592524335698, 80.20942372801901854 ) ) ;
#16885=CARTESIAN_POINT ( 'NONE',  ( -19.02544592524342804, 5.153800228976336051, 66.04057627198103830 ) ) ;
#16886=CARTESIAN_POINT ( 'NONE',  ( 14.29746914071049879, -8.314922557960816363, 73.33224293864769550 ) ) ;
#16887=CARTESIAN_POINT ( 'NONE',  ( 0.05219959533909260263, 19.03943276465977164, 54.99890960531435979 ) ) ;
#16888=CARTESIAN_POINT ( 'NONE',  ( -0.05219959533910754901, -16.53943276465976808, 67.49890960531436690 ) ) ;
#16891=CARTESIAN_POINT ( 'NONE',  ( -16.53943276465976808, 0.05219959533911058130, 36.24890960531435979 ) ) ;
#16892=CARTESIAN_POINT ( 'NONE',  ( -19.03943276465977164, 0.05219959533909376836, 81.24890960531436690 ) ) ;
#16894=CARTESIAN_POINT ( 'NONE',  ( -13.97604488694547697, 13.89961937509957934, 58.12609039468566863 ) ) ;
#16895=CARTESIAN_POINT ( 'NONE',  ( 8.224510206698742110, 14.34966873604972548, 57.08442372801901854 ) ) ;
#16896=CARTESIAN_POINT ( 'NONE',  ( 21.55341960407610458, 5.719274019375980345, 63.95724293864770260 ) ) ;
#16897=CARTESIAN_POINT ( 'NONE',  ( 9.564922557961047289, -16.46253265017146816, 25.41775706135234003 ) ) ;
#16898=CARTESIAN_POINT ( 'NONE',  ( -13.89961937509977652, 13.97604488694528158, 80.62390960531436690 ) ) ;
#16900=CARTESIAN_POINT ( 'NONE',  ( 16.51473224551069308, 9.474510206698969483, 114.1655762719810241 ) ) ;
#16901=CARTESIAN_POINT ( 'NONE',  ( -5.049401038298153566, 19.05341960407611168, 65.20724293864765286 ) ) ;
#16902=CARTESIAN_POINT ( 'NONE',  ( 0.05219959533937995610, -21.53943276465977519, 35.00109039468568284 ) ) ;
#16903=CARTESIAN_POINT ( 'NONE',  ( 8.314922557960818139, 14.29746914071049879, 104.5822429386477097 ) ) ;
#16904=CARTESIAN_POINT ( 'NONE',  ( -15.80617190586745835, -15.72974639402198527, 96.87390960531436690 ) ) ;
#16905=CARTESIAN_POINT ( 'NONE',  ( 9.564922557960805705, 16.46253265017160317, 94.58224293864769550 ) ) ;
#16907=CARTESIAN_POINT ( 'NONE',  ( 5.719274019375673035, 21.55341960407619339, 32.29275706135235424 ) ) ;
#16908=ORIENTED_EDGE ( 'NONE', *, *, #196572, .F. ) ;
#16909=CARTESIAN_POINT ( 'NONE',  ( 0.05219959533909260263, 19.03943276465977164, 84.99890960531436690 ) ) ;
#16910=DIRECTION ( 'NONE',  ( 0.000000000000000000, 0.000000000000000000, 1.000000000000000000 ) ) ;
#16911=CARTESIAN_POINT ( 'NONE',  ( -10.72451020669898014, 18.67979575497178502, 100.4155762719810241 ) ) ;
#16912=CARTESIAN_POINT ( 'NONE',  ( -13.89961937509977652, 13.97604488694528158, 45.62390960531433848 ) ) ;
#16913=CARTESIAN_POINT ( 'NONE',  ( 0.05219959533936267826, -19.03943276465977164, 105.0010903946856615 ) ) ;
#16915=CARTESIAN_POINT ( 'NONE',  ( 19.05341960407611168, 5.049401038298154454, 23.95724293864769194 ) ) ;
#16916=CARTESIAN_POINT ( 'NONE',  ( 18.67979575497194134, -10.72451020669871369, 85.83442372801901854 ) ) ;
#16917=CARTESIAN_POINT ( 'NONE',  ( -13.97604488694527625, -13.89961937509977652, 71.87390960531433848 ) ) ;
#16918=CARTESIAN_POINT ( 'NONE',  ( 10.81492255796106328, -18.62759615963255655, 50.41775706135235424 ) ) ;
#16919=CARTESIAN_POINT ( 'NONE',  ( 18.62759615963255655, 10.81492255796105972, 21.66775706135235069 ) ) ;
#16921=CARTESIAN_POINT ( 'NONE',  ( -16.46253265017160317, 9.564922557960807481, 100.8322429386477097 ) ) ;
#16923=CARTESIAN_POINT ( 'NONE',  ( -0.05219959533934338120, 16.53943276465976808, 42.50109039468567573 ) ) ;
#16924=CARTESIAN_POINT ( 'NONE',  ( 18.62759615963271287, -10.81492255796078972, 48.33224293864770260 ) ) ;
#16925=CARTESIAN_POINT ( 'NONE',  ( 5.823673210054444382, -21.52544592524334988, 40.20942372801901854 ) ) ;
#16926=CARTESIAN_POINT ( 'NONE',  ( 21.53943276465977519, 0.05219959533937863772, 71.25109039468568994 ) ) ;
#16928=CARTESIAN_POINT ( 'NONE',  ( -16.52544592524335698, -4.483927247898792601, 18.95942372801901143 ) ) ;
#16929=CARTESIAN_POINT ( 'NONE',  ( 19.02544592524343514, -5.153800228976328945, 63.54057627198103830 ) ) ;
#16930=CARTESIAN_POINT ( 'NONE',  ( 16.51473224551069308, 9.474510206698969483, 79.16557627198103830 ) ) ;
#16931=CARTESIAN_POINT ( 'NONE',  ( 8.224510206698953496, -14.34966873604960469, 107.9155762719810241 ) ) ;
#16932=CARTESIAN_POINT ( 'NONE',  ( -16.52544592524342804, 4.483927247898546575, 106.0405762719810525 ) ) ;
#16933=CARTESIAN_POINT ( 'NONE',  ( 0.05219959533907565091, 21.53943276465977519, 34.99890960531435979 ) ) ;
#16934=CARTESIAN_POINT ( 'NONE',  ( -4.483927247898782831, 16.52544592524335698, 82.70942372801900433 ) ) ;
#16935=CARTESIAN_POINT ( 'NONE',  ( 0.05219959533910956823, 16.53943276465976808, 64.99890960531435269 ) ) ;
#16936=CARTESIAN_POINT ( 'NONE',  ( 19.05341960407611168, 5.049401038298154454, 48.95724293864768129 ) ) ;
#16937=CARTESIAN_POINT ( 'NONE',  ( -15.80617190586768217, 15.72974639402176855, 73.12609039468567573 ) ) ;
#16938=CARTESIAN_POINT ( 'NONE',  ( 15.72974639402176855, 15.80617190586768217, 71.87609039468568994 ) ) ;
#16939=CARTESIAN_POINT ( 'NONE',  ( -19.05341960407617563, 5.049401038297882671, 108.5427570613523187 ) ) ;
#16940=CARTESIAN_POINT ( 'NONE',  ( 8.224510206698953496, -14.34966873604960469, 57.91557627198103120 ) ) ;
#16941=CARTESIAN_POINT ( 'NONE',  ( -21.53943276465977519, -0.05219959533937600094, 23.75109039468567929 ) ) ;
#16942=CARTESIAN_POINT ( 'NONE',  ( -18.62759615963270932, 10.81492255796079327, 65.83224293864769550 ) ) ;
#16943=CARTESIAN_POINT ( 'NONE',  ( 18.87255363501904526, 5.499999999999952038, 73.82513748171827217 ) ) ;
#16945=CARTESIAN_POINT ( 'NONE',  ( 13.89961937509977652, -13.97604488694527269, 63.12390960531435979 ) ) ;
#16946=CARTESIAN_POINT ( 'NONE',  ( -12.06949235617756955, 12.14591786802309770, 30.62390960531436335 ) ) ;
#16947=CARTESIAN_POINT ( 'NONE',  ( 4.483927247898790824, -16.52544592524335698, 110.2094237280190185 ) ) ;
#16948=CARTESIAN_POINT ( 'NONE',  ( -16.52544592524335698, -4.483927247898792601, 93.95942372801903275 ) ) ;
#16949=CARTESIAN_POINT ( 'NONE',  ( 9.564922557961047289, -16.46253265017146816, 50.41775706135233293 ) ) ;
#16951=CARTESIAN_POINT ( 'NONE',  ( 19.03943276465977164, -0.05219959533909143690, 108.7489096053143527 ) ) ;
#16952=CARTESIAN_POINT ( 'NONE',  ( -8.224510206698948167, 14.34966873604960824, 75.41557627198102409 ) ) ;
#16953=CARTESIAN_POINT ( 'NONE',  ( -0.05219959533936034679, 19.03943276465977164, 42.50109039468566152 ) ) ;
#16954=CARTESIAN_POINT ( 'NONE',  ( 13.97604488694527802, 13.89961937509977652, 29.37390960531435979 ) ) ;
#16955=CARTESIAN_POINT ( 'NONE',  ( -0.05219959533907301413, -21.53943276465977519, 22.49890960531436335 ) ) ;
#16956=CARTESIAN_POINT ( 'NONE',  ( 21.55341960407610458, 5.719274019375980345, 58.95724293864770971 ) ) ;
#16958=CARTESIAN_POINT ( 'NONE',  ( -16.55341960407611168, -4.379528057220339221, 96.45724293864770971 ) ) ;
#16959=CARTESIAN_POINT ( 'NONE',  ( 8.314922557961029526, -14.29746914071037800, 55.41775706135234714 ) ) ;
#16961=CARTESIAN_POINT ( 'NONE',  ( -12.14591786802309592, -12.06949235617757132, 91.87390960531436690 ) ) ;
#16963=CARTESIAN_POINT ( 'NONE',  ( -16.31925111598457434, 7.325300261831449333, 50.16424538967250868 ) ) ;
#16964=CARTESIAN_POINT ( 'NONE',  ( 19.02544592524343514, -5.153800228976328945, 113.5405762719810241 ) ) ;
#16967=CARTESIAN_POINT ( 'NONE',  ( 4.483927247898790824, -16.52544592524335698, 45.20942372801901854 ) ) ;
#16968=CARTESIAN_POINT ( 'NONE',  ( 16.53943276465976808, -0.05219959533910856209, 23.74890960531435269 ) ) ;
#16969=CARTESIAN_POINT ( 'NONE',  ( 0.05219959533907565091, 21.53943276465977519, 59.99890960531436690 ) ) ;
#16970=CARTESIAN_POINT ( 'NONE',  ( 0.05219959533936267826, -19.03943276465977164, 85.00109039468567573 ) ) ;
#16971=CARTESIAN_POINT ( 'NONE',  ( -21.53943276465977519, 0.05219959533907696930, 46.24890960531435979 ) ) ;
#16972=CARTESIAN_POINT ( 'NONE',  ( -0.05219959533937732626, 21.53943276465977519, 87.50109039468568994 ) ) ;
#16974=CARTESIAN_POINT ( 'NONE',  ( 8.314922557961029526, -14.29746914071037800, 50.41775706135235424 ) ) ;
#16975=CARTESIAN_POINT ( 'NONE',  ( 0.05219959533909260263, 19.03943276465977164, 39.99890960531436690 ) ) ;
#16976=CARTESIAN_POINT ( 'NONE',  ( -5.153800228976328057, -19.02544592524343514, 102.2905762719810383 ) ) ;
#16977=CARTESIAN_POINT ( 'NONE',  ( 19.05341960407611168, 5.049401038298154454, 38.95724293864767418 ) ) ;
#16978=CARTESIAN_POINT ( 'NONE',  ( -4.483927247898539470, -16.52544592524342804, 102.2905762719810383 ) ) ;
#16980=CARTESIAN_POINT ( 'NONE',  ( -13.97604488694527625, -13.89961937509977652, 101.8739096053143811 ) ) ;
#16982=CARTESIAN_POINT ( 'NONE',  ( 8.314922557961029526, -14.29746914071037800, 60.41775706135235424 ) ) ;
#16983=CARTESIAN_POINT ( 'NONE',  ( 18.62759615963271287, -10.81492255796078972, 93.33224293864769550 ) ) ;
#16984=CARTESIAN_POINT ( 'NONE',  ( -5.153800228976328057, -19.02544592524343514, 52.29057627198100988 ) ) ;
#16985=CARTESIAN_POINT ( 'NONE',  ( -18.62759615963255300, -10.81492255796106328, 29.16775706135234003 ) ) ;
#16986=CARTESIAN_POINT ( 'NONE',  ( 13.89961937509977652, -13.97604488694527269, 83.12390960531436690 ) ) ;
#16987=CARTESIAN_POINT ( 'NONE',  ( -19.03943276465977164, 0.05219959533909376836, 116.2489096053143669 ) ) ;
#16989=VERTEX_POINT ( 'NONE', #43772 ) ;
#16990=CARTESIAN_POINT ( 'NONE',  ( -5.823673210054116645, -21.52544592524344225, 112.2905762719810241 ) ) ;
#16991=CARTESIAN_POINT ( 'NONE',  ( -13.97604488694527625, -13.89961937509977652, 21.87390960531435979 ) ) ;
#16992=CARTESIAN_POINT ( 'NONE',  ( 19.02544592524343514, -5.153800228976328945, 108.5405762719810383 ) ) ;
#16993=CARTESIAN_POINT ( 'NONE',  ( 5.153800228976615827, -19.02544592524334988, 75.20942372801896170 ) ) ;
#16994=CARTESIAN_POINT ( 'NONE',  ( -0.05219959533936034679, 19.03943276465977164, 32.50109039468566863 ) ) ;
#16995=CARTESIAN_POINT ( 'NONE',  ( -15.72974639402197994, 15.80617190586746368, 95.62390960531436690 ) ) ;
#16996=CARTESIAN_POINT ( 'NONE',  ( -13.89961937509957401, -13.97604488694547875, 39.37609039468566152 ) ) ;
#16997=CARTESIAN_POINT ( 'NONE',  ( -16.52544592524335698, -4.483927247898792601, 83.95942372801900433 ) ) ;
#16999=CARTESIAN_POINT ( 'NONE',  ( 13.97604488694527802, 13.89961937509977652, 104.3739096053143385 ) ) ;
#17000=VERTEX_POINT ( 'NONE', #30583 ) ;
#17001=CARTESIAN_POINT ( 'NONE',  ( 5.049401038298161559, -19.05341960407611168, 62.70724293864769550 ) ) ;
#17002=CARTESIAN_POINT ( 'NONE',  ( 10.72451020669871369, 18.67979575497193778, 72.08442372801899012 ) ) ;
#17003=CARTESIAN_POINT ( 'NONE',  ( -0.05219959533937732626, 21.53943276465977519, 77.50109039468567573 ) ) ;
#17004=CARTESIAN_POINT ( 'NONE',  ( -5.153800228976328057, -19.02544592524343514, 72.29057627198102409 ) ) ;
#17005=CARTESIAN_POINT ( 'NONE',  ( -5.719274019375665041, -21.55341960407619695, 54.79275706135235424 ) ) ;
#17006=CARTESIAN_POINT ( 'NONE',  ( -5.049401038297874678, -19.05341960407617918, 84.79275706135233293 ) ) ;
#17007=CARTESIAN_POINT ( 'NONE',  ( 13.89961937509977652, -13.97604488694527269, 53.12390960531434558 ) ) ;
#17008=CARTESIAN_POINT ( 'NONE',  ( -13.97604488694527625, -13.89961937509977652, 96.87390960531433848 ) ) ;
#17009=CARTESIAN_POINT ( 'NONE',  ( -13.89961937509977652, 13.97604488694528158, 70.62390960531432427 ) ) ;
#17011=CARTESIAN_POINT ( 'NONE',  ( 5.049401038298161559, -19.05341960407611168, 57.70724293864769550 ) ) ;
#17012=CARTESIAN_POINT ( 'NONE',  ( 18.67979575497178502, 10.72451020669898547, 99.16557627198100988 ) ) ;
#17013=CARTESIAN_POINT ( 'NONE',  ( -8.314922557961024197, 14.29746914071037800, 72.91775706135234714 ) ) ;
#17015=CARTESIAN_POINT ( 'NONE',  ( -19.02544592524334988, -5.153800228976617603, 33.95942372801897591 ) ) ;
#17016=CARTESIAN_POINT ( 'NONE',  ( -13.97604488694527625, -13.89961937509977652, 61.87390960531435979 ) ) ;
#17017=CARTESIAN_POINT ( 'NONE',  ( 4.483927247898545687, 16.52544592524342804, 54.79057627198104541 ) ) ;
#17018=CARTESIAN_POINT ( 'NONE',  ( 14.29746914071049879, -8.314922557960816363, 93.33224293864769550 ) ) ;
#17019=CARTESIAN_POINT ( 'NONE',  ( 5.153800228976335163, 19.02544592524342804, 104.7905762719809957 ) ) ;
#17020=CARTESIAN_POINT ( 'NONE',  ( -9.564922557960796823, -16.46253265017161027, 92.08224293864769550 ) ) ;
#17021=CARTESIAN_POINT ( 'NONE',  ( 9.474510206698971260, -16.51473224551069308, 107.9155762719810383 ) ) ;
#17022=CARTESIAN_POINT ( 'NONE',  ( -18.67979575497193778, 10.72451020669871902, 113.3344237280190328 ) ) ;
#17023=CARTESIAN_POINT ( 'NONE',  ( -16.55341960407617563, 4.379528057220093196, 88.54275706135236135 ) ) ;
#17024=CARTESIAN_POINT ( 'NONE',  ( 10.72451020669871369, 18.67979575497193778, 42.08442372801901854 ) ) ;
#17025=CARTESIAN_POINT ( 'NONE',  ( -18.62759615963270932, 10.81492255796079327, 30.83224293864770260 ) ) ;
#17026=CARTESIAN_POINT ( 'NONE',  ( 18.67979575497178502, 10.72451020669898547, 104.1655762719810241 ) ) ;
#17027=CARTESIAN_POINT ( 'NONE',  ( -12.06949235617756955, 12.14591786802309770, 55.62390960531436690 ) ) ;
#17028=CARTESIAN_POINT ( 'NONE',  ( 13.97604488694527802, 13.89961937509977652, 54.37390960531435979 ) ) ;
#17029=CARTESIAN_POINT ( 'NONE',  ( 0.05219959533910956823, 16.53943276465976808, 74.99890960531435269 ) ) ;
#17030=CARTESIAN_POINT ( 'NONE',  ( -13.89961937509957401, -13.97604488694547875, 44.37609039468566863 ) ) ;
#17031=CARTESIAN_POINT ( 'NONE',  ( -16.52544592524342804, 4.483927247898546575, 116.0405762719810383 ) ) ;
#17033=CARTESIAN_POINT ( 'NONE',  ( 16.52544592524335698, 4.483927247898782831, 61.45942372801901854 ) ) ;
#17034=CARTESIAN_POINT ( 'NONE',  ( -9.474510206698964154, 16.51473224551069663, 70.41557627198102409 ) ) ;
#17036=CARTESIAN_POINT ( 'NONE',  ( 0.05219959533910956823, 16.53943276465976808, 89.99890960531438111 ) ) ;
#17037=CARTESIAN_POINT ( 'NONE',  ( 10.72451020669898902, -18.67979575497178502, 42.91557627198103120 ) ) ;
#17039=CARTESIAN_POINT ( 'NONE',  ( 12.14591786802327356, -12.06949235617739191, 110.6260903946857042 ) ) ;
#17040=CARTESIAN_POINT ( 'NONE',  ( 12.06949235617739724, 12.14591786802326823, 31.87609039468567929 ) ) ;
#17041=CARTESIAN_POINT ( 'NONE',  ( 18.62759615963255655, 10.81492255796105972, 86.66775706135234714 ) ) ;
#17042=CARTESIAN_POINT ( 'NONE',  ( -13.89961937509977652, 13.97604488694528158, 90.62390960531432427 ) ) ;
#17043=CARTESIAN_POINT ( 'NONE',  ( 5.823673210054125526, 21.52544592524343514, 114.7905762719810383 ) ) ;
#17044=CARTESIAN_POINT ( 'NONE',  ( 19.05341960407611168, 5.049401038298154454, 28.95724293864769550 ) ) ;
#17045=CARTESIAN_POINT ( 'NONE',  ( -12.06949235617739369, -12.14591786802326823, 34.37609039468568284 ) ) ;
#17046=CARTESIAN_POINT ( 'NONE',  ( -9.474510206698720793, -16.51473224551083518, 89.58442372801900433 ) ) ;
#17047=CARTESIAN_POINT ( 'NONE',  ( -5.719274019375978568, 21.55341960407610458, 90.20724293864770971 ) ) ;
#17048=CARTESIAN_POINT ( 'NONE',  ( 5.153800228976615827, -19.02544592524334988, 70.20942372801899012 ) ) ;
#17050=CARTESIAN_POINT ( 'NONE',  ( -15.72974639402176322, -15.80617190586768395, 19.37609039468568639 ) ) ;
#17052=CARTESIAN_POINT ( 'NONE',  ( 16.51473224551069308, 9.474510206698969483, 84.16557627198102409 ) ) ;
#17053=CARTESIAN_POINT ( 'NONE',  ( -14.34966873604972548, 8.224510206698743886, 33.33442372801900433 ) ) ;
#17055=CARTESIAN_POINT ( 'NONE',  ( 19.03943276465977164, 0.05219959533936151252, 61.25109039468566863 ) ) ;
#17056=CARTESIAN_POINT ( 'NONE',  ( 5.719274019375991003, -21.55341960407610458, 112.7072429386476955 ) ) ;
#17057=CARTESIAN_POINT ( 'NONE',  ( -8.314922557960811034, -14.29746914071050412, 72.08224293864769550 ) ) ;
#17058=CARTESIAN_POINT ( 'NONE',  ( -0.05219959533909027116, -19.03943276465977164, 82.49890960531436690 ) ) ;
#17059=CARTESIAN_POINT ( 'NONE',  ( -8.224510206698735004, -14.34966873604973081, 39.58442372801901143 ) ) ;
#17060=CARTESIAN_POINT ( 'NONE',  ( -19.03943276465977164, -0.05219959533935918106, 48.75109039468566863 ) ) ;
#17062=CARTESIAN_POINT ( 'NONE',  ( 21.55341960407619695, -5.719274019375665929, 61.04275706135234714 ) ) ;
#17063=CARTESIAN_POINT ( 'NONE',  ( 19.05341960407617918, -5.049401038297876454, 111.0427570613523329 ) ) ;
#17064=CARTESIAN_POINT ( 'NONE',  ( -19.05341960407611168, -5.049401038298163336, 61.45724293864769550 ) ) ;
#17065=CARTESIAN_POINT ( 'NONE',  ( 13.89961937509957401, 13.97604488694547697, 76.87609039468566152 ) ) ;
#17066=CARTESIAN_POINT ( 'NONE',  ( -16.55341960407617563, 4.379528057220093196, 53.54275706135234714 ) ) ;
#17067=CARTESIAN_POINT ( 'NONE',  ( -0.05219959533937732626, 21.53943276465977519, 97.50109039468567573 ) ) ;
#17068=CARTESIAN_POINT ( 'NONE',  ( -0.05219959533936034679, 19.03943276465977164, 67.50109039468566152 ) ) ;
#17069=CARTESIAN_POINT ( 'NONE',  ( 19.05341960407611168, 5.049401038298154454, 48.95724293864768129 ) ) ;
#17070=CARTESIAN_POINT ( 'NONE',  ( 10.81492255796078972, 18.62759615963270932, 74.58224293864768129 ) ) ;
#17071=CARTESIAN_POINT ( 'NONE',  ( -14.29746914071049879, 8.314922557960819915, 60.83224293864769550 ) ) ;
#17072=CARTESIAN_POINT ( 'NONE',  ( -13.89961937509957401, -13.97604488694547875, 64.37609039468567573 ) ) ;
#17074=CARTESIAN_POINT ( 'NONE',  ( 16.51473224551083163, -9.474510206698727899, 40.83442372801900433 ) ) ;
#17075=CARTESIAN_POINT ( 'NONE',  ( -14.34966873604972548, 8.224510206698743886, 103.3344237280190043 ) ) ;
#17076=CARTESIAN_POINT ( 'NONE',  ( -0.05219959533910754901, -16.53943276465976808, 62.49890960531436690 ) ) ;
#17077=CARTESIAN_POINT ( 'NONE',  ( -10.81492255796105439, 18.62759615963255655, 102.9177570613523756 ) ) ;
#17079=CARTESIAN_POINT ( 'NONE',  ( -21.52544592524343514, 5.823673210054127303, 91.04057627198103830 ) ) ;
#17080=CARTESIAN_POINT ( 'NONE',  ( 19.02544592524343514, -5.153800228976328945, 68.54057627198103830 ) ) ;
#17081=CARTESIAN_POINT ( 'NONE',  ( -5.719274019375665041, -21.55341960407619695, 64.79275706135234714 ) ) ;
#17082=CARTESIAN_POINT ( 'NONE',  ( 13.97604488694527802, 13.89961937509977652, 44.37390960531435269 ) ) ;
#17083=VERTEX_POINT ( 'NONE', #170084 ) ;
#17084=CARTESIAN_POINT ( 'NONE',  ( 19.05341960407611168, 5.049401038298154454, 68.95724293864769550 ) ) ;
#17085=CARTESIAN_POINT ( 'NONE',  ( 8.314922557960818139, 14.29746914071049879, 114.5822429386477097 ) ) ;
#17086=CARTESIAN_POINT ( 'NONE',  ( -5.823673210054116645, -21.52544592524344225, 22.29057627198102765 ) ) ;
#17087=CARTESIAN_POINT ( 'NONE',  ( 16.53943276465976808, -0.05219959533910856209, 68.74890960531435269 ) ) ;
#17088=CARTESIAN_POINT ( 'NONE',  ( -9.474510206698964154, 16.51473224551069663, 35.41557627198102409 ) ) ;
#17089=CARTESIAN_POINT ( 'NONE',  ( 8.314922557960818139, 14.29746914071049879, 84.58224293864769550 ) ) ;
#17090=CARTESIAN_POINT ( 'NONE',  ( -10.81492255796078084, -18.62759615963271287, 97.08224293864770971 ) ) ;
#17091=CARTESIAN_POINT ( 'NONE',  ( 15.72974639402176855, 15.80617190586768217, 31.87609039468567929 ) ) ;
#17093=CARTESIAN_POINT ( 'NONE',  ( 4.483927247898790824, -16.52544592524335698, 50.20942372801901854 ) ) ;
#17094=CARTESIAN_POINT ( 'NONE',  ( -18.62759615963270932, 10.81492255796079327, 80.83224293864769550 ) ) ;
#17095=CARTESIAN_POINT ( 'NONE',  ( 9.474510206698729675, 16.51473224551082808, 27.08442372801900433 ) ) ;
#17096=CARTESIAN_POINT ( 'NONE',  ( -9.474510206698964154, 16.51473224551069663, 100.4155762719810241 ) ) ;
#17097=CARTESIAN_POINT ( 'NONE',  ( -18.67979575497193778, 10.72451020669871902, 48.33442372801902565 ) ) ;
#17099=CARTESIAN_POINT ( 'NONE',  ( 21.55341960407610458, 5.719274019375980345, 48.95724293864770971 ) ) ;
#17100=CARTESIAN_POINT ( 'NONE',  ( -0.05219959533934338120, 16.53943276465976808, 112.5010903946857042 ) ) ;
#17101=CARTESIAN_POINT ( 'NONE',  ( -15.72974639402176322, -15.80617190586768395, 69.37609039468567573 ) ) ;
#17102=CARTESIAN_POINT ( 'NONE',  ( -21.55341960407619339, 5.719274019375674811, 103.5427570613523613 ) ) ;
#17103=CARTESIAN_POINT ( 'NONE',  ( 13.97604488694548053, -13.89961937509957401, 35.62609039468567573 ) ) ;
#17104=CARTESIAN_POINT ( 'NONE',  ( -12.06949235617739369, -12.14591786802326823, 84.37609039468570415 ) ) ;
#17105=CARTESIAN_POINT ( 'NONE',  ( 15.72974639402176855, 15.80617190586768217, 41.87609039468568284 ) ) ;
#17106=CARTESIAN_POINT ( 'NONE',  ( 13.97604488694527802, 13.89961937509977652, 44.37390960531435269 ) ) ;
#17107=CARTESIAN_POINT ( 'NONE',  ( 5.153800228976615827, -19.02544592524334988, 20.20942372801899722 ) ) ;
#17108=CARTESIAN_POINT ( 'NONE',  ( -5.719274019375978568, 21.55341960407610458, 30.20724293864769550 ) ) ;
#17109=B_SPLINE_CURVE_WITH_KNOTS ( 'NONE', 3,
 ( #182684, #137157, #198846, #86668, #41180, #148351 ),
 .UNSPECIFIED., .F., .F.,
 ( 4, 2, 4 ),
 ( 0.001769412596444650985, 0.002152742221722609914, 0.002536071847000569059 ),
 .UNSPECIFIED. ) ;
#17110=CARTESIAN_POINT ( 'NONE',  ( -5.719274019375978568, 21.55341960407610458, 115.2072429386476955 ) ) ;
#17111=CARTESIAN_POINT ( 'NONE',  ( 10.72451020669898902, -18.67979575497178502, 72.91557627198103830 ) ) ;
#17112=CARTESIAN_POINT ( 'NONE',  ( 4.379528057220092307, 16.55341960407617563, 37.29275706135235424 ) ) ;
#17114=CARTESIAN_POINT ( 'NONE',  ( -10.72451020669898014, 18.67979575497178502, 80.41557627198103830 ) ) ;
#17115=CARTESIAN_POINT ( 'NONE',  ( -4.483927247898782831, 16.52544592524335698, 62.70942372801902565 ) ) ;
#17116=CARTESIAN_POINT ( 'NONE',  ( 8.224510206698953496, -14.34966873604960469, 67.91557627198102409 ) ) ;
#17118=CARTESIAN_POINT ( 'NONE',  ( -16.46253265017146816, -9.564922557961047289, 89.16775706135234714 ) ) ;
#17120=CARTESIAN_POINT ( 'NONE',  ( 12.14591786802327356, -12.06949235617739191, 45.62609039468567573 ) ) ;
#17121=CARTESIAN_POINT ( 'NONE',  ( -5.719274019375978568, 21.55341960407610458, 115.2072429386476955 ) ) ;
#17122=CARTESIAN_POINT ( 'NONE',  ( 21.55341960407610458, 5.719274019375980345, 78.95724293864769550 ) ) ;
#17123=CARTESIAN_POINT ( 'NONE',  ( -15.80617190586745835, -15.72974639402198527, 36.87390960531435979 ) ) ;
#17124=CARTESIAN_POINT ( 'NONE',  ( -16.55341960407617563, 4.379528057220093196, 63.54275706135234003 ) ) ;
#17125=CARTESIAN_POINT ( 'NONE',  ( -16.51473224551069308, -9.474510206698971260, 66.66557627198102409 ) ) ;
#17126=CARTESIAN_POINT ( 'NONE',  ( 18.67979575497194134, -10.72451020669871369, 45.83442372801901854 ) ) ;
#17127=CARTESIAN_POINT ( 'NONE',  ( -5.049401038297874678, -19.05341960407617918, 109.7927570613523187 ) ) ;
#17128=CARTESIAN_POINT ( 'NONE',  ( -13.97604488694527625, -13.89961937509977652, 111.8739096053143243 ) ) ;
#17129=CARTESIAN_POINT ( 'NONE',  ( 9.474510206698729675, 16.51473224551082808, 22.08442372801899722 ) ) ;
#17130=CARTESIAN_POINT ( 'NONE',  ( -12.06949235617739369, -12.14591786802326823, 39.37609039468567573 ) ) ;
#17131=CARTESIAN_POINT ( 'NONE',  ( 19.05341960407611168, 5.049401038298154454, 98.95724293864766707 ) ) ;
#17132=CARTESIAN_POINT ( 'NONE',  ( 21.52544592524344225, -5.823673210054117533, 108.5405762719810241 ) ) ;
#17133=CARTESIAN_POINT ( 'NONE',  ( 5.153800228976335163, 19.02544592524342804, 59.79057627198100988 ) ) ;
#17135=CARTESIAN_POINT ( 'NONE',  ( -16.52544592524342804, 4.483927247898546575, 81.04057627198102409 ) ) ;
#17136=CARTESIAN_POINT ( 'NONE',  ( -19.03943276465977164, 0.05219959533909376836, 116.2489096053143669 ) ) ;
#17137=CARTESIAN_POINT ( 'NONE',  ( -17.05116617787826527, 6.768360034955678728, 33.65675553259197983 ) ) ;
#17138=CARTESIAN_POINT ( 'NONE',  ( -21.55341960407610458, -5.719274019375992779, 106.4572429386477097 ) ) ;
#17139=CARTESIAN_POINT ( 'NONE',  ( -5.153800228976607833, 19.02544592524334988, 57.70942372801899012 ) ) ;
#17140=CARTESIAN_POINT ( 'NONE',  ( 15.72974639402199770, -15.80617190586745480, 33.12390960531435979 ) ) ;
#17141=CARTESIAN_POINT ( 'NONE',  ( -9.564922557960796823, -16.46253265017161027, 22.08224293864768839 ) ) ;
#17142=CARTESIAN_POINT ( 'NONE',  ( 18.67979575497178502, 10.72451020669898547, 74.16557627198102409 ) ) ;
#17143=CARTESIAN_POINT ( 'NONE',  ( 5.153800228976335163, 19.02544592524342804, 104.7905762719809957 ) ) ;
#17144=CARTESIAN_POINT ( 'NONE',  ( -21.55341960407619339, 5.719274019375674811, 73.54275706135234714 ) ) ;
#17145=CARTESIAN_POINT ( 'NONE',  ( -9.564922557960796823, -16.46253265017161027, 52.08224293864768839 ) ) ;
#17146=CARTESIAN_POINT ( 'NONE',  ( 8.224510206698953496, -14.34966873604960469, 92.91557627198103830 ) ) ;
#17147=CARTESIAN_POINT ( 'NONE',  ( 8.314922557961029526, -14.29746914071037800, 30.41775706135234358 ) ) ;
#17148=CARTESIAN_POINT ( 'NONE',  ( 16.51473224551069308, 9.474510206698969483, 59.16557627198102409 ) ) ;
#17149=CARTESIAN_POINT ( 'NONE',  ( -18.62759615963255300, -10.81492255796106328, 69.16775706135234714 ) ) ;
#17151=CARTESIAN_POINT ( 'NONE',  ( 0.05219959533936267826, -19.03943276465977164, 25.00109039468566152 ) ) ;
#17152=CARTESIAN_POINT ( 'NONE',  ( 19.05341960407617918, -5.049401038297876454, 46.04275706135233293 ) ) ;
#17154=CARTESIAN_POINT ( 'NONE',  ( 5.823673210054444382, -21.52544592524334988, 30.20942372801902565 ) ) ;
#17156=CARTESIAN_POINT ( 'NONE',  ( 13.89961937509957401, 13.97604488694547697, 26.87609039468566507 ) ) ;
#17157=CARTESIAN_POINT ( 'NONE',  ( -16.46253265017160317, 9.564922557960807481, 80.83224293864769550 ) ) ;
#17158=CARTESIAN_POINT ( 'NONE',  ( 19.03943276465977164, -0.05219959533909143690, 73.74890960531435269 ) ) ;
#17159=CARTESIAN_POINT ( 'NONE',  ( -0.05219959533910754901, -16.53943276465976808, 27.49890960531435269 ) ) ;
#17160=CARTESIAN_POINT ( 'NONE',  ( 18.67979575497178502, 10.72451020669898547, 24.16557627198103120 ) ) ;
#17161=CARTESIAN_POINT ( 'NONE',  ( 18.67979575497194134, -10.72451020669871369, 80.83442372801901854 ) ) ;
#17163=CARTESIAN_POINT ( 'NONE',  ( 16.18388926212240619, 7.379444403734400915, 57.93953151366151388 ) ) ;
#17164=CARTESIAN_POINT ( 'NONE',  ( 15.80617190586769283, -15.72974639402175789, 85.62609039468568994 ) ) ;
#17165=CARTESIAN_POINT ( 'NONE',  ( 16.20579543436675252, -7.371946100355224907, 41.93479165828123456 ) ) ;
#17166=CARTESIAN_POINT ( 'NONE',  ( -16.46253265017160317, 9.564922557960807481, 95.83224293864769550 ) ) ;
#17168=CARTESIAN_POINT ( 'NONE',  ( -15.72974639402197994, 15.80617190586746368, 65.62390960531436690 ) ) ;
#17169=CARTESIAN_POINT ( 'NONE',  ( 0.05219959533910956823, 16.53943276465976808, 29.99890960531435979 ) ) ;
#17170=CARTESIAN_POINT ( 'NONE',  ( -4.483927247898539470, -16.52544592524342804, 112.2905762719810241 ) ) ;
#17171=CARTESIAN_POINT ( 'NONE',  ( -0.05219959533909027116, -19.03943276465977164, 92.49890960531436690 ) ) ;
#17172=CARTESIAN_POINT ( 'NONE',  ( -18.67979575497193778, 10.72451020669871902, 113.3344237280190328 ) ) ;
#17173=CARTESIAN_POINT ( 'NONE',  ( -13.97604488694527625, -13.89961937509977652, 21.87390960531435979 ) ) ;
#17174=CARTESIAN_POINT ( 'NONE',  ( -5.823673210054431948, 21.52544592524334988, 72.70942372801901854 ) ) ;
#17175=CARTESIAN_POINT ( 'NONE',  ( 16.46253265017160672, -9.564922557960803928, 113.3322429386476955 ) ) ;
#17176=CARTESIAN_POINT ( 'NONE',  ( 16.55341960407618274, -4.379528057220086978, 106.0427570613523471 ) ) ;
#17177=CARTESIAN_POINT ( 'NONE',  ( -9.564922557961040184, 16.46253265017147172, 67.91775706135233293 ) ) ;
#17178=CARTESIAN_POINT ( 'NONE',  ( 18.22780087662122739, 5.500000000000000888, 66.48236817873106475 ) ) ;
#17179=CARTESIAN_POINT ( 'NONE',  ( -19.02544592524342804, 5.153800228976336051, 106.0405762719810241 ) ) ;
#17180=CARTESIAN_POINT ( 'NONE',  ( -12.14591786802309592, -12.06949235617757132, 86.87390960531438111 ) ) ;
#17181=CARTESIAN_POINT ( 'NONE',  ( -13.89961937509957401, -13.97604488694547875, 64.37609039468567573 ) ) ;
#17182=CARTESIAN_POINT ( 'NONE',  ( 9.474510206698971260, -16.51473224551069308, 77.91557627198103830 ) ) ;
#17183=CARTESIAN_POINT ( 'NONE',  ( -8.314922557960811034, -14.29746914071050412, 57.08224293864769550 ) ) ;
#17184=CARTESIAN_POINT ( 'NONE',  ( 5.153800228976615827, -19.02544592524334988, 95.20942372801897591 ) ) ;
#17185=CARTESIAN_POINT ( 'NONE',  ( 5.719274019375991003, -21.55341960407610458, 52.70724293864769550 ) ) ;
#17187=CARTESIAN_POINT ( 'NONE',  ( 9.474510206698971260, -16.51473224551069308, 22.91557627198102765 ) ) ;
#17188=CARTESIAN_POINT ( 'NONE',  ( -16.21995358207306737, -7.366697692864124569, 30.06448998487844904 ) ) ;
#17189=CARTESIAN_POINT ( 'NONE',  ( -19.03943276465977164, 0.05219959533909376836, 66.24890960531436690 ) ) ;
#17190=CARTESIAN_POINT ( 'NONE',  ( -10.81492255796078084, -18.62759615963271287, 82.08224293864768129 ) ) ;
#17191=CARTESIAN_POINT ( 'NONE',  ( -4.483927247898782831, 16.52544592524335698, 97.70942372801904696 ) ) ;
#17192=CARTESIAN_POINT ( 'NONE',  ( 16.46253265017160672, -9.564922557960803928, 73.33224293864769550 ) ) ;
#17193=CARTESIAN_POINT ( 'NONE',  ( 13.89961937509957401, 13.97604488694547697, 51.87609039468566863 ) ) ;
#17194=CARTESIAN_POINT ( 'NONE',  ( 10.72451020669871369, 18.67979575497193778, 77.08442372801901854 ) ) ;
#17195=CARTESIAN_POINT ( 'NONE',  ( -10.72451020669898014, 18.67979575497178502, 60.41557627198102409 ) ) ;
#17196=CARTESIAN_POINT ( 'NONE',  ( 10.72451020669898902, -18.67979575497178502, 22.91557627198102765 ) ) ;
#17197=CARTESIAN_POINT ( 'NONE',  ( -13.89961937509977652, 13.97604488694528158, 40.62390960531435979 ) ) ;
#17198=CARTESIAN_POINT ( 'NONE',  ( 12.06949235617739724, 12.14591786802326823, 96.87609039468568994 ) ) ;
#17199=CARTESIAN_POINT ( 'NONE',  ( -12.14591786802326823, 12.06949235617739902, 28.12609039468568284 ) ) ;
#17201=CARTESIAN_POINT ( 'NONE',  ( -15.80617190586768217, 15.72974639402176855, 98.12609039468570415 ) ) ;
#17202=CARTESIAN_POINT ( 'NONE',  ( 4.379528057220339221, -16.55341960407611168, 62.70724293864769550 ) ) ;
#17204=CARTESIAN_POINT ( 'NONE',  ( -15.72974639402197994, 15.80617190586746368, 90.62390960531436690 ) ) ;
#17205=CARTESIAN_POINT ( 'NONE',  ( 21.52544592524344225, -5.823673210054117533, 88.54057627198103830 ) ) ;
#17207=CARTESIAN_POINT ( 'NONE',  ( -18.62759615963270932, 10.81492255796079327, 40.83224293864769550 ) ) ;
#17208=CARTESIAN_POINT ( 'NONE',  ( 12.14591786802327356, -12.06949235617739191, 85.62609039468568994 ) ) ;
#17209=CARTESIAN_POINT ( 'NONE',  ( -0.05219959533910754901, -16.53943276465976808, 92.49890960531436690 ) ) ;
#17210=CARTESIAN_POINT ( 'NONE',  ( 19.02544592524343514, -5.153800228976328945, 48.54057627198103120 ) ) ;
#17211=FILL_AREA_STYLE ('',( #30390 ) ) ;
#17213=CARTESIAN_POINT ( 'NONE',  ( -8.314922557961024197, 14.29746914071037800, 92.91775706135236135 ) ) ;
#17214=CARTESIAN_POINT ( 'NONE',  ( 21.52544592524334988, 5.823673210054432836, 36.45942372801901143 ) ) ;
#17215=CARTESIAN_POINT ( 'NONE',  ( -13.89961937509977652, 13.97604488694528158, 100.6239096053143669 ) ) ;
#17216=CARTESIAN_POINT ( 'NONE',  ( -10.72451020669870658, -18.67979575497194134, 64.58442372801900433 ) ) ;
#17218=CARTESIAN_POINT ( 'NONE',  ( -19.02544592524342804, 5.153800228976336051, 31.04057627198102409 ) ) ;
#17219=EDGE_CURVE ( 'NONE', #15494, #90405, #9588, .T. ) ;
#17221=CARTESIAN_POINT ( 'NONE',  ( -15.72974639402176322, -15.80617190586768395, 64.37609039468568994 ) ) ;
#17222=CARTESIAN_POINT ( 'NONE',  ( 13.89961937509977652, -13.97604488694527269, 48.12390960531435979 ) ) ;
#17223=FACE_OUTER_BOUND ( 'NONE', #41283, .T. ) ;
#17224=CARTESIAN_POINT ( 'NONE',  ( 16.51473224551069308, 9.474510206698969483, 94.16557627198103830 ) ) ;
#17225=CARTESIAN_POINT ( 'NONE',  ( 5.049401038297881783, 19.05341960407617563, 62.29275706135234003 ) ) ;
#17226=CARTESIAN_POINT ( 'NONE',  ( 10.72451020669871369, 18.67979575497193778, 47.08442372801901854 ) ) ;
#17227=CARTESIAN_POINT ( 'NONE',  ( -16.46253265017146816, -9.564922557961047289, 64.16775706135233293 ) ) ;
#17228=CARTESIAN_POINT ( 'NONE',  ( -0.05219959533909027116, -19.03943276465977164, 42.49890960531435269 ) ) ;
#17229=CARTESIAN_POINT ( 'NONE',  ( 12.14591786802327356, -12.06949235617739191, 100.6260903946857184 ) ) ;
#17230=CARTESIAN_POINT ( 'NONE',  ( 5.153800228976615827, -19.02544592524334988, 70.20942372801899012 ) ) ;
#17231=CARTESIAN_POINT ( 'NONE',  ( -16.53943276465976808, -0.05219959533934237506, 113.7510903946856757 ) ) ;
#17232=CARTESIAN_POINT ( 'NONE',  ( -9.564922557961040184, 16.46253265017147172, 47.91775706135233293 ) ) ;
#17233=CARTESIAN_POINT ( 'NONE',  ( -13.89961937509977652, 13.97604488694528158, 100.6239096053143669 ) ) ;
#17234=CARTESIAN_POINT ( 'NONE',  ( 21.52544592524334988, 5.823673210054432836, 111.4594237280190328 ) ) ;
#17235=CARTESIAN_POINT ( 'NONE',  ( 5.153800228976615827, -19.02544592524334988, 25.20942372801900433 ) ) ;
#17236=CARTESIAN_POINT ( 'NONE',  ( -9.474510206698964154, 16.51473224551069663, 30.41557627198102054 ) ) ;
#17237=CARTESIAN_POINT ( 'NONE',  ( -10.72451020669870658, -18.67979575497194134, 94.58442372801901854 ) ) ;
#17238=CARTESIAN_POINT ( 'NONE',  ( 4.483927247898790824, -16.52544592524335698, 35.20942372801901854 ) ) ;
#17239=CARTESIAN_POINT ( 'NONE',  ( 13.97604488694527802, 13.89961937509977652, 89.37390960531436690 ) ) ;
#17240=VECTOR ( 'NONE', #34661, 1000.000000000000000 ) ;
#17242=CARTESIAN_POINT ( 'NONE',  ( -19.02544592524342804, 5.153800228976336051, 76.04057627198102409 ) ) ;
#17244=CARTESIAN_POINT ( 'NONE',  ( 5.153800228976615827, -19.02544592524334988, 85.20942372801900433 ) ) ;
#17245=CARTESIAN_POINT ( 'NONE',  ( -19.03943276465977164, 0.05219959533909376836, 111.2489096053143669 ) ) ;
#17246=CARTESIAN_POINT ( 'NONE',  ( 0.05219959533937995610, -21.53943276465977519, 100.0010903946857042 ) ) ;
#17247=CARTESIAN_POINT ( 'NONE',  ( -12.06949235617756955, 12.14591786802309770, 95.62390960531436690 ) ) ;
#17248=CARTESIAN_POINT ( 'NONE',  ( 16.46253265017160672, -9.564922557960803928, 23.33224293864769194 ) ) ;
#17249=CARTESIAN_POINT ( 'NONE',  ( -15.72974639402197994, 15.80617190586746368, 45.62390960531436690 ) ) ;
#17250=CARTESIAN_POINT ( 'NONE',  ( -21.53943276465977519, 0.05219959533907696930, 31.24890960531435979 ) ) ;
#17251=CARTESIAN_POINT ( 'NONE',  ( -19.03943276465977164, 0.05219959533909376836, 26.24890960531435624 ) ) ;
#17253=CARTESIAN_POINT ( 'NONE',  ( 0.05219959533936267826, -19.03943276465977164, 60.00109039468566863 ) ) ;
#17254=CARTESIAN_POINT ( 'NONE',  ( 14.34966873604960469, 8.224510206698951720, 39.16557627198102409 ) ) ;
#17255=CARTESIAN_POINT ( 'NONE',  ( -16.51473224551069308, -9.474510206698971260, 111.6655762719810383 ) ) ;
#17256=CARTESIAN_POINT ( 'NONE',  ( -21.55341960407619339, 5.719274019375674811, 73.54275706135234714 ) ) ;
#17257=CARTESIAN_POINT ( 'NONE',  ( 15.72974639402199770, -15.80617190586745480, 73.12390960531436690 ) ) ;
#17258=CARTESIAN_POINT ( 'NONE',  ( 15.72974639402176855, 15.80617190586768217, 46.87609039468568994 ) ) ;
#17259=CARTESIAN_POINT ( 'NONE',  ( 21.52544592524344225, -5.823673210054117533, 98.54057627198105251 ) ) ;
#17260=CARTESIAN_POINT ( 'NONE',  ( -21.55341960407619339, 5.719274019375674811, 53.54275706135234714 ) ) ;
#17261=CARTESIAN_POINT ( 'NONE',  ( -0.05219959533909027116, -19.03943276465977164, 32.49890960531435979 ) ) ;
#17262=CARTESIAN_POINT ( 'NONE',  ( 5.049401038298161559, -19.05341960407611168, 87.70724293864769550 ) ) ;
#17263=CARTESIAN_POINT ( 'NONE',  ( -14.34966873604972548, 8.224510206698743886, 83.33442372801903275 ) ) ;
#17264=CARTESIAN_POINT ( 'NONE',  ( 0.05219959533910956823, 16.53943276465976808, 109.9989096053143527 ) ) ;
#17265=CARTESIAN_POINT ( 'NONE',  ( 16.46253265017160672, -9.564922557960803928, 108.3322429386476955 ) ) ;
#17266=CARTESIAN_POINT ( 'NONE',  ( 0.05219959533910956823, 16.53943276465976808, 59.99890960531436690 ) ) ;
#17267=CARTESIAN_POINT ( 'NONE',  ( 14.34966873604960469, 8.224510206698951720, 24.16557627198103120 ) ) ;
#17268=CARTESIAN_POINT ( 'NONE',  ( -13.89961937509977652, 13.97604488694528158, 65.62390960531436690 ) ) ;
#17269=CARTESIAN_POINT ( 'NONE',  ( -0.05219959533909027116, -19.03943276465977164, 37.49890960531436690 ) ) ;
#17270=CARTESIAN_POINT ( 'NONE',  ( 18.67979575497178502, 10.72451020669898547, 49.16557627198102409 ) ) ;
#17271=CARTESIAN_POINT ( 'NONE',  ( -9.474510206698720793, -16.51473224551083518, 39.58442372801899722 ) ) ;
#17272=CARTESIAN_POINT ( 'NONE',  ( -17.72662750342727733, -5.500000000000018652, 86.40179492283746754 ) ) ;
#17273=CARTESIAN_POINT ( 'NONE',  ( 0.05219959533910956823, 16.53943276465976808, 34.99890960531435979 ) ) ;
#17274=CARTESIAN_POINT ( 'NONE',  ( 16.51473224551069308, 9.474510206698969483, 114.1655762719810241 ) ) ;
#17275=CARTESIAN_POINT ( 'NONE',  ( 18.67979575497194134, -10.72451020669871369, 55.83442372801901854 ) ) ;
#17277=CARTESIAN_POINT ( 'NONE',  ( -12.14591786802326823, 12.06949235617739902, 68.12609039468567573 ) ) ;
#17278=CARTESIAN_POINT ( 'NONE',  ( 19.02544592524334988, 5.153800228976608722, 66.45942372801899012 ) ) ;
#17279=CARTESIAN_POINT ( 'NONE',  ( -4.483927247898539470, -16.52544592524342804, 47.29057627198103120 ) ) ;
#17280=CARTESIAN_POINT ( 'NONE',  ( 16.61371651742598132, -7.165104196376200996, 51.35415069993000259 ) ) ;
#17281=CARTESIAN_POINT ( 'NONE',  ( 14.29746914071049879, -8.314922557960816363, 23.33224293864769194 ) ) ;
#17282=CARTESIAN_POINT ( 'NONE',  ( -13.97604488694527625, -13.89961937509977652, 36.87390960531436690 ) ) ;
#17283=CARTESIAN_POINT ( 'NONE',  ( -16.46253265017160317, 9.564922557960807481, 55.83224293864769550 ) ) ;
#17284=CARTESIAN_POINT ( 'NONE',  ( -5.049401038298153566, 19.05341960407611168, 25.20724293864768484 ) ) ;
#17285=CARTESIAN_POINT ( 'NONE',  ( -5.719274019375665041, -21.55341960407619695, 34.79275706135235424 ) ) ;
#17286=CARTESIAN_POINT ( 'NONE',  ( 19.05341960407611168, 5.049401038298154454, 53.95724293864770260 ) ) ;
#17287=CARTESIAN_POINT ( 'NONE',  ( 19.03943276465977164, -0.05219959533909143690, 113.7489096053143669 ) ) ;
#17288=CARTESIAN_POINT ( 'NONE',  ( -13.89961937509977652, 13.97604488694528158, 45.62390960531433848 ) ) ;
#17289=CARTESIAN_POINT ( 'NONE',  ( -10.81492255796078084, -18.62759615963271287, 27.08224293864769550 ) ) ;
#17290=CARTESIAN_POINT ( 'NONE',  ( -18.62759615963255300, -10.81492255796106328, 54.16775706135235424 ) ) ;
#17291=CARTESIAN_POINT ( 'NONE',  ( -13.89961937509977652, 13.97604488694528158, 25.62390960531434558 ) ) ;
#17292=CARTESIAN_POINT ( 'NONE',  ( -15.80617190586745835, -15.72974639402198527, 26.87390960531435979 ) ) ;
#17293=AXIS2_PLACEMENT_3D ( 'NONE', #144454, #3950, #112137 ) ;
#17294=CARTESIAN_POINT ( 'NONE',  ( 4.483927247898790824, -16.52544592524335698, 75.20942372801901854 ) ) ;
#17295=CARTESIAN_POINT ( 'NONE',  ( -18.62759615963255300, -10.81492255796106328, 109.1677570613523613 ) ) ;
#17296=CARTESIAN_POINT ( 'NONE',  ( 8.224510206698742110, 14.34966873604972548, 67.08442372801901854 ) ) ;
#17297=CARTESIAN_POINT ( 'NONE',  ( 5.153800228976335163, 19.02544592524342804, 109.7905762719810099 ) ) ;
#17298=CARTESIAN_POINT ( 'NONE',  ( -16.53943276465976808, -0.05219959533934237506, 48.75109039468568284 ) ) ;
#17299=CARTESIAN_POINT ( 'NONE',  ( -14.34966873604972548, 8.224510206698743886, 28.33442372801902209 ) ) ;
#17300=CARTESIAN_POINT ( 'NONE',  ( -8.224510206698735004, -14.34966873604973081, 99.58442372801900433 ) ) ;
#17301=CARTESIAN_POINT ( 'NONE',  ( 15.80617190586769283, -15.72974639402175789, 60.62609039468567573 ) ) ;
#17302=CARTESIAN_POINT ( 'NONE',  ( 16.51473224551083163, -9.474510206698727899, 105.8344237280190043 ) ) ;
#17303=CARTESIAN_POINT ( 'NONE',  ( 21.52544592524344225, -5.823673210054117533, 108.5405762719810241 ) ) ;
#17304=CARTESIAN_POINT ( 'NONE',  ( -14.29746914071037622, -8.314922557961029526, 19.16775706135234714 ) ) ;
#17305=CARTESIAN_POINT ( 'NONE',  ( -4.379528057220086978, -16.55341960407618274, 84.79275706135234714 ) ) ;
#17307=CARTESIAN_POINT ( 'NONE',  ( 5.719274019375673035, 21.55341960407619339, 82.29275706135234714 ) ) ;
#17308=CARTESIAN_POINT ( 'NONE',  ( 5.153800228976615827, -19.02544592524334988, 80.20942372801901854 ) ) ;
#17309=CARTESIAN_POINT ( 'NONE',  ( 4.483927247898545687, 16.52544592524342804, 44.79057627198103120 ) ) ;
#17310=CARTESIAN_POINT ( 'NONE',  ( 12.14591786802309770, 12.06949235617756955, 39.37390960531436690 ) ) ;
#17311=CARTESIAN_POINT ( 'NONE',  ( -8.314922557960811034, -14.29746914071050412, 102.0822429386476955 ) ) ;
#17312=CARTESIAN_POINT ( 'NONE',  ( -0.05219959533936034679, 19.03943276465977164, 42.50109039468566152 ) ) ;
#17313=CARTESIAN_POINT ( 'NONE',  ( 16.79531203550682861, -7.028104445595345418, 56.24755011779544134 ) ) ;
#17314=CARTESIAN_POINT ( 'NONE',  ( 0.05219959533937995610, -21.53943276465977519, 35.00109039468568284 ) ) ;
#17315=CARTESIAN_POINT ( 'NONE',  ( 9.474510206698729675, 16.51473224551082808, 112.0844237280190043 ) ) ;
#17317=CARTESIAN_POINT ( 'NONE',  ( 16.46253265017160672, -9.564922557960803928, 98.33224293864769550 ) ) ;
#17318=CARTESIAN_POINT ( 'NONE',  ( 10.72451020669898902, -18.67979575497178502, 52.91557627198103830 ) ) ;
#17319=CARTESIAN_POINT ( 'NONE',  ( 5.153800228976335163, 19.02544592524342804, 84.79057627198099567 ) ) ;
#17320=CARTESIAN_POINT ( 'NONE',  ( 18.62759615963271287, -10.81492255796078972, 63.33224293864770260 ) ) ;
#17321=CARTESIAN_POINT ( 'NONE',  ( 8.224510206698953496, -14.34966873604960469, 107.9155762719810241 ) ) ;
#17322=CARTESIAN_POINT ( 'NONE',  ( -16.46253265017160317, 9.564922557960807481, 70.83224293864770971 ) ) ;
#17323=CARTESIAN_POINT ( 'NONE',  ( 19.05341960407611168, 5.049401038298154454, 23.95724293864769194 ) ) ;
#17324=CARTESIAN_POINT ( 'NONE',  ( -5.823673210054431948, 21.52544592524334988, 32.70942372801900433 ) ) ;
#17325=CARTESIAN_POINT ( 'NONE',  ( -21.55341960407619339, 5.719274019375674811, 78.54275706135236135 ) ) ;
#17326=CARTESIAN_POINT ( 'NONE',  ( 8.314922557961029526, -14.29746914071037800, 85.41775706135236135 ) ) ;
#17327=CARTESIAN_POINT ( 'NONE',  ( -15.72974639402176322, -15.80617190586768395, 24.37609039468567573 ) ) ;
#17328=CARTESIAN_POINT ( 'NONE',  ( -21.53943276465977519, -0.05219959533937600094, 28.75109039468567929 ) ) ;
#17329=CARTESIAN_POINT ( 'NONE',  ( 0.05219959533936267826, -19.03943276465977164, 60.00109039468566863 ) ) ;
#17330=CARTESIAN_POINT ( 'NONE',  ( -0.05219959533909027116, -19.03943276465977164, 82.49890960531436690 ) ) ;
#17331=CARTESIAN_POINT ( 'NONE',  ( -10.81492255796105439, 18.62759615963255655, 82.91775706135234714 ) ) ;
#17332=CARTESIAN_POINT ( 'NONE',  ( 18.62759615963271287, -10.81492255796078972, 83.33224293864769550 ) ) ;
#17333=CARTESIAN_POINT ( 'NONE',  ( -8.224510206698948167, 14.34966873604960824, 65.41557627198102409 ) ) ;
#17334=CARTESIAN_POINT ( 'NONE',  ( -10.72451020669870658, -18.67979575497194134, 99.58442372801900433 ) ) ;
#17335=CARTESIAN_POINT ( 'NONE',  ( 16.52544592524342804, -4.483927247898539470, 88.54057627198103830 ) ) ;
#17336=CARTESIAN_POINT ( 'NONE',  ( -13.97604488694527625, -13.89961937509977652, 41.87390960531435979 ) ) ;
#17337=CARTESIAN_POINT ( 'NONE',  ( 0.05219959533936267826, -19.03943276465977164, 70.00109039468566152 ) ) ;
#17338=CARTESIAN_POINT ( 'NONE',  ( -4.379528057220328563, 16.55341960407611168, 35.20724293864768839 ) ) ;
#17339=CARTESIAN_POINT ( 'NONE',  ( 5.719274019375673035, 21.55341960407619339, 92.29275706135236135 ) ) ;
#17340=CARTESIAN_POINT ( 'NONE',  ( -13.89961937509977652, 13.97604488694528158, 90.62390960531432427 ) ) ;
#17341=CARTESIAN_POINT ( 'NONE',  ( 9.564922557961047289, -16.46253265017146816, 60.41775706135233293 ) ) ;
#17342=CARTESIAN_POINT ( 'NONE',  ( 21.53943276465977519, -0.05219959533907433946, 63.74890960531435979 ) ) ;
#17343=CARTESIAN_POINT ( 'NONE',  ( 15.80617190586746368, 15.72974639402197994, 114.3739096053143527 ) ) ;
#17344=CARTESIAN_POINT ( 'NONE',  ( 16.55341960407618274, -4.379528057220086978, 21.04275706135234714 ) ) ;
#17345=CARTESIAN_POINT ( 'NONE',  ( 4.483927247898790824, -16.52544592524335698, 75.20942372801901854 ) ) ;
#17346=CARTESIAN_POINT ( 'NONE',  ( 17.50000000000001066, 5.622605283950889543, 63.81207310596114013 ) ) ;
#17347=CARTESIAN_POINT ( 'NONE',  ( -5.823673210054431948, 21.52544592524334988, 22.70942372801901499 ) ) ;
#17348=CARTESIAN_POINT ( 'NONE',  ( 8.314922557960818139, 14.29746914071049879, 99.58224293864770971 ) ) ;
#17350=CARTESIAN_POINT ( 'NONE',  ( -0.05219959533934338120, 16.53943276465976808, 37.50109039468568284 ) ) ;
#17352=CARTESIAN_POINT ( 'NONE',  ( -5.823673210054116645, -21.52544592524344225, 57.29057627198103120 ) ) ;
#17353=CARTESIAN_POINT ( 'NONE',  ( 16.53943276465976808, 0.05219959533934440121, 111.2510903946856899 ) ) ;
#17354=CARTESIAN_POINT ( 'NONE',  ( 12.06949235617739724, 12.14591786802326823, 41.87609039468568284 ) ) ;
#17355=CARTESIAN_POINT ( 'NONE',  ( 9.474510206698971260, -16.51473224551069308, 37.91557627198102409 ) ) ;
#17356=CARTESIAN_POINT ( 'NONE',  ( 8.314922557961029526, -14.29746914071037800, 85.41775706135236135 ) ) ;
#17357=CARTESIAN_POINT ( 'NONE',  ( -19.03943276465977164, -0.05219959533935918106, 78.75109039468567573 ) ) ;
#17358=CARTESIAN_POINT ( 'NONE',  ( -10.72451020669898014, 18.67979575497178502, 75.41557627198102409 ) ) ;
#17359=CARTESIAN_POINT ( 'NONE',  ( 16.53943276465976808, 0.05219959533934440121, 96.25109039468568994 ) ) ;
#17360=CARTESIAN_POINT ( 'NONE',  ( -10.72451020669870658, -18.67979575497194134, 79.58442372801903275 ) ) ;
#17361=CARTESIAN_POINT ( 'NONE',  ( -10.81492255796078084, -18.62759615963271287, 67.08224293864770971 ) ) ;
#17362=CARTESIAN_POINT ( 'NONE',  ( -21.52544592524343514, 5.823673210054127303, 51.04057627198103120 ) ) ;
#17364=CARTESIAN_POINT ( 'NONE',  ( 8.314922557961029526, -14.29746914071037800, 75.41775706135233293 ) ) ;
#17365=CARTESIAN_POINT ( 'NONE',  ( 21.52544592524344225, -5.823673210054117533, 43.54057627198103830 ) ) ;
#17367=CARTESIAN_POINT ( 'NONE',  ( 5.153800228976335163, 19.02544592524342804, 114.7905762719810241 ) ) ;
#17369=CARTESIAN_POINT ( 'NONE',  ( 5.049401038298161559, -19.05341960407611168, 32.70724293864768129 ) ) ;
#17370=CARTESIAN_POINT ( 'NONE',  ( -15.72974639402197994, 15.80617190586746368, 55.62390960531436690 ) ) ;
#17371=CARTESIAN_POINT ( 'NONE',  ( -14.34966873604972548, 8.224510206698743886, 108.3344237280190185 ) ) ;
#17372=CARTESIAN_POINT ( 'NONE',  ( 18.67979575497194134, -10.72451020669871369, 40.83442372801901854 ) ) ;
#17373=CARTESIAN_POINT ( 'NONE',  ( -13.97604488694547697, 13.89961937509957934, 98.12609039468566152 ) ) ;
#17374=CARTESIAN_POINT ( 'NONE',  ( -4.379528057220328563, 16.55341960407611168, 115.2072429386476955 ) ) ;
#17375=CARTESIAN_POINT ( 'NONE',  ( 12.14591786802327356, -12.06949235617739191, 20.62609039468568639 ) ) ;
#17376=CARTESIAN_POINT ( 'NONE',  ( 5.153800228976335163, 19.02544592524342804, 39.79057627198100988 ) ) ;
#17378=CARTESIAN_POINT ( 'NONE',  ( -19.05341960407611168, -5.049401038298163336, 96.45724293864769550 ) ) ;
#17379=CARTESIAN_POINT ( 'NONE',  ( 14.29746914071037800, 8.314922557961029526, 81.66775706135236135 ) ) ;
#17380=CARTESIAN_POINT ( 'NONE',  ( -0.05219959533936034679, 19.03943276465977164, 72.50109039468566152 ) ) ;
#17381=CARTESIAN_POINT ( 'NONE',  ( 0.05219959533936267826, -19.03943276465977164, 25.00109039468566152 ) ) ;
#17382=CARTESIAN_POINT ( 'NONE',  ( -5.823673210054116645, -21.52544592524344225, 67.29057627198103830 ) ) ;
#17383=CARTESIAN_POINT ( 'NONE',  ( 12.14591786802327356, -12.06949235617739191, 80.62609039468567573 ) ) ;
#17385=CARTESIAN_POINT ( 'NONE',  ( 19.05341960407617918, -5.049401038297876454, 86.04275706135233293 ) ) ;
#17386=CARTESIAN_POINT ( 'NONE',  ( -9.474510206698964154, 16.51473224551069663, 35.41557627198102409 ) ) ;
#17387=CARTESIAN_POINT ( 'NONE',  ( -0.05219959533909027116, -19.03943276465977164, 77.49890960531435269 ) ) ;
#17388=CARTESIAN_POINT ( 'NONE',  ( 10.72451020669871369, 18.67979575497193778, 52.08442372801901854 ) ) ;
#17389=CARTESIAN_POINT ( 'NONE',  ( -5.153800228976328057, -19.02544592524343514, 52.29057627198100988 ) ) ;
#17390=CARTESIAN_POINT ( 'NONE',  ( -19.02544592524334988, -5.153800228976617603, 68.95942372801896170 ) ) ;
#17392=CARTESIAN_POINT ( 'NONE',  ( 13.97604488694527802, 13.89961937509977652, 114.3739096053143669 ) ) ;
#17393=CARTESIAN_POINT ( 'NONE',  ( -14.29746914071049879, 8.314922557960819915, 60.83224293864769550 ) ) ;
#17394=CARTESIAN_POINT ( 'NONE',  ( 21.53943276465977519, -0.05219959533907433946, 58.74890960531436690 ) ) ;
#17396=CARTESIAN_POINT ( 'NONE',  ( -19.02544592524334988, -5.153800228976617603, 43.95942372801899012 ) ) ;
#17398=CARTESIAN_POINT ( 'NONE',  ( 19.03943276465977164, -0.05219959533909143690, 58.74890960531435979 ) ) ;
#17399=CARTESIAN_POINT ( 'NONE',  ( -5.049401038298153566, 19.05341960407611168, 80.20724293864769550 ) ) ;
#17400=CARTESIAN_POINT ( 'NONE',  ( -4.379528057220086978, -16.55341960407618274, 54.79275706135235424 ) ) ;
#17403=CARTESIAN_POINT ( 'NONE',  ( -12.14591786802326823, 12.06949235617739902, 93.12609039468568994 ) ) ;
#17405=CARTESIAN_POINT ( 'NONE',  ( 12.14591786802327356, -12.06949235617739191, 65.62609039468568994 ) ) ;
#17406=CARTESIAN_POINT ( 'NONE',  ( 0.05219959533934541429, -16.53943276465976808, 40.00109039468567573 ) ) ;
#17407=CARTESIAN_POINT ( 'NONE',  ( -19.03943276465977164, 0.05219959533909376836, 56.24890960531435979 ) ) ;
#17409=CARTESIAN_POINT ( 'NONE',  ( 18.62759615963255655, 10.81492255796105972, 56.66775706135235424 ) ) ;
#17410=CARTESIAN_POINT ( 'NONE',  ( 16.51473224551083163, -9.474510206698727899, 65.83442372801900433 ) ) ;
#17411=CARTESIAN_POINT ( 'NONE',  ( -10.72451020669870658, -18.67979575497194134, 109.5844237280190328 ) ) ;
#17412=CARTESIAN_POINT ( 'NONE',  ( 5.049401038298161559, -19.05341960407611168, 27.70724293864769550 ) ) ;
#17414=CARTESIAN_POINT ( 'NONE',  ( 10.81492255796078972, 18.62759615963270932, 59.58224293864770260 ) ) ;
#17415=CARTESIAN_POINT ( 'NONE',  ( -0.05219959533909027116, -19.03943276465977164, 112.4989096053143669 ) ) ;
#17416=CARTESIAN_POINT ( 'NONE',  ( -16.53943276465976808, 0.05219959533911058130, 96.24890960531435269 ) ) ;
#17417=CARTESIAN_POINT ( 'NONE',  ( -8.314922557961024197, 14.29746914071037800, 42.91775706135235424 ) ) ;
#17419=CARTESIAN_POINT ( 'NONE',  ( 12.06949235617757843, -12.14591786802309237, 28.12390960531435979 ) ) ;
#17420=ORIENTED_EDGE ( 'NONE', *, *, #28410, .F. ) ;
#17421=CARTESIAN_POINT ( 'NONE',  ( 10.81492255796078972, 18.62759615963270932, 109.5822429386476955 ) ) ;
#17422=CARTESIAN_POINT ( 'NONE',  ( 12.06949235617757843, -12.14591786802309237, 33.12390960531435979 ) ) ;
#17423=CARTESIAN_POINT ( 'NONE',  ( 13.89961937509977652, -13.97604488694527269, 108.1239096053143669 ) ) ;
#17424=CARTESIAN_POINT ( 'NONE',  ( 16.46253265017146816, 9.564922557961045513, 101.6677570613523329 ) ) ;
#17425=CARTESIAN_POINT ( 'NONE',  ( -5.153800228976607833, 19.02544592524334988, 32.70942372801899722 ) ) ;
#17426=CARTESIAN_POINT ( 'NONE',  ( -4.379528057220328563, 16.55341960407611168, 35.20724293864768839 ) ) ;
#17427=CARTESIAN_POINT ( 'NONE',  ( -10.72451020669898014, 18.67979575497178502, 105.4155762719810383 ) ) ;
#17428=CARTESIAN_POINT ( 'NONE',  ( 0.05219959533907565091, 21.53943276465977519, 59.99890960531436690 ) ) ;
#17429=CARTESIAN_POINT ( 'NONE',  ( 13.97604488694527802, 13.89961937509977652, 79.37390960531435269 ) ) ;
#17430=CARTESIAN_POINT ( 'NONE',  ( 0.05219959533910956823, 16.53943276465976808, 49.99890960531437401 ) ) ;
#17431=CARTESIAN_POINT ( 'NONE',  ( 16.51473224551069308, 9.474510206698969483, 84.16557627198102409 ) ) ;
#17434=CARTESIAN_POINT ( 'NONE',  ( -19.03943276465977164, -0.05219959533935918106, 43.75109039468566863 ) ) ;
#17435=CARTESIAN_POINT ( 'NONE',  ( 10.72451020669898902, -18.67979575497178502, 97.91557627198103830 ) ) ;
#17436=CARTESIAN_POINT ( 'NONE',  ( -16.53943276465976808, 0.05219959533911058130, 96.24890960531435269 ) ) ;
#17437=CARTESIAN_POINT ( 'NONE',  ( 5.823673210054444382, -21.52544592524334988, 35.20942372801901854 ) ) ;
#17439=CARTESIAN_POINT ( 'NONE',  ( -4.379528057220328563, 16.55341960407611168, 25.20724293864769550 ) ) ;
#17440=CARTESIAN_POINT ( 'NONE',  ( -5.049401038298153566, 19.05341960407611168, 30.20724293864768839 ) ) ;
#17441=CARTESIAN_POINT ( 'NONE',  ( -9.474510206698964154, 16.51473224551069663, 90.41557627198103830 ) ) ;
#17442=CARTESIAN_POINT ( 'NONE',  ( 0.05219959533907565091, 21.53943276465977519, 64.99890960531435269 ) ) ;
#17443=CARTESIAN_POINT ( 'NONE',  ( -18.56197773271731677, 5.499999999999904077, 43.55066217314453070 ) ) ;
#17444=CARTESIAN_POINT ( 'NONE',  ( 13.89961937509977652, -13.97604488694527269, 28.12390960531435624 ) ) ;
#17445=CARTESIAN_POINT ( 'NONE',  ( 10.72451020669898902, -18.67979575497178502, 52.91557627198103830 ) ) ;
#17446=CARTESIAN_POINT ( 'NONE',  ( -21.52544592524334988, -5.823673210054445271, 68.95942372801901854 ) ) ;
#17448=CARTESIAN_POINT ( 'NONE',  ( -16.52544592524335698, -4.483927247898792601, 63.95942372801901854 ) ) ;
#17449=CARTESIAN_POINT ( 'NONE',  ( -5.153800228976328057, -19.02544592524343514, 62.29057627198100988 ) ) ;
#17450=CARTESIAN_POINT ( 'NONE',  ( 19.02544592524343514, -5.153800228976328945, 58.54057627198102409 ) ) ;
#17452=CARTESIAN_POINT ( 'NONE',  ( -18.67979575497193778, 10.72451020669871902, 108.3344237280190185 ) ) ;
#17453=CARTESIAN_POINT ( 'NONE',  ( -4.379528057220086978, -16.55341960407618274, 74.79275706135234714 ) ) ;
#17454=CARTESIAN_POINT ( 'NONE',  ( -21.52544592524334988, -5.823673210054445271, 98.95942372801903275 ) ) ;
#17455=CARTESIAN_POINT ( 'NONE',  ( -9.564922557960796823, -16.46253265017161027, 62.08224293864769550 ) ) ;
#17456=CARTESIAN_POINT ( 'NONE',  ( 10.81492255796078972, 18.62759615963270932, 29.58224293864769905 ) ) ;
#17457=CARTESIAN_POINT ( 'NONE',  ( -16.51473224551082808, 9.474510206698731452, 108.3344237280190043 ) ) ;
#17458=CARTESIAN_POINT ( 'NONE',  ( -5.719274019375665041, -21.55341960407619695, 79.79275706135236135 ) ) ;
#17459=CARTESIAN_POINT ( 'NONE',  ( 16.53943276465976808, 0.05219959533934440121, 46.25109039468567573 ) ) ;
#17460=CARTESIAN_POINT ( 'NONE',  ( 18.62759615963271287, -10.81492255796078972, 93.33224293864769550 ) ) ;
#17461=CARTESIAN_POINT ( 'NONE',  ( 13.89961937509957401, 13.97604488694547697, 96.87609039468566152 ) ) ;
#17462=CARTESIAN_POINT ( 'NONE',  ( 16.51473224551069308, 9.474510206698969483, 74.16557627198103830 ) ) ;
#17463=CARTESIAN_POINT ( 'NONE',  ( -13.89961937509957401, -13.97604488694547875, 109.3760903946856331 ) ) ;
#17464=CARTESIAN_POINT ( 'NONE',  ( -13.89961937509977652, 13.97604488694528158, 35.62390960531435269 ) ) ;
#17466=CARTESIAN_POINT ( 'NONE',  ( 8.314922557961029526, -14.29746914071037800, 20.41775706135234714 ) ) ;
#17467=CARTESIAN_POINT ( 'NONE',  ( 12.14591786802309770, 12.06949235617756955, 69.37390960531436690 ) ) ;
#17468=CARTESIAN_POINT ( 'NONE',  ( -12.06949235617739369, -12.14591786802326823, 69.37609039468567573 ) ) ;
#17469=CARTESIAN_POINT ( 'NONE',  ( -0.05219959533937732626, 21.53943276465977519, 32.50109039468568284 ) ) ;
#17470=CARTESIAN_POINT ( 'NONE',  ( -13.97604488694527625, -13.89961937509977652, 46.87390960531435979 ) ) ;
#17471=CARTESIAN_POINT ( 'NONE',  ( 19.02544592524343514, -5.153800228976328945, 73.54057627198103830 ) ) ;
#17472=CARTESIAN_POINT ( 'NONE',  ( 14.34966873604972726, -8.224510206698740333, 70.83442372801901854 ) ) ;
#17475=CARTESIAN_POINT ( 'NONE',  ( -5.823673210054431948, 21.52544592524334988, 112.7094237280190328 ) ) ;
#17476=CARTESIAN_POINT ( 'NONE',  ( -0.05219959533909027116, -19.03943276465977164, 37.49890960531436690 ) ) ;
#17477=CARTESIAN_POINT ( 'NONE',  ( 13.97604488694527802, 13.89961937509977652, 99.37390960531436690 ) ) ;
#17479=CARTESIAN_POINT ( 'NONE',  ( -16.53943276465976808, -0.05219959533934237506, 33.75109039468568284 ) ) ;
#17480=CARTESIAN_POINT ( 'NONE',  ( 16.46253265017146816, 9.564922557961045513, 41.66775706135234003 ) ) ;
#17481=CARTESIAN_POINT ( 'NONE',  ( -12.14591786802326823, 12.06949235617739902, 48.12609039468568284 ) ) ;
#17482=CARTESIAN_POINT ( 'NONE',  ( -19.05341960407611168, -5.049401038298163336, 41.45724293864769550 ) ) ;
#17483=CARTESIAN_POINT ( 'NONE',  ( -13.89961937509977652, 13.97604488694528158, 100.6239096053143669 ) ) ;
#17484=CARTESIAN_POINT ( 'NONE',  ( 16.51473224551069308, 9.474510206698969483, 59.16557627198102409 ) ) ;
#17485=CARTESIAN_POINT ( 'NONE',  ( -21.52544592524343514, 5.823673210054127303, 101.0405762719810383 ) ) ;
#17486=CARTESIAN_POINT ( 'NONE',  ( 19.03943276465977164, -0.05219959533909143690, 83.74890960531436690 ) ) ;
#17487=CARTESIAN_POINT ( 'NONE',  ( 16.46253265017160672, -9.564922557960803928, 108.3322429386476955 ) ) ;
#17488=CARTESIAN_POINT ( 'NONE',  ( -19.05341960407611168, -5.049401038298163336, 66.45724293864769550 ) ) ;
#17490=CARTESIAN_POINT ( 'NONE',  ( 5.153800228976615827, -19.02544592524334988, 95.20942372801897591 ) ) ;
#17491=CARTESIAN_POINT ( 'NONE',  ( -19.03943276465977164, -0.05219959533935918106, 23.75109039468566152 ) ) ;
#17492=CARTESIAN_POINT ( 'NONE',  ( -4.483927247898539470, -16.52544592524342804, 62.29057627198102409 ) ) ;
#17493=CARTESIAN_POINT ( 'NONE',  ( -21.53943276465977519, -0.05219959533937600094, 78.75109039468568994 ) ) ;
#17494=CARTESIAN_POINT ( 'NONE',  ( -9.564922557960796823, -16.46253265017161027, 22.08224293864768839 ) ) ;
#17495=B_SPLINE_CURVE_WITH_KNOTS ( 'NONE', 3,
 ( #103421, #117584, #165100, #52899, #25604, #114574, #99404, #147934, #71085, #177281, #69077, #9420, #132752, #37744, #161087, #22582, #130743, #192435, #194439, #55910 ),
 .UNSPECIFIED., .F., .F.,
 ( 4, 2, 2, 2, 2, 2, 2, 2, 2, 4 ),
 ( 3.469446951953614189E-18, 0.0004987090165372812679, 0.0009974180330745590663, 0.001246772541343198074, 0.001496127049611837082, 0.001994836066149110326, 0.002493545082686384438, 0.002742899590955021061, 0.002992254099223657683, 0.003989672132298169478 ),
 .UNSPECIFIED. ) ;
#17496=CARTESIAN_POINT ( 'NONE',  ( 12.14591786802309770, 12.06949235617756955, 24.37390960531435979 ) ) ;
#17497=CARTESIAN_POINT ( 'NONE',  ( -21.55341960407619339, 5.719274019375674811, 93.54275706135234714 ) ) ;
#17498=CARTESIAN_POINT ( 'NONE',  ( 5.153800228976335163, 19.02544592524342804, 84.79057627198099567 ) ) ;
#17499=CARTESIAN_POINT ( 'NONE',  ( 5.823673210054444382, -21.52544592524334988, 50.20942372801901854 ) ) ;
#17500=CARTESIAN_POINT ( 'NONE',  ( -5.153800228976328057, -19.02544592524343514, 82.29057627198103830 ) ) ;
#17501=CARTESIAN_POINT ( 'NONE',  ( -4.379528057220328563, 16.55341960407611168, 90.20724293864770971 ) ) ;
#17502=CARTESIAN_POINT ( 'NONE',  ( -8.314922557960811034, -14.29746914071050412, 62.08224293864769550 ) ) ;
#17503=CARTESIAN_POINT ( 'NONE',  ( -15.72974639402197994, 15.80617190586746368, 75.62390960531439532 ) ) ;
#17504=CARTESIAN_POINT ( 'NONE',  ( 19.02544592524343514, -5.153800228976328945, 68.54057627198103830 ) ) ;
#17505=CARTESIAN_POINT ( 'NONE',  ( -21.52544592524343514, 5.823673210054127303, 86.04057627198102409 ) ) ;
#17506=CARTESIAN_POINT ( 'NONE',  ( 5.153800228976615827, -19.02544592524334988, 75.20942372801896170 ) ) ;
#17507=CARTESIAN_POINT ( 'NONE',  ( -19.20446147854525876, -5.500000000000010658, 89.38999695167676407 ) ) ;
#17508=CARTESIAN_POINT ( 'NONE',  ( 14.34966873604960469, 8.224510206698951720, 84.16557627198103830 ) ) ;
#17509=CARTESIAN_POINT ( 'NONE',  ( 9.564922557960805705, 16.46253265017160317, 54.58224293864769550 ) ) ;
#17510=CARTESIAN_POINT ( 'NONE',  ( -0.05219959533907301413, -21.53943276465977519, 62.49890960531436690 ) ) ;
#17512=CARTESIAN_POINT ( 'NONE',  ( 4.379528057220092307, 16.55341960407617563, 107.2927570613523471 ) ) ;
#17514=CARTESIAN_POINT ( 'NONE',  ( 13.89961937509957401, 13.97604488694547697, 96.87609039468566152 ) ) ;
#17515=CARTESIAN_POINT ( 'NONE',  ( -14.34966873604960291, -8.224510206698953496, 81.66557627198103830 ) ) ;
#17517=CARTESIAN_POINT ( 'NONE',  ( 13.97604488694527802, 13.89961937509977652, 74.37390960531436690 ) ) ;
#17518=CARTESIAN_POINT ( 'NONE',  ( -0.05219959533909027116, -19.03943276465977164, 32.49890960531435979 ) ) ;
#17519=CARTESIAN_POINT ( 'NONE',  ( -0.05219959533910754901, -16.53943276465976808, 62.49890960531436690 ) ) ;
#17520=CARTESIAN_POINT ( 'NONE',  ( -13.97604488694527625, -13.89961937509977652, 96.87390960531433848 ) ) ;
#17521=CARTESIAN_POINT ( 'NONE',  ( -13.97604488694547697, 13.89961937509957934, 88.12609039468563310 ) ) ;
#17522=CARTESIAN_POINT ( 'NONE',  ( -9.564922557960796823, -16.46253265017161027, 67.08224293864769550 ) ) ;
#17523=CARTESIAN_POINT ( 'NONE',  ( -19.05341960407611168, -5.049401038298163336, 91.45724293864766707 ) ) ;
#17524=CARTESIAN_POINT ( 'NONE',  ( 21.53943276465977519, -0.05219959533907433946, 78.74890960531436690 ) ) ;
#17525=CARTESIAN_POINT ( 'NONE',  ( 4.379528057220092307, 16.55341960407617563, 72.29275706135236135 ) ) ;
#17526=CARTESIAN_POINT ( 'NONE',  ( -16.36317988757098263, 7.306389748694730457, 94.09789608363175262 ) ) ;
#17527=CARTESIAN_POINT ( 'NONE',  ( 19.02544592524343514, -5.153800228976328945, 63.54057627198103830 ) ) ;
#17528=CARTESIAN_POINT ( 'NONE',  ( 10.81492255796078972, 18.62759615963270932, 64.58224293864769550 ) ) ;
#17529=CARTESIAN_POINT ( 'NONE',  ( 5.153800228976615827, -19.02544592524334988, 100.2094237280190043 ) ) ;
#17530=CARTESIAN_POINT ( 'NONE',  ( 16.53943276465976808, -0.05219959533910856209, 43.74890960531435979 ) ) ;
#17531=CARTESIAN_POINT ( 'NONE',  ( -5.823673210054431948, 21.52544592524334988, 52.70942372801902565 ) ) ;
#17533=CARTESIAN_POINT ( 'NONE',  ( -0.05219959533934338120, 16.53943276465976808, 77.50109039468567573 ) ) ;
#17534=CARTESIAN_POINT ( 'NONE',  ( -9.564922557960796823, -16.46253265017161027, 112.0822429386476955 ) ) ;
#17537=CARTESIAN_POINT ( 'NONE',  ( -14.34966873604972548, 8.224510206698743886, 88.33442372801901854 ) ) ;
#17538=CARTESIAN_POINT ( 'NONE',  ( 4.483927247898790824, -16.52544592524335698, 50.20942372801901854 ) ) ;
#17539=CARTESIAN_POINT ( 'NONE',  ( 13.97604488694527802, 13.89961937509977652, 39.37390960531435269 ) ) ;
#17540=CARTESIAN_POINT ( 'NONE',  ( -19.03943276465977164, 0.05219959533909376836, 56.24890960531435979 ) ) ;
#17541=CARTESIAN_POINT ( 'NONE',  ( 5.719274019375673035, 21.55341960407619339, 57.29275706135234714 ) ) ;
#17542=CARTESIAN_POINT ( 'NONE',  ( -16.53943276465976808, -0.05219959533934237506, 58.75109039468568994 ) ) ;
#17543=CARTESIAN_POINT ( 'NONE',  ( -0.05219959533910754901, -16.53943276465976808, 37.49890960531436690 ) ) ;
#17544=CARTESIAN_POINT ( 'NONE',  ( 16.46253265017160672, -9.564922557960803928, 48.33224293864769550 ) ) ;
#17545=CARTESIAN_POINT ( 'NONE',  ( -0.05219959533909027116, -19.03943276465977164, 37.49890960531436690 ) ) ;
#17546=CARTESIAN_POINT ( 'NONE',  ( -16.52544592524335698, -4.483927247898792601, 28.95942372801902209 ) ) ;
#17547=VECTOR ( 'NONE', #121060, 1000.000000000000000 ) ;
#17548=CARTESIAN_POINT ( 'NONE',  ( -5.049401038297874678, -19.05341960407617918, 79.79275706135233293 ) ) ;
#17549=CARTESIAN_POINT ( 'NONE',  ( -4.379528057220328563, 16.55341960407611168, 80.20724293864769550 ) ) ;
#17550=CARTESIAN_POINT ( 'NONE',  ( -5.153800228976328057, -19.02544592524343514, 47.29057627198102409 ) ) ;
#17551=CARTESIAN_POINT ( 'NONE',  ( -5.153800228976607833, 19.02544592524334988, 87.70942372801897591 ) ) ;
#17553=CARTESIAN_POINT ( 'NONE',  ( -21.53943276465977519, -0.05219959533937600094, 93.75109039468567573 ) ) ;
#17554=CARTESIAN_POINT ( 'NONE',  ( -14.34966873604972548, 8.224510206698743886, 53.33442372801901854 ) ) ;
#17556=CARTESIAN_POINT ( 'NONE',  ( 15.80617190586746368, 15.72974639402197994, 44.37390960531435979 ) ) ;
#17557=CARTESIAN_POINT ( 'NONE',  ( 12.06949235617739724, 12.14591786802326823, 41.87609039468568284 ) ) ;
#17559=CARTESIAN_POINT ( 'NONE',  ( -16.46253265017146816, -9.564922557961047289, 24.16775706135233648 ) ) ;
#17560=CARTESIAN_POINT ( 'NONE',  ( -13.97604488694527625, -13.89961937509977652, 81.87390960531436690 ) ) ;
#17561=CARTESIAN_POINT ( 'NONE',  ( 18.22780087662122384, -5.500000000000022204, 66.01540105326107266 ) ) ;
#17562=CARTESIAN_POINT ( 'NONE',  ( 19.05341960407611168, 5.049401038298154454, 48.95724293864768129 ) ) ;
#17564=CARTESIAN_POINT ( 'NONE',  ( -19.02544592524342804, 5.153800228976336051, 76.04057627198102409 ) ) ;
#17565=CARTESIAN_POINT ( 'NONE',  ( -17.49999999999999289, 5.500000000000036415, 65.79690382534171533 ) ) ;
#17566=CARTESIAN_POINT ( 'NONE',  ( -5.049401038297874678, -19.05341960407617918, 39.79275706135232582 ) ) ;
#17567=CARTESIAN_POINT ( 'NONE',  ( -19.02544592524334988, -5.153800228976617603, 18.95942372801899722 ) ) ;
#17568=CARTESIAN_POINT ( 'NONE',  ( 12.14591786802309770, 12.06949235617756955, 44.37390960531435979 ) ) ;
#17569=CARTESIAN_POINT ( 'NONE',  ( -19.05341960407611168, -5.049401038298163336, 41.45724293864769550 ) ) ;
#17570=CARTESIAN_POINT ( 'NONE',  ( -9.474510206698964154, 16.51473224551069663, 100.4155762719810241 ) ) ;
#17571=CARTESIAN_POINT ( 'NONE',  ( 21.55341960407619695, -5.719274019375665929, 71.04275706135234714 ) ) ;
#17572=CARTESIAN_POINT ( 'NONE',  ( -9.474510206698964154, 16.51473224551069663, 50.41557627198102409 ) ) ;
#17573=CARTESIAN_POINT ( 'NONE',  ( -5.823673210054431948, 21.52544592524334988, 77.70942372801900433 ) ) ;
#17574=CARTESIAN_POINT ( 'NONE',  ( -0.05219959533909027116, -19.03943276465977164, 112.4989096053143669 ) ) ;
#17575=CARTESIAN_POINT ( 'NONE',  ( -19.05341960407611168, -5.049401038298163336, 41.45724293864769550 ) ) ;
#17576=CARTESIAN_POINT ( 'NONE',  ( -18.62759615963255300, -10.81492255796106328, 19.16775706135234714 ) ) ;
#17577=CARTESIAN_POINT ( 'NONE',  ( 19.05341960407617918, -5.049401038297876454, 46.04275706135233293 ) ) ;
#17578=CARTESIAN_POINT ( 'NONE',  ( -5.153800228976328057, -19.02544592524343514, 27.29057627198103120 ) ) ;
#17579=CARTESIAN_POINT ( 'NONE',  ( -5.153800228976328057, -19.02544592524343514, 72.29057627198102409 ) ) ;
#17580=CARTESIAN_POINT ( 'NONE',  ( 19.05341960407617918, -5.049401038297876454, 106.0427570613523471 ) ) ;
#17582=CARTESIAN_POINT ( 'NONE',  ( 14.29746914071049879, -8.314922557960816363, 78.33224293864770971 ) ) ;
#17583=CARTESIAN_POINT ( 'NONE',  ( 18.67979575497178502, 10.72451020669898547, 34.16557627198102409 ) ) ;
#17584=CARTESIAN_POINT ( 'NONE',  ( -5.153800228976607833, 19.02544592524334988, 97.70942372801900433 ) ) ;
#17585=CARTESIAN_POINT ( 'NONE',  ( 21.55341960407610458, 5.719274019375980345, 108.9572429386476955 ) ) ;
#17586=CARTESIAN_POINT ( 'NONE',  ( 18.67979575497194134, -10.72451020669871369, 55.83442372801901854 ) ) ;
#17587=CARTESIAN_POINT ( 'NONE',  ( 4.483927247898790824, -16.52544592524335698, 50.20942372801901854 ) ) ;
#17588=CARTESIAN_POINT ( 'NONE',  ( 0.05219959533934541429, -16.53943276465976808, 50.00109039468568994 ) ) ;
#17589=CARTESIAN_POINT ( 'NONE',  ( 10.72451020669898902, -18.67979575497178502, 67.91557627198102409 ) ) ;
#17590=CARTESIAN_POINT ( 'NONE',  ( 5.153800228976335163, 19.02544592524342804, 44.79057627198103830 ) ) ;
#17591=CARTESIAN_POINT ( 'NONE',  ( -12.06949235617739369, -12.14591786802326823, 89.37609039468568994 ) ) ;
#17593=CARTESIAN_POINT ( 'NONE',  ( -18.67979575497178146, -10.72451020669898902, 101.6655762719810383 ) ) ;
#17594=CARTESIAN_POINT ( 'NONE',  ( -12.06949235617756955, 12.14591786802309770, 45.62390960531436690 ) ) ;
#17595=CARTESIAN_POINT ( 'NONE',  ( 19.02544592524343514, -5.153800228976328945, 73.54057627198103830 ) ) ;
#17596=CARTESIAN_POINT ( 'NONE',  ( 8.224510206698742110, 14.34966873604972548, 72.08442372801899012 ) ) ;
#17597=CARTESIAN_POINT ( 'NONE',  ( 12.06949235617739724, 12.14591786802326823, 21.87609039468567573 ) ) ;
#17598=CARTESIAN_POINT ( 'NONE',  ( 21.52544592524344225, -5.823673210054117533, 113.5405762719810383 ) ) ;
#17599=CARTESIAN_POINT ( 'NONE',  ( -14.29746914071049879, 8.314922557960819915, 40.83224293864769550 ) ) ;
#17601=CARTESIAN_POINT ( 'NONE',  ( -17.40861289039003168, 6.110651285853257342, 68.62767529172569425 ) ) ;
#17602=CARTESIAN_POINT ( 'NONE',  ( -18.62759615963270932, 10.81492255796079327, 90.83224293864769550 ) ) ;
#17603=CARTESIAN_POINT ( 'NONE',  ( -4.483927247898539470, -16.52544592524342804, 27.29057627198103120 ) ) ;
#17605=LINE ( 'NONE', #175263, #59781 ) ;
#17606=CARTESIAN_POINT ( 'NONE',  ( 15.80617190586746368, 15.72974639402197994, 104.3739096053143669 ) ) ;
#17607=CARTESIAN_POINT ( 'NONE',  ( 16.51473224551069308, 9.474510206698969483, 109.1655762719810383 ) ) ;
#17608=CARTESIAN_POINT ( 'NONE',  ( 21.52544592524334988, 5.823673210054432836, 21.45942372801901499 ) ) ;
#17609=CARTESIAN_POINT ( 'NONE',  ( 16.53943276465976808, -0.05219959533910856209, 53.74890960531437401 ) ) ;
#17610=VECTOR ( 'NONE', #40379, 1000.000000000000000 ) ;
#17611=CARTESIAN_POINT ( 'NONE',  ( -12.06949235617739369, -12.14591786802326823, 49.37609039468569705 ) ) ;
#17612=CARTESIAN_POINT ( 'NONE',  ( 16.46253265017160672, -9.564922557960803928, 63.33224293864769550 ) ) ;
#17613=CARTESIAN_POINT ( 'NONE',  ( 19.03943276465977164, 0.05219959533936151252, 56.25109039468566863 ) ) ;
#17614=CARTESIAN_POINT ( 'NONE',  ( -13.89961937509977652, 13.97604488694528158, 80.62390960531436690 ) ) ;
#17616=CARTESIAN_POINT ( 'NONE',  ( 21.53943276465977519, -0.05219959533907433946, 38.74890960531435979 ) ) ;
#17618=CARTESIAN_POINT ( 'NONE',  ( -16.46253265017160317, 9.564922557960807481, 45.83224293864769550 ) ) ;
#17619=CARTESIAN_POINT ( 'NONE',  ( -14.29746914071037622, -8.314922557961029526, 24.16775706135235424 ) ) ;
#17620=CARTESIAN_POINT ( 'NONE',  ( -5.153800228976607833, 19.02544592524334988, 62.70942372801899722 ) ) ;
#17621=CARTESIAN_POINT ( 'NONE',  ( -0.05219959533907301413, -21.53943276465977519, 107.4989096053143669 ) ) ;
#17622=CARTESIAN_POINT ( 'NONE',  ( -8.224510206698948167, 14.34966873604960824, 40.41557627198103120 ) ) ;
#17623=CARTESIAN_POINT ( 'NONE',  ( -19.03943276465977164, 0.05219959533909376836, 86.24890960531436690 ) ) ;
#17624=CARTESIAN_POINT ( 'NONE',  ( 10.81492255796078972, 18.62759615963270932, 59.58224293864770260 ) ) ;
#17625=CARTESIAN_POINT ( 'NONE',  ( -10.72451020669898014, 18.67979575497178502, 90.41557627198103830 ) ) ;
#17626=CARTESIAN_POINT ( 'NONE',  ( -14.29746914071037622, -8.314922557961029526, 29.16775706135234003 ) ) ;
#17627=CARTESIAN_POINT ( 'NONE',  ( -10.81492255796078084, -18.62759615963271287, 22.08224293864769194 ) ) ;
#17628=CARTESIAN_POINT ( 'NONE',  ( -5.823673210054431948, 21.52544592524334988, 82.70942372801900433 ) ) ;
#17629=CARTESIAN_POINT ( 'NONE',  ( -16.51473224551069308, -9.474510206698971260, 86.66557627198102409 ) ) ;
#17630=CARTESIAN_POINT ( 'NONE',  ( 19.05341960407611168, 5.049401038298154454, 33.95724293864769550 ) ) ;
#17631=CARTESIAN_POINT ( 'NONE',  ( -9.564922557960796823, -16.46253265017161027, 82.08224293864768129 ) ) ;
#17632=CARTESIAN_POINT ( 'NONE',  ( 8.314922557960818139, 14.29746914071049879, 99.58224293864770971 ) ) ;
#17633=CARTESIAN_POINT ( 'NONE',  ( -13.89961937509977652, 13.97604488694528158, 65.62390960531436690 ) ) ;
#17634=CARTESIAN_POINT ( 'NONE',  ( -14.34966873604972548, 8.224510206698743886, 23.33442372801901499 ) ) ;
#17636=CARTESIAN_POINT ( 'NONE',  ( 15.72974639402176855, 15.80617190586768217, 91.87609039468568994 ) ) ;
#17637=CARTESIAN_POINT ( 'NONE',  ( -0.05219959533909027116, -19.03943276465977164, 107.4989096053143527 ) ) ;
#17638=CARTESIAN_POINT ( 'NONE',  ( 8.224510206698742110, 14.34966873604972548, 92.08442372801901854 ) ) ;
#17640=CARTESIAN_POINT ( 'NONE',  ( -16.51473224551082808, 9.474510206698731452, 68.33442372801900433 ) ) ;
#17641=CARTESIAN_POINT ( 'NONE',  ( 16.51473224551083163, -9.474510206698727899, 25.83442372801900078 ) ) ;
#17643=CARTESIAN_POINT ( 'NONE',  ( 13.89961937509977652, -13.97604488694527269, 33.12390960531434558 ) ) ;
#17644=CARTESIAN_POINT ( 'NONE',  ( 0.05219959533910956823, 16.53943276465976808, 29.99890960531435979 ) ) ;
#17646=CARTESIAN_POINT ( 'NONE',  ( 14.29746914071037800, 8.314922557961029526, 111.6677570613523613 ) ) ;
#17647=CARTESIAN_POINT ( 'NONE',  ( 17.05587630539785948, 6.762274262135716363, 66.75819690962687503 ) ) ;
#17648=CARTESIAN_POINT ( 'NONE',  ( 12.06949235617739724, 12.14591786802326823, 76.87609039468567573 ) ) ;
#17649=CARTESIAN_POINT ( 'NONE',  ( 5.049401038298161559, -19.05341960407611168, 42.70724293864767418 ) ) ;
#17650=CARTESIAN_POINT ( 'NONE',  ( 21.55341960407619695, -5.719274019375665929, 96.04275706135236135 ) ) ;
#17651=CARTESIAN_POINT ( 'NONE',  ( -0.05219959533936034679, 19.03943276465977164, 97.50109039468567573 ) ) ;
#17652=CARTESIAN_POINT ( 'NONE',  ( -15.80617190586768217, 15.72974639402176855, 83.12609039468568994 ) ) ;
#17653=CARTESIAN_POINT ( 'NONE',  ( -5.153800228976607833, 19.02544592524334988, 52.70942372801900433 ) ) ;
#17654=CARTESIAN_POINT ( 'NONE',  ( 9.564922557960805705, 16.46253265017160317, 94.58224293864769550 ) ) ;
#17655=CARTESIAN_POINT ( 'NONE',  ( -9.564922557960796823, -16.46253265017161027, 72.08224293864770971 ) ) ;
#17656=CARTESIAN_POINT ( 'NONE',  ( -18.56197773271730966, 5.499999999999902300, 38.55066217314451649 ) ) ;
#17657=CARTESIAN_POINT ( 'NONE',  ( 12.06949235617757843, -12.14591786802309237, 73.12390960531436690 ) ) ;
#17658=CARTESIAN_POINT ( 'NONE',  ( -10.72451020669898014, 18.67979575497178502, 65.41557627198102409 ) ) ;
#17659=CARTESIAN_POINT ( 'NONE',  ( -16.51473224551069308, -9.474510206698971260, 41.66557627198103120 ) ) ;
#17660=CARTESIAN_POINT ( 'NONE',  ( -5.719274019375978568, 21.55341960407610458, 85.20724293864770971 ) ) ;
#17661=CARTESIAN_POINT ( 'NONE',  ( 14.29746914071037800, 8.314922557961029526, 71.66775706135234714 ) ) ;
#17664=CARTESIAN_POINT ( 'NONE',  ( -19.03943276465977164, 0.05219959533909376836, 51.24890960531436690 ) ) ;
#17666=CARTESIAN_POINT ( 'NONE',  ( 16.53943276465976808, -0.05219959533910856209, 73.74890960531433848 ) ) ;
#17668=CARTESIAN_POINT ( 'NONE',  ( -5.153800228976328057, -19.02544592524343514, 52.29057627198100988 ) ) ;
#17669=CARTESIAN_POINT ( 'NONE',  ( 16.51473224551069308, 9.474510206698969483, 24.16557627198102765 ) ) ;
#17670=CARTESIAN_POINT ( 'NONE',  ( -16.46253265017146816, -9.564922557961047289, 64.16775706135233293 ) ) ;
#17671=CARTESIAN_POINT ( 'NONE',  ( -4.379528057220328563, 16.55341960407611168, 75.20724293864769550 ) ) ;
#17672=CARTESIAN_POINT ( 'NONE',  ( 0.05219959533937995610, -21.53943276465977519, 50.00109039468568994 ) ) ;
#17673=CARTESIAN_POINT ( 'NONE',  ( -19.05341960407611168, -5.049401038298163336, 41.45724293864769550 ) ) ;
#17674=CARTESIAN_POINT ( 'NONE',  ( 21.52544592524344225, -5.823673210054117533, 108.5405762719810241 ) ) ;
#17676=CARTESIAN_POINT ( 'NONE',  ( 16.55341960407611168, 4.379528057220329451, 88.95724293864769550 ) ) ;
#17678=CARTESIAN_POINT ( 'NONE',  ( -0.05219959533909027116, -19.03943276465977164, 52.49890960531436690 ) ) ;
#17680=CARTESIAN_POINT ( 'NONE',  ( -16.46253265017146816, -9.564922557961047289, 94.16775706135233293 ) ) ;
#17681=CARTESIAN_POINT ( 'NONE',  ( -9.474510206698964154, 16.51473224551069663, 100.4155762719810241 ) ) ;
#17682=CARTESIAN_POINT ( 'NONE',  ( 21.55341960407619695, -5.719274019375665929, 36.04275706135234714 ) ) ;
#17683=CARTESIAN_POINT ( 'NONE',  ( 19.02544592524343514, -5.153800228976328945, 83.54057627198100988 ) ) ;
#17684=CARTESIAN_POINT ( 'NONE',  ( -16.51473224551082808, 9.474510206698731452, 73.33442372801900433 ) ) ;
#17685=CARTESIAN_POINT ( 'NONE',  ( -19.05341960407611168, -5.049401038298163336, 46.45724293864768129 ) ) ;
#17686=CARTESIAN_POINT ( 'NONE',  ( 4.379528057220339221, -16.55341960407611168, 62.70724293864769550 ) ) ;
#17687=CARTESIAN_POINT ( 'NONE',  ( 12.06949235617757843, -12.14591786802309237, 73.12390960531436690 ) ) ;
#17688=CARTESIAN_POINT ( 'NONE',  ( 9.564922557960805705, 16.46253265017160317, 74.58224293864769550 ) ) ;
#17689=CARTESIAN_POINT ( 'NONE',  ( 21.55341960407610458, 5.719274019375980345, 98.95724293864770971 ) ) ;
#17690=CARTESIAN_POINT ( 'NONE',  ( -5.049401038298153566, 19.05341960407611168, 65.20724293864765286 ) ) ;
#17692=CARTESIAN_POINT ( 'NONE',  ( 0.05219959533937995610, -21.53943276465977519, 110.0010903946856757 ) ) ;
#17693=CARTESIAN_POINT ( 'NONE',  ( 9.474510206698971260, -16.51473224551069308, 32.91557627198102409 ) ) ;
#17694=CARTESIAN_POINT ( 'NONE',  ( -14.34966873604972548, 8.224510206698743886, 113.3344237280190328 ) ) ;
#17695=CARTESIAN_POINT ( 'NONE',  ( -12.14591786802309592, -12.06949235617757132, 111.8739096053143669 ) ) ;
#17696=CARTESIAN_POINT ( 'NONE',  ( 19.03943276465977164, 0.05219959533936151252, 101.2510903946856757 ) ) ;
#17697=ORIENTED_EDGE ( 'NONE', *, *, #5625, .F. ) ;
#17698=CARTESIAN_POINT ( 'NONE',  ( -5.719274019375665041, -21.55341960407619695, 24.79275706135235779 ) ) ;
#17699=CARTESIAN_POINT ( 'NONE',  ( 9.564922557961047289, -16.46253265017146816, 60.41775706135233293 ) ) ;
#17700=CARTESIAN_POINT ( 'NONE',  ( -4.379528057220086978, -16.55341960407618274, 109.7927570613523613 ) ) ;
#17701=CARTESIAN_POINT ( 'NONE',  ( -21.55341960407610458, -5.719274019375992779, 76.45724293864769550 ) ) ;
#17702=CARTESIAN_POINT ( 'NONE',  ( -15.80617190586745835, -15.72974639402198527, 21.87390960531436690 ) ) ;
#17703=CARTESIAN_POINT ( 'NONE',  ( -12.06949235617756955, 12.14591786802309770, 50.62390960531435979 ) ) ;
#17704=CARTESIAN_POINT ( 'NONE',  ( 9.564922557960805705, 16.46253265017160317, 34.58224293864770260 ) ) ;
#17705=CARTESIAN_POINT ( 'NONE',  ( 19.03943276465977164, -0.05219959533909143690, 38.74890960531436690 ) ) ;
#17706=CARTESIAN_POINT ( 'NONE',  ( 9.564922557961047289, -16.46253265017146816, 25.41775706135234003 ) ) ;
#17707=CARTESIAN_POINT ( 'NONE',  ( -14.29746914071037622, -8.314922557961029526, 94.16775706135237556 ) ) ;
#17708=CARTESIAN_POINT ( 'NONE',  ( 16.53943276465976808, 0.05219959533934440121, 56.25109039468568284 ) ) ;
#17709=CARTESIAN_POINT ( 'NONE',  ( -5.823673210054116645, -21.52544592524344225, 22.29057627198102765 ) ) ;
#17710=CARTESIAN_POINT ( 'NONE',  ( -9.564922557960796823, -16.46253265017161027, 52.08224293864768839 ) ) ;
#17711=CARTESIAN_POINT ( 'NONE',  ( 15.72974639402176855, 15.80617190586768217, 111.8760903946856615 ) ) ;
#17712=CARTESIAN_POINT ( 'NONE',  ( 13.97604488694527802, 13.89961937509977652, 84.37390960531433848 ) ) ;
#17713=CARTESIAN_POINT ( 'NONE',  ( -0.05219959533934338120, 16.53943276465976808, 57.50109039468568994 ) ) ;
#17714=CARTESIAN_POINT ( 'NONE',  ( -12.06949235617756955, 12.14591786802309770, 110.6239096053143669 ) ) ;
#17715=CARTESIAN_POINT ( 'NONE',  ( 4.483927247898545687, 16.52544592524342804, 24.79057627198103120 ) ) ;
#17716=CARTESIAN_POINT ( 'NONE',  ( 17.50000000000000000, -5.500000000000000888, 120.0000000000000142 ) ) ;
#17717=CARTESIAN_POINT ( 'NONE',  ( 15.72974639402176855, 15.80617190586768217, 66.87609039468568994 ) ) ;
#17718=CARTESIAN_POINT ( 'NONE',  ( -16.46253265017160317, 9.564922557960807481, 90.83224293864769550 ) ) ;
#17719=CARTESIAN_POINT ( 'NONE',  ( -16.46253265017160317, 9.564922557960807481, 80.83224293864769550 ) ) ;
#17720=CARTESIAN_POINT ( 'NONE',  ( 16.51473224551069308, 9.474510206698969483, 109.1655762719810383 ) ) ;
#17721=CARTESIAN_POINT ( 'NONE',  ( 14.34966873604960469, 8.224510206698951720, 64.16557627198102409 ) ) ;
#17722=CARTESIAN_POINT ( 'NONE',  ( 12.06949235617757843, -12.14591786802309237, 23.12390960531436335 ) ) ;
#17724=CARTESIAN_POINT ( 'NONE',  ( 4.379528057220339221, -16.55341960407611168, 32.70724293864770260 ) ) ;
#17725=CARTESIAN_POINT ( 'NONE',  ( -0.05219959533934338120, 16.53943276465976808, 37.50109039468568284 ) ) ;
#17728=CARTESIAN_POINT ( 'NONE',  ( -9.474510206698720793, -16.51473224551083518, 34.58442372801899722 ) ) ;
#17729=CARTESIAN_POINT ( 'NONE',  ( 19.03943276465977164, -0.05219959533909143690, 78.74890960531436690 ) ) ;
#17730=CARTESIAN_POINT ( 'NONE',  ( 5.049401038297881783, 19.05341960407617563, 52.29275706135234003 ) ) ;
#17732=CARTESIAN_POINT ( 'NONE',  ( -5.153800228976607833, 19.02544592524334988, 97.70942372801900433 ) ) ;
#17733=CARTESIAN_POINT ( 'NONE',  ( -16.53943276465976808, -0.05219959533934237506, 78.75109039468568994 ) ) ;
#17735=CARTESIAN_POINT ( 'NONE',  ( 5.153800228976335163, 19.02544592524342804, 24.79057627198102765 ) ) ;
#17736=CARTESIAN_POINT ( 'NONE',  ( -9.474510206698964154, 16.51473224551069663, 100.4155762719810241 ) ) ;
#17737=CARTESIAN_POINT ( 'NONE',  ( -10.81492255796105439, 18.62759615963255655, 47.91775706135234714 ) ) ;
#17738=CARTESIAN_POINT ( 'NONE',  ( -19.02544592524334988, -5.153800228976617603, 83.95942372801901854 ) ) ;
#17740=CARTESIAN_POINT ( 'NONE',  ( 13.97604488694527802, 13.89961937509977652, 44.37390960531435269 ) ) ;
#17741=CARTESIAN_POINT ( 'NONE',  ( -9.564922557960796823, -16.46253265017161027, 97.08224293864769550 ) ) ;
#17742=CARTESIAN_POINT ( 'NONE',  ( -4.379528057220328563, 16.55341960407611168, 55.20724293864770260 ) ) ;
#17743=CARTESIAN_POINT ( 'NONE',  ( -5.049401038298153566, 19.05341960407611168, 45.20724293864769550 ) ) ;
#17744=CARTESIAN_POINT ( 'NONE',  ( 9.564922557960805705, 16.46253265017160317, 64.58224293864769550 ) ) ;
#17745=CARTESIAN_POINT ( 'NONE',  ( -16.51473224551082808, 9.474510206698731452, 58.33442372801900433 ) ) ;
#17746=CARTESIAN_POINT ( 'NONE',  ( 9.474510206698729675, 16.51473224551082808, 37.08442372801899722 ) ) ;
#17747=CARTESIAN_POINT ( 'NONE',  ( 5.049401038297881783, 19.05341960407617563, 47.29275706135231161 ) ) ;
#17748=CARTESIAN_POINT ( 'NONE',  ( -13.89961937509977652, 13.97604488694528158, 75.62390960531438111 ) ) ;
#17749=CARTESIAN_POINT ( 'NONE',  ( 21.52544592524344225, -5.823673210054117533, 73.54057627198102409 ) ) ;
#17750=CARTESIAN_POINT ( 'NONE',  ( 16.52544592524342804, -4.483927247898539470, 68.54057627198103830 ) ) ;
#17751=CARTESIAN_POINT ( 'NONE',  ( 16.46253265017146816, 9.564922557961045513, 31.66775706135232937 ) ) ;
#17752=CARTESIAN_POINT ( 'NONE',  ( 18.62759615963271287, -10.81492255796078972, 53.33224293864769550 ) ) ;
#17753=CARTESIAN_POINT ( 'NONE',  ( -18.62759615963270932, 10.81492255796079327, 45.83224293864769550 ) ) ;
#17754=CARTESIAN_POINT ( 'NONE',  ( 0.05219959533909260263, 19.03943276465977164, 64.99890960531436690 ) ) ;
#17755=CARTESIAN_POINT ( 'NONE',  ( 0.05219959533909260263, 19.03943276465977164, 34.99890960531435979 ) ) ;
#17756=CARTESIAN_POINT ( 'NONE',  ( 8.224510206698953496, -14.34966873604960469, 102.9155762719810383 ) ) ;
#17758=CARTESIAN_POINT ( 'NONE',  ( -10.81492255796078084, -18.62759615963271287, 112.0822429386477097 ) ) ;
#17759=CARTESIAN_POINT ( 'NONE',  ( 19.02544592524343514, -5.153800228976328945, 108.5405762719810383 ) ) ;
#17760=CARTESIAN_POINT ( 'NONE',  ( 21.55341960407619695, -5.719274019375665929, 26.04275706135235779 ) ) ;
#17761=CARTESIAN_POINT ( 'NONE',  ( -9.564922557960796823, -16.46253265017161027, 37.08224293864768839 ) ) ;
#17762=CARTESIAN_POINT ( 'NONE',  ( -5.823673210054116645, -21.52544592524344225, 107.2905762719810525 ) ) ;
#17763=CARTESIAN_POINT ( 'NONE',  ( 9.564922557961047289, -16.46253265017146816, 50.41775706135233293 ) ) ;
#17764=CARTESIAN_POINT ( 'NONE',  ( -5.153800228976328057, -19.02544592524343514, 27.29057627198103120 ) ) ;
#17765=CARTESIAN_POINT ( 'NONE',  ( -19.03943276465977164, 0.05219959533909376836, 21.24890960531436335 ) ) ;
#17766=CARTESIAN_POINT ( 'NONE',  ( -14.29746914071037622, -8.314922557961029526, 64.16775706135234714 ) ) ;
#17767=CARTESIAN_POINT ( 'NONE',  ( -5.049401038298153566, 19.05341960407611168, 30.20724293864768839 ) ) ;
#17769=CARTESIAN_POINT ( 'NONE',  ( -0.05219959533909027116, -19.03943276465977164, 72.49890960531435269 ) ) ;
#17770=CARTESIAN_POINT ( 'NONE',  ( -14.34966873604960291, -8.224510206698953496, 111.6655762719810525 ) ) ;
#17772=CARTESIAN_POINT ( 'NONE',  ( -18.62759615963270932, 10.81492255796079327, 40.83224293864769550 ) ) ;
#17773=CARTESIAN_POINT ( 'NONE',  ( 4.483927247898545687, 16.52544592524342804, 79.79057627198102409 ) ) ;
#17774=CARTESIAN_POINT ( 'NONE',  ( -14.34966873604972548, 8.224510206698743886, 33.33442372801900433 ) ) ;
#17775=CARTESIAN_POINT ( 'NONE',  ( 5.719274019375673035, 21.55341960407619339, 87.29275706135236135 ) ) ;
#17776=CARTESIAN_POINT ( 'NONE',  ( 13.89961937509977652, -13.97604488694527269, 28.12390960531435624 ) ) ;
#17777=CARTESIAN_POINT ( 'NONE',  ( 16.52544592524335698, 4.483927247898782831, 111.4594237280190328 ) ) ;
#17778=CARTESIAN_POINT ( 'NONE',  ( -12.06949235617756955, 12.14591786802309770, 60.62390960531437401 ) ) ;
#17779=CARTESIAN_POINT ( 'NONE',  ( 19.03943276465977164, -0.05219959533909143690, 48.74890960531435979 ) ) ;
#17780=CARTESIAN_POINT ( 'NONE',  ( 10.72451020669871369, 18.67979575497193778, 97.08442372801904696 ) ) ;
#17781=CARTESIAN_POINT ( 'NONE',  ( -18.62759615963270932, 10.81492255796079327, 105.8322429386476955 ) ) ;
#17782=CARTESIAN_POINT ( 'NONE',  ( -5.823673210054431948, 21.52544592524334988, 77.70942372801900433 ) ) ;
#17783=CARTESIAN_POINT ( 'NONE',  ( 12.14591786802327356, -12.06949235617739191, 35.62609039468568994 ) ) ;
#17784=CARTESIAN_POINT ( 'NONE',  ( 14.34966873604960469, 8.224510206698951720, 79.16557627198103830 ) ) ;
#17785=CARTESIAN_POINT ( 'NONE',  ( 10.81492255796106328, -18.62759615963255655, 85.41775706135236135 ) ) ;
#17786=CARTESIAN_POINT ( 'NONE',  ( -16.53943276465976808, -0.05219959533934237506, 108.7510903946857042 ) ) ;
#17788=CARTESIAN_POINT ( 'NONE',  ( 14.29746914071037800, 8.314922557961029526, 36.66775706135234714 ) ) ;
#17789=CARTESIAN_POINT ( 'NONE',  ( 14.34966873604960469, 8.224510206698951720, 39.16557627198102409 ) ) ;
#17790=CARTESIAN_POINT ( 'NONE',  ( -4.483927247898782831, 16.52544592524335698, 82.70942372801900433 ) ) ;
#17791=CARTESIAN_POINT ( 'NONE',  ( -13.97604488694527625, -13.89961937509977652, 101.8739096053143811 ) ) ;
#17792=CARTESIAN_POINT ( 'NONE',  ( 13.97604488694527802, 13.89961937509977652, 104.3739096053143385 ) ) ;
#17793=CARTESIAN_POINT ( 'NONE',  ( -15.80617190586768217, 15.72974639402176855, 103.1260903946856757 ) ) ;
#17794=CARTESIAN_POINT ( 'NONE',  ( -12.06949235617739369, -12.14591786802326823, 99.37609039468568994 ) ) ;
#17795=CARTESIAN_POINT ( 'NONE',  ( 12.06949235617757843, -12.14591786802309237, 73.12390960531436690 ) ) ;
#17796=CARTESIAN_POINT ( 'NONE',  ( -5.153800228976328057, -19.02544592524343514, 87.29057627198103830 ) ) ;
#17797=ORIENTED_EDGE ( 'NONE', *, *, #190985, .T. ) ;
#17798=CARTESIAN_POINT ( 'NONE',  ( -4.379528057220086978, -16.55341960407618274, 29.79275706135234358 ) ) ;
#17799=CARTESIAN_POINT ( 'NONE',  ( -0.05219959533909027116, -19.03943276465977164, 27.49890960531435624 ) ) ;
#17800=CARTESIAN_POINT ( 'NONE',  ( -19.02544592524342804, 5.153800228976336051, 91.04057627198100988 ) ) ;
#17801=CARTESIAN_POINT ( 'NONE',  ( -12.14591786802326823, 12.06949235617739902, 33.12609039468569705 ) ) ;
#17803=CARTESIAN_POINT ( 'NONE',  ( 16.51473224551083163, -9.474510206698727899, 30.83442372801900433 ) ) ;
#17804=CARTESIAN_POINT ( 'NONE',  ( 12.14591786802327356, -12.06949235617739191, 100.6260903946857184 ) ) ;
#17805=CARTESIAN_POINT ( 'NONE',  ( -0.05219959533936034679, 19.03943276465977164, 102.5010903946856757 ) ) ;
#17806=CARTESIAN_POINT ( 'NONE',  ( -13.97604488694527625, -13.89961937509977652, 31.87390960531435979 ) ) ;
#17807=CARTESIAN_POINT ( 'NONE',  ( 14.29746914071037800, 8.314922557961029526, 81.66775706135236135 ) ) ;
#17808=CARTESIAN_POINT ( 'NONE',  ( -0.05219959533934338120, 16.53943276465976808, 62.50109039468568284 ) ) ;
#17809=CARTESIAN_POINT ( 'NONE',  ( 16.51473224551069308, 9.474510206698969483, 34.16557627198102409 ) ) ;
#17810=CARTESIAN_POINT ( 'NONE',  ( -13.89961937509957401, -13.97604488694547875, 69.37609039468564731 ) ) ;
#17811=AXIS2_PLACEMENT_3D ( 'NONE', #55151, #23827, #8654 ) ;
#17812=CARTESIAN_POINT ( 'NONE',  ( 13.89961937509957401, 13.97604488694547697, 21.87609039468566152 ) ) ;
#17813=CARTESIAN_POINT ( 'NONE',  ( 13.89961937509977652, -13.97604488694527269, 53.12390960531434558 ) ) ;
#17814=CARTESIAN_POINT ( 'NONE',  ( -5.153800228976328057, -19.02544592524343514, 97.29057627198099567 ) ) ;
#17815=CARTESIAN_POINT ( 'NONE',  ( 4.483927247898545687, 16.52544592524342804, 84.79057627198102409 ) ) ;
#17816=CARTESIAN_POINT ( 'NONE',  ( -13.97604488694547697, 13.89961937509957934, 58.12609039468566863 ) ) ;
#17817=CARTESIAN_POINT ( 'NONE',  ( 15.80617190586746368, 15.72974639402197994, 49.37390960531436690 ) ) ;
#17818=CARTESIAN_POINT ( 'NONE',  ( -5.823673210054431948, 21.52544592524334988, 107.7094237280190328 ) ) ;
#17819=CARTESIAN_POINT ( 'NONE',  ( -0.05219959533909027116, -19.03943276465977164, 92.49890960531436690 ) ) ;
#17820=CARTESIAN_POINT ( 'NONE',  ( 13.97604488694548053, -13.89961937509957401, 25.62609039468566507 ) ) ;
#17821=CARTESIAN_POINT ( 'NONE',  ( -21.53943276465977519, 0.05219959533907696930, 61.24890960531435979 ) ) ;
#17822=CARTESIAN_POINT ( 'NONE',  ( -19.02544592524342804, 5.153800228976336051, 111.0405762719810099 ) ) ;
#17823=CARTESIAN_POINT ( 'NONE',  ( -16.46253265017146816, -9.564922557961047289, 89.16775706135234714 ) ) ;
#17824=CARTESIAN_POINT ( 'NONE',  ( -19.03943276465977164, 0.05219959533909376836, 116.2489096053143669 ) ) ;
#17825=CARTESIAN_POINT ( 'NONE',  ( -0.05219959533936034679, 19.03943276465977164, 107.5010903946856615 ) ) ;
#17826=CARTESIAN_POINT ( 'NONE',  ( -16.52544592524342804, 4.483927247898546575, 111.0405762719810525 ) ) ;
#17827=CARTESIAN_POINT ( 'NONE',  ( 5.153800228976335163, 19.02544592524342804, 94.79057627198103830 ) ) ;
#17828=CARTESIAN_POINT ( 'NONE',  ( -21.53943276465977519, 0.05219959533907696930, 81.24890960531436690 ) ) ;
#17829=CARTESIAN_POINT ( 'NONE',  ( 8.224510206698742110, 14.34966873604972548, 52.08442372801901854 ) ) ;
#17830=CARTESIAN_POINT ( 'NONE',  ( -15.80617190586768217, 15.72974639402176855, 43.12609039468568284 ) ) ;
#17831=CARTESIAN_POINT ( 'NONE',  ( 21.55341960407619695, -5.719274019375665929, 96.04275706135236135 ) ) ;
#17832=CARTESIAN_POINT ( 'NONE',  ( 12.06949235617739724, 12.14591786802326823, 101.8760903946857042 ) ) ;
#17833=CARTESIAN_POINT ( 'NONE',  ( 5.153800228976335163, 19.02544592524342804, 89.79057627198102409 ) ) ;
#17834=CARTESIAN_POINT ( 'NONE',  ( -14.34966873604960291, -8.224510206698953496, 91.66557627198103830 ) ) ;
#17835=CARTESIAN_POINT ( 'NONE',  ( -4.483927247898539470, -16.52544592524342804, 37.29057627198102409 ) ) ;
#17836=CARTESIAN_POINT ( 'NONE',  ( -16.46253265017146816, -9.564922557961047289, 64.16775706135233293 ) ) ;
#17837=CARTESIAN_POINT ( 'NONE',  ( 18.62759615963255655, 10.81492255796105972, 46.66775706135234714 ) ) ;
#17838=CARTESIAN_POINT ( 'NONE',  ( -5.049401038297874678, -19.05341960407617918, 29.79275706135232227 ) ) ;
#17839=CARTESIAN_POINT ( 'NONE',  ( -12.14591786802309592, -12.06949235617757132, 96.87390960531436690 ) ) ;
#17840=CARTESIAN_POINT ( 'NONE',  ( -21.53943276465977519, 0.05219959533907696930, 31.24890960531435979 ) ) ;
#17841=CARTESIAN_POINT ( 'NONE',  ( -8.314922557960811034, -14.29746914071050412, 27.08224293864769550 ) ) ;
#17842=CARTESIAN_POINT ( 'NONE',  ( -21.53943276465977519, -0.05219959533937600094, 88.75109039468567573 ) ) ;
#17843=CARTESIAN_POINT ( 'NONE',  ( -16.52544592524335698, -4.483927247898792601, 58.95942372801902565 ) ) ;
#17844=CARTESIAN_POINT ( 'NONE',  ( -8.314922557961024197, 14.29746914071037800, 112.9177570613523329 ) ) ;
#17845=CARTESIAN_POINT ( 'NONE',  ( -21.55341960407619339, 5.719274019375674811, 48.54275706135234714 ) ) ;
#17846=ORIENTED_EDGE ( 'NONE', *, *, #166361, .T. ) ;
#17847=CARTESIAN_POINT ( 'NONE',  ( 21.55341960407619695, -5.719274019375665929, 31.04275706135234714 ) ) ;
#17848=CARTESIAN_POINT ( 'NONE',  ( 14.34966873604960469, 8.224510206698951720, 104.1655762719810241 ) ) ;
#17849=EDGE_CURVE ( 'NONE', #61533, #22005, #93569, .T. ) ;
#17850=CARTESIAN_POINT ( 'NONE',  ( 0.05219959533909260263, 19.03943276465977164, 24.99890960531435269 ) ) ;
#17851=CARTESIAN_POINT ( 'NONE',  ( -14.29746914071049879, 8.314922557960819915, 65.83224293864769550 ) ) ;
#17852=CARTESIAN_POINT ( 'NONE',  ( -19.05341960407611168, -5.049401038298163336, 76.45724293864769550 ) ) ;
#17853=CARTESIAN_POINT ( 'NONE',  ( 12.06949235617739724, 12.14591786802326823, 106.8760903946856899 ) ) ;
#17854=CARTESIAN_POINT ( 'NONE',  ( 15.80617190586746368, 15.72974639402197994, 54.37390960531435979 ) ) ;
#17855=CARTESIAN_POINT ( 'NONE',  ( 0.05219959533910956823, 16.53943276465976808, 94.99890960531436690 ) ) ;
#17857=CARTESIAN_POINT ( 'NONE',  ( 21.52544592524344225, -5.823673210054117533, 98.54057627198105251 ) ) ;
#17858=CARTESIAN_POINT ( 'NONE',  ( 5.153800228976335163, 19.02544592524342804, 99.79057627198102409 ) ) ;
#17859=CARTESIAN_POINT ( 'NONE',  ( -16.46253265017160317, 9.564922557960807481, 50.83224293864770260 ) ) ;
#17860=CARTESIAN_POINT ( 'NONE',  ( -9.474510206698720793, -16.51473224551083518, 94.58442372801900433 ) ) ;
#17862=CARTESIAN_POINT ( 'NONE',  ( -21.52544592524343514, 5.823673210054127303, 41.04057627198103120 ) ) ;
#17863=CARTESIAN_POINT ( 'NONE',  ( -21.53943276465977519, -0.05219959533937600094, 63.75109039468568284 ) ) ;
#17864=CARTESIAN_POINT ( 'NONE',  ( -5.049401038298153566, 19.05341960407611168, 55.20724293864769550 ) ) ;
#17865=CARTESIAN_POINT ( 'NONE',  ( 5.049401038298161559, -19.05341960407611168, 82.70724293864770971 ) ) ;
#17866=CARTESIAN_POINT ( 'NONE',  ( 8.224510206698742110, 14.34966873604972548, 57.08442372801901854 ) ) ;
#17867=CARTESIAN_POINT ( 'NONE',  ( -15.72974639402176322, -15.80617190586768395, 44.37609039468567573 ) ) ;
#17868=CARTESIAN_POINT ( 'NONE',  ( 18.67979575497194134, -10.72451020669871369, 90.83442372801901854 ) ) ;
#17869=CARTESIAN_POINT ( 'NONE',  ( 21.55341960407610458, 5.719274019375980345, 103.9572429386476813 ) ) ;
#17871=CARTESIAN_POINT ( 'NONE',  ( 5.719274019375673035, 21.55341960407619339, 32.29275706135235424 ) ) ;
#17872=CARTESIAN_POINT ( 'NONE',  ( -16.52544592524335698, -4.483927247898792601, 63.95942372801901854 ) ) ;
#17873=CARTESIAN_POINT ( 'NONE',  ( -21.52544592524343514, 5.823673210054127303, 81.04057627198102409 ) ) ;
#17874=CARTESIAN_POINT ( 'NONE',  ( -13.97604488694547697, 13.89961937509957934, 33.12609039468566863 ) ) ;
#17875=CARTESIAN_POINT ( 'NONE',  ( 19.05341960407611168, 5.049401038298154454, 63.95724293864769550 ) ) ;
#17876=CARTESIAN_POINT ( 'NONE',  ( -0.05219959533934338120, 16.53943276465976808, 112.5010903946857042 ) ) ;
#17877=CARTESIAN_POINT ( 'NONE',  ( -17.49999999999999289, -3.209263204892650823, 105.2380317439373982 ) ) ;
#17878=CARTESIAN_POINT ( 'NONE',  ( -16.51473224551069308, -9.474510206698971260, 96.66557627198102409 ) ) ;
#17880=CARTESIAN_POINT ( 'NONE',  ( 19.05341960407617918, -5.049401038297876454, 81.04275706135231871 ) ) ;
#17881=CARTESIAN_POINT ( 'NONE',  ( -5.719274019375978568, 21.55341960407610458, 55.20724293864770260 ) ) ;
#17882=CARTESIAN_POINT ( 'NONE',  ( 16.55341960407611168, 4.379528057220329451, 33.95724293864769550 ) ) ;
#17883=CARTESIAN_POINT ( 'NONE',  ( 19.05341960407617918, -5.049401038297876454, 111.0427570613523329 ) ) ;
#17884=CARTESIAN_POINT ( 'NONE',  ( 9.564922557960805705, 16.46253265017160317, 34.58224293864770260 ) ) ;
#17885=CARTESIAN_POINT ( 'NONE',  ( -19.05341960407617563, 5.049401038297882671, 113.5427570613523471 ) ) ;
#17886=CARTESIAN_POINT ( 'NONE',  ( -10.72451020669898014, 18.67979575497178502, 95.41557627198102409 ) ) ;
#17887=CARTESIAN_POINT ( 'NONE',  ( 16.46253265017146816, 9.564922557961045513, 76.66775706135234714 ) ) ;
#17888=CARTESIAN_POINT ( 'NONE',  ( 0.05219959533934541429, -16.53943276465976808, 85.00109039468568994 ) ) ;
#17889=CARTESIAN_POINT ( 'NONE',  ( 0.05219959533909260263, 19.03943276465977164, 74.99890960531435269 ) ) ;
#17890=CARTESIAN_POINT ( 'NONE',  ( 4.379528057220339221, -16.55341960407611168, 82.70724293864770971 ) ) ;
#17891=CARTESIAN_POINT ( 'NONE',  ( 5.049401038298161559, -19.05341960407611168, 67.70724293864769550 ) ) ;
#17892=CARTESIAN_POINT ( 'NONE',  ( 14.29746914071049879, -8.314922557960816363, 63.33224293864770260 ) ) ;
#17893=PLANE ( 'NONE',  #167944 ) ;
#17894=CARTESIAN_POINT ( 'NONE',  ( -17.26832448383786200, -5.411067243102611890, 21.06455627637857830 ) ) ;
#17895=CARTESIAN_POINT ( 'NONE',  ( 14.29746914071049879, -8.314922557960816363, 38.33224293864768839 ) ) ;
#17896=CARTESIAN_POINT ( 'NONE',  ( -9.564922557960796823, -16.46253265017161027, 77.08224293864769550 ) ) ;
#17898=CARTESIAN_POINT ( 'NONE',  ( 19.05341960407617918, -5.049401038297876454, 41.04275706135233293 ) ) ;
#17899=CARTESIAN_POINT ( 'NONE',  ( 16.53943276465976808, 0.05219959533934440121, 41.25109039468568284 ) ) ;
#17900=CARTESIAN_POINT ( 'NONE',  ( 5.719274019375991003, -21.55341960407610458, 62.70724293864769550 ) ) ;
#17901=CARTESIAN_POINT ( 'NONE',  ( -5.049401038297874678, -19.05341960407617918, 24.79275706135233648 ) ) ;
#17902=CARTESIAN_POINT ( 'NONE',  ( -9.474510206698964154, 16.51473224551069663, 70.41557627198102409 ) ) ;
#17904=CARTESIAN_POINT ( 'NONE',  ( -5.153800228976328057, -19.02544592524343514, 112.2905762719810099 ) ) ;
#17905=CARTESIAN_POINT ( 'NONE',  ( -15.72974639402176322, -15.80617190586768395, 39.37609039468567573 ) ) ;
#17906=CARTESIAN_POINT ( 'NONE',  ( 12.14591786802309770, 12.06949235617756955, 104.3739096053143669 ) ) ;
#17907=CARTESIAN_POINT ( 'NONE',  ( -21.52544592524343514, 5.823673210054127303, 96.04057627198102409 ) ) ;
#17908=CARTESIAN_POINT ( 'NONE',  ( 19.03943276465977164, -0.05219959533909143690, 83.74890960531436690 ) ) ;
#17910=CARTESIAN_POINT ( 'NONE',  ( 21.53943276465977519, 0.05219959533937863772, 21.25109039468567218 ) ) ;
#17912=CARTESIAN_POINT ( 'NONE',  ( -13.97604488694527625, -13.89961937509977652, 86.87390960531436690 ) ) ;
#17913=CARTESIAN_POINT ( 'NONE',  ( 30.00000000000000000, -5.499999999999992895, 37.50000000000000000 ) ) ;
#17914=CARTESIAN_POINT ( 'NONE',  ( 21.52544592524344225, -5.823673210054117533, 93.54057627198103830 ) ) ;
#17915=CARTESIAN_POINT ( 'NONE',  ( 16.46253265017160672, -9.564922557960803928, 33.33224293864770260 ) ) ;
#17916=CARTESIAN_POINT ( 'NONE',  ( -9.564922557961040184, 16.46253265017147172, 107.9177570613523471 ) ) ;
#17918=CARTESIAN_POINT ( 'NONE',  ( 5.153800228976335163, 19.02544592524342804, 34.79057627198102409 ) ) ;
#17919=CARTESIAN_POINT ( 'NONE',  ( 21.52544592524334988, 5.823673210054432836, 86.45942372801901854 ) ) ;
#17920=CARTESIAN_POINT ( 'NONE',  ( 19.03943276465977164, -0.05219959533909143690, 73.74890960531435269 ) ) ;
#17921=CARTESIAN_POINT ( 'NONE',  ( 10.72451020669871369, 18.67979575497193778, 52.08442372801901854 ) ) ;
#17922=CARTESIAN_POINT ( 'NONE',  ( -21.53943276465977519, -0.05219959533937600094, 28.75109039468567929 ) ) ;
#17924=CARTESIAN_POINT ( 'NONE',  ( 9.474510206698971260, -16.51473224551069308, 82.91557627198103830 ) ) ;
#17925=CARTESIAN_POINT ( 'NONE',  ( 18.89770734986051437, 5.499999999999903189, 61.60214472496640781 ) ) ;
#17926=CARTESIAN_POINT ( 'NONE',  ( -14.29746914071037622, -8.314922557961029526, 34.16775706135234714 ) ) ;
#17927=CARTESIAN_POINT ( 'NONE',  ( -21.52544592524343514, 5.823673210054127303, 41.04057627198103120 ) ) ;
#17928=CARTESIAN_POINT ( 'NONE',  ( -15.80617190586768217, 15.72974639402176855, 43.12609039468568284 ) ) ;
#17929=CARTESIAN_POINT ( 'NONE',  ( -5.719274019375665041, -21.55341960407619695, 69.79275706135234714 ) ) ;
#17931=CARTESIAN_POINT ( 'NONE',  ( 19.03943276465977164, 0.05219959533936151252, 106.2510903946856615 ) ) ;
#17932=CARTESIAN_POINT ( 'NONE',  ( -9.474510206698964154, 16.51473224551069663, 55.41557627198103120 ) ) ;
#17933=CARTESIAN_POINT ( 'NONE',  ( 9.564922557960805705, 16.46253265017160317, 79.58224293864769550 ) ) ;
#17934=CARTESIAN_POINT ( 'NONE',  ( -12.14591786802309592, -12.06949235617757132, 106.8739096053143811 ) ) ;
#17935=CARTESIAN_POINT ( 'NONE',  ( -14.34966873604960291, -8.224510206698953496, 106.6655762719810383 ) ) ;
#17936=CARTESIAN_POINT ( 'NONE',  ( -13.97604488694527625, -13.89961937509977652, 106.8739096053143669 ) ) ;
#17937=CARTESIAN_POINT ( 'NONE',  ( -16.55341960407617563, 4.379528057220093196, 83.54275706135234714 ) ) ;
#17938=CARTESIAN_POINT ( 'NONE',  ( 16.53943276465976808, -0.05219959533910856209, 58.74890960531436690 ) ) ;
#17939=CARTESIAN_POINT ( 'NONE',  ( -19.02544592524342804, 5.153800228976336051, 51.04057627198103120 ) ) ;
#17940=CARTESIAN_POINT ( 'NONE',  ( -21.52544592524334988, -5.823673210054445271, 83.95942372801900433 ) ) ;
#17941=CARTESIAN_POINT ( 'NONE',  ( 0.05219959533937995610, -21.53943276465977519, 65.00109039468568994 ) ) ;
#17942=CARTESIAN_POINT ( 'NONE',  ( -5.049401038297874678, -19.05341960407617918, 109.7927570613523187 ) ) ;
#17943=CARTESIAN_POINT ( 'NONE',  ( -14.29746914071049879, 8.314922557960819915, 55.83224293864770260 ) ) ;
#17944=CARTESIAN_POINT ( 'NONE',  ( 0.05219959533907565091, 21.53943276465977519, 109.9989096053143527 ) ) ;
#17945=CARTESIAN_POINT ( 'NONE',  ( 10.81492255796078972, 18.62759615963270932, 59.58224293864770260 ) ) ;
#17947=CARTESIAN_POINT ( 'NONE',  ( -16.79531203550645913, -7.028104445595622529, 106.2524498822044592 ) ) ;
#17949=CARTESIAN_POINT ( 'NONE',  ( 19.03943276465977164, -0.05219959533909143690, 63.74890960531435979 ) ) ;
#17950=CARTESIAN_POINT ( 'NONE',  ( -0.05219959533910754901, -16.53943276465976808, 42.49890960531435979 ) ) ;
#17951=CARTESIAN_POINT ( 'NONE',  ( -8.224510206698735004, -14.34966873604973081, 109.5844237280190328 ) ) ;
#17952=CARTESIAN_POINT ( 'NONE',  ( -16.55341960407617563, 4.379528057220093196, 103.5427570613523613 ) ) ;
#17953=CARTESIAN_POINT ( 'NONE',  ( -9.474510206698720793, -16.51473224551083518, 49.58442372801899722 ) ) ;
#17954=CARTESIAN_POINT ( 'NONE',  ( 17.48853670773242541, 5.747243402303176651, 48.83328700250012133 ) ) ;
#17955=CARTESIAN_POINT ( 'NONE',  ( -9.564922557960796823, -16.46253265017161027, 92.08224293864769550 ) ) ;
#17956=CARTESIAN_POINT ( 'NONE',  ( -4.483927247898539470, -16.52544592524342804, 62.29057627198102409 ) ) ;
#17957=CARTESIAN_POINT ( 'NONE',  ( 18.22780087662119897, -5.500000000000096811, 48.51763182126894236 ) ) ;
#17958=CARTESIAN_POINT ( 'NONE',  ( -13.97604488694527625, -13.89961937509977652, 111.8739096053143243 ) ) ;
#17959=CARTESIAN_POINT ( 'NONE',  ( 15.72974639402199770, -15.80617190586745480, 53.12390960531436690 ) ) ;
#17960=CARTESIAN_POINT ( 'NONE',  ( -4.379528057220328563, 16.55341960407611168, 95.20724293864769550 ) ) ;
#17961=CARTESIAN_POINT ( 'NONE',  ( 8.314922557961029526, -14.29746914071037800, 45.41775706135234003 ) ) ;
#17962=CARTESIAN_POINT ( 'NONE',  ( -8.314922557960811034, -14.29746914071050412, 97.08224293864770971 ) ) ;
#17965=CARTESIAN_POINT ( 'NONE',  ( -13.97604488694547697, 13.89961937509957934, 83.12609039468564731 ) ) ;
#17966=CARTESIAN_POINT ( 'NONE',  ( 5.153800228976335163, 19.02544592524342804, 109.7905762719810099 ) ) ;
#17969=ORIENTED_EDGE ( 'NONE', *, *, #101326, .T. ) ;
#17970=CARTESIAN_POINT ( 'NONE',  ( 0.05219959533934541429, -16.53943276465976808, 40.00109039468567573 ) ) ;
#17971=CARTESIAN_POINT ( 'NONE',  ( -16.53943276465976808, 0.05219959533911058130, 31.24890960531435979 ) ) ;
#17972=CARTESIAN_POINT ( 'NONE',  ( -21.52544592524343514, 5.823673210054127303, 61.04057627198103120 ) ) ;
#17973=CARTESIAN_POINT ( 'NONE',  ( 16.46253265017146816, 9.564922557961045513, 81.66775706135233293 ) ) ;
#17974=CARTESIAN_POINT ( 'NONE',  ( 10.81492255796078972, 18.62759615963270932, 49.58224293864769550 ) ) ;
#17975=CARTESIAN_POINT ( 'NONE',  ( 5.719274019375673035, 21.55341960407619339, 87.29275706135236135 ) ) ;
#17977=CARTESIAN_POINT ( 'NONE',  ( -14.29746914071037622, -8.314922557961029526, 39.16775706135235424 ) ) ;
#17978=CARTESIAN_POINT ( 'NONE',  ( 19.02544592524343514, -5.153800228976328945, 38.54057627198103120 ) ) ;
#17979=CARTESIAN_POINT ( 'NONE',  ( -13.97604488694527625, -13.89961937509977652, 106.8739096053143669 ) ) ;
#17980=CARTESIAN_POINT ( 'NONE',  ( 9.564922557960805705, 16.46253265017160317, 29.58224293864769550 ) ) ;
#17981=CARTESIAN_POINT ( 'NONE',  ( 0.05219959533910956823, 16.53943276465976808, 104.9989096053143669 ) ) ;
#17984=CARTESIAN_POINT ( 'NONE',  ( -5.049401038298153566, 19.05341960407611168, 100.2072429386476955 ) ) ;
#17986=CARTESIAN_POINT ( 'NONE',  ( -12.14591786802326823, 12.06949235617739902, 53.12609039468568284 ) ) ;
#17987=CARTESIAN_POINT ( 'NONE',  ( -18.67979575497178146, -10.72451020669898902, 91.66557627198103830 ) ) ;
#17988=CARTESIAN_POINT ( 'NONE',  ( 16.51473224551069308, 9.474510206698969483, 49.16557627198102409 ) ) ;
#17989=CARTESIAN_POINT ( 'NONE',  ( -21.52544592524334988, -5.823673210054445271, 33.95942372801901143 ) ) ;
#17990=CARTESIAN_POINT ( 'NONE',  ( 16.51473224551069308, 9.474510206698969483, 79.16557627198103830 ) ) ;
#17992=ORIENTED_EDGE ( 'NONE', *, *, #154702, .T. ) ;
#17993=CARTESIAN_POINT ( 'NONE',  ( 14.34966873604972726, -8.224510206698740333, 50.83442372801901143 ) ) ;
#17994=CARTESIAN_POINT ( 'NONE',  ( -18.62759615963270932, 10.81492255796079327, 115.8322429386477097 ) ) ;
#17995=CARTESIAN_POINT ( 'NONE',  ( 16.55341960407611168, 4.379528057220329451, 108.9572429386476955 ) ) ;
#17996=CARTESIAN_POINT ( 'NONE',  ( 13.97604488694527802, 13.89961937509977652, 99.37390960531436690 ) ) ;
#17997=CARTESIAN_POINT ( 'NONE',  ( -9.474510206698720793, -16.51473224551083518, 74.58442372801900433 ) ) ;
#17998=CARTESIAN_POINT ( 'NONE',  ( -9.564922557961040184, 16.46253265017147172, 22.91775706135233648 ) ) ;
#17999=CARTESIAN_POINT ( 'NONE',  ( -0.05219959533907301413, -21.53943276465977519, 82.49890960531436690 ) ) ;
#18000=CARTESIAN_POINT ( 'NONE',  ( 13.89961937509957401, 13.97604488694547697, 36.87609039468565442 ) ) ;
#18001=CARTESIAN_POINT ( 'NONE',  ( -0.05219959533934338120, 16.53943276465976808, 82.50109039468568994 ) ) ;
#18002=CARTESIAN_POINT ( 'NONE',  ( -16.46253265017160317, 9.564922557960807481, 105.8322429386476955 ) ) ;
#18003=CARTESIAN_POINT ( 'NONE',  ( 9.564922557960805705, 16.46253265017160317, 59.58224293864769550 ) ) ;
#18004=CARTESIAN_POINT ( 'NONE',  ( 0.05219959533937995610, -21.53943276465977519, 65.00109039468568994 ) ) ;
#18005=CARTESIAN_POINT ( 'NONE',  ( 18.62759615963255655, 10.81492255796105972, 66.66775706135234714 ) ) ;
#18006=CARTESIAN_POINT ( 'NONE',  ( -13.89961937509977652, 13.97604488694528158, 70.62390960531432427 ) ) ;
#18007=CARTESIAN_POINT ( 'NONE',  ( -21.53943276465977519, -0.05219959533937600094, 43.75109039468568284 ) ) ;
#18008=CARTESIAN_POINT ( 'NONE',  ( 19.05341960407617918, -5.049401038297876454, 86.04275706135233293 ) ) ;
#18009=CARTESIAN_POINT ( 'NONE',  ( 9.564922557960805705, 16.46253265017160317, 49.58224293864770260 ) ) ;
#18010=CARTESIAN_POINT ( 'NONE',  ( -13.89961937509977652, 13.97604488694528158, 95.62390960531436690 ) ) ;
#18011=CARTESIAN_POINT ( 'NONE',  ( -9.564922557960796823, -16.46253265017161027, 72.08224293864770971 ) ) ;
#18012=CARTESIAN_POINT ( 'NONE',  ( 16.51473224551069308, 9.474510206698969483, 109.1655762719810383 ) ) ;
#18013=CARTESIAN_POINT ( 'NONE',  ( -5.153800228976328057, -19.02544592524343514, 52.29057627198100988 ) ) ;
#18015=CARTESIAN_POINT ( 'NONE',  ( 15.72974639402199770, -15.80617190586745480, 83.12390960531436690 ) ) ;
#18016=CARTESIAN_POINT ( 'NONE',  ( 0.05219959533934541429, -16.53943276465976808, 70.00109039468568994 ) ) ;
#18018=CARTESIAN_POINT ( 'NONE',  ( -13.89961937509957401, -13.97604488694547875, 34.37609039468566863 ) ) ;
#18019=CARTESIAN_POINT ( 'NONE',  ( -9.474510206698964154, 16.51473224551069663, 65.41557627198102409 ) ) ;
#18020=CARTESIAN_POINT ( 'NONE',  ( 8.224510206698953496, -14.34966873604960469, 57.91557627198103120 ) ) ;
#18021=CARTESIAN_POINT ( 'NONE',  ( 0.05219959533910956823, 16.53943276465976808, 99.99890960531436690 ) ) ;
#18022=CARTESIAN_POINT ( 'NONE',  ( 16.51473224551069308, 9.474510206698969483, 99.16557627198102409 ) ) ;
#18023=CARTESIAN_POINT ( 'NONE',  ( 13.89961937509977652, -13.97604488694527269, 93.12390960531436690 ) ) ;
#18024=CARTESIAN_POINT ( 'NONE',  ( 21.53943276465977519, 0.05219959533937863772, 51.25109039468568994 ) ) ;
#18025=CARTESIAN_POINT ( 'NONE',  ( 13.89961937509977652, -13.97604488694527269, 108.1239096053143669 ) ) ;
#18026=CARTESIAN_POINT ( 'NONE',  ( 5.049401038297881783, 19.05341960407617563, 22.29275706135233648 ) ) ;
#18027=CARTESIAN_POINT ( 'NONE',  ( 8.314922557961029526, -14.29746914071037800, 75.41775706135233293 ) ) ;
#18028=CARTESIAN_POINT ( 'NONE',  ( 10.72451020669871369, 18.67979575497193778, 37.08442372801901143 ) ) ;
#18029=CARTESIAN_POINT ( 'NONE',  ( 21.52544592524344225, -5.823673210054117533, 33.54057627198102409 ) ) ;
#18030=CARTESIAN_POINT ( 'NONE',  ( -5.823673210054116645, -21.52544592524344225, 107.2905762719810525 ) ) ;
#18031=CARTESIAN_POINT ( 'NONE',  ( -16.55341960407611168, -4.379528057220339221, 61.45724293864770260 ) ) ;
#18032=CARTESIAN_POINT ( 'NONE',  ( 13.97604488694527802, 13.89961937509977652, 49.37390960531434558 ) ) ;
#18033=CARTESIAN_POINT ( 'NONE',  ( -4.379528057220328563, 16.55341960407611168, 85.20724293864770971 ) ) ;
#18034=CARTESIAN_POINT ( 'NONE',  ( -18.62759615963270932, 10.81492255796079327, 40.83224293864769550 ) ) ;
#18035=CARTESIAN_POINT ( 'NONE',  ( 13.97604488694548053, -13.89961937509957401, 40.62609039468564731 ) ) ;
#18036=CARTESIAN_POINT ( 'NONE',  ( -4.379528057220328563, 16.55341960407611168, 115.2072429386476955 ) ) ;
#18038=CARTESIAN_POINT ( 'NONE',  ( -12.14591786802326823, 12.06949235617739902, 68.12609039468567573 ) ) ;
#18039=CARTESIAN_POINT ( 'NONE',  ( 9.474510206698971260, -16.51473224551069308, 72.91557627198102409 ) ) ;
#18041=CARTESIAN_POINT ( 'NONE',  ( 14.29746914071049879, -8.314922557960816363, 83.33224293864769550 ) ) ;
#18042=CARTESIAN_POINT ( 'NONE',  ( -18.62759615963270932, 10.81492255796079327, 40.83224293864769550 ) ) ;
#18044=CARTESIAN_POINT ( 'NONE',  ( 4.483927247898790824, -16.52544592524335698, 110.2094237280190185 ) ) ;
#18045=CARTESIAN_POINT ( 'NONE',  ( -12.06949235617739369, -12.14591786802326823, 19.37609039468568639 ) ) ;
#18046=CARTESIAN_POINT ( 'NONE',  ( 0.05219959533937995610, -21.53943276465977519, 85.00109039468568994 ) ) ;
#18047=CARTESIAN_POINT ( 'NONE',  ( 19.02544592524343514, -5.153800228976328945, 88.54057627198102409 ) ) ;
#18048=CARTESIAN_POINT ( 'NONE',  ( -18.62759615963270932, 10.81492255796079327, 100.8322429386477097 ) ) ;
#18049=CARTESIAN_POINT ( 'NONE',  ( 12.06949235617739724, 12.14591786802326823, 56.87609039468568994 ) ) ;
#18050=CARTESIAN_POINT ( 'NONE',  ( -19.05341960407611168, -5.049401038298163336, 31.45724293864769550 ) ) ;
#18052=CARTESIAN_POINT ( 'NONE',  ( -4.379528057220086978, -16.55341960407618274, 29.79275706135234358 ) ) ;
#18053=CARTESIAN_POINT ( 'NONE',  ( 19.02544592524334988, 5.153800228976608722, 96.45942372801897591 ) ) ;
#18054=CARTESIAN_POINT ( 'NONE',  ( -21.55341960407610458, -5.719274019375992779, 91.45724293864769550 ) ) ;
#18055=CARTESIAN_POINT ( 'NONE',  ( -5.153800228976607833, 19.02544592524334988, 72.70942372801900433 ) ) ;
#18056=CARTESIAN_POINT ( 'NONE',  ( 19.53037848336980886, -5.499999999999891642, 87.35532783611442653 ) ) ;
#18057=CARTESIAN_POINT ( 'NONE',  ( 18.62759615963271287, -10.81492255796078972, 103.3322429386476955 ) ) ;
#18058=CARTESIAN_POINT ( 'NONE',  ( 0.05219959533909260263, 19.03943276465977164, 79.99890960531436690 ) ) ;
#18059=CARTESIAN_POINT ( 'NONE',  ( 14.29746914071037800, 8.314922557961029526, 31.66775706135234358 ) ) ;
#18061=CARTESIAN_POINT ( 'NONE',  ( 19.05341960407617918, -5.049401038297876454, 56.04275706135234714 ) ) ;
#18062=CARTESIAN_POINT ( 'NONE',  ( 15.80617190586769283, -15.72974639402175789, 20.62609039468568639 ) ) ;
#18063=CARTESIAN_POINT ( 'NONE',  ( -14.34966873604960291, -8.224510206698953496, 66.66557627198102409 ) ) ;
#18064=CARTESIAN_POINT ( 'NONE',  ( 19.05341960407611168, 5.049401038298154454, 78.95724293864769550 ) ) ;
#18065=CARTESIAN_POINT ( 'NONE',  ( 0.05219959533934541429, -16.53943276465976808, 40.00109039468567573 ) ) ;
#18066=CARTESIAN_POINT ( 'NONE',  ( -9.564922557961040184, 16.46253265017147172, 47.91775706135233293 ) ) ;
#18067=CARTESIAN_POINT ( 'NONE',  ( 5.823673210054444382, -21.52544592524334988, 55.20942372801902565 ) ) ;
#18068=CARTESIAN_POINT ( 'NONE',  ( -5.049401038297874678, -19.05341960407617918, 109.7927570613523187 ) ) ;
#18069=CARTESIAN_POINT ( 'NONE',  ( 13.89961937509977652, -13.97604488694527269, 53.12390960531434558 ) ) ;
#18070=CARTESIAN_POINT ( 'NONE',  ( 19.03943276465977164, 0.05219959533936151252, 76.25109039468566152 ) ) ;
#18071=CARTESIAN_POINT ( 'NONE',  ( -21.53943276465977519, -0.05219959533937600094, 93.75109039468567573 ) ) ;
#18072=CARTESIAN_POINT ( 'NONE',  ( -16.46253265017146816, -9.564922557961047289, 69.16775706135233293 ) ) ;
#18073=CARTESIAN_POINT ( 'NONE',  ( -19.02544592524342804, 5.153800228976336051, 31.04057627198102409 ) ) ;
#18074=CARTESIAN_POINT ( 'NONE',  ( -5.719274019375978568, 21.55341960407610458, 75.20724293864769550 ) ) ;
#18075=CARTESIAN_POINT ( 'NONE',  ( 4.483927247898545687, 16.52544592524342804, 59.79057627198103120 ) ) ;
#18076=CARTESIAN_POINT ( 'NONE',  ( -13.97604488694547697, 13.89961937509957934, 68.12609039468563310 ) ) ;
#18077=CARTESIAN_POINT ( 'NONE',  ( -17.05587630539788435, -6.762274262135648861, 24.25819690962687858 ) ) ;
#18078=CARTESIAN_POINT ( 'NONE',  ( -5.049401038297874678, -19.05341960407617918, 49.79275706135231871 ) ) ;
#18079=CARTESIAN_POINT ( 'NONE',  ( 14.29746914071037800, 8.314922557961029526, 96.66775706135234714 ) ) ;
#18080=CARTESIAN_POINT ( 'NONE',  ( 4.379528057220339221, -16.55341960407611168, 57.70724293864770260 ) ) ;
#18081=CARTESIAN_POINT ( 'NONE',  ( 5.823673210054444382, -21.52544592524334988, 90.20942372801903275 ) ) ;
#18083=CARTESIAN_POINT ( 'NONE',  ( 0.05219959533907565091, 21.53943276465977519, 99.99890960531436690 ) ) ;
#18084=CARTESIAN_POINT ( 'NONE',  ( 19.03943276465977164, -0.05219959533909143690, 48.74890960531435979 ) ) ;
#18085=CARTESIAN_POINT ( 'NONE',  ( 18.67979575497194134, -10.72451020669871369, 70.83442372801901854 ) ) ;
#18086=CARTESIAN_POINT ( 'NONE',  ( 9.474510206698971260, -16.51473224551069308, 47.91557627198102409 ) ) ;
#18087=CARTESIAN_POINT ( 'NONE',  ( -16.51473224551069308, -9.474510206698971260, 71.66557627198102409 ) ) ;
#18088=CARTESIAN_POINT ( 'NONE',  ( 4.483927247898545687, 16.52544592524342804, 104.7905762719810241 ) ) ;
#18089=CARTESIAN_POINT ( 'NONE',  ( -16.46253265017160317, 9.564922557960807481, 105.8322429386476955 ) ) ;
#18091=CARTESIAN_POINT ( 'NONE',  ( 4.379528057220339221, -16.55341960407611168, 52.70724293864769550 ) ) ;
#18092=CARTESIAN_POINT ( 'NONE',  ( -19.03943276465977164, 0.05219959533909376836, 36.24890960531436690 ) ) ;
#18093=CARTESIAN_POINT ( 'NONE',  ( -14.29746914071049879, 8.314922557960819915, 80.83224293864769550 ) ) ;
#18094=CARTESIAN_POINT ( 'NONE',  ( 18.62759615963271287, -10.81492255796078972, 98.33224293864769550 ) ) ;
#18095=CARTESIAN_POINT ( 'NONE',  ( -18.62759615963255300, -10.81492255796106328, 29.16775706135234003 ) ) ;
#18097=CARTESIAN_POINT ( 'NONE',  ( -16.52544592524335698, -4.483927247898792601, 43.95942372801902565 ) ) ;
#18098=CARTESIAN_POINT ( 'NONE',  ( -21.53943276465977519, 0.05219959533907696930, 81.24890960531436690 ) ) ;
#18099=CARTESIAN_POINT ( 'NONE',  ( 21.52544592524334988, 5.823673210054432836, 111.4594237280190328 ) ) ;
#18100=B_SPLINE_CURVE_WITH_KNOTS ( 'NONE', 3,
 ( #37647, #175169, #68984, #145816, #111499, #50832 ),
 .UNSPECIFIED., .F., .F.,
 ( 4, 2, 4 ),
 ( 0.007228050697041550100, 0.007608510107495039532, 0.007988969517948528096 ),
 .UNSPECIFIED. ) ;
#18101=CARTESIAN_POINT ( 'NONE',  ( 19.05341960407611168, 5.049401038298154454, 108.9572429386477097 ) ) ;
#18102=CARTESIAN_POINT ( 'NONE',  ( -10.81492255796105439, 18.62759615963255655, 37.91775706135235424 ) ) ;
#18103=CARTESIAN_POINT ( 'NONE',  ( -5.823673210054116645, -21.52544592524344225, 37.29057627198102409 ) ) ;
#18104=CARTESIAN_POINT ( 'NONE',  ( 4.483927247898790824, -16.52544592524335698, 110.2094237280190185 ) ) ;
#18105=CARTESIAN_POINT ( 'NONE',  ( -18.62759615963255300, -10.81492255796106328, 69.16775706135234714 ) ) ;
#18106=CARTESIAN_POINT ( 'NONE',  ( 15.80617190586769283, -15.72974639402175789, 85.62609039468568994 ) ) ;
#18107=CARTESIAN_POINT ( 'NONE',  ( -19.05341960407617563, 5.049401038297882671, 33.54275706135231871 ) ) ;
#18108=CARTESIAN_POINT ( 'NONE',  ( -8.224510206698735004, -14.34966873604973081, 94.58442372801901854 ) ) ;
#18109=CARTESIAN_POINT ( 'NONE',  ( -10.81492255796105439, 18.62759615963255655, 37.91775706135235424 ) ) ;
#18110=CARTESIAN_POINT ( 'NONE',  ( -5.049401038298153566, 19.05341960407611168, 50.20724293864770260 ) ) ;
#18111=CARTESIAN_POINT ( 'NONE',  ( 15.80617190586769283, -15.72974639402175789, 105.6260903946856899 ) ) ;
#18112=CARTESIAN_POINT ( 'NONE',  ( 5.823673210054125526, 21.52544592524343514, 24.79057627198103120 ) ) ;
#18113=CARTESIAN_POINT ( 'NONE',  ( 10.81492255796106328, -18.62759615963255655, 25.41775706135235779 ) ) ;
#18114=CARTESIAN_POINT ( 'NONE',  ( 15.80617190586746368, 15.72974639402197994, 79.37390960531436690 ) ) ;
#18115=CARTESIAN_POINT ( 'NONE',  ( 17.50000000000000000, 5.499999999999997335, 120.0000000000000142 ) ) ;
#18116=CARTESIAN_POINT ( 'NONE',  ( -21.55341960407610458, -5.719274019375992779, 66.45724293864768129 ) ) ;
#18117=CARTESIAN_POINT ( 'NONE',  ( 8.224510206698742110, 14.34966873604972548, 57.08442372801901854 ) ) ;
#18118=CARTESIAN_POINT ( 'NONE',  ( 4.483927247898545687, 16.52544592524342804, 59.79057627198103120 ) ) ;
#18120=CARTESIAN_POINT ( 'NONE',  ( -9.564922557961040184, 16.46253265017147172, 87.91775706135233293 ) ) ;
#18122=CARTESIAN_POINT ( 'NONE',  ( -16.52544592524335698, -4.483927247898792601, 28.95942372801902209 ) ) ;
#18123=CARTESIAN_POINT ( 'NONE',  ( -18.67979575497178146, -10.72451020669898902, 101.6655762719810383 ) ) ;
#18124=CARTESIAN_POINT ( 'NONE',  ( 10.72451020669898902, -18.67979575497178502, 72.91557627198103830 ) ) ;
#18125=CARTESIAN_POINT ( 'NONE',  ( 13.89961937509977652, -13.97604488694527269, 113.1239096053143527 ) ) ;
#18126=CARTESIAN_POINT ( 'NONE',  ( -12.14591786802326823, 12.06949235617739902, 63.12609039468568994 ) ) ;
#18127=CARTESIAN_POINT ( 'NONE',  ( -5.049401038298153566, 19.05341960407611168, 70.20724293864769550 ) ) ;
#18128=CARTESIAN_POINT ( 'NONE',  ( -5.719274019375665041, -21.55341960407619695, 39.79275706135235424 ) ) ;
#18129=CARTESIAN_POINT ( 'NONE',  ( 16.46253265017146816, 9.564922557961045513, 111.6677570613523329 ) ) ;
#18131=CARTESIAN_POINT ( 'NONE',  ( 19.03943276465977164, -0.05219959533909143690, 103.7489096053143669 ) ) ;
#18132=CARTESIAN_POINT ( 'NONE',  ( 16.51473224551083163, -9.474510206698727899, 30.83442372801900433 ) ) ;
#18133=CARTESIAN_POINT ( 'NONE',  ( -19.02544592524342804, 5.153800228976336051, 96.04057627198103830 ) ) ;
#18134=CARTESIAN_POINT ( 'NONE',  ( -10.81492255796078084, -18.62759615963271287, 102.0822429386476955 ) ) ;
#18135=CARTESIAN_POINT ( 'NONE',  ( 19.05341960407611168, 5.049401038298154454, 63.95724293864769550 ) ) ;
#18136=CARTESIAN_POINT ( 'NONE',  ( -16.38665767535054485, 7.295008042176029939, 25.26400864214546971 ) ) ;
#18137=CARTESIAN_POINT ( 'NONE',  ( -14.34966873604960291, -8.224510206698953496, 76.66557627198103830 ) ) ;
#18138=CARTESIAN_POINT ( 'NONE',  ( -13.89961937509977652, 13.97604488694528158, 110.6239096053143243 ) ) ;
#18139=CARTESIAN_POINT ( 'NONE',  ( -19.03943276465977164, 0.05219959533909376836, 21.24890960531436335 ) ) ;
#18140=CARTESIAN_POINT ( 'NONE',  ( 0.05219959533907565091, 21.53943276465977519, 109.9989096053143527 ) ) ;
#18141=CARTESIAN_POINT ( 'NONE',  ( -16.51473224551082808, 9.474510206698731452, 58.33442372801900433 ) ) ;
#18143=CARTESIAN_POINT ( 'NONE',  ( 9.564922557960805705, 16.46253265017160317, 109.5822429386476955 ) ) ;
#18144=CARTESIAN_POINT ( 'NONE',  ( 19.02544592524343514, -5.153800228976328945, 33.54057627198102409 ) ) ;
#18145=CARTESIAN_POINT ( 'NONE',  ( 21.52544592524344225, -5.823673210054117533, 53.54057627198103120 ) ) ;
#18146=CARTESIAN_POINT ( 'NONE',  ( -13.97604488694527625, -13.89961937509977652, 96.87390960531433848 ) ) ;
#18147=CARTESIAN_POINT ( 'NONE',  ( -10.81492255796105439, 18.62759615963255655, 72.91775706135234714 ) ) ;
#18148=CARTESIAN_POINT ( 'NONE',  ( -16.46253265017160317, 9.564922557960807481, 55.83224293864769550 ) ) ;
#18149=CARTESIAN_POINT ( 'NONE',  ( 16.52544592524342804, -4.483927247898539470, 88.54057627198103830 ) ) ;
#18150=CARTESIAN_POINT ( 'NONE',  ( 8.224510206698742110, 14.34966873604972548, 42.08442372801901854 ) ) ;
#18151=CARTESIAN_POINT ( 'NONE',  ( 15.72974639402176855, 15.80617190586768217, 61.87609039468568284 ) ) ;
#18153=CARTESIAN_POINT ( 'NONE',  ( -5.049401038297874678, -19.05341960407617918, 19.79275706135233293 ) ) ;
#18154=CARTESIAN_POINT ( 'NONE',  ( 5.153800228976615827, -19.02544592524334988, 80.20942372801901854 ) ) ;
#18155=CARTESIAN_POINT ( 'NONE',  ( -16.46253265017146816, -9.564922557961047289, 39.16775706135234003 ) ) ;
#18156=SPHERICAL_SURFACE ( 'NONE', #56879, 2.000000000000000000 ) ;
#18157=CARTESIAN_POINT ( 'NONE',  ( 21.53943276465977519, 0.05219959533937863772, 36.25109039468567573 ) ) ;
#18159=CARTESIAN_POINT ( 'NONE',  ( -9.474510206698720793, -16.51473224551083518, 34.58442372801899722 ) ) ;
#18160=CARTESIAN_POINT ( 'NONE',  ( -16.46253265017160317, 9.564922557960807481, 65.83224293864769550 ) ) ;
#18161=CARTESIAN_POINT ( 'NONE',  ( -16.53943276465976808, 0.05219959533911058130, 21.24890960531436690 ) ) ;
#18162=CARTESIAN_POINT ( 'NONE',  ( -13.97604488694527625, -13.89961937509977652, 111.8739096053143243 ) ) ;
#18163=CARTESIAN_POINT ( 'NONE',  ( 15.80617190586769283, -15.72974639402175789, 90.62609039468567573 ) ) ;
#18166=CARTESIAN_POINT ( 'NONE',  ( 21.55341960407619695, -5.719274019375665929, 86.04275706135236135 ) ) ;
#18168=CARTESIAN_POINT ( 'NONE',  ( -9.474510206698964154, 16.51473224551069663, 95.41557627198102409 ) ) ;
#18170=CARTESIAN_POINT ( 'NONE',  ( -9.474510206698964154, 16.51473224551069663, 50.41557627198102409 ) ) ;
#18171=CARTESIAN_POINT ( 'NONE',  ( -21.55341960407610458, -5.719274019375992779, 51.45724293864770260 ) ) ;
#18172=CARTESIAN_POINT ( 'NONE',  ( -12.14591786802309592, -12.06949235617757132, 31.87390960531435979 ) ) ;
#18173=CARTESIAN_POINT ( 'NONE',  ( 16.53943276465976808, -0.05219959533910856209, 113.7489096053143527 ) ) ;
#18174=CARTESIAN_POINT ( 'NONE',  ( -16.46253265017160317, 9.564922557960807481, 90.83224293864769550 ) ) ;
#18175=CARTESIAN_POINT ( 'NONE',  ( 19.02544592524334988, 5.153800228976608722, 21.45942372801899012 ) ) ;
#18176=CARTESIAN_POINT ( 'NONE',  ( -14.34966873604960291, -8.224510206698953496, 96.66557627198102409 ) ) ;
#18177=CARTESIAN_POINT ( 'NONE',  ( -21.52544592524334988, -5.823673210054445271, 68.95942372801901854 ) ) ;
#18178=CARTESIAN_POINT ( 'NONE',  ( 9.474510206698971260, -16.51473224551069308, 97.91557627198102409 ) ) ;
#18179=CARTESIAN_POINT ( 'NONE',  ( -12.06949235617739369, -12.14591786802326823, 104.3760903946856899 ) ) ;
#18180=CARTESIAN_POINT ( 'NONE',  ( 19.02544592524334988, 5.153800228976608722, 66.45942372801899012 ) ) ;
#18182=CARTESIAN_POINT ( 'NONE',  ( 19.02544592524343514, -5.153800228976328945, 113.5405762719810241 ) ) ;
#18183=CARTESIAN_POINT ( 'NONE',  ( 4.379528057220339221, -16.55341960407611168, 77.70724293864770971 ) ) ;
#18185=CARTESIAN_POINT ( 'NONE',  ( 5.153800228976615827, -19.02544592524334988, 55.20942372801899722 ) ) ;
#18186=CARTESIAN_POINT ( 'NONE',  ( 9.474510206698971260, -16.51473224551069308, 57.91557627198103120 ) ) ;
#18187=CARTESIAN_POINT ( 'NONE',  ( -16.53943276465976808, 0.05219959533911058130, 66.24890960531436690 ) ) ;
#18188=CARTESIAN_POINT ( 'NONE',  ( 13.89961937509957401, 13.97604488694547697, 91.87609039468567573 ) ) ;
#18189=CARTESIAN_POINT ( 'NONE',  ( -21.53943276465977519, 0.05219959533907696930, 51.24890960531436690 ) ) ;
#18191=CARTESIAN_POINT ( 'NONE',  ( 16.55341960407611168, 4.379528057220329451, 108.9572429386476955 ) ) ;
#18192=CARTESIAN_POINT ( 'NONE',  ( -17.05587630539784172, -6.762274262135713698, 29.25819690962689279 ) ) ;
#18193=CARTESIAN_POINT ( 'NONE',  ( -13.97604488694527625, -13.89961937509977652, 61.87390960531435979 ) ) ;
#18194=CARTESIAN_POINT ( 'NONE',  ( 21.52544592524344225, -5.823673210054117533, 58.54057627198103120 ) ) ;
#18195=CARTESIAN_POINT ( 'NONE',  ( 4.379528057220092307, 16.55341960407617563, 97.29275706135234714 ) ) ;
#18196=CARTESIAN_POINT ( 'NONE',  ( 19.03943276465977164, -0.05219959533909143690, 78.74890960531436690 ) ) ;
#18197=CARTESIAN_POINT ( 'NONE',  ( -16.51473224551082808, 9.474510206698731452, 48.33442372801900433 ) ) ;
#18198=CARTESIAN_POINT ( 'NONE',  ( 10.72451020669871369, 18.67979575497193778, 87.08442372801901854 ) ) ;
#18199=CARTESIAN_POINT ( 'NONE',  ( 15.80617190586746368, 15.72974639402197994, 59.37390960531436690 ) ) ;
#18200=CARTESIAN_POINT ( 'NONE',  ( 16.51473224551069308, 9.474510206698969483, 104.1655762719810241 ) ) ;
#18201=CARTESIAN_POINT ( 'NONE',  ( -0.05219959533909027116, -19.03943276465977164, 37.49890960531436690 ) ) ;
#18202=CARTESIAN_POINT ( 'NONE',  ( -4.483927247898782831, 16.52544592524335698, 92.70942372801901854 ) ) ;
#18203=CARTESIAN_POINT ( 'NONE',  ( -12.14591786802326823, 12.06949235617739902, 23.12609039468567573 ) ) ;
#18205=CARTESIAN_POINT ( 'NONE',  ( 0.05219959533937995610, -21.53943276465977519, 95.00109039468568994 ) ) ;
#18206=CARTESIAN_POINT ( 'NONE',  ( 16.53943276465976808, -0.05219959533910856209, 63.74890960531435979 ) ) ;
#18207=CARTESIAN_POINT ( 'NONE',  ( 4.379528057220339221, -16.55341960407611168, 67.70724293864769550 ) ) ;
#18208=CARTESIAN_POINT ( 'NONE',  ( 0.05219959533907565091, 21.53943276465977519, 99.99890960531436690 ) ) ;
#18209=CARTESIAN_POINT ( 'NONE',  ( 21.55341960407610458, 5.719274019375980345, 88.95724293864769550 ) ) ;
#18210=CARTESIAN_POINT ( 'NONE',  ( 16.81555441253552630, -7.025013491695473178, 98.13685445334257906 ) ) ;
#18211=CARTESIAN_POINT ( 'NONE',  ( -21.53943276465977519, 0.05219959533907696930, 46.24890960531435979 ) ) ;
#18212=CARTESIAN_POINT ( 'NONE',  ( -8.314922557961024197, 14.29746914071037800, 62.91775706135236135 ) ) ;
#18213=CARTESIAN_POINT ( 'NONE',  ( 0.05219959533910956823, 16.53943276465976808, 89.99890960531438111 ) ) ;
#18214=CARTESIAN_POINT ( 'NONE',  ( -19.05341960407611168, -5.049401038298163336, 46.45724293864768129 ) ) ;
#18215=SURFACE_SIDE_STYLE ('',( #60714 ) ) ;
#18217=CARTESIAN_POINT ( 'NONE',  ( 12.14591786802327356, -12.06949235617739191, 95.62609039468568994 ) ) ;
#18219=CARTESIAN_POINT ( 'NONE',  ( 21.55341960407619695, -5.719274019375665929, 36.04275706135234714 ) ) ;
#18220=CARTESIAN_POINT ( 'NONE',  ( -16.51473224551069308, -9.474510206698971260, 81.66557627198103830 ) ) ;
#18221=CARTESIAN_POINT ( 'NONE',  ( -21.52544592524334988, -5.823673210054445271, 63.95942372801901854 ) ) ;
#18225=CARTESIAN_POINT ( 'NONE',  ( -21.55341960407619339, 5.719274019375674811, 63.54275706135234003 ) ) ;
#18226=CARTESIAN_POINT ( 'NONE',  ( 9.474510206698971260, -16.51473224551069308, 32.91557627198102409 ) ) ;
#18227=CARTESIAN_POINT ( 'NONE',  ( -19.03943276465977164, 0.05219959533909376836, 21.24890960531436335 ) ) ;
#18228=CARTESIAN_POINT ( 'NONE',  ( 19.03943276465977164, -0.05219959533909143690, 88.74890960531436690 ) ) ;
#18229=CARTESIAN_POINT ( 'NONE',  ( -9.474510206698720793, -16.51473224551083518, 64.58442372801900433 ) ) ;
#18230=CARTESIAN_POINT ( 'NONE',  ( 5.719274019375673035, 21.55341960407619339, 32.29275706135235424 ) ) ;
#18232=CARTESIAN_POINT ( 'NONE',  ( 0.05219959533936267826, -19.03943276465977164, 55.00109039468566863 ) ) ;
#18233=CARTESIAN_POINT ( 'NONE',  ( -0.05219959533909027116, -19.03943276465977164, 32.49890960531435979 ) ) ;
#18234=CARTESIAN_POINT ( 'NONE',  ( 12.06949235617739724, 12.14591786802326823, 106.8760903946856899 ) ) ;
#18235=CARTESIAN_POINT ( 'NONE',  ( 19.02544592524334988, 5.153800228976608722, 76.45942372801897591 ) ) ;
#18236=CARTESIAN_POINT ( 'NONE',  ( -16.55341960407611168, -4.379528057220339221, 21.45724293864769550 ) ) ;
#18237=CARTESIAN_POINT ( 'NONE',  ( 9.474510206698729675, 16.51473224551082808, 57.08442372801900433 ) ) ;
#18238=CARTESIAN_POINT ( 'NONE',  ( -9.564922557960796823, -16.46253265017161027, 102.0822429386477097 ) ) ;
#18240=CARTESIAN_POINT ( 'NONE',  ( 21.52544592524334988, 5.823673210054432836, 101.4594237280190185 ) ) ;
#18241=CARTESIAN_POINT ( 'NONE',  ( 18.67979575497194134, -10.72451020669871369, 105.8344237280190328 ) ) ;
#18242=CARTESIAN_POINT ( 'NONE',  ( 13.97604488694527802, 13.89961937509977652, 24.37390960531435624 ) ) ;
#18243=CARTESIAN_POINT ( 'NONE',  ( 15.72974639402176855, 15.80617190586768217, 91.87609039468568994 ) ) ;
#18244=CARTESIAN_POINT ( 'NONE',  ( 14.34966873604972726, -8.224510206698740333, 30.83442372801902209 ) ) ;
#18245=CARTESIAN_POINT ( 'NONE',  ( 19.05341960407611168, 5.049401038298154454, 93.95724293864769550 ) ) ;
#18247=CARTESIAN_POINT ( 'NONE',  ( 0.05219959533909260263, 19.03943276465977164, 84.99890960531436690 ) ) ;
#18249=CARTESIAN_POINT ( 'NONE',  ( 9.564922557961047289, -16.46253265017146816, 65.41775706135233293 ) ) ;
#18250=CARTESIAN_POINT ( 'NONE',  ( -5.153800228976328057, -19.02544592524343514, 107.2905762719810383 ) ) ;
#18251=CARTESIAN_POINT ( 'NONE',  ( 5.823673210054444382, -21.52544592524334988, 105.2094237280190328 ) ) ;
#18252=CARTESIAN_POINT ( 'NONE',  ( -4.379528057220328563, 16.55341960407611168, 100.2072429386476955 ) ) ;
#18253=CARTESIAN_POINT ( 'NONE',  ( 18.62759615963271287, -10.81492255796078972, 48.33224293864770260 ) ) ;
#18254=CARTESIAN_POINT ( 'NONE',  ( -21.53943276465977519, 0.05219959533907696930, 36.24890960531435979 ) ) ;
#18255=CARTESIAN_POINT ( 'NONE',  ( -4.483927247898539470, -16.52544592524342804, 102.2905762719810383 ) ) ;
#18257=CARTESIAN_POINT ( 'NONE',  ( -5.049401038297874678, -19.05341960407617918, 54.79275706135234003 ) ) ;
#18258=CARTESIAN_POINT ( 'NONE',  ( -16.55341960407617563, 4.379528057220093196, 113.5427570613523756 ) ) ;
#18259=CARTESIAN_POINT ( 'NONE',  ( -16.46253265017160317, 9.564922557960807481, 110.8322429386476955 ) ) ;
#18260=CARTESIAN_POINT ( 'NONE',  ( -21.55341960407619339, 5.719274019375674811, 78.54275706135236135 ) ) ;
#18261=CARTESIAN_POINT ( 'NONE',  ( -5.719274019375978568, 21.55341960407610458, 75.20724293864769550 ) ) ;
#18262=CARTESIAN_POINT ( 'NONE',  ( 10.81492255796106328, -18.62759615963255655, 40.41775706135234714 ) ) ;
#18263=CARTESIAN_POINT ( 'NONE',  ( -21.55341960407610458, -5.719274019375992779, 91.45724293864769550 ) ) ;
#18264=CARTESIAN_POINT ( 'NONE',  ( 10.72451020669871369, 18.67979575497193778, 52.08442372801901854 ) ) ;
#18265=CARTESIAN_POINT ( 'NONE',  ( -16.52544592524342804, 4.483927247898546575, 116.0405762719810383 ) ) ;
#18266=CARTESIAN_POINT ( 'NONE',  ( -19.02544592524342804, 5.153800228976336051, 81.04057627198103830 ) ) ;
#18267=CARTESIAN_POINT ( 'NONE',  ( 14.34966873604972726, -8.224510206698740333, 85.83442372801901854 ) ) ;
#18268=CARTESIAN_POINT ( 'NONE',  ( 8.224510206698953496, -14.34966873604960469, 102.9155762719810383 ) ) ;
#18269=CARTESIAN_POINT ( 'NONE',  ( -9.474510206698964154, 16.51473224551069663, 105.4155762719810383 ) ) ;
#18270=CARTESIAN_POINT ( 'NONE',  ( 16.55341960407611168, 4.379528057220329451, 53.95724293864770260 ) ) ;
#18271=CARTESIAN_POINT ( 'NONE',  ( 16.52544592524342804, -4.483927247898539470, 23.54057627198102765 ) ) ;
#18272=CARTESIAN_POINT ( 'NONE',  ( -16.46253265017160317, 9.564922557960807481, 65.83224293864769550 ) ) ;
#18273=CARTESIAN_POINT ( 'NONE',  ( -9.564922557960796823, -16.46253265017161027, 32.08224293864769550 ) ) ;
#18274=CARTESIAN_POINT ( 'NONE',  ( 10.81492255796078972, 18.62759615963270932, 49.58224293864769550 ) ) ;
#18275=CARTESIAN_POINT ( 'NONE',  ( -13.97604488694547697, 13.89961937509957934, 38.12609039468566152 ) ) ;
#18277=CARTESIAN_POINT ( 'NONE',  ( -16.52544592524342804, 4.483927247898546575, 41.04057627198103120 ) ) ;
#18278=CARTESIAN_POINT ( 'NONE',  ( -13.97604488694527625, -13.89961937509977652, 101.8739096053143811 ) ) ;
#18279=CARTESIAN_POINT ( 'NONE',  ( 15.80617190586769283, -15.72974639402175789, 60.62609039468567573 ) ) ;
#18280=FACE_OUTER_BOUND ( 'NONE', #95042, .T. ) ;
#18281=CARTESIAN_POINT ( 'NONE',  ( 8.314922557961029526, -14.29746914071037800, 55.41775706135234714 ) ) ;
#18282=CARTESIAN_POINT ( 'NONE',  ( 9.564922557961047289, -16.46253265017146816, 60.41775706135233293 ) ) ;
#18283=CARTESIAN_POINT ( 'NONE',  ( -16.52544592524342804, 4.483927247898546575, 26.04057627198103475 ) ) ;
#18284=LINE ( 'NONE', #79939, #133748 ) ;
#18285=CARTESIAN_POINT ( 'NONE',  ( -12.06949235617739369, -12.14591786802326823, 104.3760903946856899 ) ) ;
#18286=CARTESIAN_POINT ( 'NONE',  ( 9.564922557960805705, 16.46253265017160317, 34.58224293864770260 ) ) ;
#18287=CARTESIAN_POINT ( 'NONE',  ( -19.02544592524342804, 5.153800228976336051, 66.04057627198103830 ) ) ;
#18288=CARTESIAN_POINT ( 'NONE',  ( 5.049401038298161559, -19.05341960407611168, 32.70724293864768129 ) ) ;
#18289=CARTESIAN_POINT ( 'NONE',  ( 10.72451020669871369, 18.67979575497193778, 32.08442372801901854 ) ) ;
#18290=CARTESIAN_POINT ( 'NONE',  ( 16.51473224551069308, 9.474510206698969483, 49.16557627198102409 ) ) ;
#18291=CARTESIAN_POINT ( 'NONE',  ( 19.05341960407611168, 5.049401038298154454, 113.9572429386477097 ) ) ;
#18292=CARTESIAN_POINT ( 'NONE',  ( -5.049401038298153566, 19.05341960407611168, 45.20724293864769550 ) ) ;
#18293=CARTESIAN_POINT ( 'NONE',  ( 15.72974639402199770, -15.80617190586745480, 23.12390960531436335 ) ) ;
#18294=CARTESIAN_POINT ( 'NONE',  ( 21.53943276465977519, 0.05219959533937863772, 61.25109039468567573 ) ) ;
#18295=CARTESIAN_POINT ( 'NONE',  ( -16.55341960407611168, -4.379528057220339221, 111.4572429386476813 ) ) ;
#18296=CARTESIAN_POINT ( 'NONE',  ( 21.55341960407610458, 5.719274019375980345, 28.95724293864769905 ) ) ;
#18297=CARTESIAN_POINT ( 'NONE',  ( 4.379528057220092307, 16.55341960407617563, 72.29275706135236135 ) ) ;
#18298=CARTESIAN_POINT ( 'NONE',  ( -0.05219959533937732626, 21.53943276465977519, 97.50109039468567573 ) ) ;
#18299=CARTESIAN_POINT ( 'NONE',  ( -14.29746914071037622, -8.314922557961029526, 54.16775706135235424 ) ) ;
#18300=CARTESIAN_POINT ( 'NONE',  ( 0.05219959533909260263, 19.03943276465977164, 99.99890960531436690 ) ) ;
#18301=CARTESIAN_POINT ( 'NONE',  ( 14.34966873604972726, -8.224510206698740333, 40.83442372801901854 ) ) ;
#18302=CARTESIAN_POINT ( 'NONE',  ( 16.52544592524335698, 4.483927247898782831, 26.45942372801901854 ) ) ;
#18303=CARTESIAN_POINT ( 'NONE',  ( 0.05219959533934541429, -16.53943276465976808, 100.0010903946857042 ) ) ;
#18304=CARTESIAN_POINT ( 'NONE',  ( -21.52544592524334988, -5.823673210054445271, 58.95942372801902565 ) ) ;
#18305=CARTESIAN_POINT ( 'NONE',  ( 16.46253265017146816, 9.564922557961045513, 101.6677570613523329 ) ) ;
#18306=CARTESIAN_POINT ( 'NONE',  ( -21.53943276465977519, 0.05219959533907696930, 106.2489096053143811 ) ) ;
#18307=CARTESIAN_POINT ( 'NONE',  ( 8.224510206698953496, -14.34966873604960469, 97.91557627198103830 ) ) ;
#18308=CARTESIAN_POINT ( 'NONE',  ( 9.564922557961047289, -16.46253265017146816, 110.4177570613523471 ) ) ;
#18309=CARTESIAN_POINT ( 'NONE',  ( -12.06949235617739369, -12.14591786802326823, 79.37609039468567573 ) ) ;
#18311=CARTESIAN_POINT ( 'NONE',  ( 5.049401038297881783, 19.05341960407617563, 77.29275706135231871 ) ) ;
#18312=CARTESIAN_POINT ( 'NONE',  ( -4.483927247898539470, -16.52544592524342804, 47.29057627198103120 ) ) ;
#18313=CARTESIAN_POINT ( 'NONE',  ( -16.53943276465976808, 0.05219959533911058130, 46.24890960531435979 ) ) ;
#18314=CARTESIAN_POINT ( 'NONE',  ( 12.06949235617757843, -12.14591786802309237, 98.12390960531436690 ) ) ;
#18315=CARTESIAN_POINT ( 'NONE',  ( 13.97604488694548053, -13.89961937509957401, 35.62609039468567573 ) ) ;
#18316=CARTESIAN_POINT ( 'NONE',  ( -16.20579543436678449, 7.371946100355088127, 89.43479165828125588 ) ) ;
#18317=CARTESIAN_POINT ( 'NONE',  ( -21.53943276465977519, -0.05219959533937600094, 38.75109039468567573 ) ) ;
#18318=CARTESIAN_POINT ( 'NONE',  ( -16.46253265017146816, -9.564922557961047289, 109.1677570613523471 ) ) ;
#18320=CARTESIAN_POINT ( 'NONE',  ( -5.049401038298153566, 19.05341960407611168, 90.20724293864766707 ) ) ;
#18321=CARTESIAN_POINT ( 'NONE',  ( -13.89961937509977652, 13.97604488694528158, 95.62390960531436690 ) ) ;
#18322=CARTESIAN_POINT ( 'NONE',  ( -0.05219959533907301413, -21.53943276465977519, 52.49890960531435979 ) ) ;
#18323=CARTESIAN_POINT ( 'NONE',  ( 12.06949235617757843, -12.14591786802309237, 93.12390960531436690 ) ) ;
#18324=CARTESIAN_POINT ( 'NONE',  ( 13.97604488694527802, 13.89961937509977652, 74.37390960531436690 ) ) ;
#18325=CARTESIAN_POINT ( 'NONE',  ( 0.05219959533909260263, 19.03943276465977164, 24.99890960531435269 ) ) ;
#18327=CARTESIAN_POINT ( 'NONE',  ( 18.62759615963255655, 10.81492255796105972, 41.66775706135235424 ) ) ;
#18329=CARTESIAN_POINT ( 'NONE',  ( 10.81492255796106328, -18.62759615963255655, 70.41775706135236135 ) ) ;
#18330=CARTESIAN_POINT ( 'NONE',  ( -4.483927247898782831, 16.52544592524335698, 92.70942372801901854 ) ) ;
#18331=CARTESIAN_POINT ( 'NONE',  ( -21.55341960407619339, 5.719274019375674811, 23.54275706135235424 ) ) ;
#18332=CARTESIAN_POINT ( 'NONE',  ( 21.53943276465977519, 0.05219959533937863772, 21.25109039468567218 ) ) ;
#18333=CARTESIAN_POINT ( 'NONE',  ( 5.153800228976615827, -19.02544592524334988, 55.20942372801899722 ) ) ;
#18334=CARTESIAN_POINT ( 'NONE',  ( -9.474510206698964154, 16.51473224551069663, 80.41557627198103830 ) ) ;
#18335=CARTESIAN_POINT ( 'NONE',  ( -15.72974639402176322, -15.80617190586768395, 84.37609039468570415 ) ) ;
#18336=CARTESIAN_POINT ( 'NONE',  ( 21.55341960407610458, 5.719274019375980345, 83.95724293864770971 ) ) ;
#18337=CARTESIAN_POINT ( 'NONE',  ( 12.14591786802309770, 12.06949235617756955, 54.37390960531435979 ) ) ;
#18338=CARTESIAN_POINT ( 'NONE',  ( -18.67979575497193778, 10.72451020669871902, 103.3344237280190043 ) ) ;
#18339=CARTESIAN_POINT ( 'NONE',  ( -13.89961937509957401, -13.97604488694547875, 34.37609039468566863 ) ) ;
#18340=CARTESIAN_POINT ( 'NONE',  ( -16.52544592524342804, 4.483927247898546575, 76.04057627198102409 ) ) ;
#18341=CARTESIAN_POINT ( 'NONE',  ( 16.51473224551069308, 9.474510206698969483, 29.16557627198103475 ) ) ;
#18342=CARTESIAN_POINT ( 'NONE',  ( 5.049401038297881783, 19.05341960407617563, 67.29275706135234714 ) ) ;
#18343=CARTESIAN_POINT ( 'NONE',  ( 12.14591786802309770, 12.06949235617756955, 29.37390960531435269 ) ) ;
#18344=CARTESIAN_POINT ( 'NONE',  ( -21.52544592524334988, -5.823673210054445271, 78.95942372801901854 ) ) ;
#18345=CARTESIAN_POINT ( 'NONE',  ( 13.89961937509977652, -13.97604488694527269, 78.12390960531433848 ) ) ;
#18346=CARTESIAN_POINT ( 'NONE',  ( 5.049401038297881783, 19.05341960407617563, 57.29275706135231871 ) ) ;
#18347=CARTESIAN_POINT ( 'NONE',  ( -15.72974639402197994, 15.80617190586746368, 60.62390960531437401 ) ) ;
#18348=CARTESIAN_POINT ( 'NONE',  ( 18.67979575497178502, 10.72451020669898547, 114.1655762719810383 ) ) ;
#18349=CARTESIAN_POINT ( 'NONE',  ( 9.474510206698729675, 16.51473224551082808, 112.0844237280190043 ) ) ;
#18350=CARTESIAN_POINT ( 'NONE',  ( 12.06949235617739724, 12.14591786802326823, 81.87609039468568994 ) ) ;
#18352=CARTESIAN_POINT ( 'NONE',  ( -5.823673210054431948, 21.52544592524334988, 27.70942372801901854 ) ) ;
#18353=CARTESIAN_POINT ( 'NONE',  ( -14.29746914071049879, 8.314922557960819915, 105.8322429386476955 ) ) ;
#18355=CARTESIAN_POINT ( 'NONE',  ( 0.05219959533934541429, -16.53943276465976808, 35.00109039468568284 ) ) ;
#18356=CARTESIAN_POINT ( 'NONE',  ( -18.62759615963270932, 10.81492255796079327, 55.83224293864770260 ) ) ;
#18357=CARTESIAN_POINT ( 'NONE',  ( -16.53943276465976808, -0.05219959533934237506, 108.7510903946857042 ) ) ;
#18358=CARTESIAN_POINT ( 'NONE',  ( -16.52544592524335698, -4.483927247898792601, 38.95942372801901854 ) ) ;
#18359=CARTESIAN_POINT ( 'NONE',  ( -16.46253265017160317, 9.564922557960807481, 30.83224293864769550 ) ) ;
#18360=B_SPLINE_CURVE_WITH_KNOTS ( 'NONE', 3,
 ( #49859, #37670, #95355, #33692, #18537, #97323 ),
 .UNSPECIFIED., .F., .F.,
 ( 4, 2, 4 ),
 ( 0.003239945802372292023, 0.003620412082092145951, 0.004000878361811999878 ),
 .UNSPECIFIED. ) ;
#18361=CARTESIAN_POINT ( 'NONE',  ( 14.34966873604972726, -8.224510206698740333, 80.83442372801901854 ) ) ;
#18362=CARTESIAN_POINT ( 'NONE',  ( 13.97604488694548053, -13.89961937509957401, 70.62609039468567573 ) ) ;
#18363=CARTESIAN_POINT ( 'NONE',  ( 10.81492255796106328, -18.62759615963255655, 40.41775706135234714 ) ) ;
#18364=CARTESIAN_POINT ( 'NONE',  ( -5.719274019375978568, 21.55341960407610458, 55.20724293864770260 ) ) ;
#18365=CARTESIAN_POINT ( 'NONE',  ( 8.224510206698742110, 14.34966873604972548, 97.08442372801904696 ) ) ;
#18366=CARTESIAN_POINT ( 'NONE',  ( -5.823673210054431948, 21.52544592524334988, 77.70942372801900433 ) ) ;
#18368=CARTESIAN_POINT ( 'NONE',  ( 18.67979575497178502, 10.72451020669898547, 49.16557627198102409 ) ) ;
#18369=CARTESIAN_POINT ( 'NONE',  ( 21.55341960407610458, 5.719274019375980345, 43.95724293864769550 ) ) ;
#18370=CARTESIAN_POINT ( 'NONE',  ( 4.483927247898790824, -16.52544592524335698, 85.20942372801901854 ) ) ;
#18371=CARTESIAN_POINT ( 'NONE',  ( -18.67979575497178146, -10.72451020669898902, 46.66557627198102409 ) ) ;
#18373=CARTESIAN_POINT ( 'NONE',  ( -19.02544592524342804, 5.153800228976336051, 106.0405762719810241 ) ) ;
#18375=CARTESIAN_POINT ( 'NONE',  ( -19.03943276465977164, 0.05219959533909376836, 21.24890960531436335 ) ) ;
#18376=CARTESIAN_POINT ( 'NONE',  ( -5.719274019375978568, 21.55341960407610458, 55.20724293864770260 ) ) ;
#18377=CARTESIAN_POINT ( 'NONE',  ( 12.06949235617739724, 12.14591786802326823, 96.87609039468568994 ) ) ;
#18378=CARTESIAN_POINT ( 'NONE',  ( 5.719274019375673035, 21.55341960407619339, 47.29275706135234003 ) ) ;
#18379=CARTESIAN_POINT ( 'NONE',  ( 16.51473224551083163, -9.474510206698727899, 100.8344237280190043 ) ) ;
#18380=CARTESIAN_POINT ( 'NONE',  ( -4.483927247898539470, -16.52544592524342804, 107.2905762719810525 ) ) ;
#18381=CARTESIAN_POINT ( 'NONE',  ( 16.51473224551083163, -9.474510206698727899, 110.8344237280190043 ) ) ;
#18383=CARTESIAN_POINT ( 'NONE',  ( 13.89961937509977652, -13.97604488694527269, 38.12390960531436690 ) ) ;
#18385=CARTESIAN_POINT ( 'NONE',  ( -13.97604488694527625, -13.89961937509977652, 91.87390960531432427 ) ) ;
#18386=CARTESIAN_POINT ( 'NONE',  ( -0.05219959533934338120, 16.53943276465976808, 82.50109039468568994 ) ) ;
#18387=CARTESIAN_POINT ( 'NONE',  ( 5.719274019375673035, 21.55341960407619339, 107.2927570613523471 ) ) ;
#18388=CARTESIAN_POINT ( 'NONE',  ( -18.62759615963270932, 10.81492255796079327, 60.83224293864769550 ) ) ;
#18389=CARTESIAN_POINT ( 'NONE',  ( 14.29746914071037800, 8.314922557961029526, 86.66775706135234714 ) ) ;
#18390=CARTESIAN_POINT ( 'NONE',  ( -19.02544592524334988, -5.153800228976617603, 73.95942372801900433 ) ) ;
#18391=CARTESIAN_POINT ( 'NONE',  ( -9.564922557960796823, -16.46253265017161027, 37.08224293864768839 ) ) ;
#18392=CARTESIAN_POINT ( 'NONE',  ( 19.05341960407611168, 5.049401038298154454, 78.95724293864769550 ) ) ;
#18393=CARTESIAN_POINT ( 'NONE',  ( -15.80617190586768217, 15.72974639402176855, 48.12609039468568284 ) ) ;
#18394=CARTESIAN_POINT ( 'NONE',  ( 5.153800228976335163, 19.02544592524342804, 49.79057627198100988 ) ) ;
#18395=CARTESIAN_POINT ( 'NONE',  ( 19.02544592524334988, 5.153800228976608722, 71.45942372801900433 ) ) ;
#18397=CARTESIAN_POINT ( 'NONE',  ( 5.049401038298161559, -19.05341960407611168, 102.7072429386476955 ) ) ;
#18398=CARTESIAN_POINT ( 'NONE',  ( 12.06949235617757843, -12.14591786802309237, 68.12390960531436690 ) ) ;
#18399=CARTESIAN_POINT ( 'NONE',  ( 21.53943276465977519, -0.05219959533907433946, 63.74890960531435979 ) ) ;
#18401=( BOUNDED_CURVE ( )  B_SPLINE_CURVE ( 2, ( #1870, #92876, #3850, #76721, #186923, #185912, #157554, #78706, #62540, #47397, #142371, #79712, #141381 ),
 .UNSPECIFIED., .F., .T. ) 
 B_SPLINE_CURVE_WITH_KNOTS ( ( 3, 2, 2, 2, 2, 2, 3 ),
 ( 0.4497988574796767391, 0.4517543859649122973, 0.4561403508771929571, 0.4605263157894736725, 0.4649122807017543879, 0.4692982456140351033, 0.4712080942771805780 ),
 .UNSPECIFIED. ) 
 CURVE ( )  GEOMETRIC_REPRESENTATION_ITEM ( )  RATIONAL_B_SPLINE_CURVE ( ( 0.9831626618144004848, 0.9848076720550091867, 1.000000000000000000, 0.9659258262890683122, 1.000000000000000000, 0.9659258262890683122, 1.000000000000000000, 0.9659258262890683122, 1.000000000000000000, 0.9659258262890683122, 1.000000000000000000, 0.9851625545550088958, 0.9832469066685279868 ) ) 
 REPRESENTATION_ITEM ( '' )  );
#18402=CARTESIAN_POINT ( 'NONE',  ( -9.474510206698720793, -16.51473224551083518, 24.58442372801900078 ) ) ;
#18404=CARTESIAN_POINT ( 'NONE',  ( 16.46253265017160672, -9.564922557960803928, 63.33224293864769550 ) ) ;
#18405=CARTESIAN_POINT ( 'NONE',  ( -19.05341960407611168, -5.049401038298163336, 71.45724293864766707 ) ) ;
#18406=CARTESIAN_POINT ( 'NONE',  ( -8.314922557961024197, 14.29746914071037800, 52.91775706135235424 ) ) ;
#18409=CARTESIAN_POINT ( 'NONE',  ( 12.14591786802327356, -12.06949235617739191, 80.62609039468567573 ) ) ;
#18411=CARTESIAN_POINT ( 'NONE',  ( -8.224510206698735004, -14.34966873604973081, 69.58442372801900433 ) ) ;
#18412=CARTESIAN_POINT ( 'NONE',  ( 16.53943276465976808, 0.05219959533934440121, 36.25109039468567573 ) ) ;
#18413=CARTESIAN_POINT ( 'NONE',  ( 9.474510206698971260, -16.51473224551069308, 57.91557627198103120 ) ) ;
#18414=CARTESIAN_POINT ( 'NONE',  ( 18.22780087662119897, -5.500000000000096811, 68.51763182126893525 ) ) ;
#18415=CARTESIAN_POINT ( 'NONE',  ( 18.67979575497194134, -10.72451020669871369, 55.83442372801901854 ) ) ;
#18416=CARTESIAN_POINT ( 'NONE',  ( 0.05219959533936267826, -19.03943276465977164, 60.00109039468566863 ) ) ;
#18417=CARTESIAN_POINT ( 'NONE',  ( -18.67979575497193778, 10.72451020669871902, 108.3344237280190185 ) ) ;
#18418=CARTESIAN_POINT ( 'NONE',  ( 13.97604488694527802, 13.89961937509977652, 34.37390960531436690 ) ) ;
#18420=CARTESIAN_POINT ( 'NONE',  ( -10.72451020669898014, 18.67979575497178502, 55.41557627198102409 ) ) ;
#18421=CARTESIAN_POINT ( 'NONE',  ( 16.46253265017160672, -9.564922557960803928, 108.3322429386476955 ) ) ;
#18422=CARTESIAN_POINT ( 'NONE',  ( -14.29746914071049879, 8.314922557960819915, 105.8322429386476955 ) ) ;
#18423=CARTESIAN_POINT ( 'NONE',  ( 16.55341960407618274, -4.379528057220086978, 41.04275706135236135 ) ) ;
#18424=CARTESIAN_POINT ( 'NONE',  ( -14.29746914071049879, 8.314922557960819915, 30.83224293864770260 ) ) ;
#18426=CARTESIAN_POINT ( 'NONE',  ( 21.55341960407610458, 5.719274019375980345, 108.9572429386476955 ) ) ;
#18427=CARTESIAN_POINT ( 'NONE',  ( -12.06949235617756955, 12.14591786802309770, 45.62390960531436690 ) ) ;
#18429=CARTESIAN_POINT ( 'NONE',  ( 9.474510206698729675, 16.51473224551082808, 92.08442372801900433 ) ) ;
#18430=CARTESIAN_POINT ( 'NONE',  ( -16.51473224551082808, 9.474510206698731452, 28.33442372801900433 ) ) ;
#18431=CARTESIAN_POINT ( 'NONE',  ( 12.06949235617757843, -12.14591786802309237, 33.12390960531435979 ) ) ;
#18432=CARTESIAN_POINT ( 'NONE',  ( -21.53943276465977519, 0.05219959533907696930, 106.2489096053143811 ) ) ;
#18433=CARTESIAN_POINT ( 'NONE',  ( -21.55341960407610458, -5.719274019375992779, 51.45724293864770260 ) ) ;
#18434=CARTESIAN_POINT ( 'NONE',  ( 9.564922557960805705, 16.46253265017160317, 79.58224293864769550 ) ) ;
#18435=CARTESIAN_POINT ( 'NONE',  ( -14.34966873604960291, -8.224510206698953496, 41.66557627198103120 ) ) ;
#18436=CARTESIAN_POINT ( 'NONE',  ( -13.97604488694527625, -13.89961937509977652, 91.87390960531432427 ) ) ;
#18438=CARTESIAN_POINT ( 'NONE',  ( 13.97604488694548053, -13.89961937509957401, 35.62609039468567573 ) ) ;
#18439=CARTESIAN_POINT ( 'NONE',  ( -10.72451020669898014, 18.67979575497178502, 100.4155762719810241 ) ) ;
#18440=CARTESIAN_POINT ( 'NONE',  ( -14.29746914071049879, 8.314922557960819915, 105.8322429386476955 ) ) ;
#18441=CARTESIAN_POINT ( 'NONE',  ( 18.62759615963255655, 10.81492255796105972, 31.66775706135234358 ) ) ;
#18443=CARTESIAN_POINT ( 'NONE',  ( 8.224510206698742110, 14.34966873604972548, 112.0844237280190185 ) ) ;
#18444=CARTESIAN_POINT ( 'NONE',  ( 16.46253265017160672, -9.564922557960803928, 33.33224293864770260 ) ) ;
#18445=CARTESIAN_POINT ( 'NONE',  ( 5.049401038298161559, -19.05341960407611168, 82.70724293864770971 ) ) ;
#18447=CARTESIAN_POINT ( 'NONE',  ( 9.564922557960805705, 16.46253265017160317, 34.58224293864770260 ) ) ;
#18448=CARTESIAN_POINT ( 'NONE',  ( 4.379528057220339221, -16.55341960407611168, 37.70724293864769550 ) ) ;
#18449=CARTESIAN_POINT ( 'NONE',  ( 15.72974639402176855, 15.80617190586768217, 76.87609039468567573 ) ) ;
#18451=CARTESIAN_POINT ( 'NONE',  ( 14.34966873604972726, -8.224510206698740333, 75.83442372801900433 ) ) ;
#18452=CARTESIAN_POINT ( 'NONE',  ( 13.97604488694527802, 13.89961937509977652, 59.37390960531434558 ) ) ;
#18453=CARTESIAN_POINT ( 'NONE',  ( -19.05341960407611168, -5.049401038298163336, 66.45724293864769550 ) ) ;
#18455=CARTESIAN_POINT ( 'NONE',  ( -5.049401038297874678, -19.05341960407617918, 19.79275706135233293 ) ) ;
#18456=CARTESIAN_POINT ( 'NONE',  ( 4.483927247898790824, -16.52544592524335698, 70.20942372801904696 ) ) ;
#18457=CARTESIAN_POINT ( 'NONE',  ( 18.67979575497194134, -10.72451020669871369, 100.8344237280190185 ) ) ;
#18458=CARTESIAN_POINT ( 'NONE',  ( 13.97604488694527802, 13.89961937509977652, 59.37390960531434558 ) ) ;
#18459=CARTESIAN_POINT ( 'NONE',  ( -18.62759615963270932, 10.81492255796079327, 40.83224293864769550 ) ) ;
#18460=CARTESIAN_POINT ( 'NONE',  ( 19.05341960407617918, -5.049401038297876454, 101.0427570613523045 ) ) ;
#18461=CARTESIAN_POINT ( 'NONE',  ( -21.55341960407619339, 5.719274019375674811, 73.54275706135234714 ) ) ;
#18462=CARTESIAN_POINT ( 'NONE',  ( -0.05219959533934338120, 16.53943276465976808, 47.50109039468568994 ) ) ;
#18463=CARTESIAN_POINT ( 'NONE',  ( 15.80617190586746368, 15.72974639402197994, 104.3739096053143669 ) ) ;
#18464=CARTESIAN_POINT ( 'NONE',  ( 5.153800228976615827, -19.02544592524334988, 105.2094237280190185 ) ) ;
#18465=CARTESIAN_POINT ( 'NONE',  ( 16.46253265017160672, -9.564922557960803928, 78.33224293864769550 ) ) ;
#18466=CARTESIAN_POINT ( 'NONE',  ( -8.224510206698735004, -14.34966873604973081, 19.58442372801901143 ) ) ;
#18468=CARTESIAN_POINT ( 'NONE',  ( -14.34966873604972548, 8.224510206698743886, 23.33442372801901499 ) ) ;
#18469=CARTESIAN_POINT ( 'NONE',  ( 16.53943276465976808, -0.05219959533910856209, 68.74890960531435269 ) ) ;
#18470=CARTESIAN_POINT ( 'NONE',  ( -8.224510206698735004, -14.34966873604973081, 79.58442372801903275 ) ) ;
#18471=CARTESIAN_POINT ( 'NONE',  ( -15.80617190586745835, -15.72974639402198527, 111.8739096053143669 ) ) ;
#18472=CARTESIAN_POINT ( 'NONE',  ( -19.02544592524342804, 5.153800228976336051, 51.04057627198103120 ) ) ;
#18473=CARTESIAN_POINT ( 'NONE',  ( -19.02544592524342804, 5.153800228976336051, 71.04057627198099567 ) ) ;
#18474=CARTESIAN_POINT ( 'NONE',  ( 8.224510206698742110, 14.34966873604972548, 72.08442372801899012 ) ) ;
#18476=ORIENTED_EDGE ( 'NONE', *, *, #94811, .F. ) ;
#18477=CARTESIAN_POINT ( 'NONE',  ( 19.02544592524334988, 5.153800228976608722, 21.45942372801899012 ) ) ;
#18479=CARTESIAN_POINT ( 'NONE',  ( -19.03943276465977164, 0.05219959533909376836, 36.24890960531436690 ) ) ;
#18481=CARTESIAN_POINT ( 'NONE',  ( -13.97604488694547697, 13.89961937509957934, 113.1260903946856757 ) ) ;
#18482=CARTESIAN_POINT ( 'NONE',  ( 5.153800228976615827, -19.02544592524334988, 40.20942372801898301 ) ) ;
#18483=CARTESIAN_POINT ( 'NONE',  ( -12.06949235617739369, -12.14591786802326823, 24.37609039468567573 ) ) ;
#18484=CARTESIAN_POINT ( 'NONE',  ( 19.03943276465977164, -0.05219959533909143690, 38.74890960531436690 ) ) ;
#18485=CARTESIAN_POINT ( 'NONE',  ( -5.153800228976328057, -19.02544592524343514, 67.29057627198102409 ) ) ;
#18486=CARTESIAN_POINT ( 'NONE',  ( -0.05219959533907301413, -21.53943276465977519, 92.49890960531436690 ) ) ;
#18487=CARTESIAN_POINT ( 'NONE',  ( 9.564922557960805705, 16.46253265017160317, 109.5822429386476955 ) ) ;
#18489=CARTESIAN_POINT ( 'NONE',  ( 19.05341960407611168, 5.049401038298154454, 43.95724293864769550 ) ) ;
#18491=CARTESIAN_POINT ( 'NONE',  ( -19.03943276465977164, -0.05219959533935918106, 93.75109039468566152 ) ) ;
#18492=CARTESIAN_POINT ( 'NONE',  ( -21.52544592524343514, 5.823673210054127303, 71.04057627198103830 ) ) ;
#18493=CARTESIAN_POINT ( 'NONE',  ( -9.564922557961040184, 16.46253265017147172, 27.91775706135232582 ) ) ;
#18494=CARTESIAN_POINT ( 'NONE',  ( 4.483927247898545687, 16.52544592524342804, 64.79057627198103830 ) ) ;
#18495=CARTESIAN_POINT ( 'NONE',  ( 5.823673210054444382, -21.52544592524334988, 85.20942372801901854 ) ) ;
#18496=CARTESIAN_POINT ( 'NONE',  ( -14.29746914071049879, 8.314922557960819915, 115.8322429386477097 ) ) ;
#18497=CARTESIAN_POINT ( 'NONE',  ( -14.34966873604960291, -8.224510206698953496, 31.66557627198102054 ) ) ;
#18498=CARTESIAN_POINT ( 'NONE',  ( -18.67979575497193778, 10.72451020669871902, 93.33442372801901854 ) ) ;
#18499=CARTESIAN_POINT ( 'NONE',  ( -19.03943276465977164, 0.05219959533909376836, 76.24890960531435269 ) ) ;
#18500=CARTESIAN_POINT ( 'NONE',  ( 21.53943276465977519, 0.05219959533937863772, 41.25109039468568284 ) ) ;
#18501=CARTESIAN_POINT ( 'NONE',  ( -19.02544592524342804, 5.153800228976336051, 81.04057627198103830 ) ) ;
#18502=CARTESIAN_POINT ( 'NONE',  ( 16.55341960407611168, 4.379528057220329451, 98.95724293864770971 ) ) ;
#18503=CARTESIAN_POINT ( 'NONE',  ( 12.06949235617757843, -12.14591786802309237, 58.12390960531435979 ) ) ;
#18504=CARTESIAN_POINT ( 'NONE',  ( 10.81492255796078972, 18.62759615963270932, 74.58224293864768129 ) ) ;
#18505=CARTESIAN_POINT ( 'NONE',  ( -9.564922557960796823, -16.46253265017161027, 77.08224293864769550 ) ) ;
#18506=CARTESIAN_POINT ( 'NONE',  ( 10.81492255796078972, 18.62759615963270932, 84.58224293864769550 ) ) ;
#18507=CARTESIAN_POINT ( 'NONE',  ( 19.05341960407617918, -5.049401038297876454, 76.04275706135230450 ) ) ;
#18508=CARTESIAN_POINT ( 'NONE',  ( 9.474510206698729675, 16.51473224551082808, 32.08442372801900433 ) ) ;
#18509=CARTESIAN_POINT ( 'NONE',  ( 8.314922557960818139, 14.29746914071049879, 79.58224293864769550 ) ) ;
#18511=CARTESIAN_POINT ( 'NONE',  ( 18.67979575497178502, 10.72451020669898547, 54.16557627198103120 ) ) ;
#18513=CARTESIAN_POINT ( 'NONE',  ( 12.06949235617739724, 12.14591786802326823, 101.8760903946857042 ) ) ;
#18515=CARTESIAN_POINT ( 'NONE',  ( -0.05219959533936034679, 19.03943276465977164, 102.5010903946856757 ) ) ;
#18516=CARTESIAN_POINT ( 'NONE',  ( -14.34966873604960291, -8.224510206698953496, 66.66557627198102409 ) ) ;
#18517=CARTESIAN_POINT ( 'NONE',  ( -19.19724070472095079, -5.500000000000031974, 96.06193348274383936 ) ) ;
#18518=CARTESIAN_POINT ( 'NONE',  ( -16.51473224551069308, -9.474510206698971260, 61.66557627198103120 ) ) ;
#18519=CARTESIAN_POINT ( 'NONE',  ( 13.89961937509977652, -13.97604488694527269, 28.12390960531435624 ) ) ;
#18520=CARTESIAN_POINT ( 'NONE',  ( 12.06949235617757843, -12.14591786802309237, 48.12390960531436690 ) ) ;
#18521=CARTESIAN_POINT ( 'NONE',  ( 19.05341960407611168, 5.049401038298154454, 103.9572429386476671 ) ) ;
#18522=CARTESIAN_POINT ( 'NONE',  ( -13.89961937509957401, -13.97604488694547875, 94.37609039468566152 ) ) ;
#18523=CARTESIAN_POINT ( 'NONE',  ( -19.03943276465977164, 0.05219959533909376836, 66.24890960531436690 ) ) ;
#18524=CARTESIAN_POINT ( 'NONE',  ( 5.153800228976335163, 19.02544592524342804, 79.79057627198102409 ) ) ;
#18525=CARTESIAN_POINT ( 'NONE',  ( 5.049401038298161559, -19.05341960407611168, 82.70724293864770971 ) ) ;
#18526=CARTESIAN_POINT ( 'NONE',  ( 5.823673210054125526, 21.52544592524343514, 59.79057627198103120 ) ) ;
#18527=CARTESIAN_POINT ( 'NONE',  ( -4.483927247898782831, 16.52544592524335698, 57.70942372801901143 ) ) ;
#18528=CARTESIAN_POINT ( 'NONE',  ( -0.05219959533936034679, 19.03943276465977164, 107.5010903946856615 ) ) ;
#18529=CARTESIAN_POINT ( 'NONE',  ( -0.05219959533909027116, -19.03943276465977164, 62.49890960531435979 ) ) ;
#18530=CARTESIAN_POINT ( 'NONE',  ( 18.67979575497178502, 10.72451020669898547, 69.16557627198102409 ) ) ;
#18531=CARTESIAN_POINT ( 'NONE',  ( -13.97604488694547697, 13.89961937509957934, 88.12609039468563310 ) ) ;
#18532=CARTESIAN_POINT ( 'NONE',  ( -8.314922557960811034, -14.29746914071050412, 27.08224293864769550 ) ) ;
#18533=CARTESIAN_POINT ( 'NONE',  ( -10.72451020669870658, -18.67979575497194134, 49.58442372801901143 ) ) ;
#18535=CARTESIAN_POINT ( 'NONE',  ( -0.05219959533934338120, 16.53943276465976808, 67.50109039468568994 ) ) ;
#18536=CARTESIAN_POINT ( 'NONE',  ( -16.55341960407617563, 4.379528057220093196, 98.54275706135234714 ) ) ;
#18537=CARTESIAN_POINT ( 'NONE',  ( -18.10062525802553424, 5.500000000000031974, 73.51383468041922242 ) ) ;
#18538=CARTESIAN_POINT ( 'NONE',  ( 0.05219959533934541429, -16.53943276465976808, 85.00109039468568994 ) ) ;
#18539=CARTESIAN_POINT ( 'NONE',  ( 12.14591786802327356, -12.06949235617739191, 30.62609039468567929 ) ) ;
#18540=CARTESIAN_POINT ( 'NONE',  ( 19.02544592524343514, -5.153800228976328945, 48.54057627198103120 ) ) ;
#18541=CARTESIAN_POINT ( 'NONE',  ( -19.02544592524342804, 5.153800228976336051, 56.04057627198100988 ) ) ;
#18542=CARTESIAN_POINT ( 'NONE',  ( -5.153800228976328057, -19.02544592524343514, 62.29057627198100988 ) ) ;
#18543=CARTESIAN_POINT ( 'NONE',  ( -21.55341960407619339, 5.719274019375674811, 48.54275706135234714 ) ) ;
#18544=CARTESIAN_POINT ( 'NONE',  ( 12.06949235617739724, 12.14591786802326823, 51.87609039468568284 ) ) ;
#18545=CARTESIAN_POINT ( 'NONE',  ( -8.224510206698948167, 14.34966873604960824, 30.41557627198101699 ) ) ;
#18546=CARTESIAN_POINT ( 'NONE',  ( 13.89961937509977652, -13.97604488694527269, 23.12390960531436335 ) ) ;
#18547=CARTESIAN_POINT ( 'NONE',  ( 19.02544592524343514, -5.153800228976328945, 38.54057627198103120 ) ) ;
#18548=CARTESIAN_POINT ( 'NONE',  ( 14.29746914071037800, 8.314922557961029526, 26.66775706135235424 ) ) ;
#18549=CARTESIAN_POINT ( 'NONE',  ( 9.564922557961047289, -16.46253265017146816, 85.41775706135233293 ) ) ;
#18550=CARTESIAN_POINT ( 'NONE',  ( 16.52544592524342804, -4.483927247898539470, 78.54057627198103830 ) ) ;
#18551=CARTESIAN_POINT ( 'NONE',  ( 16.46253265017160672, -9.564922557960803928, 58.33224293864769550 ) ) ;
#18552=CARTESIAN_POINT ( 'NONE',  ( -13.97604488694547697, 13.89961937509957934, 93.12609039468566152 ) ) ;
#18553=CARTESIAN_POINT ( 'NONE',  ( 16.81555441253551564, -7.025013491695470513, 93.13685445334256485 ) ) ;
#18554=CARTESIAN_POINT ( 'NONE',  ( -10.72451020669870658, -18.67979575497194134, 74.58442372801901854 ) ) ;
#18555=CARTESIAN_POINT ( 'NONE',  ( -4.379528057220086978, -16.55341960407618274, 54.79275706135235424 ) ) ;
#18556=CARTESIAN_POINT ( 'NONE',  ( 17.13100169013299379, 6.664070546373169535, 36.73210164300151348 ) ) ;
#18557=CARTESIAN_POINT ( 'NONE',  ( 18.67979575497178502, 10.72451020669898547, 39.16557627198102409 ) ) ;
#18558=CARTESIAN_POINT ( 'NONE',  ( 12.06949235617739724, 12.14591786802326823, 36.87609039468568994 ) ) ;
#18560=CARTESIAN_POINT ( 'NONE',  ( 13.97604488694548053, -13.89961937509957401, 35.62609039468567573 ) ) ;
#18562=CARTESIAN_POINT ( 'NONE',  ( 16.51473224551069308, 9.474510206698969483, 54.16557627198103120 ) ) ;
#18563=CARTESIAN_POINT ( 'NONE',  ( -17.50000000000001421, -5.499999999999944045, 71.28230962303567253 ) ) ;
#18564=CARTESIAN_POINT ( 'NONE',  ( 13.89961937509977652, -13.97604488694527269, 73.12390960531436690 ) ) ;
#18565=CARTESIAN_POINT ( 'NONE',  ( -19.53037848336979820, 5.499999999999995559, 99.85532783611445495 ) ) ;
#18567=CARTESIAN_POINT ( 'NONE',  ( -19.03943276465977164, -0.05219959533935918106, 23.75109039468566152 ) ) ;
#18568=CARTESIAN_POINT ( 'NONE',  ( -0.05219959533910754901, -16.53943276465976808, 42.49890960531435979 ) ) ;
#18569=CARTESIAN_POINT ( 'NONE',  ( 19.02544592524343514, -5.153800228976328945, 48.54057627198103120 ) ) ;
#18570=CARTESIAN_POINT ( 'NONE',  ( 0.05219959533909260263, 19.03943276465977164, 104.9989096053143669 ) ) ;
#18571=CARTESIAN_POINT ( 'NONE',  ( -21.55341960407619339, 5.719274019375674811, 73.54275706135234714 ) ) ;
#18572=CARTESIAN_POINT ( 'NONE',  ( 19.05341960407611168, 5.049401038298154454, 48.95724293864768129 ) ) ;
#18573=CARTESIAN_POINT ( 'NONE',  ( 18.62759615963255655, 10.81492255796105972, 66.66775706135234714 ) ) ;
#18574=CARTESIAN_POINT ( 'NONE',  ( 9.474510206698971260, -16.51473224551069308, 112.9155762719810383 ) ) ;
#18575=CARTESIAN_POINT ( 'NONE',  ( -13.97604488694527625, -13.89961937509977652, 41.87390960531435979 ) ) ;
#18576=CARTESIAN_POINT ( 'NONE',  ( -15.72974639402176322, -15.80617190586768395, 24.37609039468567573 ) ) ;
#18577=CARTESIAN_POINT ( 'NONE',  ( 16.46253265017146816, 9.564922557961045513, 51.66775706135233293 ) ) ;
#18578=CARTESIAN_POINT ( 'NONE',  ( -16.46253265017160317, 9.564922557960807481, 25.83224293864769194 ) ) ;
#18579=CARTESIAN_POINT ( 'NONE',  ( -0.05219959533909027116, -19.03943276465977164, 57.49890960531435979 ) ) ;
#18580=CARTESIAN_POINT ( 'NONE',  ( -14.29746914071037622, -8.314922557961029526, 19.16775706135234714 ) ) ;
#18581=CARTESIAN_POINT ( 'NONE',  ( -12.06949235617756955, 12.14591786802309770, 75.62390960531439532 ) ) ;
#18582=CARTESIAN_POINT ( 'NONE',  ( -10.72451020669898014, 18.67979575497178502, 40.41557627198103120 ) ) ;
#18583=CARTESIAN_POINT ( 'NONE',  ( 16.46253265017146816, 9.564922557961045513, 106.6677570613523471 ) ) ;
#18584=CARTESIAN_POINT ( 'NONE',  ( -18.62759615963270932, 10.81492255796079327, 105.8322429386476955 ) ) ;
#18585=CARTESIAN_POINT ( 'NONE',  ( 5.823673210054444382, -21.52544592524334988, 55.20942372801902565 ) ) ;
#18586=CARTESIAN_POINT ( 'NONE',  ( 16.53943276465976808, 0.05219959533934440121, 56.25109039468568284 ) ) ;
#18587=CARTESIAN_POINT ( 'NONE',  ( -14.34966873604972548, 8.224510206698743886, 48.33442372801902565 ) ) ;
#18588=CARTESIAN_POINT ( 'NONE',  ( -18.62759615963270932, 10.81492255796079327, 55.83224293864770260 ) ) ;
#18589=CARTESIAN_POINT ( 'NONE',  ( -19.05341960407611168, -5.049401038298163336, 41.45724293864769550 ) ) ;
#18590=CARTESIAN_POINT ( 'NONE',  ( 4.483927247898790824, -16.52544592524335698, 70.20942372801904696 ) ) ;
#18591=CARTESIAN_POINT ( 'NONE',  ( 21.52544592524344225, -5.823673210054117533, 103.5405762719810383 ) ) ;
#18592=CARTESIAN_POINT ( 'NONE',  ( -4.379528057220328563, 16.55341960407611168, 50.20724293864769550 ) ) ;
#18593=CARTESIAN_POINT ( 'NONE',  ( 5.049401038298161559, -19.05341960407611168, 67.70724293864769550 ) ) ;
#18594=CARTESIAN_POINT ( 'NONE',  ( -14.34966873604972548, 8.224510206698743886, 78.33442372801901854 ) ) ;
#18595=CARTESIAN_POINT ( 'NONE',  ( -19.02544592524334988, -5.153800228976617603, 108.9594237280189759 ) ) ;
#18596=CARTESIAN_POINT ( 'NONE',  ( -5.719274019375978568, 21.55341960407610458, 105.2072429386477097 ) ) ;
#18597=CARTESIAN_POINT ( 'NONE',  ( 4.483927247898545687, 16.52544592524342804, 39.79057627198103830 ) ) ;
#18599=CARTESIAN_POINT ( 'NONE',  ( 19.52837319214027190, -5.499999999999988454, 92.10471352585543059 ) ) ;
#18600=CARTESIAN_POINT ( 'NONE',  ( -15.80617190586745835, -15.72974639402198527, 86.87390960531438111 ) ) ;
#18601=CARTESIAN_POINT ( 'NONE',  ( -8.314922557960811034, -14.29746914071050412, 32.08224293864769550 ) ) ;
#18603=DIRECTION ( 'NONE',  ( 0.000000000000000000, 0.000000000000000000, -1.000000000000000000 ) ) ;
#18604=CARTESIAN_POINT ( 'NONE',  ( -10.81492255796078084, -18.62759615963271287, 97.08224293864770971 ) ) ;
#18605=CARTESIAN_POINT ( 'NONE',  ( -13.97604488694527625, -13.89961937509977652, 101.8739096053143811 ) ) ;
#18606=CARTESIAN_POINT ( 'NONE',  ( -18.67979575497193778, 10.72451020669871902, 28.33442372801902209 ) ) ;
#18607=CARTESIAN_POINT ( 'NONE',  ( -0.05219959533910754901, -16.53943276465976808, 52.49890960531435979 ) ) ;
#18608=CARTESIAN_POINT ( 'NONE',  ( -16.55341960407617563, 4.379528057220093196, 53.54275706135234714 ) ) ;
#18610=CARTESIAN_POINT ( 'NONE',  ( -5.153800228976328057, -19.02544592524343514, 47.29057627198102409 ) ) ;
#18611=CARTESIAN_POINT ( 'NONE',  ( 0.05219959533936267826, -19.03943276465977164, 50.00109039468566863 ) ) ;
#18612=CARTESIAN_POINT ( 'NONE',  ( -0.05219959533909027116, -19.03943276465977164, 82.49890960531436690 ) ) ;
#18613=CARTESIAN_POINT ( 'NONE',  ( -5.719274019375978568, 21.55341960407610458, 40.20724293864769550 ) ) ;
#18614=CARTESIAN_POINT ( 'NONE',  ( 16.51473224551069308, 9.474510206698969483, 64.16557627198102409 ) ) ;
#18615=CARTESIAN_POINT ( 'NONE',  ( -9.564922557961040184, 16.46253265017147172, 112.9177570613523329 ) ) ;
#18616=CARTESIAN_POINT ( 'NONE',  ( 5.153800228976615827, -19.02544592524334988, 55.20942372801899722 ) ) ;
#18617=CARTESIAN_POINT ( 'NONE',  ( 15.72974639402199770, -15.80617190586745480, 98.12390960531436690 ) ) ;
#18618=CARTESIAN_POINT ( 'NONE',  ( 4.379528057220339221, -16.55341960407611168, 32.70724293864770260 ) ) ;
#18619=CARTESIAN_POINT ( 'NONE',  ( -9.474510206698964154, 16.51473224551069663, 80.41557627198103830 ) ) ;
#18620=CARTESIAN_POINT ( 'NONE',  ( -21.52544592524343514, 5.823673210054127303, 56.04057627198102409 ) ) ;
#18621=CARTESIAN_POINT ( 'NONE',  ( -21.55341960407610458, -5.719274019375992779, 91.45724293864769550 ) ) ;
#18622=CARTESIAN_POINT ( 'NONE',  ( -4.379528057220086978, -16.55341960407618274, 19.79275706135235069 ) ) ;
#18623=CARTESIAN_POINT ( 'NONE',  ( -5.153800228976328057, -19.02544592524343514, 112.2905762719810099 ) ) ;
#18624=CARTESIAN_POINT ( 'NONE',  ( 0.05219959533937995610, -21.53943276465977519, 95.00109039468568994 ) ) ;
#18625=CARTESIAN_POINT ( 'NONE',  ( 19.05341960407611168, 5.049401038298154454, 88.95724293864769550 ) ) ;
#18626=CARTESIAN_POINT ( 'NONE',  ( 0.05219959533909260263, 19.03943276465977164, 24.99890960531435269 ) ) ;
#18627=CARTESIAN_POINT ( 'NONE',  ( 13.89961937509977652, -13.97604488694527269, 78.12390960531433848 ) ) ;
#18628=CARTESIAN_POINT ( 'NONE',  ( -16.55341960407611168, -4.379528057220339221, 106.4572429386477097 ) ) ;
#18629=CARTESIAN_POINT ( 'NONE',  ( -16.46253265017160317, 9.564922557960807481, 65.83224293864769550 ) ) ;
#18630=CARTESIAN_POINT ( 'NONE',  ( 12.14591786802327356, -12.06949235617739191, 20.62609039468568639 ) ) ;
#18631=CARTESIAN_POINT ( 'NONE',  ( 17.49999999999999645, 4.013004640162663783, 32.05394279005592040 ) ) ;
#18632=CARTESIAN_POINT ( 'NONE',  ( 9.564922557960805705, 16.46253265017160317, 79.58224293864769550 ) ) ;
#18634=CARTESIAN_POINT ( 'NONE',  ( -21.52544592524334988, -5.823673210054445271, 98.95942372801903275 ) ) ;
#18635=CARTESIAN_POINT ( 'NONE',  ( -15.80617190586745835, -15.72974639402198527, 21.87390960531436690 ) ) ;
#18636=CARTESIAN_POINT ( 'NONE',  ( 8.224510206698742110, 14.34966873604972548, 97.08442372801904696 ) ) ;
#18638=CARTESIAN_POINT ( 'NONE',  ( -19.05341960407617563, 5.049401038297882671, 73.54275706135233293 ) ) ;
#18639=CARTESIAN_POINT ( 'NONE',  ( 19.05341960407617918, -5.049401038297876454, 21.04275706135232582 ) ) ;
#18641=CARTESIAN_POINT ( 'NONE',  ( 5.153800228976335163, 19.02544592524342804, 29.79057627198102409 ) ) ;
#18642=CARTESIAN_POINT ( 'NONE',  ( 4.379528057220339221, -16.55341960407611168, 42.70724293864770260 ) ) ;
#18644=CARTESIAN_POINT ( 'NONE',  ( -8.314922557961024197, 14.29746914071037800, 102.9177570613523756 ) ) ;
#18646=CARTESIAN_POINT ( 'NONE',  ( 14.29746914071037800, 8.314922557961029526, 76.66775706135234714 ) ) ;
#18647=CARTESIAN_POINT ( 'NONE',  ( -19.05341960407611168, -5.049401038298163336, 31.45724293864769550 ) ) ;
#18648=CARTESIAN_POINT ( 'NONE',  ( -0.05219959533937732626, 21.53943276465977519, 97.50109039468567573 ) ) ;
#18649=CARTESIAN_POINT ( 'NONE',  ( 19.05341960407617918, -5.049401038297876454, 96.04275706135231871 ) ) ;
#18650=CARTESIAN_POINT ( 'NONE',  ( 10.81492255796106328, -18.62759615963255655, 75.41775706135233293 ) ) ;
#18651=CARTESIAN_POINT ( 'NONE',  ( -9.474510206698720793, -16.51473224551083518, 49.58442372801899722 ) ) ;
#18652=CARTESIAN_POINT ( 'NONE',  ( 19.03943276465977164, -0.05219959533909143690, 78.74890960531436690 ) ) ;
#18653=CARTESIAN_POINT ( 'NONE',  ( 9.564922557960805705, 16.46253265017160317, 74.58224293864769550 ) ) ;
#18655=CARTESIAN_POINT ( 'NONE',  ( 14.29746914071049879, -8.314922557960816363, 63.33224293864770260 ) ) ;
#18656=CARTESIAN_POINT ( 'NONE',  ( -18.62759615963270932, 10.81492255796079327, 60.83224293864769550 ) ) ;
#18657=CARTESIAN_POINT ( 'NONE',  ( 16.46253265017160672, -9.564922557960803928, 48.33224293864769550 ) ) ;
#18658=CARTESIAN_POINT ( 'NONE',  ( 21.52544592524344225, -5.823673210054117533, 88.54057627198103830 ) ) ;
#18659=CARTESIAN_POINT ( 'NONE',  ( -12.14591786802326823, 12.06949235617739902, 73.12609039468567573 ) ) ;
#18661=CARTESIAN_POINT ( 'NONE',  ( -0.05219959533910754901, -16.53943276465976808, 82.49890960531436690 ) ) ;
#18663=CARTESIAN_POINT ( 'NONE',  ( 14.34966873604972726, -8.224510206698740333, 35.83442372801901143 ) ) ;
#18664=CARTESIAN_POINT ( 'NONE',  ( -0.05219959533910754901, -16.53943276465976808, 112.4989096053143669 ) ) ;
#18665=CARTESIAN_POINT ( 'NONE',  ( 9.474510206698729675, 16.51473224551082808, 72.08442372801900433 ) ) ;
#18666=CARTESIAN_POINT ( 'NONE',  ( -14.34966873604960291, -8.224510206698953496, 66.66557627198102409 ) ) ;
#18667=CARTESIAN_POINT ( 'NONE',  ( -15.72974639402176322, -15.80617190586768395, 49.37609039468569705 ) ) ;
#18668=CARTESIAN_POINT ( 'NONE',  ( 0.05219959533909260263, 19.03943276465977164, 24.99890960531435269 ) ) ;
#18669=CARTESIAN_POINT ( 'NONE',  ( -10.72451020669898014, 18.67979575497178502, 110.4155762719810383 ) ) ;
#18670=CARTESIAN_POINT ( 'NONE',  ( 19.05341960407611168, 5.049401038298154454, 113.9572429386477097 ) ) ;
#18671=CARTESIAN_POINT ( 'NONE',  ( 14.34966873604960469, 8.224510206698951720, 94.16557627198103830 ) ) ;
#18673=CARTESIAN_POINT ( 'NONE',  ( 5.153800228976335163, 19.02544592524342804, 39.79057627198100988 ) ) ;
#18675=CARTESIAN_POINT ( 'NONE',  ( 16.46253265017146816, 9.564922557961045513, 76.66775706135234714 ) ) ;
#18676=CARTESIAN_POINT ( 'NONE',  ( -18.62759615963255300, -10.81492255796106328, 39.16775706135235424 ) ) ;
#18677=CARTESIAN_POINT ( 'NONE',  ( -9.564922557960796823, -16.46253265017161027, 72.08224293864770971 ) ) ;
#18678=CARTESIAN_POINT ( 'NONE',  ( -9.564922557961040184, 16.46253265017147172, 62.91775706135233293 ) ) ;
#18679=CARTESIAN_POINT ( 'NONE',  ( 19.03943276465977164, -0.05219959533909143690, 48.74890960531435979 ) ) ;
#18680=CARTESIAN_POINT ( 'NONE',  ( 12.06949235617757843, -12.14591786802309237, 68.12390960531436690 ) ) ;
#18681=CARTESIAN_POINT ( 'NONE',  ( 16.53943276465976808, -0.05219959533910856209, 53.74890960531437401 ) ) ;
#18682=CARTESIAN_POINT ( 'NONE',  ( -19.03943276465977164, 0.05219959533909376836, 71.24890960531435269 ) ) ;
#18683=CARTESIAN_POINT ( 'NONE',  ( -18.67979575497178146, -10.72451020669898902, 106.6655762719810383 ) ) ;
#18684=CARTESIAN_POINT ( 'NONE',  ( 13.97604488694527802, 13.89961937509977652, 69.37390960531436690 ) ) ;
#18685=CARTESIAN_POINT ( 'NONE',  ( -0.05219959533907301413, -21.53943276465977519, 82.49890960531436690 ) ) ;
#18686=CARTESIAN_POINT ( 'NONE',  ( 13.89961937509957401, 13.97604488694547697, 21.87609039468566152 ) ) ;
#18687=CARTESIAN_POINT ( 'NONE',  ( -19.03943276465977164, 0.05219959533909376836, 41.24890960531435269 ) ) ;
#18688=CARTESIAN_POINT ( 'NONE',  ( 16.52544592524335698, 4.483927247898782831, 106.4594237280190328 ) ) ;
#18689=CARTESIAN_POINT ( 'NONE',  ( -8.224510206698948167, 14.34966873604960824, 100.4155762719810241 ) ) ;
#18690=CARTESIAN_POINT ( 'NONE',  ( -9.474510206698720793, -16.51473224551083518, 109.5844237280190043 ) ) ;
#18691=ORIENTED_EDGE ( 'NONE', *, *, #58823, .T. ) ;
#18692=CARTESIAN_POINT ( 'NONE',  ( -21.52544592524334988, -5.823673210054445271, 33.95942372801901143 ) ) ;
#18693=CARTESIAN_POINT ( 'NONE',  ( 19.02544592524334988, 5.153800228976608722, 56.45942372801898301 ) ) ;
#18694=CARTESIAN_POINT ( 'NONE',  ( -16.55341960407617563, 4.379528057220093196, 113.5427570613523756 ) ) ;
#18695=CARTESIAN_POINT ( 'NONE',  ( -21.53943276465977519, 0.05219959533907696930, 66.24890960531436690 ) ) ;
#18696=CARTESIAN_POINT ( 'NONE',  ( -0.05219959533909027116, -19.03943276465977164, 102.4989096053143669 ) ) ;
#18697=CARTESIAN_POINT ( 'NONE',  ( 4.379528057220339221, -16.55341960407611168, 62.70724293864769550 ) ) ;
#18698=CARTESIAN_POINT ( 'NONE',  ( 19.02544592524343514, -5.153800228976328945, 28.54057627198102409 ) ) ;
#18699=CARTESIAN_POINT ( 'NONE',  ( 19.05341960407611168, 5.049401038298154454, 38.95724293864767418 ) ) ;
#18700=CARTESIAN_POINT ( 'NONE',  ( -16.51473224551082808, 9.474510206698731452, 23.33442372801900078 ) ) ;
#18701=CARTESIAN_POINT ( 'NONE',  ( 4.483927247898790824, -16.52544592524335698, 95.20942372801903275 ) ) ;
#18702=CARTESIAN_POINT ( 'NONE',  ( -21.52544592524334988, -5.823673210054445271, 38.95942372801901854 ) ) ;
#18703=CARTESIAN_POINT ( 'NONE',  ( -4.379528057220086978, -16.55341960407618274, 44.79275706135234714 ) ) ;
#18704=CARTESIAN_POINT ( 'NONE',  ( 10.72451020669898902, -18.67979575497178502, 27.91557627198103830 ) ) ;
#18705=CARTESIAN_POINT ( 'NONE',  ( -16.51473224551069308, -9.474510206698971260, 56.66557627198103120 ) ) ;
#18706=CARTESIAN_POINT ( 'NONE',  ( 0.05219959533937995610, -21.53943276465977519, 95.00109039468568994 ) ) ;
#18707=CARTESIAN_POINT ( 'NONE',  ( -13.89961937509977652, 13.97604488694528158, 75.62390960531438111 ) ) ;
#18708=CARTESIAN_POINT ( 'NONE',  ( 16.53943276465976808, 0.05219959533934440121, 61.25109039468567573 ) ) ;
#18709=CARTESIAN_POINT ( 'NONE',  ( -16.53943276465976808, 0.05219959533911058130, 101.2489096053143669 ) ) ;
#18710=CARTESIAN_POINT ( 'NONE',  ( -8.314922557960811034, -14.29746914071050412, 27.08224293864769550 ) ) ;
#18712=CARTESIAN_POINT ( 'NONE',  ( 21.52544592524334988, 5.823673210054432836, 76.45942372801901854 ) ) ;
#18713=CARTESIAN_POINT ( 'NONE',  ( -9.564922557960796823, -16.46253265017161027, 92.08224293864769550 ) ) ;
#18714=CARTESIAN_POINT ( 'NONE',  ( -19.02544592524342804, 5.153800228976336051, 81.04057627198103830 ) ) ;
#18715=CARTESIAN_POINT ( 'NONE',  ( -19.05341960407611168, -5.049401038298163336, 106.4572429386476955 ) ) ;
#18716=CARTESIAN_POINT ( 'NONE',  ( 16.52544592524342804, -4.483927247898539470, 63.54057627198103830 ) ) ;
#18717=CARTESIAN_POINT ( 'NONE',  ( -16.53943276465976808, 0.05219959533911058130, 21.24890960531436690 ) ) ;
#18718=CARTESIAN_POINT ( 'NONE',  ( -0.05219959533910754901, -16.53943276465976808, 42.49890960531435979 ) ) ;
#18719=LINE ( 'NONE', #113682, #138407 ) ;
#18720=CARTESIAN_POINT ( 'NONE',  ( 16.46253265017146816, 9.564922557961045513, 41.66775706135234003 ) ) ;
#18721=CARTESIAN_POINT ( 'NONE',  ( 5.049401038298161559, -19.05341960407611168, 72.70724293864768129 ) ) ;
#18722=CARTESIAN_POINT ( 'NONE',  ( 19.05341960407617918, -5.049401038297876454, 51.04275706135231871 ) ) ;
#18725=CARTESIAN_POINT ( 'NONE',  ( 5.153800228976615827, -19.02544592524334988, 85.20942372801900433 ) ) ;
#18726=CARTESIAN_POINT ( 'NONE',  ( -8.224510206698735004, -14.34966873604973081, 79.58442372801903275 ) ) ;
#18728=CARTESIAN_POINT ( 'NONE',  ( -19.02544592524342804, 5.153800228976336051, 106.0405762719810241 ) ) ;
#18729=CARTESIAN_POINT ( 'NONE',  ( -0.05219959533937732626, 21.53943276465977519, 27.50109039468567929 ) ) ;
#18730=CARTESIAN_POINT ( 'NONE',  ( 9.564922557961047289, -16.46253265017146816, 95.41775706135233293 ) ) ;
#18731=CARTESIAN_POINT ( 'NONE',  ( 17.40861289039004234, 6.110651285853279546, 88.87232470827434838 ) ) ;
#18732=CARTESIAN_POINT ( 'NONE',  ( 9.474510206698971260, -16.51473224551069308, 47.91557627198102409 ) ) ;
#18734=CARTESIAN_POINT ( 'NONE',  ( 0.05219959533909260263, 19.03943276465977164, 109.9989096053143669 ) ) ;
#18735=CARTESIAN_POINT ( 'NONE',  ( 12.14591786802309770, 12.06949235617756955, 59.37390960531436690 ) ) ;
#18736=CARTESIAN_POINT ( 'NONE',  ( 16.51473224551069308, 9.474510206698969483, 49.16557627198102409 ) ) ;
#18737=CARTESIAN_POINT ( 'NONE',  ( -16.46253265017160317, 9.564922557960807481, 65.83224293864769550 ) ) ;
#18738=CARTESIAN_POINT ( 'NONE',  ( -9.564922557961040184, 16.46253265017147172, 62.91775706135233293 ) ) ;
#18739=CARTESIAN_POINT ( 'NONE',  ( 19.03943276465977164, 0.05219959533936151252, 26.25109039468566507 ) ) ;
#18740=CARTESIAN_POINT ( 'NONE',  ( -16.46253265017160317, 9.564922557960807481, 70.83224293864770971 ) ) ;
#18741=CARTESIAN_POINT ( 'NONE',  ( -5.823673210054116645, -21.52544592524344225, 62.29057627198102409 ) ) ;
#18742=CARTESIAN_POINT ( 'NONE',  ( 8.224510206698953496, -14.34966873604960469, 72.91557627198103830 ) ) ;
#18743=CARTESIAN_POINT ( 'NONE',  ( 19.03943276465977164, 0.05219959533936151252, 36.25109039468567573 ) ) ;
#18744=CARTESIAN_POINT ( 'NONE',  ( -16.46253265017160317, 9.564922557960807481, 115.8322429386477097 ) ) ;
#18745=CARTESIAN_POINT ( 'NONE',  ( -10.81492255796078084, -18.62759615963271287, 52.08224293864768839 ) ) ;
#18746=CARTESIAN_POINT ( 'NONE',  ( 0.05219959533907565091, 21.53943276465977519, 29.99890960531435979 ) ) ;
#18747=CARTESIAN_POINT ( 'NONE',  ( 5.153800228976335163, 19.02544592524342804, 49.79057627198100988 ) ) ;
#18748=CARTESIAN_POINT ( 'NONE',  ( 19.02544592524343514, -5.153800228976328945, 43.54057627198103120 ) ) ;
#18749=CARTESIAN_POINT ( 'NONE',  ( 14.29746914071049879, -8.314922557960816363, 103.3322429386476955 ) ) ;
#18751=CARTESIAN_POINT ( 'NONE',  ( -21.52544592524343514, 5.823673210054127303, 111.0405762719810525 ) ) ;
#18752=CARTESIAN_POINT ( 'NONE',  ( -9.564922557960796823, -16.46253265017161027, 112.0822429386476955 ) ) ;
#18753=CARTESIAN_POINT ( 'NONE',  ( 18.62759615963255655, 10.81492255796105972, 21.66775706135235069 ) ) ;
#18754=CARTESIAN_POINT ( 'NONE',  ( 0.05219959533910956823, 16.53943276465976808, 114.9989096053143669 ) ) ;
#18755=CARTESIAN_POINT ( 'NONE',  ( 5.719274019375991003, -21.55341960407610458, 97.70724293864772392 ) ) ;
#18756=CARTESIAN_POINT ( 'NONE',  ( -13.97604488694547697, 13.89961937509957934, 48.12609039468566863 ) ) ;
#18757=CARTESIAN_POINT ( 'NONE',  ( -19.02544592524342804, 5.153800228976336051, 26.04057627198103120 ) ) ;
#18758=CARTESIAN_POINT ( 'NONE',  ( -16.46253265017160317, 9.564922557960807481, 25.83224293864769194 ) ) ;
#18760=CARTESIAN_POINT ( 'NONE',  ( 4.379528057220092307, 16.55341960407617563, 52.29275706135236135 ) ) ;
#18761=CARTESIAN_POINT ( 'NONE',  ( -4.379528057220328563, 16.55341960407611168, 115.2072429386476955 ) ) ;
#18763=CARTESIAN_POINT ( 'NONE',  ( 13.89961937509977652, -13.97604488694527269, 78.12390960531433848 ) ) ;
#18764=CARTESIAN_POINT ( 'NONE',  ( 16.52544592524342804, -4.483927247898539470, 103.5405762719810383 ) ) ;
#18765=CARTESIAN_POINT ( 'NONE',  ( 5.823673210054125526, 21.52544592524343514, 39.79057627198103830 ) ) ;
#18766=CARTESIAN_POINT ( 'NONE',  ( -0.05219959533910754901, -16.53943276465976808, 82.49890960531436690 ) ) ;
#18767=CARTESIAN_POINT ( 'NONE',  ( -14.29746914071037622, -8.314922557961029526, 34.16775706135234714 ) ) ;
#18768=CARTESIAN_POINT ( 'NONE',  ( 21.55341960407619695, -5.719274019375665929, 91.04275706135236135 ) ) ;
#18769=CARTESIAN_POINT ( 'NONE',  ( 13.97604488694527802, 13.89961937509977652, 29.37390960531435979 ) ) ;
#18770=CARTESIAN_POINT ( 'NONE',  ( -4.483927247898782831, 16.52544592524335698, 92.70942372801901854 ) ) ;
#18771=CARTESIAN_POINT ( 'NONE',  ( -12.14591786802309592, -12.06949235617757132, 46.87390960531435979 ) ) ;
#18772=CARTESIAN_POINT ( 'NONE',  ( 5.049401038298161559, -19.05341960407611168, 52.70724293864767418 ) ) ;
#18773=CARTESIAN_POINT ( 'NONE',  ( -18.62759615963255300, -10.81492255796106328, 94.16775706135237556 ) ) ;
#18774=CARTESIAN_POINT ( 'NONE',  ( 21.55341960407610458, 5.719274019375980345, 103.9572429386476813 ) ) ;
#18775=CARTESIAN_POINT ( 'NONE',  ( 18.62759615963255655, 10.81492255796105972, 76.66775706135234714 ) ) ;
#18776=CARTESIAN_POINT ( 'NONE',  ( 12.14591786802327356, -12.06949235617739191, 40.62609039468567573 ) ) ;
#18777=CARTESIAN_POINT ( 'NONE',  ( 4.483927247898545687, 16.52544592524342804, 59.79057627198103120 ) ) ;
#18778=CARTESIAN_POINT ( 'NONE',  ( 21.52544592524334988, 5.823673210054432836, 86.45942372801901854 ) ) ;
#18780=CARTESIAN_POINT ( 'NONE',  ( 12.06949235617739724, 12.14591786802326823, 106.8760903946856899 ) ) ;
#18781=CARTESIAN_POINT ( 'NONE',  ( 17.12812012977042642, -6.668231424565811416, 46.14051240676854349 ) ) ;
#18783=CARTESIAN_POINT ( 'NONE',  ( 0.05219959533910956823, 16.53943276465976808, 34.99890960531435979 ) ) ;
#18784=CARTESIAN_POINT ( 'NONE',  ( -14.29746914071037622, -8.314922557961029526, 79.16775706135234714 ) ) ;
#18785=CARTESIAN_POINT ( 'NONE',  ( -13.97604488694527625, -13.89961937509977652, 86.87390960531436690 ) ) ;
#18787=CARTESIAN_POINT ( 'NONE',  ( -16.51473224551069308, -9.474510206698971260, 101.6655762719810241 ) ) ;
#18788=CARTESIAN_POINT ( 'NONE',  ( 5.823673210054444382, -21.52544592524334988, 105.2094237280190328 ) ) ;
#18789=CARTESIAN_POINT ( 'NONE',  ( 4.483927247898790824, -16.52544592524335698, 105.2094237280190328 ) ) ;
#18790=CARTESIAN_POINT ( 'NONE',  ( 16.53943276465976808, -0.05219959533910856209, 78.74890960531436690 ) ) ;
#18791=CARTESIAN_POINT ( 'NONE',  ( -13.89961937509977652, 13.97604488694528158, 80.62390960531436690 ) ) ;
#18793=CARTESIAN_POINT ( 'NONE',  ( 16.52544592524335698, 4.483927247898782831, 31.45942372801901854 ) ) ;
#18794=CARTESIAN_POINT ( 'NONE',  ( -13.97604488694527625, -13.89961937509977652, 31.87390960531435979 ) ) ;
#18795=CARTESIAN_POINT ( 'NONE',  ( -9.474510206698964154, 16.51473224551069663, 85.41557627198102409 ) ) ;
#18796=CARTESIAN_POINT ( 'NONE',  ( 12.06949235617739724, 12.14591786802326823, 26.87609039468567218 ) ) ;
#18798=CARTESIAN_POINT ( 'NONE',  ( 9.474510206698729675, 16.51473224551082808, 27.08442372801900433 ) ) ;
#18799=CARTESIAN_POINT ( 'NONE',  ( 4.483927247898790824, -16.52544592524335698, 90.20942372801903275 ) ) ;
#18800=CARTESIAN_POINT ( 'NONE',  ( -5.153800228976607833, 19.02544592524334988, 102.7094237280189759 ) ) ;
#18801=CARTESIAN_POINT ( 'NONE',  ( -16.51473224551069308, -9.474510206698971260, 26.66557627198103120 ) ) ;
#18802=CARTESIAN_POINT ( 'NONE',  ( -4.483927247898782831, 16.52544592524335698, 77.70942372801900433 ) ) ;
#18803=CARTESIAN_POINT ( 'NONE',  ( -16.53943276465976808, -0.05219959533934237506, 63.75109039468568284 ) ) ;
#18804=CARTESIAN_POINT ( 'NONE',  ( -16.46253265017160317, 9.564922557960807481, 25.83224293864769194 ) ) ;
#18805=CARTESIAN_POINT ( 'NONE',  ( 19.05341960407617918, -5.049401038297876454, 66.04275706135233293 ) ) ;
#18806=CARTESIAN_POINT ( 'NONE',  ( 16.51473224551083163, -9.474510206698727899, 20.83442372801899722 ) ) ;
#18807=CARTESIAN_POINT ( 'NONE',  ( -19.05341960407611168, -5.049401038298163336, 51.45724293864770260 ) ) ;
#18808=CARTESIAN_POINT ( 'NONE',  ( 13.89961937509977652, -13.97604488694527269, 93.12390960531436690 ) ) ;
#18809=CARTESIAN_POINT ( 'NONE',  ( -12.14591786802309592, -12.06949235617757132, 86.87390960531438111 ) ) ;
#18811=CARTESIAN_POINT ( 'NONE',  ( -19.05341960407617563, 5.049401038297882671, 53.54275706135231871 ) ) ;
#18812=CARTESIAN_POINT ( 'NONE',  ( -15.80617190586745835, -15.72974639402198527, 46.87390960531435979 ) ) ;
#18813=CARTESIAN_POINT ( 'NONE',  ( -10.72451020669870658, -18.67979575497194134, 104.5844237280190185 ) ) ;
#18814=CARTESIAN_POINT ( 'NONE',  ( -5.153800228976328057, -19.02544592524343514, 92.29057627198099567 ) ) ;
#18815=CARTESIAN_POINT ( 'NONE',  ( 15.80617190586769283, -15.72974639402175789, 100.6260903946857184 ) ) ;
#18816=CARTESIAN_POINT ( 'NONE',  ( -10.81492255796078084, -18.62759615963271287, 62.08224293864769550 ) ) ;
#18817=CARTESIAN_POINT ( 'NONE',  ( 19.02544592524343514, -5.153800228976328945, 93.54057627198102409 ) ) ;
#18818=CARTESIAN_POINT ( 'NONE',  ( 19.03943276465977164, 0.05219959533936151252, 91.25109039468566152 ) ) ;
#18819=CARTESIAN_POINT ( 'NONE',  ( -19.02544592524342804, 5.153800228976336051, 111.0405762719810099 ) ) ;
#18820=CARTESIAN_POINT ( 'NONE',  ( 19.02544592524334988, 5.153800228976608722, 106.4594237280190185 ) ) ;
#18821=CARTESIAN_POINT ( 'NONE',  ( 12.14591786802309770, 12.06949235617756955, 109.3739096053143811 ) ) ;
#18822=CARTESIAN_POINT ( 'NONE',  ( -16.46253265017160317, 9.564922557960807481, 80.83224293864769550 ) ) ;
#18823=CARTESIAN_POINT ( 'NONE',  ( -21.52544592524343514, 5.823673210054127303, 76.04057627198102409 ) ) ;
#18824=CARTESIAN_POINT ( 'NONE',  ( 12.14591786802327356, -12.06949235617739191, 45.62609039468567573 ) ) ;
#18825=CARTESIAN_POINT ( 'NONE',  ( -18.67979575497193778, 10.72451020669871902, 53.33442372801901854 ) ) ;
#18826=CARTESIAN_POINT ( 'NONE',  ( -5.719274019375665041, -21.55341960407619695, 94.79275706135234714 ) ) ;
#18827=CARTESIAN_POINT ( 'NONE',  ( 16.52544592524335698, 4.483927247898782831, 101.4594237280190185 ) ) ;
#18828=CARTESIAN_POINT ( 'NONE',  ( 16.51473224551069308, 9.474510206698969483, 94.16557627198103830 ) ) ;
#18829=CARTESIAN_POINT ( 'NONE',  ( 4.379528057220339221, -16.55341960407611168, 92.70724293864770971 ) ) ;
#18830=CARTESIAN_POINT ( 'NONE',  ( 12.14591786802309770, 12.06949235617756955, 29.37390960531435269 ) ) ;
#18831=CARTESIAN_POINT ( 'NONE',  ( -19.02544592524334988, -5.153800228976617603, 73.95942372801900433 ) ) ;
#18832=CARTESIAN_POINT ( 'NONE',  ( -10.72451020669870658, -18.67979575497194134, 49.58442372801901143 ) ) ;
#18833=CARTESIAN_POINT ( 'NONE',  ( 19.05341960407617918, -5.049401038297876454, 31.04275706135232227 ) ) ;
#18834=CARTESIAN_POINT ( 'NONE',  ( -14.34966873604960291, -8.224510206698953496, 86.66557627198102409 ) ) ;
#18835=CARTESIAN_POINT ( 'NONE',  ( 16.51473224551069308, 9.474510206698969483, 109.1655762719810383 ) ) ;
#18836=CARTESIAN_POINT ( 'NONE',  ( -14.34966873604960291, -8.224510206698953496, 21.66557627198102409 ) ) ;
#18837=CARTESIAN_POINT ( 'NONE',  ( -18.62759615963255300, -10.81492255796106328, 79.16775706135234714 ) ) ;
#18838=CARTESIAN_POINT ( 'NONE',  ( 0.05219959533934541429, -16.53943276465976808, 65.00109039468568994 ) ) ;
#18839=CARTESIAN_POINT ( 'NONE',  ( -4.483927247898782831, 16.52544592524335698, 112.7094237280190328 ) ) ;
#18840=CARTESIAN_POINT ( 'NONE',  ( -5.823673210054431948, 21.52544592524334988, 57.70942372801901143 ) ) ;
#18842=CARTESIAN_POINT ( 'NONE',  ( -10.81492255796105439, 18.62759615963255655, 27.91775706135234358 ) ) ;
#18843=CARTESIAN_POINT ( 'NONE',  ( -16.52544592524342804, 4.483927247898546575, 111.0405762719810525 ) ) ;
#18844=CARTESIAN_POINT ( 'NONE',  ( 17.50000000000000000, -5.500000000000000888, 28.29690382534172244 ) ) ;
#18845=CARTESIAN_POINT ( 'NONE',  ( -16.53943276465976808, 0.05219959533911058130, 61.24890960531435979 ) ) ;
#18846=CARTESIAN_POINT ( 'NONE',  ( -0.05219959533909027116, -19.03943276465977164, 77.49890960531435269 ) ) ;
#18847=CARTESIAN_POINT ( 'NONE',  ( 0.05219959533934541429, -16.53943276465976808, 105.0010903946856757 ) ) ;
#18848=CARTESIAN_POINT ( 'NONE',  ( 13.89961937509977652, -13.97604488694527269, 38.12390960531436690 ) ) ;
#18849=CARTESIAN_POINT ( 'NONE',  ( 15.80617190586746368, 15.72974639402197994, 59.37390960531436690 ) ) ;
#18850=CARTESIAN_POINT ( 'NONE',  ( 12.14591786802309770, 12.06949235617756955, 89.37390960531435269 ) ) ;
#18851=CARTESIAN_POINT ( 'NONE',  ( 5.823673210054125526, 21.52544592524343514, 89.79057627198103830 ) ) ;
#18852=CARTESIAN_POINT ( 'NONE',  ( 13.89961937509977652, -13.97604488694527269, 103.1239096053143527 ) ) ;
#18853=CARTESIAN_POINT ( 'NONE',  ( -19.05341960407611168, -5.049401038298163336, 56.45724293864768129 ) ) ;
#18854=CARTESIAN_POINT ( 'NONE',  ( -19.02544592524334988, -5.153800228976617603, 93.95942372801900433 ) ) ;
#18855=CARTESIAN_POINT ( 'NONE',  ( 10.72451020669898902, -18.67979575497178502, 42.91557627198103120 ) ) ;
#18856=CARTESIAN_POINT ( 'NONE',  ( 5.719274019375673035, 21.55341960407619339, 67.29275706135234714 ) ) ;
#18857=CARTESIAN_POINT ( 'NONE',  ( 5.153800228976335163, 19.02544592524342804, 59.79057627198100988 ) ) ;
#18858=CARTESIAN_POINT ( 'NONE',  ( -5.049401038298153566, 19.05341960407611168, 80.20724293864769550 ) ) ;
#18859=CARTESIAN_POINT ( 'NONE',  ( 14.29746914071037800, 8.314922557961029526, 61.66775706135235424 ) ) ;
#18860=CARTESIAN_POINT ( 'NONE',  ( 5.719274019375673035, 21.55341960407619339, 42.29275706135235424 ) ) ;
#18861=CARTESIAN_POINT ( 'NONE',  ( -5.823673210054431948, 21.52544592524334988, 67.70942372801901854 ) ) ;
#18862=CARTESIAN_POINT ( 'NONE',  ( -16.51473224551069308, -9.474510206698971260, 111.6655762719810383 ) ) ;
#18863=CARTESIAN_POINT ( 'NONE',  ( 10.81492255796078972, 18.62759615963270932, 94.58224293864769550 ) ) ;
#18864=CARTESIAN_POINT ( 'NONE',  ( 18.67979575497194134, -10.72451020669871369, 35.83442372801901143 ) ) ;
#18865=CARTESIAN_POINT ( 'NONE',  ( 16.53943276465976808, 0.05219959533934440121, 71.25109039468568994 ) ) ;
#18866=CARTESIAN_POINT ( 'NONE',  ( 0.05219959533907565091, 21.53943276465977519, 59.99890960531436690 ) ) ;
#18867=CARTESIAN_POINT ( 'NONE',  ( 0.05219959533936267826, -19.03943276465977164, 40.00109039468566152 ) ) ;
#18868=CARTESIAN_POINT ( 'NONE',  ( 19.05341960407611168, 5.049401038298154454, 68.95724293864769550 ) ) ;
#18869=CARTESIAN_POINT ( 'NONE',  ( -4.379528057220086978, -16.55341960407618274, 109.7927570613523613 ) ) ;
#18870=CARTESIAN_POINT ( 'NONE',  ( -17.49999999999999645, -3.471454075611748902, 105.5166741885564505 ) ) ;
#18871=CARTESIAN_POINT ( 'NONE',  ( -19.05341960407611168, -5.049401038298163336, 106.4572429386476955 ) ) ;
#18873=CARTESIAN_POINT ( 'NONE',  ( -9.564922557961040184, 16.46253265017147172, 77.91775706135234714 ) ) ;
#18874=CARTESIAN_POINT ( 'NONE',  ( 21.53943276465977519, -0.05219959533907433946, 53.74890960531437401 ) ) ;
#18875=CARTESIAN_POINT ( 'NONE',  ( -16.53943276465976808, 0.05219959533911058130, 36.24890960531435979 ) ) ;
#18876=CARTESIAN_POINT ( 'NONE',  ( -16.46253265017146816, -9.564922557961047289, 109.1677570613523471 ) ) ;
#18877=CARTESIAN_POINT ( 'NONE',  ( -19.02544592524342804, 5.153800228976336051, 31.04057627198102409 ) ) ;
#18878=CARTESIAN_POINT ( 'NONE',  ( 16.52544592524335698, 4.483927247898782831, 21.45942372801901499 ) ) ;
#18879=CARTESIAN_POINT ( 'NONE',  ( -10.81492255796078084, -18.62759615963271287, 92.08224293864769550 ) ) ;
#18880=CARTESIAN_POINT ( 'NONE',  ( 5.049401038297881783, 19.05341960407617563, 57.29275706135231871 ) ) ;
#18881=CARTESIAN_POINT ( 'NONE',  ( 12.14591786802327356, -12.06949235617739191, 80.62609039468567573 ) ) ;
#18882=CARTESIAN_POINT ( 'NONE',  ( 13.89961937509977652, -13.97604488694527269, 73.12390960531436690 ) ) ;
#18883=CARTESIAN_POINT ( 'NONE',  ( -12.06949235617756955, 12.14591786802309770, 75.62390960531439532 ) ) ;
#18884=CARTESIAN_POINT ( 'NONE',  ( 16.46253265017160672, -9.564922557960803928, 43.33224293864769550 ) ) ;
#18885=CARTESIAN_POINT ( 'NONE',  ( 0.05219959533910956823, 16.53943276465976808, 54.99890960531435269 ) ) ;
#18886=CARTESIAN_POINT ( 'NONE',  ( -13.97604488694527625, -13.89961937509977652, 21.87390960531435979 ) ) ;
#18888=CARTESIAN_POINT ( 'NONE',  ( 0.05219959533910956823, 16.53943276465976808, 29.99890960531435979 ) ) ;
#18889=CARTESIAN_POINT ( 'NONE',  ( -16.51473224551069308, -9.474510206698971260, 76.66557627198103830 ) ) ;
#18891=CARTESIAN_POINT ( 'NONE',  ( -9.474510206698720793, -16.51473224551083518, 44.58442372801900433 ) ) ;
#18892=CARTESIAN_POINT ( 'NONE',  ( -0.05219959533934338120, 16.53943276465976808, 42.50109039468567573 ) ) ;
#18893=CARTESIAN_POINT ( 'NONE',  ( 21.55341960407610458, 5.719274019375980345, 68.95724293864769550 ) ) ;
#18894=CARTESIAN_POINT ( 'NONE',  ( 9.564922557961047289, -16.46253265017146816, 20.41775706135233293 ) ) ;
#18895=CARTESIAN_POINT ( 'NONE',  ( 13.89961937509977652, -13.97604488694527269, 68.12390960531436690 ) ) ;
#18897=CARTESIAN_POINT ( 'NONE',  ( 13.97604488694527802, 13.89961937509977652, 104.3739096053143385 ) ) ;
#18898=CARTESIAN_POINT ( 'NONE',  ( -21.53943276465977519, -0.05219959533937600094, 38.75109039468567573 ) ) ;
#18899=CARTESIAN_POINT ( 'NONE',  ( 4.483927247898545687, 16.52544592524342804, 104.7905762719810241 ) ) ;
#18900=CARTESIAN_POINT ( 'NONE',  ( 5.719274019375991003, -21.55341960407610458, 107.7072429386476955 ) ) ;
#18901=CARTESIAN_POINT ( 'NONE',  ( -13.97604488694527625, -13.89961937509977652, 81.87390960531436690 ) ) ;
#18903=CARTESIAN_POINT ( 'NONE',  ( 0.05219959533937995610, -21.53943276465977519, 25.00109039468567218 ) ) ;
#18905=CARTESIAN_POINT ( 'NONE',  ( 5.153800228976335163, 19.02544592524342804, 84.79057627198099567 ) ) ;
#18908=CARTESIAN_POINT ( 'NONE',  ( 13.89961937509977652, -13.97604488694527269, 38.12390960531436690 ) ) ;
#18909=CARTESIAN_POINT ( 'NONE',  ( 5.049401038297881783, 19.05341960407617563, 107.2927570613523187 ) ) ;
#18911=CARTESIAN_POINT ( 'NONE',  ( 12.14591786802309770, 12.06949235617756955, 109.3739096053143811 ) ) ;
#18912=CARTESIAN_POINT ( 'NONE',  ( -18.62759615963255300, -10.81492255796106328, 89.16775706135236135 ) ) ;
#18913=CARTESIAN_POINT ( 'NONE',  ( -19.03943276465977164, 0.05219959533909376836, 71.24890960531435269 ) ) ;
#18914=CARTESIAN_POINT ( 'NONE',  ( 21.53943276465977519, 0.05219959533937863772, 41.25109039468568284 ) ) ;
#18915=CARTESIAN_POINT ( 'NONE',  ( -15.80617190586768217, 15.72974639402176855, 33.12609039468569705 ) ) ;
#18917=CARTESIAN_POINT ( 'NONE',  ( -19.05341960407611168, -5.049401038298163336, 81.45724293864769550 ) ) ;
#18919=CARTESIAN_POINT ( 'NONE',  ( 16.55341960407618274, -4.379528057220086978, 21.04275706135234714 ) ) ;
#18920=CARTESIAN_POINT ( 'NONE',  ( -21.55341960407610458, -5.719274019375992779, 41.45724293864769550 ) ) ;
#18921=CARTESIAN_POINT ( 'NONE',  ( -5.719274019375665041, -21.55341960407619695, 79.79275706135236135 ) ) ;
#18922=CARTESIAN_POINT ( 'NONE',  ( 0.05219959533909260263, 19.03943276465977164, 114.9989096053143669 ) ) ;
#18923=CARTESIAN_POINT ( 'NONE',  ( -13.97604488694547697, 13.89961937509957934, 93.12609039468566152 ) ) ;
#18924=CARTESIAN_POINT ( 'NONE',  ( 19.03943276465977164, -0.05219959533909143690, 53.74890960531436690 ) ) ;
#18925=CARTESIAN_POINT ( 'NONE',  ( -13.89961937509977652, 13.97604488694528158, 85.62390960531433848 ) ) ;
#18927=CARTESIAN_POINT ( 'NONE',  ( -16.55341960407611168, -4.379528057220339221, 101.4572429386476955 ) ) ;
#18928=CARTESIAN_POINT ( 'NONE',  ( 8.314922557960818139, 14.29746914071049879, 109.5822429386476955 ) ) ;
#18929=CARTESIAN_POINT ( 'NONE',  ( 9.564922557960805705, 16.46253265017160317, 114.5822429386476955 ) ) ;
#18930=CARTESIAN_POINT ( 'NONE',  ( -14.34966873604972548, 8.224510206698743886, 78.33442372801901854 ) ) ;
#18931=CARTESIAN_POINT ( 'NONE',  ( 14.29746914071049879, -8.314922557960816363, 53.33224293864769550 ) ) ;
#18932=CARTESIAN_POINT ( 'NONE',  ( 9.474510206698971260, -16.51473224551069308, 37.91557627198102409 ) ) ;
#18933=CARTESIAN_POINT ( 'NONE',  ( 5.719274019375673035, 21.55341960407619339, 82.29275706135234714 ) ) ;
#18934=CARTESIAN_POINT ( 'NONE',  ( 0.05219959533937995610, -21.53943276465977519, 75.00109039468568994 ) ) ;
#18935=CARTESIAN_POINT ( 'NONE',  ( -19.02544592524334988, -5.153800228976617603, 88.95942372801897591 ) ) ;
#18936=CARTESIAN_POINT ( 'NONE',  ( -4.483927247898539470, -16.52544592524342804, 62.29057627198102409 ) ) ;
#18937=CARTESIAN_POINT ( 'NONE',  ( -5.823673210054116645, -21.52544592524344225, 107.2905762719810525 ) ) ;
#18938=CARTESIAN_POINT ( 'NONE',  ( -10.72451020669898014, 18.67979575497178502, 50.41557627198103120 ) ) ;
#18941=CARTESIAN_POINT ( 'NONE',  ( -9.564922557960796823, -16.46253265017161027, 72.08224293864770971 ) ) ;
#18942=CARTESIAN_POINT ( 'NONE',  ( -0.05219959533910754901, -16.53943276465976808, 32.49890960531435979 ) ) ;
#18943=CARTESIAN_POINT ( 'NONE',  ( -4.483927247898539470, -16.52544592524342804, 27.29057627198103120 ) ) ;
#18944=CARTESIAN_POINT ( 'NONE',  ( -16.53943276465976808, -0.05219959533934237506, 88.75109039468567573 ) ) ;
#18945=CARTESIAN_POINT ( 'NONE',  ( 9.474510206698729675, 16.51473224551082808, 37.08442372801899722 ) ) ;
#18946=CARTESIAN_POINT ( 'NONE',  ( 16.79531203550649110, 7.028104445595497296, 48.75244988220443787 ) ) ;
#18947=CARTESIAN_POINT ( 'NONE',  ( -13.89961937509977652, 13.97604488694528158, 85.62390960531433848 ) ) ;
#18948=CARTESIAN_POINT ( 'NONE',  ( -4.483927247898539470, -16.52544592524342804, 57.29057627198103120 ) ) ;
#18949=CARTESIAN_POINT ( 'NONE',  ( 16.21995358207306381, -7.366697692864171643, 102.4355100151216647 ) ) ;
#18950=CARTESIAN_POINT ( 'NONE',  ( -15.80617190586745835, -15.72974639402198527, 26.87390960531435979 ) ) ;
#18951=CARTESIAN_POINT ( 'NONE',  ( 5.823673210054125526, 21.52544592524343514, 59.79057627198103120 ) ) ;
#18952=ORIENTED_EDGE ( 'NONE', *, *, #151324, .T. ) ;
#18953=CARTESIAN_POINT ( 'NONE',  ( 8.224510206698953496, -14.34966873604960469, 97.91557627198103830 ) ) ;
#18954=CARTESIAN_POINT ( 'NONE',  ( -8.314922557961024197, 14.29746914071037800, 42.91775706135235424 ) ) ;
#18955=CARTESIAN_POINT ( 'NONE',  ( 0.05219959533910956823, 16.53943276465976808, 79.99890960531435269 ) ) ;
#18957=CARTESIAN_POINT ( 'NONE',  ( 5.049401038297881783, 19.05341960407617563, 82.29275706135229029 ) ) ;
#18958=CARTESIAN_POINT ( 'NONE',  ( 13.97604488694527802, 13.89961937509977652, 114.3739096053143669 ) ) ;
#18960=CARTESIAN_POINT ( 'NONE',  ( -13.97604488694527625, -13.89961937509977830, 41.87390960531435269 ) ) ;
#18961=CARTESIAN_POINT ( 'NONE',  ( -8.314922557961024197, 14.29746914071037800, 27.91775706135234358 ) ) ;
#18962=CARTESIAN_POINT ( 'NONE',  ( -16.52544592524342804, 4.483927247898546575, 31.04057627198102409 ) ) ;
#18963=CARTESIAN_POINT ( 'NONE',  ( -21.53943276465977519, 0.05219959533907696930, 61.24890960531435979 ) ) ;
#18964=CARTESIAN_POINT ( 'NONE',  ( -16.51473224551082808, 9.474510206698731452, 88.33442372801900433 ) ) ;
#18965=CARTESIAN_POINT ( 'NONE',  ( 10.81492255796078972, 18.62759615963270932, 54.58224293864769550 ) ) ;
#18966=CARTESIAN_POINT ( 'NONE',  ( -21.55341960407619339, 5.719274019375674811, 83.54275706135234714 ) ) ;
#18968=CARTESIAN_POINT ( 'NONE',  ( 8.224510206698742110, 14.34966873604972548, 37.08442372801901143 ) ) ;
#18969=CARTESIAN_POINT ( 'NONE',  ( 16.46253265017160672, -9.564922557960803928, 23.33224293864769194 ) ) ;
#18970=CARTESIAN_POINT ( 'NONE',  ( -5.049401038298153566, 19.05341960407611168, 85.20724293864766707 ) ) ;
#18971=CARTESIAN_POINT ( 'NONE',  ( 13.89961937509977652, -13.97604488694527269, 38.12390960531436690 ) ) ;
#18972=CARTESIAN_POINT ( 'NONE',  ( -16.53943276465976808, 0.05219959533911058130, 106.2489096053143811 ) ) ;
#18974=CARTESIAN_POINT ( 'NONE',  ( -13.97604488694527625, -13.89961937509977652, 106.8739096053143669 ) ) ;
#18975=ORIENTED_EDGE ( 'NONE', *, *, #73081, .F. ) ;
#18976=CARTESIAN_POINT ( 'NONE',  ( 8.224510206698742110, 14.34966873604972548, 62.08442372801901143 ) ) ;
#18977=CARTESIAN_POINT ( 'NONE',  ( 10.81492255796078972, 18.62759615963270932, 94.58224293864769550 ) ) ;
#18978=CARTESIAN_POINT ( 'NONE',  ( -0.05219959533909027116, -19.03943276465977164, 37.49890960531436690 ) ) ;
#18979=CARTESIAN_POINT ( 'NONE',  ( 19.02544592524334988, 5.153800228976608722, 71.45942372801900433 ) ) ;
#18980=CARTESIAN_POINT ( 'NONE',  ( 18.67979575497194134, -10.72451020669871369, 30.83442372801902209 ) ) ;
#18981=CARTESIAN_POINT ( 'NONE',  ( -13.89961937509977652, 13.97604488694528158, 70.62390960531432427 ) ) ;
#18982=CARTESIAN_POINT ( 'NONE',  ( -19.02544592524342804, 5.153800228976336051, 101.0405762719810241 ) ) ;
#18983=VERTEX_POINT ( 'NONE', #86043 ) ;
#18984=CARTESIAN_POINT ( 'NONE',  ( 4.483927247898790824, -16.52544592524335698, 35.20942372801901854 ) ) ;
#18985=CARTESIAN_POINT ( 'NONE',  ( 21.53943276465977519, 0.05219959533937863772, 21.25109039468567218 ) ) ;
#18986=CARTESIAN_POINT ( 'NONE',  ( -12.06949235617756955, 12.14591786802309770, 100.6239096053143811 ) ) ;
#18987=CARTESIAN_POINT ( 'NONE',  ( -5.049401038298153566, 19.05341960407611168, 90.20724293864766707 ) ) ;
#18988=CARTESIAN_POINT ( 'NONE',  ( -19.05341960407617563, 5.049401038297882671, 78.54275706135233293 ) ) ;
#18989=CARTESIAN_POINT ( 'NONE',  ( 15.72974639402199770, -15.80617190586745480, 83.12390960531436690 ) ) ;
#18990=CARTESIAN_POINT ( 'NONE',  ( -16.55341960407611168, -4.379528057220339221, 46.45724293864769550 ) ) ;
#18991=CARTESIAN_POINT ( 'NONE',  ( 16.51473224551083163, -9.474510206698727899, 20.83442372801899722 ) ) ;
#18992=CARTESIAN_POINT ( 'NONE',  ( 14.34966873604972726, -8.224510206698740333, 75.83442372801900433 ) ) ;
#18993=CARTESIAN_POINT ( 'NONE',  ( -9.474510206698964154, 16.51473224551069663, 110.4155762719810383 ) ) ;
#18994=CARTESIAN_POINT ( 'NONE',  ( 5.049401038298161559, -19.05341960407611168, 47.70724293864770260 ) ) ;
#18995=CARTESIAN_POINT ( 'NONE',  ( -18.67979575497193778, 10.72451020669871902, 53.33442372801901854 ) ) ;
#18996=CARTESIAN_POINT ( 'NONE',  ( -18.67979575497193778, 10.72451020669871902, 63.33442372801900433 ) ) ;
#18997=CARTESIAN_POINT ( 'NONE',  ( -19.02544592524342804, 5.153800228976336051, 66.04057627198103830 ) ) ;
#18998=CARTESIAN_POINT ( 'NONE',  ( 18.67979575497194134, -10.72451020669871369, 45.83442372801901854 ) ) ;
#18999=CARTESIAN_POINT ( 'NONE',  ( 5.049401038297881783, 19.05341960407617563, 87.29275706135234714 ) ) ;
#19001=CARTESIAN_POINT ( 'NONE',  ( -16.46253265017160317, 9.564922557960807481, 55.83224293864769550 ) ) ;
#19002=CARTESIAN_POINT ( 'NONE',  ( 14.29746914071037800, 8.314922557961029526, 86.66775706135234714 ) ) ;
#19003=CARTESIAN_POINT ( 'NONE',  ( -19.05341960407611168, -5.049401038298163336, 61.45724293864769550 ) ) ;
#19004=CARTESIAN_POINT ( 'NONE',  ( 19.02544592524343514, -5.153800228976328945, 113.5405762719810241 ) ) ;
#19005=CARTESIAN_POINT ( 'NONE',  ( 9.474510206698971260, -16.51473224551069308, 47.91557627198102409 ) ) ;
#19006=CARTESIAN_POINT ( 'NONE',  ( -18.62759615963270932, 10.81492255796079327, 85.83224293864768129 ) ) ;
#19007=CARTESIAN_POINT ( 'NONE',  ( -14.34966873604972548, 8.224510206698743886, 68.33442372801900433 ) ) ;
#19009=CARTESIAN_POINT ( 'NONE',  ( 16.51473224551083163, -9.474510206698727899, 35.83442372801899722 ) ) ;
#19010=CARTESIAN_POINT ( 'NONE',  ( -13.97604488694527625, -13.89961937509977652, 66.87390960531436690 ) ) ;
#19011=CARTESIAN_POINT ( 'NONE',  ( 16.53943276465976808, -0.05219959533910856209, 53.74890960531437401 ) ) ;
#19012=CARTESIAN_POINT ( 'NONE',  ( 4.483927247898545687, 16.52544592524342804, 94.79057627198105251 ) ) ;
#19013=CARTESIAN_POINT ( 'NONE',  ( -19.05341960407611168, -5.049401038298163336, 106.4572429386476955 ) ) ;
#19014=CARTESIAN_POINT ( 'NONE',  ( 5.049401038298161559, -19.05341960407611168, 87.70724293864769550 ) ) ;
#19015=CARTESIAN_POINT ( 'NONE',  ( 15.72974639402176855, 15.80617190586768217, 46.87609039468568994 ) ) ;
#19016=CARTESIAN_POINT ( 'NONE',  ( 19.02544592524343514, -5.153800228976328945, 103.5405762719809957 ) ) ;
#19017=CARTESIAN_POINT ( 'NONE',  ( 9.474510206698729675, 16.51473224551082808, 22.08442372801899722 ) ) ;
#19018=CARTESIAN_POINT ( 'NONE',  ( 8.314922557961029526, -14.29746914071037800, 85.41775706135236135 ) ) ;
#19019=CARTESIAN_POINT ( 'NONE',  ( 18.67979575497194134, -10.72451020669871369, 45.83442372801901854 ) ) ;
#19020=CARTESIAN_POINT ( 'NONE',  ( 13.97604488694527802, 13.89961937509977652, 109.3739096053143669 ) ) ;
#19021=CARTESIAN_POINT ( 'NONE',  ( 15.80617190586746368, 15.72974639402197994, 104.3739096053143669 ) ) ;
#19022=CARTESIAN_POINT ( 'NONE',  ( -8.224510206698948167, 14.34966873604960824, 65.41557627198102409 ) ) ;
#19023=CARTESIAN_POINT ( 'NONE',  ( 0.05219959533909260263, 19.03943276465977164, 54.99890960531435979 ) ) ;
#19024=CARTESIAN_POINT ( 'NONE',  ( 4.483927247898545687, 16.52544592524342804, 79.79057627198102409 ) ) ;
#19025=CARTESIAN_POINT ( 'NONE',  ( 0.05219959533907565091, 21.53943276465977519, 29.99890960531435979 ) ) ;
#19026=CARTESIAN_POINT ( 'NONE',  ( 19.05341960407617918, -5.049401038297876454, 46.04275706135233293 ) ) ;
#19027=CARTESIAN_POINT ( 'NONE',  ( 16.52544592524342804, -4.483927247898539470, 113.5405762719810383 ) ) ;
#19029=CARTESIAN_POINT ( 'NONE',  ( -8.314922557961024197, 14.29746914071037800, 62.91775706135236135 ) ) ;
#19030=CARTESIAN_POINT ( 'NONE',  ( 16.46253265017160672, -9.564922557960803928, 73.33224293864769550 ) ) ;
#19032=CARTESIAN_POINT ( 'NONE',  ( -0.05219959533910754901, -16.53943276465976808, 92.49890960531436690 ) ) ;
#19033=CARTESIAN_POINT ( 'NONE',  ( 21.53943276465977519, -0.05219959533907433946, 33.74890960531436690 ) ) ;
#19034=CARTESIAN_POINT ( 'NONE',  ( 4.379528057220092307, 16.55341960407617563, 102.2927570613523613 ) ) ;
#19035=CARTESIAN_POINT ( 'NONE',  ( 16.46253265017146816, 9.564922557961045513, 111.6677570613523329 ) ) ;
#19036=CARTESIAN_POINT ( 'NONE',  ( -21.55341960407619339, 5.719274019375674811, 83.54275706135234714 ) ) ;
#19037=CARTESIAN_POINT ( 'NONE',  ( -9.564922557960796823, -16.46253265017161027, 82.08224293864768129 ) ) ;
#19038=CARTESIAN_POINT ( 'NONE',  ( 21.55341960407610458, 5.719274019375980345, 98.95724293864770971 ) ) ;
#19039=CARTESIAN_POINT ( 'NONE',  ( -4.379528057220086978, -16.55341960407618274, 59.79275706135234714 ) ) ;
#19040=CARTESIAN_POINT ( 'NONE',  ( -19.05341960407611168, -5.049401038298163336, 26.45724293864769550 ) ) ;
#19041=CARTESIAN_POINT ( 'NONE',  ( 8.224510206698742110, 14.34966873604972548, 37.08442372801901143 ) ) ;
#19042=CARTESIAN_POINT ( 'NONE',  ( -16.46253265017146816, -9.564922557961047289, 99.16775706135233293 ) ) ;
#19043=CARTESIAN_POINT ( 'NONE',  ( -21.53943276465977519, 0.05219959533907696930, 86.24890960531436690 ) ) ;
#19044=CARTESIAN_POINT ( 'NONE',  ( -19.05341960407617563, 5.049401038297882671, 58.54275706135234003 ) ) ;
#19045=CARTESIAN_POINT ( 'NONE',  ( 18.39635199886970440, -5.499999999999976019, 88.51967076360000419 ) ) ;
#19046=CARTESIAN_POINT ( 'NONE',  ( -18.67979575497178146, -10.72451020669898902, 106.6655762719810383 ) ) ;
#19048=CARTESIAN_POINT ( 'NONE',  ( 19.03943276465977164, -0.05219959533909143690, 83.74890960531436690 ) ) ;
#19049=CARTESIAN_POINT ( 'NONE',  ( -14.34966873604972548, 8.224510206698743886, 38.33442372801900433 ) ) ;
#19051=CARTESIAN_POINT ( 'NONE',  ( 13.97604488694548053, -13.89961937509957401, 65.62609039468567573 ) ) ;
#19052=CARTESIAN_POINT ( 'NONE',  ( -10.81492255796078084, -18.62759615963271287, 112.0822429386477097 ) ) ;
#19053=CARTESIAN_POINT ( 'NONE',  ( 14.29746914071049879, -8.314922557960816363, 58.33224293864768839 ) ) ;
#19054=CARTESIAN_POINT ( 'NONE',  ( -16.51473224551069308, -9.474510206698971260, 66.66557627198102409 ) ) ;
#19055=CARTESIAN_POINT ( 'NONE',  ( 16.53943276465976808, 0.05219959533934440121, 41.25109039468568284 ) ) ;
#19056=CARTESIAN_POINT ( 'NONE',  ( -9.564922557961040184, 16.46253265017147172, 42.91775706135234003 ) ) ;
#19057=CARTESIAN_POINT ( 'NONE',  ( 21.52544592524334988, 5.823673210054432836, 51.45942372801901854 ) ) ;
#19058=CARTESIAN_POINT ( 'NONE',  ( 13.97604488694548053, -13.89961937509957401, 105.6260903946856757 ) ) ;
#19059=CARTESIAN_POINT ( 'NONE',  ( -0.05219959533909027116, -19.03943276465977164, 57.49890960531435979 ) ) ;
#19060=CARTESIAN_POINT ( 'NONE',  ( -19.05341960407617563, 5.049401038297882671, 83.54275706135233293 ) ) ;
#19061=CARTESIAN_POINT ( 'NONE',  ( -18.67979575497193778, 10.72451020669871902, 88.33442372801901854 ) ) ;
#19062=CARTESIAN_POINT ( 'NONE',  ( 5.049401038297881783, 19.05341960407617563, 72.29275706135234714 ) ) ;
#19063=CARTESIAN_POINT ( 'NONE',  ( -9.474510206698964154, 16.51473224551069663, 30.41557627198102054 ) ) ;
#19064=CARTESIAN_POINT ( 'NONE',  ( 21.53943276465977519, -0.05219959533907433946, 58.74890960531436690 ) ) ;
#19065=CARTESIAN_POINT ( 'NONE',  ( -0.05219959533910754901, -16.53943276465976808, 62.49890960531436690 ) ) ;
#19066=CARTESIAN_POINT ( 'NONE',  ( 19.03943276465977164, 0.05219959533936151252, 66.25109039468567573 ) ) ;
#19067=CARTESIAN_POINT ( 'NONE',  ( -16.21995358207306737, -7.366697692864065949, 25.06448998487843483 ) ) ;
#19068=CARTESIAN_POINT ( 'NONE',  ( 9.564922557961047289, -16.46253265017146816, 30.41775706135232937 ) ) ;
#19069=CARTESIAN_POINT ( 'NONE',  ( 12.06949235617739724, 12.14591786802326823, 91.87609039468568994 ) ) ;
#19070=CARTESIAN_POINT ( 'NONE',  ( 4.379528057220339221, -16.55341960407611168, 47.70724293864770260 ) ) ;
#19071=CARTESIAN_POINT ( 'NONE',  ( 21.53943276465977519, 0.05219959533937863772, 86.25109039468568994 ) ) ;
#19073=CARTESIAN_POINT ( 'NONE',  ( -10.81492255796078084, -18.62759615963271287, 97.08224293864770971 ) ) ;
#19074=CARTESIAN_POINT ( 'NONE',  ( -5.049401038298153566, 19.05341960407611168, 45.20724293864769550 ) ) ;
#19075=CARTESIAN_POINT ( 'NONE',  ( -15.80617190586768217, 15.72974639402176855, 73.12609039468567573 ) ) ;
#19076=CARTESIAN_POINT ( 'NONE',  ( -5.153800228976328057, -19.02544592524343514, 47.29057627198102409 ) ) ;
#19077=CARTESIAN_POINT ( 'NONE',  ( -13.97604488694527625, -13.89961937509977652, 61.87390960531435979 ) ) ;
#19078=CARTESIAN_POINT ( 'NONE',  ( 16.53943276465976808, -0.05219959533910856209, 103.7489096053143669 ) ) ;
#19079=CARTESIAN_POINT ( 'NONE',  ( 19.03943276465977164, -0.05219959533909143690, 113.7489096053143669 ) ) ;
#19080=CARTESIAN_POINT ( 'NONE',  ( -16.55341960407611168, -4.379528057220339221, 51.45724293864770260 ) ) ;
#19081=CARTESIAN_POINT ( 'NONE',  ( 16.46253265017160672, -9.564922557960803928, 28.33224293864769550 ) ) ;
#19082=CARTESIAN_POINT ( 'NONE',  ( -16.55341960407611168, -4.379528057220339221, 86.45724293864770971 ) ) ;
#19083=CARTESIAN_POINT ( 'NONE',  ( 5.823673210054125526, 21.52544592524343514, 94.79057627198105251 ) ) ;
#19084=CARTESIAN_POINT ( 'NONE',  ( -18.62759615963255300, -10.81492255796106328, 39.16775706135235424 ) ) ;
#19086=CARTESIAN_POINT ( 'NONE',  ( -4.379528057220086978, -16.55341960407618274, 34.79275706135235424 ) ) ;
#19087=CARTESIAN_POINT ( 'NONE',  ( -18.62759615963270932, 10.81492255796079327, 85.83224293864768129 ) ) ;
#19088=CARTESIAN_POINT ( 'NONE',  ( 18.62759615963255655, 10.81492255796105972, 106.6677570613523756 ) ) ;
#19089=CARTESIAN_POINT ( 'NONE',  ( 9.564922557960805705, 16.46253265017160317, 99.58224293864770971 ) ) ;
#19090=CARTESIAN_POINT ( 'NONE',  ( -10.72451020669870658, -18.67979575497194134, 39.58442372801901143 ) ) ;
#19091=CARTESIAN_POINT ( 'NONE',  ( -10.81492255796078084, -18.62759615963271287, 27.08224293864769550 ) ) ;
#19092=CARTESIAN_POINT ( 'NONE',  ( -12.14591786802326823, 12.06949235617739902, 103.1260903946856757 ) ) ;
#19093=CARTESIAN_POINT ( 'NONE',  ( 15.72974639402176855, 15.80617190586768217, 56.87609039468568994 ) ) ;
#19094=CARTESIAN_POINT ( 'NONE',  ( -5.719274019375665041, -21.55341960407619695, 89.79275706135236135 ) ) ;
#19095=CARTESIAN_POINT ( 'NONE',  ( 13.89961937509957401, 13.97604488694547697, 26.87609039468566507 ) ) ;
#19096=CARTESIAN_POINT ( 'NONE',  ( 16.52544592524335698, 4.483927247898782831, 86.45942372801901854 ) ) ;
#19097=CARTESIAN_POINT ( 'NONE',  ( -18.62759615963255300, -10.81492255796106328, 44.16775706135234714 ) ) ;
#19098=CARTESIAN_POINT ( 'NONE',  ( 5.049401038298161559, -19.05341960407611168, 47.70724293864770260 ) ) ;
#19099=CARTESIAN_POINT ( 'NONE',  ( -15.80617190586768217, 15.72974639402176855, 98.12609039468570415 ) ) ;
#19100=CARTESIAN_POINT ( 'NONE',  ( 16.51473224551069308, 9.474510206698969483, 109.1655762719810383 ) ) ;
#19101=CARTESIAN_POINT ( 'NONE',  ( -10.72451020669898014, 18.67979575497178502, 105.4155762719810383 ) ) ;
#19102=CARTESIAN_POINT ( 'NONE',  ( 15.72974639402199770, -15.80617190586745480, 63.12390960531435979 ) ) ;
#19104=CARTESIAN_POINT ( 'NONE',  ( -18.62759615963270932, 10.81492255796079327, 65.83224293864769550 ) ) ;
#19105=CARTESIAN_POINT ( 'NONE',  ( 4.379528057220092307, 16.55341960407617563, 57.29275706135234714 ) ) ;
#19106=CARTESIAN_POINT ( 'NONE',  ( -16.55341960407611168, -4.379528057220339221, 66.45724293864768129 ) ) ;
#19108=CARTESIAN_POINT ( 'NONE',  ( -19.02544592524334988, -5.153800228976617603, 88.95942372801897591 ) ) ;
#19110=CARTESIAN_POINT ( 'NONE',  ( 12.14591786802327356, -12.06949235617739191, 20.62609039468568639 ) ) ;
#19111=CARTESIAN_POINT ( 'NONE',  ( -0.05219959533907301413, -21.53943276465977519, 97.49890960531436690 ) ) ;
#19112=CARTESIAN_POINT ( 'NONE',  ( 18.62759615963271287, -10.81492255796078972, 68.33224293864769550 ) ) ;
#19113=CARTESIAN_POINT ( 'NONE',  ( -19.05341960407611168, -5.049401038298163336, 111.4572429386476671 ) ) ;
#19114=CARTESIAN_POINT ( 'NONE',  ( -14.29746914071037622, -8.314922557961029526, 54.16775706135235424 ) ) ;
#19115=CARTESIAN_POINT ( 'NONE',  ( -9.474510206698964154, 16.51473224551069663, 70.41557627198102409 ) ) ;
#19116=CARTESIAN_POINT ( 'NONE',  ( 10.81492255796106328, -18.62759615963255655, 45.41775706135234003 ) ) ;
#19117=CARTESIAN_POINT ( 'NONE',  ( -0.05219959533936034679, 19.03943276465977164, 112.5010903946856757 ) ) ;
#19118=CARTESIAN_POINT ( 'NONE',  ( 5.153800228976335163, 19.02544592524342804, 109.7905762719810099 ) ) ;
#19119=CARTESIAN_POINT ( 'NONE',  ( 13.89961937509977652, -13.97604488694527269, 93.12390960531436690 ) ) ;
#19120=CARTESIAN_POINT ( 'NONE',  ( -21.52544592524343514, 5.823673210054127303, 86.04057627198102409 ) ) ;
#19121=CARTESIAN_POINT ( 'NONE',  ( 13.89961937509977652, -13.97604488694527269, 58.12390960531436690 ) ) ;
#19123=CARTESIAN_POINT ( 'NONE',  ( -8.314922557960811034, -14.29746914071050412, 67.08224293864770971 ) ) ;
#19124=CARTESIAN_POINT ( 'NONE',  ( -0.05219959533907301413, -21.53943276465977519, 22.49890960531436335 ) ) ;
#19126=CARTESIAN_POINT ( 'NONE',  ( 0.05219959533907565091, 21.53943276465977519, 104.9989096053143669 ) ) ;
#19127=CARTESIAN_POINT ( 'NONE',  ( 5.049401038297881783, 19.05341960407617563, 62.29275706135234003 ) ) ;
#19128=CARTESIAN_POINT ( 'NONE',  ( -15.72974639402197994, 15.80617190586746368, 25.62390960531435624 ) ) ;
#19130=CARTESIAN_POINT ( 'NONE',  ( 21.55341960407610458, 5.719274019375980345, 53.95724293864770260 ) ) ;
#19131=CARTESIAN_POINT ( 'NONE',  ( -9.564922557960796823, -16.46253265017161027, 92.08224293864769550 ) ) ;
#19132=CARTESIAN_POINT ( 'NONE',  ( -5.719274019375665041, -21.55341960407619695, 84.79275706135234714 ) ) ;
#19133=CARTESIAN_POINT ( 'NONE',  ( 5.049401038298161559, -19.05341960407611168, 57.70724293864769550 ) ) ;
#19134=CARTESIAN_POINT ( 'NONE',  ( 12.06949235617757843, -12.14591786802309237, 83.12390960531436690 ) ) ;
#19135=CARTESIAN_POINT ( 'NONE',  ( -8.314922557961024197, 14.29746914071037800, 37.91775706135235424 ) ) ;
#19136=CARTESIAN_POINT ( 'NONE',  ( 5.719274019375673035, 21.55341960407619339, 62.29275706135236845 ) ) ;
#19137=ORIENTED_EDGE ( 'NONE', *, *, #154603, .F. ) ;
#19138=CARTESIAN_POINT ( 'NONE',  ( 13.89961937509957401, 13.97604488694547697, 31.87609039468566863 ) ) ;
#19139=CARTESIAN_POINT ( 'NONE',  ( 13.89961937509957401, 13.97604488694547697, 81.87609039468564731 ) ) ;
#19140=EDGE_CURVE ( 'NONE', #101009, #45569, #1689, .T. ) ;
#19141=CARTESIAN_POINT ( 'NONE',  ( 19.03943276465977164, 0.05219959533936151252, 46.25109039468566863 ) ) ;
#19142=FACE_OUTER_BOUND ( 'NONE', #84103, .T. ) ;
#19143=CARTESIAN_POINT ( 'NONE',  ( -10.72451020669870658, -18.67979575497194134, 34.58442372801900433 ) ) ;
#19144=CARTESIAN_POINT ( 'NONE',  ( -19.25918095147781273, -5.499999999999586997, 44.45284276293936188 ) ) ;
#19145=CARTESIAN_POINT ( 'NONE',  ( 16.46253265017146816, 9.564922557961045513, 36.66775706135233293 ) ) ;
#19146=CARTESIAN_POINT ( 'NONE',  ( -5.153800228976328057, -19.02544592524343514, 52.29057627198100988 ) ) ;
#19147=CARTESIAN_POINT ( 'NONE',  ( 5.049401038297881783, 19.05341960407617563, 27.29275706135232937 ) ) ;
#19148=CARTESIAN_POINT ( 'NONE',  ( 4.379528057220092307, 16.55341960407617563, 102.2927570613523613 ) ) ;
#19149=CARTESIAN_POINT ( 'NONE',  ( 0.05219959533909260263, 19.03943276465977164, 109.9989096053143669 ) ) ;
#19150=CARTESIAN_POINT ( 'NONE',  ( 18.67979575497194134, -10.72451020669871369, 85.83442372801901854 ) ) ;
#19154=CARTESIAN_POINT ( 'NONE',  ( -5.823673210054431948, 21.52544592524334988, 82.70942372801900433 ) ) ;
#19156=CARTESIAN_POINT ( 'NONE',  ( 19.05341960407611168, 5.049401038298154454, 103.9572429386476671 ) ) ;
#19158=CARTESIAN_POINT ( 'NONE',  ( 19.02544592524343514, -5.153800228976328945, 48.54057627198103120 ) ) ;
#19159=CARTESIAN_POINT ( 'NONE',  ( 5.823673210054125526, 21.52544592524343514, 49.79057627198102409 ) ) ;
#19160=CARTESIAN_POINT ( 'NONE',  ( 16.55341960407611168, 4.379528057220329451, 28.95724293864769905 ) ) ;
#19161=CARTESIAN_POINT ( 'NONE',  ( 8.314922557960818139, 14.29746914071049879, 99.58224293864770971 ) ) ;
#19162=CARTESIAN_POINT ( 'NONE',  ( 19.03943276465977164, -0.05219959533909143690, 93.74890960531435269 ) ) ;
#19163=CARTESIAN_POINT ( 'NONE',  ( -19.03943276465977164, -0.05219959533935918106, 18.75109039468567218 ) ) ;
#19164=CARTESIAN_POINT ( 'NONE',  ( 9.474510206698971260, -16.51473224551069308, 42.91557627198103120 ) ) ;
#19165=CARTESIAN_POINT ( 'NONE',  ( -8.224510206698948167, 14.34966873604960824, 100.4155762719810241 ) ) ;
#19166=CARTESIAN_POINT ( 'NONE',  ( 18.62759615963255655, 10.81492255796105972, 56.66775706135235424 ) ) ;
#19167=CARTESIAN_POINT ( 'NONE',  ( -14.34966873604972548, 8.224510206698743886, 113.3344237280190328 ) ) ;
#19168=CARTESIAN_POINT ( 'NONE',  ( 0.05219959533936267826, -19.03943276465977164, 70.00109039468566152 ) ) ;
#19170=CARTESIAN_POINT ( 'NONE',  ( 13.97604488694527802, 13.89961937509977652, 109.3739096053143669 ) ) ;
#19171=CARTESIAN_POINT ( 'NONE',  ( -8.314922557960811034, -14.29746914071050412, 77.08224293864769550 ) ) ;
#19172=CARTESIAN_POINT ( 'NONE',  ( 19.02544592524334988, 5.153800228976608722, 56.45942372801898301 ) ) ;
#19173=CARTESIAN_POINT ( 'NONE',  ( 19.03943276465977164, -0.05219959533909143690, 68.74890960531436690 ) ) ;
#19174=VECTOR ( 'NONE', #3909, 1000.000000000000000 ) ;
#19175=CARTESIAN_POINT ( 'NONE',  ( 4.483927247898545687, 16.52544592524342804, 59.79057627198103120 ) ) ;
#19176=CARTESIAN_POINT ( 'NONE',  ( 9.474510206698729675, 16.51473224551082808, 92.08442372801900433 ) ) ;
#19177=CARTESIAN_POINT ( 'NONE',  ( 15.72974639402199770, -15.80617190586745480, 43.12390960531435269 ) ) ;
#19179=CARTESIAN_POINT ( 'NONE',  ( 4.379528057220339221, -16.55341960407611168, 97.70724293864772392 ) ) ;
#19181=CARTESIAN_POINT ( 'NONE',  ( -5.049401038298153566, 19.05341960407611168, 65.20724293864765286 ) ) ;
#19182=CARTESIAN_POINT ( 'NONE',  ( 21.53943276465977519, -0.05219959533907433946, 63.74890960531435979 ) ) ;
#19183=CARTESIAN_POINT ( 'NONE',  ( 0.05219959533909260263, 19.03943276465977164, 39.99890960531436690 ) ) ;
#19184=CARTESIAN_POINT ( 'NONE',  ( 12.06949235617739724, 12.14591786802326823, 96.87609039468568994 ) ) ;
#19185=CARTESIAN_POINT ( 'NONE',  ( -19.05341960407611168, -5.049401038298163336, 76.45724293864769550 ) ) ;
#19186=CARTESIAN_POINT ( 'NONE',  ( 19.03943276465977164, 0.05219959533936151252, 56.25109039468566863 ) ) ;
#19187=CARTESIAN_POINT ( 'NONE',  ( 18.67979575497194134, -10.72451020669871369, 80.83442372801901854 ) ) ;
#19188=CARTESIAN_POINT ( 'NONE',  ( -5.823673210054116645, -21.52544592524344225, 52.29057627198102409 ) ) ;
#19189=CARTESIAN_POINT ( 'NONE',  ( 16.51473224551069308, 9.474510206698969483, 109.1655762719810383 ) ) ;
#19190=CARTESIAN_POINT ( 'NONE',  ( -9.564922557960796823, -16.46253265017161027, 22.08224293864768839 ) ) ;
#19191=CARTESIAN_POINT ( 'NONE',  ( -12.14591786802326823, 12.06949235617739902, 83.12609039468568994 ) ) ;
#19192=CARTESIAN_POINT ( 'NONE',  ( -13.97604488694547697, 13.89961937509957934, 103.1260903946856473 ) ) ;
#19193=CARTESIAN_POINT ( 'NONE',  ( -19.02544592524342804, 5.153800228976336051, 26.04057627198103120 ) ) ;
#19194=CARTESIAN_POINT ( 'NONE',  ( 19.19724070472095789, 5.499999999999972466, 78.56193348274385357 ) ) ;
#19195=CARTESIAN_POINT ( 'NONE',  ( -21.53943276465977519, -0.05219959533937600094, 98.75109039468568994 ) ) ;
#19197=CARTESIAN_POINT ( 'NONE',  ( -12.06949235617756955, 12.14591786802309770, 55.62390960531436690 ) ) ;
#19198=CARTESIAN_POINT ( 'NONE',  ( 8.314922557960818139, 14.29746914071049879, 64.58224293864769550 ) ) ;
#19199=CARTESIAN_POINT ( 'NONE',  ( 21.55341960407610458, 5.719274019375980345, 98.95724293864770971 ) ) ;
#19200=CARTESIAN_POINT ( 'NONE',  ( 0.05219959533907565091, 21.53943276465977519, 94.99890960531436690 ) ) ;
#19202=CARTESIAN_POINT ( 'NONE',  ( 15.80617190586746368, 15.72974639402197994, 29.37390960531435269 ) ) ;
#19203=CARTESIAN_POINT ( 'NONE',  ( -4.483927247898782831, 16.52544592524335698, 67.70942372801901854 ) ) ;
#19204=CARTESIAN_POINT ( 'NONE',  ( -12.06949235617756955, 12.14591786802309770, 95.62390960531436690 ) ) ;
#19205=CARTESIAN_POINT ( 'NONE',  ( 19.05341960407611168, 5.049401038298154454, 48.95724293864768129 ) ) ;
#19207=CARTESIAN_POINT ( 'NONE',  ( -8.224510206698735004, -14.34966873604973081, 89.58442372801901854 ) ) ;
#19208=CARTESIAN_POINT ( 'NONE',  ( 15.72974639402176855, 15.80617190586768217, 36.87609039468568994 ) ) ;
#19209=CARTESIAN_POINT ( 'NONE',  ( 0.05219959533909260263, 19.03943276465977164, 79.99890960531436690 ) ) ;
#19210=CARTESIAN_POINT ( 'NONE',  ( 10.81492255796106328, -18.62759615963255655, 65.41775706135234714 ) ) ;
#19211=CARTESIAN_POINT ( 'NONE',  ( -17.49999999999999289, 5.500000000000037303, 80.79690382534172954 ) ) ;
#19214=CARTESIAN_POINT ( 'NONE',  ( -21.55341960407619339, 5.719274019375674811, 53.54275706135234714 ) ) ;
#19215=CARTESIAN_POINT ( 'NONE',  ( 13.89961937509977652, -13.97604488694527269, 43.12390960531434558 ) ) ;
#19216=CARTESIAN_POINT ( 'NONE',  ( 17.50000000001358202, -5.500000000000038192, 58.29690382535058291 ) ) ;
#19217=CARTESIAN_POINT ( 'NONE',  ( -9.564922557960796823, -16.46253265017161027, 87.08224293864769550 ) ) ;
#19218=CARTESIAN_POINT ( 'NONE',  ( 19.02544592524334988, 5.153800228976608722, 61.45942372801900433 ) ) ;
#19219=CARTESIAN_POINT ( 'NONE',  ( -5.719274019375665041, -21.55341960407619695, 34.79275706135235424 ) ) ;
#19220=CARTESIAN_POINT ( 'NONE',  ( -9.564922557961040184, 16.46253265017147172, 57.91775706135233293 ) ) ;
#19221=CARTESIAN_POINT ( 'NONE',  ( 16.46253265017160672, -9.564922557960803928, 23.33224293864769194 ) ) ;
#19222=CARTESIAN_POINT ( 'NONE',  ( -0.05219959533934338120, 16.53943276465976808, 107.5010903946856899 ) ) ;
#19223=CARTESIAN_POINT ( 'NONE',  ( -13.97604488694547697, 13.89961937509957934, 68.12609039468563310 ) ) ;
#19224=CARTESIAN_POINT ( 'NONE',  ( -12.06949235617756955, 12.14591786802309770, 25.62390960531435624 ) ) ;
#19225=CARTESIAN_POINT ( 'NONE',  ( -19.03943276465977164, -0.05219959533935918106, 48.75109039468566863 ) ) ;
#19227=CARTESIAN_POINT ( 'NONE',  ( 19.05341960407611168, 5.049401038298154454, 88.95724293864769550 ) ) ;
#19228=CARTESIAN_POINT ( 'NONE',  ( 21.55341960407619695, -5.719274019375665929, 96.04275706135236135 ) ) ;
#19229=CARTESIAN_POINT ( 'NONE',  ( -15.80617190586768217, 15.72974639402176855, 103.1260903946856757 ) ) ;
#19231=CARTESIAN_POINT ( 'NONE',  ( 5.719274019375673035, 21.55341960407619339, 92.29275706135236135 ) ) ;
#19232=CARTESIAN_POINT ( 'NONE',  ( -16.53943276465976808, -0.05219959533934237506, 28.75109039468567929 ) ) ;
#19234=CARTESIAN_POINT ( 'NONE',  ( 9.474510206698971260, -16.51473224551069308, 97.91557627198102409 ) ) ;
#19235=CARTESIAN_POINT ( 'NONE',  ( 21.55341960407610458, 5.719274019375980345, 23.95724293864769550 ) ) ;
#19237=CARTESIAN_POINT ( 'NONE',  ( 19.03943276465977164, -0.05219959533909143690, 83.74890960531436690 ) ) ;
#19238=CARTESIAN_POINT ( 'NONE',  ( -16.18388926212247725, 7.379444403734496838, 99.56046848633765478 ) ) ;
#19239=CARTESIAN_POINT ( 'NONE',  ( -19.05341960407617563, 5.049401038297882671, 68.54275706135230450 ) ) ;
#19240=B_SPLINE_CURVE_WITH_KNOTS ( 'NONE', 3,
 ( #87520, #89514, #72362, #134036, #195729, #45004, #103699, #135047, #58191, #57202, #181544, #74358, #43022, #136024, #152181, #167361, #28859, #90499, #173315, #33799, #65123, #122818, #34790, #169320, #186514, #45988, #107643, #3447, #93468, #155155, #124814, #156144 ),
 .UNSPECIFIED., .F., .F.,
 ( 4, 2, 2, 2, 2, 2, 2, 2, 2, 2, 2, 2, 2, 2, 2, 4 ),
 ( 2.969368287472575283E-17, 0.0003712461730036979452, 0.0007424923460073661833, 0.001113738519011034421, 0.001484984692014702659, 0.002227477038022038919, 0.002598723211025717565, 0.002969969384029395778, 0.003341215557033074424, 0.003712461730036753071, 0.004083707903040432151, 0.004454954076044110797, 0.004826200249047790311, 0.005197446422051468957, 0.005568692595055147604, 0.005939938768058825383 ),
 .UNSPECIFIED. ) ;
#19241=CARTESIAN_POINT ( 'NONE',  ( 5.049401038298161559, -19.05341960407611168, 112.7072429386476813 ) ) ;
#19242=CARTESIAN_POINT ( 'NONE',  ( 0.05219959533937995610, -21.53943276465977519, 105.0010903946856757 ) ) ;
#19243=CARTESIAN_POINT ( 'NONE',  ( -4.379528057220328563, 16.55341960407611168, 95.20724293864769550 ) ) ;
#19244=CARTESIAN_POINT ( 'NONE',  ( -10.72451020669898014, 18.67979575497178502, 40.41557627198103120 ) ) ;
#19245=CARTESIAN_POINT ( 'NONE',  ( 21.52544592524344225, -5.823673210054117533, 38.54057627198103120 ) ) ;
#19246=CARTESIAN_POINT ( 'NONE',  ( -14.34966873604960291, -8.224510206698953496, 111.6655762719810525 ) ) ;
#19248=CARTESIAN_POINT ( 'NONE',  ( 13.97604488694548053, -13.89961937509957401, 55.62609039468566863 ) ) ;
#19249=CARTESIAN_POINT ( 'NONE',  ( -12.14591786802309592, -12.06949235617757132, 26.87390960531435979 ) ) ;
#19250=CARTESIAN_POINT ( 'NONE',  ( -19.02544592524342804, 5.153800228976336051, 101.0405762719810241 ) ) ;
#19251=CARTESIAN_POINT ( 'NONE',  ( 10.81492255796106328, -18.62759615963255655, 80.41775706135234714 ) ) ;
#19252=CARTESIAN_POINT ( 'NONE',  ( -15.80617190586745835, -15.72974639402198527, 66.87390960531436690 ) ) ;
#19253=CARTESIAN_POINT ( 'NONE',  ( -18.62759615963255300, -10.81492255796106328, 39.16775706135235424 ) ) ;
#19254=CARTESIAN_POINT ( 'NONE',  ( 21.53943276465977519, -0.05219959533907433946, 98.74890960531438111 ) ) ;
#19255=CARTESIAN_POINT ( 'NONE',  ( -10.72451020669870658, -18.67979575497194134, 54.58442372801901143 ) ) ;
#19256=CARTESIAN_POINT ( 'NONE',  ( -5.153800228976328057, -19.02544592524343514, 22.29057627198102765 ) ) ;
#19257=EDGE_CURVE ( 'NONE', #137960, #94779, #107170, .T. ) ;
#19258=CARTESIAN_POINT ( 'NONE',  ( 19.05341960407611168, 5.049401038298154454, 78.95724293864769550 ) ) ;
#19259=CARTESIAN_POINT ( 'NONE',  ( -0.05219959533934338120, 16.53943276465976808, 77.50109039468567573 ) ) ;
#19260=CARTESIAN_POINT ( 'NONE',  ( -12.06949235617756955, 12.14591786802309770, 105.6239096053143669 ) ) ;
#19261=CARTESIAN_POINT ( 'NONE',  ( -9.564922557960796823, -16.46253265017161027, 102.0822429386477097 ) ) ;
#19262=CARTESIAN_POINT ( 'NONE',  ( 12.14591786802309770, 12.06949235617756955, 59.37390960531436690 ) ) ;
#19263=CARTESIAN_POINT ( 'NONE',  ( -16.52544592524342804, 4.483927247898546575, 26.04057627198103475 ) ) ;
#19264=CARTESIAN_POINT ( 'NONE',  ( -19.05341960407611168, -5.049401038298163336, 56.45724293864768129 ) ) ;
#19265=CARTESIAN_POINT ( 'NONE',  ( -16.46253265017160317, 9.564922557960807481, 40.83224293864769550 ) ) ;
#19266=CARTESIAN_POINT ( 'NONE',  ( -15.72974639402197994, 15.80617190586746368, 50.62390960531435979 ) ) ;
#19267=CARTESIAN_POINT ( 'NONE',  ( -9.564922557961040184, 16.46253265017147172, 22.91775706135233648 ) ) ;
#19268=CARTESIAN_POINT ( 'NONE',  ( 18.22780087662126647, 5.499999999999818812, 51.48236817873107896 ) ) ;
#19269=CARTESIAN_POINT ( 'NONE',  ( -8.314922557960811034, -14.29746914071050412, 42.08224293864769550 ) ) ;
#19270=CARTESIAN_POINT ( 'NONE',  ( 18.62759615963255655, 10.81492255796105972, 46.66775706135234714 ) ) ;
#19271=FACE_OUTER_BOUND ( 'NONE', #79322, .T. ) ;
#19272=CARTESIAN_POINT ( 'NONE',  ( 0.05219959533934541429, -16.53943276465976808, 65.00109039468568994 ) ) ;
#19273=CARTESIAN_POINT ( 'NONE',  ( 16.46253265017146816, 9.564922557961045513, 61.66775706135234003 ) ) ;
#19274=CARTESIAN_POINT ( 'NONE',  ( 8.314922557960818139, 14.29746914071049879, 29.58224293864769905 ) ) ;
#19275=CARTESIAN_POINT ( 'NONE',  ( 4.379528057220092307, 16.55341960407617563, 102.2927570613523613 ) ) ;
#19276=CARTESIAN_POINT ( 'NONE',  ( -5.049401038298153566, 19.05341960407611168, 35.20724293864768839 ) ) ;
#19277=CARTESIAN_POINT ( 'NONE',  ( -5.153800228976328057, -19.02544592524343514, 67.29057627198102409 ) ) ;
#19278=CARTESIAN_POINT ( 'NONE',  ( -19.02544592524342804, 5.153800228976336051, 26.04057627198103120 ) ) ;
#19279=CARTESIAN_POINT ( 'NONE',  ( 21.55341960407619695, -5.719274019375665929, 31.04275706135234714 ) ) ;
#19280=CARTESIAN_POINT ( 'NONE',  ( 5.153800228976335163, 19.02544592524342804, 39.79057627198100988 ) ) ;
#19282=CARTESIAN_POINT ( 'NONE',  ( 5.049401038298161559, -19.05341960407611168, 42.70724293864767418 ) ) ;
#19283=CARTESIAN_POINT ( 'NONE',  ( 5.049401038298161559, -19.05341960407611168, 112.7072429386476813 ) ) ;
#19285=CARTESIAN_POINT ( 'NONE',  ( -5.823673210054431948, 21.52544592524334988, 57.70942372801901143 ) ) ;
#19286=CARTESIAN_POINT ( 'NONE',  ( 0.05219959533910956823, 16.53943276465976808, 104.9989096053143669 ) ) ;
#19287=CARTESIAN_POINT ( 'NONE',  ( 13.89961937509977652, -13.97604488694527269, 113.1239096053143527 ) ) ;
#19288=CARTESIAN_POINT ( 'NONE',  ( 12.06949235617739724, 12.14591786802326823, 81.87609039468568994 ) ) ;
#19289=CARTESIAN_POINT ( 'NONE',  ( 5.719274019375673035, 21.55341960407619339, 92.29275706135236135 ) ) ;
#19290=CARTESIAN_POINT ( 'NONE',  ( -16.52544592524335698, -4.483927247898792601, 48.95942372801902565 ) ) ;
#19291=CARTESIAN_POINT ( 'NONE',  ( -19.03943276465977164, 0.05219959533909376836, 96.24890960531436690 ) ) ;
#19292=CARTESIAN_POINT ( 'NONE',  ( -8.224510206698735004, -14.34966873604973081, 39.58442372801901143 ) ) ;
#19293=CARTESIAN_POINT ( 'NONE',  ( -0.05219959533934338120, 16.53943276465976808, 27.50109039468567929 ) ) ;
#19294=CARTESIAN_POINT ( 'NONE',  ( -14.34966873604972548, 8.224510206698743886, 98.33442372801901854 ) ) ;
#19295=CARTESIAN_POINT ( 'NONE',  ( 9.474510206698729675, 16.51473224551082808, 107.0844237280190043 ) ) ;
#19296=CARTESIAN_POINT ( 'NONE',  ( -5.823673210054116645, -21.52544592524344225, 102.2905762719810383 ) ) ;
#19297=CARTESIAN_POINT ( 'NONE',  ( -14.34966873604960291, -8.224510206698953496, 101.6655762719810383 ) ) ;
#19298=CARTESIAN_POINT ( 'NONE',  ( 9.564922557961047289, -16.46253265017146816, 100.4177570613523329 ) ) ;
#19299=CARTESIAN_POINT ( 'NONE',  ( -16.55341960407617563, 4.379528057220093196, 68.54275706135234714 ) ) ;
#19301=CARTESIAN_POINT ( 'NONE',  ( 19.05341960407617918, -5.049401038297876454, 66.04275706135233293 ) ) ;
#19302=CARTESIAN_POINT ( 'NONE',  ( -16.53943276465976808, 0.05219959533911058130, 51.24890960531436690 ) ) ;
#19303=CARTESIAN_POINT ( 'NONE',  ( 14.34966873604960469, 8.224510206698951720, 49.16557627198102409 ) ) ;
#19304=CARTESIAN_POINT ( 'NONE',  ( -16.52544592524342804, 4.483927247898546575, 96.04057627198102409 ) ) ;
#19305=CARTESIAN_POINT ( 'NONE',  ( -16.51473224551082808, 9.474510206698731452, 28.33442372801900433 ) ) ;
#19306=CARTESIAN_POINT ( 'NONE',  ( -16.61371651742601330, 7.165104196376141488, 88.85415069993000259 ) ) ;
#19307=CARTESIAN_POINT ( 'NONE',  ( 15.72974639402176855, 15.80617190586768217, 36.87609039468568994 ) ) ;
#19308=CARTESIAN_POINT ( 'NONE',  ( -19.03943276465977164, -0.05219959533935918106, 93.75109039468566152 ) ) ;
#19310=CARTESIAN_POINT ( 'NONE',  ( -5.049401038298153566, 19.05341960407611168, 95.20724293864770971 ) ) ;
#19311=CARTESIAN_POINT ( 'NONE',  ( -0.05219959533909027116, -19.03943276465977164, 92.49890960531436690 ) ) ;
#19312=CARTESIAN_POINT ( 'NONE',  ( -18.62759615963270932, 10.81492255796079327, 60.83224293864769550 ) ) ;
#19313=CARTESIAN_POINT ( 'NONE',  ( 16.53943276465976808, -0.05219959533910856209, 88.74890960531436690 ) ) ;
#19314=CARTESIAN_POINT ( 'NONE',  ( -19.02544592524342804, 5.153800228976336051, 76.04057627198102409 ) ) ;
#19315=CARTESIAN_POINT ( 'NONE',  ( 16.46253265017160672, -9.564922557960803928, 33.33224293864770260 ) ) ;
#19316=CARTESIAN_POINT ( 'NONE',  ( 15.80617190586769283, -15.72974639402175789, 40.62609039468567573 ) ) ;
#19318=CARTESIAN_POINT ( 'NONE',  ( -18.62759615963255300, -10.81492255796106328, 79.16775706135234714 ) ) ;
#19319=CARTESIAN_POINT ( 'NONE',  ( -19.02544592524342804, 5.153800228976336051, 61.04057627198103120 ) ) ;
#19320=CARTESIAN_POINT ( 'NONE',  ( 12.06949235617739724, 12.14591786802326823, 81.87609039468568994 ) ) ;
#19321=CARTESIAN_POINT ( 'NONE',  ( 18.67979575497194134, -10.72451020669871369, 35.83442372801901143 ) ) ;
#19322=CARTESIAN_POINT ( 'NONE',  ( -15.80617190586768217, 15.72974639402176855, 28.12609039468568284 ) ) ;
#19323=CARTESIAN_POINT ( 'NONE',  ( -19.03943276465977164, -0.05219959533935918106, 48.75109039468566863 ) ) ;
#19324=CARTESIAN_POINT ( 'NONE',  ( 13.97604488694527802, 13.89961937509977652, 79.37390960531435269 ) ) ;
#19325=CARTESIAN_POINT ( 'NONE',  ( -5.049401038297874678, -19.05341960407617918, 29.79275706135232227 ) ) ;
#19326=CARTESIAN_POINT ( 'NONE',  ( -10.81492255796105439, 18.62759615963255655, 87.91775706135234714 ) ) ;
#19327=CARTESIAN_POINT ( 'NONE',  ( -21.52544592524343514, 5.823673210054127303, 71.04057627198103830 ) ) ;
#19328=CARTESIAN_POINT ( 'NONE',  ( -4.483927247898539470, -16.52544592524342804, 57.29057627198103120 ) ) ;
#19329=CARTESIAN_POINT ( 'NONE',  ( -0.05219959533937732626, 21.53943276465977519, 87.50109039468568994 ) ) ;
#19330=CARTESIAN_POINT ( 'NONE',  ( -9.474510206698720793, -16.51473224551083518, 29.58442372801900433 ) ) ;
#19331=CARTESIAN_POINT ( 'NONE',  ( 16.55341960407611168, 4.379528057220329451, 68.95724293864769550 ) ) ;
#19332=CARTESIAN_POINT ( 'NONE',  ( 16.51473224551069308, 9.474510206698969483, 24.16557627198102765 ) ) ;
#19333=CARTESIAN_POINT ( 'NONE',  ( 16.46253265017146816, 9.564922557961045513, 66.66775706135233293 ) ) ;
#19334=CARTESIAN_POINT ( 'NONE',  ( 4.379528057220339221, -16.55341960407611168, 32.70724293864770260 ) ) ;
#19335=CARTESIAN_POINT ( 'NONE',  ( -21.55341960407619339, 5.719274019375674811, 83.54275706135234714 ) ) ;
#19337=CARTESIAN_POINT ( 'NONE',  ( 16.51473224551069308, 9.474510206698969483, 74.16557627198103830 ) ) ;
#19338=CARTESIAN_POINT ( 'NONE',  ( 19.02544592524334988, 5.153800228976608722, 41.45942372801900433 ) ) ;
#19339=CARTESIAN_POINT ( 'NONE',  ( 15.80617190586746368, 15.72974639402197994, 54.37390960531435979 ) ) ;
#19340=CARTESIAN_POINT ( 'NONE',  ( 15.72974639402176855, 15.80617190586768217, 21.87609039468567573 ) ) ;
#19341=CARTESIAN_POINT ( 'NONE',  ( -16.51473224551082808, 9.474510206698731452, 108.3344237280190043 ) ) ;
#19342=CARTESIAN_POINT ( 'NONE',  ( -12.14591786802326823, 12.06949235617739902, 68.12609039468567573 ) ) ;
#19343=CARTESIAN_POINT ( 'NONE',  ( 10.72451020669898902, -18.67979575497178502, 102.9155762719810383 ) ) ;
#19344=CARTESIAN_POINT ( 'NONE',  ( 14.29746914071049879, -8.314922557960816363, 108.3322429386477097 ) ) ;
#19345=CARTESIAN_POINT ( 'NONE',  ( -17.50000000000149569, -3.202012800152222560, 30.07177583972730517 ) ) ;
#19346=CARTESIAN_POINT ( 'NONE',  ( 4.483927247898790824, -16.52544592524335698, 35.20942372801901854 ) ) ;
#19347=CARTESIAN_POINT ( 'NONE',  ( -15.72974639402197994, 15.80617190586746368, 65.62390960531436690 ) ) ;
#19348=CARTESIAN_POINT ( 'NONE',  ( 16.52544592524335698, 4.483927247898782831, 101.4594237280190185 ) ) ;
#19349=CARTESIAN_POINT ( 'NONE',  ( -16.51473224551069308, -9.474510206698971260, 31.66557627198102054 ) ) ;
#19350=CARTESIAN_POINT ( 'NONE',  ( 14.34966873604972726, -8.224510206698740333, 65.83442372801900433 ) ) ;
#19351=CARTESIAN_POINT ( 'NONE',  ( -5.049401038297874678, -19.05341960407617918, 64.79275706135233293 ) ) ;
#19352=CARTESIAN_POINT ( 'NONE',  ( 15.80617190586769283, -15.72974639402175789, 40.62609039468567573 ) ) ;
#19353=CARTESIAN_POINT ( 'NONE',  ( 15.80617190586746368, 15.72974639402197994, 64.37390960531435269 ) ) ;
#19354=CARTESIAN_POINT ( 'NONE',  ( -0.05219959533934338120, 16.53943276465976808, 97.50109039468567573 ) ) ;
#19355=CARTESIAN_POINT ( 'NONE',  ( 18.62759615963255655, 10.81492255796105972, 81.66775706135236135 ) ) ;
#19356=CARTESIAN_POINT ( 'NONE',  ( -18.62759615963270932, 10.81492255796079327, 50.83224293864770971 ) ) ;
#19357=CARTESIAN_POINT ( 'NONE',  ( 10.81492255796078972, 18.62759615963270932, 29.58224293864769905 ) ) ;
#19358=CARTESIAN_POINT ( 'NONE',  ( 0.05219959533934541429, -16.53943276465976808, 75.00109039468568994 ) ) ;
#19359=CARTESIAN_POINT ( 'NONE',  ( -21.52544592524343514, 5.823673210054127303, 41.04057627198103120 ) ) ;
#19360=ORIENTED_EDGE ( 'NONE', *, *, #9292, .F. ) ;
#19361=CARTESIAN_POINT ( 'NONE',  ( 5.049401038298161559, -19.05341960407611168, 102.7072429386476955 ) ) ;
#19363=CARTESIAN_POINT ( 'NONE',  ( -16.51473224551069308, -9.474510206698971260, 26.66557627198103120 ) ) ;
#19364=CARTESIAN_POINT ( 'NONE',  ( -15.80617190586745835, -15.72974639402198527, 61.87390960531436690 ) ) ;
#19365=CARTESIAN_POINT ( 'NONE',  ( -0.05219959533934338120, 16.53943276465976808, 92.50109039468567573 ) ) ;
#19366=CARTESIAN_POINT ( 'NONE',  ( -21.52544592524334988, -5.823673210054445271, 43.95942372801902565 ) ) ;
#19367=CARTESIAN_POINT ( 'NONE',  ( -9.564922557961040184, 16.46253265017147172, 107.9177570613523471 ) ) ;
#19368=CARTESIAN_POINT ( 'NONE',  ( 12.14591786802309770, 12.06949235617756955, 99.37390960531436690 ) ) ;
#19369=CARTESIAN_POINT ( 'NONE',  ( 14.34966873604972726, -8.224510206698740333, 20.83442372801901143 ) ) ;
#19370=CARTESIAN_POINT ( 'NONE',  ( -19.03943276465977164, 0.05219959533909376836, 41.24890960531435269 ) ) ;
#19371=CARTESIAN_POINT ( 'NONE',  ( 18.22780087662123805, -5.499999999999989342, 63.51763182126896368 ) ) ;
#19372=CARTESIAN_POINT ( 'NONE',  ( -16.46253265017160317, 9.564922557960807481, 90.83224293864769550 ) ) ;
#19373=CARTESIAN_POINT ( 'NONE',  ( -12.14591786802326823, 12.06949235617739902, 73.12609039468567573 ) ) ;
#19374=CARTESIAN_POINT ( 'NONE',  ( 21.55341960407619695, -5.719274019375665929, 106.0427570613523471 ) ) ;
#19375=CARTESIAN_POINT ( 'NONE',  ( -0.05219959533907301413, -21.53943276465977519, 57.49890960531435979 ) ) ;
#19376=CARTESIAN_POINT ( 'NONE',  ( -4.483927247898782831, 16.52544592524335698, 87.70942372801901854 ) ) ;
#19377=CARTESIAN_POINT ( 'NONE',  ( 5.153800228976615827, -19.02544592524334988, 75.20942372801896170 ) ) ;
#19378=CARTESIAN_POINT ( 'NONE',  ( -16.51473224551069308, -9.474510206698971260, 41.66557627198103120 ) ) ;
#19379=CARTESIAN_POINT ( 'NONE',  ( -9.564922557960796823, -16.46253265017161027, 77.08224293864769550 ) ) ;
#19380=CARTESIAN_POINT ( 'NONE',  ( 19.02544592524343514, -5.153800228976328945, 38.54057627198103120 ) ) ;
#19381=CARTESIAN_POINT ( 'NONE',  ( 19.05341960407617918, -5.049401038297876454, 76.04275706135230450 ) ) ;
#19383=CARTESIAN_POINT ( 'NONE',  ( -0.05219959533909027116, -19.03943276465977164, 97.49890960531436690 ) ) ;
#19384=CARTESIAN_POINT ( 'NONE',  ( -8.314922557960811034, -14.29746914071050412, 52.08224293864768839 ) ) ;
#19385=CARTESIAN_POINT ( 'NONE',  ( 18.62759615963271287, -10.81492255796078972, 58.33224293864768839 ) ) ;
#19386=CARTESIAN_POINT ( 'NONE',  ( -17.49999999999998934, 3.805241302050261343, 105.3735247278259237 ) ) ;
#19387=CARTESIAN_POINT ( 'NONE',  ( 0.05219959533936267826, -19.03943276465977164, 35.00109039468566863 ) ) ;
#19389=CARTESIAN_POINT ( 'NONE',  ( 9.474510206698971260, -16.51473224551069308, 57.91557627198103120 ) ) ;
#19390=CARTESIAN_POINT ( 'NONE',  ( -13.89961937509977652, 13.97604488694528158, 75.62390960531438111 ) ) ;
#19391=CARTESIAN_POINT ( 'NONE',  ( -14.34966873604972548, 8.224510206698743886, 43.33442372801901143 ) ) ;
#19393=CARTESIAN_POINT ( 'NONE',  ( -16.29526858892874941, 7.335722546920128373, 109.2032940219979622 ) ) ;
#19394=CARTESIAN_POINT ( 'NONE',  ( -8.224510206698735004, -14.34966873604973081, 79.58442372801903275 ) ) ;
#19395=CARTESIAN_POINT ( 'NONE',  ( 4.379528057220092307, 16.55341960407617563, 67.29275706135234714 ) ) ;
#19396=CARTESIAN_POINT ( 'NONE',  ( -21.52544592524343514, 5.823673210054127303, 101.0405762719810383 ) ) ;
#19397=CARTESIAN_POINT ( 'NONE',  ( 16.55341960407618274, -4.379528057220086978, 46.04275706135234714 ) ) ;
#19398=CARTESIAN_POINT ( 'NONE',  ( -19.03943276465977164, 0.05219959533909376836, 46.24890960531435979 ) ) ;
#19400=CARTESIAN_POINT ( 'NONE',  ( -10.72451020669870658, -18.67979575497194134, 49.58442372801901143 ) ) ;
#19401=CARTESIAN_POINT ( 'NONE',  ( -0.05219959533936034679, 19.03943276465977164, 62.50109039468566863 ) ) ;
#19402=CARTESIAN_POINT ( 'NONE',  ( 10.72451020669871369, 18.67979575497193778, 92.08442372801901854 ) ) ;
#19403=CARTESIAN_POINT ( 'NONE',  ( -5.049401038298153566, 19.05341960407611168, 35.20724293864768839 ) ) ;
#19404=CARTESIAN_POINT ( 'NONE',  ( 18.87255363501902039, 5.499999999999939604, 43.82513748171827928 ) ) ;
#19405=CARTESIAN_POINT ( 'NONE',  ( -18.67979575497178146, -10.72451020669898902, 51.66557627198102409 ) ) ;
#19406=CARTESIAN_POINT ( 'NONE',  ( -16.46253265017160317, 9.564922557960807481, 100.8322429386477097 ) ) ;
#19407=CARTESIAN_POINT ( 'NONE',  ( -16.55341960407611168, -4.379528057220339221, 101.4572429386476955 ) ) ;
#19408=CARTESIAN_POINT ( 'NONE',  ( 16.52544592524335698, 4.483927247898782831, 41.45942372801901143 ) ) ;
#19409=CARTESIAN_POINT ( 'NONE',  ( 8.314922557961029526, -14.29746914071037800, 110.4177570613523756 ) ) ;
#19411=CARTESIAN_POINT ( 'NONE',  ( -21.55341960407610458, -5.719274019375992779, 106.4572429386477097 ) ) ;
#19412=CARTESIAN_POINT ( 'NONE',  ( 14.29746914071049879, -8.314922557960816363, 43.33224293864769550 ) ) ;
#19413=FACE_OUTER_BOUND ( 'NONE', #174506, .T. ) ;
#19414=CARTESIAN_POINT ( 'NONE',  ( 0.05219959533936267826, -19.03943276465977164, 100.0010903946856757 ) ) ;
#19415=CARTESIAN_POINT ( 'NONE',  ( -9.474510206698720793, -16.51473224551083518, 29.58442372801900433 ) ) ;
#19416=CARTESIAN_POINT ( 'NONE',  ( 0.05219959533910956823, 16.53943276465976808, 24.99890960531435624 ) ) ;
#19417=CARTESIAN_POINT ( 'NONE',  ( -15.80617190586745835, -15.72974639402198527, 86.87390960531438111 ) ) ;
#19418=CARTESIAN_POINT ( 'NONE',  ( -21.53943276465977519, 0.05219959533907696930, 51.24890960531436690 ) ) ;
#19419=CARTESIAN_POINT ( 'NONE',  ( 0.05219959533909260263, 19.03943276465977164, 69.99890960531435269 ) ) ;
#19420=CARTESIAN_POINT ( 'NONE',  ( -16.52544592524342804, 4.483927247898546575, 41.04057627198103120 ) ) ;
#19421=CARTESIAN_POINT ( 'NONE',  ( -13.89961937509977652, 13.97604488694528158, 85.62390960531433848 ) ) ;
#19424=CARTESIAN_POINT ( 'NONE',  ( 19.02544592524334988, 5.153800228976608722, 46.45942372801899012 ) ) ;
#19425=CARTESIAN_POINT ( 'NONE',  ( -5.823673210054116645, -21.52544592524344225, 87.29057627198103830 ) ) ;
#19426=CARTESIAN_POINT ( 'NONE',  ( -16.52544592524342804, 4.483927247898546575, 101.0405762719810383 ) ) ;
#19427=CARTESIAN_POINT ( 'NONE',  ( 5.823673210054444382, -21.52544592524334988, 40.20942372801901854 ) ) ;
#19429=CARTESIAN_POINT ( 'NONE',  ( 14.29746914071037800, 8.314922557961029526, 101.6677570613523613 ) ) ;
#19430=CARTESIAN_POINT ( 'NONE',  ( -19.03943276465977164, 0.05219959533909376836, 41.24890960531435269 ) ) ;
#19431=CARTESIAN_POINT ( 'NONE',  ( 19.05341960407611168, 5.049401038298154454, 88.95724293864769550 ) ) ;
#19433=CARTESIAN_POINT ( 'NONE',  ( -16.46253265017160317, 9.564922557960807481, 35.83224293864768839 ) ) ;
#19434=CARTESIAN_POINT ( 'NONE',  ( -4.483927247898539470, -16.52544592524342804, 42.29057627198103120 ) ) ;
#19435=CARTESIAN_POINT ( 'NONE',  ( 15.72974639402176855, 15.80617190586768217, 71.87609039468568994 ) ) ;
#19437=CARTESIAN_POINT ( 'NONE',  ( 4.483927247898790824, -16.52544592524335698, 75.20942372801901854 ) ) ;
#19438=CARTESIAN_POINT ( 'NONE',  ( 9.474510206698971260, -16.51473224551069308, 62.91557627198102409 ) ) ;
#19439=CARTESIAN_POINT ( 'NONE',  ( -9.564922557960796823, -16.46253265017161027, 62.08224293864769550 ) ) ;
#19441=CARTESIAN_POINT ( 'NONE',  ( 15.72974639402176855, 15.80617190586768217, 101.8760903946857042 ) ) ;
#19442=CARTESIAN_POINT ( 'NONE',  ( -14.29746914071037622, -8.314922557961029526, 79.16775706135234714 ) ) ;
#19443=CARTESIAN_POINT ( 'NONE',  ( -15.80617190586768217, 15.72974639402176855, 98.12609039468570415 ) ) ;
#19444=CARTESIAN_POINT ( 'NONE',  ( 9.564922557960805705, 16.46253265017160317, 64.58224293864769550 ) ) ;
#19445=CARTESIAN_POINT ( 'NONE',  ( -15.72974639402197994, 15.80617190586746368, 40.62390960531435269 ) ) ;
#19446=CARTESIAN_POINT ( 'NONE',  ( 5.049401038297881783, 19.05341960407617563, 112.2927570613523471 ) ) ;
#19447=CARTESIAN_POINT ( 'NONE',  ( -21.53943276465977519, -0.05219959533937600094, 73.75109039468567573 ) ) ;
#19448=CARTESIAN_POINT ( 'NONE',  ( 4.483927247898790824, -16.52544592524335698, 50.20942372801901854 ) ) ;
#19449=CARTESIAN_POINT ( 'NONE',  ( -21.52544592524343514, 5.823673210054127303, 96.04057627198102409 ) ) ;
#19450=CARTESIAN_POINT ( 'NONE',  ( 16.46253265017146816, 9.564922557961045513, 101.6677570613523329 ) ) ;
#19451=CARTESIAN_POINT ( 'NONE',  ( -16.46253265017160317, 9.564922557960807481, 75.83224293864769550 ) ) ;
#19452=CARTESIAN_POINT ( 'NONE',  ( -19.03943276465977164, -0.05219959533935918106, 103.7510903946856757 ) ) ;
#19454=CARTESIAN_POINT ( 'NONE',  ( 19.02544592524334988, 5.153800228976608722, 96.45942372801897591 ) ) ;
#19455=CARTESIAN_POINT ( 'NONE',  ( -0.05219959533910754901, -16.53943276465976808, 62.49890960531436690 ) ) ;
#19456=CARTESIAN_POINT ( 'NONE',  ( -8.224510206698735004, -14.34966873604973081, 74.58442372801901854 ) ) ;
#19457=CARTESIAN_POINT ( 'NONE',  ( 0.05219959533907565091, 21.53943276465977519, 114.9989096053143669 ) ) ;
#19458=CARTESIAN_POINT ( 'NONE',  ( -9.474510206698964154, 16.51473224551069663, 55.41557627198103120 ) ) ;
#19459=CARTESIAN_POINT ( 'NONE',  ( -9.474510206698964154, 16.51473224551069663, 60.41557627198102409 ) ) ;
#19460=B_SPLINE_CURVE_WITH_KNOTS ( 'NONE', 3,
 ( #24339, #25350, #194190, #86991, #164846, #146655 ),
 .UNSPECIFIED., .F., .F.,
 ( 4, 2, 4 ),
 ( 0.003989672132298042843, 0.004372778065220470425, 0.004755883998142898875 ),
 .UNSPECIFIED. ) ;
#19461=CARTESIAN_POINT ( 'NONE',  ( -12.06949235617739369, -12.14591786802326823, 74.37609039468568994 ) ) ;
#19464=CARTESIAN_POINT ( 'NONE',  ( 9.564922557961047289, -16.46253265017146816, 20.41775706135233293 ) ) ;
#19465=CARTESIAN_POINT ( 'NONE',  ( -0.05219959533909027116, -19.03943276465977164, 32.49890960531435979 ) ) ;
#19467=CARTESIAN_POINT ( 'NONE',  ( -19.05341960407617563, 5.049401038297882671, 113.5427570613523471 ) ) ;
#19468=CARTESIAN_POINT ( 'NONE',  ( 16.51473224551083163, -9.474510206698727899, 50.83442372801899722 ) ) ;
#19469=CARTESIAN_POINT ( 'NONE',  ( 16.55341960407618274, -4.379528057220086978, 31.04275706135234714 ) ) ;
#19470=CARTESIAN_POINT ( 'NONE',  ( 16.46253265017160672, -9.564922557960803928, 38.33224293864768839 ) ) ;
#19471=CARTESIAN_POINT ( 'NONE',  ( 0.05219959533909260263, 19.03943276465977164, 59.99890960531436690 ) ) ;
#19472=CARTESIAN_POINT ( 'NONE',  ( 15.80617190586746368, 15.72974639402197994, 89.37390960531435269 ) ) ;
#19473=CARTESIAN_POINT ( 'NONE',  ( 13.89961937509977652, -13.97604488694527269, 53.12390960531434558 ) ) ;
#19475=CARTESIAN_POINT ( 'NONE',  ( -16.51473224551082808, 9.474510206698731452, 98.33442372801900433 ) ) ;
#19476=CARTESIAN_POINT ( 'NONE',  ( -16.53943276465976808, 0.05219959533911058130, 71.24890960531435269 ) ) ;
#19477=CARTESIAN_POINT ( 'NONE',  ( 16.51473224551083163, -9.474510206698727899, 20.83442372801899722 ) ) ;
#19478=CARTESIAN_POINT ( 'NONE',  ( 8.224510206698953496, -14.34966873604960469, 57.91557627198103120 ) ) ;
#19479=CARTESIAN_POINT ( 'NONE',  ( -0.05219959533937732626, 21.53943276465977519, 82.50109039468568994 ) ) ;
#19480=CARTESIAN_POINT ( 'NONE',  ( -19.02544592524342804, 5.153800228976336051, 26.04057627198103120 ) ) ;
#19481=CARTESIAN_POINT ( 'NONE',  ( -5.719274019375665041, -21.55341960407619695, 84.79275706135234714 ) ) ;
#19483=CARTESIAN_POINT ( 'NONE',  ( -16.52544592524342804, 4.483927247898546575, 26.04057627198103475 ) ) ;
#19484=CARTESIAN_POINT ( 'NONE',  ( 18.67979575497194134, -10.72451020669871369, 70.83442372801901854 ) ) ;
#19485=CARTESIAN_POINT ( 'NONE',  ( 19.02544592524343514, -5.153800228976328945, 73.54057627198103830 ) ) ;
#19486=CARTESIAN_POINT ( 'NONE',  ( 10.81492255796106328, -18.62759615963255655, 40.41775706135234714 ) ) ;
#19487=CARTESIAN_POINT ( 'NONE',  ( -0.05219959533909027116, -19.03943276465977164, 82.49890960531436690 ) ) ;
#19488=CARTESIAN_POINT ( 'NONE',  ( 12.06949235617757843, -12.14591786802309237, 98.12390960531436690 ) ) ;
#19489=CARTESIAN_POINT ( 'NONE',  ( -8.314922557960811034, -14.29746914071050412, 57.08224293864769550 ) ) ;
#19490=CARTESIAN_POINT ( 'NONE',  ( -15.80617190586745835, -15.72974639402198527, 66.87390960531436690 ) ) ;
#19491=CARTESIAN_POINT ( 'NONE',  ( -19.02544592524342804, 5.153800228976336051, 81.04057627198103830 ) ) ;
#19492=CARTESIAN_POINT ( 'NONE',  ( 15.72974639402199770, -15.80617190586745480, 88.12390960531436690 ) ) ;
#19493=CARTESIAN_POINT ( 'NONE',  ( -19.02544592524334988, -5.153800228976617603, 68.95942372801896170 ) ) ;
#19494=CARTESIAN_POINT ( 'NONE',  ( -13.89961937509957401, -13.97604488694547697, 34.37609039468566863 ) ) ;
#19495=CARTESIAN_POINT ( 'NONE',  ( 12.06949235617757843, -12.14591786802309237, 83.12390960531436690 ) ) ;
#19496=CARTESIAN_POINT ( 'NONE',  ( 21.53943276465977519, -0.05219959533907433946, 48.74890960531435979 ) ) ;
#19498=CARTESIAN_POINT ( 'NONE',  ( -4.379528057220086978, -16.55341960407618274, 104.7927570613523898 ) ) ;
#19500=CARTESIAN_POINT ( 'NONE',  ( 13.89961937509957401, 13.97604488694547697, 101.8760903946856331 ) ) ;
#19501=CARTESIAN_POINT ( 'NONE',  ( 16.55341960407611168, 4.379528057220329451, 63.95724293864770260 ) ) ;
#19502=CARTESIAN_POINT ( 'NONE',  ( -19.25176906914649777, -5.499999999999796607, 95.99927264242279534 ) ) ;
#19503=CARTESIAN_POINT ( 'NONE',  ( 16.46253265017160672, -9.564922557960803928, 63.33224293864769550 ) ) ;
#19504=CARTESIAN_POINT ( 'NONE',  ( -16.53943276465976808, 0.05219959533911058130, 56.24890960531436690 ) ) ;
#19505=CARTESIAN_POINT ( 'NONE',  ( 0.05219959533909260263, 19.03943276465977164, 94.99890960531436690 ) ) ;
#19506=CARTESIAN_POINT ( 'NONE',  ( -19.05341960407617563, 5.049401038297882671, 83.54275706135233293 ) ) ;
#19507=CARTESIAN_POINT ( 'NONE',  ( -9.474510206698964154, 16.51473224551069663, 70.41557627198102409 ) ) ;
#19508=CARTESIAN_POINT ( 'NONE',  ( -13.89961937509977652, 13.97604488694528158, 85.62390960531433848 ) ) ;
#19509=CARTESIAN_POINT ( 'NONE',  ( -19.05341960407611168, -5.049401038298163336, 81.45724293864769550 ) ) ;
#19510=CARTESIAN_POINT ( 'NONE',  ( -0.05219959533907301413, -21.53943276465977519, 57.49890960531435979 ) ) ;
#19511=CARTESIAN_POINT ( 'NONE',  ( 4.483927247898790824, -16.52544592524335698, 60.20942372801902565 ) ) ;
#19512=CARTESIAN_POINT ( 'NONE',  ( 18.09918380851993547, 5.500000000000009770, 98.98618307335611632 ) ) ;
#19513=CARTESIAN_POINT ( 'NONE',  ( 5.049401038298161559, -19.05341960407611168, 52.70724293864767418 ) ) ;
#19514=CARTESIAN_POINT ( 'NONE',  ( 15.80617190586746368, 15.72974639402197994, 54.37390960531435979 ) ) ;
#19515=CARTESIAN_POINT ( 'NONE',  ( -19.02544592524334988, -5.153800228976617603, 93.95942372801900433 ) ) ;
#19516=CARTESIAN_POINT ( 'NONE',  ( -14.29746914071049879, 8.314922557960819915, 30.83224293864770260 ) ) ;
#19517=CARTESIAN_POINT ( 'NONE',  ( 15.72974639402176855, 15.80617190586768217, 41.87609039468568284 ) ) ;
#19518=CARTESIAN_POINT ( 'NONE',  ( 13.89961937509957401, 13.97604488694547697, 36.87609039468565442 ) ) ;
#19519=CARTESIAN_POINT ( 'NONE',  ( -4.483927247898782831, 16.52544592524335698, 57.70942372801901143 ) ) ;
#19520=CARTESIAN_POINT ( 'NONE',  ( 4.483927247898790824, -16.52544592524335698, 100.2094237280190043 ) ) ;
#19521=CARTESIAN_POINT ( 'NONE',  ( 19.46398650005391318, -5.499999999999944045, 42.68269651486371430 ) ) ;
#19522=CARTESIAN_POINT ( 'NONE',  ( -4.483927247898782831, 16.52544592524335698, 82.70942372801900433 ) ) ;
#19523=CARTESIAN_POINT ( 'NONE',  ( 16.55341960407618274, -4.379528057220086978, 36.04275706135234714 ) ) ;
#19524=CARTESIAN_POINT ( 'NONE',  ( 16.51473224551069308, 9.474510206698969483, 49.16557627198102409 ) ) ;
#19525=CARTESIAN_POINT ( 'NONE',  ( -13.89961937509977652, 13.97604488694528158, 45.62390960531433848 ) ) ;
#19526=CARTESIAN_POINT ( 'NONE',  ( -13.97604488694527625, -13.89961937509977652, 56.87390960531434558 ) ) ;
#19527=CARTESIAN_POINT ( 'NONE',  ( -21.53943276465977519, -0.05219959533937600094, 58.75109039468568994 ) ) ;
#19528=CARTESIAN_POINT ( 'NONE',  ( -14.29746914071037622, -8.314922557961029526, 44.16775706135234714 ) ) ;
#19529=CARTESIAN_POINT ( 'NONE',  ( 8.314922557961029526, -14.29746914071037800, 110.4177570613523756 ) ) ;
#19530=CARTESIAN_POINT ( 'NONE',  ( 19.05341960407611168, 5.049401038298154454, 23.95724293864769194 ) ) ;
#19531=CARTESIAN_POINT ( 'NONE',  ( -5.049401038297874678, -19.05341960407617918, 24.79275706135233648 ) ) ;
#19532=CARTESIAN_POINT ( 'NONE',  ( 19.05341960407617918, -5.049401038297876454, 106.0427570613523471 ) ) ;
#19533=CARTESIAN_POINT ( 'NONE',  ( -9.474510206698720793, -16.51473224551083518, 79.58442372801899012 ) ) ;
#19534=CARTESIAN_POINT ( 'NONE',  ( 14.34966873604960469, 8.224510206698951720, 89.16557627198102409 ) ) ;
#19535=CARTESIAN_POINT ( 'NONE',  ( -19.03943276465977164, 0.05219959533909376836, 41.24890960531435269 ) ) ;
#19536=CARTESIAN_POINT ( 'NONE',  ( 19.03943276465977164, 0.05219959533936151252, 71.25109039468566152 ) ) ;
#19538=CARTESIAN_POINT ( 'NONE',  ( -15.72974639402176322, -15.80617190586768395, 79.37609039468567573 ) ) ;
#19539=CARTESIAN_POINT ( 'NONE',  ( 12.14591786802327356, -12.06949235617739191, 45.62609039468567573 ) ) ;
#19540=CARTESIAN_POINT ( 'NONE',  ( -17.50000000000000000, 5.499999999999992895, 23.71769037696436300 ) ) ;
#19541=CARTESIAN_POINT ( 'NONE',  ( -21.52544592524343514, 5.823673210054127303, 31.04057627198102409 ) ) ;
#19542=CARTESIAN_POINT ( 'NONE',  ( 14.34966873604972726, -8.224510206698740333, 30.83442372801902209 ) ) ;
#19543=CARTESIAN_POINT ( 'NONE',  ( -16.51473224551069308, -9.474510206698971260, 26.66557627198103120 ) ) ;
#19544=CARTESIAN_POINT ( 'NONE',  ( 19.02544592524334988, 5.153800228976608722, 26.45942372801899722 ) ) ;
#19546=CARTESIAN_POINT ( 'NONE',  ( 13.97604488694527802, 13.89961937509977652, 44.37390960531435269 ) ) ;
#19548=CARTESIAN_POINT ( 'NONE',  ( -5.049401038298153566, 19.05341960407611168, 65.20724293864765286 ) ) ;
#19549=CARTESIAN_POINT ( 'NONE',  ( 17.50000000000000000, -5.500000000000000888, 113.2969038253417153 ) ) ;
#19551=CARTESIAN_POINT ( 'NONE',  ( -9.564922557961040184, 16.46253265017147172, 22.91775706135233648 ) ) ;
#19552=CARTESIAN_POINT ( 'NONE',  ( 8.314922557960818139, 14.29746914071049879, 39.58224293864769550 ) ) ;
#19553=CARTESIAN_POINT ( 'NONE',  ( 9.474510206698971260, -16.51473224551069308, 42.91557627198103120 ) ) ;
#19554=CARTESIAN_POINT ( 'NONE',  ( -0.05219959533909027116, -19.03943276465977164, 97.49890960531436690 ) ) ;
#19555=CARTESIAN_POINT ( 'NONE',  ( 15.80617190586769283, -15.72974639402175789, 70.62609039468567573 ) ) ;
#19556=CARTESIAN_POINT ( 'NONE',  ( 13.89961937509977652, -13.97604488694527269, 53.12390960531434558 ) ) ;
#19557=CARTESIAN_POINT ( 'NONE',  ( 0.05219959533937995610, -21.53943276465977519, 70.00109039468568994 ) ) ;
#19558=CARTESIAN_POINT ( 'NONE',  ( -19.03943276465977164, 0.05219959533909376836, 116.2489096053143669 ) ) ;
#19559=CARTESIAN_POINT ( 'NONE',  ( -19.03943276465977164, 0.05219959533909376836, 31.24890960531435979 ) ) ;
#19560=CARTESIAN_POINT ( 'NONE',  ( 10.81492255796106328, -18.62759615963255655, 25.41775706135235779 ) ) ;
#19561=CARTESIAN_POINT ( 'NONE',  ( -9.564922557961040184, 16.46253265017147172, 42.91775706135234003 ) ) ;
#19562=CARTESIAN_POINT ( 'NONE',  ( -16.55341960407611168, -4.379528057220339221, 111.4572429386476813 ) ) ;
#19563=CARTESIAN_POINT ( 'NONE',  ( 9.474510206698971260, -16.51473224551069308, 57.91557627198103120 ) ) ;
#19564=CARTESIAN_POINT ( 'NONE',  ( -9.474510206698720793, -16.51473224551083518, 109.5844237280190043 ) ) ;
#19565=CARTESIAN_POINT ( 'NONE',  ( 16.53943276465976808, -0.05219959533910856209, 78.74890960531436690 ) ) ;
#19566=CARTESIAN_POINT ( 'NONE',  ( 9.474510206698971260, -16.51473224551069308, 112.9155762719810383 ) ) ;
#19567=CARTESIAN_POINT ( 'NONE',  ( -13.97604488694547697, 13.89961937509957934, 93.12609039468566152 ) ) ;
#19568=CARTESIAN_POINT ( 'NONE',  ( 21.52544592524344225, -5.823673210054117533, 108.5405762719810241 ) ) ;
#19569=CARTESIAN_POINT ( 'NONE',  ( -15.72974639402176322, -15.80617190586768395, 54.37609039468568994 ) ) ;
#19570=CARTESIAN_POINT ( 'NONE',  ( 8.224510206698742110, 14.34966873604972548, 57.08442372801901854 ) ) ;
#19571=CARTESIAN_POINT ( 'NONE',  ( -16.55341960407617563, 4.379528057220093196, 53.54275706135234714 ) ) ;
#19572=CARTESIAN_POINT ( 'NONE',  ( 21.53943276465977519, -0.05219959533907433946, 48.74890960531435979 ) ) ;
#19574=CARTESIAN_POINT ( 'NONE',  ( 13.97604488694527802, 13.89961937509977652, 54.37390960531435979 ) ) ;
#19576=CARTESIAN_POINT ( 'NONE',  ( -14.29746914071037622, -8.314922557961029526, 79.16775706135234714 ) ) ;
#19577=CARTESIAN_POINT ( 'NONE',  ( -18.62759615963270932, 10.81492255796079327, 105.8322429386476955 ) ) ;
#19578=CARTESIAN_POINT ( 'NONE',  ( -0.05219959533910754901, -16.53943276465976808, 57.49890960531435979 ) ) ;
#19579=CARTESIAN_POINT ( 'NONE',  ( -19.05341960407611168, -5.049401038298163336, 66.45724293864769550 ) ) ;
#19580=CARTESIAN_POINT ( 'NONE',  ( -16.53943276465976808, -0.05219959533934237506, 78.75109039468568994 ) ) ;
#19581=CARTESIAN_POINT ( 'NONE',  ( -19.03943276465977164, -0.05219959533935918106, 103.7510903946856757 ) ) ;
#19582=CARTESIAN_POINT ( 'NONE',  ( -5.823673210054116645, -21.52544592524344225, 97.29057627198105251 ) ) ;
#19583=CARTESIAN_POINT ( 'NONE',  ( -16.53943276465976808, 0.05219959533911058130, 46.24890960531435979 ) ) ;
#19584=ORIENTED_EDGE ( 'NONE', *, *, #83145, .T. ) ;
#19585=CARTESIAN_POINT ( 'NONE',  ( -16.36317988757058828, 7.306389748694926745, 69.09789608363226421 ) ) ;
#19586=CARTESIAN_POINT ( 'NONE',  ( -21.53943276465977519, 0.05219959533907696930, 76.24890960531435269 ) ) ;
#19587=CARTESIAN_POINT ( 'NONE',  ( 16.53943276465976808, -0.05219959533910856209, 23.74890960531435269 ) ) ;
#19589=CARTESIAN_POINT ( 'NONE',  ( -17.26058549869089020, -6.457015423128631859, 56.37745837476069966 ) ) ;
#19590=CARTESIAN_POINT ( 'NONE',  ( -21.53943276465977519, 0.05219959533907696930, 96.24890960531435269 ) ) ;
#19591=CARTESIAN_POINT ( 'NONE',  ( 21.55341960407619695, -5.719274019375665929, 26.04275706135235779 ) ) ;
#19592=CARTESIAN_POINT ( 'NONE',  ( 8.314922557960818139, 14.29746914071049879, 34.58224293864770260 ) ) ;
#19593=CARTESIAN_POINT ( 'NONE',  ( -4.379528057220086978, -16.55341960407618274, 49.79275706135234714 ) ) ;
#19595=CARTESIAN_POINT ( 'NONE',  ( 16.46253265017160672, -9.564922557960803928, 53.33224293864768839 ) ) ;
#19596=CARTESIAN_POINT ( 'NONE',  ( -19.03943276465977164, 0.05219959533909376836, 76.24890960531435269 ) ) ;
#19598=CARTESIAN_POINT ( 'NONE',  ( -5.719274019375978568, 21.55341960407610458, 35.20724293864768839 ) ) ;
#19600=CARTESIAN_POINT ( 'NONE',  ( 4.483927247898790824, -16.52544592524335698, 25.20942372801901854 ) ) ;
#19601=CARTESIAN_POINT ( 'NONE',  ( -5.153800228976607833, 19.02544592524334988, 52.70942372801900433 ) ) ;
#19602=CARTESIAN_POINT ( 'NONE',  ( 0.05219959533907565091, 21.53943276465977519, 104.9989096053143669 ) ) ;
#19603=CARTESIAN_POINT ( 'NONE',  ( -14.29746914071049879, 8.314922557960819915, 40.83224293864769550 ) ) ;
#19604=CARTESIAN_POINT ( 'NONE',  ( 16.46253265017160672, -9.564922557960803928, 73.33224293864769550 ) ) ;
#19605=CARTESIAN_POINT ( 'NONE',  ( -5.719274019375978568, 21.55341960407610458, 65.20724293864768129 ) ) ;
#19606=CARTESIAN_POINT ( 'NONE',  ( -21.53943276465977519, 0.05219959533907696930, 96.24890960531435269 ) ) ;
#19607=CARTESIAN_POINT ( 'NONE',  ( 4.483927247898790824, -16.52544592524335698, 20.20942372801900788 ) ) ;
#19608=CARTESIAN_POINT ( 'NONE',  ( -5.049401038298153566, 19.05341960407611168, 115.2072429386477097 ) ) ;
#19609=CARTESIAN_POINT ( 'NONE',  ( -5.719274019375665041, -21.55341960407619695, 84.79275706135234714 ) ) ;
#19610=CARTESIAN_POINT ( 'NONE',  ( 5.153800228976335163, 19.02544592524342804, 74.79057627198103830 ) ) ;
#19611=CARTESIAN_POINT ( 'NONE',  ( -16.46253265017160317, 9.564922557960807481, 25.83224293864769194 ) ) ;
#19612=CARTESIAN_POINT ( 'NONE',  ( 9.564922557960805705, 16.46253265017160317, 89.58224293864769550 ) ) ;
#19613=CARTESIAN_POINT ( 'NONE',  ( -16.52544592524342804, 4.483927247898546575, 101.0405762719810383 ) ) ;
#19614=CARTESIAN_POINT ( 'NONE',  ( 19.02544592524334988, 5.153800228976608722, 101.4594237280189759 ) ) ;
#19617=CARTESIAN_POINT ( 'NONE',  ( 16.51473224551069308, 9.474510206698969483, 79.16557627198103830 ) ) ;
#19618=CARTESIAN_POINT ( 'NONE',  ( 5.719274019375673035, 21.55341960407619339, 97.29275706135234714 ) ) ;
#19619=CARTESIAN_POINT ( 'NONE',  ( -19.02544592524342804, 5.153800228976336051, 111.0405762719810099 ) ) ;
#19620=CARTESIAN_POINT ( 'NONE',  ( -4.379528057220086978, -16.55341960407618274, 94.79275706135234714 ) ) ;
#19621=CARTESIAN_POINT ( 'NONE',  ( -17.40861289039003879, -6.110651285853241355, 76.37232470827430575 ) ) ;
#19622=CARTESIAN_POINT ( 'NONE',  ( 9.564922557961047289, -16.46253265017146816, 60.41775706135233293 ) ) ;
#19623=CARTESIAN_POINT ( 'NONE',  ( -5.823673210054431948, 21.52544592524334988, 107.7094237280190328 ) ) ;
#19625=CARTESIAN_POINT ( 'NONE',  ( 5.049401038298161559, -19.05341960407611168, 22.70724293864769194 ) ) ;
#19626=CARTESIAN_POINT ( 'NONE',  ( 4.483927247898790824, -16.52544592524335698, 110.2094237280190185 ) ) ;
#19628=CARTESIAN_POINT ( 'NONE',  ( 4.379528057220092307, 16.55341960407617563, 102.2927570613523613 ) ) ;
#19629=CARTESIAN_POINT ( 'NONE',  ( -18.39639308325438094, -5.499999999999988454, 86.48252246182198633 ) ) ;
#19630=CARTESIAN_POINT ( 'NONE',  ( 14.34966873604972726, -8.224510206698740333, 85.83442372801901854 ) ) ;
#19631=CARTESIAN_POINT ( 'NONE',  ( 16.51473224551069308, 9.474510206698969483, 84.16557627198102409 ) ) ;
#19632=CARTESIAN_POINT ( 'NONE',  ( -18.67979575497193778, 10.72451020669871902, 93.33442372801901854 ) ) ;
#19633=CARTESIAN_POINT ( 'NONE',  ( 9.474510206698729675, 16.51473224551082808, 107.0844237280190043 ) ) ;
#19634=CARTESIAN_POINT ( 'NONE',  ( 5.823673210054444382, -21.52544592524334988, 70.20942372801904696 ) ) ;
#19635=CARTESIAN_POINT ( 'NONE',  ( 5.049401038297881783, 19.05341960407617563, 57.29275706135231871 ) ) ;
#19636=CARTESIAN_POINT ( 'NONE',  ( 16.46253265017160672, -9.564922557960803928, 73.33224293864769550 ) ) ;
#19637=CARTESIAN_POINT ( 'NONE',  ( 0.05219959533909260263, 19.03943276465977164, 64.99890960531436690 ) ) ;
#19638=CARTESIAN_POINT ( 'NONE',  ( 16.36317988757055630, 7.306389748694925856, 73.40210391636770737 ) ) ;
#19639=CARTESIAN_POINT ( 'NONE',  ( 15.72974639402199770, -15.80617190586745480, 43.12390960531435269 ) ) ;
#19640=CARTESIAN_POINT ( 'NONE',  ( -5.049401038298153566, 19.05341960407611168, 40.20724293864768839 ) ) ;
#19641=CARTESIAN_POINT ( 'NONE',  ( -0.05219959533907301413, -21.53943276465977519, 87.49890960531436690 ) ) ;
#19642=CARTESIAN_POINT ( 'NONE',  ( 4.379528057220092307, 16.55341960407617563, 82.29275706135234714 ) ) ;
#19645=CARTESIAN_POINT ( 'NONE',  ( -12.14591786802309592, -12.06949235617757132, 81.87390960531435269 ) ) ;
#19647=CARTESIAN_POINT ( 'NONE',  ( 8.224510206698742110, 14.34966873604972548, 32.08442372801901854 ) ) ;
#19648=CARTESIAN_POINT ( 'NONE',  ( 5.049401038298161559, -19.05341960407611168, 22.70724293864769194 ) ) ;
#19649=CARTESIAN_POINT ( 'NONE',  ( 13.89961937509957401, 13.97604488694547697, 66.87609039468567573 ) ) ;
#19650=CARTESIAN_POINT ( 'NONE',  ( -0.05219959533910754901, -16.53943276465976808, 67.49890960531436690 ) ) ;
#19651=CARTESIAN_POINT ( 'NONE',  ( 21.53943276465977519, 0.05219959533937863772, 46.25109039468567573 ) ) ;
#19653=CARTESIAN_POINT ( 'NONE',  ( 10.72451020669898902, -18.67979575497178502, 87.91557627198103830 ) ) ;
#19655=CARTESIAN_POINT ( 'NONE',  ( -4.379528057220328563, 16.55341960407611168, 70.20724293864769550 ) ) ;
#19657=CARTESIAN_POINT ( 'NONE',  ( -9.564922557960796823, -16.46253265017161027, 42.08224293864769550 ) ) ;
#19659=CARTESIAN_POINT ( 'NONE',  ( -19.05341960407617563, 5.049401038297882671, 78.54275706135233293 ) ) ;
#19660=CARTESIAN_POINT ( 'NONE',  ( -10.72451020669870658, -18.67979575497194134, 29.58442372801901854 ) ) ;
#19661=CARTESIAN_POINT ( 'NONE',  ( 13.89961937509977652, -13.97604488694527269, 68.12390960531436690 ) ) ;
#19662=CARTESIAN_POINT ( 'NONE',  ( 5.153800228976615827, -19.02544592524334988, 55.20942372801899722 ) ) ;
#19663=CARTESIAN_POINT ( 'NONE',  ( -9.564922557960796823, -16.46253265017161027, 42.08224293864769550 ) ) ;
#19664=CARTESIAN_POINT ( 'NONE',  ( 16.55341960407611168, 4.379528057220329451, 63.95724293864770260 ) ) ;
#19665=CARTESIAN_POINT ( 'NONE',  ( 4.483927247898545687, 16.52544592524342804, 49.79057627198102409 ) ) ;
#19666=CARTESIAN_POINT ( 'NONE',  ( 5.049401038298161559, -19.05341960407611168, 82.70724293864770971 ) ) ;
#19667=CARTESIAN_POINT ( 'NONE',  ( 5.823673210054125526, 21.52544592524343514, 99.79057627198103830 ) ) ;
#19668=CARTESIAN_POINT ( 'NONE',  ( -13.89961937509977652, 13.97604488694528158, 70.62390960531432427 ) ) ;
#19669=CARTESIAN_POINT ( 'NONE',  ( 18.67979575497178502, 10.72451020669898547, 74.16557627198102409 ) ) ;
#19670=CARTESIAN_POINT ( 'NONE',  ( -21.55341960407619339, 5.719274019375674811, 113.5427570613523756 ) ) ;
#19671=CARTESIAN_POINT ( 'NONE',  ( 19.05341960407611168, 5.049401038298154454, 28.95724293864769550 ) ) ;
#19672=CARTESIAN_POINT ( 'NONE',  ( -12.14591786802326823, 12.06949235617739902, 108.1260903946856757 ) ) ;
#19673=CARTESIAN_POINT ( 'NONE',  ( 14.34966873604960469, 8.224510206698951720, 99.16557627198100988 ) ) ;
#19674=CARTESIAN_POINT ( 'NONE',  ( -19.02544592524334988, -5.153800228976617603, 108.9594237280189759 ) ) ;
#19676=CARTESIAN_POINT ( 'NONE',  ( -18.67979575497193778, 10.72451020669871902, 28.33442372801902209 ) ) ;
#19677=CARTESIAN_POINT ( 'NONE',  ( 19.02544592524334988, 5.153800228976608722, 51.45942372801900433 ) ) ;
#19678=CARTESIAN_POINT ( 'NONE',  ( 14.29746914071049879, -8.314922557960816363, 23.33224293864769194 ) ) ;
#19679=CARTESIAN_POINT ( 'NONE',  ( 10.72451020669898902, -18.67979575497178502, 72.91557627198103830 ) ) ;
#19680=CARTESIAN_POINT ( 'NONE',  ( -0.05219959533909027116, -19.03943276465977164, 97.49890960531436690 ) ) ;
#19681=CARTESIAN_POINT ( 'NONE',  ( -16.53943276465976808, 0.05219959533911058130, 56.24890960531436690 ) ) ;
#19682=CARTESIAN_POINT ( 'NONE',  ( -19.05341960407611168, -5.049401038298163336, 26.45724293864769550 ) ) ;
#19683=CARTESIAN_POINT ( 'NONE',  ( -5.153800228976328057, -19.02544592524343514, 37.29057627198102409 ) ) ;
#19684=CARTESIAN_POINT ( 'NONE',  ( 0.05219959533937995610, -21.53943276465977519, 105.0010903946856757 ) ) ;
#19685=CARTESIAN_POINT ( 'NONE',  ( 14.29746914071037800, 8.314922557961029526, 86.66775706135234714 ) ) ;
#19686=CARTESIAN_POINT ( 'NONE',  ( -10.72451020669870658, -18.67979575497194134, 44.58442372801901854 ) ) ;
#19687=CARTESIAN_POINT ( 'NONE',  ( 4.483927247898790824, -16.52544592524335698, 45.20942372801901854 ) ) ;
#19688=CARTESIAN_POINT ( 'NONE',  ( 5.719274019375991003, -21.55341960407610458, 22.70724293864769194 ) ) ;
#19689=CARTESIAN_POINT ( 'NONE',  ( 5.153800228976335163, 19.02544592524342804, 54.79057627198103120 ) ) ;
#19690=CARTESIAN_POINT ( 'NONE',  ( -13.89961937509977652, 13.97604488694528158, 60.62390960531436690 ) ) ;
#19691=CARTESIAN_POINT ( 'NONE',  ( 8.224510206698742110, 14.34966873604972548, 57.08442372801901854 ) ) ;
#19692=CARTESIAN_POINT ( 'NONE',  ( -4.483927247898539470, -16.52544592524342804, 112.2905762719810241 ) ) ;
#19693=CARTESIAN_POINT ( 'NONE',  ( -8.314922557960811034, -14.29746914071050412, 22.08224293864769194 ) ) ;
#19695=CARTESIAN_POINT ( 'NONE',  ( -15.80617190586768217, 15.72974639402176855, 63.12609039468568994 ) ) ;
#19696=CARTESIAN_POINT ( 'NONE',  ( -5.049401038298153566, 19.05341960407611168, 90.20724293864766707 ) ) ;
#19697=CARTESIAN_POINT ( 'NONE',  ( 13.97604488694527802, 13.89961937509977652, 84.37390960531433848 ) ) ;
#19698=CARTESIAN_POINT ( 'NONE',  ( 13.89961937509977652, -13.97604488694527269, 108.1239096053143669 ) ) ;
#19699=CARTESIAN_POINT ( 'NONE',  ( 8.224510206698953496, -14.34966873604960469, 42.91557627198103120 ) ) ;
#19700=CARTESIAN_POINT ( 'NONE',  ( -8.224510206698948167, 14.34966873604960824, 25.41557627198103120 ) ) ;
#19701=CARTESIAN_POINT ( 'NONE',  ( 4.483927247898545687, 16.52544592524342804, 34.79057627198103120 ) ) ;
#19702=CARTESIAN_POINT ( 'NONE',  ( 17.60691670004651144, 5.500000000000060396, 56.63333313366439370 ) ) ;
#19703=CARTESIAN_POINT ( 'NONE',  ( 19.03943276465977164, 0.05219959533936151252, 31.25109039468566863 ) ) ;
#19704=CARTESIAN_POINT ( 'NONE',  ( -13.89961937509977652, 13.97604488694528158, 80.62390960531436690 ) ) ;
#19705=CARTESIAN_POINT ( 'NONE',  ( -5.153800228976607833, 19.02544592524334988, 47.70942372801900433 ) ) ;
#19707=DIRECTION ( 'NONE',  ( -0.000000000000000000, -0.000000000000000000, 1.000000000000000000 ) ) ;
#19708=CARTESIAN_POINT ( 'NONE',  ( -16.51473224551082808, 9.474510206698731452, 83.33442372801899012 ) ) ;
#19709=CARTESIAN_POINT ( 'NONE',  ( -12.06949235617739369, -12.14591786802326823, 69.37609039468567573 ) ) ;
#19711=CARTESIAN_POINT ( 'NONE',  ( -5.049401038298153566, 19.05341960407611168, 105.2072429386476671 ) ) ;
#19712=CARTESIAN_POINT ( 'NONE',  ( -5.719274019375665041, -21.55341960407619695, 29.79275706135234358 ) ) ;
#19713=CARTESIAN_POINT ( 'NONE',  ( 19.05341960407617918, -5.049401038297876454, 91.04275706135234714 ) ) ;
#19714=CARTESIAN_POINT ( 'NONE',  ( 9.474510206698971260, -16.51473224551069308, 112.9155762719810383 ) ) ;
#19715=CARTESIAN_POINT ( 'NONE',  ( -0.05219959533909027116, -19.03943276465977164, 52.49890960531436690 ) ) ;
#19716=CARTESIAN_POINT ( 'NONE',  ( 5.049401038298161559, -19.05341960407611168, 87.70724293864769550 ) ) ;
#19717=CARTESIAN_POINT ( 'NONE',  ( -16.52544592524342804, 4.483927247898546575, 46.04057627198103830 ) ) ;
#19718=CARTESIAN_POINT ( 'NONE',  ( 16.51473224551069308, 9.474510206698969483, 44.16557627198103120 ) ) ;
#19719=CARTESIAN_POINT ( 'NONE',  ( 19.05341960407617918, -5.049401038297876454, 66.04275706135233293 ) ) ;
#19720=CARTESIAN_POINT ( 'NONE',  ( 16.51473224551083163, -9.474510206698727899, 25.83442372801900078 ) ) ;
#19721=CARTESIAN_POINT ( 'NONE',  ( -19.05341960407611168, -5.049401038298163336, 71.45724293864766707 ) ) ;
#19722=ADVANCED_FACE ( 'NONE', ( #142484 ), #97944, .T. ) ;
#19723=CARTESIAN_POINT ( 'NONE',  ( -5.823673210054116645, -21.52544592524344225, 67.29057627198103830 ) ) ;
#19724=CARTESIAN_POINT ( 'NONE',  ( 16.52544592524342804, -4.483927247898539470, 63.54057627198103830 ) ) ;
#19725=CARTESIAN_POINT ( 'NONE',  ( -15.80617190586768217, 15.72974639402176855, 113.1260903946856899 ) ) ;
#19727=CARTESIAN_POINT ( 'NONE',  ( -21.53943276465977519, 0.05219959533907696930, 21.24890960531436690 ) ) ;
#19728=CARTESIAN_POINT ( 'NONE',  ( 19.05341960407611168, 5.049401038298154454, 58.95724293864768129 ) ) ;
#19729=CARTESIAN_POINT ( 'NONE',  ( 13.89961937509977652, -13.97604488694527269, 38.12390960531436690 ) ) ;
#19730=CARTESIAN_POINT ( 'NONE',  ( 8.314922557960818139, 14.29746914071049879, 99.58224293864770971 ) ) ;
#19731=CARTESIAN_POINT ( 'NONE',  ( -5.719274019375978568, 21.55341960407610458, 105.2072429386477097 ) ) ;
#19733=CARTESIAN_POINT ( 'NONE',  ( 18.62759615963255655, 10.81492255796105972, 26.66775706135235424 ) ) ;
#19734=CARTESIAN_POINT ( 'NONE',  ( -16.51473224551069308, -9.474510206698971260, 26.66557627198103120 ) ) ;
#19735=CARTESIAN_POINT ( 'NONE',  ( -15.72974639402176322, -15.80617190586768395, 79.37609039468567573 ) ) ;
#19736=CARTESIAN_POINT ( 'NONE',  ( -10.81492255796078084, -18.62759615963271287, 92.08224293864769550 ) ) ;
#19737=CARTESIAN_POINT ( 'NONE',  ( 9.564922557961047289, -16.46253265017146816, 35.41775706135233293 ) ) ;
#19738=CARTESIAN_POINT ( 'NONE',  ( -19.03943276465977164, 0.05219959533909376836, 26.24890960531435624 ) ) ;
#19739=PLANE ( 'NONE',  #72096 ) ;
#19741=CARTESIAN_POINT ( 'NONE',  ( 4.379528057220092307, 16.55341960407617563, 47.29275706135234003 ) ) ;
#19742=CARTESIAN_POINT ( 'NONE',  ( -16.53943276465976808, 0.05219959533911058130, 106.2489096053143811 ) ) ;
#19744=CARTESIAN_POINT ( 'NONE',  ( 19.02544592524343514, -5.153800228976328945, 73.54057627198103830 ) ) ;
#19745=CARTESIAN_POINT ( 'NONE',  ( -4.379528057220328563, 16.55341960407611168, 100.2072429386476955 ) ) ;
#19746=CARTESIAN_POINT ( 'NONE',  ( 18.67979575497178502, 10.72451020669898547, 49.16557627198102409 ) ) ;
#19747=CARTESIAN_POINT ( 'NONE',  ( 16.55341960407611168, 4.379528057220329451, 68.95724293864769550 ) ) ;
#19748=CARTESIAN_POINT ( 'NONE',  ( 4.483927247898790824, -16.52544592524335698, 40.20942372801901854 ) ) ;
#19749=CARTESIAN_POINT ( 'NONE',  ( 15.72974639402176855, 15.80617190586768217, 86.87609039468568994 ) ) ;
#19750=CARTESIAN_POINT ( 'NONE',  ( 17.05587630539786659, -6.762274262135687053, 78.24180309037315340 ) ) ;
#19751=CARTESIAN_POINT ( 'NONE',  ( -4.483927247898782831, 16.52544592524335698, 102.7094237280190185 ) ) ;
#19752=CARTESIAN_POINT ( 'NONE',  ( -16.55341960407611168, -4.379528057220339221, 46.45724293864769550 ) ) ;
#19753=CARTESIAN_POINT ( 'NONE',  ( 5.049401038298161559, -19.05341960407611168, 42.70724293864767418 ) ) ;
#19754=CARTESIAN_POINT ( 'NONE',  ( 18.67979575497194134, -10.72451020669871369, 90.83442372801901854 ) ) ;
#19755=CARTESIAN_POINT ( 'NONE',  ( -21.52544592524343514, 5.823673210054127303, 106.0405762719810525 ) ) ;
#19756=CARTESIAN_POINT ( 'NONE',  ( -5.719274019375665041, -21.55341960407619695, 59.79275706135234714 ) ) ;
#19757=CARTESIAN_POINT ( 'NONE',  ( 14.34966873604972726, -8.224510206698740333, 45.83442372801901854 ) ) ;
#19758=CARTESIAN_POINT ( 'NONE',  ( 8.224510206698953496, -14.34966873604960469, 62.91557627198102409 ) ) ;
#19759=CARTESIAN_POINT ( 'NONE',  ( 5.719274019375673035, 21.55341960407619339, 82.29275706135234714 ) ) ;
#19760=CARTESIAN_POINT ( 'NONE',  ( -16.53943276465976808, 0.05219959533911058130, 26.24890960531435624 ) ) ;
#19761=CARTESIAN_POINT ( 'NONE',  ( 16.52216118717208460, 7.221426719304522734, 28.57599021046994636 ) ) ;
#19763=CARTESIAN_POINT ( 'NONE',  ( -8.314922557960811034, -14.29746914071050412, 32.08224293864769550 ) ) ;
#19764=CARTESIAN_POINT ( 'NONE',  ( -16.53943276465976808, -0.05219959533934237506, 73.75109039468567573 ) ) ;
#19765=CARTESIAN_POINT ( 'NONE',  ( 19.02544592524343514, -5.153800228976328945, 88.54057627198102409 ) ) ;
#19766=CARTESIAN_POINT ( 'NONE',  ( -16.46253265017160317, 9.564922557960807481, 105.8322429386476955 ) ) ;
#19767=CARTESIAN_POINT ( 'NONE',  ( 0.05219959533937995610, -21.53943276465977519, 80.00109039468568994 ) ) ;
#19768=CARTESIAN_POINT ( 'NONE',  ( -8.224510206698735004, -14.34966873604973081, 84.58442372801903275 ) ) ;
#19769=CARTESIAN_POINT ( 'NONE',  ( 14.29746914071049879, -8.314922557960816363, 63.33224293864770260 ) ) ;
#19770=CARTESIAN_POINT ( 'NONE',  ( 16.51473224551069308, 9.474510206698969483, 69.16557627198102409 ) ) ;
#19772=CARTESIAN_POINT ( 'NONE',  ( 12.14591786802327356, -12.06949235617739191, 30.62609039468567929 ) ) ;
#19773=CARTESIAN_POINT ( 'NONE',  ( -19.03943276465977164, 0.05219959533909376836, 26.24890960531435624 ) ) ;
#19774=CARTESIAN_POINT ( 'NONE',  ( 19.02544592524343514, -5.153800228976328945, 73.54057627198103830 ) ) ;
#19775=CARTESIAN_POINT ( 'NONE',  ( 19.03943276465977164, 0.05219959533936151252, 111.2510903946856757 ) ) ;
#19777=CARTESIAN_POINT ( 'NONE',  ( 9.564922557961047289, -16.46253265017146816, 25.41775706135234003 ) ) ;
#19778=CARTESIAN_POINT ( 'NONE',  ( 14.34966873604972726, -8.224510206698740333, 85.83442372801901854 ) ) ;
#19779=CARTESIAN_POINT ( 'NONE',  ( -9.564922557961040184, 16.46253265017147172, 102.9177570613523329 ) ) ;
#19780=CARTESIAN_POINT ( 'NONE',  ( 8.224510206698953496, -14.34966873604960469, 112.9155762719810383 ) ) ;
#19781=CARTESIAN_POINT ( 'NONE',  ( 16.53943276465976808, 0.05219959533934440121, 71.25109039468568994 ) ) ;
#19782=CARTESIAN_POINT ( 'NONE',  ( 4.483927247898790824, -16.52544592524335698, 55.20942372801902565 ) ) ;
#19784=CARTESIAN_POINT ( 'NONE',  ( 13.97604488694548053, -13.89961937509957401, 75.62609039468564731 ) ) ;
#19785=CARTESIAN_POINT ( 'NONE',  ( -15.80617190586768217, 15.72974639402176855, 108.1260903946856757 ) ) ;
#19786=CARTESIAN_POINT ( 'NONE',  ( 19.03943276465977164, -0.05219959533909143690, 48.74890960531435979 ) ) ;
#19787=CARTESIAN_POINT ( 'NONE',  ( -16.51473224551069308, -9.474510206698971260, 81.66557627198103830 ) ) ;
#19788=CARTESIAN_POINT ( 'NONE',  ( 14.34966873604960469, 8.224510206698951720, 74.16557627198102409 ) ) ;
#19789=CARTESIAN_POINT ( 'NONE',  ( -16.51473224551082808, 9.474510206698731452, 43.33442372801900433 ) ) ;
#19790=CARTESIAN_POINT ( 'NONE',  ( -18.62759615963270932, 10.81492255796079327, 30.83224293864770260 ) ) ;
#19791=CARTESIAN_POINT ( 'NONE',  ( 15.72974639402176855, 15.80617190586768217, 111.8760903946856615 ) ) ;
#19792=CARTESIAN_POINT ( 'NONE',  ( -16.51473224551069308, -9.474510206698971260, 91.66557627198103830 ) ) ;
#19793=CARTESIAN_POINT ( 'NONE',  ( -10.81492255796105439, 18.62759615963255655, 107.9177570613523471 ) ) ;
#19794=CARTESIAN_POINT ( 'NONE',  ( -21.52544592524343514, 5.823673210054127303, 66.04057627198103830 ) ) ;
#19795=CARTESIAN_POINT ( 'NONE',  ( -19.02544592524342804, 5.153800228976336051, 91.04057627198100988 ) ) ;
#19796=CARTESIAN_POINT ( 'NONE',  ( -13.89961937509957401, -13.97604488694547875, 89.37609039468563310 ) ) ;
#19797=CARTESIAN_POINT ( 'NONE',  ( 16.51473224551069308, 9.474510206698969483, 104.1655762719810241 ) ) ;
#19798=CARTESIAN_POINT ( 'NONE',  ( 19.05341960407617918, -5.049401038297876454, 101.0427570613523045 ) ) ;
#19799=CARTESIAN_POINT ( 'NONE',  ( -19.05341960407611168, -5.049401038298163336, 21.45724293864768839 ) ) ;
#19800=CARTESIAN_POINT ( 'NONE',  ( -9.564922557960796823, -16.46253265017161027, 87.08224293864769550 ) ) ;
#19801=CARTESIAN_POINT ( 'NONE',  ( 10.72451020669898902, -18.67979575497178502, 57.91557627198103120 ) ) ;
#19802=CARTESIAN_POINT ( 'NONE',  ( -16.53943276465976808, -0.05219959533934237506, 48.75109039468568284 ) ) ;
#19803=CARTESIAN_POINT ( 'NONE',  ( 5.823673210054444382, -21.52544592524334988, 45.20942372801901854 ) ) ;
#19804=CARTESIAN_POINT ( 'NONE',  ( 18.62759615963255655, 10.81492255796105972, 91.66775706135234714 ) ) ;
#19805=CARTESIAN_POINT ( 'NONE',  ( -14.34966873604972548, 8.224510206698743886, 98.33442372801901854 ) ) ;
#19806=CARTESIAN_POINT ( 'NONE',  ( -9.564922557960796823, -16.46253265017161027, 92.08224293864769550 ) ) ;
#19807=CARTESIAN_POINT ( 'NONE',  ( 16.55341960407611168, 4.379528057220329451, 93.95724293864770971 ) ) ;
#19808=CARTESIAN_POINT ( 'NONE',  ( 16.52544592524335698, 4.483927247898782831, 111.4594237280190328 ) ) ;
#19809=CARTESIAN_POINT ( 'NONE',  ( -9.474510206698720793, -16.51473224551083518, 69.58442372801901854 ) ) ;
#19811=CARTESIAN_POINT ( 'NONE',  ( 5.823673210054444382, -21.52544592524334988, 40.20942372801901854 ) ) ;
#19812=CARTESIAN_POINT ( 'NONE',  ( -12.06949235617756955, 12.14591786802309770, 95.62390960531436690 ) ) ;
#19813=CARTESIAN_POINT ( 'NONE',  ( -10.81492255796078084, -18.62759615963271287, 22.08224293864769194 ) ) ;
#19814=CARTESIAN_POINT ( 'NONE',  ( -12.06949235617739369, -12.14591786802326823, 109.3760903946857042 ) ) ;
#19815=CARTESIAN_POINT ( 'NONE',  ( 21.52544592524334988, 5.823673210054432836, 81.45942372801900433 ) ) ;
#19816=CARTESIAN_POINT ( 'NONE',  ( -8.314922557961024197, 14.29746914071037800, 57.91775706135234714 ) ) ;
#19817=CARTESIAN_POINT ( 'NONE',  ( 21.55341960407619695, -5.719274019375665929, 46.04275706135234714 ) ) ;
#19819=CARTESIAN_POINT ( 'NONE',  ( 18.62759615963255655, 10.81492255796105972, 26.66775706135235424 ) ) ;
#19820=CARTESIAN_POINT ( 'NONE',  ( 16.55341960407611168, 4.379528057220329451, 103.9572429386476813 ) ) ;
#19821=CARTESIAN_POINT ( 'NONE',  ( -16.46253265017160317, 9.564922557960807481, 25.83224293864769194 ) ) ;
#19822=CARTESIAN_POINT ( 'NONE',  ( 4.483927247898545687, 16.52544592524342804, 69.79057627198102409 ) ) ;
#19823=CARTESIAN_POINT ( 'NONE',  ( 9.564922557960805705, 16.46253265017160317, 59.58224293864769550 ) ) ;
#19824=CARTESIAN_POINT ( 'NONE',  ( -0.05219959533934338120, 16.53943276465976808, 112.5010903946857042 ) ) ;
#19825=CARTESIAN_POINT ( 'NONE',  ( 19.05341960407611168, 5.049401038298154454, 38.95724293864767418 ) ) ;
#19826=CARTESIAN_POINT ( 'NONE',  ( 10.81492255796078972, 18.62759615963270932, 49.58224293864769550 ) ) ;
#19827=CARTESIAN_POINT ( 'NONE',  ( 16.52544592524342804, -4.483927247898539470, 78.54057627198103830 ) ) ;
#19828=CARTESIAN_POINT ( 'NONE',  ( -18.67979575497178146, -10.72451020669898902, 86.66557627198102409 ) ) ;
#19829=CARTESIAN_POINT ( 'NONE',  ( 16.51473224551069308, 9.474510206698969483, 94.16557627198103830 ) ) ;
#19830=CARTESIAN_POINT ( 'NONE',  ( -13.97604488694527625, -13.89961937509977652, 51.87390960531436690 ) ) ;
#19831=CARTESIAN_POINT ( 'NONE',  ( 16.46253265017146816, 9.564922557961045513, 96.66775706135233293 ) ) ;
#19832=CARTESIAN_POINT ( 'NONE',  ( 15.80617190586746368, 15.72974639402197994, 44.37390960531435979 ) ) ;
#19833=CARTESIAN_POINT ( 'NONE',  ( 10.81492255796106328, -18.62759615963255655, 65.41775706135234714 ) ) ;
#19834=CARTESIAN_POINT ( 'NONE',  ( 0.05219959533909260263, 19.03943276465977164, 49.99890960531435979 ) ) ;
#19835=CARTESIAN_POINT ( 'NONE',  ( 19.05341960407611168, 5.049401038298154454, 83.95724293864766707 ) ) ;
#19837=CARTESIAN_POINT ( 'NONE',  ( -12.14591786802326823, 12.06949235617739902, 68.12609039468567573 ) ) ;
#19838=CARTESIAN_POINT ( 'NONE',  ( -5.719274019375665041, -21.55341960407619695, 39.79275706135235424 ) ) ;
#19839=CARTESIAN_POINT ( 'NONE',  ( -21.52544592524334988, -5.823673210054445271, 73.95942372801901854 ) ) ;
#19840=CARTESIAN_POINT ( 'NONE',  ( -16.46253265017160317, 9.564922557960807481, 110.8322429386476955 ) ) ;
#19841=CARTESIAN_POINT ( 'NONE',  ( 21.52544592524344225, -5.823673210054117533, 98.54057627198105251 ) ) ;
#19842=CARTESIAN_POINT ( 'NONE',  ( -15.72974639402176322, -15.80617190586768395, 34.37609039468568284 ) ) ;
#19843=CARTESIAN_POINT ( 'NONE',  ( -16.53943276465976808, -0.05219959533934237506, 68.75109039468568994 ) ) ;
#19844=CARTESIAN_POINT ( 'NONE',  ( -21.53943276465977519, 0.05219959533907696930, 61.24890960531435979 ) ) ;
#19845=CARTESIAN_POINT ( 'NONE',  ( -9.474510206698720793, -16.51473224551083518, 29.58442372801900433 ) ) ;
#19846=CARTESIAN_POINT ( 'NONE',  ( -19.03943276465977164, 0.05219959533909376836, 66.24890960531436690 ) ) ;
#19847=CARTESIAN_POINT ( 'NONE',  ( -0.05219959533934338120, 16.53943276465976808, 102.5010903946856899 ) ) ;
#19848=CARTESIAN_POINT ( 'NONE',  ( -17.50000000000147793, -3.202012800152224337, 105.0717758397275361 ) ) ;
#19849=CARTESIAN_POINT ( 'NONE',  ( -19.03943276465977164, 0.05219959533909376836, 106.2489096053143669 ) ) ;
#19852=CARTESIAN_POINT ( 'NONE',  ( 16.46253265017146816, 9.564922557961045513, 76.66775706135234714 ) ) ;
#19853=CARTESIAN_POINT ( 'NONE',  ( 10.72451020669898902, -18.67979575497178502, 62.91557627198102409 ) ) ;
#19854=CARTESIAN_POINT ( 'NONE',  ( 0.05219959533910956823, 16.53943276465976808, 39.99890960531436690 ) ) ;
#19855=CARTESIAN_POINT ( 'NONE',  ( 0.05219959533936267826, -19.03943276465977164, 100.0010903946856757 ) ) ;
#19857=CARTESIAN_POINT ( 'NONE',  ( -16.51473224551082808, 9.474510206698731452, 113.3344237280190043 ) ) ;
#19858=CARTESIAN_POINT ( 'NONE',  ( 15.72974639402199770, -15.80617190586745480, 83.12390960531436690 ) ) ;
#19859=CARTESIAN_POINT ( 'NONE',  ( 0.05219959533936267826, -19.03943276465977164, 60.00109039468566863 ) ) ;
#19860=CARTESIAN_POINT ( 'NONE',  ( -4.483927247898782831, 16.52544592524335698, 77.70942372801900433 ) ) ;
#19861=CARTESIAN_POINT ( 'NONE',  ( 13.97604488694527802, 13.89961937509977652, 64.37390960531436690 ) ) ;
#19862=CARTESIAN_POINT ( 'NONE',  ( 14.34966873604960469, 8.224510206698951720, 69.16557627198102409 ) ) ;
#19863=CARTESIAN_POINT ( 'NONE',  ( 19.02544592524343514, -5.153800228976328945, 53.54057627198102409 ) ) ;
#19864=CARTESIAN_POINT ( 'NONE',  ( 4.379528057220339221, -16.55341960407611168, 52.70724293864769550 ) ) ;
#19865=CARTESIAN_POINT ( 'NONE',  ( 13.97604488694527802, 13.89961937509977652, 24.37390960531435624 ) ) ;
#19867=CARTESIAN_POINT ( 'NONE',  ( 4.483927247898545687, 16.52544592524342804, 29.79057627198102409 ) ) ;
#19868=CARTESIAN_POINT ( 'NONE',  ( -19.02544592524342804, 5.153800228976336051, 81.04057627198103830 ) ) ;
#19870=CARTESIAN_POINT ( 'NONE',  ( 9.474510206698729675, 16.51473224551082808, 42.08442372801900433 ) ) ;
#19871=CARTESIAN_POINT ( 'NONE',  ( 12.06949235617739724, 12.14591786802326823, 51.87609039468568284 ) ) ;
#19872=CARTESIAN_POINT ( 'NONE',  ( -0.05219959533907301413, -21.53943276465977519, 52.49890960531435979 ) ) ;
#19873=CARTESIAN_POINT ( 'NONE',  ( -18.67979575497193778, 10.72451020669871902, 113.3344237280190328 ) ) ;
#19874=CARTESIAN_POINT ( 'NONE',  ( 13.97604488694527802, 13.89961937509977652, 74.37390960531436690 ) ) ;
#19876=CARTESIAN_POINT ( 'NONE',  ( -19.03943276465977164, 0.05219959533909376836, 106.2489096053143669 ) ) ;
#19877=CARTESIAN_POINT ( 'NONE',  ( 10.81492255796106328, -18.62759615963255655, 40.41775706135234714 ) ) ;
#19878=CARTESIAN_POINT ( 'NONE',  ( 14.34966873604960469, 8.224510206698951720, 89.16557627198102409 ) ) ;
#19879=CARTESIAN_POINT ( 'NONE',  ( -21.55341960407610458, -5.719274019375992779, 81.45724293864769550 ) ) ;
#19880=CARTESIAN_POINT ( 'NONE',  ( -9.564922557960796823, -16.46253265017161027, 87.08224293864769550 ) ) ;
#19882=CARTESIAN_POINT ( 'NONE',  ( 10.72451020669871369, 18.67979575497193778, 22.08442372801901143 ) ) ;
#19883=ORIENTED_EDGE ( 'NONE', *, *, #32278, .T. ) ;
#19884=CARTESIAN_POINT ( 'NONE',  ( 5.153800228976335163, 19.02544592524342804, 89.79057627198102409 ) ) ;
#19885=CARTESIAN_POINT ( 'NONE',  ( -17.72662750342728089, -5.500000000000020428, 76.40179492283743912 ) ) ;
#19886=CARTESIAN_POINT ( 'NONE',  ( 0.05219959533909260263, 19.03943276465977164, 24.99890960531435269 ) ) ;
#19887=CARTESIAN_POINT ( 'NONE',  ( -19.03943276465977164, 0.05219959533909376836, 36.24890960531436690 ) ) ;
#19888=CARTESIAN_POINT ( 'NONE',  ( -5.153800228976607833, 19.02544592524334988, 102.7094237280189759 ) ) ;
#19890=CARTESIAN_POINT ( 'NONE',  ( -13.97604488694527625, -13.89961937509977652, 21.87390960531435979 ) ) ;
#19891=CARTESIAN_POINT ( 'NONE',  ( 10.81492255796106328, -18.62759615963255655, 85.41775706135236135 ) ) ;
#19892=CARTESIAN_POINT ( 'NONE',  ( 16.51473224551069308, 9.474510206698969483, 69.16557627198102409 ) ) ;
#19893=CARTESIAN_POINT ( 'NONE',  ( 18.62759615963255655, 10.81492255796105972, 36.66775706135234714 ) ) ;
#19894=CARTESIAN_POINT ( 'NONE',  ( 21.55341960407619695, -5.719274019375665929, 26.04275706135235779 ) ) ;
#19896=CARTESIAN_POINT ( 'NONE',  ( -9.474510206698964154, 16.51473224551069663, 80.41557627198103830 ) ) ;
#19898=CARTESIAN_POINT ( 'NONE',  ( 16.53943276465976808, 0.05219959533934440121, 21.25109039468567218 ) ) ;
#19899=CARTESIAN_POINT ( 'NONE',  ( 15.72974639402199770, -15.80617190586745480, 48.12390960531436690 ) ) ;
#19900=CARTESIAN_POINT ( 'NONE',  ( -5.823673210054431948, 21.52544592524334988, 57.70942372801901143 ) ) ;
#19901=CARTESIAN_POINT ( 'NONE',  ( 19.03943276465977164, -0.05219959533909143690, 103.7489096053143669 ) ) ;
#19902=CARTESIAN_POINT ( 'NONE',  ( -13.89961937509957401, -13.97604488694547875, 94.37609039468566152 ) ) ;
#19903=CARTESIAN_POINT ( 'NONE',  ( -16.46253265017160317, 9.564922557960807481, 65.83224293864769550 ) ) ;
#19904=CARTESIAN_POINT ( 'NONE',  ( -5.049401038298153566, 19.05341960407611168, 90.20724293864766707 ) ) ;
#19905=CARTESIAN_POINT ( 'NONE',  ( -4.379528057220328563, 16.55341960407611168, 95.20724293864769550 ) ) ;
#19906=CARTESIAN_POINT ( 'NONE',  ( -14.34966873604960291, -8.224510206698953496, 101.6655762719810383 ) ) ;
#19907=CARTESIAN_POINT ( 'NONE',  ( 19.03943276465977164, -0.05219959533909143690, 113.7489096053143669 ) ) ;
#19908=CARTESIAN_POINT ( 'NONE',  ( -14.34966873604960291, -8.224510206698953496, 51.66557627198102409 ) ) ;
#19909=CARTESIAN_POINT ( 'NONE',  ( 13.89961937509977652, -13.97604488694527269, 43.12390960531434558 ) ) ;
#19910=CARTESIAN_POINT ( 'NONE',  ( 21.52544592524334988, 5.823673210054432836, 76.45942372801901854 ) ) ;
#19911=CARTESIAN_POINT ( 'NONE',  ( -0.05219959533936034679, 19.03943276465977164, 87.50109039468567573 ) ) ;
#19912=CARTESIAN_POINT ( 'NONE',  ( 14.34966873604960469, 8.224510206698951720, 59.16557627198103120 ) ) ;
#19913=CARTESIAN_POINT ( 'NONE',  ( -0.05219959533907301413, -21.53943276465977519, 112.4989096053143669 ) ) ;
#19914=CARTESIAN_POINT ( 'NONE',  ( 10.72451020669898902, -18.67979575497178502, 52.91557627198103830 ) ) ;
#19917=CARTESIAN_POINT ( 'NONE',  ( 5.049401038298161559, -19.05341960407611168, 67.70724293864769550 ) ) ;
#19918=CARTESIAN_POINT ( 'NONE',  ( 12.06949235617757843, -12.14591786802309237, 38.12390960531436690 ) ) ;
#19919=CARTESIAN_POINT ( 'NONE',  ( -16.53943276465976808, 0.05219959533911058130, 21.24890960531436690 ) ) ;
#19920=CARTESIAN_POINT ( 'NONE',  ( -0.05219959533934338120, 16.53943276465976808, 87.50109039468568994 ) ) ;
#19921=CARTESIAN_POINT ( 'NONE',  ( 19.02544592524334988, 5.153800228976608722, 36.45942372801900433 ) ) ;
#19923=CARTESIAN_POINT ( 'NONE',  ( 0.05219959533909260263, 19.03943276465977164, 89.99890960531436690 ) ) ;
#19924=CARTESIAN_POINT ( 'NONE',  ( -19.03943276465977164, 0.05219959533909376836, 51.24890960531436690 ) ) ;
#19926=CARTESIAN_POINT ( 'NONE',  ( 12.06949235617757843, -12.14591786802309237, 58.12390960531435979 ) ) ;
#19927=CARTESIAN_POINT ( 'NONE',  ( -5.049401038298153566, 19.05341960407611168, 25.20724293864768484 ) ) ;
#19928=CARTESIAN_POINT ( 'NONE',  ( 10.72451020669898902, -18.67979575497178502, 22.91557627198102765 ) ) ;
#19929=CARTESIAN_POINT ( 'NONE',  ( -15.72974639402197994, 15.80617190586746368, 60.62390960531437401 ) ) ;
#19930=CARTESIAN_POINT ( 'NONE',  ( 14.34966873604960469, 8.224510206698951720, 89.16557627198102409 ) ) ;
#19931=CARTESIAN_POINT ( 'NONE',  ( -4.483927247898782831, 16.52544592524335698, 37.70942372801900433 ) ) ;
#19932=CARTESIAN_POINT ( 'NONE',  ( 8.224510206698953496, -14.34966873604960469, 77.91557627198102409 ) ) ;
#19933=CARTESIAN_POINT ( 'NONE',  ( -19.25663599770061296, 5.499999999999451994, 63.99419308057201050 ) ) ;
#19934=CARTESIAN_POINT ( 'NONE',  ( -13.89961937509957401, -13.97604488694547875, 74.37609039468566152 ) ) ;
#19935=CARTESIAN_POINT ( 'NONE',  ( -9.564922557960796823, -16.46253265017161027, 112.0822429386476955 ) ) ;
#19939=CARTESIAN_POINT ( 'NONE',  ( 4.483927247898790824, -16.52544592524335698, 35.20942372801901854 ) ) ;
#19940=CARTESIAN_POINT ( 'NONE',  ( 16.52544592524335698, 4.483927247898782831, 106.4594237280190328 ) ) ;
#19941=CARTESIAN_POINT ( 'NONE',  ( 5.153800228976615827, -19.02544592524334988, 75.20942372801896170 ) ) ;
#19942=CARTESIAN_POINT ( 'NONE',  ( 15.72974639402199770, -15.80617190586745480, 53.12390960531436690 ) ) ;
#19943=CARTESIAN_POINT ( 'NONE',  ( -10.81492255796105439, 18.62759615963255655, 72.91775706135234714 ) ) ;
#19944=CARTESIAN_POINT ( 'NONE',  ( -15.49999999999999822, -5.500000000000000888, 120.0000000000000142 ) ) ;
#19945=CARTESIAN_POINT ( 'NONE',  ( -16.53943276465976808, -0.05219959533934237506, 33.75109039468568284 ) ) ;
#19946=CARTESIAN_POINT ( 'NONE',  ( 13.97604488694527802, 13.89961937509977652, 24.37390960531435624 ) ) ;
#19947=CARTESIAN_POINT ( 'NONE',  ( -5.153800228976328057, -19.02544592524343514, 87.29057627198103830 ) ) ;
#19949=CARTESIAN_POINT ( 'NONE',  ( -16.53943276465976808, 0.05219959533911058130, 101.2489096053143669 ) ) ;
#19950=CARTESIAN_POINT ( 'NONE',  ( 5.049401038298161559, -19.05341960407611168, 102.7072429386476955 ) ) ;
#19951=ORIENTED_EDGE ( 'NONE', *, *, #121376, .T. ) ;
#19952=CARTESIAN_POINT ( 'NONE',  ( 8.224510206698742110, 14.34966873604972548, 57.08442372801901854 ) ) ;
#19953=CARTESIAN_POINT ( 'NONE',  ( 19.02544592524334988, 5.153800228976608722, 106.4594237280190185 ) ) ;
#19954=CARTESIAN_POINT ( 'NONE',  ( 15.72974639402199770, -15.80617190586745480, 78.12390960531436690 ) ) ;
#19955=CARTESIAN_POINT ( 'NONE',  ( 9.474510206698971260, -16.51473224551069308, 37.91557627198102409 ) ) ;
#19956=CARTESIAN_POINT ( 'NONE',  ( -5.153800228976607833, 19.02544592524334988, 67.70942372801900433 ) ) ;
#19957=CARTESIAN_POINT ( 'NONE',  ( 0.05219959533907565091, 21.53943276465977519, 109.9989096053143527 ) ) ;
#19958=CARTESIAN_POINT ( 'NONE',  ( 16.46253265017160672, -9.564922557960803928, 68.33224293864770971 ) ) ;
#19959=CARTESIAN_POINT ( 'NONE',  ( 9.474510206698971260, -16.51473224551069308, 102.9155762719810241 ) ) ;
#19961=CARTESIAN_POINT ( 'NONE',  ( -4.379528057220086978, -16.55341960407618274, 29.79275706135234358 ) ) ;
#19962=CARTESIAN_POINT ( 'NONE',  ( -15.72974639402197994, 15.80617190586746368, 105.6239096053143669 ) ) ;
#19963=CARTESIAN_POINT ( 'NONE',  ( 0.05219959533910956823, 16.53943276465976808, 104.9989096053143669 ) ) ;
#19964=CARTESIAN_POINT ( 'NONE',  ( 13.97604488694527802, 13.89961937509977652, 94.37390960531436690 ) ) ;
#19965=CARTESIAN_POINT ( 'NONE',  ( -19.02544592524334988, -5.153800228976617603, 78.95942372801900433 ) ) ;
#19966=CARTESIAN_POINT ( 'NONE',  ( -0.05219959533907301413, -21.53943276465977519, 92.49890960531436690 ) ) ;
#19967=CARTESIAN_POINT ( 'NONE',  ( -14.29746914071049879, 8.314922557960819915, 45.83224293864769550 ) ) ;
#19968=CARTESIAN_POINT ( 'NONE',  ( -16.46253265017146816, -9.564922557961047289, 24.16775706135233648 ) ) ;
#19969=CARTESIAN_POINT ( 'NONE',  ( 16.52544592524335698, 4.483927247898782831, 61.45942372801901854 ) ) ;
#19970=CARTESIAN_POINT ( 'NONE',  ( 0.05219959533909260263, 19.03943276465977164, 89.99890960531436690 ) ) ;
#19971=CARTESIAN_POINT ( 'NONE',  ( -16.51473224551069308, -9.474510206698971260, 46.66557627198102409 ) ) ;
#19972=CARTESIAN_POINT ( 'NONE',  ( -15.80617190586768217, 15.72974639402176855, 53.12609039468568284 ) ) ;
#19973=CARTESIAN_POINT ( 'NONE',  ( -5.719274019375665041, -21.55341960407619695, 69.79275706135234714 ) ) ;
#19974=CARTESIAN_POINT ( 'NONE',  ( -19.05341960407611168, -5.049401038298163336, 56.45724293864768129 ) ) ;
#19975=CARTESIAN_POINT ( 'NONE',  ( -21.52544592524334988, -5.823673210054445271, 38.95942372801901854 ) ) ;
#19976=CARTESIAN_POINT ( 'NONE',  ( -19.02544592524334988, -5.153800228976617603, 68.95942372801896170 ) ) ;
#19977=CARTESIAN_POINT ( 'NONE',  ( -0.05219959533909027116, -19.03943276465977164, 37.49890960531436690 ) ) ;
#19978=CARTESIAN_POINT ( 'NONE',  ( -0.05219959533934338120, 16.53943276465976808, 82.50109039468568994 ) ) ;
#19979=CARTESIAN_POINT ( 'NONE',  ( -13.89961937509977652, 13.97604488694528158, 55.62390960531434558 ) ) ;
#19980=CARTESIAN_POINT ( 'NONE',  ( -13.97604488694527625, -13.89961937509977652, 106.8739096053143669 ) ) ;
#19981=CARTESIAN_POINT ( 'NONE',  ( 5.049401038298161559, -19.05341960407611168, 42.70724293864767418 ) ) ;
#19982=CARTESIAN_POINT ( 'NONE',  ( 21.53943276465977519, -0.05219959533907433946, 88.74890960531436690 ) ) ;
#19983=CARTESIAN_POINT ( 'NONE',  ( -8.314922557961024197, 14.29746914071037800, 67.91775706135234714 ) ) ;
#19985=CARTESIAN_POINT ( 'NONE',  ( 5.153800228976615827, -19.02544592524334988, 35.20942372801899722 ) ) ;
#19986=CARTESIAN_POINT ( 'NONE',  ( 19.02544592524343514, -5.153800228976328945, 58.54057627198102409 ) ) ;
#19987=CARTESIAN_POINT ( 'NONE',  ( -8.224510206698948167, 14.34966873604960824, 40.41557627198103120 ) ) ;
#19988=CARTESIAN_POINT ( 'NONE',  ( -16.53943276465976808, 0.05219959533911058130, 86.24890960531436690 ) ) ;
#19989=CARTESIAN_POINT ( 'NONE',  ( -13.89961937509977652, 13.97604488694528158, 100.6239096053143669 ) ) ;
#19990=CARTESIAN_POINT ( 'NONE',  ( 9.564922557960805705, 16.46253265017160317, 89.58224293864769550 ) ) ;
#19991=CARTESIAN_POINT ( 'NONE',  ( -0.05219959533937732626, 21.53943276465977519, 52.50109039468567573 ) ) ;
#19992=CARTESIAN_POINT ( 'NONE',  ( -19.05341960407611168, -5.049401038298163336, 96.45724293864769550 ) ) ;
#19993=CARTESIAN_POINT ( 'NONE',  ( 18.67979575497194134, -10.72451020669871369, 95.83442372801903275 ) ) ;
#19994=CARTESIAN_POINT ( 'NONE',  ( -0.05219959533934338120, 16.53943276465976808, 82.50109039468568994 ) ) ;
#19995=CARTESIAN_POINT ( 'NONE',  ( 5.823673210054444382, -21.52544592524334988, 30.20942372801902565 ) ) ;
#19996=CARTESIAN_POINT ( 'NONE',  ( 5.823673210054125526, 21.52544592524343514, 99.79057627198103830 ) ) ;
#19997=CARTESIAN_POINT ( 'NONE',  ( 12.14591786802309770, 12.06949235617756955, 59.37390960531436690 ) ) ;
#19998=CARTESIAN_POINT ( 'NONE',  ( -19.02544592524342804, 5.153800228976336051, 46.04057627198101699 ) ) ;
#19999=CARTESIAN_POINT ( 'NONE',  ( 14.29746914071049879, -8.314922557960816363, 73.33224293864769550 ) ) ;
#20000=B_SPLINE_CURVE_WITH_KNOTS ( 'NONE', 3,
 ( #14381, #27600, #136728, #196451, #167087, #59887, #135758, #121553, #57921, #12425, #30549, #122547, #92201, #184237, #153885, #15382, #191, #168067, #74088, #120561, #198410, #58895 ),
 .UNSPECIFIED., .F., .F.,
 ( 4, 2, 2, 2, 2, 2, 2, 2, 2, 2, 4 ),
 ( 8.673617379884035472E-19, 0.001309639967555435757, 0.001964459951333159381, 0.002291869943222021953, 0.002455574939166439794, 0.002619279935110857202, 0.002782984931055275044, 0.002946689926999692885, 0.003274099918888501246, 0.003928919902666100188, 0.005238559870221296336 ),
 .UNSPECIFIED. ) ;
#20001=CARTESIAN_POINT ( 'NONE',  ( -10.72451020669898014, 18.67979575497178502, 25.41557627198103120 ) ) ;
#20002=CARTESIAN_POINT ( 'NONE',  ( -13.89961937509957401, -13.97604488694547875, 34.37609039468566863 ) ) ;
#20003=CARTESIAN_POINT ( 'NONE',  ( 0.05219959533910956823, 16.53943276465976808, 114.9989096053143669 ) ) ;
#20005=CARTESIAN_POINT ( 'NONE',  ( 8.224510206698742110, 14.34966873604972548, 62.08442372801901143 ) ) ;
#20006=CARTESIAN_POINT ( 'NONE',  ( 19.05341960407611168, 5.049401038298154454, 63.95724293864769550 ) ) ;
#20007=CARTESIAN_POINT ( 'NONE',  ( -16.93440711220026884, -5.601562513631294316, 20.60331890504276942 ) ) ;
#20008=CARTESIAN_POINT ( 'NONE',  ( 14.34966873604960469, 8.224510206698951720, 94.16557627198103830 ) ) ;
#20009=CARTESIAN_POINT ( 'NONE',  ( 5.719274019375991003, -21.55341960407610458, 32.70724293864770260 ) ) ;
#20010=EDGE_LOOP ( 'NONE', ( #136354, #26591, #168948, #151907 ) ) ;
#20011=CARTESIAN_POINT ( 'NONE',  ( -4.483927247898782831, 16.52544592524335698, 102.7094237280190185 ) ) ;
#20012=CARTESIAN_POINT ( 'NONE',  ( -16.51473224551082808, 9.474510206698731452, 108.3344237280190043 ) ) ;
#20013=CARTESIAN_POINT ( 'NONE',  ( -15.72974639402176322, -15.80617190586768395, 74.37609039468568994 ) ) ;
#20014=CARTESIAN_POINT ( 'NONE',  ( 16.51473224551069308, 9.474510206698969483, 94.16557627198103830 ) ) ;
#20015=CARTESIAN_POINT ( 'NONE',  ( 15.80617190586746368, 15.72974639402197994, 109.3739096053143811 ) ) ;
#20016=CARTESIAN_POINT ( 'NONE',  ( 14.34966873604972726, -8.224510206698740333, 55.83442372801901854 ) ) ;
#20017=CARTESIAN_POINT ( 'NONE',  ( 19.02544592524343514, -5.153800228976328945, 28.54057627198102409 ) ) ;
#20018=CARTESIAN_POINT ( 'NONE',  ( 14.34966873604972726, -8.224510206698740333, 20.83442372801901143 ) ) ;
#20019=CARTESIAN_POINT ( 'NONE',  ( -9.564922557961040184, 16.46253265017147172, 97.91775706135233293 ) ) ;
#20020=EDGE_CURVE ( 'NONE', #40349, #175270, #101863, .T. ) ;
#20021=CARTESIAN_POINT ( 'NONE',  ( -21.55341960407610458, -5.719274019375992779, 86.45724293864770971 ) ) ;
#20022=CARTESIAN_POINT ( 'NONE',  ( -19.02544592524334988, -5.153800228976617603, 58.95942372801900433 ) ) ;
#20023=CARTESIAN_POINT ( 'NONE',  ( 19.48894818550246200, -5.499999999999907629, 87.60307310435239003 ) ) ;
#20024=CARTESIAN_POINT ( 'NONE',  ( -15.72974639402197994, 15.80617190586746368, 100.6239096053143811 ) ) ;
#20026=CARTESIAN_POINT ( 'NONE',  ( 13.97604488694527802, 13.89961937509977652, 84.37390960531433848 ) ) ;
#20028=CARTESIAN_POINT ( 'NONE',  ( 12.14591786802327356, -12.06949235617739191, 30.62609039468567929 ) ) ;
#20030=CARTESIAN_POINT ( 'NONE',  ( -15.72974639402197994, 15.80617190586746368, 110.6239096053143669 ) ) ;
#20031=CARTESIAN_POINT ( 'NONE',  ( -16.52544592524342804, 4.483927247898546575, 61.04057627198103120 ) ) ;
#20032=CARTESIAN_POINT ( 'NONE',  ( 0.05219959533909260263, 19.03943276465977164, 74.99890960531435269 ) ) ;
#20033=CARTESIAN_POINT ( 'NONE',  ( 4.483927247898790824, -16.52544592524335698, 40.20942372801901854 ) ) ;
#20034=CARTESIAN_POINT ( 'NONE',  ( -19.05341960407617563, 5.049401038297882671, 43.54275706135232582 ) ) ;
#20035=CARTESIAN_POINT ( 'NONE',  ( 21.53943276465977519, 0.05219959533937863772, 51.25109039468568994 ) ) ;
#20036=CARTESIAN_POINT ( 'NONE',  ( -19.03943276465977164, -0.05219959533935918106, 103.7510903946856757 ) ) ;
#20037=CARTESIAN_POINT ( 'NONE',  ( 16.46253265017160672, -9.564922557960803928, 53.33224293864768839 ) ) ;
#20038=CARTESIAN_POINT ( 'NONE',  ( 13.97604488694548053, -13.89961937509957401, 85.62609039468568994 ) ) ;
#20039=CARTESIAN_POINT ( 'NONE',  ( 5.823673210054444382, -21.52544592524334988, 80.20942372801901854 ) ) ;
#20040=CARTESIAN_POINT ( 'NONE',  ( 9.564922557961047289, -16.46253265017146816, 60.41775706135233293 ) ) ;
#20041=CARTESIAN_POINT ( 'NONE',  ( 0.05219959533909260263, 19.03943276465977164, 34.99890960531435979 ) ) ;
#20042=CARTESIAN_POINT ( 'NONE',  ( 15.72974639402199770, -15.80617190586745480, 53.12390960531436690 ) ) ;
#20043=CARTESIAN_POINT ( 'NONE',  ( -4.379528057220328563, 16.55341960407611168, 65.20724293864768129 ) ) ;
#20044=CARTESIAN_POINT ( 'NONE',  ( -17.49999999999999645, -5.500000000000000888, 24.20309617465829533 ) ) ;
#20045=CARTESIAN_POINT ( 'NONE',  ( -0.05219959533936034679, 19.03943276465977164, 32.50109039468566863 ) ) ;
#20046=CARTESIAN_POINT ( 'NONE',  ( 8.224510206698742110, 14.34966873604972548, 102.0844237280190185 ) ) ;
#20047=CARTESIAN_POINT ( 'NONE',  ( -8.314922557960811034, -14.29746914071050412, 47.08224293864770260 ) ) ;
#20048=CARTESIAN_POINT ( 'NONE',  ( -0.05219959533937732626, 21.53943276465977519, 87.50109039468568994 ) ) ;
#20049=CARTESIAN_POINT ( 'NONE',  ( -18.62759615963255300, -10.81492255796106328, 79.16775706135234714 ) ) ;
#20050=CARTESIAN_POINT ( 'NONE',  ( 21.52544592524344225, -5.823673210054117533, 98.54057627198105251 ) ) ;
#20051=CARTESIAN_POINT ( 'NONE',  ( 13.89961937509977652, -13.97604488694527269, 53.12390960531434558 ) ) ;
#20052=CARTESIAN_POINT ( 'NONE',  ( -0.05219959533937732626, 21.53943276465977519, 67.50109039468568994 ) ) ;
#20053=CARTESIAN_POINT ( 'NONE',  ( -16.46253265017160317, 9.564922557960807481, 45.83224293864769550 ) ) ;
#20054=CARTESIAN_POINT ( 'NONE',  ( 9.474510206698971260, -16.51473224551069308, 62.91557627198102409 ) ) ;
#20055=CARTESIAN_POINT ( 'NONE',  ( -16.53943276465976808, 0.05219959533911058130, 101.2489096053143669 ) ) ;
#20056=CARTESIAN_POINT ( 'NONE',  ( -0.05219959533907301413, -21.53943276465977519, 22.49890960531436335 ) ) ;
#20057=CARTESIAN_POINT ( 'NONE',  ( -0.05219959533910754901, -16.53943276465976808, 47.49890960531435979 ) ) ;
#20058=CARTESIAN_POINT ( 'NONE',  ( 4.379528057220339221, -16.55341960407611168, 107.7072429386476955 ) ) ;
#20059=CARTESIAN_POINT ( 'NONE',  ( -4.483927247898539470, -16.52544592524342804, 72.29057627198102409 ) ) ;
#20060=CARTESIAN_POINT ( 'NONE',  ( -21.55341960407610458, -5.719274019375992779, 86.45724293864770971 ) ) ;
#20061=CARTESIAN_POINT ( 'NONE',  ( -21.53943276465977519, -0.05219959533937600094, 38.75109039468567573 ) ) ;
#20063=CARTESIAN_POINT ( 'NONE',  ( 14.34966873604972726, -8.224510206698740333, 30.83442372801902209 ) ) ;
#20064=CARTESIAN_POINT ( 'NONE',  ( -10.81492255796078084, -18.62759615963271287, 87.08224293864769550 ) ) ;
#20066=CARTESIAN_POINT ( 'NONE',  ( -15.80617190586768217, 15.72974639402176855, 103.1260903946856757 ) ) ;
#20067=CARTESIAN_POINT ( 'NONE',  ( 5.049401038298161559, -19.05341960407611168, 97.70724293864766707 ) ) ;
#20068=CARTESIAN_POINT ( 'NONE',  ( -21.55341960407619339, 5.719274019375674811, 43.54275706135235424 ) ) ;
#20069=CARTESIAN_POINT ( 'NONE',  ( 5.823673210054125526, 21.52544592524343514, 24.79057627198103120 ) ) ;
#20070=CARTESIAN_POINT ( 'NONE',  ( -8.224510206698735004, -14.34966873604973081, 109.5844237280190328 ) ) ;
#20071=CARTESIAN_POINT ( 'NONE',  ( 21.53943276465977519, 0.05219959533937863772, 51.25109039468568994 ) ) ;
#20072=CARTESIAN_POINT ( 'NONE',  ( 18.62759615963255655, 10.81492255796105972, 86.66775706135234714 ) ) ;
#20073=CARTESIAN_POINT ( 'NONE',  ( -19.03943276465977164, -0.05219959533935918106, 18.75109039468567218 ) ) ;
#20074=CARTESIAN_POINT ( 'NONE',  ( 8.224510206698742110, 14.34966873604972548, 72.08442372801899012 ) ) ;
#20075=CARTESIAN_POINT ( 'NONE',  ( -15.72974639402176322, -15.80617190586768395, 39.37609039468567573 ) ) ;
#20076=CARTESIAN_POINT ( 'NONE',  ( 13.97604488694527802, 13.89961937509977652, 34.37390960531436690 ) ) ;
#20077=CARTESIAN_POINT ( 'NONE',  ( 18.67979575497194134, -10.72451020669871369, 100.8344237280190185 ) ) ;
#20078=CARTESIAN_POINT ( 'NONE',  ( -5.153800228976328057, -19.02544592524343514, 102.2905762719810383 ) ) ;
#20079=CARTESIAN_POINT ( 'NONE',  ( 18.62759615963271287, -10.81492255796078972, 98.33224293864769550 ) ) ;
#20080=CARTESIAN_POINT ( 'NONE',  ( 19.53091890409950793, 5.500000000000031974, 82.56097431831419442 ) ) ;
#20081=CARTESIAN_POINT ( 'NONE',  ( -15.80617190586745835, -15.72974639402198527, 61.87390960531436690 ) ) ;
#20082=CARTESIAN_POINT ( 'NONE',  ( -8.314922557961024197, 14.29746914071037800, 47.91775706135234714 ) ) ;
#20083=CARTESIAN_POINT ( 'NONE',  ( 12.14591786802309770, 12.06949235617756955, 44.37390960531435979 ) ) ;
#20084=CARTESIAN_POINT ( 'NONE',  ( 19.43099193148530190, -5.499999999999960032, 101.7672081453054886 ) ) ;
#20085=CARTESIAN_POINT ( 'NONE',  ( -5.153800228976607833, 19.02544592524334988, 87.70942372801897591 ) ) ;
#20087=EDGE_CURVE ( 'NONE', #148926, #24966, #25159, .T. ) ;
#20088=CARTESIAN_POINT ( 'NONE',  ( 0.05219959533934541429, -16.53943276465976808, 30.00109039468568284 ) ) ;
#20089=CARTESIAN_POINT ( 'NONE',  ( -10.81492255796078084, -18.62759615963271287, 97.08224293864770971 ) ) ;
#20090=CARTESIAN_POINT ( 'NONE',  ( -10.81492255796078084, -18.62759615963271287, 72.08224293864769550 ) ) ;
#20091=CARTESIAN_POINT ( 'NONE',  ( -16.46253265017160317, 9.564922557960807481, 115.8322429386477097 ) ) ;
#20092=CARTESIAN_POINT ( 'NONE',  ( 4.379528057220092307, 16.55341960407617563, 42.29275706135235424 ) ) ;
#20093=CARTESIAN_POINT ( 'NONE',  ( -13.89961937509977652, 13.97604488694528158, 75.62390960531438111 ) ) ;
#20094=CARTESIAN_POINT ( 'NONE',  ( 18.67979575497194134, -10.72451020669871369, 30.83442372801902209 ) ) ;
#20095=CARTESIAN_POINT ( 'NONE',  ( 19.03943276465977164, 0.05219959533936151252, 96.25109039468567573 ) ) ;
#20096=CARTESIAN_POINT ( 'NONE',  ( 19.02544592524343514, -5.153800228976328945, 108.5405762719810383 ) ) ;
#20097=CARTESIAN_POINT ( 'NONE',  ( 19.02544592524343514, -5.153800228976328945, 83.54057627198100988 ) ) ;
#20098=CARTESIAN_POINT ( 'NONE',  ( -15.72974639402197994, 15.80617190586746368, 90.62390960531436690 ) ) ;
#20099=CARTESIAN_POINT ( 'NONE',  ( 19.05341960407611168, 5.049401038298154454, 58.95724293864768129 ) ) ;
#20101=CARTESIAN_POINT ( 'NONE',  ( 4.379528057220339221, -16.55341960407611168, 62.70724293864769550 ) ) ;
#20102=CARTESIAN_POINT ( 'NONE',  ( 19.02544592524343514, -5.153800228976328945, 113.5405762719810241 ) ) ;
#20104=CARTESIAN_POINT ( 'NONE',  ( -5.719274019375978568, 21.55341960407610458, 95.20724293864769550 ) ) ;
#20105=CARTESIAN_POINT ( 'NONE',  ( -5.153800228976607833, 19.02544592524334988, 67.70942372801900433 ) ) ;
#20106=CARTESIAN_POINT ( 'NONE',  ( -19.02544592524342804, 5.153800228976336051, 116.0405762719810383 ) ) ;
#20107=CARTESIAN_POINT ( 'NONE',  ( 19.34837522270367671, 5.499999999999740652, 68.36337684832577111 ) ) ;
#20108=CARTESIAN_POINT ( 'NONE',  ( -21.55341960407610458, -5.719274019375992779, 51.45724293864770260 ) ) ;
#20109=CARTESIAN_POINT ( 'NONE',  ( 16.51473224551069308, 9.474510206698969483, 84.16557627198102409 ) ) ;
#20110=CARTESIAN_POINT ( 'NONE',  ( -21.55341960407619339, 5.719274019375674811, 83.54275706135234714 ) ) ;
#20111=CARTESIAN_POINT ( 'NONE',  ( 0.05219959533909260263, 19.03943276465977164, 54.99890960531435979 ) ) ;
#20112=EDGE_CURVE ( 'NONE', #165180, #69839, #178948, .T. ) ;
#20113=CARTESIAN_POINT ( 'NONE',  ( -8.314922557960811034, -14.29746914071050412, 87.08224293864769550 ) ) ;
#20114=CARTESIAN_POINT ( 'NONE',  ( -12.14591786802326823, 12.06949235617739902, 33.12609039468569705 ) ) ;
#20115=CARTESIAN_POINT ( 'NONE',  ( 21.55341960407619695, -5.719274019375665929, 66.04275706135236135 ) ) ;
#20117=CARTESIAN_POINT ( 'NONE',  ( 5.153800228976615827, -19.02544592524334988, 20.20942372801899722 ) ) ;
#20118=CARTESIAN_POINT ( 'NONE',  ( -16.46253265017146816, -9.564922557961047289, 79.16775706135234714 ) ) ;
#20120=CARTESIAN_POINT ( 'NONE',  ( -0.05219959533937732626, 21.53943276465977519, 42.50109039468567573 ) ) ;
#20122=CARTESIAN_POINT ( 'NONE',  ( -0.05219959533936034679, 19.03943276465977164, 37.50109039468567573 ) ) ;
#20123=CARTESIAN_POINT ( 'NONE',  ( 19.03943276465977164, -0.05219959533909143690, 53.74890960531436690 ) ) ;
#20124=CARTESIAN_POINT ( 'NONE',  ( 16.46253265017146816, 9.564922557961045513, 36.66775706135233293 ) ) ;
#20125=CARTESIAN_POINT ( 'NONE',  ( -14.34966873604972548, 8.224510206698743886, 103.3344237280190043 ) ) ;
#20126=CARTESIAN_POINT ( 'NONE',  ( -0.05219959533909027116, -19.03943276465977164, 102.4989096053143669 ) ) ;
#20127=CARTESIAN_POINT ( 'NONE',  ( 15.80617190586769283, -15.72974639402175789, 70.62609039468567573 ) ) ;
#20129=CARTESIAN_POINT ( 'NONE',  ( -17.97182807773873137, 5.499999999999966249, 98.53038844047286204 ) ) ;
#20130=CARTESIAN_POINT ( 'NONE',  ( 15.72974639402176855, 15.80617190586768217, 86.87609039468568994 ) ) ;
#20132=CARTESIAN_POINT ( 'NONE',  ( -5.153800228976328057, -19.02544592524343514, 102.2905762719810383 ) ) ;
#20133=CARTESIAN_POINT ( 'NONE',  ( 5.153800228976615827, -19.02544592524334988, 20.20942372801899722 ) ) ;
#20135=CARTESIAN_POINT ( 'NONE',  ( -9.564922557960796823, -16.46253265017161027, 37.08224293864768839 ) ) ;
#20136=CARTESIAN_POINT ( 'NONE',  ( -10.72451020669898014, 18.67979575497178502, 60.41557627198102409 ) ) ;
#20137=CARTESIAN_POINT ( 'NONE',  ( -14.29746914071049879, 8.314922557960819915, 25.83224293864769194 ) ) ;
#20138=CARTESIAN_POINT ( 'NONE',  ( -16.52544592524342804, 4.483927247898546575, 101.0405762719810383 ) ) ;
#20139=CARTESIAN_POINT ( 'NONE',  ( -5.049401038298153566, 19.05341960407611168, 80.20724293864769550 ) ) ;
#20140=CARTESIAN_POINT ( 'NONE',  ( -13.97604488694547697, 13.89961937509957934, 28.12609039468565797 ) ) ;
#20141=CARTESIAN_POINT ( 'NONE',  ( 13.97604488694527802, 13.89961937509977652, 39.37390960531435269 ) ) ;
#20142=CARTESIAN_POINT ( 'NONE',  ( 4.379528057220339221, -16.55341960407611168, 102.7072429386476955 ) ) ;
#20143=CARTESIAN_POINT ( 'NONE',  ( 18.62759615963255655, 10.81492255796105972, 51.66775706135234714 ) ) ;
#20144=CARTESIAN_POINT ( 'NONE',  ( 15.80617190586746368, 15.72974639402197994, 89.37390960531435269 ) ) ;
#20145=CARTESIAN_POINT ( 'NONE',  ( 13.97604488694548053, -13.89961937509957401, 70.62609039468567573 ) ) ;
#20146=FACE_OUTER_BOUND ( 'NONE', #121604, .T. ) ;
#20147=CARTESIAN_POINT ( 'NONE',  ( -13.97604488694527625, -13.89961937509977652, 106.8739096053143669 ) ) ;
#20148=CARTESIAN_POINT ( 'NONE',  ( 12.14591786802309770, 12.06949235617756955, 79.37390960531436690 ) ) ;
#20149=CARTESIAN_POINT ( 'NONE',  ( 16.46253265017146816, 9.564922557961045513, 46.66775706135233293 ) ) ;
#20150=CARTESIAN_POINT ( 'NONE',  ( 13.89961937509977652, -13.97604488694527269, 63.12390960531435979 ) ) ;
#20151=CARTESIAN_POINT ( 'NONE',  ( -14.29746914071049879, 8.314922557960819915, 60.83224293864769550 ) ) ;
#20152=CARTESIAN_POINT ( 'NONE',  ( -16.46253265017146816, -9.564922557961047289, 74.16775706135234714 ) ) ;
#20153=CARTESIAN_POINT ( 'NONE',  ( 17.31747979337948706, 6.344076630961010821, 33.87944868065184068 ) ) ;
#20154=CARTESIAN_POINT ( 'NONE',  ( 5.823673210054125526, 21.52544592524343514, 39.79057627198103830 ) ) ;
#20156=CARTESIAN_POINT ( 'NONE',  ( 14.34966873604960469, 8.224510206698951720, 104.1655762719810241 ) ) ;
#20157=CARTESIAN_POINT ( 'NONE',  ( -17.50000000000001421, -3.565345528327753755, 25.57505513193517999 ) ) ;
#20158=CARTESIAN_POINT ( 'NONE',  ( 9.474510206698971260, -16.51473224551069308, 52.91557627198102409 ) ) ;
#20159=CARTESIAN_POINT ( 'NONE',  ( -21.53943276465977519, 0.05219959533907696930, 56.24890960531436690 ) ) ;
#20160=CARTESIAN_POINT ( 'NONE',  ( 19.03943276465977164, -0.05219959533909143690, 23.74890960531435269 ) ) ;
#20161=CARTESIAN_POINT ( 'NONE',  ( 4.483927247898790824, -16.52544592524335698, 85.20942372801901854 ) ) ;
#20162=CARTESIAN_POINT ( 'NONE',  ( -13.89961937509977652, 13.97604488694528158, 75.62390960531438111 ) ) ;
#20163=CARTESIAN_POINT ( 'NONE',  ( -19.03943276465977164, -0.05219959533935918106, 53.75109039468566863 ) ) ;
#20164=CARTESIAN_POINT ( 'NONE',  ( -18.67979575497193778, 10.72451020669871902, 63.33442372801900433 ) ) ;
#20165=CARTESIAN_POINT ( 'NONE',  ( 10.81492255796078972, 18.62759615963270932, 44.58224293864769550 ) ) ;
#20166=CARTESIAN_POINT ( 'NONE',  ( -19.05341960407611168, -5.049401038298163336, 26.45724293864769550 ) ) ;
#20167=CARTESIAN_POINT ( 'NONE',  ( 4.483927247898790824, -16.52544592524335698, 90.20942372801903275 ) ) ;
#20168=CARTESIAN_POINT ( 'NONE',  ( -9.564922557961040184, 16.46253265017147172, 107.9177570613523471 ) ) ;
#20170=CARTESIAN_POINT ( 'NONE',  ( -10.81492255796105439, 18.62759615963255655, 97.91775706135236135 ) ) ;
#20171=ORIENTED_EDGE ( 'NONE', *, *, #132474, .T. ) ;
#20172=CARTESIAN_POINT ( 'NONE',  ( -8.224510206698948167, 14.34966873604960824, 40.41557627198103120 ) ) ;
#20173=CARTESIAN_POINT ( 'NONE',  ( -16.52544592524342804, 4.483927247898546575, 71.04057627198103830 ) ) ;
#20174=CARTESIAN_POINT ( 'NONE',  ( -5.719274019375978568, 21.55341960407610458, 95.20724293864769550 ) ) ;
#20175=CARTESIAN_POINT ( 'NONE',  ( -5.719274019375978568, 21.55341960407610458, 95.20724293864769550 ) ) ;
#20177=CARTESIAN_POINT ( 'NONE',  ( -5.823673210054116645, -21.52544592524344225, 27.29057627198103120 ) ) ;
#20178=CARTESIAN_POINT ( 'NONE',  ( -12.14591786802326823, 12.06949235617739902, 63.12609039468568994 ) ) ;
#20179=CARTESIAN_POINT ( 'NONE',  ( 0.05219959533910956823, 16.53943276465976808, 74.99890960531435269 ) ) ;
#20180=CARTESIAN_POINT ( 'NONE',  ( -9.564922557960796823, -16.46253265017161027, 52.08224293864768839 ) ) ;
#20182=CARTESIAN_POINT ( 'NONE',  ( -8.224510206698735004, -14.34966873604973081, 94.58442372801901854 ) ) ;
#20183=CARTESIAN_POINT ( 'NONE',  ( -18.67979575497193778, 10.72451020669871902, 23.33442372801901499 ) ) ;
#20184=CARTESIAN_POINT ( 'NONE',  ( 16.46253265017160672, -9.564922557960803928, 78.33224293864769550 ) ) ;
#20185=CARTESIAN_POINT ( 'NONE',  ( 15.80617190586769283, -15.72974639402175789, 55.62609039468568284 ) ) ;
#20186=CARTESIAN_POINT ( 'NONE',  ( 13.97604488694527802, 13.89961937509977652, 104.3739096053143385 ) ) ;
#20189=CARTESIAN_POINT ( 'NONE',  ( -5.719274019375665041, -21.55341960407619695, 49.79275706135234714 ) ) ;
#20190=CARTESIAN_POINT ( 'NONE',  ( -16.51473224551069308, -9.474510206698971260, 31.66557627198102054 ) ) ;
#20192=CARTESIAN_POINT ( 'NONE',  ( -19.03943276465977164, -0.05219959533935918106, 53.75109039468566863 ) ) ;
#20193=CARTESIAN_POINT ( 'NONE',  ( 15.80617190586769283, -15.72974639402175789, 25.62609039468567929 ) ) ;
#20194=CARTESIAN_POINT ( 'NONE',  ( 9.474510206698729675, 16.51473224551082808, 57.08442372801900433 ) ) ;
#20195=CARTESIAN_POINT ( 'NONE',  ( 9.474510206698971260, -16.51473224551069308, 22.91557627198102765 ) ) ;
#20196=CARTESIAN_POINT ( 'NONE',  ( -14.29746914071037622, -8.314922557961029526, 89.16775706135236135 ) ) ;
#20197=CARTESIAN_POINT ( 'NONE',  ( -19.05341960407617563, 5.049401038297882671, 58.54275706135234003 ) ) ;
#20198=CARTESIAN_POINT ( 'NONE',  ( -12.14591786802309592, -12.06949235617757132, 26.87390960531435979 ) ) ;
#20200=ORIENTED_EDGE ( 'NONE', *, *, #149359, .F. ) ;
#20201=CARTESIAN_POINT ( 'NONE',  ( 5.153800228976335163, 19.02544592524342804, 89.79057627198102409 ) ) ;
#20202=CARTESIAN_POINT ( 'NONE',  ( -18.67979575497193778, 10.72451020669871902, 88.33442372801901854 ) ) ;
#20203=CARTESIAN_POINT ( 'NONE',  ( 10.81492255796106328, -18.62759615963255655, 110.4177570613523756 ) ) ;
#20204=CARTESIAN_POINT ( 'NONE',  ( -16.99472585857189699, -5.499999999999960032, 20.67116795353343051 ) ) ;
#20205=CARTESIAN_POINT ( 'NONE',  ( 18.67979575497194134, -10.72451020669871369, 80.83442372801901854 ) ) ;
#20206=CARTESIAN_POINT ( 'NONE',  ( -16.52544592524335698, -4.483927247898792601, 38.95942372801901854 ) ) ;
#20207=CARTESIAN_POINT ( 'NONE',  ( 19.02544592524343514, -5.153800228976328945, 73.54057627198103830 ) ) ;
#20208=CARTESIAN_POINT ( 'NONE',  ( 21.52544592524344225, -5.823673210054117533, 28.54057627198103120 ) ) ;
#20210=CARTESIAN_POINT ( 'NONE',  ( -19.03943276465977164, 0.05219959533909376836, 61.24890960531436690 ) ) ;
#20211=CARTESIAN_POINT ( 'NONE',  ( -0.05219959533910754901, -16.53943276465976808, 27.49890960531435269 ) ) ;
#20212=CARTESIAN_POINT ( 'NONE',  ( -19.53091890409952214, -5.500000000000038192, 40.06097431831420863 ) ) ;
#20213=CARTESIAN_POINT ( 'NONE',  ( -16.46253265017146816, -9.564922557961047289, 74.16775706135234714 ) ) ;
#20214=CARTESIAN_POINT ( 'NONE',  ( 13.89961937509977652, -13.97604488694527269, 103.1239096053143527 ) ) ;
#20215=CARTESIAN_POINT ( 'NONE',  ( -0.05219959533937732626, 21.53943276465977519, 102.5010903946856899 ) ) ;
#20216=CARTESIAN_POINT ( 'NONE',  ( -8.314922557960811034, -14.29746914071050412, 82.08224293864768129 ) ) ;
#20217=CARTESIAN_POINT ( 'NONE',  ( -5.823673210054116645, -21.52544592524344225, 47.29057627198103120 ) ) ;
#20218=CARTESIAN_POINT ( 'NONE',  ( 5.719274019375991003, -21.55341960407610458, 37.70724293864769550 ) ) ;
#20219=CARTESIAN_POINT ( 'NONE',  ( 16.55341960407611168, 4.379528057220329451, 98.95724293864770971 ) ) ;
#20221=CARTESIAN_POINT ( 'NONE',  ( 9.474510206698729675, 16.51473224551082808, 52.08442372801900433 ) ) ;
#20222=CARTESIAN_POINT ( 'NONE',  ( -12.06949235617756955, 12.14591786802309770, 25.62390960531435624 ) ) ;
#20223=CARTESIAN_POINT ( 'NONE',  ( -9.474510206698964154, 16.51473224551069663, 95.41557627198102409 ) ) ;
#20224=CARTESIAN_POINT ( 'NONE',  ( -0.05219959533937732626, 21.53943276465977519, 72.50109039468568994 ) ) ;
#20225=CARTESIAN_POINT ( 'NONE',  ( 18.67979575497178502, 10.72451020669898547, 59.16557627198103120 ) ) ;
#20226=CARTESIAN_POINT ( 'NONE',  ( -10.81492255796105439, 18.62759615963255655, 47.91775706135234714 ) ) ;
#20227=CARTESIAN_POINT ( 'NONE',  ( -0.05219959533907301413, -21.53943276465977519, 97.49890960531436690 ) ) ;
#20228=CARTESIAN_POINT ( 'NONE',  ( -10.81492255796105439, 18.62759615963255655, 37.91775706135235424 ) ) ;
#20229=CARTESIAN_POINT ( 'NONE',  ( -16.51473224551069308, -9.474510206698971260, 31.66557627198102054 ) ) ;
#20230=CARTESIAN_POINT ( 'NONE',  ( 5.153800228976615827, -19.02544592524334988, 70.20942372801899012 ) ) ;
#20231=CARTESIAN_POINT ( 'NONE',  ( -16.55341960407611168, -4.379528057220339221, 101.4572429386476955 ) ) ;
#20232=CARTESIAN_POINT ( 'NONE',  ( 19.03943276465977164, -0.05219959533909143690, 108.7489096053143527 ) ) ;
#20233=CARTESIAN_POINT ( 'NONE',  ( -0.05219959533910754901, -16.53943276465976808, 57.49890960531435979 ) ) ;
#20234=CARTESIAN_POINT ( 'NONE',  ( -8.314922557960811034, -14.29746914071050412, 22.08224293864769194 ) ) ;
#20235=CARTESIAN_POINT ( 'NONE',  ( -13.97604488694527625, -13.89961937509977652, 51.87390960531436690 ) ) ;
#20236=CARTESIAN_POINT ( 'NONE',  ( -4.379528057220328563, 16.55341960407611168, 115.2072429386476955 ) ) ;
#20237=CARTESIAN_POINT ( 'NONE',  ( -10.72451020669898014, 18.67979575497178502, 35.41557627198102409 ) ) ;
#20238=CARTESIAN_POINT ( 'NONE',  ( -9.474510206698720793, -16.51473224551083518, 29.58442372801900433 ) ) ;
#20239=CARTESIAN_POINT ( 'NONE',  ( -16.79531203550648755, -7.028104445595491079, 41.25244988220442366 ) ) ;
#20240=CARTESIAN_POINT ( 'NONE',  ( -8.314922557960811034, -14.29746914071050412, 37.08224293864768129 ) ) ;
#20241=CARTESIAN_POINT ( 'NONE',  ( 18.67979575497194134, -10.72451020669871369, 40.83442372801901854 ) ) ;
#20242=CARTESIAN_POINT ( 'NONE',  ( -5.153800228976328057, -19.02544592524343514, 112.2905762719810099 ) ) ;
#20243=CARTESIAN_POINT ( 'NONE',  ( -8.224510206698735004, -14.34966873604973081, 64.58442372801900433 ) ) ;
#20244=CARTESIAN_POINT ( 'NONE',  ( -5.153800228976607833, 19.02544592524334988, 67.70942372801900433 ) ) ;
#20245=CARTESIAN_POINT ( 'NONE',  ( 8.224510206698953496, -14.34966873604960469, 32.91557627198102409 ) ) ;
#20246=CARTESIAN_POINT ( 'NONE',  ( -4.483927247898782831, 16.52544592524335698, 102.7094237280190185 ) ) ;
#20247=CARTESIAN_POINT ( 'NONE',  ( -13.89961937509977652, 13.97604488694528158, 40.62390960531435979 ) ) ;
#20249=CARTESIAN_POINT ( 'NONE',  ( 13.89961937509977652, -13.97604488694527269, 58.12390960531436690 ) ) ;
#20251=CARTESIAN_POINT ( 'NONE',  ( -19.03943276465977164, 0.05219959533909376836, 31.24890960531435979 ) ) ;
#20252=CARTESIAN_POINT ( 'NONE',  ( -18.62759615963255300, -10.81492255796106328, 34.16775706135234714 ) ) ;
#20253=CARTESIAN_POINT ( 'NONE',  ( 13.97604488694527802, 13.89961937509977652, 39.37390960531435269 ) ) ;
#20255=CARTESIAN_POINT ( 'NONE',  ( 0.05219959533909260263, 19.03943276465977164, 34.99890960531435979 ) ) ;
#20256=CARTESIAN_POINT ( 'NONE',  ( -13.97604488694527625, -13.89961937509977652, 111.8739096053143243 ) ) ;
#20257=CARTESIAN_POINT ( 'NONE',  ( -18.62759615963255300, -10.81492255796106328, 59.16775706135234714 ) ) ;
#20258=CARTESIAN_POINT ( 'NONE',  ( -16.52544592524342804, 4.483927247898546575, 101.0405762719810383 ) ) ;
#20259=CARTESIAN_POINT ( 'NONE',  ( -9.474510206698964154, 16.51473224551069663, 105.4155762719810383 ) ) ;
#20260=CARTESIAN_POINT ( 'NONE',  ( 16.53943276465976808, 0.05219959533934440121, 76.25109039468568994 ) ) ;
#20261=CARTESIAN_POINT ( 'NONE',  ( -0.05219959533937732626, 21.53943276465977519, 92.50109039468567573 ) ) ;
#20262=CARTESIAN_POINT ( 'NONE',  ( -0.05219959533934338120, 16.53943276465976808, 52.50109039468567573 ) ) ;
#20263=CARTESIAN_POINT ( 'NONE',  ( -9.564922557960796823, -16.46253265017161027, 92.08224293864769550 ) ) ;
#20264=CARTESIAN_POINT ( 'NONE',  ( 8.314922557961029526, -14.29746914071037800, 40.41775706135234714 ) ) ;
#20265=CARTESIAN_POINT ( 'NONE',  ( 14.29746914071037800, 8.314922557961029526, 21.66775706135235069 ) ) ;
#20266=CARTESIAN_POINT ( 'NONE',  ( 14.34966873604972726, -8.224510206698740333, 85.83442372801901854 ) ) ;
#20267=CARTESIAN_POINT ( 'NONE',  ( 19.03943276465977164, 0.05219959533936151252, 111.2510903946856757 ) ) ;
#20268=CARTESIAN_POINT ( 'NONE',  ( 21.53943276465977519, -0.05219959533907433946, 103.7489096053143669 ) ) ;
#20269=CARTESIAN_POINT ( 'NONE',  ( 0.05219959533910956823, 16.53943276465976808, 104.9989096053143669 ) ) ;
#20270=CARTESIAN_POINT ( 'NONE',  ( 19.05341960407617918, -5.049401038297876454, 111.0427570613523329 ) ) ;
#20271=CARTESIAN_POINT ( 'NONE',  ( 16.53943276465976808, 0.05219959533934440121, 66.25109039468567573 ) ) ;
#20272=CARTESIAN_POINT ( 'NONE',  ( -16.19135201231350507, 7.376712067592058553, 44.81319145947880145 ) ) ;
#20273=CARTESIAN_POINT ( 'NONE',  ( -19.02544592524334988, -5.153800228976617603, 73.95942372801900433 ) ) ;
#20274=CARTESIAN_POINT ( 'NONE',  ( -8.314922557960811034, -14.29746914071050412, 42.08224293864769550 ) ) ;
#20275=CARTESIAN_POINT ( 'NONE',  ( -16.55341960407611168, -4.379528057220339221, 26.45724293864768839 ) ) ;
#20276=CARTESIAN_POINT ( 'NONE',  ( -0.05219959533910754901, -16.53943276465976808, 87.49890960531436690 ) ) ;
#20277=CARTESIAN_POINT ( 'NONE',  ( -5.153800228976607833, 19.02544592524334988, 32.70942372801899722 ) ) ;
#20279=CARTESIAN_POINT ( 'NONE',  ( 5.719274019375673035, 21.55341960407619339, 42.29275706135235424 ) ) ;
#20280=CARTESIAN_POINT ( 'NONE',  ( 19.02544592524334988, 5.153800228976608722, 96.45942372801897591 ) ) ;
#20281=CARTESIAN_POINT ( 'NONE',  ( 5.049401038298161559, -19.05341960407611168, 112.7072429386476813 ) ) ;
#20282=CARTESIAN_POINT ( 'NONE',  ( 0.05219959533909260263, 19.03943276465977164, 84.99890960531436690 ) ) ;
#20283=CARTESIAN_POINT ( 'NONE',  ( 16.46253265017160672, -9.564922557960803928, 88.33224293864769550 ) ) ;
#20284=CARTESIAN_POINT ( 'NONE',  ( 10.72451020669898902, -18.67979575497178502, 57.91557627198103120 ) ) ;
#20285=CARTESIAN_POINT ( 'NONE',  ( -0.05219959533910754901, -16.53943276465976808, 97.49890960531436690 ) ) ;
#20286=CARTESIAN_POINT ( 'NONE',  ( -19.02544592524342804, 5.153800228976336051, 71.04057627198099567 ) ) ;
#20287=CARTESIAN_POINT ( 'NONE',  ( 0.05219959533910956823, 16.53943276465976808, 114.9989096053143669 ) ) ;
#20288=CARTESIAN_POINT ( 'NONE',  ( 10.72451020669871369, 18.67979575497193778, 42.08442372801901854 ) ) ;
#20289=CARTESIAN_POINT ( 'NONE',  ( -21.55341960407619339, 5.719274019375674811, 73.54275706135234714 ) ) ;
#20290=CARTESIAN_POINT ( 'NONE',  ( -13.89961937509977652, 13.97604488694528158, 55.62390960531434558 ) ) ;
#20291=CARTESIAN_POINT ( 'NONE',  ( -4.379528057220086978, -16.55341960407618274, 74.79275706135234714 ) ) ;
#20292=CARTESIAN_POINT ( 'NONE',  ( -21.53943276465977519, -0.05219959533937600094, 28.75109039468567929 ) ) ;
#20293=CARTESIAN_POINT ( 'NONE',  ( 21.55341960407619695, -5.719274019375665929, 31.04275706135234714 ) ) ;
#20294=CARTESIAN_POINT ( 'NONE',  ( 13.97604488694548053, -13.89961937509957401, 55.62609039468566863 ) ) ;
#20295=CARTESIAN_POINT ( 'NONE',  ( 5.049401038298161559, -19.05341960407611168, 82.70724293864770971 ) ) ;
#20296=CARTESIAN_POINT ( 'NONE',  ( -5.153800228976607833, 19.02544592524334988, 27.70942372801899722 ) ) ;
#20297=CARTESIAN_POINT ( 'NONE',  ( -5.823673210054431948, 21.52544592524334988, 77.70942372801900433 ) ) ;
#20298=CARTESIAN_POINT ( 'NONE',  ( -10.81492255796078084, -18.62759615963271287, 72.08224293864769550 ) ) ;
#20299=CARTESIAN_POINT ( 'NONE',  ( -14.29746914071049879, 8.314922557960819915, 55.83224293864770260 ) ) ;
#20300=CARTESIAN_POINT ( 'NONE',  ( -15.80617190586768217, 15.72974639402176855, 88.12609039468570415 ) ) ;
#20301=CARTESIAN_POINT ( 'NONE',  ( -19.05341960407617563, 5.049401038297882671, 28.54275706135232937 ) ) ;
#20302=CARTESIAN_POINT ( 'NONE',  ( -8.224510206698948167, 14.34966873604960824, 75.41557627198102409 ) ) ;
#20303=CARTESIAN_POINT ( 'NONE',  ( -19.05341960407611168, -5.049401038298163336, 21.45724293864768839 ) ) ;
#20304=CARTESIAN_POINT ( 'NONE',  ( 19.05341960407617918, -5.049401038297876454, 56.04275706135234714 ) ) ;
#20305=CARTESIAN_POINT ( 'NONE',  ( 16.55341960407611168, 4.379528057220329451, 38.95724293864768839 ) ) ;
#20306=CARTESIAN_POINT ( 'NONE',  ( 10.81492255796106328, -18.62759615963255655, 85.41775706135236135 ) ) ;
#20307=CARTESIAN_POINT ( 'NONE',  ( -0.05219959533909027116, -19.03943276465977164, 72.49890960531435269 ) ) ;
#20308=CARTESIAN_POINT ( 'NONE',  ( 9.474510206698729675, 16.51473224551082808, 52.08442372801900433 ) ) ;
#20309=CARTESIAN_POINT ( 'NONE',  ( -15.80617190586745835, -15.72974639402198527, 46.87390960531435979 ) ) ;
#20310=CARTESIAN_POINT ( 'NONE',  ( 5.719274019375673035, 21.55341960407619339, 42.29275706135235424 ) ) ;
#20311=CARTESIAN_POINT ( 'NONE',  ( 5.823673210054125526, 21.52544592524343514, 99.79057627198103830 ) ) ;
#20312=CARTESIAN_POINT ( 'NONE',  ( 16.51473224551083163, -9.474510206698727899, 95.83442372801900433 ) ) ;
#20313=CARTESIAN_POINT ( 'NONE',  ( -14.34966873604972548, 8.224510206698743886, 63.33442372801900433 ) ) ;
#20315=CARTESIAN_POINT ( 'NONE',  ( 21.52544592524344225, -5.823673210054117533, 103.5405762719810383 ) ) ;
#20316=CARTESIAN_POINT ( 'NONE',  ( -8.314922557960811034, -14.29746914071050412, 97.08224293864770971 ) ) ;
#20317=CARTESIAN_POINT ( 'NONE',  ( -17.49999999999999289, -5.068104630630435814, 29.27181594659970898 ) ) ;
#20318=CARTESIAN_POINT ( 'NONE',  ( -16.53943276465976808, -0.05219959533934237506, 33.75109039468568284 ) ) ;
#20319=CARTESIAN_POINT ( 'NONE',  ( 5.823673210054125526, 21.52544592524343514, 64.79057627198103830 ) ) ;
#20320=CARTESIAN_POINT ( 'NONE',  ( -8.314922557961024197, 14.29746914071037800, 107.9177570613523471 ) ) ;
#20321=CARTESIAN_POINT ( 'NONE',  ( 9.564922557960805705, 16.46253265017160317, 29.58224293864769550 ) ) ;
#20322=CARTESIAN_POINT ( 'NONE',  ( -4.483927247898782831, 16.52544592524335698, 67.70942372801901854 ) ) ;
#20323=CARTESIAN_POINT ( 'NONE',  ( -9.474510206698720793, -16.51473224551083518, 59.58442372801900433 ) ) ;
#20324=CARTESIAN_POINT ( 'NONE',  ( 21.53943276465977519, 0.05219959533937863772, 36.25109039468567573 ) ) ;
#20325=CARTESIAN_POINT ( 'NONE',  ( 10.72451020669898902, -18.67979575497178502, 52.91557627198103830 ) ) ;
#20326=CARTESIAN_POINT ( 'NONE',  ( 4.483927247898790824, -16.52544592524335698, 100.2094237280190043 ) ) ;
#20327=CARTESIAN_POINT ( 'NONE',  ( -5.719274019375665041, -21.55341960407619695, 74.79275706135234714 ) ) ;
#20328=CARTESIAN_POINT ( 'NONE',  ( 5.719274019375991003, -21.55341960407610458, 52.70724293864769550 ) ) ;
#20329=CARTESIAN_POINT ( 'NONE',  ( 10.72451020669898902, -18.67979575497178502, 37.91557627198102409 ) ) ;
#20330=VERTEX_POINT ( 'NONE', #10974 ) ;
#20331=CARTESIAN_POINT ( 'NONE',  ( -14.34966873604972548, 8.224510206698743886, 73.33442372801901854 ) ) ;
#20332=CARTESIAN_POINT ( 'NONE',  ( -21.55341960407610458, -5.719274019375992779, 26.45724293864768839 ) ) ;
#20334=CARTESIAN_POINT ( 'NONE',  ( 0.05219959533909260263, 19.03943276465977164, 94.99890960531436690 ) ) ;
#20335=CARTESIAN_POINT ( 'NONE',  ( -12.14591786802326823, 12.06949235617739902, 108.1260903946856757 ) ) ;
#20337=CARTESIAN_POINT ( 'NONE',  ( 16.53943276465976808, -0.05219959533910856209, 103.7489096053143669 ) ) ;
#20338=CARTESIAN_POINT ( 'NONE',  ( 5.823673210054125526, 21.52544592524343514, 59.79057627198103120 ) ) ;
#20339=CARTESIAN_POINT ( 'NONE',  ( 8.224510206698742110, 14.34966873604972548, 97.08442372801904696 ) ) ;
#20340=CARTESIAN_POINT ( 'NONE',  ( 21.55341960407619695, -5.719274019375665929, 51.04275706135234714 ) ) ;
#20341=CARTESIAN_POINT ( 'NONE',  ( -16.46253265017146816, -9.564922557961047289, 109.1677570613523471 ) ) ;
#20342=CARTESIAN_POINT ( 'NONE',  ( -8.224510206698948167, 14.34966873604960824, 105.4155762719810383 ) ) ;
#20343=CARTESIAN_POINT ( 'NONE',  ( 19.02544592524343514, -5.153800228976328945, 48.54057627198103120 ) ) ;
#20344=CARTESIAN_POINT ( 'NONE',  ( 9.474510206698971260, -16.51473224551069308, 22.91557627198102765 ) ) ;
#20345=CARTESIAN_POINT ( 'NONE',  ( 17.50000000000000000, -5.499999999999992895, 38.29690382534171533 ) ) ;
#20346=CARTESIAN_POINT ( 'NONE',  ( -16.51473224551069308, -9.474510206698971260, 86.66557627198102409 ) ) ;
#20347=EDGE_CURVE ( 'NONE', #20566, #145773, #158736, .T. ) ;
#20348=CARTESIAN_POINT ( 'NONE',  ( -12.06949235617739369, -12.14591786802326823, 74.37609039468568994 ) ) ;
#20349=CARTESIAN_POINT ( 'NONE',  ( 15.72974639402176855, 15.80617190586768217, 106.8760903946856899 ) ) ;
#20350=CARTESIAN_POINT ( 'NONE',  ( -15.80617190586745835, -15.72974639402198527, 61.87390960531436690 ) ) ;
#20351=CARTESIAN_POINT ( 'NONE',  ( 4.379528057220092307, 16.55341960407617563, 67.29275706135234714 ) ) ;
#20352=CARTESIAN_POINT ( 'NONE',  ( 19.02544592524334988, 5.153800228976608722, 86.45942372801900433 ) ) ;
#20354=CARTESIAN_POINT ( 'NONE',  ( 9.474510206698971260, -16.51473224551069308, 37.91557627198102409 ) ) ;
#20355=CARTESIAN_POINT ( 'NONE',  ( 9.474510206698971260, -16.51473224551069308, 82.91557627198103830 ) ) ;
#20356=CARTESIAN_POINT ( 'NONE',  ( 19.02544592524343514, -5.153800228976328945, 28.54057627198102409 ) ) ;
#20357=CARTESIAN_POINT ( 'NONE',  ( -5.049401038297874678, -19.05341960407617918, 74.79275706135231871 ) ) ;
#20359=CARTESIAN_POINT ( 'NONE',  ( 19.02544592524343514, -5.153800228976328945, 93.54057627198102409 ) ) ;
#20360=CARTESIAN_POINT ( 'NONE',  ( 4.483927247898545687, 16.52544592524342804, 44.79057627198103120 ) ) ;
#20361=CARTESIAN_POINT ( 'NONE',  ( -10.72451020669898014, 18.67979575497178502, 55.41557627198102409 ) ) ;
#20364=CARTESIAN_POINT ( 'NONE',  ( 5.049401038297881783, 19.05341960407617563, 27.29275706135232937 ) ) ;
#20365=CARTESIAN_POINT ( 'NONE',  ( 9.474510206698971260, -16.51473224551069308, 52.91557627198102409 ) ) ;
#20366=CARTESIAN_POINT ( 'NONE',  ( 16.51473224551069308, 9.474510206698969483, 59.16557627198102409 ) ) ;
#20367=CARTESIAN_POINT ( 'NONE',  ( 14.34966873604972726, -8.224510206698740333, 40.83442372801901854 ) ) ;
#20368=CARTESIAN_POINT ( 'NONE',  ( -19.52851543214744012, -5.499999999999989342, 100.3935772176258041 ) ) ;
#20370=CARTESIAN_POINT ( 'NONE',  ( -12.06949235617739369, -12.14591786802326823, 69.37609039468567573 ) ) ;
#20371=CARTESIAN_POINT ( 'NONE',  ( -18.62759615963270932, 10.81492255796079327, 95.83224293864770971 ) ) ;
#20373=CARTESIAN_POINT ( 'NONE',  ( 14.29746914071037800, 8.314922557961029526, 41.66775706135235424 ) ) ;
#20374=CARTESIAN_POINT ( 'NONE',  ( 5.153800228976335163, 19.02544592524342804, 39.79057627198100988 ) ) ;
#20376=CARTESIAN_POINT ( 'NONE',  ( -21.53943276465977519, -0.05219959533937600094, 53.75109039468568994 ) ) ;
#20377=CARTESIAN_POINT ( 'NONE',  ( -19.02544592524334988, -5.153800228976617603, 58.95942372801900433 ) ) ;
#20378=CARTESIAN_POINT ( 'NONE',  ( -10.72451020669870658, -18.67979575497194134, 94.58442372801901854 ) ) ;
#20380=CARTESIAN_POINT ( 'NONE',  ( 4.379528057220339221, -16.55341960407611168, 47.70724293864770260 ) ) ;
#20381=CARTESIAN_POINT ( 'NONE',  ( 19.53091890409951503, 5.500000000000023981, 42.56097431831420863 ) ) ;
#20382=CARTESIAN_POINT ( 'NONE',  ( -15.72974639402197994, 15.80617190586746368, 60.62390960531437401 ) ) ;
#20384=CARTESIAN_POINT ( 'NONE',  ( 19.02544592524343514, -5.153800228976328945, 98.54057627198100988 ) ) ;
#20385=CARTESIAN_POINT ( 'NONE',  ( 14.34966873604960469, 8.224510206698951720, 99.16557627198100988 ) ) ;
#20386=CARTESIAN_POINT ( 'NONE',  ( 16.53943276465976808, 0.05219959533934440121, 21.25109039468567218 ) ) ;
#20387=CARTESIAN_POINT ( 'NONE',  ( 12.14591786802327356, -12.06949235617739191, 105.6260903946856899 ) ) ;
#20389=CARTESIAN_POINT ( 'NONE',  ( 18.67979575497178502, 10.72451020669898547, 109.1655762719810383 ) ) ;
#20391=CARTESIAN_POINT ( 'NONE',  ( -8.224510206698948167, 14.34966873604960824, 25.41557627198103120 ) ) ;
#20392=CARTESIAN_POINT ( 'NONE',  ( 5.049401038298161559, -19.05341960407611168, 112.7072429386476813 ) ) ;
#20393=CARTESIAN_POINT ( 'NONE',  ( 16.46253265017146816, 9.564922557961045513, 91.66775706135234714 ) ) ;
#20394=CARTESIAN_POINT ( 'NONE',  ( -5.823673210054431948, 21.52544592524334988, 102.7094237280190185 ) ) ;
#20395=CARTESIAN_POINT ( 'NONE',  ( -14.34966873604960291, -8.224510206698953496, 26.66557627198103475 ) ) ;
#20396=CARTESIAN_POINT ( 'NONE',  ( 10.72451020669898902, -18.67979575497178502, 87.91557627198103830 ) ) ;
#20397=CARTESIAN_POINT ( 'NONE',  ( -21.53943276465977519, 0.05219959533907696930, 56.24890960531436690 ) ) ;
#20398=CARTESIAN_POINT ( 'NONE',  ( 19.05341960407611168, 5.049401038298154454, 58.95724293864768129 ) ) ;
#20399=CARTESIAN_POINT ( 'NONE',  ( 8.314922557960818139, 14.29746914071049879, 29.58224293864769905 ) ) ;
#20400=CARTESIAN_POINT ( 'NONE',  ( -9.564922557960796823, -16.46253265017161027, 82.08224293864768129 ) ) ;
#20403=CARTESIAN_POINT ( 'NONE',  ( 13.89961937509957401, 13.97604488694547697, 41.87609039468566152 ) ) ;
#20404=CARTESIAN_POINT ( 'NONE',  ( -21.53943276465977519, 0.05219959533907696930, 86.24890960531436690 ) ) ;
#20405=CARTESIAN_POINT ( 'NONE',  ( 4.379528057220339221, -16.55341960407611168, 82.70724293864770971 ) ) ;
#20406=CARTESIAN_POINT ( 'NONE',  ( 18.67979575497194134, -10.72451020669871369, 35.83442372801901143 ) ) ;
#20408=CARTESIAN_POINT ( 'NONE',  ( -4.379528057220086978, -16.55341960407618274, 109.7927570613523613 ) ) ;
#20409=CARTESIAN_POINT ( 'NONE',  ( 5.049401038298161559, -19.05341960407611168, 32.70724293864768129 ) ) ;
#20410=CARTESIAN_POINT ( 'NONE',  ( -5.153800228976328057, -19.02544592524343514, 82.29057627198103830 ) ) ;
#20411=CARTESIAN_POINT ( 'NONE',  ( -5.153800228976328057, -19.02544592524343514, 32.29057627198102409 ) ) ;
#20412=CARTESIAN_POINT ( 'NONE',  ( 16.55341960407611168, 4.379528057220329451, 48.95724293864770971 ) ) ;
#20413=CARTESIAN_POINT ( 'NONE',  ( -21.52544592524334988, -5.823673210054445271, 73.95942372801901854 ) ) ;
#20415=CARTESIAN_POINT ( 'NONE',  ( 8.314922557961029526, -14.29746914071037800, 65.41775706135234714 ) ) ;
#20416=CARTESIAN_POINT ( 'NONE',  ( 9.474510206698971260, -16.51473224551069308, 42.91557627198103120 ) ) ;
#20417=CARTESIAN_POINT ( 'NONE',  ( 19.02544592524343514, -5.153800228976328945, 48.54057627198103120 ) ) ;
#20419=CARTESIAN_POINT ( 'NONE',  ( -9.474510206698720793, -16.51473224551083518, 19.58442372801899722 ) ) ;
#20420=CARTESIAN_POINT ( 'NONE',  ( 16.52544592524335698, 4.483927247898782831, 56.45942372801902565 ) ) ;
#20421=CARTESIAN_POINT ( 'NONE',  ( -15.80617190586768217, 15.72974639402176855, 103.1260903946856757 ) ) ;
#20422=CARTESIAN_POINT ( 'NONE',  ( -5.719274019375978568, 21.55341960407610458, 35.20724293864768839 ) ) ;
#20423=CARTESIAN_POINT ( 'NONE',  ( -13.89961937509957401, -13.97604488694547875, 109.3760903946856331 ) ) ;
#20424=CARTESIAN_POINT ( 'NONE',  ( -5.823673210054431948, 21.52544592524334988, 67.70942372801901854 ) ) ;
#20425=CARTESIAN_POINT ( 'NONE',  ( 4.379528057220092307, 16.55341960407617563, 32.29275706135235424 ) ) ;
#20426=CARTESIAN_POINT ( 'NONE',  ( 0.05219959533907565091, 21.53943276465977519, 99.99890960531436690 ) ) ;
#20427=CARTESIAN_POINT ( 'NONE',  ( 16.51473224551083163, -9.474510206698727899, 95.83442372801900433 ) ) ;
#20428=CARTESIAN_POINT ( 'NONE',  ( -0.05219959533909027116, -19.03943276465977164, 67.49890960531436690 ) ) ;
#20429=CARTESIAN_POINT ( 'NONE',  ( 16.53943276465976808, 0.05219959533934440121, 21.25109039468567218 ) ) ;
#20430=CARTESIAN_POINT ( 'NONE',  ( -19.02544592524334988, -5.153800228976617603, 108.9594237280189759 ) ) ;
#20431=CARTESIAN_POINT ( 'NONE',  ( 16.55341960407611168, 4.379528057220329451, 63.95724293864770260 ) ) ;
#20432=CARTESIAN_POINT ( 'NONE',  ( -14.34966873604972548, 8.224510206698743886, 73.33442372801901854 ) ) ;
#20433=CARTESIAN_POINT ( 'NONE',  ( -5.823673210054431948, 21.52544592524334988, 22.70942372801901499 ) ) ;
#20434=CARTESIAN_POINT ( 'NONE',  ( 19.05341960407611168, 5.049401038298154454, 48.95724293864768129 ) ) ;
#20435=CARTESIAN_POINT ( 'NONE',  ( 16.46253265017160672, -9.564922557960803928, 53.33224293864768839 ) ) ;
#20436=CARTESIAN_POINT ( 'NONE',  ( -14.34966873604972548, 8.224510206698743886, 68.33442372801900433 ) ) ;
#20440=CARTESIAN_POINT ( 'NONE',  ( -19.03943276465977164, -0.05219959533935918106, 23.75109039468566152 ) ) ;
#20441=ADVANCED_FACE ( 'NONE', ( #58460 ), #143836, .F. ) ;
#20442=CARTESIAN_POINT ( 'NONE',  ( -19.05341960407611168, -5.049401038298163336, 26.45724293864769550 ) ) ;
#20443=ORIENTED_EDGE ( 'NONE', *, *, #3493, .T. ) ;
#20444=CARTESIAN_POINT ( 'NONE',  ( -19.02544592524334988, -5.153800228976617603, 108.9594237280189759 ) ) ;
#20445=CARTESIAN_POINT ( 'NONE',  ( -21.55341960407610458, -5.719274019375992779, 46.45724293864769550 ) ) ;
#20446=CARTESIAN_POINT ( 'NONE',  ( 5.153800228976615827, -19.02544592524334988, 50.20942372801897591 ) ) ;
#20447=CARTESIAN_POINT ( 'NONE',  ( 12.14591786802327356, -12.06949235617739191, 35.62609039468568994 ) ) ;
#20448=CARTESIAN_POINT ( 'NONE',  ( -16.51473224551069308, -9.474510206698971260, 41.66557627198103120 ) ) ;
#20449=CARTESIAN_POINT ( 'NONE',  ( -9.564922557960796823, -16.46253265017161027, 47.08224293864769550 ) ) ;
#20450=CARTESIAN_POINT ( 'NONE',  ( -21.53943276465977519, 0.05219959533907696930, 86.24890960531436690 ) ) ;
#20451=CARTESIAN_POINT ( 'NONE',  ( 13.97604488694527802, 13.89961937509977652, 109.3739096053143669 ) ) ;
#20452=AXIS2_PLACEMENT_3D ( 'NONE', #155420, #125082, #16910 ) ;
#20453=CARTESIAN_POINT ( 'NONE',  ( -13.89961937509977652, 13.97604488694528158, 55.62390960531434558 ) ) ;
#20455=CARTESIAN_POINT ( 'NONE',  ( 13.89961937509957401, 13.97604488694547697, 91.87609039468567573 ) ) ;
#20456=CARTESIAN_POINT ( 'NONE',  ( -16.52544592524342804, 4.483927247898546575, 61.04057627198103120 ) ) ;
#20457=CARTESIAN_POINT ( 'NONE',  ( 5.153800228976615827, -19.02544592524334988, 25.20942372801900433 ) ) ;
#20459=CARTESIAN_POINT ( 'NONE',  ( 21.53943276465977519, -0.05219959533907433946, 93.74890960531436690 ) ) ;
#20460=CARTESIAN_POINT ( 'NONE',  ( 15.72974639402176855, 15.80617190586768217, 86.87609039468568994 ) ) ;
#20461=CARTESIAN_POINT ( 'NONE',  ( 19.05341960407611168, 5.049401038298154454, 23.95724293864769194 ) ) ;
#20462=CARTESIAN_POINT ( 'NONE',  ( -18.67979575497193778, 10.72451020669871902, 73.33442372801901854 ) ) ;
#20463=CARTESIAN_POINT ( 'NONE',  ( -12.14591786802309592, -12.06949235617757132, 21.87390960531436690 ) ) ;
#20464=CARTESIAN_POINT ( 'NONE',  ( 21.53943276465977519, 0.05219959533937863772, 76.25109039468568994 ) ) ;
#20465=CARTESIAN_POINT ( 'NONE',  ( 0.05219959533909260263, 19.03943276465977164, 69.99890960531435269 ) ) ;
#20466=CARTESIAN_POINT ( 'NONE',  ( -15.80617190586768217, 15.72974639402176855, 43.12609039468568284 ) ) ;
#20467=CARTESIAN_POINT ( 'NONE',  ( 9.474510206698971260, -16.51473224551069308, 87.91557627198102409 ) ) ;
#20468=CARTESIAN_POINT ( 'NONE',  ( -14.29746914071049879, 8.314922557960819915, 95.83224293864770971 ) ) ;
#20469=CARTESIAN_POINT ( 'NONE',  ( 4.379528057220339221, -16.55341960407611168, 62.70724293864769550 ) ) ;
#20470=CARTESIAN_POINT ( 'NONE',  ( 10.81492255796078972, 18.62759615963270932, 69.58224293864769550 ) ) ;
#20471=CARTESIAN_POINT ( 'NONE',  ( -19.05341960407611168, -5.049401038298163336, 56.45724293864768129 ) ) ;
#20472=CARTESIAN_POINT ( 'NONE',  ( -5.719274019375978568, 21.55341960407610458, 80.20724293864769550 ) ) ;
#20473=CARTESIAN_POINT ( 'NONE',  ( 19.03943276465977164, 0.05219959533936151252, 71.25109039468566152 ) ) ;
#20474=CARTESIAN_POINT ( 'NONE',  ( -5.049401038297874678, -19.05341960407618274, 34.79275706135233293 ) ) ;
#20475=CARTESIAN_POINT ( 'NONE',  ( -14.29746914071049879, 8.314922557960819915, 80.83224293864769550 ) ) ;
#20476=CARTESIAN_POINT ( 'NONE',  ( 18.62759615963271287, -10.81492255796078972, 53.33224293864769550 ) ) ;
#20477=CARTESIAN_POINT ( 'NONE',  ( 17.44279575226824619, 5.990770900252460507, 101.6644243248568245 ) ) ;
#20478=CARTESIAN_POINT ( 'NONE',  ( -12.14591786802326823, 12.06949235617739902, 98.12609039468570415 ) ) ;
#20480=CARTESIAN_POINT ( 'NONE',  ( 19.03943276465977164, 0.05219959533936151252, 96.25109039468567573 ) ) ;
#20481=CARTESIAN_POINT ( 'NONE',  ( 4.483927247898545687, 16.52544592524342804, 69.79057627198102409 ) ) ;
#20482=CARTESIAN_POINT ( 'NONE',  ( -19.39056639909676605, -5.500000000000018652, 95.78948781074342378 ) ) ;
#20483=CARTESIAN_POINT ( 'NONE',  ( -19.02544592524342804, 5.153800228976336051, 61.04057627198103120 ) ) ;
#20484=CARTESIAN_POINT ( 'NONE',  ( -4.483927247898539470, -16.52544592524342804, 47.29057627198103120 ) ) ;
#20486=CARTESIAN_POINT ( 'NONE',  ( -5.153800228976328057, -19.02544592524343514, 102.2905762719810383 ) ) ;
#20487=CARTESIAN_POINT ( 'NONE',  ( -16.46253265017146816, -9.564922557961047289, 74.16775706135234714 ) ) ;
#20488=CARTESIAN_POINT ( 'NONE',  ( -16.51473224551069308, -9.474510206698971260, 71.66557627198102409 ) ) ;
#20489=CARTESIAN_POINT ( 'NONE',  ( -16.51473224551069308, -9.474510206698971260, 91.66557627198103830 ) ) ;
#20490=CARTESIAN_POINT ( 'NONE',  ( 9.564922557960805705, 16.46253265017160317, 79.58224293864769550 ) ) ;
#20491=CARTESIAN_POINT ( 'NONE',  ( -18.67979575497178146, -10.72451020669898902, 56.66557627198103830 ) ) ;
#20492=CARTESIAN_POINT ( 'NONE',  ( -0.05219959533934338120, 16.53943276465976808, 57.50109039468568994 ) ) ;
#20493=CARTESIAN_POINT ( 'NONE',  ( 9.564922557961047289, -16.46253265017146816, 105.4177570613523471 ) ) ;
#20494=CARTESIAN_POINT ( 'NONE',  ( -19.03943276465977164, 0.05219959533909376836, 46.24890960531435979 ) ) ;
#20495=CARTESIAN_POINT ( 'NONE',  ( -21.53943276465977519, 0.05219959533907696930, 61.24890960531435979 ) ) ;
#20496=CARTESIAN_POINT ( 'NONE',  ( -19.05341960407617563, 5.049401038297882671, 93.54275706135234714 ) ) ;
#20497=CARTESIAN_POINT ( 'NONE',  ( 8.314922557960818139, 14.29746914071049879, 29.58224293864769905 ) ) ;
#20498=CARTESIAN_POINT ( 'NONE',  ( -5.823673210054431948, 21.52544592524334988, 32.70942372801900433 ) ) ;
#20499=CARTESIAN_POINT ( 'NONE',  ( -5.153800228976607833, 19.02544592524334988, 32.70942372801899722 ) ) ;
#20500=CARTESIAN_POINT ( 'NONE',  ( 16.53943276465976808, 0.05219959533934440121, 61.25109039468567573 ) ) ;
#20501=CARTESIAN_POINT ( 'NONE',  ( -14.34966873604972548, 8.224510206698743886, 88.33442372801901854 ) ) ;
#20502=CARTESIAN_POINT ( 'NONE',  ( 18.22780087662114212, -5.499999999999987566, 41.01540105326107977 ) ) ;
#20503=CARTESIAN_POINT ( 'NONE',  ( 12.14591786802327356, -12.06949235617739191, 85.62609039468568994 ) ) ;
#20504=CARTESIAN_POINT ( 'NONE',  ( 5.719274019375991003, -21.55341960407610458, 22.70724293864769194 ) ) ;
#20505=CARTESIAN_POINT ( 'NONE',  ( -8.224510206698735004, -14.34966873604973081, 29.58442372801901854 ) ) ;
#20506=CARTESIAN_POINT ( 'NONE',  ( -13.97604488694527625, -13.89961937509977652, 46.87390960531435979 ) ) ;
#20507=CARTESIAN_POINT ( 'NONE',  ( 5.049401038298161559, -19.05341960407611168, 47.70724293864770260 ) ) ;
#20508=CARTESIAN_POINT ( 'NONE',  ( 16.46253265017160672, -9.564922557960803928, 58.33224293864769550 ) ) ;
#20509=CARTESIAN_POINT ( 'NONE',  ( -5.719274019375665041, -21.55341960407619695, 34.79275706135235424 ) ) ;
#20510=CARTESIAN_POINT ( 'NONE',  ( 8.314922557961029526, -14.29746914071037800, 50.41775706135235424 ) ) ;
#20511=CARTESIAN_POINT ( 'NONE',  ( 14.34966873604972726, -8.224510206698740333, 110.8344237280190043 ) ) ;
#20512=CARTESIAN_POINT ( 'NONE',  ( -13.97604488694527625, -13.89961937509977652, 21.87390960531435979 ) ) ;
#20513=CARTESIAN_POINT ( 'NONE',  ( -5.823673210054431948, 21.52544592524334988, 107.7094237280190328 ) ) ;
#20514=CARTESIAN_POINT ( 'NONE',  ( 5.049401038297881783, 19.05341960407617563, 112.2927570613523471 ) ) ;
#20515=CARTESIAN_POINT ( 'NONE',  ( 19.05341960407617918, -5.049401038297876454, 66.04275706135233293 ) ) ;
#20516=CARTESIAN_POINT ( 'NONE',  ( -16.52544592524342804, 4.483927247898546575, 71.04057627198103830 ) ) ;
#20517=CARTESIAN_POINT ( 'NONE',  ( 16.51473224551069308, 9.474510206698969483, 39.16557627198103120 ) ) ;
#20518=CARTESIAN_POINT ( 'NONE',  ( -9.474510206698720793, -16.51473224551083518, 69.58442372801901854 ) ) ;
#20519=CARTESIAN_POINT ( 'NONE',  ( 16.62475595723698163, 7.163666690055251252, 76.97286648189535185 ) ) ;
#20520=CARTESIAN_POINT ( 'NONE',  ( -21.55341960407619339, 5.719274019375674811, 83.54275706135234714 ) ) ;
#20521=CARTESIAN_POINT ( 'NONE',  ( 12.14591786802327356, -12.06949235617739191, 35.62609039468568994 ) ) ;
#20522=CARTESIAN_POINT ( 'NONE',  ( 16.61371651742603461, 7.165104196376044676, 38.64584930007005426 ) ) ;
#20523=CARTESIAN_POINT ( 'NONE',  ( 18.62759615963271287, -10.81492255796078972, 33.33224293864769550 ) ) ;
#20524=CARTESIAN_POINT ( 'NONE',  ( 8.314922557961029526, -14.29746914071037800, 25.41775706135235779 ) ) ;
#20525=CARTESIAN_POINT ( 'NONE',  ( -9.474510206698964154, 16.51473224551069663, 30.41557627198102054 ) ) ;
#20526=CARTESIAN_POINT ( 'NONE',  ( -13.97604488694547697, 13.89961937509957934, 28.12609039468565797 ) ) ;
#20527=CARTESIAN_POINT ( 'NONE',  ( 17.60769864724391098, -5.499999999999979572, 66.15024842019164453 ) ) ;
#20528=CARTESIAN_POINT ( 'NONE',  ( -13.89961937509977652, 13.97604488694528158, 40.62390960531435979 ) ) ;
#20530=CARTESIAN_POINT ( 'NONE',  ( -13.97604488694527625, -13.89961937509977652, 71.87390960531433848 ) ) ;
#20531=CARTESIAN_POINT ( 'NONE',  ( -19.53091890409951858, -5.500000000000036415, 55.06097431831419442 ) ) ;
#20532=CARTESIAN_POINT ( 'NONE',  ( 19.02544592524334988, 5.153800228976608722, 26.45942372801899722 ) ) ;
#20533=CARTESIAN_POINT ( 'NONE',  ( 16.55341960407611168, 4.379528057220329451, 28.95724293864769905 ) ) ;
#20534=CARTESIAN_POINT ( 'NONE',  ( 16.46253265017160672, -9.564922557960803928, 28.33224293864769550 ) ) ;
#20535=CARTESIAN_POINT ( 'NONE',  ( -16.51473224551069308, -9.474510206698971260, 91.66557627198103830 ) ) ;
#20536=CARTESIAN_POINT ( 'NONE',  ( -21.53943276465977519, -0.05219959533937600094, 68.75109039468568994 ) ) ;
#20537=CARTESIAN_POINT ( 'NONE',  ( -0.05219959533909027116, -19.03943276465977164, 57.49890960531435979 ) ) ;
#20539=CARTESIAN_POINT ( 'NONE',  ( 10.72451020669871369, 18.67979575497193778, 67.08442372801901854 ) ) ;
#20540=CARTESIAN_POINT ( 'NONE',  ( -19.05341960407617563, 5.049401038297882671, 93.54275706135234714 ) ) ;
#20541=CARTESIAN_POINT ( 'NONE',  ( 15.72974639402199770, -15.80617190586745480, 23.12390960531436335 ) ) ;
#20542=CARTESIAN_POINT ( 'NONE',  ( 19.03943276465977164, -0.05219959533909143690, 33.74890960531435979 ) ) ;
#20543=CARTESIAN_POINT ( 'NONE',  ( -21.52544592524343514, 5.823673210054127303, 116.0405762719810383 ) ) ;
#20544=CARTESIAN_POINT ( 'NONE',  ( -5.153800228976607833, 19.02544592524334988, 32.70942372801899722 ) ) ;
#20545=CARTESIAN_POINT ( 'NONE',  ( 12.14591786802309770, 12.06949235617756955, 104.3739096053143669 ) ) ;
#20546=CARTESIAN_POINT ( 'NONE',  ( -5.153800228976328057, -19.02544592524343514, 62.29057627198100988 ) ) ;
#20547=CARTESIAN_POINT ( 'NONE',  ( -19.05341960407617563, 5.049401038297882671, 108.5427570613523187 ) ) ;
#20548=CARTESIAN_POINT ( 'NONE',  ( -16.52544592524342804, 4.483927247898546575, 76.04057627198102409 ) ) ;
#20549=CARTESIAN_POINT ( 'NONE',  ( 5.823673210054125526, 21.52544592524343514, 29.79057627198102409 ) ) ;
#20550=CARTESIAN_POINT ( 'NONE',  ( -19.05341960407617563, 5.049401038297882671, 83.54275706135233293 ) ) ;
#20551=CARTESIAN_POINT ( 'NONE',  ( -0.05219959533907301413, -21.53943276465977519, 87.49890960531436690 ) ) ;
#20552=CARTESIAN_POINT ( 'NONE',  ( -5.719274019375665041, -21.55341960407619695, 49.79275706135234714 ) ) ;
#20553=CARTESIAN_POINT ( 'NONE',  ( -4.483927247898782831, 16.52544592524335698, 57.70942372801901143 ) ) ;
#20554=CARTESIAN_POINT ( 'NONE',  ( 8.314922557961029526, -14.29746914071037800, 50.41775706135235424 ) ) ;
#20555=CARTESIAN_POINT ( 'NONE',  ( 15.80617190586769283, -15.72974639402175789, 45.62609039468567573 ) ) ;
#20556=CARTESIAN_POINT ( 'NONE',  ( 18.62759615963271287, -10.81492255796078972, 48.33224293864770260 ) ) ;
#20557=CARTESIAN_POINT ( 'NONE',  ( -19.03943276465977164, 0.05219959533909376836, 51.24890960531436690 ) ) ;
#20559=CARTESIAN_POINT ( 'NONE',  ( 12.06949235617739724, 12.14591786802326823, 81.87609039468568994 ) ) ;
#20560=CARTESIAN_POINT ( 'NONE',  ( 15.72974639402199770, -15.80617190586745480, 103.1239096053143811 ) ) ;
#20561=CARTESIAN_POINT ( 'NONE',  ( -12.14591786802309592, -12.06949235617757132, 51.87390960531437401 ) ) ;
#20562=CARTESIAN_POINT ( 'NONE',  ( -14.34966873604972548, 8.224510206698743886, 58.33442372801901143 ) ) ;
#20563=CARTESIAN_POINT ( 'NONE',  ( 16.51473224551083163, -9.474510206698727899, 100.8344237280190043 ) ) ;
#20564=CARTESIAN_POINT ( 'NONE',  ( -21.52544592524343514, 5.823673210054127303, 96.04057627198102409 ) ) ;
#20565=CARTESIAN_POINT ( 'NONE',  ( -16.52544592524342804, 4.483927247898546575, 41.04057627198103120 ) ) ;
#20566=VERTEX_POINT ( 'NONE', #166652 ) ;
#20567=CARTESIAN_POINT ( 'NONE',  ( 18.56453257813365809, -5.499999999999952038, 93.49000423690691264 ) ) ;
#20568=CARTESIAN_POINT ( 'NONE',  ( -5.719274019375978568, 21.55341960407610458, 80.20724293864769550 ) ) ;
#20569=CARTESIAN_POINT ( 'NONE',  ( -16.55341960407611168, -4.379528057220339221, 31.45724293864769550 ) ) ;
#20572=CARTESIAN_POINT ( 'NONE',  ( 10.81492255796078972, 18.62759615963270932, 104.5822429386477097 ) ) ;
#20573=CARTESIAN_POINT ( 'NONE',  ( 21.52544592524344225, -5.823673210054117533, 113.5405762719810383 ) ) ;
#20574=CARTESIAN_POINT ( 'NONE',  ( -14.29746914071049879, 8.314922557960819915, 40.83224293864769550 ) ) ;
#20575=CARTESIAN_POINT ( 'NONE',  ( -4.379528057220086978, -16.55341960407618274, 54.79275706135235424 ) ) ;
#20576=CARTESIAN_POINT ( 'NONE',  ( -16.46253265017160317, 9.564922557960807481, 45.83224293864769550 ) ) ;
#20578=CARTESIAN_POINT ( 'NONE',  ( 5.049401038298161559, -19.05341960407611168, 62.70724293864769550 ) ) ;
#20580=CARTESIAN_POINT ( 'NONE',  ( -15.72974639402197994, 15.80617190586746368, 30.62390960531436335 ) ) ;
#20582=CARTESIAN_POINT ( 'NONE',  ( -16.53943276465976808, -0.05219959533934237506, 18.75109039468568639 ) ) ;
#20583=CARTESIAN_POINT ( 'NONE',  ( -13.89961937509957401, -13.97604488694547875, 44.37609039468566863 ) ) ;
#20584=CARTESIAN_POINT ( 'NONE',  ( -15.72974639402197994, 15.80617190586746368, 100.6239096053143811 ) ) ;
#20585=CARTESIAN_POINT ( 'NONE',  ( 14.34966873604960469, 8.224510206698951720, 29.16557627198103120 ) ) ;
#20586=CARTESIAN_POINT ( 'NONE',  ( -13.97604488694527625, -13.89961937509977652, 81.87390960531436690 ) ) ;
#20587=CARTESIAN_POINT ( 'NONE',  ( -21.53943276465977519, 0.05219959533907696930, 51.24890960531436690 ) ) ;
#20588=CARTESIAN_POINT ( 'NONE',  ( 0.05219959533907565091, 21.53943276465977519, 79.99890960531435269 ) ) ;
#20589=CARTESIAN_POINT ( 'NONE',  ( -0.05219959533934338120, 16.53943276465976808, 22.50109039468567573 ) ) ;
#20590=CARTESIAN_POINT ( 'NONE',  ( 21.55341960407610458, 5.719274019375980345, 23.95724293864769550 ) ) ;
#20591=CARTESIAN_POINT ( 'NONE',  ( -21.52544592524334988, -5.823673210054445271, 73.95942372801901854 ) ) ;
#20592=CARTESIAN_POINT ( 'NONE',  ( 19.05341960407611168, 5.049401038298154454, 68.95724293864769550 ) ) ;
#20593=CARTESIAN_POINT ( 'NONE',  ( 13.89961937509977652, -13.97604488694527269, 33.12390960531434558 ) ) ;
#20594=CARTESIAN_POINT ( 'NONE',  ( 13.97604488694527802, 13.89961937509977652, 89.37390960531436690 ) ) ;
#20595=CARTESIAN_POINT ( 'NONE',  ( -16.53943276465976808, 0.05219959533911058130, 86.24890960531436690 ) ) ;
#20597=CARTESIAN_POINT ( 'NONE',  ( 19.05341960407617918, -5.049401038297876454, 106.0427570613523471 ) ) ;
#20599=CARTESIAN_POINT ( 'NONE',  ( -5.049401038298153566, 19.05341960407611168, 80.20724293864769550 ) ) ;
#20600=CARTESIAN_POINT ( 'NONE',  ( -5.823673210054431948, 21.52544592524334988, 82.70942372801900433 ) ) ;
#20601=CARTESIAN_POINT ( 'NONE',  ( -5.153800228976328057, -19.02544592524343514, 112.2905762719810099 ) ) ;
#20602=CARTESIAN_POINT ( 'NONE',  ( -12.06949235617739369, -12.14591786802326823, 79.37609039468567573 ) ) ;
#20603=CARTESIAN_POINT ( 'NONE',  ( -16.38665767535051287, -7.295008042176176488, 74.73599135785458714 ) ) ;
#20604=CARTESIAN_POINT ( 'NONE',  ( -5.049401038297874678, -19.05341960407617918, 54.79275706135234003 ) ) ;
#20605=CARTESIAN_POINT ( 'NONE',  ( 21.53943276465977519, 0.05219959533937863772, 111.2510903946856899 ) ) ;
#20609=CARTESIAN_POINT ( 'NONE',  ( -4.483927247898782831, 16.52544592524335698, 112.7094237280190328 ) ) ;
#20612=CARTESIAN_POINT ( 'NONE',  ( -0.05219959533934338120, 16.53943276465976808, 107.5010903946856899 ) ) ;
#20614=CARTESIAN_POINT ( 'NONE',  ( -12.14591786802326823, 12.06949235617739902, 83.12609039468568994 ) ) ;
#20615=CARTESIAN_POINT ( 'NONE',  ( 19.03943276465977164, -0.05219959533909143690, 23.74890960531435269 ) ) ;
#20616=CARTESIAN_POINT ( 'NONE',  ( -18.67979575497193778, 10.72451020669871902, 88.33442372801901854 ) ) ;
#20617=CARTESIAN_POINT ( 'NONE',  ( 9.474510206698729675, 16.51473224551082808, 102.0844237280190043 ) ) ;
#20618=CARTESIAN_POINT ( 'NONE',  ( 10.72451020669871369, 18.67979575497193778, 67.08442372801901854 ) ) ;
#20619=CARTESIAN_POINT ( 'NONE',  ( -19.02544592524334988, -5.153800228976617603, 43.95942372801899012 ) ) ;
#20620=CARTESIAN_POINT ( 'NONE',  ( -9.474510206698964154, 16.51473224551069663, 80.41557627198103830 ) ) ;
#20621=CARTESIAN_POINT ( 'NONE',  ( -19.05341960407611168, -5.049401038298163336, 76.45724293864769550 ) ) ;
#20625=CARTESIAN_POINT ( 'NONE',  ( -5.719274019375978568, 21.55341960407610458, 50.20724293864769550 ) ) ;
#20626=CARTESIAN_POINT ( 'NONE',  ( -13.97604488694527625, -13.89961937509977652, 46.87390960531435979 ) ) ;
#20627=CARTESIAN_POINT ( 'NONE',  ( 4.483927247898790824, -16.52544592524335698, 80.20942372801901854 ) ) ;
#20629=CARTESIAN_POINT ( 'NONE',  ( 16.53943276465976808, -0.05219959533910856209, 78.74890960531436690 ) ) ;
#20631=CARTESIAN_POINT ( 'NONE',  ( -4.379528057220086978, -16.55341960407618274, 44.79275706135234714 ) ) ;
#20632=CARTESIAN_POINT ( 'NONE',  ( 8.314922557960818139, 14.29746914071049879, 109.5822429386476955 ) ) ;
#20633=CARTESIAN_POINT ( 'NONE',  ( 13.89961937509957401, 13.97604488694547697, 51.87609039468566863 ) ) ;
#20634=CARTESIAN_POINT ( 'NONE',  ( -8.314922557960811034, -14.29746914071050412, 72.08224293864769550 ) ) ;
#20635=CARTESIAN_POINT ( 'NONE',  ( 15.72974639402176855, 15.80617190586768217, 26.87609039468567218 ) ) ;
#20636=CARTESIAN_POINT ( 'NONE',  ( 13.89961937509977652, -13.97604488694527269, 23.12390960531436335 ) ) ;
#20637=CARTESIAN_POINT ( 'NONE',  ( -15.80617190586745835, -15.72974639402198527, 86.87390960531438111 ) ) ;
#20638=CARTESIAN_POINT ( 'NONE',  ( -5.049401038298153566, 19.05341960407611168, 105.2072429386476671 ) ) ;
#20639=CARTESIAN_POINT ( 'NONE',  ( 16.55341960407611168, 4.379528057220329451, 68.95724293864769550 ) ) ;
#20642=CARTESIAN_POINT ( 'NONE',  ( -16.51473224551082808, 9.474510206698731452, 83.33442372801899012 ) ) ;
#20643=CARTESIAN_POINT ( 'NONE',  ( -10.72451020669870658, -18.67979575497194134, 24.58442372801901499 ) ) ;
#20644=CARTESIAN_POINT ( 'NONE',  ( -16.51473224551069308, -9.474510206698971260, 71.66557627198102409 ) ) ;
#20645=CARTESIAN_POINT ( 'NONE',  ( -19.03943276465977164, -0.05219959533935918106, 58.75109039468566863 ) ) ;
#20646=CARTESIAN_POINT ( 'NONE',  ( 19.05341960407611168, 5.049401038298154454, 38.95724293864767418 ) ) ;
#20647=CARTESIAN_POINT ( 'NONE',  ( 16.55341960407611168, 4.379528057220329451, 68.95724293864769550 ) ) ;
#20648=CARTESIAN_POINT ( 'NONE',  ( 16.53943276465976808, -0.05219959533910856209, 58.74890960531436690 ) ) ;
#20649=CARTESIAN_POINT ( 'NONE',  ( -0.05219959533909027116, -19.03943276465977164, 82.49890960531436690 ) ) ;
#20650=CARTESIAN_POINT ( 'NONE',  ( -18.67979575497178146, -10.72451020669898902, 91.66557627198103830 ) ) ;
#20651=CARTESIAN_POINT ( 'NONE',  ( 16.46253265017160672, -9.564922557960803928, 68.33224293864770971 ) ) ;
#20652=CARTESIAN_POINT ( 'NONE',  ( 21.53943276465977519, -0.05219959533907433946, 83.74890960531435269 ) ) ;
#20653=CARTESIAN_POINT ( 'NONE',  ( -10.81492255796105439, 18.62759615963255655, 112.9177570613523329 ) ) ;
#20654=CARTESIAN_POINT ( 'NONE',  ( 13.89961937509977652, -13.97604488694527269, 28.12390960531435624 ) ) ;
#20655=CARTESIAN_POINT ( 'NONE',  ( 4.379528057220092307, 16.55341960407617563, 112.2927570613523471 ) ) ;
#20656=CARTESIAN_POINT ( 'NONE',  ( 4.379528057220339221, -16.55341960407611168, 92.70724293864770971 ) ) ;
#20657=CARTESIAN_POINT ( 'NONE',  ( -5.049401038297874678, -19.05341960407617918, 99.79275706135234714 ) ) ;
#20658=ORIENTED_EDGE ( 'NONE', *, *, #184816, .F. ) ;
#20659=CARTESIAN_POINT ( 'NONE',  ( 5.719274019375991003, -21.55341960407610458, 112.7072429386476955 ) ) ;
#20660=CARTESIAN_POINT ( 'NONE',  ( -19.05341960407617563, 5.049401038297882671, 58.54275706135234003 ) ) ;
#20661=CARTESIAN_POINT ( 'NONE',  ( -4.483927247898539470, -16.52544592524342804, 27.29057627198103120 ) ) ;
#20662=CARTESIAN_POINT ( 'NONE',  ( 9.474510206698729675, 16.51473224551082808, 42.08442372801900433 ) ) ;
#20663=CARTESIAN_POINT ( 'NONE',  ( -13.89961937509977652, 13.97604488694528158, 105.6239096053143527 ) ) ;
#20664=CARTESIAN_POINT ( 'NONE',  ( 16.52544592524342804, -4.483927247898539470, 53.54057627198103120 ) ) ;
#20666=CARTESIAN_POINT ( 'NONE',  ( 9.474510206698971260, -16.51473224551069308, 32.91557627198102409 ) ) ;
#20667=CARTESIAN_POINT ( 'NONE',  ( -10.72451020669870658, -18.67979575497194134, 104.5844237280190185 ) ) ;
#20668=CARTESIAN_POINT ( 'NONE',  ( 12.06949235617739724, 12.14591786802326823, 86.87609039468568994 ) ) ;
#20669=CARTESIAN_POINT ( 'NONE',  ( 5.823673210054444382, -21.52544592524334988, 40.20942372801901854 ) ) ;
#20670=CARTESIAN_POINT ( 'NONE',  ( 0.05219959533934541429, -16.53943276465976808, 50.00109039468568994 ) ) ;
#20671=CARTESIAN_POINT ( 'NONE',  ( -0.05219959533909027116, -19.03943276465977164, 102.4989096053143669 ) ) ;
#20672=CARTESIAN_POINT ( 'NONE',  ( 16.46253265017160672, -9.564922557960803928, 48.33224293864769550 ) ) ;
#20673=CARTESIAN_POINT ( 'NONE',  ( -0.05219959533909027116, -19.03943276465977164, 67.49890960531436690 ) ) ;
#20674=CARTESIAN_POINT ( 'NONE',  ( 12.06949235617739724, 12.14591786802326823, 46.87609039468568994 ) ) ;
#20675=CARTESIAN_POINT ( 'NONE',  ( -12.14591786802309592, -12.06949235617757132, 111.8739096053143669 ) ) ;
#20676=CARTESIAN_POINT ( 'NONE',  ( 16.53943276465976808, 0.05219959533934440121, 111.2510903946856899 ) ) ;
#20678=CARTESIAN_POINT ( 'NONE',  ( 18.62759615963255655, 10.81492255796105972, 61.66775706135235424 ) ) ;
#20679=CARTESIAN_POINT ( 'NONE',  ( 16.51473224551069308, 9.474510206698969483, 89.16557627198103830 ) ) ;
#20680=CARTESIAN_POINT ( 'NONE',  ( 5.153800228976335163, 19.02544592524342804, 79.79057627198102409 ) ) ;
#20681=CARTESIAN_POINT ( 'NONE',  ( -13.89961937509977652, 13.97604488694528158, 95.62390960531436690 ) ) ;
#20682=CARTESIAN_POINT ( 'NONE',  ( 12.14591786802309770, 12.06949235617756955, 39.37390960531436690 ) ) ;
#20683=CARTESIAN_POINT ( 'NONE',  ( 16.53943276465976808, -0.05219959533910856209, 23.74890960531435269 ) ) ;
#20685=CARTESIAN_POINT ( 'NONE',  ( -4.483927247898539470, -16.52544592524342804, 42.29057627198103120 ) ) ;
#20688=CARTESIAN_POINT ( 'NONE',  ( 13.89961937509977652, -13.97604488694527269, 68.12390960531436690 ) ) ;
#20689=CARTESIAN_POINT ( 'NONE',  ( -0.05219959533936034679, 19.03943276465977164, 52.50109039468566863 ) ) ;
#20691=CARTESIAN_POINT ( 'NONE',  ( -0.05219959533909027116, -19.03943276465977164, 67.49890960531436690 ) ) ;
#20692=CARTESIAN_POINT ( 'NONE',  ( 13.97604488694548053, -13.89961937509957401, 85.62609039468568994 ) ) ;
#20693=CARTESIAN_POINT ( 'NONE',  ( -14.34966873604972548, 8.224510206698743886, 63.33442372801900433 ) ) ;
#20695=CARTESIAN_POINT ( 'NONE',  ( -5.049401038298153566, 19.05341960407611168, 95.20724293864770971 ) ) ;
#20696=CARTESIAN_POINT ( 'NONE',  ( -10.81492255796105439, 18.62759615963255655, 27.91775706135234358 ) ) ;
#20697=CARTESIAN_POINT ( 'NONE',  ( 16.51473224551083163, -9.474510206698727899, 95.83442372801900433 ) ) ;
#20698=CARTESIAN_POINT ( 'NONE',  ( 17.40805194822030444, 6.112264579159356614, 86.66628727489388950 ) ) ;
#20699=CARTESIAN_POINT ( 'NONE',  ( 9.474510206698971260, -16.51473224551069308, 42.91557627198103120 ) ) ;
#20700=CARTESIAN_POINT ( 'NONE',  ( 9.564922557960805705, 16.46253265017160317, 89.58224293864769550 ) ) ;
#20701=CARTESIAN_POINT ( 'NONE',  ( -4.483927247898539470, -16.52544592524342804, 52.29057627198102409 ) ) ;
#20702=CARTESIAN_POINT ( 'NONE',  ( -19.03943276465977164, 0.05219959533909376836, 56.24890960531435979 ) ) ;
#20703=CARTESIAN_POINT ( 'NONE',  ( 0.05219959533936267826, -19.03943276465977164, 65.00109039468567573 ) ) ;
#20705=CARTESIAN_POINT ( 'NONE',  ( 16.51473224551083163, -9.474510206698727899, 35.83442372801899722 ) ) ;
#20706=CARTESIAN_POINT ( 'NONE',  ( -5.049401038298153566, 19.05341960407611168, 65.20724293864765286 ) ) ;
#20708=CARTESIAN_POINT ( 'NONE',  ( 10.72451020669898902, -18.67979575497178502, 57.91557627198103120 ) ) ;
#20709=CARTESIAN_POINT ( 'NONE',  ( -12.14591786802309592, -12.06949235617757132, 66.87390960531436690 ) ) ;
#20710=CARTESIAN_POINT ( 'NONE',  ( 19.02544592524334988, 5.153800228976608722, 26.45942372801899722 ) ) ;
#20711=CARTESIAN_POINT ( 'NONE',  ( 16.51473224551069308, 9.474510206698969483, 109.1655762719810383 ) ) ;
#20712=CARTESIAN_POINT ( 'NONE',  ( 18.67979575497178502, 10.72451020669898547, 29.16557627198103120 ) ) ;
#20713=CARTESIAN_POINT ( 'NONE',  ( -0.05219959533909027116, -19.03943276465977164, 57.49890960531435979 ) ) ;
#20714=CARTESIAN_POINT ( 'NONE',  ( -19.02544592524342804, 5.153800228976336051, 36.04057627198100988 ) ) ;
#20715=CARTESIAN_POINT ( 'NONE',  ( 4.483927247898545687, 16.52544592524342804, 104.7905762719810241 ) ) ;
#20716=CARTESIAN_POINT ( 'NONE',  ( -15.72974639402176322, -15.80617190586768395, 19.37609039468568639 ) ) ;
#20717=CARTESIAN_POINT ( 'NONE',  ( -13.97604488694527625, -13.89961937509977652, 111.8739096053143243 ) ) ;
#20718=CARTESIAN_POINT ( 'NONE',  ( 10.81492255796106328, -18.62759615963255655, 25.41775706135235779 ) ) ;
#20719=CARTESIAN_POINT ( 'NONE',  ( -0.05219959533909027116, -19.03943276465977164, 107.4989096053143527 ) ) ;
#20720=CARTESIAN_POINT ( 'NONE',  ( -8.224510206698948167, 14.34966873604960824, 115.4155762719810241 ) ) ;
#20721=CARTESIAN_POINT ( 'NONE',  ( 5.719274019375673035, 21.55341960407619339, 72.29275706135236135 ) ) ;
#20722=CARTESIAN_POINT ( 'NONE',  ( 18.67979575497178502, 10.72451020669898547, 94.16557627198103830 ) ) ;
#20724=CARTESIAN_POINT ( 'NONE',  ( 18.39635199886969730, -5.499999999999973355, 78.51967076359997577 ) ) ;
#20725=CARTESIAN_POINT ( 'NONE',  ( -5.049401038298153566, 19.05341960407611168, 60.20724293864768129 ) ) ;
#20726=CARTESIAN_POINT ( 'NONE',  ( -8.314922557961024197, 14.29746914071037800, 42.91775706135235424 ) ) ;
#20727=CARTESIAN_POINT ( 'NONE',  ( 12.06949235617757843, -12.14591786802309237, 103.1239096053143811 ) ) ;
#20729=CARTESIAN_POINT ( 'NONE',  ( -9.474510206698964154, 16.51473224551069663, 65.41557627198102409 ) ) ;
#20730=CARTESIAN_POINT ( 'NONE',  ( 14.34966873604960469, 8.224510206698951720, 99.16557627198100988 ) ) ;
#20731=CARTESIAN_POINT ( 'NONE',  ( -15.72974639402197994, 15.80617190586746368, 45.62390960531436690 ) ) ;
#20732=CARTESIAN_POINT ( 'NONE',  ( 14.34966873604960469, 8.224510206698951720, 59.16557627198103120 ) ) ;
#20733=CARTESIAN_POINT ( 'NONE',  ( -13.89961937509957401, -13.97604488694547875, 109.3760903946856331 ) ) ;
#20734=CARTESIAN_POINT ( 'NONE',  ( 18.62759615963255655, 10.81492255796105972, 91.66775706135234714 ) ) ;
#20735=CLOSED_SHELL ( 'NONE', ( #53954, #62013, #15330, #8758, #131099, #36061, #118478, #58975, #100272, #118076, #29180, #174575, #139677, #118804, #126981, #25179, #21859, #20987, #40707, #167499, #80645, #33166, #39556, #142192, #94239, #88055, #23155, #105774, #36457, #4267, #142831, #78668, #172386, #178138, #117993, #88662, #191817, #178327, #23384, #4997, #134178, #104476, #179718, #170147, #171155, #146080, #131794, #53484, #135466, #167295, #66940, #161317, #151556, #150985, #37984, #3115, #127113, #80812, #98642, #156677, #192253, #112604, #3634, #174610, #150382, #41490, #140471, #35819, #173686, #19722, #187715, #51167, #190456, #152031, #104135, #54195, #122206, #105509, #112590, #71917, #150746, #195963, #199055, #50148, #169454, #107904, #100461, #119850, #104879, #113246, #83445, #55872, #86379, #49614, #99315, #119326, #56930, #108877, #147415, #66633, #36976, #41657, #5652, #29559, #30297, #83247, #173443, #29760, #156805, #20441 ) ) ;
#20736=CARTESIAN_POINT ( 'NONE',  ( 16.19135201231366139, -7.376712067591920885, 77.31319145947969673 ) ) ;
#20737=CARTESIAN_POINT ( 'NONE',  ( 0.05219959533934541429, -16.53943276465976808, 95.00109039468568994 ) ) ;
#20738=CARTESIAN_POINT ( 'NONE',  ( -16.53943276465976808, 0.05219959533911058130, 46.24890960531435979 ) ) ;
#20739=CARTESIAN_POINT ( 'NONE',  ( -5.049401038298153566, 19.05341960407611168, 40.20724293864768839 ) ) ;
#20740=CARTESIAN_POINT ( 'NONE',  ( 5.153800228976335163, 19.02544592524342804, 89.79057627198102409 ) ) ;
#20741=CARTESIAN_POINT ( 'NONE',  ( -5.719274019375978568, 21.55341960407610458, 90.20724293864770971 ) ) ;
#20742=( BOUNDED_SURFACE ( )  B_SPLINE_SURFACE ( 3, 2, ( 
 ( #43237, #178766, #25091, #86733, #193937, #150430, #181755, #148418, #104904, #133238, #165591, #101908, #163590, #102908, #194930, #118087, #27089, #26086, #88736, #164592, #28092, #87730, #149415, #72584, #134258, #195945, #119092, #178418, #148075, #177426, #37896, #130892, #128882, #83381, #191569, #97537, #147074, #190582, #159224, #176421, #36879, #99554, #20719, #192582, #82376, #161236, #70234, #22730, #144064, #55058, #174421, #38897, #52058, #5545, #127891, #146055, #6539, #84378, #113714, #98545, #7539, #193586, #54065, #116729, #100554, #145058, #69224, #115739, #162233, #68219, #39882, #86391, #101549, #67224, #23732, #175411, #160238, #66231, #189594, #85381, #8558, #51067, #53048, #21728, #129871, #112728, #35890, #131902, #114728, #163241, #24741, #149077, #198558, #117733, #121694, #166239, #87392, #44872, #41903, #90365, #10565, #72229, #13535, #75201, #165244, #103569, #106528, #12562, #151071, #168205, #197568, #73242, #179428, #28728, #40893, #74228, #194584, #134913, #102566, #167230, #133904, #196590, #60027, #164251, #59035, #150071, #195595, #181414, #26738, #135896, #56054, #183390, #58060, #120702, #57067, #104557, #29702, #132895, #105544, #25746, #42892, #136872, #91333, #9566, #118742, #180430, #27739, #71232, #11576, #88377, #119731, #43879, #89382, #182401, #152050, #104444, #28616, #105431, #165130, #14409, #29591, #91222, #199433, #90253, #89270, #182287, #180317, #134799, #42782, #148961, #198441, #41785, #10450, #27630, #88265, #150961, #72110, #43767, #133783, #12456, #121581, #74116, #195476, #106412, #25632, #151936, #103452, #56952, #179314, #197458, #57950, #135787, #26622, #149953, #58924, #44757, #167114, #168093, #13425, #196480, #120592, #75089, #136756, #119621, #152913, #137749, #76073, #118626, #59913, #11458, #73130, #117616, #40778, #183276, #102447, #164135, #166128, #181304, #87276, #95221, #61888, #15410, #33558, #31573, #122575, #107399, #123558, #81038, #124569, #48736, #94221, #3213, #45747, #77068, #153915, #96211, #79055, #110390, #169072, #125569, #30578, #186265, #142714, #188248, #92229, #187267, #156907, #46746, #184265, #185253, #126548, #138738, #47744, #172072, #18404, #108405, #157900, #173075, #34552, #60901, #80053, #32568, #141723, #170081, #78053, #109397, #219, #64887, #93224, #154909, #171077, #16407, #155901, #139722, #49722, #1211, #17398, #111389, #140728, #62889, #19389, #2217, #63899, #128533, #158876, #65872, #84029, #144705, #114363, #66870, #36526, #176068, #131546, #192230, #54704, #38547, #83031, #22378, #160887, #130532, #21373, #116376, #24391, #193230, #20365, #7189, #143709, #51706, #86040, #4194, #115388, #145707, #127546, #191226, #190228, #113369, #189246, #50724, #68873, #112382, #6191, #98180, #174074, #8202, #161884, #67871, #37535, #82013, #53711, #35543, #97190, #5189, #177076, #178065, #39533, #100203, #23379, #101191, #85025, #175060, #146705, #159884, #69877, #129526, #162882, #52700, #99199, #12223, #10214, #164897, #72893, #179074, #28388, #71874, #40544, #57718, #118389, #181071, #102214, #121351, #183044, #134561, #133543, #106183, #27387, #195234, #29366, #163903, #73886, #167866, #88030, #25399, #135556, #120359, #43535, #197228, #182052, #89033, #90026, #165890, #9215, #87041, #105200, #180083, #132550, #55704, #166887, #148726, #42546, #104209, #151709, #26391, #44527, #58690, #150724, #147728, #194238, #41552, #13202, #74865, #56717, #136527, #117377, #59679, #198208, #103215, #70882, #149718, #11217, #196249, #119388, #97691, #159382, #46504, #123325, #129036, #96709, #35054, #190737, #81527, #154677, #60667, #112883, #122340, #158397, #75841, #16172, #199199, #51222, #30344, #77826, #82535, #184031, #143214, #31340, #15176, #65389, #185019, #19886, #137518, #144217, #142227, #4695, #138506, #188756, #5701, #14172, #189750, #45513, #127050, #20877, #175565, #67378, #107168, #168839, #111897, #52211 ),
 ( #50241, #113868, #3712, #66386, #91985, #173585, #90997, #152683, #153680, #128048, #174577, #76835, #200188, #61657, #108164, #169846, #36042, #92991, #24898, #84530, #134062, #149232, #10723, #118901, #148229, #8718, #101711, #99708, #54219, #162385, #68373, #117894, #161392, #130025, #147227, #7695, #37041, #40038, #38052, #21884, #70387, #41056, #132055, #53206, #25900, #145213, #9723, #22884, #191724, #98701, #116881, #177580, #193744, #146207, #69377, #55212, #164408, #86545, #87545, #71387, #115890, #178573, #163402, #133051, #39047, #72387, #57227, #195753, #114884, #194741, #176578, #131047, #160395, #83534, #56213, #179584, #6695, #23888, #192737, #100705, #85540, #102719, #183544, #103723, #59187, #74381, #150236, #184531, #138023, #182556, #152204, #196746, #60182, #180585, #62158, #42059, #153181, #107666, #30852, #121852, #168361, #169343, #198715, #165403, #45030, #26896, #199706, #88539, #91494, #73399, #46011, #14684, #181567, #135070, #76346, #151226, #11732, #58213, #43045, #485, #44039, #29857, #13688, #122843, #119882, #104711, #166401, #15678, #106688, #61171, #27897, #136046, #12715, #77339, #92499, #154188, #139005, #89540, #105699, #197721, #120856, #167386, #28882, #90522, #75355, #137025, #81286, #63158, #48996, #112638, #16669, #173338, #64163, #48010, #95481, #156167, #126802, #108671, #174330, #172332, #188510, #171346, #18661, #35800, #47012, #19645, #78318, #157167, #189503, #5453, #50978, #139991, #93492, #141980, #82281, #125828, #79324, #159132, #158153, #124837, #20629, #31841, #80307, #187531, #3468, #143973, #155179, #142970, #65145, #123822, #110652, #97446, #170349, #111652, #49987, #1480, #94485, #4447, #34810, #185520, #186537, #96465, #109666, #32835, #17666, #140994, #2482, #33821, #66137, #127800, #146980, #114630, #148987, #160145, #193491, #25659, #7447, #144966, #131812, #39793, #163148, #116640, #101457, #8467, #147989, #85288, #128794, #83290, #24651, #37799, #51966, #175320, #86300, #6447, #100465, #162144, #9478, #145965, #102474, #54970, #23640, #67136, #113625, #161142, #178330, #71142, #68128, #55967, #36786, #179341, #70141, #129779, #164161, #99462, #132808, #191476, #52954, #194494, #117644, #69131, #177336, #176329, #22639, #38807, #40804, #87304, #190494, #98452, #130799, #21636, #84286, #192490, #53973, #115646, #30604, #137774, #26648, #13450, #149979, #57975, #92257, #10477, #121607, #167143, #133813, #197483, #73156, #119647, #72137, #56977, #75114, #195504, #89296, #104470, #180342, #14436, #168118, #12480, #182314, #88291, #90278, #118651, #41810, #103478, #183302, #199460, #60927, #151962, #198468, #122601, #28642, #165156, #136782, #11485, #29614, #134826, #44784, #196505, #76099, #106437, #181329, #42808, #91246, #166155, #27656, #150988, #74141, #135813, #58950, #59939, #43794, #152937, #120618, #105457, #184291, #45772, #107425, #169097, #61913, #18427, #123584, #79079, #174097, #81061, #185278, #80077, #126571, #139748, #15436, #154934, #19412, #170105, #140752, #64910, #141746, #1235, #50747, #65896, #127570, #35566, #188272, #125592, #3236, #16431, #171101, #2240, #46770, #34577, #78079, #108429, #63923, #124594, #153941, #156930, #62914, #138764, #187289, #157922, #48760, #31599, #142738, #93248, #49745, #186289, #47769, #77095, #33582, #111414, #109422, #110414, #4218, #245, #173100, #32594, #172096, #189271, #94246, #112405, #155927, #17422, #95245, #96234, #37561, #52724, #132577, #131573, #98205, #194265, #5214, #192256, #160911, #68899, #55732, #66895, #54731, #53738, #117406, #22404, #147756, #143735, #85052, #130558, #128558, #67896, #116403, #8229, #70909, #179103, #115412, #190253, #83056, #51730, #97214, #158900, #84055, #159909, #20391, #177101, #144730, #82038, #113393, #23404, #175083, #99224, #36551, #161910, #69907, #193257, #146733, #178092, #38572, #39562, #100228, #21398, #6217, #101220, #129549 ),
 ( #191249, #145733, #114389, #176091, #7214, #162909, #24417, #86066, #9242, #134590, #10242, #44554, #198235, #42573, #12250, #56747, #120385, #40572, #122368, #102242, #13228, #167893, #91023, #182079, #28416, #29393, #58716, #163930, #43562, #25427, #59706, #87068, #151735, #133573, #106209, #74891, #41579, #195263, #136554, #11247, #148753, #71901, #103243, #60692, #104236, #90053, #26418, #118418, #14200, #75868, #27415, #164925, #199227, #105227, #88058, #180111, #149745, #166915, #72921, #181099, #196276, #121379, #183071, #152709, #137544, #57745, #119415, #165919, #89061, #150752, #73912, #135582, #197254, #168865, #92014, #141521, #10, #17191, #78845, #18195, #62678, #19184, #171865, #140523, #65668, #30370, #77854, #33354, #95013, #123353, #172867, #153707, #96009, #2013, #61684, #80833, #16199, #64685, #185046, #46534, #188044, #49514, #139521, #1004, #142510, #187063, #125367, #3988, #156701, #47538, #15203, #3008, #76862, #48533, #138532, #109192, #108193, #126347, #169875, #170871, #34348, #31368, #79852, #124359, #93018, #155696, #186054, #110187, #154706, #157693, #32362, #111177, #94015, #63692, #184057, #107194, #45540, #20161, #160670, #193018, #9004, #54495, #81806, #96989, #145493, #85826, #67659, #82814, #162669, #161670, #128327, #24175, #35336, #22162, #191012, #98980, #147514, #158671, #84809, #83813, #127330, #52488, #177857, #173868, #115167, #6973, #143493, #97970, #146488, #38329, #100985, #189042, #68653, #4978, #23166, #190026, #50517, #66664, #130309, #114148, #192004, #112180, #51500, #7979, #53490, #113160, #175849, #39326, #174850, #176860, #99985, #36316, #159662, #69663, #131330, #21159, #144496, #116167, #5979, #129316, #37322, #44320, #105979, #57509, #133331, #29160, #150517, #118176, #152481, #163683, #197022, #90797, #11002, #148514, #135348, #43325, #166680, #120155, #104992, #12015, #151504, #88824, #132338, #86828, #28181, #41337, #55493, #178859, #89823, #10004, #104000, #165678, #12996, #149505, #167664, #58488, #27177, #70671, #117163, #164684, #181845, #74659, #71664, #59471, #40325, #182838, #73676, #195022, #194030, #102998, #136326, #56498, #179867, #198001, #121144, #26178, #87819, #102001, #25186, #72674, #134351, #196033, #119178, #180863, #42339, #45314, #78613, #198994, #77628, #122137, #171635, #153475, #139297, #2775, #106964, #63457, #154475, #138309, #185819, #46299, #16959, #60462, #64451, #62445, #140287, #61457, #108962, #126121, #137313, #109956, #168638, #47306, #79616, #95774, #141285, #30138, #183824, #32130, #172628, #15968, #169643, #49285, #170642, #110943, #775, #187816, #91781, #1778, #93788, #14971, #184813, #33124, #125133, #34116, #13968, #155468, #76631, #199990, #123128, #75635, #107956, #124119, #31139, #92787, #186831, #48299, #94781, #156462, #17961, #115936, #97737, #35101, #21929, #130071, #53253, #6740, #191770, #37087, #38099, #175611, #18954, #173631, #114931, #128092, #142275, #65434, #176624, #96753, #190780, #52255, #99754, #36087, #192781, #145259, #113912, #39094, #3757, #51267, #68418, #161438, #158443, #146254, #127095, #69426, #98746, #19931, #54264, #189796, #22930, #81572, #143258, #84576, #7740, #112927, #174622, #177626, #160439, #83580, #157460, #131093, #20922, #188804, #80599, #50287, #111944, #4742, #82580, #66431, #159426, #144261, #5748, #67424, #129080, #152975, #43830, #24945, #75151, #133096, #106476, #85587, #92295, #152000, #168155, #148276, #198506, #153979, #23932, #199498, #193789, #136822, #169137, #185314, #30642, #55258, #70433, #121644, #61952, #105494, #58987, #138802, #137814, #101760, #283, #8764, #59977, #167180, #183339, #123619, #132099, #60964, #100750, #28679, #178619, #29652, #76136, #122638, #14474, #184328, #44821, #45810, #91284, #162431, #116926, #107461, #71432, #147273, #40082, #15476, #163448, #77133, #86593, #9768, #182352, #197519, #120654, #90314, #13486 ),
 ( #186324, #47806, #50780, #112440, #154970, #174129, #16466, #19446, #35600, #97246, #126604, #34610, #158934, #64945, #128591, #188306, #108464, #4253, #170141, #157955, #139784, #20423, #81094, #109456, #1272, #142772, #17457, #31636, #93285, #171139, #66928, #110450, #96269, #80111, #189303, #78115, #62949, #124629, #82073, #49783, #65932, #32628, #111448, #94282, #172131, #46805, #143766, #155960, #173135, #127604, #79113, #140786, #2275, #5247, #63958, #33617, #125627, #187325, #48796, #95280, #156963, #18460, #141779, #3273, #161941, #54763, #52752, #7245, #115442, #21427, #70940, #114421, #83087, #100260, #160942, #71933, #193289, #191277, #175114, #23436, #194297, #85083, #6248, #179135, #98237, #101252, #176122, #116437, #148785, #130592, #67927, #178126, #162941, #86097, #39593, #24448, #69940, #132608, #8260, #51761, #129581, #147788, #22435, #36582, #159940, #9274, #37593, #146767, #131604, #55763, #68930, #25460, #117437, #40603, #190285, #144763, #84084, #102274, #163962, #99255, #87100, #145763, #10274, #113422, #192288, #53768, #177133, #38604, #72951, #134621, #137575, #184090, #199259, #196305, #57775, #136583, #74920, #30403, #121408, #197283, #103275, #152740, #164955, #198263, #118450, #58746, #41610, #91053, #119445, #120415, #122400, #26448, #183102, #73943, #181130, #105257, #165950, #59739, #180141, #45573, #182106, #44583, #42604, #28446, #107226, #56777, #29422, #88090, #166943, #60726, #15234, #168897, #149776, #11278, #151764, #92049, #135612, #89091, #153738, #167922, #104268, #133603, #27450, #90082, #43591, #13257, #195296, #150783, #14230, #106240, #12278, #75901, #127366, #123385, #64719, #110219, #185077, #47571, #96042, #188078, #50551, #112211, #171900, #46566, #62711, #31400, #173901, #35370, #63724, #139554, #97022, #156736, #124393, #158703, #169907, #1038, #186088, #76893, #108227, #79884, #42, #155727, #170902, #93051, #80868, #34382, #78877, #48566, #154738, #16234, #77886, #142544, #109223, #49549, #4022, #189078, #18229, #126381, #65700, #95047, #138564, #141554, #61717, #157729, #32394, #111212, #94049, #17225, #172904, #140556, #2044, #19218, #125399, #187096, #33388, #3043, #40361, #83845, #8014, #53523, #162705, #5014, #174884, #113195, #55527, #38364, #69697, #128360, #84845, #190056, #145527, #102036, #147548, #51532, #146523, #193053, #6015, #81838, #21194, #85859, #36350, #7006, #131364, #54530, #67694, #117201, #132373, #194066, #20192, #116203, #192042, #177892, #82850, #37356, #68688, #98003, #101020, #144529, #159697, #130343, #191047, #143526, #23202, #129352, #66696, #115201, #24210, #176893, #52520, #9036, #114181, #39362, #175885, #99014, #160705, #100019, #22196, #161706, #70705, #178893, #135383, #90828, #151538, #14000, #198034, #42370, #181877, #120187, #89855, #180895, #75667, #183859, #152512, #179903, #166711, #103035, #11034, #45346, #163719, #74693, #43356, #86863, #150548, #29194, #41369, #12047, #136358, #13027, #72710, #60493, #137344, #199024, #25221, #59502, #197053, #28215, #26212, #104033, #88855, #195056, #44352, #87851, #56534, #73711, #134382, #148547, #121177, #164717, #10038, #58521, #167697, #105027, #149539, #122169, #71698, #182871, #196068, #118212, #133365, #106011, #165712, #57541, #119210, #27209, #170676, #79651, #63492, #2809, #109990, #139330, #16994, #93821, #1813, #77661, #64487, #110979, #141320, #200023, #78648, #123161, #169675, #172664, #106998, #48335, #155501, #91815, #47340, #46333, #92821, #168671, #15004, #125167, #153507, #62482, #809, #138343, #126154, #156496, #124154, #140323, #184849, #76664, #61491, #187850, #107989, #171670, #49319, #30172, #31171, #154507, #16003, #185854, #108995, #32164, #186866, #33159, #17998, #94818, #180553, #91464, #121820, #88506, #42027, #60151, #58184, #149200, #134028, #150202, #107637, #151197, #75325, #120825, #29827, #72354, #103691, #165370, #122812 ),
 ( #11700, #184502, #14653, #26864, #57194, #105668, #45982, #27866, #43015, #169314, #183515, #73367, #87512, #195721, #182525, #12685, #59156, #10690, #118869, #44998, #44006, #135039, #74351, #137991, #196715, #136995, #167354, #119852, #181536, #106658, #198684, #61140, #104682, #28852, #166369, #89507, #136017, #197691, #90492, #152174, #13657, #168331, #153151, #76313, #199674, #123793, #157138, #189475, #171318, #108641, #95453, #3441, #126775, #80280, #65117, #110622, #111624, #48968, #92469, #46981, #188480, #1451, #15649, #138976, #49960, #170319, #64135, #125799, #173309, #109635, #66109, #18634, #187501, #112612, #77307, #124808, #141952, #34784, #31811, #19618, #454, #142941, #172304, #93462, #127775, #63129, #96439, #155148, #16641, #158126, #81260, #4423, #78288, #139962, #33793, #50953, #30821, #154158, #94457, #62129, #185491, #186508, #47982, #32805, #156138, #17636, #79296, #140965, #2453, #163121, #67108, #23615, #114602, #98421, #145939, #6420, #177309, #159106, #24624, #22611, #38781, #21605, #69104, #86272, #97420, #70114, #128766, #7420, #39766, #55939, #192462, #132781, #176299, #129753, #9450, #8441, #175292, #71115, #82252, #130770, #37771, #53945, #194468, #143943, #131785, #115621, #174304, #99434, #147963, #20600, #162118, #100437, #5424, #144938, #193465, #85262, #35773, #190465, #146953, #51938, #160118, #113598, #36758, #83264, #161115, #68101, #191450, #54942, #52927, #84257, #116614, #178302, #101430, #170621, #108940, #2754, #155448, #125111, #64430, #19910, #80579, #143238, #127075, #171616, #110923, #49265, #18934, #109934, #4721, #112907, #81552, #32110, #95754, #93767, #140265, #174601, #92765, #3737, #172609, #15947, #79595, #16938, #1757, #154455, #139277, #157439, #77606, #33104, #186809, #62425, #96733, #50266, #94760, #126100, #78592, #754, #124097, #158422, #185796, #65414, #66410, #128072, #34096, #142253, #189775, #188783, #47284, #111924, #63435, #173610, #48279, #35080, #156442, #51247, #17941, #141264, #187796, #8744, #6719, #97716, #82559, #37066, #56240, #99732, #23913, #69405, #178600, #20901, #190760, #129059, #71412, #54243, #85567, #144241, #100730, #5725, #161416, #159406, #67404, #98725, #117921, #22908, #147253, #131071, #40063, #52235, #113892, #175590, #133076, #115915, #70414, #160419, #162411, #21908, #84554, #36067, #163428, #83559, #132081, #193770, #145238, #68397, #130049, #101740, #191749, #146232, #55239, #116907, #53232, #194766, #148255, #9748, #114908, #24926, #7719, #86571, #176602, #38076, #192760, #177605, #39073, #103751, #72414, #89568, #150265, #61199, #182584, #180613, #164434, #12744, #183573, #74409, #195781, #168390, #87571, #90550, #165430, #44067, #119909, #57254, #118928, #151254, #42086, #11759, #136075, #106716, #167414, #29885, #13717, #58241, #197749, #59216, #105727, #196773, #91523, #199733, #153210, #26925, #28910, #88567, #73426, #179610, #41083, #152232, #120885, #102746, #166430, #135097, #181595, #25928, #149258, #75383, #10750, #43072, #104739, #134091, #45058, #137055, #27925, #198745, #60210, #121880, #14715, #76375, #138052, #95512, #50019, #173371, #2513, #110682, #111684, #141026, #4479, #64193, #184559, #80339, #46040, #33852, #15708, #126835, #157198, #123852, #77368, #18692, #93525, #172362, #156198, #65176, #107695, #139036, #516, #158186, #125860, #142011, #30882, #187560, #92529, #48041, #143001, #34841, #154218, #49027, #3500, #108701, #169374, #185550, #188541, #62188, #109697, #96496, #19676, #170380, #81318, #122871, #47044, #31871, #155210, #94516, #16699, #78349, #140023, #171379, #1512, #63189, #124869, #186568, #32866, #17698, #79355, #69164, #67167, #51009, #99494, #70175, #161174, #82313, #57758, #174362, #177367, #190523, #130831, #6479, #144003, #5484, #176361, #128824, #98484, #37834, #193526, #54005, #119428, #100496, #144998, #84318, #22671, #192522, #83321 ),
 ( #51997, #175350, #66169, #112670, #115679, #189537, #68159, #160177, #35832, #131843, #23673, #129811, #145997, #113656, #97478, #159164, #181112, #20659, #38838, #42586, #104249, #7480, #162175, #165932, #85321, #150765, #147013, #127831, #8498, #36818, #27430, #21667, #89074, #191510, #52987, #114665, #185060, #183085, #73926, #58729, #13241, #32376, #75883, #15217, #197267, #1019, #60706, #76876, #59723, #107209, #62692, #135595, #108210, #105240, #45555, #77868, #94029, #139535, #166928, #182092, #30384, #170885, #152724, #167907, #47552, #46548, #74904, #109205, #120399, #168879, #137558, #184071, #12262, #43576, #169889, #92031, #28429, #199241, #124374, #90066, #24, #153721, #151748, #44568, #31383, #123367, #186069, #136568, #138546, #198248, #121393, #106223, #29407, #91037, #122382, #14214, #61698, #93032, #154720, #16213, #48547, #20175, #19200, #191028, #112194, #81821, #128341, #143508, #141536, #82830, #4994, #5996, #190040, #34363, #173883, #35353, #66679, #172883, #67675, #175866, #144511, #171880, #158686, #95027, #3025, #37338, #155709, #51514, #97004, #78858, #142526, #18209, #64701, #17205, #2026, #113176, #140538, #96024, #49529, #125381, #159679, #174866, #157710, #127346, #33369, #63706, #187078, #21175, #110201, #36332, #129333, #52503, #97985, #114163, #156717, #79867, #126363, #188059, #111192, #80849, #4004, #65683, #189060, #50532, #133346, #100000, #53505, #71679, #69679, #160685, #145508, #115182, #87833, #6989, #10020, #23182, #102017, #39342, #176875, #38344, #161686, #84825, #86844, #146505, #26194, #148529, #149519, #195037, #177874, #117180, #55510, #25202, #116183, #11016, #119192, #72689, #7995, #163700, #131346, #193034, #180877, #98996, #56514, #178875, #22177, #85842, #54511, #101001, #83827, #68670, #118192, #130324, #162686, #24192, #192021, #103015, #179883, #147532, #70688, #9020, #132354, #194046, #164698, #40342, #41351, #134364, #196048, #57523, #30151, #31150, #60473, #124132, #183838, #104014, #200003, #165692, #153487, #135364, #46312, #76643, #43338, #197035, #14983, #13009, #27190, #88837, #105006, #62459, #105991, #91793, #75647, #184826, #150530, #58502, #120168, #77639, #122149, #138321, #12029, #106977, #73692, #167677, #42352, #169654, #181859, #168651, #61469, #28195, #166692, #89837, #107967, #151518, #29174, #123140, #92798, #74673, #139308, #154486, #15980, #136340, #787, #13981, #198015, #59484, #121158, #90810, #182851, #44334, #152493, #137325, #199006, #45327, #67434, #188814, #186843, #170654, #18965, #189806, #80611, #143269, #1791, #142288, #3768, #19942, #64465, #20932, #173643, #65445, #185831, #32142, #79628, #35112, #96764, #125144, #174632, #93799, #97749, #127107, #63469, #82590, #17974, #66441, #48312, #109967, #51278, #36097, #112939, #171646, #33136, #50297, #111954, #144271, #158453, #49296, #155479, #4752, #16971, #81583, #78625, #110955, #140300, #128102, #94794, #172639, #159437, #156473, #5758, #126132, #141296, #157472, #2786, #47318, #187827, #108973, #34127, #95786, #176634, #23943, #117952, #52265, #24956, #21940, #162442, #194796, #10780, #56269, #83590, #98756, #147284, #87600, #69436, #84586, #164463, #163458, #130083, #25957, #37097, #85597, #192792, #100760, #149286, #160449, #86603, #8774, #129091, #54274, #179643, #175623, #116937, #70443, #145270, #99764, #148286, #40093, #102776, #190791, #132109, #6751, #114941, #68430, #113923, #191782, #115947, #53264, #38109, #193802, #161449, #22940, #146266, #55268, #177637, #7752, #178630, #131104, #101771, #39104, #9780, #71442, #133107, #41112, #90584, #134122, #88599, #106749, #43104, #57283, #180643, #167446, #154252, #118957, #166460, #121915, #60244, #11791, #61234, #42118, #184594, #28943, #150295, #107729, #104772, #153247, #73455, #135128, #76410, #122906, #138086, #196802, #58270, #75418, #13750, #169411, #183608, #136107, #103780, #91559, #165460 ),
 ( #195811, #26956, #119939, #92564, #197783, #45092, #105760, #14749, #181624, #27957, #89598, #30916, #152265, #168424, #151286, #137092, #12775, #59249, #72447, #199767, #74440, #198778, #29919, #120918, #182617, #44102, #46075, #31906, #2549, #126871, #3535, #63225, #112706, #127868, #189572, #97514, #188578, #187596, #80376, #78383, #32901, #141063, #47077, #96531, #140059, #108738, #125896, #186603, #15743, #18728, #16735, #550, #49065, #19711, #110720, #93559, #4515, #123889, #50059, #1550, #142048, #156234, #155245, #124905, #48075, #109731, #65212, #171415, #143037, #111720, #66208, #173406, #94554, #33891, #172402, #34877, #17736, #51044, #35868, #174398, #79393, #158221, #64231, #95548, #77402, #157235, #81353, #139072, #170414, #62221, #185587, #194561, #115715, #190559, #70211, #114704, #5521, #131878, #38874, #39859, #177403, #20695, #175385, #193563, #129847, #144039, #67201, #116705, #36854, #192558, #54041, #55035, #37872, #56031, #147049, #100531, #40869, #128859, #53023, #8532, #178395, #98521, #148052, #52033, #71209, #162210, #160214, #117709, #191546, #101525, #21704, #83358, #163216, #9543, #24718, #145034, #6516, #23709, #85356, #179405, #86367, #22707, #113690, #132872, #68195, #159200, #176397, #84354, #99530, #82351, #161212, #146032, #7515, #69200, #130868, #42870, #26716, #74205, #134891, #105522, #87369, #91310, #151049, #167208, #150048, #197545, #153002, #25723, #198534, #195571, #135874, #168182, #184354, #29678, #57044, #72206, #120680, #60992, #104535, #58038, #137843, #136849, #103546, #199524, #10542, #59013, #166216, #182379, #122666, #133880, #60005, #43857, #102543, #27717, #14501, #149054, #90341, #28705, #118718, #73220, #121672, #13512, #76163, #164226, #152026, #180407, #88355, #41879, #165221, #11554, #89360, #196567, #119708, #181392, #12540, #75177, #183367, #44849, #106505, #96292, #125653, #33641, #34633, #63983, #127628, #187350, #107487, #3297, #169165, #156987, #138830, #49808, #80134, #46832, #310, #18485, #16494, #30669, #92322, #108492, #65957, #109485, #95303, #79141, #188329, #154007, #61978, #123644, #81116, #48820, #141804, #15503, #110473, #77160, #171168, #45836, #173158, #185341, #172155, #64969, #31664, #170171, #93314, #111473, #154998, #32655, #126628, #157979, #78143, #142796, #19471, #4277, #139811, #1299, #17484, #62977, #124657, #186353, #94309, #47833, #155987, #140812, #2302, #99280, #159966, #70966, #192313, #190311, #174155, #22461, #193315, #84109, #5275, #178153, #97271, #100287, #113447, #53793, #129606, #66957, #128618, #51787, #175140, #177157, #36607, #116464, #38630, #39618, #23461, #67952, #7270, #145788, #115468, #6274, #101277, #9300, #162967, #98264, #161965, #21453, #83114, #189328, #50805, #85108, #68954, #112463, #176148, #144791, #191302, #35626, #158959, #146794, #20449, #52778, #114447, #82100, #54789, #8287, #37618, #160967, #130617, #24473, #69965, #131631, #143792, #86123, #147814, #57800, #152766, #59766, #40628, #58772, #105281, #118476, #194322, #133631, #198288, #148811, #119471, #43617, #120440, #180167, #29447, #44610, #106265, #14256, #166969, #104293, #197308, #195323, #149801, #181154, #163987, #13281, #56803, #25484, #42629, #103301, #132634, #135638, #41636, #117461, #165974, #136608, #27476, #10301, #121434, #102298, #28471, #164980, #182133, #72977, #71958, #26475, #88117, #11307, #90106, #134646, #183127, #151790, #167949, #74945, #196332, #150807, #89119, #91079, #12303, #55790, #179160, #87126, #73969, #78900, #15260, #123409, #160490, #75927, #187117, #32416, #199285, #62735, #138589, #185102, #137602, #122425, #140578, #60752, #154760, #169932, #45599, #82628, #36136, #77909, #47592, #92076, #184117, #107252, #144310, #168923, #48589, #5800, #129132, #155750, #63747, #67473, #94071, #30429, #17248, #153765, #97788, #76918, #112978, #70, #190830, #174671, #61741, #46591, #159477 ) ),
 .UNSPECIFIED., .T., .F., .T. ) 
 B_SPLINE_SURFACE_WITH_KNOTS ( ( 4, 3, 4 ),
 ( 3, 2, 2, 2, 2, 2, 2, 2, 2, 2, 2, 2, 2, 2, 2, 2, 2, 2, 2, 2, 2, 2, 2, 2, 2, 2, 2, 2, 2, 2, 2, 2, 2, 2, 2, 2, 2, 2, 2, 2, 2, 2, 2, 2, 2, 2, 2, 2, 2, 2, 2, 2, 2, 2, 2, 2, 2, 2, 2, 2, 2, 2, 2, 2, 2, 2, 2, 2, 2, 2, 2, 2, 2, 2, 2, 2, 2, 2, 2, 2, 2, 2, 2, 2, 2, 2, 2, 2, 2, 2, 2, 2, 2, 2, 2, 2, 2, 2, 2, 2, 2, 2, 2, 2, 2, 2, 2, 2, 2, 2, 2, 2, 2, 2, 2, 2, 2, 2, 2, 2, 2, 2, 2, 2, 2, 2, 2, 2, 2, 2, 2, 2, 2, 2, 2, 2, 2, 2, 2, 2, 2, 2, 2, 2, 2, 2, 2, 2, 2, 2, 2, 2, 2, 2, 2, 2, 2, 2, 2, 2, 2, 2, 2, 2, 2, 2, 2, 2, 2, 2, 2, 2, 2, 2, 2, 2, 2, 2, 2, 2, 2, 2, 2, 2, 2, 2, 2, 2, 2, 2, 2, 2, 2, 2, 2, 2, 2, 2, 2, 2, 2, 2, 2, 2, 2, 2, 2, 2, 2, 2, 2, 2, 2, 2, 2, 2, 2, 2, 2, 2, 2, 2, 2, 2, 2, 2, 2, 2, 3 ),
 ( 0.000000000000000000, 0.5000000000000000000, 1.000000000000000000 ),
 ( 0.000000000000000000, 0.004385964912280701511, 0.008771929824561403022, 0.01315789473684210453, 0.01754385964912280604, 0.02192982456140350755, 0.02631578947368420907, 0.03070175438596491058, 0.03508771929824561209, 0.03947368421052631360, 0.04385964912280701511, 0.04824561403508771662, 0.05263157894736841813, 0.05701754385964911964, 0.06140350877192982115, 0.06578947368421052266, 0.07017543859649122417, 0.07456140350877192569, 0.07894736842105262720, 0.08333333333333332871, 0.08771929824561403022, 0.09210526315789473173, 0.09649122807017543324, 0.1008771929824561348, 0.1052631578947368363, 0.1096491228070175378, 0.1140350877192982393, 0.1184210526315789408, 0.1228070175438596423, 0.1271929824561403577, 0.1315789473684210453, 0.1359649122807017607, 0.1403508771929824483, 0.1447368421052631637, 0.1491228070175438514, 0.1535087719298245668, 0.1578947368421052544, 0.1622807017543859698, 0.1666666666666666574, 0.1710526315789473728, 0.1754385964912280604, 0.1798245614035087758, 0.1842105263157894635, 0.1885964912280701788, 0.1929824561403508665, 0.1973684210526315819, 0.2017543859649122695, 0.2061403508771929849, 0.2105263157894736725, 0.2149122807017543879, 0.2192982456140350755, 0.2236842105263157909, 0.2280701754385964786, 0.2324561403508771940, 0.2368421052631578816, 0.2412280701754385970, 0.2456140350877192846, 0.2500000000000000000, 0.2543859649122807154, 0.2587719298245614308, 0.2631578947368420907, 0.2675438596491228060, 0.2719298245614035214, 0.2763157894736842368, 0.2807017543859648967, 0.2850877192982456121, 0.2894736842105263275, 0.2938596491228070429, 0.2982456140350877027, 0.3026315789473684181, 0.3070175438596491335, 0.3114035087719298489, 0.3157894736842105088, 0.3201754385964912242, 0.3245614035087719396, 0.3289473684210526550, 0.3333333333333333148, 0.3377192982456140302, 0.3421052631578947456, 0.3464912280701754610, 0.3508771929824561209, 0.3552631578947368363, 0.3596491228070175517, 0.3640350877192982670, 0.3684210526315789269, 0.3728070175438596423, 0.3771929824561403577, 0.3815789473684210731, 0.3859649122807017330, 0.3903508771929824483, 0.3947368421052631637, 0.3991228070175438791, 0.4035087719298245390, 0.4078947368421052544, 0.4122807017543859698, 0.4166666666666666852, 0.4210526315789473450, 0.4254385964912280604, 0.4298245614035087758, 0.4342105263157894912, 0.4385964912280701511, 0.4429824561403508665, 0.4473684210526315819, 0.4517543859649122973, 0.4561403508771929571, 0.4605263157894736725, 0.4649122807017543879, 0.4692982456140351033, 0.4736842105263157632, 0.4780701754385964786, 0.4824561403508771940, 0.4868421052631579093, 0.4912280701754385692, 0.4956140350877192846, 0.5000000000000000000, 0.5043859649122807154, 0.5087719298245614308, 0.5131578947368421462, 0.5175438596491228616, 0.5219298245614034659, 0.5263157894736841813, 0.5307017543859648967, 0.5350877192982456121, 0.5394736842105263275, 0.5438596491228070429, 0.5482456140350877583, 0.5526315789473684736, 0.5570175438596490780, 0.5614035087719297934, 0.5657894736842105088, 0.5701754385964912242, 0.5745614035087719396, 0.5789473684210526550, 0.5833333333333333703, 0.5877192982456140857, 0.5921052631578946901, 0.5964912280701754055, 0.6008771929824561209, 0.6052631578947368363, 0.6096491228070175517, 0.6140350877192982670, 0.6184210526315789824, 0.6228070175438596978, 0.6271929824561403022, 0.6315789473684210176, 0.6359649122807017330, 0.6403508771929824483, 0.6447368421052631637, 0.6491228070175438791, 0.6535087719298245945, 0.6578947368421053099, 0.6622807017543859143, 0.6666666666666666297, 0.6710526315789473450, 0.6754385964912280604, 0.6798245614035087758, 0.6842105263157894912, 0.6885964912280702066, 0.6929824561403509220, 0.6973684210526315264, 0.7017543859649122417, 0.7061403508771929571, 0.7105263157894736725, 0.7149122807017543879, 0.7192982456140351033, 0.7236842105263158187, 0.7280701754385965341, 0.7324561403508771384, 0.7368421052631578538, 0.7412280701754385692, 0.7456140350877192846, 0.7500000000000000000, 0.7543859649122807154, 0.7587719298245614308, 0.7631578947368421462, 0.7675438596491228616, 0.7719298245614034659, 0.7763157894736841813, 0.7807017543859648967, 0.7850877192982456121, 0.7894736842105263275, 0.7938596491228070429, 0.7982456140350877583, 0.8026315789473684736, 0.8070175438596490780, 0.8114035087719297934, 0.8157894736842105088, 0.8201754385964912242, 0.8245614035087719396, 0.8289473684210526550, 0.8333333333333333703, 0.8377192982456140857, 0.8421052631578946901, 0.8464912280701754055, 0.8508771929824561209, 0.8552631578947368363, 0.8596491228070175517, 0.8640350877192982670, 0.8684210526315789824, 0.8728070175438596978, 0.8771929824561403022, 0.8815789473684210176, 0.8859649122807017330, 0.8903508771929824483, 0.8947368421052631637, 0.8991228070175438791, 0.9035087719298245945, 0.9078947368421053099, 0.9122807017543859143, 0.9166666666666666297, 0.9210526315789473450, 0.9254385964912280604, 0.9298245614035087758, 0.9342105263157894912, 0.9385964912280702066, 0.9429824561403509220, 0.9473684210526315264, 0.9517543859649122417, 0.9561403508771929571, 0.9605263157894736725, 0.9649122807017543879, 0.9692982456140351033, 0.9736842105263158187, 0.9780701754385965341, 0.9824561403508771384, 0.9868421052631578538, 0.9912280701754385692, 0.9956140350877192846, 1.000000000000000000 ),
 .UNSPECIFIED. ) 
 GEOMETRIC_REPRESENTATION_ITEM ( )  RATIONAL_B_SPLINE_SURFACE ( (
 ( 1.000000000000000000, 0.9659258262890683122, 1.000000000000000000, 0.9659258262890683122, 1.000000000000000000, 0.9659258262890683122, 1.000000000000000000, 0.9659258262890683122, 1.000000000000000000, 0.9659258262890683122, 1.000000000000000000, 0.9659258262890683122, 1.000000000000000000, 0.9659258262890683122, 1.000000000000000000, 0.9659258262890683122, 1.000000000000000000, 0.9659258262890683122, 1.000000000000000000, 0.9659258262890683122, 1.000000000000000000, 0.9659258262890683122, 1.000000000000000000, 0.9659258262890683122, 1.000000000000000000, 0.9659258262890683122, 1.000000000000000000, 0.9659258262890683122, 1.000000000000000000, 0.9659258262890683122, 1.000000000000000000, 0.9659258262890683122, 1.000000000000000000, 0.9659258262890683122, 1.000000000000000000, 0.9659258262890683122, 1.000000000000000000, 0.9659258262890683122, 1.000000000000000000, 0.9659258262890683122, 1.000000000000000000, 0.9659258262890683122, 1.000000000000000000, 0.9659258262890683122, 1.000000000000000000, 0.9659258262890683122, 1.000000000000000000, 0.9659258262890683122, 1.000000000000000000, 0.9659258262890683122, 1.000000000000000000, 0.9659258262890683122, 1.000000000000000000, 0.9659258262890683122, 1.000000000000000000, 0.9659258262890683122, 1.000000000000000000, 0.9659258262890683122, 1.000000000000000000, 0.9659258262890683122, 1.000000000000000000, 0.9659258262890683122, 1.000000000000000000, 0.9659258262890683122, 1.000000000000000000, 0.9659258262890683122, 1.000000000000000000, 0.9659258262890683122, 1.000000000000000000, 0.9659258262890683122, 1.000000000000000000, 0.9659258262890683122, 1.000000000000000000, 0.9659258262890683122, 1.000000000000000000, 0.9659258262890683122, 1.000000000000000000, 0.9659258262890683122, 1.000000000000000000, 0.9659258262890683122, 1.000000000000000000, 0.9659258262890683122, 1.000000000000000000, 0.9659258262890683122, 1.000000000000000000, 0.9659258262890683122, 1.000000000000000000, 0.9659258262890683122, 1.000000000000000000, 0.9659258262890683122, 1.000000000000000000, 0.9659258262890683122, 1.000000000000000000, 0.9659258262890683122, 1.000000000000000000, 0.9659258262890683122, 1.000000000000000000, 0.9659258262890683122, 1.000000000000000000, 0.9659258262890683122, 1.000000000000000000, 0.9659258262890683122, 1.000000000000000000, 0.9659258262890683122, 1.000000000000000000, 0.9659258262890683122, 1.000000000000000000, 0.9659258262890683122, 1.000000000000000000, 0.9659258262890683122, 1.000000000000000000, 0.9659258262890683122, 1.000000000000000000, 0.9659258262890683122, 1.000000000000000000, 0.9659258262890683122, 1.000000000000000000, 0.9659258262890683122, 1.000000000000000000, 0.9659258262890683122, 1.000000000000000000, 0.9659258262890683122, 1.000000000000000000, 0.9659258262890683122, 1.000000000000000000, 0.9659258262890683122, 1.000000000000000000, 0.9659258262890683122, 1.000000000000000000, 0.9659258262890683122, 1.000000000000000000, 0.9659258262890683122, 1.000000000000000000, 0.9659258262890683122, 1.000000000000000000, 0.9659258262890683122, 1.000000000000000000, 0.9659258262890683122, 1.000000000000000000, 0.9659258262890683122, 1.000000000000000000, 0.9659258262890683122, 1.000000000000000000, 0.9659258262890683122, 1.000000000000000000, 0.9659258262890683122, 1.000000000000000000, 0.9659258262890683122, 1.000000000000000000, 0.9659258262890683122, 1.000000000000000000, 0.9659258262890683122, 1.000000000000000000, 0.9659258262890683122, 1.000000000000000000, 0.9659258262890683122, 1.000000000000000000, 0.9659258262890683122, 1.000000000000000000, 0.9659258262890683122, 1.000000000000000000, 0.9659258262890683122, 1.000000000000000000, 0.9659258262890683122, 1.000000000000000000, 0.9659258262890683122, 1.000000000000000000, 0.9659258262890683122, 1.000000000000000000, 0.9659258262890683122, 1.000000000000000000, 0.9659258262890683122, 1.000000000000000000, 0.9659258262890683122, 1.000000000000000000, 0.9659258262890683122, 1.000000000000000000, 0.9659258262890683122, 1.000000000000000000, 0.9659258262890683122, 1.000000000000000000, 0.9659258262890683122, 1.000000000000000000, 0.9659258262890683122, 1.000000000000000000, 0.9659258262890683122, 1.000000000000000000, 0.9659258262890683122, 1.000000000000000000, 0.9659258262890683122, 1.000000000000000000, 0.9659258262890683122, 1.000000000000000000, 0.9659258262890683122, 1.000000000000000000, 0.9659258262890683122, 1.000000000000000000, 0.9659258262890683122, 1.000000000000000000, 0.9659258262890683122, 1.000000000000000000, 0.9659258262890683122, 1.000000000000000000, 0.9659258262890683122, 1.000000000000000000, 0.9659258262890683122, 1.000000000000000000, 0.9659258262890683122, 1.000000000000000000, 0.9659258262890683122, 1.000000000000000000, 0.9659258262890683122, 1.000000000000000000, 0.9659258262890683122, 1.000000000000000000, 0.9659258262890683122, 1.000000000000000000, 0.9659258262890683122, 1.000000000000000000, 0.9659258262890683122, 1.000000000000000000, 0.9659258262890683122, 1.000000000000000000, 0.9659258262890683122, 1.000000000000000000, 0.9659258262890683122, 1.000000000000000000, 0.9659258262890683122, 1.000000000000000000, 0.9659258262890683122, 1.000000000000000000, 0.9659258262890683122, 1.000000000000000000, 0.9659258262890683122, 1.000000000000000000, 0.9659258262890683122, 1.000000000000000000, 0.9659258262890683122, 1.000000000000000000, 0.9659258262890683122, 1.000000000000000000, 0.9659258262890683122, 1.000000000000000000, 0.9659258262890683122, 1.000000000000000000, 0.9659258262890683122, 1.000000000000000000, 0.9659258262890683122, 1.000000000000000000, 0.9659258262890683122, 1.000000000000000000, 0.9659258262890683122, 1.000000000000000000, 0.9659258262890683122, 1.000000000000000000, 0.9659258262890683122, 1.000000000000000000, 0.9659258262890683122, 1.000000000000000000, 0.9659258262890683122, 1.000000000000000000, 0.9659258262890683122, 1.000000000000000000, 0.9659258262890683122, 1.000000000000000000, 0.9659258262890683122, 1.000000000000000000, 0.9659258262890683122, 1.000000000000000000, 0.9659258262890683122, 1.000000000000000000, 0.9659258262890683122, 1.000000000000000000, 0.9659258262890683122, 1.000000000000000000, 0.9659258262890683122, 1.000000000000000000, 0.9659258262890683122, 1.000000000000000000, 0.9659258262890683122, 1.000000000000000000, 0.9659258262890683122, 1.000000000000000000, 0.9659258262890683122, 1.000000000000000000, 0.9659258262890683122, 1.000000000000000000, 0.9659258262890683122, 1.000000000000000000, 0.9659258262890683122, 1.000000000000000000, 0.9659258262890683122, 1.000000000000000000, 0.9659258262890683122, 1.000000000000000000, 0.9659258262890683122, 1.000000000000000000, 0.9659258262890683122, 1.000000000000000000, 0.9659258262890683122, 1.000000000000000000, 0.9659258262890683122, 1.000000000000000000, 0.9659258262890683122, 1.000000000000000000, 0.9659258262890683122, 1.000000000000000000, 0.9659258262890683122, 1.000000000000000000, 0.9659258262890683122, 1.000000000000000000, 0.9659258262890683122, 1.000000000000000000, 0.9659258262890683122, 1.000000000000000000, 0.9659258262890683122, 1.000000000000000000, 0.9659258262890683122, 1.000000000000000000, 0.9659258262890683122, 1.000000000000000000, 0.9659258262890683122, 1.000000000000000000, 0.9659258262890683122, 1.000000000000000000, 0.9659258262890683122, 1.000000000000000000, 0.9659258262890683122, 1.000000000000000000, 0.9659258262890683122, 1.000000000000000000, 0.9659258262890683122, 1.000000000000000000, 0.9659258262890683122, 1.000000000000000000, 0.9659258262890683122, 1.000000000000000000, 0.9659258262890683122, 1.000000000000000000, 0.9659258262890683122, 1.000000000000000000, 0.9659258262890683122, 1.000000000000000000, 0.9659258262890683122, 1.000000000000000000, 0.9659258262890683122, 1.000000000000000000, 0.9659258262890683122, 1.000000000000000000, 0.9659258262890683122, 1.000000000000000000, 0.9659258262890683122, 1.000000000000000000, 0.9659258262890683122, 1.000000000000000000, 0.9659258262890683122, 1.000000000000000000, 0.9659258262890683122, 1.000000000000000000, 0.9659258262890683122, 1.000000000000000000, 0.9659258262890683122, 1.000000000000000000, 0.9659258262890683122, 1.000000000000000000, 0.9659258262890683122, 1.000000000000000000, 0.9659258262890683122, 1.000000000000000000, 0.9659258262890683122, 1.000000000000000000, 0.9659258262890683122, 1.000000000000000000, 0.9659258262890683122, 1.000000000000000000, 0.9659258262890683122, 1.000000000000000000, 0.9659258262890683122, 1.000000000000000000, 0.9659258262890683122, 1.000000000000000000, 0.9659258262890683122, 1.000000000000000000, 0.9659258262890683122, 1.000000000000000000, 0.9659258262890683122, 1.000000000000000000, 0.9659258262890683122, 1.000000000000000000, 0.9659258262890683122, 1.000000000000000000, 0.9659258262890683122, 1.000000000000000000, 0.9659258262890683122, 1.000000000000000000, 0.9659258262890683122, 1.000000000000000000, 0.9659258262890683122, 1.000000000000000000, 0.9659258262890683122, 1.000000000000000000, 0.9659258262890683122, 1.000000000000000000, 0.9659258262890683122, 1.000000000000000000, 0.9659258262890683122, 1.000000000000000000, 0.9659258262890683122, 1.000000000000000000, 0.9659258262890683122, 1.000000000000000000, 0.9659258262890683122, 1.000000000000000000, 0.9659258262890683122, 1.000000000000000000, 0.9659258262890683122, 1.000000000000000000, 0.9659258262890683122, 1.000000000000000000, 0.9659258262890683122, 1.000000000000000000, 0.9659258262890683122, 1.000000000000000000, 0.9659258262890683122, 1.000000000000000000, 0.9659258262890683122, 1.000000000000000000, 0.9659258262890683122, 1.000000000000000000, 0.9659258262890683122, 1.000000000000000000, 0.9659258262890683122, 1.000000000000000000, 0.9659258262890683122, 1.000000000000000000, 0.9659258262890683122, 1.000000000000000000, 0.9659258262890683122, 1.000000000000000000, 0.9659258262890683122, 1.000000000000000000, 0.9659258262890683122, 1.000000000000000000, 0.9659258262890683122, 1.000000000000000000, 0.9659258262890683122, 1.000000000000000000, 0.9659258262890683122, 1.000000000000000000, 0.9659258262890683122, 1.000000000000000000, 0.9659258262890683122, 1.000000000000000000, 0.9659258262890683122, 1.000000000000000000, 0.9659258262890683122, 1.000000000000000000),
 ( 0.3333333333333333703, 0.3219752754296894559, 0.3333333333333333703, 0.3219752754296894559, 0.3333333333333333703, 0.3219752754296894559, 0.3333333333333333703, 0.3219752754296894559, 0.3333333333333333703, 0.3219752754296894559, 0.3333333333333333703, 0.3219752754296894559, 0.3333333333333333703, 0.3219752754296894559, 0.3333333333333333703, 0.3219752754296894559, 0.3333333333333333703, 0.3219752754296894559, 0.3333333333333333703, 0.3219752754296894559, 0.3333333333333333703, 0.3219752754296894559, 0.3333333333333333703, 0.3219752754296894559, 0.3333333333333333703, 0.3219752754296894559, 0.3333333333333333703, 0.3219752754296894559, 0.3333333333333333703, 0.3219752754296894559, 0.3333333333333333703, 0.3219752754296894559, 0.3333333333333333703, 0.3219752754296894559, 0.3333333333333333703, 0.3219752754296894559, 0.3333333333333333703, 0.3219752754296894559, 0.3333333333333333703, 0.3219752754296894559, 0.3333333333333333703, 0.3219752754296894559, 0.3333333333333333703, 0.3219752754296894559, 0.3333333333333333703, 0.3219752754296894559, 0.3333333333333333703, 0.3219752754296894559, 0.3333333333333333703, 0.3219752754296894559, 0.3333333333333333703, 0.3219752754296894559, 0.3333333333333333703, 0.3219752754296894559, 0.3333333333333333703, 0.3219752754296894559, 0.3333333333333333703, 0.3219752754296894559, 0.3333333333333333703, 0.3219752754296894559, 0.3333333333333333703, 0.3219752754296894559, 0.3333333333333333703, 0.3219752754296894559, 0.3333333333333333703, 0.3219752754296894559, 0.3333333333333333703, 0.3219752754296894559, 0.3333333333333333703, 0.3219752754296894559, 0.3333333333333333703, 0.3219752754296894559, 0.3333333333333333703, 0.3219752754296894559, 0.3333333333333333703, 0.3219752754296894559, 0.3333333333333333703, 0.3219752754296894559, 0.3333333333333333703, 0.3219752754296894559, 0.3333333333333333703, 0.3219752754296894559, 0.3333333333333333703, 0.3219752754296894559, 0.3333333333333333703, 0.3219752754296894559, 0.3333333333333333703, 0.3219752754296894559, 0.3333333333333333703, 0.3219752754296894559, 0.3333333333333333703, 0.3219752754296894559, 0.3333333333333333703, 0.3219752754296894559, 0.3333333333333333703, 0.3219752754296894559, 0.3333333333333333703, 0.3219752754296894559, 0.3333333333333333703, 0.3219752754296894559, 0.3333333333333333703, 0.3219752754296894559, 0.3333333333333333703, 0.3219752754296894559, 0.3333333333333333703, 0.3219752754296894559, 0.3333333333333333703, 0.3219752754296894559, 0.3333333333333333703, 0.3219752754296894559, 0.3333333333333333703, 0.3219752754296894559, 0.3333333333333333703, 0.3219752754296894559, 0.3333333333333333703, 0.3219752754296894559, 0.3333333333333333703, 0.3219752754296894559, 0.3333333333333333703, 0.3219752754296894559, 0.3333333333333333703, 0.3219752754296894559, 0.3333333333333333703, 0.3219752754296894559, 0.3333333333333333703, 0.3219752754296894559, 0.3333333333333333703, 0.3219752754296894559, 0.3333333333333333703, 0.3219752754296894559, 0.3333333333333333703, 0.3219752754296894559, 0.3333333333333333703, 0.3219752754296894559, 0.3333333333333333703, 0.3219752754296894559, 0.3333333333333333703, 0.3219752754296894559, 0.3333333333333333703, 0.3219752754296894559, 0.3333333333333333703, 0.3219752754296894559, 0.3333333333333333703, 0.3219752754296894559, 0.3333333333333333703, 0.3219752754296894559, 0.3333333333333333703, 0.3219752754296894559, 0.3333333333333333703, 0.3219752754296894559, 0.3333333333333333703, 0.3219752754296894559, 0.3333333333333333703, 0.3219752754296894559, 0.3333333333333333703, 0.3219752754296894559, 0.3333333333333333703, 0.3219752754296894559, 0.3333333333333333703, 0.3219752754296894559, 0.3333333333333333703, 0.3219752754296894559, 0.3333333333333333703, 0.3219752754296894559, 0.3333333333333333703, 0.3219752754296894559, 0.3333333333333333703, 0.3219752754296894559, 0.3333333333333333703, 0.3219752754296894559, 0.3333333333333333703, 0.3219752754296894559, 0.3333333333333333703, 0.3219752754296894559, 0.3333333333333333703, 0.3219752754296894559, 0.3333333333333333703, 0.3219752754296894559, 0.3333333333333333703, 0.3219752754296894559, 0.3333333333333333703, 0.3219752754296894559, 0.3333333333333333703, 0.3219752754296894559, 0.3333333333333333703, 0.3219752754296894559, 0.3333333333333333703, 0.3219752754296894559, 0.3333333333333333703, 0.3219752754296894559, 0.3333333333333333703, 0.3219752754296894559, 0.3333333333333333703, 0.3219752754296894559, 0.3333333333333333703, 0.3219752754296894559, 0.3333333333333333703, 0.3219752754296894559, 0.3333333333333333703, 0.3219752754296894559, 0.3333333333333333703, 0.3219752754296894559, 0.3333333333333333703, 0.3219752754296894559, 0.3333333333333333703, 0.3219752754296894559, 0.3333333333333333703, 0.3219752754296894559, 0.3333333333333333703, 0.3219752754296894559, 0.3333333333333333703, 0.3219752754296894559, 0.3333333333333333703, 0.3219752754296894559, 0.3333333333333333703, 0.3219752754296894559, 0.3333333333333333703, 0.3219752754296894559, 0.3333333333333333703, 0.3219752754296894559, 0.3333333333333333703, 0.3219752754296894559, 0.3333333333333333703, 0.3219752754296894559, 0.3333333333333333703, 0.3219752754296894559, 0.3333333333333333703, 0.3219752754296894559, 0.3333333333333333703, 0.3219752754296894559, 0.3333333333333333703, 0.3219752754296894559, 0.3333333333333333703, 0.3219752754296894559, 0.3333333333333333703, 0.3219752754296894559, 0.3333333333333333703, 0.3219752754296894559, 0.3333333333333333703, 0.3219752754296894559, 0.3333333333333333703, 0.3219752754296894559, 0.3333333333333333703, 0.3219752754296894559, 0.3333333333333333703, 0.3219752754296894559, 0.3333333333333333703, 0.3219752754296894559, 0.3333333333333333703, 0.3219752754296894559, 0.3333333333333333703, 0.3219752754296894559, 0.3333333333333333703, 0.3219752754296894559, 0.3333333333333333703, 0.3219752754296894559, 0.3333333333333333703, 0.3219752754296894559, 0.3333333333333333703, 0.3219752754296894559, 0.3333333333333333703, 0.3219752754296894559, 0.3333333333333333703, 0.3219752754296894559, 0.3333333333333333703, 0.3219752754296894559, 0.3333333333333333703, 0.3219752754296894559, 0.3333333333333333703, 0.3219752754296894559, 0.3333333333333333703, 0.3219752754296894559, 0.3333333333333333703, 0.3219752754296894559, 0.3333333333333333703, 0.3219752754296894559, 0.3333333333333333703, 0.3219752754296894559, 0.3333333333333333703, 0.3219752754296894559, 0.3333333333333333703, 0.3219752754296894559, 0.3333333333333333703, 0.3219752754296894559, 0.3333333333333333703, 0.3219752754296894559, 0.3333333333333333703, 0.3219752754296894559, 0.3333333333333333703, 0.3219752754296894559, 0.3333333333333333703, 0.3219752754296894559, 0.3333333333333333703, 0.3219752754296894559, 0.3333333333333333703, 0.3219752754296894559, 0.3333333333333333703, 0.3219752754296894559, 0.3333333333333333703, 0.3219752754296894559, 0.3333333333333333703, 0.3219752754296894559, 0.3333333333333333703, 0.3219752754296894559, 0.3333333333333333703, 0.3219752754296894559, 0.3333333333333333703, 0.3219752754296894559, 0.3333333333333333703, 0.3219752754296894559, 0.3333333333333333703, 0.3219752754296894559, 0.3333333333333333703, 0.3219752754296894559, 0.3333333333333333703, 0.3219752754296894559, 0.3333333333333333703, 0.3219752754296894559, 0.3333333333333333703, 0.3219752754296894559, 0.3333333333333333703, 0.3219752754296894559, 0.3333333333333333703, 0.3219752754296894559, 0.3333333333333333703, 0.3219752754296894559, 0.3333333333333333703, 0.3219752754296894559, 0.3333333333333333703, 0.3219752754296894559, 0.3333333333333333703, 0.3219752754296894559, 0.3333333333333333703, 0.3219752754296894559, 0.3333333333333333703, 0.3219752754296894559, 0.3333333333333333703, 0.3219752754296894559, 0.3333333333333333703, 0.3219752754296894559, 0.3333333333333333703, 0.3219752754296894559, 0.3333333333333333703, 0.3219752754296894559, 0.3333333333333333703, 0.3219752754296894559, 0.3333333333333333703, 0.3219752754296894559, 0.3333333333333333703, 0.3219752754296894559, 0.3333333333333333703, 0.3219752754296894559, 0.3333333333333333703, 0.3219752754296894559, 0.3333333333333333703, 0.3219752754296894559, 0.3333333333333333703, 0.3219752754296894559, 0.3333333333333333703, 0.3219752754296894559, 0.3333333333333333703, 0.3219752754296894559, 0.3333333333333333703, 0.3219752754296894559, 0.3333333333333333703, 0.3219752754296894559, 0.3333333333333333703, 0.3219752754296894559, 0.3333333333333333703, 0.3219752754296894559, 0.3333333333333333703, 0.3219752754296894559, 0.3333333333333333703, 0.3219752754296894559, 0.3333333333333333703, 0.3219752754296894559, 0.3333333333333333703, 0.3219752754296894559, 0.3333333333333333703, 0.3219752754296894559, 0.3333333333333333703, 0.3219752754296894559, 0.3333333333333333703, 0.3219752754296894559, 0.3333333333333333703, 0.3219752754296894559, 0.3333333333333333703, 0.3219752754296894559, 0.3333333333333333703, 0.3219752754296894559, 0.3333333333333333703, 0.3219752754296894559, 0.3333333333333333703, 0.3219752754296894559, 0.3333333333333333703, 0.3219752754296894559, 0.3333333333333333703, 0.3219752754296894559, 0.3333333333333333703, 0.3219752754296894559, 0.3333333333333333703, 0.3219752754296894559, 0.3333333333333333703, 0.3219752754296894559, 0.3333333333333333703, 0.3219752754296894559, 0.3333333333333333703, 0.3219752754296894559, 0.3333333333333333703, 0.3219752754296894559, 0.3333333333333333703, 0.3219752754296894559, 0.3333333333333333703, 0.3219752754296894559, 0.3333333333333333703, 0.3219752754296894559, 0.3333333333333333703, 0.3219752754296894559, 0.3333333333333333703, 0.3219752754296894559, 0.3333333333333333703, 0.3219752754296894559, 0.3333333333333333703, 0.3219752754296894559, 0.3333333333333333703, 0.3219752754296894559, 0.3333333333333333703, 0.3219752754296894559, 0.3333333333333333703, 0.3219752754296894559, 0.3333333333333333703, 0.3219752754296894559, 0.3333333333333333703, 0.3219752754296894559, 0.3333333333333333703, 0.3219752754296894559, 0.3333333333333333703, 0.3219752754296894559, 0.3333333333333333703, 0.3219752754296894559, 0.3333333333333333703, 0.3219752754296894559, 0.3333333333333333703, 0.3219752754296894559, 0.3333333333333333703, 0.3219752754296894559, 0.3333333333333333703, 0.3219752754296894559, 0.3333333333333333703, 0.3219752754296894559, 0.3333333333333333703, 0.3219752754296894559, 0.3333333333333333703, 0.3219752754296894559, 0.3333333333333333703, 0.3219752754296894559, 0.3333333333333333703),
 ( 0.3333333333333333703, 0.3219752754296894559, 0.3333333333333333703, 0.3219752754296894559, 0.3333333333333333703, 0.3219752754296894559, 0.3333333333333333703, 0.3219752754296894559, 0.3333333333333333703, 0.3219752754296894559, 0.3333333333333333703, 0.3219752754296894559, 0.3333333333333333703, 0.3219752754296894559, 0.3333333333333333703, 0.3219752754296894559, 0.3333333333333333703, 0.3219752754296894559, 0.3333333333333333703, 0.3219752754296894559, 0.3333333333333333703, 0.3219752754296894559, 0.3333333333333333703, 0.3219752754296894559, 0.3333333333333333703, 0.3219752754296894559, 0.3333333333333333703, 0.3219752754296894559, 0.3333333333333333703, 0.3219752754296894559, 0.3333333333333333703, 0.3219752754296894559, 0.3333333333333333703, 0.3219752754296894559, 0.3333333333333333703, 0.3219752754296894559, 0.3333333333333333703, 0.3219752754296894559, 0.3333333333333333703, 0.3219752754296894559, 0.3333333333333333703, 0.3219752754296894559, 0.3333333333333333703, 0.3219752754296894559, 0.3333333333333333703, 0.3219752754296894559, 0.3333333333333333703, 0.3219752754296894559, 0.3333333333333333703, 0.3219752754296894559, 0.3333333333333333703, 0.3219752754296894559, 0.3333333333333333703, 0.3219752754296894559, 0.3333333333333333703, 0.3219752754296894559, 0.3333333333333333703, 0.3219752754296894559, 0.3333333333333333703, 0.3219752754296894559, 0.3333333333333333703, 0.3219752754296894559, 0.3333333333333333703, 0.3219752754296894559, 0.3333333333333333703, 0.3219752754296894559, 0.3333333333333333703, 0.3219752754296894559, 0.3333333333333333703, 0.3219752754296894559, 0.3333333333333333703, 0.3219752754296894559, 0.3333333333333333703, 0.3219752754296894559, 0.3333333333333333703, 0.3219752754296894559, 0.3333333333333333703, 0.3219752754296894559, 0.3333333333333333703, 0.3219752754296894559, 0.3333333333333333703, 0.3219752754296894559, 0.3333333333333333703, 0.3219752754296894559, 0.3333333333333333703, 0.3219752754296894559, 0.3333333333333333703, 0.3219752754296894559, 0.3333333333333333703, 0.3219752754296894559, 0.3333333333333333703, 0.3219752754296894559, 0.3333333333333333703, 0.3219752754296894559, 0.3333333333333333703, 0.3219752754296894559, 0.3333333333333333703, 0.3219752754296894559, 0.3333333333333333703, 0.3219752754296894559, 0.3333333333333333703, 0.3219752754296894559, 0.3333333333333333703, 0.3219752754296894559, 0.3333333333333333703, 0.3219752754296894559, 0.3333333333333333703, 0.3219752754296894559, 0.3333333333333333703, 0.3219752754296894559, 0.3333333333333333703, 0.3219752754296894559, 0.3333333333333333703, 0.3219752754296894559, 0.3333333333333333703, 0.3219752754296894559, 0.3333333333333333703, 0.3219752754296894559, 0.3333333333333333703, 0.3219752754296894559, 0.3333333333333333703, 0.3219752754296894559, 0.3333333333333333703, 0.3219752754296894559, 0.3333333333333333703, 0.3219752754296894559, 0.3333333333333333703, 0.3219752754296894559, 0.3333333333333333703, 0.3219752754296894559, 0.3333333333333333703, 0.3219752754296894559, 0.3333333333333333703, 0.3219752754296894559, 0.3333333333333333703, 0.3219752754296894559, 0.3333333333333333703, 0.3219752754296894559, 0.3333333333333333703, 0.3219752754296894559, 0.3333333333333333703, 0.3219752754296894559, 0.3333333333333333703, 0.3219752754296894559, 0.3333333333333333703, 0.3219752754296894559, 0.3333333333333333703, 0.3219752754296894559, 0.3333333333333333703, 0.3219752754296894559, 0.3333333333333333703, 0.3219752754296894559, 0.3333333333333333703, 0.3219752754296894559, 0.3333333333333333703, 0.3219752754296894559, 0.3333333333333333703, 0.3219752754296894559, 0.3333333333333333703, 0.3219752754296894559, 0.3333333333333333703, 0.3219752754296894559, 0.3333333333333333703, 0.3219752754296894559, 0.3333333333333333703, 0.3219752754296894559, 0.3333333333333333703, 0.3219752754296894559, 0.3333333333333333703, 0.3219752754296894559, 0.3333333333333333703, 0.3219752754296894559, 0.3333333333333333703, 0.3219752754296894559, 0.3333333333333333703, 0.3219752754296894559, 0.3333333333333333703, 0.3219752754296894559, 0.3333333333333333703, 0.3219752754296894559, 0.3333333333333333703, 0.3219752754296894559, 0.3333333333333333703, 0.3219752754296894559, 0.3333333333333333703, 0.3219752754296894559, 0.3333333333333333703, 0.3219752754296894559, 0.3333333333333333703, 0.3219752754296894559, 0.3333333333333333703, 0.3219752754296894559, 0.3333333333333333703, 0.3219752754296894559, 0.3333333333333333703, 0.3219752754296894559, 0.3333333333333333703, 0.3219752754296894559, 0.3333333333333333703, 0.3219752754296894559, 0.3333333333333333703, 0.3219752754296894559, 0.3333333333333333703, 0.3219752754296894559, 0.3333333333333333703, 0.3219752754296894559, 0.3333333333333333703, 0.3219752754296894559, 0.3333333333333333703, 0.3219752754296894559, 0.3333333333333333703, 0.3219752754296894559, 0.3333333333333333703, 0.3219752754296894559, 0.3333333333333333703, 0.3219752754296894559, 0.3333333333333333703, 0.3219752754296894559, 0.3333333333333333703, 0.3219752754296894559, 0.3333333333333333703, 0.3219752754296894559, 0.3333333333333333703, 0.3219752754296894559, 0.3333333333333333703, 0.3219752754296894559, 0.3333333333333333703, 0.3219752754296894559, 0.3333333333333333703, 0.3219752754296894559, 0.3333333333333333703, 0.3219752754296894559, 0.3333333333333333703, 0.3219752754296894559, 0.3333333333333333703, 0.3219752754296894559, 0.3333333333333333703, 0.3219752754296894559, 0.3333333333333333703, 0.3219752754296894559, 0.3333333333333333703, 0.3219752754296894559, 0.3333333333333333703, 0.3219752754296894559, 0.3333333333333333703, 0.3219752754296894559, 0.3333333333333333703, 0.3219752754296894559, 0.3333333333333333703, 0.3219752754296894559, 0.3333333333333333703, 0.3219752754296894559, 0.3333333333333333703, 0.3219752754296894559, 0.3333333333333333703, 0.3219752754296894559, 0.3333333333333333703, 0.3219752754296894559, 0.3333333333333333703, 0.3219752754296894559, 0.3333333333333333703, 0.3219752754296894559, 0.3333333333333333703, 0.3219752754296894559, 0.3333333333333333703, 0.3219752754296894559, 0.3333333333333333703, 0.3219752754296894559, 0.3333333333333333703, 0.3219752754296894559, 0.3333333333333333703, 0.3219752754296894559, 0.3333333333333333703, 0.3219752754296894559, 0.3333333333333333703, 0.3219752754296894559, 0.3333333333333333703, 0.3219752754296894559, 0.3333333333333333703, 0.3219752754296894559, 0.3333333333333333703, 0.3219752754296894559, 0.3333333333333333703, 0.3219752754296894559, 0.3333333333333333703, 0.3219752754296894559, 0.3333333333333333703, 0.3219752754296894559, 0.3333333333333333703, 0.3219752754296894559, 0.3333333333333333703, 0.3219752754296894559, 0.3333333333333333703, 0.3219752754296894559, 0.3333333333333333703, 0.3219752754296894559, 0.3333333333333333703, 0.3219752754296894559, 0.3333333333333333703, 0.3219752754296894559, 0.3333333333333333703, 0.3219752754296894559, 0.3333333333333333703, 0.3219752754296894559, 0.3333333333333333703, 0.3219752754296894559, 0.3333333333333333703, 0.3219752754296894559, 0.3333333333333333703, 0.3219752754296894559, 0.3333333333333333703, 0.3219752754296894559, 0.3333333333333333703, 0.3219752754296894559, 0.3333333333333333703, 0.3219752754296894559, 0.3333333333333333703, 0.3219752754296894559, 0.3333333333333333703, 0.3219752754296894559, 0.3333333333333333703, 0.3219752754296894559, 0.3333333333333333703, 0.3219752754296894559, 0.3333333333333333703, 0.3219752754296894559, 0.3333333333333333703, 0.3219752754296894559, 0.3333333333333333703, 0.3219752754296894559, 0.3333333333333333703, 0.3219752754296894559, 0.3333333333333333703, 0.3219752754296894559, 0.3333333333333333703, 0.3219752754296894559, 0.3333333333333333703, 0.3219752754296894559, 0.3333333333333333703, 0.3219752754296894559, 0.3333333333333333703, 0.3219752754296894559, 0.3333333333333333703, 0.3219752754296894559, 0.3333333333333333703, 0.3219752754296894559, 0.3333333333333333703, 0.3219752754296894559, 0.3333333333333333703, 0.3219752754296894559, 0.3333333333333333703, 0.3219752754296894559, 0.3333333333333333703, 0.3219752754296894559, 0.3333333333333333703, 0.3219752754296894559, 0.3333333333333333703, 0.3219752754296894559, 0.3333333333333333703, 0.3219752754296894559, 0.3333333333333333703, 0.3219752754296894559, 0.3333333333333333703, 0.3219752754296894559, 0.3333333333333333703, 0.3219752754296894559, 0.3333333333333333703, 0.3219752754296894559, 0.3333333333333333703, 0.3219752754296894559, 0.3333333333333333703, 0.3219752754296894559, 0.3333333333333333703, 0.3219752754296894559, 0.3333333333333333703, 0.3219752754296894559, 0.3333333333333333703, 0.3219752754296894559, 0.3333333333333333703, 0.3219752754296894559, 0.3333333333333333703, 0.3219752754296894559, 0.3333333333333333703, 0.3219752754296894559, 0.3333333333333333703, 0.3219752754296894559, 0.3333333333333333703, 0.3219752754296894559, 0.3333333333333333703, 0.3219752754296894559, 0.3333333333333333703, 0.3219752754296894559, 0.3333333333333333703, 0.3219752754296894559, 0.3333333333333333703, 0.3219752754296894559, 0.3333333333333333703, 0.3219752754296894559, 0.3333333333333333703, 0.3219752754296894559, 0.3333333333333333703, 0.3219752754296894559, 0.3333333333333333703, 0.3219752754296894559, 0.3333333333333333703, 0.3219752754296894559, 0.3333333333333333703, 0.3219752754296894559, 0.3333333333333333703, 0.3219752754296894559, 0.3333333333333333703, 0.3219752754296894559, 0.3333333333333333703, 0.3219752754296894559, 0.3333333333333333703, 0.3219752754296894559, 0.3333333333333333703, 0.3219752754296894559, 0.3333333333333333703, 0.3219752754296894559, 0.3333333333333333703, 0.3219752754296894559, 0.3333333333333333703, 0.3219752754296894559, 0.3333333333333333703, 0.3219752754296894559, 0.3333333333333333703, 0.3219752754296894559, 0.3333333333333333703, 0.3219752754296894559, 0.3333333333333333703, 0.3219752754296894559, 0.3333333333333333703, 0.3219752754296894559, 0.3333333333333333703, 0.3219752754296894559, 0.3333333333333333703, 0.3219752754296894559, 0.3333333333333333703, 0.3219752754296894559, 0.3333333333333333703, 0.3219752754296894559, 0.3333333333333333703, 0.3219752754296894559, 0.3333333333333333703, 0.3219752754296894559, 0.3333333333333333703, 0.3219752754296894559, 0.3333333333333333703, 0.3219752754296894559, 0.3333333333333333703, 0.3219752754296894559, 0.3333333333333333703, 0.3219752754296894559, 0.3333333333333333703, 0.3219752754296894559, 0.3333333333333333703),
 ( 1.000000000000000000, 0.9659258262890683122, 1.000000000000000000, 0.9659258262890683122, 1.000000000000000000, 0.9659258262890683122, 1.000000000000000000, 0.9659258262890683122, 1.000000000000000000, 0.9659258262890683122, 1.000000000000000000, 0.9659258262890683122, 1.000000000000000000, 0.9659258262890683122, 1.000000000000000000, 0.9659258262890683122, 1.000000000000000000, 0.9659258262890683122, 1.000000000000000000, 0.9659258262890683122, 1.000000000000000000, 0.9659258262890683122, 1.000000000000000000, 0.9659258262890683122, 1.000000000000000000, 0.9659258262890683122, 1.000000000000000000, 0.9659258262890683122, 1.000000000000000000, 0.9659258262890683122, 1.000000000000000000, 0.9659258262890683122, 1.000000000000000000, 0.9659258262890683122, 1.000000000000000000, 0.9659258262890683122, 1.000000000000000000, 0.9659258262890683122, 1.000000000000000000, 0.9659258262890683122, 1.000000000000000000, 0.9659258262890683122, 1.000000000000000000, 0.9659258262890683122, 1.000000000000000000, 0.9659258262890683122, 1.000000000000000000, 0.9659258262890683122, 1.000000000000000000, 0.9659258262890683122, 1.000000000000000000, 0.9659258262890683122, 1.000000000000000000, 0.9659258262890683122, 1.000000000000000000, 0.9659258262890683122, 1.000000000000000000, 0.9659258262890683122, 1.000000000000000000, 0.9659258262890683122, 1.000000000000000000, 0.9659258262890683122, 1.000000000000000000, 0.9659258262890683122, 1.000000000000000000, 0.9659258262890683122, 1.000000000000000000, 0.9659258262890683122, 1.000000000000000000, 0.9659258262890683122, 1.000000000000000000, 0.9659258262890683122, 1.000000000000000000, 0.9659258262890683122, 1.000000000000000000, 0.9659258262890683122, 1.000000000000000000, 0.9659258262890683122, 1.000000000000000000, 0.9659258262890683122, 1.000000000000000000, 0.9659258262890683122, 1.000000000000000000, 0.9659258262890683122, 1.000000000000000000, 0.9659258262890683122, 1.000000000000000000, 0.9659258262890683122, 1.000000000000000000, 0.9659258262890683122, 1.000000000000000000, 0.9659258262890683122, 1.000000000000000000, 0.9659258262890683122, 1.000000000000000000, 0.9659258262890683122, 1.000000000000000000, 0.9659258262890683122, 1.000000000000000000, 0.9659258262890683122, 1.000000000000000000, 0.9659258262890683122, 1.000000000000000000, 0.9659258262890683122, 1.000000000000000000, 0.9659258262890683122, 1.000000000000000000, 0.9659258262890683122, 1.000000000000000000, 0.9659258262890683122, 1.000000000000000000, 0.9659258262890683122, 1.000000000000000000, 0.9659258262890683122, 1.000000000000000000, 0.9659258262890683122, 1.000000000000000000, 0.9659258262890683122, 1.000000000000000000, 0.9659258262890683122, 1.000000000000000000, 0.9659258262890683122, 1.000000000000000000, 0.9659258262890683122, 1.000000000000000000, 0.9659258262890683122, 1.000000000000000000, 0.9659258262890683122, 1.000000000000000000, 0.9659258262890683122, 1.000000000000000000, 0.9659258262890683122, 1.000000000000000000, 0.9659258262890683122, 1.000000000000000000, 0.9659258262890683122, 1.000000000000000000, 0.9659258262890683122, 1.000000000000000000, 0.9659258262890683122, 1.000000000000000000, 0.9659258262890683122, 1.000000000000000000, 0.9659258262890683122, 1.000000000000000000, 0.9659258262890683122, 1.000000000000000000, 0.9659258262890683122, 1.000000000000000000, 0.9659258262890683122, 1.000000000000000000, 0.9659258262890683122, 1.000000000000000000, 0.9659258262890683122, 1.000000000000000000, 0.9659258262890683122, 1.000000000000000000, 0.9659258262890683122, 1.000000000000000000, 0.9659258262890683122, 1.000000000000000000, 0.9659258262890683122, 1.000000000000000000, 0.9659258262890683122, 1.000000000000000000, 0.9659258262890683122, 1.000000000000000000, 0.9659258262890683122, 1.000000000000000000, 0.9659258262890683122, 1.000000000000000000, 0.9659258262890683122, 1.000000000000000000, 0.9659258262890683122, 1.000000000000000000, 0.9659258262890683122, 1.000000000000000000, 0.9659258262890683122, 1.000000000000000000, 0.9659258262890683122, 1.000000000000000000, 0.9659258262890683122, 1.000000000000000000, 0.9659258262890683122, 1.000000000000000000, 0.9659258262890683122, 1.000000000000000000, 0.9659258262890683122, 1.000000000000000000, 0.9659258262890683122, 1.000000000000000000, 0.9659258262890683122, 1.000000000000000000, 0.9659258262890683122, 1.000000000000000000, 0.9659258262890683122, 1.000000000000000000, 0.9659258262890683122, 1.000000000000000000, 0.9659258262890683122, 1.000000000000000000, 0.9659258262890683122, 1.000000000000000000, 0.9659258262890683122, 1.000000000000000000, 0.9659258262890683122, 1.000000000000000000, 0.9659258262890683122, 1.000000000000000000, 0.9659258262890683122, 1.000000000000000000, 0.9659258262890683122, 1.000000000000000000, 0.9659258262890683122, 1.000000000000000000, 0.9659258262890683122, 1.000000000000000000, 0.9659258262890683122, 1.000000000000000000, 0.9659258262890683122, 1.000000000000000000, 0.9659258262890683122, 1.000000000000000000, 0.9659258262890683122, 1.000000000000000000, 0.9659258262890683122, 1.000000000000000000, 0.9659258262890683122, 1.000000000000000000, 0.9659258262890683122, 1.000000000000000000, 0.9659258262890683122, 1.000000000000000000, 0.9659258262890683122, 1.000000000000000000, 0.9659258262890683122, 1.000000000000000000, 0.9659258262890683122, 1.000000000000000000, 0.9659258262890683122, 1.000000000000000000, 0.9659258262890683122, 1.000000000000000000, 0.9659258262890683122, 1.000000000000000000, 0.9659258262890683122, 1.000000000000000000, 0.9659258262890683122, 1.000000000000000000, 0.9659258262890683122, 1.000000000000000000, 0.9659258262890683122, 1.000000000000000000, 0.9659258262890683122, 1.000000000000000000, 0.9659258262890683122, 1.000000000000000000, 0.9659258262890683122, 1.000000000000000000, 0.9659258262890683122, 1.000000000000000000, 0.9659258262890683122, 1.000000000000000000, 0.9659258262890683122, 1.000000000000000000, 0.9659258262890683122, 1.000000000000000000, 0.9659258262890683122, 1.000000000000000000, 0.9659258262890683122, 1.000000000000000000, 0.9659258262890683122, 1.000000000000000000, 0.9659258262890683122, 1.000000000000000000, 0.9659258262890683122, 1.000000000000000000, 0.9659258262890683122, 1.000000000000000000, 0.9659258262890683122, 1.000000000000000000, 0.9659258262890683122, 1.000000000000000000, 0.9659258262890683122, 1.000000000000000000, 0.9659258262890683122, 1.000000000000000000, 0.9659258262890683122, 1.000000000000000000, 0.9659258262890683122, 1.000000000000000000, 0.9659258262890683122, 1.000000000000000000, 0.9659258262890683122, 1.000000000000000000, 0.9659258262890683122, 1.000000000000000000, 0.9659258262890683122, 1.000000000000000000, 0.9659258262890683122, 1.000000000000000000, 0.9659258262890683122, 1.000000000000000000, 0.9659258262890683122, 1.000000000000000000, 0.9659258262890683122, 1.000000000000000000, 0.9659258262890683122, 1.000000000000000000, 0.9659258262890683122, 1.000000000000000000, 0.9659258262890683122, 1.000000000000000000, 0.9659258262890683122, 1.000000000000000000, 0.9659258262890683122, 1.000000000000000000, 0.9659258262890683122, 1.000000000000000000, 0.9659258262890683122, 1.000000000000000000, 0.9659258262890683122, 1.000000000000000000, 0.9659258262890683122, 1.000000000000000000, 0.9659258262890683122, 1.000000000000000000, 0.9659258262890683122, 1.000000000000000000, 0.9659258262890683122, 1.000000000000000000, 0.9659258262890683122, 1.000000000000000000, 0.9659258262890683122, 1.000000000000000000, 0.9659258262890683122, 1.000000000000000000, 0.9659258262890683122, 1.000000000000000000, 0.9659258262890683122, 1.000000000000000000, 0.9659258262890683122, 1.000000000000000000, 0.9659258262890683122, 1.000000000000000000, 0.9659258262890683122, 1.000000000000000000, 0.9659258262890683122, 1.000000000000000000, 0.9659258262890683122, 1.000000000000000000, 0.9659258262890683122, 1.000000000000000000, 0.9659258262890683122, 1.000000000000000000, 0.9659258262890683122, 1.000000000000000000, 0.9659258262890683122, 1.000000000000000000, 0.9659258262890683122, 1.000000000000000000, 0.9659258262890683122, 1.000000000000000000, 0.9659258262890683122, 1.000000000000000000, 0.9659258262890683122, 1.000000000000000000, 0.9659258262890683122, 1.000000000000000000, 0.9659258262890683122, 1.000000000000000000, 0.9659258262890683122, 1.000000000000000000, 0.9659258262890683122, 1.000000000000000000, 0.9659258262890683122, 1.000000000000000000, 0.9659258262890683122, 1.000000000000000000, 0.9659258262890683122, 1.000000000000000000, 0.9659258262890683122, 1.000000000000000000, 0.9659258262890683122, 1.000000000000000000, 0.9659258262890683122, 1.000000000000000000, 0.9659258262890683122, 1.000000000000000000, 0.9659258262890683122, 1.000000000000000000, 0.9659258262890683122, 1.000000000000000000, 0.9659258262890683122, 1.000000000000000000, 0.9659258262890683122, 1.000000000000000000, 0.9659258262890683122, 1.000000000000000000, 0.9659258262890683122, 1.000000000000000000, 0.9659258262890683122, 1.000000000000000000, 0.9659258262890683122, 1.000000000000000000, 0.9659258262890683122, 1.000000000000000000, 0.9659258262890683122, 1.000000000000000000, 0.9659258262890683122, 1.000000000000000000, 0.9659258262890683122, 1.000000000000000000, 0.9659258262890683122, 1.000000000000000000, 0.9659258262890683122, 1.000000000000000000, 0.9659258262890683122, 1.000000000000000000, 0.9659258262890683122, 1.000000000000000000, 0.9659258262890683122, 1.000000000000000000, 0.9659258262890683122, 1.000000000000000000, 0.9659258262890683122, 1.000000000000000000, 0.9659258262890683122, 1.000000000000000000, 0.9659258262890683122, 1.000000000000000000, 0.9659258262890683122, 1.000000000000000000, 0.9659258262890683122, 1.000000000000000000, 0.9659258262890683122, 1.000000000000000000, 0.9659258262890683122, 1.000000000000000000, 0.9659258262890683122, 1.000000000000000000, 0.9659258262890683122, 1.000000000000000000, 0.9659258262890683122, 1.000000000000000000, 0.9659258262890683122, 1.000000000000000000, 0.9659258262890683122, 1.000000000000000000, 0.9659258262890683122, 1.000000000000000000, 0.9659258262890683122, 1.000000000000000000, 0.9659258262890683122, 1.000000000000000000, 0.9659258262890683122, 1.000000000000000000),
 ( 0.3333333333333333703, 0.3219752754296894559, 0.3333333333333333703, 0.3219752754296894559, 0.3333333333333333703, 0.3219752754296894559, 0.3333333333333333703, 0.3219752754296894559, 0.3333333333333333703, 0.3219752754296894559, 0.3333333333333333703, 0.3219752754296894559, 0.3333333333333333703, 0.3219752754296894559, 0.3333333333333333703, 0.3219752754296894559, 0.3333333333333333703, 0.3219752754296894559, 0.3333333333333333703, 0.3219752754296894559, 0.3333333333333333703, 0.3219752754296894559, 0.3333333333333333703, 0.3219752754296894559, 0.3333333333333333703, 0.3219752754296894559, 0.3333333333333333703, 0.3219752754296894559, 0.3333333333333333703, 0.3219752754296894559, 0.3333333333333333703, 0.3219752754296894559, 0.3333333333333333703, 0.3219752754296894559, 0.3333333333333333703, 0.3219752754296894559, 0.3333333333333333703, 0.3219752754296894559, 0.3333333333333333703, 0.3219752754296894559, 0.3333333333333333703, 0.3219752754296894559, 0.3333333333333333703, 0.3219752754296894559, 0.3333333333333333703, 0.3219752754296894559, 0.3333333333333333703, 0.3219752754296894559, 0.3333333333333333703, 0.3219752754296894559, 0.3333333333333333703, 0.3219752754296894559, 0.3333333333333333703, 0.3219752754296894559, 0.3333333333333333703, 0.3219752754296894559, 0.3333333333333333703, 0.3219752754296894559, 0.3333333333333333703, 0.3219752754296894559, 0.3333333333333333703, 0.3219752754296894559, 0.3333333333333333703, 0.3219752754296894559, 0.3333333333333333703, 0.3219752754296894559, 0.3333333333333333703, 0.3219752754296894559, 0.3333333333333333703, 0.3219752754296894559, 0.3333333333333333703, 0.3219752754296894559, 0.3333333333333333703, 0.3219752754296894559, 0.3333333333333333703, 0.3219752754296894559, 0.3333333333333333703, 0.3219752754296894559, 0.3333333333333333703, 0.3219752754296894559, 0.3333333333333333703, 0.3219752754296894559, 0.3333333333333333703, 0.3219752754296894559, 0.3333333333333333703, 0.3219752754296894559, 0.3333333333333333703, 0.3219752754296894559, 0.3333333333333333703, 0.3219752754296894559, 0.3333333333333333703, 0.3219752754296894559, 0.3333333333333333703, 0.3219752754296894559, 0.3333333333333333703, 0.3219752754296894559, 0.3333333333333333703, 0.3219752754296894559, 0.3333333333333333703, 0.3219752754296894559, 0.3333333333333333703, 0.3219752754296894559, 0.3333333333333333703, 0.3219752754296894559, 0.3333333333333333703, 0.3219752754296894559, 0.3333333333333333703, 0.3219752754296894559, 0.3333333333333333703, 0.3219752754296894559, 0.3333333333333333703, 0.3219752754296894559, 0.3333333333333333703, 0.3219752754296894559, 0.3333333333333333703, 0.3219752754296894559, 0.3333333333333333703, 0.3219752754296894559, 0.3333333333333333703, 0.3219752754296894559, 0.3333333333333333703, 0.3219752754296894559, 0.3333333333333333703, 0.3219752754296894559, 0.3333333333333333703, 0.3219752754296894559, 0.3333333333333333703, 0.3219752754296894559, 0.3333333333333333703, 0.3219752754296894559, 0.3333333333333333703, 0.3219752754296894559, 0.3333333333333333703, 0.3219752754296894559, 0.3333333333333333703, 0.3219752754296894559, 0.3333333333333333703, 0.3219752754296894559, 0.3333333333333333703, 0.3219752754296894559, 0.3333333333333333703, 0.3219752754296894559, 0.3333333333333333703, 0.3219752754296894559, 0.3333333333333333703, 0.3219752754296894559, 0.3333333333333333703, 0.3219752754296894559, 0.3333333333333333703, 0.3219752754296894559, 0.3333333333333333703, 0.3219752754296894559, 0.3333333333333333703, 0.3219752754296894559, 0.3333333333333333703, 0.3219752754296894559, 0.3333333333333333703, 0.3219752754296894559, 0.3333333333333333703, 0.3219752754296894559, 0.3333333333333333703, 0.3219752754296894559, 0.3333333333333333703, 0.3219752754296894559, 0.3333333333333333703, 0.3219752754296894559, 0.3333333333333333703, 0.3219752754296894559, 0.3333333333333333703, 0.3219752754296894559, 0.3333333333333333703, 0.3219752754296894559, 0.3333333333333333703, 0.3219752754296894559, 0.3333333333333333703, 0.3219752754296894559, 0.3333333333333333703, 0.3219752754296894559, 0.3333333333333333703, 0.3219752754296894559, 0.3333333333333333703, 0.3219752754296894559, 0.3333333333333333703, 0.3219752754296894559, 0.3333333333333333703, 0.3219752754296894559, 0.3333333333333333703, 0.3219752754296894559, 0.3333333333333333703, 0.3219752754296894559, 0.3333333333333333703, 0.3219752754296894559, 0.3333333333333333703, 0.3219752754296894559, 0.3333333333333333703, 0.3219752754296894559, 0.3333333333333333703, 0.3219752754296894559, 0.3333333333333333703, 0.3219752754296894559, 0.3333333333333333703, 0.3219752754296894559, 0.3333333333333333703, 0.3219752754296894559, 0.3333333333333333703, 0.3219752754296894559, 0.3333333333333333703, 0.3219752754296894559, 0.3333333333333333703, 0.3219752754296894559, 0.3333333333333333703, 0.3219752754296894559, 0.3333333333333333703, 0.3219752754296894559, 0.3333333333333333703, 0.3219752754296894559, 0.3333333333333333703, 0.3219752754296894559, 0.3333333333333333703, 0.3219752754296894559, 0.3333333333333333703, 0.3219752754296894559, 0.3333333333333333703, 0.3219752754296894559, 0.3333333333333333703, 0.3219752754296894559, 0.3333333333333333703, 0.3219752754296894559, 0.3333333333333333703, 0.3219752754296894559, 0.3333333333333333703, 0.3219752754296894559, 0.3333333333333333703, 0.3219752754296894559, 0.3333333333333333703, 0.3219752754296894559, 0.3333333333333333703, 0.3219752754296894559, 0.3333333333333333703, 0.3219752754296894559, 0.3333333333333333703, 0.3219752754296894559, 0.3333333333333333703, 0.3219752754296894559, 0.3333333333333333703, 0.3219752754296894559, 0.3333333333333333703, 0.3219752754296894559, 0.3333333333333333703, 0.3219752754296894559, 0.3333333333333333703, 0.3219752754296894559, 0.3333333333333333703, 0.3219752754296894559, 0.3333333333333333703, 0.3219752754296894559, 0.3333333333333333703, 0.3219752754296894559, 0.3333333333333333703, 0.3219752754296894559, 0.3333333333333333703, 0.3219752754296894559, 0.3333333333333333703, 0.3219752754296894559, 0.3333333333333333703, 0.3219752754296894559, 0.3333333333333333703, 0.3219752754296894559, 0.3333333333333333703, 0.3219752754296894559, 0.3333333333333333703, 0.3219752754296894559, 0.3333333333333333703, 0.3219752754296894559, 0.3333333333333333703, 0.3219752754296894559, 0.3333333333333333703, 0.3219752754296894559, 0.3333333333333333703, 0.3219752754296894559, 0.3333333333333333703, 0.3219752754296894559, 0.3333333333333333703, 0.3219752754296894559, 0.3333333333333333703, 0.3219752754296894559, 0.3333333333333333703, 0.3219752754296894559, 0.3333333333333333703, 0.3219752754296894559, 0.3333333333333333703, 0.3219752754296894559, 0.3333333333333333703, 0.3219752754296894559, 0.3333333333333333703, 0.3219752754296894559, 0.3333333333333333703, 0.3219752754296894559, 0.3333333333333333703, 0.3219752754296894559, 0.3333333333333333703, 0.3219752754296894559, 0.3333333333333333703, 0.3219752754296894559, 0.3333333333333333703, 0.3219752754296894559, 0.3333333333333333703, 0.3219752754296894559, 0.3333333333333333703, 0.3219752754296894559, 0.3333333333333333703, 0.3219752754296894559, 0.3333333333333333703, 0.3219752754296894559, 0.3333333333333333703, 0.3219752754296894559, 0.3333333333333333703, 0.3219752754296894559, 0.3333333333333333703, 0.3219752754296894559, 0.3333333333333333703, 0.3219752754296894559, 0.3333333333333333703, 0.3219752754296894559, 0.3333333333333333703, 0.3219752754296894559, 0.3333333333333333703, 0.3219752754296894559, 0.3333333333333333703, 0.3219752754296894559, 0.3333333333333333703, 0.3219752754296894559, 0.3333333333333333703, 0.3219752754296894559, 0.3333333333333333703, 0.3219752754296894559, 0.3333333333333333703, 0.3219752754296894559, 0.3333333333333333703, 0.3219752754296894559, 0.3333333333333333703, 0.3219752754296894559, 0.3333333333333333703, 0.3219752754296894559, 0.3333333333333333703, 0.3219752754296894559, 0.3333333333333333703, 0.3219752754296894559, 0.3333333333333333703, 0.3219752754296894559, 0.3333333333333333703, 0.3219752754296894559, 0.3333333333333333703, 0.3219752754296894559, 0.3333333333333333703, 0.3219752754296894559, 0.3333333333333333703, 0.3219752754296894559, 0.3333333333333333703, 0.3219752754296894559, 0.3333333333333333703, 0.3219752754296894559, 0.3333333333333333703, 0.3219752754296894559, 0.3333333333333333703, 0.3219752754296894559, 0.3333333333333333703, 0.3219752754296894559, 0.3333333333333333703, 0.3219752754296894559, 0.3333333333333333703, 0.3219752754296894559, 0.3333333333333333703, 0.3219752754296894559, 0.3333333333333333703, 0.3219752754296894559, 0.3333333333333333703, 0.3219752754296894559, 0.3333333333333333703, 0.3219752754296894559, 0.3333333333333333703, 0.3219752754296894559, 0.3333333333333333703, 0.3219752754296894559, 0.3333333333333333703, 0.3219752754296894559, 0.3333333333333333703, 0.3219752754296894559, 0.3333333333333333703, 0.3219752754296894559, 0.3333333333333333703, 0.3219752754296894559, 0.3333333333333333703, 0.3219752754296894559, 0.3333333333333333703, 0.3219752754296894559, 0.3333333333333333703, 0.3219752754296894559, 0.3333333333333333703, 0.3219752754296894559, 0.3333333333333333703, 0.3219752754296894559, 0.3333333333333333703, 0.3219752754296894559, 0.3333333333333333703, 0.3219752754296894559, 0.3333333333333333703, 0.3219752754296894559, 0.3333333333333333703, 0.3219752754296894559, 0.3333333333333333703, 0.3219752754296894559, 0.3333333333333333703, 0.3219752754296894559, 0.3333333333333333703, 0.3219752754296894559, 0.3333333333333333703, 0.3219752754296894559, 0.3333333333333333703, 0.3219752754296894559, 0.3333333333333333703, 0.3219752754296894559, 0.3333333333333333703, 0.3219752754296894559, 0.3333333333333333703, 0.3219752754296894559, 0.3333333333333333703, 0.3219752754296894559, 0.3333333333333333703, 0.3219752754296894559, 0.3333333333333333703, 0.3219752754296894559, 0.3333333333333333703, 0.3219752754296894559, 0.3333333333333333703, 0.3219752754296894559, 0.3333333333333333703, 0.3219752754296894559, 0.3333333333333333703, 0.3219752754296894559, 0.3333333333333333703, 0.3219752754296894559, 0.3333333333333333703, 0.3219752754296894559, 0.3333333333333333703, 0.3219752754296894559, 0.3333333333333333703, 0.3219752754296894559, 0.3333333333333333703, 0.3219752754296894559, 0.3333333333333333703, 0.3219752754296894559, 0.3333333333333333703, 0.3219752754296894559, 0.3333333333333333703, 0.3219752754296894559, 0.3333333333333333703),
 ( 0.3333333333333333703, 0.3219752754296894559, 0.3333333333333333703, 0.3219752754296894559, 0.3333333333333333703, 0.3219752754296894559, 0.3333333333333333703, 0.3219752754296894559, 0.3333333333333333703, 0.3219752754296894559, 0.3333333333333333703, 0.3219752754296894559, 0.3333333333333333703, 0.3219752754296894559, 0.3333333333333333703, 0.3219752754296894559, 0.3333333333333333703, 0.3219752754296894559, 0.3333333333333333703, 0.3219752754296894559, 0.3333333333333333703, 0.3219752754296894559, 0.3333333333333333703, 0.3219752754296894559, 0.3333333333333333703, 0.3219752754296894559, 0.3333333333333333703, 0.3219752754296894559, 0.3333333333333333703, 0.3219752754296894559, 0.3333333333333333703, 0.3219752754296894559, 0.3333333333333333703, 0.3219752754296894559, 0.3333333333333333703, 0.3219752754296894559, 0.3333333333333333703, 0.3219752754296894559, 0.3333333333333333703, 0.3219752754296894559, 0.3333333333333333703, 0.3219752754296894559, 0.3333333333333333703, 0.3219752754296894559, 0.3333333333333333703, 0.3219752754296894559, 0.3333333333333333703, 0.3219752754296894559, 0.3333333333333333703, 0.3219752754296894559, 0.3333333333333333703, 0.3219752754296894559, 0.3333333333333333703, 0.3219752754296894559, 0.3333333333333333703, 0.3219752754296894559, 0.3333333333333333703, 0.3219752754296894559, 0.3333333333333333703, 0.3219752754296894559, 0.3333333333333333703, 0.3219752754296894559, 0.3333333333333333703, 0.3219752754296894559, 0.3333333333333333703, 0.3219752754296894559, 0.3333333333333333703, 0.3219752754296894559, 0.3333333333333333703, 0.3219752754296894559, 0.3333333333333333703, 0.3219752754296894559, 0.3333333333333333703, 0.3219752754296894559, 0.3333333333333333703, 0.3219752754296894559, 0.3333333333333333703, 0.3219752754296894559, 0.3333333333333333703, 0.3219752754296894559, 0.3333333333333333703, 0.3219752754296894559, 0.3333333333333333703, 0.3219752754296894559, 0.3333333333333333703, 0.3219752754296894559, 0.3333333333333333703, 0.3219752754296894559, 0.3333333333333333703, 0.3219752754296894559, 0.3333333333333333703, 0.3219752754296894559, 0.3333333333333333703, 0.3219752754296894559, 0.3333333333333333703, 0.3219752754296894559, 0.3333333333333333703, 0.3219752754296894559, 0.3333333333333333703, 0.3219752754296894559, 0.3333333333333333703, 0.3219752754296894559, 0.3333333333333333703, 0.3219752754296894559, 0.3333333333333333703, 0.3219752754296894559, 0.3333333333333333703, 0.3219752754296894559, 0.3333333333333333703, 0.3219752754296894559, 0.3333333333333333703, 0.3219752754296894559, 0.3333333333333333703, 0.3219752754296894559, 0.3333333333333333703, 0.3219752754296894559, 0.3333333333333333703, 0.3219752754296894559, 0.3333333333333333703, 0.3219752754296894559, 0.3333333333333333703, 0.3219752754296894559, 0.3333333333333333703, 0.3219752754296894559, 0.3333333333333333703, 0.3219752754296894559, 0.3333333333333333703, 0.3219752754296894559, 0.3333333333333333703, 0.3219752754296894559, 0.3333333333333333703, 0.3219752754296894559, 0.3333333333333333703, 0.3219752754296894559, 0.3333333333333333703, 0.3219752754296894559, 0.3333333333333333703, 0.3219752754296894559, 0.3333333333333333703, 0.3219752754296894559, 0.3333333333333333703, 0.3219752754296894559, 0.3333333333333333703, 0.3219752754296894559, 0.3333333333333333703, 0.3219752754296894559, 0.3333333333333333703, 0.3219752754296894559, 0.3333333333333333703, 0.3219752754296894559, 0.3333333333333333703, 0.3219752754296894559, 0.3333333333333333703, 0.3219752754296894559, 0.3333333333333333703, 0.3219752754296894559, 0.3333333333333333703, 0.3219752754296894559, 0.3333333333333333703, 0.3219752754296894559, 0.3333333333333333703, 0.3219752754296894559, 0.3333333333333333703, 0.3219752754296894559, 0.3333333333333333703, 0.3219752754296894559, 0.3333333333333333703, 0.3219752754296894559, 0.3333333333333333703, 0.3219752754296894559, 0.3333333333333333703, 0.3219752754296894559, 0.3333333333333333703, 0.3219752754296894559, 0.3333333333333333703, 0.3219752754296894559, 0.3333333333333333703, 0.3219752754296894559, 0.3333333333333333703, 0.3219752754296894559, 0.3333333333333333703, 0.3219752754296894559, 0.3333333333333333703, 0.3219752754296894559, 0.3333333333333333703, 0.3219752754296894559, 0.3333333333333333703, 0.3219752754296894559, 0.3333333333333333703, 0.3219752754296894559, 0.3333333333333333703, 0.3219752754296894559, 0.3333333333333333703, 0.3219752754296894559, 0.3333333333333333703, 0.3219752754296894559, 0.3333333333333333703, 0.3219752754296894559, 0.3333333333333333703, 0.3219752754296894559, 0.3333333333333333703, 0.3219752754296894559, 0.3333333333333333703, 0.3219752754296894559, 0.3333333333333333703, 0.3219752754296894559, 0.3333333333333333703, 0.3219752754296894559, 0.3333333333333333703, 0.3219752754296894559, 0.3333333333333333703, 0.3219752754296894559, 0.3333333333333333703, 0.3219752754296894559, 0.3333333333333333703, 0.3219752754296894559, 0.3333333333333333703, 0.3219752754296894559, 0.3333333333333333703, 0.3219752754296894559, 0.3333333333333333703, 0.3219752754296894559, 0.3333333333333333703, 0.3219752754296894559, 0.3333333333333333703, 0.3219752754296894559, 0.3333333333333333703, 0.3219752754296894559, 0.3333333333333333703, 0.3219752754296894559, 0.3333333333333333703, 0.3219752754296894559, 0.3333333333333333703, 0.3219752754296894559, 0.3333333333333333703, 0.3219752754296894559, 0.3333333333333333703, 0.3219752754296894559, 0.3333333333333333703, 0.3219752754296894559, 0.3333333333333333703, 0.3219752754296894559, 0.3333333333333333703, 0.3219752754296894559, 0.3333333333333333703, 0.3219752754296894559, 0.3333333333333333703, 0.3219752754296894559, 0.3333333333333333703, 0.3219752754296894559, 0.3333333333333333703, 0.3219752754296894559, 0.3333333333333333703, 0.3219752754296894559, 0.3333333333333333703, 0.3219752754296894559, 0.3333333333333333703, 0.3219752754296894559, 0.3333333333333333703, 0.3219752754296894559, 0.3333333333333333703, 0.3219752754296894559, 0.3333333333333333703, 0.3219752754296894559, 0.3333333333333333703, 0.3219752754296894559, 0.3333333333333333703, 0.3219752754296894559, 0.3333333333333333703, 0.3219752754296894559, 0.3333333333333333703, 0.3219752754296894559, 0.3333333333333333703, 0.3219752754296894559, 0.3333333333333333703, 0.3219752754296894559, 0.3333333333333333703, 0.3219752754296894559, 0.3333333333333333703, 0.3219752754296894559, 0.3333333333333333703, 0.3219752754296894559, 0.3333333333333333703, 0.3219752754296894559, 0.3333333333333333703, 0.3219752754296894559, 0.3333333333333333703, 0.3219752754296894559, 0.3333333333333333703, 0.3219752754296894559, 0.3333333333333333703, 0.3219752754296894559, 0.3333333333333333703, 0.3219752754296894559, 0.3333333333333333703, 0.3219752754296894559, 0.3333333333333333703, 0.3219752754296894559, 0.3333333333333333703, 0.3219752754296894559, 0.3333333333333333703, 0.3219752754296894559, 0.3333333333333333703, 0.3219752754296894559, 0.3333333333333333703, 0.3219752754296894559, 0.3333333333333333703, 0.3219752754296894559, 0.3333333333333333703, 0.3219752754296894559, 0.3333333333333333703, 0.3219752754296894559, 0.3333333333333333703, 0.3219752754296894559, 0.3333333333333333703, 0.3219752754296894559, 0.3333333333333333703, 0.3219752754296894559, 0.3333333333333333703, 0.3219752754296894559, 0.3333333333333333703, 0.3219752754296894559, 0.3333333333333333703, 0.3219752754296894559, 0.3333333333333333703, 0.3219752754296894559, 0.3333333333333333703, 0.3219752754296894559, 0.3333333333333333703, 0.3219752754296894559, 0.3333333333333333703, 0.3219752754296894559, 0.3333333333333333703, 0.3219752754296894559, 0.3333333333333333703, 0.3219752754296894559, 0.3333333333333333703, 0.3219752754296894559, 0.3333333333333333703, 0.3219752754296894559, 0.3333333333333333703, 0.3219752754296894559, 0.3333333333333333703, 0.3219752754296894559, 0.3333333333333333703, 0.3219752754296894559, 0.3333333333333333703, 0.3219752754296894559, 0.3333333333333333703, 0.3219752754296894559, 0.3333333333333333703, 0.3219752754296894559, 0.3333333333333333703, 0.3219752754296894559, 0.3333333333333333703, 0.3219752754296894559, 0.3333333333333333703, 0.3219752754296894559, 0.3333333333333333703, 0.3219752754296894559, 0.3333333333333333703, 0.3219752754296894559, 0.3333333333333333703, 0.3219752754296894559, 0.3333333333333333703, 0.3219752754296894559, 0.3333333333333333703, 0.3219752754296894559, 0.3333333333333333703, 0.3219752754296894559, 0.3333333333333333703, 0.3219752754296894559, 0.3333333333333333703, 0.3219752754296894559, 0.3333333333333333703, 0.3219752754296894559, 0.3333333333333333703, 0.3219752754296894559, 0.3333333333333333703, 0.3219752754296894559, 0.3333333333333333703, 0.3219752754296894559, 0.3333333333333333703, 0.3219752754296894559, 0.3333333333333333703, 0.3219752754296894559, 0.3333333333333333703, 0.3219752754296894559, 0.3333333333333333703, 0.3219752754296894559, 0.3333333333333333703, 0.3219752754296894559, 0.3333333333333333703, 0.3219752754296894559, 0.3333333333333333703, 0.3219752754296894559, 0.3333333333333333703, 0.3219752754296894559, 0.3333333333333333703, 0.3219752754296894559, 0.3333333333333333703, 0.3219752754296894559, 0.3333333333333333703, 0.3219752754296894559, 0.3333333333333333703, 0.3219752754296894559, 0.3333333333333333703, 0.3219752754296894559, 0.3333333333333333703, 0.3219752754296894559, 0.3333333333333333703, 0.3219752754296894559, 0.3333333333333333703, 0.3219752754296894559, 0.3333333333333333703, 0.3219752754296894559, 0.3333333333333333703, 0.3219752754296894559, 0.3333333333333333703, 0.3219752754296894559, 0.3333333333333333703, 0.3219752754296894559, 0.3333333333333333703, 0.3219752754296894559, 0.3333333333333333703, 0.3219752754296894559, 0.3333333333333333703, 0.3219752754296894559, 0.3333333333333333703, 0.3219752754296894559, 0.3333333333333333703, 0.3219752754296894559, 0.3333333333333333703, 0.3219752754296894559, 0.3333333333333333703, 0.3219752754296894559, 0.3333333333333333703, 0.3219752754296894559, 0.3333333333333333703, 0.3219752754296894559, 0.3333333333333333703, 0.3219752754296894559, 0.3333333333333333703, 0.3219752754296894559, 0.3333333333333333703, 0.3219752754296894559, 0.3333333333333333703, 0.3219752754296894559, 0.3333333333333333703, 0.3219752754296894559, 0.3333333333333333703, 0.3219752754296894559, 0.3333333333333333703, 0.3219752754296894559, 0.3333333333333333703, 0.3219752754296894559, 0.3333333333333333703),
 ( 1.000000000000000000, 0.9659258262890683122, 1.000000000000000000, 0.9659258262890683122, 1.000000000000000000, 0.9659258262890683122, 1.000000000000000000, 0.9659258262890683122, 1.000000000000000000, 0.9659258262890683122, 1.000000000000000000, 0.9659258262890683122, 1.000000000000000000, 0.9659258262890683122, 1.000000000000000000, 0.9659258262890683122, 1.000000000000000000, 0.9659258262890683122, 1.000000000000000000, 0.9659258262890683122, 1.000000000000000000, 0.9659258262890683122, 1.000000000000000000, 0.9659258262890683122, 1.000000000000000000, 0.9659258262890683122, 1.000000000000000000, 0.9659258262890683122, 1.000000000000000000, 0.9659258262890683122, 1.000000000000000000, 0.9659258262890683122, 1.000000000000000000, 0.9659258262890683122, 1.000000000000000000, 0.9659258262890683122, 1.000000000000000000, 0.9659258262890683122, 1.000000000000000000, 0.9659258262890683122, 1.000000000000000000, 0.9659258262890683122, 1.000000000000000000, 0.9659258262890683122, 1.000000000000000000, 0.9659258262890683122, 1.000000000000000000, 0.9659258262890683122, 1.000000000000000000, 0.9659258262890683122, 1.000000000000000000, 0.9659258262890683122, 1.000000000000000000, 0.9659258262890683122, 1.000000000000000000, 0.9659258262890683122, 1.000000000000000000, 0.9659258262890683122, 1.000000000000000000, 0.9659258262890683122, 1.000000000000000000, 0.9659258262890683122, 1.000000000000000000, 0.9659258262890683122, 1.000000000000000000, 0.9659258262890683122, 1.000000000000000000, 0.9659258262890683122, 1.000000000000000000, 0.9659258262890683122, 1.000000000000000000, 0.9659258262890683122, 1.000000000000000000, 0.9659258262890683122, 1.000000000000000000, 0.9659258262890683122, 1.000000000000000000, 0.9659258262890683122, 1.000000000000000000, 0.9659258262890683122, 1.000000000000000000, 0.9659258262890683122, 1.000000000000000000, 0.9659258262890683122, 1.000000000000000000, 0.9659258262890683122, 1.000000000000000000, 0.9659258262890683122, 1.000000000000000000, 0.9659258262890683122, 1.000000000000000000, 0.9659258262890683122, 1.000000000000000000, 0.9659258262890683122, 1.000000000000000000, 0.9659258262890683122, 1.000000000000000000, 0.9659258262890683122, 1.000000000000000000, 0.9659258262890683122, 1.000000000000000000, 0.9659258262890683122, 1.000000000000000000, 0.9659258262890683122, 1.000000000000000000, 0.9659258262890683122, 1.000000000000000000, 0.9659258262890683122, 1.000000000000000000, 0.9659258262890683122, 1.000000000000000000, 0.9659258262890683122, 1.000000000000000000, 0.9659258262890683122, 1.000000000000000000, 0.9659258262890683122, 1.000000000000000000, 0.9659258262890683122, 1.000000000000000000, 0.9659258262890683122, 1.000000000000000000, 0.9659258262890683122, 1.000000000000000000, 0.9659258262890683122, 1.000000000000000000, 0.9659258262890683122, 1.000000000000000000, 0.9659258262890683122, 1.000000000000000000, 0.9659258262890683122, 1.000000000000000000, 0.9659258262890683122, 1.000000000000000000, 0.9659258262890683122, 1.000000000000000000, 0.9659258262890683122, 1.000000000000000000, 0.9659258262890683122, 1.000000000000000000, 0.9659258262890683122, 1.000000000000000000, 0.9659258262890683122, 1.000000000000000000, 0.9659258262890683122, 1.000000000000000000, 0.9659258262890683122, 1.000000000000000000, 0.9659258262890683122, 1.000000000000000000, 0.9659258262890683122, 1.000000000000000000, 0.9659258262890683122, 1.000000000000000000, 0.9659258262890683122, 1.000000000000000000, 0.9659258262890683122, 1.000000000000000000, 0.9659258262890683122, 1.000000000000000000, 0.9659258262890683122, 1.000000000000000000, 0.9659258262890683122, 1.000000000000000000, 0.9659258262890683122, 1.000000000000000000, 0.9659258262890683122, 1.000000000000000000, 0.9659258262890683122, 1.000000000000000000, 0.9659258262890683122, 1.000000000000000000, 0.9659258262890683122, 1.000000000000000000, 0.9659258262890683122, 1.000000000000000000, 0.9659258262890683122, 1.000000000000000000, 0.9659258262890683122, 1.000000000000000000, 0.9659258262890683122, 1.000000000000000000, 0.9659258262890683122, 1.000000000000000000, 0.9659258262890683122, 1.000000000000000000, 0.9659258262890683122, 1.000000000000000000, 0.9659258262890683122, 1.000000000000000000, 0.9659258262890683122, 1.000000000000000000, 0.9659258262890683122, 1.000000000000000000, 0.9659258262890683122, 1.000000000000000000, 0.9659258262890683122, 1.000000000000000000, 0.9659258262890683122, 1.000000000000000000, 0.9659258262890683122, 1.000000000000000000, 0.9659258262890683122, 1.000000000000000000, 0.9659258262890683122, 1.000000000000000000, 0.9659258262890683122, 1.000000000000000000, 0.9659258262890683122, 1.000000000000000000, 0.9659258262890683122, 1.000000000000000000, 0.9659258262890683122, 1.000000000000000000, 0.9659258262890683122, 1.000000000000000000, 0.9659258262890683122, 1.000000000000000000, 0.9659258262890683122, 1.000000000000000000, 0.9659258262890683122, 1.000000000000000000, 0.9659258262890683122, 1.000000000000000000, 0.9659258262890683122, 1.000000000000000000, 0.9659258262890683122, 1.000000000000000000, 0.9659258262890683122, 1.000000000000000000, 0.9659258262890683122, 1.000000000000000000, 0.9659258262890683122, 1.000000000000000000, 0.9659258262890683122, 1.000000000000000000, 0.9659258262890683122, 1.000000000000000000, 0.9659258262890683122, 1.000000000000000000, 0.9659258262890683122, 1.000000000000000000, 0.9659258262890683122, 1.000000000000000000, 0.9659258262890683122, 1.000000000000000000, 0.9659258262890683122, 1.000000000000000000, 0.9659258262890683122, 1.000000000000000000, 0.9659258262890683122, 1.000000000000000000, 0.9659258262890683122, 1.000000000000000000, 0.9659258262890683122, 1.000000000000000000, 0.9659258262890683122, 1.000000000000000000, 0.9659258262890683122, 1.000000000000000000, 0.9659258262890683122, 1.000000000000000000, 0.9659258262890683122, 1.000000000000000000, 0.9659258262890683122, 1.000000000000000000, 0.9659258262890683122, 1.000000000000000000, 0.9659258262890683122, 1.000000000000000000, 0.9659258262890683122, 1.000000000000000000, 0.9659258262890683122, 1.000000000000000000, 0.9659258262890683122, 1.000000000000000000, 0.9659258262890683122, 1.000000000000000000, 0.9659258262890683122, 1.000000000000000000, 0.9659258262890683122, 1.000000000000000000, 0.9659258262890683122, 1.000000000000000000, 0.9659258262890683122, 1.000000000000000000, 0.9659258262890683122, 1.000000000000000000, 0.9659258262890683122, 1.000000000000000000, 0.9659258262890683122, 1.000000000000000000, 0.9659258262890683122, 1.000000000000000000, 0.9659258262890683122, 1.000000000000000000, 0.9659258262890683122, 1.000000000000000000, 0.9659258262890683122, 1.000000000000000000, 0.9659258262890683122, 1.000000000000000000, 0.9659258262890683122, 1.000000000000000000, 0.9659258262890683122, 1.000000000000000000, 0.9659258262890683122, 1.000000000000000000, 0.9659258262890683122, 1.000000000000000000, 0.9659258262890683122, 1.000000000000000000, 0.9659258262890683122, 1.000000000000000000, 0.9659258262890683122, 1.000000000000000000, 0.9659258262890683122, 1.000000000000000000, 0.9659258262890683122, 1.000000000000000000, 0.9659258262890683122, 1.000000000000000000, 0.9659258262890683122, 1.000000000000000000, 0.9659258262890683122, 1.000000000000000000, 0.9659258262890683122, 1.000000000000000000, 0.9659258262890683122, 1.000000000000000000, 0.9659258262890683122, 1.000000000000000000, 0.9659258262890683122, 1.000000000000000000, 0.9659258262890683122, 1.000000000000000000, 0.9659258262890683122, 1.000000000000000000, 0.9659258262890683122, 1.000000000000000000, 0.9659258262890683122, 1.000000000000000000, 0.9659258262890683122, 1.000000000000000000, 0.9659258262890683122, 1.000000000000000000, 0.9659258262890683122, 1.000000000000000000, 0.9659258262890683122, 1.000000000000000000, 0.9659258262890683122, 1.000000000000000000, 0.9659258262890683122, 1.000000000000000000, 0.9659258262890683122, 1.000000000000000000, 0.9659258262890683122, 1.000000000000000000, 0.9659258262890683122, 1.000000000000000000, 0.9659258262890683122, 1.000000000000000000, 0.9659258262890683122, 1.000000000000000000, 0.9659258262890683122, 1.000000000000000000, 0.9659258262890683122, 1.000000000000000000, 0.9659258262890683122, 1.000000000000000000, 0.9659258262890683122, 1.000000000000000000, 0.9659258262890683122, 1.000000000000000000, 0.9659258262890683122, 1.000000000000000000, 0.9659258262890683122, 1.000000000000000000, 0.9659258262890683122, 1.000000000000000000, 0.9659258262890683122, 1.000000000000000000, 0.9659258262890683122, 1.000000000000000000, 0.9659258262890683122, 1.000000000000000000, 0.9659258262890683122, 1.000000000000000000, 0.9659258262890683122, 1.000000000000000000, 0.9659258262890683122, 1.000000000000000000, 0.9659258262890683122, 1.000000000000000000, 0.9659258262890683122, 1.000000000000000000, 0.9659258262890683122, 1.000000000000000000, 0.9659258262890683122, 1.000000000000000000, 0.9659258262890683122, 1.000000000000000000, 0.9659258262890683122, 1.000000000000000000, 0.9659258262890683122, 1.000000000000000000, 0.9659258262890683122, 1.000000000000000000, 0.9659258262890683122, 1.000000000000000000, 0.9659258262890683122, 1.000000000000000000, 0.9659258262890683122, 1.000000000000000000, 0.9659258262890683122, 1.000000000000000000, 0.9659258262890683122, 1.000000000000000000, 0.9659258262890683122, 1.000000000000000000, 0.9659258262890683122, 1.000000000000000000, 0.9659258262890683122, 1.000000000000000000, 0.9659258262890683122, 1.000000000000000000, 0.9659258262890683122, 1.000000000000000000, 0.9659258262890683122, 1.000000000000000000, 0.9659258262890683122, 1.000000000000000000, 0.9659258262890683122, 1.000000000000000000, 0.9659258262890683122, 1.000000000000000000, 0.9659258262890683122, 1.000000000000000000, 0.9659258262890683122, 1.000000000000000000, 0.9659258262890683122, 1.000000000000000000, 0.9659258262890683122, 1.000000000000000000, 0.9659258262890683122, 1.000000000000000000, 0.9659258262890683122, 1.000000000000000000, 0.9659258262890683122, 1.000000000000000000, 0.9659258262890683122, 1.000000000000000000, 0.9659258262890683122, 1.000000000000000000, 0.9659258262890683122, 1.000000000000000000, 0.9659258262890683122, 1.000000000000000000) ) ) 
 REPRESENTATION_ITEM ( '' )  SURFACE ( )  );
#20743=CARTESIAN_POINT ( 'NONE',  ( -12.14591786802326823, 12.06949235617739902, 33.12609039468569705 ) ) ;
#20744=CARTESIAN_POINT ( 'NONE',  ( -4.379528057220328563, 16.55341960407611168, 65.20724293864768129 ) ) ;
#20745=CARTESIAN_POINT ( 'NONE',  ( -21.53943276465977519, -0.05219959533937600094, 83.75109039468568994 ) ) ;
#20746=CARTESIAN_POINT ( 'NONE',  ( 14.34966873604972726, -8.224510206698740333, 105.8344237280190328 ) ) ;
#20747=CARTESIAN_POINT ( 'NONE',  ( 17.26172910966779384, 6.454744622555870670, 26.69353091350777518 ) ) ;
#20748=CARTESIAN_POINT ( 'NONE',  ( -18.87255363501903105, -5.499999999999950262, 66.32513748171827217 ) ) ;
#20749=CARTESIAN_POINT ( 'NONE',  ( 14.34966873604960469, 8.224510206698951720, 24.16557627198103120 ) ) ;
#20750=CARTESIAN_POINT ( 'NONE',  ( -8.314922557961024197, 14.29746914071037800, 72.91775706135234714 ) ) ;
#20751=CARTESIAN_POINT ( 'NONE',  ( 16.51473224551069308, 9.474510206698969483, 84.16557627198102409 ) ) ;
#20752=CARTESIAN_POINT ( 'NONE',  ( -5.153800228976328057, -19.02544592524343514, 97.29057627198099567 ) ) ;
#20753=CARTESIAN_POINT ( 'NONE',  ( 5.719274019375673035, 21.55341960407619339, 92.29275706135236135 ) ) ;
#20754=CARTESIAN_POINT ( 'NONE',  ( -0.05219959533934338120, 16.53943276465976808, 87.50109039468568994 ) ) ;
#20755=CARTESIAN_POINT ( 'NONE',  ( -16.52544592524342804, 4.483927247898546575, 56.04057627198102409 ) ) ;
#20756=CARTESIAN_POINT ( 'NONE',  ( -0.05219959533909027116, -19.03943276465977164, 72.49890960531435269 ) ) ;
#20758=CARTESIAN_POINT ( 'NONE',  ( -9.564922557961040184, 16.46253265017147172, 107.9177570613523471 ) ) ;
#20759=CARTESIAN_POINT ( 'NONE',  ( -16.51473224551069308, -9.474510206698971260, 21.66557627198102765 ) ) ;
#20760=CARTESIAN_POINT ( 'NONE',  ( -16.46253265017160317, 9.564922557960807481, 80.83224293864769550 ) ) ;
#20761=CARTESIAN_POINT ( 'NONE',  ( -5.049401038297874678, -19.05341960407617918, 109.7927570613523187 ) ) ;
#20763=CARTESIAN_POINT ( 'NONE',  ( -19.05341960407617563, 5.049401038297882671, 23.54275706135233648 ) ) ;
#20764=CARTESIAN_POINT ( 'NONE',  ( 4.379528057220092307, 16.55341960407617563, 82.29275706135234714 ) ) ;
#20765=CARTESIAN_POINT ( 'NONE',  ( 19.03943276465977164, 0.05219959533936151252, 111.2510903946856757 ) ) ;
#20766=CARTESIAN_POINT ( 'NONE',  ( 16.53943276465976808, -0.05219959533910856209, 113.7489096053143527 ) ) ;
#20767=CARTESIAN_POINT ( 'NONE',  ( 4.483927247898790824, -16.52544592524335698, 60.20942372801902565 ) ) ;
#20768=CARTESIAN_POINT ( 'NONE',  ( -12.14591786802326823, 12.06949235617739902, 48.12609039468568284 ) ) ;
#20769=CARTESIAN_POINT ( 'NONE',  ( -9.474510206698964154, 16.51473224551069663, 25.41557627198103120 ) ) ;
#20770=CARTESIAN_POINT ( 'NONE',  ( 9.564922557961047289, -16.46253265017146816, 70.41775706135233293 ) ) ;
#20771=CARTESIAN_POINT ( 'NONE',  ( -5.719274019375665041, -21.55341960407619695, 109.7927570613523613 ) ) ;
#20772=CARTESIAN_POINT ( 'NONE',  ( -9.474510206698964154, 16.51473224551069663, 40.41557627198103120 ) ) ;
#20773=CARTESIAN_POINT ( 'NONE',  ( 19.05341960407611168, 5.049401038298154454, 78.95724293864769550 ) ) ;
#20774=CARTESIAN_POINT ( 'NONE',  ( 14.29746914071049879, -8.314922557960816363, 73.33224293864769550 ) ) ;
#20776=CARTESIAN_POINT ( 'NONE',  ( 13.97604488694548053, -13.89961937509957401, 35.62609039468567573 ) ) ;
#20777=CARTESIAN_POINT ( 'NONE',  ( -15.72974639402197994, 15.80617190586746368, 40.62390960531435269 ) ) ;
#20778=CARTESIAN_POINT ( 'NONE',  ( -15.80617190586768217, 15.72974639402176855, 108.1260903946856757 ) ) ;
#20779=CARTESIAN_POINT ( 'NONE',  ( 13.89961937509977652, -13.97604488694527269, 88.12390960531438111 ) ) ;
#20780=CARTESIAN_POINT ( 'NONE',  ( 21.53943276465977519, 0.05219959533937863772, 101.2510903946856757 ) ) ;
#20781=CARTESIAN_POINT ( 'NONE',  ( -10.81492255796078084, -18.62759615963271287, 67.08224293864770971 ) ) ;
#20782=CARTESIAN_POINT ( 'NONE',  ( -9.474510206698964154, 16.51473224551069663, 100.4155762719810241 ) ) ;
#20783=CARTESIAN_POINT ( 'NONE',  ( -19.05341960407617563, 5.049401038297882671, 78.54275706135233293 ) ) ;
#20784=CARTESIAN_POINT ( 'NONE',  ( -0.05219959533909027116, -19.03943276465977164, 97.49890960531436690 ) ) ;
#20785=CARTESIAN_POINT ( 'NONE',  ( 16.51473224551083163, -9.474510206698727899, 95.83442372801900433 ) ) ;
#20786=CARTESIAN_POINT ( 'NONE',  ( -12.14591786802326823, 12.06949235617739902, 53.12609039468568284 ) ) ;
#20787=CARTESIAN_POINT ( 'NONE',  ( -19.03943276465977164, 0.05219959533909376836, 21.24890960531436335 ) ) ;
#20788=CARTESIAN_POINT ( 'NONE',  ( 5.153800228976335163, 19.02544592524342804, 79.79057627198102409 ) ) ;
#20789=CARTESIAN_POINT ( 'NONE',  ( 5.719274019375991003, -21.55341960407610458, 67.70724293864769550 ) ) ;
#20790=CARTESIAN_POINT ( 'NONE',  ( -16.55341960407617563, 4.379528057220093196, 33.54275706135234714 ) ) ;
#20791=CARTESIAN_POINT ( 'NONE',  ( -21.55341960407619339, 5.719274019375674811, 33.54275706135234714 ) ) ;
#20792=CARTESIAN_POINT ( 'NONE',  ( 18.67979575497194134, -10.72451020669871369, 90.83442372801901854 ) ) ;
#20793=CARTESIAN_POINT ( 'NONE',  ( -16.52544592524335698, -4.483927247898792601, 93.95942372801903275 ) ) ;
#20794=CARTESIAN_POINT ( 'NONE',  ( 5.049401038298161559, -19.05341960407611168, 82.70724293864770971 ) ) ;
#20795=CARTESIAN_POINT ( 'NONE',  ( -0.05219959533910754901, -16.53943276465976808, 77.49890960531433848 ) ) ;
#20796=CARTESIAN_POINT ( 'NONE',  ( 14.34966873604960469, 8.224510206698951720, 24.16557627198103120 ) ) ;
#20797=CARTESIAN_POINT ( 'NONE',  ( 5.153800228976615827, -19.02544592524334988, 70.20942372801899012 ) ) ;
#20798=CARTESIAN_POINT ( 'NONE',  ( -5.719274019375665041, -21.55341960407619695, 49.79275706135234714 ) ) ;
#20799=CARTESIAN_POINT ( 'NONE',  ( 16.53943276465976808, -0.05219959533910856209, 98.74890960531438111 ) ) ;
#20800=CARTESIAN_POINT ( 'NONE',  ( 0.05219959533909260263, 19.03943276465977164, 109.9989096053143669 ) ) ;
#20801=CARTESIAN_POINT ( 'NONE',  ( -8.314922557961024197, 14.29746914071037800, 107.9177570613523471 ) ) ;
#20802=CARTESIAN_POINT ( 'NONE',  ( 21.53943276465977519, 0.05219959533937863772, 86.25109039468568994 ) ) ;
#20803=CARTESIAN_POINT ( 'NONE',  ( 8.314922557961029526, -14.29746914071037800, 40.41775706135234714 ) ) ;
#20804=CARTESIAN_POINT ( 'NONE',  ( -15.72974639402176322, -15.80617190586768395, 44.37609039468567573 ) ) ;
#20806=CARTESIAN_POINT ( 'NONE',  ( -0.05219959533907301413, -21.53943276465977519, 112.4989096053143669 ) ) ;
#20807=CARTESIAN_POINT ( 'NONE',  ( -4.483927247898539470, -16.52544592524342804, 97.29057627198105251 ) ) ;
#20808=CARTESIAN_POINT ( 'NONE',  ( 17.50000000000005329, -4.049696124445820722, 26.68039670665946161 ) ) ;
#20809=CARTESIAN_POINT ( 'NONE',  ( 0.05219959533910956823, 16.53943276465976808, 64.99890960531435269 ) ) ;
#20810=CARTESIAN_POINT ( 'NONE',  ( -12.14591786802326823, 12.06949235617739902, 113.1260903946856899 ) ) ;
#20811=CARTESIAN_POINT ( 'NONE',  ( -9.474510206698964154, 16.51473224551069663, 35.41557627198102409 ) ) ;
#20812=CARTESIAN_POINT ( 'NONE',  ( -10.81492255796078084, -18.62759615963271287, 37.08224293864768129 ) ) ;
#20813=CARTESIAN_POINT ( 'NONE',  ( 14.29746914071049879, -8.314922557960816363, 83.33224293864769550 ) ) ;
#20814=CARTESIAN_POINT ( 'NONE',  ( -5.823673210054116645, -21.52544592524344225, 82.29057627198103830 ) ) ;
#20815=CARTESIAN_POINT ( 'NONE',  ( -5.153800228976328057, -19.02544592524343514, 87.29057627198103830 ) ) ;
#20817=CARTESIAN_POINT ( 'NONE',  ( 9.474510206698971260, -16.51473224551069308, 42.91557627198103120 ) ) ;
#20818=CARTESIAN_POINT ( 'NONE',  ( -5.049401038297874678, -19.05341960407617918, 89.79275706135230450 ) ) ;
#20819=CARTESIAN_POINT ( 'NONE',  ( 5.719274019375991003, -21.55341960407610458, 27.70724293864769905 ) ) ;
#20820=CARTESIAN_POINT ( 'NONE',  ( -21.55341960407619339, 5.719274019375674811, 73.54275706135234714 ) ) ;
#20821=CARTESIAN_POINT ( 'NONE',  ( 19.05341960407611168, 5.049401038298154454, 48.95724293864768129 ) ) ;
#20822=CARTESIAN_POINT ( 'NONE',  ( -13.97604488694527625, -13.89961937509977652, 86.87390960531436690 ) ) ;
#20824=CARTESIAN_POINT ( 'NONE',  ( 0.05219959533934541429, -16.53943276465976808, 60.00109039468568284 ) ) ;
#20825=CARTESIAN_POINT ( 'NONE',  ( 0.05219959533937995610, -21.53943276465977519, 45.00109039468568284 ) ) ;
#20826=AXIS2_PLACEMENT_3D ( 'NONE', #186359, #142800, #63988 ) ;
#20827=CARTESIAN_POINT ( 'NONE',  ( 15.72974639402176855, 15.80617190586768217, 66.87609039468568994 ) ) ;
#20828=CARTESIAN_POINT ( 'NONE',  ( 10.81492255796078972, 18.62759615963270932, 24.58224293864768839 ) ) ;
#20829=CARTESIAN_POINT ( 'NONE',  ( 21.53943276465977519, -0.05219959533907433946, 98.74890960531438111 ) ) ;
#20830=CARTESIAN_POINT ( 'NONE',  ( -18.67979575497193778, 10.72451020669871902, 23.33442372801901499 ) ) ;
#20831=CARTESIAN_POINT ( 'NONE',  ( 0.05219959533934541429, -16.53943276465976808, 60.00109039468568284 ) ) ;
#20832=CARTESIAN_POINT ( 'NONE',  ( -15.80617190586745835, -15.72974639402198527, 66.87390960531436690 ) ) ;
#20833=CARTESIAN_POINT ( 'NONE',  ( 15.72974639402176855, 15.80617190586768217, 111.8760903946856615 ) ) ;
#20834=CARTESIAN_POINT ( 'NONE',  ( -16.51473224551069308, -9.474510206698971260, 66.66557627198102409 ) ) ;
#20835=CARTESIAN_POINT ( 'NONE',  ( -8.224510206698735004, -14.34966873604973081, 104.5844237280190185 ) ) ;
#20837=CARTESIAN_POINT ( 'NONE',  ( -9.474510206698964154, 16.51473224551069663, 90.41557627198103830 ) ) ;
#20838=CARTESIAN_POINT ( 'NONE',  ( -0.05219959533934338120, 16.53943276465976808, 42.50109039468567573 ) ) ;
#20840=CARTESIAN_POINT ( 'NONE',  ( 9.474510206698729675, 16.51473224551082808, 82.08442372801899012 ) ) ;
#20841=CARTESIAN_POINT ( 'NONE',  ( -18.62759615963270932, 10.81492255796079327, 60.83224293864769550 ) ) ;
#20842=CARTESIAN_POINT ( 'NONE',  ( -4.379528057220328563, 16.55341960407611168, 25.20724293864769550 ) ) ;
#20843=CARTESIAN_POINT ( 'NONE',  ( 16.51473224551083163, -9.474510206698727899, 100.8344237280190043 ) ) ;
#20844=CARTESIAN_POINT ( 'NONE',  ( -17.49999999999999645, 5.499999999999997335, 120.0000000000000142 ) ) ;
#20845=CARTESIAN_POINT ( 'NONE',  ( 0.05219959533936267826, -19.03943276465977164, 95.00109039468567573 ) ) ;
#20846=CARTESIAN_POINT ( 'NONE',  ( -18.67979575497178146, -10.72451020669898902, 86.66557627198102409 ) ) ;
#20847=CARTESIAN_POINT ( 'NONE',  ( -19.05341960407617563, 5.049401038297882671, 63.54275706135234003 ) ) ;
#20849=CARTESIAN_POINT ( 'NONE',  ( 16.51473224551069308, 9.474510206698969483, 74.16557627198103830 ) ) ;
#20850=CARTESIAN_POINT ( 'NONE',  ( 14.29746914071049879, -8.314922557960816363, 58.33224293864768839 ) ) ;
#20853=CARTESIAN_POINT ( 'NONE',  ( 9.564922557960805705, 16.46253265017160317, 49.58224293864770260 ) ) ;
#20854=CARTESIAN_POINT ( 'NONE',  ( 14.34966873604960469, 8.224510206698951720, 54.16557627198103120 ) ) ;
#20856=CARTESIAN_POINT ( 'NONE',  ( 12.06949235617757843, -12.14591786802309237, 28.12390960531435979 ) ) ;
#20857=CARTESIAN_POINT ( 'NONE',  ( -19.03943276465977164, 0.05219959533909376836, 66.24890960531436690 ) ) ;
#20859=CARTESIAN_POINT ( 'NONE',  ( -9.564922557961040184, 16.46253265017147172, 32.91775706135233293 ) ) ;
#20860=CARTESIAN_POINT ( 'NONE',  ( -4.379528057220086978, -16.55341960407618274, 49.79275706135234714 ) ) ;
#20861=CARTESIAN_POINT ( 'NONE',  ( 10.72451020669898902, -18.67979575497178502, 52.91557627198103830 ) ) ;
#20862=CARTESIAN_POINT ( 'NONE',  ( 18.62759615963255655, 10.81492255796105972, 111.6677570613523613 ) ) ;
#20863=CARTESIAN_POINT ( 'NONE',  ( -5.153800228976328057, -19.02544592524343514, 72.29057627198102409 ) ) ;
#20864=CARTESIAN_POINT ( 'NONE',  ( -16.46253265017160317, 9.564922557960807481, 115.8322429386477097 ) ) ;
#20865=CARTESIAN_POINT ( 'NONE',  ( 19.02544592524343514, -5.153800228976328945, 108.5405762719810383 ) ) ;
#20867=CARTESIAN_POINT ( 'NONE',  ( -18.62759615963255300, -10.81492255796106328, 44.16775706135234714 ) ) ;
#20868=CARTESIAN_POINT ( 'NONE',  ( 4.483927247898545687, 16.52544592524342804, 89.79057627198103830 ) ) ;
#20869=CARTESIAN_POINT ( 'NONE',  ( 5.719274019375991003, -21.55341960407610458, 87.70724293864769550 ) ) ;
#20870=CARTESIAN_POINT ( 'NONE',  ( 19.05341960407611168, 5.049401038298154454, 83.95724293864766707 ) ) ;
#20871=CARTESIAN_POINT ( 'NONE',  ( 17.49999999999998579, -5.500000000000023981, 68.29690382534171533 ) ) ;
#20872=CARTESIAN_POINT ( 'NONE',  ( 16.46253265017160672, -9.564922557960803928, 93.33224293864769550 ) ) ;
#20873=CARTESIAN_POINT ( 'NONE',  ( -5.719274019375665041, -21.55341960407619695, 19.79275706135235069 ) ) ;
#20874=ORIENTED_EDGE ( 'NONE', *, *, #64542, .T. ) ;
#20875=CARTESIAN_POINT ( 'NONE',  ( -13.97604488694527625, -13.89961937509977652, 76.87390960531433848 ) ) ;
#20876=CARTESIAN_POINT ( 'NONE',  ( 19.48894818550245489, -5.499999999999906741, 97.60307310435237582 ) ) ;
#20877=CARTESIAN_POINT ( 'NONE',  ( -0.05219959533909027116, -19.03943276465977164, 22.49890960531436690 ) ) ;
#20878=CARTESIAN_POINT ( 'NONE',  ( -19.02544592524342804, 5.153800228976336051, 36.04057627198100988 ) ) ;
#20879=CARTESIAN_POINT ( 'NONE',  ( 5.153800228976615827, -19.02544592524334988, 110.2094237280189901 ) ) ;
#20881=CARTESIAN_POINT ( 'NONE',  ( -16.55341960407611168, -4.379528057220339221, 111.4572429386476813 ) ) ;
#20882=CARTESIAN_POINT ( 'NONE',  ( -21.52544592524334988, -5.823673210054445271, 73.95942372801901854 ) ) ;
#20883=CARTESIAN_POINT ( 'NONE',  ( 13.89961937509977652, -13.97604488694527269, 58.12390960531436690 ) ) ;
#20884=CARTESIAN_POINT ( 'NONE',  ( -10.72451020669870658, -18.67979575497194134, 39.58442372801901143 ) ) ;
#20885=CARTESIAN_POINT ( 'NONE',  ( -21.53943276465977519, 0.05219959533907696930, 111.2489096053143669 ) ) ;
#20887=CARTESIAN_POINT ( 'NONE',  ( -5.049401038298153566, 19.05341960407611168, 90.20724293864766707 ) ) ;
#20889=CARTESIAN_POINT ( 'NONE',  ( 16.53943276465976808, 0.05219959533934440121, 31.25109039468568639 ) ) ;
#20890=CARTESIAN_POINT ( 'NONE',  ( 15.72974639402199770, -15.80617190586745480, 43.12390960531435269 ) ) ;
#20891=CARTESIAN_POINT ( 'NONE',  ( 15.72974639402176855, 15.80617190586768217, 56.87609039468568994 ) ) ;
#20892=CARTESIAN_POINT ( 'NONE',  ( -16.46253265017160317, 9.564922557960807481, 115.8322429386477097 ) ) ;
#20893=CARTESIAN_POINT ( 'NONE',  ( 19.03943276465977164, 0.05219959533936151252, 91.25109039468566152 ) ) ;
#20894=CARTESIAN_POINT ( 'NONE',  ( 9.564922557960805705, 16.46253265017160317, 44.58224293864769550 ) ) ;
#20895=CARTESIAN_POINT ( 'NONE',  ( 9.474510206698971260, -16.51473224551069308, 82.91557627198103830 ) ) ;
#20896=CARTESIAN_POINT ( 'NONE',  ( -0.05219959533910754901, -16.53943276465976808, 97.49890960531436690 ) ) ;
#20897=CARTESIAN_POINT ( 'NONE',  ( -14.34966873604960291, -8.224510206698953496, 96.66557627198102409 ) ) ;
#20898=CARTESIAN_POINT ( 'NONE',  ( 5.153800228976335163, 19.02544592524342804, 109.7905762719810099 ) ) ;
#20899=CARTESIAN_POINT ( 'NONE',  ( 0.05219959533910956823, 16.53943276465976808, 59.99890960531436690 ) ) ;
#20900=CARTESIAN_POINT ( 'NONE',  ( 9.474510206698971260, -16.51473224551069308, 47.91557627198102409 ) ) ;
#20901=CARTESIAN_POINT ( 'NONE',  ( 5.719274019375673035, 21.55341960407619339, 62.29275706135236845 ) ) ;
#20902=CARTESIAN_POINT ( 'NONE',  ( 16.46253265017146816, 9.564922557961045513, 86.66775706135233293 ) ) ;
#20903=CARTESIAN_POINT ( 'NONE',  ( 14.29746914071049879, -8.314922557960816363, 68.33224293864769550 ) ) ;
#20904=CARTESIAN_POINT ( 'NONE',  ( 0.05219959533907565091, 21.53943276465977519, 114.9989096053143669 ) ) ;
#20905=CARTESIAN_POINT ( 'NONE',  ( -18.62759615963270932, 10.81492255796079327, 40.83224293864769550 ) ) ;
#20906=CARTESIAN_POINT ( 'NONE',  ( 13.97604488694527802, 13.89961937509977652, 109.3739096053143669 ) ) ;
#20908=CARTESIAN_POINT ( 'NONE',  ( -13.89961937509977652, 13.97604488694528158, 55.62390960531434558 ) ) ;
#20909=CARTESIAN_POINT ( 'NONE',  ( -16.53943276465976808, 0.05219959533911058130, 41.24890960531435269 ) ) ;
#20911=CARTESIAN_POINT ( 'NONE',  ( -0.05219959533934338120, 16.53943276465976808, 107.5010903946856899 ) ) ;
#20912=CARTESIAN_POINT ( 'NONE',  ( 14.29746914071037800, 8.314922557961029526, 81.66775706135236135 ) ) ;
#20913=CARTESIAN_POINT ( 'NONE',  ( 16.51473224551083163, -9.474510206698727899, 35.83442372801899722 ) ) ;
#20914=CARTESIAN_POINT ( 'NONE',  ( -17.48847506799968343, 5.747544572773791494, 70.82697437843283694 ) ) ;
#20915=CARTESIAN_POINT ( 'NONE',  ( -5.153800228976328057, -19.02544592524343514, 97.29057627198099567 ) ) ;
#20916=CARTESIAN_POINT ( 'NONE',  ( -9.474510206698964154, 16.51473224551069663, 50.41557627198102409 ) ) ;
#20917=CARTESIAN_POINT ( 'NONE',  ( 12.14591786802309770, 12.06949235617756955, 59.37390960531436690 ) ) ;
#20918=CARTESIAN_POINT ( 'NONE',  ( 17.97161686094259991, -5.499999999999974243, 48.49637206859247840 ) ) ;
#20919=CARTESIAN_POINT ( 'NONE',  ( 0.05219959533907565091, 21.53943276465977519, 24.99890960531435624 ) ) ;
#20920=CARTESIAN_POINT ( 'NONE',  ( 15.72974639402199770, -15.80617190586745480, 43.12390960531435269 ) ) ;
#20921=CARTESIAN_POINT ( 'NONE',  ( 12.06949235617757843, -12.14591786802309237, 83.12390960531436690 ) ) ;
#20922=CARTESIAN_POINT ( 'NONE',  ( -8.224510206698735004, -14.34966873604973081, 34.58442372801900433 ) ) ;
#20923=CARTESIAN_POINT ( 'NONE',  ( 16.55341960407611168, 4.379528057220329451, 73.95724293864769550 ) ) ;
#20924=CARTESIAN_POINT ( 'NONE',  ( -19.02130022317636815, 5.499999999999598543, 65.78188669246574705 ) ) ;
#20925=CARTESIAN_POINT ( 'NONE',  ( -9.564922557961040184, 16.46253265017147172, 72.91775706135233293 ) ) ;
#20926=CARTESIAN_POINT ( 'NONE',  ( 9.474510206698971260, -16.51473224551069308, 112.9155762719810383 ) ) ;
#20929=CARTESIAN_POINT ( 'NONE',  ( 4.483927247898790824, -16.52544592524335698, 25.20942372801901854 ) ) ;
#20930=CARTESIAN_POINT ( 'NONE',  ( -16.52544592524335698, -4.483927247898792601, 103.9594237280190185 ) ) ;
#20931=CARTESIAN_POINT ( 'NONE',  ( 19.05341960407617918, -5.049401038297876454, 71.04275706135234714 ) ) ;
#20932=CARTESIAN_POINT ( 'NONE',  ( 5.719274019375991003, -21.55341960407610458, 52.70724293864769550 ) ) ;
#20933=CARTESIAN_POINT ( 'NONE',  ( -5.823673210054431948, 21.52544592524334988, 62.70942372801902565 ) ) ;
#20934=CARTESIAN_POINT ( 'NONE',  ( 18.22780087662121673, 5.500000000000056843, 38.98459894673893444 ) ) ;
#20935=CARTESIAN_POINT ( 'NONE',  ( 0.05219959533934541429, -16.53943276465976808, 35.00109039468568284 ) ) ;
#20937=CARTESIAN_POINT ( 'NONE',  ( -16.51473224551069308, -9.474510206698971260, 91.66557627198103830 ) ) ;
#20938=CARTESIAN_POINT ( 'NONE',  ( 13.89961937509977652, -13.97604488694527269, 23.12390960531436335 ) ) ;
#20939=CARTESIAN_POINT ( 'NONE',  ( 0.05219959533910956823, 16.53943276465976808, 89.99890960531438111 ) ) ;
#20941=CARTESIAN_POINT ( 'NONE',  ( -16.46253265017160317, 9.564922557960807481, 105.8322429386476955 ) ) ;
#20943=CARTESIAN_POINT ( 'NONE',  ( 9.474510206698729675, 16.51473224551082808, 102.0844237280190043 ) ) ;
#20944=CARTESIAN_POINT ( 'NONE',  ( -10.72451020669898014, 18.67979575497178502, 80.41557627198103830 ) ) ;
#20945=CARTESIAN_POINT ( 'NONE',  ( 13.97604488694527802, 13.89961937509977652, 44.37390960531435269 ) ) ;
#20946=CARTESIAN_POINT ( 'NONE',  ( 9.564922557961047289, -16.46253265017146816, 65.41775706135233293 ) ) ;
#20947=CARTESIAN_POINT ( 'NONE',  ( 15.80617190586746368, 15.72974639402197994, 114.3739096053143527 ) ) ;
#20948=CARTESIAN_POINT ( 'NONE',  ( -16.51473224551069308, -9.474510206698971260, 71.66557627198102409 ) ) ;
#20949=CARTESIAN_POINT ( 'NONE',  ( 19.05341960407611168, 5.049401038298154454, 103.9572429386476671 ) ) ;
#20950=VERTEX_POINT ( 'NONE', #64172 ) ;
#20951=CARTESIAN_POINT ( 'NONE',  ( 12.14591786802327356, -12.06949235617739191, 30.62609039468567929 ) ) ;
#20952=CARTESIAN_POINT ( 'NONE',  ( -18.62759615963270932, 10.81492255796079327, 100.8322429386477097 ) ) ;
#20953=CARTESIAN_POINT ( 'NONE',  ( 4.483927247898545687, 16.52544592524342804, 104.7905762719810241 ) ) ;
#20954=CARTESIAN_POINT ( 'NONE',  ( -5.049401038298153566, 19.05341960407611168, 95.20724293864770971 ) ) ;
#20955=CARTESIAN_POINT ( 'NONE',  ( 9.474510206698729675, 16.51473224551082808, 67.08442372801900433 ) ) ;
#20956=CARTESIAN_POINT ( 'NONE',  ( 21.52544592524344225, -5.823673210054117533, 88.54057627198103830 ) ) ;
#20957=CARTESIAN_POINT ( 'NONE',  ( -16.53943276465976808, 0.05219959533911058130, 41.24890960531435269 ) ) ;
#20958=CARTESIAN_POINT ( 'NONE',  ( 21.52544592524334988, 5.823673210054432836, 111.4594237280190328 ) ) ;
#20959=CARTESIAN_POINT ( 'NONE',  ( 16.55341960407618274, -4.379528057220086978, 61.04275706135234714 ) ) ;
#20960=CARTESIAN_POINT ( 'NONE',  ( -0.05219959533909027116, -19.03943276465977164, 97.49890960531436690 ) ) ;
#20961=CARTESIAN_POINT ( 'NONE',  ( -9.564922557960796823, -16.46253265017161027, 42.08224293864769550 ) ) ;
#20962=CARTESIAN_POINT ( 'NONE',  ( 10.81492255796106328, -18.62759615963255655, 50.41775706135235424 ) ) ;
#20963=CARTESIAN_POINT ( 'NONE',  ( 10.81492255796106328, -18.62759615963255655, 65.41775706135234714 ) ) ;
#20964=CARTESIAN_POINT ( 'NONE',  ( 19.03943276465977164, -0.05219959533909143690, 63.74890960531435979 ) ) ;
#20965=CARTESIAN_POINT ( 'NONE',  ( 10.72451020669871369, 18.67979575497193778, 32.08442372801901854 ) ) ;
#20966=CARTESIAN_POINT ( 'NONE',  ( 0.05219959533936267826, -19.03943276465977164, 80.00109039468567573 ) ) ;
#20967=CARTESIAN_POINT ( 'NONE',  ( 16.46253265017146816, 9.564922557961045513, 71.66775706135233293 ) ) ;
#20968=CARTESIAN_POINT ( 'NONE',  ( -19.03943276465977164, 0.05219959533909376836, 41.24890960531435269 ) ) ;
#20969=CARTESIAN_POINT ( 'NONE',  ( 14.29746914071037800, 8.314922557961029526, 91.66775706135234714 ) ) ;
#20970=CARTESIAN_POINT ( 'NONE',  ( 5.153800228976335163, 19.02544592524342804, 54.79057627198103120 ) ) ;
#20972=CARTESIAN_POINT ( 'NONE',  ( 16.51473224551069308, 9.474510206698969483, 99.16557627198102409 ) ) ;
#20973=CARTESIAN_POINT ( 'NONE',  ( -5.049401038298153566, 19.05341960407611168, 45.20724293864769550 ) ) ;
#20974=CARTESIAN_POINT ( 'NONE',  ( -18.67979575497178146, -10.72451020669898902, 91.66557627198103830 ) ) ;
#20975=CARTESIAN_POINT ( 'NONE',  ( 4.379528057220092307, 16.55341960407617563, 57.29275706135234714 ) ) ;
#20976=CARTESIAN_POINT ( 'NONE',  ( 16.46253265017146816, 9.564922557961045513, 26.66775706135234003 ) ) ;
#20977=CARTESIAN_POINT ( 'NONE',  ( 19.05341960407611168, 5.049401038298154454, 48.95724293864768129 ) ) ;
#20978=CARTESIAN_POINT ( 'NONE',  ( -12.06949235617756955, 12.14591786802309770, 40.62390960531435269 ) ) ;
#20979=CARTESIAN_POINT ( 'NONE',  ( 4.483927247898545687, 16.52544592524342804, 74.79057627198105251 ) ) ;
#20980=CARTESIAN_POINT ( 'NONE',  ( 16.46253265017160672, -9.564922557960803928, 98.33224293864769550 ) ) ;
#20981=CARTESIAN_POINT ( 'NONE',  ( 13.89961937509977652, -13.97604488694527269, 78.12390960531433848 ) ) ;
#20982=CARTESIAN_POINT ( 'NONE',  ( -18.62759615963255300, -10.81492255796106328, 34.16775706135234714 ) ) ;
#20983=CARTESIAN_POINT ( 'NONE',  ( 19.03943276465977164, -0.05219959533909143690, 88.74890960531436690 ) ) ;
#20984=EDGE_CURVE ( 'NONE', #93070, #137808, #154116, .T. ) ;
#20985=CARTESIAN_POINT ( 'NONE',  ( -18.67979575497193778, 10.72451020669871902, 93.33442372801901854 ) ) ;
#20986=CARTESIAN_POINT ( 'NONE',  ( 8.224510206698742110, 14.34966873604972548, 77.08442372801901854 ) ) ;
#20987=ADVANCED_FACE ( 'NONE', ( #94494 ), #181639, .T. ) ;
#20988=CARTESIAN_POINT ( 'NONE',  ( -15.80617190586768217, 15.72974639402176855, 23.12609039468567573 ) ) ;
#20989=CARTESIAN_POINT ( 'NONE',  ( 5.719274019375991003, -21.55341960407610458, 92.70724293864770971 ) ) ;
#20990=CARTESIAN_POINT ( 'NONE',  ( -12.14591786802309592, -12.06949235617757132, 46.87390960531435979 ) ) ;
#20992=CARTESIAN_POINT ( 'NONE',  ( 0.05219959533909260263, 19.03943276465977164, 44.99890960531435979 ) ) ;
#20993=CARTESIAN_POINT ( 'NONE',  ( 14.34966873604960469, 8.224510206698951720, 69.16557627198102409 ) ) ;
#20994=CARTESIAN_POINT ( 'NONE',  ( -5.823673210054116645, -21.52544592524344225, 27.29057627198103120 ) ) ;
#20995=CARTESIAN_POINT ( 'NONE',  ( 19.02544592524334988, 5.153800228976608722, 31.45942372801900433 ) ) ;
#20996=CARTESIAN_POINT ( 'NONE',  ( 0.05219959533910956823, 16.53943276465976808, 99.99890960531436690 ) ) ;
#20998=CARTESIAN_POINT ( 'NONE',  ( -8.314922557961024197, 14.29746914071037800, 67.91775706135234714 ) ) ;
#20999=CARTESIAN_POINT ( 'NONE',  ( 19.02544592524343514, -5.153800228976328945, 63.54057627198103830 ) ) ;
#21000=CARTESIAN_POINT ( 'NONE',  ( -16.95034065685311830, -6.644554250676003804, 21.23116604354659032 ) ) ;
#21001=CARTESIAN_POINT ( 'NONE',  ( -21.52544592524343514, 5.823673210054127303, 36.04057627198102409 ) ) ;
#21002=CARTESIAN_POINT ( 'NONE',  ( -16.55341960407617563, 4.379528057220093196, 93.54275706135234714 ) ) ;
#21003=CARTESIAN_POINT ( 'NONE',  ( -9.564922557961040184, 16.46253265017147172, 107.9177570613523471 ) ) ;
#21004=CARTESIAN_POINT ( 'NONE',  ( -21.53943276465977519, -0.05219959533937600094, 83.75109039468568994 ) ) ;
#21005=CARTESIAN_POINT ( 'NONE',  ( -16.46253265017160317, 9.564922557960807481, 70.83224293864770971 ) ) ;
#21006=CARTESIAN_POINT ( 'NONE',  ( 0.05219959533907565091, 21.53943276465977519, 109.9989096053143527 ) ) ;
#21007=CARTESIAN_POINT ( 'NONE',  ( -14.34966873604972548, 8.224510206698743886, 58.33442372801901143 ) ) ;
#21008=CARTESIAN_POINT ( 'NONE',  ( -16.55341960407611168, -4.379528057220339221, 111.4572429386476813 ) ) ;
#21009=CARTESIAN_POINT ( 'NONE',  ( 12.06949235617739724, 12.14591786802326823, 21.87609039468567573 ) ) ;
#21010=CARTESIAN_POINT ( 'NONE',  ( 5.153800228976615827, -19.02544592524334988, 80.20942372801901854 ) ) ;
#21011=CARTESIAN_POINT ( 'NONE',  ( 10.81492255796078972, 18.62759615963270932, 74.58224293864768129 ) ) ;
#21012=CARTESIAN_POINT ( 'NONE',  ( -13.89961937509957401, -13.97604488694547875, 49.37609039468567573 ) ) ;
#21013=LINE ( 'NONE', #82669, #44616 ) ;
#21014=CARTESIAN_POINT ( 'NONE',  ( -10.72451020669898014, 18.67979575497178502, 110.4155762719810383 ) ) ;
#21016=CARTESIAN_POINT ( 'NONE',  ( 9.474510206698971260, -16.51473224551069308, 82.91557627198103830 ) ) ;
#21019=CARTESIAN_POINT ( 'NONE',  ( -4.483927247898782831, 16.52544592524335698, 32.70942372801900433 ) ) ;
#21021=CARTESIAN_POINT ( 'NONE',  ( -5.719274019375978568, 21.55341960407610458, 100.2072429386476955 ) ) ;
#21022=CARTESIAN_POINT ( 'NONE',  ( 16.52544592524342804, -4.483927247898539470, 63.54057627198103830 ) ) ;
#21023=CARTESIAN_POINT ( 'NONE',  ( -9.564922557960796823, -16.46253265017161027, 72.08224293864770971 ) ) ;
#21025=CARTESIAN_POINT ( 'NONE',  ( 0.05219959533937995610, -21.53943276465977519, 90.00109039468567573 ) ) ;
#21027=CARTESIAN_POINT ( 'NONE',  ( 4.379528057220092307, 16.55341960407617563, 37.29275706135235424 ) ) ;
#21028=CARTESIAN_POINT ( 'NONE',  ( -5.153800228976607833, 19.02544592524334988, 37.70942372801899722 ) ) ;
#21029=CARTESIAN_POINT ( 'NONE',  ( 21.53943276465977519, 0.05219959533937863772, 46.25109039468567573 ) ) ;
#21030=CARTESIAN_POINT ( 'NONE',  ( -0.05219959533907301413, -21.53943276465977519, 62.49890960531436690 ) ) ;
#21031=CARTESIAN_POINT ( 'NONE',  ( -16.46253265017146816, -9.564922557961047289, 109.1677570613523471 ) ) ;
#21032=CARTESIAN_POINT ( 'NONE',  ( -13.89961937509977652, 13.97604488694528158, 50.62390960531435979 ) ) ;
#21033=CARTESIAN_POINT ( 'NONE',  ( 0.05219959533936267826, -19.03943276465977164, 65.00109039468567573 ) ) ;
#21034=CARTESIAN_POINT ( 'NONE',  ( 0.05219959533937995610, -21.53943276465977519, 80.00109039468568994 ) ) ;
#21035=CARTESIAN_POINT ( 'NONE',  ( 5.049401038297881783, 19.05341960407617563, 67.29275706135234714 ) ) ;
#21036=CARTESIAN_POINT ( 'NONE',  ( -16.51473224551069308, -9.474510206698971260, 31.66557627198102054 ) ) ;
#21037=CARTESIAN_POINT ( 'NONE',  ( -15.72974639402197994, 15.80617190586746368, 55.62390960531436690 ) ) ;
#21038=CARTESIAN_POINT ( 'NONE',  ( -12.14591786802309592, -12.06949235617757132, 56.87390960531436690 ) ) ;
#21040=CARTESIAN_POINT ( 'NONE',  ( -19.05341960407617563, 5.049401038297882671, 28.54275706135232937 ) ) ;
#21041=CARTESIAN_POINT ( 'NONE',  ( -16.52544592524335698, -4.483927247898792601, 83.95942372801900433 ) ) ;
#21042=CARTESIAN_POINT ( 'NONE',  ( -14.29746914071049879, 8.314922557960819915, 50.83224293864770971 ) ) ;
#21043=CARTESIAN_POINT ( 'NONE',  ( -5.719274019375665041, -21.55341960407619695, 84.79275706135234714 ) ) ;
#21044=CARTESIAN_POINT ( 'NONE',  ( 18.62759615963255655, 10.81492255796105972, 76.66775706135234714 ) ) ;
#21045=CARTESIAN_POINT ( 'NONE',  ( 21.53943276465977519, -0.05219959533907433946, 98.74890960531438111 ) ) ;
#21046=CARTESIAN_POINT ( 'NONE',  ( 16.51473224551069308, 9.474510206698969483, 49.16557627198102409 ) ) ;
#21047=CARTESIAN_POINT ( 'NONE',  ( 5.823673210054444382, -21.52544592524334988, 60.20942372801902565 ) ) ;
#21048=CARTESIAN_POINT ( 'NONE',  ( -19.02544592524342804, 5.153800228976336051, 36.04057627198100988 ) ) ;
#21049=CARTESIAN_POINT ( 'NONE',  ( -0.05219959533909027116, -19.03943276465977164, 52.49890960531436690 ) ) ;
#21050=CARTESIAN_POINT ( 'NONE',  ( 16.52544592524342804, -4.483927247898539470, 103.5405762719810383 ) ) ;
#21051=CARTESIAN_POINT ( 'NONE',  ( 0.05219959533909260263, 19.03943276465977164, 104.9989096053143669 ) ) ;
#21052=CARTESIAN_POINT ( 'NONE',  ( -8.224510206698948167, 14.34966873604960824, 55.41557627198102409 ) ) ;
#21053=CARTESIAN_POINT ( 'NONE',  ( 16.52544592524342804, -4.483927247898539470, 108.5405762719810241 ) ) ;
#21054=VECTOR ( 'NONE', #112894, 1000.000000000000000 ) ;
#21055=CARTESIAN_POINT ( 'NONE',  ( 21.55341960407610458, 5.719274019375980345, 78.95724293864769550 ) ) ;
#21056=CARTESIAN_POINT ( 'NONE',  ( 15.72974639402176855, 15.80617190586768217, 41.87609039468568284 ) ) ;
#21059=CARTESIAN_POINT ( 'NONE',  ( 14.29746914071037800, 8.314922557961029526, 36.66775706135234714 ) ) ;
#21061=CARTESIAN_POINT ( 'NONE',  ( 21.53943276465977519, -0.05219959533907433946, 88.74890960531436690 ) ) ;
#21062=CARTESIAN_POINT ( 'NONE',  ( 15.80617190586769283, -15.72974639402175789, 110.6260903946857042 ) ) ;
#21063=CARTESIAN_POINT ( 'NONE',  ( 19.03943276465977164, -0.05219959533909143690, 98.74890960531436690 ) ) ;
#21064=CARTESIAN_POINT ( 'NONE',  ( -5.823673210054431948, 21.52544592524334988, 32.70942372801900433 ) ) ;
#21065=CARTESIAN_POINT ( 'NONE',  ( -18.67979575497178146, -10.72451020669898902, 36.66557627198103120 ) ) ;
#21066=CARTESIAN_POINT ( 'NONE',  ( -16.55341960407617563, 4.379528057220093196, 98.54275706135234714 ) ) ;
#21067=CARTESIAN_POINT ( 'NONE',  ( -18.62759615963255300, -10.81492255796106328, 49.16775706135234003 ) ) ;
#21068=CARTESIAN_POINT ( 'NONE',  ( -21.55341960407619339, 5.719274019375674811, 78.54275706135236135 ) ) ;
#21069=CARTESIAN_POINT ( 'NONE',  ( -21.53943276465977519, -0.05219959533937600094, 108.7510903946857042 ) ) ;
#21070=CARTESIAN_POINT ( 'NONE',  ( -14.34966873604972548, 8.224510206698743886, 73.33442372801901854 ) ) ;
#21071=CARTESIAN_POINT ( 'NONE',  ( -21.55341960407619339, 5.719274019375674811, 43.54275706135235424 ) ) ;
#21072=CARTESIAN_POINT ( 'NONE',  ( 0.05219959533909260263, 19.03943276465977164, 29.99890960531435979 ) ) ;
#21073=CARTESIAN_POINT ( 'NONE',  ( -15.72974639402176322, -15.80617190586768395, 104.3760903946856899 ) ) ;
#21074=CARTESIAN_POINT ( 'NONE',  ( -13.89961937509977652, 13.97604488694528158, 110.6239096053143243 ) ) ;
#21075=CARTESIAN_POINT ( 'NONE',  ( 15.80617190586746368, 15.72974639402197994, 109.3739096053143811 ) ) ;
#21076=CARTESIAN_POINT ( 'NONE',  ( -22.00000000000000000, -5.510910596163089556E-15, 47.50000000000000000 ) ) ;
#21077=CARTESIAN_POINT ( 'NONE',  ( 15.72974639402199770, -15.80617190586745480, 73.12390960531436690 ) ) ;
#21078=CARTESIAN_POINT ( 'NONE',  ( -16.53943276465976808, -0.05219959533934237506, 48.75109039468568284 ) ) ;
#21079=CARTESIAN_POINT ( 'NONE',  ( 16.52544592524342804, -4.483927247898539470, 48.54057627198103120 ) ) ;
#21081=CARTESIAN_POINT ( 'NONE',  ( 9.474510206698729675, 16.51473224551082808, 87.08442372801900433 ) ) ;
#21082=CARTESIAN_POINT ( 'NONE',  ( -16.20579543436678449, 7.371946100355082798, 104.4347916582812985 ) ) ;
#21083=CARTESIAN_POINT ( 'NONE',  ( -8.314922557961024197, 14.29746914071037800, 32.91775706135234714 ) ) ;
#21084=CARTESIAN_POINT ( 'NONE',  ( -18.62759615963270932, 10.81492255796079327, 95.83224293864770971 ) ) ;
#21085=CARTESIAN_POINT ( 'NONE',  ( 18.62759615963271287, -10.81492255796078972, 73.33224293864769550 ) ) ;
#21086=CARTESIAN_POINT ( 'NONE',  ( -9.564922557960796823, -16.46253265017161027, 112.0822429386476955 ) ) ;
#21087=CARTESIAN_POINT ( 'NONE',  ( -4.379528057220086978, -16.55341960407618274, 39.79275706135235424 ) ) ;
#21088=CARTESIAN_POINT ( 'NONE',  ( 5.049401038298161559, -19.05341960407611168, 57.70724293864769550 ) ) ;
#21089=CARTESIAN_POINT ( 'NONE',  ( -5.719274019375665041, -21.55341960407619695, 24.79275706135235779 ) ) ;
#21090=CARTESIAN_POINT ( 'NONE',  ( 9.474510206698729675, 16.51473224551082808, 102.0844237280190043 ) ) ;
#21091=CARTESIAN_POINT ( 'NONE',  ( 16.51473224551069308, 9.474510206698969483, 104.1655762719810241 ) ) ;
#21092=CARTESIAN_POINT ( 'NONE',  ( 19.03943276465977164, -0.05219959533909143690, 93.74890960531435269 ) ) ;
#21093=CARTESIAN_POINT ( 'NONE',  ( 5.719274019375991003, -21.55341960407610458, 92.70724293864770971 ) ) ;
#21094=CARTESIAN_POINT ( 'NONE',  ( 19.05341960407611168, 5.049401038298154454, 53.95724293864770260 ) ) ;
#21096=CARTESIAN_POINT ( 'NONE',  ( 4.483927247898545687, 16.52544592524342804, 69.79057627198102409 ) ) ;
#21098=CARTESIAN_POINT ( 'NONE',  ( 9.564922557960805705, 16.46253265017160317, 109.5822429386476955 ) ) ;
#21099=CARTESIAN_POINT ( 'NONE',  ( -17.60728821186567217, 5.500000000000031974, 60.86690927743003954 ) ) ;
#21100=CARTESIAN_POINT ( 'NONE',  ( -19.05341960407617563, 5.049401038297882671, 83.54275706135233293 ) ) ;
#21102=CARTESIAN_POINT ( 'NONE',  ( -10.72451020669898014, 18.67979575497178502, 95.41557627198102409 ) ) ;
#21103=CARTESIAN_POINT ( 'NONE',  ( -16.51473224551082808, 9.474510206698731452, 48.33442372801900433 ) ) ;
#21104=CARTESIAN_POINT ( 'NONE',  ( -5.719274019375978568, 21.55341960407610458, 25.20724293864769550 ) ) ;
#21106=CARTESIAN_POINT ( 'NONE',  ( 5.719274019375991003, -21.55341960407610458, 57.70724293864770260 ) ) ;
#21107=CARTESIAN_POINT ( 'NONE',  ( -16.51473224551069308, -9.474510206698971260, 81.66557627198103830 ) ) ;
#21108=CARTESIAN_POINT ( 'NONE',  ( -15.80617190586768217, 15.72974639402176855, 78.12609039468570415 ) ) ;
#21109=CARTESIAN_POINT ( 'NONE',  ( 19.05341960407611168, 5.049401038298154454, 38.95724293864767418 ) ) ;
#21110=CARTESIAN_POINT ( 'NONE',  ( 0.05219959533910956823, 16.53943276465976808, 79.99890960531435269 ) ) ;
#21111=CARTESIAN_POINT ( 'NONE',  ( 4.483927247898790824, -16.52544592524335698, 20.20942372801900788 ) ) ;
#21112=CARTESIAN_POINT ( 'NONE',  ( -21.53943276465977519, -0.05219959533937600094, 63.75109039468568284 ) ) ;
#21114=CARTESIAN_POINT ( 'NONE',  ( -5.153800228976607833, 19.02544592524334988, 22.70942372801899012 ) ) ;
#21115=CARTESIAN_POINT ( 'NONE',  ( -16.46253265017146816, -9.564922557961047289, 74.16775706135234714 ) ) ;
#21116=CARTESIAN_POINT ( 'NONE',  ( -0.05219959533937732626, 21.53943276465977519, 27.50109039468567929 ) ) ;
#21118=CARTESIAN_POINT ( 'NONE',  ( -21.53943276465977519, -0.05219959533937600094, 113.7510903946856757 ) ) ;
#21119=CARTESIAN_POINT ( 'NONE',  ( 19.02544592524343514, -5.153800228976328945, 53.54057627198102409 ) ) ;
#21120=CARTESIAN_POINT ( 'NONE',  ( -19.03943276465977164, -0.05219959533935918106, 33.75109039468566863 ) ) ;
#21121=CARTESIAN_POINT ( 'NONE',  ( -16.55341960407617563, 4.379528057220093196, 108.5427570613523756 ) ) ;
#21122=CARTESIAN_POINT ( 'NONE',  ( -16.51473224551069308, -9.474510206698971260, 96.66557627198102409 ) ) ;
#21123=CARTESIAN_POINT ( 'NONE',  ( 10.72451020669871369, 18.67979575497193778, 67.08442372801901854 ) ) ;
#21125=CARTESIAN_POINT ( 'NONE',  ( -17.50000000000003197, -3.237210098469649466, 35.28763012620480310 ) ) ;
#21126=B_SPLINE_CURVE_WITH_KNOTS ( 'NONE', 3,
 ( #18844, #129960, #100643, #115828, #85475, #114818, #191660, #193679, #175499, #176510, #54155, #36972, #83470, #145147, #97623, #177517, #130981, #35976, #20808, #192672, #38987, #70326 ),
 .UNSPECIFIED., .F., .F.,
 ( 4, 2, 2, 2, 2, 2, 2, 2, 2, 2, 4 ),
 ( 7.806255641895631925E-18, 0.001309639967555302834, 0.001964459951332950347, 0.002291869943221771719, 0.002455574939166182621, 0.002619279935110593090, 0.002782984931055003559, 0.002946689926999414462, 0.003274099918888229328, 0.003928919902665864265, 0.005238559870221130670 ),
 .UNSPECIFIED. ) ;
#21127=CARTESIAN_POINT ( 'NONE',  ( -21.52544592524334988, -5.823673210054445271, 83.95942372801900433 ) ) ;
#21128=CARTESIAN_POINT ( 'NONE',  ( 15.72974639402176855, 15.80617190586768217, 101.8760903946857042 ) ) ;
#21130=CARTESIAN_POINT ( 'NONE',  ( -13.89961937509977652, 13.97604488694528158, 100.6239096053143669 ) ) ;
#21131=CARTESIAN_POINT ( 'NONE',  ( 19.03943276465977164, 0.05219959533936151252, 21.25109039468565797 ) ) ;
#21133=CARTESIAN_POINT ( 'NONE',  ( 16.46253265017160672, -9.564922557960803928, 38.33224293864768839 ) ) ;
#21134=CARTESIAN_POINT ( 'NONE',  ( -10.72451020669898014, 18.67979575497178502, 55.41557627198102409 ) ) ;
#21135=CARTESIAN_POINT ( 'NONE',  ( -4.483927247898539470, -16.52544592524342804, 22.29057627198102765 ) ) ;
#21136=CARTESIAN_POINT ( 'NONE',  ( 0.05219959533910956823, 16.53943276465976808, 94.99890960531436690 ) ) ;
#21137=CARTESIAN_POINT ( 'NONE',  ( -5.049401038298153566, 19.05341960407611168, 75.20724293864769550 ) ) ;
#21138=CARTESIAN_POINT ( 'NONE',  ( 21.55341960407619695, -5.719274019375665929, 106.0427570613523471 ) ) ;
#21139=CARTESIAN_POINT ( 'NONE',  ( -9.564922557960796823, -16.46253265017161027, 37.08224293864768839 ) ) ;
#21140=CARTESIAN_POINT ( 'NONE',  ( 14.29746914071049879, -8.314922557960816363, 108.3322429386477097 ) ) ;
#21141=CARTESIAN_POINT ( 'NONE',  ( 5.823673210054444382, -21.52544592524334988, 60.20942372801902565 ) ) ;
#21142=CARTESIAN_POINT ( 'NONE',  ( -10.81492255796078084, -18.62759615963271287, 87.08224293864769550 ) ) ;
#21143=CARTESIAN_POINT ( 'NONE',  ( 13.89961937509957401, 13.97604488694547697, 51.87609039468566863 ) ) ;
#21145=CARTESIAN_POINT ( 'NONE',  ( -5.153800228976328057, -19.02544592524343514, 102.2905762719810383 ) ) ;
#21146=CARTESIAN_POINT ( 'NONE',  ( -12.14591786802309592, -12.06949235617757132, 71.87390960531438111 ) ) ;
#21148=CARTESIAN_POINT ( 'NONE',  ( 19.02544592524334988, 5.153800228976608722, 51.45942372801900433 ) ) ;
#21149=CARTESIAN_POINT ( 'NONE',  ( 13.89961937509977652, -13.97604488694527269, 68.12390960531436690 ) ) ;
#21150=CARTESIAN_POINT ( 'NONE',  ( 8.314922557960818139, 14.29746914071049879, 54.58224293864769550 ) ) ;
#21151=CARTESIAN_POINT ( 'NONE',  ( -13.89961937509957401, -13.97604488694547875, 74.37609039468566152 ) ) ;
#21152=CARTESIAN_POINT ( 'NONE',  ( 17.59860650958994555, -7.585241751806880650, 90.92337014262493256 ) ) ;
#21153=CARTESIAN_POINT ( 'NONE',  ( -5.719274019375978568, 21.55341960407610458, 35.20724293864768839 ) ) ;
#21154=CARTESIAN_POINT ( 'NONE',  ( -0.05219959533910754901, -16.53943276465976808, 107.4989096053143669 ) ) ;
#21156=CARTESIAN_POINT ( 'NONE',  ( 13.89961937509977652, -13.97604488694527269, 58.12390960531436690 ) ) ;
#21157=CARTESIAN_POINT ( 'NONE',  ( -5.823673210054116645, -21.52544592524344225, 62.29057627198102409 ) ) ;
#21158=CARTESIAN_POINT ( 'NONE',  ( 19.02544592524343514, -5.153800228976328945, 33.54057627198102409 ) ) ;
#21159=CARTESIAN_POINT ( 'NONE',  ( -12.14591786802326823, 12.06949235617739902, 73.12609039468567573 ) ) ;
#21160=CARTESIAN_POINT ( 'NONE',  ( -16.46253265017160317, 9.564922557960807481, 55.83224293864769550 ) ) ;
#21161=CARTESIAN_POINT ( 'NONE',  ( 16.46253265017146816, 9.564922557961045513, 51.66775706135233293 ) ) ;
#21162=CARTESIAN_POINT ( 'NONE',  ( -5.719274019375665041, -21.55341960407619695, 69.79275706135234714 ) ) ;
#21163=CARTESIAN_POINT ( 'NONE',  ( 21.53943276465977519, -0.05219959533907433946, 53.74890960531437401 ) ) ;
#21164=CARTESIAN_POINT ( 'NONE',  ( -13.97604488694527625, -13.89961937509977652, 21.87390960531435979 ) ) ;
#21165=CARTESIAN_POINT ( 'NONE',  ( 14.29746914071037800, 8.314922557961029526, 86.66775706135234714 ) ) ;
#21166=CARTESIAN_POINT ( 'NONE',  ( -9.474510206698720793, -16.51473224551083518, 99.58442372801900433 ) ) ;
#21168=CARTESIAN_POINT ( 'NONE',  ( 16.79531203550650886, 7.028104445595489302, 53.75244988220445208 ) ) ;
#21169=CARTESIAN_POINT ( 'NONE',  ( -10.81492255796078084, -18.62759615963271287, 57.08224293864769550 ) ) ;
#21170=CARTESIAN_POINT ( 'NONE',  ( -10.72451020669870658, -18.67979575497194134, 94.58442372801901854 ) ) ;
#21172=CARTESIAN_POINT ( 'NONE',  ( 0.05219959533910956823, 16.53943276465976808, 39.99890960531436690 ) ) ;
#21173=CARTESIAN_POINT ( 'NONE',  ( 0.05219959533910956823, 16.53943276465976808, 54.99890960531435269 ) ) ;
#21174=CARTESIAN_POINT ( 'NONE',  ( -21.55341960407610458, -5.719274019375992779, 86.45724293864770971 ) ) ;
#21175=CARTESIAN_POINT ( 'NONE',  ( -15.72974639402197994, 15.80617190586746368, 85.62390960531436690 ) ) ;
#21177=CARTESIAN_POINT ( 'NONE',  ( 5.719274019375991003, -21.55341960407610458, 27.70724293864769905 ) ) ;
#21178=CARTESIAN_POINT ( 'NONE',  ( -14.34966873604972548, 8.224510206698743886, 73.33442372801901854 ) ) ;
#21180=CARTESIAN_POINT ( 'NONE',  ( -14.29746914071049879, 8.314922557960819915, 80.83224293864769550 ) ) ;
#21181=CARTESIAN_POINT ( 'NONE',  ( 13.97604488694527802, 13.89961937509977652, 34.37390960531436690 ) ) ;
#21184=CARTESIAN_POINT ( 'NONE',  ( -4.379528057220086978, -16.55341960407618274, 99.79275706135234714 ) ) ;
#21185=CARTESIAN_POINT ( 'NONE',  ( -18.62759615963255300, -10.81492255796106328, 24.16775706135235424 ) ) ;
#21186=CARTESIAN_POINT ( 'NONE',  ( 13.89961937509977652, -13.97604488694527269, 83.12390960531436690 ) ) ;
#21187=CARTESIAN_POINT ( 'NONE',  ( -21.52544592524334988, -5.823673210054445271, 48.95942372801902565 ) ) ;
#21188=CARTESIAN_POINT ( 'NONE',  ( -13.89961937509977652, 13.97604488694528158, 110.6239096053143243 ) ) ;
#21191=CARTESIAN_POINT ( 'NONE',  ( -10.81492255796105439, 18.62759615963255655, 42.91775706135235424 ) ) ;
#21192=CARTESIAN_POINT ( 'NONE',  ( -16.46253265017160317, 9.564922557960807481, 35.83224293864768839 ) ) ;
#21193=CARTESIAN_POINT ( 'NONE',  ( 9.564922557960805705, 16.46253265017160317, 99.58224293864770971 ) ) ;
#21194=CARTESIAN_POINT ( 'NONE',  ( 16.51473224551083163, -9.474510206698727899, 55.83442372801899722 ) ) ;
#21195=CARTESIAN_POINT ( 'NONE',  ( -15.72974639402176322, -15.80617190586768395, 29.37609039468568284 ) ) ;
#21196=CARTESIAN_POINT ( 'NONE',  ( 13.89961937509957401, 13.97604488694547697, 56.87609039468564731 ) ) ;
#21197=CARTESIAN_POINT ( 'NONE',  ( 13.89961937509977652, -13.97604488694527269, 23.12390960531436335 ) ) ;
#21198=CARTESIAN_POINT ( 'NONE',  ( -0.05219959533934338120, 16.53943276465976808, 92.50109039468567573 ) ) ;
#21199=CARTESIAN_POINT ( 'NONE',  ( -19.05341960407617563, 5.049401038297882671, 68.54275706135230450 ) ) ;
#21200=CARTESIAN_POINT ( 'NONE',  ( -4.379528057220086978, -16.55341960407618274, 109.7927570613523613 ) ) ;
#21203=CARTESIAN_POINT ( 'NONE',  ( -16.46253265017160317, 9.564922557960807481, 90.83224293864769550 ) ) ;
#21204=CARTESIAN_POINT ( 'NONE',  ( 10.72451020669871369, 18.67979575497193778, 97.08442372801904696 ) ) ;
#21205=CARTESIAN_POINT ( 'NONE',  ( -10.81492255796105439, 18.62759615963255655, 112.9177570613523329 ) ) ;
#21206=CARTESIAN_POINT ( 'NONE',  ( 17.97058386085786097, 5.500000000000042633, 66.50390968646219392 ) ) ;
#21207=CARTESIAN_POINT ( 'NONE',  ( 13.89961937509977652, -13.97604488694527269, 103.1239096053143527 ) ) ;
#21208=CARTESIAN_POINT ( 'NONE',  ( -10.72451020669870658, -18.67979575497194134, 69.58442372801900433 ) ) ;
#21209=CARTESIAN_POINT ( 'NONE',  ( 19.03943276465977164, 0.05219959533936151252, 111.2510903946856757 ) ) ;
#21210=CARTESIAN_POINT ( 'NONE',  ( 9.564922557960805705, 16.46253265017160317, 79.58224293864769550 ) ) ;
#21211=CARTESIAN_POINT ( 'NONE',  ( -21.52544592524343514, 5.823673210054127303, 26.04057627198103475 ) ) ;
#21212=CARTESIAN_POINT ( 'NONE',  ( -16.46253265017160317, 9.564922557960807481, 95.83224293864769550 ) ) ;
#21214=CARTESIAN_POINT ( 'NONE',  ( 0.05219959533909260263, 19.03943276465977164, 84.99890960531436690 ) ) ;
#21215=CARTESIAN_POINT ( 'NONE',  ( 9.474510206698971260, -16.51473224551069308, 62.91557627198102409 ) ) ;
#21216=CARTESIAN_POINT ( 'NONE',  ( -14.29746914071049879, 8.314922557960819915, 25.83224293864769194 ) ) ;
#21217=CARTESIAN_POINT ( 'NONE',  ( -17.05116617787851752, 6.768360034955478000, 98.65675553259194430 ) ) ;
#21218=CARTESIAN_POINT ( 'NONE',  ( 9.474510206698729675, 16.51473224551082808, 72.08442372801900433 ) ) ;
#21219=B_SPLINE_CURVE_WITH_KNOTS ( 'NONE', 3,
 ( #81526, #143213, #139249, #3710, #112882, #188755, #34069, #109904, #50240, #79569, #32082, #124066, #49239, #725, #111896, #62397, #47255, #15919, #128047, #77577 ),
 .UNSPECIFIED., .F., .F.,
 ( 4, 2, 2, 2, 2, 2, 2, 2, 2, 4 ),
 ( 0.004000878361812005950, 0.004499404418916031455, 0.004997930476020056960, 0.005496456533124082465, 0.005994982590228108837, 0.006244245618780100773, 0.006493508647332092709, 0.006992034704436076581, 0.007490560761540060453, 0.007989086818644044324 ),
 .UNSPECIFIED. ) ;
#21220=CARTESIAN_POINT ( 'NONE',  ( -5.153800228976328057, -19.02544592524343514, 92.29057627198099567 ) ) ;
#21221=CARTESIAN_POINT ( 'NONE',  ( 16.53943276465976808, -0.05219959533910856209, 88.74890960531436690 ) ) ;
#21222=CARTESIAN_POINT ( 'NONE',  ( -0.05219959533907301413, -21.53943276465977519, 47.49890960531435979 ) ) ;
#21223=CARTESIAN_POINT ( 'NONE',  ( 10.72451020669898902, -18.67979575497178502, 27.91557627198103830 ) ) ;
#21224=CARTESIAN_POINT ( 'NONE',  ( -16.53943276465976808, 0.05219959533911058130, 101.2489096053143669 ) ) ;
#21225=CARTESIAN_POINT ( 'NONE',  ( -17.26058549869088665, 6.457015423128606990, 53.62254162523932166 ) ) ;
#21226=CARTESIAN_POINT ( 'NONE',  ( 5.153800228976615827, -19.02544592524334988, 45.20942372801901143 ) ) ;
#21227=CARTESIAN_POINT ( 'NONE',  ( -8.314922557960811034, -14.29746914071050412, 32.08224293864769550 ) ) ;
#21228=CARTESIAN_POINT ( 'NONE',  ( -9.564922557960796823, -16.46253265017161027, 107.0822429386476955 ) ) ;
#21229=EDGE_CURVE ( 'NONE', #71844, #46822, #122394, .T. ) ;
#21230=CARTESIAN_POINT ( 'NONE',  ( 21.53943276465977519, 0.05219959533937863772, 61.25109039468567573 ) ) ;
#21231=CARTESIAN_POINT ( 'NONE',  ( -0.05219959533907301413, -21.53943276465977519, 52.49890960531435979 ) ) ;
#21232=CARTESIAN_POINT ( 'NONE',  ( -5.719274019375665041, -21.55341960407619695, 39.79275706135235424 ) ) ;
#21233=CARTESIAN_POINT ( 'NONE',  ( 10.72451020669898902, -18.67979575497178502, 77.91557627198102409 ) ) ;
#21234=CARTESIAN_POINT ( 'NONE',  ( 5.823673210054444382, -21.52544592524334988, 35.20942372801901854 ) ) ;
#21235=CARTESIAN_POINT ( 'NONE',  ( 8.314922557960818139, 14.29746914071049879, 109.5822429386476955 ) ) ;
#21236=CARTESIAN_POINT ( 'NONE',  ( 19.02544592524334988, 5.153800228976608722, 71.45942372801900433 ) ) ;
#21237=CARTESIAN_POINT ( 'NONE',  ( -19.05341960407611168, -5.049401038298163336, 46.45724293864768129 ) ) ;
#21238=CARTESIAN_POINT ( 'NONE',  ( 4.379528057220339221, -16.55341960407611168, 107.7072429386476955 ) ) ;
#21239=CARTESIAN_POINT ( 'NONE',  ( -16.46253265017160317, 9.564922557960807481, 110.8322429386476955 ) ) ;
#21241=CARTESIAN_POINT ( 'NONE',  ( 12.06949235617757843, -12.14591786802309237, 43.12390960531435269 ) ) ;
#21242=CARTESIAN_POINT ( 'NONE',  ( 0.05219959533934541429, -16.53943276465976808, 100.0010903946857042 ) ) ;
#21243=CARTESIAN_POINT ( 'NONE',  ( 13.89961937509977652, -13.97604488694527269, 48.12390960531435979 ) ) ;
#21244=CARTESIAN_POINT ( 'NONE',  ( -0.05219959533909027116, -19.03943276465977164, 27.49890960531435624 ) ) ;
#21245=CARTESIAN_POINT ( 'NONE',  ( -18.67979575497193778, 10.72451020669871902, 113.3344237280190328 ) ) ;
#21246=CARTESIAN_POINT ( 'NONE',  ( -17.40861289039002813, -6.110651285853283099, 41.37232470827433417 ) ) ;
#21247=CARTESIAN_POINT ( 'NONE',  ( 12.06949235617757843, -12.14591786802309237, 43.12390960531435269 ) ) ;
#21248=CARTESIAN_POINT ( 'NONE',  ( -21.55341960407619339, 5.719274019375674811, 48.54275706135234714 ) ) ;
#21250=CARTESIAN_POINT ( 'NONE',  ( -16.52544592524335698, -4.483927247898792601, 53.95942372801900433 ) ) ;
#21251=CARTESIAN_POINT ( 'NONE',  ( -4.379528057220328563, 16.55341960407611168, 30.20724293864769550 ) ) ;
#21252=CARTESIAN_POINT ( 'NONE',  ( 14.29746914071037800, 8.314922557961029526, 101.6677570613523613 ) ) ;
#21253=CARTESIAN_POINT ( 'NONE',  ( -8.314922557961024197, 14.29746914071037800, 27.91775706135234358 ) ) ;
#21254=CARTESIAN_POINT ( 'NONE',  ( 16.51473224551069308, 9.474510206698969483, 54.16557627198103120 ) ) ;
#21255=CARTESIAN_POINT ( 'NONE',  ( 12.14591786802309770, 12.06949235617756955, 109.3739096053143811 ) ) ;
#21256=CARTESIAN_POINT ( 'NONE',  ( 18.67979575497194134, -10.72451020669871369, 25.83442372801901499 ) ) ;
#21257=CARTESIAN_POINT ( 'NONE',  ( -16.46253265017160317, 9.564922557960807481, 40.83224293864769550 ) ) ;
#21258=CARTESIAN_POINT ( 'NONE',  ( 13.89961937509977652, -13.97604488694527269, 113.1239096053143527 ) ) ;
#21259=CARTESIAN_POINT ( 'NONE',  ( -13.97604488694527625, -13.89961937509977652, 31.87390960531435979 ) ) ;
#21260=CARTESIAN_POINT ( 'NONE',  ( 5.153800228976335163, 19.02544592524342804, 114.7905762719810241 ) ) ;
#21261=CARTESIAN_POINT ( 'NONE',  ( -16.79531203550646978, -7.028104445595714900, 36.25244988220443787 ) ) ;
#21262=CARTESIAN_POINT ( 'NONE',  ( 16.51473224551069308, 9.474510206698969483, 104.1655762719810241 ) ) ;
#21263=CARTESIAN_POINT ( 'NONE',  ( -18.62759615963255300, -10.81492255796106328, 49.16775706135234003 ) ) ;
#21264=CARTESIAN_POINT ( 'NONE',  ( -14.29746914071049879, 8.314922557960819915, 110.8322429386476955 ) ) ;
#21265=CARTESIAN_POINT ( 'NONE',  ( -16.51473224551069308, -9.474510206698971260, 111.6655762719810383 ) ) ;
#21266=CARTESIAN_POINT ( 'NONE',  ( -8.314922557961024197, 14.29746914071037800, 77.91775706135231871 ) ) ;
#21267=CARTESIAN_POINT ( 'NONE',  ( -18.67979575497193778, 10.72451020669871902, 93.33442372801901854 ) ) ;
#21268=CARTESIAN_POINT ( 'NONE',  ( -16.55341960407617563, 4.379528057220093196, 58.54275706135235424 ) ) ;
#21269=CARTESIAN_POINT ( 'NONE',  ( -13.97604488694527625, -13.89961937509977652, 96.87390960531433848 ) ) ;
#21270=CARTESIAN_POINT ( 'NONE',  ( 4.379528057220092307, 16.55341960407617563, 42.29275706135235424 ) ) ;
#21271=CARTESIAN_POINT ( 'NONE',  ( 12.14591786802327356, -12.06949235617739191, 20.62609039468568639 ) ) ;
#21272=CARTESIAN_POINT ( 'NONE',  ( -14.34966873604972548, 8.224510206698743886, 78.33442372801901854 ) ) ;
#21273=CARTESIAN_POINT ( 'NONE',  ( -0.05219959533936034679, 19.03943276465977164, 102.5010903946856757 ) ) ;
#21274=CARTESIAN_POINT ( 'NONE',  ( -9.474510206698964154, 16.51473224551069663, 80.41557627198103830 ) ) ;
#21275=CARTESIAN_POINT ( 'NONE',  ( -0.05219959533907301413, -21.53943276465977519, 92.49890960531436690 ) ) ;
#21276=CARTESIAN_POINT ( 'NONE',  ( 12.14591786802309770, 12.06949235617756955, 99.37390960531436690 ) ) ;
#21277=CARTESIAN_POINT ( 'NONE',  ( -9.564922557961040184, 16.46253265017147172, 97.91775706135233293 ) ) ;
#21278=CARTESIAN_POINT ( 'NONE',  ( -16.55341960407617563, 4.379528057220093196, 78.54275706135236135 ) ) ;
#21280=CARTESIAN_POINT ( 'NONE',  ( 5.153800228976615827, -19.02544592524334988, 75.20942372801896170 ) ) ;
#21281=CARTESIAN_POINT ( 'NONE',  ( 14.34966873604960469, 8.224510206698951720, 49.16557627198102409 ) ) ;
#21282=CARTESIAN_POINT ( 'NONE',  ( 16.55341960407611168, 4.379528057220329451, 93.95724293864770971 ) ) ;
#21283=CARTESIAN_POINT ( 'NONE',  ( 5.049401038297881783, 19.05341960407617563, 37.29275706135232582 ) ) ;
#21284=CARTESIAN_POINT ( 'NONE',  ( -16.29526858892876007, 7.335722546920116827, 89.20329402199797642 ) ) ;
#21285=CARTESIAN_POINT ( 'NONE',  ( 5.823673210054444382, -21.52544592524334988, 35.20942372801901854 ) ) ;
#21286=CARTESIAN_POINT ( 'NONE',  ( -13.97604488694547697, 13.89961937509957934, 98.12609039468566152 ) ) ;
#21287=CARTESIAN_POINT ( 'NONE',  ( -19.02544592524342804, 5.153800228976336051, 111.0405762719810099 ) ) ;
#21288=CARTESIAN_POINT ( 'NONE',  ( 5.153800228976335163, 19.02544592524342804, 89.79057627198102409 ) ) ;
#21289=CARTESIAN_POINT ( 'NONE',  ( -10.81492255796105439, 18.62759615963255655, 107.9177570613523471 ) ) ;
#21290=CARTESIAN_POINT ( 'NONE',  ( -9.474510206698964154, 16.51473224551069663, 85.41557627198102409 ) ) ;
#21291=CARTESIAN_POINT ( 'NONE',  ( 15.72974639402199770, -15.80617190586745480, 38.12390960531436690 ) ) ;
#21292=CARTESIAN_POINT ( 'NONE',  ( 4.483927247898545687, 16.52544592524342804, 99.79057627198103830 ) ) ;
#21293=CARTESIAN_POINT ( 'NONE',  ( -5.153800228976328057, -19.02544592524343514, 62.29057627198100988 ) ) ;
#21294=CARTESIAN_POINT ( 'NONE',  ( -16.52544592524342804, 4.483927247898546575, 106.0405762719810525 ) ) ;
#21295=CARTESIAN_POINT ( 'NONE',  ( -21.52544592524334988, -5.823673210054445271, 23.95942372801901143 ) ) ;
#21296=CARTESIAN_POINT ( 'NONE',  ( 21.52544592524334988, 5.823673210054432836, 71.45942372801901854 ) ) ;
#21297=CARTESIAN_POINT ( 'NONE',  ( 16.51473224551069308, 9.474510206698969483, 49.16557627198102409 ) ) ;
#21299=CARTESIAN_POINT ( 'NONE',  ( 8.314922557961029526, -14.29746914071037800, 80.41775706135234714 ) ) ;
#21300=CARTESIAN_POINT ( 'NONE',  ( -15.80617190586768217, 15.72974639402176855, 23.12609039468567573 ) ) ;
#21301=ORIENTED_EDGE ( 'NONE', *, *, #100282, .T. ) ;
#21302=CARTESIAN_POINT ( 'NONE',  ( -0.05219959533937732626, 21.53943276465977519, 27.50109039468567929 ) ) ;
#21303=CARTESIAN_POINT ( 'NONE',  ( 5.153800228976615827, -19.02544592524334988, 50.20942372801897591 ) ) ;
#21304=CARTESIAN_POINT ( 'NONE',  ( 16.51473224551069308, 9.474510206698969483, 64.16557627198102409 ) ) ;
#21305=CARTESIAN_POINT ( 'NONE',  ( 0.05219959533936267826, -19.03943276465977164, 30.00109039468566863 ) ) ;
#21306=CARTESIAN_POINT ( 'NONE',  ( 10.72451020669871369, 18.67979575497193778, 77.08442372801901854 ) ) ;
#21307=CARTESIAN_POINT ( 'NONE',  ( -0.05219959533907301413, -21.53943276465977519, 72.49890960531435269 ) ) ;
#21308=CARTESIAN_POINT ( 'NONE',  ( -0.05219959533910754901, -16.53943276465976808, 47.49890960531435979 ) ) ;
#21309=CARTESIAN_POINT ( 'NONE',  ( -18.62759615963255300, -10.81492255796106328, 89.16775706135236135 ) ) ;
#21310=CARTESIAN_POINT ( 'NONE',  ( -9.564922557961040184, 16.46253265017147172, 32.91775706135233293 ) ) ;
#21311=CARTESIAN_POINT ( 'NONE',  ( -8.314922557960811034, -14.29746914071050412, 72.08224293864769550 ) ) ;
#21312=CARTESIAN_POINT ( 'NONE',  ( -16.52544592524342804, 4.483927247898546575, 116.0405762719810383 ) ) ;
#21313=CARTESIAN_POINT ( 'NONE',  ( -5.153800228976607833, 19.02544592524334988, 52.70942372801900433 ) ) ;
#21314=CARTESIAN_POINT ( 'NONE',  ( -14.34966873604960291, -8.224510206698953496, 21.66557627198102409 ) ) ;
#21315=CARTESIAN_POINT ( 'NONE',  ( -10.81492255796105439, 18.62759615963255655, 77.91775706135231871 ) ) ;
#21316=CARTESIAN_POINT ( 'NONE',  ( 9.474510206698971260, -16.51473224551069308, 82.91557627198103830 ) ) ;
#21317=CARTESIAN_POINT ( 'NONE',  ( 19.05341960407617918, -5.049401038297876454, 51.04275706135231871 ) ) ;
#21318=CARTESIAN_POINT ( 'NONE',  ( -18.67979575497178146, -10.72451020669898902, 51.66557627198102409 ) ) ;
#21319=CARTESIAN_POINT ( 'NONE',  ( -18.67979575497193778, 10.72451020669871902, 43.33442372801901143 ) ) ;
#21320=CARTESIAN_POINT ( 'NONE',  ( -15.80617190586745835, -15.72974639402198527, 106.8739096053143811 ) ) ;
#21321=CARTESIAN_POINT ( 'NONE',  ( -16.46253265017146816, -9.564922557961047289, 94.16775706135233293 ) ) ;
#21322=CARTESIAN_POINT ( 'NONE',  ( 4.483927247898790824, -16.52544592524335698, 60.20942372801902565 ) ) ;
#21324=CARTESIAN_POINT ( 'NONE',  ( 18.67979575497178502, 10.72451020669898547, 109.1655762719810383 ) ) ;
#21325=CARTESIAN_POINT ( 'NONE',  ( -16.55341960407611168, -4.379528057220339221, 91.45724293864769550 ) ) ;
#21327=CARTESIAN_POINT ( 'NONE',  ( 14.34966873604972726, -8.224510206698740333, 40.83442372801901854 ) ) ;
#21328=CARTESIAN_POINT ( 'NONE',  ( -10.81492255796078084, -18.62759615963271287, 47.08224293864770260 ) ) ;
#21329=CARTESIAN_POINT ( 'NONE',  ( 8.224510206698742110, 14.34966873604972548, 87.08442372801901854 ) ) ;
#21330=CARTESIAN_POINT ( 'NONE',  ( -5.153800228976328057, -19.02544592524343514, 32.29057627198102409 ) ) ;
#21331=CARTESIAN_POINT ( 'NONE',  ( 4.483927247898790824, -16.52544592524335698, 60.20942372801902565 ) ) ;
#21332=CARTESIAN_POINT ( 'NONE',  ( -21.52544592524334988, -5.823673210054445271, 38.95942372801901854 ) ) ;
#21333=CARTESIAN_POINT ( 'NONE',  ( -5.823673210054116645, -21.52544592524344225, 52.29057627198102409 ) ) ;
#21334=CARTESIAN_POINT ( 'NONE',  ( 12.06949235617739724, 12.14591786802326823, 86.87609039468568994 ) ) ;
#21335=CARTESIAN_POINT ( 'NONE',  ( 5.823673210054444382, -21.52544592524334988, 70.20942372801904696 ) ) ;
#21336=CARTESIAN_POINT ( 'NONE',  ( 21.52544592524344225, -5.823673210054117533, 53.54057627198103120 ) ) ;
#21337=CARTESIAN_POINT ( 'NONE',  ( 5.823673210054125526, 21.52544592524343514, 39.79057627198103830 ) ) ;
#21338=VERTEX_POINT ( 'NONE', #47563 ) ;
#21339=CARTESIAN_POINT ( 'NONE',  ( 8.224510206698742110, 14.34966873604972548, 62.08442372801901143 ) ) ;
#21340=CARTESIAN_POINT ( 'NONE',  ( 15.72974639402199770, -15.80617190586745480, 38.12390960531436690 ) ) ;
#21341=EDGE_LOOP ( 'NONE', ( #181036, #99429, #128568, #179130 ) ) ;
#21342=CARTESIAN_POINT ( 'NONE',  ( -9.474510206698964154, 16.51473224551069663, 95.41557627198102409 ) ) ;
#21343=CARTESIAN_POINT ( 'NONE',  ( -16.55341960407611168, -4.379528057220339221, 21.45724293864769550 ) ) ;
#21344=CARTESIAN_POINT ( 'NONE',  ( 17.50000000000000000, -5.499999999999992895, 38.29690382534171533 ) ) ;
#21345=CARTESIAN_POINT ( 'NONE',  ( 14.29746914071049879, -8.314922557960816363, 113.3322429386476955 ) ) ;
#21346=CARTESIAN_POINT ( 'NONE',  ( 21.55341960407610458, 5.719274019375980345, 63.95724293864770260 ) ) ;
#21347=CARTESIAN_POINT ( 'NONE',  ( 9.564922557960805705, 16.46253265017160317, 39.58224293864768839 ) ) ;
#21348=CARTESIAN_POINT ( 'NONE',  ( 14.29746914071037800, 8.314922557961029526, 91.66775706135234714 ) ) ;
#21349=CARTESIAN_POINT ( 'NONE',  ( 18.67979575497194134, -10.72451020669871369, 30.83442372801902209 ) ) ;
#21350=CARTESIAN_POINT ( 'NONE',  ( -9.564922557961040184, 16.46253265017147172, 87.91775706135233293 ) ) ;
#21351=CARTESIAN_POINT ( 'NONE',  ( 4.483927247898545687, 16.52544592524342804, 104.7905762719810241 ) ) ;
#21352=CARTESIAN_POINT ( 'NONE',  ( 5.049401038298161559, -19.05341960407611168, 47.70724293864770260 ) ) ;
#21354=CARTESIAN_POINT ( 'NONE',  ( -19.05341960407611168, -5.049401038298163336, 21.45724293864768839 ) ) ;
#21356=CARTESIAN_POINT ( 'NONE',  ( -9.564922557960796823, -16.46253265017161027, 77.08224293864769550 ) ) ;
#21357=CARTESIAN_POINT ( 'NONE',  ( 16.55341960407618274, -4.379528057220086978, 56.04275706135235424 ) ) ;
#21358=CARTESIAN_POINT ( 'NONE',  ( -10.81492255796105439, 18.62759615963255655, 107.9177570613523471 ) ) ;
#21359=CARTESIAN_POINT ( 'NONE',  ( -15.72974639402197994, 15.80617190586746368, 45.62390960531436690 ) ) ;
#21360=CARTESIAN_POINT ( 'NONE',  ( 14.34966873604972726, -8.224510206698740333, 70.83442372801901854 ) ) ;
#21361=CARTESIAN_POINT ( 'NONE',  ( -16.51473224551082808, 9.474510206698731452, 68.33442372801900433 ) ) ;
#21362=CARTESIAN_POINT ( 'NONE',  ( 21.53943276465977519, 0.05219959533937863772, 61.25109039468567573 ) ) ;
#21363=CARTESIAN_POINT ( 'NONE',  ( 9.564922557960805705, 16.46253265017160317, 74.58224293864769550 ) ) ;
#21364=CARTESIAN_POINT ( 'NONE',  ( 5.153800228976335163, 19.02544592524342804, 34.79057627198102409 ) ) ;
#21365=CARTESIAN_POINT ( 'NONE',  ( 13.89961937509957401, 13.97604488694547697, 61.87609039468566863 ) ) ;
#21367=CARTESIAN_POINT ( 'NONE',  ( -5.049401038298153566, 19.05341960407611168, 90.20724293864766707 ) ) ;
#21368=CARTESIAN_POINT ( 'NONE',  ( 4.483927247898545687, 16.52544592524342804, 49.79057627198102409 ) ) ;
#21369=CARTESIAN_POINT ( 'NONE',  ( -5.719274019375978568, 21.55341960407610458, 50.20724293864769550 ) ) ;
#21370=CARTESIAN_POINT ( 'NONE',  ( -17.50000000000001776, 4.049696124445901546, 104.1803967066594794 ) ) ;
#21371=CARTESIAN_POINT ( 'NONE',  ( -5.049401038297874678, -19.05341960407617918, 29.79275706135232227 ) ) ;
#21373=CARTESIAN_POINT ( 'NONE',  ( 19.03943276465977164, -0.05219959533909143690, 53.74890960531436690 ) ) ;
#21374=CARTESIAN_POINT ( 'NONE',  ( -0.05219959533934338120, 16.53943276465976808, 32.50109039468568284 ) ) ;
#21376=CARTESIAN_POINT ( 'NONE',  ( 14.34966873604972726, -8.224510206698740333, 75.83442372801900433 ) ) ;
#21377=CARTESIAN_POINT ( 'NONE',  ( 0.05219959533907565091, 21.53943276465977519, 94.99890960531436690 ) ) ;
#21378=CARTESIAN_POINT ( 'NONE',  ( -5.049401038298153566, 19.05341960407611168, 45.20724293864769550 ) ) ;
#21380=CARTESIAN_POINT ( 'NONE',  ( 15.80617190586769283, -15.72974639402175789, 45.62609039468567573 ) ) ;
#21381=CARTESIAN_POINT ( 'NONE',  ( 16.51473224551083163, -9.474510206698727899, 45.83442372801900433 ) ) ;
#21382=CARTESIAN_POINT ( 'NONE',  ( 5.049401038298161559, -19.05341960407611168, 52.70724293864767418 ) ) ;
#21383=CARTESIAN_POINT ( 'NONE',  ( 15.72974639402176855, 15.80617190586768217, 96.87609039468568994 ) ) ;
#21385=CARTESIAN_POINT ( 'NONE',  ( 16.79531203550648044, 7.028104445595620753, 98.75244988220443076 ) ) ;
#21386=CARTESIAN_POINT ( 'NONE',  ( 14.29746914071049879, -8.314922557960816363, 38.33224293864768839 ) ) ;
#21388=CARTESIAN_POINT ( 'NONE',  ( 21.53943276465977519, -0.05219959533907433946, 48.74890960531435979 ) ) ;
#21390=CARTESIAN_POINT ( 'NONE',  ( -13.97604488694527625, -13.89961937509977652, 96.87390960531433848 ) ) ;
#21391=CARTESIAN_POINT ( 'NONE',  ( 16.53943276465976808, -0.05219959533910856209, 98.74890960531438111 ) ) ;
#21392=CARTESIAN_POINT ( 'NONE',  ( -4.379528057220086978, -16.55341960407618274, 24.79275706135235779 ) ) ;
#21393=CARTESIAN_POINT ( 'NONE',  ( -8.224510206698735004, -14.34966873604973081, 104.5844237280190185 ) ) ;
#21396=CARTESIAN_POINT ( 'NONE',  ( 9.564922557960805705, 16.46253265017160317, 104.5822429386476955 ) ) ;
#21397=CARTESIAN_POINT ( 'NONE',  ( 5.719274019375991003, -21.55341960407610458, 107.7072429386476955 ) ) ;
#21398=CARTESIAN_POINT ( 'NONE',  ( -12.14591786802309592, -12.06949235617757132, 21.87390960531436690 ) ) ;
#21399=CARTESIAN_POINT ( 'NONE',  ( 19.03943276465977164, -0.05219959533909143690, 98.74890960531436690 ) ) ;
#21400=CARTESIAN_POINT ( 'NONE',  ( 19.03943276465977164, 0.05219959533936151252, 91.25109039468566152 ) ) ;
#21401=CARTESIAN_POINT ( 'NONE',  ( -5.049401038297874678, -19.05341960407617918, 19.79275706135233293 ) ) ;
#21402=CARTESIAN_POINT ( 'NONE',  ( 10.81492255796078972, 18.62759615963270932, 89.58224293864768129 ) ) ;
#21403=CARTESIAN_POINT ( 'NONE',  ( -0.05219959533907301413, -21.53943276465977519, 57.49890960531435979 ) ) ;
#21404=CARTESIAN_POINT ( 'NONE',  ( -16.51473224551069308, -9.474510206698971260, 66.66557627198102409 ) ) ;
#21405=CARTESIAN_POINT ( 'NONE',  ( 14.34966873604960469, 8.224510206698951720, 29.16557627198103120 ) ) ;
#21406=CARTESIAN_POINT ( 'NONE',  ( 0.05219959533909260263, 19.03943276465977164, 74.99890960531435269 ) ) ;
#21408=CARTESIAN_POINT ( 'NONE',  ( 19.36337904590688552, -5.500000000000142997, 62.91494137495619299 ) ) ;
#21409=CARTESIAN_POINT ( 'NONE',  ( 5.049401038297881783, 19.05341960407617563, 37.29275706135232582 ) ) ;
#21410=CARTESIAN_POINT ( 'NONE',  ( 21.53943276465977519, -0.05219959533907433946, 78.74890960531436690 ) ) ;
#21411=CARTESIAN_POINT ( 'NONE',  ( -16.53943276465976808, 0.05219959533911058130, 81.24890960531436690 ) ) ;
#21412=CARTESIAN_POINT ( 'NONE',  ( -15.72974639402176322, -15.80617190586768395, 34.37609039468568284 ) ) ;
#21414=CARTESIAN_POINT ( 'NONE',  ( -14.34966873604972548, 8.224510206698743886, 113.3344237280190328 ) ) ;
#21415=CARTESIAN_POINT ( 'NONE',  ( 5.049401038298161559, -19.05341960407611168, 27.70724293864769550 ) ) ;
#21416=CARTESIAN_POINT ( 'NONE',  ( 19.05341960407611168, 5.049401038298154454, 83.95724293864766707 ) ) ;
#21417=CARTESIAN_POINT ( 'NONE',  ( 12.14591786802309770, 12.06949235617756955, 39.37390960531436690 ) ) ;
#21418=CARTESIAN_POINT ( 'NONE',  ( -21.53943276465977519, -0.05219959533937600094, 63.75109039468568284 ) ) ;
#21420=CARTESIAN_POINT ( 'NONE',  ( 0.05219959533909260263, 19.03943276465977164, 44.99890960531435979 ) ) ;
#21421=CARTESIAN_POINT ( 'NONE',  ( 5.049401038298161559, -19.05341960407611168, 57.70724293864769550 ) ) ;
#21422=ORIENTED_EDGE ( 'NONE', *, *, #98443, .T. ) ;
#21423=CARTESIAN_POINT ( 'NONE',  ( 10.72451020669871369, 18.67979575497193778, 112.0844237280190185 ) ) ;
#21424=CARTESIAN_POINT ( 'NONE',  ( 8.314922557961029526, -14.29746914071037800, 60.41775706135235424 ) ) ;
#21425=CARTESIAN_POINT ( 'NONE',  ( -10.72451020669870658, -18.67979575497194134, 89.58442372801901854 ) ) ;
#21426=CARTESIAN_POINT ( 'NONE',  ( -16.46253265017160317, 9.564922557960807481, 110.8322429386476955 ) ) ;
#21427=CARTESIAN_POINT ( 'NONE',  ( -13.89961937509957401, -13.97604488694547875, 99.37609039468567573 ) ) ;
#21428=CARTESIAN_POINT ( 'NONE',  ( 21.55341960407619695, -5.719274019375665929, 71.04275706135234714 ) ) ;
#21429=CARTESIAN_POINT ( 'NONE',  ( -4.379528057220086978, -16.55341960407618274, 29.79275706135234358 ) ) ;
#21430=CARTESIAN_POINT ( 'NONE',  ( 18.62759615963271287, -10.81492255796078972, 83.33224293864769550 ) ) ;
#21431=CARTESIAN_POINT ( 'NONE',  ( -5.153800228976607833, 19.02544592524334988, 92.70942372801901854 ) ) ;
#21432=CARTESIAN_POINT ( 'NONE',  ( -9.474510206698964154, 16.51473224551069663, 60.41557627198102409 ) ) ;
#21433=CARTESIAN_POINT ( 'NONE',  ( -16.52544592524335698, -4.483927247898792601, 18.95942372801901143 ) ) ;
#21434=CARTESIAN_POINT ( 'NONE',  ( -13.89961937509957401, -13.97604488694547875, 99.37609039468567573 ) ) ;
#21435=CARTESIAN_POINT ( 'NONE',  ( 4.483927247898545687, 16.52544592524342804, 54.79057627198104541 ) ) ;
#21436=CARTESIAN_POINT ( 'NONE',  ( -19.03943276465977164, -0.05219959533935918106, 83.75109039468567573 ) ) ;
#21438=CARTESIAN_POINT ( 'NONE',  ( -4.379528057220086978, -16.55341960407618274, 59.79275706135234714 ) ) ;
#21439=CARTESIAN_POINT ( 'NONE',  ( -15.72974639402197994, 15.80617190586746368, 110.6239096053143669 ) ) ;
#21440=CARTESIAN_POINT ( 'NONE',  ( -19.03943276465977164, 0.05219959533909376836, 36.24890960531436690 ) ) ;
#21441=CARTESIAN_POINT ( 'NONE',  ( -5.049401038298153566, 19.05341960407611168, 50.20724293864770260 ) ) ;
#21442=CARTESIAN_POINT ( 'NONE',  ( -4.379528057220086978, -16.55341960407618274, 54.79275706135235424 ) ) ;
#21445=CARTESIAN_POINT ( 'NONE',  ( -16.51473224551069308, -9.474510206698971260, 106.6655762719810383 ) ) ;
#21446=DIRECTION ( 'NONE',  ( -6.948002486793210646E-15, 0.9991276842514723588, -0.04175967627138119781 ) ) ;
#21448=CARTESIAN_POINT ( 'NONE',  ( 12.14591786802327356, -12.06949235617739191, 20.62609039468568639 ) ) ;
#21449=CARTESIAN_POINT ( 'NONE',  ( 18.62759615963271287, -10.81492255796078972, 43.33224293864769550 ) ) ;
#21450=CARTESIAN_POINT ( 'NONE',  ( -19.02544592524334988, -5.153800228976617603, 43.95942372801899012 ) ) ;
#21451=CARTESIAN_POINT ( 'NONE',  ( -14.34966873604972548, 8.224510206698743886, 33.33442372801900433 ) ) ;
#21452=CARTESIAN_POINT ( 'NONE',  ( -9.474510206698964154, 16.51473224551069663, 25.41557627198103120 ) ) ;
#21453=CARTESIAN_POINT ( 'NONE',  ( 5.153800228976335163, 19.02544592524342804, 49.79057627198100988 ) ) ;
#21454=CARTESIAN_POINT ( 'NONE',  ( 21.53943276465977519, -0.05219959533907433946, 83.74890960531435269 ) ) ;
#21455=CARTESIAN_POINT ( 'NONE',  ( -13.97604488694527625, -13.89961937509977652, 111.8739096053143243 ) ) ;
#21456=CARTESIAN_POINT ( 'NONE',  ( 0.05219959533909260263, 19.03943276465977164, 49.99890960531435979 ) ) ;
#21458=CARTESIAN_POINT ( 'NONE',  ( 16.51473224551083163, -9.474510206698727899, 90.83442372801900433 ) ) ;
#21459=CARTESIAN_POINT ( 'NONE',  ( 8.224510206698953496, -14.34966873604960469, 62.91557627198102409 ) ) ;
#21460=CARTESIAN_POINT ( 'NONE',  ( 0.05219959533937995610, -21.53943276465977519, 105.0010903946856757 ) ) ;
#21461=CARTESIAN_POINT ( 'NONE',  ( -5.719274019375978568, 21.55341960407610458, 100.2072429386476955 ) ) ;
#21462=CARTESIAN_POINT ( 'NONE',  ( 21.52544592524334988, 5.823673210054432836, 91.45942372801901854 ) ) ;
#21463=CARTESIAN_POINT ( 'NONE',  ( 18.67979575497194134, -10.72451020669871369, 75.83442372801900433 ) ) ;
#21464=CARTESIAN_POINT ( 'NONE',  ( 13.89961937509977652, -13.97604488694527269, 113.1239096053143527 ) ) ;
#21465=CARTESIAN_POINT ( 'NONE',  ( -4.379528057220086978, -16.55341960407618274, 99.79275706135234714 ) ) ;
#21466=CARTESIAN_POINT ( 'NONE',  ( -0.05219959533937732626, 21.53943276465977519, 77.50109039468567573 ) ) ;
#21467=CARTESIAN_POINT ( 'NONE',  ( -13.97604488694527625, -13.89961937509977652, 61.87390960531435979 ) ) ;
#21469=CARTESIAN_POINT ( 'NONE',  ( 15.80617190586769283, -15.72974639402175789, 40.62609039468567573 ) ) ;
#21470=CARTESIAN_POINT ( 'NONE',  ( -9.474510206698964154, 16.51473224551069663, 80.41557627198103830 ) ) ;
#21471=CARTESIAN_POINT ( 'NONE',  ( -8.314922557960811034, -14.29746914071050412, 82.08224293864768129 ) ) ;
#21472=CARTESIAN_POINT ( 'NONE',  ( 0.05219959533910956823, 16.53943276465976808, 54.99890960531435269 ) ) ;
#21473=CARTESIAN_POINT ( 'NONE',  ( 5.823673210054125526, 21.52544592524343514, 64.79057627198103830 ) ) ;
#21474=CARTESIAN_POINT ( 'NONE',  ( 0.05219959533909260263, 19.03943276465977164, 64.99890960531436690 ) ) ;
#21475=CARTESIAN_POINT ( 'NONE',  ( 5.719274019375991003, -21.55341960407610458, 72.70724293864769550 ) ) ;
#21476=CARTESIAN_POINT ( 'NONE',  ( 5.049401038297881783, 19.05341960407617563, 62.29275706135234003 ) ) ;
#21478=CARTESIAN_POINT ( 'NONE',  ( 19.03943276465977164, 0.05219959533936151252, 36.25109039468567573 ) ) ;
#21479=CARTESIAN_POINT ( 'NONE',  ( -12.06949235617756955, 12.14591786802309770, 80.62390960531438111 ) ) ;
#21480=CARTESIAN_POINT ( 'NONE',  ( 10.81492255796078972, 18.62759615963270932, 54.58224293864769550 ) ) ;
#21481=CARTESIAN_POINT ( 'NONE',  ( 17.50000000000000000, -5.499999999999992895, 96.21769037696437010 ) ) ;
#21482=CARTESIAN_POINT ( 'NONE',  ( -14.34966873604972548, 8.224510206698743886, 98.33442372801901854 ) ) ;
#21484=CARTESIAN_POINT ( 'NONE',  ( 5.153800228976615827, -19.02544592524334988, 100.2094237280190043 ) ) ;
#21486=CARTESIAN_POINT ( 'NONE',  ( -16.55341960407611168, -4.379528057220339221, 66.45724293864768129 ) ) ;
#21488=CARTESIAN_POINT ( 'NONE',  ( 19.03943276465977164, -0.05219959533909143690, 63.74890960531435979 ) ) ;
#21489=CARTESIAN_POINT ( 'NONE',  ( 0.05219959533910956823, 16.53943276465976808, 49.99890960531437401 ) ) ;
#21490=CARTESIAN_POINT ( 'NONE',  ( -19.05341960407611168, -5.049401038298163336, 91.45724293864766707 ) ) ;
#21491=CARTESIAN_POINT ( 'NONE',  ( 16.46253265017146816, 9.564922557961045513, 81.66775706135233293 ) ) ;
#21492=CARTESIAN_POINT ( 'NONE',  ( -19.05341960407611168, -5.049401038298163336, 71.45724293864766707 ) ) ;
#21493=CARTESIAN_POINT ( 'NONE',  ( 19.05341960407611168, 5.049401038298154454, 83.95724293864766707 ) ) ;
#21494=CARTESIAN_POINT ( 'NONE',  ( 19.03943276465977164, -0.05219959533909143690, 68.74890960531436690 ) ) ;
#21495=CARTESIAN_POINT ( 'NONE',  ( 15.80617190586746368, 15.72974639402197994, 69.37390960531436690 ) ) ;
#21496=CARTESIAN_POINT ( 'NONE',  ( -16.52544592524335698, -4.483927247898792601, 58.95942372801902565 ) ) ;
#21498=CARTESIAN_POINT ( 'NONE',  ( -0.05219959533909027116, -19.03943276465977164, 52.49890960531436690 ) ) ;
#21499=CARTESIAN_POINT ( 'NONE',  ( 5.823673210054125526, 21.52544592524343514, 59.79057627198103120 ) ) ;
#21500=CARTESIAN_POINT ( 'NONE',  ( -0.05219959533936034679, 19.03943276465977164, 87.50109039468567573 ) ) ;
#21501=CARTESIAN_POINT ( 'NONE',  ( -12.14591786802309592, -12.06949235617757132, 21.87390960531436690 ) ) ;
#21502=CARTESIAN_POINT ( 'NONE',  ( -16.51473224551082808, 9.474510206698731452, 43.33442372801900433 ) ) ;
#21503=CARTESIAN_POINT ( 'NONE',  ( -4.379528057220086978, -16.55341960407618274, 64.79275706135234714 ) ) ;
#21504=CARTESIAN_POINT ( 'NONE',  ( -14.34966873604972548, 8.224510206698743886, 93.33442372801901854 ) ) ;
#21505=CARTESIAN_POINT ( 'NONE',  ( 19.02130022317639657, -5.499999999999599432, 43.28188669246573994 ) ) ;
#21506=CARTESIAN_POINT ( 'NONE',  ( 12.06949235617739724, 12.14591786802326823, 86.87609039468568994 ) ) ;
#21507=CARTESIAN_POINT ( 'NONE',  ( 5.719274019375991003, -21.55341960407610458, 27.70724293864769905 ) ) ;
#21508=CARTESIAN_POINT ( 'NONE',  ( 16.52544592524335698, 4.483927247898782831, 36.45942372801901143 ) ) ;
#21509=CARTESIAN_POINT ( 'NONE',  ( 13.89961937509977652, -13.97604488694527269, 43.12390960531434558 ) ) ;
#21510=CARTESIAN_POINT ( 'NONE',  ( 19.03943276465977164, -0.05219959533909143690, 53.74890960531436690 ) ) ;
#21511=CARTESIAN_POINT ( 'NONE',  ( 13.89961937509977652, -13.97604488694527269, 43.12390960531434558 ) ) ;
#21512=CARTESIAN_POINT ( 'NONE',  ( -18.67979575497193778, 10.72451020669871902, 38.33442372801900433 ) ) ;
#21513=CARTESIAN_POINT ( 'NONE',  ( -16.53943276465976808, -0.05219959533934237506, 53.75109039468568994 ) ) ;
#21514=CARTESIAN_POINT ( 'NONE',  ( 8.314922557960818139, 14.29746914071049879, 24.58224293864768839 ) ) ;
#21515=CARTESIAN_POINT ( 'NONE',  ( 9.474510206698971260, -16.51473224551069308, 32.91557627198102409 ) ) ;
#21516=CARTESIAN_POINT ( 'NONE',  ( -16.46253265017146816, -9.564922557961047289, 24.16775706135233648 ) ) ;
#21517=CARTESIAN_POINT ( 'NONE',  ( -12.06949235617739369, -12.14591786802326823, 19.37609039468568639 ) ) ;
#21518=CARTESIAN_POINT ( 'NONE',  ( 19.02544592524334988, 5.153800228976608722, 66.45942372801899012 ) ) ;
#21519=CARTESIAN_POINT ( 'NONE',  ( 16.55341960407611168, 4.379528057220329451, 68.95724293864769550 ) ) ;
#21520=CARTESIAN_POINT ( 'NONE',  ( -19.05341960407611168, -5.049401038298163336, 41.45724293864769550 ) ) ;
#21521=CARTESIAN_POINT ( 'NONE',  ( -9.564922557961040184, 16.46253265017147172, 72.91775706135233293 ) ) ;
#21522=CARTESIAN_POINT ( 'NONE',  ( 16.19135201231366139, -7.376712067591919109, 92.31319145947965410 ) ) ;
#21523=CARTESIAN_POINT ( 'NONE',  ( 18.62759615963255655, 10.81492255796105972, 76.66775706135234714 ) ) ;
#21524=CARTESIAN_POINT ( 'NONE',  ( 16.55341960407618274, -4.379528057220086978, 36.04275706135234714 ) ) ;
#21526=CARTESIAN_POINT ( 'NONE',  ( 18.67979575497178502, 10.72451020669898547, 34.16557627198102409 ) ) ;
#21527=CARTESIAN_POINT ( 'NONE',  ( 0.05219959533934541429, -16.53943276465976808, 30.00109039468568284 ) ) ;
#21529=CARTESIAN_POINT ( 'NONE',  ( -0.05219959533936034679, 19.03943276465977164, 22.50109039468566152 ) ) ;
#21530=CARTESIAN_POINT ( 'NONE',  ( 17.97182807773875979, -5.499999999999868550, 66.03038844047287625 ) ) ;
#21531=CARTESIAN_POINT ( 'NONE',  ( -5.153800228976328057, -19.02544592524343514, 37.29057627198102409 ) ) ;
#21533=CARTESIAN_POINT ( 'NONE',  ( 19.02544592524343514, -5.153800228976328945, 58.54057627198102409 ) ) ;
#21534=AXIS2_PLACEMENT_3D ( 'NONE', #28893, #63171, #78331 ) ;
#21535=CARTESIAN_POINT ( 'NONE',  ( 21.53943276465977519, 0.05219959533937863772, 71.25109039468568994 ) ) ;
#21536=CARTESIAN_POINT ( 'NONE',  ( -19.03943276465977164, -0.05219959533935918106, 18.75109039468567218 ) ) ;
#21537=CARTESIAN_POINT ( 'NONE',  ( 8.314922557960818139, 14.29746914071049879, 29.58224293864769905 ) ) ;
#21538=CARTESIAN_POINT ( 'NONE',  ( -16.46253265017160317, 9.564922557960807481, 30.83224293864769550 ) ) ;
#21539=CARTESIAN_POINT ( 'NONE',  ( 16.51473224551069308, 9.474510206698969483, 89.16557627198103830 ) ) ;
#21540=CARTESIAN_POINT ( 'NONE',  ( -10.72451020669870658, -18.67979575497194134, 69.58442372801900433 ) ) ;
#21541=CARTESIAN_POINT ( 'NONE',  ( -9.474510206698964154, 16.51473224551069663, 40.41557627198103120 ) ) ;
#21542=CARTESIAN_POINT ( 'NONE',  ( -10.81492255796105439, 18.62759615963255655, 72.91775706135234714 ) ) ;
#21543=CARTESIAN_POINT ( 'NONE',  ( 19.02544592524334988, 5.153800228976608722, 96.45942372801897591 ) ) ;
#21544=CARTESIAN_POINT ( 'NONE',  ( 0.05219959533909260263, 19.03943276465977164, 99.99890960531436690 ) ) ;
#21545=CARTESIAN_POINT ( 'NONE',  ( -19.03943276465977164, 0.05219959533909376836, 41.24890960531435269 ) ) ;
#21546=CARTESIAN_POINT ( 'NONE',  ( 21.55341960407610458, 5.719274019375980345, 103.9572429386476813 ) ) ;
#21547=CARTESIAN_POINT ( 'NONE',  ( 13.97604488694548053, -13.89961937509957401, 35.62609039468567573 ) ) ;
#21548=CARTESIAN_POINT ( 'NONE',  ( 14.29746914071049879, -8.314922557960816363, 108.3322429386477097 ) ) ;
#21549=CARTESIAN_POINT ( 'NONE',  ( 19.02544592524343514, -5.153800228976328945, 68.54057627198103830 ) ) ;
#21550=CARTESIAN_POINT ( 'NONE',  ( -9.474510206698720793, -16.51473224551083518, 104.5844237280190043 ) ) ;
#21551=CARTESIAN_POINT ( 'NONE',  ( -12.06949235617756955, 12.14591786802309770, 55.62390960531436690 ) ) ;
#21552=CARTESIAN_POINT ( 'NONE',  ( 10.81492255796078972, 18.62759615963270932, 29.58224293864769905 ) ) ;
#21553=CARTESIAN_POINT ( 'NONE',  ( 19.02544592524334988, 5.153800228976608722, 81.45942372801897591 ) ) ;
#21554=CARTESIAN_POINT ( 'NONE',  ( -5.823673210054116645, -21.52544592524344225, 87.29057627198103830 ) ) ;
#21555=CARTESIAN_POINT ( 'NONE',  ( 15.72974639402176855, 15.80617190586768217, 41.87609039468568284 ) ) ;
#21556=CARTESIAN_POINT ( 'NONE',  ( 0.05219959533934541429, -16.53943276465976808, 40.00109039468567573 ) ) ;
#21557=CARTESIAN_POINT ( 'NONE',  ( -8.224510206698735004, -14.34966873604973081, 39.58442372801901143 ) ) ;
#21558=CARTESIAN_POINT ( 'NONE',  ( -10.81492255796105439, 18.62759615963255655, 47.91775706135234714 ) ) ;
#21559=CARTESIAN_POINT ( 'NONE',  ( 5.823673210054125526, 21.52544592524343514, 54.79057627198104541 ) ) ;
#21560=CARTESIAN_POINT ( 'NONE',  ( -19.02544592524342804, 5.153800228976336051, 31.04057627198102409 ) ) ;
#21562=CARTESIAN_POINT ( 'NONE',  ( 16.55341960407618274, -4.379528057220086978, 71.04275706135234714 ) ) ;
#21563=CARTESIAN_POINT ( 'NONE',  ( 21.53943276465977519, -0.05219959533907433946, 108.7489096053143669 ) ) ;
#21564=CARTESIAN_POINT ( 'NONE',  ( 12.06949235617757843, -12.14591786802309237, 38.12390960531436690 ) ) ;
#21565=CARTESIAN_POINT ( 'NONE',  ( -16.55341960407617563, 4.379528057220093196, 63.54275706135234003 ) ) ;
#21566=CARTESIAN_POINT ( 'NONE',  ( 19.02544592524334988, 5.153800228976608722, 106.4594237280190185 ) ) ;
#21567=CARTESIAN_POINT ( 'NONE',  ( 0.05219959533907565091, 21.53943276465977519, 94.99890960531436690 ) ) ;
#21568=CARTESIAN_POINT ( 'NONE',  ( -14.29746914071049879, 8.314922557960819915, 35.83224293864768839 ) ) ;
#21570=CARTESIAN_POINT ( 'NONE',  ( -14.29746914071037622, -8.314922557961029526, 79.16775706135234714 ) ) ;
#21571=CARTESIAN_POINT ( 'NONE',  ( 18.39635199886970440, -5.499999999999975131, 93.51967076360001840 ) ) ;
#21572=( BOUNDED_CURVE ( )  B_SPLINE_CURVE ( 2, ( #127101, #111950, #49291, #36093, #172634, #80605, #5754, #83586, #187822, #18960, #110949, #34122, #94787 ),
 .UNSPECIFIED., .F., .F. ) 
 B_SPLINE_CURVE_WITH_KNOTS ( ( 3, 2, 2, 2, 2, 2, 3 ),
 ( 0.7655883311638873590, 0.7675438596491228616, 0.7719298245614034659, 0.7763157894736841813, 0.7807017543859648967, 0.7850877192982456121, 0.7869975679613910868 ),
 .UNSPECIFIED. ) 
 CURVE ( )  GEOMETRIC_REPRESENTATION_ITEM ( )  RATIONAL_B_SPLINE_CURVE ( ( 0.9831626618144007068, 0.9848076720550096308, 1.000000000000000000, 0.9659258262890683122, 1.000000000000000000, 0.9659258262890683122, 1.000000000000000000, 0.9659258262890683122, 1.000000000000000000, 0.9659258262890683122, 1.000000000000000000, 0.9851625545550091179, 0.9832469066685282089 ) ) 
 REPRESENTATION_ITEM ( '' )  );
#21573=CARTESIAN_POINT ( 'NONE',  ( -0.05219959533907301413, -21.53943276465977519, 72.49890960531435269 ) ) ;
#21574=CARTESIAN_POINT ( 'NONE',  ( 12.14591786802327356, -12.06949235617739191, 105.6260903946856899 ) ) ;
#21576=CARTESIAN_POINT ( 'NONE',  ( -16.62475595723696031, -7.163666690055266351, 54.47286648189535896 ) ) ;
#21577=CARTESIAN_POINT ( 'NONE',  ( -0.05219959533907301413, -21.53943276465977519, 97.49890960531436690 ) ) ;
#21578=CARTESIAN_POINT ( 'NONE',  ( 18.67979575497178502, 10.72451020669898547, 109.1655762719810383 ) ) ;
#21579=CARTESIAN_POINT ( 'NONE',  ( 4.379528057220339221, -16.55341960407611168, 42.70724293864770260 ) ) ;
#21580=CARTESIAN_POINT ( 'NONE',  ( 4.379528057220092307, 16.55341960407617563, 42.29275706135235424 ) ) ;
#21581=CARTESIAN_POINT ( 'NONE',  ( -5.049401038298153566, 19.05341960407611168, 45.20724293864769550 ) ) ;
#21582=CARTESIAN_POINT ( 'NONE',  ( -0.05219959533909027116, -19.03943276465977164, 62.49890960531435979 ) ) ;
#21584=CARTESIAN_POINT ( 'NONE',  ( 13.89961937509977652, -13.97604488694527269, 113.1239096053143527 ) ) ;
#21585=CARTESIAN_POINT ( 'NONE',  ( -17.58332526062525858, 7.635886036038558977, 65.92334959558466778 ) ) ;
#21586=CARTESIAN_POINT ( 'NONE',  ( 0.05219959533936267826, -19.03943276465977164, 110.0010903946856757 ) ) ;
#21587=CARTESIAN_POINT ( 'NONE',  ( -9.564922557961040184, 16.46253265017147172, 47.91775706135233293 ) ) ;
#21588=CARTESIAN_POINT ( 'NONE',  ( -18.67979575497178146, -10.72451020669898902, 86.66557627198102409 ) ) ;
#21589=CARTESIAN_POINT ( 'NONE',  ( 16.55341960407611168, 4.379528057220329451, 23.95724293864769550 ) ) ;
#21590=CARTESIAN_POINT ( 'NONE',  ( 13.89961937509977652, -13.97604488694527269, 73.12390960531436690 ) ) ;
#21591=CARTESIAN_POINT ( 'NONE',  ( -18.67979575497178146, -10.72451020669898902, 46.66557627198102409 ) ) ;
#21592=CARTESIAN_POINT ( 'NONE',  ( 18.62759615963271287, -10.81492255796078972, 83.33224293864769550 ) ) ;
#21593=CARTESIAN_POINT ( 'NONE',  ( 16.53943276465976808, 0.05219959533934440121, 31.25109039468568639 ) ) ;
#21595=CARTESIAN_POINT ( 'NONE',  ( -21.53943276465977519, 0.05219959533907696930, 21.24890960531436690 ) ) ;
#21596=CARTESIAN_POINT ( 'NONE',  ( 5.719274019375673035, 21.55341960407619339, 77.29275706135234714 ) ) ;
#21597=CARTESIAN_POINT ( 'NONE',  ( -16.46253265017160317, 9.564922557960807481, 75.83224293864769550 ) ) ;
#21598=CARTESIAN_POINT ( 'NONE',  ( -19.03943276465977164, 0.05219959533909376836, 21.24890960531436335 ) ) ;
#21599=CARTESIAN_POINT ( 'NONE',  ( 9.474510206698971260, -16.51473224551069308, 72.91557627198102409 ) ) ;
#21600=CARTESIAN_POINT ( 'NONE',  ( 16.53943276465976808, -0.05219959533910856209, 93.74890960531436690 ) ) ;
#21602=CARTESIAN_POINT ( 'NONE',  ( -19.03943276465977164, -0.05219959533935918106, 108.7510903946856615 ) ) ;
#21604=CARTESIAN_POINT ( 'NONE',  ( 0.05219959533909260263, 19.03943276465977164, 79.99890960531436690 ) ) ;
#21605=CARTESIAN_POINT ( 'NONE',  ( -21.55341960407619339, 5.719274019375674811, 88.54275706135236135 ) ) ;
#21606=CARTESIAN_POINT ( 'NONE',  ( 9.474510206698971260, -16.51473224551069308, 97.91557627198102409 ) ) ;
#21607=CARTESIAN_POINT ( 'NONE',  ( -14.29746914071037622, -8.314922557961029526, 84.16775706135234714 ) ) ;
#21610=CARTESIAN_POINT ( 'NONE',  ( 16.51473224551083163, -9.474510206698727899, 60.83442372801900433 ) ) ;
#21611=CARTESIAN_POINT ( 'NONE',  ( 16.46253265017146816, 9.564922557961045513, 21.66775706135233648 ) ) ;
#21615=CARTESIAN_POINT ( 'NONE',  ( -12.14591786802326823, 12.06949235617739902, 113.1260903946856899 ) ) ;
#21616=CARTESIAN_POINT ( 'NONE',  ( -22.00000000000000000, -5.510910596163089556E-15, 45.00000000000000000 ) ) ;
#21617=CARTESIAN_POINT ( 'NONE',  ( -8.314922557961024197, 14.29746914071037800, 107.9177570613523471 ) ) ;
#21618=CARTESIAN_POINT ( 'NONE',  ( 16.18388926212237422, 7.379444403734556346, 67.93953151366154941 ) ) ;
#21619=CARTESIAN_POINT ( 'NONE',  ( -12.06949235617739369, -12.14591786802326823, 79.37609039468567573 ) ) ;
#21620=CARTESIAN_POINT ( 'NONE',  ( -21.53943276465977519, -0.05219959533937600094, 78.75109039468568994 ) ) ;
#21621=CARTESIAN_POINT ( 'NONE',  ( -19.05341960407617563, 5.049401038297882671, 108.5427570613523187 ) ) ;
#21622=CARTESIAN_POINT ( 'NONE',  ( 21.52544592524334988, 5.823673210054432836, 61.45942372801901854 ) ) ;
#21623=CARTESIAN_POINT ( 'NONE',  ( -9.474510206698720793, -16.51473224551083518, 44.58442372801900433 ) ) ;
#21624=CARTESIAN_POINT ( 'NONE',  ( 0.05219959533909260263, 19.03943276465977164, 79.99890960531436690 ) ) ;
#21625=CARTESIAN_POINT ( 'NONE',  ( 16.46253265017160672, -9.564922557960803928, 58.33224293864769550 ) ) ;
#21626=FACE_OUTER_BOUND ( 'NONE', #29794, .T. ) ;
#21627=CARTESIAN_POINT ( 'NONE',  ( -21.53943276465977519, 0.05219959533907696930, 96.24890960531435269 ) ) ;
#21629=CARTESIAN_POINT ( 'NONE',  ( 15.72974639402199770, -15.80617190586745480, 48.12390960531436690 ) ) ;
#21630=CARTESIAN_POINT ( 'NONE',  ( -9.564922557960796823, -16.46253265017161027, 52.08224293864768839 ) ) ;
#21631=CARTESIAN_POINT ( 'NONE',  ( -14.34966873604972548, 8.224510206698743886, 68.33442372801900433 ) ) ;
#21632=UNCERTAINTY_MEASURE_WITH_UNIT (LENGTH_MEASURE( 1.000000000000000082E-05 ), #176802, 'distance_accuracy_value', 'NONE');
#21635=CARTESIAN_POINT ( 'NONE',  ( -18.67979575497193778, 10.72451020669871902, 38.33442372801900433 ) ) ;
#21636=CARTESIAN_POINT ( 'NONE',  ( -4.379528057220328563, 16.55341960407611168, 60.20724293864768839 ) ) ;
#21638=CARTESIAN_POINT ( 'NONE',  ( 0.05219959533934541429, -16.53943276465976808, 45.00109039468568284 ) ) ;
#21639=CARTESIAN_POINT ( 'NONE',  ( -12.14591786802309592, -12.06949235617757132, 101.8739096053143811 ) ) ;
#21640=CARTESIAN_POINT ( 'NONE',  ( 16.46253265017146816, 9.564922557961045513, 56.66775706135233293 ) ) ;
#21642=CARTESIAN_POINT ( 'NONE',  ( -16.55341960407611168, -4.379528057220339221, 71.45724293864769550 ) ) ;
#21643=CARTESIAN_POINT ( 'NONE',  ( 18.67979575497194134, -10.72451020669871369, 25.83442372801901499 ) ) ;
#21644=CARTESIAN_POINT ( 'NONE',  ( -19.03943276465977164, 0.05219959533909376836, 21.24890960531436335 ) ) ;
#21645=CARTESIAN_POINT ( 'NONE',  ( -21.55341960407610458, -5.719274019375992779, 96.45724293864770971 ) ) ;
#21646=CARTESIAN_POINT ( 'NONE',  ( 5.049401038298161559, -19.05341960407611168, 107.7072429386476955 ) ) ;
#21647=CARTESIAN_POINT ( 'NONE',  ( -8.224510206698948167, 14.34966873604960824, 80.41557627198103830 ) ) ;
#21650=CARTESIAN_POINT ( 'NONE',  ( -13.89961937509957401, -13.97604488694547875, 84.37609039468567573 ) ) ;
#21651=CARTESIAN_POINT ( 'NONE',  ( -15.72974639402197994, 15.80617190586746368, 115.6239096053143669 ) ) ;
#21652=CARTESIAN_POINT ( 'NONE',  ( 5.049401038298161559, -19.05341960407611168, 72.70724293864768129 ) ) ;
#21653=CARTESIAN_POINT ( 'NONE',  ( -9.474510206698720793, -16.51473224551083518, 54.58442372801899722 ) ) ;
#21654=CARTESIAN_POINT ( 'NONE',  ( 16.51473224551069308, 9.474510206698969483, 34.16557627198102409 ) ) ;
#21655=CARTESIAN_POINT ( 'NONE',  ( 8.314922557960818139, 14.29746914071049879, 69.58224293864769550 ) ) ;
#21656=CARTESIAN_POINT ( 'NONE',  ( 12.06949235617757843, -12.14591786802309237, 53.12390960531436690 ) ) ;
#21657=CARTESIAN_POINT ( 'NONE',  ( -19.03943276465977164, 0.05219959533909376836, 66.24890960531436690 ) ) ;
#21658=CARTESIAN_POINT ( 'NONE',  ( 0.05219959533907565091, 21.53943276465977519, 89.99890960531438111 ) ) ;
#21659=CARTESIAN_POINT ( 'NONE',  ( 5.049401038298161559, -19.05341960407611168, 57.70724293864769550 ) ) ;
#21660=CARTESIAN_POINT ( 'NONE',  ( 21.52544592524344225, -5.823673210054117533, 78.54057627198103830 ) ) ;
#21661=CARTESIAN_POINT ( 'NONE',  ( 18.62759615963255655, 10.81492255796105972, 106.6677570613523756 ) ) ;
#21662=CARTESIAN_POINT ( 'NONE',  ( -19.05341960407611168, -5.049401038298163336, 26.45724293864769550 ) ) ;
#21663=CARTESIAN_POINT ( 'NONE',  ( -12.06949235617739369, -12.14591786802326823, 109.3760903946857042 ) ) ;
#21664=CARTESIAN_POINT ( 'NONE',  ( 4.483927247898545687, 16.52544592524342804, 94.79057627198105251 ) ) ;
#21665=CARTESIAN_POINT ( 'NONE',  ( 16.51473224551083163, -9.474510206698727899, 85.83442372801900433 ) ) ;
#21667=CARTESIAN_POINT ( 'NONE',  ( 5.823673210054125526, 21.52544592524343514, 109.7905762719810383 ) ) ;
#21668=CARTESIAN_POINT ( 'NONE',  ( 5.049401038297881783, 19.05341960407617563, 47.29275706135231161 ) ) ;
#21669=CARTESIAN_POINT ( 'NONE',  ( 14.34966873604972726, -8.224510206698740333, 105.8344237280190328 ) ) ;
#21670=CARTESIAN_POINT ( 'NONE',  ( 16.51473224551083163, -9.474510206698727899, 25.83442372801900078 ) ) ;
#21671=CARTESIAN_POINT ( 'NONE',  ( 9.564922557960805705, 16.46253265017160317, 99.58224293864770971 ) ) ;
#21672=CARTESIAN_POINT ( 'NONE',  ( 15.72974639402199770, -15.80617190586745480, 68.12390960531436690 ) ) ;
#21674=CARTESIAN_POINT ( 'NONE',  ( 0.05219959533909260263, 19.03943276465977164, 29.99890960531435979 ) ) ;
#21675=CARTESIAN_POINT ( 'NONE',  ( -5.719274019375665041, -21.55341960407619695, 104.7927570613523898 ) ) ;
#21676=CARTESIAN_POINT ( 'NONE',  ( -4.379528057220086978, -16.55341960407618274, 74.79275706135234714 ) ) ;
#21677=CARTESIAN_POINT ( 'NONE',  ( 15.80617190586769283, -15.72974639402175789, 30.62609039468567929 ) ) ;
#21678=CARTESIAN_POINT ( 'NONE',  ( -4.379528057220086978, -16.55341960407618274, 39.79275706135235424 ) ) ;
#21679=CARTESIAN_POINT ( 'NONE',  ( -5.153800228976328057, -19.02544592524343514, 107.2905762719810383 ) ) ;
#21680=CARTESIAN_POINT ( 'NONE',  ( -19.03943276465977164, 0.05219959533909376836, 56.24890960531435979 ) ) ;
#21681=CARTESIAN_POINT ( 'NONE',  ( -19.05341960407611168, -5.049401038298163336, 61.45724293864769550 ) ) ;
#21683=CARTESIAN_POINT ( 'NONE',  ( 16.52544592524335698, 4.483927247898782831, 41.45942372801901143 ) ) ;
#21684=CARTESIAN_POINT ( 'NONE',  ( -0.05219959533910754901, -16.53943276465976808, 87.49890960531436690 ) ) ;
#21685=CARTESIAN_POINT ( 'NONE',  ( -0.05219959533934338120, 16.53943276465976808, 107.5010903946856899 ) ) ;
#21686=CARTESIAN_POINT ( 'NONE',  ( -16.46253265017160317, 9.564922557960807481, 50.83224293864770260 ) ) ;
#21687=CARTESIAN_POINT ( 'NONE',  ( -18.62759615963255300, -10.81492255796106328, 59.16775706135234714 ) ) ;
#21688=CARTESIAN_POINT ( 'NONE',  ( 16.51473224551069308, 9.474510206698969483, 79.16557627198103830 ) ) ;
#21689=CARTESIAN_POINT ( 'NONE',  ( 19.05341960407611168, 5.049401038298154454, 63.95724293864769550 ) ) ;
#21690=CARTESIAN_POINT ( 'NONE',  ( -5.049401038298153566, 19.05341960407611168, 90.20724293864766707 ) ) ;
#21691=CARTESIAN_POINT ( 'NONE',  ( 12.14591786802309770, 12.06949235617756955, 44.37390960531435979 ) ) ;
#21692=CARTESIAN_POINT ( 'NONE',  ( -12.06949235617756955, 12.14591786802309770, 25.62390960531435624 ) ) ;
#21693=CARTESIAN_POINT ( 'NONE',  ( -8.224510206698948167, 14.34966873604960824, 45.41557627198103830 ) ) ;
#21695=CARTESIAN_POINT ( 'NONE',  ( -13.89961937509957401, -13.97604488694547875, 44.37609039468566863 ) ) ;
#21696=CARTESIAN_POINT ( 'NONE',  ( -20.49784845693389101, -5.510910596163089556E-15, 45.00000000000000000 ) ) ;
#21697=CARTESIAN_POINT ( 'NONE',  ( -16.46253265017160317, 9.564922557960807481, 60.83224293864769550 ) ) ;
#21698=CARTESIAN_POINT ( 'NONE',  ( -0.05219959533936034679, 19.03943276465977164, 32.50109039468566863 ) ) ;
#21701=CARTESIAN_POINT ( 'NONE',  ( -16.51473224551082808, 9.474510206698731452, 78.33442372801900433 ) ) ;
#21702=CARTESIAN_POINT ( 'NONE',  ( -16.55341960407617563, 4.379528057220093196, 63.54275706135234003 ) ) ;
#21703=CARTESIAN_POINT ( 'NONE',  ( 16.88567814943162659, 6.947325034625703388, 93.79001122652590539 ) ) ;
#21704=CARTESIAN_POINT ( 'NONE',  ( 16.51473224551069308, 9.474510206698969483, 89.16557627198103830 ) ) ;
#21705=CARTESIAN_POINT ( 'NONE',  ( -21.55341960407619339, 5.719274019375674811, 23.54275706135235424 ) ) ;
#21706=CARTESIAN_POINT ( 'NONE',  ( -19.03943276465977164, -0.05219959533935918106, 73.75109039468566152 ) ) ;
#21708=CARTESIAN_POINT ( 'NONE',  ( 19.05341960407611168, 5.049401038298154454, 43.95724293864769550 ) ) ;
#21709=CARTESIAN_POINT ( 'NONE',  ( 19.03943276465977164, -0.05219959533909143690, 83.74890960531436690 ) ) ;
#21710=CARTESIAN_POINT ( 'NONE',  ( -16.55341960407611168, -4.379528057220339221, 46.45724293864769550 ) ) ;
#21711=CARTESIAN_POINT ( 'NONE',  ( -19.05341960407611168, -5.049401038298163336, 56.45724293864768129 ) ) ;
#21712=CARTESIAN_POINT ( 'NONE',  ( -16.51473224551082808, 9.474510206698731452, 53.33442372801900433 ) ) ;
#21714=CARTESIAN_POINT ( 'NONE',  ( 4.379528057220339221, -16.55341960407611168, 87.70724293864769550 ) ) ;
#21715=CARTESIAN_POINT ( 'NONE',  ( -13.97604488694547697, 13.89961937509957934, 28.12609039468565797 ) ) ;
#21716=CARTESIAN_POINT ( 'NONE',  ( 0.05219959533909260263, 19.03943276465977164, 69.99890960531435269 ) ) ;
#21717=CARTESIAN_POINT ( 'NONE',  ( 21.55341960407610458, 5.719274019375980345, 68.95724293864769550 ) ) ;
#21718=CARTESIAN_POINT ( 'NONE',  ( -16.52544592524342804, 4.483927247898546575, 61.04057627198103120 ) ) ;
#21719=CARTESIAN_POINT ( 'NONE',  ( 9.564922557961047289, -16.46253265017146816, 20.41775706135233293 ) ) ;
#21720=CARTESIAN_POINT ( 'NONE',  ( -16.51473224551069308, -9.474510206698971260, 101.6655762719810241 ) ) ;
#21721=CARTESIAN_POINT ( 'NONE',  ( -21.53943276465977519, 0.05219959533907696930, 26.24890960531435624 ) ) ;
#21722=CARTESIAN_POINT ( 'NONE',  ( 9.474510206698971260, -16.51473224551069308, 57.91557627198103120 ) ) ;
#21723=CARTESIAN_POINT ( 'NONE',  ( -19.03943276465977164, 0.05219959533909376836, 36.24890960531436690 ) ) ;
#21724=CARTESIAN_POINT ( 'NONE',  ( 4.379528057220339221, -16.55341960407611168, 97.70724293864772392 ) ) ;
#21725=CARTESIAN_POINT ( 'NONE',  ( 5.823673210054125526, 21.52544592524343514, 109.7905762719810383 ) ) ;
#21726=CARTESIAN_POINT ( 'NONE',  ( 16.46253265017160672, -9.564922557960803928, 103.3322429386476955 ) ) ;
#21727=CARTESIAN_POINT ( 'NONE',  ( -21.53943276465977519, 0.05219959533907696930, 116.2489096053143669 ) ) ;
#21728=CARTESIAN_POINT ( 'NONE',  ( 19.05341960407611168, 5.049401038298154454, 98.95724293864766707 ) ) ;
#21729=CARTESIAN_POINT ( 'NONE',  ( 16.53943276465976808, -0.05219959533910856209, 113.7489096053143527 ) ) ;
#21730=CARTESIAN_POINT ( 'NONE',  ( 18.62759615963255655, 10.81492255796105972, 76.66775706135234714 ) ) ;
#21731=CARTESIAN_POINT ( 'NONE',  ( 21.55341960407610458, 5.719274019375980345, 93.95724293864770971 ) ) ;
#21735=CARTESIAN_POINT ( 'NONE',  ( -12.14591786802326823, 12.06949235617739902, 48.12609039468568284 ) ) ;
#21737=CARTESIAN_POINT ( 'NONE',  ( -12.06949235617756955, 12.14591786802309770, 110.6239096053143669 ) ) ;
#21739=CARTESIAN_POINT ( 'NONE',  ( 19.05341960407611168, 5.049401038298154454, 63.95724293864769550 ) ) ;
#21740=CARTESIAN_POINT ( 'NONE',  ( 8.224510206698953496, -14.34966873604960469, 97.91557627198103830 ) ) ;
#21741=CARTESIAN_POINT ( 'NONE',  ( -18.67979575497178146, -10.72451020669898902, 46.66557627198102409 ) ) ;
#21742=CARTESIAN_POINT ( 'NONE',  ( 14.29746914071049879, -8.314922557960816363, 63.33224293864770260 ) ) ;
#21743=CARTESIAN_POINT ( 'NONE',  ( -8.314922557961024197, 14.29746914071037800, 22.91775706135235069 ) ) ;
#21744=CARTESIAN_POINT ( 'NONE',  ( 15.80617190586769283, -15.72974639402175789, 70.62609039468567573 ) ) ;
#21745=CARTESIAN_POINT ( 'NONE',  ( 16.38665767535050932, -7.295008042176168495, 77.76400864214544129 ) ) ;
#21746=CARTESIAN_POINT ( 'NONE',  ( -16.53943276465976808, -0.05219959533934237506, 103.7510903946857042 ) ) ;
#21747=CARTESIAN_POINT ( 'NONE',  ( 0.05219959533910956823, 16.53943276465976808, 39.99890960531436690 ) ) ;
#21748=CARTESIAN_POINT ( 'NONE',  ( 19.03943276465977164, -0.05219959533909143690, 33.74890960531435979 ) ) ;
#21749=CARTESIAN_POINT ( 'NONE',  ( -5.153800228976328057, -19.02544592524343514, 92.29057627198099567 ) ) ;
#21750=CARTESIAN_POINT ( 'NONE',  ( -18.62759615963270932, 10.81492255796079327, 100.8322429386477097 ) ) ;
#21751=CARTESIAN_POINT ( 'NONE',  ( 16.53943276465976808, 0.05219959533934440121, 31.25109039468568639 ) ) ;
#21752=CARTESIAN_POINT ( 'NONE',  ( -16.52544592524342804, 4.483927247898546575, 71.04057627198103830 ) ) ;
#21753=CARTESIAN_POINT ( 'NONE',  ( -18.67979575497193778, 10.72451020669871902, 78.33442372801901854 ) ) ;
#21754=CARTESIAN_POINT ( 'NONE',  ( -16.52544592524335698, -4.483927247898792601, 103.9594237280190185 ) ) ;
#21755=CARTESIAN_POINT ( 'NONE',  ( 17.48853670773249291, -5.747243402302948390, 46.16671299749997814 ) ) ;
#21756=CARTESIAN_POINT ( 'NONE',  ( -19.53091890409951858, -5.500000000000037303, 65.06097431831420863 ) ) ;
#21757=CARTESIAN_POINT ( 'NONE',  ( 12.06949235617757843, -12.14591786802309237, 23.12390960531436335 ) ) ;
#21758=CARTESIAN_POINT ( 'NONE',  ( -4.483927247898782831, 16.52544592524335698, 77.70942372801900433 ) ) ;
#21759=CARTESIAN_POINT ( 'NONE',  ( 16.46253265017160672, -9.564922557960803928, 88.33224293864769550 ) ) ;
#21760=CARTESIAN_POINT ( 'NONE',  ( -9.564922557960796823, -16.46253265017161027, 102.0822429386477097 ) ) ;
#21761=CARTESIAN_POINT ( 'NONE',  ( -18.67979575497193778, 10.72451020669871902, 88.33442372801901854 ) ) ;
#21763=CARTESIAN_POINT ( 'NONE',  ( -8.224510206698735004, -14.34966873604973081, 89.58442372801901854 ) ) ;
#21764=CARTESIAN_POINT ( 'NONE',  ( 14.34966873604960469, 8.224510206698951720, 59.16557627198103120 ) ) ;
#21765=CARTESIAN_POINT ( 'NONE',  ( -16.46253265017160317, 9.564922557960807481, 65.83224293864769550 ) ) ;
#21767=CARTESIAN_POINT ( 'NONE',  ( -4.379528057220086978, -16.55341960407618274, 19.79275706135235069 ) ) ;
#21768=CARTESIAN_POINT ( 'NONE',  ( 12.14591786802309770, 12.06949235617756955, 104.3739096053143669 ) ) ;
#21769=CARTESIAN_POINT ( 'NONE',  ( -19.03943276465977164, 0.05219959533909376836, 76.24890960531435269 ) ) ;
#21770=CARTESIAN_POINT ( 'NONE',  ( 14.29746914071037800, 8.314922557961029526, 21.66775706135235069 ) ) ;
#21772=CARTESIAN_POINT ( 'NONE',  ( -5.823673210054431948, 21.52544592524334988, 112.7094237280190328 ) ) ;
#21773=CARTESIAN_POINT ( 'NONE',  ( 0.05219959533934541429, -16.53943276465976808, 80.00109039468568994 ) ) ;
#21774=CARTESIAN_POINT ( 'NONE',  ( -9.564922557961040184, 16.46253265017147172, 97.91775706135233293 ) ) ;
#21775=CARTESIAN_POINT ( 'NONE',  ( -4.379528057220328563, 16.55341960407611168, 115.2072429386476955 ) ) ;
#21776=CARTESIAN_POINT ( 'NONE',  ( -16.55341960407617563, 4.379528057220093196, 63.54275706135234003 ) ) ;
#21777=CARTESIAN_POINT ( 'NONE',  ( -12.06949235617739369, -12.14591786802326823, 49.37609039468569705 ) ) ;
#21779=CARTESIAN_POINT ( 'NONE',  ( 16.46253265017146816, 9.564922557961045513, 71.66775706135233293 ) ) ;
#21780=CARTESIAN_POINT ( 'NONE',  ( 15.72974639402176855, 15.80617190586768217, 96.87609039468568994 ) ) ;
#21781=CARTESIAN_POINT ( 'NONE',  ( -16.46253265017160317, 9.564922557960807481, 35.83224293864768839 ) ) ;
#21782=CARTESIAN_POINT ( 'NONE',  ( -19.05341960407611168, -5.049401038298163336, 76.45724293864769550 ) ) ;
#21783=CARTESIAN_POINT ( 'NONE',  ( 16.53943276465976808, -0.05219959533910856209, 73.74890960531433848 ) ) ;
#21784=CARTESIAN_POINT ( 'NONE',  ( -18.67979575497193778, 10.72451020669871902, 93.33442372801901854 ) ) ;
#21785=CARTESIAN_POINT ( 'NONE',  ( 13.89961937509957401, 13.97604488694547697, 41.87609039468566152 ) ) ;
#21786=CARTESIAN_POINT ( 'NONE',  ( -21.53943276465977519, 0.05219959533907696930, 36.24890960531435979 ) ) ;
#21787=CARTESIAN_POINT ( 'NONE',  ( 10.72451020669871369, 18.67979575497193778, 112.0844237280190185 ) ) ;
#21788=CARTESIAN_POINT ( 'NONE',  ( -19.05341960407611168, -5.049401038298163336, 76.45724293864769550 ) ) ;
#21789=CARTESIAN_POINT ( 'NONE',  ( 21.55341960407619695, -5.719274019375665929, 111.0427570613523613 ) ) ;
#21790=CARTESIAN_POINT ( 'NONE',  ( 21.55341960407610458, 5.719274019375980345, 68.95724293864769550 ) ) ;
#21791=CARTESIAN_POINT ( 'NONE',  ( -9.564922557960796823, -16.46253265017161027, 97.08224293864769550 ) ) ;
#21792=CARTESIAN_POINT ( 'NONE',  ( 9.564922557961047289, -16.46253265017146816, 70.41775706135233293 ) ) ;
#21793=CARTESIAN_POINT ( 'NONE',  ( -19.05341960407611168, -5.049401038298163336, 96.45724293864769550 ) ) ;
#21794=CARTESIAN_POINT ( 'NONE',  ( 19.05341960407617918, -5.049401038297876454, 96.04275706135231871 ) ) ;
#21795=CARTESIAN_POINT ( 'NONE',  ( -12.06949235617739369, -12.14591786802326823, 44.37609039468567573 ) ) ;
#21796=CARTESIAN_POINT ( 'NONE',  ( 8.314922557960818139, 14.29746914071049879, 114.5822429386477097 ) ) ;
#21797=CARTESIAN_POINT ( 'NONE',  ( -5.049401038298153566, 19.05341960407611168, 80.20724293864769550 ) ) ;
#21798=CARTESIAN_POINT ( 'NONE',  ( -15.80617190586745835, -15.72974639402198527, 56.87390960531436690 ) ) ;
#21799=CARTESIAN_POINT ( 'NONE',  ( 12.06949235617739724, 12.14591786802326823, 26.87609039468567218 ) ) ;
#21800=CARTESIAN_POINT ( 'NONE',  ( -18.62759615963255300, -10.81492255796106328, 39.16775706135235424 ) ) ;
#21801=CARTESIAN_POINT ( 'NONE',  ( -18.62759615963255300, -10.81492255796106328, 79.16775706135234714 ) ) ;
#21802=CARTESIAN_POINT ( 'NONE',  ( 4.379528057220092307, 16.55341960407617563, 87.29275706135236135 ) ) ;
#21803=CARTESIAN_POINT ( 'NONE',  ( -9.474510206698964154, 16.51473224551069663, 90.41557627198103830 ) ) ;
#21804=CARTESIAN_POINT ( 'NONE',  ( 0.05219959533910956823, 16.53943276465976808, 79.99890960531435269 ) ) ;
#21805=CARTESIAN_POINT ( 'NONE',  ( 4.379528057220092307, 16.55341960407617563, 112.2927570613523471 ) ) ;
#21806=CARTESIAN_POINT ( 'NONE',  ( 19.02544592524334988, 5.153800228976608722, 61.45942372801900433 ) ) ;
#21808=CARTESIAN_POINT ( 'NONE',  ( 21.52544592524334988, 5.823673210054432836, 41.45942372801901143 ) ) ;
#21809=CARTESIAN_POINT ( 'NONE',  ( 14.29746914071049879, -8.314922557960816363, 98.33224293864769550 ) ) ;
#21810=CARTESIAN_POINT ( 'NONE',  ( -5.049401038298153566, 19.05341960407611168, 110.2072429386476671 ) ) ;
#21811=CARTESIAN_POINT ( 'NONE',  ( -8.314922557961024197, 14.29746914071037800, 97.91775706135236135 ) ) ;
#21812=CARTESIAN_POINT ( 'NONE',  ( -10.81492255796105439, 18.62759615963255655, 82.91775706135234714 ) ) ;
#21813=CARTESIAN_POINT ( 'NONE',  ( -14.29746914071037622, -8.314922557961029526, 49.16775706135234003 ) ) ;
#21814=CARTESIAN_POINT ( 'NONE',  ( 18.67979575497194134, -10.72451020669871369, 45.83442372801901854 ) ) ;
#21815=VERTEX_POINT ( 'NONE', #19211 ) ;
#21816=CARTESIAN_POINT ( 'NONE',  ( 18.62759615963271287, -10.81492255796078972, 108.3322429386477097 ) ) ;
#21817=CARTESIAN_POINT ( 'NONE',  ( -12.06949235617756955, 12.14591786802309770, 95.62390960531436690 ) ) ;
#21818=CARTESIAN_POINT ( 'NONE',  ( -19.53091890409952214, -5.500000000000036415, 50.06097431831421574 ) ) ;
#21819=CARTESIAN_POINT ( 'NONE',  ( -0.05219959533910754901, -16.53943276465976808, 67.49890960531436690 ) ) ;
#21820=CARTESIAN_POINT ( 'NONE',  ( -0.05219959533934338120, 16.53943276465976808, 97.50109039468567573 ) ) ;
#21821=CARTESIAN_POINT ( 'NONE',  ( 0.05219959533909260263, 19.03943276465977164, 44.99890960531435979 ) ) ;
#21822=CARTESIAN_POINT ( 'NONE',  ( -18.67979575497178146, -10.72451020669898902, 41.66557627198103120 ) ) ;
#21823=CARTESIAN_POINT ( 'NONE',  ( 12.14591786802309770, 12.06949235617756955, 74.37390960531436690 ) ) ;
#21824=CARTESIAN_POINT ( 'NONE',  ( 15.80617190586746368, 15.72974639402197994, 74.37390960531436690 ) ) ;
#21825=CARTESIAN_POINT ( 'NONE',  ( -5.049401038298153566, 19.05341960407611168, 85.20724293864766707 ) ) ;
#21826=CARTESIAN_POINT ( 'NONE',  ( 19.03943276465977164, -0.05219959533909143690, 38.74890960531436690 ) ) ;
#21827=CARTESIAN_POINT ( 'NONE',  ( -16.46253265017146816, -9.564922557961047289, 89.16775706135234714 ) ) ;
#21828=CARTESIAN_POINT ( 'NONE',  ( -15.72974639402197994, 15.80617190586746368, 35.62390960531437401 ) ) ;
#21829=CARTESIAN_POINT ( 'NONE',  ( 21.55341960407619695, -5.719274019375665929, 56.04275706135235424 ) ) ;
#21830=CARTESIAN_POINT ( 'NONE',  ( -9.564922557960796823, -16.46253265017161027, 57.08224293864769550 ) ) ;
#21831=CARTESIAN_POINT ( 'NONE',  ( -5.049401038298153566, 19.05341960407611168, 85.20724293864766707 ) ) ;
#21833=CARTESIAN_POINT ( 'NONE',  ( -4.379528057220086978, -16.55341960407618274, 54.79275706135235424 ) ) ;
#21834=CARTESIAN_POINT ( 'NONE',  ( 21.53943276465977519, 0.05219959533937863772, 36.25109039468567573 ) ) ;
#21835=CARTESIAN_POINT ( 'NONE',  ( -15.72974639402176322, -15.80617190586768395, 69.37609039468567573 ) ) ;
#21836=CARTESIAN_POINT ( 'NONE',  ( -21.53943276465977519, 0.05219959533907696930, 26.24890960531435624 ) ) ;
#21837=CARTESIAN_POINT ( 'NONE',  ( -5.823673210054116645, -21.52544592524344225, 87.29057627198103830 ) ) ;
#21838=CARTESIAN_POINT ( 'NONE',  ( -21.55341960407619339, 5.719274019375674811, 28.54275706135234358 ) ) ;
#21839=CARTESIAN_POINT ( 'NONE',  ( -16.55341960407617563, 4.379528057220093196, 63.54275706135234003 ) ) ;
#21841=CARTESIAN_POINT ( 'NONE',  ( 21.52544592524344225, -5.823673210054117533, 63.54057627198103830 ) ) ;
#21842=CARTESIAN_POINT ( 'NONE',  ( 13.89961937509957401, 13.97604488694547697, 21.87609039468566152 ) ) ;
#21843=CARTESIAN_POINT ( 'NONE',  ( -0.05219959533909027116, -19.03943276465977164, 67.49890960531436690 ) ) ;
#21844=CARTESIAN_POINT ( 'NONE',  ( -16.55341960407617563, 4.379528057220093196, 103.5427570613523613 ) ) ;
#21845=CARTESIAN_POINT ( 'NONE',  ( -17.49999999999999645, -3.805241302050224039, 104.6264752721741331 ) ) ;
#21846=CARTESIAN_POINT ( 'NONE',  ( 19.03943276465977164, -0.05219959533909143690, 83.74890960531436690 ) ) ;
#21847=CARTESIAN_POINT ( 'NONE',  ( -0.05219959533936034679, 19.03943276465977164, 52.50109039468566863 ) ) ;
#21848=CARTESIAN_POINT ( 'NONE',  ( -16.51473224551082808, 9.474510206698731452, 78.33442372801900433 ) ) ;
#21849=CARTESIAN_POINT ( 'NONE',  ( -21.55341960407610458, -5.719274019375992779, 51.45724293864770260 ) ) ;
#21850=CARTESIAN_POINT ( 'NONE',  ( 8.224510206698742110, 14.34966873604972548, 112.0844237280190185 ) ) ;
#21851=CARTESIAN_POINT ( 'NONE',  ( 16.46253265017146816, 9.564922557961045513, 101.6677570613523329 ) ) ;
#21852=CARTESIAN_POINT ( 'NONE',  ( -9.474510206698964154, 16.51473224551069663, 40.41557627198103120 ) ) ;
#21853=CARTESIAN_POINT ( 'NONE',  ( 16.46253265017146816, 9.564922557961045513, 91.66775706135234714 ) ) ;
#21854=CARTESIAN_POINT ( 'NONE',  ( 21.52544592524344225, -5.823673210054117533, 88.54057627198103830 ) ) ;
#21855=CARTESIAN_POINT ( 'NONE',  ( -0.05219959533936034679, 19.03943276465977164, 52.50109039468566863 ) ) ;
#21857=CARTESIAN_POINT ( 'NONE',  ( 9.474510206698971260, -16.51473224551069308, 57.91557627198103120 ) ) ;
#21858=CARTESIAN_POINT ( 'NONE',  ( 8.314922557960818139, 14.29746914071049879, 64.58224293864769550 ) ) ;
#21859=ADVANCED_FACE ( 'NONE', ( #138558 ), #128447, .T. ) ;
#21860=CARTESIAN_POINT ( 'NONE',  ( -13.97604488694527625, -13.89961937509977652, 51.87390960531436690 ) ) ;
#21861=CARTESIAN_POINT ( 'NONE',  ( -12.14591786802309592, -12.06949235617757132, 56.87390960531436690 ) ) ;
#21862=CARTESIAN_POINT ( 'NONE',  ( 17.97182807773875624, -5.499999999999865885, 56.03038844047289047 ) ) ;
#21864=CARTESIAN_POINT ( 'NONE',  ( -12.06949235617756955, 12.14591786802309770, 30.62390960531436335 ) ) ;
#21865=CARTESIAN_POINT ( 'NONE',  ( -9.474510206698964154, 16.51473224551069663, 65.41557627198102409 ) ) ;
#21867=CARTESIAN_POINT ( 'NONE',  ( 19.03943276465977164, 0.05219959533936151252, 41.25109039468566152 ) ) ;
#21868=CARTESIAN_POINT ( 'NONE',  ( 16.52544592524335698, 4.483927247898782831, 46.45942372801901854 ) ) ;
#21869=CARTESIAN_POINT ( 'NONE',  ( 15.80617190586746368, 15.72974639402197994, 44.37390960531435979 ) ) ;
#21870=CARTESIAN_POINT ( 'NONE',  ( 15.72974639402176855, 15.80617190586768217, 101.8760903946857042 ) ) ;
#21871=CARTESIAN_POINT ( 'NONE',  ( -19.05341960407611168, -5.049401038298163336, 66.45724293864769550 ) ) ;
#21873=CARTESIAN_POINT ( 'NONE',  ( -19.03943276465977164, 0.05219959533909376836, 101.2489096053143669 ) ) ;
#21875=CARTESIAN_POINT ( 'NONE',  ( -18.62759615963255300, -10.81492255796106328, 29.16775706135234003 ) ) ;
#21876=CARTESIAN_POINT ( 'NONE',  ( 8.224510206698953496, -14.34966873604960469, 97.91557627198103830 ) ) ;
#21877=CARTESIAN_POINT ( 'NONE',  ( 21.55341960407610458, 5.719274019375980345, 88.95724293864769550 ) ) ;
#21878=CARTESIAN_POINT ( 'NONE',  ( -16.51473224551069308, -9.474510206698971260, 86.66557627198102409 ) ) ;
#21879=CARTESIAN_POINT ( 'NONE',  ( -13.97604488694527625, -13.89961937509977652, 86.87390960531436690 ) ) ;
#21880=CARTESIAN_POINT ( 'NONE',  ( -15.72974639402197994, 15.80617190586746368, 105.6239096053143669 ) ) ;
#21882=CARTESIAN_POINT ( 'NONE',  ( -13.97604488694527625, -13.89961937509977652, 71.87390960531433848 ) ) ;
#21884=CARTESIAN_POINT ( 'NONE',  ( 12.06949235617757843, -12.14591786802309237, 108.1239096053143811 ) ) ;
#21885=CARTESIAN_POINT ( 'NONE',  ( 9.564922557960805705, 16.46253265017160317, 29.58224293864769550 ) ) ;
#21886=CARTESIAN_POINT ( 'NONE',  ( -16.51473224551082808, 9.474510206698731452, 98.33442372801900433 ) ) ;
#21887=CARTESIAN_POINT ( 'NONE',  ( -16.53943276465976808, 0.05219959533911058130, 111.2489096053143669 ) ) ;
#21888=CARTESIAN_POINT ( 'NONE',  ( 10.72451020669871369, 18.67979575497193778, 67.08442372801901854 ) ) ;
#21889=CARTESIAN_POINT ( 'NONE',  ( 5.153800228976335163, 19.02544592524342804, 59.79057627198100988 ) ) ;
#21890=CARTESIAN_POINT ( 'NONE',  ( -5.823673210054431948, 21.52544592524334988, 32.70942372801900433 ) ) ;
#21891=CARTESIAN_POINT ( 'NONE',  ( -10.81492255796078084, -18.62759615963271287, 107.0822429386476955 ) ) ;
#21893=CARTESIAN_POINT ( 'NONE',  ( 19.02544592524343514, -5.153800228976328945, 78.54057627198099567 ) ) ;
#21895=CARTESIAN_POINT ( 'NONE',  ( 4.379528057220092307, 16.55341960407617563, 27.29275706135234358 ) ) ;
#21896=CARTESIAN_POINT ( 'NONE',  ( -18.62759615963270932, 10.81492255796079327, 35.83224293864768839 ) ) ;
#21897=CARTESIAN_POINT ( 'NONE',  ( 21.53943276465977519, 0.05219959533937863772, 61.25109039468567573 ) ) ;
#21898=CARTESIAN_POINT ( 'NONE',  ( 19.03943276465977164, -0.05219959533909143690, 113.7489096053143669 ) ) ;
#21899=CARTESIAN_POINT ( 'NONE',  ( -19.05341960407617563, 5.049401038297882671, 98.54275706135233293 ) ) ;
#21900=CARTESIAN_POINT ( 'NONE',  ( 16.46253265017160672, -9.564922557960803928, 53.33224293864768839 ) ) ;
#21901=CARTESIAN_POINT ( 'NONE',  ( -9.474510206698964154, 16.51473224551069663, 70.41557627198102409 ) ) ;
#21902=CARTESIAN_POINT ( 'NONE',  ( 8.224510206698953496, -14.34966873604960469, 97.91557627198103830 ) ) ;
#21903=CARTESIAN_POINT ( 'NONE',  ( -16.51473224551069308, -9.474510206698971260, 111.6655762719810383 ) ) ;
#21904=CARTESIAN_POINT ( 'NONE',  ( 4.379528057220339221, -16.55341960407611168, 97.70724293864772392 ) ) ;
#21905=CARTESIAN_POINT ( 'NONE',  ( -0.05219959533907301413, -21.53943276465977519, 22.49890960531436335 ) ) ;
#21906=CARTESIAN_POINT ( 'NONE',  ( -16.55341960407611168, -4.379528057220339221, 61.45724293864770260 ) ) ;
#21907=CARTESIAN_POINT ( 'NONE',  ( 5.049401038298161559, -19.05341960407611168, 42.70724293864767418 ) ) ;
#21908=CARTESIAN_POINT ( 'NONE',  ( 15.72974639402176855, 15.80617190586768217, 56.87609039468568994 ) ) ;
#21909=CARTESIAN_POINT ( 'NONE',  ( -9.564922557961040184, 16.46253265017147172, 97.91775706135233293 ) ) ;
#21910=CARTESIAN_POINT ( 'NONE',  ( -8.314922557960811034, -14.29746914071050412, 52.08224293864768839 ) ) ;
#21911=CARTESIAN_POINT ( 'NONE',  ( -5.719274019375665041, -21.55341960407619695, 19.79275706135235069 ) ) ;
#21912=CARTESIAN_POINT ( 'NONE',  ( -10.81492255796078084, -18.62759615963271287, 47.08224293864770260 ) ) ;
#21913=CARTESIAN_POINT ( 'NONE',  ( 19.03943276465977164, -0.05219959533909143690, 113.7489096053143669 ) ) ;
#21915=CARTESIAN_POINT ( 'NONE',  ( -19.05341960407611168, -5.049401038298163336, 61.45724293864769550 ) ) ;
#21916=CARTESIAN_POINT ( 'NONE',  ( 16.55341960407618274, -4.379528057220086978, 111.0427570613523613 ) ) ;
#21918=CARTESIAN_POINT ( 'NONE',  ( 12.14591786802327356, -12.06949235617739191, 105.6260903946856899 ) ) ;
#21919=CARTESIAN_POINT ( 'NONE',  ( -14.34966873604972548, 8.224510206698743886, 88.33442372801901854 ) ) ;
#21920=CARTESIAN_POINT ( 'NONE',  ( 9.564922557961047289, -16.46253265017146816, 45.41775706135232582 ) ) ;
#21922=CARTESIAN_POINT ( 'NONE',  ( -0.05219959533909027116, -19.03943276465977164, 87.49890960531436690 ) ) ;
#21923=CARTESIAN_POINT ( 'NONE',  ( 0.05219959533909260263, 19.03943276465977164, 49.99890960531435979 ) ) ;
#21924=CARTESIAN_POINT ( 'NONE',  ( -4.483927247898539470, -16.52544592524342804, 67.29057627198103830 ) ) ;
#21925=CARTESIAN_POINT ( 'NONE',  ( 17.48853670773245383, -5.747243402303093163, 101.1667129974999426 ) ) ;
#21926=CARTESIAN_POINT ( 'NONE',  ( 9.474510206698971260, -16.51473224551069308, 107.9155762719810383 ) ) ;
#21927=CARTESIAN_POINT ( 'NONE',  ( 10.81492255796078972, 18.62759615963270932, 39.58224293864769550 ) ) ;
#21928=CARTESIAN_POINT ( 'NONE',  ( 0.05219959533910956823, 16.53943276465976808, 89.99890960531438111 ) ) ;
#21929=CARTESIAN_POINT ( 'NONE',  ( -8.224510206698735004, -14.34966873604973081, 44.58442372801901854 ) ) ;
#21930=CARTESIAN_POINT ( 'NONE',  ( -12.06949235617756955, 12.14591786802309770, 80.62390960531438111 ) ) ;
#21931=DIRECTION ( 'NONE',  ( -0.000000000000000000, -0.000000000000000000, 1.000000000000000000 ) ) ;
#21932=CARTESIAN_POINT ( 'NONE',  ( 13.89961937509957401, 13.97604488694547697, 76.87609039468566152 ) ) ;
#21933=CARTESIAN_POINT ( 'NONE',  ( -5.153800228976328057, -19.02544592524343514, 97.29057627198099567 ) ) ;
#21934=CARTESIAN_POINT ( 'NONE',  ( 5.049401038297881783, 19.05341960407617563, 77.29275706135231871 ) ) ;
#21936=CARTESIAN_POINT ( 'NONE',  ( 0.05219959533934541429, -16.53943276465976808, 35.00109039468568284 ) ) ;
#21937=CARTESIAN_POINT ( 'NONE',  ( 4.379528057220092307, 16.55341960407617563, 107.2927570613523471 ) ) ;
#21938=CARTESIAN_POINT ( 'NONE',  ( 16.51473224551083163, -9.474510206698727899, 75.83442372801900433 ) ) ;
#21939=( BOUNDED_SURFACE ( )  B_SPLINE_SURFACE ( 3, 2, ( 
 ( #70636, #71628, #133294, #118140, #119143, #88786, #10963, #162632, #7946, #194984, #131295, #100948, #191970, #53456, #164646, #56462, #176824, #178821, #54462, #24139, #150479, #40291, #72637, #42302, #132302, #85791, #23130, #195998, #134312, #193994, #163646, #69629, #179830, #84775, #192984, #116132, #26141, #180824, #103963, #87783, #57471, #165641, #27139, #177821, #11974, #147477, #8967, #117127, #101965, #185779, #124078, #91742, #136287, #89783, #107917, #105941, #196983, #181808, #197963, #155431, #198958, #123090, #168602, #77589, #120117, #151468, #28143, #170603, #153437, #184776, #43286, #199954, #104955, #60425, #16921, #62408, #166641, #61419, #169602, #121106, #58449, #59433, #736, #12957, #182800, #154436, #108923, #44283, #32093, #47266, #93750, #135310, #46262, #106929, #31100, #167626, #152444, #122098, #74621, #15930, #29123, #90761, #45276, #13930, #30102, #75597, #76595, #137276, #92748, #183789, #14935, #138271, #139260, #35064, #79579, #33087, #51232, #49249, #140248, #125093, #141248, #98710, #142237, #66396, #111907, #20887, #63418, #94743, #171599, #113877, #96719, #128058, #186791, #143224, #48262, #3722, #160404, #5711, #109915, #4706, #112893, #64414, #1740, #2737, #144227, #156423, #126083, #97701, #52220, #187779, #175574, #190746, #37051, #78574, #189760, #50251, #174587, #110907, #95737, #65399, #17924, #159392, #172593, #34079, #188767, #157423, #173595, #18917, #36052, #80562, #158407, #82545, #19896, #127060, #67388, #81537, #129045, #146216, #191733, #10733, #25911, #21893, #133061, #149242, #7704, #40048, #72397, #9733, #134073, #56223, #100714, #101722, #178583, #148239, #195763, #118911, #179594, #192745, #38061, #24908, #161401, #69387, #103733, #83543, #194751, #163412, #145222, #8728, #84539, #131056, #180595, #70397, #41066, #57237, #162394, #115899, #53215, #87555, #102729, #23897, #193754, #99717, #86555, #6704, #68382, #130034, #117905, #42069, #114893, #71397, #164418, #176587, #22893, #54228, #177589, #39056, #85549, #147236, #132065, #55222, #116891, #30863, #181577, #151236, #184541, #139017, #12725, #62169, #77350, #497, #47023, #76357, #137035, #29867, #27907, #182566, #90532, #196756, #46021, #89550, #58223, #75365, #136056, #198725, #119892, #91504, #43055, #60192, #169354, #121862, #104721, #154199, #73409, #138034, #74391, #135080, #15689, #92510, #165413, #199715, #123833, #197731, #183554, #185531, #153191, #26906, #61181, #44049, #45040, #106698, #14694, #88549, #150247, #122853, #59197, #166412, #168371, #120866, #105709, #11742, #167396, #107677, #28892, #152214, #13698, #171359, #17678, #69904, #95493, #127812, #159144, #187542, #2494, #78330, #112650, #66149, #110664, #80319, #124849, #188522, #108682, #193254, #170360, #81298, #35812, #23401, #49999, #96477, #97458, #126816, #31852, #111664, #93505, #189517, #155191, #16681, #85048, #146729, #65157, #109678, #63170, #142982, #79336, #140003, #1492, #32847, #131570, #172344, #158165, #141992, #50990, #186549, #48021, #94497, #8226, #173351, #19657, #156179, #34822, #141006, #33833, #174342, #64175, #125840, #49009, #157179, #4460, #18673, #3480, #119412, #24414, #180108, #74888, #182075, #162905, #181096, #27412, #40569, #116400, #55729, #120382, #70906, #102239, #73909, #28413, #163927, #151732, #166912, #90050, #136551, #165914, #26415, #42570, #117402, #71898, #41576, #86063, #135579, #179100, #147753, #164921, #25424, #88054, #9239, #104233, #132573, #149742, #58713, #11243, #194262, #43558, #87065, #89058, #148750, #10238, #105224, #13225, #54727, #150749, #178089, #133569, #72918, #39559, #12247, #101216, #197251, #195260, #134587, #196273, #56744, #118415, #103240, #57742, #168861, #14196, #1000, #137541, #45536, #79848, #198231, #109188, #154700, #121375, #185042, #60689, #107190, #156697, #46529, #17187, #48529, #76857, #92010, #167890, #2009, #155692, #6, #169871 ),
 ( #62674, #183068, #61680, #106206, #170867, #199223, #138528, #63688, #91020, #47534, #123349, #122364, #31364, #30366, #124355, #44551, #187059, #108189, #186050, #78841, #93014, #33350, #16195, #110183, #29389, #32358, #77850, #152706, #153703, #140519, #94011, #171862, #95009, #139517, #125363, #18191, #75865, #184053, #59703, #15198, #3983, #99980, #21154, #189037, #23161, #34343, #81801, #191007, #97965, #114143, #126342, #65663, #173863, #113155, #68648, #129311, #191999, #175844, #20156, #159657, #82809, #67654, #130304, #38324, #98975, #112175, #157688, #144491, #80828, #50512, #141517, #3004, #52483, #5974, #64680, #128322, #127325, #35331, #161665, #190021, #160665, #53485, #143488, #96984, #111172, #145488, #22157, #4973, #174845, #19179, #37317, #188039, #49509, #172862, #83808, #115162, #176855, #6968, #96004, #142505, #158666, #66659, #51495, #36311, #42333, #7974, #84804, #135342, #73670, #41331, #85821, #39321, #57503, #55487, #146483, #131325, #147509, #104986, #148508, #72668, #118170, #27171, #69658, #100980, #177852, #120149, #102992, #134345, #193013, #149499, #54490, #9998, #166673, #12009, #116162, #10996, #119172, #70666, #162664, #8999, #150511, #24170, #132333, #103993, #58482, #194024, #181839, #88818, #117157, #178853, #40319, #43319, #164678, #196028, #101995, #180857, #163677, #71658, #25180, #197016, #86822, #165672, #133325, #195016, #56492, #179861, #26172, #87813, #13962, #47299, #1772, #75629, #125127, #140280, #63450, #109949, #139291, #199984, #92780, #90791, #45308, #153469, #59465, #108956, #152475, #121138, #138303, #198988, #61451, #182832, #154469, #44314, #123121, #32124, #184806, #105973, #16952, #136320, #768, #137307, #197995, #78606, #93781, #28175, #46292, #60456, #122131, #107949, #155462, #15961, #186824, #62438, #106958, #169636, #31132, #77621, #48293, #89817, #185812, #183818, #167658, #124112, #29154, #168632, #151498, #12990, #170635, #74653, #30132, #14965, #91775, #76625, #130066, #158438, #190775, #21924, #50281, #65428, #141279, #175606, #129074, #173626, #143253, #187810, #51262, #171630, #53249, #33118, #144256, #98741, #83575, #112922, #159421, #160434, #189791, #94775, #174617, #156457, #52250, #17956, #79609, #145254, #6735, #128087, #172623, #126115, #5743, #142269, #2769, #64445, #34111, #191765, #35096, #20917, #4737, #36082, #49279, #95768, #68413, #19926, #157454, #110937, #97732, #18948, #80594, #3751, #111939, #82575, #67419, #113907, #37082, #127089, #188798, #96748, #81567, #66426, #195797, #133091, #176619, #131088, #149273, #85582, #73440, #41098, #42101, #72429, #148271, #9763, #10765, #193784, #150279, #102762, #71427, #196787, #161433, #8759, #164450, #25943, #134107, #147268, #23927, #26939, #194781, #192776, #11776, #70429, #57269, #54260, #115931, #118943, #180628, #132095, #55253, #135111, #117937, #56255, #114926, #87586, #178614, #84571, #103765, #146249, #179626, #99749, #40077, #22925, #165444, #177621, #116921, #88581, #7735, #38094, #101755, #39089, #86588, #163443, #69421, #100745, #162426, #24940, #122886, #105742, #153226, #47059, #181609, #154233, #151268, #91538, #123867, #140038, #185565, #12758, #27940, #76391, #16714, #198760, #13732, #93540, #92545, #59230, #155225, #166444, #77383, #15723, #75399, #104754, #89582, #139051, #14730, #78364, #121895, #108718, #74423, #46055, #138067, #136089, #28925, #531, #169389, #31886, #58255, #199748, #60226, #184574, #197764, #183588, #119924, #170395, #120899, #107710, #30898, #44084, #43087, #182599, #167429, #90565, #152247, #62203, #137070, #45073, #106731, #168405, #29900, #61214, #112687, #173388, #66187, #64211, #18710, #126853, #32883, #82331, #125877, #94533, #111702, #172380, #34858, #156215, #127849, #17715, #96513, #5502, #158203, #79373, #190540, #109713, #174379, #187577, #171396, #52014, #67184, #1527, #19693, #49045, #33871, #81335, #128841 ),
 ( #141044, #110700, #83338, #63206, #35849, #143018, #124886, #188559, #95530, #157217, #160195, #50038, #20676, #113673, #80357, #142030, #2530, #175367, #159181, #3518, #4496, #65194, #189554, #186585, #48057, #51026, #97495, #36835, #98501, #144021, #21685, #133862, #163197, #26698, #86350, #6496, #102526, #68176, #145015, #195553, #57027, #101507, #146014, #99511, #117692, #115696, #129828, #191527, #7497, #165203, #8515, #132855, #178377, #87351, #53004, #161192, #37852, #180391, #24701, #194543, #114683, #72188, #164209, #39841, #148036, #179389, #23690, #41862, #56014, #9525, #176378, #22688, #38856, #40852, #25706, #149037, #177385, #54023, #118700, #71191, #84335, #103528, #100513, #10525, #69182, #130848, #192540, #162192, #85338, #147031, #70193, #131860, #193544, #55017, #116687, #152010, #58023, #107471, #119693, #152985, #73204, #13496, #196552, #60974, #27701, #28689, #153989, #181376, #137825, #90325, #12525, #59987, #120664, #91294, #134875, #77143, #136833, #14484, #135859, #183349, #138813, #11535, #184338, #42854, #121655, #15486, #170153, #293, #104519, #166200, #106487, #46815, #75161, #43840, #123629, #122649, #89343, #185325, #151035, #169148, #45820, #105505, #74190, #197530, #30652, #44831, #108475, #198516, #61962, #58998, #76146, #168165, #182362, #167191, #92306, #199508, #88338, #150029, #29662, #172140, #96278, #16476, #32638, #66939, #18470, #94292, #190295, #111458, #79124, #113432, #124640, #33626, #81103, #188315, #4262, #157964, #65942, #127613, #142781, #189312, #173144, #112449, #49793, #93295, #47817, #50790, #2286, #51772, #19456, #174138, #34619, #35610, #97255, #158943, #20432, #82083, #143776, #5257, #128602, #31646, #154981, #109466, #78125, #63968, #139794, #1283, #62959, #186335, #64954, #126613, #171150, #110459, #155970, #17468, #140797, #125638, #187335, #48805, #95289, #156973, #80120, #141789, #3283, #87109, #131615, #52763, #10285, #7255, #55772, #114432, #176133, #179145, #40613, #130604, #68940, #71943, #178136, #116448, #133613, #162952, #38614, #144773, #194306, #6258, #39603, #159950, #100271, #83098, #147799, #37603, #115453, #102283, #67938, #24458, #177143, #99266, #146778, #192299, #101262, #21438, #163972, #23446, #86108, #22445, #69950, #25469, #98248, #70949, #129591, #8272, #148795, #56788, #195307, #191287, #160952, #193299, #175125, #161951, #53778, #36592, #9284, #84095, #145774, #85093, #117446, #132619, #54774, #164965, #88101, #78643, #13267, #156491, #182116, #171665, #26458, #106250, #151774, #149786, #89102, #140318, #29432, #94813, #17993, #74930, #58756, #183112, #103285, #119456, #79646, #105267, #181140, #141315, #198273, #165960, #2804, #11289, #120425, #41621, #118460, #33154, #109985, #136593, #42614, #72962, #91063, #150793, #180152, #134631, #104278, #196316, #43602, #167932, #59750, #63486, #57785, #27461, #12289, #73954, #121420, #152750, #135622, #44594, #197293, #166953, #28456, #48330, #90092, #14240, #1808, #125162, #186861, #142307, #37115, #157491, #65464, #190810, #83610, #127127, #145288, #21959, #6771, #130104, #144289, #128123, #159455, #3787, #35132, #143287, #172659, #52284, #188833, #95805, #66460, #50318, #189825, #34146, #97768, #18984, #51297, #175641, #112958, #80630, #160468, #110974, #5779, #111973, #173665, #98774, #68450, #64482, #174651, #96784, #158473, #36116, #126149, #67453, #187845, #113942, #81603, #20951, #82608, #129111, #49314, #19961, #4773, #15646, #61137, #47980, #184499, #92466, #126772, #42268, #156135, #1449, #168328, #31809, #107633, #154154, #3438, #93460, #64132, #95450, #123790, #138974, #14650, #48965, #2450, #46979, #16639, #122809, #124806, #106655, #29824, #91460, #17634, #172301, #157135, #186504, #32803, #33790, #63127, #153148, #109633, #76310, #125797, #77305, #141948, #18630, #80277, #137988, #79294, #78286, #171316, #169311, #62127, #170316, #199671 ),
 ( #94455, #452, #45979, #30817, #185489, #140963, #187499, #110619, #65114, #108638, #155146, #139959, #161112, #68098, #69100, #6417, #49957, #4419, #22608, #159103, #146950, #114599, #115617, #145935, #21602, #83260, #84254, #67104, #23612, #176296, #144935, #70111, #34780, #82249, #37768, #99430, #7417, #20597, #97416, #100434, #129750, #66106, #85258, #143940, #130767, #127772, #189472, #192459, #53942, #5421, #128763, #8439, #191447, #52923, #188476, #177306, #51935, #158123, #38778, #19614, #162115, #173306, #113595, #96436, #111621, #50950, #190462, #81257, #142938, #112609, #175289, #174301, #160114, #36754, #35770, #98418, #120588, #180313, #196476, #179310, #26618, #182282, #54939, #27626, #24621, #165126, #197454, #13421, #58920, #86269, #101426, #149948, #90249, #72106, #87273, #167110, #166124, #132777, #28611, #39763, #150957, #89265, #148957, #194464, #151932, #163118, #12451, #74113, #10446, #178299, #147959, #135783, #88261, #131780, #195472, #43763, #9446, #119617, #11454, #71111, #102443, #105427, #42778, #193462, #116611, #73126, #133779, #57946, #55935, #117610, #40774, #118622, #164130, #25628, #134795, #56948, #41781, #103447, #181300, #104440, #32678, #93335, #63001, #15524, #185362, #124678, #80155, #140834, #3319, #187373, #31686, #171189, #109507, #79164, #61015, #110496, #169186, #186375, #47854, #48842, #155020, #188353, #2323, #94331, #34656, #199545, #46854, #64005, #125675, #172178, #108513, #61999, #64992, #156009, #30693, #49831, #170192, #33663, #92343, #154029, #157009, #18507, #16516, #78164, #111495, #17506, #95325, #173180, #141826, #139832, #122687, #126650, #184376, #153025, #137865, #1321, #45857, #14525, #77181, #76185, #107510, #138851, #331, #123665, #20473, #67975, #128640, #99305, #81138, #85134, #144813, #160990, #143816, #191324, #146818, #19493, #192337, #189350, #129629, #161989, #178177, #23485, #50828, #65981, #114469, #54813, #36631, #51811, #131657, #130643, #158001, #142819, #97295, #116488, #159990, #84132, #52802, #38654, #4299, #112485, #174178, #193339, #176172, #145811, #127651, #22484, #35648, #21476, #96315, #8313, #158981, #7294, #68978, #82123, #5297, #66980, #69989, #190334, #113470, #115493, #175165, #98288, #83137, #6296, #37641, #53818, #177181, #100311, #104315, #102321, #56825, #165003, #70990, #120463, #164011, #132658, #149823, #10324, #73000, #194346, #165998, #55814, #134668, #43639, #196354, #117486, #28492, #147839, #150829, #25507, #179184, #101303, #119494, #180190, #11329, #87151, #71980, #57822, #166989, #27499, #90126, #73991, #118499, #181176, #42653, #89141, #41660, #151810, #59788, #13301, #40652, #12326, #148834, #133654, #121456, #39642, #135660, #197332, #162992, #26497, #195345, #103323, #198309, #88139, #58795, #74966, #182154, #105302, #9325, #136628, #24497, #86148, #154782, #199308, #62759, #183148, #64764, #44633, #155773, #110264, #33434, #124440, #170948, #171945, #1084, #106285, #186136, #167970, #140601, #29469, #91102, #95093, #156782, #139598, #184139, #137624, #17271, #153786, #14281, #16279, #187140, #77931, #60775, #18275, #152790, #94094, #107273, #122447, #75950, #47615, #123430, #93098, #45621, #15281, #109269, #79928, #32440, #141601, #78924, #61762, #2091, #63771, #125444, #92, #3088, #168944, #30451, #92098, #48612, #76941, #138610, #185123, #46613, #108275, #169953, #31444, #113242, #189125, #35415, #84894, #174933, #145578, #176944, #5061, #20238, #96087, #130395, #83895, #128406, #98050, #142590, #6064, #126427, #8067, #188124, #99066, #53575, #38414, #67742, #114231, #115252, #144577, #49595, #129400, #111258, #7055, #172950, #34428, #100071, #161756, #82899, #127415, #80913, #160754, #97067, #157776, #19267, #50597, #146573, #190103, #175936, #159749, #68737, #4070, #65747, #112256, #23251, #191096, #37408, #173948, #52571, #158749, #51578, #81886, #143578, #66746, #22246 ),
 ( #36396, #192092, #21245, #134431, #132420, #86910, #195103, #101066, #150597, #194112, #162751, #179950, #40411, #103083, #24259, #196117, #27256, #85910, #164764, #26259, #104080, #148593, #105075, #57587, #87900, #151584, #116247, #163767, #119257, #180941, #88906, #102083, #178941, #181924, #149586, #147597, #166761, #25267, #12095, #9082, #70752, #73758, #135430, #10085, #71743, #28263, #72760, #11084, #89901, #42417, #133414, #39406, #197101, #55575, #165762, #54575, #56585, #177939, #58568, #117249, #118260, #120233, #41417, #43405, #69744, #131413, #193100, #45391, #16048, #198081, #1859, #61536, #77707, #60539, #108036, #63541, #136403, #109042, #106056, #46377, #78695, #94866, #140372, #167742, #182917, #31215, #171718, #153553, #168716, #48382, #47387, #14046, #110039, #121226, #32212, #170720, #30218, #59548, #44402, #93868, #169722, #33207, #76711, #125215, #29240, #855, #92866, #90873, #183906, #155547, #124202, #186911, #13073, #154553, #15050, #139373, #152557, #75712, #74740, #200068, #137390, #199070, #62529, #122215, #107044, #91860, #185902, #138386, #123205, #184895, #17041, #129164, #52338, #5831, #190861, #36167, #37167, #174703, #18046, #172714, #113994, #127178, #141370, #64535, #21004, #19036, #173718, #81656, #187897, #98826, #80683, #49364, #66514, #188888, #189875, #111028, #82659, #34197, #51350, #160520, #113010, #95859, #145341, #126201, #67507, #142359, #157542, #79699, #97819, #96840, #128176, #3839, #50369, #159508, #83663, #144343, #6823, #175692, #35186, #22011, #68501, #130156, #158525, #191853, #176707, #53334, #65518, #115013, #112029, #20013, #38181, #156547, #2857, #143339, #4826, #86672, #162514, #8846, #61049, #148355, #121730, #153060, #178704, #193873, #69510, #106563, #60062, #101842, #71510, #116016, #179713, #99837, #184411, #161521, #75236, #29736, #14562, #41185, #87671, #91369, #118023, #23013, #102848, #84659, #183422, #146337, #7825, #76220, #137899, #56341, #100831, #54345, #136907, #70514, #131176, #192866, #24016, #122721, #163528, #152084, #133178, #44906, #177706, #39173, #85671, #199581, #164533, #13569, #147358, #26026, #132182, #25028, #55339, #117009, #40166, #198594, #168240, #9851, #194868, #46889, #111531, #62036, #31721, #65028, #19527, #93369, #142854, #158036, #81172, #127685, #157046, #17541, #30730, #34692, #94365, #110533, #155056, #140871, #96349, #169221, #141862, #138885, #79202, #173216, #45892, #4333, #365, #15558, #64041, #66017, #186412, #1357, #107545, #80190, #108549, #92377, #154063, #126684, #3353, #63036, #77216, #123700, #188388, #2360, #185398, #109542, #170228, #16551, #33698, #125711, #78198, #139868, #49865, #18543, #124714, #47889, #187410, #171224, #172214, #32713, #156044, #48878, #95361, #51847, #147872, #69011, #36666, #71023, #82157, #115528, #9358, #129662, #67016, #53854, #162024, #85166, #38689, #23520, #130677, #70022, #7327, #50862, #5332, #146854, #160025, #174214, #97330, #8347, #128675, #22518, #84165, #131691, #68010, #24531, #177216, #145845, #189385, #35682, #83173, #100345, #193372, #54848, #21512, #98325, #101336, #192371, #190372, #86182, #144847, #116522, #113506, #175201, #178210, #39674, #6330, #191358, #112520, #163025, #159016, #20509, #143853, #52836, #114505, #176207, #37676, #99341, #161024, #196387, #40684, #105334, #72015, #73032, #198344, #25542, #182187, #134704, #56859, #104348, #165036, #135692, #27532, #14316, #179218, #26529, #43672, #120496, #151842, #88173, #41693, #44664, #89173, #10358, #168003, #149857, #13332, #133688, #195381, #136662, #59818, #11362, #57856, #29499, #197364, #74022, #91132, #167022, #119528, #102354, #74997, #164043, #58829, #117520, #181211, #87186, #28523, #118534, #42687, #121488, #148867, #90159, #166032, #180223, #150865, #12359, #183182, #103358, #106317, #152822, #132691, #194379, #55846, #64796, #199341, #171978, #168975, #109301, #141631 ),
 ( #92131, #61793, #95124, #49628, #123463, #172980, #188155, #111291, #157805, #187173, #47650, #140632, #138643, #93128, #1116, #107303, #156814, #124, #30480, #186168, #46645, #170980, #153818, #2122, #15313, #32473, #79962, #94126, #76972, #126457, #184170, #48644, #185155, #108305, #137654, #155805, #16311, #17303, #169985, #31476, #78957, #3121, #63804, #34458, #110296, #154813, #125477, #33466, #18306, #77961, #96117, #75981, #60806, #139628, #122479, #62790, #124471, #45652, #101096, #4098, #20268, #54604, #6095, #81914, #177968, #99098, #66774, #19296, #112286, #145610, #39436, #159780, #97096, #83929, #192127, #115284, #68770, #53608, #160790, #100102, #37438, #80944, #35444, #176977, #190132, #65777, #127446, #38447, #158780, #52603, #114265, #161786, #98082, #116278, #7089, #175969, #142619, #189152, #113271, #130428, #23281, #84925, #51607, #128435, #131444, #22278, #143607, #50625, #174963, #146605, #5091, #36427, #8098, #69776, #21275, #82932, #173976, #193131, #144610, #67774, #129431, #191129, #132451, #181955, #194142, #27291, #147628, #26292, #70783, #135461, #102114, #103116, #28293, #55606, #12125, #164797, #86943, #134463, #195137, #165794, #9116, #151614, #11118, #88938, #10117, #57620, #13106, #85939, #58597, #117280, #196148, #89933, #44432, #74771, #178974, #40441, #180971, #121255, #87933, #118292, #198114, #197130, #163799, #59581, #25301, #43437, #120263, #179983, #148627, #71777, #105106, #119288, #182949, #149620, #136433, #133447, #150629, #42448, #56618, #41451, #166792, #73789, #162782, #24290, #104112, #72793, #170750, #91890, #167772, #107072, #171748, #122244, #153581, #125243, #79729, #15079, #2886, #18074, #141398, #187925, #17070, #77735, #32239, #168743, #123232, #31245, #137421, #186941, #30247, #199101, #16077, #76740, #139401, #60568, #93897, #183934, #883, #110068, #62558, #45419, #94895, #14078, #78724, #138415, #200095, #29270, #185930, #46407, #124234, #61563, #184923, #47415, #33237, #155575, #156579, #140400, #108066, #109071, #1888, #63569, #169750, #64565, #126230, #106086, #92895, #48412, #154581, #90901, #152587, #75744, #160553, #5861, #172745, #36196, #112058, #158552, #7856, #157571, #161551, #67537, #127206, #84689, #81685, #130188, #188920, #50398, #53368, #115046, #4859, #143367, #146369, #52369, #190893, #69543, #37202, #113041, #19064, #68533, #80711, #114026, #34226, #174733, #142389, #22043, #173746, #189905, #176738, #3868, #98858, #51380, #35215, #21037, #66544, #175723, #95888, #38211, #97850, #83694, #96868, #144374, #99867, #65547, #145372, #20042, #82690, #23044, #131207, #49394, #128208, #159539, #129195, #111057, #6854, #191884, #180742, #43204, #27056, #71540, #10879, #149383, #119060, #9880, #104871, #12876, #120036, #8877, #195912, #132213, #40196, #74541, #192898, #103879, #72549, #116047, #179744, #55368, #101876, #54375, #39205, #57387, #177736, #133206, #86701, #162543, #196902, #150398, #194897, #164560, #70545, #134227, #100861, #24047, #85703, #165559, #181722, #166560, #42218, #88702, #28059, #11894, #147389, #73557, #193904, #135230, #117038, #178733, #89700, #151386, #58369, #163558, #25058, #148386, #56371, #118054, #41214, #102875, #26054, #87698, #123991, #169514, #78490, #121018, #90682, #29042, #171517, #154352, #185689, #44201, #651, #105860, #61336, #156340, #63333, #167547, #62321, #108838, #122018, #197881, #137190, #1655, #152364, #183709, #155350, #109834, #45195, #33006, #48178, #94661, #17840, #47179, #107830, #170519, #198877, #153349, #123007, #13849, #16840, #60344, #75516, #46177, #106849, #31014, #168524, #32008, #30022, #92664, #140163, #15845, #91660, #125011, #14851, #93665, #76513, #138189, #59350, #77504, #199872, #139175, #184693, #186707, #136206, #182716, #175491, #172511, #112808, #145139, #161319, #6622, #33996, #49168, #97615, #37979, #19813, #34983, #114810, #113796, #80480 ),
 ( #67304, #174501, #187698, #50164, #98625, #190663, #53131, #176502, #35968, #81454, #144143, #64333, #142154, #99636, #66311, #3638, #79498, #159305, #126975, #141167, #95652, #5627, #2656, #143140, #157340, #128963, #52139, #36964, #160319, #21810, #20800, #83462, #82455, #126001, #18835, #68301, #111822, #110827, #65316, #129952, #188684, #191652, #173510, #96636, #158324, #4620, #127972, #189675, #51147, #69306, #116812, #72316, #10653, #162316, #11663, #130972, #135001, #179515, #100635, #58148, #55141, #103655, #23817, #85467, #26825, #88466, #178503, #39969, #119816, #25832, #164337, #181501, #133992, #86476, #192663, #41989, #54146, #87476, #7622, #148161, #115819, #195683, #147156, #163330, #150163, #177509, #57154, #24826, #8644, #194672, #101639, #149163, #38979, #73329, #71318, #118833, #70318, #117822, #196679, #146136, #165333, #131985, #193670, #42979, #104644, #9652, #132981, #22812, #180516, #84458, #56141, #40983, #102652, #135983, #185450, #197654, #30781, #151161, #29788, #74316, #138934, #105629, #106618, #31771, #59120, #15608, #168292, #90454, #137950, #198648, #169275, #12649, #155106, #14615, #92428, #13621, #61100, #16599, #89470, #62088, #120786, #199633, #93419, #47943, #78247, #182486, #43967, #184463, #124767, #91424, #121782, #1409, #414, #167318, #63088, #28814, #46940, #123751, #183476, #152138, #75288, #108600, #122773, #186465, #153111, #139920, #136959, #154114, #45942, #60114, #44960, #170277, #77265, #166331, #27829, #107597, #76272, #177017, #94417, #110582, #147668, #96400, #172263, #70822, #192168, #157097, #194180, #2412, #38486, #132491, #49917, #187460, #100143, #84963, #8139, #161824, #146645, #53648, #193170, #130471, #171277, #125760, #69816, #80241, #156097, #17595, #131483, #48928, #142903, #7129, #54642, #188438, #9156, #23319, #68812, #109594, #79254, #3402, #116317, #178006, #33753, #101134, #140926, #24329, #115326, #95412, #32765, #141911, #39473, #111582, #64092, #162820, #85979, #18593, #65077, #126735, #173267, #34741, #158087, #19579, #81222, #167807, #12163, #133484, #90937, #87972, #136469, #195176, #56657, #59619, #121292, #11158, #149660, #152624, #58634, #197169, #14114, #43475, #119327, #25340, #74807, #86981, #120300, #40481, #181013, #163839, #28330, #118330, #196188, #182985, #148668, #105143, #57660, #180023, #27329, #72832, #181993, #102153, #44469, #104150, #166829, #103155, #150665, #106123, #179013, #151649, #10156, #88975, #29307, #137459, #75781, #71816, #41491, #73828, #55644, #42487, #134502, #117317, #89969, #164836, #26332, #165832, #198149, #13144, #135498, #45455, #168779, #156615, #93932, #34263, #62592, #49431, #107109, #186977, #32275, #30282, #169786, #18110, #110104, #172782, #95922, #155611, #139436, #63604, #183968, #200129, #157607, #185966, #61598, #19098, #78758, #46442, #80747, #91927, #125280, #199138, #918, #76776, #48447, #171783, #94930, #33271, #79764, #140435, #141435, #17106, #60605, #15115, #2922, #31279, #153619, #138448, #64600, #123267, #1925, #126264, #184958, #187961, #108102, #124270, #122280, #111092, #92930, #154617, #16111, #77769, #47450, #109106, #170785, #158587, #128241, #161583, #116079, #189938, #39236, #54407, #177767, #24080, #53401, #114062, #6887, #4894, #159575, #67571, #173783, #23077, #66576, #35250, #52403, #113073, #175760, #96903, #68565, #20076, #37236, #146400, #98892, #81720, #131241, #50434, #115079, #51413, #143406, #3904, #22075, #82728, #160586, #174765, #36231, #83726, #69575, #130222, #192929, #176771, #21072, #145405, #191918, #38243, #144409, #100892, #162576, #142425, #97883, #99898, #5895, #129229, #65584, #127244, #84722, #7890, #188957, #190926, #112093, #9913, #85735, #132245, #180774, #8909, #179777, #56406, #55400, #58401, #73589, #41246, #10911, #40232, #57419, #147422, #70577, #117070, #135261, #166592, #89731, #103910, #11925, #151417, #42249 ) ),
 .UNSPECIFIED., .T., .F., .F. ) 
 B_SPLINE_SURFACE_WITH_KNOTS ( ( 4, 3, 4 ),
 ( 3, 2, 2, 2, 2, 2, 2, 2, 2, 2, 2, 2, 2, 2, 2, 2, 2, 2, 2, 2, 2, 2, 2, 2, 2, 2, 2, 2, 2, 2, 2, 2, 2, 2, 2, 2, 2, 2, 2, 2, 2, 2, 2, 2, 2, 2, 2, 2, 2, 2, 2, 2, 2, 2, 2, 2, 2, 2, 2, 2, 2, 2, 2, 2, 2, 2, 2, 2, 2, 2, 2, 2, 2, 2, 2, 2, 2, 2, 2, 2, 2, 2, 2, 2, 2, 2, 2, 2, 2, 2, 2, 2, 2, 2, 2, 2, 2, 2, 2, 2, 2, 2, 2, 2, 2, 2, 2, 2, 2, 2, 2, 2, 2, 2, 2, 2, 2, 2, 2, 2, 2, 2, 2, 2, 2, 2, 2, 2, 2, 2, 2, 2, 2, 2, 2, 2, 2, 2, 2, 2, 2, 2, 2, 2, 2, 2, 2, 2, 2, 2, 2, 2, 2, 2, 2, 2, 2, 2, 2, 2, 2, 2, 2, 2, 2, 2, 2, 2, 2, 2, 2, 2, 2, 2, 2, 2, 2, 2, 2, 2, 2, 2, 2, 2, 2, 2, 2, 2, 2, 2, 2, 2, 2, 2, 2, 2, 2, 2, 2, 2, 2, 2, 2, 2, 2, 2, 2, 2, 2, 2, 2, 2, 2, 2, 2, 2, 2, 2, 2, 2, 2, 2, 2, 2, 2, 2, 2, 2, 3 ),
 ( 0.000000000000000000, 0.5000000000000000000, 1.000000000000000000 ),
 ( 0.000000000000000000, 0.004385964912280701511, 0.008771929824561403022, 0.01315789473684210453, 0.01754385964912280604, 0.02192982456140350755, 0.02631578947368420907, 0.03070175438596491058, 0.03508771929824561209, 0.03947368421052631360, 0.04385964912280701511, 0.04824561403508771662, 0.05263157894736841813, 0.05701754385964911964, 0.06140350877192982115, 0.06578947368421052266, 0.07017543859649122417, 0.07456140350877192569, 0.07894736842105262720, 0.08333333333333332871, 0.08771929824561403022, 0.09210526315789473173, 0.09649122807017543324, 0.1008771929824561348, 0.1052631578947368363, 0.1096491228070175378, 0.1140350877192982393, 0.1184210526315789408, 0.1228070175438596423, 0.1271929824561403577, 0.1315789473684210453, 0.1359649122807017607, 0.1403508771929824483, 0.1447368421052631637, 0.1491228070175438514, 0.1535087719298245668, 0.1578947368421052544, 0.1622807017543859698, 0.1666666666666666574, 0.1710526315789473728, 0.1754385964912280604, 0.1798245614035087758, 0.1842105263157894635, 0.1885964912280701788, 0.1929824561403508665, 0.1973684210526315819, 0.2017543859649122695, 0.2061403508771929849, 0.2105263157894736725, 0.2149122807017543879, 0.2192982456140350755, 0.2236842105263157909, 0.2280701754385964786, 0.2324561403508771940, 0.2368421052631578816, 0.2412280701754385970, 0.2456140350877192846, 0.2500000000000000000, 0.2543859649122807154, 0.2587719298245614308, 0.2631578947368420907, 0.2675438596491228060, 0.2719298245614035214, 0.2763157894736842368, 0.2807017543859648967, 0.2850877192982456121, 0.2894736842105263275, 0.2938596491228070429, 0.2982456140350877027, 0.3026315789473684181, 0.3070175438596491335, 0.3114035087719298489, 0.3157894736842105088, 0.3201754385964912242, 0.3245614035087719396, 0.3289473684210526550, 0.3333333333333333148, 0.3377192982456140302, 0.3421052631578947456, 0.3464912280701754610, 0.3508771929824561209, 0.3552631578947368363, 0.3596491228070175517, 0.3640350877192982670, 0.3684210526315789269, 0.3728070175438596423, 0.3771929824561403577, 0.3815789473684210731, 0.3859649122807017330, 0.3903508771929824483, 0.3947368421052631637, 0.3991228070175438791, 0.4035087719298245390, 0.4078947368421052544, 0.4122807017543859698, 0.4166666666666666852, 0.4210526315789473450, 0.4254385964912280604, 0.4298245614035087758, 0.4342105263157894912, 0.4385964912280701511, 0.4429824561403508665, 0.4473684210526315819, 0.4517543859649122973, 0.4561403508771929571, 0.4605263157894736725, 0.4649122807017543879, 0.4692982456140351033, 0.4736842105263157632, 0.4780701754385964786, 0.4824561403508771940, 0.4868421052631579093, 0.4912280701754385692, 0.4956140350877192846, 0.5000000000000000000, 0.5043859649122807154, 0.5087719298245614308, 0.5131578947368421462, 0.5175438596491228616, 0.5219298245614034659, 0.5263157894736841813, 0.5307017543859648967, 0.5350877192982456121, 0.5394736842105263275, 0.5438596491228070429, 0.5482456140350877583, 0.5526315789473684736, 0.5570175438596490780, 0.5614035087719297934, 0.5657894736842105088, 0.5701754385964912242, 0.5745614035087719396, 0.5789473684210526550, 0.5833333333333333703, 0.5877192982456140857, 0.5921052631578946901, 0.5964912280701754055, 0.6008771929824561209, 0.6052631578947368363, 0.6096491228070175517, 0.6140350877192982670, 0.6184210526315789824, 0.6228070175438596978, 0.6271929824561403022, 0.6315789473684210176, 0.6359649122807017330, 0.6403508771929824483, 0.6447368421052631637, 0.6491228070175438791, 0.6535087719298245945, 0.6578947368421053099, 0.6622807017543859143, 0.6666666666666666297, 0.6710526315789473450, 0.6754385964912280604, 0.6798245614035087758, 0.6842105263157894912, 0.6885964912280702066, 0.6929824561403509220, 0.6973684210526315264, 0.7017543859649122417, 0.7061403508771929571, 0.7105263157894736725, 0.7149122807017543879, 0.7192982456140351033, 0.7236842105263158187, 0.7280701754385965341, 0.7324561403508771384, 0.7368421052631578538, 0.7412280701754385692, 0.7456140350877192846, 0.7500000000000000000, 0.7543859649122807154, 0.7587719298245614308, 0.7631578947368421462, 0.7675438596491228616, 0.7719298245614034659, 0.7763157894736841813, 0.7807017543859648967, 0.7850877192982456121, 0.7894736842105263275, 0.7938596491228070429, 0.7982456140350877583, 0.8026315789473684736, 0.8070175438596490780, 0.8114035087719297934, 0.8157894736842105088, 0.8201754385964912242, 0.8245614035087719396, 0.8289473684210526550, 0.8333333333333333703, 0.8377192982456140857, 0.8421052631578946901, 0.8464912280701754055, 0.8508771929824561209, 0.8552631578947368363, 0.8596491228070175517, 0.8640350877192982670, 0.8684210526315789824, 0.8728070175438596978, 0.8771929824561403022, 0.8815789473684210176, 0.8859649122807017330, 0.8903508771929824483, 0.8947368421052631637, 0.8991228070175438791, 0.9035087719298245945, 0.9078947368421053099, 0.9122807017543859143, 0.9166666666666666297, 0.9210526315789473450, 0.9254385964912280604, 0.9298245614035087758, 0.9342105263157894912, 0.9385964912280702066, 0.9429824561403509220, 0.9473684210526315264, 0.9517543859649122417, 0.9561403508771929571, 0.9605263157894736725, 0.9649122807017543879, 0.9692982456140351033, 0.9736842105263158187, 0.9780701754385965341, 0.9824561403508771384, 0.9868421052631578538, 0.9912280701754385692, 0.9956140350877192846, 1.000000000000000000 ),
 .UNSPECIFIED. ) 
 GEOMETRIC_REPRESENTATION_ITEM ( )  RATIONAL_B_SPLINE_SURFACE ( (
 ( 1.000000000000000000, 0.9659258262890683122, 1.000000000000000000, 0.9659258262890683122, 1.000000000000000000, 0.9659258262890683122, 1.000000000000000000, 0.9659258262890683122, 1.000000000000000000, 0.9659258262890683122, 1.000000000000000000, 0.9659258262890683122, 1.000000000000000000, 0.9659258262890683122, 1.000000000000000000, 0.9659258262890683122, 1.000000000000000000, 0.9659258262890683122, 1.000000000000000000, 0.9659258262890683122, 1.000000000000000000, 0.9659258262890683122, 1.000000000000000000, 0.9659258262890683122, 1.000000000000000000, 0.9659258262890683122, 1.000000000000000000, 0.9659258262890683122, 1.000000000000000000, 0.9659258262890683122, 1.000000000000000000, 0.9659258262890683122, 1.000000000000000000, 0.9659258262890683122, 1.000000000000000000, 0.9659258262890683122, 1.000000000000000000, 0.9659258262890683122, 1.000000000000000000, 0.9659258262890683122, 1.000000000000000000, 0.9659258262890683122, 1.000000000000000000, 0.9659258262890683122, 1.000000000000000000, 0.9659258262890683122, 1.000000000000000000, 0.9659258262890683122, 1.000000000000000000, 0.9659258262890683122, 1.000000000000000000, 0.9659258262890683122, 1.000000000000000000, 0.9659258262890683122, 1.000000000000000000, 0.9659258262890683122, 1.000000000000000000, 0.9659258262890683122, 1.000000000000000000, 0.9659258262890683122, 1.000000000000000000, 0.9659258262890683122, 1.000000000000000000, 0.9659258262890683122, 1.000000000000000000, 0.9659258262890683122, 1.000000000000000000, 0.9659258262890683122, 1.000000000000000000, 0.9659258262890683122, 1.000000000000000000, 0.9659258262890683122, 1.000000000000000000, 0.9659258262890683122, 1.000000000000000000, 0.9659258262890683122, 1.000000000000000000, 0.9659258262890683122, 1.000000000000000000, 0.9659258262890683122, 1.000000000000000000, 0.9659258262890683122, 1.000000000000000000, 0.9659258262890683122, 1.000000000000000000, 0.9659258262890683122, 1.000000000000000000, 0.9659258262890683122, 1.000000000000000000, 0.9659258262890683122, 1.000000000000000000, 0.9659258262890683122, 1.000000000000000000, 0.9659258262890683122, 1.000000000000000000, 0.9659258262890683122, 1.000000000000000000, 0.9659258262890683122, 1.000000000000000000, 0.9659258262890683122, 1.000000000000000000, 0.9659258262890683122, 1.000000000000000000, 0.9659258262890683122, 1.000000000000000000, 0.9659258262890683122, 1.000000000000000000, 0.9659258262890683122, 1.000000000000000000, 0.9659258262890683122, 1.000000000000000000, 0.9659258262890683122, 1.000000000000000000, 0.9659258262890683122, 1.000000000000000000, 0.9659258262890683122, 1.000000000000000000, 0.9659258262890683122, 1.000000000000000000, 0.9659258262890683122, 1.000000000000000000, 0.9659258262890683122, 1.000000000000000000, 0.9659258262890683122, 1.000000000000000000, 0.9659258262890683122, 1.000000000000000000, 0.9659258262890683122, 1.000000000000000000, 0.9659258262890683122, 1.000000000000000000, 0.9659258262890683122, 1.000000000000000000, 0.9659258262890683122, 1.000000000000000000, 0.9659258262890683122, 1.000000000000000000, 0.9659258262890683122, 1.000000000000000000, 0.9659258262890683122, 1.000000000000000000, 0.9659258262890683122, 1.000000000000000000, 0.9659258262890683122, 1.000000000000000000, 0.9659258262890683122, 1.000000000000000000, 0.9659258262890683122, 1.000000000000000000, 0.9659258262890683122, 1.000000000000000000, 0.9659258262890683122, 1.000000000000000000, 0.9659258262890683122, 1.000000000000000000, 0.9659258262890683122, 1.000000000000000000, 0.9659258262890683122, 1.000000000000000000, 0.9659258262890683122, 1.000000000000000000, 0.9659258262890683122, 1.000000000000000000, 0.9659258262890683122, 1.000000000000000000, 0.9659258262890683122, 1.000000000000000000, 0.9659258262890683122, 1.000000000000000000, 0.9659258262890683122, 1.000000000000000000, 0.9659258262890683122, 1.000000000000000000, 0.9659258262890683122, 1.000000000000000000, 0.9659258262890683122, 1.000000000000000000, 0.9659258262890683122, 1.000000000000000000, 0.9659258262890683122, 1.000000000000000000, 0.9659258262890683122, 1.000000000000000000, 0.9659258262890683122, 1.000000000000000000, 0.9659258262890683122, 1.000000000000000000, 0.9659258262890683122, 1.000000000000000000, 0.9659258262890683122, 1.000000000000000000, 0.9659258262890683122, 1.000000000000000000, 0.9659258262890683122, 1.000000000000000000, 0.9659258262890683122, 1.000000000000000000, 0.9659258262890683122, 1.000000000000000000, 0.9659258262890683122, 1.000000000000000000, 0.9659258262890683122, 1.000000000000000000, 0.9659258262890683122, 1.000000000000000000, 0.9659258262890683122, 1.000000000000000000, 0.9659258262890683122, 1.000000000000000000, 0.9659258262890683122, 1.000000000000000000, 0.9659258262890683122, 1.000000000000000000, 0.9659258262890683122, 1.000000000000000000, 0.9659258262890683122, 1.000000000000000000, 0.9659258262890683122, 1.000000000000000000, 0.9659258262890683122, 1.000000000000000000, 0.9659258262890683122, 1.000000000000000000, 0.9659258262890683122, 1.000000000000000000, 0.9659258262890683122, 1.000000000000000000, 0.9659258262890683122, 1.000000000000000000, 0.9659258262890683122, 1.000000000000000000, 0.9659258262890683122, 1.000000000000000000, 0.9659258262890683122, 1.000000000000000000, 0.9659258262890683122, 1.000000000000000000, 0.9659258262890683122, 1.000000000000000000, 0.9659258262890683122, 1.000000000000000000, 0.9659258262890683122, 1.000000000000000000, 0.9659258262890683122, 1.000000000000000000, 0.9659258262890683122, 1.000000000000000000, 0.9659258262890683122, 1.000000000000000000, 0.9659258262890683122, 1.000000000000000000, 0.9659258262890683122, 1.000000000000000000, 0.9659258262890683122, 1.000000000000000000, 0.9659258262890683122, 1.000000000000000000, 0.9659258262890683122, 1.000000000000000000, 0.9659258262890683122, 1.000000000000000000, 0.9659258262890683122, 1.000000000000000000, 0.9659258262890683122, 1.000000000000000000, 0.9659258262890683122, 1.000000000000000000, 0.9659258262890683122, 1.000000000000000000, 0.9659258262890683122, 1.000000000000000000, 0.9659258262890683122, 1.000000000000000000, 0.9659258262890683122, 1.000000000000000000, 0.9659258262890683122, 1.000000000000000000, 0.9659258262890683122, 1.000000000000000000, 0.9659258262890683122, 1.000000000000000000, 0.9659258262890683122, 1.000000000000000000, 0.9659258262890683122, 1.000000000000000000, 0.9659258262890683122, 1.000000000000000000, 0.9659258262890683122, 1.000000000000000000, 0.9659258262890683122, 1.000000000000000000, 0.9659258262890683122, 1.000000000000000000, 0.9659258262890683122, 1.000000000000000000, 0.9659258262890683122, 1.000000000000000000, 0.9659258262890683122, 1.000000000000000000, 0.9659258262890683122, 1.000000000000000000, 0.9659258262890683122, 1.000000000000000000, 0.9659258262890683122, 1.000000000000000000, 0.9659258262890683122, 1.000000000000000000, 0.9659258262890683122, 1.000000000000000000, 0.9659258262890683122, 1.000000000000000000, 0.9659258262890683122, 1.000000000000000000, 0.9659258262890683122, 1.000000000000000000, 0.9659258262890683122, 1.000000000000000000, 0.9659258262890683122, 1.000000000000000000, 0.9659258262890683122, 1.000000000000000000, 0.9659258262890683122, 1.000000000000000000, 0.9659258262890683122, 1.000000000000000000, 0.9659258262890683122, 1.000000000000000000, 0.9659258262890683122, 1.000000000000000000, 0.9659258262890683122, 1.000000000000000000, 0.9659258262890683122, 1.000000000000000000, 0.9659258262890683122, 1.000000000000000000, 0.9659258262890683122, 1.000000000000000000, 0.9659258262890683122, 1.000000000000000000, 0.9659258262890683122, 1.000000000000000000, 0.9659258262890683122, 1.000000000000000000, 0.9659258262890683122, 1.000000000000000000, 0.9659258262890683122, 1.000000000000000000, 0.9659258262890683122, 1.000000000000000000, 0.9659258262890683122, 1.000000000000000000, 0.9659258262890683122, 1.000000000000000000, 0.9659258262890683122, 1.000000000000000000, 0.9659258262890683122, 1.000000000000000000, 0.9659258262890683122, 1.000000000000000000, 0.9659258262890683122, 1.000000000000000000, 0.9659258262890683122, 1.000000000000000000, 0.9659258262890683122, 1.000000000000000000, 0.9659258262890683122, 1.000000000000000000, 0.9659258262890683122, 1.000000000000000000, 0.9659258262890683122, 1.000000000000000000, 0.9659258262890683122, 1.000000000000000000, 0.9659258262890683122, 1.000000000000000000, 0.9659258262890683122, 1.000000000000000000, 0.9659258262890683122, 1.000000000000000000, 0.9659258262890683122, 1.000000000000000000, 0.9659258262890683122, 1.000000000000000000, 0.9659258262890683122, 1.000000000000000000, 0.9659258262890683122, 1.000000000000000000, 0.9659258262890683122, 1.000000000000000000, 0.9659258262890683122, 1.000000000000000000, 0.9659258262890683122, 1.000000000000000000, 0.9659258262890683122, 1.000000000000000000, 0.9659258262890683122, 1.000000000000000000, 0.9659258262890683122, 1.000000000000000000, 0.9659258262890683122, 1.000000000000000000, 0.9659258262890683122, 1.000000000000000000, 0.9659258262890683122, 1.000000000000000000, 0.9659258262890683122, 1.000000000000000000, 0.9659258262890683122, 1.000000000000000000, 0.9659258262890683122, 1.000000000000000000, 0.9659258262890683122, 1.000000000000000000, 0.9659258262890683122, 1.000000000000000000, 0.9659258262890683122, 1.000000000000000000, 0.9659258262890683122, 1.000000000000000000, 0.9659258262890683122, 1.000000000000000000, 0.9659258262890683122, 1.000000000000000000, 0.9659258262890683122, 1.000000000000000000, 0.9659258262890683122, 1.000000000000000000, 0.9659258262890683122, 1.000000000000000000, 0.9659258262890683122, 1.000000000000000000, 0.9659258262890683122, 1.000000000000000000, 0.9659258262890683122, 1.000000000000000000, 0.9659258262890683122, 1.000000000000000000, 0.9659258262890683122, 1.000000000000000000, 0.9659258262890683122, 1.000000000000000000, 0.9659258262890683122, 1.000000000000000000, 0.9659258262890683122, 1.000000000000000000, 0.9659258262890683122, 1.000000000000000000, 0.9659258262890683122, 1.000000000000000000, 0.9659258262890683122, 1.000000000000000000, 0.9659258262890683122, 1.000000000000000000, 0.9659258262890683122, 1.000000000000000000, 0.9659258262890683122, 1.000000000000000000),
 ( 0.3333333333333333703, 0.3219752754296894559, 0.3333333333333333703, 0.3219752754296894559, 0.3333333333333333703, 0.3219752754296894559, 0.3333333333333333703, 0.3219752754296894559, 0.3333333333333333703, 0.3219752754296894559, 0.3333333333333333703, 0.3219752754296894559, 0.3333333333333333703, 0.3219752754296894559, 0.3333333333333333703, 0.3219752754296894559, 0.3333333333333333703, 0.3219752754296894559, 0.3333333333333333703, 0.3219752754296894559, 0.3333333333333333703, 0.3219752754296894559, 0.3333333333333333703, 0.3219752754296894559, 0.3333333333333333703, 0.3219752754296894559, 0.3333333333333333703, 0.3219752754296894559, 0.3333333333333333703, 0.3219752754296894559, 0.3333333333333333703, 0.3219752754296894559, 0.3333333333333333703, 0.3219752754296894559, 0.3333333333333333703, 0.3219752754296894559, 0.3333333333333333703, 0.3219752754296894559, 0.3333333333333333703, 0.3219752754296894559, 0.3333333333333333703, 0.3219752754296894559, 0.3333333333333333703, 0.3219752754296894559, 0.3333333333333333703, 0.3219752754296894559, 0.3333333333333333703, 0.3219752754296894559, 0.3333333333333333703, 0.3219752754296894559, 0.3333333333333333703, 0.3219752754296894559, 0.3333333333333333703, 0.3219752754296894559, 0.3333333333333333703, 0.3219752754296894559, 0.3333333333333333703, 0.3219752754296894559, 0.3333333333333333703, 0.3219752754296894559, 0.3333333333333333703, 0.3219752754296894559, 0.3333333333333333703, 0.3219752754296894559, 0.3333333333333333703, 0.3219752754296894559, 0.3333333333333333703, 0.3219752754296894559, 0.3333333333333333703, 0.3219752754296894559, 0.3333333333333333703, 0.3219752754296894559, 0.3333333333333333703, 0.3219752754296894559, 0.3333333333333333703, 0.3219752754296894559, 0.3333333333333333703, 0.3219752754296894559, 0.3333333333333333703, 0.3219752754296894559, 0.3333333333333333703, 0.3219752754296894559, 0.3333333333333333703, 0.3219752754296894559, 0.3333333333333333703, 0.3219752754296894559, 0.3333333333333333703, 0.3219752754296894559, 0.3333333333333333703, 0.3219752754296894559, 0.3333333333333333703, 0.3219752754296894559, 0.3333333333333333703, 0.3219752754296894559, 0.3333333333333333703, 0.3219752754296894559, 0.3333333333333333703, 0.3219752754296894559, 0.3333333333333333703, 0.3219752754296894559, 0.3333333333333333703, 0.3219752754296894559, 0.3333333333333333703, 0.3219752754296894559, 0.3333333333333333703, 0.3219752754296894559, 0.3333333333333333703, 0.3219752754296894559, 0.3333333333333333703, 0.3219752754296894559, 0.3333333333333333703, 0.3219752754296894559, 0.3333333333333333703, 0.3219752754296894559, 0.3333333333333333703, 0.3219752754296894559, 0.3333333333333333703, 0.3219752754296894559, 0.3333333333333333703, 0.3219752754296894559, 0.3333333333333333703, 0.3219752754296894559, 0.3333333333333333703, 0.3219752754296894559, 0.3333333333333333703, 0.3219752754296894559, 0.3333333333333333703, 0.3219752754296894559, 0.3333333333333333703, 0.3219752754296894559, 0.3333333333333333703, 0.3219752754296894559, 0.3333333333333333703, 0.3219752754296894559, 0.3333333333333333703, 0.3219752754296894559, 0.3333333333333333703, 0.3219752754296894559, 0.3333333333333333703, 0.3219752754296894559, 0.3333333333333333703, 0.3219752754296894559, 0.3333333333333333703, 0.3219752754296894559, 0.3333333333333333703, 0.3219752754296894559, 0.3333333333333333703, 0.3219752754296894559, 0.3333333333333333703, 0.3219752754296894559, 0.3333333333333333703, 0.3219752754296894559, 0.3333333333333333703, 0.3219752754296894559, 0.3333333333333333703, 0.3219752754296894559, 0.3333333333333333703, 0.3219752754296894559, 0.3333333333333333703, 0.3219752754296894559, 0.3333333333333333703, 0.3219752754296894559, 0.3333333333333333703, 0.3219752754296894559, 0.3333333333333333703, 0.3219752754296894559, 0.3333333333333333703, 0.3219752754296894559, 0.3333333333333333703, 0.3219752754296894559, 0.3333333333333333703, 0.3219752754296894559, 0.3333333333333333703, 0.3219752754296894559, 0.3333333333333333703, 0.3219752754296894559, 0.3333333333333333703, 0.3219752754296894559, 0.3333333333333333703, 0.3219752754296894559, 0.3333333333333333703, 0.3219752754296894559, 0.3333333333333333703, 0.3219752754296894559, 0.3333333333333333703, 0.3219752754296894559, 0.3333333333333333703, 0.3219752754296894559, 0.3333333333333333703, 0.3219752754296894559, 0.3333333333333333703, 0.3219752754296894559, 0.3333333333333333703, 0.3219752754296894559, 0.3333333333333333703, 0.3219752754296894559, 0.3333333333333333703, 0.3219752754296894559, 0.3333333333333333703, 0.3219752754296894559, 0.3333333333333333703, 0.3219752754296894559, 0.3333333333333333703, 0.3219752754296894559, 0.3333333333333333703, 0.3219752754296894559, 0.3333333333333333703, 0.3219752754296894559, 0.3333333333333333703, 0.3219752754296894559, 0.3333333333333333703, 0.3219752754296894559, 0.3333333333333333703, 0.3219752754296894559, 0.3333333333333333703, 0.3219752754296894559, 0.3333333333333333703, 0.3219752754296894559, 0.3333333333333333703, 0.3219752754296894559, 0.3333333333333333703, 0.3219752754296894559, 0.3333333333333333703, 0.3219752754296894559, 0.3333333333333333703, 0.3219752754296894559, 0.3333333333333333703, 0.3219752754296894559, 0.3333333333333333703, 0.3219752754296894559, 0.3333333333333333703, 0.3219752754296894559, 0.3333333333333333703, 0.3219752754296894559, 0.3333333333333333703, 0.3219752754296894559, 0.3333333333333333703, 0.3219752754296894559, 0.3333333333333333703, 0.3219752754296894559, 0.3333333333333333703, 0.3219752754296894559, 0.3333333333333333703, 0.3219752754296894559, 0.3333333333333333703, 0.3219752754296894559, 0.3333333333333333703, 0.3219752754296894559, 0.3333333333333333703, 0.3219752754296894559, 0.3333333333333333703, 0.3219752754296894559, 0.3333333333333333703, 0.3219752754296894559, 0.3333333333333333703, 0.3219752754296894559, 0.3333333333333333703, 0.3219752754296894559, 0.3333333333333333703, 0.3219752754296894559, 0.3333333333333333703, 0.3219752754296894559, 0.3333333333333333703, 0.3219752754296894559, 0.3333333333333333703, 0.3219752754296894559, 0.3333333333333333703, 0.3219752754296894559, 0.3333333333333333703, 0.3219752754296894559, 0.3333333333333333703, 0.3219752754296894559, 0.3333333333333333703, 0.3219752754296894559, 0.3333333333333333703, 0.3219752754296894559, 0.3333333333333333703, 0.3219752754296894559, 0.3333333333333333703, 0.3219752754296894559, 0.3333333333333333703, 0.3219752754296894559, 0.3333333333333333703, 0.3219752754296894559, 0.3333333333333333703, 0.3219752754296894559, 0.3333333333333333703, 0.3219752754296894559, 0.3333333333333333703, 0.3219752754296894559, 0.3333333333333333703, 0.3219752754296894559, 0.3333333333333333703, 0.3219752754296894559, 0.3333333333333333703, 0.3219752754296894559, 0.3333333333333333703, 0.3219752754296894559, 0.3333333333333333703, 0.3219752754296894559, 0.3333333333333333703, 0.3219752754296894559, 0.3333333333333333703, 0.3219752754296894559, 0.3333333333333333703, 0.3219752754296894559, 0.3333333333333333703, 0.3219752754296894559, 0.3333333333333333703, 0.3219752754296894559, 0.3333333333333333703, 0.3219752754296894559, 0.3333333333333333703, 0.3219752754296894559, 0.3333333333333333703, 0.3219752754296894559, 0.3333333333333333703, 0.3219752754296894559, 0.3333333333333333703, 0.3219752754296894559, 0.3333333333333333703, 0.3219752754296894559, 0.3333333333333333703, 0.3219752754296894559, 0.3333333333333333703, 0.3219752754296894559, 0.3333333333333333703, 0.3219752754296894559, 0.3333333333333333703, 0.3219752754296894559, 0.3333333333333333703, 0.3219752754296894559, 0.3333333333333333703, 0.3219752754296894559, 0.3333333333333333703, 0.3219752754296894559, 0.3333333333333333703, 0.3219752754296894559, 0.3333333333333333703, 0.3219752754296894559, 0.3333333333333333703, 0.3219752754296894559, 0.3333333333333333703, 0.3219752754296894559, 0.3333333333333333703, 0.3219752754296894559, 0.3333333333333333703, 0.3219752754296894559, 0.3333333333333333703, 0.3219752754296894559, 0.3333333333333333703, 0.3219752754296894559, 0.3333333333333333703, 0.3219752754296894559, 0.3333333333333333703, 0.3219752754296894559, 0.3333333333333333703, 0.3219752754296894559, 0.3333333333333333703, 0.3219752754296894559, 0.3333333333333333703, 0.3219752754296894559, 0.3333333333333333703, 0.3219752754296894559, 0.3333333333333333703, 0.3219752754296894559, 0.3333333333333333703, 0.3219752754296894559, 0.3333333333333333703, 0.3219752754296894559, 0.3333333333333333703, 0.3219752754296894559, 0.3333333333333333703, 0.3219752754296894559, 0.3333333333333333703, 0.3219752754296894559, 0.3333333333333333703, 0.3219752754296894559, 0.3333333333333333703, 0.3219752754296894559, 0.3333333333333333703, 0.3219752754296894559, 0.3333333333333333703, 0.3219752754296894559, 0.3333333333333333703, 0.3219752754296894559, 0.3333333333333333703, 0.3219752754296894559, 0.3333333333333333703, 0.3219752754296894559, 0.3333333333333333703, 0.3219752754296894559, 0.3333333333333333703, 0.3219752754296894559, 0.3333333333333333703, 0.3219752754296894559, 0.3333333333333333703, 0.3219752754296894559, 0.3333333333333333703, 0.3219752754296894559, 0.3333333333333333703, 0.3219752754296894559, 0.3333333333333333703, 0.3219752754296894559, 0.3333333333333333703, 0.3219752754296894559, 0.3333333333333333703, 0.3219752754296894559, 0.3333333333333333703, 0.3219752754296894559, 0.3333333333333333703, 0.3219752754296894559, 0.3333333333333333703, 0.3219752754296894559, 0.3333333333333333703, 0.3219752754296894559, 0.3333333333333333703, 0.3219752754296894559, 0.3333333333333333703, 0.3219752754296894559, 0.3333333333333333703, 0.3219752754296894559, 0.3333333333333333703, 0.3219752754296894559, 0.3333333333333333703, 0.3219752754296894559, 0.3333333333333333703, 0.3219752754296894559, 0.3333333333333333703, 0.3219752754296894559, 0.3333333333333333703, 0.3219752754296894559, 0.3333333333333333703, 0.3219752754296894559, 0.3333333333333333703, 0.3219752754296894559, 0.3333333333333333703, 0.3219752754296894559, 0.3333333333333333703, 0.3219752754296894559, 0.3333333333333333703, 0.3219752754296894559, 0.3333333333333333703, 0.3219752754296894559, 0.3333333333333333703, 0.3219752754296894559, 0.3333333333333333703, 0.3219752754296894559, 0.3333333333333333703, 0.3219752754296894559, 0.3333333333333333703, 0.3219752754296894559, 0.3333333333333333703, 0.3219752754296894559, 0.3333333333333333703, 0.3219752754296894559, 0.3333333333333333703),
 ( 0.3333333333333333703, 0.3219752754296894559, 0.3333333333333333703, 0.3219752754296894559, 0.3333333333333333703, 0.3219752754296894559, 0.3333333333333333703, 0.3219752754296894559, 0.3333333333333333703, 0.3219752754296894559, 0.3333333333333333703, 0.3219752754296894559, 0.3333333333333333703, 0.3219752754296894559, 0.3333333333333333703, 0.3219752754296894559, 0.3333333333333333703, 0.3219752754296894559, 0.3333333333333333703, 0.3219752754296894559, 0.3333333333333333703, 0.3219752754296894559, 0.3333333333333333703, 0.3219752754296894559, 0.3333333333333333703, 0.3219752754296894559, 0.3333333333333333703, 0.3219752754296894559, 0.3333333333333333703, 0.3219752754296894559, 0.3333333333333333703, 0.3219752754296894559, 0.3333333333333333703, 0.3219752754296894559, 0.3333333333333333703, 0.3219752754296894559, 0.3333333333333333703, 0.3219752754296894559, 0.3333333333333333703, 0.3219752754296894559, 0.3333333333333333703, 0.3219752754296894559, 0.3333333333333333703, 0.3219752754296894559, 0.3333333333333333703, 0.3219752754296894559, 0.3333333333333333703, 0.3219752754296894559, 0.3333333333333333703, 0.3219752754296894559, 0.3333333333333333703, 0.3219752754296894559, 0.3333333333333333703, 0.3219752754296894559, 0.3333333333333333703, 0.3219752754296894559, 0.3333333333333333703, 0.3219752754296894559, 0.3333333333333333703, 0.3219752754296894559, 0.3333333333333333703, 0.3219752754296894559, 0.3333333333333333703, 0.3219752754296894559, 0.3333333333333333703, 0.3219752754296894559, 0.3333333333333333703, 0.3219752754296894559, 0.3333333333333333703, 0.3219752754296894559, 0.3333333333333333703, 0.3219752754296894559, 0.3333333333333333703, 0.3219752754296894559, 0.3333333333333333703, 0.3219752754296894559, 0.3333333333333333703, 0.3219752754296894559, 0.3333333333333333703, 0.3219752754296894559, 0.3333333333333333703, 0.3219752754296894559, 0.3333333333333333703, 0.3219752754296894559, 0.3333333333333333703, 0.3219752754296894559, 0.3333333333333333703, 0.3219752754296894559, 0.3333333333333333703, 0.3219752754296894559, 0.3333333333333333703, 0.3219752754296894559, 0.3333333333333333703, 0.3219752754296894559, 0.3333333333333333703, 0.3219752754296894559, 0.3333333333333333703, 0.3219752754296894559, 0.3333333333333333703, 0.3219752754296894559, 0.3333333333333333703, 0.3219752754296894559, 0.3333333333333333703, 0.3219752754296894559, 0.3333333333333333703, 0.3219752754296894559, 0.3333333333333333703, 0.3219752754296894559, 0.3333333333333333703, 0.3219752754296894559, 0.3333333333333333703, 0.3219752754296894559, 0.3333333333333333703, 0.3219752754296894559, 0.3333333333333333703, 0.3219752754296894559, 0.3333333333333333703, 0.3219752754296894559, 0.3333333333333333703, 0.3219752754296894559, 0.3333333333333333703, 0.3219752754296894559, 0.3333333333333333703, 0.3219752754296894559, 0.3333333333333333703, 0.3219752754296894559, 0.3333333333333333703, 0.3219752754296894559, 0.3333333333333333703, 0.3219752754296894559, 0.3333333333333333703, 0.3219752754296894559, 0.3333333333333333703, 0.3219752754296894559, 0.3333333333333333703, 0.3219752754296894559, 0.3333333333333333703, 0.3219752754296894559, 0.3333333333333333703, 0.3219752754296894559, 0.3333333333333333703, 0.3219752754296894559, 0.3333333333333333703, 0.3219752754296894559, 0.3333333333333333703, 0.3219752754296894559, 0.3333333333333333703, 0.3219752754296894559, 0.3333333333333333703, 0.3219752754296894559, 0.3333333333333333703, 0.3219752754296894559, 0.3333333333333333703, 0.3219752754296894559, 0.3333333333333333703, 0.3219752754296894559, 0.3333333333333333703, 0.3219752754296894559, 0.3333333333333333703, 0.3219752754296894559, 0.3333333333333333703, 0.3219752754296894559, 0.3333333333333333703, 0.3219752754296894559, 0.3333333333333333703, 0.3219752754296894559, 0.3333333333333333703, 0.3219752754296894559, 0.3333333333333333703, 0.3219752754296894559, 0.3333333333333333703, 0.3219752754296894559, 0.3333333333333333703, 0.3219752754296894559, 0.3333333333333333703, 0.3219752754296894559, 0.3333333333333333703, 0.3219752754296894559, 0.3333333333333333703, 0.3219752754296894559, 0.3333333333333333703, 0.3219752754296894559, 0.3333333333333333703, 0.3219752754296894559, 0.3333333333333333703, 0.3219752754296894559, 0.3333333333333333703, 0.3219752754296894559, 0.3333333333333333703, 0.3219752754296894559, 0.3333333333333333703, 0.3219752754296894559, 0.3333333333333333703, 0.3219752754296894559, 0.3333333333333333703, 0.3219752754296894559, 0.3333333333333333703, 0.3219752754296894559, 0.3333333333333333703, 0.3219752754296894559, 0.3333333333333333703, 0.3219752754296894559, 0.3333333333333333703, 0.3219752754296894559, 0.3333333333333333703, 0.3219752754296894559, 0.3333333333333333703, 0.3219752754296894559, 0.3333333333333333703, 0.3219752754296894559, 0.3333333333333333703, 0.3219752754296894559, 0.3333333333333333703, 0.3219752754296894559, 0.3333333333333333703, 0.3219752754296894559, 0.3333333333333333703, 0.3219752754296894559, 0.3333333333333333703, 0.3219752754296894559, 0.3333333333333333703, 0.3219752754296894559, 0.3333333333333333703, 0.3219752754296894559, 0.3333333333333333703, 0.3219752754296894559, 0.3333333333333333703, 0.3219752754296894559, 0.3333333333333333703, 0.3219752754296894559, 0.3333333333333333703, 0.3219752754296894559, 0.3333333333333333703, 0.3219752754296894559, 0.3333333333333333703, 0.3219752754296894559, 0.3333333333333333703, 0.3219752754296894559, 0.3333333333333333703, 0.3219752754296894559, 0.3333333333333333703, 0.3219752754296894559, 0.3333333333333333703, 0.3219752754296894559, 0.3333333333333333703, 0.3219752754296894559, 0.3333333333333333703, 0.3219752754296894559, 0.3333333333333333703, 0.3219752754296894559, 0.3333333333333333703, 0.3219752754296894559, 0.3333333333333333703, 0.3219752754296894559, 0.3333333333333333703, 0.3219752754296894559, 0.3333333333333333703, 0.3219752754296894559, 0.3333333333333333703, 0.3219752754296894559, 0.3333333333333333703, 0.3219752754296894559, 0.3333333333333333703, 0.3219752754296894559, 0.3333333333333333703, 0.3219752754296894559, 0.3333333333333333703, 0.3219752754296894559, 0.3333333333333333703, 0.3219752754296894559, 0.3333333333333333703, 0.3219752754296894559, 0.3333333333333333703, 0.3219752754296894559, 0.3333333333333333703, 0.3219752754296894559, 0.3333333333333333703, 0.3219752754296894559, 0.3333333333333333703, 0.3219752754296894559, 0.3333333333333333703, 0.3219752754296894559, 0.3333333333333333703, 0.3219752754296894559, 0.3333333333333333703, 0.3219752754296894559, 0.3333333333333333703, 0.3219752754296894559, 0.3333333333333333703, 0.3219752754296894559, 0.3333333333333333703, 0.3219752754296894559, 0.3333333333333333703, 0.3219752754296894559, 0.3333333333333333703, 0.3219752754296894559, 0.3333333333333333703, 0.3219752754296894559, 0.3333333333333333703, 0.3219752754296894559, 0.3333333333333333703, 0.3219752754296894559, 0.3333333333333333703, 0.3219752754296894559, 0.3333333333333333703, 0.3219752754296894559, 0.3333333333333333703, 0.3219752754296894559, 0.3333333333333333703, 0.3219752754296894559, 0.3333333333333333703, 0.3219752754296894559, 0.3333333333333333703, 0.3219752754296894559, 0.3333333333333333703, 0.3219752754296894559, 0.3333333333333333703, 0.3219752754296894559, 0.3333333333333333703, 0.3219752754296894559, 0.3333333333333333703, 0.3219752754296894559, 0.3333333333333333703, 0.3219752754296894559, 0.3333333333333333703, 0.3219752754296894559, 0.3333333333333333703, 0.3219752754296894559, 0.3333333333333333703, 0.3219752754296894559, 0.3333333333333333703, 0.3219752754296894559, 0.3333333333333333703, 0.3219752754296894559, 0.3333333333333333703, 0.3219752754296894559, 0.3333333333333333703, 0.3219752754296894559, 0.3333333333333333703, 0.3219752754296894559, 0.3333333333333333703, 0.3219752754296894559, 0.3333333333333333703, 0.3219752754296894559, 0.3333333333333333703, 0.3219752754296894559, 0.3333333333333333703, 0.3219752754296894559, 0.3333333333333333703, 0.3219752754296894559, 0.3333333333333333703, 0.3219752754296894559, 0.3333333333333333703, 0.3219752754296894559, 0.3333333333333333703, 0.3219752754296894559, 0.3333333333333333703, 0.3219752754296894559, 0.3333333333333333703, 0.3219752754296894559, 0.3333333333333333703, 0.3219752754296894559, 0.3333333333333333703, 0.3219752754296894559, 0.3333333333333333703, 0.3219752754296894559, 0.3333333333333333703, 0.3219752754296894559, 0.3333333333333333703, 0.3219752754296894559, 0.3333333333333333703, 0.3219752754296894559, 0.3333333333333333703, 0.3219752754296894559, 0.3333333333333333703, 0.3219752754296894559, 0.3333333333333333703, 0.3219752754296894559, 0.3333333333333333703, 0.3219752754296894559, 0.3333333333333333703, 0.3219752754296894559, 0.3333333333333333703, 0.3219752754296894559, 0.3333333333333333703, 0.3219752754296894559, 0.3333333333333333703, 0.3219752754296894559, 0.3333333333333333703, 0.3219752754296894559, 0.3333333333333333703, 0.3219752754296894559, 0.3333333333333333703, 0.3219752754296894559, 0.3333333333333333703, 0.3219752754296894559, 0.3333333333333333703, 0.3219752754296894559, 0.3333333333333333703, 0.3219752754296894559, 0.3333333333333333703, 0.3219752754296894559, 0.3333333333333333703, 0.3219752754296894559, 0.3333333333333333703, 0.3219752754296894559, 0.3333333333333333703, 0.3219752754296894559, 0.3333333333333333703, 0.3219752754296894559, 0.3333333333333333703, 0.3219752754296894559, 0.3333333333333333703, 0.3219752754296894559, 0.3333333333333333703, 0.3219752754296894559, 0.3333333333333333703, 0.3219752754296894559, 0.3333333333333333703, 0.3219752754296894559, 0.3333333333333333703, 0.3219752754296894559, 0.3333333333333333703, 0.3219752754296894559, 0.3333333333333333703, 0.3219752754296894559, 0.3333333333333333703, 0.3219752754296894559, 0.3333333333333333703, 0.3219752754296894559, 0.3333333333333333703, 0.3219752754296894559, 0.3333333333333333703, 0.3219752754296894559, 0.3333333333333333703, 0.3219752754296894559, 0.3333333333333333703, 0.3219752754296894559, 0.3333333333333333703, 0.3219752754296894559, 0.3333333333333333703, 0.3219752754296894559, 0.3333333333333333703, 0.3219752754296894559, 0.3333333333333333703, 0.3219752754296894559, 0.3333333333333333703, 0.3219752754296894559, 0.3333333333333333703, 0.3219752754296894559, 0.3333333333333333703, 0.3219752754296894559, 0.3333333333333333703, 0.3219752754296894559, 0.3333333333333333703, 0.3219752754296894559, 0.3333333333333333703),
 ( 1.000000000000000000, 0.9659258262890683122, 1.000000000000000000, 0.9659258262890683122, 1.000000000000000000, 0.9659258262890683122, 1.000000000000000000, 0.9659258262890683122, 1.000000000000000000, 0.9659258262890683122, 1.000000000000000000, 0.9659258262890683122, 1.000000000000000000, 0.9659258262890683122, 1.000000000000000000, 0.9659258262890683122, 1.000000000000000000, 0.9659258262890683122, 1.000000000000000000, 0.9659258262890683122, 1.000000000000000000, 0.9659258262890683122, 1.000000000000000000, 0.9659258262890683122, 1.000000000000000000, 0.9659258262890683122, 1.000000000000000000, 0.9659258262890683122, 1.000000000000000000, 0.9659258262890683122, 1.000000000000000000, 0.9659258262890683122, 1.000000000000000000, 0.9659258262890683122, 1.000000000000000000, 0.9659258262890683122, 1.000000000000000000, 0.9659258262890683122, 1.000000000000000000, 0.9659258262890683122, 1.000000000000000000, 0.9659258262890683122, 1.000000000000000000, 0.9659258262890683122, 1.000000000000000000, 0.9659258262890683122, 1.000000000000000000, 0.9659258262890683122, 1.000000000000000000, 0.9659258262890683122, 1.000000000000000000, 0.9659258262890683122, 1.000000000000000000, 0.9659258262890683122, 1.000000000000000000, 0.9659258262890683122, 1.000000000000000000, 0.9659258262890683122, 1.000000000000000000, 0.9659258262890683122, 1.000000000000000000, 0.9659258262890683122, 1.000000000000000000, 0.9659258262890683122, 1.000000000000000000, 0.9659258262890683122, 1.000000000000000000, 0.9659258262890683122, 1.000000000000000000, 0.9659258262890683122, 1.000000000000000000, 0.9659258262890683122, 1.000000000000000000, 0.9659258262890683122, 1.000000000000000000, 0.9659258262890683122, 1.000000000000000000, 0.9659258262890683122, 1.000000000000000000, 0.9659258262890683122, 1.000000000000000000, 0.9659258262890683122, 1.000000000000000000, 0.9659258262890683122, 1.000000000000000000, 0.9659258262890683122, 1.000000000000000000, 0.9659258262890683122, 1.000000000000000000, 0.9659258262890683122, 1.000000000000000000, 0.9659258262890683122, 1.000000000000000000, 0.9659258262890683122, 1.000000000000000000, 0.9659258262890683122, 1.000000000000000000, 0.9659258262890683122, 1.000000000000000000, 0.9659258262890683122, 1.000000000000000000, 0.9659258262890683122, 1.000000000000000000, 0.9659258262890683122, 1.000000000000000000, 0.9659258262890683122, 1.000000000000000000, 0.9659258262890683122, 1.000000000000000000, 0.9659258262890683122, 1.000000000000000000, 0.9659258262890683122, 1.000000000000000000, 0.9659258262890683122, 1.000000000000000000, 0.9659258262890683122, 1.000000000000000000, 0.9659258262890683122, 1.000000000000000000, 0.9659258262890683122, 1.000000000000000000, 0.9659258262890683122, 1.000000000000000000, 0.9659258262890683122, 1.000000000000000000, 0.9659258262890683122, 1.000000000000000000, 0.9659258262890683122, 1.000000000000000000, 0.9659258262890683122, 1.000000000000000000, 0.9659258262890683122, 1.000000000000000000, 0.9659258262890683122, 1.000000000000000000, 0.9659258262890683122, 1.000000000000000000, 0.9659258262890683122, 1.000000000000000000, 0.9659258262890683122, 1.000000000000000000, 0.9659258262890683122, 1.000000000000000000, 0.9659258262890683122, 1.000000000000000000, 0.9659258262890683122, 1.000000000000000000, 0.9659258262890683122, 1.000000000000000000, 0.9659258262890683122, 1.000000000000000000, 0.9659258262890683122, 1.000000000000000000, 0.9659258262890683122, 1.000000000000000000, 0.9659258262890683122, 1.000000000000000000, 0.9659258262890683122, 1.000000000000000000, 0.9659258262890683122, 1.000000000000000000, 0.9659258262890683122, 1.000000000000000000, 0.9659258262890683122, 1.000000000000000000, 0.9659258262890683122, 1.000000000000000000, 0.9659258262890683122, 1.000000000000000000, 0.9659258262890683122, 1.000000000000000000, 0.9659258262890683122, 1.000000000000000000, 0.9659258262890683122, 1.000000000000000000, 0.9659258262890683122, 1.000000000000000000, 0.9659258262890683122, 1.000000000000000000, 0.9659258262890683122, 1.000000000000000000, 0.9659258262890683122, 1.000000000000000000, 0.9659258262890683122, 1.000000000000000000, 0.9659258262890683122, 1.000000000000000000, 0.9659258262890683122, 1.000000000000000000, 0.9659258262890683122, 1.000000000000000000, 0.9659258262890683122, 1.000000000000000000, 0.9659258262890683122, 1.000000000000000000, 0.9659258262890683122, 1.000000000000000000, 0.9659258262890683122, 1.000000000000000000, 0.9659258262890683122, 1.000000000000000000, 0.9659258262890683122, 1.000000000000000000, 0.9659258262890683122, 1.000000000000000000, 0.9659258262890683122, 1.000000000000000000, 0.9659258262890683122, 1.000000000000000000, 0.9659258262890683122, 1.000000000000000000, 0.9659258262890683122, 1.000000000000000000, 0.9659258262890683122, 1.000000000000000000, 0.9659258262890683122, 1.000000000000000000, 0.9659258262890683122, 1.000000000000000000, 0.9659258262890683122, 1.000000000000000000, 0.9659258262890683122, 1.000000000000000000, 0.9659258262890683122, 1.000000000000000000, 0.9659258262890683122, 1.000000000000000000, 0.9659258262890683122, 1.000000000000000000, 0.9659258262890683122, 1.000000000000000000, 0.9659258262890683122, 1.000000000000000000, 0.9659258262890683122, 1.000000000000000000, 0.9659258262890683122, 1.000000000000000000, 0.9659258262890683122, 1.000000000000000000, 0.9659258262890683122, 1.000000000000000000, 0.9659258262890683122, 1.000000000000000000, 0.9659258262890683122, 1.000000000000000000, 0.9659258262890683122, 1.000000000000000000, 0.9659258262890683122, 1.000000000000000000, 0.9659258262890683122, 1.000000000000000000, 0.9659258262890683122, 1.000000000000000000, 0.9659258262890683122, 1.000000000000000000, 0.9659258262890683122, 1.000000000000000000, 0.9659258262890683122, 1.000000000000000000, 0.9659258262890683122, 1.000000000000000000, 0.9659258262890683122, 1.000000000000000000, 0.9659258262890683122, 1.000000000000000000, 0.9659258262890683122, 1.000000000000000000, 0.9659258262890683122, 1.000000000000000000, 0.9659258262890683122, 1.000000000000000000, 0.9659258262890683122, 1.000000000000000000, 0.9659258262890683122, 1.000000000000000000, 0.9659258262890683122, 1.000000000000000000, 0.9659258262890683122, 1.000000000000000000, 0.9659258262890683122, 1.000000000000000000, 0.9659258262890683122, 1.000000000000000000, 0.9659258262890683122, 1.000000000000000000, 0.9659258262890683122, 1.000000000000000000, 0.9659258262890683122, 1.000000000000000000, 0.9659258262890683122, 1.000000000000000000, 0.9659258262890683122, 1.000000000000000000, 0.9659258262890683122, 1.000000000000000000, 0.9659258262890683122, 1.000000000000000000, 0.9659258262890683122, 1.000000000000000000, 0.9659258262890683122, 1.000000000000000000, 0.9659258262890683122, 1.000000000000000000, 0.9659258262890683122, 1.000000000000000000, 0.9659258262890683122, 1.000000000000000000, 0.9659258262890683122, 1.000000000000000000, 0.9659258262890683122, 1.000000000000000000, 0.9659258262890683122, 1.000000000000000000, 0.9659258262890683122, 1.000000000000000000, 0.9659258262890683122, 1.000000000000000000, 0.9659258262890683122, 1.000000000000000000, 0.9659258262890683122, 1.000000000000000000, 0.9659258262890683122, 1.000000000000000000, 0.9659258262890683122, 1.000000000000000000, 0.9659258262890683122, 1.000000000000000000, 0.9659258262890683122, 1.000000000000000000, 0.9659258262890683122, 1.000000000000000000, 0.9659258262890683122, 1.000000000000000000, 0.9659258262890683122, 1.000000000000000000, 0.9659258262890683122, 1.000000000000000000, 0.9659258262890683122, 1.000000000000000000, 0.9659258262890683122, 1.000000000000000000, 0.9659258262890683122, 1.000000000000000000, 0.9659258262890683122, 1.000000000000000000, 0.9659258262890683122, 1.000000000000000000, 0.9659258262890683122, 1.000000000000000000, 0.9659258262890683122, 1.000000000000000000, 0.9659258262890683122, 1.000000000000000000, 0.9659258262890683122, 1.000000000000000000, 0.9659258262890683122, 1.000000000000000000, 0.9659258262890683122, 1.000000000000000000, 0.9659258262890683122, 1.000000000000000000, 0.9659258262890683122, 1.000000000000000000, 0.9659258262890683122, 1.000000000000000000, 0.9659258262890683122, 1.000000000000000000, 0.9659258262890683122, 1.000000000000000000, 0.9659258262890683122, 1.000000000000000000, 0.9659258262890683122, 1.000000000000000000, 0.9659258262890683122, 1.000000000000000000, 0.9659258262890683122, 1.000000000000000000, 0.9659258262890683122, 1.000000000000000000, 0.9659258262890683122, 1.000000000000000000, 0.9659258262890683122, 1.000000000000000000, 0.9659258262890683122, 1.000000000000000000, 0.9659258262890683122, 1.000000000000000000, 0.9659258262890683122, 1.000000000000000000, 0.9659258262890683122, 1.000000000000000000, 0.9659258262890683122, 1.000000000000000000, 0.9659258262890683122, 1.000000000000000000, 0.9659258262890683122, 1.000000000000000000, 0.9659258262890683122, 1.000000000000000000, 0.9659258262890683122, 1.000000000000000000, 0.9659258262890683122, 1.000000000000000000, 0.9659258262890683122, 1.000000000000000000, 0.9659258262890683122, 1.000000000000000000, 0.9659258262890683122, 1.000000000000000000, 0.9659258262890683122, 1.000000000000000000, 0.9659258262890683122, 1.000000000000000000, 0.9659258262890683122, 1.000000000000000000, 0.9659258262890683122, 1.000000000000000000, 0.9659258262890683122, 1.000000000000000000, 0.9659258262890683122, 1.000000000000000000, 0.9659258262890683122, 1.000000000000000000, 0.9659258262890683122, 1.000000000000000000, 0.9659258262890683122, 1.000000000000000000, 0.9659258262890683122, 1.000000000000000000, 0.9659258262890683122, 1.000000000000000000, 0.9659258262890683122, 1.000000000000000000, 0.9659258262890683122, 1.000000000000000000, 0.9659258262890683122, 1.000000000000000000, 0.9659258262890683122, 1.000000000000000000, 0.9659258262890683122, 1.000000000000000000, 0.9659258262890683122, 1.000000000000000000, 0.9659258262890683122, 1.000000000000000000, 0.9659258262890683122, 1.000000000000000000, 0.9659258262890683122, 1.000000000000000000, 0.9659258262890683122, 1.000000000000000000, 0.9659258262890683122, 1.000000000000000000, 0.9659258262890683122, 1.000000000000000000, 0.9659258262890683122, 1.000000000000000000),
 ( 0.3333333333333333703, 0.3219752754296894559, 0.3333333333333333703, 0.3219752754296894559, 0.3333333333333333703, 0.3219752754296894559, 0.3333333333333333703, 0.3219752754296894559, 0.3333333333333333703, 0.3219752754296894559, 0.3333333333333333703, 0.3219752754296894559, 0.3333333333333333703, 0.3219752754296894559, 0.3333333333333333703, 0.3219752754296894559, 0.3333333333333333703, 0.3219752754296894559, 0.3333333333333333703, 0.3219752754296894559, 0.3333333333333333703, 0.3219752754296894559, 0.3333333333333333703, 0.3219752754296894559, 0.3333333333333333703, 0.3219752754296894559, 0.3333333333333333703, 0.3219752754296894559, 0.3333333333333333703, 0.3219752754296894559, 0.3333333333333333703, 0.3219752754296894559, 0.3333333333333333703, 0.3219752754296894559, 0.3333333333333333703, 0.3219752754296894559, 0.3333333333333333703, 0.3219752754296894559, 0.3333333333333333703, 0.3219752754296894559, 0.3333333333333333703, 0.3219752754296894559, 0.3333333333333333703, 0.3219752754296894559, 0.3333333333333333703, 0.3219752754296894559, 0.3333333333333333703, 0.3219752754296894559, 0.3333333333333333703, 0.3219752754296894559, 0.3333333333333333703, 0.3219752754296894559, 0.3333333333333333703, 0.3219752754296894559, 0.3333333333333333703, 0.3219752754296894559, 0.3333333333333333703, 0.3219752754296894559, 0.3333333333333333703, 0.3219752754296894559, 0.3333333333333333703, 0.3219752754296894559, 0.3333333333333333703, 0.3219752754296894559, 0.3333333333333333703, 0.3219752754296894559, 0.3333333333333333703, 0.3219752754296894559, 0.3333333333333333703, 0.3219752754296894559, 0.3333333333333333703, 0.3219752754296894559, 0.3333333333333333703, 0.3219752754296894559, 0.3333333333333333703, 0.3219752754296894559, 0.3333333333333333703, 0.3219752754296894559, 0.3333333333333333703, 0.3219752754296894559, 0.3333333333333333703, 0.3219752754296894559, 0.3333333333333333703, 0.3219752754296894559, 0.3333333333333333703, 0.3219752754296894559, 0.3333333333333333703, 0.3219752754296894559, 0.3333333333333333703, 0.3219752754296894559, 0.3333333333333333703, 0.3219752754296894559, 0.3333333333333333703, 0.3219752754296894559, 0.3333333333333333703, 0.3219752754296894559, 0.3333333333333333703, 0.3219752754296894559, 0.3333333333333333703, 0.3219752754296894559, 0.3333333333333333703, 0.3219752754296894559, 0.3333333333333333703, 0.3219752754296894559, 0.3333333333333333703, 0.3219752754296894559, 0.3333333333333333703, 0.3219752754296894559, 0.3333333333333333703, 0.3219752754296894559, 0.3333333333333333703, 0.3219752754296894559, 0.3333333333333333703, 0.3219752754296894559, 0.3333333333333333703, 0.3219752754296894559, 0.3333333333333333703, 0.3219752754296894559, 0.3333333333333333703, 0.3219752754296894559, 0.3333333333333333703, 0.3219752754296894559, 0.3333333333333333703, 0.3219752754296894559, 0.3333333333333333703, 0.3219752754296894559, 0.3333333333333333703, 0.3219752754296894559, 0.3333333333333333703, 0.3219752754296894559, 0.3333333333333333703, 0.3219752754296894559, 0.3333333333333333703, 0.3219752754296894559, 0.3333333333333333703, 0.3219752754296894559, 0.3333333333333333703, 0.3219752754296894559, 0.3333333333333333703, 0.3219752754296894559, 0.3333333333333333703, 0.3219752754296894559, 0.3333333333333333703, 0.3219752754296894559, 0.3333333333333333703, 0.3219752754296894559, 0.3333333333333333703, 0.3219752754296894559, 0.3333333333333333703, 0.3219752754296894559, 0.3333333333333333703, 0.3219752754296894559, 0.3333333333333333703, 0.3219752754296894559, 0.3333333333333333703, 0.3219752754296894559, 0.3333333333333333703, 0.3219752754296894559, 0.3333333333333333703, 0.3219752754296894559, 0.3333333333333333703, 0.3219752754296894559, 0.3333333333333333703, 0.3219752754296894559, 0.3333333333333333703, 0.3219752754296894559, 0.3333333333333333703, 0.3219752754296894559, 0.3333333333333333703, 0.3219752754296894559, 0.3333333333333333703, 0.3219752754296894559, 0.3333333333333333703, 0.3219752754296894559, 0.3333333333333333703, 0.3219752754296894559, 0.3333333333333333703, 0.3219752754296894559, 0.3333333333333333703, 0.3219752754296894559, 0.3333333333333333703, 0.3219752754296894559, 0.3333333333333333703, 0.3219752754296894559, 0.3333333333333333703, 0.3219752754296894559, 0.3333333333333333703, 0.3219752754296894559, 0.3333333333333333703, 0.3219752754296894559, 0.3333333333333333703, 0.3219752754296894559, 0.3333333333333333703, 0.3219752754296894559, 0.3333333333333333703, 0.3219752754296894559, 0.3333333333333333703, 0.3219752754296894559, 0.3333333333333333703, 0.3219752754296894559, 0.3333333333333333703, 0.3219752754296894559, 0.3333333333333333703, 0.3219752754296894559, 0.3333333333333333703, 0.3219752754296894559, 0.3333333333333333703, 0.3219752754296894559, 0.3333333333333333703, 0.3219752754296894559, 0.3333333333333333703, 0.3219752754296894559, 0.3333333333333333703, 0.3219752754296894559, 0.3333333333333333703, 0.3219752754296894559, 0.3333333333333333703, 0.3219752754296894559, 0.3333333333333333703, 0.3219752754296894559, 0.3333333333333333703, 0.3219752754296894559, 0.3333333333333333703, 0.3219752754296894559, 0.3333333333333333703, 0.3219752754296894559, 0.3333333333333333703, 0.3219752754296894559, 0.3333333333333333703, 0.3219752754296894559, 0.3333333333333333703, 0.3219752754296894559, 0.3333333333333333703, 0.3219752754296894559, 0.3333333333333333703, 0.3219752754296894559, 0.3333333333333333703, 0.3219752754296894559, 0.3333333333333333703, 0.3219752754296894559, 0.3333333333333333703, 0.3219752754296894559, 0.3333333333333333703, 0.3219752754296894559, 0.3333333333333333703, 0.3219752754296894559, 0.3333333333333333703, 0.3219752754296894559, 0.3333333333333333703, 0.3219752754296894559, 0.3333333333333333703, 0.3219752754296894559, 0.3333333333333333703, 0.3219752754296894559, 0.3333333333333333703, 0.3219752754296894559, 0.3333333333333333703, 0.3219752754296894559, 0.3333333333333333703, 0.3219752754296894559, 0.3333333333333333703, 0.3219752754296894559, 0.3333333333333333703, 0.3219752754296894559, 0.3333333333333333703, 0.3219752754296894559, 0.3333333333333333703, 0.3219752754296894559, 0.3333333333333333703, 0.3219752754296894559, 0.3333333333333333703, 0.3219752754296894559, 0.3333333333333333703, 0.3219752754296894559, 0.3333333333333333703, 0.3219752754296894559, 0.3333333333333333703, 0.3219752754296894559, 0.3333333333333333703, 0.3219752754296894559, 0.3333333333333333703, 0.3219752754296894559, 0.3333333333333333703, 0.3219752754296894559, 0.3333333333333333703, 0.3219752754296894559, 0.3333333333333333703, 0.3219752754296894559, 0.3333333333333333703, 0.3219752754296894559, 0.3333333333333333703, 0.3219752754296894559, 0.3333333333333333703, 0.3219752754296894559, 0.3333333333333333703, 0.3219752754296894559, 0.3333333333333333703, 0.3219752754296894559, 0.3333333333333333703, 0.3219752754296894559, 0.3333333333333333703, 0.3219752754296894559, 0.3333333333333333703, 0.3219752754296894559, 0.3333333333333333703, 0.3219752754296894559, 0.3333333333333333703, 0.3219752754296894559, 0.3333333333333333703, 0.3219752754296894559, 0.3333333333333333703, 0.3219752754296894559, 0.3333333333333333703, 0.3219752754296894559, 0.3333333333333333703, 0.3219752754296894559, 0.3333333333333333703, 0.3219752754296894559, 0.3333333333333333703, 0.3219752754296894559, 0.3333333333333333703, 0.3219752754296894559, 0.3333333333333333703, 0.3219752754296894559, 0.3333333333333333703, 0.3219752754296894559, 0.3333333333333333703, 0.3219752754296894559, 0.3333333333333333703, 0.3219752754296894559, 0.3333333333333333703, 0.3219752754296894559, 0.3333333333333333703, 0.3219752754296894559, 0.3333333333333333703, 0.3219752754296894559, 0.3333333333333333703, 0.3219752754296894559, 0.3333333333333333703, 0.3219752754296894559, 0.3333333333333333703, 0.3219752754296894559, 0.3333333333333333703, 0.3219752754296894559, 0.3333333333333333703, 0.3219752754296894559, 0.3333333333333333703, 0.3219752754296894559, 0.3333333333333333703, 0.3219752754296894559, 0.3333333333333333703, 0.3219752754296894559, 0.3333333333333333703, 0.3219752754296894559, 0.3333333333333333703, 0.3219752754296894559, 0.3333333333333333703, 0.3219752754296894559, 0.3333333333333333703, 0.3219752754296894559, 0.3333333333333333703, 0.3219752754296894559, 0.3333333333333333703, 0.3219752754296894559, 0.3333333333333333703, 0.3219752754296894559, 0.3333333333333333703, 0.3219752754296894559, 0.3333333333333333703, 0.3219752754296894559, 0.3333333333333333703, 0.3219752754296894559, 0.3333333333333333703, 0.3219752754296894559, 0.3333333333333333703, 0.3219752754296894559, 0.3333333333333333703, 0.3219752754296894559, 0.3333333333333333703, 0.3219752754296894559, 0.3333333333333333703, 0.3219752754296894559, 0.3333333333333333703, 0.3219752754296894559, 0.3333333333333333703, 0.3219752754296894559, 0.3333333333333333703, 0.3219752754296894559, 0.3333333333333333703, 0.3219752754296894559, 0.3333333333333333703, 0.3219752754296894559, 0.3333333333333333703, 0.3219752754296894559, 0.3333333333333333703, 0.3219752754296894559, 0.3333333333333333703, 0.3219752754296894559, 0.3333333333333333703, 0.3219752754296894559, 0.3333333333333333703, 0.3219752754296894559, 0.3333333333333333703, 0.3219752754296894559, 0.3333333333333333703, 0.3219752754296894559, 0.3333333333333333703, 0.3219752754296894559, 0.3333333333333333703, 0.3219752754296894559, 0.3333333333333333703, 0.3219752754296894559, 0.3333333333333333703, 0.3219752754296894559, 0.3333333333333333703, 0.3219752754296894559, 0.3333333333333333703, 0.3219752754296894559, 0.3333333333333333703, 0.3219752754296894559, 0.3333333333333333703, 0.3219752754296894559, 0.3333333333333333703, 0.3219752754296894559, 0.3333333333333333703, 0.3219752754296894559, 0.3333333333333333703, 0.3219752754296894559, 0.3333333333333333703, 0.3219752754296894559, 0.3333333333333333703, 0.3219752754296894559, 0.3333333333333333703, 0.3219752754296894559, 0.3333333333333333703, 0.3219752754296894559, 0.3333333333333333703, 0.3219752754296894559, 0.3333333333333333703, 0.3219752754296894559, 0.3333333333333333703, 0.3219752754296894559, 0.3333333333333333703, 0.3219752754296894559, 0.3333333333333333703, 0.3219752754296894559, 0.3333333333333333703, 0.3219752754296894559, 0.3333333333333333703, 0.3219752754296894559, 0.3333333333333333703, 0.3219752754296894559, 0.3333333333333333703, 0.3219752754296894559, 0.3333333333333333703, 0.3219752754296894559, 0.3333333333333333703),
 ( 0.3333333333333333703, 0.3219752754296894559, 0.3333333333333333703, 0.3219752754296894559, 0.3333333333333333703, 0.3219752754296894559, 0.3333333333333333703, 0.3219752754296894559, 0.3333333333333333703, 0.3219752754296894559, 0.3333333333333333703, 0.3219752754296894559, 0.3333333333333333703, 0.3219752754296894559, 0.3333333333333333703, 0.3219752754296894559, 0.3333333333333333703, 0.3219752754296894559, 0.3333333333333333703, 0.3219752754296894559, 0.3333333333333333703, 0.3219752754296894559, 0.3333333333333333703, 0.3219752754296894559, 0.3333333333333333703, 0.3219752754296894559, 0.3333333333333333703, 0.3219752754296894559, 0.3333333333333333703, 0.3219752754296894559, 0.3333333333333333703, 0.3219752754296894559, 0.3333333333333333703, 0.3219752754296894559, 0.3333333333333333703, 0.3219752754296894559, 0.3333333333333333703, 0.3219752754296894559, 0.3333333333333333703, 0.3219752754296894559, 0.3333333333333333703, 0.3219752754296894559, 0.3333333333333333703, 0.3219752754296894559, 0.3333333333333333703, 0.3219752754296894559, 0.3333333333333333703, 0.3219752754296894559, 0.3333333333333333703, 0.3219752754296894559, 0.3333333333333333703, 0.3219752754296894559, 0.3333333333333333703, 0.3219752754296894559, 0.3333333333333333703, 0.3219752754296894559, 0.3333333333333333703, 0.3219752754296894559, 0.3333333333333333703, 0.3219752754296894559, 0.3333333333333333703, 0.3219752754296894559, 0.3333333333333333703, 0.3219752754296894559, 0.3333333333333333703, 0.3219752754296894559, 0.3333333333333333703, 0.3219752754296894559, 0.3333333333333333703, 0.3219752754296894559, 0.3333333333333333703, 0.3219752754296894559, 0.3333333333333333703, 0.3219752754296894559, 0.3333333333333333703, 0.3219752754296894559, 0.3333333333333333703, 0.3219752754296894559, 0.3333333333333333703, 0.3219752754296894559, 0.3333333333333333703, 0.3219752754296894559, 0.3333333333333333703, 0.3219752754296894559, 0.3333333333333333703, 0.3219752754296894559, 0.3333333333333333703, 0.3219752754296894559, 0.3333333333333333703, 0.3219752754296894559, 0.3333333333333333703, 0.3219752754296894559, 0.3333333333333333703, 0.3219752754296894559, 0.3333333333333333703, 0.3219752754296894559, 0.3333333333333333703, 0.3219752754296894559, 0.3333333333333333703, 0.3219752754296894559, 0.3333333333333333703, 0.3219752754296894559, 0.3333333333333333703, 0.3219752754296894559, 0.3333333333333333703, 0.3219752754296894559, 0.3333333333333333703, 0.3219752754296894559, 0.3333333333333333703, 0.3219752754296894559, 0.3333333333333333703, 0.3219752754296894559, 0.3333333333333333703, 0.3219752754296894559, 0.3333333333333333703, 0.3219752754296894559, 0.3333333333333333703, 0.3219752754296894559, 0.3333333333333333703, 0.3219752754296894559, 0.3333333333333333703, 0.3219752754296894559, 0.3333333333333333703, 0.3219752754296894559, 0.3333333333333333703, 0.3219752754296894559, 0.3333333333333333703, 0.3219752754296894559, 0.3333333333333333703, 0.3219752754296894559, 0.3333333333333333703, 0.3219752754296894559, 0.3333333333333333703, 0.3219752754296894559, 0.3333333333333333703, 0.3219752754296894559, 0.3333333333333333703, 0.3219752754296894559, 0.3333333333333333703, 0.3219752754296894559, 0.3333333333333333703, 0.3219752754296894559, 0.3333333333333333703, 0.3219752754296894559, 0.3333333333333333703, 0.3219752754296894559, 0.3333333333333333703, 0.3219752754296894559, 0.3333333333333333703, 0.3219752754296894559, 0.3333333333333333703, 0.3219752754296894559, 0.3333333333333333703, 0.3219752754296894559, 0.3333333333333333703, 0.3219752754296894559, 0.3333333333333333703, 0.3219752754296894559, 0.3333333333333333703, 0.3219752754296894559, 0.3333333333333333703, 0.3219752754296894559, 0.3333333333333333703, 0.3219752754296894559, 0.3333333333333333703, 0.3219752754296894559, 0.3333333333333333703, 0.3219752754296894559, 0.3333333333333333703, 0.3219752754296894559, 0.3333333333333333703, 0.3219752754296894559, 0.3333333333333333703, 0.3219752754296894559, 0.3333333333333333703, 0.3219752754296894559, 0.3333333333333333703, 0.3219752754296894559, 0.3333333333333333703, 0.3219752754296894559, 0.3333333333333333703, 0.3219752754296894559, 0.3333333333333333703, 0.3219752754296894559, 0.3333333333333333703, 0.3219752754296894559, 0.3333333333333333703, 0.3219752754296894559, 0.3333333333333333703, 0.3219752754296894559, 0.3333333333333333703, 0.3219752754296894559, 0.3333333333333333703, 0.3219752754296894559, 0.3333333333333333703, 0.3219752754296894559, 0.3333333333333333703, 0.3219752754296894559, 0.3333333333333333703, 0.3219752754296894559, 0.3333333333333333703, 0.3219752754296894559, 0.3333333333333333703, 0.3219752754296894559, 0.3333333333333333703, 0.3219752754296894559, 0.3333333333333333703, 0.3219752754296894559, 0.3333333333333333703, 0.3219752754296894559, 0.3333333333333333703, 0.3219752754296894559, 0.3333333333333333703, 0.3219752754296894559, 0.3333333333333333703, 0.3219752754296894559, 0.3333333333333333703, 0.3219752754296894559, 0.3333333333333333703, 0.3219752754296894559, 0.3333333333333333703, 0.3219752754296894559, 0.3333333333333333703, 0.3219752754296894559, 0.3333333333333333703, 0.3219752754296894559, 0.3333333333333333703, 0.3219752754296894559, 0.3333333333333333703, 0.3219752754296894559, 0.3333333333333333703, 0.3219752754296894559, 0.3333333333333333703, 0.3219752754296894559, 0.3333333333333333703, 0.3219752754296894559, 0.3333333333333333703, 0.3219752754296894559, 0.3333333333333333703, 0.3219752754296894559, 0.3333333333333333703, 0.3219752754296894559, 0.3333333333333333703, 0.3219752754296894559, 0.3333333333333333703, 0.3219752754296894559, 0.3333333333333333703, 0.3219752754296894559, 0.3333333333333333703, 0.3219752754296894559, 0.3333333333333333703, 0.3219752754296894559, 0.3333333333333333703, 0.3219752754296894559, 0.3333333333333333703, 0.3219752754296894559, 0.3333333333333333703, 0.3219752754296894559, 0.3333333333333333703, 0.3219752754296894559, 0.3333333333333333703, 0.3219752754296894559, 0.3333333333333333703, 0.3219752754296894559, 0.3333333333333333703, 0.3219752754296894559, 0.3333333333333333703, 0.3219752754296894559, 0.3333333333333333703, 0.3219752754296894559, 0.3333333333333333703, 0.3219752754296894559, 0.3333333333333333703, 0.3219752754296894559, 0.3333333333333333703, 0.3219752754296894559, 0.3333333333333333703, 0.3219752754296894559, 0.3333333333333333703, 0.3219752754296894559, 0.3333333333333333703, 0.3219752754296894559, 0.3333333333333333703, 0.3219752754296894559, 0.3333333333333333703, 0.3219752754296894559, 0.3333333333333333703, 0.3219752754296894559, 0.3333333333333333703, 0.3219752754296894559, 0.3333333333333333703, 0.3219752754296894559, 0.3333333333333333703, 0.3219752754296894559, 0.3333333333333333703, 0.3219752754296894559, 0.3333333333333333703, 0.3219752754296894559, 0.3333333333333333703, 0.3219752754296894559, 0.3333333333333333703, 0.3219752754296894559, 0.3333333333333333703, 0.3219752754296894559, 0.3333333333333333703, 0.3219752754296894559, 0.3333333333333333703, 0.3219752754296894559, 0.3333333333333333703, 0.3219752754296894559, 0.3333333333333333703, 0.3219752754296894559, 0.3333333333333333703, 0.3219752754296894559, 0.3333333333333333703, 0.3219752754296894559, 0.3333333333333333703, 0.3219752754296894559, 0.3333333333333333703, 0.3219752754296894559, 0.3333333333333333703, 0.3219752754296894559, 0.3333333333333333703, 0.3219752754296894559, 0.3333333333333333703, 0.3219752754296894559, 0.3333333333333333703, 0.3219752754296894559, 0.3333333333333333703, 0.3219752754296894559, 0.3333333333333333703, 0.3219752754296894559, 0.3333333333333333703, 0.3219752754296894559, 0.3333333333333333703, 0.3219752754296894559, 0.3333333333333333703, 0.3219752754296894559, 0.3333333333333333703, 0.3219752754296894559, 0.3333333333333333703, 0.3219752754296894559, 0.3333333333333333703, 0.3219752754296894559, 0.3333333333333333703, 0.3219752754296894559, 0.3333333333333333703, 0.3219752754296894559, 0.3333333333333333703, 0.3219752754296894559, 0.3333333333333333703, 0.3219752754296894559, 0.3333333333333333703, 0.3219752754296894559, 0.3333333333333333703, 0.3219752754296894559, 0.3333333333333333703, 0.3219752754296894559, 0.3333333333333333703, 0.3219752754296894559, 0.3333333333333333703, 0.3219752754296894559, 0.3333333333333333703, 0.3219752754296894559, 0.3333333333333333703, 0.3219752754296894559, 0.3333333333333333703, 0.3219752754296894559, 0.3333333333333333703, 0.3219752754296894559, 0.3333333333333333703, 0.3219752754296894559, 0.3333333333333333703, 0.3219752754296894559, 0.3333333333333333703, 0.3219752754296894559, 0.3333333333333333703, 0.3219752754296894559, 0.3333333333333333703, 0.3219752754296894559, 0.3333333333333333703, 0.3219752754296894559, 0.3333333333333333703, 0.3219752754296894559, 0.3333333333333333703, 0.3219752754296894559, 0.3333333333333333703, 0.3219752754296894559, 0.3333333333333333703, 0.3219752754296894559, 0.3333333333333333703, 0.3219752754296894559, 0.3333333333333333703, 0.3219752754296894559, 0.3333333333333333703, 0.3219752754296894559, 0.3333333333333333703, 0.3219752754296894559, 0.3333333333333333703, 0.3219752754296894559, 0.3333333333333333703, 0.3219752754296894559, 0.3333333333333333703, 0.3219752754296894559, 0.3333333333333333703, 0.3219752754296894559, 0.3333333333333333703, 0.3219752754296894559, 0.3333333333333333703, 0.3219752754296894559, 0.3333333333333333703, 0.3219752754296894559, 0.3333333333333333703, 0.3219752754296894559, 0.3333333333333333703, 0.3219752754296894559, 0.3333333333333333703, 0.3219752754296894559, 0.3333333333333333703, 0.3219752754296894559, 0.3333333333333333703, 0.3219752754296894559, 0.3333333333333333703, 0.3219752754296894559, 0.3333333333333333703, 0.3219752754296894559, 0.3333333333333333703, 0.3219752754296894559, 0.3333333333333333703, 0.3219752754296894559, 0.3333333333333333703, 0.3219752754296894559, 0.3333333333333333703, 0.3219752754296894559, 0.3333333333333333703, 0.3219752754296894559, 0.3333333333333333703, 0.3219752754296894559, 0.3333333333333333703, 0.3219752754296894559, 0.3333333333333333703, 0.3219752754296894559, 0.3333333333333333703, 0.3219752754296894559, 0.3333333333333333703, 0.3219752754296894559, 0.3333333333333333703, 0.3219752754296894559, 0.3333333333333333703, 0.3219752754296894559, 0.3333333333333333703, 0.3219752754296894559, 0.3333333333333333703, 0.3219752754296894559, 0.3333333333333333703, 0.3219752754296894559, 0.3333333333333333703),
 ( 1.000000000000000000, 0.9659258262890683122, 1.000000000000000000, 0.9659258262890683122, 1.000000000000000000, 0.9659258262890683122, 1.000000000000000000, 0.9659258262890683122, 1.000000000000000000, 0.9659258262890683122, 1.000000000000000000, 0.9659258262890683122, 1.000000000000000000, 0.9659258262890683122, 1.000000000000000000, 0.9659258262890683122, 1.000000000000000000, 0.9659258262890683122, 1.000000000000000000, 0.9659258262890683122, 1.000000000000000000, 0.9659258262890683122, 1.000000000000000000, 0.9659258262890683122, 1.000000000000000000, 0.9659258262890683122, 1.000000000000000000, 0.9659258262890683122, 1.000000000000000000, 0.9659258262890683122, 1.000000000000000000, 0.9659258262890683122, 1.000000000000000000, 0.9659258262890683122, 1.000000000000000000, 0.9659258262890683122, 1.000000000000000000, 0.9659258262890683122, 1.000000000000000000, 0.9659258262890683122, 1.000000000000000000, 0.9659258262890683122, 1.000000000000000000, 0.9659258262890683122, 1.000000000000000000, 0.9659258262890683122, 1.000000000000000000, 0.9659258262890683122, 1.000000000000000000, 0.9659258262890683122, 1.000000000000000000, 0.9659258262890683122, 1.000000000000000000, 0.9659258262890683122, 1.000000000000000000, 0.9659258262890683122, 1.000000000000000000, 0.9659258262890683122, 1.000000000000000000, 0.9659258262890683122, 1.000000000000000000, 0.9659258262890683122, 1.000000000000000000, 0.9659258262890683122, 1.000000000000000000, 0.9659258262890683122, 1.000000000000000000, 0.9659258262890683122, 1.000000000000000000, 0.9659258262890683122, 1.000000000000000000, 0.9659258262890683122, 1.000000000000000000, 0.9659258262890683122, 1.000000000000000000, 0.9659258262890683122, 1.000000000000000000, 0.9659258262890683122, 1.000000000000000000, 0.9659258262890683122, 1.000000000000000000, 0.9659258262890683122, 1.000000000000000000, 0.9659258262890683122, 1.000000000000000000, 0.9659258262890683122, 1.000000000000000000, 0.9659258262890683122, 1.000000000000000000, 0.9659258262890683122, 1.000000000000000000, 0.9659258262890683122, 1.000000000000000000, 0.9659258262890683122, 1.000000000000000000, 0.9659258262890683122, 1.000000000000000000, 0.9659258262890683122, 1.000000000000000000, 0.9659258262890683122, 1.000000000000000000, 0.9659258262890683122, 1.000000000000000000, 0.9659258262890683122, 1.000000000000000000, 0.9659258262890683122, 1.000000000000000000, 0.9659258262890683122, 1.000000000000000000, 0.9659258262890683122, 1.000000000000000000, 0.9659258262890683122, 1.000000000000000000, 0.9659258262890683122, 1.000000000000000000, 0.9659258262890683122, 1.000000000000000000, 0.9659258262890683122, 1.000000000000000000, 0.9659258262890683122, 1.000000000000000000, 0.9659258262890683122, 1.000000000000000000, 0.9659258262890683122, 1.000000000000000000, 0.9659258262890683122, 1.000000000000000000, 0.9659258262890683122, 1.000000000000000000, 0.9659258262890683122, 1.000000000000000000, 0.9659258262890683122, 1.000000000000000000, 0.9659258262890683122, 1.000000000000000000, 0.9659258262890683122, 1.000000000000000000, 0.9659258262890683122, 1.000000000000000000, 0.9659258262890683122, 1.000000000000000000, 0.9659258262890683122, 1.000000000000000000, 0.9659258262890683122, 1.000000000000000000, 0.9659258262890683122, 1.000000000000000000, 0.9659258262890683122, 1.000000000000000000, 0.9659258262890683122, 1.000000000000000000, 0.9659258262890683122, 1.000000000000000000, 0.9659258262890683122, 1.000000000000000000, 0.9659258262890683122, 1.000000000000000000, 0.9659258262890683122, 1.000000000000000000, 0.9659258262890683122, 1.000000000000000000, 0.9659258262890683122, 1.000000000000000000, 0.9659258262890683122, 1.000000000000000000, 0.9659258262890683122, 1.000000000000000000, 0.9659258262890683122, 1.000000000000000000, 0.9659258262890683122, 1.000000000000000000, 0.9659258262890683122, 1.000000000000000000, 0.9659258262890683122, 1.000000000000000000, 0.9659258262890683122, 1.000000000000000000, 0.9659258262890683122, 1.000000000000000000, 0.9659258262890683122, 1.000000000000000000, 0.9659258262890683122, 1.000000000000000000, 0.9659258262890683122, 1.000000000000000000, 0.9659258262890683122, 1.000000000000000000, 0.9659258262890683122, 1.000000000000000000, 0.9659258262890683122, 1.000000000000000000, 0.9659258262890683122, 1.000000000000000000, 0.9659258262890683122, 1.000000000000000000, 0.9659258262890683122, 1.000000000000000000, 0.9659258262890683122, 1.000000000000000000, 0.9659258262890683122, 1.000000000000000000, 0.9659258262890683122, 1.000000000000000000, 0.9659258262890683122, 1.000000000000000000, 0.9659258262890683122, 1.000000000000000000, 0.9659258262890683122, 1.000000000000000000, 0.9659258262890683122, 1.000000000000000000, 0.9659258262890683122, 1.000000000000000000, 0.9659258262890683122, 1.000000000000000000, 0.9659258262890683122, 1.000000000000000000, 0.9659258262890683122, 1.000000000000000000, 0.9659258262890683122, 1.000000000000000000, 0.9659258262890683122, 1.000000000000000000, 0.9659258262890683122, 1.000000000000000000, 0.9659258262890683122, 1.000000000000000000, 0.9659258262890683122, 1.000000000000000000, 0.9659258262890683122, 1.000000000000000000, 0.9659258262890683122, 1.000000000000000000, 0.9659258262890683122, 1.000000000000000000, 0.9659258262890683122, 1.000000000000000000, 0.9659258262890683122, 1.000000000000000000, 0.9659258262890683122, 1.000000000000000000, 0.9659258262890683122, 1.000000000000000000, 0.9659258262890683122, 1.000000000000000000, 0.9659258262890683122, 1.000000000000000000, 0.9659258262890683122, 1.000000000000000000, 0.9659258262890683122, 1.000000000000000000, 0.9659258262890683122, 1.000000000000000000, 0.9659258262890683122, 1.000000000000000000, 0.9659258262890683122, 1.000000000000000000, 0.9659258262890683122, 1.000000000000000000, 0.9659258262890683122, 1.000000000000000000, 0.9659258262890683122, 1.000000000000000000, 0.9659258262890683122, 1.000000000000000000, 0.9659258262890683122, 1.000000000000000000, 0.9659258262890683122, 1.000000000000000000, 0.9659258262890683122, 1.000000000000000000, 0.9659258262890683122, 1.000000000000000000, 0.9659258262890683122, 1.000000000000000000, 0.9659258262890683122, 1.000000000000000000, 0.9659258262890683122, 1.000000000000000000, 0.9659258262890683122, 1.000000000000000000, 0.9659258262890683122, 1.000000000000000000, 0.9659258262890683122, 1.000000000000000000, 0.9659258262890683122, 1.000000000000000000, 0.9659258262890683122, 1.000000000000000000, 0.9659258262890683122, 1.000000000000000000, 0.9659258262890683122, 1.000000000000000000, 0.9659258262890683122, 1.000000000000000000, 0.9659258262890683122, 1.000000000000000000, 0.9659258262890683122, 1.000000000000000000, 0.9659258262890683122, 1.000000000000000000, 0.9659258262890683122, 1.000000000000000000, 0.9659258262890683122, 1.000000000000000000, 0.9659258262890683122, 1.000000000000000000, 0.9659258262890683122, 1.000000000000000000, 0.9659258262890683122, 1.000000000000000000, 0.9659258262890683122, 1.000000000000000000, 0.9659258262890683122, 1.000000000000000000, 0.9659258262890683122, 1.000000000000000000, 0.9659258262890683122, 1.000000000000000000, 0.9659258262890683122, 1.000000000000000000, 0.9659258262890683122, 1.000000000000000000, 0.9659258262890683122, 1.000000000000000000, 0.9659258262890683122, 1.000000000000000000, 0.9659258262890683122, 1.000000000000000000, 0.9659258262890683122, 1.000000000000000000, 0.9659258262890683122, 1.000000000000000000, 0.9659258262890683122, 1.000000000000000000, 0.9659258262890683122, 1.000000000000000000, 0.9659258262890683122, 1.000000000000000000, 0.9659258262890683122, 1.000000000000000000, 0.9659258262890683122, 1.000000000000000000, 0.9659258262890683122, 1.000000000000000000, 0.9659258262890683122, 1.000000000000000000, 0.9659258262890683122, 1.000000000000000000, 0.9659258262890683122, 1.000000000000000000, 0.9659258262890683122, 1.000000000000000000, 0.9659258262890683122, 1.000000000000000000, 0.9659258262890683122, 1.000000000000000000, 0.9659258262890683122, 1.000000000000000000, 0.9659258262890683122, 1.000000000000000000, 0.9659258262890683122, 1.000000000000000000, 0.9659258262890683122, 1.000000000000000000, 0.9659258262890683122, 1.000000000000000000, 0.9659258262890683122, 1.000000000000000000, 0.9659258262890683122, 1.000000000000000000, 0.9659258262890683122, 1.000000000000000000, 0.9659258262890683122, 1.000000000000000000, 0.9659258262890683122, 1.000000000000000000, 0.9659258262890683122, 1.000000000000000000, 0.9659258262890683122, 1.000000000000000000, 0.9659258262890683122, 1.000000000000000000, 0.9659258262890683122, 1.000000000000000000, 0.9659258262890683122, 1.000000000000000000, 0.9659258262890683122, 1.000000000000000000, 0.9659258262890683122, 1.000000000000000000, 0.9659258262890683122, 1.000000000000000000, 0.9659258262890683122, 1.000000000000000000, 0.9659258262890683122, 1.000000000000000000, 0.9659258262890683122, 1.000000000000000000, 0.9659258262890683122, 1.000000000000000000, 0.9659258262890683122, 1.000000000000000000, 0.9659258262890683122, 1.000000000000000000, 0.9659258262890683122, 1.000000000000000000, 0.9659258262890683122, 1.000000000000000000, 0.9659258262890683122, 1.000000000000000000, 0.9659258262890683122, 1.000000000000000000, 0.9659258262890683122, 1.000000000000000000, 0.9659258262890683122, 1.000000000000000000, 0.9659258262890683122, 1.000000000000000000, 0.9659258262890683122, 1.000000000000000000, 0.9659258262890683122, 1.000000000000000000, 0.9659258262890683122, 1.000000000000000000, 0.9659258262890683122, 1.000000000000000000, 0.9659258262890683122, 1.000000000000000000, 0.9659258262890683122, 1.000000000000000000, 0.9659258262890683122, 1.000000000000000000, 0.9659258262890683122, 1.000000000000000000, 0.9659258262890683122, 1.000000000000000000, 0.9659258262890683122, 1.000000000000000000, 0.9659258262890683122, 1.000000000000000000, 0.9659258262890683122, 1.000000000000000000, 0.9659258262890683122, 1.000000000000000000, 0.9659258262890683122, 1.000000000000000000, 0.9659258262890683122, 1.000000000000000000, 0.9659258262890683122, 1.000000000000000000, 0.9659258262890683122, 1.000000000000000000, 0.9659258262890683122, 1.000000000000000000, 0.9659258262890683122, 1.000000000000000000) ) ) 
 REPRESENTATION_ITEM ( '' )  SURFACE ( )  );
#21940=CARTESIAN_POINT ( 'NONE',  ( -21.52544592524343514, 5.823673210054127303, 41.04057627198103120 ) ) ;
#21941=CARTESIAN_POINT ( 'NONE',  ( 15.72974639402176855, 15.80617190586768217, 66.87609039468568994 ) ) ;
#21943=CARTESIAN_POINT ( 'NONE',  ( 16.55341960407618274, -4.379528057220086978, 36.04275706135234714 ) ) ;
#21945=CARTESIAN_POINT ( 'NONE',  ( -9.474510206698964154, 16.51473224551069663, 90.41557627198103830 ) ) ;
#21947=CARTESIAN_POINT ( 'NONE',  ( -19.03943276465977164, 0.05219959533909376836, 26.24890960531435624 ) ) ;
#21948=CARTESIAN_POINT ( 'NONE',  ( -8.314922557960811034, -14.29746914071050412, 82.08224293864768129 ) ) ;
#21950=CARTESIAN_POINT ( 'NONE',  ( -0.05219959533909027116, -19.03943276465977164, 82.49890960531436690 ) ) ;
#21951=CARTESIAN_POINT ( 'NONE',  ( -9.564922557961040184, 16.46253265017147172, 107.9177570613523471 ) ) ;
#21952=CARTESIAN_POINT ( 'NONE',  ( 18.67979575497178502, 10.72451020669898547, 79.16557627198103830 ) ) ;
#21953=CARTESIAN_POINT ( 'NONE',  ( -13.97604488694527625, -13.89961937509977652, 46.87390960531435979 ) ) ;
#21954=CARTESIAN_POINT ( 'NONE',  ( 9.564922557961047289, -16.46253265017146816, 75.41775706135234714 ) ) ;
#21955=CARTESIAN_POINT ( 'NONE',  ( -18.62759615963255300, -10.81492255796106328, 19.16775706135234714 ) ) ;
#21956=CARTESIAN_POINT ( 'NONE',  ( 5.049401038298161559, -19.05341960407611168, 72.70724293864768129 ) ) ;
#21957=CARTESIAN_POINT ( 'NONE',  ( 16.46253265017160672, -9.564922557960803928, 103.3322429386476955 ) ) ;
#21958=EDGE_LOOP ( 'NONE', ( #92255, #31727, #20171, #184052, #194551, #101490, #20874, #110591 ) ) ;
#21959=CARTESIAN_POINT ( 'NONE',  ( -16.52544592524335698, -4.483927247898792601, 38.95942372801901854 ) ) ;
#21960=CARTESIAN_POINT ( 'NONE',  ( 5.823673210054125526, 21.52544592524343514, 104.7905762719810241 ) ) ;
#21961=CARTESIAN_POINT ( 'NONE',  ( -4.483927247898539470, -16.52544592524342804, 102.2905762719810383 ) ) ;
#21962=CARTESIAN_POINT ( 'NONE',  ( 13.97604488694527802, 13.89961937509977652, 89.37390960531436690 ) ) ;
#21963=CARTESIAN_POINT ( 'NONE',  ( 9.474510206698729675, 16.51473224551082808, 57.08442372801900433 ) ) ;
#21964=CARTESIAN_POINT ( 'NONE',  ( 21.53943276465977519, -0.05219959533907433946, 93.74890960531436690 ) ) ;
#21965=CARTESIAN_POINT ( 'NONE',  ( 5.719274019375991003, -21.55341960407610458, 72.70724293864769550 ) ) ;
#21966=CARTESIAN_POINT ( 'NONE',  ( 8.314922557960818139, 14.29746914071049879, 44.58224293864769550 ) ) ;
#21967=CARTESIAN_POINT ( 'NONE',  ( 13.97604488694548053, -13.89961937509957401, 20.62609039468567573 ) ) ;
#21968=CARTESIAN_POINT ( 'NONE',  ( 0.05219959533934541429, -16.53943276465976808, 65.00109039468568994 ) ) ;
#21969=CARTESIAN_POINT ( 'NONE',  ( -19.05341960407611168, -5.049401038298163336, 86.45724293864769550 ) ) ;
#21970=CARTESIAN_POINT ( 'NONE',  ( 5.049401038298161559, -19.05341960407611168, 42.70724293864767418 ) ) ;
#21971=CARTESIAN_POINT ( 'NONE',  ( -18.67979575497193778, 10.72451020669871902, 48.33442372801902565 ) ) ;
#21972=CARTESIAN_POINT ( 'NONE',  ( -21.53943276465977519, -0.05219959533937600094, 63.75109039468568284 ) ) ;
#21973=CARTESIAN_POINT ( 'NONE',  ( 5.049401038298161559, -19.05341960407611168, 57.70724293864769550 ) ) ;
#21974=CARTESIAN_POINT ( 'NONE',  ( 15.72974639402176855, 15.80617190586768217, 41.87609039468568284 ) ) ;
#21975=CARTESIAN_POINT ( 'NONE',  ( -19.03943276465977164, -0.05219959533935918106, 78.75109039468567573 ) ) ;
#21976=CARTESIAN_POINT ( 'NONE',  ( 9.564922557961047289, -16.46253265017146816, 70.41775706135233293 ) ) ;
#21977=CARTESIAN_POINT ( 'NONE',  ( 13.89961937509977652, -13.97604488694527269, 33.12390960531434558 ) ) ;
#21978=CARTESIAN_POINT ( 'NONE',  ( 12.06949235617739724, 12.14591786802326823, 91.87609039468568994 ) ) ;
#21979=CARTESIAN_POINT ( 'NONE',  ( 0.05219959533909260263, 19.03943276465977164, 49.99890960531435979 ) ) ;
#21981=CARTESIAN_POINT ( 'NONE',  ( -5.049401038298153566, 19.05341960407611168, 105.2072429386476671 ) ) ;
#21982=CARTESIAN_POINT ( 'NONE',  ( -19.03943276465977164, 0.05219959533909376836, 36.24890960531436690 ) ) ;
#21983=CARTESIAN_POINT ( 'NONE',  ( -10.81492255796078084, -18.62759615963271287, 82.08224293864768129 ) ) ;
#21984=CARTESIAN_POINT ( 'NONE',  ( -4.379528057220086978, -16.55341960407618274, 54.79275706135235424 ) ) ;
#21985=CARTESIAN_POINT ( 'NONE',  ( 9.564922557961047289, -16.46253265017146816, 20.41775706135233293 ) ) ;
#21986=CARTESIAN_POINT ( 'NONE',  ( 9.474510206698971260, -16.51473224551069308, 57.91557627198103120 ) ) ;
#21987=CARTESIAN_POINT ( 'NONE',  ( -12.06949235617756955, 12.14591786802309770, 50.62390960531435979 ) ) ;
#21988=CARTESIAN_POINT ( 'NONE',  ( -12.06949235617756955, 12.14591786802309770, 80.62390960531438111 ) ) ;
#21989=CARTESIAN_POINT ( 'NONE',  ( 16.46253265017160672, -9.564922557960803928, 73.33224293864769550 ) ) ;
#21990=CARTESIAN_POINT ( 'NONE',  ( -0.05219959533937732626, 21.53943276465977519, 37.50109039468568284 ) ) ;
#21991=CARTESIAN_POINT ( 'NONE',  ( -19.03943276465977164, 0.05219959533909376836, 86.24890960531436690 ) ) ;
#21992=CARTESIAN_POINT ( 'NONE',  ( 21.52544592524334988, 5.823673210054432836, 96.45942372801901854 ) ) ;
#21993=CARTESIAN_POINT ( 'NONE',  ( 8.314922557961029526, -14.29746914071037800, 80.41775706135234714 ) ) ;
#21994=CARTESIAN_POINT ( 'NONE',  ( 21.52544592524334988, 5.823673210054432836, 31.45942372801901854 ) ) ;
#21995=CARTESIAN_POINT ( 'NONE',  ( 19.03943276465977164, -0.05219959533909143690, 113.7489096053143669 ) ) ;
#21996=CARTESIAN_POINT ( 'NONE',  ( -15.72974639402197994, 15.80617190586746368, 85.62390960531436690 ) ) ;
#21997=CARTESIAN_POINT ( 'NONE',  ( -14.34966873604960291, -8.224510206698953496, 41.66557627198103120 ) ) ;
#21998=CARTESIAN_POINT ( 'NONE',  ( -9.564922557960796823, -16.46253265017161027, 37.08224293864768839 ) ) ;
#21999=CARTESIAN_POINT ( 'NONE',  ( 16.55341960407611168, 4.379528057220329451, 63.95724293864770260 ) ) ;
#22000=CARTESIAN_POINT ( 'NONE',  ( 15.72974639402199770, -15.80617190586745480, 28.12390960531435979 ) ) ;
#22001=CARTESIAN_POINT ( 'NONE',  ( 5.153800228976615827, -19.02544592524334988, 30.20942372801900433 ) ) ;
#22002=EDGE_CURVE ( 'NONE', #55198, #133171, #122580, .T. ) ;
#22003=CARTESIAN_POINT ( 'NONE',  ( 12.14591786802309770, 12.06949235617756955, 94.37390960531436690 ) ) ;
#22004=CARTESIAN_POINT ( 'NONE',  ( -19.03943276465977164, 0.05219959533909376836, 106.2489096053143669 ) ) ;
#22005=VERTEX_POINT ( 'NONE', #28190 ) ;
#22006=CARTESIAN_POINT ( 'NONE',  ( -0.05219959533934338120, 16.53943276465976808, 47.50109039468568994 ) ) ;
#22007=CARTESIAN_POINT ( 'NONE',  ( -13.89961937509977652, 13.97604488694528158, 55.62390960531434558 ) ) ;
#22009=CARTESIAN_POINT ( 'NONE',  ( -4.379528057220086978, -16.55341960407618274, 89.79275706135236135 ) ) ;
#22010=CARTESIAN_POINT ( 'NONE',  ( 13.97604488694548053, -13.89961937509957401, 110.6260903946856615 ) ) ;
#22011=CARTESIAN_POINT ( 'NONE',  ( 21.52544592524334988, 5.823673210054432836, 76.45942372801901854 ) ) ;
#22012=CARTESIAN_POINT ( 'NONE',  ( -13.97604488694527625, -13.89961937509977652, 76.87390960531433848 ) ) ;
#22013=CARTESIAN_POINT ( 'NONE',  ( -15.72974639402197994, 15.80617190586746368, 105.6239096053143669 ) ) ;
#22014=CARTESIAN_POINT ( 'NONE',  ( 0.05219959533934541429, -16.53943276465976808, 60.00109039468568284 ) ) ;
#22015=CARTESIAN_POINT ( 'NONE',  ( 12.06949235617757843, -12.14591786802309237, 113.1239096053143953 ) ) ;
#22016=CARTESIAN_POINT ( 'NONE',  ( -16.53943276465976808, -0.05219959533934237506, 18.75109039468568639 ) ) ;
#22017=CARTESIAN_POINT ( 'NONE',  ( -5.049401038297874678, -19.05341960407617918, 84.79275706135233293 ) ) ;
#22018=CARTESIAN_POINT ( 'NONE',  ( 10.72451020669898902, -18.67979575497178502, 77.91557627198102409 ) ) ;
#22019=CARTESIAN_POINT ( 'NONE',  ( -19.03943276465977164, -0.05219959533935918106, 48.75109039468566863 ) ) ;
#22021=CARTESIAN_POINT ( 'NONE',  ( 18.67979575497178502, 10.72451020669898547, 109.1655762719810383 ) ) ;
#22022=CARTESIAN_POINT ( 'NONE',  ( 17.50000000000147793, 3.254303733634570595, 27.47604106928601553 ) ) ;
#22023=CARTESIAN_POINT ( 'NONE',  ( -5.153800228976328057, -19.02544592524343514, 67.29057627198102409 ) ) ;
#22025=CARTESIAN_POINT ( 'NONE',  ( 14.34966873604972726, -8.224510206698740333, 20.83442372801901143 ) ) ;
#22027=CARTESIAN_POINT ( 'NONE',  ( 5.823673210054444382, -21.52544592524334988, 50.20942372801901854 ) ) ;
#22028=CARTESIAN_POINT ( 'NONE',  ( -5.823673210054116645, -21.52544592524344225, 97.29057627198105251 ) ) ;
#22029=CARTESIAN_POINT ( 'NONE',  ( 14.34966873604960469, 8.224510206698951720, 59.16557627198103120 ) ) ;
#22030=CARTESIAN_POINT ( 'NONE',  ( 13.89961937509977652, -13.97604488694527269, 68.12390960531436690 ) ) ;
#22031=CARTESIAN_POINT ( 'NONE',  ( -18.67979575497193778, 10.72451020669871902, 78.33442372801901854 ) ) ;
#22032=CARTESIAN_POINT ( 'NONE',  ( 16.53943276465976808, 0.05219959533934440121, 26.25109039468567573 ) ) ;
#22033=CARTESIAN_POINT ( 'NONE',  ( -5.153800228976607833, 19.02544592524334988, 32.70942372801899722 ) ) ;
#22034=CARTESIAN_POINT ( 'NONE',  ( 18.67979575497194134, -10.72451020669871369, 50.83442372801901143 ) ) ;
#22035=CARTESIAN_POINT ( 'NONE',  ( 21.52544592524334988, 5.823673210054432836, 21.45942372801901499 ) ) ;
#22036=CARTESIAN_POINT ( 'NONE',  ( 21.52544592524344225, -5.823673210054117533, 63.54057627198103830 ) ) ;
#22037=B_SPLINE_CURVE_WITH_KNOTS ( 'NONE', 3,
 ( #46387, #14057, #863, #170728, #136413, #108045 ),
 .UNSPECIFIED., .F., .F.,
 ( 4, 2, 4 ),
 ( 0.003989672132298100089, 0.004372778065220536345, 0.004755883998142971733 ),
 .UNSPECIFIED. ) ;
#22038=CARTESIAN_POINT ( 'NONE',  ( -5.049401038297874678, -19.05341960407617918, 99.79275706135234714 ) ) ;
#22039=CARTESIAN_POINT ( 'NONE',  ( -13.89961937509957401, -13.97604488694547875, 64.37609039468567573 ) ) ;
#22040=CARTESIAN_POINT ( 'NONE',  ( 15.72974639402176855, 15.80617190586768217, 86.87609039468568994 ) ) ;
#22041=CARTESIAN_POINT ( 'NONE',  ( -0.05219959533936034679, 19.03943276465977164, 47.50109039468566863 ) ) ;
#22042=CARTESIAN_POINT ( 'NONE',  ( -5.049401038298153566, 19.05341960407611168, 35.20724293864768839 ) ) ;
#22043=CARTESIAN_POINT ( 'NONE',  ( -5.823673210054116645, -21.52544592524344225, 57.29057627198103120 ) ) ;
#22044=CARTESIAN_POINT ( 'NONE',  ( 4.483927247898545687, 16.52544592524342804, 54.79057627198104541 ) ) ;
#22045=CARTESIAN_POINT ( 'NONE',  ( -17.26058549869091152, -6.457015423128557252, 26.37745837476068900 ) ) ;
#22046=CARTESIAN_POINT ( 'NONE',  ( -5.049401038297874678, -19.05341960407617918, 29.79275706135232227 ) ) ;
#22047=CARTESIAN_POINT ( 'NONE',  ( 4.483927247898790824, -16.52544592524335698, 85.20942372801901854 ) ) ;
#22048=CARTESIAN_POINT ( 'NONE',  ( 0.05219959533910956823, 16.53943276465976808, 54.99890960531435269 ) ) ;
#22049=CARTESIAN_POINT ( 'NONE',  ( -15.80617190586768217, 15.72974639402176855, 88.12609039468570415 ) ) ;
#22050=CARTESIAN_POINT ( 'NONE',  ( 21.53943276465977519, 0.05219959533937863772, 81.25109039468568994 ) ) ;
#22051=CARTESIAN_POINT ( 'NONE',  ( -21.52544592524343514, 5.823673210054127303, 81.04057627198102409 ) ) ;
#22052=CARTESIAN_POINT ( 'NONE',  ( 0.05219959533909260263, 19.03943276465977164, 39.99890960531436690 ) ) ;
#22053=CARTESIAN_POINT ( 'NONE',  ( 15.72974639402176855, 15.80617190586768217, 51.87609039468568284 ) ) ;
#22054=CARTESIAN_POINT ( 'NONE',  ( -5.153800228976328057, -19.02544592524343514, 37.29057627198102409 ) ) ;
#22055=CARTESIAN_POINT ( 'NONE',  ( 0.05219959533909260263, 19.03943276465977164, 49.99890960531435979 ) ) ;
#22056=CARTESIAN_POINT ( 'NONE',  ( 4.379528057220339221, -16.55341960407611168, 102.7072429386476955 ) ) ;
#22057=CARTESIAN_POINT ( 'NONE',  ( -16.46253265017160317, 9.564922557960807481, 95.83224293864769550 ) ) ;
#22058=CARTESIAN_POINT ( 'NONE',  ( 12.06949235617757843, -12.14591786802309237, 48.12390960531436690 ) ) ;
#22059=CARTESIAN_POINT ( 'NONE',  ( -16.52544592524342804, 4.483927247898546575, 106.0405762719810525 ) ) ;
#22060=CARTESIAN_POINT ( 'NONE',  ( 18.67979575497178502, 10.72451020669898547, 84.16557627198103830 ) ) ;
#22061=CARTESIAN_POINT ( 'NONE',  ( 21.52544592524334988, 5.823673210054432836, 21.45942372801901499 ) ) ;
#22063=CARTESIAN_POINT ( 'NONE',  ( -0.05219959533934338120, 16.53943276465976808, 37.50109039468568284 ) ) ;
#22065=CARTESIAN_POINT ( 'NONE',  ( -18.67979575497178146, -10.72451020669898902, 66.66557627198102409 ) ) ;
#22066=CARTESIAN_POINT ( 'NONE',  ( -21.52544592524334988, -5.823673210054445271, 88.95942372801901854 ) ) ;
#22067=CARTESIAN_POINT ( 'NONE',  ( -19.03943276465977164, 0.05219959533909376836, 91.24890960531436690 ) ) ;
#22068=CARTESIAN_POINT ( 'NONE',  ( 21.55341960407619695, -5.719274019375665929, 26.04275706135235779 ) ) ;
#22069=CARTESIAN_POINT ( 'NONE',  ( -15.80617190586745835, -15.72974639402198527, 26.87390960531435979 ) ) ;
#22070=CARTESIAN_POINT ( 'NONE',  ( -12.14591786802326823, 12.06949235617739902, 88.12609039468570415 ) ) ;
#22071=CARTESIAN_POINT ( 'NONE',  ( 18.62759615963255655, 10.81492255796105972, 81.66775706135236135 ) ) ;
#22072=CARTESIAN_POINT ( 'NONE',  ( 5.049401038297881783, 19.05341960407617563, 22.29275706135233648 ) ) ;
#22073=CARTESIAN_POINT ( 'NONE',  ( -16.53943276465976808, -0.05219959533934237506, 73.75109039468567573 ) ) ;
#22074=CARTESIAN_POINT ( 'NONE',  ( -15.80617190586768217, 15.72974639402176855, 28.12609039468568284 ) ) ;
#22075=CARTESIAN_POINT ( 'NONE',  ( -9.564922557960796823, -16.46253265017161027, 32.08224293864769550 ) ) ;
#22076=CARTESIAN_POINT ( 'NONE',  ( -5.719274019375665041, -21.55341960407619695, 109.7927570613523613 ) ) ;
#22077=CARTESIAN_POINT ( 'NONE',  ( 13.89961937509977652, -13.97604488694527269, 103.1239096053143527 ) ) ;
#22078=CARTESIAN_POINT ( 'NONE',  ( 0.05219959533907565091, 21.53943276465977519, 99.99890960531436690 ) ) ;
#22079=CARTESIAN_POINT ( 'NONE',  ( 17.50000000001358202, -5.500000000000038192, 88.29690382535061133 ) ) ;
#22080=CARTESIAN_POINT ( 'NONE',  ( -0.05219959533907301413, -21.53943276465977519, 62.49890960531436690 ) ) ;
#22081=CARTESIAN_POINT ( 'NONE',  ( -12.06949235617739369, -12.14591786802326823, 49.37609039468569705 ) ) ;
#22082=CARTESIAN_POINT ( 'NONE',  ( 16.52544592524342804, -4.483927247898539470, 53.54057627198103120 ) ) ;
#22084=CARTESIAN_POINT ( 'NONE',  ( 9.474510206698729675, 16.51473224551082808, 72.08442372801900433 ) ) ;
#22087=CARTESIAN_POINT ( 'NONE',  ( -0.05219959533934338120, 16.53943276465976808, 22.50109039468567573 ) ) ;
#22088=CARTESIAN_POINT ( 'NONE',  ( -21.52544592524343514, 5.823673210054127303, 96.04057627198102409 ) ) ;
#22089=CARTESIAN_POINT ( 'NONE',  ( 14.29746914071049879, -8.314922557960816363, 68.33224293864769550 ) ) ;
#22090=CARTESIAN_POINT ( 'NONE',  ( 16.51473224551069308, 9.474510206698969483, 104.1655762719810241 ) ) ;
#22091=CARTESIAN_POINT ( 'NONE',  ( -8.314922557961024197, 14.29746914071037800, 37.91775706135235424 ) ) ;
#22092=CARTESIAN_POINT ( 'NONE',  ( 0.05219959533909260263, 19.03943276465977164, 59.99890960531436690 ) ) ;
#22093=CARTESIAN_POINT ( 'NONE',  ( 10.81492255796106328, -18.62759615963255655, 35.41775706135234003 ) ) ;
#22094=CARTESIAN_POINT ( 'NONE',  ( 19.02544592524334988, 5.153800228976608722, 96.45942372801897591 ) ) ;
#22095=CARTESIAN_POINT ( 'NONE',  ( 19.03943276465977164, -0.05219959533909143690, 98.74890960531436690 ) ) ;
#22096=CARTESIAN_POINT ( 'NONE',  ( -5.049401038298153566, 19.05341960407611168, 90.20724293864766707 ) ) ;
#22097=CARTESIAN_POINT ( 'NONE',  ( 21.52544592524344225, -5.823673210054117533, 88.54057627198103830 ) ) ;
#22098=CARTESIAN_POINT ( 'NONE',  ( -19.05341960407611168, -5.049401038298163336, 46.45724293864768129 ) ) ;
#22100=CARTESIAN_POINT ( 'NONE',  ( -4.379528057220328563, 16.55341960407611168, 70.20724293864769550 ) ) ;
#22101=CARTESIAN_POINT ( 'NONE',  ( 13.97604488694527802, 13.89961937509977652, 99.37390960531436690 ) ) ;
#22102=CARTESIAN_POINT ( 'NONE',  ( -17.97161686093721400, 5.500000000000142997, 60.99637206859166838 ) ) ;
#22103=CARTESIAN_POINT ( 'NONE',  ( -19.02544592524334988, -5.153800228976617603, 83.95942372801901854 ) ) ;
#22104=CARTESIAN_POINT ( 'NONE',  ( 15.72974639402199770, -15.80617190586745480, 88.12390960531436690 ) ) ;
#22105=CARTESIAN_POINT ( 'NONE',  ( 16.46253265017146816, 9.564922557961045513, 46.66775706135233293 ) ) ;
#22106=CARTESIAN_POINT ( 'NONE',  ( -18.62759615963270932, 10.81492255796079327, 25.83224293864769194 ) ) ;
#22108=CARTESIAN_POINT ( 'NONE',  ( 5.823673210054125526, 21.52544592524343514, 44.79057627198103120 ) ) ;
#22109=CARTESIAN_POINT ( 'NONE',  ( 5.049401038298161559, -19.05341960407611168, 87.70724293864769550 ) ) ;
#22110=CARTESIAN_POINT ( 'NONE',  ( 15.72974639402176855, 15.80617190586768217, 61.87609039468568284 ) ) ;
#22111=CARTESIAN_POINT ( 'NONE',  ( -19.03943276465977164, 0.05219959533909376836, 36.24890960531436690 ) ) ;
#22112=CARTESIAN_POINT ( 'NONE',  ( -4.483927247898539470, -16.52544592524342804, 67.29057627198103830 ) ) ;
#22113=CARTESIAN_POINT ( 'NONE',  ( 16.52544592524335698, 4.483927247898782831, 21.45942372801901499 ) ) ;
#22114=CARTESIAN_POINT ( 'NONE',  ( 5.719274019375673035, 21.55341960407619339, 47.29275706135234003 ) ) ;
#22115=ORIENTED_EDGE ( 'NONE', *, *, #199224, .F. ) ;
#22116=CARTESIAN_POINT ( 'NONE',  ( 0.05219959533909260263, 19.03943276465977164, 114.9989096053143669 ) ) ;
#22117=CARTESIAN_POINT ( 'NONE',  ( 0.05219959533936267826, -19.03943276465977164, 80.00109039468567573 ) ) ;
#22119=CARTESIAN_POINT ( 'NONE',  ( 5.719274019375673035, 21.55341960407619339, 22.29275706135235069 ) ) ;
#22121=CARTESIAN_POINT ( 'NONE',  ( -15.80617190586768217, 15.72974639402176855, 113.1260903946856899 ) ) ;
#22122=CARTESIAN_POINT ( 'NONE',  ( 5.153800228976335163, 19.02544592524342804, 54.79057627198103120 ) ) ;
#22123=CARTESIAN_POINT ( 'NONE',  ( -5.153800228976607833, 19.02544592524334988, 22.70942372801899012 ) ) ;
#22124=CARTESIAN_POINT ( 'NONE',  ( -16.55341960407617563, 4.379528057220093196, 103.5427570613523613 ) ) ;
#22125=CARTESIAN_POINT ( 'NONE',  ( 0.05219959533909260263, 19.03943276465977164, 104.9989096053143669 ) ) ;
#22126=CARTESIAN_POINT ( 'NONE',  ( -18.67979575497193778, 10.72451020669871902, 78.33442372801901854 ) ) ;
#22128=CARTESIAN_POINT ( 'NONE',  ( -17.50000000000002487, -4.049696124445982370, 35.81960329334061299 ) ) ;
#22129=CARTESIAN_POINT ( 'NONE',  ( 30.00000000000000000, 5.499999999999992895, 102.5000000000000142 ) ) ;
#22130=CARTESIAN_POINT ( 'NONE',  ( -21.53943276465977519, -0.05219959533937600094, 73.75109039468567573 ) ) ;
#22131=CARTESIAN_POINT ( 'NONE',  ( -18.62759615963255300, -10.81492255796106328, 99.16775706135234714 ) ) ;
#22133=CARTESIAN_POINT ( 'NONE',  ( -5.153800228976328057, -19.02544592524343514, 87.29057627198103830 ) ) ;
#22135=CARTESIAN_POINT ( 'NONE',  ( 9.474510206698729675, 16.51473224551082808, 22.08442372801899722 ) ) ;
#22137=CARTESIAN_POINT ( 'NONE',  ( -19.02544592524342804, 5.153800228976336051, 41.04057627198103120 ) ) ;
#22138=CARTESIAN_POINT ( 'NONE',  ( -18.67979575497178146, -10.72451020669898902, 51.66557627198102409 ) ) ;
#22139=CARTESIAN_POINT ( 'NONE',  ( -12.06949235617739369, -12.14591786802326823, 104.3760903946856899 ) ) ;
#22140=CARTESIAN_POINT ( 'NONE',  ( -12.14591786802309592, -12.06949235617757132, 96.87390960531436690 ) ) ;
#22141=CARTESIAN_POINT ( 'NONE',  ( 0.05219959533909260263, 19.03943276465977164, 84.99890960531436690 ) ) ;
#22142=CARTESIAN_POINT ( 'NONE',  ( -0.05219959533937732626, 21.53943276465977519, 97.50109039468567573 ) ) ;
#22143=CARTESIAN_POINT ( 'NONE',  ( -0.05219959533909027116, -19.03943276465977164, 42.49890960531435269 ) ) ;
#22144=CARTESIAN_POINT ( 'NONE',  ( 4.379528057220339221, -16.55341960407611168, 92.70724293864770971 ) ) ;
#22145=CARTESIAN_POINT ( 'NONE',  ( 21.52544592524334988, 5.823673210054432836, 56.45942372801902565 ) ) ;
#22146=CARTESIAN_POINT ( 'NONE',  ( 21.52544592524344225, -5.823673210054117533, 83.54057627198102409 ) ) ;
#22147=CARTESIAN_POINT ( 'NONE',  ( -19.05341960407617563, 5.049401038297882671, 53.54275706135231871 ) ) ;
#22148=CARTESIAN_POINT ( 'NONE',  ( -5.153800228976328057, -19.02544592524343514, 47.29057627198102409 ) ) ;
#22149=CARTESIAN_POINT ( 'NONE',  ( 9.474510206698971260, -16.51473224551069308, 97.91557627198102409 ) ) ;
#22150=CARTESIAN_POINT ( 'NONE',  ( 8.224510206698953496, -14.34966873604960469, 72.91557627198103830 ) ) ;
#22151=CARTESIAN_POINT ( 'NONE',  ( -13.97604488694547697, 13.89961937509957934, 43.12609039468566152 ) ) ;
#22152=CARTESIAN_POINT ( 'NONE',  ( 19.02544592524343514, -5.153800228976328945, 68.54057627198103830 ) ) ;
#22153=CARTESIAN_POINT ( 'NONE',  ( 16.52544592524342804, -4.483927247898539470, 43.54057627198103830 ) ) ;
#22154=CARTESIAN_POINT ( 'NONE',  ( -5.049401038297874678, -19.05341960407617918, 79.79275706135233293 ) ) ;
#22155=CARTESIAN_POINT ( 'NONE',  ( -19.53037848336980886, 5.499999999999899636, 84.85532783611448338 ) ) ;
#22156=CARTESIAN_POINT ( 'NONE',  ( -21.55341960407610458, -5.719274019375992779, 31.45724293864769550 ) ) ;
#22157=CARTESIAN_POINT ( 'NONE',  ( 14.29746914071049879, -8.314922557960816363, 98.33224293864769550 ) ) ;
#22158=CARTESIAN_POINT ( 'NONE',  ( -17.50000000000001421, -3.305555262949453788, 25.37482847843392264 ) ) ;
#22159=CARTESIAN_POINT ( 'NONE',  ( -16.46253265017160317, 9.564922557960807481, 60.83224293864769550 ) ) ;
#22160=CARTESIAN_POINT ( 'NONE',  ( 15.72974639402199770, -15.80617190586745480, 58.12390960531435979 ) ) ;
#22161=CARTESIAN_POINT ( 'NONE',  ( 19.03943276465977164, -0.05219959533909143690, 33.74890960531435979 ) ) ;
#22162=CARTESIAN_POINT ( 'NONE',  ( 12.06949235617739724, 12.14591786802326823, 81.87609039468568994 ) ) ;
#22163=CARTESIAN_POINT ( 'NONE',  ( 9.564922557960805705, 16.46253265017160317, 54.58224293864769550 ) ) ;
#22164=CARTESIAN_POINT ( 'NONE',  ( 19.03943276465977164, 0.05219959533936151252, 41.25109039468566152 ) ) ;
#22165=CARTESIAN_POINT ( 'NONE',  ( -5.719274019375665041, -21.55341960407619695, 74.79275706135234714 ) ) ;
#22166=CARTESIAN_POINT ( 'NONE',  ( 5.823673210054125526, 21.52544592524343514, 54.79057627198104541 ) ) ;
#22167=CARTESIAN_POINT ( 'NONE',  ( -13.97604488694527625, -13.89961937509977652, 26.87390960531434558 ) ) ;
#22168=CARTESIAN_POINT ( 'NONE',  ( -8.314922557961024197, 14.29746914071037800, 82.91775706135234714 ) ) ;
#22169=CARTESIAN_POINT ( 'NONE',  ( -19.02544592524334988, -5.153800228976617603, 103.9594237280190043 ) ) ;
#22170=CARTESIAN_POINT ( 'NONE',  ( 30.00000000000000000, 5.499999999999992895, 37.50000000000000000 ) ) ;
#22172=CARTESIAN_POINT ( 'NONE',  ( 5.823673210054125526, 21.52544592524343514, 44.79057627198103120 ) ) ;
#22173=CARTESIAN_POINT ( 'NONE',  ( -21.53943276465977519, -0.05219959533937600094, 78.75109039468568994 ) ) ;
#22174=CARTESIAN_POINT ( 'NONE',  ( -16.55341960407611168, -4.379528057220339221, 51.45724293864770260 ) ) ;
#22175=CARTESIAN_POINT ( 'NONE',  ( 16.55341960407611168, 4.379528057220329451, 58.95724293864770971 ) ) ;
#22176=CARTESIAN_POINT ( 'NONE',  ( -21.52544592524343514, 5.823673210054127303, 81.04057627198102409 ) ) ;
#22177=CARTESIAN_POINT ( 'NONE',  ( 21.53943276465977519, -0.05219959533907433946, 73.74890960531433848 ) ) ;
#22179=CARTESIAN_POINT ( 'NONE',  ( -10.72451020669898014, 18.67979575497178502, 30.41557627198101699 ) ) ;
#22180=CARTESIAN_POINT ( 'NONE',  ( -14.29746914071037622, -8.314922557961029526, 59.16775706135234714 ) ) ;
#22181=CARTESIAN_POINT ( 'NONE',  ( 14.29746914071049879, -8.314922557960816363, 83.33224293864769550 ) ) ;
#22182=CARTESIAN_POINT ( 'NONE',  ( 16.46253265017160672, -9.564922557960803928, 28.33224293864769550 ) ) ;
#22184=CARTESIAN_POINT ( 'NONE',  ( 17.60779699588838199, 5.500000000000005329, 48.84981316670106111 ) ) ;
#22186=CARTESIAN_POINT ( 'NONE',  ( 4.483927247898790824, -16.52544592524335698, 85.20942372801901854 ) ) ;
#22187=CARTESIAN_POINT ( 'NONE',  ( 10.72451020669898902, -18.67979575497178502, 112.9155762719810383 ) ) ;
#22188=CARTESIAN_POINT ( 'NONE',  ( -13.97604488694527625, -13.89961937509977652, 81.87390960531436690 ) ) ;
#22189=CARTESIAN_POINT ( 'NONE',  ( -21.53943276465977519, -0.05219959533937600094, 58.75109039468568994 ) ) ;
#22190=CARTESIAN_POINT ( 'NONE',  ( -9.564922557960796823, -16.46253265017161027, 107.0822429386476955 ) ) ;
#22193=CARTESIAN_POINT ( 'NONE',  ( -21.55341960407619339, 5.719274019375674811, 48.54275706135234714 ) ) ;
#22194=CARTESIAN_POINT ( 'NONE',  ( -5.049401038298153566, 19.05341960407611168, 35.20724293864768839 ) ) ;
#22195=CARTESIAN_POINT ( 'NONE',  ( 19.03943276465977164, -0.05219959533909143690, 108.7489096053143527 ) ) ;
#22196=CARTESIAN_POINT ( 'NONE',  ( -9.564922557961040184, 16.46253265017147172, 47.91775706135233293 ) ) ;
#22197=CARTESIAN_POINT ( 'NONE',  ( 5.823673210054444382, -21.52544592524334988, 30.20942372801902565 ) ) ;
#22198=CARTESIAN_POINT ( 'NONE',  ( 19.05341960407617918, -5.049401038297876454, 51.04275706135231871 ) ) ;
#22199=CARTESIAN_POINT ( 'NONE',  ( 13.89961937509977652, -13.97604488694527269, 28.12390960531435624 ) ) ;
#22200=CARTESIAN_POINT ( 'NONE',  ( 16.55341960407618274, -4.379528057220086978, 91.04275706135236135 ) ) ;
#22201=CARTESIAN_POINT ( 'NONE',  ( -13.89961937509957401, -13.97604488694547875, 59.37609039468566863 ) ) ;
#22202=CARTESIAN_POINT ( 'NONE',  ( -4.379528057220086978, -16.55341960407618274, 104.7927570613523898 ) ) ;
#22203=LINE ( 'NONE', #131369, #28078 ) ;
#22204=CARTESIAN_POINT ( 'NONE',  ( -5.153800228976328057, -19.02544592524343514, 87.29057627198103830 ) ) ;
#22205=CARTESIAN_POINT ( 'NONE',  ( 15.72974639402176855, 15.80617190586768217, 91.87609039468568994 ) ) ;
#22206=CARTESIAN_POINT ( 'NONE',  ( 5.719274019375673035, 21.55341960407619339, 102.2927570613523613 ) ) ;
#22209=CARTESIAN_POINT ( 'NONE',  ( 19.03943276465977164, -0.05219959533909143690, 98.74890960531436690 ) ) ;
#22210=CARTESIAN_POINT ( 'NONE',  ( -10.81492255796105439, 18.62759615963255655, 77.91775706135231871 ) ) ;
#22211=CARTESIAN_POINT ( 'NONE',  ( 14.29746914071037800, 8.314922557961029526, 21.66775706135235069 ) ) ;
#22212=CARTESIAN_POINT ( 'NONE',  ( -9.474510206698964154, 16.51473224551069663, 85.41557627198102409 ) ) ;
#22213=CARTESIAN_POINT ( 'NONE',  ( -21.53943276465977519, 0.05219959533907696930, 26.24890960531435624 ) ) ;
#22214=CARTESIAN_POINT ( 'NONE',  ( -13.89961937509977652, 13.97604488694528158, 90.62390960531432427 ) ) ;
#22215=CARTESIAN_POINT ( 'NONE',  ( -16.20579543436679160, -7.371946100355096121, 90.56520834171878676 ) ) ;
#22216=CARTESIAN_POINT ( 'NONE',  ( -5.049401038298153566, 19.05341960407611168, 75.20724293864769550 ) ) ;
#22217=CARTESIAN_POINT ( 'NONE',  ( -19.02544592524342804, 5.153800228976336051, 61.04057627198103120 ) ) ;
#22218=CARTESIAN_POINT ( 'NONE',  ( 4.483927247898790824, -16.52544592524335698, 95.20942372801903275 ) ) ;
#22220=CARTESIAN_POINT ( 'NONE',  ( 13.89961937509957401, 13.97604488694547697, 66.87609039468567573 ) ) ;
#22221=CARTESIAN_POINT ( 'NONE',  ( -16.51473224551069308, -9.474510206698971260, 86.66557627198102409 ) ) ;
#22222=CARTESIAN_POINT ( 'NONE',  ( -14.34966873604960291, -8.224510206698953496, 86.66557627198102409 ) ) ;
#22223=CARTESIAN_POINT ( 'NONE',  ( -5.823673210054116645, -21.52544592524344225, 32.29057627198102409 ) ) ;
#22224=CARTESIAN_POINT ( 'NONE',  ( -5.719274019375978568, 21.55341960407610458, 25.20724293864769550 ) ) ;
#22225=CARTESIAN_POINT ( 'NONE',  ( -16.53943276465976808, 0.05219959533911058130, 111.2489096053143669 ) ) ;
#22227=CARTESIAN_POINT ( 'NONE',  ( -13.89961937509957401, -13.97604488694547875, 44.37609039468566863 ) ) ;
#22228=CARTESIAN_POINT ( 'NONE',  ( -8.314922557960811034, -14.29746914071050412, 27.08224293864769550 ) ) ;
#22229=CARTESIAN_POINT ( 'NONE',  ( -5.153800228976328057, -19.02544592524343514, 107.2905762719810383 ) ) ;
#22230=CARTESIAN_POINT ( 'NONE',  ( -21.53943276465977519, -0.05219959533937600094, 68.75109039468568994 ) ) ;
#22231=CARTESIAN_POINT ( 'NONE',  ( 5.719274019375991003, -21.55341960407610458, 62.70724293864769550 ) ) ;
#22232=CARTESIAN_POINT ( 'NONE',  ( 0.05219959533937995610, -21.53943276465977519, 35.00109039468568284 ) ) ;
#22233=CARTESIAN_POINT ( 'NONE',  ( -5.823673210054116645, -21.52544592524344225, 77.29057627198102409 ) ) ;
#22234=CARTESIAN_POINT ( 'NONE',  ( -15.80617190586768217, 15.72974639402176855, 43.12609039468568284 ) ) ;
#22235=CARTESIAN_POINT ( 'NONE',  ( 0.05219959533910956823, 16.53943276465976808, 104.9989096053143669 ) ) ;
#22236=CARTESIAN_POINT ( 'NONE',  ( 5.049401038297881783, 19.05341960407617563, 72.29275706135234714 ) ) ;
#22237=CARTESIAN_POINT ( 'NONE',  ( -5.049401038298153566, 19.05341960407611168, 40.20724293864768839 ) ) ;
#22238=CARTESIAN_POINT ( 'NONE',  ( 16.55341960407611168, 4.379528057220329451, 88.95724293864769550 ) ) ;
#22239=CARTESIAN_POINT ( 'NONE',  ( 9.564922557960805705, 16.46253265017160317, 94.58224293864769550 ) ) ;
#22240=CARTESIAN_POINT ( 'NONE',  ( 9.564922557960805705, 16.46253265017160317, 94.58224293864769550 ) ) ;
#22241=CARTESIAN_POINT ( 'NONE',  ( 16.55341960407611168, 4.379528057220329451, 108.9572429386476955 ) ) ;
#22242=CARTESIAN_POINT ( 'NONE',  ( -14.34966873604960291, -8.224510206698953496, 41.66557627198103120 ) ) ;
#22243=CARTESIAN_POINT ( 'NONE',  ( 8.314922557961029526, -14.29746914071037800, 95.41775706135234714 ) ) ;
#22244=CARTESIAN_POINT ( 'NONE',  ( 19.05341960407611168, 5.049401038298154454, 48.95724293864768129 ) ) ;
#22245=CARTESIAN_POINT ( 'NONE',  ( 16.51473224551069308, 9.474510206698969483, 24.16557627198102765 ) ) ;
#22246=CARTESIAN_POINT ( 'NONE',  ( -19.03943276465977164, -0.05219959533935918106, 18.75109039468567218 ) ) ;
#22247=FACE_OUTER_BOUND ( 'NONE', #164526, .T. ) ;
#22248=CARTESIAN_POINT ( 'NONE',  ( 4.379528057220092307, 16.55341960407617563, 112.2927570613523471 ) ) ;
#22249=CARTESIAN_POINT ( 'NONE',  ( -15.80617190586768217, 15.72974639402176855, 43.12609039468568284 ) ) ;
#22250=DIRECTION ( 'NONE',  ( 0.000000000000000000, 0.000000000000000000, 1.000000000000000000 ) ) ;
#22251=CARTESIAN_POINT ( 'NONE',  ( -16.52544592524335698, -4.483927247898792601, 48.95942372801902565 ) ) ;
#22252=CARTESIAN_POINT ( 'NONE',  ( 14.34966873604960469, 8.224510206698951720, 34.16557627198102409 ) ) ;
#22253=CARTESIAN_POINT ( 'NONE',  ( -9.564922557960796823, -16.46253265017161027, 52.08224293864768839 ) ) ;
#22254=CARTESIAN_POINT ( 'NONE',  ( -16.55341960407617563, 4.379528057220093196, 103.5427570613523613 ) ) ;
#22255=CARTESIAN_POINT ( 'NONE',  ( 12.14591786802327356, -12.06949235617739191, 20.62609039468568639 ) ) ;
#22256=CARTESIAN_POINT ( 'NONE',  ( -5.153800228976328057, -19.02544592524343514, 52.29057627198100988 ) ) ;
#22257=CARTESIAN_POINT ( 'NONE',  ( 16.53943276465976808, -0.05219959533910856209, 113.7489096053143527 ) ) ;
#22258=CARTESIAN_POINT ( 'NONE',  ( 21.53943276465977519, -0.05219959533907433946, 113.7489096053143527 ) ) ;
#22259=CARTESIAN_POINT ( 'NONE',  ( 16.51473224551069308, 9.474510206698969483, 44.16557627198103120 ) ) ;
#22260=CARTESIAN_POINT ( 'NONE',  ( -13.97604488694527625, -13.89961937509977652, 106.8739096053143669 ) ) ;
#22261=CARTESIAN_POINT ( 'NONE',  ( -19.03943276465977164, 0.05219959533909376836, 26.24890960531435624 ) ) ;
#22262=CARTESIAN_POINT ( 'NONE',  ( -19.03943276465977164, 0.05219959533909376836, 111.2489096053143669 ) ) ;
#22264=CARTESIAN_POINT ( 'NONE',  ( 16.51473224551069308, 9.474510206698969483, 99.16557627198102409 ) ) ;
#22265=CARTESIAN_POINT ( 'NONE',  ( 18.67979575497194134, -10.72451020669871369, 40.83442372801901854 ) ) ;
#22266=CARTESIAN_POINT ( 'NONE',  ( 14.34966873604960469, 8.224510206698951720, 99.16557627198100988 ) ) ;
#22267=CARTESIAN_POINT ( 'NONE',  ( 0.05219959533909260263, 19.03943276465977164, 109.9989096053143669 ) ) ;
#22268=CARTESIAN_POINT ( 'NONE',  ( -5.049401038297874678, -19.05341960407618274, 69.79275706135233293 ) ) ;
#22269=CARTESIAN_POINT ( 'NONE',  ( 14.29746914071037800, 8.314922557961029526, 61.66775706135235424 ) ) ;
#22270=CARTESIAN_POINT ( 'NONE',  ( -10.81492255796105439, 18.62759615963255655, 97.91775706135236135 ) ) ;
#22271=CARTESIAN_POINT ( 'NONE',  ( -16.52544592524335698, -4.483927247898792601, 58.95942372801902565 ) ) ;
#22272=CARTESIAN_POINT ( 'NONE',  ( 9.474510206698971260, -16.51473224551069308, 82.91557627198103830 ) ) ;
#22273=CARTESIAN_POINT ( 'NONE',  ( -16.53943276465976808, -0.05219959533934237506, 38.75109039468567573 ) ) ;
#22274=CARTESIAN_POINT ( 'NONE',  ( -0.05219959533936034679, 19.03943276465977164, 107.5010903946856615 ) ) ;
#22275=CARTESIAN_POINT ( 'NONE',  ( -16.53943276465976808, -0.05219959533934237506, 83.75109039468568994 ) ) ;
#22276=CARTESIAN_POINT ( 'NONE',  ( -19.05341960407617563, 5.049401038297882671, 93.54275706135234714 ) ) ;
#22277=CARTESIAN_POINT ( 'NONE',  ( 19.05341960407611168, 5.049401038298154454, 78.95724293864769550 ) ) ;
#22278=CARTESIAN_POINT ( 'NONE',  ( 15.80617190586746368, 15.72974639402197994, 94.37390960531436690 ) ) ;
#22279=CARTESIAN_POINT ( 'NONE',  ( 4.483927247898545687, 16.52544592524342804, 94.79057627198105251 ) ) ;
#22280=CARTESIAN_POINT ( 'NONE',  ( -16.46253265017146816, -9.564922557961047289, 104.1677570613523329 ) ) ;
#22281=CARTESIAN_POINT ( 'NONE',  ( 14.34966873604972726, -8.224510206698740333, 70.83442372801901854 ) ) ;
#22283=CARTESIAN_POINT ( 'NONE',  ( 19.02544592524334988, 5.153800228976608722, 71.45942372801900433 ) ) ;
#22284=CARTESIAN_POINT ( 'NONE',  ( -16.53943276465976808, 0.05219959533911058130, 31.24890960531435979 ) ) ;
#22285=CARTESIAN_POINT ( 'NONE',  ( -14.29746914071049879, 8.314922557960819915, 90.83224293864769550 ) ) ;
#22286=CARTESIAN_POINT ( 'NONE',  ( 9.564922557961047289, -16.46253265017146816, 35.41775706135233293 ) ) ;
#22287=CARTESIAN_POINT ( 'NONE',  ( -17.26172910966779739, 6.454744622555856459, 90.80646908649227100 ) ) ;
#22288=CARTESIAN_POINT ( 'NONE',  ( 0.05219959533937995610, -21.53943276465977519, 30.00109039468568284 ) ) ;
#22289=CARTESIAN_POINT ( 'NONE',  ( -9.474510206698720793, -16.51473224551083518, 99.58442372801900433 ) ) ;
#22290=CARTESIAN_POINT ( 'NONE',  ( -16.46253265017160317, 9.564922557960807481, 110.8322429386476955 ) ) ;
#22291=CARTESIAN_POINT ( 'NONE',  ( -19.03943276465977164, 0.05219959533909376836, 96.24890960531436690 ) ) ;
#22292=CARTESIAN_POINT ( 'NONE',  ( 5.719274019375673035, 21.55341960407619339, 97.29275706135234714 ) ) ;
#22293=CARTESIAN_POINT ( 'NONE',  ( 5.153800228976335163, 19.02544592524342804, 79.79057627198102409 ) ) ;
#22294=CARTESIAN_POINT ( 'NONE',  ( -5.719274019375978568, 21.55341960407610458, 45.20724293864769550 ) ) ;
#22295=CARTESIAN_POINT ( 'NONE',  ( -16.55341960407611168, -4.379528057220339221, 96.45724293864770971 ) ) ;
#22296=CARTESIAN_POINT ( 'NONE',  ( -5.049401038298153566, 19.05341960407611168, 60.20724293864768129 ) ) ;
#22297=CARTESIAN_POINT ( 'NONE',  ( -16.51473224551069308, -9.474510206698971260, 21.66557627198102765 ) ) ;
#22298=CARTESIAN_POINT ( 'NONE',  ( 18.67979575497194134, -10.72451020669871369, 30.83442372801902209 ) ) ;
#22299=CARTESIAN_POINT ( 'NONE',  ( -21.52544592524334988, -5.823673210054445271, 58.95942372801902565 ) ) ;
#22300=CARTESIAN_POINT ( 'NONE',  ( -16.46253265017160317, 9.564922557960807481, 50.83224293864770260 ) ) ;
#22301=CARTESIAN_POINT ( 'NONE',  ( 14.29746914071037800, 8.314922557961029526, 81.66775706135236135 ) ) ;
#22302=CARTESIAN_POINT ( 'NONE',  ( 21.52544592524344225, -5.823673210054117533, 108.5405762719810241 ) ) ;
#22304=CARTESIAN_POINT ( 'NONE',  ( -15.72974639402197994, 15.80617190586746368, 110.6239096053143669 ) ) ;
#22305=CARTESIAN_POINT ( 'NONE',  ( -13.97604488694547697, 13.89961937509957934, 53.12609039468565442 ) ) ;
#22306=CARTESIAN_POINT ( 'NONE',  ( 5.153800228976335163, 19.02544592524342804, 64.79057627198100988 ) ) ;
#22307=CARTESIAN_POINT ( 'NONE',  ( -5.049401038297874678, -19.05341960407617918, 34.79275706135233293 ) ) ;
#22308=CARTESIAN_POINT ( 'NONE',  ( -5.719274019375665041, -21.55341960407619695, 64.79275706135234714 ) ) ;
#22309=CARTESIAN_POINT ( 'NONE',  ( -18.62759615963270932, 10.81492255796079327, 70.83224293864770971 ) ) ;
#22310=CARTESIAN_POINT ( 'NONE',  ( -8.314922557960811034, -14.29746914071050412, 52.08224293864768839 ) ) ;
#22311=CARTESIAN_POINT ( 'NONE',  ( 5.823673210054444382, -21.52544592524334988, 90.20942372801903275 ) ) ;
#22312=CARTESIAN_POINT ( 'NONE',  ( -9.474510206698720793, -16.51473224551083518, 24.58442372801900078 ) ) ;
#22313=CARTESIAN_POINT ( 'NONE',  ( -14.29746914071049879, 8.314922557960819915, 65.83224293864769550 ) ) ;
#22314=CARTESIAN_POINT ( 'NONE',  ( 16.53943276465976808, -0.05219959533910856209, 113.7489096053143527 ) ) ;
#22315=CARTESIAN_POINT ( 'NONE',  ( 9.474510206698729675, 16.51473224551082808, 62.08442372801899722 ) ) ;
#22316=CARTESIAN_POINT ( 'NONE',  ( -8.224510206698735004, -14.34966873604973081, 109.5844237280190328 ) ) ;
#22317=CARTESIAN_POINT ( 'NONE',  ( 10.81492255796106328, -18.62759615963255655, 80.41775706135234714 ) ) ;
#22318=CARTESIAN_POINT ( 'NONE',  ( -13.89961937509957401, -13.97604488694547875, 49.37609039468567573 ) ) ;
#22319=CARTESIAN_POINT ( 'NONE',  ( 21.53943276465977519, -0.05219959533907433946, 53.74890960531437401 ) ) ;
#22320=CARTESIAN_POINT ( 'NONE',  ( 5.823673210054444382, -21.52544592524334988, 50.20942372801901854 ) ) ;
#22322=CARTESIAN_POINT ( 'NONE',  ( -21.55341960407610458, -5.719274019375992779, 106.4572429386477097 ) ) ;
#22323=CARTESIAN_POINT ( 'NONE',  ( 5.049401038297881783, 19.05341960407617563, 102.2927570613523045 ) ) ;
#22324=CARTESIAN_POINT ( 'NONE',  ( 4.379528057220092307, 16.55341960407617563, 62.29275706135236845 ) ) ;
#22325=CARTESIAN_POINT ( 'NONE',  ( -30.00000000000000000, -1.163414459189985801E-14, 95.00000000000000000 ) ) ;
#22326=CARTESIAN_POINT ( 'NONE',  ( -21.53943276465977519, 0.05219959533907696930, 111.2489096053143669 ) ) ;
#22327=CARTESIAN_POINT ( 'NONE',  ( -14.29746914071049879, 8.314922557960819915, 95.83224293864770971 ) ) ;
#22328=CARTESIAN_POINT ( 'NONE',  ( -16.81555441253552985, -7.025013491695489165, 99.36314554665746357 ) ) ;
#22329=CARTESIAN_POINT ( 'NONE',  ( 12.06949235617739724, 12.14591786802326823, 26.87609039468567218 ) ) ;
#22330=CARTESIAN_POINT ( 'NONE',  ( -10.72451020669898014, 18.67979575497178502, 55.41557627198102409 ) ) ;
#22331=CARTESIAN_POINT ( 'NONE',  ( -0.05219959533934338120, 16.53943276465976808, 92.50109039468567573 ) ) ;
#22333=CARTESIAN_POINT ( 'NONE',  ( -12.06949235617739369, -12.14591786802326823, 64.37609039468568994 ) ) ;
#22334=CARTESIAN_POINT ( 'NONE',  ( -18.67979575497193778, 10.72451020669871902, 38.33442372801900433 ) ) ;
#22335=CARTESIAN_POINT ( 'NONE',  ( -15.72974639402197994, 15.80617190586746368, 60.62390960531437401 ) ) ;
#22336=CARTESIAN_POINT ( 'NONE',  ( 16.55341960407618274, -4.379528057220086978, 81.04275706135236135 ) ) ;
#22337=CARTESIAN_POINT ( 'NONE',  ( 5.153800228976335163, 19.02544592524342804, 99.79057627198102409 ) ) ;
#22338=CARTESIAN_POINT ( 'NONE',  ( -5.823673210054431948, 21.52544592524334988, 67.70942372801901854 ) ) ;
#22339=CARTESIAN_POINT ( 'NONE',  ( 5.719274019375991003, -21.55341960407610458, 47.70724293864770260 ) ) ;
#22340=CARTESIAN_POINT ( 'NONE',  ( 18.62759615963271287, -10.81492255796078972, 33.33224293864769550 ) ) ;
#22342=CARTESIAN_POINT ( 'NONE',  ( 19.02544592524334988, 5.153800228976608722, 51.45942372801900433 ) ) ;
#22343=CARTESIAN_POINT ( 'NONE',  ( -8.224510206698735004, -14.34966873604973081, 59.58442372801901854 ) ) ;
#22344=CARTESIAN_POINT ( 'NONE',  ( 21.55341960407610458, 5.719274019375980345, 38.95724293864768839 ) ) ;
#22346=CARTESIAN_POINT ( 'NONE',  ( -19.02544592524342804, 5.153800228976336051, 101.0405762719810241 ) ) ;
#22347=CARTESIAN_POINT ( 'NONE',  ( 14.34966873604972726, -8.224510206698740333, 110.8344237280190043 ) ) ;
#22349=CARTESIAN_POINT ( 'NONE',  ( 14.29746914071049879, -8.314922557960816363, 108.3322429386477097 ) ) ;
#22350=CARTESIAN_POINT ( 'NONE',  ( 18.67979575497178502, 10.72451020669898547, 54.16557627198103120 ) ) ;
#22351=CARTESIAN_POINT ( 'NONE',  ( 13.97604488694527802, 13.89961937509977652, 39.37390960531435269 ) ) ;
#22352=CARTESIAN_POINT ( 'NONE',  ( -4.379528057220086978, -16.55341960407618274, 89.79275706135236135 ) ) ;
#22353=CARTESIAN_POINT ( 'NONE',  ( 10.81492255796106328, -18.62759615963255655, 30.41775706135234358 ) ) ;
#22354=CARTESIAN_POINT ( 'NONE',  ( -19.02544592524334988, -5.153800228976617603, 83.95942372801901854 ) ) ;
#22355=CARTESIAN_POINT ( 'NONE',  ( -8.314922557960811034, -14.29746914071050412, 107.0822429386476955 ) ) ;
#22356=CARTESIAN_POINT ( 'NONE',  ( 5.049401038298161559, -19.05341960407611168, 52.70724293864767418 ) ) ;
#22357=CARTESIAN_POINT ( 'NONE',  ( -13.89961937509977652, 13.97604488694528158, 30.62390960531435269 ) ) ;
#22359=CARTESIAN_POINT ( 'NONE',  ( -5.153800228976328057, -19.02544592524343514, 72.29057627198102409 ) ) ;
#22360=CARTESIAN_POINT ( 'NONE',  ( -12.14591786802326823, 12.06949235617739902, 68.12609039468567573 ) ) ;
#22361=CARTESIAN_POINT ( 'NONE',  ( 10.81492255796106328, -18.62759615963255655, 110.4177570613523756 ) ) ;
#22362=CARTESIAN_POINT ( 'NONE',  ( 0.05219959533907565091, 21.53943276465977519, 44.99890960531435979 ) ) ;
#22363=CARTESIAN_POINT ( 'NONE',  ( 14.29746914071037800, 8.314922557961029526, 71.66775706135234714 ) ) ;
#22364=CARTESIAN_POINT ( 'NONE',  ( 13.89961937509957401, 13.97604488694547697, 46.87609039468565442 ) ) ;
#22365=CARTESIAN_POINT ( 'NONE',  ( -9.564922557961040184, 16.46253265017147172, 72.91775706135233293 ) ) ;
#22367=CARTESIAN_POINT ( 'NONE',  ( 5.719274019375673035, 21.55341960407619339, 57.29275706135234714 ) ) ;
#22368=CARTESIAN_POINT ( 'NONE',  ( -19.03943276465977164, 0.05219959533909376836, 61.24890960531436690 ) ) ;
#22369=CARTESIAN_POINT ( 'NONE',  ( 9.474510206698971260, -16.51473224551069308, 37.91557627198102409 ) ) ;
#22370=CARTESIAN_POINT ( 'NONE',  ( -13.89961937509957401, -13.97604488694547875, 59.37609039468566863 ) ) ;
#22371=CARTESIAN_POINT ( 'NONE',  ( -9.474510206698964154, 16.51473224551069663, 115.4155762719810241 ) ) ;
#22372=CARTESIAN_POINT ( 'NONE',  ( -13.89961937509977652, 13.97604488694528158, 95.62390960531436690 ) ) ;
#22373=CARTESIAN_POINT ( 'NONE',  ( -4.483927247898539470, -16.52544592524342804, 57.29057627198103120 ) ) ;
#22374=CARTESIAN_POINT ( 'NONE',  ( -15.80617190586745835, -15.72974639402198527, 51.87390960531437401 ) ) ;
#22376=CARTESIAN_POINT ( 'NONE',  ( 5.719274019375673035, 21.55341960407619339, 112.2927570613523471 ) ) ;
#22378=CARTESIAN_POINT ( 'NONE',  ( 13.97604488694527802, 13.89961937509977652, 54.37390960531435979 ) ) ;
#22382=CARTESIAN_POINT ( 'NONE',  ( -12.14591786802326823, 12.06949235617739902, 73.12609039468567573 ) ) ;
#22383=CARTESIAN_POINT ( 'NONE',  ( -21.55341960407610458, -5.719274019375992779, 96.45724293864770971 ) ) ;
#22384=CARTESIAN_POINT ( 'NONE',  ( -12.06949235617756955, 12.14591786802309770, 55.62390960531436690 ) ) ;
#22385=CARTESIAN_POINT ( 'NONE',  ( 16.46253265017160672, -9.564922557960803928, 38.33224293864768839 ) ) ;
#22387=CARTESIAN_POINT ( 'NONE',  ( 15.80617190586769283, -15.72974639402175789, 35.62609039468568994 ) ) ;
#22388=CARTESIAN_POINT ( 'NONE',  ( 0.05219959533936267826, -19.03943276465977164, 55.00109039468566863 ) ) ;
#22389=CARTESIAN_POINT ( 'NONE',  ( 19.03943276465977164, -0.05219959533909143690, 43.74890960531435979 ) ) ;
#22390=CARTESIAN_POINT ( 'NONE',  ( 18.67979575497194134, -10.72451020669871369, 90.83442372801901854 ) ) ;
#22391=CARTESIAN_POINT ( 'NONE',  ( 17.31747979337949062, 6.344076630961054342, 98.87944868065186199 ) ) ;
#22393=CARTESIAN_POINT ( 'NONE',  ( -12.06949235617756955, 12.14591786802309770, 40.62390960531435269 ) ) ;
#22395=CARTESIAN_POINT ( 'NONE',  ( -21.53943276465977519, 0.05219959533907696930, 36.24890960531435979 ) ) ;
#22397=CARTESIAN_POINT ( 'NONE',  ( 0.05219959533909260263, 19.03943276465977164, 99.99890960531436690 ) ) ;
#22398=CARTESIAN_POINT ( 'NONE',  ( -8.314922557960811034, -14.29746914071050412, 87.08224293864769550 ) ) ;
#22399=CARTESIAN_POINT ( 'NONE',  ( -4.483927247898782831, 16.52544592524335698, 27.70942372801901854 ) ) ;
#22400=CARTESIAN_POINT ( 'NONE',  ( 4.379528057220092307, 16.55341960407617563, 112.2927570613523471 ) ) ;
#22402=CARTESIAN_POINT ( 'NONE',  ( -16.46253265017160317, 9.564922557960807481, 100.8322429386477097 ) ) ;
#22403=CARTESIAN_POINT ( 'NONE',  ( -15.80617190586745835, -15.72974639402198527, 101.8739096053143811 ) ) ;
#22404=CARTESIAN_POINT ( 'NONE',  ( 12.14591786802309770, 12.06949235617756955, 29.37390960531435269 ) ) ;
#22405=CARTESIAN_POINT ( 'NONE',  ( -19.05341960407611168, -5.049401038298163336, 101.4572429386476955 ) ) ;
#22406=CARTESIAN_POINT ( 'NONE',  ( -0.05219959533936034679, 19.03943276465977164, 97.50109039468567573 ) ) ;
#22407=CARTESIAN_POINT ( 'NONE',  ( -13.89961937509957401, -13.97604488694547875, 19.37609039468566507 ) ) ;
#22408=CARTESIAN_POINT ( 'NONE',  ( 0.05219959533907565091, 21.53943276465977519, 89.99890960531438111 ) ) ;
#22409=CARTESIAN_POINT ( 'NONE',  ( 10.72451020669898902, -18.67979575497178502, 47.91557627198102409 ) ) ;
#22410=CARTESIAN_POINT ( 'NONE',  ( -5.153800228976328057, -19.02544592524343514, 57.29057627198103120 ) ) ;
#22411=CARTESIAN_POINT ( 'NONE',  ( 12.06949235617757843, -12.14591786802309237, 33.12390960531435979 ) ) ;
#22412=CARTESIAN_POINT ( 'NONE',  ( -13.89961937509977652, 13.97604488694528158, 80.62390960531436690 ) ) ;
#22415=CARTESIAN_POINT ( 'NONE',  ( -16.46253265017146816, -9.564922557961047289, 24.16775706135233648 ) ) ;
#22416=CARTESIAN_POINT ( 'NONE',  ( 12.06949235617757843, -12.14591786802309237, 93.12390960531436690 ) ) ;
#22417=CARTESIAN_POINT ( 'NONE',  ( 21.52544592524334988, 5.823673210054432836, 21.45942372801901499 ) ) ;
#22419=CARTESIAN_POINT ( 'NONE',  ( 8.224510206698742110, 14.34966873604972548, 102.0844237280190185 ) ) ;
#22420=CARTESIAN_POINT ( 'NONE',  ( 16.46253265017160672, -9.564922557960803928, 23.33224293864769194 ) ) ;
#22421=CARTESIAN_POINT ( 'NONE',  ( 19.05341960407611168, 5.049401038298154454, 73.95724293864768129 ) ) ;
#22422=CARTESIAN_POINT ( 'NONE',  ( 16.46253265017146816, 9.564922557961045513, 91.66775706135234714 ) ) ;
#22423=CARTESIAN_POINT ( 'NONE',  ( 14.29746914071049879, -8.314922557960816363, 43.33224293864769550 ) ) ;
#22424=CARTESIAN_POINT ( 'NONE',  ( -21.52544592524334988, -5.823673210054445271, 53.95942372801900433 ) ) ;
#22426=CARTESIAN_POINT ( 'NONE',  ( -10.72451020669870658, -18.67979575497194134, 89.58442372801901854 ) ) ;
#22427=CARTESIAN_POINT ( 'NONE',  ( -0.05219959533909027116, -19.03943276465977164, 42.49890960531435269 ) ) ;
#22428=CARTESIAN_POINT ( 'NONE',  ( 9.474510206698971260, -16.51473224551069308, 57.91557627198103120 ) ) ;
#22430=CARTESIAN_POINT ( 'NONE',  ( -5.719274019375665041, -21.55341960407619695, 89.79275706135236135 ) ) ;
#22431=CARTESIAN_POINT ( 'NONE',  ( 4.379528057220092307, 16.55341960407617563, 57.29275706135234714 ) ) ;
#22432=CARTESIAN_POINT ( 'NONE',  ( 5.719274019375673035, 21.55341960407619339, 87.29275706135236135 ) ) ;
#22433=CARTESIAN_POINT ( 'NONE',  ( 5.719274019375991003, -21.55341960407610458, 22.70724293864769194 ) ) ;
#22434=ORIENTED_EDGE ( 'NONE', *, *, #91774, .F. ) ;
#22435=CARTESIAN_POINT ( 'NONE',  ( -0.05219959533936034679, 19.03943276465977164, 92.50109039468566152 ) ) ;
#22436=CARTESIAN_POINT ( 'NONE',  ( -18.67979575497193778, 10.72451020669871902, 68.33442372801900433 ) ) ;
#22437=CARTESIAN_POINT ( 'NONE',  ( -0.05219959533934338120, 16.53943276465976808, 42.50109039468567573 ) ) ;
#22438=CARTESIAN_POINT ( 'NONE',  ( 0.05219959533907565091, 21.53943276465977519, 89.99890960531438111 ) ) ;
#22439=CARTESIAN_POINT ( 'NONE',  ( 19.03943276465977164, 0.05219959533936151252, 81.25109039468567573 ) ) ;
#22440=CARTESIAN_POINT ( 'NONE',  ( -19.05341960407611168, -5.049401038298163336, 71.45724293864766707 ) ) ;
#22441=CARTESIAN_POINT ( 'NONE',  ( -13.97604488694547697, 13.89961937509957934, 98.12609039468566152 ) ) ;
#22442=CARTESIAN_POINT ( 'NONE',  ( -16.46253265017146816, -9.564922557961047289, 109.1677570613523471 ) ) ;
#22443=CARTESIAN_POINT ( 'NONE',  ( -16.53943276465976808, 0.05219959533911058130, 46.24890960531435979 ) ) ;
#22444=CARTESIAN_POINT ( 'NONE',  ( 16.51473224551083163, -9.474510206698727899, 70.83442372801900433 ) ) ;
#22445=CARTESIAN_POINT ( 'NONE',  ( -16.52544592524335698, -4.483927247898792601, 58.95942372801902565 ) ) ;
#22447=CARTESIAN_POINT ( 'NONE',  ( 9.474510206698971260, -16.51473224551069308, 37.91557627198102409 ) ) ;
#22448=CARTESIAN_POINT ( 'NONE',  ( 19.03943276465977164, -0.05219959533909143690, 58.74890960531435979 ) ) ;
#22449=CARTESIAN_POINT ( 'NONE',  ( -4.379528057220086978, -16.55341960407618274, 64.79275706135234714 ) ) ;
#22452=CARTESIAN_POINT ( 'NONE',  ( -19.02544592524342804, 5.153800228976336051, 101.0405762719810241 ) ) ;
#22453=CARTESIAN_POINT ( 'NONE',  ( -5.153800228976328057, -19.02544592524343514, 22.29057627198102765 ) ) ;
#22455=CARTESIAN_POINT ( 'NONE',  ( -0.05219959533934338120, 16.53943276465976808, 22.50109039468567573 ) ) ;
#22457=CARTESIAN_POINT ( 'NONE',  ( -5.823673210054116645, -21.52544592524344225, 37.29057627198102409 ) ) ;
#22458=CARTESIAN_POINT ( 'NONE',  ( 9.564922557961047289, -16.46253265017146816, 25.41775706135234003 ) ) ;
#22459=CARTESIAN_POINT ( 'NONE',  ( 16.52544592524335698, 4.483927247898782831, 26.45942372801901854 ) ) ;
#22460=CARTESIAN_POINT ( 'NONE',  ( 13.89961937509977652, -13.97604488694527269, 33.12390960531434558 ) ) ;
#22461=CARTESIAN_POINT ( 'NONE',  ( -19.02544592524342804, 5.153800228976336051, 56.04057627198100988 ) ) ;
#22462=CARTESIAN_POINT ( 'NONE',  ( -0.05219959533907301413, -21.53943276465977519, 82.49890960531436690 ) ) ;
#22463=CARTESIAN_POINT ( 'NONE',  ( -9.474510206698964154, 16.51473224551069663, 100.4155762719810241 ) ) ;
#22464=CARTESIAN_POINT ( 'NONE',  ( 5.153800228976335163, 19.02544592524342804, 54.79057627198103120 ) ) ;
#22466=CARTESIAN_POINT ( 'NONE',  ( -5.153800228976607833, 19.02544592524334988, 77.70942372801900433 ) ) ;
#22467=CARTESIAN_POINT ( 'NONE',  ( -8.314922557960811034, -14.29746914071050412, 67.08224293864770971 ) ) ;
#22468=CARTESIAN_POINT ( 'NONE',  ( 5.719274019375991003, -21.55341960407610458, 42.70724293864770260 ) ) ;
#22469=CARTESIAN_POINT ( 'NONE',  ( 18.62759615963255655, 10.81492255796105972, 111.6677570613523613 ) ) ;
#22470=CARTESIAN_POINT ( 'NONE',  ( 21.55341960407610458, 5.719274019375980345, 103.9572429386476813 ) ) ;
#22471=CARTESIAN_POINT ( 'NONE',  ( 18.62759615963255655, 10.81492255796105972, 76.66775706135234714 ) ) ;
#22472=CARTESIAN_POINT ( 'NONE',  ( 21.53943276465977519, 0.05219959533937863772, 71.25109039468568994 ) ) ;
#22473=CARTESIAN_POINT ( 'NONE',  ( -16.46253265017160317, 9.564922557960807481, 105.8322429386476955 ) ) ;
#22474=CARTESIAN_POINT ( 'NONE',  ( 14.34966873604972726, -8.224510206698740333, 105.8344237280190328 ) ) ;
#22475=CARTESIAN_POINT ( 'NONE',  ( 21.52544592524334988, 5.823673210054432836, 81.45942372801900433 ) ) ;
#22476=CARTESIAN_POINT ( 'NONE',  ( 0.05219959533909260263, 19.03943276465977164, 59.99890960531436690 ) ) ;
#22477=CARTESIAN_POINT ( 'NONE',  ( 0.05219959533937995610, -21.53943276465977519, 25.00109039468567218 ) ) ;
#22478=CARTESIAN_POINT ( 'NONE',  ( -16.51473224551069308, -9.474510206698971260, 66.66557627198102409 ) ) ;
#22479=CARTESIAN_POINT ( 'NONE',  ( 0.05219959533910956823, 16.53943276465976808, 74.99890960531435269 ) ) ;
#22480=CARTESIAN_POINT ( 'NONE',  ( -14.34966873604960291, -8.224510206698953496, 46.66557627198102409 ) ) ;
#22481=CARTESIAN_POINT ( 'NONE',  ( 5.823673210054125526, 21.52544592524343514, 54.79057627198104541 ) ) ;
#22482=CARTESIAN_POINT ( 'NONE',  ( -16.51473224551069308, -9.474510206698971260, 66.66557627198102409 ) ) ;
#22483=CARTESIAN_POINT ( 'NONE',  ( -21.52544592524343514, 5.823673210054127303, 66.04057627198103830 ) ) ;
#22484=CARTESIAN_POINT ( 'NONE',  ( -5.153800228976607833, 19.02544592524334988, 62.70942372801899722 ) ) ;
#22485=CARTESIAN_POINT ( 'NONE',  ( -19.03943276465977164, -0.05219959533935918106, 23.75109039468566152 ) ) ;
#22486=CARTESIAN_POINT ( 'NONE',  ( -16.55341960407611168, -4.379528057220339221, 66.45724293864768129 ) ) ;
#22487=CARTESIAN_POINT ( 'NONE',  ( -5.823673210054116645, -21.52544592524344225, 57.29057627198103120 ) ) ;
#22490=LINE ( 'NONE', #84137, #185093 ) ;
#22491=CARTESIAN_POINT ( 'NONE',  ( -12.14591786802326823, 12.06949235617739902, 93.12609039468568994 ) ) ;
#22493=CARTESIAN_POINT ( 'NONE',  ( 5.153800228976615827, -19.02544592524334988, 85.20942372801900433 ) ) ;
#22494=CARTESIAN_POINT ( 'NONE',  ( -8.314922557960811034, -14.29746914071050412, 72.08224293864769550 ) ) ;
#22495=CARTESIAN_POINT ( 'NONE',  ( -18.87255363501902394, -5.499999999999947597, 61.32513748171826506 ) ) ;
#22496=CARTESIAN_POINT ( 'NONE',  ( -5.153800228976328057, -19.02544592524343514, 62.29057627198100988 ) ) ;
#22497=CARTESIAN_POINT ( 'NONE',  ( 4.483927247898545687, 16.52544592524342804, 54.79057627198104541 ) ) ;
#22498=CARTESIAN_POINT ( 'NONE',  ( 19.03943276465977164, -0.05219959533909143690, 83.74890960531436690 ) ) ;
#22499=CARTESIAN_POINT ( 'NONE',  ( 16.51473224551083163, -9.474510206698727899, 80.83442372801899012 ) ) ;
#22500=CARTESIAN_POINT ( 'NONE',  ( 5.049401038298161559, -19.05341960407611168, 57.70724293864769550 ) ) ;
#22501=CARTESIAN_POINT ( 'NONE',  ( -9.564922557960796823, -16.46253265017161027, 82.08224293864768129 ) ) ;
#22502=CARTESIAN_POINT ( 'NONE',  ( -9.474510206698964154, 16.51473224551069663, 70.41557627198102409 ) ) ;
#22503=CARTESIAN_POINT ( 'NONE',  ( 15.80617190586746368, 15.72974639402197994, 59.37390960531436690 ) ) ;
#22505=CARTESIAN_POINT ( 'NONE',  ( 13.89961937509977652, -13.97604488694527269, 48.12390960531435979 ) ) ;
#22506=CARTESIAN_POINT ( 'NONE',  ( -18.62759615963270932, 10.81492255796079327, 60.83224293864769550 ) ) ;
#22507=CARTESIAN_POINT ( 'NONE',  ( 0.05219959533936267826, -19.03943276465977164, 85.00109039468567573 ) ) ;
#22508=CARTESIAN_POINT ( 'NONE',  ( 8.224510206698742110, 14.34966873604972548, 112.0844237280190185 ) ) ;
#22509=CARTESIAN_POINT ( 'NONE',  ( -19.02544592524334988, -5.153800228976617603, 33.95942372801897591 ) ) ;
#22510=CARTESIAN_POINT ( 'NONE',  ( 4.483927247898790824, -16.52544592524335698, 60.20942372801902565 ) ) ;
#22511=CARTESIAN_POINT ( 'NONE',  ( -4.379528057220086978, -16.55341960407618274, 99.79275706135234714 ) ) ;
#22512=CARTESIAN_POINT ( 'NONE',  ( 19.48894818550243002, -5.500000000000108358, 42.60307310435238293 ) ) ;
#22513=CARTESIAN_POINT ( 'NONE',  ( -4.379528057220086978, -16.55341960407618274, 79.79275706135236135 ) ) ;
#22514=CARTESIAN_POINT ( 'NONE',  ( -16.46253265017160317, 9.564922557960807481, 115.8322429386477097 ) ) ;
#22515=CARTESIAN_POINT ( 'NONE',  ( 9.564922557960805705, 16.46253265017160317, 34.58224293864770260 ) ) ;
#22516=CARTESIAN_POINT ( 'NONE',  ( 8.224510206698742110, 14.34966873604972548, 42.08442372801901854 ) ) ;
#22517=CARTESIAN_POINT ( 'NONE',  ( -13.97604488694527625, -13.89961937509977652, 46.87390960531435979 ) ) ;
#22518=CARTESIAN_POINT ( 'NONE',  ( 21.55341960407619695, -5.719274019375665929, 41.04275706135236135 ) ) ;
#22519=CARTESIAN_POINT ( 'NONE',  ( -16.52544592524335698, -4.483927247898792601, 48.95942372801902565 ) ) ;
#22520=CARTESIAN_POINT ( 'NONE',  ( 4.379528057220092307, 16.55341960407617563, 112.2927570613523471 ) ) ;
#22521=CARTESIAN_POINT ( 'NONE',  ( 9.564922557960805705, 16.46253265017160317, 34.58224293864770260 ) ) ;
#22522=CARTESIAN_POINT ( 'NONE',  ( -19.05341960407617563, 5.049401038297882671, 23.54275706135233648 ) ) ;
#22523=CARTESIAN_POINT ( 'NONE',  ( -4.379528057220086978, -16.55341960407618274, 19.79275706135235069 ) ) ;
#22524=CARTESIAN_POINT ( 'NONE',  ( 19.05341960407617918, -5.049401038297876454, 71.04275706135234714 ) ) ;
#22525=CARTESIAN_POINT ( 'NONE',  ( -0.05219959533910754901, -16.53943276465976808, 72.49890960531435269 ) ) ;
#22526=CARTESIAN_POINT ( 'NONE',  ( 13.89961937509977652, -13.97604488694527269, 38.12390960531436690 ) ) ;
#22527=CARTESIAN_POINT ( 'NONE',  ( -13.97604488694547697, 13.89961937509957934, 78.12609039468567573 ) ) ;
#22528=CARTESIAN_POINT ( 'NONE',  ( 16.36317988757060604, -7.306389748694920527, 91.59789608363225000 ) ) ;
#22529=CARTESIAN_POINT ( 'NONE',  ( 21.55341960407619695, -5.719274019375665929, 81.04275706135236135 ) ) ;
#22530=CARTESIAN_POINT ( 'NONE',  ( -16.52544592524335698, -4.483927247898792601, 38.95942372801901854 ) ) ;
#22531=CARTESIAN_POINT ( 'NONE',  ( 19.26498983726237668, -5.499999999999590550, 58.05319577422003618 ) ) ;
#22532=CARTESIAN_POINT ( 'NONE',  ( 10.72451020669898902, -18.67979575497178502, 32.91557627198102409 ) ) ;
#22533=CARTESIAN_POINT ( 'NONE',  ( -14.34966873604972548, 8.224510206698743886, 23.33442372801901499 ) ) ;
#22534=CARTESIAN_POINT ( 'NONE',  ( -16.46253265017160317, 9.564922557960807481, 115.8322429386477097 ) ) ;
#22536=CARTESIAN_POINT ( 'NONE',  ( -19.02544592524342804, 5.153800228976336051, 36.04057627198100988 ) ) ;
#22538=CARTESIAN_POINT ( 'NONE',  ( 16.51473224551069308, 9.474510206698969483, 59.16557627198102409 ) ) ;
#22539=CARTESIAN_POINT ( 'NONE',  ( -15.80617190586768217, 15.72974639402176855, 63.12609039468568994 ) ) ;
#22540=CARTESIAN_POINT ( 'NONE',  ( 10.72451020669871369, 18.67979575497193778, 107.0844237280190043 ) ) ;
#22541=CARTESIAN_POINT ( 'NONE',  ( 4.379528057220339221, -16.55341960407611168, 22.70724293864769194 ) ) ;
#22542=CARTESIAN_POINT ( 'NONE',  ( -19.02544592524342804, 5.153800228976336051, 31.04057627198102409 ) ) ;
#22543=CARTESIAN_POINT ( 'NONE',  ( -16.46253265017160317, 9.564922557960807481, 95.83224293864769550 ) ) ;
#22544=CARTESIAN_POINT ( 'NONE',  ( 18.62759615963255655, 10.81492255796105972, 61.66775706135235424 ) ) ;
#22545=CARTESIAN_POINT ( 'NONE',  ( 5.049401038298161559, -19.05341960407611168, 32.70724293864768129 ) ) ;
#22547=CARTESIAN_POINT ( 'NONE',  ( 15.80617190586769283, -15.72974639402175789, 65.62609039468568994 ) ) ;
#22548=CARTESIAN_POINT ( 'NONE',  ( -9.474510206698720793, -16.51473224551083518, 99.58442372801900433 ) ) ;
#22549=CARTESIAN_POINT ( 'NONE',  ( -16.51473224551069308, -9.474510206698971260, 111.6655762719810383 ) ) ;
#22550=CARTESIAN_POINT ( 'NONE',  ( 4.379528057220339221, -16.55341960407611168, 112.7072429386476955 ) ) ;
#22551=CARTESIAN_POINT ( 'NONE',  ( -21.55341960407610458, -5.719274019375992779, 111.4572429386476813 ) ) ;
#22552=CARTESIAN_POINT ( 'NONE',  ( -0.05219959533936034679, 19.03943276465977164, 32.50109039468566863 ) ) ;
#22553=CARTESIAN_POINT ( 'NONE',  ( -16.55341960407611168, -4.379528057220339221, 106.4572429386477097 ) ) ;
#22554=CARTESIAN_POINT ( 'NONE',  ( 9.474510206698971260, -16.51473224551069308, 62.91557627198102409 ) ) ;
#22555=CARTESIAN_POINT ( 'NONE',  ( 9.474510206698729675, 16.51473224551082808, 97.08442372801900433 ) ) ;
#22556=CARTESIAN_POINT ( 'NONE',  ( 16.53943276465976808, -0.05219959533910856209, 63.74890960531435979 ) ) ;
#22557=CARTESIAN_POINT ( 'NONE',  ( 19.02544592524334988, 5.153800228976608722, 21.45942372801899012 ) ) ;
#22558=CARTESIAN_POINT ( 'NONE',  ( 5.153800228976335163, 19.02544592524342804, 114.7905762719810241 ) ) ;
#22559=CARTESIAN_POINT ( 'NONE',  ( 9.474510206698729675, 16.51473224551082808, 87.08442372801900433 ) ) ;
#22560=CARTESIAN_POINT ( 'NONE',  ( -5.719274019375978568, 21.55341960407610458, 85.20724293864770971 ) ) ;
#22561=CARTESIAN_POINT ( 'NONE',  ( 5.719274019375673035, 21.55341960407619339, 47.29275706135234003 ) ) ;
#22562=CARTESIAN_POINT ( 'NONE',  ( -12.06949235617739369, -12.14591786802326823, 39.37609039468567573 ) ) ;
#22563=CARTESIAN_POINT ( 'NONE',  ( -12.06949235617739369, -12.14591786802326823, 104.3760903946856899 ) ) ;
#22564=CARTESIAN_POINT ( 'NONE',  ( 16.55341960407618274, -4.379528057220086978, 36.04275706135234714 ) ) ;
#22565=CARTESIAN_POINT ( 'NONE',  ( -21.53943276465977519, -0.05219959533937600094, 43.75109039468568284 ) ) ;
#22566=CARTESIAN_POINT ( 'NONE',  ( -0.05219959533907301413, -21.53943276465977519, 52.49890960531435979 ) ) ;
#22567=CARTESIAN_POINT ( 'NONE',  ( 16.46253265017160672, -9.564922557960803928, 38.33224293864768839 ) ) ;
#22569=CARTESIAN_POINT ( 'NONE',  ( -8.314922557961024197, 14.29746914071037800, 77.91775706135231871 ) ) ;
#22570=CARTESIAN_POINT ( 'NONE',  ( 0.05219959533907565091, 21.53943276465977519, 94.99890960531436690 ) ) ;
#22571=CARTESIAN_POINT ( 'NONE',  ( 16.53943276465976808, -0.05219959533910856209, 33.74890960531436690 ) ) ;
#22572=CARTESIAN_POINT ( 'NONE',  ( -12.14591786802326823, 12.06949235617739902, 58.12609039468568994 ) ) ;
#22573=CARTESIAN_POINT ( 'NONE',  ( 13.97604488694548053, -13.89961937509957401, 105.6260903946856757 ) ) ;
#22574=CARTESIAN_POINT ( 'NONE',  ( 18.62759615963271287, -10.81492255796078972, 103.3322429386476955 ) ) ;
#22575=CARTESIAN_POINT ( 'NONE',  ( -4.379528057220328563, 16.55341960407611168, 25.20724293864769550 ) ) ;
#22576=VERTEX_POINT ( 'NONE', #138315 ) ;
#22577=CARTESIAN_POINT ( 'NONE',  ( 8.224510206698742110, 14.34966873604972548, 77.08442372801901854 ) ) ;
#22579=CARTESIAN_POINT ( 'NONE',  ( -10.72451020669898014, 18.67979575497178502, 80.41557627198103830 ) ) ;
#22580=CARTESIAN_POINT ( 'NONE',  ( 8.314922557961029526, -14.29746914071037800, 105.4177570613523613 ) ) ;
#22582=CARTESIAN_POINT ( 'NONE',  ( 19.25918095147778786, 5.499999999999572786, 86.95284276293935477 ) ) ;
#22583=CARTESIAN_POINT ( 'NONE',  ( 21.52544592524344225, -5.823673210054117533, 88.54057627198103830 ) ) ;
#22584=CARTESIAN_POINT ( 'NONE',  ( 15.80617190586746368, 15.72974639402197994, 104.3739096053143669 ) ) ;
#22585=CARTESIAN_POINT ( 'NONE',  ( 8.314922557960818139, 14.29746914071049879, 39.58224293864769550 ) ) ;
#22586=CARTESIAN_POINT ( 'NONE',  ( 8.314922557961029526, -14.29746914071037800, 30.41775706135234358 ) ) ;
#22587=CARTESIAN_POINT ( 'NONE',  ( -0.05219959533909027116, -19.03943276465977164, 52.49890960531436690 ) ) ;
#22588=CARTESIAN_POINT ( 'NONE',  ( 16.46253265017160672, -9.564922557960803928, 73.33224293864769550 ) ) ;
#22589=ORIENTED_EDGE ( 'NONE', *, *, #123102, .F. ) ;
#22590=CARTESIAN_POINT ( 'NONE',  ( 19.03943276465977164, -0.05219959533909143690, 113.7489096053143669 ) ) ;
#22591=CARTESIAN_POINT ( 'NONE',  ( -19.02544592524342804, 5.153800228976336051, 116.0405762719810383 ) ) ;
#22592=CARTESIAN_POINT ( 'NONE',  ( -5.049401038297874678, -19.05341960407617918, 99.79275706135234714 ) ) ;
#22593=CARTESIAN_POINT ( 'NONE',  ( 16.46253265017146816, 9.564922557961045513, 46.66775706135233293 ) ) ;
#22594=CARTESIAN_POINT ( 'NONE',  ( -0.05219959533907301413, -21.53943276465977519, 92.49890960531436690 ) ) ;
#22595=CARTESIAN_POINT ( 'NONE',  ( -16.55341960407611168, -4.379528057220339221, 26.45724293864768839 ) ) ;
#22596=B_SPLINE_CURVE_WITH_KNOTS ( 'NONE', 3,
 ( #129312, #173864, #98976, #6969, #4974, #96985, #114144, #159658, #24171, #161666, #176856, #23162, #112176, #22158, #175845, #160666, #20157, #67655, #177853, #65664, #145489, #99981 ),
 .UNSPECIFIED., .F., .F.,
 ( 4, 2, 2, 2, 2, 2, 2, 2, 2, 2, 4 ),
 ( 2.776912483567713316E-17, 0.001309639967555188992, 0.001964459951332769502, 0.002291869943221559649, 0.002455574939165955373, 0.002619279935110351096, 0.002782984931054747254, 0.002946689926999142544, 0.003274099918887933124, 0.003928919902665513851, 0.005238559870220677039 ),
 .UNSPECIFIED. ) ;
#22597=CARTESIAN_POINT ( 'NONE',  ( 18.67979575497178502, 10.72451020669898547, 49.16557627198102409 ) ) ;
#22598=CARTESIAN_POINT ( 'NONE',  ( -15.80617190586745835, -15.72974639402198527, 86.87390960531438111 ) ) ;
#22599=CARTESIAN_POINT ( 'NONE',  ( -13.89961937509957401, -13.97604488694547875, 104.3760903946856757 ) ) ;
#22600=CARTESIAN_POINT ( 'NONE',  ( 19.05341960407611168, 5.049401038298154454, 98.95724293864766707 ) ) ;
#22601=CARTESIAN_POINT ( 'NONE',  ( 21.53943276465977519, 0.05219959533937863772, 71.25109039468568994 ) ) ;
#22602=CARTESIAN_POINT ( 'NONE',  ( 0.05219959533909260263, 19.03943276465977164, 69.99890960531435269 ) ) ;
#22605=CARTESIAN_POINT ( 'NONE',  ( -13.97604488694527625, -13.89961937509977652, 66.87390960531436690 ) ) ;
#22606=CARTESIAN_POINT ( 'NONE',  ( 0.05219959533910956823, 16.53943276465976808, 94.99890960531436690 ) ) ;
#22608=CARTESIAN_POINT ( 'NONE',  ( 0.05219959533936267826, -19.03943276465977164, 110.0010903946856757 ) ) ;
#22609=CARTESIAN_POINT ( 'NONE',  ( 16.81555441253553340, -7.025013491695478507, 83.13685445334260748 ) ) ;
#22610=CARTESIAN_POINT ( 'NONE',  ( -16.46253265017160317, 9.564922557960807481, 70.83224293864770971 ) ) ;
#22611=CARTESIAN_POINT ( 'NONE',  ( -21.52544592524334988, -5.823673210054445271, 88.95942372801901854 ) ) ;
#22612=CARTESIAN_POINT ( 'NONE',  ( 19.05341960407611168, 5.049401038298154454, 93.95724293864769550 ) ) ;
#22614=CARTESIAN_POINT ( 'NONE',  ( 8.314922557961029526, -14.29746914071037800, 75.41775706135233293 ) ) ;
#22616=CARTESIAN_POINT ( 'NONE',  ( -9.564922557961040184, 16.46253265017147172, 57.91775706135233293 ) ) ;
#22617=CARTESIAN_POINT ( 'NONE',  ( -21.53943276465977519, -0.05219959533937600094, 108.7510903946857042 ) ) ;
#22620=CARTESIAN_POINT ( 'NONE',  ( 14.34966873604972726, -8.224510206698740333, 110.8344237280190043 ) ) ;
#22622=CARTESIAN_POINT ( 'NONE',  ( -4.483927247898782831, 16.52544592524335698, 92.70942372801901854 ) ) ;
#22624=CARTESIAN_POINT ( 'NONE',  ( -16.53943276465976808, -0.05219959533934237506, 73.75109039468567573 ) ) ;
#22625=CARTESIAN_POINT ( 'NONE',  ( 5.823673210054444382, -21.52544592524334988, 75.20942372801901854 ) ) ;
#22626=CARTESIAN_POINT ( 'NONE',  ( -16.46253265017146816, -9.564922557961047289, 94.16775706135233293 ) ) ;
#22627=CARTESIAN_POINT ( 'NONE',  ( -16.51473224551082808, 9.474510206698731452, 38.33442372801899722 ) ) ;
#22628=CARTESIAN_POINT ( 'NONE',  ( -19.05341960407611168, -5.049401038298163336, 76.45724293864769550 ) ) ;
#22629=CARTESIAN_POINT ( 'NONE',  ( 16.46253265017160672, -9.564922557960803928, 63.33224293864769550 ) ) ;
#22630=CARTESIAN_POINT ( 'NONE',  ( 17.72696623605161292, -5.499999999999851674, 41.09811031808418136 ) ) ;
#22631=CARTESIAN_POINT ( 'NONE',  ( -5.823673210054116645, -21.52544592524344225, 82.29057627198103830 ) ) ;
#22633=CARTESIAN_POINT ( 'NONE',  ( 21.55341960407610458, 5.719274019375980345, 43.95724293864769550 ) ) ;
#22634=CARTESIAN_POINT ( 'NONE',  ( 16.51473224551069308, 9.474510206698969483, 34.16557627198102409 ) ) ;
#22635=CARTESIAN_POINT ( 'NONE',  ( -12.14591786802326823, 12.06949235617739902, 68.12609039468567573 ) ) ;
#22638=CARTESIAN_POINT ( 'NONE',  ( -5.719274019375665041, -21.55341960407619695, 49.79275706135234714 ) ) ;
#22639=CARTESIAN_POINT ( 'NONE',  ( -14.34966873604960291, -8.224510206698953496, 61.66557627198103120 ) ) ;
#22641=CARTESIAN_POINT ( 'NONE',  ( -12.06949235617739369, -12.14591786802326823, 39.37609039468567573 ) ) ;
#22642=CARTESIAN_POINT ( 'NONE',  ( -8.224510206698948167, 14.34966873604960824, 105.4155762719810383 ) ) ;
#22643=CARTESIAN_POINT ( 'NONE',  ( -13.97604488694547697, 13.89961937509957934, 58.12609039468566863 ) ) ;
#22644=CARTESIAN_POINT ( 'NONE',  ( -16.55341960407611168, -4.379528057220339221, 56.45724293864768839 ) ) ;
#22645=CARTESIAN_POINT ( 'NONE',  ( -10.81492255796105439, 18.62759615963255655, 27.91775706135234358 ) ) ;
#22646=CARTESIAN_POINT ( 'NONE',  ( -13.97604488694527625, -13.89961937509977652, 26.87390960531434558 ) ) ;
#22647=CARTESIAN_POINT ( 'NONE',  ( -18.67979575497178146, -10.72451020669898902, 91.66557627198103830 ) ) ;
#22648=CARTESIAN_POINT ( 'NONE',  ( 16.46253265017160672, -9.564922557960803928, 98.33224293864769550 ) ) ;
#22649=CARTESIAN_POINT ( 'NONE',  ( 14.34966873604960469, 8.224510206698951720, 74.16557627198102409 ) ) ;
#22650=CARTESIAN_POINT ( 'NONE',  ( -16.51473224551069308, -9.474510206698971260, 111.6655762719810383 ) ) ;
#22652=CARTESIAN_POINT ( 'NONE',  ( -9.564922557961040184, 16.46253265017147172, 82.91775706135233293 ) ) ;
#22653=CARTESIAN_POINT ( 'NONE',  ( -5.719274019375665041, -21.55341960407619695, 19.79275706135235069 ) ) ;
#22654=CARTESIAN_POINT ( 'NONE',  ( 19.05341960407611168, 5.049401038298154454, 63.95724293864769550 ) ) ;
#22655=CARTESIAN_POINT ( 'NONE',  ( 13.89961937509957401, 13.97604488694547697, 51.87609039468566863 ) ) ;
#22656=CARTESIAN_POINT ( 'NONE',  ( -5.049401038298153566, 19.05341960407611168, 30.20724293864768839 ) ) ;
#22657=CARTESIAN_POINT ( 'NONE',  ( -18.67979575497193778, 10.72451020669871902, 63.33442372801900433 ) ) ;
#22659=CARTESIAN_POINT ( 'NONE',  ( 8.224510206698953496, -14.34966873604960469, 52.91557627198103830 ) ) ;
#22660=CARTESIAN_POINT ( 'NONE',  ( -9.474510206698964154, 16.51473224551069663, 60.41557627198102409 ) ) ;
#22661=CARTESIAN_POINT ( 'NONE',  ( 18.62759615963271287, -10.81492255796078972, 88.33224293864769550 ) ) ;
#22662=CARTESIAN_POINT ( 'NONE',  ( 0.05219959533909260263, 19.03943276465977164, 54.99890960531435979 ) ) ;
#22664=CARTESIAN_POINT ( 'NONE',  ( 15.80617190586746368, 15.72974639402197994, 79.37390960531436690 ) ) ;
#22665=CARTESIAN_POINT ( 'NONE',  ( -18.62759615963255300, -10.81492255796106328, 94.16775706135237556 ) ) ;
#22666=CARTESIAN_POINT ( 'NONE',  ( 19.02544592524343514, -5.153800228976328945, 23.54057627198102054 ) ) ;
#22667=CARTESIAN_POINT ( 'NONE',  ( -12.14591786802326823, 12.06949235617739902, 93.12609039468568994 ) ) ;
#22668=CARTESIAN_POINT ( 'NONE',  ( -16.55341960407611168, -4.379528057220339221, 96.45724293864770971 ) ) ;
#22669=CARTESIAN_POINT ( 'NONE',  ( -16.51473224551082808, 9.474510206698731452, 88.33442372801900433 ) ) ;
#22671=CARTESIAN_POINT ( 'NONE',  ( -18.62759615963255300, -10.81492255796106328, 19.16775706135234714 ) ) ;
#22672=CARTESIAN_POINT ( 'NONE',  ( 0.05219959533936267826, -19.03943276465977164, 35.00109039468566863 ) ) ;
#22673=CARTESIAN_POINT ( 'NONE',  ( 16.52544592524335698, 4.483927247898782831, 106.4594237280190328 ) ) ;
#22674=CARTESIAN_POINT ( 'NONE',  ( 5.153800228976615827, -19.02544592524334988, 25.20942372801900433 ) ) ;
#22675=CARTESIAN_POINT ( 'NONE',  ( -16.46253265017160317, 9.564922557960807481, 100.8322429386477097 ) ) ;
#22676=CARTESIAN_POINT ( 'NONE',  ( 18.67979575497178502, 10.72451020669898547, 59.16557627198103120 ) ) ;
#22677=CARTESIAN_POINT ( 'NONE',  ( -16.51473224551069308, -9.474510206698971260, 21.66557627198102765 ) ) ;
#22678=CARTESIAN_POINT ( 'NONE',  ( 16.51473224551069308, 9.474510206698969483, 24.16557627198102765 ) ) ;
#22679=CARTESIAN_POINT ( 'NONE',  ( 10.72451020669871369, 18.67979575497193778, 107.0844237280190043 ) ) ;
#22680=CARTESIAN_POINT ( 'NONE',  ( -4.483927247898782831, 16.52544592524335698, 77.70942372801900433 ) ) ;
#22681=CARTESIAN_POINT ( 'NONE',  ( 21.53943276465977519, 0.05219959533937863772, 31.25109039468568639 ) ) ;
#22682=CARTESIAN_POINT ( 'NONE',  ( -16.53943276465976808, -0.05219959533934237506, 38.75109039468567573 ) ) ;
#22683=CARTESIAN_POINT ( 'NONE',  ( -19.05341960407611168, -5.049401038298163336, 101.4572429386476955 ) ) ;
#22684=CARTESIAN_POINT ( 'NONE',  ( -19.02544592524342804, 5.153800228976336051, 41.04057627198103120 ) ) ;
#22685=CARTESIAN_POINT ( 'NONE',  ( -19.02544592524342804, 5.153800228976336051, 71.04057627198099567 ) ) ;
#22686=CARTESIAN_POINT ( 'NONE',  ( 0.05219959533934541429, -16.53943276465976808, 50.00109039468568994 ) ) ;
#22687=CARTESIAN_POINT ( 'NONE',  ( 16.53943276465976808, -0.05219959533910856209, 88.74890960531436690 ) ) ;
#22688=CARTESIAN_POINT ( 'NONE',  ( -16.52544592524335698, -4.483927247898792601, 98.95942372801903275 ) ) ;
#22689=CARTESIAN_POINT ( 'NONE',  ( 9.564922557960805705, 16.46253265017160317, 49.58224293864770260 ) ) ;
#22690=CARTESIAN_POINT ( 'NONE',  ( -18.67979575497193778, 10.72451020669871902, 63.33442372801900433 ) ) ;
#22691=CARTESIAN_POINT ( 'NONE',  ( 9.564922557960805705, 16.46253265017160317, 74.58224293864769550 ) ) ;
#22692=CARTESIAN_POINT ( 'NONE',  ( 19.03943276465977164, -0.05219959533909143690, 63.74890960531435979 ) ) ;
#22693=CARTESIAN_POINT ( 'NONE',  ( -19.03943276465977164, 0.05219959533909376836, 101.2489096053143669 ) ) ;
#22694=CARTESIAN_POINT ( 'NONE',  ( -8.314922557960811034, -14.29746914071050412, 47.08224293864770260 ) ) ;
#22695=CARTESIAN_POINT ( 'NONE',  ( 4.379528057220092307, 16.55341960407617563, 102.2927570613523613 ) ) ;
#22696=CARTESIAN_POINT ( 'NONE',  ( 12.14591786802309770, 12.06949235617756955, 29.37390960531435269 ) ) ;
#22698=CARTESIAN_POINT ( 'NONE',  ( 5.049401038297881783, 19.05341960407617563, 42.29275706135234003 ) ) ;
#22699=CARTESIAN_POINT ( 'NONE',  ( -13.89961937509977652, 13.97604488694528158, 110.6239096053143243 ) ) ;
#22700=CARTESIAN_POINT ( 'NONE',  ( 13.97604488694527802, 13.89961937509977652, 64.37390960531436690 ) ) ;
#22701=CARTESIAN_POINT ( 'NONE',  ( 13.89961937509957401, 13.97604488694547697, 36.87609039468565442 ) ) ;
#22703=CARTESIAN_POINT ( 'NONE',  ( 17.49999999999999645, 3.242565516156353134, 37.49999999998637179 ) ) ;
#22704=CARTESIAN_POINT ( 'NONE',  ( 5.049401038297881783, 19.05341960407617563, 87.29275706135234714 ) ) ;
#22705=CARTESIAN_POINT ( 'NONE',  ( 16.53943276465976808, 0.05219959533934440121, 66.25109039468567573 ) ) ;
#22706=CARTESIAN_POINT ( 'NONE',  ( 17.26058549869090797, 6.457015423128543929, 93.87745837476069255 ) ) ;
#22707=CARTESIAN_POINT ( 'NONE',  ( -13.97604488694527625, -13.89961937509977652, 86.87390960531436690 ) ) ;
#22708=CARTESIAN_POINT ( 'NONE',  ( -0.05219959533937732626, 21.53943276465977519, 32.50109039468568284 ) ) ;
#22709=CARTESIAN_POINT ( 'NONE',  ( 9.564922557961047289, -16.46253265017146816, 70.41775706135233293 ) ) ;
#22710=CARTESIAN_POINT ( 'NONE',  ( -16.46253265017160317, 9.564922557960807481, 115.8322429386477097 ) ) ;
#22711=CARTESIAN_POINT ( 'NONE',  ( -13.97604488694527625, -13.89961937509977652, 31.87390960531435979 ) ) ;
#22712=CARTESIAN_POINT ( 'NONE',  ( -0.05219959533909027116, -19.03943276465977164, 87.49890960531436690 ) ) ;
#22713=CARTESIAN_POINT ( 'NONE',  ( -16.53943276465976808, 0.05219959533911058130, 46.24890960531435979 ) ) ;
#22714=CARTESIAN_POINT ( 'NONE',  ( -13.97604488694527625, -13.89961937509977652, 41.87390960531435979 ) ) ;
#22715=CARTESIAN_POINT ( 'NONE',  ( -19.03943276465977164, -0.05219959533935918106, 48.75109039468566863 ) ) ;
#22716=CARTESIAN_POINT ( 'NONE',  ( 16.53943276465976808, -0.05219959533910856209, 88.74890960531436690 ) ) ;
#22717=CARTESIAN_POINT ( 'NONE',  ( -0.05219959533936034679, 19.03943276465977164, 32.50109039468566863 ) ) ;
#22718=CARTESIAN_POINT ( 'NONE',  ( 19.05341960407611168, 5.049401038298154454, 58.95724293864768129 ) ) ;
#22719=CARTESIAN_POINT ( 'NONE',  ( -18.62759615963270932, 10.81492255796079327, 60.83224293864769550 ) ) ;
#22720=CARTESIAN_POINT ( 'NONE',  ( 14.34966873604960469, 8.224510206698951720, 59.16557627198103120 ) ) ;
#22721=CARTESIAN_POINT ( 'NONE',  ( -0.05219959533936034679, 19.03943276465977164, 27.50109039468566507 ) ) ;
#22722=CARTESIAN_POINT ( 'NONE',  ( 19.05341960407611168, 5.049401038298154454, 108.9572429386477097 ) ) ;
#22723=CARTESIAN_POINT ( 'NONE',  ( -10.81492255796078084, -18.62759615963271287, 22.08224293864769194 ) ) ;
#22724=CARTESIAN_POINT ( 'NONE',  ( 16.51473224551069308, 9.474510206698969483, 54.16557627198103120 ) ) ;
#22725=CARTESIAN_POINT ( 'NONE',  ( -9.474510206698964154, 16.51473224551069663, 25.41557627198103120 ) ) ;
#22726=CARTESIAN_POINT ( 'NONE',  ( -12.14591786802309592, -12.06949235617757132, 91.87390960531436690 ) ) ;
#22727=CARTESIAN_POINT ( 'NONE',  ( -18.62759615963270932, 10.81492255796079327, 100.8322429386477097 ) ) ;
#22728=CARTESIAN_POINT ( 'NONE',  ( 16.51473224551069308, 9.474510206698969483, 99.16557627198102409 ) ) ;
#22729=CARTESIAN_POINT ( 'NONE',  ( -15.72974639402197994, 15.80617190586746368, 105.6239096053143669 ) ) ;
#22730=CARTESIAN_POINT ( 'NONE',  ( -19.05341960407611168, -5.049401038298163336, 106.4572429386476955 ) ) ;
#22731=CARTESIAN_POINT ( 'NONE',  ( -9.564922557960796823, -16.46253265017161027, 27.08224293864769550 ) ) ;
#22732=CARTESIAN_POINT ( 'NONE',  ( 0.05219959533937995610, -21.53943276465977519, 75.00109039468568994 ) ) ;
#22733=CARTESIAN_POINT ( 'NONE',  ( -21.53943276465977519, 0.05219959533907696930, 96.24890960531435269 ) ) ;
#22734=CARTESIAN_POINT ( 'NONE',  ( 16.20579543436677739, -7.371946100355110332, 106.9347916582812559 ) ) ;
#22735=CARTESIAN_POINT ( 'NONE',  ( 19.36337904590693881, -5.499999999999943157, 77.91494137495617167 ) ) ;
#22737=CARTESIAN_POINT ( 'NONE',  ( 12.14591786802327356, -12.06949235617739191, 35.62609039468568994 ) ) ;
#22738=CARTESIAN_POINT ( 'NONE',  ( -8.314922557960811034, -14.29746914071050412, 107.0822429386476955 ) ) ;
#22739=CARTESIAN_POINT ( 'NONE',  ( -17.50000000000000355, -3.345213924137315331, 110.4123137690565102 ) ) ;
#22740=CARTESIAN_POINT ( 'NONE',  ( -13.89961937509977652, 13.97604488694528158, 55.62390960531434558 ) ) ;
#22741=CARTESIAN_POINT ( 'NONE',  ( 12.14591786802309770, 12.06949235617756955, 94.37390960531436690 ) ) ;
#22742=CARTESIAN_POINT ( 'NONE',  ( 10.72451020669898902, -18.67979575497178502, 37.91557627198102409 ) ) ;
#22743=CARTESIAN_POINT ( 'NONE',  ( -16.55341960407611168, -4.379528057220339221, 61.45724293864770260 ) ) ;
#22744=CARTESIAN_POINT ( 'NONE',  ( 0.05219959533934541429, -16.53943276465976808, 25.00109039468567218 ) ) ;
#22745=CARTESIAN_POINT ( 'NONE',  ( -5.719274019375665041, -21.55341960407619695, 69.79275706135234714 ) ) ;
#22746=CARTESIAN_POINT ( 'NONE',  ( 17.40805194822031154, -6.112264579159332634, 78.33371272510611050 ) ) ;
#22747=CARTESIAN_POINT ( 'NONE',  ( -19.03943276465977164, 0.05219959533909376836, 116.2489096053143669 ) ) ;
#22748=CARTESIAN_POINT ( 'NONE',  ( 12.06949235617739724, 12.14591786802326823, 96.87609039468568994 ) ) ;
#22749=CARTESIAN_POINT ( 'NONE',  ( -5.049401038298153566, 19.05341960407611168, 45.20724293864769550 ) ) ;
#22750=CARTESIAN_POINT ( 'NONE',  ( -9.474510206698964154, 16.51473224551069663, 95.41557627198102409 ) ) ;
#22751=CARTESIAN_POINT ( 'NONE',  ( -21.52544592524343514, 5.823673210054127303, 96.04057627198102409 ) ) ;
#22752=CARTESIAN_POINT ( 'NONE',  ( -14.29746914071037622, -8.314922557961029526, 24.16775706135235424 ) ) ;
#22753=CARTESIAN_POINT ( 'NONE',  ( 4.379528057220339221, -16.55341960407611168, 67.70724293864769550 ) ) ;
#22754=CARTESIAN_POINT ( 'NONE',  ( 21.55341960407619695, -5.719274019375665929, 71.04275706135234714 ) ) ;
#22755=CARTESIAN_POINT ( 'NONE',  ( 8.314922557961029526, -14.29746914071037800, 105.4177570613523613 ) ) ;
#22756=CARTESIAN_POINT ( 'NONE',  ( 17.48847506799950224, -5.747544572775292515, 48.32697437843292931 ) ) ;
#22758=CARTESIAN_POINT ( 'NONE',  ( -16.55341960407611168, -4.379528057220339221, 26.45724293864768839 ) ) ;
#22759=CARTESIAN_POINT ( 'NONE',  ( 12.06949235617739724, 12.14591786802326823, 71.87609039468568994 ) ) ;
#22760=CARTESIAN_POINT ( 'NONE',  ( 5.153800228976335163, 19.02544592524342804, 79.79057627198102409 ) ) ;
#22761=CARTESIAN_POINT ( 'NONE',  ( 19.03943276465977164, -0.05219959533909143690, 88.74890960531436690 ) ) ;
#22762=CARTESIAN_POINT ( 'NONE',  ( 21.52544592524334988, 5.823673210054432836, 86.45942372801901854 ) ) ;
#22763=CARTESIAN_POINT ( 'NONE',  ( -12.06949235617739369, -12.14591786802326823, 84.37609039468570415 ) ) ;
#22764=CARTESIAN_POINT ( 'NONE',  ( 4.379528057220339221, -16.55341960407611168, 62.70724293864769550 ) ) ;
#22765=CARTESIAN_POINT ( 'NONE',  ( 5.049401038298161559, -19.05341960407611168, 62.70724293864769550 ) ) ;
#22766=VERTEX_POINT ( 'NONE', #150525 ) ;
#22767=( BOUNDED_CURVE ( )  B_SPLINE_CURVE ( 2, ( #29210, #46347, #169690, #150566, #183877, #90844, #152529, #108004, #199040, #196087, #60510, #57557, #119227 ),
 .UNSPECIFIED., .F., .T. ) 
 B_SPLINE_CURVE_WITH_KNOTS ( ( 3, 2, 2, 2, 2, 2, 3 ),
 ( 0.3971672785323083210, 0.3991228070175438791, 0.4035087719298245390, 0.4078947368421052544, 0.4122807017543859698, 0.4166666666666666852, 0.4185765153298121599 ),
 .UNSPECIFIED. ) 
 CURVE ( )  GEOMETRIC_REPRESENTATION_ITEM ( )  RATIONAL_B_SPLINE_CURVE ( ( 0.9831626618144004848, 0.9848076720550091867, 1.000000000000000000, 0.9659258262890683122, 1.000000000000000000, 0.9659258262890683122, 1.000000000000000000, 0.9659258262890683122, 1.000000000000000000, 0.9659258262890683122, 1.000000000000000000, 0.9851625545550088958, 0.9832469066685279868 ) ) 
 REPRESENTATION_ITEM ( '' )  );
#22768=CARTESIAN_POINT ( 'NONE',  ( -19.02544592524334988, -5.153800228976617603, 103.9594237280190043 ) ) ;
#22769=CARTESIAN_POINT ( 'NONE',  ( 8.314922557960818139, 14.29746914071049879, 114.5822429386477097 ) ) ;
#22770=CARTESIAN_POINT ( 'NONE',  ( -13.89961937509977652, 13.97604488694528158, 80.62390960531436690 ) ) ;
#22771=CARTESIAN_POINT ( 'NONE',  ( -19.05341960407617563, 5.049401038297882671, 108.5427570613523187 ) ) ;
#22773=CARTESIAN_POINT ( 'NONE',  ( -5.049401038297874678, -19.05341960407617918, 24.79275706135233648 ) ) ;
#22774=CARTESIAN_POINT ( 'NONE',  ( 8.314922557961029526, -14.29746914071037800, 85.41775706135236135 ) ) ;
#22775=CARTESIAN_POINT ( 'NONE',  ( 5.153800228976615827, -19.02544592524334988, 90.20942372801900433 ) ) ;
#22776=CARTESIAN_POINT ( 'NONE',  ( -16.52544592524342804, 4.483927247898546575, 111.0405762719810525 ) ) ;
#22777=CARTESIAN_POINT ( 'NONE',  ( -16.53943276465976808, -0.05219959533934237506, 68.75109039468568994 ) ) ;
#22779=CARTESIAN_POINT ( 'NONE',  ( 13.89961937509957401, 13.97604488694547697, 61.87609039468566863 ) ) ;
#22780=CARTESIAN_POINT ( 'NONE',  ( 21.53943276465977519, 0.05219959533937863772, 101.2510903946856757 ) ) ;
#22781=CARTESIAN_POINT ( 'NONE',  ( 19.03943276465977164, -0.05219959533909143690, 38.74890960531436690 ) ) ;
#22782=CARTESIAN_POINT ( 'NONE',  ( -5.049401038298153566, 19.05341960407611168, 80.20724293864769550 ) ) ;
#22783=CARTESIAN_POINT ( 'NONE',  ( -8.224510206698948167, 14.34966873604960824, 75.41557627198102409 ) ) ;
#22785=CARTESIAN_POINT ( 'NONE',  ( 18.62759615963255655, 10.81492255796105972, 91.66775706135234714 ) ) ;
#22786=CARTESIAN_POINT ( 'NONE',  ( 13.89961937509957401, 13.97604488694547697, 61.87609039468566863 ) ) ;
#22787=CARTESIAN_POINT ( 'NONE',  ( -5.049401038297874678, -19.05341960407617918, 44.79275706135232582 ) ) ;
#22788=CARTESIAN_POINT ( 'NONE',  ( 18.62759615963271287, -10.81492255796078972, 33.33224293864769550 ) ) ;
#22789=CARTESIAN_POINT ( 'NONE',  ( 21.55341960407619695, -5.719274019375665929, 101.0427570613523756 ) ) ;
#22790=CARTESIAN_POINT ( 'NONE',  ( 16.51473224551069308, 9.474510206698969483, 84.16557627198102409 ) ) ;
#22792=CARTESIAN_POINT ( 'NONE',  ( 18.67979575497194134, -10.72451020669871369, 100.8344237280190185 ) ) ;
#22793=CARTESIAN_POINT ( 'NONE',  ( -18.67979575497178146, -10.72451020669898902, 51.66557627198102409 ) ) ;
#22794=CARTESIAN_POINT ( 'NONE',  ( 16.51473224551069308, 9.474510206698969483, 94.16557627198103830 ) ) ;
#22795=CARTESIAN_POINT ( 'NONE',  ( -19.03943276465977164, -0.05219959533935918106, 73.75109039468566152 ) ) ;
#22796=CARTESIAN_POINT ( 'NONE',  ( -19.02544592524342804, 5.153800228976336051, 106.0405762719810241 ) ) ;
#22797=CARTESIAN_POINT ( 'NONE',  ( 13.89961937509957401, 13.97604488694547697, 96.87609039468566152 ) ) ;
#22798=CARTESIAN_POINT ( 'NONE',  ( -8.314922557961024197, 14.29746914071037800, 37.91775706135235424 ) ) ;
#22799=CARTESIAN_POINT ( 'NONE',  ( -16.55341960407611168, -4.379528057220339221, 101.4572429386476955 ) ) ;
#22800=CARTESIAN_POINT ( 'NONE',  ( -16.46253265017160317, 9.564922557960807481, 85.83224293864769550 ) ) ;
#22801=CARTESIAN_POINT ( 'NONE',  ( 18.67979575497178502, 10.72451020669898547, 59.16557627198103120 ) ) ;
#22802=CARTESIAN_POINT ( 'NONE',  ( -12.06949235617739369, -12.14591786802326823, 34.37609039468568284 ) ) ;
#22803=CARTESIAN_POINT ( 'NONE',  ( 18.62759615963255655, 10.81492255796105972, 31.66775706135234358 ) ) ;
#22804=CARTESIAN_POINT ( 'NONE',  ( 10.81492255796106328, -18.62759615963255655, 85.41775706135236135 ) ) ;
#22805=CARTESIAN_POINT ( 'NONE',  ( 16.52544592524335698, 4.483927247898782831, 76.45942372801901854 ) ) ;
#22806=CARTESIAN_POINT ( 'NONE',  ( -9.474510206698964154, 16.51473224551069663, 80.41557627198103830 ) ) ;
#22807=CARTESIAN_POINT ( 'NONE',  ( 14.34966873604960469, 8.224510206698951720, 84.16557627198103830 ) ) ;
#22808=CARTESIAN_POINT ( 'NONE',  ( 14.29746914071037800, 8.314922557961029526, 111.6677570613523613 ) ) ;
#22809=CARTESIAN_POINT ( 'NONE',  ( -5.153800228976607833, 19.02544592524334988, 52.70942372801900433 ) ) ;
#22810=CARTESIAN_POINT ( 'NONE',  ( -10.81492255796105439, 18.62759615963255655, 32.91775706135234714 ) ) ;
#22811=CARTESIAN_POINT ( 'NONE',  ( 4.483927247898545687, 16.52544592524342804, 74.79057627198105251 ) ) ;
#22812=CARTESIAN_POINT ( 'NONE',  ( 19.05341960407611168, 5.049401038298154454, 93.95724293864769550 ) ) ;
#22813=CARTESIAN_POINT ( 'NONE',  ( -12.14591786802326823, 12.06949235617739902, 108.1260903946856757 ) ) ;
#22814=CARTESIAN_POINT ( 'NONE',  ( -21.53943276465977519, -0.05219959533937600094, 68.75109039468568994 ) ) ;
#22815=CARTESIAN_POINT ( 'NONE',  ( 4.379528057220092307, 16.55341960407617563, 47.29275706135234003 ) ) ;
#22816=CARTESIAN_POINT ( 'NONE',  ( 21.55341960407619695, -5.719274019375665929, 41.04275706135236135 ) ) ;
#22817=ORIENTED_EDGE ( 'NONE', *, *, #167117, .F. ) ;
#22818=CARTESIAN_POINT ( 'NONE',  ( 10.81492255796078972, 18.62759615963270932, 109.5822429386476955 ) ) ;
#22819=CARTESIAN_POINT ( 'NONE',  ( -8.224510206698948167, 14.34966873604960824, 85.41557627198102409 ) ) ;
#22820=CARTESIAN_POINT ( 'NONE',  ( -19.19724070472091526, -5.500000000000167866, 51.06193348274386778 ) ) ;
#22821=CARTESIAN_POINT ( 'NONE',  ( -14.34966873604960291, -8.224510206698953496, 46.66557627198102409 ) ) ;
#22822=CARTESIAN_POINT ( 'NONE',  ( -0.05219959533909027116, -19.03943276465977164, 22.49890960531436690 ) ) ;
#22823=CARTESIAN_POINT ( 'NONE',  ( 18.62759615963271287, -10.81492255796078972, 48.33224293864770260 ) ) ;
#22824=CARTESIAN_POINT ( 'NONE',  ( -14.29746914071049879, 8.314922557960819915, 75.83224293864769550 ) ) ;
#22825=CARTESIAN_POINT ( 'NONE',  ( -21.52544592524343514, 5.823673210054127303, 86.04057627198102409 ) ) ;
#22826=CARTESIAN_POINT ( 'NONE',  ( -19.03943276465977164, 0.05219959533909376836, 86.24890960531436690 ) ) ;
#22827=CARTESIAN_POINT ( 'NONE',  ( -9.564922557960796823, -16.46253265017161027, 42.08224293864769550 ) ) ;
#22828=CARTESIAN_POINT ( 'NONE',  ( 19.02544592524334988, 5.153800228976608722, 76.45942372801897591 ) ) ;
#22829=CARTESIAN_POINT ( 'NONE',  ( -21.53943276465977519, 0.05219959533907696930, 26.24890960531435624 ) ) ;
#22830=CARTESIAN_POINT ( 'NONE',  ( -21.53943276465977519, -0.05219959533937600094, 58.75109039468568994 ) ) ;
#22831=CARTESIAN_POINT ( 'NONE',  ( 18.67979575497178502, 10.72451020669898547, 64.16557627198102409 ) ) ;
#22832=CARTESIAN_POINT ( 'NONE',  ( -16.46253265017160317, 9.564922557960807481, 35.83224293864768839 ) ) ;
#22833=CARTESIAN_POINT ( 'NONE',  ( 13.97604488694527802, 13.89961937509977652, 69.37390960531436690 ) ) ;
#22835=CARTESIAN_POINT ( 'NONE',  ( 8.224510206698742110, 14.34966873604972548, 52.08442372801901854 ) ) ;
#22836=CARTESIAN_POINT ( 'NONE',  ( -10.72451020669870658, -18.67979575497194134, 24.58442372801901499 ) ) ;
#22837=CARTESIAN_POINT ( 'NONE',  ( 10.81492255796106328, -18.62759615963255655, 70.41775706135236135 ) ) ;
#22838=CARTESIAN_POINT ( 'NONE',  ( -10.72451020669898014, 18.67979575497178502, 25.41557627198103120 ) ) ;
#22839=CARTESIAN_POINT ( 'NONE',  ( -10.81492255796078084, -18.62759615963271287, 82.08224293864768129 ) ) ;
#22840=CARTESIAN_POINT ( 'NONE',  ( -10.72451020669870658, -18.67979575497194134, 29.58442372801901854 ) ) ;
#22841=CARTESIAN_POINT ( 'NONE',  ( 16.55341960407618274, -4.379528057220086978, 51.04275706135234714 ) ) ;
#22842=CARTESIAN_POINT ( 'NONE',  ( -5.823673210054116645, -21.52544592524344225, 67.29057627198103830 ) ) ;
#22843=CARTESIAN_POINT ( 'NONE',  ( -9.564922557961040184, 16.46253265017147172, 22.91775706135233648 ) ) ;
#22844=CARTESIAN_POINT ( 'NONE',  ( 13.89961937509977652, -13.97604488694527269, 58.12390960531436690 ) ) ;
#22845=CARTESIAN_POINT ( 'NONE',  ( -13.97604488694527625, -13.89961937509977652, 111.8739096053143243 ) ) ;
#22846=CARTESIAN_POINT ( 'NONE',  ( -13.89961937509977652, 13.97604488694528158, 90.62390960531432427 ) ) ;
#22847=CARTESIAN_POINT ( 'NONE',  ( 17.50000000000001421, 5.047551163040773226, 103.6653608652058836 ) ) ;
#22848=CARTESIAN_POINT ( 'NONE',  ( -19.02544592524334988, -5.153800228976617603, 63.95942372801899012 ) ) ;
#22849=CARTESIAN_POINT ( 'NONE',  ( -15.80617190586745835, -15.72974639402198527, 46.87390960531435979 ) ) ;
#22850=CARTESIAN_POINT ( 'NONE',  ( 14.29746914071049879, -8.314922557960816363, 28.33224293864769550 ) ) ;
#22851=CARTESIAN_POINT ( 'NONE',  ( 9.474510206698729675, 16.51473224551082808, 102.0844237280190043 ) ) ;
#22852=CARTESIAN_POINT ( 'NONE',  ( 17.97182807773873492, -5.500000000000077272, 51.03038844047286204 ) ) ;
#22853=CARTESIAN_POINT ( 'NONE',  ( 19.03943276465977164, 0.05219959533936151252, 26.25109039468566507 ) ) ;
#22854=CARTESIAN_POINT ( 'NONE',  ( -9.474510206698720793, -16.51473224551083518, 94.58442372801900433 ) ) ;
#22855=CARTESIAN_POINT ( 'NONE',  ( -15.72974639402197994, 15.80617190586746368, 85.62390960531436690 ) ) ;
#22856=CARTESIAN_POINT ( 'NONE',  ( -16.46253265017146816, -9.564922557961047289, 59.16775706135233293 ) ) ;
#22858=CARTESIAN_POINT ( 'NONE',  ( 16.51473224551069308, 9.474510206698969483, 54.16557627198103120 ) ) ;
#22859=CARTESIAN_POINT ( 'NONE',  ( 16.52544592524342804, -4.483927247898539470, 63.54057627198103830 ) ) ;
#22860=CARTESIAN_POINT ( 'NONE',  ( 19.03943276465977164, -0.05219959533909143690, 53.74890960531436690 ) ) ;
#22861=CARTESIAN_POINT ( 'NONE',  ( 12.06949235617757843, -12.14591786802309237, 58.12390960531435979 ) ) ;
#22863=CARTESIAN_POINT ( 'NONE',  ( -4.379528057220328563, 16.55341960407611168, 25.20724293864769550 ) ) ;
#22864=CARTESIAN_POINT ( 'NONE',  ( 13.97604488694527802, 13.89961937509977652, 64.37390960531436690 ) ) ;
#22865=CARTESIAN_POINT ( 'NONE',  ( -19.05341960407617563, 5.049401038297882671, 28.54275706135232937 ) ) ;
#22866=CARTESIAN_POINT ( 'NONE',  ( 16.52544592524335698, 4.483927247898782831, 31.45942372801901854 ) ) ;
#22867=CARTESIAN_POINT ( 'NONE',  ( -21.52544592524343514, 5.823673210054127303, 56.04057627198102409 ) ) ;
#22868=CARTESIAN_POINT ( 'NONE',  ( 18.67979575497194134, -10.72451020669871369, 110.8344237280190043 ) ) ;
#22870=CARTESIAN_POINT ( 'NONE',  ( 13.97604488694527802, 13.89961937509977652, 59.37390960531434558 ) ) ;
#22872=CARTESIAN_POINT ( 'NONE',  ( 5.153800228976335163, 19.02544592524342804, 94.79057627198103830 ) ) ;
#22873=CARTESIAN_POINT ( 'NONE',  ( -17.72560187377284890, -5.500000000000053291, 44.07814504131320632 ) ) ;
#22874=CARTESIAN_POINT ( 'NONE',  ( -15.72974639402176322, -15.80617190586768395, 24.37609039468567573 ) ) ;
#22875=CARTESIAN_POINT ( 'NONE',  ( -12.14591786802309592, -12.06949235617757132, 96.87390960531436690 ) ) ;
#22876=CARTESIAN_POINT ( 'NONE',  ( 18.62759615963271287, -10.81492255796078972, 93.33224293864769550 ) ) ;
#22877=CARTESIAN_POINT ( 'NONE',  ( -9.564922557960796823, -16.46253265017161027, 67.08224293864769550 ) ) ;
#22878=CARTESIAN_POINT ( 'NONE',  ( 5.049401038298161559, -19.05341960407611168, 87.70724293864769550 ) ) ;
#22879=CARTESIAN_POINT ( 'NONE',  ( -21.52544592524343514, 5.823673210054127303, 111.0405762719810525 ) ) ;
#22880=EDGE_CURVE ( 'NONE', #44580, #196699, #122143, .T. ) ;
#22882=CARTESIAN_POINT ( 'NONE',  ( -19.05341960407611168, -5.049401038298163336, 76.45724293864769550 ) ) ;
#22883=CARTESIAN_POINT ( 'NONE',  ( 18.39443945427639093, -5.500000000000021316, 96.01745347608654413 ) ) ;
#22884=CARTESIAN_POINT ( 'NONE',  ( -16.55341960407611168, -4.379528057220339221, 106.4572429386477097 ) ) ;
#22886=CARTESIAN_POINT ( 'NONE',  ( -19.05341960407617563, 5.049401038297882671, 93.54275706135234714 ) ) ;
#22887=CARTESIAN_POINT ( 'NONE',  ( -4.379528057220328563, 16.55341960407611168, 95.20724293864769550 ) ) ;
#22888=CARTESIAN_POINT ( 'NONE',  ( -18.67979575497193778, 10.72451020669871902, 73.33442372801901854 ) ) ;
#22889=CARTESIAN_POINT ( 'NONE',  ( -5.153800228976328057, -19.02544592524343514, 67.29057627198102409 ) ) ;
#22890=CARTESIAN_POINT ( 'NONE',  ( 10.72451020669871369, 18.67979575497193778, 32.08442372801901854 ) ) ;
#22891=CARTESIAN_POINT ( 'NONE',  ( -18.62759615963270932, 10.81492255796079327, 115.8322429386477097 ) ) ;
#22893=CARTESIAN_POINT ( 'NONE',  ( 9.474510206698971260, -16.51473224551069308, 67.91557627198102409 ) ) ;
#22895=CARTESIAN_POINT ( 'NONE',  ( 8.224510206698742110, 14.34966873604972548, 32.08442372801901854 ) ) ;
#22896=CARTESIAN_POINT ( 'NONE',  ( -21.53943276465977519, 0.05219959533907696930, 31.24890960531435979 ) ) ;
#22897=CARTESIAN_POINT ( 'NONE',  ( -21.53943276465977519, -0.05219959533937600094, 68.75109039468568994 ) ) ;
#22898=CARTESIAN_POINT ( 'NONE',  ( -5.153800228976328057, -19.02544592524343514, 107.2905762719810383 ) ) ;
#22899=CARTESIAN_POINT ( 'NONE',  ( -5.049401038297874678, -19.05341960407617918, 99.79275706135234714 ) ) ;
#22900=CARTESIAN_POINT ( 'NONE',  ( -19.05341960407611168, -5.049401038298163336, 46.45724293864768129 ) ) ;
#22901=CARTESIAN_POINT ( 'NONE',  ( 9.474510206698971260, -16.51473224551069308, 67.91557627198102409 ) ) ;
#22902=CARTESIAN_POINT ( 'NONE',  ( 12.14591786802309770, 12.06949235617756955, 89.37390960531435269 ) ) ;
#22903=CARTESIAN_POINT ( 'NONE',  ( 0.05219959533909260263, 19.03943276465977164, 99.99890960531436690 ) ) ;
#22904=CARTESIAN_POINT ( 'NONE',  ( -12.14591786802309592, -12.06949235617757132, 96.87390960531436690 ) ) ;
#22905=CARTESIAN_POINT ( 'NONE',  ( 19.03943276465977164, -0.05219959533909143690, 93.74890960531435269 ) ) ;
#22906=CARTESIAN_POINT ( 'NONE',  ( 8.224510206698953496, -14.34966873604960469, 47.91557627198102409 ) ) ;
#22907=CARTESIAN_POINT ( 'NONE',  ( -5.153800228976328057, -19.02544592524343514, 47.29057627198102409 ) ) ;
#22908=CARTESIAN_POINT ( 'NONE',  ( -15.72974639402176322, -15.80617190586768395, 59.37609039468568284 ) ) ;
#22909=CARTESIAN_POINT ( 'NONE',  ( -16.51473224551082808, 9.474510206698731452, 93.33442372801900433 ) ) ;
#22910=CARTESIAN_POINT ( 'NONE',  ( -4.379528057220328563, 16.55341960407611168, 50.20724293864769550 ) ) ;
#22911=CARTESIAN_POINT ( 'NONE',  ( 15.72974639402199770, -15.80617190586745480, 103.1239096053143811 ) ) ;
#22912=CARTESIAN_POINT ( 'NONE',  ( -10.81492255796078084, -18.62759615963271287, 52.08224293864768839 ) ) ;
#22913=CARTESIAN_POINT ( 'NONE',  ( 18.89770734986045397, 5.500000000000087930, 71.60214472496640781 ) ) ;
#22914=CARTESIAN_POINT ( 'NONE',  ( 12.14591786802309770, 12.06949235617756955, 84.37390960531438111 ) ) ;
#22916=CARTESIAN_POINT ( 'NONE',  ( 19.02544592524343514, -5.153800228976328945, 53.54057627198102409 ) ) ;
#22917=CARTESIAN_POINT ( 'NONE',  ( 14.29746914071037800, 8.314922557961029526, 111.6677570613523613 ) ) ;
#22918=CARTESIAN_POINT ( 'NONE',  ( -8.314922557961024197, 14.29746914071037800, 107.9177570613523471 ) ) ;
#22919=CARTESIAN_POINT ( 'NONE',  ( -14.29746914071037622, -8.314922557961029526, 89.16775706135236135 ) ) ;
#22920=CARTESIAN_POINT ( 'NONE',  ( -16.51473224551082808, 9.474510206698731452, 38.33442372801899722 ) ) ;
#22921=CARTESIAN_POINT ( 'NONE',  ( 30.00000000000000000, 5.499999999999992895, 37.50000000000000000 ) ) ;
#22922=CARTESIAN_POINT ( 'NONE',  ( -9.474510206698964154, 16.51473224551069663, 110.4155762719810383 ) ) ;
#22923=CARTESIAN_POINT ( 'NONE',  ( -0.05219959533909027116, -19.03943276465977164, 82.49890960531436690 ) ) ;
#22924=CARTESIAN_POINT ( 'NONE',  ( 16.51473224551069308, 9.474510206698969483, 39.16557627198103120 ) ) ;
#22925=CARTESIAN_POINT ( 'NONE',  ( 12.14591786802309770, 12.06949235617756955, 44.37390960531435979 ) ) ;
#22927=CARTESIAN_POINT ( 'NONE',  ( 9.564922557960805705, 16.46253265017160317, 109.5822429386476955 ) ) ;
#22928=CARTESIAN_POINT ( 'NONE',  ( -0.05219959533907301413, -21.53943276465977519, 42.49890960531435979 ) ) ;
#22929=CARTESIAN_POINT ( 'NONE',  ( 12.14591786802309770, 12.06949235617756955, 89.37390960531435269 ) ) ;
#22930=CARTESIAN_POINT ( 'NONE',  ( 8.224510206698742110, 14.34966873604972548, 37.08442372801901143 ) ) ;
#22931=CARTESIAN_POINT ( 'NONE',  ( 8.224510206698953496, -14.34966873604960469, 62.91557627198102409 ) ) ;
#22933=CARTESIAN_POINT ( 'NONE',  ( 13.97604488694548053, -13.89961937509957401, 65.62609039468567573 ) ) ;
#22934=CARTESIAN_POINT ( 'NONE',  ( -19.03943276465977164, 0.05219959533909376836, 96.24890960531436690 ) ) ;
#22935=CARTESIAN_POINT ( 'NONE',  ( -13.89961937509957401, -13.97604488694547875, 79.37609039468567573 ) ) ;
#22936=CARTESIAN_POINT ( 'NONE',  ( 9.564922557961047289, -16.46253265017146816, 40.41775706135234003 ) ) ;
#22937=CARTESIAN_POINT ( 'NONE',  ( -16.53943276465976808, -0.05219959533934237506, 33.75109039468568284 ) ) ;
#22938=CARTESIAN_POINT ( 'NONE',  ( 14.29746914071037800, 8.314922557961029526, 106.6677570613523756 ) ) ;
#22939=CARTESIAN_POINT ( 'NONE',  ( -19.05341960407617563, 5.049401038297882671, 73.54275706135233293 ) ) ;
#22940=CARTESIAN_POINT ( 'NONE',  ( -21.55341960407610458, -5.719274019375992779, 31.45724293864769550 ) ) ;
#22941=CARTESIAN_POINT ( 'NONE',  ( 5.719274019375673035, 21.55341960407619339, 72.29275706135236135 ) ) ;
#22943=CARTESIAN_POINT ( 'NONE',  ( 16.53943276465976808, 0.05219959533934440121, 21.25109039468567218 ) ) ;
#22944=CARTESIAN_POINT ( 'NONE',  ( -16.51473224551069308, -9.474510206698971260, 21.66557627198102765 ) ) ;
#22945=CARTESIAN_POINT ( 'NONE',  ( -19.03943276465977164, 0.05219959533909376836, 86.24890960531436690 ) ) ;
#22946=CARTESIAN_POINT ( 'NONE',  ( 9.474510206698971260, -16.51473224551069308, 22.91557627198102765 ) ) ;
#22947=CARTESIAN_POINT ( 'NONE',  ( -16.55341960407611168, -4.379528057220339221, 91.45724293864769550 ) ) ;
#22948=CARTESIAN_POINT ( 'NONE',  ( -5.153800228976328057, -19.02544592524343514, 82.29057627198103830 ) ) ;
#22949=CARTESIAN_POINT ( 'NONE',  ( 16.51473224551069308, 9.474510206698969483, 84.16557627198102409 ) ) ;
#22951=CARTESIAN_POINT ( 'NONE',  ( 13.89961937509957401, 13.97604488694547697, 96.87609039468566152 ) ) ;
#22952=CARTESIAN_POINT ( 'NONE',  ( 10.72451020669898902, -18.67979575497178502, 82.91557627198103830 ) ) ;
#22953=CARTESIAN_POINT ( 'NONE',  ( 13.97604488694527802, 13.89961937509977652, 29.37390960531435979 ) ) ;
#22954=CARTESIAN_POINT ( 'NONE',  ( 5.049401038297881783, 19.05341960407617563, 67.29275706135234714 ) ) ;
#22955=CARTESIAN_POINT ( 'NONE',  ( 5.823673210054125526, 21.52544592524343514, 109.7905762719810383 ) ) ;
#22956=CARTESIAN_POINT ( 'NONE',  ( -9.564922557960796823, -16.46253265017161027, 67.08224293864769550 ) ) ;
#22957=CARTESIAN_POINT ( 'NONE',  ( 5.049401038298161559, -19.05341960407611168, 107.7072429386476955 ) ) ;
#22958=VERTEX_POINT ( 'NONE', #105987 ) ;
#22959=CARTESIAN_POINT ( 'NONE',  ( -10.72451020669898014, 18.67979575497178502, 100.4155762719810241 ) ) ;
#22960=CARTESIAN_POINT ( 'NONE',  ( 8.314922557960818139, 14.29746914071049879, 89.58224293864768129 ) ) ;
#22961=CARTESIAN_POINT ( 'NONE',  ( 9.564922557960805705, 16.46253265017160317, 84.58224293864769550 ) ) ;
#22962=CARTESIAN_POINT ( 'NONE',  ( -0.05219959533936034679, 19.03943276465977164, 67.50109039468566152 ) ) ;
#22963=CARTESIAN_POINT ( 'NONE',  ( 15.80617190586746368, 15.72974639402197994, 89.37390960531435269 ) ) ;
#22964=CARTESIAN_POINT ( 'NONE',  ( 15.72974639402199770, -15.80617190586745480, 68.12390960531436690 ) ) ;
#22965=CARTESIAN_POINT ( 'NONE',  ( -16.52544592524342804, 4.483927247898546575, 41.04057627198103120 ) ) ;
#22966=CARTESIAN_POINT ( 'NONE',  ( -18.62759615963255300, -10.81492255796106328, 99.16775706135234714 ) ) ;
#22967=CARTESIAN_POINT ( 'NONE',  ( -16.53943276465976808, -0.05219959533934237506, 63.75109039468568284 ) ) ;
#22968=CARTESIAN_POINT ( 'NONE',  ( -0.05219959533909027116, -19.03943276465977164, 92.49890960531436690 ) ) ;
#22969=CARTESIAN_POINT ( 'NONE',  ( 5.153800228976335163, 19.02544592524342804, 39.79057627198100988 ) ) ;
#22970=CARTESIAN_POINT ( 'NONE',  ( 21.52544592524334988, 5.823673210054432836, 46.45942372801901854 ) ) ;
#22971=CARTESIAN_POINT ( 'NONE',  ( -15.80617190586768217, 15.72974639402176855, 48.12609039468568284 ) ) ;
#22972=CARTESIAN_POINT ( 'NONE',  ( 19.03943276465977164, -0.05219959533909143690, 58.74890960531435979 ) ) ;
#22973=CARTESIAN_POINT ( 'NONE',  ( -10.72451020669870658, -18.67979575497194134, 39.58442372801901143 ) ) ;
#22974=CARTESIAN_POINT ( 'NONE',  ( 16.46253265017146816, 9.564922557961045513, 71.66775706135233293 ) ) ;
#22975=CARTESIAN_POINT ( 'NONE',  ( -16.46253265017146816, -9.564922557961047289, 79.16775706135234714 ) ) ;
#22976=CARTESIAN_POINT ( 'NONE',  ( -19.02544592524342804, 5.153800228976336051, 36.04057627198100988 ) ) ;
#22977=CARTESIAN_POINT ( 'NONE',  ( 8.314922557961029526, -14.29746914071037800, 80.41775706135234714 ) ) ;
#22978=CARTESIAN_POINT ( 'NONE',  ( -13.89961937509977652, 13.97604488694528158, 50.62390960531435979 ) ) ;
#22980=CARTESIAN_POINT ( 'NONE',  ( 19.05341960407611168, 5.049401038298154454, 93.95724293864769550 ) ) ;
#22981=CARTESIAN_POINT ( 'NONE',  ( 19.03943276465977164, -0.05219959533909143690, 33.74890960531435979 ) ) ;
#22982=CARTESIAN_POINT ( 'NONE',  ( -5.823673210054116645, -21.52544592524344225, 77.29057627198102409 ) ) ;
#22983=CARTESIAN_POINT ( 'NONE',  ( 16.53943276465976808, 0.05219959533934440121, 61.25109039468567573 ) ) ;
#22984=CARTESIAN_POINT ( 'NONE',  ( -19.05341960407617563, 5.049401038297882671, 23.54275706135233648 ) ) ;
#22987=CARTESIAN_POINT ( 'NONE',  ( -9.564922557960796823, -16.46253265017161027, 52.08224293864768839 ) ) ;
#22988=CARTESIAN_POINT ( 'NONE',  ( 12.06949235617757843, -12.14591786802309237, 43.12390960531435269 ) ) ;
#22989=CARTESIAN_POINT ( 'NONE',  ( -14.29746914071049879, 8.314922557960819915, 80.83224293864769550 ) ) ;
#22990=CARTESIAN_POINT ( 'NONE',  ( 9.474510206698971260, -16.51473224551069308, 82.91557627198103830 ) ) ;
#22991=CARTESIAN_POINT ( 'NONE',  ( 15.80617190586769283, -15.72974639402175789, 30.62609039468567929 ) ) ;
#22992=CARTESIAN_POINT ( 'NONE',  ( -19.02544592524342804, 5.153800228976336051, 96.04057627198103830 ) ) ;
#22993=CARTESIAN_POINT ( 'NONE',  ( 5.719274019375673035, 21.55341960407619339, 97.29275706135234714 ) ) ;
#22994=CARTESIAN_POINT ( 'NONE',  ( 8.314922557961029526, -14.29746914071037800, 65.41775706135234714 ) ) ;
#22995=CARTESIAN_POINT ( 'NONE',  ( 18.62759615963255655, 10.81492255796105972, 31.66775706135234358 ) ) ;
#22996=CARTESIAN_POINT ( 'NONE',  ( -13.89961937509977652, 13.97604488694528158, 105.6239096053143527 ) ) ;
#22997=B_SPLINE_CURVE_WITH_KNOTS ( 'NONE', 3,
 ( #66011, #189379, #50856, #68004, #114499, #112514 ),
 .UNSPECIFIED., .F., .F.,
 ( 4, 2, 4 ),
 ( 0.003239945802372208323, 0.003620412082092060516, 0.004000878361811913142 ),
 .UNSPECIFIED. ) ;
#22998=EDGE_CURVE ( 'NONE', #88472, #5512, #16601, .T. ) ;
#22999=CARTESIAN_POINT ( 'NONE',  ( 21.52544592524344225, -5.823673210054117533, 83.54057627198102409 ) ) ;
#23000=CARTESIAN_POINT ( 'NONE',  ( -12.06949235617756955, 12.14591786802309770, 45.62390960531436690 ) ) ;
#23001=CARTESIAN_POINT ( 'NONE',  ( -13.97604488694527625, -13.89961937509977652, 46.87390960531435979 ) ) ;
#23002=CARTESIAN_POINT ( 'NONE',  ( -14.34966873604960291, -8.224510206698953496, 71.66557627198100988 ) ) ;
#23003=CARTESIAN_POINT ( 'NONE',  ( -10.81492255796078084, -18.62759615963271287, 32.08224293864769550 ) ) ;
#23004=CARTESIAN_POINT ( 'NONE',  ( 16.51473224551083163, -9.474510206698727899, 30.83442372801900433 ) ) ;
#23005=CARTESIAN_POINT ( 'NONE',  ( 14.34966873604960469, 8.224510206698951720, 99.16557627198100988 ) ) ;
#23006=CARTESIAN_POINT ( 'NONE',  ( -19.02544592524342804, 5.153800228976336051, 111.0405762719810099 ) ) ;
#23008=CARTESIAN_POINT ( 'NONE',  ( 0.05219959533934541429, -16.53943276465976808, 60.00109039468568284 ) ) ;
#23009=CARTESIAN_POINT ( 'NONE',  ( 9.564922557960805705, 16.46253265017160317, 49.58224293864770260 ) ) ;
#23011=CARTESIAN_POINT ( 'NONE',  ( -0.05219959533934338120, 16.53943276465976808, 97.50109039468567573 ) ) ;
#23012=CARTESIAN_POINT ( 'NONE',  ( -0.05219959533936034679, 19.03943276465977164, 102.5010903946856757 ) ) ;
#23013=CARTESIAN_POINT ( 'NONE',  ( -5.823673210054431948, 21.52544592524334988, 67.70942372801901854 ) ) ;
#23014=CARTESIAN_POINT ( 'NONE',  ( 16.51473224551069308, 9.474510206698969483, 74.16557627198103830 ) ) ;
#23015=CARTESIAN_POINT ( 'NONE',  ( -5.823673210054116645, -21.52544592524344225, 87.29057627198103830 ) ) ;
#23016=CARTESIAN_POINT ( 'NONE',  ( -4.483927247898782831, 16.52544592524335698, 37.70942372801900433 ) ) ;
#23017=CARTESIAN_POINT ( 'NONE',  ( 19.03943276465977164, -0.05219959533909143690, 23.74890960531435269 ) ) ;
#23018=CARTESIAN_POINT ( 'NONE',  ( 16.51473224551083163, -9.474510206698727899, 80.83442372801899012 ) ) ;
#23019=CARTESIAN_POINT ( 'NONE',  ( 5.823673210054125526, 21.52544592524343514, 74.79057627198105251 ) ) ;
#23020=CARTESIAN_POINT ( 'NONE',  ( 9.564922557961047289, -16.46253265017146816, 45.41775706135232582 ) ) ;
#23021=CARTESIAN_POINT ( 'NONE',  ( -16.46253265017160317, 9.564922557960807481, 115.8322429386477097 ) ) ;
#23023=CARTESIAN_POINT ( 'NONE',  ( -10.72451020669898014, 18.67979575497178502, 95.41557627198102409 ) ) ;
#23025=CARTESIAN_POINT ( 'NONE',  ( -13.89961937509977652, 13.97604488694528158, 65.62390960531436690 ) ) ;
#23027=CARTESIAN_POINT ( 'NONE',  ( -19.05341960407617563, 5.049401038297882671, 108.5427570613523187 ) ) ;
#23029=CARTESIAN_POINT ( 'NONE',  ( -19.02544592524342804, 5.153800228976336051, 41.04057627198103120 ) ) ;
#23030=CARTESIAN_POINT ( 'NONE',  ( -18.62759615963270932, 10.81492255796079327, 100.8322429386477097 ) ) ;
#23031=CARTESIAN_POINT ( 'NONE',  ( -4.483927247898539470, -16.52544592524342804, 57.29057627198103120 ) ) ;
#23032=CARTESIAN_POINT ( 'NONE',  ( -19.05341960407611168, -5.049401038298163336, 56.45724293864768129 ) ) ;
#23033=CARTESIAN_POINT ( 'NONE',  ( 21.52544592524334988, 5.823673210054432836, 76.45942372801901854 ) ) ;
#23034=CARTESIAN_POINT ( 'NONE',  ( 0.05219959533934541429, -16.53943276465976808, 20.00109039468568639 ) ) ;
#23035=CARTESIAN_POINT ( 'NONE',  ( 5.049401038297881783, 19.05341960407617563, 27.29275706135232937 ) ) ;
#23036=CARTESIAN_POINT ( 'NONE',  ( 15.72974639402176855, 15.80617190586768217, 36.87609039468568994 ) ) ;
#23037=CARTESIAN_POINT ( 'NONE',  ( -5.823673210054116645, -21.52544592524344225, 107.2905762719810525 ) ) ;
#23038=CARTESIAN_POINT ( 'NONE',  ( 10.81492255796078972, 18.62759615963270932, 54.58224293864769550 ) ) ;
#23039=CARTESIAN_POINT ( 'NONE',  ( 5.049401038297881783, 19.05341960407617563, 102.2927570613523045 ) ) ;
#23040=CARTESIAN_POINT ( 'NONE',  ( -13.89961937509957401, -13.97604488694547875, 74.37609039468566152 ) ) ;
#23041=CARTESIAN_POINT ( 'NONE',  ( 21.52544592524334988, 5.823673210054432836, 81.45942372801900433 ) ) ;
#23042=CARTESIAN_POINT ( 'NONE',  ( 19.05341960407617918, -5.049401038297876454, 51.04275706135231871 ) ) ;
#23043=CARTESIAN_POINT ( 'NONE',  ( -9.564922557960796823, -16.46253265017161027, 22.08224293864768839 ) ) ;
#23044=CARTESIAN_POINT ( 'NONE',  ( 5.719274019375991003, -21.55341960407610458, 52.70724293864769550 ) ) ;
#23045=CARTESIAN_POINT ( 'NONE',  ( 16.53943276465976808, -0.05219959533910856209, 43.74890960531435979 ) ) ;
#23046=CARTESIAN_POINT ( 'NONE',  ( -16.29526858892873875, -7.335722546920240283, 25.79670597800208753 ) ) ;
#23047=CARTESIAN_POINT ( 'NONE',  ( -21.53943276465977519, -0.05219959533937600094, 113.7510903946856757 ) ) ;
#23048=CARTESIAN_POINT ( 'NONE',  ( -14.29746914071037622, -8.314922557961029526, 89.16775706135236135 ) ) ;
#23049=CARTESIAN_POINT ( 'NONE',  ( 0.05219959533910956823, 16.53943276465976808, 44.99890960531435979 ) ) ;
#23050=CARTESIAN_POINT ( 'NONE',  ( -21.52544592524334988, -5.823673210054445271, 73.95942372801901854 ) ) ;
#23051=CARTESIAN_POINT ( 'NONE',  ( -0.05219959533937732626, 21.53943276465977519, 82.50109039468568994 ) ) ;
#23052=CARTESIAN_POINT ( 'NONE',  ( -21.55341960407610458, -5.719274019375992779, 76.45724293864769550 ) ) ;
#23053=CARTESIAN_POINT ( 'NONE',  ( 16.51473224551069308, 9.474510206698969483, 39.16557627198103120 ) ) ;
#23054=CARTESIAN_POINT ( 'NONE',  ( 5.823673210054444382, -21.52544592524334988, 50.20942372801901854 ) ) ;
#23055=CARTESIAN_POINT ( 'NONE',  ( -5.049401038298153566, 19.05341960407611168, 30.20724293864768839 ) ) ;
#23056=VERTEX_POINT ( 'NONE', #1292 ) ;
#23057=CARTESIAN_POINT ( 'NONE',  ( -13.97604488694527625, -13.89961937509977652, 51.87390960531436690 ) ) ;
#23058=CARTESIAN_POINT ( 'NONE',  ( 12.14591786802309770, 12.06949235617756955, 94.37390960531436690 ) ) ;
#23059=CARTESIAN_POINT ( 'NONE',  ( 19.02544592524343514, -5.153800228976328945, 98.54057627198100988 ) ) ;
#23060=CARTESIAN_POINT ( 'NONE',  ( 14.34966873604960469, 8.224510206698951720, 39.16557627198102409 ) ) ;
#23061=CARTESIAN_POINT ( 'NONE',  ( -14.29746914071049879, 8.314922557960819915, 115.8322429386477097 ) ) ;
#23062=CARTESIAN_POINT ( 'NONE',  ( -15.72974639402197994, 15.80617190586746368, 85.62390960531436690 ) ) ;
#23063=CARTESIAN_POINT ( 'NONE',  ( 18.62759615963255655, 10.81492255796105972, 21.66775706135235069 ) ) ;
#23065=CARTESIAN_POINT ( 'NONE',  ( -16.55341960407617563, 4.379528057220093196, 43.54275706135235424 ) ) ;
#23066=CARTESIAN_POINT ( 'NONE',  ( -0.05219959533907301413, -21.53943276465977519, 67.49890960531436690 ) ) ;
#23067=CARTESIAN_POINT ( 'NONE',  ( 18.67979575497194134, -10.72451020669871369, 100.8344237280190185 ) ) ;
#23068=CARTESIAN_POINT ( 'NONE',  ( -5.049401038298153566, 19.05341960407611168, 90.20724293864766707 ) ) ;
#23069=CARTESIAN_POINT ( 'NONE',  ( 5.823673210054444382, -21.52544592524334988, 25.20942372801901854 ) ) ;
#23070=CARTESIAN_POINT ( 'NONE',  ( 15.80617190586746368, 15.72974639402197994, 29.37390960531435269 ) ) ;
#23071=CARTESIAN_POINT ( 'NONE',  ( 12.06949235617739724, 12.14591786802326823, 86.87609039468568994 ) ) ;
#23072=CARTESIAN_POINT ( 'NONE',  ( -15.72974639402176322, -15.80617190586768395, 74.37609039468568994 ) ) ;
#23073=B_SPLINE_CURVE_WITH_KNOTS ( 'NONE', 3,
 ( #20934, #191784, #189808, #83592, #114943, #177639, #132111, #116939, #84588, #178632, #54276, #192794 ),
 .UNSPECIFIED., .F., .F.,
 ( 4, 2, 2, 2, 2, 4 ),
 ( 0.002244533994399181866, 0.002800305961463223602, 0.003078191944995248373, 0.003356077928527273144, 0.003911849895591323553, 0.004467621862655373095 ),
 .UNSPECIFIED. ) ;
#23074=CARTESIAN_POINT ( 'NONE',  ( -21.55341960407619339, 5.719274019375674811, 108.5427570613523756 ) ) ;
#23075=CARTESIAN_POINT ( 'NONE',  ( 12.14591786802327356, -12.06949235617739191, 80.62609039468567573 ) ) ;
#23076=CARTESIAN_POINT ( 'NONE',  ( -21.55341960407619339, 5.719274019375674811, 33.54275706135234714 ) ) ;
#23077=CARTESIAN_POINT ( 'NONE',  ( -19.02544592524342804, 5.153800228976336051, 36.04057627198100988 ) ) ;
#23078=CARTESIAN_POINT ( 'NONE',  ( 21.55341960407619695, -5.719274019375665929, 91.04275706135236135 ) ) ;
#23079=CARTESIAN_POINT ( 'NONE',  ( 9.474510206698971260, -16.51473224551069308, 107.9155762719810383 ) ) ;
#23080=CARTESIAN_POINT ( 'NONE',  ( -5.823673210054116645, -21.52544592524344225, 107.2905762719810525 ) ) ;
#23081=CARTESIAN_POINT ( 'NONE',  ( 18.22780087662121673, 5.500000000000056843, 83.98459894673892734 ) ) ;
#23082=CARTESIAN_POINT ( 'NONE',  ( -10.72451020669898014, 18.67979575497178502, 55.41557627198102409 ) ) ;
#23083=CARTESIAN_POINT ( 'NONE',  ( -16.46253265017160317, 9.564922557960807481, 95.83224293864769550 ) ) ;
#23084=CARTESIAN_POINT ( 'NONE',  ( -8.314922557960811034, -14.29746914071050412, 47.08224293864770260 ) ) ;
#23086=CARTESIAN_POINT ( 'NONE',  ( -19.05341960407617563, 5.049401038297882671, 78.54275706135233293 ) ) ;
#23087=CARTESIAN_POINT ( 'NONE',  ( -16.62475595723699229, 7.163666690055301878, 105.5271335181047476 ) ) ;
#23088=CARTESIAN_POINT ( 'NONE',  ( 16.46253265017146816, 9.564922557961045513, 111.6677570613523329 ) ) ;
#23089=CARTESIAN_POINT ( 'NONE',  ( -18.62759615963270932, 10.81492255796079327, 90.83224293864769550 ) ) ;
#23090=CARTESIAN_POINT ( 'NONE',  ( -0.05219959533910754901, -16.53943276465976808, 62.49890960531436690 ) ) ;
#23091=CARTESIAN_POINT ( 'NONE',  ( -16.46253265017160317, 9.564922557960807481, 105.8322429386476955 ) ) ;
#23092=CARTESIAN_POINT ( 'NONE',  ( -14.34966873604972548, 8.224510206698743886, 48.33442372801902565 ) ) ;
#23093=CARTESIAN_POINT ( 'NONE',  ( 9.474510206698971260, -16.51473224551069308, 52.91557627198102409 ) ) ;
#23094=CARTESIAN_POINT ( 'NONE',  ( -10.81492255796105439, 18.62759615963255655, 27.91775706135234358 ) ) ;
#23095=CARTESIAN_POINT ( 'NONE',  ( 16.46253265017146816, 9.564922557961045513, 91.66775706135234714 ) ) ;
#23096=CARTESIAN_POINT ( 'NONE',  ( 13.97604488694527802, 13.89961937509977652, 94.37390960531436690 ) ) ;
#23097=CARTESIAN_POINT ( 'NONE',  ( 19.05341960407611168, 5.049401038298154454, 88.95724293864769550 ) ) ;
#23098=CARTESIAN_POINT ( 'NONE',  ( 5.823673210054125526, 21.52544592524343514, 94.79057627198105251 ) ) ;
#23099=CARTESIAN_POINT ( 'NONE',  ( -19.02544592524342804, 5.153800228976336051, 51.04057627198103120 ) ) ;
#23100=CARTESIAN_POINT ( 'NONE',  ( -16.88567814943164791, -6.947325034625601248, 61.29001122652586986 ) ) ;
#23101=CARTESIAN_POINT ( 'NONE',  ( 12.14591786802309770, 12.06949235617756955, 74.37390960531436690 ) ) ;
#23102=CARTESIAN_POINT ( 'NONE',  ( -0.05219959533909027116, -19.03943276465977164, 102.4989096053143669 ) ) ;
#23104=CARTESIAN_POINT ( 'NONE',  ( 19.05341960407617918, -5.049401038297876454, 61.04275706135232582 ) ) ;
#23105=CARTESIAN_POINT ( 'NONE',  ( 5.823673210054125526, 21.52544592524343514, 84.79057627198102409 ) ) ;
#23106=CARTESIAN_POINT ( 'NONE',  ( -19.03943276465977164, -0.05219959533935918106, 53.75109039468566863 ) ) ;
#23107=CARTESIAN_POINT ( 'NONE',  ( 16.46253265017160672, -9.564922557960803928, 98.33224293864769550 ) ) ;
#23108=CARTESIAN_POINT ( 'NONE',  ( 17.60691670004650433, 5.500000000000060396, 76.63333313366442212 ) ) ;
#23109=CARTESIAN_POINT ( 'NONE',  ( 10.81492255796078972, 18.62759615963270932, 39.58224293864769550 ) ) ;
#23110=CARTESIAN_POINT ( 'NONE',  ( 13.97604488694527802, 13.89961937509977652, 89.37390960531436690 ) ) ;
#23111=EDGE_CURVE ( 'NONE', #14026, #142736, #166211, .T. ) ;
#23112=CARTESIAN_POINT ( 'NONE',  ( 10.72451020669871369, 18.67979575497193778, 62.08442372801901143 ) ) ;
#23113=CARTESIAN_POINT ( 'NONE',  ( 16.46253265017160672, -9.564922557960803928, 33.33224293864770260 ) ) ;
#23114=CARTESIAN_POINT ( 'NONE',  ( 12.06949235617757843, -12.14591786802309237, 78.12390960531436690 ) ) ;
#23115=CARTESIAN_POINT ( 'NONE',  ( 8.314922557961029526, -14.29746914071037800, 25.41775706135235779 ) ) ;
#23116=CARTESIAN_POINT ( 'NONE',  ( 5.823673210054444382, -21.52544592524334988, 55.20942372801902565 ) ) ;
#23119=CARTESIAN_POINT ( 'NONE',  ( -13.89961937509957401, -13.97604488694547875, 69.37609039468564731 ) ) ;
#23120=CARTESIAN_POINT ( 'NONE',  ( -17.49999999999999645, 5.499999999999997335, 120.0000000000000142 ) ) ;
#23121=CARTESIAN_POINT ( 'NONE',  ( -18.62759615963255300, -10.81492255796106328, 24.16775706135235424 ) ) ;
#23123=CARTESIAN_POINT ( 'NONE',  ( -13.89961937509957401, -13.97604488694547875, 19.37609039468566507 ) ) ;
#23124=CARTESIAN_POINT ( 'NONE',  ( -19.03943276465977164, 0.05219959533909376836, 56.24890960531435979 ) ) ;
#23125=CARTESIAN_POINT ( 'NONE',  ( 21.52544592524334988, 5.823673210054432836, 111.4594237280190328 ) ) ;
#23126=CARTESIAN_POINT ( 'NONE',  ( 14.29746914071037800, 8.314922557961029526, 106.6677570613523756 ) ) ;
#23127=CARTESIAN_POINT ( 'NONE',  ( -0.05219959533909027116, -19.03943276465977164, 107.4989096053143527 ) ) ;
#23128=CARTESIAN_POINT ( 'NONE',  ( -15.72974639402176322, -15.80617190586768395, 74.37609039468568994 ) ) ;
#23130=CARTESIAN_POINT ( 'NONE',  ( -16.46253265017160317, 9.564922557960807481, 110.8322429386476955 ) ) ;
#23132=CARTESIAN_POINT ( 'NONE',  ( 16.53943276465976808, 0.05219959533934440121, 66.25109039468567573 ) ) ;
#23133=CARTESIAN_POINT ( 'NONE',  ( 21.55341960407619695, -5.719274019375665929, 76.04275706135237556 ) ) ;
#23134=CARTESIAN_POINT ( 'NONE',  ( 21.52544592524334988, 5.823673210054432836, 106.4594237280190328 ) ) ;
#23135=CARTESIAN_POINT ( 'NONE',  ( 17.50000000000000711, -5.499999999999978684, 41.21769037696436300 ) ) ;
#23136=CARTESIAN_POINT ( 'NONE',  ( 16.46253265017160672, -9.564922557960803928, 83.33224293864768129 ) ) ;
#23137=CARTESIAN_POINT ( 'NONE',  ( 16.46253265017160672, -9.564922557960803928, 108.3322429386476955 ) ) ;
#23138=ORIENTED_EDGE ( 'NONE', *, *, #80326, .F. ) ;
#23140=CARTESIAN_POINT ( 'NONE',  ( 16.51473224551069308, 9.474510206698969483, 44.16557627198103120 ) ) ;
#23141=CARTESIAN_POINT ( 'NONE',  ( 5.719274019375991003, -21.55341960407610458, 37.70724293864769550 ) ) ;
#23143=CARTESIAN_POINT ( 'NONE',  ( 4.379528057220092307, 16.55341960407617563, 102.2927570613523613 ) ) ;
#23144=CARTESIAN_POINT ( 'NONE',  ( -12.06949235617756955, 12.14591786802309770, 95.62390960531436690 ) ) ;
#23145=CARTESIAN_POINT ( 'NONE',  ( -9.564922557960796823, -16.46253265017161027, 87.08224293864769550 ) ) ;
#23146=CARTESIAN_POINT ( 'NONE',  ( 15.72974639402176855, 15.80617190586768217, 106.8760903946856899 ) ) ;
#23147=CARTESIAN_POINT ( 'NONE',  ( 16.51473224551069308, 9.474510206698969483, 39.16557627198103120 ) ) ;
#23148=CARTESIAN_POINT ( 'NONE',  ( -8.314922557960811034, -14.29746914071050412, 92.08224293864769550 ) ) ;
#23149=CARTESIAN_POINT ( 'NONE',  ( 5.719274019375673035, 21.55341960407619339, 52.29275706135236135 ) ) ;
#23150=CARTESIAN_POINT ( 'NONE',  ( 15.72974639402199770, -15.80617190586745480, 88.12390960531436690 ) ) ;
#23151=CARTESIAN_POINT ( 'NONE',  ( 16.51473224551083163, -9.474510206698727899, 55.83442372801899722 ) ) ;
#23153=CARTESIAN_POINT ( 'NONE',  ( -9.474510206698964154, 16.51473224551069663, 90.41557627198103830 ) ) ;
#23154=CARTESIAN_POINT ( 'NONE',  ( -16.52544592524342804, 4.483927247898546575, 66.04057627198103830 ) ) ;
#23155=ADVANCED_FACE ( 'NONE', ( #62970 ), #175108, .T. ) ;
#23156=CARTESIAN_POINT ( 'NONE',  ( -9.474510206698720793, -16.51473224551083518, 49.58442372801899722 ) ) ;
#23157=CARTESIAN_POINT ( 'NONE',  ( -4.483927247898539470, -16.52544592524342804, 42.29057627198103120 ) ) ;
#23158=CARTESIAN_POINT ( 'NONE',  ( 16.46253265017146816, 9.564922557961045513, 76.66775706135234714 ) ) ;
#23159=CARTESIAN_POINT ( 'NONE',  ( -18.39443945427639093, 5.500000000000031086, 83.51745347608650150 ) ) ;
#23160=CARTESIAN_POINT ( 'NONE',  ( 15.80617190586746368, 15.72974639402197994, 34.37390960531435979 ) ) ;
#23161=CARTESIAN_POINT ( 'NONE',  ( -8.314922557960811034, -14.29746914071050412, 107.0822429386476955 ) ) ;
#23162=CARTESIAN_POINT ( 'NONE',  ( -17.49999999999996803, -3.209263204892610855, 25.23803174393711402 ) ) ;
#23163=CARTESIAN_POINT ( 'NONE',  ( 16.51473224551069308, 9.474510206698969483, 44.16557627198103120 ) ) ;
#23164=CARTESIAN_POINT ( 'NONE',  ( 5.719274019375991003, -21.55341960407610458, 47.70724293864770260 ) ) ;
#23165=CARTESIAN_POINT ( 'NONE',  ( -19.05341960407611168, -5.049401038298163336, 26.45724293864769550 ) ) ;
#23166=CARTESIAN_POINT ( 'NONE',  ( -0.05219959533934338120, 16.53943276465976808, 77.50109039468567573 ) ) ;
#23167=CARTESIAN_POINT ( 'NONE',  ( 16.46253265017160672, -9.564922557960803928, 63.33224293864769550 ) ) ;
#23168=CARTESIAN_POINT ( 'NONE',  ( 13.97604488694548053, -13.89961937509957401, 35.62609039468567573 ) ) ;
#23169=CARTESIAN_POINT ( 'NONE',  ( 10.81492255796106328, -18.62759615963255655, 70.41775706135236135 ) ) ;
#23170=CARTESIAN_POINT ( 'NONE',  ( 21.52544592524344225, -5.823673210054117533, 53.54057627198103120 ) ) ;
#23171=CARTESIAN_POINT ( 'NONE',  ( -0.05219959533909027116, -19.03943276465977164, 22.49890960531436690 ) ) ;
#23172=CARTESIAN_POINT ( 'NONE',  ( 16.51473224551083163, -9.474510206698727899, 110.8344237280190043 ) ) ;
#23175=CARTESIAN_POINT ( 'NONE',  ( 15.72974639402199770, -15.80617190586745480, 43.12390960531435269 ) ) ;
#23176=CARTESIAN_POINT ( 'NONE',  ( 17.49999999999998579, -5.500000000000023981, 68.29690382534171533 ) ) ;
#23177=CARTESIAN_POINT ( 'NONE',  ( 21.52544592524334988, 5.823673210054432836, 81.45942372801900433 ) ) ;
#23179=CARTESIAN_POINT ( 'NONE',  ( -12.14591786802309592, -12.06949235617757132, 41.87390960531435979 ) ) ;
#23180=CARTESIAN_POINT ( 'NONE',  ( 16.53943276465976808, -0.05219959533910856209, 58.74890960531436690 ) ) ;
#23181=CARTESIAN_POINT ( 'NONE',  ( 15.80617190586746368, 15.72974639402197994, 84.37390960531438111 ) ) ;
#23182=CARTESIAN_POINT ( 'NONE',  ( 5.823673210054125526, 21.52544592524343514, 79.79057627198102409 ) ) ;
#23184=CARTESIAN_POINT ( 'NONE',  ( 5.719274019375991003, -21.55341960407610458, 37.70724293864769550 ) ) ;
#23185=CARTESIAN_POINT ( 'NONE',  ( 14.29746914071037800, 8.314922557961029526, 51.66775706135234714 ) ) ;
#23186=CARTESIAN_POINT ( 'NONE',  ( -12.14591786802309592, -12.06949235617757132, 81.87390960531435269 ) ) ;
#23187=CARTESIAN_POINT ( 'NONE',  ( -19.03943276465977164, 0.05219959533909376836, 56.24890960531435979 ) ) ;
#23188=CARTESIAN_POINT ( 'NONE',  ( 13.89961937509977652, -13.97604488694527269, 33.12390960531434558 ) ) ;
#23190=CARTESIAN_POINT ( 'NONE',  ( -17.49999999999999645, 5.499999999999997335, 30.79690382534172599 ) ) ;
#23192=CARTESIAN_POINT ( 'NONE',  ( -4.379528057220086978, -16.55341960407618274, 84.79275706135234714 ) ) ;
#23193=CARTESIAN_POINT ( 'NONE',  ( 18.67979575497178502, 10.72451020669898547, 114.1655762719810383 ) ) ;
#23194=CARTESIAN_POINT ( 'NONE',  ( 5.153800228976335163, 19.02544592524342804, 64.79057627198100988 ) ) ;
#23195=CARTESIAN_POINT ( 'NONE',  ( 5.823673210054444382, -21.52544592524334988, 60.20942372801902565 ) ) ;
#23196=CARTESIAN_POINT ( 'NONE',  ( 9.564922557960805705, 16.46253265017160317, 104.5822429386476955 ) ) ;
#23198=EDGE_LOOP ( 'NONE', ( #178889, #79567, #165701, #74174 ) ) ;
#23199=CARTESIAN_POINT ( 'NONE',  ( 21.55341960407619695, -5.719274019375665929, 51.04275706135234714 ) ) ;
#23200=CARTESIAN_POINT ( 'NONE',  ( 16.46253265017160672, -9.564922557960803928, 23.33224293864769194 ) ) ;
#23201=CARTESIAN_POINT ( 'NONE',  ( 13.89961937509977652, -13.97604488694527269, 103.1239096053143527 ) ) ;
#23202=CARTESIAN_POINT ( 'NONE',  ( 16.51473224551083163, -9.474510206698727899, 50.83442372801899722 ) ) ;
#23203=CARTESIAN_POINT ( 'NONE',  ( -18.62759615963270932, 10.81492255796079327, 115.8322429386477097 ) ) ;
#23204=CARTESIAN_POINT ( 'NONE',  ( 19.02544592524334988, 5.153800228976608722, 41.45942372801900433 ) ) ;
#23205=CARTESIAN_POINT ( 'NONE',  ( -13.97604488694527625, -13.89961937509977652, 26.87390960531434558 ) ) ;
#23206=CARTESIAN_POINT ( 'NONE',  ( 16.53943276465976808, 0.05219959533934440121, 91.25109039468568994 ) ) ;
#23207=CARTESIAN_POINT ( 'NONE',  ( 5.049401038297881783, 19.05341960407617563, 62.29275706135234003 ) ) ;
#23208=CARTESIAN_POINT ( 'NONE',  ( 12.06949235617739724, 12.14591786802326823, 111.8760903946856615 ) ) ;
#23210=CARTESIAN_POINT ( 'NONE',  ( 16.51473224551069308, 9.474510206698969483, 89.16557627198103830 ) ) ;
#23211=CARTESIAN_POINT ( 'NONE',  ( 0.05219959533937995610, -21.53943276465977519, 90.00109039468567573 ) ) ;
#23212=CARTESIAN_POINT ( 'NONE',  ( 0.05219959533937995610, -21.53943276465977519, 100.0010903946857042 ) ) ;
#23214=CARTESIAN_POINT ( 'NONE',  ( -19.03943276465977164, 0.05219959533909376836, 106.2489096053143669 ) ) ;
#23215=CARTESIAN_POINT ( 'NONE',  ( 15.72974639402176855, 15.80617190586768217, 76.87609039468567573 ) ) ;
#23216=CARTESIAN_POINT ( 'NONE',  ( 16.55341960407618274, -4.379528057220086978, 21.04275706135234714 ) ) ;
#23217=CARTESIAN_POINT ( 'NONE',  ( 16.51473224551069308, 9.474510206698969483, 79.16557627198103830 ) ) ;
#23218=CARTESIAN_POINT ( 'NONE',  ( -10.72451020669898014, 18.67979575497178502, 30.41557627198101699 ) ) ;
#23219=CARTESIAN_POINT ( 'NONE',  ( -0.05219959533909027116, -19.03943276465977164, 97.49890960531436690 ) ) ;
#23220=CARTESIAN_POINT ( 'NONE',  ( -16.31925111598456724, -7.325300261831609205, 89.83575461032749843 ) ) ;
#23221=CARTESIAN_POINT ( 'NONE',  ( -9.564922557960796823, -16.46253265017161027, 82.08224293864768129 ) ) ;
#23222=CARTESIAN_POINT ( 'NONE',  ( -16.51473224551069308, -9.474510206698971260, 71.66557627198102409 ) ) ;
#23223=CARTESIAN_POINT ( 'NONE',  ( 12.14591786802327356, -12.06949235617739191, 100.6260903946857184 ) ) ;
#23225=CARTESIAN_POINT ( 'NONE',  ( -16.51473224551082808, 9.474510206698731452, 53.33442372801900433 ) ) ;
#23226=CARTESIAN_POINT ( 'NONE',  ( -0.05219959533909027116, -19.03943276465977164, 92.49890960531436690 ) ) ;
#23227=CARTESIAN_POINT ( 'NONE',  ( -16.53943276465976808, 0.05219959533911058130, 91.24890960531436690 ) ) ;
#23228=CARTESIAN_POINT ( 'NONE',  ( -15.80617190586745835, -15.72974639402198527, 36.87390960531435979 ) ) ;
#23229=CARTESIAN_POINT ( 'NONE',  ( 5.719274019375991003, -21.55341960407610458, 22.70724293864769194 ) ) ;
#23230=CARTESIAN_POINT ( 'NONE',  ( -12.14591786802309592, -12.06949235617757132, 86.87390960531438111 ) ) ;
#23231=CARTESIAN_POINT ( 'NONE',  ( -16.18388926212242396, 7.379444403734377822, 54.56046848633847191 ) ) ;
#23232=CARTESIAN_POINT ( 'NONE',  ( 0.05219959533936267826, -19.03943276465977164, 45.00109039468566863 ) ) ;
#23233=CARTESIAN_POINT ( 'NONE',  ( -8.224510206698735004, -14.34966873604973081, 99.58442372801900433 ) ) ;
#23234=CARTESIAN_POINT ( 'NONE',  ( -9.564922557960796823, -16.46253265017161027, 102.0822429386477097 ) ) ;
#23235=CARTESIAN_POINT ( 'NONE',  ( -5.719274019375665041, -21.55341960407619695, 64.79275706135234714 ) ) ;
#23236=CARTESIAN_POINT ( 'NONE',  ( 21.55341960407610458, 5.719274019375980345, 58.95724293864770971 ) ) ;
#23237=CARTESIAN_POINT ( 'NONE',  ( -10.81492255796105439, 18.62759615963255655, 27.91775706135234358 ) ) ;
#23238=CARTESIAN_POINT ( 'NONE',  ( 5.823673210054125526, 21.52544592524343514, 89.79057627198103830 ) ) ;
#23239=CARTESIAN_POINT ( 'NONE',  ( -10.72451020669870658, -18.67979575497194134, 34.58442372801900433 ) ) ;
#23240=CARTESIAN_POINT ( 'NONE',  ( 14.34966873604960469, 8.224510206698951720, 109.1655762719810383 ) ) ;
#23241=CARTESIAN_POINT ( 'NONE',  ( 19.02544592524334988, 5.153800228976608722, 66.45942372801899012 ) ) ;
#23242=CARTESIAN_POINT ( 'NONE',  ( -16.46253265017160317, 9.564922557960807481, 45.83224293864769550 ) ) ;
#23243=CARTESIAN_POINT ( 'NONE',  ( -8.314922557960811034, -14.29746914071050412, 97.08224293864770971 ) ) ;
#23244=CARTESIAN_POINT ( 'NONE',  ( -0.05219959533909027116, -19.03943276465977164, 102.4989096053143669 ) ) ;
#23245=CARTESIAN_POINT ( 'NONE',  ( 9.564922557960805705, 16.46253265017160317, 99.58224293864770971 ) ) ;
#23246=CARTESIAN_POINT ( 'NONE',  ( -4.379528057220328563, 16.55341960407611168, 115.2072429386476955 ) ) ;
#23247=CARTESIAN_POINT ( 'NONE',  ( 8.314922557960818139, 14.29746914071049879, 34.58224293864770260 ) ) ;
#23248=CARTESIAN_POINT ( 'NONE',  ( -12.06949235617739369, -12.14591786802326823, 104.3760903946856899 ) ) ;
#23249=CARTESIAN_POINT ( 'NONE',  ( -9.474510206698964154, 16.51473224551069663, 50.41557627198102409 ) ) ;
#23250=CARTESIAN_POINT ( 'NONE',  ( 0.05219959533909260263, 19.03943276465977164, 24.99890960531435269 ) ) ;
#23251=CARTESIAN_POINT ( 'NONE',  ( 16.51473224551083163, -9.474510206698727899, 20.83442372801899722 ) ) ;
#23252=CARTESIAN_POINT ( 'NONE',  ( -5.153800228976328057, -19.02544592524343514, 112.2905762719810099 ) ) ;
#23253=CARTESIAN_POINT ( 'NONE',  ( 14.34966873604960469, 8.224510206698951720, 29.16557627198103120 ) ) ;
#23254=CARTESIAN_POINT ( 'NONE',  ( -15.80617190586768217, 15.72974639402176855, 33.12609039468569705 ) ) ;
#23255=CARTESIAN_POINT ( 'NONE',  ( 16.51473224551069308, 9.474510206698969483, 99.16557627198102409 ) ) ;
#23256=CARTESIAN_POINT ( 'NONE',  ( 16.55341960407618274, -4.379528057220086978, 51.04275706135234714 ) ) ;
#23257=CARTESIAN_POINT ( 'NONE',  ( -16.53943276465976808, -0.05219959533934237506, 113.7510903946856757 ) ) ;
#23258=CARTESIAN_POINT ( 'NONE',  ( -0.05219959533934338120, 16.53943276465976808, 87.50109039468568994 ) ) ;
#23259=CARTESIAN_POINT ( 'NONE',  ( -8.224510206698735004, -14.34966873604973081, 29.58442372801901854 ) ) ;
#23260=CARTESIAN_POINT ( 'NONE',  ( -0.05219959533909027116, -19.03943276465977164, 52.49890960531436690 ) ) ;
#23261=CARTESIAN_POINT ( 'NONE',  ( -8.224510206698948167, 14.34966873604960824, 105.4155762719810383 ) ) ;
#23262=CARTESIAN_POINT ( 'NONE',  ( 0.05219959533907565091, 21.53943276465977519, 114.9989096053143669 ) ) ;
#23263=CARTESIAN_POINT ( 'NONE',  ( 19.02544592524343514, -5.153800228976328945, 38.54057627198103120 ) ) ;
#23264=CARTESIAN_POINT ( 'NONE',  ( -19.02544592524342804, 5.153800228976336051, 111.0405762719810099 ) ) ;
#23265=CARTESIAN_POINT ( 'NONE',  ( -19.03943276465977164, 0.05219959533909376836, 31.24890960531435979 ) ) ;
#23266=CARTESIAN_POINT ( 'NONE',  ( 13.97604488694527802, 13.89961937509977652, 99.37390960531436690 ) ) ;
#23268=CARTESIAN_POINT ( 'NONE',  ( -16.51473224551069308, -9.474510206698971260, 101.6655762719810241 ) ) ;
#23269=CARTESIAN_POINT ( 'NONE',  ( -15.72974639402176322, -15.80617190586768395, 44.37609039468567573 ) ) ;
#23270=CARTESIAN_POINT ( 'NONE',  ( -12.14591786802309592, -12.06949235617757132, 101.8739096053143811 ) ) ;
#23271=CARTESIAN_POINT ( 'NONE',  ( -19.05341960407611168, -5.049401038298163336, 111.4572429386476671 ) ) ;
#23272=CARTESIAN_POINT ( 'NONE',  ( -13.89961937509957401, -13.97604488694547697, 69.37609039468566152 ) ) ;
#23273=CARTESIAN_POINT ( 'NONE',  ( -14.34966873604972548, 8.224510206698743886, 58.33442372801901143 ) ) ;
#23274=CARTESIAN_POINT ( 'NONE',  ( 18.67979575497194134, -10.72451020669871369, 80.83442372801901854 ) ) ;
#23275=CARTESIAN_POINT ( 'NONE',  ( 8.224510206698742110, 14.34966873604972548, 47.08442372801901854 ) ) ;
#23276=CARTESIAN_POINT ( 'NONE',  ( -13.89961937509977652, 13.97604488694528158, 75.62390960531438111 ) ) ;
#23277=CARTESIAN_POINT ( 'NONE',  ( 13.97604488694548053, -13.89961937509957401, 110.6260903946856615 ) ) ;
#23278=CARTESIAN_POINT ( 'NONE',  ( 8.314922557961029526, -14.29746914071037800, 85.41775706135236135 ) ) ;
#23279=CARTESIAN_POINT ( 'NONE',  ( -9.474510206698720793, -16.51473224551083518, 99.58442372801900433 ) ) ;
#23280=CARTESIAN_POINT ( 'NONE',  ( 16.51473224551069308, 9.474510206698969483, 69.16557627198102409 ) ) ;
#23281=CARTESIAN_POINT ( 'NONE',  ( -10.72451020669898014, 18.67979575497178502, 95.41557627198102409 ) ) ;
#23282=CARTESIAN_POINT ( 'NONE',  ( -12.06949235617756955, 12.14591786802309770, 85.62390960531436690 ) ) ;
#23283=CARTESIAN_POINT ( 'NONE',  ( -5.049401038297874678, -19.05341960407617918, 84.79275706135233293 ) ) ;
#23284=CARTESIAN_POINT ( 'NONE',  ( -8.314922557961024197, 14.29746914071037800, 62.91775706135236135 ) ) ;
#23286=CARTESIAN_POINT ( 'NONE',  ( -19.02544592524334988, -5.153800228976617603, 68.95942372801896170 ) ) ;
#23287=CARTESIAN_POINT ( 'NONE',  ( -14.34966873604960291, -8.224510206698953496, 31.66557627198102054 ) ) ;
#23288=CARTESIAN_POINT ( 'NONE',  ( 4.483927247898545687, 16.52544592524342804, 74.79057627198105251 ) ) ;
#23289=CARTESIAN_POINT ( 'NONE',  ( -9.564922557961040184, 16.46253265017147172, 22.91775706135233648 ) ) ;
#23290=CARTESIAN_POINT ( 'NONE',  ( -16.81555441253465943, 7.025013491696270762, 40.63685445334211011 ) ) ;
#23291=CARTESIAN_POINT ( 'NONE',  ( -18.67979575497193778, 10.72451020669871902, 28.33442372801902209 ) ) ;
#23292=CARTESIAN_POINT ( 'NONE',  ( 19.03943276465977164, -0.05219959533909143690, 108.7489096053143527 ) ) ;
#23293=CARTESIAN_POINT ( 'NONE',  ( 0.05219959533909260263, 19.03943276465977164, 79.99890960531436690 ) ) ;
#23294=CARTESIAN_POINT ( 'NONE',  ( 10.72451020669871369, 18.67979575497193778, 97.08442372801904696 ) ) ;
#23295=CARTESIAN_POINT ( 'NONE',  ( 9.474510206698971260, -16.51473224551069308, 82.91557627198103830 ) ) ;
#23296=CARTESIAN_POINT ( 'NONE',  ( 5.823673210054125526, 21.52544592524343514, 44.79057627198103120 ) ) ;
#23297=CARTESIAN_POINT ( 'NONE',  ( -16.52544592524342804, 4.483927247898546575, 86.04057627198102409 ) ) ;
#23298=CARTESIAN_POINT ( 'NONE',  ( 13.89961937509977652, -13.97604488694527269, 63.12390960531435979 ) ) ;
#23299=CARTESIAN_POINT ( 'NONE',  ( 14.34966873604960469, 8.224510206698951720, 114.1655762719810383 ) ) ;
#23300=CARTESIAN_POINT ( 'NONE',  ( 18.62759615963255655, 10.81492255796105972, 31.66775706135234358 ) ) ;
#23301=CARTESIAN_POINT ( 'NONE',  ( 10.72451020669871369, 18.67979575497193778, 57.08442372801901854 ) ) ;
#23302=CARTESIAN_POINT ( 'NONE',  ( -9.474510206698964154, 16.51473224551069663, 50.41557627198102409 ) ) ;
#23303=CARTESIAN_POINT ( 'NONE',  ( -4.483927247898782831, 16.52544592524335698, 72.70942372801901854 ) ) ;
#23304=CARTESIAN_POINT ( 'NONE',  ( 21.55341960407610458, 5.719274019375980345, 108.9572429386476955 ) ) ;
#23305=CARTESIAN_POINT ( 'NONE',  ( -21.55341960407610458, -5.719274019375992779, 106.4572429386477097 ) ) ;
#23306=CARTESIAN_POINT ( 'NONE',  ( 9.474510206698729675, 16.51473224551082808, 37.08442372801899722 ) ) ;
#23307=CARTESIAN_POINT ( 'NONE',  ( -19.05341960407611168, -5.049401038298163336, 66.45724293864769550 ) ) ;
#23308=CARTESIAN_POINT ( 'NONE',  ( -9.564922557961040184, 16.46253265017147172, 37.91775706135233293 ) ) ;
#23309=CARTESIAN_POINT ( 'NONE',  ( -10.72451020669870658, -18.67979575497194134, 69.58442372801900433 ) ) ;
#23310=CARTESIAN_POINT ( 'NONE',  ( 21.53943276465977519, -0.05219959533907433946, 63.74890960531435979 ) ) ;
#23311=CARTESIAN_POINT ( 'NONE',  ( 16.53943276465976808, -0.05219959533910856209, 43.74890960531435979 ) ) ;
#23312=CARTESIAN_POINT ( 'NONE',  ( 5.719274019375673035, 21.55341960407619339, 92.29275706135236135 ) ) ;
#23313=CARTESIAN_POINT ( 'NONE',  ( -21.52544592524334988, -5.823673210054445271, 108.9594237280190185 ) ) ;
#23314=CARTESIAN_POINT ( 'NONE',  ( -14.29746914071049879, 8.314922557960819915, 60.83224293864769550 ) ) ;
#23315=CARTESIAN_POINT ( 'NONE',  ( -12.14591786802309592, -12.06949235617757132, 101.8739096053143811 ) ) ;
#23316=CARTESIAN_POINT ( 'NONE',  ( 9.564922557961047289, -16.46253265017146816, 55.41775706135234003 ) ) ;
#23317=CARTESIAN_POINT ( 'NONE',  ( 4.483927247898545687, 16.52544592524342804, 24.79057627198103120 ) ) ;
#23318=CARTESIAN_POINT ( 'NONE',  ( -15.80617190586768217, 15.72974639402176855, 68.12609039468567573 ) ) ;
#23319=CARTESIAN_POINT ( 'NONE',  ( -13.97604488694527625, -13.89961937509977652, 71.87390960531433848 ) ) ;
#23320=CARTESIAN_POINT ( 'NONE',  ( -13.89961937509957401, -13.97604488694547875, 54.37609039468565442 ) ) ;
#23321=CARTESIAN_POINT ( 'NONE',  ( -15.72974639402197994, 15.80617190586746368, 55.62390960531436690 ) ) ;
#23322=CARTESIAN_POINT ( 'NONE',  ( 15.80617190586769283, -15.72974639402175789, 45.62609039468567573 ) ) ;
#23323=CARTESIAN_POINT ( 'NONE',  ( -18.62759615963270932, 10.81492255796079327, 100.8322429386477097 ) ) ;
#23324=CARTESIAN_POINT ( 'NONE',  ( 13.89961937509957401, 13.97604488694547697, 96.87609039468566152 ) ) ;
#23325=CARTESIAN_POINT ( 'NONE',  ( -8.314922557961024197, 14.29746914071037800, 62.91775706135236135 ) ) ;
#23327=CARTESIAN_POINT ( 'NONE',  ( -18.67979575497178146, -10.72451020669898902, 111.6655762719810525 ) ) ;
#23328=CARTESIAN_POINT ( 'NONE',  ( 16.53943276465976808, -0.05219959533910856209, 93.74890960531436690 ) ) ;
#23329=CARTESIAN_POINT ( 'NONE',  ( -17.49999999999997868, -5.076555817581236418, 31.17951492049776263 ) ) ;
#23330=CARTESIAN_POINT ( 'NONE',  ( -19.03943276465977164, -0.05219959533935918106, 113.7510903946856757 ) ) ;
#23331=CARTESIAN_POINT ( 'NONE',  ( -15.72974639402197994, 15.80617190586746368, 50.62390960531435979 ) ) ;
#23332=CARTESIAN_POINT ( 'NONE',  ( 4.379528057220092307, 16.55341960407617563, 87.29275706135236135 ) ) ;
#23334=CARTESIAN_POINT ( 'NONE',  ( 12.06949235617739724, 12.14591786802326823, 66.87609039468568994 ) ) ;
#23335=CARTESIAN_POINT ( 'NONE',  ( -15.80617190586768217, 15.72974639402176855, 23.12609039468567573 ) ) ;
#23336=CARTESIAN_POINT ( 'NONE',  ( -5.719274019375978568, 21.55341960407610458, 45.20724293864769550 ) ) ;
#23337=CARTESIAN_POINT ( 'NONE',  ( 12.14591786802327356, -12.06949235617739191, 85.62609039468568994 ) ) ;
#23338=CARTESIAN_POINT ( 'NONE',  ( -5.153800228976328057, -19.02544592524343514, 102.2905762719810383 ) ) ;
#23339=CARTESIAN_POINT ( 'NONE',  ( -10.72451020669870658, -18.67979575497194134, 64.58442372801900433 ) ) ;
#23340=CARTESIAN_POINT ( 'NONE',  ( -21.55341960407610458, -5.719274019375992779, 46.45724293864769550 ) ) ;
#23341=CARTESIAN_POINT ( 'NONE',  ( -18.67979575497178146, -10.72451020669898902, 31.66557627198102054 ) ) ;
#23343=CARTESIAN_POINT ( 'NONE',  ( 16.51473224551083163, -9.474510206698727899, 55.83442372801899722 ) ) ;
#23344=CARTESIAN_POINT ( 'NONE',  ( 16.55341960407618274, -4.379528057220086978, 66.04275706135236135 ) ) ;
#23345=CARTESIAN_POINT ( 'NONE',  ( 21.55341960407610458, 5.719274019375980345, 28.95724293864769905 ) ) ;
#23347=CARTESIAN_POINT ( 'NONE',  ( 13.97604488694527802, 13.89961937509977652, 84.37390960531433848 ) ) ;
#23348=CARTESIAN_POINT ( 'NONE',  ( 12.14591786802309770, 12.06949235617756955, 24.37390960531435979 ) ) ;
#23349=CARTESIAN_POINT ( 'NONE',  ( -17.60728821186566151, 5.500000000000029310, 85.86690927743002533 ) ) ;
#23350=CARTESIAN_POINT ( 'NONE',  ( -16.53943276465976808, 0.05219959533911058130, 106.2489096053143811 ) ) ;
#23351=CARTESIAN_POINT ( 'NONE',  ( 21.55341960407610458, 5.719274019375980345, 43.95724293864769550 ) ) ;
#23352=CARTESIAN_POINT ( 'NONE',  ( -9.564922557960796823, -16.46253265017161027, 47.08224293864769550 ) ) ;
#23353=CARTESIAN_POINT ( 'NONE',  ( 4.483927247898790824, -16.52544592524335698, 75.20942372801901854 ) ) ;
#23354=CARTESIAN_POINT ( 'NONE',  ( -21.52544592524334988, -5.823673210054445271, 38.95942372801901854 ) ) ;
#23355=CARTESIAN_POINT ( 'NONE',  ( 19.03943276465977164, 0.05219959533936151252, 91.25109039468566152 ) ) ;
#23356=CARTESIAN_POINT ( 'NONE',  ( -4.379528057220328563, 16.55341960407611168, 85.20724293864770971 ) ) ;
#23357=CARTESIAN_POINT ( 'NONE',  ( 13.97604488694527802, 13.89961937509977652, 54.37390960531435979 ) ) ;
#23358=CARTESIAN_POINT ( 'NONE',  ( -13.97604488694527625, -13.89961937509977652, 26.87390960531434558 ) ) ;
#23359=CARTESIAN_POINT ( 'NONE',  ( -15.72974639402176322, -15.80617190586768395, 109.3760903946857042 ) ) ;
#23360=CARTESIAN_POINT ( 'NONE',  ( 16.51473224551069308, 9.474510206698969483, 79.16557627198103830 ) ) ;
#23361=CARTESIAN_POINT ( 'NONE',  ( -12.14591786802326823, 12.06949235617739902, 63.12609039468568994 ) ) ;
#23362=CARTESIAN_POINT ( 'NONE',  ( 0.05219959533937995610, -21.53943276465977519, 90.00109039468567573 ) ) ;
#23363=CARTESIAN_POINT ( 'NONE',  ( 5.823673210054125526, 21.52544592524343514, 49.79057627198102409 ) ) ;
#23364=CARTESIAN_POINT ( 'NONE',  ( -14.29746914071037622, -8.314922557961029526, 79.16775706135234714 ) ) ;
#23365=CARTESIAN_POINT ( 'NONE',  ( -9.474510206698720793, -16.51473224551083518, 49.58442372801899722 ) ) ;
#23366=CARTESIAN_POINT ( 'NONE',  ( -13.89961937509957401, -13.97604488694547875, 69.37609039468564731 ) ) ;
#23368=CARTESIAN_POINT ( 'NONE',  ( 18.67979575497194134, -10.72451020669871369, 65.83442372801900433 ) ) ;
#23369=CARTESIAN_POINT ( 'NONE',  ( -16.51473224551069308, -9.474510206698971260, 71.66557627198102409 ) ) ;
#23370=CARTESIAN_POINT ( 'NONE',  ( 19.03943276465977164, -0.05219959533909143690, 33.74890960531435979 ) ) ;
#23371=CARTESIAN_POINT ( 'NONE',  ( -5.153800228976607833, 19.02544592524334988, 62.70942372801899722 ) ) ;
#23372=CARTESIAN_POINT ( 'NONE',  ( -9.564922557960796823, -16.46253265017161027, 107.0822429386476955 ) ) ;
#23373=CARTESIAN_POINT ( 'NONE',  ( -9.474510206698964154, 16.51473224551069663, 90.41557627198103830 ) ) ;
#23374=CARTESIAN_POINT ( 'NONE',  ( 12.06949235617757843, -12.14591786802309237, 48.12390960531436690 ) ) ;
#23375=CARTESIAN_POINT ( 'NONE',  ( 10.72451020669898902, -18.67979575497178502, 52.91557627198103830 ) ) ;
#23377=CARTESIAN_POINT ( 'NONE',  ( -15.72974639402176322, -15.80617190586768395, 109.3760903946857042 ) ) ;
#23378=CARTESIAN_POINT ( 'NONE',  ( -16.88567814943162659, -6.947325034625696283, 81.29001122652589117 ) ) ;
#23379=CARTESIAN_POINT ( 'NONE',  ( -19.03943276465977164, 0.05219959533909376836, 46.24890960531435979 ) ) ;
#23382=CARTESIAN_POINT ( 'NONE',  ( -14.34966873604972548, 8.224510206698743886, 68.33442372801900433 ) ) ;
#23383=CARTESIAN_POINT ( 'NONE',  ( -10.81492255796078084, -18.62759615963271287, 77.08224293864769550 ) ) ;
#23384=ADVANCED_FACE ( 'NONE', ( #84843 ), #87142, .T. ) ;
#23385=CARTESIAN_POINT ( 'NONE',  ( -12.14591786802309592, -12.06949235617757132, 46.87390960531435979 ) ) ;
#23386=CARTESIAN_POINT ( 'NONE',  ( -13.97604488694527625, -13.89961937509977652, 41.87390960531435979 ) ) ;
#23388=CARTESIAN_POINT ( 'NONE',  ( -18.62759615963255300, -10.81492255796106328, 39.16775706135235424 ) ) ;
#23389=CARTESIAN_POINT ( 'NONE',  ( -5.153800228976607833, 19.02544592524334988, 52.70942372801900433 ) ) ;
#23390=CARTESIAN_POINT ( 'NONE',  ( 19.05341960407611168, 5.049401038298154454, 33.95724293864769550 ) ) ;
#23391=CARTESIAN_POINT ( 'NONE',  ( 10.81492255796106328, -18.62759615963255655, 100.4177570613523471 ) ) ;
#23393=CARTESIAN_POINT ( 'NONE',  ( -4.483927247898539470, -16.52544592524342804, 37.29057627198102409 ) ) ;
#23395=CARTESIAN_POINT ( 'NONE',  ( 0.05219959533907565091, 21.53943276465977519, 34.99890960531435979 ) ) ;
#23396=CARTESIAN_POINT ( 'NONE',  ( 19.03943276465977164, -0.05219959533909143690, 83.74890960531436690 ) ) ;
#23397=CARTESIAN_POINT ( 'NONE',  ( 14.29746914071049879, -8.314922557960816363, 83.33224293864769550 ) ) ;
#23398=CARTESIAN_POINT ( 'NONE',  ( -0.05219959533934338120, 16.53943276465976808, 22.50109039468567573 ) ) ;
#23399=CARTESIAN_POINT ( 'NONE',  ( 14.34966873604972726, -8.224510206698740333, 110.8344237280190043 ) ) ;
#23401=CARTESIAN_POINT ( 'NONE',  ( 19.02544592524343514, -5.153800228976328945, 48.54057627198103120 ) ) ;
#23402=CARTESIAN_POINT ( 'NONE',  ( 16.46253265017160672, -9.564922557960803928, 98.33224293864769550 ) ) ;
#23403=CARTESIAN_POINT ( 'NONE',  ( 0.05219959533907565091, 21.53943276465977519, 84.99890960531436690 ) ) ;
#23404=CARTESIAN_POINT ( 'NONE',  ( 12.14591786802309770, 12.06949235617756955, 24.37390960531435979 ) ) ;
#23405=CARTESIAN_POINT ( 'NONE',  ( 13.97604488694527802, 13.89961937509977652, 104.3739096053143385 ) ) ;
#23406=CARTESIAN_POINT ( 'NONE',  ( 13.97604488694548053, -13.89961937509957401, 75.62609039468564731 ) ) ;
#23407=CARTESIAN_POINT ( 'NONE',  ( 10.81492255796106328, -18.62759615963255655, 105.4177570613523613 ) ) ;
#23408=CARTESIAN_POINT ( 'NONE',  ( 18.67979575497178502, 10.72451020669898547, 89.16557627198102409 ) ) ;
#23409=CARTESIAN_POINT ( 'NONE',  ( 0.05219959533907565091, 21.53943276465977519, 34.99890960531435979 ) ) ;
#23410=CARTESIAN_POINT ( 'NONE',  ( -5.153800228976328057, -19.02544592524343514, 62.29057627198100988 ) ) ;
#23411=CARTESIAN_POINT ( 'NONE',  ( -4.379528057220328563, 16.55341960407611168, 35.20724293864768839 ) ) ;
#23412=CARTESIAN_POINT ( 'NONE',  ( 19.05341960407611168, 5.049401038298154454, 83.95724293864766707 ) ) ;
#23415=CARTESIAN_POINT ( 'NONE',  ( -5.153800228976607833, 19.02544592524334988, 22.70942372801899012 ) ) ;
#23416=CARTESIAN_POINT ( 'NONE',  ( 16.53943276465976808, -0.05219959533910856209, 83.74890960531435269 ) ) ;
#23417=CARTESIAN_POINT ( 'NONE',  ( 18.67979575497194134, -10.72451020669871369, 25.83442372801901499 ) ) ;
#23419=CARTESIAN_POINT ( 'NONE',  ( 15.80617190586746368, 15.72974639402197994, 69.37390960531436690 ) ) ;
#23420=CARTESIAN_POINT ( 'NONE',  ( -12.06949235617739369, -12.14591786802326823, 89.37609039468568994 ) ) ;
#23421=CARTESIAN_POINT ( 'NONE',  ( 19.05341960407611168, 5.049401038298154454, 23.95724293864769194 ) ) ;
#23422=CARTESIAN_POINT ( 'NONE',  ( -0.05219959533909027116, -19.03943276465977164, 67.49890960531436690 ) ) ;
#23424=CARTESIAN_POINT ( 'NONE',  ( 13.89961937509977652, -13.97604488694527269, 23.12390960531436335 ) ) ;
#23425=CARTESIAN_POINT ( 'NONE',  ( -8.224510206698948167, 14.34966873604960824, 35.41557627198102409 ) ) ;
#23426=CARTESIAN_POINT ( 'NONE',  ( -21.55341960407619339, 5.719274019375674811, 58.54275706135235424 ) ) ;
#23428=CARTESIAN_POINT ( 'NONE',  ( -10.81492255796105439, 18.62759615963255655, 92.91775706135236135 ) ) ;
#23429=CARTESIAN_POINT ( 'NONE',  ( -9.564922557960796823, -16.46253265017161027, 42.08224293864769550 ) ) ;
#23430=CARTESIAN_POINT ( 'NONE',  ( 19.05341960407611168, 5.049401038298154454, 48.95724293864768129 ) ) ;
#23432=CARTESIAN_POINT ( 'NONE',  ( -21.55341960407619339, 5.719274019375674811, 88.54275706135236135 ) ) ;
#23433=CARTESIAN_POINT ( 'NONE',  ( 8.224510206698742110, 14.34966873604972548, 62.08442372801901143 ) ) ;
#23434=CARTESIAN_POINT ( 'NONE',  ( -5.719274019375665041, -21.55341960407619695, 79.79275706135236135 ) ) ;
#23435=CARTESIAN_POINT ( 'NONE',  ( 5.719274019375991003, -21.55341960407610458, 27.70724293864769905 ) ) ;
#23436=CARTESIAN_POINT ( 'NONE',  ( 5.049401038297881783, 19.05341960407617563, 97.29275706135233293 ) ) ;
#23437=CARTESIAN_POINT ( 'NONE',  ( -15.80617190586768217, 15.72974639402176855, 58.12609039468568994 ) ) ;
#23438=CARTESIAN_POINT ( 'NONE',  ( -4.379528057220086978, -16.55341960407618274, 34.79275706135235424 ) ) ;
#23439=CARTESIAN_POINT ( 'NONE',  ( 10.72451020669898902, -18.67979575497178502, 87.91557627198103830 ) ) ;
#23440=CARTESIAN_POINT ( 'NONE',  ( -16.46253265017146816, -9.564922557961047289, 84.16775706135233293 ) ) ;
#23441=CARTESIAN_POINT ( 'NONE',  ( 16.51473224551069308, 9.474510206698969483, 69.16557627198102409 ) ) ;
#23442=CARTESIAN_POINT ( 'NONE',  ( -9.474510206698720793, -16.51473224551083518, 99.58442372801900433 ) ) ;
#23443=CARTESIAN_POINT ( 'NONE',  ( -13.97604488694547697, 13.89961937509957934, 108.1260903946856331 ) ) ;
#23444=CARTESIAN_POINT ( 'NONE',  ( -12.14591786802309592, -12.06949235617757132, 46.87390960531435979 ) ) ;
#23445=CARTESIAN_POINT ( 'NONE',  ( -0.05219959533936034679, 19.03943276465977164, 72.50109039468566152 ) ) ;
#23446=CARTESIAN_POINT ( 'NONE',  ( -12.06949235617739369, -12.14591786802326823, 59.37609039468568284 ) ) ;
#23447=CARTESIAN_POINT ( 'NONE',  ( 19.02544592524334988, 5.153800228976608722, 41.45942372801900433 ) ) ;
#23448=CARTESIAN_POINT ( 'NONE',  ( 19.05341960407611168, 5.049401038298154454, 43.95724293864769550 ) ) ;
#23449=CARTESIAN_POINT ( 'NONE',  ( 16.51473224551069308, 9.474510206698969483, 59.16557627198102409 ) ) ;
#23450=CARTESIAN_POINT ( 'NONE',  ( -4.379528057220086978, -16.55341960407618274, 59.79275706135234714 ) ) ;
#23453=CARTESIAN_POINT ( 'NONE',  ( 19.05341960407611168, 5.049401038298154454, 103.9572429386476671 ) ) ;
#23456=CARTESIAN_POINT ( 'NONE',  ( -0.05219959533936034679, 19.03943276465977164, 102.5010903946856757 ) ) ;
#23457=CARTESIAN_POINT ( 'NONE',  ( 18.62759615963271287, -10.81492255796078972, 33.33224293864769550 ) ) ;
#23458=CARTESIAN_POINT ( 'NONE',  ( -16.46253265017146816, -9.564922557961047289, 34.16775706135233293 ) ) ;
#23459=CARTESIAN_POINT ( 'NONE',  ( -8.224510206698735004, -14.34966873604973081, 19.58442372801901143 ) ) ;
#23460=CARTESIAN_POINT ( 'NONE',  ( 5.153800228976335163, 19.02544592524342804, 24.79057627198102765 ) ) ;
#23461=CARTESIAN_POINT ( 'NONE',  ( -9.564922557960796823, -16.46253265017161027, 52.08224293864768839 ) ) ;
#23462=CARTESIAN_POINT ( 'NONE',  ( 10.72451020669898902, -18.67979575497178502, 67.91557627198102409 ) ) ;
#23463=CARTESIAN_POINT ( 'NONE',  ( 5.153800228976335163, 19.02544592524342804, 104.7905762719809957 ) ) ;
#23464=CARTESIAN_POINT ( 'NONE',  ( 5.153800228976335163, 19.02544592524342804, 34.79057627198102409 ) ) ;
#23466=CARTESIAN_POINT ( 'NONE',  ( 16.46253265017146816, 9.564922557961045513, 86.66775706135233293 ) ) ;
#23467=CARTESIAN_POINT ( 'NONE',  ( 16.52544592524342804, -4.483927247898539470, 63.54057627198103830 ) ) ;
#23468=CARTESIAN_POINT ( 'NONE',  ( 18.62759615963271287, -10.81492255796078972, 48.33224293864770260 ) ) ;
#23469=CARTESIAN_POINT ( 'NONE',  ( 5.719274019375673035, 21.55341960407619339, 107.2927570613523471 ) ) ;
#23470=CARTESIAN_POINT ( 'NONE',  ( 10.72451020669898902, -18.67979575497178502, 102.9155762719810383 ) ) ;
#23471=CARTESIAN_POINT ( 'NONE',  ( -0.05219959533937732626, 21.53943276465977519, 67.50109039468568994 ) ) ;
#23472=CARTESIAN_POINT ( 'NONE',  ( -15.80617190586768217, 15.72974639402176855, 83.12609039468568994 ) ) ;
#23473=CARTESIAN_POINT ( 'NONE',  ( 5.049401038298161559, -19.05341960407611168, 107.7072429386476955 ) ) ;
#23474=CARTESIAN_POINT ( 'NONE',  ( 4.379528057220092307, 16.55341960407617563, 107.2927570613523471 ) ) ;
#23475=CARTESIAN_POINT ( 'NONE',  ( -15.72974639402176322, -15.80617190586768395, 74.37609039468568994 ) ) ;
#23476=CARTESIAN_POINT ( 'NONE',  ( -19.05341960407611168, -5.049401038298163336, 71.45724293864766707 ) ) ;
#23477=CARTESIAN_POINT ( 'NONE',  ( 19.05341960407617918, -5.049401038297876454, 31.04275706135232227 ) ) ;
#23478=CARTESIAN_POINT ( 'NONE',  ( 18.62759615963255655, 10.81492255796105972, 26.66775706135235424 ) ) ;
#23479=CARTESIAN_POINT ( 'NONE',  ( 5.153800228976335163, 19.02544592524342804, 69.79057627198103830 ) ) ;
#23480=CARTESIAN_POINT ( 'NONE',  ( -16.52544592524342804, 4.483927247898546575, 81.04057627198102409 ) ) ;
#23481=CARTESIAN_POINT ( 'NONE',  ( 8.314922557960818139, 14.29746914071049879, 44.58224293864769550 ) ) ;
#23482=CARTESIAN_POINT ( 'NONE',  ( 18.62759615963271287, -10.81492255796078972, 53.33224293864769550 ) ) ;
#23483=CARTESIAN_POINT ( 'NONE',  ( 16.46253265017160672, -9.564922557960803928, 63.33224293864769550 ) ) ;
#23484=CARTESIAN_POINT ( 'NONE',  ( 10.81492255796078972, 18.62759615963270932, 69.58224293864769550 ) ) ;
#23485=CARTESIAN_POINT ( 'NONE',  ( -5.153800228976607833, 19.02544592524334988, 67.70942372801900433 ) ) ;
#23487=CARTESIAN_POINT ( 'NONE',  ( -8.314922557960811034, -14.29746914071050412, 62.08224293864769550 ) ) ;
#23488=CARTESIAN_POINT ( 'NONE',  ( 5.719274019375991003, -21.55341960407610458, 42.70724293864770260 ) ) ;
#23490=CARTESIAN_POINT ( 'NONE',  ( 17.50000000000000000, 5.622605283950862010, 103.8120731059611046 ) ) ;
#23491=CARTESIAN_POINT ( 'NONE',  ( 8.314922557961029526, -14.29746914071037800, 90.41775706135236135 ) ) ;
#23493=CARTESIAN_POINT ( 'NONE',  ( -9.564922557961040184, 16.46253265017147172, 82.91775706135233293 ) ) ;
#23494=CARTESIAN_POINT ( 'NONE',  ( -8.224510206698948167, 14.34966873604960824, 50.41557627198103120 ) ) ;
#23496=CARTESIAN_POINT ( 'NONE',  ( -0.05219959533909027116, -19.03943276465977164, 52.49890960531436690 ) ) ;
#23497=CARTESIAN_POINT ( 'NONE',  ( 8.314922557960818139, 14.29746914071049879, 34.58224293864770260 ) ) ;
#23498=CARTESIAN_POINT ( 'NONE',  ( -16.51473224551069308, -9.474510206698971260, 81.66557627198103830 ) ) ;
#23499=CARTESIAN_POINT ( 'NONE',  ( -13.97604488694547697, 13.89961937509957934, 78.12609039468567573 ) ) ;
#23500=CARTESIAN_POINT ( 'NONE',  ( 13.89961937509977652, -13.97604488694527269, 53.12390960531434558 ) ) ;
#23501=CARTESIAN_POINT ( 'NONE',  ( 5.719274019375673035, 21.55341960407619339, 62.29275706135236845 ) ) ;
#23502=CARTESIAN_POINT ( 'NONE',  ( -19.05341960407611168, -5.049401038298163336, 71.45724293864766707 ) ) ;
#23503=CARTESIAN_POINT ( 'NONE',  ( -19.05341960407611168, -5.049401038298163336, 21.45724293864768839 ) ) ;
#23504=CARTESIAN_POINT ( 'NONE',  ( 16.51473224551069308, 9.474510206698969483, 79.16557627198103830 ) ) ;
#23505=CARTESIAN_POINT ( 'NONE',  ( 21.55341960407610458, 5.719274019375980345, 53.95724293864770260 ) ) ;
#23506=CARTESIAN_POINT ( 'NONE',  ( -13.89961937509977652, 13.97604488694528158, 45.62390960531433848 ) ) ;
#23507=CARTESIAN_POINT ( 'NONE',  ( -21.53943276465977519, 0.05219959533907696930, 56.24890960531436690 ) ) ;
#23508=CARTESIAN_POINT ( 'NONE',  ( 13.89961937509957401, 13.97604488694547697, 86.87609039468567573 ) ) ;
#23509=CARTESIAN_POINT ( 'NONE',  ( 4.483927247898790824, -16.52544592524335698, 100.2094237280190043 ) ) ;
#23511=CARTESIAN_POINT ( 'NONE',  ( 19.05341960407617918, -5.049401038297876454, 41.04275706135233293 ) ) ;
#23512=CARTESIAN_POINT ( 'NONE',  ( 0.05219959533934541429, -16.53943276465976808, 55.00109039468568284 ) ) ;
#23513=CARTESIAN_POINT ( 'NONE',  ( 8.314922557961029526, -14.29746914071037800, 80.41775706135234714 ) ) ;
#23515=CARTESIAN_POINT ( 'NONE',  ( 12.14591786802327356, -12.06949235617739191, 70.62609039468567573 ) ) ;
#23516=CARTESIAN_POINT ( 'NONE',  ( -15.80617190586745835, -15.72974639402198527, 21.87390960531436690 ) ) ;
#23517=CARTESIAN_POINT ( 'NONE',  ( -0.05219959533909027116, -19.03943276465977164, 37.49890960531436690 ) ) ;
#23518=CARTESIAN_POINT ( 'NONE',  ( 16.52544592524335698, 4.483927247898782831, 31.45942372801901854 ) ) ;
#23519=CARTESIAN_POINT ( 'NONE',  ( 16.46253265017160672, -9.564922557960803928, 53.33224293864768839 ) ) ;
#23520=CARTESIAN_POINT ( 'NONE',  ( -21.55341960407619339, 5.719274019375674811, 43.54275706135235424 ) ) ;
#23521=CARTESIAN_POINT ( 'NONE',  ( 12.14591786802327356, -12.06949235617739191, 35.62609039468568994 ) ) ;
#23522=CARTESIAN_POINT ( 'NONE',  ( -16.55341960407611168, -4.379528057220339221, 21.45724293864769550 ) ) ;
#23524=CARTESIAN_POINT ( 'NONE',  ( 0.05219959533936267826, -19.03943276465977164, 20.00109039468567218 ) ) ;
#23525=CARTESIAN_POINT ( 'NONE',  ( 19.02544592524334988, 5.153800228976608722, 111.4594237280190043 ) ) ;
#23526=CARTESIAN_POINT ( 'NONE',  ( 16.46253265017146816, 9.564922557961045513, 66.66775706135233293 ) ) ;
#23527=CARTESIAN_POINT ( 'NONE',  ( 4.379528057220339221, -16.55341960407611168, 72.70724293864769550 ) ) ;
#23528=CARTESIAN_POINT ( 'NONE',  ( -16.46253265017160317, 9.564922557960807481, 35.83224293864768839 ) ) ;
#23529=CARTESIAN_POINT ( 'NONE',  ( -5.153800228976607833, 19.02544592524334988, 72.70942372801900433 ) ) ;
#23530=CARTESIAN_POINT ( 'NONE',  ( 16.31925111598407696, -7.325300261831841020, 57.66424538967171998 ) ) ;
#23531=CARTESIAN_POINT ( 'NONE',  ( -5.823673210054431948, 21.52544592524334988, 67.70942372801901854 ) ) ;
#23532=CARTESIAN_POINT ( 'NONE',  ( -0.05219959533934338120, 16.53943276465976808, 42.50109039468567573 ) ) ;
#23534=CARTESIAN_POINT ( 'NONE',  ( -16.51473224551069308, -9.474510206698971260, 111.6655762719810383 ) ) ;
#23535=CARTESIAN_POINT ( 'NONE',  ( 14.34966873604972726, -8.224510206698740333, 20.83442372801901143 ) ) ;
#23536=CARTESIAN_POINT ( 'NONE',  ( 9.474510206698971260, -16.51473224551069308, 112.9155762719810383 ) ) ;
#23538=CARTESIAN_POINT ( 'NONE',  ( -9.474510206698964154, 16.51473224551069663, 30.41557627198102054 ) ) ;
#23539=CARTESIAN_POINT ( 'NONE',  ( 5.719274019375673035, 21.55341960407619339, 107.2927570613523471 ) ) ;
#23540=CARTESIAN_POINT ( 'NONE',  ( 5.049401038298161559, -19.05341960407611168, 62.70724293864769550 ) ) ;
#23541=CARTESIAN_POINT ( 'NONE',  ( 21.55341960407619695, -5.719274019375665929, 71.04275706135234714 ) ) ;
#23542=CARTESIAN_POINT ( 'NONE',  ( 21.55341960407619695, -5.719274019375665929, 101.0427570613523756 ) ) ;
#23543=CARTESIAN_POINT ( 'NONE',  ( 14.29746914071037800, 8.314922557961029526, 111.6677570613523613 ) ) ;
#23544=CARTESIAN_POINT ( 'NONE',  ( -16.51473224551069308, -9.474510206698971260, 26.66557627198103120 ) ) ;
#23545=CARTESIAN_POINT ( 'NONE',  ( 13.89961937509977652, -13.97604488694527269, 98.12390960531433848 ) ) ;
#23546=CARTESIAN_POINT ( 'NONE',  ( -5.823673210054431948, 21.52544592524334988, 62.70942372801902565 ) ) ;
#23547=CARTESIAN_POINT ( 'NONE',  ( -19.02544592524342804, 5.153800228976336051, 31.04057627198102409 ) ) ;
#23548=CARTESIAN_POINT ( 'NONE',  ( -0.05219959533937732626, 21.53943276465977519, 52.50109039468567573 ) ) ;
#23549=CARTESIAN_POINT ( 'NONE',  ( 0.05219959533936267826, -19.03943276465977164, 85.00109039468567573 ) ) ;
#23550=CARTESIAN_POINT ( 'NONE',  ( -19.05341960407611168, -5.049401038298163336, 106.4572429386476955 ) ) ;
#23551=CARTESIAN_POINT ( 'NONE',  ( 5.049401038298161559, -19.05341960407611168, 27.70724293864769550 ) ) ;
#23552=CARTESIAN_POINT ( 'NONE',  ( 15.72974639402199770, -15.80617190586745480, 108.1239096053143811 ) ) ;
#23553=CARTESIAN_POINT ( 'NONE',  ( 13.89961937509957401, 13.97604488694547697, 36.87609039468565442 ) ) ;
#23554=CARTESIAN_POINT ( 'NONE',  ( -8.314922557960811034, -14.29746914071050412, 107.0822429386476955 ) ) ;
#23555=CARTESIAN_POINT ( 'NONE',  ( -0.05219959533909027116, -19.03943276465977164, 52.49890960531436690 ) ) ;
#23556=CARTESIAN_POINT ( 'NONE',  ( 19.03943276465977164, 0.05219959533936151252, 101.2510903946856757 ) ) ;
#23557=CARTESIAN_POINT ( 'NONE',  ( -14.34966873604960291, -8.224510206698953496, 56.66557627198103830 ) ) ;
#23558=CARTESIAN_POINT ( 'NONE',  ( 21.53943276465977519, 0.05219959533937863772, 106.2510903946856757 ) ) ;
#23559=CARTESIAN_POINT ( 'NONE',  ( 19.05341960407611168, 5.049401038298154454, 113.9572429386477097 ) ) ;
#23560=CARTESIAN_POINT ( 'NONE',  ( -9.474510206698720793, -16.51473224551083518, 84.58442372801900433 ) ) ;
#23561=CARTESIAN_POINT ( 'NONE',  ( 5.719274019375991003, -21.55341960407610458, 92.70724293864770971 ) ) ;
#23562=CARTESIAN_POINT ( 'NONE',  ( 18.67979575497194134, -10.72451020669871369, 45.83442372801901854 ) ) ;
#23563=CARTESIAN_POINT ( 'NONE',  ( -8.224510206698735004, -14.34966873604973081, 39.58442372801901143 ) ) ;
#23564=CARTESIAN_POINT ( 'NONE',  ( 16.53943276465976808, 0.05219959533934440121, 101.2510903946856757 ) ) ;
#23565=CARTESIAN_POINT ( 'NONE',  ( -4.483927247898782831, 16.52544592524335698, 47.70942372801902565 ) ) ;
#23566=CARTESIAN_POINT ( 'NONE',  ( -18.67979575497193778, 10.72451020669871902, 53.33442372801901854 ) ) ;
#23567=CARTESIAN_POINT ( 'NONE',  ( -21.55341960407610458, -5.719274019375992779, 41.45724293864769550 ) ) ;
#23568=CARTESIAN_POINT ( 'NONE',  ( -5.049401038298153566, 19.05341960407611168, 35.20724293864768839 ) ) ;
#23570=CARTESIAN_POINT ( 'NONE',  ( -16.52544592524335698, -4.483927247898792601, 68.95942372801901854 ) ) ;
#23571=CARTESIAN_POINT ( 'NONE',  ( -21.53943276465977519, 0.05219959533907696930, 91.24890960531436690 ) ) ;
#23572=CARTESIAN_POINT ( 'NONE',  ( -0.05219959533910754901, -16.53943276465976808, 37.49890960531436690 ) ) ;
#23573=CARTESIAN_POINT ( 'NONE',  ( -0.05219959533934338120, 16.53943276465976808, 67.50109039468568994 ) ) ;
#23574=CARTESIAN_POINT ( 'NONE',  ( -9.564922557960796823, -16.46253265017161027, 52.08224293864768839 ) ) ;
#23575=CARTESIAN_POINT ( 'NONE',  ( 19.05341960407617918, -5.049401038297876454, 106.0427570613523471 ) ) ;
#23576=CARTESIAN_POINT ( 'NONE',  ( 18.62759615963271287, -10.81492255796078972, 83.33224293864769550 ) ) ;
#23577=CARTESIAN_POINT ( 'NONE',  ( -4.379528057220328563, 16.55341960407611168, 35.20724293864768839 ) ) ;
#23579=CARTESIAN_POINT ( 'NONE',  ( 12.14591786802327356, -12.06949235617739191, 80.62609039468567573 ) ) ;
#23581=CARTESIAN_POINT ( 'NONE',  ( 21.55341960407610458, 5.719274019375980345, 68.95724293864769550 ) ) ;
#23583=CARTESIAN_POINT ( 'NONE',  ( 14.29746914071037800, 8.314922557961029526, 106.6677570613523756 ) ) ;
#23586=CARTESIAN_POINT ( 'NONE',  ( 10.72451020669898902, -18.67979575497178502, 82.91557627198103830 ) ) ;
#23587=CARTESIAN_POINT ( 'NONE',  ( 21.53943276465977519, -0.05219959533907433946, 113.7489096053143527 ) ) ;
#23588=CARTESIAN_POINT ( 'NONE',  ( 16.55341960407611168, 4.379528057220329451, 33.95724293864769550 ) ) ;
#23589=CARTESIAN_POINT ( 'NONE',  ( 14.34966873604972726, -8.224510206698740333, 30.83442372801902209 ) ) ;
#23590=CARTESIAN_POINT ( 'NONE',  ( 9.474510206698971260, -16.51473224551069308, 37.91557627198102409 ) ) ;
#23591=CARTESIAN_POINT ( 'NONE',  ( -13.89961937509977652, 13.97604488694528158, 70.62390960531432427 ) ) ;
#23594=CARTESIAN_POINT ( 'NONE',  ( -5.049401038298153566, 19.05341960407611168, 115.2072429386477097 ) ) ;
#23596=CARTESIAN_POINT ( 'NONE',  ( -16.46253265017146816, -9.564922557961047289, 104.1677570613523329 ) ) ;
#23597=CARTESIAN_POINT ( 'NONE',  ( -0.05219959533936034679, 19.03943276465977164, 42.50109039468566152 ) ) ;
#23598=CARTESIAN_POINT ( 'NONE',  ( -5.823673210054116645, -21.52544592524344225, 92.29057627198103830 ) ) ;
#23599=CARTESIAN_POINT ( 'NONE',  ( 14.29746914071049879, -8.314922557960816363, 23.33224293864769194 ) ) ;
#23601=CARTESIAN_POINT ( 'NONE',  ( -10.72451020669898014, 18.67979575497178502, 40.41557627198103120 ) ) ;
#23602=CARTESIAN_POINT ( 'NONE',  ( 21.52544592524344225, -5.823673210054117533, 88.54057627198103830 ) ) ;
#23603=CARTESIAN_POINT ( 'NONE',  ( -0.05219959533936034679, 19.03943276465977164, 112.5010903946856757 ) ) ;
#23604=CARTESIAN_POINT ( 'NONE',  ( 9.564922557960805705, 16.46253265017160317, 99.58224293864770971 ) ) ;
#23605=CARTESIAN_POINT ( 'NONE',  ( -5.719274019375665041, -21.55341960407619695, 79.79275706135236135 ) ) ;
#23606=CARTESIAN_POINT ( 'NONE',  ( -0.05219959533909027116, -19.03943276465977164, 72.49890960531435269 ) ) ;
#23607=CARTESIAN_POINT ( 'NONE',  ( 12.14591786802309770, 12.06949235617756955, 104.3739096053143669 ) ) ;
#23609=CARTESIAN_POINT ( 'NONE',  ( -19.02544592524342804, 5.153800228976336051, 71.04057627198099567 ) ) ;
#23610=CARTESIAN_POINT ( 'NONE',  ( -12.14591786802309592, -12.06949235617757132, 91.87390960531436690 ) ) ;
#23612=CARTESIAN_POINT ( 'NONE',  ( -9.564922557961040184, 16.46253265017147172, 107.9177570613523471 ) ) ;
#23614=CARTESIAN_POINT ( 'NONE',  ( 5.153800228976335163, 19.02544592524342804, 54.79057627198103120 ) ) ;
#23615=CARTESIAN_POINT ( 'NONE',  ( 15.80617190586769283, -15.72974639402175789, 90.62609039468567573 ) ) ;
#23616=CARTESIAN_POINT ( 'NONE',  ( -0.05219959533909027116, -19.03943276465977164, 102.4989096053143669 ) ) ;
#23617=CARTESIAN_POINT ( 'NONE',  ( 14.29746914071037800, 8.314922557961029526, 81.66775706135236135 ) ) ;
#23618=CARTESIAN_POINT ( 'NONE',  ( -16.62475595723696742, -7.163666690055377373, 74.47286648189532343 ) ) ;
#23619=CARTESIAN_POINT ( 'NONE',  ( 9.474510206698729675, 16.51473224551082808, 62.08442372801899722 ) ) ;
#23620=CARTESIAN_POINT ( 'NONE',  ( 0.05219959533937995610, -21.53943276465977519, 105.0010903946856757 ) ) ;
#23622=CARTESIAN_POINT ( 'NONE',  ( -4.483927247898539470, -16.52544592524342804, 22.29057627198102765 ) ) ;
#23624=CARTESIAN_POINT ( 'NONE',  ( -16.52544592524335698, -4.483927247898792601, 88.95942372801901854 ) ) ;
#23626=CARTESIAN_POINT ( 'NONE',  ( -16.52544592524335698, -4.483927247898792601, 63.95942372801901854 ) ) ;
#23627=CARTESIAN_POINT ( 'NONE',  ( 18.62759615963255655, 10.81492255796105972, 81.66775706135236135 ) ) ;
#23628=CARTESIAN_POINT ( 'NONE',  ( 9.564922557961047289, -16.46253265017146816, 95.41775706135233293 ) ) ;
#23629=CARTESIAN_POINT ( 'NONE',  ( 19.02544592524334988, 5.153800228976608722, 41.45942372801900433 ) ) ;
#23630=CARTESIAN_POINT ( 'NONE',  ( -16.46253265017160317, 9.564922557960807481, 70.83224293864770971 ) ) ;
#23631=CARTESIAN_POINT ( 'NONE',  ( -16.46253265017160317, 9.564922557960807481, 60.83224293864769550 ) ) ;
#23633=CARTESIAN_POINT ( 'NONE',  ( -0.05219959533907301413, -21.53943276465977519, 77.49890960531433848 ) ) ;
#23634=CARTESIAN_POINT ( 'NONE',  ( -21.55341960407610458, -5.719274019375992779, 51.45724293864770260 ) ) ;
#23635=CARTESIAN_POINT ( 'NONE',  ( -0.05219959533909027116, -19.03943276465977164, 32.49890960531435979 ) ) ;
#23636=CARTESIAN_POINT ( 'NONE',  ( -16.53943276465976808, -0.05219959533934237506, 68.75109039468568994 ) ) ;
#23639=CARTESIAN_POINT ( 'NONE',  ( -21.52544592524334988, -5.823673210054445271, 48.95942372801902565 ) ) ;
#23640=CARTESIAN_POINT ( 'NONE',  ( -16.53943276465976808, 0.05219959533911058130, 66.24890960531436690 ) ) ;
#23642=CARTESIAN_POINT ( 'NONE',  ( 14.34966873604972726, -8.224510206698740333, 25.83442372801901499 ) ) ;
#23643=CARTESIAN_POINT ( 'NONE',  ( -0.05219959533936034679, 19.03943276465977164, 57.50109039468566863 ) ) ;
#23644=CARTESIAN_POINT ( 'NONE',  ( -4.379528057220328563, 16.55341960407611168, 55.20724293864770260 ) ) ;
#23645=CARTESIAN_POINT ( 'NONE',  ( 5.719274019375673035, 21.55341960407619339, 37.29275706135235424 ) ) ;
#23647=CARTESIAN_POINT ( 'NONE',  ( -15.80617190586745835, -15.72974639402198527, 71.87390960531438111 ) ) ;
#23648=CARTESIAN_POINT ( 'NONE',  ( -0.05219959533909027116, -19.03943276465977164, 102.4989096053143669 ) ) ;
#23649=CARTESIAN_POINT ( 'NONE',  ( 4.379528057220339221, -16.55341960407611168, 72.70724293864769550 ) ) ;
#23650=CARTESIAN_POINT ( 'NONE',  ( 5.153800228976335163, 19.02544592524342804, 114.7905762719810241 ) ) ;
#23651=CARTESIAN_POINT ( 'NONE',  ( 17.97214573761829470, 5.500000000000074607, 43.96970049038656470 ) ) ;
#23652=CARTESIAN_POINT ( 'NONE',  ( -19.05341960407617563, 5.049401038297882671, 73.54275706135233293 ) ) ;
#23653=CARTESIAN_POINT ( 'NONE',  ( 15.80617190586769283, -15.72974639402175789, 25.62609039468567929 ) ) ;
#23654=CARTESIAN_POINT ( 'NONE',  ( -13.89961937509977652, 13.97604488694528158, 55.62390960531434558 ) ) ;
#23655=CARTESIAN_POINT ( 'NONE',  ( -19.03943276465977164, -0.05219959533935918106, 43.75109039468566863 ) ) ;
#23656=CARTESIAN_POINT ( 'NONE',  ( -19.05341960407611168, -5.049401038298163336, 26.45724293864769550 ) ) ;
#23658=CARTESIAN_POINT ( 'NONE',  ( -10.72451020669870658, -18.67979575497194134, 69.58442372801900433 ) ) ;
#23659=CARTESIAN_POINT ( 'NONE',  ( 18.22780087662114212, -5.499999999999987566, 41.01540105326107977 ) ) ;
#23660=CARTESIAN_POINT ( 'NONE',  ( -4.483927247898539470, -16.52544592524342804, 42.29057627198103120 ) ) ;
#23661=CARTESIAN_POINT ( 'NONE',  ( 9.474510206698971260, -16.51473224551069308, 57.91557627198103120 ) ) ;
#23662=CARTESIAN_POINT ( 'NONE',  ( -5.823673210054116645, -21.52544592524344225, 92.29057627198103830 ) ) ;
#23663=CARTESIAN_POINT ( 'NONE',  ( 9.564922557960805705, 16.46253265017160317, 64.58224293864769550 ) ) ;
#23665=CARTESIAN_POINT ( 'NONE',  ( 18.67979575497178502, 10.72451020669898547, 64.16557627198102409 ) ) ;
#23667=CARTESIAN_POINT ( 'NONE',  ( 18.67979575497194134, -10.72451020669871369, 105.8344237280190328 ) ) ;
#23669=CARTESIAN_POINT ( 'NONE',  ( -0.05219959533934338120, 16.53943276465976808, 92.50109039468567573 ) ) ;
#23670=CARTESIAN_POINT ( 'NONE',  ( -16.52544592524342804, 4.483927247898546575, 86.04057627198102409 ) ) ;
#23671=CARTESIAN_POINT ( 'NONE',  ( 5.049401038297881783, 19.05341960407617563, 97.29275706135233293 ) ) ;
#23672=ORIENTED_EDGE ( 'NONE', *, *, #141950, .F. ) ;
#23673=CARTESIAN_POINT ( 'NONE',  ( 18.67979575497178502, 10.72451020669898547, 114.1655762719810383 ) ) ;
#23674=CARTESIAN_POINT ( 'NONE',  ( -5.049401038297874678, -19.05341960407617918, 34.79275706135233293 ) ) ;
#23675=CARTESIAN_POINT ( 'NONE',  ( -4.483927247898782831, 16.52544592524335698, 97.70942372801904696 ) ) ;
#23676=CARTESIAN_POINT ( 'NONE',  ( -19.02544592524334988, -5.153800228976617603, 23.95942372801900078 ) ) ;
#23677=CARTESIAN_POINT ( 'NONE',  ( -9.474510206698964154, 16.51473224551069663, 95.41557627198102409 ) ) ;
#23678=CARTESIAN_POINT ( 'NONE',  ( -21.53943276465977519, 0.05219959533907696930, 61.24890960531435979 ) ) ;
#23680=CARTESIAN_POINT ( 'NONE',  ( 19.02544592524343514, -5.153800228976328945, 23.54057627198102054 ) ) ;
#23681=CARTESIAN_POINT ( 'NONE',  ( 0.05219959533937995610, -21.53943276465977519, 110.0010903946856757 ) ) ;
#23682=CARTESIAN_POINT ( 'NONE',  ( 14.29746914071037800, 8.314922557961029526, 76.66775706135234714 ) ) ;
#23683=CARTESIAN_POINT ( 'NONE',  ( -15.72974639402176322, -15.80617190586768395, 29.37609039468568284 ) ) ;
#23684=CARTESIAN_POINT ( 'NONE',  ( -0.05219959533934338120, 16.53943276465976808, 27.50109039468567929 ) ) ;
#23685=CARTESIAN_POINT ( 'NONE',  ( -19.03943276465977164, 0.05219959533909376836, 101.2489096053143669 ) ) ;
#23686=CARTESIAN_POINT ( 'NONE',  ( -19.03943276465977164, 0.05219959533909376836, 36.24890960531436690 ) ) ;
#23687=CARTESIAN_POINT ( 'NONE',  ( 0.05219959533909260263, 19.03943276465977164, 64.99890960531436690 ) ) ;
#23688=CARTESIAN_POINT ( 'NONE',  ( 14.29746914071037800, 8.314922557961029526, 51.66775706135234714 ) ) ;
#23689=CARTESIAN_POINT ( 'NONE',  ( -16.52544592524342804, 4.483927247898546575, 86.04057627198102409 ) ) ;
#23690=CARTESIAN_POINT ( 'NONE',  ( 0.05219959533934541429, -16.53943276465976808, 100.0010903946857042 ) ) ;
#23691=CARTESIAN_POINT ( 'NONE',  ( -18.62759615963255300, -10.81492255796106328, 49.16775706135234003 ) ) ;
#23692=CARTESIAN_POINT ( 'NONE',  ( 13.89961937509977652, -13.97604488694527269, 73.12390960531436690 ) ) ;
#23693=CARTESIAN_POINT ( 'NONE',  ( 19.03943276465977164, -0.05219959533909143690, 68.74890960531436690 ) ) ;
#23694=CARTESIAN_POINT ( 'NONE',  ( 13.97604488694527802, 13.89961937509977652, 94.37390960531436690 ) ) ;
#23695=CARTESIAN_POINT ( 'NONE',  ( 8.224510206698953496, -14.34966873604960469, 32.91557627198102409 ) ) ;
#23696=CARTESIAN_POINT ( 'NONE',  ( -4.483927247898782831, 16.52544592524335698, 97.70942372801904696 ) ) ;
#23697=ORIENTED_EDGE ( 'NONE', *, *, #45727, .T. ) ;
#23698=CARTESIAN_POINT ( 'NONE',  ( 16.46253265017146816, 9.564922557961045513, 46.66775706135233293 ) ) ;
#23699=CARTESIAN_POINT ( 'NONE',  ( 0.05219959533909260263, 19.03943276465977164, 114.9989096053143669 ) ) ;
#23700=CARTESIAN_POINT ( 'NONE',  ( -19.02544592524342804, 5.153800228976336051, 61.04057627198103120 ) ) ;
#23701=CARTESIAN_POINT ( 'NONE',  ( 5.049401038297881783, 19.05341960407617563, 42.29275706135234003 ) ) ;
#23703=CARTESIAN_POINT ( 'NONE',  ( 19.35633801406911303, -5.499999999999579892, 71.63373818172765084 ) ) ;
#23704=CARTESIAN_POINT ( 'NONE',  ( 12.14591786802327356, -12.06949235617739191, 60.62609039468567573 ) ) ;
#23705=CARTESIAN_POINT ( 'NONE',  ( 16.51473224551083163, -9.474510206698727899, 70.83442372801900433 ) ) ;
#23706=CARTESIAN_POINT ( 'NONE',  ( -4.379528057220086978, -16.55341960407618274, 64.79275706135234714 ) ) ;
#23708=( BOUNDED_CURVE ( )  B_SPLINE_CURVE ( 2, ( #89808, #149491, #85813, #101988, #150502, #87805, #11999, #73662, #7967, #147499, #163669, #72660, #135334 ),
 .UNSPECIFIED., .F., .T. ) 
 B_SPLINE_CURVE_WITH_KNOTS ( ( 3, 2, 2, 2, 2, 2, 3 ),
 ( 0.7392725416902030666, 0.7412280701754385692, 0.7456140350877192846, 0.7500000000000000000, 0.7543859649122807154, 0.7587719298245614308, 0.7606817784877069055 ),
 .UNSPECIFIED. ) 
 CURVE ( )  GEOMETRIC_REPRESENTATION_ITEM ( )  RATIONAL_B_SPLINE_CURVE ( ( 0.9831626618144007068, 0.9848076720550096308, 1.000000000000000000, 0.9659258262890683122, 1.000000000000000000, 0.9659258262890683122, 1.000000000000000000, 0.9659258262890683122, 1.000000000000000000, 0.9659258262890683122, 1.000000000000000000, 0.9851625545550091179, 0.9832469066685282089 ) ) 
 REPRESENTATION_ITEM ( '' )  );
#23709=CARTESIAN_POINT ( 'NONE',  ( 5.049401038298161559, -19.05341960407611168, 87.70724293864769550 ) ) ;
#23710=CARTESIAN_POINT ( 'NONE',  ( -21.53943276465977519, 0.05219959533907696930, 116.2489096053143669 ) ) ;
#23711=CARTESIAN_POINT ( 'NONE',  ( 19.02544592524334988, 5.153800228976608722, 81.45942372801897591 ) ) ;
#23712=CARTESIAN_POINT ( 'NONE',  ( 19.03943276465977164, -0.05219959533909143690, 108.7489096053143527 ) ) ;
#23713=CARTESIAN_POINT ( 'NONE',  ( -19.05341960407611168, -5.049401038298163336, 31.45724293864769550 ) ) ;
#23714=CARTESIAN_POINT ( 'NONE',  ( -9.474510206698964154, 16.51473224551069663, 75.41557627198103830 ) ) ;
#23715=CARTESIAN_POINT ( 'NONE',  ( -4.483927247898539470, -16.52544592524342804, 42.29057627198103120 ) ) ;
#23716=CARTESIAN_POINT ( 'NONE',  ( 0.05219959533909260263, 19.03943276465977164, 34.99890960531435979 ) ) ;
#23717=CARTESIAN_POINT ( 'NONE',  ( 13.89961937509957401, 13.97604488694547697, 51.87609039468566863 ) ) ;
#23718=CARTESIAN_POINT ( 'NONE',  ( -16.53943276465976808, 0.05219959533911058130, 81.24890960531436690 ) ) ;
#23719=CARTESIAN_POINT ( 'NONE',  ( -21.52544592524334988, -5.823673210054445271, 108.9594237280190185 ) ) ;
#23720=CARTESIAN_POINT ( 'NONE',  ( 16.51473224551069308, 9.474510206698969483, 59.16557627198102409 ) ) ;
#23721=CARTESIAN_POINT ( 'NONE',  ( -15.72974639402197994, 15.80617190586746368, 55.62390960531436690 ) ) ;
#23722=CARTESIAN_POINT ( 'NONE',  ( 8.224510206698953496, -14.34966873604960469, 47.91557627198102409 ) ) ;
#23723=CARTESIAN_POINT ( 'NONE',  ( 19.02544592524334988, 5.153800228976608722, 21.45942372801899012 ) ) ;
#23724=CARTESIAN_POINT ( 'NONE',  ( -9.474510206698964154, 16.51473224551069663, 110.4155762719810383 ) ) ;
#23725=CARTESIAN_POINT ( 'NONE',  ( 19.03943276465977164, -0.05219959533909143690, 103.7489096053143669 ) ) ;
#23726=CARTESIAN_POINT ( 'NONE',  ( -19.03943276465977164, 0.05219959533909376836, 36.24890960531436690 ) ) ;
#23727=CARTESIAN_POINT ( 'NONE',  ( 13.89961937509977652, -13.97604488694527269, 23.12390960531436335 ) ) ;
#23728=CARTESIAN_POINT ( 'NONE',  ( -4.379528057220328563, 16.55341960407611168, 85.20724293864770971 ) ) ;
#23729=CARTESIAN_POINT ( 'NONE',  ( -18.67979575497178146, -10.72451020669898902, 101.6655762719810383 ) ) ;
#23730=CARTESIAN_POINT ( 'NONE',  ( -0.05219959533909027116, -19.03943276465977164, 107.4989096053143527 ) ) ;
#23731=CARTESIAN_POINT ( 'NONE',  ( 21.53943276465977519, -0.05219959533907433946, 113.7489096053143527 ) ) ;
#23732=CARTESIAN_POINT ( 'NONE',  ( -16.46253265017160317, 9.564922557960807481, 100.8322429386477097 ) ) ;
#23734=CARTESIAN_POINT ( 'NONE',  ( 16.53943276465976808, -0.05219959533910856209, 108.7489096053143669 ) ) ;
#23735=CARTESIAN_POINT ( 'NONE',  ( -0.05219959533937732626, 21.53943276465977519, 77.50109039468567573 ) ) ;
#23736=CARTESIAN_POINT ( 'NONE',  ( 15.80617190586746368, 15.72974639402197994, 84.37390960531438111 ) ) ;
#23737=CARTESIAN_POINT ( 'NONE',  ( 17.13100169013301510, -6.664070546373136672, 108.2678983569985434 ) ) ;
#23738=CARTESIAN_POINT ( 'NONE',  ( 19.52217212775661892, -5.499999999999912070, 77.43993709005262360 ) ) ;
#23739=CARTESIAN_POINT ( 'NONE',  ( 5.823673210054125526, 21.52544592524343514, 34.79057627198103120 ) ) ;
#23741=CARTESIAN_POINT ( 'NONE',  ( -0.05219959533934338120, 16.53943276465976808, 27.50109039468567929 ) ) ;
#23742=CARTESIAN_POINT ( 'NONE',  ( -8.314922557960811034, -14.29746914071050412, 112.0822429386477097 ) ) ;
#23743=CARTESIAN_POINT ( 'NONE',  ( -17.50000000000000711, -3.305555262949610107, 110.3748284784340399 ) ) ;
#23744=CARTESIAN_POINT ( 'NONE',  ( 13.97604488694527802, 13.89961937509977652, 54.37390960531435979 ) ) ;
#23745=CARTESIAN_POINT ( 'NONE',  ( 4.483927247898545687, 16.52544592524342804, 84.79057627198102409 ) ) ;
#23747=CARTESIAN_POINT ( 'NONE',  ( -21.53943276465977519, 0.05219959533907696930, 31.24890960531435979 ) ) ;
#23748=CARTESIAN_POINT ( 'NONE',  ( -4.379528057220328563, 16.55341960407611168, 70.20724293864769550 ) ) ;
#23749=CARTESIAN_POINT ( 'NONE',  ( -4.379528057220086978, -16.55341960407618274, 19.79275706135235069 ) ) ;
#23750=CARTESIAN_POINT ( 'NONE',  ( -21.52544592524334988, -5.823673210054445271, 73.95942372801901854 ) ) ;
#23751=CARTESIAN_POINT ( 'NONE',  ( 16.61371651742601685, -7.165104196376138823, 76.35415069992995996 ) ) ;
#23752=CARTESIAN_POINT ( 'NONE',  ( -21.53943276465977519, 0.05219959533907696930, 21.24890960531436690 ) ) ;
#23753=CARTESIAN_POINT ( 'NONE',  ( -12.06949235617739369, -12.14591786802326823, 89.37609039468568994 ) ) ;
#23754=CARTESIAN_POINT ( 'NONE',  ( 9.474510206698971260, -16.51473224551069308, 37.91557627198102409 ) ) ;
#23755=CARTESIAN_POINT ( 'NONE',  ( -5.049401038298153566, 19.05341960407611168, 90.20724293864766707 ) ) ;
#23756=CARTESIAN_POINT ( 'NONE',  ( -21.52544592524343514, 5.823673210054127303, 91.04057627198103830 ) ) ;
#23757=CARTESIAN_POINT ( 'NONE',  ( -4.483927247898782831, 16.52544592524335698, 32.70942372801900433 ) ) ;
#23758=CARTESIAN_POINT ( 'NONE',  ( -12.06949235617756955, 12.14591786802309770, 55.62390960531436690 ) ) ;
#23759=CARTESIAN_POINT ( 'NONE',  ( -5.823673210054431948, 21.52544592524334988, 77.70942372801900433 ) ) ;
#23761=CARTESIAN_POINT ( 'NONE',  ( 4.483927247898790824, -16.52544592524335698, 95.20942372801903275 ) ) ;
#23764=CARTESIAN_POINT ( 'NONE',  ( -0.05219959533910754901, -16.53943276465976808, 22.49890960531436335 ) ) ;
#23765=CARTESIAN_POINT ( 'NONE',  ( 12.14591786802327356, -12.06949235617739191, 60.62609039468567573 ) ) ;
#23766=CARTESIAN_POINT ( 'NONE',  ( 19.02544592524343514, -5.153800228976328945, 68.54057627198103830 ) ) ;
#23767=CARTESIAN_POINT ( 'NONE',  ( 0.05219959533909260263, 19.03943276465977164, 89.99890960531436690 ) ) ;
#23768=CARTESIAN_POINT ( 'NONE',  ( 21.52544592524334988, 5.823673210054432836, 71.45942372801901854 ) ) ;
#23769=CARTESIAN_POINT ( 'NONE',  ( 16.52544592524335698, 4.483927247898782831, 91.45942372801901854 ) ) ;
#23770=CARTESIAN_POINT ( 'NONE',  ( 16.53943276465976808, -0.05219959533910856209, 53.74890960531437401 ) ) ;
#23771=CARTESIAN_POINT ( 'NONE',  ( 19.03943276465977164, -0.05219959533909143690, 68.74890960531436690 ) ) ;
#23772=ORIENTED_EDGE ( 'NONE', *, *, #8686, .T. ) ;
#23773=CARTESIAN_POINT ( 'NONE',  ( -13.97604488694547697, 13.89961937509957934, 108.1260903946856331 ) ) ;
#23774=CARTESIAN_POINT ( 'NONE',  ( -16.53943276465976808, 0.05219959533911058130, 106.2489096053143811 ) ) ;
#23775=CARTESIAN_POINT ( 'NONE',  ( -5.049401038298153566, 19.05341960407611168, 80.20724293864769550 ) ) ;
#23776=CARTESIAN_POINT ( 'NONE',  ( -0.05219959533936034679, 19.03943276465977164, 107.5010903946856615 ) ) ;
#23778=CARTESIAN_POINT ( 'NONE',  ( -10.72451020669870658, -18.67979575497194134, 104.5844237280190185 ) ) ;
#23779=CARTESIAN_POINT ( 'NONE',  ( 8.224510206698742110, 14.34966873604972548, 82.08442372801901854 ) ) ;
#23780=CARTESIAN_POINT ( 'NONE',  ( -5.153800228976607833, 19.02544592524334988, 92.70942372801901854 ) ) ;
#23781=CARTESIAN_POINT ( 'NONE',  ( 16.55341960407611168, 4.379528057220329451, 108.9572429386476955 ) ) ;
#23782=CARTESIAN_POINT ( 'NONE',  ( 12.06949235617739724, 12.14591786802326823, 61.87609039468568284 ) ) ;
#23784=CARTESIAN_POINT ( 'NONE',  ( -16.46253265017146816, -9.564922557961047289, 54.16775706135234003 ) ) ;
#23785=CARTESIAN_POINT ( 'NONE',  ( -15.80617190586768217, 15.72974639402176855, 98.12609039468570415 ) ) ;
#23786=CARTESIAN_POINT ( 'NONE',  ( 19.02544592524343514, -5.153800228976328945, 38.54057627198103120 ) ) ;
#23787=CARTESIAN_POINT ( 'NONE',  ( -13.89961937509977652, 13.97604488694528158, 75.62390960531438111 ) ) ;
#23788=CARTESIAN_POINT ( 'NONE',  ( 16.55341960407611168, 4.379528057220329451, 73.95724293864769550 ) ) ;
#23789=CARTESIAN_POINT ( 'NONE',  ( -21.53943276465977519, -0.05219959533937600094, 93.75109039468567573 ) ) ;
#23791=CARTESIAN_POINT ( 'NONE',  ( 16.51473224551083163, -9.474510206698727899, 45.83442372801900433 ) ) ;
#23792=CARTESIAN_POINT ( 'NONE',  ( 13.89961937509957401, 13.97604488694547697, 36.87609039468565442 ) ) ;
#23793=CARTESIAN_POINT ( 'NONE',  ( 18.62759615963271287, -10.81492255796078972, 38.33224293864768839 ) ) ;
#23794=CARTESIAN_POINT ( 'NONE',  ( 15.72974639402176855, 15.80617190586768217, 91.87609039468568994 ) ) ;
#23795=CARTESIAN_POINT ( 'NONE',  ( -5.153800228976328057, -19.02544592524343514, 77.29057627198099567 ) ) ;
#23796=CARTESIAN_POINT ( 'NONE',  ( 10.72451020669871369, 18.67979575497193778, 87.08442372801901854 ) ) ;
#23797=CARTESIAN_POINT ( 'NONE',  ( 15.80617190586746368, 15.72974639402197994, 54.37390960531435979 ) ) ;
#23798=CARTESIAN_POINT ( 'NONE',  ( 16.51473224551069308, 9.474510206698969483, 84.16557627198102409 ) ) ;
#23799=CARTESIAN_POINT ( 'NONE',  ( -19.05341960407617563, 5.049401038297882671, 68.54275706135230450 ) ) ;
#23800=CARTESIAN_POINT ( 'NONE',  ( 13.97604488694527802, 13.89961937509977652, 84.37390960531433848 ) ) ;
#23801=CARTESIAN_POINT ( 'NONE',  ( 19.02544592524334988, 5.153800228976608722, 101.4594237280189759 ) ) ;
#23802=CARTESIAN_POINT ( 'NONE',  ( -14.29746914071037622, -8.314922557961029526, 39.16775706135235424 ) ) ;
#23803=CARTESIAN_POINT ( 'NONE',  ( -4.483927247898539470, -16.52544592524342804, 97.29057627198105251 ) ) ;
#23804=CARTESIAN_POINT ( 'NONE',  ( 9.474510206698971260, -16.51473224551069308, 72.91557627198102409 ) ) ;
#23805=CARTESIAN_POINT ( 'NONE',  ( 18.67979575497178502, 10.72451020669898547, 69.16557627198102409 ) ) ;
#23806=CARTESIAN_POINT ( 'NONE',  ( -16.52544592524335698, -4.483927247898792601, 33.95942372801901143 ) ) ;
#23807=CARTESIAN_POINT ( 'NONE',  ( -21.55341960407619339, 5.719274019375674811, 38.54275706135234714 ) ) ;
#23808=CARTESIAN_POINT ( 'NONE',  ( 15.72974639402176855, 15.80617190586768217, 81.87609039468568994 ) ) ;
#23809=CARTESIAN_POINT ( 'NONE',  ( 16.55341960407618274, -4.379528057220086978, 86.04275706135236135 ) ) ;
#23811=CARTESIAN_POINT ( 'NONE',  ( 19.05341960407611168, 5.049401038298154454, 68.95724293864769550 ) ) ;
#23812=CARTESIAN_POINT ( 'NONE',  ( -0.05219959533910754901, -16.53943276465976808, 82.49890960531436690 ) ) ;
#23813=CARTESIAN_POINT ( 'NONE',  ( -12.14591786802326823, 12.06949235617739902, 103.1260903946856757 ) ) ;
#23814=CARTESIAN_POINT ( 'NONE',  ( 5.153800228976615827, -19.02544592524334988, 50.20942372801897591 ) ) ;
#23815=CARTESIAN_POINT ( 'NONE',  ( 10.72451020669871369, 18.67979575497193778, 32.08442372801901854 ) ) ;
#23816=CARTESIAN_POINT ( 'NONE',  ( -14.29746914071049879, 8.314922557960819915, 75.83224293864769550 ) ) ;
#23817=CARTESIAN_POINT ( 'NONE',  ( 16.46253265017160672, -9.564922557960803928, 103.3322429386476955 ) ) ;
#23818=CARTESIAN_POINT ( 'NONE',  ( 16.53943276465976808, 0.05219959533934440121, 106.2510903946856757 ) ) ;
#23819=CARTESIAN_POINT ( 'NONE',  ( -18.62759615963255300, -10.81492255796106328, 69.16775706135234714 ) ) ;
#23820=CARTESIAN_POINT ( 'NONE',  ( 16.55341960407618274, -4.379528057220086978, 51.04275706135234714 ) ) ;
#23821=CARTESIAN_POINT ( 'NONE',  ( -10.72451020669870658, -18.67979575497194134, 39.58442372801901143 ) ) ;
#23822=CARTESIAN_POINT ( 'NONE',  ( 16.52544592524342804, -4.483927247898539470, 73.54057627198102409 ) ) ;
#23823=ORIENTED_EDGE ( 'NONE', *, *, #61085, .F. ) ;
#23824=CARTESIAN_POINT ( 'NONE',  ( 21.53943276465977519, 0.05219959533937863772, 21.25109039468567218 ) ) ;
#23826=CARTESIAN_POINT ( 'NONE',  ( -16.55341960407611168, -4.379528057220339221, 51.45724293864770260 ) ) ;
#23827=DIRECTION ( 'NONE',  ( -1.000000000000000000, -0.000000000000000000, -0.000000000000000000 ) ) ;
#23828=CARTESIAN_POINT ( 'NONE',  ( -21.52544592524343514, 5.823673210054127303, 41.04057627198103120 ) ) ;
#23829=CARTESIAN_POINT ( 'NONE',  ( 0.05219959533910956823, 16.53943276465976808, 79.99890960531435269 ) ) ;
#23830=CARTESIAN_POINT ( 'NONE',  ( -5.719274019375978568, 21.55341960407610458, 80.20724293864769550 ) ) ;
#23831=CARTESIAN_POINT ( 'NONE',  ( 19.02544592524343514, -5.153800228976328945, 93.54057627198102409 ) ) ;
#23832=CARTESIAN_POINT ( 'NONE',  ( 0.05219959533909260263, 19.03943276465977164, 34.99890960531435979 ) ) ;
#23833=CARTESIAN_POINT ( 'NONE',  ( -0.05219959533936034679, 19.03943276465977164, 77.50109039468566152 ) ) ;
#23835=CARTESIAN_POINT ( 'NONE',  ( 15.80617190586769283, -15.72974639402175789, 55.62609039468568284 ) ) ;
#23836=CARTESIAN_POINT ( 'NONE',  ( -21.53943276465977519, 0.05219959533907696930, 66.24890960531436690 ) ) ;
#23837=CARTESIAN_POINT ( 'NONE',  ( 19.05341960407611168, 5.049401038298154454, 33.95724293864769550 ) ) ;
#23838=CARTESIAN_POINT ( 'NONE',  ( 0.05219959533909260263, 19.03943276465977164, 69.99890960531435269 ) ) ;
#23840=CARTESIAN_POINT ( 'NONE',  ( 16.53943276465976808, 0.05219959533934440121, 56.25109039468568284 ) ) ;
#23841=CARTESIAN_POINT ( 'NONE',  ( -5.719274019375665041, -21.55341960407619695, 29.79275706135234358 ) ) ;
#23842=CARTESIAN_POINT ( 'NONE',  ( 5.719274019375673035, 21.55341960407619339, 62.29275706135236845 ) ) ;
#23843=CARTESIAN_POINT ( 'NONE',  ( -5.153800228976328057, -19.02544592524343514, 107.2905762719810383 ) ) ;
#23844=CARTESIAN_POINT ( 'NONE',  ( 0.05219959533907565091, 21.53943276465977519, 79.99890960531435269 ) ) ;
#23845=CARTESIAN_POINT ( 'NONE',  ( 21.52544592524334988, 5.823673210054432836, 26.45942372801901854 ) ) ;
#23846=CARTESIAN_POINT ( 'NONE',  ( 16.53943276465976808, 0.05219959533934440121, 46.25109039468567573 ) ) ;
#23847=CARTESIAN_POINT ( 'NONE',  ( -18.67979575497178146, -10.72451020669898902, 51.66557627198102409 ) ) ;
#23848=CARTESIAN_POINT ( 'NONE',  ( -21.52544592524334988, -5.823673210054445271, 108.9594237280190185 ) ) ;
#23849=CARTESIAN_POINT ( 'NONE',  ( -19.03943276465977164, 0.05219959533909376836, 56.24890960531435979 ) ) ;
#23851=CARTESIAN_POINT ( 'NONE',  ( 9.564922557960805705, 16.46253265017160317, 89.58224293864769550 ) ) ;
#23853=CARTESIAN_POINT ( 'NONE',  ( -19.02544592524334988, -5.153800228976617603, 73.95942372801900433 ) ) ;
#23854=CARTESIAN_POINT ( 'NONE',  ( -0.05219959533907301413, -21.53943276465977519, 42.49890960531435979 ) ) ;
#23855=CARTESIAN_POINT ( 'NONE',  ( -14.34966873604960291, -8.224510206698953496, 21.66557627198102409 ) ) ;
#23856=CARTESIAN_POINT ( 'NONE',  ( -0.05219959533936034679, 19.03943276465977164, 97.50109039468567573 ) ) ;
#23858=CARTESIAN_POINT ( 'NONE',  ( 13.89961937509957401, 13.97604488694547697, 26.87609039468566507 ) ) ;
#23859=CARTESIAN_POINT ( 'NONE',  ( 0.05219959533936267826, -19.03943276465977164, 100.0010903946856757 ) ) ;
#23860=CARTESIAN_POINT ( 'NONE',  ( -0.05219959533936034679, 19.03943276465977164, 42.50109039468566152 ) ) ;
#23861=CARTESIAN_POINT ( 'NONE',  ( 16.19135201231367915, 7.376712067591916444, 107.6868085405203743 ) ) ;
#23862=CARTESIAN_POINT ( 'NONE',  ( -5.049401038298153566, 19.05341960407611168, 55.20724293864769550 ) ) ;
#23863=CARTESIAN_POINT ( 'NONE',  ( 8.314922557960818139, 14.29746914071049879, 59.58224293864770260 ) ) ;
#23864=CARTESIAN_POINT ( 'NONE',  ( -9.564922557960796823, -16.46253265017161027, 32.08224293864769550 ) ) ;
#23865=CARTESIAN_POINT ( 'NONE',  ( -12.06949235617756955, 12.14591786802309770, 45.62390960531436690 ) ) ;
#23867=CARTESIAN_POINT ( 'NONE',  ( -12.06949235617739369, -12.14591786802326823, 104.3760903946856899 ) ) ;
#23868=CARTESIAN_POINT ( 'NONE',  ( -5.153800228976328057, -19.02544592524343514, 62.29057627198100988 ) ) ;
#23869=CARTESIAN_POINT ( 'NONE',  ( 13.97604488694548053, -13.89961937509957401, 20.62609039468567573 ) ) ;
#23870=CARTESIAN_POINT ( 'NONE',  ( -14.34966873604972548, 8.224510206698743886, 28.33442372801902209 ) ) ;
#23871=CARTESIAN_POINT ( 'NONE',  ( -5.719274019375978568, 21.55341960407610458, 50.20724293864769550 ) ) ;
#23872=CARTESIAN_POINT ( 'NONE',  ( 21.55341960407619695, -5.719274019375665929, 111.0427570613523613 ) ) ;
#23873=ORIENTED_EDGE ( 'NONE', *, *, #59341, .F. ) ;
#23874=CARTESIAN_POINT ( 'NONE',  ( 9.564922557960805705, 16.46253265017160317, 59.58224293864769550 ) ) ;
#23875=CARTESIAN_POINT ( 'NONE',  ( 5.049401038298161559, -19.05341960407611168, 107.7072429386476955 ) ) ;
#23876=CARTESIAN_POINT ( 'NONE',  ( 0.05219959533909260263, 19.03943276465977164, 94.99890960531436690 ) ) ;
#23878=CARTESIAN_POINT ( 'NONE',  ( -21.53943276465977519, -0.05219959533937600094, 28.75109039468567929 ) ) ;
#23879=CARTESIAN_POINT ( 'NONE',  ( -12.06949235617756955, 12.14591786802309770, 90.62390960531436690 ) ) ;
#23880=CARTESIAN_POINT ( 'NONE',  ( 21.53943276465977519, -0.05219959533907433946, 83.74890960531435269 ) ) ;
#23881=CARTESIAN_POINT ( 'NONE',  ( 5.049401038298161559, -19.05341960407611168, 62.70724293864769550 ) ) ;
#23882=CARTESIAN_POINT ( 'NONE',  ( -9.564922557960796823, -16.46253265017161027, 72.08224293864770971 ) ) ;
#23883=CARTESIAN_POINT ( 'NONE',  ( -15.72974639402197994, 15.80617190586746368, 110.6239096053143669 ) ) ;
#23884=VERTEX_POINT ( 'NONE', #147228 ) ;
#23885=CARTESIAN_POINT ( 'NONE',  ( 9.474510206698971260, -16.51473224551069308, 77.91557627198103830 ) ) ;
#23887=CARTESIAN_POINT ( 'NONE',  ( 30.00000000000000000, -5.499999999999992895, 102.5000000000000142 ) ) ;
#23888=CARTESIAN_POINT ( 'NONE',  ( -4.379528057220328563, 16.55341960407611168, 100.2072429386476955 ) ) ;
#23889=CARTESIAN_POINT ( 'NONE',  ( 0.05219959533909260263, 19.03943276465977164, 24.99890960531435269 ) ) ;
#23890=CARTESIAN_POINT ( 'NONE',  ( 13.89961937509957401, 13.97604488694547697, 96.87609039468566152 ) ) ;
#23891=CARTESIAN_POINT ( 'NONE',  ( -4.483927247898539470, -16.52544592524342804, 102.2905762719810383 ) ) ;
#23892=CARTESIAN_POINT ( 'NONE',  ( 21.53943276465977519, 0.05219959533937863772, 76.25109039468568994 ) ) ;
#23893=CARTESIAN_POINT ( 'NONE',  ( -19.05341960407611168, -5.049401038298163336, 66.45724293864769550 ) ) ;
#23894=CARTESIAN_POINT ( 'NONE',  ( -10.81492255796105439, 18.62759615963255655, 27.91775706135234358 ) ) ;
#23895=CARTESIAN_POINT ( 'NONE',  ( 18.67979575497178502, 10.72451020669898547, 109.1655762719810383 ) ) ;
#23897=CARTESIAN_POINT ( 'NONE',  ( -13.89961937509977652, 13.97604488694528158, 70.62390960531432427 ) ) ;
#23899=CARTESIAN_POINT ( 'NONE',  ( -14.29746914071037622, -8.314922557961029526, 19.16775706135234714 ) ) ;
#23900=CARTESIAN_POINT ( 'NONE',  ( 21.55341960407610458, 5.719274019375980345, 23.95724293864769550 ) ) ;
#23901=CARTESIAN_POINT ( 'NONE',  ( 15.80617190586769283, -15.72974639402175789, 60.62609039468567573 ) ) ;
#23902=CARTESIAN_POINT ( 'NONE',  ( -9.564922557960796823, -16.46253265017161027, 102.0822429386477097 ) ) ;
#23903=CARTESIAN_POINT ( 'NONE',  ( 0.05219959533936267826, -19.03943276465977164, 80.00109039468567573 ) ) ;
#23904=CARTESIAN_POINT ( 'NONE',  ( -5.049401038298153566, 19.05341960407611168, 50.20724293864770260 ) ) ;
#23905=CARTESIAN_POINT ( 'NONE',  ( 5.049401038298161559, -19.05341960407611168, 67.70724293864769550 ) ) ;
#23906=CARTESIAN_POINT ( 'NONE',  ( 12.06949235617757843, -12.14591786802309237, 93.12390960531436690 ) ) ;
#23907=CARTESIAN_POINT ( 'NONE',  ( 13.89961937509977652, -13.97604488694527269, 103.1239096053143527 ) ) ;
#23908=CARTESIAN_POINT ( 'NONE',  ( -8.314922557960811034, -14.29746914071050412, 97.08224293864770971 ) ) ;
#23909=CARTESIAN_POINT ( 'NONE',  ( -0.05219959533909027116, -19.03943276465977164, 97.49890960531436690 ) ) ;
#23910=CARTESIAN_POINT ( 'NONE',  ( 4.483927247898545687, 16.52544592524342804, 39.79057627198103830 ) ) ;
#23911=CARTESIAN_POINT ( 'NONE',  ( 19.03943276465977164, -0.05219959533909143690, 33.74890960531435979 ) ) ;
#23913=CARTESIAN_POINT ( 'NONE',  ( -10.81492255796105439, 18.62759615963255655, 62.91775706135236135 ) ) ;
#23914=CARTESIAN_POINT ( 'NONE',  ( 5.153800228976615827, -19.02544592524334988, 75.20942372801896170 ) ) ;
#23915=CARTESIAN_POINT ( 'NONE',  ( -8.224510206698948167, 14.34966873604960824, 45.41557627198103830 ) ) ;
#23916=CARTESIAN_POINT ( 'NONE',  ( -15.72974639402197994, 15.80617190586746368, 95.62390960531436690 ) ) ;
#23917=CARTESIAN_POINT ( 'NONE',  ( 15.72974639402199770, -15.80617190586745480, 38.12390960531436690 ) ) ;
#23918=CARTESIAN_POINT ( 'NONE',  ( -0.05219959533910754901, -16.53943276465976808, 77.49890960531433848 ) ) ;
#23919=CARTESIAN_POINT ( 'NONE',  ( 5.153800228976335163, 19.02544592524342804, 54.79057627198103120 ) ) ;
#23920=CARTESIAN_POINT ( 'NONE',  ( -4.379528057220328563, 16.55341960407611168, 25.20724293864769550 ) ) ;
#23921=CARTESIAN_POINT ( 'NONE',  ( -16.55341960407617563, 4.379528057220093196, 103.5427570613523613 ) ) ;
#23922=CARTESIAN_POINT ( 'NONE',  ( -4.379528057220086978, -16.55341960407618274, 74.79275706135234714 ) ) ;
#23923=CARTESIAN_POINT ( 'NONE',  ( 19.03943276465977164, 0.05219959533936151252, 31.25109039468566863 ) ) ;
#23924=CARTESIAN_POINT ( 'NONE',  ( -19.05341960407611168, -5.049401038298163336, 111.4572429386476671 ) ) ;
#23925=CARTESIAN_POINT ( 'NONE',  ( 9.564922557960805705, 16.46253265017160317, 84.58224293864769550 ) ) ;
#23926=CARTESIAN_POINT ( 'NONE',  ( -19.05341960407611168, -5.049401038298163336, 41.45724293864769550 ) ) ;
#23927=CARTESIAN_POINT ( 'NONE',  ( 8.314922557960818139, 14.29746914071049879, 49.58224293864769550 ) ) ;
#23928=CARTESIAN_POINT ( 'NONE',  ( 30.00000000000000000, 5.499999999999992895, 37.50000000000000000 ) ) ;
#23929=CARTESIAN_POINT ( 'NONE',  ( 16.51473224551069308, 9.474510206698969483, 104.1655762719810241 ) ) ;
#23930=CARTESIAN_POINT ( 'NONE',  ( -15.72974639402197994, 15.80617190586746368, 45.62390960531436690 ) ) ;
#23931=CARTESIAN_POINT ( 'NONE',  ( 12.14591786802309770, 12.06949235617756955, 79.37390960531436690 ) ) ;
#23932=CARTESIAN_POINT ( 'NONE',  ( -14.29746914071037622, -8.314922557961029526, 29.16775706135234003 ) ) ;
#23934=CARTESIAN_POINT ( 'NONE',  ( -14.34966873604960291, -8.224510206698953496, 71.66557627198100988 ) ) ;
#23936=CARTESIAN_POINT ( 'NONE',  ( -5.049401038297874678, -19.05341960407617918, 59.79275706135231871 ) ) ;
#23937=CARTESIAN_POINT ( 'NONE',  ( -0.05219959533909027116, -19.03943276465977164, 107.4989096053143527 ) ) ;
#23938=CARTESIAN_POINT ( 'NONE',  ( 13.89961937509957401, 13.97604488694547697, 76.87609039468566152 ) ) ;
#23939=CARTESIAN_POINT ( 'NONE',  ( -16.46253265017146816, -9.564922557961047289, 94.16775706135233293 ) ) ;
#23940=CARTESIAN_POINT ( 'NONE',  ( -8.314922557961024197, 14.29746914071037800, 22.91775706135235069 ) ) ;
#23941=CARTESIAN_POINT ( 'NONE',  ( -8.224510206698735004, -14.34966873604973081, 109.5844237280190328 ) ) ;
#23942=CARTESIAN_POINT ( 'NONE',  ( -9.474510206698720793, -16.51473224551083518, 74.58442372801900433 ) ) ;
#23943=CARTESIAN_POINT ( 'NONE',  ( -15.80617190586745835, -15.72974639402198527, 41.87390960531435979 ) ) ;
#23944=CARTESIAN_POINT ( 'NONE',  ( -21.55341960407619339, 5.719274019375674811, 63.54275706135234003 ) ) ;
#23946=CARTESIAN_POINT ( 'NONE',  ( 19.03943276465977164, 0.05219959533936151252, 111.2510903946856757 ) ) ;
#23947=CARTESIAN_POINT ( 'NONE',  ( 17.49999999999997868, 3.373831961294261106, 22.36044703459066341 ) ) ;
#23948=CARTESIAN_POINT ( 'NONE',  ( 9.474510206698971260, -16.51473224551069308, 77.91557627198103830 ) ) ;
#23949=CARTESIAN_POINT ( 'NONE',  ( -13.97604488694527625, -13.89961937509977652, 26.87390960531434558 ) ) ;
#23950=CARTESIAN_POINT ( 'NONE',  ( -0.05219959533910754901, -16.53943276465976808, 92.49890960531436690 ) ) ;
#23951=CARTESIAN_POINT ( 'NONE',  ( -13.97604488694527625, -13.89961937509977652, 81.87390960531436690 ) ) ;
#23952=CARTESIAN_POINT ( 'NONE',  ( 13.97604488694527802, 13.89961937509977652, 84.37390960531433848 ) ) ;
#23954=CARTESIAN_POINT ( 'NONE',  ( 19.02544592524334988, 5.153800228976608722, 86.45942372801900433 ) ) ;
#23955=CARTESIAN_POINT ( 'NONE',  ( 21.52544592524344225, -5.823673210054117533, 73.54057627198102409 ) ) ;
#23956=CARTESIAN_POINT ( 'NONE',  ( 13.97604488694527802, 13.89961937509977652, 34.37390960531436690 ) ) ;
#23957=CARTESIAN_POINT ( 'NONE',  ( -9.474510206698720793, -16.51473224551083518, 54.58442372801899722 ) ) ;
#23958=CARTESIAN_POINT ( 'NONE',  ( -16.46253265017160317, 9.564922557960807481, 55.83224293864769550 ) ) ;
#23959=CARTESIAN_POINT ( 'NONE',  ( -0.05219959533909027116, -19.03943276465977164, 87.49890960531436690 ) ) ;
#23961=CARTESIAN_POINT ( 'NONE',  ( 0.05219959533907565091, 21.53943276465977519, 104.9989096053143669 ) ) ;
#23962=CARTESIAN_POINT ( 'NONE',  ( -4.483927247898539470, -16.52544592524342804, 87.29057627198103830 ) ) ;
#23963=CARTESIAN_POINT ( 'NONE',  ( -13.97604488694527625, -13.89961937509977652, 86.87390960531436690 ) ) ;
#23964=CARTESIAN_POINT ( 'NONE',  ( 19.02544592524334988, 5.153800228976608722, 61.45942372801900433 ) ) ;
#23965=CARTESIAN_POINT ( 'NONE',  ( 15.72974639402199770, -15.80617190586745480, 93.12390960531436690 ) ) ;
#23966=CARTESIAN_POINT ( 'NONE',  ( -10.81492255796078084, -18.62759615963271287, 72.08224293864769550 ) ) ;
#23967=CARTESIAN_POINT ( 'NONE',  ( -8.224510206698948167, 14.34966873604960824, 35.41557627198102409 ) ) ;
#23968=CARTESIAN_POINT ( 'NONE',  ( -5.719274019375665041, -21.55341960407619695, 99.79275706135234714 ) ) ;
#23969=CARTESIAN_POINT ( 'NONE',  ( 8.314922557961029526, -14.29746914071037800, 60.41775706135235424 ) ) ;
#23970=CARTESIAN_POINT ( 'NONE',  ( 9.474510206698971260, -16.51473224551069308, 97.91557627198102409 ) ) ;
#23971=CARTESIAN_POINT ( 'NONE',  ( 16.46253265017160672, -9.564922557960803928, 33.33224293864770260 ) ) ;
#23973=CARTESIAN_POINT ( 'NONE',  ( -0.05219959533937732626, 21.53943276465977519, 42.50109039468567573 ) ) ;
#23974=CARTESIAN_POINT ( 'NONE',  ( 0.05219959533937995610, -21.53943276465977519, 60.00109039468568284 ) ) ;
#23975=CARTESIAN_POINT ( 'NONE',  ( 13.97604488694527802, 13.89961937509977652, 44.37390960531435269 ) ) ;
#23976=CARTESIAN_POINT ( 'NONE',  ( 21.55341960407619695, -5.719274019375665929, 41.04275706135236135 ) ) ;
#23977=CARTESIAN_POINT ( 'NONE',  ( 16.46253265017146816, 9.564922557961045513, 76.66775706135234714 ) ) ;
#23978=CARTESIAN_POINT ( 'NONE',  ( 19.03943276465977164, 0.05219959533936151252, 76.25109039468566152 ) ) ;
#23979=CARTESIAN_POINT ( 'NONE',  ( 19.03943276465977164, -0.05219959533909143690, 23.74890960531435269 ) ) ;
#23980=CARTESIAN_POINT ( 'NONE',  ( -0.05219959533934338120, 16.53943276465976808, 77.50109039468567573 ) ) ;
#23981=CARTESIAN_POINT ( 'NONE',  ( 5.049401038298161559, -19.05341960407611168, 57.70724293864769550 ) ) ;
#23983=CARTESIAN_POINT ( 'NONE',  ( 9.474510206698971260, -16.51473224551069308, 102.9155762719810241 ) ) ;
#23984=CARTESIAN_POINT ( 'NONE',  ( -13.89961937509977652, 13.97604488694528158, 40.62390960531435979 ) ) ;
#23985=CARTESIAN_POINT ( 'NONE',  ( 5.719274019375991003, -21.55341960407610458, 67.70724293864769550 ) ) ;
#23986=CARTESIAN_POINT ( 'NONE',  ( 8.314922557961029526, -14.29746914071037800, 65.41775706135234714 ) ) ;
#23987=CARTESIAN_POINT ( 'NONE',  ( 0.05219959533937995610, -21.53943276465977519, 110.0010903946856757 ) ) ;
#23988=CARTESIAN_POINT ( 'NONE',  ( 0.05219959533909260263, 19.03943276465977164, 49.99890960531435979 ) ) ;
#23989=CARTESIAN_POINT ( 'NONE',  ( -12.06949235617756955, 12.14591786802309770, 45.62390960531436690 ) ) ;
#23990=CARTESIAN_POINT ( 'NONE',  ( 16.55341960407611168, 4.379528057220329451, 83.95724293864770971 ) ) ;
#23991=CARTESIAN_POINT ( 'NONE',  ( -19.03943276465977164, 0.05219959533909376836, 81.24890960531436690 ) ) ;
#23992=CARTESIAN_POINT ( 'NONE',  ( -21.53943276465977519, -0.05219959533937600094, 38.75109039468567573 ) ) ;
#23993=CARTESIAN_POINT ( 'NONE',  ( 9.474510206698971260, -16.51473224551069308, 92.91557627198103830 ) ) ;
#23994=CARTESIAN_POINT ( 'NONE',  ( -10.72451020669870658, -18.67979575497194134, 99.58442372801900433 ) ) ;
#23995=CARTESIAN_POINT ( 'NONE',  ( -4.483927247898782831, 16.52544592524335698, 67.70942372801901854 ) ) ;
#23996=CARTESIAN_POINT ( 'NONE',  ( -13.97604488694527625, -13.89961937509977652, 101.8739096053143811 ) ) ;
#23997=CARTESIAN_POINT ( 'NONE',  ( -18.62759615963270932, 10.81492255796079327, 85.83224293864768129 ) ) ;
#23999=CARTESIAN_POINT ( 'NONE',  ( -8.314922557960811034, -14.29746914071050412, 47.08224293864770260 ) ) ;
#24000=CARTESIAN_POINT ( 'NONE',  ( 13.89961937509977652, -13.97604488694527269, 48.12390960531435979 ) ) ;
#24001=CARTESIAN_POINT ( 'NONE',  ( 12.06949235617739724, 12.14591786802326823, 51.87609039468568284 ) ) ;
#24002=CARTESIAN_POINT ( 'NONE',  ( -8.314922557960811034, -14.29746914071050412, 67.08224293864770971 ) ) ;
#24003=CARTESIAN_POINT ( 'NONE',  ( 16.46253265017160672, -9.564922557960803928, 108.3322429386476955 ) ) ;
#24004=CARTESIAN_POINT ( 'NONE',  ( 5.823673210054125526, 21.52544592524343514, 29.79057627198102409 ) ) ;
#24005=CARTESIAN_POINT ( 'NONE',  ( -16.46253265017146816, -9.564922557961047289, 29.16775706135232937 ) ) ;
#24006=CARTESIAN_POINT ( 'NONE',  ( -16.53943276465976808, 0.05219959533911058130, 101.2489096053143669 ) ) ;
#24007=CARTESIAN_POINT ( 'NONE',  ( 5.049401038298161559, -19.05341960407611168, 107.7072429386476955 ) ) ;
#24009=CARTESIAN_POINT ( 'NONE',  ( -16.55341960407617563, 4.379528057220093196, 58.54275706135235424 ) ) ;
#24010=CARTESIAN_POINT ( 'NONE',  ( 19.05341960407611168, 5.049401038298154454, 58.95724293864768129 ) ) ;
#24012=CARTESIAN_POINT ( 'NONE',  ( 5.049401038297881783, 19.05341960407617563, 57.29275706135231871 ) ) ;
#24014=CARTESIAN_POINT ( 'NONE',  ( 0.05219959533934541429, -16.53943276465976808, 95.00109039468568994 ) ) ;
#24015=CARTESIAN_POINT ( 'NONE',  ( 9.474510206698729675, 16.51473224551082808, 92.08442372801900433 ) ) ;
#24016=CARTESIAN_POINT ( 'NONE',  ( -10.72451020669870658, -18.67979575497194134, 64.58442372801900433 ) ) ;
#24017=CARTESIAN_POINT ( 'NONE',  ( -13.97604488694527625, -13.89961937509977652, 71.87390960531433848 ) ) ;
#24018=CARTESIAN_POINT ( 'NONE',  ( -5.719274019375978568, 21.55341960407610458, 90.20724293864770971 ) ) ;
#24019=CARTESIAN_POINT ( 'NONE',  ( -4.483927247898539470, -16.52544592524342804, 107.2905762719810525 ) ) ;
#24021=CARTESIAN_POINT ( 'NONE',  ( 19.02544592524334988, 5.153800228976608722, 81.45942372801897591 ) ) ;
#24022=CARTESIAN_POINT ( 'NONE',  ( -18.67979575497178146, -10.72451020669898902, 81.66557627198103830 ) ) ;
#24023=CARTESIAN_POINT ( 'NONE',  ( -9.474510206698720793, -16.51473224551083518, 44.58442372801900433 ) ) ;
#24024=CARTESIAN_POINT ( 'NONE',  ( 19.49671883438227837, 5.500000000000021316, 97.39279849105680853 ) ) ;
#24025=CARTESIAN_POINT ( 'NONE',  ( 21.55341960407610458, 5.719274019375980345, 93.95724293864770971 ) ) ;
#24027=CARTESIAN_POINT ( 'NONE',  ( 5.049401038298161559, -19.05341960407611168, 67.70724293864769550 ) ) ;
#24028=CARTESIAN_POINT ( 'NONE',  ( 30.00000000000000000, 5.499999999999992895, 102.5000000000000142 ) ) ;
#24029=CARTESIAN_POINT ( 'NONE',  ( -16.51473224551082808, 9.474510206698731452, 113.3344237280190043 ) ) ;
#24031=CARTESIAN_POINT ( 'NONE',  ( -16.51473224551069308, -9.474510206698971260, 51.66557627198102409 ) ) ;
#24032=CARTESIAN_POINT ( 'NONE',  ( 16.51473224551069308, 9.474510206698969483, 114.1655762719810241 ) ) ;
#24033=CARTESIAN_POINT ( 'NONE',  ( 5.823673210054125526, 21.52544592524343514, 99.79057627198103830 ) ) ;
#24034=CARTESIAN_POINT ( 'NONE',  ( -12.14591786802309592, -12.06949235617757132, 46.87390960531435979 ) ) ;
#24035=CARTESIAN_POINT ( 'NONE',  ( -0.05219959533937732626, 21.53943276465977519, 77.50109039468567573 ) ) ;
#24036=CARTESIAN_POINT ( 'NONE',  ( 4.483927247898790824, -16.52544592524335698, 30.20942372801902565 ) ) ;
#24037=CARTESIAN_POINT ( 'NONE',  ( -5.049401038297874678, -19.05341960407617918, 24.79275706135233648 ) ) ;
#24038=CARTESIAN_POINT ( 'NONE',  ( 16.55341960407611168, 4.379528057220329451, 23.95724293864769550 ) ) ;
#24039=CARTESIAN_POINT ( 'NONE',  ( -21.53943276465977519, -0.05219959533937600094, 38.75109039468567573 ) ) ;
#24040=CARTESIAN_POINT ( 'NONE',  ( 18.67979575497178502, 10.72451020669898547, 114.1655762719810383 ) ) ;
#24041=CARTESIAN_POINT ( 'NONE',  ( -5.719274019375978568, 21.55341960407610458, 60.20724293864768839 ) ) ;
#24042=CARTESIAN_POINT ( 'NONE',  ( -16.46253265017146816, -9.564922557961047289, 89.16775706135234714 ) ) ;
#24043=CARTESIAN_POINT ( 'NONE',  ( -0.05219959533936034679, 19.03943276465977164, 72.50109039468566152 ) ) ;
#24044=CARTESIAN_POINT ( 'NONE',  ( -10.72451020669870658, -18.67979575497194134, 74.58442372801901854 ) ) ;
#24045=CARTESIAN_POINT ( 'NONE',  ( -19.02544592524334988, -5.153800228976617603, 53.95942372801898301 ) ) ;
#24046=CARTESIAN_POINT ( 'NONE',  ( 12.14591786802309770, 12.06949235617756955, 114.3739096053143527 ) ) ;
#24047=CARTESIAN_POINT ( 'NONE',  ( 15.72974639402199770, -15.80617190586745480, 43.12390960531435269 ) ) ;
#24048=CARTESIAN_POINT ( 'NONE',  ( -12.06949235617756955, 12.14591786802309770, 45.62390960531436690 ) ) ;
#24049=CARTESIAN_POINT ( 'NONE',  ( -18.39443945427638383, 5.500000000000031086, 93.51745347608651571 ) ) ;
#24050=CARTESIAN_POINT ( 'NONE',  ( 15.80617190586769283, -15.72974639402175789, 110.6260903946857042 ) ) ;
#24051=CARTESIAN_POINT ( 'NONE',  ( 16.55341960407618274, -4.379528057220086978, 81.04275706135236135 ) ) ;
#24052=CARTESIAN_POINT ( 'NONE',  ( -4.483927247898539470, -16.52544592524342804, 37.29057627198102409 ) ) ;
#24053=CARTESIAN_POINT ( 'NONE',  ( 18.62759615963255655, 10.81492255796105972, 71.66775706135234714 ) ) ;
#24054=CARTESIAN_POINT ( 'NONE',  ( -21.53943276465977519, -0.05219959533937600094, 78.75109039468568994 ) ) ;
#24055=CARTESIAN_POINT ( 'NONE',  ( 0.05219959533907565091, 21.53943276465977519, 84.99890960531436690 ) ) ;
#24057=CARTESIAN_POINT ( 'NONE',  ( -9.564922557960796823, -16.46253265017161027, 32.08224293864769550 ) ) ;
#24058=CARTESIAN_POINT ( 'NONE',  ( -21.52544592524334988, -5.823673210054445271, 58.95942372801902565 ) ) ;
#24059=CARTESIAN_POINT ( 'NONE',  ( 19.05341960407611168, 5.049401038298154454, 38.95724293864767418 ) ) ;
#24060=CARTESIAN_POINT ( 'NONE',  ( 9.564922557960805705, 16.46253265017160317, 49.58224293864770260 ) ) ;
#24061=CARTESIAN_POINT ( 'NONE',  ( -4.379528057220328563, 16.55341960407611168, 95.20724293864769550 ) ) ;
#24062=CARTESIAN_POINT ( 'NONE',  ( 13.97604488694527802, 13.89961937509977652, 104.3739096053143385 ) ) ;
#24063=CARTESIAN_POINT ( 'NONE',  ( 4.483927247898545687, 16.52544592524342804, 39.79057627198103830 ) ) ;
#24064=CARTESIAN_POINT ( 'NONE',  ( -16.51473224551069308, -9.474510206698971260, 21.66557627198102765 ) ) ;
#24065=CARTESIAN_POINT ( 'NONE',  ( -5.823673210054116645, -21.52544592524344225, 82.29057627198103830 ) ) ;
#24066=CARTESIAN_POINT ( 'NONE',  ( -10.81492255796105439, 18.62759615963255655, 22.91775706135235069 ) ) ;
#24068=CARTESIAN_POINT ( 'NONE',  ( -16.55341960407617563, 4.379528057220093196, 28.54275706135234358 ) ) ;
#24069=CARTESIAN_POINT ( 'NONE',  ( -0.05219959533907301413, -21.53943276465977519, 72.49890960531435269 ) ) ;
#24070=CARTESIAN_POINT ( 'NONE',  ( 5.719274019375673035, 21.55341960407619339, 97.29275706135234714 ) ) ;
#24071=CARTESIAN_POINT ( 'NONE',  ( 13.89961937509977652, -13.97604488694527269, 78.12390960531433848 ) ) ;
#24072=CARTESIAN_POINT ( 'NONE',  ( 21.52544592524334988, 5.823673210054432836, 31.45942372801901854 ) ) ;
#24073=CARTESIAN_POINT ( 'NONE',  ( 9.564922557960805705, 16.46253265017160317, 109.5822429386476955 ) ) ;
#24074=CARTESIAN_POINT ( 'NONE',  ( 12.14591786802327356, -12.06949235617739191, 90.62609039468567573 ) ) ;
#24075=CARTESIAN_POINT ( 'NONE',  ( -21.53943276465977519, -0.05219959533937600094, 68.75109039468568994 ) ) ;
#24076=CARTESIAN_POINT ( 'NONE',  ( 18.62759615963255655, 10.81492255796105972, 111.6677570613523613 ) ) ;
#24077=CARTESIAN_POINT ( 'NONE',  ( -0.05219959533934338120, 16.53943276465976808, 77.50109039468567573 ) ) ;
#24078=CARTESIAN_POINT ( 'NONE',  ( -15.80617190586768217, 15.72974639402176855, 33.12609039468569705 ) ) ;
#24080=CARTESIAN_POINT ( 'NONE',  ( 5.049401038298161559, -19.05341960407611168, 37.70724293864768839 ) ) ;
#24081=CARTESIAN_POINT ( 'NONE',  ( 18.67979575497194134, -10.72451020669871369, 95.83442372801903275 ) ) ;
#24082=CARTESIAN_POINT ( 'NONE',  ( -16.46253265017160317, 9.564922557960807481, 90.83224293864769550 ) ) ;
#24083=CARTESIAN_POINT ( 'NONE',  ( -21.55341960407610458, -5.719274019375992779, 86.45724293864770971 ) ) ;
#24084=CARTESIAN_POINT ( 'NONE',  ( -19.02544592524334988, -5.153800228976617603, 53.95942372801898301 ) ) ;
#24086=CARTESIAN_POINT ( 'NONE',  ( 0.05219959533907565091, 21.53943276465977519, 54.99890960531435269 ) ) ;
#24087=CARTESIAN_POINT ( 'NONE',  ( -13.89961937509977652, 13.97604488694528158, 90.62390960531432427 ) ) ;
#24088=CARTESIAN_POINT ( 'NONE',  ( 8.314922557960818139, 14.29746914071049879, 44.58224293864769550 ) ) ;
#24090=CARTESIAN_POINT ( 'NONE',  ( 19.05341960407617918, -5.049401038297876454, 76.04275706135230450 ) ) ;
#24092=CARTESIAN_POINT ( 'NONE',  ( -17.50000000000000000, 5.622605283950888655, 103.6879268940388954 ) ) ;
#24093=CARTESIAN_POINT ( 'NONE',  ( -13.97604488694547697, 13.89961937509957934, 103.1260903946856473 ) ) ;
#24094=CARTESIAN_POINT ( 'NONE',  ( 5.823673210054125526, 21.52544592524343514, 84.79057627198102409 ) ) ;
#24095=CARTESIAN_POINT ( 'NONE',  ( 16.52544592524342804, -4.483927247898539470, 63.54057627198103830 ) ) ;
#24096=CARTESIAN_POINT ( 'NONE',  ( -5.049401038298153566, 19.05341960407611168, 105.2072429386476671 ) ) ;
#24097=CARTESIAN_POINT ( 'NONE',  ( -16.55341960407617563, 4.379528057220093196, 43.54275706135235424 ) ) ;
#24098=CARTESIAN_POINT ( 'NONE',  ( 19.02544592524343514, -5.153800228976328945, 53.54057627198102409 ) ) ;
#24099=CARTESIAN_POINT ( 'NONE',  ( -18.62759615963270932, 10.81492255796079327, 115.8322429386477097 ) ) ;
#24100=CARTESIAN_POINT ( 'NONE',  ( 19.03943276465977164, 0.05219959533936151252, 101.2510903946856757 ) ) ;
#24101=CARTESIAN_POINT ( 'NONE',  ( 13.89961937509977652, -13.97604488694527269, 98.12390960531433848 ) ) ;
#24102=CARTESIAN_POINT ( 'NONE',  ( 19.03943276465977164, -0.05219959533909143690, 78.74890960531436690 ) ) ;
#24103=CARTESIAN_POINT ( 'NONE',  ( -18.67979575497178146, -10.72451020669898902, 71.66557627198100988 ) ) ;
#24104=CARTESIAN_POINT ( 'NONE',  ( -13.97604488694527625, -13.89961937509977652, 51.87390960531436690 ) ) ;
#24106=CARTESIAN_POINT ( 'NONE',  ( 16.55341960407611168, 4.379528057220329451, 53.95724293864770260 ) ) ;
#24107=CARTESIAN_POINT ( 'NONE',  ( -16.46253265017160317, 9.564922557960807481, 100.8322429386477097 ) ) ;
#24109=CARTESIAN_POINT ( 'NONE',  ( 9.564922557961047289, -16.46253265017146816, 70.41775706135233293 ) ) ;
#24110=CARTESIAN_POINT ( 'NONE',  ( 10.81492255796078972, 18.62759615963270932, 94.58224293864769550 ) ) ;
#24111=CARTESIAN_POINT ( 'NONE',  ( 16.46253265017146816, 9.564922557961045513, 51.66775706135233293 ) ) ;
#24112=CARTESIAN_POINT ( 'NONE',  ( -13.89961937509977652, 13.97604488694528158, 95.62390960531436690 ) ) ;
#24113=SURFACE_STYLE_FILL_AREA ( #7922 ) ;
#24114=CARTESIAN_POINT ( 'NONE',  ( -18.67979575497178146, -10.72451020669898902, 36.66557627198103120 ) ) ;
#24116=CARTESIAN_POINT ( 'NONE',  ( 9.564922557960805705, 16.46253265017160317, 69.58224293864770971 ) ) ;
#24117=CARTESIAN_POINT ( 'NONE',  ( 15.80617190586769283, -15.72974639402175789, 65.62609039468568994 ) ) ;
#24118=CARTESIAN_POINT ( 'NONE',  ( 9.474510206698971260, -16.51473224551069308, 42.91557627198103120 ) ) ;
#24119=CARTESIAN_POINT ( 'NONE',  ( 14.29746914071049879, -8.314922557960816363, 78.33224293864770971 ) ) ;
#24121=CARTESIAN_POINT ( 'NONE',  ( 12.06949235617739724, 12.14591786802326823, 21.87609039468567573 ) ) ;
#24122=B_SPLINE_CURVE_WITH_KNOTS ( 'NONE', 3,
 ( #37000, #158360, #142189, #127011, #21845, #36003, #159339, #81489, #82493, #19848, #63368, #17877, #144176, #157377, #79531, #18870, #129000, #143176, #190698, #112844, #52173, #2690 ),
 .UNSPECIFIED., .F., .F.,
 ( 4, 2, 2, 2, 2, 2, 2, 2, 2, 2, 4 ),
 ( 8.673617379884035472E-19, 0.001309639967555459826, 0.001964459951333189305, 0.002291869943222054045, 0.002455574939166472754, 0.002619279935110891463, 0.002782984931055310605, 0.002946689926999729314, 0.003274099918888538976, 0.003928919902666159168, 0.005238559870221396950 ),
 .UNSPECIFIED. ) ;
#24123=CARTESIAN_POINT ( 'NONE',  ( 21.53943276465977519, 0.05219959533937863772, 46.25109039468567573 ) ) ;
#24125=CARTESIAN_POINT ( 'NONE',  ( -19.05341960407611168, -5.049401038298163336, 111.4572429386476671 ) ) ;
#24126=CARTESIAN_POINT ( 'NONE',  ( 16.46253265017146816, 9.564922557961045513, 66.66775706135233293 ) ) ;
#24128=CARTESIAN_POINT ( 'NONE',  ( 21.52544592524334988, 5.823673210054432836, 21.45942372801901499 ) ) ;
#24129=CARTESIAN_POINT ( 'NONE',  ( 5.153800228976335163, 19.02544592524342804, 54.79057627198103120 ) ) ;
#24132=CARTESIAN_POINT ( 'NONE',  ( 0.05219959533936267826, -19.03943276465977164, 25.00109039468566152 ) ) ;
#24133=CARTESIAN_POINT ( 'NONE',  ( 5.049401038298161559, -19.05341960407611168, 42.70724293864767418 ) ) ;
#24134=CARTESIAN_POINT ( 'NONE',  ( 5.153800228976615827, -19.02544592524334988, 20.20942372801899722 ) ) ;
#24135=CARTESIAN_POINT ( 'NONE',  ( 8.314922557961029526, -14.29746914071037800, 85.41775706135236135 ) ) ;
#24136=CARTESIAN_POINT ( 'NONE',  ( -19.03943276465977164, 0.05219959533909376836, 106.2489096053143669 ) ) ;
#24137=CARTESIAN_POINT ( 'NONE',  ( -10.72451020669870658, -18.67979575497194134, 69.58442372801900433 ) ) ;
#24139=CARTESIAN_POINT ( 'NONE',  ( -5.153800228976328057, -19.02544592524343514, 112.2905762719810099 ) ) ;
#24141=CARTESIAN_POINT ( 'NONE',  ( -4.483927247898782831, 16.52544592524335698, 67.70942372801901854 ) ) ;
#24142=CARTESIAN_POINT ( 'NONE',  ( -5.719274019375665041, -21.55341960407619695, 69.79275706135234714 ) ) ;
#24143=CARTESIAN_POINT ( 'NONE',  ( 18.62759615963255655, 10.81492255796105972, 106.6677570613523756 ) ) ;
#24145=CARTESIAN_POINT ( 'NONE',  ( 12.14591786802327356, -12.06949235617739191, 45.62609039468567573 ) ) ;
#24146=CARTESIAN_POINT ( 'NONE',  ( 13.89961937509977652, -13.97604488694527269, 88.12390960531438111 ) ) ;
#24147=CARTESIAN_POINT ( 'NONE',  ( -9.474510206698964154, 16.51473224551069663, 115.4155762719810241 ) ) ;
#24151=CARTESIAN_POINT ( 'NONE',  ( 5.153800228976335163, 19.02544592524342804, 39.79057627198100988 ) ) ;
#24152=CARTESIAN_POINT ( 'NONE',  ( 15.72974639402199770, -15.80617190586745480, 43.12390960531435269 ) ) ;
#24153=CARTESIAN_POINT ( 'NONE',  ( -4.483927247898782831, 16.52544592524335698, 112.7094237280190328 ) ) ;
#24154=CARTESIAN_POINT ( 'NONE',  ( -8.224510206698948167, 14.34966873604960824, 85.41557627198102409 ) ) ;
#24155=CARTESIAN_POINT ( 'NONE',  ( 9.564922557960805705, 16.46253265017160317, 84.58224293864769550 ) ) ;
#24156=CARTESIAN_POINT ( 'NONE',  ( 15.72974639402176855, 15.80617190586768217, 101.8760903946857042 ) ) ;
#24157=CARTESIAN_POINT ( 'NONE',  ( 8.314922557961029526, -14.29746914071037800, 30.41775706135234358 ) ) ;
#24158=CARTESIAN_POINT ( 'NONE',  ( 8.224510206698953496, -14.34966873604960469, 82.91557627198103830 ) ) ;
#24159=CARTESIAN_POINT ( 'NONE',  ( 5.719274019375673035, 21.55341960407619339, 42.29275706135235424 ) ) ;
#24160=CARTESIAN_POINT ( 'NONE',  ( -0.05219959533907301413, -21.53943276465977519, 82.49890960531436690 ) ) ;
#24161=CARTESIAN_POINT ( 'NONE',  ( -19.02544592524334988, -5.153800228976617603, 53.95942372801898301 ) ) ;
#24163=CARTESIAN_POINT ( 'NONE',  ( 0.05219959533909260263, 19.03943276465977164, 94.99890960531436690 ) ) ;
#24164=CARTESIAN_POINT ( 'NONE',  ( -14.34966873604960291, -8.224510206698953496, 66.66557627198102409 ) ) ;
#24165=CARTESIAN_POINT ( 'NONE',  ( 16.52544592524342804, -4.483927247898539470, 48.54057627198103120 ) ) ;
#24166=CARTESIAN_POINT ( 'NONE',  ( 14.29746914071049879, -8.314922557960816363, 28.33224293864769550 ) ) ;
#24167=CARTESIAN_POINT ( 'NONE',  ( 19.05341960407617918, -5.049401038297876454, 76.04275706135230450 ) ) ;
#24169=CARTESIAN_POINT ( 'NONE',  ( 19.03943276465977164, -0.05219959533909143690, 113.7489096053143669 ) ) ;
#24170=CARTESIAN_POINT ( 'NONE',  ( -12.14591786802309592, -12.06949235617757132, 86.87390960531438111 ) ) ;
#24171=CARTESIAN_POINT ( 'NONE',  ( -17.50000000000147438, -3.254303733634695384, 24.97604106928582013 ) ) ;
#24172=CARTESIAN_POINT ( 'NONE',  ( 19.03943276465977164, -0.05219959533909143690, 43.74890960531435979 ) ) ;
#24173=CARTESIAN_POINT ( 'NONE',  ( 10.72451020669898902, -18.67979575497178502, 42.91557627198103120 ) ) ;
#24174=CARTESIAN_POINT ( 'NONE',  ( 13.97604488694527802, 13.89961937509977652, 29.37390960531435979 ) ) ;
#24175=CARTESIAN_POINT ( 'NONE',  ( 4.379528057220092307, 16.55341960407617563, 82.29275706135234714 ) ) ;
#24176=CARTESIAN_POINT ( 'NONE',  ( 13.97604488694527802, 13.89961937509977652, 59.37390960531434558 ) ) ;
#24177=CARTESIAN_POINT ( 'NONE',  ( -16.51473224551082808, 9.474510206698731452, 38.33442372801899722 ) ) ;
#24179=CARTESIAN_POINT ( 'NONE',  ( -21.52544592524334988, -5.823673210054445271, 53.95942372801900433 ) ) ;
#24180=CARTESIAN_POINT ( 'NONE',  ( 15.72974639402199770, -15.80617190586745480, 33.12390960531435979 ) ) ;
#24181=CARTESIAN_POINT ( 'NONE',  ( -4.483927247898539470, -16.52544592524342804, 107.2905762719810525 ) ) ;
#24182=CARTESIAN_POINT ( 'NONE',  ( 19.02544592524334988, 5.153800228976608722, 91.45942372801900433 ) ) ;
#24184=CARTESIAN_POINT ( 'NONE',  ( 17.50000000000004263, 3.926509638708173711, 37.08294989138502729 ) ) ;
#24185=CARTESIAN_POINT ( 'NONE',  ( -10.81492255796078084, -18.62759615963271287, 52.08224293864768839 ) ) ;
#24186=CARTESIAN_POINT ( 'NONE',  ( 17.26172910966779739, -6.454744622555849354, 68.30646908649225679 ) ) ;
#24187=CARTESIAN_POINT ( 'NONE',  ( 21.53943276465977519, 0.05219959533937863772, 86.25109039468568994 ) ) ;
#24188=CARTESIAN_POINT ( 'NONE',  ( 16.53943276465976808, -0.05219959533910856209, 43.74890960531435979 ) ) ;
#24189=CARTESIAN_POINT ( 'NONE',  ( -14.29746914071037622, -8.314922557961029526, 54.16775706135235424 ) ) ;
#24190=CARTESIAN_POINT ( 'NONE',  ( -4.483927247898539470, -16.52544592524342804, 57.29057627198103120 ) ) ;
#24191=CARTESIAN_POINT ( 'NONE',  ( -15.80617190586745835, -15.72974639402198527, 81.87390960531435269 ) ) ;
#24192=CARTESIAN_POINT ( 'NONE',  ( -15.80617190586745835, -15.72974639402198527, 71.87390960531438111 ) ) ;
#24194=CARTESIAN_POINT ( 'NONE',  ( 19.03943276465977164, -0.05219959533909143690, 108.7489096053143527 ) ) ;
#24195=CARTESIAN_POINT ( 'NONE',  ( -16.51473224551069308, -9.474510206698971260, 56.66557627198103120 ) ) ;
#24196=CARTESIAN_POINT ( 'NONE',  ( 13.97604488694527802, 13.89961937509977652, 29.37390960531435979 ) ) ;
#24199=CIRCLE ( 'NONE', #8003, 2.000000000000000000 ) ;
#24200=CARTESIAN_POINT ( 'NONE',  ( 12.06949235617739724, 12.14591786802326823, 86.87609039468568994 ) ) ;
#24201=CARTESIAN_POINT ( 'NONE',  ( 5.823673210054444382, -21.52544592524334988, 20.20942372801900788 ) ) ;
#24202=CARTESIAN_POINT ( 'NONE',  ( 13.97604488694527802, 13.89961937509977652, 69.37390960531436690 ) ) ;
#24203=CARTESIAN_POINT ( 'NONE',  ( 15.72974639402176855, 15.80617190586768217, 56.87609039468568994 ) ) ;
#24204=CARTESIAN_POINT ( 'NONE',  ( 9.564922557960805705, 16.46253265017160317, 114.5822429386476955 ) ) ;
#24207=CARTESIAN_POINT ( 'NONE',  ( 15.80617190586769283, -15.72974639402175789, 50.62609039468568994 ) ) ;
#24208=CARTESIAN_POINT ( 'NONE',  ( 19.05341960407611168, 5.049401038298154454, 113.9572429386477097 ) ) ;
#24209=CARTESIAN_POINT ( 'NONE',  ( -19.02544592524342804, 5.153800228976336051, 106.0405762719810241 ) ) ;
#24210=CARTESIAN_POINT ( 'NONE',  ( 0.05219959533936267826, -19.03943276465977164, 50.00109039468566863 ) ) ;
#24211=CARTESIAN_POINT ( 'NONE',  ( -5.823673210054116645, -21.52544592524344225, 107.2905762719810525 ) ) ;
#24212=CARTESIAN_POINT ( 'NONE',  ( 19.02544592524334988, 5.153800228976608722, 51.45942372801900433 ) ) ;
#24213=CARTESIAN_POINT ( 'NONE',  ( -9.474510206698720793, -16.51473224551083518, 54.58442372801899722 ) ) ;
#24214=CARTESIAN_POINT ( 'NONE',  ( 16.55341960407618274, -4.379528057220086978, 111.0427570613523613 ) ) ;
#24217=CARTESIAN_POINT ( 'NONE',  ( 16.46253265017160672, -9.564922557960803928, 73.33224293864769550 ) ) ;
#24219=CARTESIAN_POINT ( 'NONE',  ( -21.53943276465977519, -0.05219959533937600094, 78.75109039468568994 ) ) ;
#24220=CARTESIAN_POINT ( 'NONE',  ( -5.823673210054431948, 21.52544592524334988, 87.70942372801901854 ) ) ;
#24222=CARTESIAN_POINT ( 'NONE',  ( -16.51473224551069308, -9.474510206698971260, 106.6655762719810383 ) ) ;
#24223=CARTESIAN_POINT ( 'NONE',  ( 18.62759615963255655, 10.81492255796105972, 76.66775706135234714 ) ) ;
#24224=CARTESIAN_POINT ( 'NONE',  ( -14.34966873604972548, 8.224510206698743886, 23.33442372801901499 ) ) ;
#24225=CARTESIAN_POINT ( 'NONE',  ( 13.89961937509977652, -13.97604488694527269, 83.12390960531436690 ) ) ;
#24226=CARTESIAN_POINT ( 'NONE',  ( -19.03943276465977164, 0.05219959533909376836, 116.2489096053143669 ) ) ;
#24227=CARTESIAN_POINT ( 'NONE',  ( 9.564922557960805705, 16.46253265017160317, 89.58224293864769550 ) ) ;
#24228=CARTESIAN_POINT ( 'NONE',  ( -17.59860650958993844, 7.585241751806885979, 88.42337014262494677 ) ) ;
#24229=CARTESIAN_POINT ( 'NONE',  ( -13.89961937509977652, 13.97604488694528158, 80.62390960531436690 ) ) ;
#24230=CARTESIAN_POINT ( 'NONE',  ( -16.51473224551069308, -9.474510206698971260, 61.66557627198103120 ) ) ;
#24231=CARTESIAN_POINT ( 'NONE',  ( 21.53943276465977519, -0.05219959533907433946, 113.7489096053143527 ) ) ;
#24232=CARTESIAN_POINT ( 'NONE',  ( -14.34966873604972548, 8.224510206698743886, 103.3344237280190043 ) ) ;
#24234=VECTOR ( 'NONE', #7822, 1000.000000000000000 ) ;
#24235=CARTESIAN_POINT ( 'NONE',  ( -19.05341960407617563, 5.049401038297882671, 53.54275706135231871 ) ) ;
#24236=CARTESIAN_POINT ( 'NONE',  ( -9.564922557960796823, -16.46253265017161027, 92.08224293864769550 ) ) ;
#24237=CARTESIAN_POINT ( 'NONE',  ( -12.06949235617756955, 12.14591786802309770, 85.62390960531436690 ) ) ;
#24238=CARTESIAN_POINT ( 'NONE',  ( -5.049401038298153566, 19.05341960407611168, 30.20724293864768839 ) ) ;
#24239=CONICAL_SURFACE ( 'NONE', #169549, 2.500000000000002220, 1.029744260000000189 ) ;
#24240=CARTESIAN_POINT ( 'NONE',  ( 0.05219959533907565091, 21.53943276465977519, 34.99890960531435979 ) ) ;
#24241=CARTESIAN_POINT ( 'NONE',  ( 0.05219959533907565091, 21.53943276465977519, 29.99890960531435979 ) ) ;
#24242=CARTESIAN_POINT ( 'NONE',  ( -12.14591786802309592, -12.06949235617757132, 96.87390960531436690 ) ) ;
#24244=CARTESIAN_POINT ( 'NONE',  ( -13.89961937509957401, -13.97604488694547875, 49.37609039468567573 ) ) ;
#24245=CARTESIAN_POINT ( 'NONE',  ( -14.34966873604972548, 8.224510206698743886, 108.3344237280190185 ) ) ;
#24246=CARTESIAN_POINT ( 'NONE',  ( 19.02544592524343514, -5.153800228976328945, 83.54057627198100988 ) ) ;
#24247=CARTESIAN_POINT ( 'NONE',  ( -18.62759615963255300, -10.81492255796106328, 64.16775706135234714 ) ) ;
#24248=CARTESIAN_POINT ( 'NONE',  ( -10.81492255796078084, -18.62759615963271287, 57.08224293864769550 ) ) ;
#24249=CARTESIAN_POINT ( 'NONE',  ( -21.52544592524334988, -5.823673210054445271, 28.95942372801902209 ) ) ;
#24250=CARTESIAN_POINT ( 'NONE',  ( 10.81492255796078972, 18.62759615963270932, 84.58224293864769550 ) ) ;
#24251=CARTESIAN_POINT ( 'NONE',  ( -4.379528057220328563, 16.55341960407611168, 110.2072429386477239 ) ) ;
#24252=CARTESIAN_POINT ( 'NONE',  ( -19.02544592524334988, -5.153800228976617603, 73.95942372801900433 ) ) ;
#24253=CARTESIAN_POINT ( 'NONE',  ( -19.02544592524342804, 5.153800228976336051, 51.04057627198103120 ) ) ;
#24254=CARTESIAN_POINT ( 'NONE',  ( 13.89961937509977652, -13.97604488694527269, 93.12390960531436690 ) ) ;
#24255=CARTESIAN_POINT ( 'NONE',  ( 19.02544592524343514, -5.153800228976328945, 88.54057627198102409 ) ) ;
#24256=CARTESIAN_POINT ( 'NONE',  ( 16.51473224551069308, 9.474510206698969483, 24.16557627198102765 ) ) ;
#24257=CARTESIAN_POINT ( 'NONE',  ( -0.05219959533910754901, -16.53943276465976808, 47.49890960531435979 ) ) ;
#24258=CARTESIAN_POINT ( 'NONE',  ( 12.14591786802327356, -12.06949235617739191, 40.62609039468567573 ) ) ;
#24259=CARTESIAN_POINT ( 'NONE',  ( 18.67979575497194134, -10.72451020669871369, 110.8344237280190043 ) ) ;
#24261=CARTESIAN_POINT ( 'NONE',  ( 0.05219959533909260263, 19.03943276465977164, 114.9989096053143669 ) ) ;
#24262=CARTESIAN_POINT ( 'NONE',  ( 16.53943276465976808, -0.05219959533910856209, 28.74890960531435624 ) ) ;
#24263=CARTESIAN_POINT ( 'NONE',  ( -10.81492255796105439, 18.62759615963255655, 27.91775706135234358 ) ) ;
#24264=CARTESIAN_POINT ( 'NONE',  ( 19.03943276465977164, -0.05219959533909143690, 108.7489096053143527 ) ) ;
#24265=CARTESIAN_POINT ( 'NONE',  ( -8.224510206698735004, -14.34966873604973081, 109.5844237280190328 ) ) ;
#24266=CARTESIAN_POINT ( 'NONE',  ( 16.55341960407618274, -4.379528057220086978, 96.04275706135236135 ) ) ;
#24267=CARTESIAN_POINT ( 'NONE',  ( 8.314922557961029526, -14.29746914071037800, 25.41775706135235779 ) ) ;
#24268=CARTESIAN_POINT ( 'NONE',  ( 5.153800228976335163, 19.02544592524342804, 44.79057627198103830 ) ) ;
#24269=CARTESIAN_POINT ( 'NONE',  ( 14.34966873604960469, 8.224510206698951720, 114.1655762719810383 ) ) ;
#24270=CARTESIAN_POINT ( 'NONE',  ( -15.72974639402176322, -15.80617190586768395, 24.37609039468567573 ) ) ;
#24271=CARTESIAN_POINT ( 'NONE',  ( -5.153800228976328057, -19.02544592524343514, 37.29057627198102409 ) ) ;
#24272=CARTESIAN_POINT ( 'NONE',  ( 19.05341960407611168, 5.049401038298154454, 103.9572429386476671 ) ) ;
#24273=CARTESIAN_POINT ( 'NONE',  ( 5.823673210054444382, -21.52544592524334988, 35.20942372801901854 ) ) ;
#24274=CARTESIAN_POINT ( 'NONE',  ( 0.05219959533909260263, 19.03943276465977164, 29.99890960531435979 ) ) ;
#24275=CARTESIAN_POINT ( 'NONE',  ( 16.46253265017160672, -9.564922557960803928, 108.3322429386476955 ) ) ;
#24277=CARTESIAN_POINT ( 'NONE',  ( 9.474510206698971260, -16.51473224551069308, 102.9155762719810241 ) ) ;
#24278=CARTESIAN_POINT ( 'NONE',  ( 15.80617190586769283, -15.72974639402175789, 45.62609039468567573 ) ) ;
#24279=CARTESIAN_POINT ( 'NONE',  ( -0.05219959533910754901, -16.53943276465976808, 97.49890960531436690 ) ) ;
#24280=CARTESIAN_POINT ( 'NONE',  ( 13.97604488694527802, 13.89961937509977652, 99.37390960531436690 ) ) ;
#24282=CARTESIAN_POINT ( 'NONE',  ( -12.06949235617739369, -12.14591786802326823, 69.37609039468567573 ) ) ;
#24283=CARTESIAN_POINT ( 'NONE',  ( 21.52544592524334988, 5.823673210054432836, 81.45942372801900433 ) ) ;
#24284=CARTESIAN_POINT ( 'NONE',  ( -16.53943276465976808, -0.05219959533934237506, 38.75109039468567573 ) ) ;
#24285=CARTESIAN_POINT ( 'NONE',  ( 19.05341960407611168, 5.049401038298154454, 78.95724293864769550 ) ) ;
#24286=CARTESIAN_POINT ( 'NONE',  ( -9.564922557961040184, 16.46253265017147172, 107.9177570613523471 ) ) ;
#24287=CARTESIAN_POINT ( 'NONE',  ( 0.05219959533934541429, -16.53943276465976808, 80.00109039468568994 ) ) ;
#24288=CARTESIAN_POINT ( 'NONE',  ( -9.564922557961040184, 16.46253265017147172, 92.91775706135233293 ) ) ;
#24289=CARTESIAN_POINT ( 'NONE',  ( -19.02544592524342804, 5.153800228976336051, 61.04057627198103120 ) ) ;
#24290=CARTESIAN_POINT ( 'NONE',  ( 15.72974639402199770, -15.80617190586745480, 78.12390960531436690 ) ) ;
#24291=CARTESIAN_POINT ( 'NONE',  ( -16.53943276465976808, 0.05219959533911058130, 86.24890960531436690 ) ) ;
#24292=CARTESIAN_POINT ( 'NONE',  ( 0.05219959533936267826, -19.03943276465977164, 90.00109039468567573 ) ) ;
#24293=CARTESIAN_POINT ( 'NONE',  ( 4.483927247898790824, -16.52544592524335698, 55.20942372801902565 ) ) ;
#24294=CARTESIAN_POINT ( 'NONE',  ( 17.50000000000002132, -5.624438216177543914, 63.31670344914647330 ) ) ;
#24295=CARTESIAN_POINT ( 'NONE',  ( 13.97604488694548053, -13.89961937509957401, 55.62609039468566863 ) ) ;
#24297=CARTESIAN_POINT ( 'NONE',  ( -0.05219959533910754901, -16.53943276465976808, 37.49890960531436690 ) ) ;
#24298=CARTESIAN_POINT ( 'NONE',  ( -8.224510206698948167, 14.34966873604960824, 85.41557627198102409 ) ) ;
#24299=CARTESIAN_POINT ( 'NONE',  ( 15.80617190586769283, -15.72974639402175789, 110.6260903946857042 ) ) ;
#24300=CARTESIAN_POINT ( 'NONE',  ( -16.21995358207276539, 7.366697692864364377, 39.93551001512066989 ) ) ;
#24301=CARTESIAN_POINT ( 'NONE',  ( -5.719274019375665041, -21.55341960407619695, 24.79275706135235779 ) ) ;
#24302=CARTESIAN_POINT ( 'NONE',  ( 9.564922557960805705, 16.46253265017160317, 109.5822429386476955 ) ) ;
#24303=CARTESIAN_POINT ( 'NONE',  ( 16.46253265017160672, -9.564922557960803928, 83.33224293864768129 ) ) ;
#24304=CARTESIAN_POINT ( 'NONE',  ( -21.53943276465977519, -0.05219959533937600094, 98.75109039468568994 ) ) ;
#24305=CARTESIAN_POINT ( 'NONE',  ( -0.05219959533909027116, -19.03943276465977164, 77.49890960531435269 ) ) ;
#24306=CARTESIAN_POINT ( 'NONE',  ( -0.05219959533907301413, -21.53943276465977519, 42.49890960531435979 ) ) ;
#24307=CARTESIAN_POINT ( 'NONE',  ( 14.29746914071049879, -8.314922557960816363, 83.33224293864769550 ) ) ;
#24308=CARTESIAN_POINT ( 'NONE',  ( 19.02544592524343514, -5.153800228976328945, 63.54057627198103830 ) ) ;
#24309=CARTESIAN_POINT ( 'NONE',  ( 16.52544592524342804, -4.483927247898539470, 113.5405762719810383 ) ) ;
#24310=CARTESIAN_POINT ( 'NONE',  ( 21.53943276465977519, 0.05219959533937863772, 26.25109039468567573 ) ) ;
#24311=CARTESIAN_POINT ( 'NONE',  ( 5.719274019375673035, 21.55341960407619339, 67.29275706135234714 ) ) ;
#24312=CARTESIAN_POINT ( 'NONE',  ( 19.05341960407611168, 5.049401038298154454, 43.95724293864769550 ) ) ;
#24313=CARTESIAN_POINT ( 'NONE',  ( -12.14591786802326823, 12.06949235617739902, 58.12609039468568994 ) ) ;
#24314=CARTESIAN_POINT ( 'NONE',  ( -0.05219959533937732626, 21.53943276465977519, 22.50109039468567573 ) ) ;
#24315=CARTESIAN_POINT ( 'NONE',  ( 21.52544592524344225, -5.823673210054117533, 113.5405762719810383 ) ) ;
#24316=CARTESIAN_POINT ( 'NONE',  ( -16.51473224551082808, 9.474510206698731452, 33.33442372801899722 ) ) ;
#24317=CARTESIAN_POINT ( 'NONE',  ( 5.153800228976335163, 19.02544592524342804, 69.79057627198103830 ) ) ;
#24319=CARTESIAN_POINT ( 'NONE',  ( 10.72451020669871369, 18.67979575497193778, 67.08442372801901854 ) ) ;
#24320=CARTESIAN_POINT ( 'NONE',  ( 21.55341960407610458, 5.719274019375980345, 58.95724293864770971 ) ) ;
#24321=CARTESIAN_POINT ( 'NONE',  ( -12.14591786802309592, -12.06949235617757132, 41.87390960531435979 ) ) ;
#24322=CARTESIAN_POINT ( 'NONE',  ( -15.72974639402176322, -15.80617190586768395, 74.37609039468568994 ) ) ;
#24323=CARTESIAN_POINT ( 'NONE',  ( -10.72451020669870658, -18.67979575497194134, 104.5844237280190185 ) ) ;
#24324=CARTESIAN_POINT ( 'NONE',  ( -12.06949235617756955, 12.14591786802309770, 55.62390960531436690 ) ) ;
#24325=CARTESIAN_POINT ( 'NONE',  ( 4.483927247898545687, 16.52544592524342804, 99.79057627198103830 ) ) ;
#24326=CARTESIAN_POINT ( 'NONE',  ( 19.02544592524334988, 5.153800228976608722, 56.45942372801898301 ) ) ;
#24327=CARTESIAN_POINT ( 'NONE',  ( -12.06949235617756955, 12.14591786802309770, 25.62390960531435624 ) ) ;
#24328=CARTESIAN_POINT ( 'NONE',  ( -0.05219959533937732626, 21.53943276465977519, 62.50109039468568284 ) ) ;
#24329=CARTESIAN_POINT ( 'NONE',  ( 5.153800228976335163, 19.02544592524342804, 69.79057627198103830 ) ) ;
#24330=CARTESIAN_POINT ( 'NONE',  ( -16.46253265017146816, -9.564922557961047289, 29.16775706135232937 ) ) ;
#24331=CARTESIAN_POINT ( 'NONE',  ( 10.72451020669898902, -18.67979575497178502, 32.91557627198102409 ) ) ;
#24332=CARTESIAN_POINT ( 'NONE',  ( -5.719274019375665041, -21.55341960407619695, 49.79275706135234714 ) ) ;
#24333=CARTESIAN_POINT ( 'NONE',  ( 5.719274019375991003, -21.55341960407610458, 97.70724293864772392 ) ) ;
#24334=CARTESIAN_POINT ( 'NONE',  ( -16.51473224551082808, 9.474510206698731452, 103.3344237280190043 ) ) ;
#24335=CARTESIAN_POINT ( 'NONE',  ( -16.53943276465976808, -0.05219959533934237506, 58.75109039468568994 ) ) ;
#24336=CARTESIAN_POINT ( 'NONE',  ( -18.09805431107246676, 5.500000000000103029, 56.01606229291885342 ) ) ;
#24337=CARTESIAN_POINT ( 'NONE',  ( -18.67979575497178146, -10.72451020669898902, 91.66557627198103830 ) ) ;
#24338=CARTESIAN_POINT ( 'NONE',  ( 4.483927247898545687, 16.52544592524342804, 89.79057627198103830 ) ) ;
#24339=CARTESIAN_POINT ( 'NONE',  ( 18.22780087662126647, 5.499999999999818812, 41.48236817873107185 ) ) ;
#24340=CARTESIAN_POINT ( 'NONE',  ( -4.379528057220086978, -16.55341960407618274, 24.79275706135235779 ) ) ;
#24341=CARTESIAN_POINT ( 'NONE',  ( 5.823673210054125526, 21.52544592524343514, 54.79057627198104541 ) ) ;
#24342=CARTESIAN_POINT ( 'NONE',  ( -16.55341960407617563, 4.379528057220093196, 93.54275706135234714 ) ) ;
#24343=CARTESIAN_POINT ( 'NONE',  ( 9.474510206698971260, -16.51473224551069308, 22.91557627198102765 ) ) ;
#24344=CARTESIAN_POINT ( 'NONE',  ( -12.14591786802326823, 12.06949235617739902, 53.12609039468568284 ) ) ;
#24345=CARTESIAN_POINT ( 'NONE',  ( -18.67979575497193778, 10.72451020669871902, 28.33442372801902209 ) ) ;
#24346=CARTESIAN_POINT ( 'NONE',  ( 10.81492255796078972, 18.62759615963270932, 44.58224293864769550 ) ) ;
#24347=CARTESIAN_POINT ( 'NONE',  ( -16.53943276465976808, -0.05219959533934237506, 78.75109039468568994 ) ) ;
#24348=CARTESIAN_POINT ( 'NONE',  ( -9.564922557960796823, -16.46253265017161027, 102.0822429386477097 ) ) ;
#24349=CARTESIAN_POINT ( 'NONE',  ( 15.80617190586769283, -15.72974639402175789, 75.62609039468567573 ) ) ;
#24350=CARTESIAN_POINT ( 'NONE',  ( 5.719274019375991003, -21.55341960407610458, 42.70724293864770260 ) ) ;
#24351=CARTESIAN_POINT ( 'NONE',  ( 19.05341960407611168, 5.049401038298154454, 113.9572429386477097 ) ) ;
#24353=CARTESIAN_POINT ( 'NONE',  ( -19.03943276465977164, -0.05219959533935918106, 48.75109039468566863 ) ) ;
#24354=CARTESIAN_POINT ( 'NONE',  ( 12.14591786802327356, -12.06949235617739191, 65.62609039468568994 ) ) ;
#24355=CARTESIAN_POINT ( 'NONE',  ( -15.80617190586745835, -15.72974639402198527, 36.87390960531435979 ) ) ;
#24357=CARTESIAN_POINT ( 'NONE',  ( -9.564922557960796823, -16.46253265017161027, 92.08224293864769550 ) ) ;
#24358=CARTESIAN_POINT ( 'NONE',  ( 4.483927247898790824, -16.52544592524335698, 110.2094237280190185 ) ) ;
#24360=CARTESIAN_POINT ( 'NONE',  ( -4.483927247898539470, -16.52544592524342804, 107.2905762719810525 ) ) ;
#24361=CARTESIAN_POINT ( 'NONE',  ( -21.55341960407610458, -5.719274019375992779, 51.45724293864770260 ) ) ;
#24362=CARTESIAN_POINT ( 'NONE',  ( 5.049401038298161559, -19.05341960407611168, 42.70724293864767418 ) ) ;
#24363=CARTESIAN_POINT ( 'NONE',  ( 4.379528057220092307, 16.55341960407617563, 82.29275706135234714 ) ) ;
#24364=CARTESIAN_POINT ( 'NONE',  ( 15.72974639402176855, 15.80617190586768217, 36.87609039468568994 ) ) ;
#24365=CARTESIAN_POINT ( 'NONE',  ( 16.46253265017146816, 9.564922557961045513, 91.66775706135234714 ) ) ;
#24366=CARTESIAN_POINT ( 'NONE',  ( 14.29746914071049879, -8.314922557960816363, 83.33224293864769550 ) ) ;
#24367=CARTESIAN_POINT ( 'NONE',  ( -5.049401038298153566, 19.05341960407611168, 50.20724293864770260 ) ) ;
#24369=CARTESIAN_POINT ( 'NONE',  ( -5.049401038298153566, 19.05341960407611168, 30.20724293864768839 ) ) ;
#24370=CARTESIAN_POINT ( 'NONE',  ( 18.67979575497194134, -10.72451020669871369, 110.8344237280190043 ) ) ;
#24371=CARTESIAN_POINT ( 'NONE',  ( -19.03943276465977164, 0.05219959533909376836, 76.24890960531435269 ) ) ;
#24372=CARTESIAN_POINT ( 'NONE',  ( -16.55341960407617563, 4.379528057220093196, 63.54275706135234003 ) ) ;
#24373=CARTESIAN_POINT ( 'NONE',  ( -0.05219959533937732626, 21.53943276465977519, 97.50109039468567573 ) ) ;
#24374=CARTESIAN_POINT ( 'NONE',  ( 10.72451020669898902, -18.67979575497178502, 52.91557627198103830 ) ) ;
#24375=CARTESIAN_POINT ( 'NONE',  ( 14.34966873604972726, -8.224510206698740333, 75.83442372801900433 ) ) ;
#24376=CARTESIAN_POINT ( 'NONE',  ( 19.03943276465977164, 0.05219959533936151252, 56.25109039468566863 ) ) ;
#24377=CARTESIAN_POINT ( 'NONE',  ( 5.049401038297881783, 19.05341960407617563, 67.29275706135234714 ) ) ;
#24379=CARTESIAN_POINT ( 'NONE',  ( 18.62759615963255655, 10.81492255796105972, 66.66775706135234714 ) ) ;
#24380=CARTESIAN_POINT ( 'NONE',  ( 9.564922557960805705, 16.46253265017160317, 69.58224293864770971 ) ) ;
#24381=CARTESIAN_POINT ( 'NONE',  ( 16.46253265017160672, -9.564922557960803928, 23.33224293864769194 ) ) ;
#24382=CARTESIAN_POINT ( 'NONE',  ( 19.05341960407617918, -5.049401038297876454, 66.04275706135233293 ) ) ;
#24383=CARTESIAN_POINT ( 'NONE',  ( 16.46253265017160672, -9.564922557960803928, 113.3322429386476955 ) ) ;
#24384=CARTESIAN_POINT ( 'NONE',  ( -13.97604488694527625, -13.89961937509977652, 81.87390960531436690 ) ) ;
#24385=CARTESIAN_POINT ( 'NONE',  ( -4.483927247898539470, -16.52544592524342804, 32.29057627198102409 ) ) ;
#24386=CARTESIAN_POINT ( 'NONE',  ( 18.62759615963271287, -10.81492255796078972, 48.33224293864770260 ) ) ;
#24389=CARTESIAN_POINT ( 'NONE',  ( -0.05219959533937732626, 21.53943276465977519, 107.5010903946856899 ) ) ;
#24391=CARTESIAN_POINT ( 'NONE',  ( 16.46253265017160672, -9.564922557960803928, 53.33224293864768839 ) ) ;
#24392=CARTESIAN_POINT ( 'NONE',  ( -13.97604488694527625, -13.89961937509977652, 26.87390960531434558 ) ) ;
#24395=CARTESIAN_POINT ( 'NONE',  ( -8.314922557961024197, 14.29746914071037800, 57.91775706135234714 ) ) ;
#24396=CARTESIAN_POINT ( 'NONE',  ( -18.67979575497178146, -10.72451020669898902, 76.66557627198103830 ) ) ;
#24397=CARTESIAN_POINT ( 'NONE',  ( 0.05219959533910956823, 16.53943276465976808, 59.99890960531436690 ) ) ;
#24398=CARTESIAN_POINT ( 'NONE',  ( 0.05219959533909260263, 19.03943276465977164, 24.99890960531435269 ) ) ;
#24400=CARTESIAN_POINT ( 'NONE',  ( 21.53943276465977519, 0.05219959533937863772, 41.25109039468568284 ) ) ;
#24401=CARTESIAN_POINT ( 'NONE',  ( -5.049401038297874678, -19.05341960407617918, 49.79275706135231871 ) ) ;
#24402=CARTESIAN_POINT ( 'NONE',  ( 16.51473224551069308, 9.474510206698969483, 29.16557627198103475 ) ) ;
#24403=CARTESIAN_POINT ( 'NONE',  ( -15.80617190586768217, 15.72974639402176855, 83.12609039468568994 ) ) ;
#24404=CARTESIAN_POINT ( 'NONE',  ( 16.19135201231366850, 7.376712067591940425, 97.68680854052031748 ) ) ;
#24405=CARTESIAN_POINT ( 'NONE',  ( -16.55341960407611168, -4.379528057220339221, 41.45724293864769550 ) ) ;
#24407=CARTESIAN_POINT ( 'NONE',  ( 0.05219959533907565091, 21.53943276465977519, 44.99890960531435979 ) ) ;
#24409=CARTESIAN_POINT ( 'NONE',  ( 13.89961937509977652, -13.97604488694527269, 88.12390960531438111 ) ) ;
#24410=CARTESIAN_POINT ( 'NONE',  ( 0.05219959533910956823, 16.53943276465976808, 89.99890960531438111 ) ) ;
#24411=CARTESIAN_POINT ( 'NONE',  ( -12.14591786802326823, 12.06949235617739902, 23.12609039468567573 ) ) ;
#24412=CARTESIAN_POINT ( 'NONE',  ( 15.72974639402199770, -15.80617190586745480, 63.12390960531435979 ) ) ;
#24414=CARTESIAN_POINT ( 'NONE',  ( 16.51473224551069308, 9.474510206698969483, 39.16557627198103120 ) ) ;
#24415=CARTESIAN_POINT ( 'NONE',  ( -13.97604488694527625, -13.89961937509977652, 81.87390960531436690 ) ) ;
#24416=CARTESIAN_POINT ( 'NONE',  ( 15.80617190586746368, 15.72974639402197994, 94.37390960531436690 ) ) ;
#24417=CARTESIAN_POINT ( 'NONE',  ( -0.05219959533934338120, 16.53943276465976808, 112.5010903946857042 ) ) ;
#24418=CARTESIAN_POINT ( 'NONE',  ( 13.89961937509977652, -13.97604488694527269, 98.12390960531433848 ) ) ;
#24419=CARTESIAN_POINT ( 'NONE',  ( -13.89961937509957401, -13.97604488694547875, 74.37609039468566152 ) ) ;
#24420=CARTESIAN_POINT ( 'NONE',  ( -18.67979575497193778, 10.72451020669871902, 103.3344237280190043 ) ) ;
#24421=CARTESIAN_POINT ( 'NONE',  ( -21.53943276465977519, 0.05219959533907696930, 71.24890960531435269 ) ) ;
#24422=CARTESIAN_POINT ( 'NONE',  ( 21.55341960407610458, 5.719274019375980345, 43.95724293864769550 ) ) ;
#24423=CARTESIAN_POINT ( 'NONE',  ( 19.03943276465977164, -0.05219959533909143690, 48.74890960531435979 ) ) ;
#24424=CARTESIAN_POINT ( 'NONE',  ( -14.34966873604960291, -8.224510206698953496, 26.66557627198103475 ) ) ;
#24425=CARTESIAN_POINT ( 'NONE',  ( 13.97604488694527802, 13.89961937509977652, 74.37390960531436690 ) ) ;
#24426=ORIENTED_EDGE ( 'NONE', *, *, #8545, .F. ) ;
#24428=CARTESIAN_POINT ( 'NONE',  ( -5.153800228976607833, 19.02544592524334988, 32.70942372801899722 ) ) ;
#24429=CARTESIAN_POINT ( 'NONE',  ( -16.55341960407611168, -4.379528057220339221, 86.45724293864770971 ) ) ;
#24430=CARTESIAN_POINT ( 'NONE',  ( -21.55341960407619339, 5.719274019375674811, 23.54275706135235424 ) ) ;
#24432=CARTESIAN_POINT ( 'NONE',  ( 18.67979575497178502, 10.72451020669898547, 69.16557627198102409 ) ) ;
#24433=CARTESIAN_POINT ( 'NONE',  ( 16.53943276465976808, 0.05219959533934440121, 96.25109039468568994 ) ) ;
#24434=CARTESIAN_POINT ( 'NONE',  ( -19.03943276465977164, 0.05219959533909376836, 21.24890960531436335 ) ) ;
#24435=CARTESIAN_POINT ( 'NONE',  ( 16.51473224551069308, 9.474510206698969483, 74.16557627198103830 ) ) ;
#24436=CARTESIAN_POINT ( 'NONE',  ( -19.05341960407611168, -5.049401038298163336, 21.45724293864768839 ) ) ;
#24437=CARTESIAN_POINT ( 'NONE',  ( 16.53943276465976808, -0.05219959533910856209, 23.74890960531435269 ) ) ;
#24438=CARTESIAN_POINT ( 'NONE',  ( -5.719274019375665041, -21.55341960407619695, 59.79275706135234714 ) ) ;
#24439=CARTESIAN_POINT ( 'NONE',  ( 13.89961937509977652, -13.97604488694527269, 113.1239096053143527 ) ) ;
#24440=CARTESIAN_POINT ( 'NONE',  ( -15.72974639402176322, -15.80617190586768395, 89.37609039468568994 ) ) ;
#24441=CARTESIAN_POINT ( 'NONE',  ( 16.51473224551069308, 9.474510206698969483, 49.16557627198102409 ) ) ;
#24442=CARTESIAN_POINT ( 'NONE',  ( 5.049401038298161559, -19.05341960407611168, 52.70724293864767418 ) ) ;
#24444=CARTESIAN_POINT ( 'NONE',  ( -10.72451020669870658, -18.67979575497194134, 89.58442372801901854 ) ) ;
#24445=CARTESIAN_POINT ( 'NONE',  ( 4.483927247898790824, -16.52544592524335698, 65.20942372801901854 ) ) ;
#24446=CARTESIAN_POINT ( 'NONE',  ( -10.72451020669870658, -18.67979575497194134, 84.58442372801903275 ) ) ;
#24447=CARTESIAN_POINT ( 'NONE',  ( -19.03943276465977164, 0.05219959533909376836, 116.2489096053143669 ) ) ;
#24448=CARTESIAN_POINT ( 'NONE',  ( -19.02544592524334988, -5.153800228976617603, 93.95942372801900433 ) ) ;
#24449=CARTESIAN_POINT ( 'NONE',  ( -18.62759615963255300, -10.81492255796106328, 59.16775706135234714 ) ) ;
#24450=CARTESIAN_POINT ( 'NONE',  ( -8.224510206698735004, -14.34966873604973081, 39.58442372801901143 ) ) ;
#24451=CARTESIAN_POINT ( 'NONE',  ( -10.72451020669898014, 18.67979575497178502, 85.41557627198102409 ) ) ;
#24452=CARTESIAN_POINT ( 'NONE',  ( 13.97604488694548053, -13.89961937509957401, 85.62609039468568994 ) ) ;
#24453=CARTESIAN_POINT ( 'NONE',  ( 19.03943276465977164, -0.05219959533909143690, 68.74890960531436690 ) ) ;
#24454=CARTESIAN_POINT ( 'NONE',  ( 16.46253265017146816, 9.564922557961045513, 91.66775706135234714 ) ) ;
#24455=CARTESIAN_POINT ( 'NONE',  ( -9.474510206698720793, -16.51473224551083518, 89.58442372801900433 ) ) ;
#24456=CARTESIAN_POINT ( 'NONE',  ( -16.53943276465976808, 0.05219959533911058130, 51.24890960531436690 ) ) ;
#24457=CARTESIAN_POINT ( 'NONE',  ( 19.02544592524334988, 5.153800228976608722, 81.45942372801897591 ) ) ;
#24458=CARTESIAN_POINT ( 'NONE',  ( 16.55341960407618274, -4.379528057220086978, 61.04275706135234714 ) ) ;
#24459=CARTESIAN_POINT ( 'NONE',  ( 19.03943276465977164, 0.05219959533936151252, 36.25109039468567573 ) ) ;
#24460=CARTESIAN_POINT ( 'NONE',  ( -5.049401038298153566, 19.05341960407611168, 35.20724293864768839 ) ) ;
#24461=CARTESIAN_POINT ( 'NONE',  ( 19.02544592524343514, -5.153800228976328945, 43.54057627198103120 ) ) ;
#24462=CARTESIAN_POINT ( 'NONE',  ( -16.55341960407617563, 4.379528057220093196, 53.54275706135234714 ) ) ;
#24465=CARTESIAN_POINT ( 'NONE',  ( -5.153800228976328057, -19.02544592524343514, 107.2905762719810383 ) ) ;
#24466=CARTESIAN_POINT ( 'NONE',  ( 16.46253265017160672, -9.564922557960803928, 28.33224293864769550 ) ) ;
#24468=CARTESIAN_POINT ( 'NONE',  ( 19.03943276465977164, 0.05219959533936151252, 96.25109039468567573 ) ) ;
#24469=CARTESIAN_POINT ( 'NONE',  ( 21.55341960407610458, 5.719274019375980345, 43.95724293864769550 ) ) ;
#24470=CARTESIAN_POINT ( 'NONE',  ( -5.049401038297874678, -19.05341960407617918, 29.79275706135232227 ) ) ;
#24471=CARTESIAN_POINT ( 'NONE',  ( -16.51473224551082808, 9.474510206698731452, 108.3344237280190043 ) ) ;
#24472=CARTESIAN_POINT ( 'NONE',  ( -19.03943276465977164, 0.05219959533909376836, 26.24890960531435624 ) ) ;
#24473=CARTESIAN_POINT ( 'NONE',  ( -5.049401038298153566, 19.05341960407611168, 45.20724293864769550 ) ) ;
#24474=CARTESIAN_POINT ( 'NONE',  ( -21.55341960407610458, -5.719274019375992779, 66.45724293864768129 ) ) ;
#24475=CARTESIAN_POINT ( 'NONE',  ( 19.02544592524343514, -5.153800228976328945, 98.54057627198100988 ) ) ;
#24476=CARTESIAN_POINT ( 'NONE',  ( -5.153800228976328057, -19.02544592524343514, 32.29057627198102409 ) ) ;
#24478=CARTESIAN_POINT ( 'NONE',  ( -19.05341960407617563, 5.049401038297882671, 83.54275706135233293 ) ) ;
#24479=CARTESIAN_POINT ( 'NONE',  ( -12.06949235617756955, 12.14591786802309770, 55.62390960531436690 ) ) ;
#24480=CARTESIAN_POINT ( 'NONE',  ( -21.53943276465977519, 0.05219959533907696930, 36.24890960531435979 ) ) ;
#24481=CARTESIAN_POINT ( 'NONE',  ( 15.80617190586769283, -15.72974639402175789, 105.6260903946856899 ) ) ;
#24482=CARTESIAN_POINT ( 'NONE',  ( 10.72451020669898902, -18.67979575497178502, 92.91557627198103830 ) ) ;
#24483=CARTESIAN_POINT ( 'NONE',  ( 10.81492255796106328, -18.62759615963255655, 75.41775706135233293 ) ) ;
#24484=CARTESIAN_POINT ( 'NONE',  ( -10.81492255796105439, 18.62759615963255655, 72.91775706135234714 ) ) ;
#24485=CARTESIAN_POINT ( 'NONE',  ( 13.97604488694527802, 13.89961937509977652, 114.3739096053143669 ) ) ;
#24486=CARTESIAN_POINT ( 'NONE',  ( 16.55341960407618274, -4.379528057220086978, 106.0427570613523471 ) ) ;
#24487=CARTESIAN_POINT ( 'NONE',  ( -10.81492255796105439, 18.62759615963255655, 57.91775706135234714 ) ) ;
#24488=CARTESIAN_POINT ( 'NONE',  ( 16.51473224551069308, 9.474510206698969483, 64.16557627198102409 ) ) ;
#24489=CARTESIAN_POINT ( 'NONE',  ( -5.153800228976607833, 19.02544592524334988, 37.70942372801899722 ) ) ;
#24490=CARTESIAN_POINT ( 'NONE',  ( 15.72974639402176855, 15.80617190586768217, 36.87609039468568994 ) ) ;
#24491=CARTESIAN_POINT ( 'NONE',  ( -19.05341960407611168, -5.049401038298163336, 71.45724293864766707 ) ) ;
#24492=CARTESIAN_POINT ( 'NONE',  ( -12.14591786802309592, -12.06949235617757132, 81.87390960531435269 ) ) ;
#24493=CARTESIAN_POINT ( 'NONE',  ( -16.55341960407611168, -4.379528057220339221, 41.45724293864769550 ) ) ;
#24494=CARTESIAN_POINT ( 'NONE',  ( -15.72974639402197994, 15.80617190586746368, 60.62390960531437401 ) ) ;
#24495=CARTESIAN_POINT ( 'NONE',  ( -5.153800228976328057, -19.02544592524343514, 57.29057627198103120 ) ) ;
#24496=CARTESIAN_POINT ( 'NONE',  ( -21.53943276465977519, 0.05219959533907696930, 71.24890960531435269 ) ) ;
#24497=CARTESIAN_POINT ( 'NONE',  ( 0.05219959533936267826, -19.03943276465977164, 45.00109039468566863 ) ) ;
#24498=CARTESIAN_POINT ( 'NONE',  ( -9.564922557961040184, 16.46253265017147172, 22.91775706135233648 ) ) ;
#24499=CARTESIAN_POINT ( 'NONE',  ( 12.06949235617757843, -12.14591786802309237, 63.12390960531435979 ) ) ;
#24500=CARTESIAN_POINT ( 'NONE',  ( 10.81492255796078972, 18.62759615963270932, 39.58224293864769550 ) ) ;
#24501=VERTEX_POINT ( 'NONE', #58214 ) ;
#24504=CARTESIAN_POINT ( 'NONE',  ( -12.06949235617739369, -12.14591786802326823, 89.37609039468568994 ) ) ;
#24506=CARTESIAN_POINT ( 'NONE',  ( -16.51473224551082808, 9.474510206698731452, 93.33442372801900433 ) ) ;
#24507=CARTESIAN_POINT ( 'NONE',  ( -16.53943276465976808, 0.05219959533911058130, 61.24890960531435979 ) ) ;
#24510=CARTESIAN_POINT ( 'NONE',  ( 5.153800228976335163, 19.02544592524342804, 44.79057627198103830 ) ) ;
#24511=CARTESIAN_POINT ( 'NONE',  ( 14.34966873604960469, 8.224510206698951720, 34.16557627198102409 ) ) ;
#24512=CARTESIAN_POINT ( 'NONE',  ( -9.564922557960796823, -16.46253265017161027, 92.08224293864769550 ) ) ;
#24513=CARTESIAN_POINT ( 'NONE',  ( 19.03943276465977164, -0.05219959533909143690, 53.74890960531436690 ) ) ;
#24514=CARTESIAN_POINT ( 'NONE',  ( -5.823673210054431948, 21.52544592524334988, 62.70942372801902565 ) ) ;
#24515=CARTESIAN_POINT ( 'NONE',  ( 0.05219959533909260263, 19.03943276465977164, 74.99890960531435269 ) ) ;
#24516=CARTESIAN_POINT ( 'NONE',  ( -5.049401038298153566, 19.05341960407611168, 30.20724293864768839 ) ) ;
#24517=CARTESIAN_POINT ( 'NONE',  ( -19.05341960407611168, -5.049401038298163336, 76.45724293864769550 ) ) ;
#24518=CARTESIAN_POINT ( 'NONE',  ( 0.05219959533907565091, 21.53943276465977519, 44.99890960531435979 ) ) ;
#24519=CARTESIAN_POINT ( 'NONE',  ( 5.153800228976335163, 19.02544592524342804, 39.79057627198100988 ) ) ;
#24520=CARTESIAN_POINT ( 'NONE',  ( -21.52544592524343514, 5.823673210054127303, 41.04057627198103120 ) ) ;
#24521=CARTESIAN_POINT ( 'NONE',  ( 12.06949235617739724, 12.14591786802326823, 106.8760903946856899 ) ) ;
#24522=CARTESIAN_POINT ( 'NONE',  ( -19.02544592524334988, -5.153800228976617603, 28.95942372801900433 ) ) ;
#24523=CARTESIAN_POINT ( 'NONE',  ( 16.52544592524335698, 4.483927247898782831, 46.45942372801901854 ) ) ;
#24524=CARTESIAN_POINT ( 'NONE',  ( -14.29746914071037622, -8.314922557961029526, 74.16775706135231871 ) ) ;
#24525=DIRECTION ( 'NONE',  ( -1.000000000000000000, 0.000000000000000000, -0.000000000000000000 ) ) ;
#24526=CARTESIAN_POINT ( 'NONE',  ( -14.34966873604972548, 8.224510206698743886, 63.33442372801900433 ) ) ;
#24527=CARTESIAN_POINT ( 'NONE',  ( 21.53943276465977519, -0.05219959533907433946, 28.74890960531435624 ) ) ;
#24528=CARTESIAN_POINT ( 'NONE',  ( -16.51473224551069308, -9.474510206698971260, 31.66557627198102054 ) ) ;
#24529=CARTESIAN_POINT ( 'NONE',  ( 8.314922557961029526, -14.29746914071037800, 40.41775706135234714 ) ) ;
#24530=CARTESIAN_POINT ( 'NONE',  ( 19.03943276465977164, -0.05219959533909143690, 53.74890960531436690 ) ) ;
#24531=CARTESIAN_POINT ( 'NONE',  ( 5.823673210054444382, -21.52544592524334988, 40.20942372801901854 ) ) ;
#24532=CARTESIAN_POINT ( 'NONE',  ( 8.314922557961029526, -14.29746914071037800, 40.41775706135234714 ) ) ;
#24533=CARTESIAN_POINT ( 'NONE',  ( 4.379528057220092307, 16.55341960407617563, 97.29275706135234714 ) ) ;
#24535=CARTESIAN_POINT ( 'NONE',  ( 21.53943276465977519, 0.05219959533937863772, 96.25109039468568994 ) ) ;
#24536=CARTESIAN_POINT ( 'NONE',  ( -0.05219959533936034679, 19.03943276465977164, 97.50109039468567573 ) ) ;
#24538=CARTESIAN_POINT ( 'NONE',  ( -19.03943276465977164, -0.05219959533935918106, 73.75109039468566152 ) ) ;
#24539=CARTESIAN_POINT ( 'NONE',  ( -12.14591786802309592, -12.06949235617757132, 66.87390960531436690 ) ) ;
#24540=CARTESIAN_POINT ( 'NONE',  ( -13.97604488694527625, -13.89961937509977652, 21.87390960531435979 ) ) ;
#24541=CARTESIAN_POINT ( 'NONE',  ( 16.46253265017146816, 9.564922557961045513, 56.66775706135233293 ) ) ;
#24542=CARTESIAN_POINT ( 'NONE',  ( 17.44270441346520428, 5.991230190322989202, 78.86335079264232206 ) ) ;
#24543=CARTESIAN_POINT ( 'NONE',  ( -15.80617190586768217, 15.72974639402176855, 63.12609039468568994 ) ) ;
#24544=CARTESIAN_POINT ( 'NONE',  ( -14.29746914071037622, -8.314922557961029526, 24.16775706135235424 ) ) ;
#24545=CARTESIAN_POINT ( 'NONE',  ( -18.22780087662123805, 5.499999999999981348, 91.01763182126894947 ) ) ;
#24546=CARTESIAN_POINT ( 'NONE',  ( 21.52544592524344225, -5.823673210054117533, 28.54057627198103120 ) ) ;
#24547=CARTESIAN_POINT ( 'NONE',  ( -16.51473224551082808, 9.474510206698731452, 103.3344237280190043 ) ) ;
#24548=CARTESIAN_POINT ( 'NONE',  ( 19.03943276465977164, -0.05219959533909143690, 113.7489096053143669 ) ) ;
#24550=CARTESIAN_POINT ( 'NONE',  ( -16.53943276465976808, 0.05219959533911058130, 116.2489096053143669 ) ) ;
#24551=CARTESIAN_POINT ( 'NONE',  ( -19.03943276465977164, -0.05219959533935918106, 18.75109039468567218 ) ) ;
#24552=CARTESIAN_POINT ( 'NONE',  ( 5.049401038298161559, -19.05341960407611168, 57.70724293864769550 ) ) ;
#24554=CARTESIAN_POINT ( 'NONE',  ( -21.55341960407619339, 5.719274019375674811, 68.54275706135234714 ) ) ;
#24555=CARTESIAN_POINT ( 'NONE',  ( -15.80617190586768217, 15.72974639402176855, 98.12609039468570415 ) ) ;
#24556=CARTESIAN_POINT ( 'NONE',  ( 14.34966873604960469, 8.224510206698951720, 29.16557627198103120 ) ) ;
#24557=CARTESIAN_POINT ( 'NONE',  ( 5.049401038298161559, -19.05341960407611168, 82.70724293864770971 ) ) ;
#24558=CARTESIAN_POINT ( 'NONE',  ( 18.67979575497194134, -10.72451020669871369, 60.83442372801901854 ) ) ;
#24559=CARTESIAN_POINT ( 'NONE',  ( -10.72451020669870658, -18.67979575497194134, 49.58442372801901143 ) ) ;
#24560=CARTESIAN_POINT ( 'NONE',  ( 19.05341960407617918, -5.049401038297876454, 86.04275706135233293 ) ) ;
#24561=CARTESIAN_POINT ( 'NONE',  ( 16.46253265017160672, -9.564922557960803928, 108.3322429386476955 ) ) ;
#24562=CARTESIAN_POINT ( 'NONE',  ( -0.05219959533909027116, -19.03943276465977164, 22.49890960531436690 ) ) ;
#24563=CARTESIAN_POINT ( 'NONE',  ( -5.719274019375978568, 21.55341960407610458, 90.20724293864770971 ) ) ;
#24564=CARTESIAN_POINT ( 'NONE',  ( -13.97604488694547697, 13.89961937509957934, 33.12609039468566863 ) ) ;
#24565=CARTESIAN_POINT ( 'NONE',  ( -16.53943276465976808, 0.05219959533911058130, 96.24890960531435269 ) ) ;
#24566=CARTESIAN_POINT ( 'NONE',  ( -13.97604488694527625, -13.89961937509977652, 51.87390960531436690 ) ) ;
#24567=CARTESIAN_POINT ( 'NONE',  ( 19.02544592524334988, 5.153800228976608722, 96.45942372801897591 ) ) ;
#24568=CARTESIAN_POINT ( 'NONE',  ( -16.55341960407611168, -4.379528057220339221, 56.45724293864768839 ) ) ;
#24569=CARTESIAN_POINT ( 'NONE',  ( -21.52544592524334988, -5.823673210054445271, 108.9594237280190185 ) ) ;
#24570=CARTESIAN_POINT ( 'NONE',  ( 9.564922557960805705, 16.46253265017160317, 99.58224293864770971 ) ) ;
#24571=CARTESIAN_POINT ( 'NONE',  ( 16.46253265017146816, 9.564922557961045513, 71.66775706135233293 ) ) ;
#24572=CARTESIAN_POINT ( 'NONE',  ( 21.52544592524344225, -5.823673210054117533, 93.54057627198103830 ) ) ;
#24573=CARTESIAN_POINT ( 'NONE',  ( -10.81492255796105439, 18.62759615963255655, 47.91775706135234714 ) ) ;
#24574=CARTESIAN_POINT ( 'NONE',  ( -4.379528057220086978, -16.55341960407618274, 39.79275706135235424 ) ) ;
#24575=CARTESIAN_POINT ( 'NONE',  ( -16.53943276465976808, -0.05219959533934237506, 93.75109039468567573 ) ) ;
#24576=CARTESIAN_POINT ( 'NONE',  ( 14.29746914071037800, 8.314922557961029526, 41.66775706135235424 ) ) ;
#24577=CARTESIAN_POINT ( 'NONE',  ( 10.72451020669871369, 18.67979575497193778, 37.08442372801901143 ) ) ;
#24578=CARTESIAN_POINT ( 'NONE',  ( -10.72451020669898014, 18.67979575497178502, 40.41557627198103120 ) ) ;
#24579=CARTESIAN_POINT ( 'NONE',  ( -5.153800228976328057, -19.02544592524343514, 37.29057627198102409 ) ) ;
#24581=CARTESIAN_POINT ( 'NONE',  ( -14.29746914071037622, -8.314922557961029526, 59.16775706135234714 ) ) ;
#24583=CARTESIAN_POINT ( 'NONE',  ( -18.67979575497178146, -10.72451020669898902, 86.66557627198102409 ) ) ;
#24584=CARTESIAN_POINT ( 'NONE',  ( -12.06949235617756955, 12.14591786802309770, 35.62390960531437401 ) ) ;
#24585=CARTESIAN_POINT ( 'NONE',  ( -16.52544592524335698, -4.483927247898792601, 63.95942372801901854 ) ) ;
#24586=CARTESIAN_POINT ( 'NONE',  ( -19.05341960407611168, -5.049401038298163336, 61.45724293864769550 ) ) ;
#24587=CARTESIAN_POINT ( 'NONE',  ( 5.049401038297881783, 19.05341960407617563, 87.29275706135234714 ) ) ;
#24588=CARTESIAN_POINT ( 'NONE',  ( -10.72451020669898014, 18.67979575497178502, 80.41557627198103830 ) ) ;
#24589=CARTESIAN_POINT ( 'NONE',  ( 8.314922557960818139, 14.29746914071049879, 34.58224293864770260 ) ) ;
#24592=CARTESIAN_POINT ( 'NONE',  ( 15.80617190586746368, 15.72974639402197994, 59.37390960531436690 ) ) ;
#24594=CARTESIAN_POINT ( 'NONE',  ( -16.53943276465976808, -0.05219959533934237506, 103.7510903946857042 ) ) ;
#24597=CARTESIAN_POINT ( 'NONE',  ( 18.62759615963271287, -10.81492255796078972, 93.33224293864769550 ) ) ;
#24599=CARTESIAN_POINT ( 'NONE',  ( -8.314922557960811034, -14.29746914071050412, 22.08224293864769194 ) ) ;
#24600=CARTESIAN_POINT ( 'NONE',  ( 16.55341960407618274, -4.379528057220086978, 31.04275706135234714 ) ) ;
#24601=CARTESIAN_POINT ( 'NONE',  ( -5.049401038298153566, 19.05341960407611168, 30.20724293864768839 ) ) ;
#24602=CARTESIAN_POINT ( 'NONE',  ( -13.97604488694527625, -13.89961937509977652, 66.87390960531436690 ) ) ;
#24604=CARTESIAN_POINT ( 'NONE',  ( 21.53943276465977519, -0.05219959533907433946, 23.74890960531435269 ) ) ;
#24605=CARTESIAN_POINT ( 'NONE',  ( 5.153800228976335163, 19.02544592524342804, 114.7905762719810241 ) ) ;
#24606=CARTESIAN_POINT ( 'NONE',  ( 19.02544592524334988, 5.153800228976608722, 111.4594237280190043 ) ) ;
#24607=CARTESIAN_POINT ( 'NONE',  ( -16.51473224551082808, 9.474510206698731452, 33.33442372801899722 ) ) ;
#24608=CARTESIAN_POINT ( 'NONE',  ( 21.53943276465977519, -0.05219959533907433946, 83.74890960531435269 ) ) ;
#24609=CARTESIAN_POINT ( 'NONE',  ( 0.05219959533910956823, 16.53943276465976808, 24.99890960531435624 ) ) ;
#24610=CARTESIAN_POINT ( 'NONE',  ( 5.719274019375991003, -21.55341960407610458, 47.70724293864770260 ) ) ;
#24611=CARTESIAN_POINT ( 'NONE',  ( 21.52544592524344225, -5.823673210054117533, 83.54057627198102409 ) ) ;
#24612=CARTESIAN_POINT ( 'NONE',  ( 5.153800228976615827, -19.02544592524334988, 110.2094237280189901 ) ) ;
#24613=CARTESIAN_POINT ( 'NONE',  ( 19.03943276465977164, -0.05219959533909143690, 108.7489096053143527 ) ) ;
#24614=CARTESIAN_POINT ( 'NONE',  ( -0.05219959533937732626, 21.53943276465977519, 77.50109039468567573 ) ) ;
#24615=CARTESIAN_POINT ( 'NONE',  ( -5.049401038298153566, 19.05341960407611168, 55.20724293864769550 ) ) ;
#24616=CARTESIAN_POINT ( 'NONE',  ( -0.05219959533910754901, -16.53943276465976808, 102.4989096053143811 ) ) ;
#24618=CARTESIAN_POINT ( 'NONE',  ( -5.153800228976328057, -19.02544592524343514, 72.29057627198102409 ) ) ;
#24619=CARTESIAN_POINT ( 'NONE',  ( -4.379528057220328563, 16.55341960407611168, 95.20724293864769550 ) ) ;
#24621=CARTESIAN_POINT ( 'NONE',  ( 19.03943276465977164, 0.05219959533936151252, 96.25109039468567573 ) ) ;
#24622=CARTESIAN_POINT ( 'NONE',  ( 19.35543954521081034, 5.499999999999526601, 92.08901960356452321 ) ) ;
#24623=CARTESIAN_POINT ( 'NONE',  ( -9.474510206698964154, 16.51473224551069663, 65.41557627198102409 ) ) ;
#24624=CARTESIAN_POINT ( 'NONE',  ( -18.62759615963255300, -10.81492255796106328, 89.16775706135236135 ) ) ;
#24625=CARTESIAN_POINT ( 'NONE',  ( -0.05219959533909027116, -19.03943276465977164, 97.49890960531436690 ) ) ;
#24626=CARTESIAN_POINT ( 'NONE',  ( 4.483927247898790824, -16.52544592524335698, 75.20942372801901854 ) ) ;
#24628=CARTESIAN_POINT ( 'NONE',  ( 0.05219959533936267826, -19.03943276465977164, 50.00109039468566863 ) ) ;
#24629=CARTESIAN_POINT ( 'NONE',  ( 15.80617190586769283, -15.72974639402175789, 105.6260903946856899 ) ) ;
#24632=CARTESIAN_POINT ( 'NONE',  ( 0.05219959533934541429, -16.53943276465976808, 100.0010903946857042 ) ) ;
#24634=CARTESIAN_POINT ( 'NONE',  ( -4.483927247898782831, 16.52544592524335698, 87.70942372801901854 ) ) ;
#24635=CARTESIAN_POINT ( 'NONE',  ( 17.44270441346519718, 5.991230190322989202, 68.86335079264230785 ) ) ;
#24636=CARTESIAN_POINT ( 'NONE',  ( 8.314922557961029526, -14.29746914071037800, 70.41775706135236135 ) ) ;
#24638=CARTESIAN_POINT ( 'NONE',  ( 10.81492255796106328, -18.62759615963255655, 75.41775706135233293 ) ) ;
#24640=CARTESIAN_POINT ( 'NONE',  ( -19.03943276465977164, -0.05219959533935918106, 83.75109039468567573 ) ) ;
#24641=CARTESIAN_POINT ( 'NONE',  ( 9.564922557961047289, -16.46253265017146816, 20.41775706135233293 ) ) ;
#24642=CARTESIAN_POINT ( 'NONE',  ( 16.46253265017160672, -9.564922557960803928, 63.33224293864769550 ) ) ;
#24643=CARTESIAN_POINT ( 'NONE',  ( 19.02544592524343514, -5.153800228976328945, 53.54057627198102409 ) ) ;
#24644=DIRECTION ( 'NONE',  ( 0.000000000000000000, 0.000000000000000000, -1.000000000000000000 ) ) ;
#24645=CARTESIAN_POINT ( 'NONE',  ( -18.62759615963270932, 10.81492255796079327, 85.83224293864768129 ) ) ;
#24646=CARTESIAN_POINT ( 'NONE',  ( 18.62759615963271287, -10.81492255796078972, 33.33224293864769550 ) ) ;
#24647=CARTESIAN_POINT ( 'NONE',  ( -5.049401038298153566, 19.05341960407611168, 35.20724293864768839 ) ) ;
#24648=CARTESIAN_POINT ( 'NONE',  ( -12.06949235617739369, -12.14591786802326823, 69.37609039468567573 ) ) ;
#24650=CARTESIAN_POINT ( 'NONE',  ( 21.53943276465977519, 0.05219959533937863772, 26.25109039468567573 ) ) ;
#24651=CARTESIAN_POINT ( 'NONE',  ( 16.53943276465976808, -0.05219959533910856209, 68.74890960531435269 ) ) ;
#24653=CARTESIAN_POINT ( 'NONE',  ( 16.53943276465976808, 0.05219959533934440121, 21.25109039468567218 ) ) ;
#24654=CARTESIAN_POINT ( 'NONE',  ( -19.02544592524334988, -5.153800228976617603, 48.95942372801900433 ) ) ;
#24655=CARTESIAN_POINT ( 'NONE',  ( -16.53943276465976808, 0.05219959533911058130, 56.24890960531436690 ) ) ;
#24656=CARTESIAN_POINT ( 'NONE',  ( -15.72974639402176322, -15.80617190586768395, 34.37609039468568284 ) ) ;
#24658=CARTESIAN_POINT ( 'NONE',  ( 21.53943276465977519, -0.05219959533907433946, 78.74890960531436690 ) ) ;
#24659=CARTESIAN_POINT ( 'NONE',  ( 9.564922557960805705, 16.46253265017160317, 99.58224293864770971 ) ) ;
#24660=CARTESIAN_POINT ( 'NONE',  ( -14.34966873604960291, -8.224510206698953496, 66.66557627198102409 ) ) ;
#24663=CARTESIAN_POINT ( 'NONE',  ( -19.02544592524334988, -5.153800228976617603, 63.95942372801899012 ) ) ;
#24664=CARTESIAN_POINT ( 'NONE',  ( 5.823673210054125526, 21.52544592524343514, 109.7905762719810383 ) ) ;
#24665=CARTESIAN_POINT ( 'NONE',  ( 13.89961937509977652, -13.97604488694527269, 58.12390960531436690 ) ) ;
#24666=CARTESIAN_POINT ( 'NONE',  ( -0.05219959533936034679, 19.03943276465977164, 42.50109039468566152 ) ) ;
#24667=CARTESIAN_POINT ( 'NONE',  ( 5.153800228976335163, 19.02544592524342804, 34.79057627198102409 ) ) ;
#24669=CARTESIAN_POINT ( 'NONE',  ( -21.53943276465977519, -0.05219959533937600094, 63.75109039468568284 ) ) ;
#24670=CARTESIAN_POINT ( 'NONE',  ( -17.44279575226823908, -5.990770900252440079, 69.16442432485682446 ) ) ;
#24671=CARTESIAN_POINT ( 'NONE',  ( 12.06949235617757843, -12.14591786802309237, 38.12390960531436690 ) ) ;
#24672=CARTESIAN_POINT ( 'NONE',  ( -19.02544592524342804, 5.153800228976336051, 66.04057627198103830 ) ) ;
#24673=CARTESIAN_POINT ( 'NONE',  ( -0.05219959533907301413, -21.53943276465977519, 72.49890960531435269 ) ) ;
#24674=CARTESIAN_POINT ( 'NONE',  ( -19.05341960407611168, -5.049401038298163336, 61.45724293864769550 ) ) ;
#24676=CARTESIAN_POINT ( 'NONE',  ( 21.52544592524344225, -5.823673210054117533, 63.54057627198103830 ) ) ;
#24678=CARTESIAN_POINT ( 'NONE',  ( -5.719274019375665041, -21.55341960407619695, 99.79275706135234714 ) ) ;
#24680=CARTESIAN_POINT ( 'NONE',  ( -14.29746914071037622, -8.314922557961029526, 99.16775706135234714 ) ) ;
#24681=CARTESIAN_POINT ( 'NONE',  ( -8.224510206698948167, 14.34966873604960824, 80.41557627198103830 ) ) ;
#24682=CARTESIAN_POINT ( 'NONE',  ( 19.02544592524334988, 5.153800228976608722, 96.45942372801897591 ) ) ;
#24684=CARTESIAN_POINT ( 'NONE',  ( -19.05341960407617563, 5.049401038297882671, 38.54275706135233293 ) ) ;
#24685=CARTESIAN_POINT ( 'NONE',  ( 0.05219959533934541429, -16.53943276465976808, 105.0010903946856757 ) ) ;
#24686=CARTESIAN_POINT ( 'NONE',  ( -9.474510206698720793, -16.51473224551083518, 29.58442372801900433 ) ) ;
#24687=CARTESIAN_POINT ( 'NONE',  ( 19.03943276465977164, -0.05219959533909143690, 83.74890960531436690 ) ) ;
#24688=CARTESIAN_POINT ( 'NONE',  ( -18.67979575497178146, -10.72451020669898902, 66.66557627198102409 ) ) ;
#24690=CARTESIAN_POINT ( 'NONE',  ( -8.314922557960811034, -14.29746914071050412, 112.0822429386477097 ) ) ;
#24691=CARTESIAN_POINT ( 'NONE',  ( 10.72451020669871369, 18.67979575497193778, 92.08442372801901854 ) ) ;
#24692=CARTESIAN_POINT ( 'NONE',  ( -12.06949235617739369, -12.14591786802326823, 74.37609039468568994 ) ) ;
#24693=CARTESIAN_POINT ( 'NONE',  ( 21.55341960407619695, -5.719274019375665929, 31.04275706135234714 ) ) ;
#24694=CARTESIAN_POINT ( 'NONE',  ( -16.55341960407617563, 4.379528057220093196, 33.54275706135234714 ) ) ;
#24695=CARTESIAN_POINT ( 'NONE',  ( -16.51473224551069308, -9.474510206698971260, 111.6655762719810383 ) ) ;
#24696=CARTESIAN_POINT ( 'NONE',  ( -19.02544592524342804, 5.153800228976336051, 36.04057627198100988 ) ) ;
#24697=CARTESIAN_POINT ( 'NONE',  ( -19.05341960407611168, -5.049401038298163336, 46.45724293864768129 ) ) ;
#24699=CARTESIAN_POINT ( 'NONE',  ( 8.314922557961029526, -14.29746914071037800, 50.41775706135235424 ) ) ;
#24700=CARTESIAN_POINT ( 'NONE',  ( -16.55341960407611168, -4.379528057220339221, 91.45724293864769550 ) ) ;
#24701=CARTESIAN_POINT ( 'NONE',  ( 14.29746914071037800, 8.314922557961029526, 101.6677570613523613 ) ) ;
#24702=CARTESIAN_POINT ( 'NONE',  ( -18.62759615963255300, -10.81492255796106328, 39.16775706135235424 ) ) ;
#24703=CARTESIAN_POINT ( 'NONE',  ( -0.05219959533909027116, -19.03943276465977164, 77.49890960531435269 ) ) ;
#24704=CARTESIAN_POINT ( 'NONE',  ( 13.89961937509977652, -13.97604488694527269, 68.12390960531436690 ) ) ;
#24705=CARTESIAN_POINT ( 'NONE',  ( -9.474510206698964154, 16.51473224551069663, 100.4155762719810241 ) ) ;
#24706=CARTESIAN_POINT ( 'NONE',  ( 16.52544592524342804, -4.483927247898539470, 28.54057627198103120 ) ) ;
#24707=CARTESIAN_POINT ( 'NONE',  ( 12.06949235617739724, 12.14591786802326823, 96.87609039468568994 ) ) ;
#24709=CARTESIAN_POINT ( 'NONE',  ( 0.05219959533936267826, -19.03943276465977164, 40.00109039468566152 ) ) ;
#24710=CARTESIAN_POINT ( 'NONE',  ( 9.474510206698971260, -16.51473224551069308, 107.9155762719810383 ) ) ;
#24711=CARTESIAN_POINT ( 'NONE',  ( -13.97604488694527625, -13.89961937509977652, 56.87390960531434558 ) ) ;
#24712=CARTESIAN_POINT ( 'NONE',  ( -16.46253265017146816, -9.564922557961047289, 34.16775706135233293 ) ) ;
#24714=CARTESIAN_POINT ( 'NONE',  ( 16.52544592524335698, 4.483927247898782831, 46.45942372801901854 ) ) ;
#24715=CARTESIAN_POINT ( 'NONE',  ( -13.97604488694547697, 13.89961937509957934, 78.12609039468567573 ) ) ;
#24716=CARTESIAN_POINT ( 'NONE',  ( 8.224510206698742110, 14.34966873604972548, 52.08442372801901854 ) ) ;
#24718=CARTESIAN_POINT ( 'NONE',  ( 16.46253265017160672, -9.564922557960803928, 88.33224293864769550 ) ) ;
#24719=CARTESIAN_POINT ( 'NONE',  ( 15.80617190586746368, 15.72974639402197994, 114.3739096053143527 ) ) ;
#24720=CARTESIAN_POINT ( 'NONE',  ( -5.049401038297874678, -19.05341960407617918, 79.79275706135233293 ) ) ;
#24721=CARTESIAN_POINT ( 'NONE',  ( 5.153800228976335163, 19.02544592524342804, 109.7905762719810099 ) ) ;
#24722=CARTESIAN_POINT ( 'NONE',  ( -19.03943276465977164, 0.05219959533909376836, 36.24890960531436690 ) ) ;
#24723=CARTESIAN_POINT ( 'NONE',  ( -19.05341960407611168, -5.049401038298163336, 71.45724293864766707 ) ) ;
#24724=CARTESIAN_POINT ( 'NONE',  ( -8.224510206698948167, 14.34966873604960824, 40.41557627198103120 ) ) ;
#24725=CARTESIAN_POINT ( 'NONE',  ( -13.97604488694527625, -13.89961937509977652, 31.87390960531435979 ) ) ;
#24726=CARTESIAN_POINT ( 'NONE',  ( 16.51473224551083163, -9.474510206698727899, 50.83442372801899722 ) ) ;
#24727=CARTESIAN_POINT ( 'NONE',  ( 14.29746914071049879, -8.314922557960816363, 83.33224293864769550 ) ) ;
#24728=CARTESIAN_POINT ( 'NONE',  ( 13.89961937509957401, 13.97604488694547697, 21.87609039468566152 ) ) ;
#24729=CARTESIAN_POINT ( 'NONE',  ( -0.05219959533909027116, -19.03943276465977164, 47.49890960531435979 ) ) ;
#24730=CARTESIAN_POINT ( 'NONE',  ( 10.81492255796078972, 18.62759615963270932, 49.58224293864769550 ) ) ;
#24731=CARTESIAN_POINT ( 'NONE',  ( -12.06949235617756955, 12.14591786802309770, 55.62390960531436690 ) ) ;
#24732=CARTESIAN_POINT ( 'NONE',  ( -5.823673210054431948, 21.52544592524334988, 97.70942372801904696 ) ) ;
#24733=CARTESIAN_POINT ( 'NONE',  ( 9.474510206698971260, -16.51473224551069308, 107.9155762719810383 ) ) ;
#24734=CARTESIAN_POINT ( 'NONE',  ( 5.049401038298161559, -19.05341960407611168, 112.7072429386476813 ) ) ;
#24735=CARTESIAN_POINT ( 'NONE',  ( 13.89961937509977652, -13.97604488694527269, 38.12390960531436690 ) ) ;
#24736=CARTESIAN_POINT ( 'NONE',  ( 16.46253265017160672, -9.564922557960803928, 23.33224293864769194 ) ) ;
#24737=CARTESIAN_POINT ( 'NONE',  ( 14.29746914071049879, -8.314922557960816363, 93.33224293864769550 ) ) ;
#24738=CARTESIAN_POINT ( 'NONE',  ( 10.81492255796078972, 18.62759615963270932, 94.58224293864769550 ) ) ;
#24739=CARTESIAN_POINT ( 'NONE',  ( -13.97604488694527625, -13.89961937509977652, 96.87390960531433848 ) ) ;
#24740=CARTESIAN_POINT ( 'NONE',  ( -15.80617190586745835, -15.72974639402198527, 111.8739096053143669 ) ) ;
#24741=CARTESIAN_POINT ( 'NONE',  ( -0.05219959533909027116, -19.03943276465977164, 97.49890960531436690 ) ) ;
#24742=CARTESIAN_POINT ( 'NONE',  ( 13.97604488694548053, -13.89961937509957401, 65.62609039468567573 ) ) ;
#24743=CARTESIAN_POINT ( 'NONE',  ( 12.06949235617757843, -12.14591786802309237, 103.1239096053143811 ) ) ;
#24745=CARTESIAN_POINT ( 'NONE',  ( -13.89961937509977652, 13.97604488694528158, 75.62390960531438111 ) ) ;
#24746=CARTESIAN_POINT ( 'NONE',  ( -5.823673210054116645, -21.52544592524344225, 82.29057627198103830 ) ) ;
#24750=CARTESIAN_POINT ( 'NONE',  ( 5.823673210054125526, 21.52544592524343514, 29.79057627198102409 ) ) ;
#24752=CARTESIAN_POINT ( 'NONE',  ( 8.224510206698742110, 14.34966873604972548, 32.08442372801901854 ) ) ;
#24753=CARTESIAN_POINT ( 'NONE',  ( -16.55341960407611168, -4.379528057220339221, 96.45724293864770971 ) ) ;
#24754=CARTESIAN_POINT ( 'NONE',  ( 19.53037848336977689, -5.500000000000094147, 52.35532783611441943 ) ) ;
#24755=CARTESIAN_POINT ( 'NONE',  ( -19.03943276465977164, 0.05219959533909376836, 91.24890960531436690 ) ) ;
#24756=CARTESIAN_POINT ( 'NONE',  ( -0.05219959533909027116, -19.03943276465977164, 57.49890960531435979 ) ) ;
#24757=CARTESIAN_POINT ( 'NONE',  ( 14.34966873604960469, 8.224510206698951720, 79.16557627198103830 ) ) ;
#24758=CARTESIAN_POINT ( 'NONE',  ( 21.55341960407610458, 5.719274019375980345, 33.95724293864769550 ) ) ;
#24759=CARTESIAN_POINT ( 'NONE',  ( 14.29746914071049879, -8.314922557960816363, 53.33224293864769550 ) ) ;
#24760=CARTESIAN_POINT ( 'NONE',  ( 16.52544592524335698, 4.483927247898782831, 26.45942372801901854 ) ) ;
#24761=CARTESIAN_POINT ( 'NONE',  ( 5.823673210054444382, -21.52544592524334988, 75.20942372801901854 ) ) ;
#24763=CARTESIAN_POINT ( 'NONE',  ( 10.72451020669898902, -18.67979575497178502, 22.91557627198102765 ) ) ;
#24764=CARTESIAN_POINT ( 'NONE',  ( 0.05219959533934541429, -16.53943276465976808, 90.00109039468567573 ) ) ;
#24765=CARTESIAN_POINT ( 'NONE',  ( 0.05219959533909260263, 19.03943276465977164, 29.99890960531435979 ) ) ;
#24766=CARTESIAN_POINT ( 'NONE',  ( -19.02544592524342804, 5.153800228976336051, 91.04057627198100988 ) ) ;
#24767=CARTESIAN_POINT ( 'NONE',  ( -15.72974639402197994, 15.80617190586746368, 100.6239096053143811 ) ) ;
#24768=CARTESIAN_POINT ( 'NONE',  ( -12.06949235617739369, -12.14591786802326823, 29.37609039468568284 ) ) ;
#24769=CARTESIAN_POINT ( 'NONE',  ( -16.53943276465976808, 0.05219959533911058130, 56.24890960531436690 ) ) ;
#24770=CARTESIAN_POINT ( 'NONE',  ( 18.62759615963255655, 10.81492255796105972, 76.66775706135234714 ) ) ;
#24771=CARTESIAN_POINT ( 'NONE',  ( 14.29746914071037800, 8.314922557961029526, 91.66775706135234714 ) ) ;
#24772=CARTESIAN_POINT ( 'NONE',  ( -5.719274019375978568, 21.55341960407610458, 25.20724293864769550 ) ) ;
#24773=CARTESIAN_POINT ( 'NONE',  ( 17.31747979337949417, 6.344076630961017926, 28.87944868065185489 ) ) ;
#24774=CARTESIAN_POINT ( 'NONE',  ( -17.13100169013300444, 6.664070546373148218, 80.76789835699848652 ) ) ;
#24775=CARTESIAN_POINT ( 'NONE',  ( -16.52544592524335698, -4.483927247898792601, 103.9594237280190185 ) ) ;
#24776=CARTESIAN_POINT ( 'NONE',  ( 12.06949235617739724, 12.14591786802326823, 66.87609039468568994 ) ) ;
#24777=CARTESIAN_POINT ( 'NONE',  ( 19.03943276465977164, -0.05219959533909143690, 78.74890960531436690 ) ) ;
#24778=CARTESIAN_POINT ( 'NONE',  ( -0.05219959533909027116, -19.03943276465977164, 87.49890960531436690 ) ) ;
#24779=CARTESIAN_POINT ( 'NONE',  ( 18.62759615963255655, 10.81492255796105972, 66.66775706135234714 ) ) ;
#24780=CARTESIAN_POINT ( 'NONE',  ( 12.06949235617739724, 12.14591786802326823, 81.87609039468568994 ) ) ;
#24781=CARTESIAN_POINT ( 'NONE',  ( 14.34966873604960469, 8.224510206698951720, 49.16557627198102409 ) ) ;
#24782=CARTESIAN_POINT ( 'NONE',  ( -5.049401038298153566, 19.05341960407611168, 60.20724293864768129 ) ) ;
#24784=CARTESIAN_POINT ( 'NONE',  ( 9.474510206698729675, 16.51473224551082808, 112.0844237280190043 ) ) ;
#24785=CARTESIAN_POINT ( 'NONE',  ( -14.34966873604960291, -8.224510206698953496, 111.6655762719810525 ) ) ;
#24786=CARTESIAN_POINT ( 'NONE',  ( -19.03943276465977164, 0.05219959533909376836, 71.24890960531435269 ) ) ;
#24787=CARTESIAN_POINT ( 'NONE',  ( 13.97604488694548053, -13.89961937509957401, 95.62609039468563310 ) ) ;
#24789=CARTESIAN_POINT ( 'NONE',  ( -18.67979575497193778, 10.72451020669871902, 98.33442372801901854 ) ) ;
#24790=CARTESIAN_POINT ( 'NONE',  ( -16.53943276465976808, -0.05219959533934237506, 68.75109039468568994 ) ) ;
#24791=CARTESIAN_POINT ( 'NONE',  ( 5.049401038297881783, 19.05341960407617563, 97.29275706135233293 ) ) ;
#24792=CARTESIAN_POINT ( 'NONE',  ( -21.53943276465977519, 0.05219959533907696930, 66.24890960531436690 ) ) ;
#24793=CARTESIAN_POINT ( 'NONE',  ( 14.29746914071037800, 8.314922557961029526, 51.66775706135234714 ) ) ;
#24795=CARTESIAN_POINT ( 'NONE',  ( -19.02544592524334988, -5.153800228976617603, 58.95942372801900433 ) ) ;
#24796=CARTESIAN_POINT ( 'NONE',  ( -5.823673210054431948, 21.52544592524334988, 97.70942372801904696 ) ) ;
#24797=CARTESIAN_POINT ( 'NONE',  ( -5.153800228976328057, -19.02544592524343514, 37.29057627198102409 ) ) ;
#24798=CARTESIAN_POINT ( 'NONE',  ( 16.51473224551069308, 9.474510206698969483, 69.16557627198102409 ) ) ;
#24799=CARTESIAN_POINT ( 'NONE',  ( -14.29746914071049879, 8.314922557960819915, 60.83224293864769550 ) ) ;
#24800=CARTESIAN_POINT ( 'NONE',  ( 21.53943276465977519, 0.05219959533937863772, 86.25109039468568994 ) ) ;
#24801=CARTESIAN_POINT ( 'NONE',  ( 16.51473224551083163, -9.474510206698727899, 50.83442372801899722 ) ) ;
#24802=CARTESIAN_POINT ( 'NONE',  ( 5.049401038297881783, 19.05341960407617563, 32.29275706135233293 ) ) ;
#24803=CARTESIAN_POINT ( 'NONE',  ( 13.89961937509977652, -13.97604488694527269, 113.1239096053143527 ) ) ;
#24804=CARTESIAN_POINT ( 'NONE',  ( 21.52544592524334988, 5.823673210054432836, 101.4594237280190185 ) ) ;
#24805=CARTESIAN_POINT ( 'NONE',  ( -13.89961937509977652, 13.97604488694528158, 80.62390960531436690 ) ) ;
#24806=CARTESIAN_POINT ( 'NONE',  ( -5.719274019375665041, -21.55341960407619695, 94.79275706135234714 ) ) ;
#24807=CARTESIAN_POINT ( 'NONE',  ( 21.52544592524344225, -5.823673210054117533, 53.54057627198103120 ) ) ;
#24808=CARTESIAN_POINT ( 'NONE',  ( -19.03943276465977164, 0.05219959533909376836, 81.24890960531436690 ) ) ;
#24809=CARTESIAN_POINT ( 'NONE',  ( 19.05341960407617918, -5.049401038297876454, 71.04275706135234714 ) ) ;
#24810=CARTESIAN_POINT ( 'NONE',  ( 16.51473224551069308, 9.474510206698969483, 44.16557627198103120 ) ) ;
#24811=CARTESIAN_POINT ( 'NONE',  ( -9.474510206698964154, 16.51473224551069663, 85.41557627198102409 ) ) ;
#24812=CARTESIAN_POINT ( 'NONE',  ( 19.03943276465977164, 0.05219959533936151252, 86.25109039468567573 ) ) ;
#24813=CARTESIAN_POINT ( 'NONE',  ( -14.29746914071037622, -8.314922557961029526, 44.16775706135234714 ) ) ;
#24814=CARTESIAN_POINT ( 'NONE',  ( -16.53943276465976808, 0.05219959533911058130, 101.2489096053143669 ) ) ;
#24815=CARTESIAN_POINT ( 'NONE',  ( -16.51473224551069308, -9.474510206698971260, 71.66557627198102409 ) ) ;
#24816=CARTESIAN_POINT ( 'NONE',  ( 21.52544592524344225, -5.823673210054117533, 48.54057627198103120 ) ) ;
#24817=CARTESIAN_POINT ( 'NONE',  ( -16.53943276465976808, -0.05219959533934237506, 33.75109039468568284 ) ) ;
#24818=CARTESIAN_POINT ( 'NONE',  ( -18.67979575497193778, 10.72451020669871902, 38.33442372801900433 ) ) ;
#24819=CARTESIAN_POINT ( 'NONE',  ( -0.05219959533937732626, 21.53943276465977519, 77.50109039468567573 ) ) ;
#24820=CARTESIAN_POINT ( 'NONE',  ( 12.06949235617739724, 12.14591786802326823, 86.87609039468568994 ) ) ;
#24821=CARTESIAN_POINT ( 'NONE',  ( -13.97604488694527625, -13.89961937509977652, 76.87390960531433848 ) ) ;
#24822=CARTESIAN_POINT ( 'NONE',  ( -4.483927247898782831, 16.52544592524335698, 102.7094237280190185 ) ) ;
#24823=CARTESIAN_POINT ( 'NONE',  ( 19.05341960407617918, -5.049401038297876454, 56.04275706135234714 ) ) ;
#24824=CARTESIAN_POINT ( 'NONE',  ( 5.719274019375673035, 21.55341960407619339, 27.29275706135234358 ) ) ;
#24825=CARTESIAN_POINT ( 'NONE',  ( -4.379528057220328563, 16.55341960407611168, 80.20724293864769550 ) ) ;
#24826=CARTESIAN_POINT ( 'NONE',  ( 13.89961937509977652, -13.97604488694527269, 98.12390960531433848 ) ) ;
#24827=CARTESIAN_POINT ( 'NONE',  ( 4.379528057220092307, 16.55341960407617563, 102.2927570613523613 ) ) ;
#24828=CARTESIAN_POINT ( 'NONE',  ( 5.823673210054444382, -21.52544592524334988, 75.20942372801901854 ) ) ;
#24829=CARTESIAN_POINT ( 'NONE',  ( -12.06949235617739369, -12.14591786802326823, 44.37609039468567573 ) ) ;
#24830=CARTESIAN_POINT ( 'NONE',  ( 21.52544592524334988, 5.823673210054432836, 31.45942372801901854 ) ) ;
#24831=CARTESIAN_POINT ( 'NONE',  ( -12.06949235617756955, 12.14591786802309770, 70.62390960531436690 ) ) ;
#24833=CARTESIAN_POINT ( 'NONE',  ( 21.52544592524344225, -5.823673210054117533, 108.5405762719810241 ) ) ;
#24834=CARTESIAN_POINT ( 'NONE',  ( -16.52544592524342804, 4.483927247898546575, 56.04057627198102409 ) ) ;
#24835=CARTESIAN_POINT ( 'NONE',  ( 9.474510206698971260, -16.51473224551069308, 27.91557627198103120 ) ) ;
#24836=CARTESIAN_POINT ( 'NONE',  ( -21.55341960407610458, -5.719274019375992779, 31.45724293864769550 ) ) ;
#24837=CARTESIAN_POINT ( 'NONE',  ( 15.80617190586769283, -15.72974639402175789, 50.62609039468568994 ) ) ;
#24838=CARTESIAN_POINT ( 'NONE',  ( 8.314922557960818139, 14.29746914071049879, 69.58224293864769550 ) ) ;
#24840=CARTESIAN_POINT ( 'NONE',  ( 0.05219959533907565091, 21.53943276465977519, 74.99890960531435269 ) ) ;
#24841=CARTESIAN_POINT ( 'NONE',  ( -19.03943276465977164, 0.05219959533909376836, 71.24890960531435269 ) ) ;
#24842=CARTESIAN_POINT ( 'NONE',  ( 19.02544592524343514, -5.153800228976328945, 43.54057627198103120 ) ) ;
#24843=CARTESIAN_POINT ( 'NONE',  ( 13.89961937509957401, 13.97604488694547697, 76.87609039468566152 ) ) ;
#24844=CARTESIAN_POINT ( 'NONE',  ( 5.719274019375673035, 21.55341960407619339, 52.29275706135236135 ) ) ;
#24845=CARTESIAN_POINT ( 'NONE',  ( -21.52544592524343514, 5.823673210054127303, 66.04057627198103830 ) ) ;
#24846=CARTESIAN_POINT ( 'NONE',  ( 16.51473224551069308, 9.474510206698969483, 44.16557627198103120 ) ) ;
#24847=CARTESIAN_POINT ( 'NONE',  ( -5.153800228976328057, -19.02544592524343514, 67.29057627198102409 ) ) ;
#24849=CARTESIAN_POINT ( 'NONE',  ( 16.53943276465976808, 0.05219959533934440121, 46.25109039468567573 ) ) ;
#24850=CARTESIAN_POINT ( 'NONE',  ( -21.52544592524334988, -5.823673210054445271, 28.95942372801902209 ) ) ;
#24851=CARTESIAN_POINT ( 'NONE',  ( 21.53943276465977519, 0.05219959533937863772, 56.25109039468568284 ) ) ;
#24852=CARTESIAN_POINT ( 'NONE',  ( 9.564922557960805705, 16.46253265017160317, 104.5822429386476955 ) ) ;
#24853=CARTESIAN_POINT ( 'NONE',  ( 5.823673210054125526, 21.52544592524343514, 79.79057627198102409 ) ) ;
#24854=CARTESIAN_POINT ( 'NONE',  ( -21.53943276465977519, -0.05219959533937600094, 28.75109039468567929 ) ) ;
#24855=CARTESIAN_POINT ( 'NONE',  ( -14.34966873604972548, 8.224510206698743886, 53.33442372801901854 ) ) ;
#24856=CARTESIAN_POINT ( 'NONE',  ( 18.62759615963271287, -10.81492255796078972, 43.33224293864769550 ) ) ;
#24857=CARTESIAN_POINT ( 'NONE',  ( -15.80617190586768217, 15.72974639402176855, 113.1260903946856899 ) ) ;
#24858=CARTESIAN_POINT ( 'NONE',  ( -19.05341960407611168, -5.049401038298163336, 56.45724293864768129 ) ) ;
#24859=CARTESIAN_POINT ( 'NONE',  ( -19.03943276465977164, 0.05219959533909376836, 106.2489096053143669 ) ) ;
#24860=CARTESIAN_POINT ( 'NONE',  ( 13.97604488694527802, 13.89961937509977652, 84.37390960531433848 ) ) ;
#24862=CARTESIAN_POINT ( 'NONE',  ( 19.03943276465977164, 0.05219959533936151252, 66.25109039468567573 ) ) ;
#24863=CARTESIAN_POINT ( 'NONE',  ( 5.719274019375991003, -21.55341960407610458, 47.70724293864770260 ) ) ;
#24865=CARTESIAN_POINT ( 'NONE',  ( -0.05219959533910754901, -16.53943276465976808, 27.49890960531435269 ) ) ;
#24866=CARTESIAN_POINT ( 'NONE',  ( 16.51473224551083163, -9.474510206698727899, 80.83442372801899012 ) ) ;
#24867=CARTESIAN_POINT ( 'NONE',  ( -16.36317988757059538, 7.306389748694926745, 59.09789608363227842 ) ) ;
#24868=CARTESIAN_POINT ( 'NONE',  ( 21.53943276465977519, 0.05219959533937863772, 111.2510903946856899 ) ) ;
#24869=CARTESIAN_POINT ( 'NONE',  ( -0.05219959533936034679, 19.03943276465977164, 97.50109039468567573 ) ) ;
#24870=CARTESIAN_POINT ( 'NONE',  ( -9.564922557961040184, 16.46253265017147172, 47.91775706135233293 ) ) ;
#24872=CARTESIAN_POINT ( 'NONE',  ( -19.02544592524342804, 5.153800228976336051, 51.04057627198103120 ) ) ;
#24873=CARTESIAN_POINT ( 'NONE',  ( -8.224510206698948167, 14.34966873604960824, 50.41557627198103120 ) ) ;
#24874=CARTESIAN_POINT ( 'NONE',  ( -13.97604488694527625, -13.89961937509977652, 31.87390960531435979 ) ) ;
#24875=CARTESIAN_POINT ( 'NONE',  ( 14.34966873604960469, 8.224510206698951720, 44.16557627198103120 ) ) ;
#24877=CARTESIAN_POINT ( 'NONE',  ( 16.55341960407618274, -4.379528057220086978, 111.0427570613523613 ) ) ;
#24878=CARTESIAN_POINT ( 'NONE',  ( 5.153800228976335163, 19.02544592524342804, 64.79057627198100988 ) ) ;
#24879=CARTESIAN_POINT ( 'NONE',  ( 16.46253265017146816, 9.564922557961045513, 21.66775706135233648 ) ) ;
#24880=CARTESIAN_POINT ( 'NONE',  ( 0.05219959533934541429, -16.53943276465976808, 40.00109039468567573 ) ) ;
#24881=CARTESIAN_POINT ( 'NONE',  ( 5.823673210054125526, 21.52544592524343514, 34.79057627198103120 ) ) ;
#24882=CARTESIAN_POINT ( 'NONE',  ( 15.80617190586769283, -15.72974639402175789, 90.62609039468567573 ) ) ;
#24884=CARTESIAN_POINT ( 'NONE',  ( -16.51473224551069308, -9.474510206698971260, 66.66557627198102409 ) ) ;
#24885=CARTESIAN_POINT ( 'NONE',  ( 5.153800228976335163, 19.02544592524342804, 104.7905762719809957 ) ) ;
#24886=CARTESIAN_POINT ( 'NONE',  ( 0.05219959533909260263, 19.03943276465977164, 99.99890960531436690 ) ) ;
#24888=CARTESIAN_POINT ( 'NONE',  ( -5.719274019375665041, -21.55341960407619695, 29.79275706135234358 ) ) ;
#24890=CARTESIAN_POINT ( 'NONE',  ( 8.314922557960818139, 14.29746914071049879, 79.58224293864769550 ) ) ;
#24891=CARTESIAN_POINT ( 'NONE',  ( -10.72451020669898014, 18.67979575497178502, 80.41557627198103830 ) ) ;
#24892=CARTESIAN_POINT ( 'NONE',  ( 16.51473224551069308, 9.474510206698969483, 69.16557627198102409 ) ) ;
#24893=CARTESIAN_POINT ( 'NONE',  ( 19.02544592524343514, -5.153800228976328945, 73.54057627198103830 ) ) ;
#24894=CARTESIAN_POINT ( 'NONE',  ( -15.72974639402176322, -15.80617190586768395, 19.37609039468568639 ) ) ;
#24895=VERTEX_POINT ( 'NONE', #75356 ) ;
#24896=CARTESIAN_POINT ( 'NONE',  ( -13.89961937509977652, 13.97604488694528158, 75.62390960531438111 ) ) ;
#24898=CARTESIAN_POINT ( 'NONE',  ( -0.05219959533910754901, -16.53943276465976808, 112.4989096053143669 ) ) ;
#24899=CARTESIAN_POINT ( 'NONE',  ( 9.564922557960805705, 16.46253265017160317, 24.58224293864769194 ) ) ;
#24900=CARTESIAN_POINT ( 'NONE',  ( 19.03943276465977164, -0.05219959533909143690, 68.74890960531436690 ) ) ;
#24901=CARTESIAN_POINT ( 'NONE',  ( 5.153800228976615827, -19.02544592524334988, 95.20942372801897591 ) ) ;
#24902=CARTESIAN_POINT ( 'NONE',  ( -12.14591786802309592, -12.06949235617757132, 96.87390960531436690 ) ) ;
#24903=CARTESIAN_POINT ( 'NONE',  ( 18.67979575497194134, -10.72451020669871369, 65.83442372801900433 ) ) ;
#24904=CARTESIAN_POINT ( 'NONE',  ( -9.564922557960796823, -16.46253265017161027, 52.08224293864768839 ) ) ;
#24905=CARTESIAN_POINT ( 'NONE',  ( -5.823673210054116645, -21.52544592524344225, 112.2905762719810241 ) ) ;
#24906=CARTESIAN_POINT ( 'NONE',  ( -21.53943276465977519, 0.05219959533907696930, 106.2489096053143811 ) ) ;
#24908=CARTESIAN_POINT ( 'NONE',  ( 5.153800228976335163, 19.02544592524342804, 74.79057627198103830 ) ) ;
#24909=CARTESIAN_POINT ( 'NONE',  ( 16.81555441253555117, 7.025013491695454526, 111.8631455466574636 ) ) ;
#24910=CARTESIAN_POINT ( 'NONE',  ( -13.89961937509957401, -13.97604488694547875, 104.3760903946856757 ) ) ;
#24911=CARTESIAN_POINT ( 'NONE',  ( -10.72451020669898014, 18.67979575497178502, 35.41557627198102409 ) ) ;
#24912=CARTESIAN_POINT ( 'NONE',  ( -5.823673210054431948, 21.52544592524334988, 52.70942372801902565 ) ) ;
#24913=CARTESIAN_POINT ( 'NONE',  ( -19.03943276465977164, 0.05219959533909376836, 96.24890960531436690 ) ) ;
#24914=( BOUNDED_CURVE ( )  B_SPLINE_CURVE ( 2, ( #39108, #80615, #142292, #197786, #71445, #195814, #12778, #103783, #43107, #181627, #180646, #165463, #134125 ),
 .UNSPECIFIED., .F., .F. ) 
 B_SPLINE_CURVE_WITH_KNOTS ( ( 3, 2, 2, 2, 2, 2, 3 ),
 ( 0.6077392741438721879, 0.6096491228070175517, 0.6140350877192982670, 0.6184210526315789824, 0.6228070175438596978, 0.6271929824561403022, 0.6291485109413760268 ),
 .UNSPECIFIED. ) 
 CURVE ( )  GEOMETRIC_REPRESENTATION_ITEM ( )  RATIONAL_B_SPLINE_CURVE ( ( 0.9832469066685285419, 0.9851625545550100060, 1.000000000000000000, 0.9659258262890683122, 1.000000000000000000, 0.9659258262890683122, 1.000000000000000000, 0.9659258262890683122, 1.000000000000000000, 0.9659258262890683122, 1.000000000000000000, 0.9848076720550078544, 0.9831626618144001517 ) ) 
 REPRESENTATION_ITEM ( '' )  );
#24915=CARTESIAN_POINT ( 'NONE',  ( -19.03943276465977164, -0.05219959533935918106, 78.75109039468567573 ) ) ;
#24916=CARTESIAN_POINT ( 'NONE',  ( -19.03943276465977164, 0.05219959533909376836, 51.24890960531436690 ) ) ;
#24917=CARTESIAN_POINT ( 'NONE',  ( 5.049401038298161559, -19.05341960407611168, 77.70724293864765286 ) ) ;
#24919=CARTESIAN_POINT ( 'NONE',  ( -16.53943276465976808, 0.05219959533911058130, 81.24890960531436690 ) ) ;
#24920=CARTESIAN_POINT ( 'NONE',  ( -13.89961937509977652, 13.97604488694528158, 105.6239096053143527 ) ) ;
#24921=CARTESIAN_POINT ( 'NONE',  ( -12.06949235617756955, 12.14591786802309770, 90.62390960531436690 ) ) ;
#24922=CARTESIAN_POINT ( 'NONE',  ( 5.153800228976335163, 19.02544592524342804, 94.79057627198103830 ) ) ;
#24923=CARTESIAN_POINT ( 'NONE',  ( -8.314922557960811034, -14.29746914071050412, 37.08224293864768129 ) ) ;
#24924=CARTESIAN_POINT ( 'NONE',  ( -13.97604488694527625, -13.89961937509977652, 26.87390960531434558 ) ) ;
#24926=CARTESIAN_POINT ( 'NONE',  ( -5.823673210054431948, 21.52544592524334988, 52.70942372801902565 ) ) ;
#24927=CARTESIAN_POINT ( 'NONE',  ( -16.51473224551082808, 9.474510206698731452, 73.33442372801900433 ) ) ;
#24928=CARTESIAN_POINT ( 'NONE',  ( 4.379528057220339221, -16.55341960407611168, 42.70724293864770260 ) ) ;
#24929=CARTESIAN_POINT ( 'NONE',  ( 18.67979575497178502, 10.72451020669898547, 99.16557627198100988 ) ) ;
#24930=CARTESIAN_POINT ( 'NONE',  ( -5.823673210054116645, -21.52544592524344225, 37.29057627198102409 ) ) ;
#24931=CARTESIAN_POINT ( 'NONE',  ( 16.53943276465976808, -0.05219959533910856209, 88.74890960531436690 ) ) ;
#24932=CARTESIAN_POINT ( 'NONE',  ( -19.02544592524342804, 5.153800228976336051, 51.04057627198103120 ) ) ;
#24933=CARTESIAN_POINT ( 'NONE',  ( 8.224510206698953496, -14.34966873604960469, 22.91557627198102765 ) ) ;
#24934=CARTESIAN_POINT ( 'NONE',  ( 16.55341960407618274, -4.379528057220086978, 101.0427570613523756 ) ) ;
#24935=CARTESIAN_POINT ( 'NONE',  ( -0.05219959533934338120, 16.53943276465976808, 67.50109039468568994 ) ) ;
#24936=CARTESIAN_POINT ( 'NONE',  ( 13.97604488694548053, -13.89961937509957401, 25.62609039468566507 ) ) ;
#24937=CARTESIAN_POINT ( 'NONE',  ( -13.89961937509977652, 13.97604488694528158, 105.6239096053143527 ) ) ;
#24938=CARTESIAN_POINT ( 'NONE',  ( -9.474510206698964154, 16.51473224551069663, 80.41557627198103830 ) ) ;
#24939=CARTESIAN_POINT ( 'NONE',  ( 19.02544592524343514, -5.153800228976328945, 38.54057627198103120 ) ) ;
#24940=CARTESIAN_POINT ( 'NONE',  ( -16.55341960407611168, -4.379528057220339221, 41.45724293864769550 ) ) ;
#24941=LINE ( 'NONE', #23928, #111366 ) ;
#24942=CARTESIAN_POINT ( 'NONE',  ( -16.46253265017160317, 9.564922557960807481, 110.8322429386476955 ) ) ;
#24943=CARTESIAN_POINT ( 'NONE',  ( -21.53943276465977519, 0.05219959533907696930, 36.24890960531435979 ) ) ;
#24944=CARTESIAN_POINT ( 'NONE',  ( -8.314922557960811034, -14.29746914071050412, 77.08224293864769550 ) ) ;
#24945=CARTESIAN_POINT ( 'NONE',  ( 16.52544592524335698, 4.483927247898782831, 31.45942372801901854 ) ) ;
#24947=CARTESIAN_POINT ( 'NONE',  ( 16.55341960407611168, 4.379528057220329451, 68.95724293864769550 ) ) ;
#24948=CARTESIAN_POINT ( 'NONE',  ( 17.50000000000000000, -3.512728167237040289, 32.72809995181130915 ) ) ;
#24949=CARTESIAN_POINT ( 'NONE',  ( 0.05219959533936267826, -19.03943276465977164, 70.00109039468566152 ) ) ;
#24950=CARTESIAN_POINT ( 'NONE',  ( 0.05219959533909260263, 19.03943276465977164, 104.9989096053143669 ) ) ;
#24951=CARTESIAN_POINT ( 'NONE',  ( 19.03943276465977164, 0.05219959533936151252, 76.25109039468566152 ) ) ;
#24952=CARTESIAN_POINT ( 'NONE',  ( -16.46253265017146816, -9.564922557961047289, 39.16775706135234003 ) ) ;
#24953=CARTESIAN_POINT ( 'NONE',  ( -13.89961937509957401, -13.97604488694547875, 109.3760903946856331 ) ) ;
#24954=CARTESIAN_POINT ( 'NONE',  ( 12.06949235617739724, 12.14591786802326823, 91.87609039468568994 ) ) ;
#24955=CARTESIAN_POINT ( 'NONE',  ( 9.474510206698971260, -16.51473224551069308, 37.91557627198102409 ) ) ;
#24956=CARTESIAN_POINT ( 'NONE',  ( -21.53943276465977519, 0.05219959533907696930, 41.24890960531435269 ) ) ;
#24957=CARTESIAN_POINT ( 'NONE',  ( 21.53943276465977519, 0.05219959533937863772, 56.25109039468568284 ) ) ;
#24959=CARTESIAN_POINT ( 'NONE',  ( 0.05219959533934541429, -16.53943276465976808, 20.00109039468568639 ) ) ;
#24961=CARTESIAN_POINT ( 'NONE',  ( 19.02544592524343514, -5.153800228976328945, 68.54057627198103830 ) ) ;
#24963=CARTESIAN_POINT ( 'NONE',  ( 12.06949235617757843, -12.14591786802309237, 93.12390960531436690 ) ) ;
#24964=CARTESIAN_POINT ( 'NONE',  ( -0.05219959533909027116, -19.03943276465977164, 82.49890960531436690 ) ) ;
#24965=CARTESIAN_POINT ( 'NONE',  ( -19.03943276465977164, 0.05219959533909376836, 81.24890960531436690 ) ) ;
#24966=VERTEX_POINT ( 'NONE', #121853 ) ;
#24967=CARTESIAN_POINT ( 'NONE',  ( 9.474510206698729675, 16.51473224551082808, 92.08442372801900433 ) ) ;
#24968=CARTESIAN_POINT ( 'NONE',  ( -15.72974639402197994, 15.80617190586746368, 60.62390960531437401 ) ) ;
#24969=CARTESIAN_POINT ( 'NONE',  ( -19.05341960407611168, -5.049401038298163336, 26.45724293864769550 ) ) ;
#24970=CARTESIAN_POINT ( 'NONE',  ( 13.97604488694548053, -13.89961937509957401, 50.62609039468566152 ) ) ;
#24971=CARTESIAN_POINT ( 'NONE',  ( -13.97604488694527625, -13.89961937509977652, 56.87390960531434558 ) ) ;
#24972=CARTESIAN_POINT ( 'NONE',  ( -9.564922557960796823, -16.46253265017161027, 92.08224293864769550 ) ) ;
#24973=ORIENTED_EDGE ( 'NONE', *, *, #198449, .F. ) ;
#24974=CARTESIAN_POINT ( 'NONE',  ( -15.72974639402197994, 15.80617190586746368, 90.62390960531436690 ) ) ;
#24975=CARTESIAN_POINT ( 'NONE',  ( 4.379528057220339221, -16.55341960407611168, 92.70724293864770971 ) ) ;
#24976=CARTESIAN_POINT ( 'NONE',  ( -19.02544592524334988, -5.153800228976617603, 58.95942372801900433 ) ) ;
#24977=CARTESIAN_POINT ( 'NONE',  ( -21.53943276465977519, 0.05219959533907696930, 96.24890960531435269 ) ) ;
#24978=CARTESIAN_POINT ( 'NONE',  ( 21.55341960407610458, 5.719274019375980345, 78.95724293864769550 ) ) ;
#24979=CARTESIAN_POINT ( 'NONE',  ( 0.05219959533910956823, 16.53943276465976808, 34.99890960531435979 ) ) ;
#24980=CARTESIAN_POINT ( 'NONE',  ( -0.05219959533937732626, 21.53943276465977519, 102.5010903946856899 ) ) ;
#24981=CARTESIAN_POINT ( 'NONE',  ( 8.224510206698742110, 14.34966873604972548, 57.08442372801901854 ) ) ;
#24982=CARTESIAN_POINT ( 'NONE',  ( -0.05219959533909027116, -19.03943276465977164, 82.49890960531436690 ) ) ;
#24983=CARTESIAN_POINT ( 'NONE',  ( -13.89961937509977652, 13.97604488694528158, 35.62390960531435269 ) ) ;
#24985=CARTESIAN_POINT ( 'NONE',  ( -21.52544592524334988, -5.823673210054445271, 43.95942372801902565 ) ) ;
#24986=CARTESIAN_POINT ( 'NONE',  ( -10.72451020669870658, -18.67979575497194134, 59.58442372801901854 ) ) ;
#24987=CARTESIAN_POINT ( 'NONE',  ( 16.46253265017160672, -9.564922557960803928, 48.33224293864769550 ) ) ;
#24988=CARTESIAN_POINT ( 'NONE',  ( 21.55341960407619695, -5.719274019375665929, 21.04275706135234714 ) ) ;
#24990=CARTESIAN_POINT ( 'NONE',  ( -16.51473224551082808, 9.474510206698731452, 58.33442372801900433 ) ) ;
#24991=CARTESIAN_POINT ( 'NONE',  ( 16.51473224551083163, -9.474510206698727899, 75.83442372801900433 ) ) ;
#24992=CARTESIAN_POINT ( 'NONE',  ( 4.483927247898790824, -16.52544592524335698, 30.20942372801902565 ) ) ;
#24993=CARTESIAN_POINT ( 'NONE',  ( -5.153800228976328057, -19.02544592524343514, 32.29057627198102409 ) ) ;
#24994=CARTESIAN_POINT ( 'NONE',  ( 16.53943276465976808, 0.05219959533934440121, 76.25109039468568994 ) ) ;
#24995=CARTESIAN_POINT ( 'NONE',  ( -5.049401038298153566, 19.05341960407611168, 45.20724293864769550 ) ) ;
#24997=CARTESIAN_POINT ( 'NONE',  ( 5.049401038298161559, -19.05341960407611168, 102.7072429386476955 ) ) ;
#24998=CARTESIAN_POINT ( 'NONE',  ( -16.46253265017160317, 9.564922557960807481, 30.83224293864769550 ) ) ;
#24999=CARTESIAN_POINT ( 'NONE',  ( 15.80617190586746368, 15.72974639402197994, 74.37390960531436690 ) ) ;
#25000=CARTESIAN_POINT ( 'NONE',  ( 14.29746914071037800, 8.314922557961029526, 61.66775706135235424 ) ) ;
#25001=CARTESIAN_POINT ( 'NONE',  ( -19.02544592524334988, -5.153800228976617603, 23.95942372801900078 ) ) ;
#25002=CARTESIAN_POINT ( 'NONE',  ( 9.474510206698971260, -16.51473224551069308, 37.91557627198102409 ) ) ;
#25003=CARTESIAN_POINT ( 'NONE',  ( -14.34966873604960291, -8.224510206698953496, 31.66557627198102054 ) ) ;
#25004=CARTESIAN_POINT ( 'NONE',  ( -8.314922557960811034, -14.29746914071050412, 72.08224293864769550 ) ) ;
#25005=CARTESIAN_POINT ( 'NONE',  ( -19.03943276465977164, 0.05219959533909376836, 71.24890960531435269 ) ) ;
#25006=CARTESIAN_POINT ( 'NONE',  ( -18.67979575497193778, 10.72451020669871902, 33.33442372801900433 ) ) ;
#25007=CARTESIAN_POINT ( 'NONE',  ( 13.97604488694527802, 13.89961937509977652, 79.37390960531435269 ) ) ;
#25008=CARTESIAN_POINT ( 'NONE',  ( 10.72451020669871369, 18.67979575497193778, 92.08442372801901854 ) ) ;
#25009=CARTESIAN_POINT ( 'NONE',  ( 0.05219959533934541429, -16.53943276465976808, 60.00109039468568284 ) ) ;
#25010=CARTESIAN_POINT ( 'NONE',  ( -9.474510206698964154, 16.51473224551069663, 110.4155762719810383 ) ) ;
#25012=CARTESIAN_POINT ( 'NONE',  ( -0.05219959533910754901, -16.53943276465976808, 42.49890960531435979 ) ) ;
#25013=CARTESIAN_POINT ( 'NONE',  ( -19.02544592524342804, 5.153800228976336051, 31.04057627198102409 ) ) ;
#25014=CARTESIAN_POINT ( 'NONE',  ( -16.52544592524335698, -4.483927247898792601, 58.95942372801902565 ) ) ;
#25015=CARTESIAN_POINT ( 'NONE',  ( -16.53943276465976808, 0.05219959533911058130, 51.24890960531436690 ) ) ;
#25016=CARTESIAN_POINT ( 'NONE',  ( -5.153800228976328057, -19.02544592524343514, 107.2905762719810383 ) ) ;
#25017=CARTESIAN_POINT ( 'NONE',  ( -0.05219959533907301413, -21.53943276465977519, 32.49890960531435979 ) ) ;
#25018=CARTESIAN_POINT ( 'NONE',  ( -5.719274019375665041, -21.55341960407619695, 109.7927570613523613 ) ) ;
#25019=CARTESIAN_POINT ( 'NONE',  ( 12.14591786802309770, 12.06949235617756955, 104.3739096053143669 ) ) ;
#25020=CARTESIAN_POINT ( 'NONE',  ( 16.46253265017160672, -9.564922557960803928, 98.33224293864769550 ) ) ;
#25022=CARTESIAN_POINT ( 'NONE',  ( -8.314922557961024197, 14.29746914071037800, 47.91775706135234714 ) ) ;
#25023=CARTESIAN_POINT ( 'NONE',  ( -5.049401038298153566, 19.05341960407611168, 60.20724293864768129 ) ) ;
#25025=CARTESIAN_POINT ( 'NONE',  ( -13.97604488694547697, 13.89961937509957934, 48.12609039468566863 ) ) ;
#25026=CARTESIAN_POINT ( 'NONE',  ( 8.224510206698742110, 14.34966873604972548, 77.08442372801901854 ) ) ;
#25027=CARTESIAN_POINT ( 'NONE',  ( 19.03943276465977164, 0.05219959533936151252, 96.25109039468567573 ) ) ;
#25028=CARTESIAN_POINT ( 'NONE',  ( 21.52544592524334988, 5.823673210054432836, 61.45942372801901854 ) ) ;
#25029=CARTESIAN_POINT ( 'NONE',  ( 13.97604488694527802, 13.89961937509977652, 79.37390960531435269 ) ) ;
#25030=CARTESIAN_POINT ( 'NONE',  ( -18.67979575497178146, -10.72451020669898902, 96.66557627198102409 ) ) ;
#25031=CARTESIAN_POINT ( 'NONE',  ( 16.46253265017160672, -9.564922557960803928, 23.33224293864769194 ) ) ;
#25033=CARTESIAN_POINT ( 'NONE',  ( 0.05219959533936267826, -19.03943276465977164, 85.00109039468567573 ) ) ;
#25034=CARTESIAN_POINT ( 'NONE',  ( -21.55341960407610458, -5.719274019375992779, 71.45724293864769550 ) ) ;
#25035=CARTESIAN_POINT ( 'NONE',  ( 19.03943276465977164, 0.05219959533936151252, 36.25109039468567573 ) ) ;
#25036=FACE_BOUND ( 'NONE', #33199, .T. ) ;
#25037=CARTESIAN_POINT ( 'NONE',  ( 21.52544592524344225, -5.823673210054117533, 88.54057627198103830 ) ) ;
#25039=CARTESIAN_POINT ( 'NONE',  ( -16.46253265017160317, 9.564922557960807481, 60.83224293864769550 ) ) ;
#25040=CARTESIAN_POINT ( 'NONE',  ( 13.89961937509978007, -13.97604488694527269, 93.12390960531435269 ) ) ;
#25041=CARTESIAN_POINT ( 'NONE',  ( -16.53943276465976808, -0.05219959533934237506, 18.75109039468568639 ) ) ;
#25042=LINE ( 'NONE', #182700, #28874 ) ;
#25043=CARTESIAN_POINT ( 'NONE',  ( -19.05341960407611168, -5.049401038298163336, 46.45724293864768129 ) ) ;
#25044=CARTESIAN_POINT ( 'NONE',  ( -19.02544592524342804, 5.153800228976336051, 106.0405762719810241 ) ) ;
#25045=CARTESIAN_POINT ( 'NONE',  ( 10.81492255796078972, 18.62759615963270932, 99.58224293864770971 ) ) ;
#25046=CARTESIAN_POINT ( 'NONE',  ( 4.483927247898545687, 16.52544592524342804, 49.79057627198102409 ) ) ;
#25047=CARTESIAN_POINT ( 'NONE',  ( -15.80617190586768217, 15.72974639402176855, 73.12609039468567573 ) ) ;
#25048=CARTESIAN_POINT ( 'NONE',  ( 8.314922557961029526, -14.29746914071037800, 30.41775706135234358 ) ) ;
#25049=CARTESIAN_POINT ( 'NONE',  ( 5.153800228976615827, -19.02544592524334988, 35.20942372801899722 ) ) ;
#25050=CARTESIAN_POINT ( 'NONE',  ( -12.06949235617756955, 12.14591786802309770, 35.62390960531437401 ) ) ;
#25051=CARTESIAN_POINT ( 'NONE',  ( -18.62759615963270932, 10.81492255796079327, 110.8322429386476955 ) ) ;
#25052=CARTESIAN_POINT ( 'NONE',  ( 16.55341960407611168, 4.379528057220329451, 48.95724293864770971 ) ) ;
#25053=CARTESIAN_POINT ( 'NONE',  ( -13.97604488694547697, 13.89961937509957934, 93.12609039468566152 ) ) ;
#25054=CARTESIAN_POINT ( 'NONE',  ( -0.05219959533936034679, 19.03943276465977164, 67.50109039468566152 ) ) ;
#25055=CARTESIAN_POINT ( 'NONE',  ( -15.80617190586768217, 15.72974639402176855, 73.12609039468567573 ) ) ;
#25056=CARTESIAN_POINT ( 'NONE',  ( -9.474510206698720793, -16.51473224551083518, 49.58442372801899722 ) ) ;
#25057=CARTESIAN_POINT ( 'NONE',  ( 9.564922557960805705, 16.46253265017160317, 24.58224293864769194 ) ) ;
#25058=CARTESIAN_POINT ( 'NONE',  ( 18.67979575497178502, 10.72451020669898547, 39.16557627198102409 ) ) ;
#25059=CARTESIAN_POINT ( 'NONE',  ( -12.14591786802309592, -12.06949235617757132, 46.87390960531435979 ) ) ;
#25060=CARTESIAN_POINT ( 'NONE',  ( -19.26498983726236602, 5.499999999999802824, 95.55319577422001487 ) ) ;
#25061=CARTESIAN_POINT ( 'NONE',  ( 9.474510206698729675, 16.51473224551082808, 22.08442372801899722 ) ) ;
#25062=CARTESIAN_POINT ( 'NONE',  ( -16.52544592524335698, -4.483927247898792601, 78.95942372801901854 ) ) ;
#25063=CARTESIAN_POINT ( 'NONE',  ( 8.314922557960818139, 14.29746914071049879, 39.58224293864769550 ) ) ;
#25064=CARTESIAN_POINT ( 'NONE',  ( 18.62759615963255655, 10.81492255796105972, 76.66775706135234714 ) ) ;
#25065=CARTESIAN_POINT ( 'NONE',  ( -18.67979575497193778, 10.72451020669871902, 68.33442372801900433 ) ) ;
#25066=CARTESIAN_POINT ( 'NONE',  ( 5.823673210054125526, 21.52544592524343514, 79.79057627198102409 ) ) ;
#25067=CARTESIAN_POINT ( 'NONE',  ( -9.474510206698964154, 16.51473224551069663, 40.41557627198103120 ) ) ;
#25068=CARTESIAN_POINT ( 'NONE',  ( -18.62759615963255300, -10.81492255796106328, 54.16775706135235424 ) ) ;
#25069=CARTESIAN_POINT ( 'NONE',  ( -16.46253265017160317, 9.564922557960807481, 35.83224293864768839 ) ) ;
#25070=CARTESIAN_POINT ( 'NONE',  ( 5.049401038298161559, -19.05341960407611168, 47.70724293864770260 ) ) ;
#25071=CARTESIAN_POINT ( 'NONE',  ( 12.14591786802309770, 12.06949235617756955, 99.37390960531436690 ) ) ;
#25072=CARTESIAN_POINT ( 'NONE',  ( 16.46253265017160672, -9.564922557960803928, 93.33224293864769550 ) ) ;
#25073=CARTESIAN_POINT ( 'NONE',  ( -16.52544592524342804, 4.483927247898546575, 46.04057627198103830 ) ) ;
#25074=CARTESIAN_POINT ( 'NONE',  ( -16.53943276465976808, 0.05219959533911058130, 96.24890960531435269 ) ) ;
#25075=CARTESIAN_POINT ( 'NONE',  ( -15.72974639402197994, 15.80617190586746368, 75.62390960531439532 ) ) ;
#25076=CARTESIAN_POINT ( 'NONE',  ( -15.72974639402176322, -15.80617190586768395, 19.37609039468568639 ) ) ;
#25078=CARTESIAN_POINT ( 'NONE',  ( 19.05341960407611168, 5.049401038298154454, 83.95724293864766707 ) ) ;
#25079=CARTESIAN_POINT ( 'NONE',  ( -4.379528057220086978, -16.55341960407618274, 19.79275706135235069 ) ) ;
#25080=CARTESIAN_POINT ( 'NONE',  ( -21.53943276465977519, 0.05219959533907696930, 66.24890960531436690 ) ) ;
#25081=CARTESIAN_POINT ( 'NONE',  ( -18.67979575497193778, 10.72451020669871902, 93.33442372801901854 ) ) ;
#25082=CARTESIAN_POINT ( 'NONE',  ( 5.153800228976335163, 19.02544592524342804, 74.79057627198103830 ) ) ;
#25083=CARTESIAN_POINT ( 'NONE',  ( -15.80617190586768217, 15.72974639402176855, 28.12609039468568284 ) ) ;
#25085=CARTESIAN_POINT ( 'NONE',  ( -19.03943276465977164, 0.05219959533909376836, 116.2489096053143669 ) ) ;
#25086=CARTESIAN_POINT ( 'NONE',  ( 16.53943276465976808, 0.05219959533934440121, 86.25109039468568994 ) ) ;
#25087=CARTESIAN_POINT ( 'NONE',  ( -0.05219959533937732626, 21.53943276465977519, 72.50109039468568994 ) ) ;
#25088=CARTESIAN_POINT ( 'NONE',  ( 0.05219959533937995610, -21.53943276465977519, 105.0010903946856757 ) ) ;
#25089=CARTESIAN_POINT ( 'NONE',  ( 14.34966873604972726, -8.224510206698740333, 65.83442372801900433 ) ) ;
#25090=CARTESIAN_POINT ( 'NONE',  ( -0.05219959533937732626, 21.53943276465977519, 22.50109039468567573 ) ) ;
#25091=CARTESIAN_POINT ( 'NONE',  ( -16.46253265017160317, 9.564922557960807481, 115.8322429386477097 ) ) ;
#25092=CARTESIAN_POINT ( 'NONE',  ( 0.05219959533937995610, -21.53943276465977519, 90.00109039468567573 ) ) ;
#25093=CARTESIAN_POINT ( 'NONE',  ( -13.97604488694527625, -13.89961937509977652, 96.87390960531433848 ) ) ;
#25094=CARTESIAN_POINT ( 'NONE',  ( 18.62759615963271287, -10.81492255796078972, 83.33224293864769550 ) ) ;
#25095=CARTESIAN_POINT ( 'NONE',  ( 16.46253265017146816, 9.564922557961045513, 56.66775706135233293 ) ) ;
#25097=CARTESIAN_POINT ( 'NONE',  ( -10.81492255796078084, -18.62759615963271287, 57.08224293864769550 ) ) ;
#25098=CARTESIAN_POINT ( 'NONE',  ( -9.564922557960796823, -16.46253265017161027, 97.08224293864769550 ) ) ;
#25099=CARTESIAN_POINT ( 'NONE',  ( 8.224510206698953496, -14.34966873604960469, 37.91557627198102409 ) ) ;
#25101=CARTESIAN_POINT ( 'NONE',  ( -0.05219959533936034679, 19.03943276465977164, 77.50109039468566152 ) ) ;
#25102=CARTESIAN_POINT ( 'NONE',  ( -17.05587630539787014, 6.762274262135693270, 105.7418030903731534 ) ) ;
#25103=CARTESIAN_POINT ( 'NONE',  ( -16.53943276465976808, -0.05219959533934237506, 18.75109039468568639 ) ) ;
#25104=CARTESIAN_POINT ( 'NONE',  ( -5.823673210054116645, -21.52544592524344225, 87.29057627198103830 ) ) ;
#25105=CARTESIAN_POINT ( 'NONE',  ( -16.53943276465976808, 0.05219959533911058130, 61.24890960531435979 ) ) ;
#25106=CARTESIAN_POINT ( 'NONE',  ( 5.049401038298161559, -19.05341960407611168, 102.7072429386476955 ) ) ;
#25107=CARTESIAN_POINT ( 'NONE',  ( -14.34966873604972548, 8.224510206698743886, 33.33442372801900433 ) ) ;
#25108=CARTESIAN_POINT ( 'NONE',  ( -0.05219959533909027116, -19.03943276465977164, 57.49890960531435979 ) ) ;
#25109=CARTESIAN_POINT ( 'NONE',  ( 21.53943276465977519, 0.05219959533937863772, 21.25109039468567218 ) ) ;
#25110=CARTESIAN_POINT ( 'NONE',  ( 16.51473224551083163, -9.474510206698727899, 80.83442372801899012 ) ) ;
#25111=CARTESIAN_POINT ( 'NONE',  ( 5.153800228976335163, 19.02544592524342804, 94.79057627198103830 ) ) ;
#25112=CARTESIAN_POINT ( 'NONE',  ( -13.89961937509977652, 13.97604488694528158, 70.62390960531432427 ) ) ;
#25113=CARTESIAN_POINT ( 'NONE',  ( -21.53943276465977519, 0.05219959533907696930, 76.24890960531435269 ) ) ;
#25114=CARTESIAN_POINT ( 'NONE',  ( 16.51473224551069308, 9.474510206698969483, 49.16557627198102409 ) ) ;
#25116=CARTESIAN_POINT ( 'NONE',  ( 4.379528057220339221, -16.55341960407611168, 57.70724293864770260 ) ) ;
#25117=CARTESIAN_POINT ( 'NONE',  ( 5.153800228976335163, 19.02544592524342804, 104.7905762719809957 ) ) ;
#25119=CARTESIAN_POINT ( 'NONE',  ( -16.51473224551082808, 9.474510206698731452, 63.33442372801900433 ) ) ;
#25120=CARTESIAN_POINT ( 'NONE',  ( 21.53943276465977519, -0.05219959533907433946, 83.74890960531435269 ) ) ;
#25121=CARTESIAN_POINT ( 'NONE',  ( -0.05219959533936034679, 19.03943276465977164, 52.50109039468566863 ) ) ;
#25122=CARTESIAN_POINT ( 'NONE',  ( -16.51473224551069308, -9.474510206698971260, 106.6655762719810383 ) ) ;
#25123=CARTESIAN_POINT ( 'NONE',  ( -17.97058386085787873, -5.499999999999975131, 74.00390968646215129 ) ) ;
#25124=CARTESIAN_POINT ( 'NONE',  ( 21.52544592524344225, -5.823673210054117533, 48.54057627198103120 ) ) ;
#25127=CARTESIAN_POINT ( 'NONE',  ( 16.46253265017160672, -9.564922557960803928, 68.33224293864770971 ) ) ;
#25128=CARTESIAN_POINT ( 'NONE',  ( 21.55341960407619695, -5.719274019375665929, 71.04275706135234714 ) ) ;
#25129=CARTESIAN_POINT ( 'NONE',  ( 13.89961937509977652, -13.97604488694527269, 38.12390960531436690 ) ) ;
#25130=CARTESIAN_POINT ( 'NONE',  ( -8.224510206698948167, 14.34966873604960824, 80.41557627198103830 ) ) ;
#25132=CARTESIAN_POINT ( 'NONE',  ( 5.719274019375673035, 21.55341960407619339, 57.29275706135234714 ) ) ;
#25133=VERTEX_POINT ( 'NONE', #111415 ) ;
#25134=CARTESIAN_POINT ( 'NONE',  ( 16.46253265017160672, -9.564922557960803928, 108.3322429386476955 ) ) ;
#25135=CARTESIAN_POINT ( 'NONE',  ( -9.564922557961040184, 16.46253265017147172, 72.91775706135233293 ) ) ;
#25137=CARTESIAN_POINT ( 'NONE',  ( 5.719274019375673035, 21.55341960407619339, 27.29275706135234358 ) ) ;
#25138=CARTESIAN_POINT ( 'NONE',  ( 5.153800228976335163, 19.02544592524342804, 64.79057627198100988 ) ) ;
#25139=CARTESIAN_POINT ( 'NONE',  ( 16.53943276465976808, 0.05219959533934440121, 41.25109039468568284 ) ) ;
#25141=CARTESIAN_POINT ( 'NONE',  ( 9.564922557961047289, -16.46253265017146816, 20.41775706135233293 ) ) ;
#25142=CARTESIAN_POINT ( 'NONE',  ( 19.05341960407611168, 5.049401038298154454, 38.95724293864767418 ) ) ;
#25143=CARTESIAN_POINT ( 'NONE',  ( -10.81492255796105439, 18.62759615963255655, 112.9177570613523329 ) ) ;
#25144=CARTESIAN_POINT ( 'NONE',  ( 16.53943276465976808, 0.05219959533934440121, 86.25109039468568994 ) ) ;
#25145=CARTESIAN_POINT ( 'NONE',  ( -13.89961937509977652, 13.97604488694528158, 85.62390960531433848 ) ) ;
#25146=CARTESIAN_POINT ( 'NONE',  ( -5.823673210054431948, 21.52544592524334988, 62.70942372801902565 ) ) ;
#25150=CARTESIAN_POINT ( 'NONE',  ( -14.29746914071037622, -8.314922557961029526, 49.16775706135234003 ) ) ;
#25151=CARTESIAN_POINT ( 'NONE',  ( -5.719274019375665041, -21.55341960407619695, 74.79275706135234714 ) ) ;
#25152=CARTESIAN_POINT ( 'NONE',  ( -0.05219959533937732626, 21.53943276465977519, 107.5010903946856899 ) ) ;
#25154=CARTESIAN_POINT ( 'NONE',  ( 12.14591786802327356, -12.06949235617739191, 30.62609039468567929 ) ) ;
#25155=CARTESIAN_POINT ( 'NONE',  ( 5.049401038298161559, -19.05341960407611168, 92.70724293864769550 ) ) ;
#25156=CARTESIAN_POINT ( 'NONE',  ( 19.05341960407611168, 5.049401038298154454, 113.9572429386477097 ) ) ;
#25159=LINE ( 'NONE', #161644, #82490 ) ;
#25160=CARTESIAN_POINT ( 'NONE',  ( -19.03943276465977164, 0.05219959533909376836, 26.24890960531435624 ) ) ;
#25161=CARTESIAN_POINT ( 'NONE',  ( -0.05219959533907301413, -21.53943276465977519, 42.49890960531435979 ) ) ;
#25162=CARTESIAN_POINT ( 'NONE',  ( 4.483927247898790824, -16.52544592524335698, 105.2094237280190328 ) ) ;
#25163=CARTESIAN_POINT ( 'NONE',  ( 16.52544592524342804, -4.483927247898539470, 78.54057627198103830 ) ) ;
#25164=CARTESIAN_POINT ( 'NONE',  ( -16.51473224551069308, -9.474510206698971260, 71.66557627198102409 ) ) ;
#25165=CARTESIAN_POINT ( 'NONE',  ( 15.80617190586769283, -15.72974639402175789, 110.6260903946857042 ) ) ;
#25166=CARTESIAN_POINT ( 'NONE',  ( 14.29746914071037800, 8.314922557961029526, 21.66775706135235069 ) ) ;
#25167=CARTESIAN_POINT ( 'NONE',  ( -12.06949235617756955, 12.14591786802309770, 90.62390960531436690 ) ) ;
#25168=CARTESIAN_POINT ( 'NONE',  ( -0.05219959533937732626, 21.53943276465977519, 47.50109039468568994 ) ) ;
#25169=CARTESIAN_POINT ( 'NONE',  ( 15.80617190586746368, 15.72974639402197994, 79.37390960531436690 ) ) ;
#25170=CARTESIAN_POINT ( 'NONE',  ( -0.05219959533936034679, 19.03943276465977164, 52.50109039468566863 ) ) ;
#25172=CARTESIAN_POINT ( 'NONE',  ( 9.564922557960805705, 16.46253265017160317, 94.58224293864769550 ) ) ;
#25173=CARTESIAN_POINT ( 'NONE',  ( 8.314922557960818139, 14.29746914071049879, 69.58224293864769550 ) ) ;
#25174=CARTESIAN_POINT ( 'NONE',  ( 14.34966873604960469, 8.224510206698951720, 49.16557627198102409 ) ) ;
#25175=CARTESIAN_POINT ( 'NONE',  ( -0.05219959533910754901, -16.53943276465976808, 22.49890960531436335 ) ) ;
#25176=CARTESIAN_POINT ( 'NONE',  ( 16.51473224551083163, -9.474510206698727899, 65.83442372801900433 ) ) ;
#25177=CARTESIAN_POINT ( 'NONE',  ( 13.97604488694548053, -13.89961937509957401, 90.62609039468566152 ) ) ;
#25178=CARTESIAN_POINT ( 'NONE',  ( -19.02544592524342804, 5.153800228976336051, 116.0405762719810383 ) ) ;
#25179=ADVANCED_FACE ( 'NONE', ( #19413 ), #183994, .T. ) ;
#25180=CARTESIAN_POINT ( 'NONE',  ( 14.29746914071049879, -8.314922557960816363, 83.33224293864769550 ) ) ;
#25182=CARTESIAN_POINT ( 'NONE',  ( -5.153800228976328057, -19.02544592524343514, 47.29057627198102409 ) ) ;
#25183=CARTESIAN_POINT ( 'NONE',  ( 10.72451020669898902, -18.67979575497178502, 52.91557627198103830 ) ) ;
#25184=CARTESIAN_POINT ( 'NONE',  ( 10.81492255796078972, 18.62759615963270932, 74.58224293864768129 ) ) ;
#25185=CARTESIAN_POINT ( 'NONE',  ( 16.53943276465976808, -0.05219959533910856209, 113.7489096053143527 ) ) ;
#25186=CARTESIAN_POINT ( 'NONE',  ( 0.05219959533934541429, -16.53943276465976808, 60.00109039468568284 ) ) ;
#25187=CARTESIAN_POINT ( 'NONE',  ( -5.153800228976328057, -19.02544592524343514, 57.29057627198103120 ) ) ;
#25188=CARTESIAN_POINT ( 'NONE',  ( -9.564922557961040184, 16.46253265017147172, 37.91775706135233293 ) ) ;
#25189=CARTESIAN_POINT ( 'NONE',  ( -21.55341960407619339, 5.719274019375674811, 48.54275706135234714 ) ) ;
#25190=CARTESIAN_POINT ( 'NONE',  ( 4.483927247898545687, 16.52544592524342804, 109.7905762719810383 ) ) ;
#25191=CARTESIAN_POINT ( 'NONE',  ( 16.46253265017146816, 9.564922557961045513, 96.66775706135233293 ) ) ;
#25193=DIRECTION ( 'NONE',  ( 0.000000000000000000, 0.000000000000000000, 1.000000000000000000 ) ) ;
#25194=CARTESIAN_POINT ( 'NONE',  ( -15.80617190586745835, -15.72974639402198527, 51.87390960531437401 ) ) ;
#25195=CARTESIAN_POINT ( 'NONE',  ( 16.20579543436674541, -7.371946100355224019, 66.93479165828121324 ) ) ;
#25196=CARTESIAN_POINT ( 'NONE',  ( 21.53943276465977519, 0.05219959533937863772, 81.25109039468568994 ) ) ;
#25197=CARTESIAN_POINT ( 'NONE',  ( 12.14591786802309770, 12.06949235617756955, 39.37390960531436690 ) ) ;
#25198=CARTESIAN_POINT ( 'NONE',  ( -0.05219959533934338120, 16.53943276465976808, 57.50109039468568994 ) ) ;
#25199=CARTESIAN_POINT ( 'NONE',  ( 12.06949235617757843, -12.14591786802309237, 38.12390960531436690 ) ) ;
#25200=CARTESIAN_POINT ( 'NONE',  ( 15.80617190586746368, 15.72974639402197994, 79.37390960531436690 ) ) ;
#25202=CARTESIAN_POINT ( 'NONE',  ( -21.55341960407610458, -5.719274019375992779, 76.45724293864769550 ) ) ;
#25204=CARTESIAN_POINT ( 'NONE',  ( -19.05341960407617563, 5.049401038297882671, 78.54275706135233293 ) ) ;
#25205=CARTESIAN_POINT ( 'NONE',  ( 9.564922557960805705, 16.46253265017160317, 114.5822429386476955 ) ) ;
#25206=CARTESIAN_POINT ( 'NONE',  ( -0.05219959533909027116, -19.03943276465977164, 47.49890960531435979 ) ) ;
#25207=CARTESIAN_POINT ( 'NONE',  ( -19.05341960407611168, -5.049401038298163336, 36.45724293864766707 ) ) ;
#25209=LINE ( 'NONE', #145514, #196311 ) ;
#25211=CARTESIAN_POINT ( 'NONE',  ( 14.29746914071037800, 8.314922557961029526, 81.66775706135236135 ) ) ;
#25212=CARTESIAN_POINT ( 'NONE',  ( 15.72974639402199770, -15.80617190586745480, 108.1239096053143811 ) ) ;
#25213=CARTESIAN_POINT ( 'NONE',  ( 16.51473224551069308, 9.474510206698969483, 69.16557627198102409 ) ) ;
#25214=CARTESIAN_POINT ( 'NONE',  ( 0.05219959533937995610, -21.53943276465977519, 40.00109039468567573 ) ) ;
#25215=CARTESIAN_POINT ( 'NONE',  ( 0.05219959533909260263, 19.03943276465977164, 89.99890960531436690 ) ) ;
#25218=CARTESIAN_POINT ( 'NONE',  ( -18.67979575497193778, 10.72451020669871902, 33.33442372801900433 ) ) ;
#25219=CARTESIAN_POINT ( 'NONE',  ( 13.89961937509977652, -13.97604488694527269, 28.12390960531435624 ) ) ;
#25220=CARTESIAN_POINT ( 'NONE',  ( -5.049401038298153566, 19.05341960407611168, 110.2072429386476671 ) ) ;
#25221=CARTESIAN_POINT ( 'NONE',  ( 9.564922557961047289, -16.46253265017146816, 40.41775706135234003 ) ) ;
#25222=CARTESIAN_POINT ( 'NONE',  ( -15.72974639402176322, -15.80617190586768395, 19.37609039468568639 ) ) ;
#25223=CARTESIAN_POINT ( 'NONE',  ( -0.05219959533936034679, 19.03943276465977164, 42.50109039468566152 ) ) ;
#25224=CARTESIAN_POINT ( 'NONE',  ( -19.02544592524334988, -5.153800228976617603, 48.95942372801900433 ) ) ;
#25225=CARTESIAN_POINT ( 'NONE',  ( 12.14591786802327356, -12.06949235617739191, 85.62609039468568994 ) ) ;
#25226=CARTESIAN_POINT ( 'NONE',  ( -19.03943276465977164, 0.05219959533909376836, 116.2489096053143669 ) ) ;
#25228=CARTESIAN_POINT ( 'NONE',  ( 0.05219959533909260263, 19.03943276465977164, 74.99890960531435269 ) ) ;
#25229=CARTESIAN_POINT ( 'NONE',  ( 21.55341960407619695, -5.719274019375665929, 81.04275706135236135 ) ) ;
#25230=CARTESIAN_POINT ( 'NONE',  ( 21.55341960407619695, -5.719274019375665929, 96.04275706135236135 ) ) ;
#25232=CARTESIAN_POINT ( 'NONE',  ( -16.46253265017160317, 9.564922557960807481, 90.83224293864769550 ) ) ;
#25233=CARTESIAN_POINT ( 'NONE',  ( -10.81492255796105439, 18.62759615963255655, 57.91775706135234714 ) ) ;
#25234=CARTESIAN_POINT ( 'NONE',  ( -13.97604488694547697, 13.89961937509957934, 108.1260903946856331 ) ) ;
#25235=CARTESIAN_POINT ( 'NONE',  ( -13.97604488694527625, -13.89961937509977652, 71.87390960531433848 ) ) ;
#25236=CARTESIAN_POINT ( 'NONE',  ( 0.05219959533909260263, 19.03943276465977164, 109.9989096053143669 ) ) ;
#25237=CARTESIAN_POINT ( 'NONE',  ( -19.05341960407611168, -5.049401038298163336, 86.45724293864769550 ) ) ;
#25239=CARTESIAN_POINT ( 'NONE',  ( -16.51473224551069308, -9.474510206698971260, 66.66557627198102409 ) ) ;
#25240=CARTESIAN_POINT ( 'NONE',  ( 19.02544592524343514, -5.153800228976328945, 53.54057627198102409 ) ) ;
#25241=CARTESIAN_POINT ( 'NONE',  ( 21.55341960407619695, -5.719274019375665929, 21.04275706135234714 ) ) ;
#25242=CARTESIAN_POINT ( 'NONE',  ( -8.224510206698735004, -14.34966873604973081, 104.5844237280190185 ) ) ;
#25244=CARTESIAN_POINT ( 'NONE',  ( -19.05341960407617563, 5.049401038297882671, 58.54275706135234003 ) ) ;
#25245=CARTESIAN_POINT ( 'NONE',  ( -16.46253265017160317, 9.564922557960807481, 90.83224293864769550 ) ) ;
#25246=CARTESIAN_POINT ( 'NONE',  ( -16.53943276465976808, 0.05219959533911058130, 76.24890960531435269 ) ) ;
#25247=CARTESIAN_POINT ( 'NONE',  ( -14.34966873604960291, -8.224510206698953496, 111.6655762719810525 ) ) ;
#25248=CARTESIAN_POINT ( 'NONE',  ( 0.05219959533907565091, 21.53943276465977519, 29.99890960531435979 ) ) ;
#25249=CARTESIAN_POINT ( 'NONE',  ( -15.80617190586745835, -15.72974639402198527, 21.87390960531436690 ) ) ;
#25250=CARTESIAN_POINT ( 'NONE',  ( -4.483927247898539470, -16.52544592524342804, 92.29057627198103830 ) ) ;
#25251=CARTESIAN_POINT ( 'NONE',  ( -16.88567814943165502, 6.947325034625572826, 53.70998877347415146 ) ) ;
#25252=CARTESIAN_POINT ( 'NONE',  ( -16.51473224551082808, 9.474510206698731452, 48.33442372801900433 ) ) ;
#25253=CARTESIAN_POINT ( 'NONE',  ( -12.06949235617739369, -12.14591786802326823, 109.3760903946857042 ) ) ;
#25254=CARTESIAN_POINT ( 'NONE',  ( -5.049401038298153566, 19.05341960407611168, 85.20724293864766707 ) ) ;
#25255=CARTESIAN_POINT ( 'NONE',  ( -15.72974639402176322, -15.80617190586768395, 49.37609039468569705 ) ) ;
#25256=CARTESIAN_POINT ( 'NONE',  ( -5.823673210054116645, -21.52544592524344225, 47.29057627198103120 ) ) ;
#25257=CARTESIAN_POINT ( 'NONE',  ( 0.05219959533937995610, -21.53943276465977519, 30.00109039468568284 ) ) ;
#25258=CARTESIAN_POINT ( 'NONE',  ( -21.53943276465977519, 0.05219959533907696930, 86.24890960531436690 ) ) ;
#25259=CARTESIAN_POINT ( 'NONE',  ( -4.483927247898539470, -16.52544592524342804, 102.2905762719810383 ) ) ;
#25260=CARTESIAN_POINT ( 'NONE',  ( -19.03943276465977164, -0.05219959533935918106, 63.75109039468566863 ) ) ;
#25261=CARTESIAN_POINT ( 'NONE',  ( 5.049401038298161559, -19.05341960407611168, 42.70724293864767418 ) ) ;
#25262=CARTESIAN_POINT ( 'NONE',  ( -5.049401038298153566, 19.05341960407611168, 95.20724293864770971 ) ) ;
#25263=CARTESIAN_POINT ( 'NONE',  ( 0.05219959533909260263, 19.03943276465977164, 99.99890960531436690 ) ) ;
#25264=CARTESIAN_POINT ( 'NONE',  ( -19.03943276465977164, 0.05219959533909376836, 21.24890960531436335 ) ) ;
#25265=CARTESIAN_POINT ( 'NONE',  ( 4.483927247898545687, 16.52544592524342804, 44.79057627198103120 ) ) ;
#25266=CARTESIAN_POINT ( 'NONE',  ( 4.379528057220092307, 16.55341960407617563, 37.29275706135235424 ) ) ;
#25267=CARTESIAN_POINT ( 'NONE',  ( 21.55341960407619695, -5.719274019375665929, 106.0427570613523471 ) ) ;
#25269=CARTESIAN_POINT ( 'NONE',  ( 16.46253265017160672, -9.564922557960803928, 113.3322429386476955 ) ) ;
#25270=CARTESIAN_POINT ( 'NONE',  ( 12.06949235617739724, 12.14591786802326823, 111.8760903946856615 ) ) ;
#25271=CARTESIAN_POINT ( 'NONE',  ( 21.53943276465977519, 0.05219959533937863772, 36.25109039468567573 ) ) ;
#25272=CARTESIAN_POINT ( 'NONE',  ( -19.03943276465977164, 0.05219959533909376836, 106.2489096053143669 ) ) ;
#25273=CARTESIAN_POINT ( 'NONE',  ( -14.34966873604972548, 8.224510206698743886, 53.33442372801901854 ) ) ;
#25274=CARTESIAN_POINT ( 'NONE',  ( 14.29746914071037800, 8.314922557961029526, 101.6677570613523613 ) ) ;
#25275=CARTESIAN_POINT ( 'NONE',  ( 0.05219959533934541429, -16.53943276465976808, 95.00109039468568994 ) ) ;
#25276=CARTESIAN_POINT ( 'NONE',  ( 8.224510206698742110, 14.34966873604972548, 32.08442372801901854 ) ) ;
#25277=CARTESIAN_POINT ( 'NONE',  ( 16.46253265017160672, -9.564922557960803928, 48.33224293864769550 ) ) ;
#25278=CARTESIAN_POINT ( 'NONE',  ( 16.55341960407611168, 4.379528057220329451, 103.9572429386476813 ) ) ;
#25279=CARTESIAN_POINT ( 'NONE',  ( -15.80617190586768217, 15.72974639402176855, 23.12609039468567573 ) ) ;
#25280=CARTESIAN_POINT ( 'NONE',  ( 13.89961937509977652, -13.97604488694527269, 38.12390960531436690 ) ) ;
#25281=CARTESIAN_POINT ( 'NONE',  ( -16.46253265017160317, 9.564922557960807481, 110.8322429386476955 ) ) ;
#25282=CARTESIAN_POINT ( 'NONE',  ( 10.81492255796106328, -18.62759615963255655, 30.41775706135234358 ) ) ;
#25283=CARTESIAN_POINT ( 'NONE',  ( 16.46253265017160672, -9.564922557960803928, 23.33224293864769194 ) ) ;
#25284=CARTESIAN_POINT ( 'NONE',  ( 5.049401038298161559, -19.05341960407611168, 107.7072429386476955 ) ) ;
#25286=CARTESIAN_POINT ( 'NONE',  ( -5.153800228976328057, -19.02544592524343514, 97.29057627198099567 ) ) ;
#25287=CARTESIAN_POINT ( 'NONE',  ( 15.80617190586769283, -15.72974639402175789, 50.62609039468568994 ) ) ;
#25288=CARTESIAN_POINT ( 'NONE',  ( 8.314922557960818139, 14.29746914071049879, 89.58224293864768129 ) ) ;
#25289=CARTESIAN_POINT ( 'NONE',  ( 13.89961937509977652, -13.97604488694527269, 103.1239096053143527 ) ) ;
#25290=CARTESIAN_POINT ( 'NONE',  ( 9.564922557961047289, -16.46253265017146816, 70.41775706135233293 ) ) ;
#25291=CARTESIAN_POINT ( 'NONE',  ( 16.55341960407618274, -4.379528057220086978, 66.04275706135236135 ) ) ;
#25292=CARTESIAN_POINT ( 'NONE',  ( 21.55341960407619695, -5.719274019375665929, 76.04275706135237556 ) ) ;
#25294=CARTESIAN_POINT ( 'NONE',  ( -4.379528057220086978, -16.55341960407618274, 34.79275706135235424 ) ) ;
#25295=CARTESIAN_POINT ( 'NONE',  ( 16.51473224551069308, 9.474510206698969483, 79.16557627198103830 ) ) ;
#25296=CARTESIAN_POINT ( 'NONE',  ( -16.46253265017146816, -9.564922557961047289, 104.1677570613523329 ) ) ;
#25297=CARTESIAN_POINT ( 'NONE',  ( 12.14591786802327356, -12.06949235617739191, 75.62609039468567573 ) ) ;
#25298=CARTESIAN_POINT ( 'NONE',  ( -10.81492255796105439, 18.62759615963255655, 112.9177570613523329 ) ) ;
#25299=CARTESIAN_POINT ( 'NONE',  ( -13.89961937509957401, -13.97604488694547875, 94.37609039468566152 ) ) ;
#25300=CARTESIAN_POINT ( 'NONE',  ( 9.564922557960805705, 16.46253265017160317, 59.58224293864769550 ) ) ;
#25301=CARTESIAN_POINT ( 'NONE',  ( -10.81492255796078084, -18.62759615963271287, 82.08224293864768129 ) ) ;
#25302=CARTESIAN_POINT ( 'NONE',  ( 12.14591786802309770, 12.06949235617756955, 94.37390960531436690 ) ) ;
#25303=CARTESIAN_POINT ( 'NONE',  ( 9.474510206698729675, 16.51473224551082808, 92.08442372801900433 ) ) ;
#25304=CARTESIAN_POINT ( 'NONE',  ( 0.05219959533934541429, -16.53943276465976808, 65.00109039468568994 ) ) ;
#25305=CARTESIAN_POINT ( 'NONE',  ( -19.49149378614660577, 5.499999999999577227, 79.43757513605360998 ) ) ;
#25306=CARTESIAN_POINT ( 'NONE',  ( 13.89961937509957401, 13.97604488694547697, 51.87609039468566863 ) ) ;
#25307=CARTESIAN_POINT ( 'NONE',  ( 14.29746914071049879, -8.314922557960816363, 28.33224293864769550 ) ) ;
#25308=CARTESIAN_POINT ( 'NONE',  ( 0.05219959533910956823, 16.53943276465976808, 84.99890960531436690 ) ) ;
#25309=CARTESIAN_POINT ( 'NONE',  ( 18.62759615963255655, 10.81492255796105972, 111.6677570613523613 ) ) ;
#25310=CARTESIAN_POINT ( 'NONE',  ( -17.26172910966715790, 6.454744622556963130, 40.80646908649207205 ) ) ;
#25311=CARTESIAN_POINT ( 'NONE',  ( 10.72451020669871369, 18.67979575497193778, 22.08442372801901143 ) ) ;
#25312=CARTESIAN_POINT ( 'NONE',  ( 16.46253265017160672, -9.564922557960803928, 98.33224293864769550 ) ) ;
#25313=CARTESIAN_POINT ( 'NONE',  ( 13.97604488694527802, 13.89961937509977652, 79.37390960531435269 ) ) ;
#25314=CARTESIAN_POINT ( 'NONE',  ( -15.80617190586768217, 15.72974639402176855, 98.12609039468570415 ) ) ;
#25315=CARTESIAN_POINT ( 'NONE',  ( 9.564922557960805705, 16.46253265017160317, 79.58224293864769550 ) ) ;
#25316=CARTESIAN_POINT ( 'NONE',  ( 15.72974639402199770, -15.80617190586745480, 48.12390960531436690 ) ) ;
#25317=CARTESIAN_POINT ( 'NONE',  ( -8.314922557960811034, -14.29746914071050412, 87.08224293864769550 ) ) ;
#25318=CARTESIAN_POINT ( 'NONE',  ( -0.05219959533909027116, -19.03943276465977164, 57.49890960531435979 ) ) ;
#25319=CARTESIAN_POINT ( 'NONE',  ( 4.483927247898545687, 16.52544592524342804, 99.79057627198103830 ) ) ;
#25320=CARTESIAN_POINT ( 'NONE',  ( -10.72451020669870658, -18.67979575497194134, 29.58442372801901854 ) ) ;
#25321=CARTESIAN_POINT ( 'NONE',  ( 10.72451020669871369, 18.67979575497193778, 67.08442372801901854 ) ) ;
#25322=CARTESIAN_POINT ( 'NONE',  ( 9.564922557960805705, 16.46253265017160317, 49.58224293864770260 ) ) ;
#25323=CARTESIAN_POINT ( 'NONE',  ( -16.55341960407617563, 4.379528057220093196, 58.54275706135235424 ) ) ;
#25324=CARTESIAN_POINT ( 'NONE',  ( -10.72451020669898014, 18.67979575497178502, 110.4155762719810383 ) ) ;
#25325=CARTESIAN_POINT ( 'NONE',  ( -10.72451020669898014, 18.67979575497178502, 110.4155762719810383 ) ) ;
#25326=CARTESIAN_POINT ( 'NONE',  ( -0.05219959533936034679, 19.03943276465977164, 42.50109039468566152 ) ) ;
#25327=CARTESIAN_POINT ( 'NONE',  ( -16.51473224551069308, -9.474510206698971260, 71.66557627198102409 ) ) ;
#25329=CARTESIAN_POINT ( 'NONE',  ( 15.72974639402176855, 15.80617190586768217, 71.87609039468568994 ) ) ;
#25331=CARTESIAN_POINT ( 'NONE',  ( -21.52544592524343514, 5.823673210054127303, 56.04057627198102409 ) ) ;
#25332=CARTESIAN_POINT ( 'NONE',  ( 4.379528057220339221, -16.55341960407611168, 37.70724293864769550 ) ) ;
#25333=CARTESIAN_POINT ( 'NONE',  ( 15.80617190586769283, -15.72974639402175789, 70.62609039468567573 ) ) ;
#25334=CARTESIAN_POINT ( 'NONE',  ( 9.564922557961047289, -16.46253265017146816, 20.41775706135233293 ) ) ;
#25335=CARTESIAN_POINT ( 'NONE',  ( -0.05219959533910754901, -16.53943276465976808, 57.49890960531435979 ) ) ;
#25336=CARTESIAN_POINT ( 'NONE',  ( -4.379528057220328563, 16.55341960407611168, 100.2072429386476955 ) ) ;
#25337=CARTESIAN_POINT ( 'NONE',  ( -16.46253265017146816, -9.564922557961047289, 49.16775706135233293 ) ) ;
#25338=CARTESIAN_POINT ( 'NONE',  ( -16.53943276465976808, 0.05219959533911058130, 21.24890960531436690 ) ) ;
#25339=CARTESIAN_POINT ( 'NONE',  ( 15.80617190586769283, -15.72974639402175789, 70.62609039468567573 ) ) ;
#25340=CARTESIAN_POINT ( 'NONE',  ( -5.153800228976328057, -19.02544592524343514, 62.29057627198100988 ) ) ;
#25341=CARTESIAN_POINT ( 'NONE',  ( -9.474510206698720793, -16.51473224551083518, 34.58442372801899722 ) ) ;
#25342=CARTESIAN_POINT ( 'NONE',  ( 10.81492255796078972, 18.62759615963270932, 44.58224293864769550 ) ) ;
#25343=CARTESIAN_POINT ( 'NONE',  ( 0.05219959533937995610, -21.53943276465977519, 35.00109039468568284 ) ) ;
#25344=CARTESIAN_POINT ( 'NONE',  ( -21.55341960407610458, -5.719274019375992779, 86.45724293864770971 ) ) ;
#25345=CARTESIAN_POINT ( 'NONE',  ( 9.564922557961047289, -16.46253265017146816, 90.41775706135234714 ) ) ;
#25346=CARTESIAN_POINT ( 'NONE',  ( 16.52544592524335698, 4.483927247898782831, 46.45942372801901854 ) ) ;
#25347=CARTESIAN_POINT ( 'NONE',  ( -17.72517630440430025, 5.500000000000144773, 55.92175719257211597 ) ) ;
#25348=CARTESIAN_POINT ( 'NONE',  ( 15.72974639402199770, -15.80617190586745480, 88.12390960531436690 ) ) ;
#25349=CARTESIAN_POINT ( 'NONE',  ( -8.314922557960811034, -14.29746914071050412, 92.08224293864769550 ) ) ;
#25350=CARTESIAN_POINT ( 'NONE',  ( 18.09867054820433907, 5.499999999999817923, 41.48393025253587751 ) ) ;
#25351=CARTESIAN_POINT ( 'NONE',  ( -16.55341960407617563, 4.379528057220093196, 23.54275706135235424 ) ) ;
#25352=CARTESIAN_POINT ( 'NONE',  ( 5.719274019375991003, -21.55341960407610458, 52.70724293864769550 ) ) ;
#25353=CARTESIAN_POINT ( 'NONE',  ( -14.34966873604972548, 8.224510206698743886, 88.33442372801901854 ) ) ;
#25354=CARTESIAN_POINT ( 'NONE',  ( 16.51473224551069308, 9.474510206698969483, 24.16557627198102765 ) ) ;
#25355=CARTESIAN_POINT ( 'NONE',  ( -12.14591786802326823, 12.06949235617739902, 58.12609039468568994 ) ) ;
#25356=CARTESIAN_POINT ( 'NONE',  ( 21.55341960407619695, -5.719274019375665929, 26.04275706135235779 ) ) ;
#25357=CARTESIAN_POINT ( 'NONE',  ( -0.05219959533907301413, -21.53943276465977519, 47.49890960531435979 ) ) ;
#25358=CARTESIAN_POINT ( 'NONE',  ( -8.314922557961024197, 14.29746914071037800, 77.91775706135231871 ) ) ;
#25359=CARTESIAN_POINT ( 'NONE',  ( -16.51473224551069308, -9.474510206698971260, 96.66557627198102409 ) ) ;
#25360=CARTESIAN_POINT ( 'NONE',  ( -0.05219959533937732626, 21.53943276465977519, 57.50109039468568994 ) ) ;
#25361=CARTESIAN_POINT ( 'NONE',  ( -19.03943276465977164, 0.05219959533909376836, 26.24890960531435624 ) ) ;
#25362=CARTESIAN_POINT ( 'NONE',  ( -18.67979575497178146, -10.72451020669898902, 41.66557627198103120 ) ) ;
#25363=CARTESIAN_POINT ( 'NONE',  ( 5.153800228976335163, 19.02544592524342804, 109.7905762719810099 ) ) ;
#25365=CARTESIAN_POINT ( 'NONE',  ( 9.474510206698729675, 16.51473224551082808, 42.08442372801900433 ) ) ;
#25366=CARTESIAN_POINT ( 'NONE',  ( 8.314922557961029526, -14.29746914071037800, 60.41775706135235424 ) ) ;
#25367=CARTESIAN_POINT ( 'NONE',  ( 19.05341960407611168, 5.049401038298154454, 113.9572429386477097 ) ) ;
#25369=CARTESIAN_POINT ( 'NONE',  ( -13.97604488694527625, -13.89961937509977652, 86.87390960531436690 ) ) ;
#25370=CARTESIAN_POINT ( 'NONE',  ( -14.29746914071037622, -8.314922557961029526, 99.16775706135234714 ) ) ;
#25371=CARTESIAN_POINT ( 'NONE',  ( 17.49999999999999645, 5.500000000000007994, 73.78230962303568674 ) ) ;
#25372=CARTESIAN_POINT ( 'NONE',  ( -8.314922557960811034, -14.29746914071050412, 97.08224293864770971 ) ) ;
#25373=CARTESIAN_POINT ( 'NONE',  ( 18.62759615963271287, -10.81492255796078972, 53.33224293864769550 ) ) ;
#25374=CARTESIAN_POINT ( 'NONE',  ( 5.049401038298161559, -19.05341960407611168, 37.70724293864768839 ) ) ;
#25375=CARTESIAN_POINT ( 'NONE',  ( -0.05219959533934338120, 16.53943276465976808, 77.50109039468567573 ) ) ;
#25376=CARTESIAN_POINT ( 'NONE',  ( -21.52544592524334988, -5.823673210054445271, 33.95942372801901143 ) ) ;
#25377=CARTESIAN_POINT ( 'NONE',  ( -19.02544592524334988, -5.153800228976617603, 93.95942372801900433 ) ) ;
#25378=CARTESIAN_POINT ( 'NONE',  ( -16.46253265017160317, 9.564922557960807481, 40.83224293864769550 ) ) ;
#25379=CARTESIAN_POINT ( 'NONE',  ( -19.03943276465977164, 0.05219959533909376836, 116.2489096053143669 ) ) ;
#25380=CARTESIAN_POINT ( 'NONE',  ( 21.55341960407619695, -5.719274019375665929, 101.0427570613523756 ) ) ;
#25381=CARTESIAN_POINT ( 'NONE',  ( 16.51473224551069308, 9.474510206698969483, 84.16557627198102409 ) ) ;
#25382=CARTESIAN_POINT ( 'NONE',  ( -14.34966873604972548, 8.224510206698743886, 58.33442372801901143 ) ) ;
#25383=CARTESIAN_POINT ( 'NONE',  ( -21.55341960407619339, 5.719274019375674811, 93.54275706135234714 ) ) ;
#25384=CARTESIAN_POINT ( 'NONE',  ( 0.05219959533934541429, -16.53943276465976808, 60.00109039468568284 ) ) ;
#25385=CARTESIAN_POINT ( 'NONE',  ( 16.51473224551083163, -9.474510206698727899, 50.83442372801899722 ) ) ;
#25386=CARTESIAN_POINT ( 'NONE',  ( 19.02544592524334988, 5.153800228976608722, 66.45942372801899012 ) ) ;
#25388=CARTESIAN_POINT ( 'NONE',  ( -10.81492255796105439, 18.62759615963255655, 57.91775706135234714 ) ) ;
#25389=CARTESIAN_POINT ( 'NONE',  ( -9.564922557960796823, -16.46253265017161027, 67.08224293864769550 ) ) ;
#25390=CARTESIAN_POINT ( 'NONE',  ( 19.05341960407611168, 5.049401038298154454, 23.95724293864769194 ) ) ;
#25391=CARTESIAN_POINT ( 'NONE',  ( 9.564922557961047289, -16.46253265017146816, 55.41775706135234003 ) ) ;
#25392=CARTESIAN_POINT ( 'NONE',  ( -13.89961937509977652, 13.97604488694528158, 110.6239096053143243 ) ) ;
#25393=CARTESIAN_POINT ( 'NONE',  ( -19.05341960407611168, -5.049401038298163336, 81.45724293864769550 ) ) ;
#25394=CARTESIAN_POINT ( 'NONE',  ( 8.224510206698953496, -14.34966873604960469, 32.91557627198102409 ) ) ;
#25395=CARTESIAN_POINT ( 'NONE',  ( -0.05219959533907301413, -21.53943276465977519, 52.49890960531435979 ) ) ;
#25397=CARTESIAN_POINT ( 'NONE',  ( -19.03943276465977164, -0.05219959533935918106, 18.75109039468567218 ) ) ;
#25399=CARTESIAN_POINT ( 'NONE',  ( 19.05341960407611168, 5.049401038298154454, 38.95724293864767418 ) ) ;
#25400=CARTESIAN_POINT ( 'NONE',  ( -5.049401038298153566, 19.05341960407611168, 25.20724293864768484 ) ) ;
#25402=CARTESIAN_POINT ( 'NONE',  ( -18.67979575497193778, 10.72451020669871902, 68.33442372801900433 ) ) ;
#25404=CARTESIAN_POINT ( 'NONE',  ( -16.52544592524335698, -4.483927247898792601, 68.95942372801901854 ) ) ;
#25405=CARTESIAN_POINT ( 'NONE',  ( 10.72451020669898902, -18.67979575497178502, 77.91557627198102409 ) ) ;
#25406=CARTESIAN_POINT ( 'NONE',  ( -16.55341960407611168, -4.379528057220339221, 51.45724293864770260 ) ) ;
#25407=CARTESIAN_POINT ( 'NONE',  ( -9.564922557960796823, -16.46253265017161027, 32.08224293864769550 ) ) ;
#25408=CARTESIAN_POINT ( 'NONE',  ( -19.02544592524342804, 5.153800228976336051, 111.0405762719810099 ) ) ;
#25409=CARTESIAN_POINT ( 'NONE',  ( -5.823673210054431948, 21.52544592524334988, 37.70942372801900433 ) ) ;
#25410=CARTESIAN_POINT ( 'NONE',  ( 19.02544592524334988, 5.153800228976608722, 51.45942372801900433 ) ) ;
#25411=CARTESIAN_POINT ( 'NONE',  ( 5.049401038298161559, -19.05341960407611168, 27.70724293864769550 ) ) ;
#25412=CARTESIAN_POINT ( 'NONE',  ( -5.719274019375665041, -21.55341960407619695, 84.79275706135234714 ) ) ;
#25413=CARTESIAN_POINT ( 'NONE',  ( 16.88567814943165857, -6.947325034625568385, 31.20998877347416212 ) ) ;
#25414=CARTESIAN_POINT ( 'NONE',  ( 16.52544592524342804, -4.483927247898539470, 33.54057627198102409 ) ) ;
#25416=CARTESIAN_POINT ( 'NONE',  ( -5.823673210054116645, -21.52544592524344225, 37.29057627198102409 ) ) ;
#25418=CARTESIAN_POINT ( 'NONE',  ( 19.03943276465977164, -0.05219959533909143690, 88.74890960531436690 ) ) ;
#25419=CARTESIAN_POINT ( 'NONE',  ( -4.379528057220328563, 16.55341960407611168, 90.20724293864770971 ) ) ;
#25420=CARTESIAN_POINT ( 'NONE',  ( 13.89961937509957401, 13.97604488694547697, 101.8760903946856331 ) ) ;
#25421=CARTESIAN_POINT ( 'NONE',  ( -15.80617190586745835, -15.72974639402198527, 56.87390960531436690 ) ) ;
#25424=CARTESIAN_POINT ( 'NONE',  ( 5.049401038298161559, -19.05341960407611168, 32.70724293864768129 ) ) ;
#25425=CARTESIAN_POINT ( 'NONE',  ( -5.153800228976328057, -19.02544592524343514, 92.29057627198099567 ) ) ;
#25426=CARTESIAN_POINT ( 'NONE',  ( 10.72451020669898902, -18.67979575497178502, 82.91557627198103830 ) ) ;
#25427=CARTESIAN_POINT ( 'NONE',  ( -4.483927247898782831, 16.52544592524335698, 107.7094237280190328 ) ) ;
#25428=CARTESIAN_POINT ( 'NONE',  ( 19.02544592524343514, -5.153800228976328945, 103.5405762719809957 ) ) ;
#25429=CARTESIAN_POINT ( 'NONE',  ( -9.474510206698720793, -16.51473224551083518, 79.58442372801899012 ) ) ;
#25430=CARTESIAN_POINT ( 'NONE',  ( 15.80617190586769283, -15.72974639402175789, 95.62609039468568994 ) ) ;
#25431=CARTESIAN_POINT ( 'NONE',  ( 15.80617190586746368, 15.72974639402197994, 74.37390960531436690 ) ) ;
#25432=CARTESIAN_POINT ( 'NONE',  ( -21.52544592524343514, 5.823673210054127303, 41.04057627198103120 ) ) ;
#25433=CARTESIAN_POINT ( 'NONE',  ( 16.51473224551069308, 9.474510206698969483, 44.16557627198103120 ) ) ;
#25434=CARTESIAN_POINT ( 'NONE',  ( 8.314922557961029526, -14.29746914071037800, 110.4177570613523756 ) ) ;
#25435=CARTESIAN_POINT ( 'NONE',  ( -5.049401038298153566, 19.05341960407611168, 70.20724293864769550 ) ) ;
#25437=CARTESIAN_POINT ( 'NONE',  ( 17.50000000000000000, 5.499999999999992895, 38.78230962303566542 ) ) ;
#25438=CARTESIAN_POINT ( 'NONE',  ( -19.03943276465977164, -0.05219959533935918106, 28.75109039468566507 ) ) ;
#25439=CARTESIAN_POINT ( 'NONE',  ( -0.05219959533910754901, -16.53943276465976808, 72.49890960531435269 ) ) ;
#25440=CARTESIAN_POINT ( 'NONE',  ( -15.80617190586768217, 15.72974639402176855, 28.12609039468568284 ) ) ;
#25443=CARTESIAN_POINT ( 'NONE',  ( -0.05219959533907301413, -21.53943276465977519, 62.49890960531436690 ) ) ;
#25444=CARTESIAN_POINT ( 'NONE',  ( -8.314922557961024197, 14.29746914071037800, 97.91775706135236135 ) ) ;
#25445=CARTESIAN_POINT ( 'NONE',  ( 9.474510206698971260, -16.51473224551069308, 22.91557627198102765 ) ) ;
#25446=CARTESIAN_POINT ( 'NONE',  ( 19.05341960407611168, 5.049401038298154454, 78.95724293864769550 ) ) ;
#25447=CARTESIAN_POINT ( 'NONE',  ( 16.46253265017160672, -9.564922557960803928, 23.33224293864769194 ) ) ;
#25448=CARTESIAN_POINT ( 'NONE',  ( -4.379528057220328563, 16.55341960407611168, 25.20724293864769550 ) ) ;
#25450=CARTESIAN_POINT ( 'NONE',  ( 0.05219959533937995610, -21.53943276465977519, 60.00109039468568284 ) ) ;
#25451=CARTESIAN_POINT ( 'NONE',  ( 16.51473224551069308, 9.474510206698969483, 114.1655762719810241 ) ) ;
#25452=CARTESIAN_POINT ( 'NONE',  ( -18.67979575497193778, 10.72451020669871902, 93.33442372801901854 ) ) ;
#25453=CARTESIAN_POINT ( 'NONE',  ( -13.97604488694527625, -13.89961937509977652, 31.87390960531435979 ) ) ;
#25454=CARTESIAN_POINT ( 'NONE',  ( 0.05219959533909260263, 19.03943276465977164, 44.99890960531435979 ) ) ;
#25456=CARTESIAN_POINT ( 'NONE',  ( -21.53943276465977519, -0.05219959533937600094, 93.75109039468567573 ) ) ;
#25457=CARTESIAN_POINT ( 'NONE',  ( -14.34966873604972548, 8.224510206698743886, 48.33442372801902565 ) ) ;
#25458=CARTESIAN_POINT ( 'NONE',  ( -18.67979575497193778, 10.72451020669871902, 83.33442372801903275 ) ) ;
#25459=CARTESIAN_POINT ( 'NONE',  ( -5.823673210054116645, -21.52544592524344225, 22.29057627198102765 ) ) ;
#25460=CARTESIAN_POINT ( 'NONE',  ( 13.97604488694548053, -13.89961937509957401, 90.62609039468567573 ) ) ;
#25461=CARTESIAN_POINT ( 'NONE',  ( -0.05219959533937732626, 21.53943276465977519, 52.50109039468567573 ) ) ;
#25462=CARTESIAN_POINT ( 'NONE',  ( -9.564922557961040184, 16.46253265017147172, 112.9177570613523329 ) ) ;
#25463=CARTESIAN_POINT ( 'NONE',  ( -19.05341960407617563, 5.049401038297882671, 88.54275706135230450 ) ) ;
#25464=CARTESIAN_POINT ( 'NONE',  ( -5.049401038298153566, 19.05341960407611168, 50.20724293864770260 ) ) ;
#25465=CARTESIAN_POINT ( 'NONE',  ( 0.05219959533936267826, -19.03943276465977164, 95.00109039468567573 ) ) ;
#25466=CARTESIAN_POINT ( 'NONE',  ( 13.97604488694548053, -13.89961937509957401, 85.62609039468568994 ) ) ;
#25467=CARTESIAN_POINT ( 'NONE',  ( -8.224510206698948167, 14.34966873604960824, 50.41557627198103120 ) ) ;
#25468=CARTESIAN_POINT ( 'NONE',  ( 13.97604488694548053, -13.89961937509957401, 75.62609039468564731 ) ) ;
#25469=CARTESIAN_POINT ( 'NONE',  ( -16.55341960407617563, 4.379528057220093196, 58.54275706135235424 ) ) ;
#25470=CARTESIAN_POINT ( 'NONE',  ( 16.46253265017146816, 9.564922557961045513, 26.66775706135234003 ) ) ;
#25471=CARTESIAN_POINT ( 'NONE',  ( 9.564922557960805705, 16.46253265017160317, 44.58224293864769550 ) ) ;
#25472=CARTESIAN_POINT ( 'NONE',  ( -19.05341960407611168, -5.049401038298163336, 41.45724293864769550 ) ) ;
#25473=CARTESIAN_POINT ( 'NONE',  ( -12.14591786802326823, 12.06949235617739902, 58.12609039468568994 ) ) ;
#25476=CARTESIAN_POINT ( 'NONE',  ( -9.564922557960796823, -16.46253265017161027, 102.0822429386477097 ) ) ;
#25479=CARTESIAN_POINT ( 'NONE',  ( -0.05219959533936034679, 19.03943276465977164, 97.50109039468567573 ) ) ;
#25480=CARTESIAN_POINT ( 'NONE',  ( -10.72451020669898014, 18.67979575497178502, 35.41557627198102409 ) ) ;
#25481=CARTESIAN_POINT ( 'NONE',  ( 5.153800228976615827, -19.02544592524334988, 30.20942372801900433 ) ) ;
#25482=CARTESIAN_POINT ( 'NONE',  ( -9.564922557961040184, 16.46253265017147172, 112.9177570613523329 ) ) ;
#25483=CARTESIAN_POINT ( 'NONE',  ( -0.05219959533909027116, -19.03943276465977164, 27.49890960531435624 ) ) ;
#25484=CARTESIAN_POINT ( 'NONE',  ( 13.89961937509977652, -13.97604488694527269, 38.12390960531436690 ) ) ;
#25485=CARTESIAN_POINT ( 'NONE',  ( 18.67979575497178502, 10.72451020669898547, 79.16557627198103830 ) ) ;
#25486=CARTESIAN_POINT ( 'NONE',  ( 5.049401038298161559, -19.05341960407611168, 37.70724293864768839 ) ) ;
#25488=CARTESIAN_POINT ( 'NONE',  ( -19.03943276465977164, -0.05219959533935918106, 83.75109039468567573 ) ) ;
#25489=CARTESIAN_POINT ( 'NONE',  ( 8.314922557960818139, 14.29746914071049879, 54.58224293864769550 ) ) ;
#25490=CARTESIAN_POINT ( 'NONE',  ( 0.05219959533907565091, 21.53943276465977519, 29.99890960531435979 ) ) ;
#25491=CARTESIAN_POINT ( 'NONE',  ( -5.823673210054431948, 21.52544592524334988, 102.7094237280190185 ) ) ;
#25492=CARTESIAN_POINT ( 'NONE',  ( 21.52544592524344225, -5.823673210054117533, 88.54057627198103830 ) ) ;
#25493=CARTESIAN_POINT ( 'NONE',  ( 0.05219959533937995610, -21.53943276465977519, 70.00109039468568994 ) ) ;
#25494=CARTESIAN_POINT ( 'NONE',  ( 15.80617190586769283, -15.72974639402175789, 60.62609039468567573 ) ) ;
#25495=CARTESIAN_POINT ( 'NONE',  ( -5.153800228976328057, -19.02544592524343514, 107.2905762719810383 ) ) ;
#25496=CARTESIAN_POINT ( 'NONE',  ( 14.29746914071037800, 8.314922557961029526, 111.6677570613523613 ) ) ;
#25497=CARTESIAN_POINT ( 'NONE',  ( -18.67979575497193778, 10.72451020669871902, 68.33442372801900433 ) ) ;
#25498=CARTESIAN_POINT ( 'NONE',  ( 5.049401038298161559, -19.05341960407611168, 57.70724293864769550 ) ) ;
#25499=CARTESIAN_POINT ( 'NONE',  ( 0.05219959533936267826, -19.03943276465977164, 35.00109039468566863 ) ) ;
#25500=CARTESIAN_POINT ( 'NONE',  ( 5.823673210054444382, -21.52544592524334988, 35.20942372801901854 ) ) ;
#25501=CARTESIAN_POINT ( 'NONE',  ( 13.89961937509977652, -13.97604488694527269, 68.12390960531436690 ) ) ;
#25502=CARTESIAN_POINT ( 'NONE',  ( 16.55341960407611168, 4.379528057220329451, 83.95724293864770971 ) ) ;
#25503=CARTESIAN_POINT ( 'NONE',  ( 4.379528057220339221, -16.55341960407611168, 47.70724293864770260 ) ) ;
#25504=CARTESIAN_POINT ( 'NONE',  ( 18.62759615963271287, -10.81492255796078972, 63.33224293864770260 ) ) ;
#25505=CARTESIAN_POINT ( 'NONE',  ( 19.03943276465977164, -0.05219959533909143690, 48.74890960531435979 ) ) ;
#25506=CARTESIAN_POINT ( 'NONE',  ( -10.81492255796078084, -18.62759615963271287, 67.08224293864770971 ) ) ;
#25507=CARTESIAN_POINT ( 'NONE',  ( -19.05341960407617563, 5.049401038297882671, 53.54275706135231871 ) ) ;
#25509=CARTESIAN_POINT ( 'NONE',  ( 16.52544592524342804, -4.483927247898539470, 63.54057627198103830 ) ) ;
#25510=CARTESIAN_POINT ( 'NONE',  ( -0.05219959533907301413, -21.53943276465977519, 42.49890960531435979 ) ) ;
#25512=CARTESIAN_POINT ( 'NONE',  ( 16.61371651742599909, 7.165104196376152146, 103.6458493000700543 ) ) ;
#25513=CARTESIAN_POINT ( 'NONE',  ( 16.52544592524335698, 4.483927247898782831, 81.45942372801900433 ) ) ;
#25515=CARTESIAN_POINT ( 'NONE',  ( -13.97604488694547697, 13.89961937509957934, 93.12609039468566152 ) ) ;
#25516=CARTESIAN_POINT ( 'NONE',  ( -14.29746914071049879, 8.314922557960819915, 50.83224293864770971 ) ) ;
#25518=CARTESIAN_POINT ( 'NONE',  ( 16.51473224551069308, 9.474510206698969483, 54.16557627198103120 ) ) ;
#25519=CARTESIAN_POINT ( 'NONE',  ( 12.06949235617757843, -12.14591786802309237, 43.12390960531435269 ) ) ;
#25520=CARTESIAN_POINT ( 'NONE',  ( -5.049401038298153566, 19.05341960407611168, 90.20724293864766707 ) ) ;
#25521=CARTESIAN_POINT ( 'NONE',  ( -5.049401038298153566, 19.05341960407611168, 50.20724293864770260 ) ) ;
#25522=CARTESIAN_POINT ( 'NONE',  ( -5.719274019375665041, -21.55341960407619695, 64.79275706135234714 ) ) ;
#25523=CARTESIAN_POINT ( 'NONE',  ( -13.89961937509977652, 13.97604488694528158, 65.62390960531436690 ) ) ;
#25524=CARTESIAN_POINT ( 'NONE',  ( 19.02544592524343514, -5.153800228976328945, 33.54057627198102409 ) ) ;
#25525=CARTESIAN_POINT ( 'NONE',  ( -13.89961937509977652, 13.97604488694528158, 75.62390960531438111 ) ) ;
#25526=EDGE_CURVE ( 'NONE', #22766, #45079, #71615, .T. ) ;
#25527=CARTESIAN_POINT ( 'NONE',  ( -10.72451020669898014, 18.67979575497178502, 50.41557627198103120 ) ) ;
#25529=CARTESIAN_POINT ( 'NONE',  ( -19.02544592524342804, 5.153800228976336051, 31.04057627198102409 ) ) ;
#25530=CARTESIAN_POINT ( 'NONE',  ( -15.80617190586745835, -15.72974639402198527, 46.87390960531435979 ) ) ;
#25531=CARTESIAN_POINT ( 'NONE',  ( 0.05219959533934541429, -16.53943276465976808, 105.0010903946856757 ) ) ;
#25532=CARTESIAN_POINT ( 'NONE',  ( -0.05219959533936034679, 19.03943276465977164, 27.50109039468566507 ) ) ;
#25533=CARTESIAN_POINT ( 'NONE',  ( -4.483927247898782831, 16.52544592524335698, 42.70942372801901854 ) ) ;
#25534=CARTESIAN_POINT ( 'NONE',  ( 4.483927247898790824, -16.52544592524335698, 85.20942372801901854 ) ) ;
#25536=CARTESIAN_POINT ( 'NONE',  ( 4.379528057220092307, 16.55341960407617563, 67.29275706135234714 ) ) ;
#25537=CARTESIAN_POINT ( 'NONE',  ( 8.224510206698742110, 14.34966873604972548, 52.08442372801901854 ) ) ;
#25538=CARTESIAN_POINT ( 'NONE',  ( 5.049401038298161559, -19.05341960407611168, 102.7072429386476955 ) ) ;
#25539=CARTESIAN_POINT ( 'NONE',  ( 13.97604488694527802, 13.89961937509977652, 34.37390960531436690 ) ) ;
#25540=CARTESIAN_POINT ( 'NONE',  ( 8.224510206698742110, 14.34966873604972548, 37.08442372801901143 ) ) ;
#25541=CARTESIAN_POINT ( 'NONE',  ( -9.564922557960796823, -16.46253265017161027, 42.08224293864769550 ) ) ;
#25542=CARTESIAN_POINT ( 'NONE',  ( 15.72974639402176855, 15.80617190586768217, 31.87609039468567929 ) ) ;
#25543=CARTESIAN_POINT ( 'NONE',  ( 12.06949235617739724, 12.14591786802326823, 31.87609039468567929 ) ) ;
#25544=CARTESIAN_POINT ( 'NONE',  ( -16.55341960407617563, 4.379528057220093196, 93.54275706135234714 ) ) ;
#25546=CARTESIAN_POINT ( 'NONE',  ( -15.72974639402176322, -15.80617190586768395, 94.37609039468568994 ) ) ;
#25547=CARTESIAN_POINT ( 'NONE',  ( -5.153800228976607833, 19.02544592524334988, 92.70942372801901854 ) ) ;
#25548=CARTESIAN_POINT ( 'NONE',  ( -13.89961937509957401, -13.97604488694547875, 54.37609039468565442 ) ) ;
#25549=CARTESIAN_POINT ( 'NONE',  ( 8.314922557960818139, 14.29746914071049879, 54.58224293864769550 ) ) ;
#25550=CARTESIAN_POINT ( 'NONE',  ( -19.03943276465977164, 0.05219959533909376836, 31.24890960531435979 ) ) ;
#25551=CARTESIAN_POINT ( 'NONE',  ( 13.89961937509957401, 13.97604488694547697, 56.87609039468564731 ) ) ;
#25553=CARTESIAN_POINT ( 'NONE',  ( -15.72974639402176322, -15.80617190586768395, 64.37609039468568994 ) ) ;
#25554=CARTESIAN_POINT ( 'NONE',  ( -16.55341960407617563, 4.379528057220093196, 33.54275706135234714 ) ) ;
#25555=CARTESIAN_POINT ( 'NONE',  ( 19.01533133064926773, -5.499999999999448441, 56.26586590595741200 ) ) ;
#25556=CARTESIAN_POINT ( 'NONE',  ( -5.823673210054116645, -21.52544592524344225, 27.29057627198103120 ) ) ;
#25557=CARTESIAN_POINT ( 'NONE',  ( 9.474510206698729675, 16.51473224551082808, 102.0844237280190043 ) ) ;
#25558=CARTESIAN_POINT ( 'NONE',  ( -5.049401038298153566, 19.05341960407611168, 110.2072429386476671 ) ) ;
#25560=CARTESIAN_POINT ( 'NONE',  ( 16.46253265017160672, -9.564922557960803928, 28.33224293864769550 ) ) ;
#25561=CARTESIAN_POINT ( 'NONE',  ( -0.05219959533937732626, 21.53943276465977519, 112.5010903946857042 ) ) ;
#25562=CARTESIAN_POINT ( 'NONE',  ( 9.474510206698971260, -16.51473224551069308, 42.91557627198103120 ) ) ;
#25563=CARTESIAN_POINT ( 'NONE',  ( -0.05219959533937732626, 21.53943276465977519, 62.50109039468568284 ) ) ;
#25564=CARTESIAN_POINT ( 'NONE',  ( 10.81492255796106328, -18.62759615963255655, 105.4177570613523613 ) ) ;
#25565=CARTESIAN_POINT ( 'NONE',  ( 12.14591786802327356, -12.06949235617739191, 105.6260903946856899 ) ) ;
#25566=CARTESIAN_POINT ( 'NONE',  ( 16.51473224551069308, 9.474510206698969483, 74.16557627198103830 ) ) ;
#25567=CARTESIAN_POINT ( 'NONE',  ( 0.05219959533937995610, -21.53943276465977519, 60.00109039468568284 ) ) ;
#25568=CARTESIAN_POINT ( 'NONE',  ( -10.81492255796105439, 18.62759615963255655, 47.91775706135234714 ) ) ;
#25569=CARTESIAN_POINT ( 'NONE',  ( -19.02544592524334988, -5.153800228976617603, 78.95942372801900433 ) ) ;
#25570=CARTESIAN_POINT ( 'NONE',  ( 9.474510206698971260, -16.51473224551069308, 107.9155762719810383 ) ) ;
#25571=CARTESIAN_POINT ( 'NONE',  ( -14.34966873604960291, -8.224510206698953496, 111.6655762719810525 ) ) ;
#25572=CARTESIAN_POINT ( 'NONE',  ( -5.823673210054116645, -21.52544592524344225, 92.29057627198103830 ) ) ;
#25573=CARTESIAN_POINT ( 'NONE',  ( -5.049401038297874678, -19.05341960407617918, 19.79275706135233293 ) ) ;
#25574=CARTESIAN_POINT ( 'NONE',  ( 0.05219959533910956823, 16.53943276465976808, 94.99890960531436690 ) ) ;
#25575=CARTESIAN_POINT ( 'NONE',  ( 13.89961937509977652, -13.97604488694527269, 53.12390960531434558 ) ) ;
#25576=CARTESIAN_POINT ( 'NONE',  ( 16.46253265017146816, 9.564922557961045513, 101.6677570613523329 ) ) ;
#25577=CARTESIAN_POINT ( 'NONE',  ( -12.14591786802309592, -12.06949235617757132, 61.87390960531436690 ) ) ;
#25578=CARTESIAN_POINT ( 'NONE',  ( -21.53943276465977519, -0.05219959533937600094, 103.7510903946857042 ) ) ;
#25579=CARTESIAN_POINT ( 'NONE',  ( -9.564922557960796823, -16.46253265017161027, 102.0822429386477097 ) ) ;
#25580=CARTESIAN_POINT ( 'NONE',  ( 9.474510206698729675, 16.51473224551082808, 72.08442372801900433 ) ) ;
#25581=CARTESIAN_POINT ( 'NONE',  ( -18.62759615963270932, 10.81492255796079327, 80.83224293864769550 ) ) ;
#25582=CARTESIAN_POINT ( 'NONE',  ( 10.72451020669871369, 18.67979575497193778, 32.08442372801901854 ) ) ;
#25583=CARTESIAN_POINT ( 'NONE',  ( 4.379528057220092307, 16.55341960407617563, 37.29275706135235424 ) ) ;
#25584=CARTESIAN_POINT ( 'NONE',  ( 8.314922557961029526, -14.29746914071037800, 90.41775706135236135 ) ) ;
#25585=CARTESIAN_POINT ( 'NONE',  ( 0.05219959533934541429, -16.53943276465976808, 45.00109039468568284 ) ) ;
#25586=CARTESIAN_POINT ( 'NONE',  ( -15.72974639402176322, -15.80617190586768395, 39.37609039468567573 ) ) ;
#25587=CARTESIAN_POINT ( 'NONE',  ( -10.72451020669898014, 18.67979575497178502, 45.41557627198103830 ) ) ;
#25588=CARTESIAN_POINT ( 'NONE',  ( -13.97604488694527625, -13.89961937509977652, 36.87390960531436690 ) ) ;
#25590=CARTESIAN_POINT ( 'NONE',  ( -16.52544592524335698, -4.483927247898792601, 58.95942372801902565 ) ) ;
#25591=CARTESIAN_POINT ( 'NONE',  ( 10.81492255796078972, 18.62759615963270932, 89.58224293864768129 ) ) ;
#25592=CARTESIAN_POINT ( 'NONE',  ( 14.29746914071049879, -8.314922557960816363, 43.33224293864769550 ) ) ;
#25593=CARTESIAN_POINT ( 'NONE',  ( -16.53943276465976808, -0.05219959533934237506, 43.75109039468568284 ) ) ;
#25594=CARTESIAN_POINT ( 'NONE',  ( -5.049401038298153566, 19.05341960407611168, 65.20724293864765286 ) ) ;
#25595=CARTESIAN_POINT ( 'NONE',  ( -14.29746914071037622, -8.314922557961029526, 89.16775706135236135 ) ) ;
#25596=CARTESIAN_POINT ( 'NONE',  ( -19.05341960407617563, 5.049401038297882671, 88.54275706135230450 ) ) ;
#25597=CARTESIAN_POINT ( 'NONE',  ( -21.55341960407610458, -5.719274019375992779, 91.45724293864769550 ) ) ;
#25598=CARTESIAN_POINT ( 'NONE',  ( 16.52544592524342804, -4.483927247898539470, 33.54057627198102409 ) ) ;
#25599=ORIENTED_EDGE ( 'NONE', *, *, #143390, .F. ) ;
#25601=CARTESIAN_POINT ( 'NONE',  ( 21.53943276465977519, -0.05219959533907433946, 63.74890960531435979 ) ) ;
#25602=CARTESIAN_POINT ( 'NONE',  ( -0.05219959533934338120, 16.53943276465976808, 107.5010903946856899 ) ) ;
#25604=CARTESIAN_POINT ( 'NONE',  ( 19.01529144963336648, 5.499999999999968914, 88.73431955728439391 ) ) ;
#25605=CARTESIAN_POINT ( 'NONE',  ( 21.55341960407610458, 5.719274019375980345, 83.95724293864770971 ) ) ;
#25606=CARTESIAN_POINT ( 'NONE',  ( -8.314922557960811034, -14.29746914071050412, 27.08224293864769550 ) ) ;
#25607=CARTESIAN_POINT ( 'NONE',  ( 16.52544592524335698, 4.483927247898782831, 41.45942372801901143 ) ) ;
#25608=CARTESIAN_POINT ( 'NONE',  ( -19.05341960407611168, -5.049401038298163336, 36.45724293864766707 ) ) ;
#25609=CARTESIAN_POINT ( 'NONE',  ( -16.51473224551069308, -9.474510206698971260, 51.66557627198102409 ) ) ;
#25611=CARTESIAN_POINT ( 'NONE',  ( -13.89961937509977652, 13.97604488694528158, 115.6239096053143669 ) ) ;
#25612=CARTESIAN_POINT ( 'NONE',  ( 0.05219959533909260263, 19.03943276465977164, 114.9989096053143669 ) ) ;
#25613=CARTESIAN_POINT ( 'NONE',  ( -14.29746914071037622, -8.314922557961029526, 109.1677570613523613 ) ) ;
#25614=CARTESIAN_POINT ( 'NONE',  ( -19.02544592524334988, -5.153800228976617603, 88.95942372801897591 ) ) ;
#25615=CARTESIAN_POINT ( 'NONE',  ( -5.049401038297874678, -19.05341960407617918, 39.79275706135232582 ) ) ;
#25616=CARTESIAN_POINT ( 'NONE',  ( 5.719274019375991003, -21.55341960407610458, 92.70724293864770971 ) ) ;
#25617=CARTESIAN_POINT ( 'NONE',  ( 8.314922557961029526, -14.29746914071037800, 110.4177570613523756 ) ) ;
#25618=CARTESIAN_POINT ( 'NONE',  ( 18.67979575497178502, 10.72451020669898547, 39.16557627198102409 ) ) ;
#25619=CARTESIAN_POINT ( 'NONE',  ( -19.05341960407617563, 5.049401038297882671, 103.5427570613523329 ) ) ;
#25620=CARTESIAN_POINT ( 'NONE',  ( -9.474510206698964154, 16.51473224551069663, 110.4155762719810383 ) ) ;
#25621=CARTESIAN_POINT ( 'NONE',  ( -21.53943276465977519, -0.05219959533937600094, 68.75109039468568994 ) ) ;
#25622=CARTESIAN_POINT ( 'NONE',  ( -5.049401038298153566, 19.05341960407611168, 65.20724293864765286 ) ) ;
#25623=CARTESIAN_POINT ( 'NONE',  ( -12.14591786802309592, -12.06949235617757132, 101.8739096053143811 ) ) ;
#25625=CARTESIAN_POINT ( 'NONE',  ( -19.05341960407611168, -5.049401038298163336, 71.45724293864766707 ) ) ;
#25626=CARTESIAN_POINT ( 'NONE',  ( -0.05219959533910754901, -16.53943276465976808, 72.49890960531435269 ) ) ;
#25628=CARTESIAN_POINT ( 'NONE',  ( 19.05341960407617918, -5.049401038297876454, 86.04275706135233293 ) ) ;
#25629=CARTESIAN_POINT ( 'NONE',  ( 19.53091890409952924, 5.499999999999984901, 92.56097431831422284 ) ) ;
#25630=CARTESIAN_POINT ( 'NONE',  ( -9.474510206698964154, 16.51473224551069663, 60.41557627198102409 ) ) ;
#25632=CARTESIAN_POINT ( 'NONE',  ( 9.474510206698971260, -16.51473224551069308, 77.91557627198103830 ) ) ;
#25633=CARTESIAN_POINT ( 'NONE',  ( 13.97604488694527802, 13.89961937509977652, 99.37390960531436690 ) ) ;
#25634=CARTESIAN_POINT ( 'NONE',  ( -12.06949235617739369, -12.14591786802326823, 59.37609039468568284 ) ) ;
#25636=CARTESIAN_POINT ( 'NONE',  ( 19.02544592524334988, 5.153800228976608722, 41.45942372801900433 ) ) ;
#25637=CARTESIAN_POINT ( 'NONE',  ( 5.823673210054444382, -21.52544592524334988, 95.20942372801903275 ) ) ;
#25639=CARTESIAN_POINT ( 'NONE',  ( 16.46253265017160672, -9.564922557960803928, 108.3322429386476955 ) ) ;
#25640=CARTESIAN_POINT ( 'NONE',  ( 12.14591786802327356, -12.06949235617739191, 100.6260903946857184 ) ) ;
#25641=CARTESIAN_POINT ( 'NONE',  ( 18.22780087662122384, -5.500000000000022204, 76.01540105326107266 ) ) ;
#25642=CARTESIAN_POINT ( 'NONE',  ( -8.224510206698735004, -14.34966873604973081, 94.58442372801901854 ) ) ;
#25643=CARTESIAN_POINT ( 'NONE',  ( -16.79531203550651242, 7.028104445595467986, 28.74755011779559055 ) ) ;
#25644=CARTESIAN_POINT ( 'NONE',  ( -16.53943276465976808, -0.05219959533934237506, 63.75109039468568284 ) ) ;
#25645=ORIENTED_EDGE ( 'NONE', *, *, #191495, .T. ) ;
#25646=CARTESIAN_POINT ( 'NONE',  ( 0.05219959533937995610, -21.53943276465977519, 85.00109039468568994 ) ) ;
#25647=CARTESIAN_POINT ( 'NONE',  ( -19.02544592524334988, -5.153800228976617603, 83.95942372801901854 ) ) ;
#25648=CARTESIAN_POINT ( 'NONE',  ( 5.153800228976615827, -19.02544592524334988, 25.20942372801900433 ) ) ;
#25649=CARTESIAN_POINT ( 'NONE',  ( -5.153800228976328057, -19.02544592524343514, 62.29057627198100988 ) ) ;
#25650=CARTESIAN_POINT ( 'NONE',  ( 13.97604488694527802, 13.89961937509977652, 44.37390960531435269 ) ) ;
#25652=CARTESIAN_POINT ( 'NONE',  ( 5.823673210054125526, 21.52544592524343514, 79.79057627198102409 ) ) ;
#25654=CARTESIAN_POINT ( 'NONE',  ( 21.52544592524344225, -5.823673210054117533, 38.54057627198103120 ) ) ;
#25655=CARTESIAN_POINT ( 'NONE',  ( -19.05341960407611168, -5.049401038298163336, 36.45724293864766707 ) ) ;
#25656=CARTESIAN_POINT ( 'NONE',  ( 14.29746914071037800, 8.314922557961029526, 56.66775706135235424 ) ) ;
#25658=CARTESIAN_POINT ( 'NONE',  ( 10.72451020669871369, 18.67979575497193778, 37.08442372801901143 ) ) ;
#25659=CARTESIAN_POINT ( 'NONE',  ( -16.55341960407611168, -4.379528057220339221, 71.45724293864769550 ) ) ;
#25661=CARTESIAN_POINT ( 'NONE',  ( -8.224510206698735004, -14.34966873604973081, 19.58442372801901143 ) ) ;
#25662=CARTESIAN_POINT ( 'NONE',  ( 9.474510206698729675, 16.51473224551082808, 37.08442372801899722 ) ) ;
#25663=CARTESIAN_POINT ( 'NONE',  ( 4.483927247898545687, 16.52544592524342804, 59.79057627198103120 ) ) ;
#25664=CARTESIAN_POINT ( 'NONE',  ( 21.53943276465977519, 0.05219959533937863772, 21.25109039468567218 ) ) ;
#25666=CARTESIAN_POINT ( 'NONE',  ( 21.53943276465977519, -0.05219959533907433946, 83.74890960531435269 ) ) ;
#25667=CARTESIAN_POINT ( 'NONE',  ( 19.03943276465977164, -0.05219959533909143690, 93.74890960531435269 ) ) ;
#25668=CARTESIAN_POINT ( 'NONE',  ( -0.05219959533910754901, -16.53943276465976808, 57.49890960531435979 ) ) ;
#25670=CARTESIAN_POINT ( 'NONE',  ( 18.22780087662121673, 5.500000000000056843, 43.98459894673892734 ) ) ;
#25671=CARTESIAN_POINT ( 'NONE',  ( -9.474510206698720793, -16.51473224551083518, 69.58442372801901854 ) ) ;
#25672=CARTESIAN_POINT ( 'NONE',  ( 15.72974639402199770, -15.80617190586745480, 113.1239096053143953 ) ) ;
#25673=CARTESIAN_POINT ( 'NONE',  ( -9.474510206698964154, 16.51473224551069663, 50.41557627198102409 ) ) ;
#25674=CARTESIAN_POINT ( 'NONE',  ( 16.46253265017146816, 9.564922557961045513, 46.66775706135233293 ) ) ;
#25675=CARTESIAN_POINT ( 'NONE',  ( -9.474510206698964154, 16.51473224551069663, 25.41557627198103120 ) ) ;
#25676=CARTESIAN_POINT ( 'NONE',  ( 21.53943276465977519, 0.05219959533937863772, 66.25109039468567573 ) ) ;
#25677=CARTESIAN_POINT ( 'NONE',  ( -17.48847506799969054, -5.747544572773760407, 69.17302562156721990 ) ) ;
#25678=CARTESIAN_POINT ( 'NONE',  ( -16.53943276465976808, 0.05219959533911058130, 46.24890960531435979 ) ) ;
#25679=CARTESIAN_POINT ( 'NONE',  ( 0.05219959533909260263, 19.03943276465977164, 64.99890960531436690 ) ) ;
#25680=CARTESIAN_POINT ( 'NONE',  ( 18.67979575497178502, 10.72451020669898547, 69.16557627198102409 ) ) ;
#25681=CARTESIAN_POINT ( 'NONE',  ( 19.03943276465977164, -0.05219959533909143690, 53.74890960531436690 ) ) ;
#25682=CARTESIAN_POINT ( 'NONE',  ( 10.81492255796078972, 18.62759615963270932, 64.58224293864769550 ) ) ;
#25684=CARTESIAN_POINT ( 'NONE',  ( -10.72451020669870658, -18.67979575497194134, 94.58442372801901854 ) ) ;
#25686=CARTESIAN_POINT ( 'NONE',  ( -12.14591786802326823, 12.06949235617739902, 98.12609039468570415 ) ) ;
#25687=CARTESIAN_POINT ( 'NONE',  ( 14.34966873604960469, 8.224510206698951720, 89.16557627198102409 ) ) ;
#25688=CARTESIAN_POINT ( 'NONE',  ( 13.89961937509957401, 13.97604488694547697, 86.87609039468567573 ) ) ;
#25689=ORIENTED_EDGE ( 'NONE', *, *, #120968, .F. ) ;
#25690=CARTESIAN_POINT ( 'NONE',  ( -5.153800228976607833, 19.02544592524334988, 42.70942372801901143 ) ) ;
#25691=CARTESIAN_POINT ( 'NONE',  ( -16.53943276465976808, -0.05219959533934237506, 83.75109039468568994 ) ) ;
#25692=CARTESIAN_POINT ( 'NONE',  ( 9.474510206698729675, 16.51473224551082808, 32.08442372801900433 ) ) ;
#25693=CARTESIAN_POINT ( 'NONE',  ( -19.02544592524342804, 5.153800228976336051, 86.04057627198103830 ) ) ;
#25694=CARTESIAN_POINT ( 'NONE',  ( -10.72451020669898014, 18.67979575497178502, 55.41557627198102409 ) ) ;
#25696=CARTESIAN_POINT ( 'NONE',  ( -5.049401038298153566, 19.05341960407611168, 25.20724293864768484 ) ) ;
#25697=CARTESIAN_POINT ( 'NONE',  ( -21.53943276465977519, -0.05219959533937600094, 98.75109039468568994 ) ) ;
#25698=CARTESIAN_POINT ( 'NONE',  ( 4.483927247898790824, -16.52544592524335698, 75.20942372801901854 ) ) ;
#25699=CARTESIAN_POINT ( 'NONE',  ( -5.719274019375665041, -21.55341960407619695, 24.79275706135235779 ) ) ;
#25700=CARTESIAN_POINT ( 'NONE',  ( 8.314922557961029526, -14.29746914071037800, 30.41775706135234358 ) ) ;
#25701=CARTESIAN_POINT ( 'NONE',  ( -19.05341960407611168, -5.049401038298163336, 91.45724293864766707 ) ) ;
#25702=CARTESIAN_POINT ( 'NONE',  ( 16.51473224551069308, 9.474510206698969483, 39.16557627198103120 ) ) ;
#25703=CARTESIAN_POINT ( 'NONE',  ( -19.03943276465977164, 0.05219959533909376836, 46.24890960531435979 ) ) ;
#25704=CARTESIAN_POINT ( 'NONE',  ( 4.483927247898790824, -16.52544592524335698, 40.20942372801901854 ) ) ;
#25705=CARTESIAN_POINT ( 'NONE',  ( -4.379528057220328563, 16.55341960407611168, 90.20724293864770971 ) ) ;
#25706=CARTESIAN_POINT ( 'NONE',  ( -14.34966873604972548, 8.224510206698743886, 98.33442372801901854 ) ) ;
#25707=CARTESIAN_POINT ( 'NONE',  ( 15.72974639402176855, 15.80617190586768217, 36.87609039468568994 ) ) ;
#25708=CARTESIAN_POINT ( 'NONE',  ( -19.02544592524342804, 5.153800228976336051, 81.04057627198103830 ) ) ;
#25709=CARTESIAN_POINT ( 'NONE',  ( 5.153800228976335163, 19.02544592524342804, 59.79057627198100988 ) ) ;
#25710=CARTESIAN_POINT ( 'NONE',  ( -13.89961937509977652, 13.97604488694528158, 80.62390960531436690 ) ) ;
#25711=CARTESIAN_POINT ( 'NONE',  ( 8.224510206698953496, -14.34966873604960469, 37.91557627198102409 ) ) ;
#25712=CARTESIAN_POINT ( 'NONE',  ( 0.05219959533934541429, -16.53943276465976808, 100.0010903946857042 ) ) ;
#25714=CARTESIAN_POINT ( 'NONE',  ( -19.05341960407617563, 5.049401038297882671, 48.54275706135233293 ) ) ;
#25716=CARTESIAN_POINT ( 'NONE',  ( 0.05219959533909260263, 19.03943276465977164, 49.99890960531435979 ) ) ;
#25717=CARTESIAN_POINT ( 'NONE',  ( 13.97604488694548053, -13.89961937509957401, 45.62609039468566863 ) ) ;
#25719=CARTESIAN_POINT ( 'NONE',  ( -14.34966873604972548, 8.224510206698743886, 38.33442372801900433 ) ) ;
#25720=CARTESIAN_POINT ( 'NONE',  ( 16.51473224551083163, -9.474510206698727899, 75.83442372801900433 ) ) ;
#25721=CARTESIAN_POINT ( 'NONE',  ( 4.379528057220092307, 16.55341960407617563, 57.29275706135234714 ) ) ;
#25722=DIRECTION ( 'NONE',  ( -0.000000000000000000, 1.000000000000000000, 0.000000000000000000 ) ) ;
#25723=CARTESIAN_POINT ( 'NONE',  ( -19.05341960407611168, -5.049401038298163336, 81.45724293864769550 ) ) ;
#25724=CARTESIAN_POINT ( 'NONE',  ( 21.52544592524344225, -5.823673210054117533, 113.5405762719810383 ) ) ;
#25725=CARTESIAN_POINT ( 'NONE',  ( -16.51473224551082808, 9.474510206698731452, 73.33442372801900433 ) ) ;
#25726=CARTESIAN_POINT ( 'NONE',  ( -16.46253265017160317, 9.564922557960807481, 105.8322429386476955 ) ) ;
#25727=CARTESIAN_POINT ( 'NONE',  ( -13.89961937509977652, 13.97604488694528158, 30.62390960531435269 ) ) ;
#25728=CARTESIAN_POINT ( 'NONE',  ( -13.97604488694527625, -13.89961937509977652, 76.87390960531433848 ) ) ;
#25729=CARTESIAN_POINT ( 'NONE',  ( 0.05219959533910956823, 16.53943276465976808, 39.99890960531436690 ) ) ;
#25730=CARTESIAN_POINT ( 'NONE',  ( -16.46253265017160317, 9.564922557960807481, 30.83224293864769550 ) ) ;
#25731=CARTESIAN_POINT ( 'NONE',  ( 5.153800228976615827, -19.02544592524334988, 55.20942372801899722 ) ) ;
#25732=CARTESIAN_POINT ( 'NONE',  ( 8.224510206698953496, -14.34966873604960469, 67.91557627198102409 ) ) ;
#25733=CARTESIAN_POINT ( 'NONE',  ( 19.02544592524334988, 5.153800228976608722, 21.45942372801899012 ) ) ;
#25734=CARTESIAN_POINT ( 'NONE',  ( 16.46253265017160672, -9.564922557960803928, 48.33224293864769550 ) ) ;
#25735=CARTESIAN_POINT ( 'NONE',  ( -18.62759615963270932, 10.81492255796079327, 50.83224293864770971 ) ) ;
#25736=CARTESIAN_POINT ( 'NONE',  ( 4.379528057220339221, -16.55341960407611168, 57.70724293864770260 ) ) ;
#25737=CARTESIAN_POINT ( 'NONE',  ( 10.72451020669871369, 18.67979575497193778, 102.0844237280190185 ) ) ;
#25738=CARTESIAN_POINT ( 'NONE',  ( -13.97604488694527625, -13.89961937509977652, 96.87390960531433848 ) ) ;
#25739=CARTESIAN_POINT ( 'NONE',  ( -19.02544592524342804, 5.153800228976336051, 106.0405762719810241 ) ) ;
#25740=CARTESIAN_POINT ( 'NONE',  ( 19.03943276465977164, -0.05219959533909143690, 38.74890960531436690 ) ) ;
#25741=CARTESIAN_POINT ( 'NONE',  ( -5.153800228976328057, -19.02544592524343514, 32.29057627198102409 ) ) ;
#25742=CARTESIAN_POINT ( 'NONE',  ( -4.483927247898539470, -16.52544592524342804, 92.29057627198103830 ) ) ;
#25743=CARTESIAN_POINT ( 'NONE',  ( 10.72451020669898902, -18.67979575497178502, 97.91557627198103830 ) ) ;
#25744=CARTESIAN_POINT ( 'NONE',  ( -19.03943276465977164, 0.05219959533909376836, 101.2489096053143669 ) ) ;
#25745=CARTESIAN_POINT ( 'NONE',  ( -21.52544592524343514, 5.823673210054127303, 116.0405762719810383 ) ) ;
#25746=CARTESIAN_POINT ( 'NONE',  ( -5.153800228976328057, -19.02544592524343514, 87.29057627198103830 ) ) ;
#25748=CARTESIAN_POINT ( 'NONE',  ( -12.06949235617756955, 12.14591786802309770, 100.6239096053143811 ) ) ;
#25749=CARTESIAN_POINT ( 'NONE',  ( -13.97604488694527625, -13.89961937509977652, 71.87390960531433848 ) ) ;
#25750=CARTESIAN_POINT ( 'NONE',  ( -15.80617190586745835, -15.72974639402198527, 81.87390960531435269 ) ) ;
#25753=CARTESIAN_POINT ( 'NONE',  ( -10.72451020669898014, 18.67979575497178502, 25.41557627198103120 ) ) ;
#25755=CARTESIAN_POINT ( 'NONE',  ( 14.34966873604972726, -8.224510206698740333, 35.83442372801901143 ) ) ;
#25756=CARTESIAN_POINT ( 'NONE',  ( 16.52544592524342804, -4.483927247898539470, 88.54057627198103830 ) ) ;
#25757=CARTESIAN_POINT ( 'NONE',  ( -17.50000000000014211, -3.417042746626972605, 109.8261960376752597 ) ) ;
#25758=CARTESIAN_POINT ( 'NONE',  ( 9.564922557960805705, 16.46253265017160317, 84.58224293864769550 ) ) ;
#25759=CARTESIAN_POINT ( 'NONE',  ( 13.89961937509977652, -13.97604488694527269, 43.12390960531434558 ) ) ;
#25760=CARTESIAN_POINT ( 'NONE',  ( -8.224510206698948167, 14.34966873604960824, 80.41557627198103830 ) ) ;
#25761=CARTESIAN_POINT ( 'NONE',  ( -10.81492255796078084, -18.62759615963271287, 27.08224293864769550 ) ) ;
#25762=CARTESIAN_POINT ( 'NONE',  ( 16.53943276465976808, -0.05219959533910856209, 48.74890960531435979 ) ) ;
#25763=CARTESIAN_POINT ( 'NONE',  ( 16.46253265017146816, 9.564922557961045513, 101.6677570613523329 ) ) ;
#25764=CARTESIAN_POINT ( 'NONE',  ( 18.62759615963255655, 10.81492255796105972, 76.66775706135234714 ) ) ;
#25766=CARTESIAN_POINT ( 'NONE',  ( -5.049401038298153566, 19.05341960407611168, 110.2072429386476671 ) ) ;
#25767=CARTESIAN_POINT ( 'NONE',  ( 16.52544592524335698, 4.483927247898782831, 86.45942372801901854 ) ) ;
#25768=CARTESIAN_POINT ( 'NONE',  ( -5.153800228976328057, -19.02544592524343514, 27.29057627198103120 ) ) ;
#25769=CARTESIAN_POINT ( 'NONE',  ( 19.03943276465977164, -0.05219959533909143690, 78.74890960531436690 ) ) ;
#25770=CARTESIAN_POINT ( 'NONE',  ( -5.719274019375978568, 21.55341960407610458, 85.20724293864770971 ) ) ;
#25771=CARTESIAN_POINT ( 'NONE',  ( -12.06949235617739369, -12.14591786802326823, 24.37609039468567573 ) ) ;
#25772=CARTESIAN_POINT ( 'NONE',  ( -4.483927247898539470, -16.52544592524342804, 57.29057627198103120 ) ) ;
#25773=CARTESIAN_POINT ( 'NONE',  ( -21.53943276465977519, -0.05219959533937600094, 73.75109039468567573 ) ) ;
#25774=CARTESIAN_POINT ( 'NONE',  ( 16.55341960407618274, -4.379528057220086978, 91.04275706135236135 ) ) ;
#25775=CARTESIAN_POINT ( 'NONE',  ( -10.72451020669898014, 18.67979575497178502, 25.41557627198103120 ) ) ;
#25776=CARTESIAN_POINT ( 'NONE',  ( 5.153800228976335163, 19.02544592524342804, 109.7905762719810241 ) ) ;
#25778=CARTESIAN_POINT ( 'NONE',  ( -16.53943276465976808, 0.05219959533911058130, 21.24890960531436690 ) ) ;
#25779=CARTESIAN_POINT ( 'NONE',  ( -8.314922557961024197, 14.29746914071037800, 57.91775706135234714 ) ) ;
#25780=CARTESIAN_POINT ( 'NONE',  ( 13.89961937509977652, -13.97604488694527269, 68.12390960531436690 ) ) ;
#25781=CARTESIAN_POINT ( 'NONE',  ( -5.153800228976328057, -19.02544592524343514, 87.29057627198103830 ) ) ;
#25782=CARTESIAN_POINT ( 'NONE',  ( 21.52544592524334988, 5.823673210054432836, 76.45942372801901854 ) ) ;
#25783=CARTESIAN_POINT ( 'NONE',  ( 8.224510206698742110, 14.34966873604972548, 72.08442372801899012 ) ) ;
#25784=CARTESIAN_POINT ( 'NONE',  ( -12.06949235617756955, 12.14591786802309770, 40.62390960531435269 ) ) ;
#25785=CARTESIAN_POINT ( 'NONE',  ( -9.564922557960796823, -16.46253265017161027, 57.08224293864769550 ) ) ;
#25786=CARTESIAN_POINT ( 'NONE',  ( -19.05341960407611168, -5.049401038298163336, 46.45724293864768129 ) ) ;
#25788=CARTESIAN_POINT ( 'NONE',  ( -19.05341960407617563, 5.049401038297882671, 93.54275706135234714 ) ) ;
#25789=CARTESIAN_POINT ( 'NONE',  ( 12.06949235617757843, -12.14591786802309237, 93.12390960531436690 ) ) ;
#25790=CARTESIAN_POINT ( 'NONE',  ( -19.05341960407611168, -5.049401038298163336, 61.45724293864769550 ) ) ;
#25791=CARTESIAN_POINT ( 'NONE',  ( -19.05341960407617563, 5.049401038297882671, 103.5427570613523329 ) ) ;
#25793=CARTESIAN_POINT ( 'NONE',  ( 18.67979575497194134, -10.72451020669871369, 100.8344237280190185 ) ) ;
#25794=CARTESIAN_POINT ( 'NONE',  ( -4.483927247898782831, 16.52544592524335698, 67.70942372801901854 ) ) ;
#25795=CARTESIAN_POINT ( 'NONE',  ( -16.51473224551082808, 9.474510206698731452, 88.33442372801900433 ) ) ;
#25796=CARTESIAN_POINT ( 'NONE',  ( -5.823673210054116645, -21.52544592524344225, 67.29057627198103830 ) ) ;
#25797=CARTESIAN_POINT ( 'NONE',  ( 14.29746914071037800, 8.314922557961029526, 46.66775706135234714 ) ) ;
#25799=CARTESIAN_POINT ( 'NONE',  ( -13.89961937509957401, -13.97604488694547875, 54.37609039468565442 ) ) ;
#25800=CARTESIAN_POINT ( 'NONE',  ( -15.72974639402176322, -15.80617190586768395, 94.37609039468568994 ) ) ;
#25801=CARTESIAN_POINT ( 'NONE',  ( 9.474510206698971260, -16.51473224551069308, 27.91557627198103120 ) ) ;
#25802=CARTESIAN_POINT ( 'NONE',  ( -13.97604488694527625, -13.89961937509977652, 61.87390960531435979 ) ) ;
#25803=CARTESIAN_POINT ( 'NONE',  ( 12.14591786802309770, 12.06949235617756955, 54.37390960531435979 ) ) ;
#25804=CARTESIAN_POINT ( 'NONE',  ( 21.53943276465977519, 0.05219959533937863772, 91.25109039468568994 ) ) ;
#25805=CARTESIAN_POINT ( 'NONE',  ( 5.049401038297881783, 19.05341960407617563, 42.29275706135234003 ) ) ;
#25806=CARTESIAN_POINT ( 'NONE',  ( 5.153800228976615827, -19.02544592524334988, 25.20942372801900433 ) ) ;
#25807=CARTESIAN_POINT ( 'NONE',  ( 5.049401038298161559, -19.05341960407611168, 112.7072429386476813 ) ) ;
#25808=CARTESIAN_POINT ( 'NONE',  ( 5.719274019375673035, 21.55341960407619339, 92.29275706135236135 ) ) ;
#25809=CARTESIAN_POINT ( 'NONE',  ( -16.51473224551069308, -9.474510206698971260, 71.66557627198102409 ) ) ;
#25810=CARTESIAN_POINT ( 'NONE',  ( -10.81492255796105439, 18.62759615963255655, 87.91775706135234714 ) ) ;
#25811=CARTESIAN_POINT ( 'NONE',  ( 15.72974639402199770, -15.80617190586745480, 48.12390960531436690 ) ) ;
#25812=CARTESIAN_POINT ( 'NONE',  ( -0.05219959533909027116, -19.03943276465977164, 82.49890960531436690 ) ) ;
#25813=CARTESIAN_POINT ( 'NONE',  ( 5.049401038297881783, 19.05341960407617563, 67.29275706135234714 ) ) ;
#25814=CARTESIAN_POINT ( 'NONE',  ( -9.564922557960796823, -16.46253265017161027, 47.08224293864769550 ) ) ;
#25815=CARTESIAN_POINT ( 'NONE',  ( 9.474510206698971260, -16.51473224551069308, 92.91557627198103830 ) ) ;
#25816=CARTESIAN_POINT ( 'NONE',  ( 5.153800228976615827, -19.02544592524334988, 85.20942372801900433 ) ) ;
#25817=CARTESIAN_POINT ( 'NONE',  ( 4.483927247898790824, -16.52544592524335698, 45.20942372801901854 ) ) ;
#25818=CARTESIAN_POINT ( 'NONE',  ( -8.314922557960811034, -14.29746914071050412, 107.0822429386476955 ) ) ;
#25819=CARTESIAN_POINT ( 'NONE',  ( -16.51473224551069308, -9.474510206698971260, 76.66557627198103830 ) ) ;
#25820=CARTESIAN_POINT ( 'NONE',  ( 10.72451020669898902, -18.67979575497178502, 47.91557627198102409 ) ) ;
#25822=CARTESIAN_POINT ( 'NONE',  ( -4.379528057220086978, -16.55341960407618274, 19.79275706135235069 ) ) ;
#25823=CARTESIAN_POINT ( 'NONE',  ( 10.81492255796106328, -18.62759615963255655, 25.41775706135235779 ) ) ;
#25824=CARTESIAN_POINT ( 'NONE',  ( -15.72974639402176322, -15.80617190586768395, 89.37609039468568994 ) ) ;
#25825=CARTESIAN_POINT ( 'NONE',  ( -16.55341960407617563, 4.379528057220093196, 78.54275706135236135 ) ) ;
#25826=CARTESIAN_POINT ( 'NONE',  ( 19.05341960407611168, 5.049401038298154454, 78.95724293864769550 ) ) ;
#25827=CARTESIAN_POINT ( 'NONE',  ( 16.53943276465976808, 0.05219959533934440121, 106.2510903946856757 ) ) ;
#25828=CARTESIAN_POINT ( 'NONE',  ( -9.564922557961040184, 16.46253265017147172, 57.91775706135233293 ) ) ;
#25830=CARTESIAN_POINT ( 'NONE',  ( -10.81492255796105439, 18.62759615963255655, 27.91775706135234358 ) ) ;
#25831=CARTESIAN_POINT ( 'NONE',  ( -8.314922557960811034, -14.29746914071050412, 77.08224293864769550 ) ) ;
#25832=CARTESIAN_POINT ( 'NONE',  ( -13.97604488694527625, -13.89961937509977652, 101.8739096053143811 ) ) ;
#25833=CARTESIAN_POINT ( 'NONE',  ( -14.34966873604972548, 8.224510206698743886, 88.33442372801901854 ) ) ;
#25834=CARTESIAN_POINT ( 'NONE',  ( 0.05219959533937995610, -21.53943276465977519, 70.00109039468568994 ) ) ;
#25835=CARTESIAN_POINT ( 'NONE',  ( 4.379528057220092307, 16.55341960407617563, 32.29275706135235424 ) ) ;
#25836=CARTESIAN_POINT ( 'NONE',  ( 10.72451020669871369, 18.67979575497193778, 32.08442372801901854 ) ) ;
#25837=CARTESIAN_POINT ( 'NONE',  ( 0.05219959533910956823, 16.53943276465976808, 64.99890960531435269 ) ) ;
#25838=ORIENTED_EDGE ( 'NONE', *, *, #63994, .T. ) ;
#25839=CARTESIAN_POINT ( 'NONE',  ( -0.05219959533907301413, -21.53943276465977519, 97.49890960531436690 ) ) ;
#25840=CARTESIAN_POINT ( 'NONE',  ( 8.224510206698953496, -14.34966873604960469, 57.91557627198103120 ) ) ;
#25841=ORIENTED_EDGE ( 'NONE', *, *, #52789, .T. ) ;
#25842=CARTESIAN_POINT ( 'NONE',  ( -19.05341960407611168, -5.049401038298163336, 31.45724293864769550 ) ) ;
#25843=CARTESIAN_POINT ( 'NONE',  ( -10.81492255796078084, -18.62759615963271287, 27.08224293864769550 ) ) ;
#25844=CARTESIAN_POINT ( 'NONE',  ( -21.53943276465977519, -0.05219959533937600094, 53.75109039468568994 ) ) ;
#25845=CARTESIAN_POINT ( 'NONE',  ( 14.29746914071049879, -8.314922557960816363, 58.33224293864768839 ) ) ;
#25847=CARTESIAN_POINT ( 'NONE',  ( -18.67979575497178146, -10.72451020669898902, 61.66557627198103120 ) ) ;
#25848=CARTESIAN_POINT ( 'NONE',  ( 16.46253265017160672, -9.564922557960803928, 68.33224293864770971 ) ) ;
#25849=CARTESIAN_POINT ( 'NONE',  ( 9.564922557960805705, 16.46253265017160317, 29.58224293864769550 ) ) ;
#25850=CARTESIAN_POINT ( 'NONE',  ( -16.51473224551082808, 9.474510206698731452, 78.33442372801900433 ) ) ;
#25851=CARTESIAN_POINT ( 'NONE',  ( 18.62759615963271287, -10.81492255796078972, 63.33224293864770260 ) ) ;
#25852=CARTESIAN_POINT ( 'NONE',  ( -19.02544592524342804, 5.153800228976336051, 41.04057627198103120 ) ) ;
#25853=CARTESIAN_POINT ( 'NONE',  ( -9.564922557960796823, -16.46253265017161027, 77.08224293864769550 ) ) ;
#25854=CARTESIAN_POINT ( 'NONE',  ( -0.05219959533934338120, 16.53943276465976808, 52.50109039468567573 ) ) ;
#25855=CARTESIAN_POINT ( 'NONE',  ( 21.55341960407619695, -5.719274019375665929, 26.04275706135235779 ) ) ;
#25856=CARTESIAN_POINT ( 'NONE',  ( 5.823673210054444382, -21.52544592524334988, 65.20942372801901854 ) ) ;
#25857=CARTESIAN_POINT ( 'NONE',  ( -16.51473224551069308, -9.474510206698971260, 101.6655762719810241 ) ) ;
#25858=CARTESIAN_POINT ( 'NONE',  ( 15.80617190586746368, 15.72974639402197994, 89.37390960531435269 ) ) ;
#25859=CARTESIAN_POINT ( 'NONE',  ( 10.72451020669898902, -18.67979575497178502, 102.9155762719810383 ) ) ;
#25860=CARTESIAN_POINT ( 'NONE',  ( 16.52544592524335698, 4.483927247898782831, 51.45942372801901854 ) ) ;
#25861=CARTESIAN_POINT ( 'NONE',  ( -0.05219959533907301413, -21.53943276465977519, 52.49890960531435979 ) ) ;
#25862=CARTESIAN_POINT ( 'NONE',  ( 21.52544592524334988, 5.823673210054432836, 101.4594237280190185 ) ) ;
#25863=CARTESIAN_POINT ( 'NONE',  ( -13.89961937509977652, 13.97604488694528158, 50.62390960531435979 ) ) ;
#25864=CARTESIAN_POINT ( 'NONE',  ( -16.46253265017160317, 9.564922557960807481, 115.8322429386477097 ) ) ;
#25865=CARTESIAN_POINT ( 'NONE',  ( -13.89961937509977652, 13.97604488694528158, 80.62390960531436690 ) ) ;
#25866=EDGE_CURVE ( 'NONE', #192458, #121091, #57793, .T. ) ;
#25867=CARTESIAN_POINT ( 'NONE',  ( 16.36317988757097908, -7.306389748694713582, 86.59789608363178104 ) ) ;
#25868=CARTESIAN_POINT ( 'NONE',  ( -19.05341960407617563, 5.049401038297882671, 73.54275706135233293 ) ) ;
#25869=CARTESIAN_POINT ( 'NONE',  ( 21.52544592524344225, -5.823673210054117533, 43.54057627198103830 ) ) ;
#25870=CARTESIAN_POINT ( 'NONE',  ( 16.53943276465976808, 0.05219959533934440121, 111.2510903946856899 ) ) ;
#25871=CARTESIAN_POINT ( 'NONE',  ( -19.03943276465977164, -0.05219959533935918106, 88.75109039468567573 ) ) ;
#25872=CARTESIAN_POINT ( 'NONE',  ( -16.19135201231370047, 7.376712067591781441, 59.81319145947970384 ) ) ;
#25873=CARTESIAN_POINT ( 'NONE',  ( 16.51473224551083163, -9.474510206698727899, 20.83442372801899722 ) ) ;
#25874=CARTESIAN_POINT ( 'NONE',  ( -9.564922557961040184, 16.46253265017147172, 87.91775706135233293 ) ) ;
#25875=CARTESIAN_POINT ( 'NONE',  ( -16.51473224551082808, 9.474510206698731452, 38.33442372801899722 ) ) ;
#25877=CARTESIAN_POINT ( 'NONE',  ( -9.564922557960796823, -16.46253265017161027, 52.08224293864768839 ) ) ;
#25878=CARTESIAN_POINT ( 'NONE',  ( -16.53943276465976808, 0.05219959533911058130, 46.24890960531435979 ) ) ;
#25879=CARTESIAN_POINT ( 'NONE',  ( -9.564922557960796823, -16.46253265017161027, 37.08224293864768839 ) ) ;
#25880=CARTESIAN_POINT ( 'NONE',  ( -8.224510206698948167, 14.34966873604960824, 40.41557627198103120 ) ) ;
#25882=CARTESIAN_POINT ( 'NONE',  ( -4.483927247898782831, 16.52544592524335698, 107.7094237280190328 ) ) ;
#25883=CARTESIAN_POINT ( 'NONE',  ( -16.51473224551069308, -9.474510206698971260, 51.66557627198102409 ) ) ;
#25884=CARTESIAN_POINT ( 'NONE',  ( 19.02544592524334988, 5.153800228976608722, 21.45942372801899012 ) ) ;
#25885=CARTESIAN_POINT ( 'NONE',  ( 0.05219959533934541429, -16.53943276465976808, 35.00109039468568284 ) ) ;
#25886=CARTESIAN_POINT ( 'NONE',  ( -0.05219959533907301413, -21.53943276465977519, 42.49890960531435979 ) ) ;
#25887=CARTESIAN_POINT ( 'NONE',  ( -18.67979575497193778, 10.72451020669871902, 88.33442372801901854 ) ) ;
#25889=CARTESIAN_POINT ( 'NONE',  ( -5.153800228976328057, -19.02544592524343514, 102.2905762719810383 ) ) ;
#25890=CARTESIAN_POINT ( 'NONE',  ( 9.474510206698971260, -16.51473224551069308, 92.91557627198103830 ) ) ;
#25892=CARTESIAN_POINT ( 'NONE',  ( -10.72451020669870658, -18.67979575497194134, 19.58442372801901143 ) ) ;
#25893=CARTESIAN_POINT ( 'NONE',  ( 12.14591786802309770, 12.06949235617756955, 74.37390960531436690 ) ) ;
#25894=CARTESIAN_POINT ( 'NONE',  ( -15.72974639402197994, 15.80617190586746368, 80.62390960531438111 ) ) ;
#25895=CARTESIAN_POINT ( 'NONE',  ( 16.51473224551069308, 9.474510206698969483, 74.16557627198103830 ) ) ;
#25896=CARTESIAN_POINT ( 'NONE',  ( 13.97604488694527802, 13.89961937509977652, 74.37390960531436690 ) ) ;
#25897=CARTESIAN_POINT ( 'NONE',  ( 21.53943276465977519, -0.05219959533907433946, 108.7489096053143669 ) ) ;
#25898=ORIENTED_EDGE ( 'NONE', *, *, #118723, .F. ) ;
#25899=CARTESIAN_POINT ( 'NONE',  ( 16.46253265017160672, -9.564922557960803928, 63.33224293864769550 ) ) ;
#25900=CARTESIAN_POINT ( 'NONE',  ( -8.314922557960811034, -14.29746914071050412, 107.0822429386476955 ) ) ;
#25902=CARTESIAN_POINT ( 'NONE',  ( -9.474510206698964154, 16.51473224551069663, 60.41557627198102409 ) ) ;
#25903=CARTESIAN_POINT ( 'NONE',  ( 9.474510206698729675, 16.51473224551082808, 87.08442372801900433 ) ) ;
#25904=CARTESIAN_POINT ( 'NONE',  ( -0.05219959533910754901, -16.53943276465976808, 102.4989096053143811 ) ) ;
#25905=CARTESIAN_POINT ( 'NONE',  ( 0.05219959533937995610, -21.53943276465977519, 65.00109039468568994 ) ) ;
#25906=CARTESIAN_POINT ( 'NONE',  ( 9.474510206698971260, -16.51473224551069308, 42.91557627198103120 ) ) ;
#25907=CARTESIAN_POINT ( 'NONE',  ( -0.05219959533907301413, -21.53943276465977519, 112.4989096053143669 ) ) ;
#25908=B_SPLINE_CURVE_WITH_KNOTS ( 'NONE', 3,
 ( #475, #46002, #17656, #77328, #107657, #138996, #79316, #62149, #123813, #185511, #108661, #37790, #52946, #191468, #143964, #98444, #51958, #163141, #7439, #146972 ),
 .UNSPECIFIED., .F., .F.,
 ( 4, 2, 2, 2, 2, 2, 2, 2, 2, 4 ),
 ( 0.004000878361811907070, 0.004499404418915900483, 0.004997930476019893896, 0.005496456533123887309, 0.005994982590227879854, 0.006244245618779876994, 0.006493508647331874134, 0.006992034704435890098, 0.007490560761539906062, 0.007989086818643922894 ),
 .UNSPECIFIED. ) ;
#25909=CARTESIAN_POINT ( 'NONE',  ( 12.14591786802309770, 12.06949235617756955, 99.37390960531436690 ) ) ;
#25911=CARTESIAN_POINT ( 'NONE',  ( 19.03943276465977164, -0.05219959533909143690, 78.74890960531436690 ) ) ;
#25913=CARTESIAN_POINT ( 'NONE',  ( -16.51473224551082808, 9.474510206698731452, 108.3344237280190043 ) ) ;
#25914=CARTESIAN_POINT ( 'NONE',  ( 18.62759615963271287, -10.81492255796078972, 28.33224293864769550 ) ) ;
#25915=CARTESIAN_POINT ( 'NONE',  ( -0.05219959533937732626, 21.53943276465977519, 47.50109039468568994 ) ) ;
#25916=CARTESIAN_POINT ( 'NONE',  ( -16.46253265017160317, 9.564922557960807481, 100.8322429386477097 ) ) ;
#25917=CARTESIAN_POINT ( 'NONE',  ( 16.46253265017146816, 9.564922557961045513, 76.66775706135234714 ) ) ;
#25918=CARTESIAN_POINT ( 'NONE',  ( -16.51473224551069308, -9.474510206698971260, 66.66557627198102409 ) ) ;
#25919=CARTESIAN_POINT ( 'NONE',  ( -4.483927247898539470, -16.52544592524342804, 87.29057627198103830 ) ) ;
#25920=CARTESIAN_POINT ( 'NONE',  ( -13.97604488694527625, -13.89961937509977652, 96.87390960531433848 ) ) ;
#25921=CARTESIAN_POINT ( 'NONE',  ( -14.29746914071049879, 8.314922557960819915, 80.83224293864769550 ) ) ;
#25922=CARTESIAN_POINT ( 'NONE',  ( 13.89961937509977652, -13.97604488694527269, 93.12390960531436690 ) ) ;
#25923=EDGE_CURVE ( 'NONE', #53380, #83853, #150801, .T. ) ;
#25924=CARTESIAN_POINT ( 'NONE',  ( 13.89961937509977652, -13.97604488694527269, 48.12390960531435979 ) ) ;
#25925=CARTESIAN_POINT ( 'NONE',  ( 8.314922557960818139, 14.29746914071049879, 44.58224293864769550 ) ) ;
#25926=CARTESIAN_POINT ( 'NONE',  ( 0.05219959533909260263, 19.03943276465977164, 29.99890960531435979 ) ) ;
#25927=EDGE_LOOP ( 'NONE', ( #72413, #118591, #153995, #166852 ) ) ;
#25928=CARTESIAN_POINT ( 'NONE',  ( 21.55341960407619695, -5.719274019375665929, 41.04275706135236135 ) ) ;
#25929=CARTESIAN_POINT ( 'NONE',  ( -19.02544592524334988, -5.153800228976617603, 78.95942372801900433 ) ) ;
#25930=CARTESIAN_POINT ( 'NONE',  ( -12.06949235617756955, 12.14591786802309770, 45.62390960531436690 ) ) ;
#25931=CARTESIAN_POINT ( 'NONE',  ( -21.52544592524343514, 5.823673210054127303, 96.04057627198102409 ) ) ;
#25932=CARTESIAN_POINT ( 'NONE',  ( 21.55341960407610458, 5.719274019375980345, 28.95724293864769905 ) ) ;
#25933=CARTESIAN_POINT ( 'NONE',  ( -8.224510206698948167, 14.34966873604960824, 80.41557627198103830 ) ) ;
#25934=CARTESIAN_POINT ( 'NONE',  ( -19.02544592524342804, 5.153800228976336051, 41.04057627198103120 ) ) ;
#25935=CARTESIAN_POINT ( 'NONE',  ( -16.55341960407611168, -4.379528057220339221, 26.45724293864768839 ) ) ;
#25936=CARTESIAN_POINT ( 'NONE',  ( 8.224510206698742110, 14.34966873604972548, 92.08442372801901854 ) ) ;
#25937=CARTESIAN_POINT ( 'NONE',  ( 16.53943276465976808, 0.05219959533934440121, 66.25109039468567573 ) ) ;
#25938=CARTESIAN_POINT ( 'NONE',  ( -9.564922557961040184, 16.46253265017147172, 27.91775706135232582 ) ) ;
#25939=CARTESIAN_POINT ( 'NONE',  ( -0.05219959533909027116, -19.03943276465977164, 87.49890960531436690 ) ) ;
#25940=CARTESIAN_POINT ( 'NONE',  ( -16.46253265017160317, 9.564922557960807481, 75.83224293864769550 ) ) ;
#25941=CARTESIAN_POINT ( 'NONE',  ( 14.34966873604972726, -8.224510206698740333, 75.83442372801900433 ) ) ;
#25942=CARTESIAN_POINT ( 'NONE',  ( -9.564922557960796823, -16.46253265017161027, 42.08224293864769550 ) ) ;
#25943=CARTESIAN_POINT ( 'NONE',  ( -4.379528057220328563, 16.55341960407611168, 50.20724293864769550 ) ) ;
#25945=CARTESIAN_POINT ( 'NONE',  ( 0.05219959533909260263, 19.03943276465977164, 104.9989096053143669 ) ) ;
#25946=CARTESIAN_POINT ( 'NONE',  ( 18.67979575497178502, 10.72451020669898547, 29.16557627198103120 ) ) ;
#25947=CARTESIAN_POINT ( 'NONE',  ( -8.224510206698948167, 14.34966873604960824, 70.41557627198102409 ) ) ;
#25948=CARTESIAN_POINT ( 'NONE',  ( -16.55341960407611168, -4.379528057220339221, 71.45724293864769550 ) ) ;
#25949=CARTESIAN_POINT ( 'NONE',  ( 17.50000000000150280, -3.202012800152198135, 32.42822416027275523 ) ) ;
#25950=CARTESIAN_POINT ( 'NONE',  ( -9.564922557961040184, 16.46253265017147172, 62.91775706135233293 ) ) ;
#25951=CARTESIAN_POINT ( 'NONE',  ( 13.89961937509977652, -13.97604488694527269, 98.12390960531433848 ) ) ;
#25952=CARTESIAN_POINT ( 'NONE',  ( -19.05341960407617563, 5.049401038297882671, 83.54275706135233293 ) ) ;
#25954=CARTESIAN_POINT ( 'NONE',  ( 9.564922557961047289, -16.46253265017146816, 105.4177570613523471 ) ) ;
#25955=CARTESIAN_POINT ( 'NONE',  ( -14.34966873604972548, 8.224510206698743886, 98.33442372801901854 ) ) ;
#25956=CARTESIAN_POINT ( 'NONE',  ( 9.474510206698971260, -16.51473224551069308, 42.91557627198103120 ) ) ;
#25957=CARTESIAN_POINT ( 'NONE',  ( 15.72974639402199770, -15.80617190586745480, 38.12390960531436690 ) ) ;
#25958=CARTESIAN_POINT ( 'NONE',  ( 21.53943276465977519, 0.05219959533937863772, 51.25109039468568994 ) ) ;
#25959=CARTESIAN_POINT ( 'NONE',  ( 16.52544592524335698, 4.483927247898782831, 26.45942372801901854 ) ) ;
#25961=CARTESIAN_POINT ( 'NONE',  ( -16.46253265017160317, 9.564922557960807481, 80.83224293864769550 ) ) ;
#25962=CARTESIAN_POINT ( 'NONE',  ( 5.049401038298161559, -19.05341960407611168, 112.7072429386476813 ) ) ;
#25963=CARTESIAN_POINT ( 'NONE',  ( 12.14591786802309770, 12.06949235617756955, 69.37390960531436690 ) ) ;
#25964=CARTESIAN_POINT ( 'NONE',  ( 16.51473224551069308, 9.474510206698969483, 79.16557627198103830 ) ) ;
#25965=CARTESIAN_POINT ( 'NONE',  ( 5.153800228976335163, 19.02544592524342804, 89.79057627198102409 ) ) ;
#25967=CARTESIAN_POINT ( 'NONE',  ( 19.03943276465977164, 0.05219959533936151252, 96.25109039468567573 ) ) ;
#25968=CARTESIAN_POINT ( 'NONE',  ( 18.62759615963271287, -10.81492255796078972, 58.33224293864768839 ) ) ;
#25969=CARTESIAN_POINT ( 'NONE',  ( -16.51473224551069308, -9.474510206698971260, 26.66557627198103120 ) ) ;
#25970=CARTESIAN_POINT ( 'NONE',  ( 0.05219959533936267826, -19.03943276465977164, 60.00109039468566863 ) ) ;
#25971=CARTESIAN_POINT ( 'NONE',  ( 13.97604488694527802, 13.89961937509977652, 59.37390960531434558 ) ) ;
#25972=CARTESIAN_POINT ( 'NONE',  ( -13.97604488694527625, -13.89961937509977652, 96.87390960531433848 ) ) ;
#25974=CARTESIAN_POINT ( 'NONE',  ( 21.55341960407610458, 5.719274019375980345, 88.95724293864769550 ) ) ;
#25975=CARTESIAN_POINT ( 'NONE',  ( 14.29746914071049879, -8.314922557960816363, 93.33224293864769550 ) ) ;
#25976=CARTESIAN_POINT ( 'NONE',  ( 9.474510206698729675, 16.51473224551082808, 47.08442372801900433 ) ) ;
#25977=CARTESIAN_POINT ( 'NONE',  ( 10.81492255796078972, 18.62759615963270932, 94.58224293864769550 ) ) ;
#25978=CARTESIAN_POINT ( 'NONE',  ( -15.80617190586745835, -15.72974639402198527, 76.87390960531439532 ) ) ;
#25979=CARTESIAN_POINT ( 'NONE',  ( -8.314922557960811034, -14.29746914071050412, 37.08224293864768129 ) ) ;
#25980=CARTESIAN_POINT ( 'NONE',  ( 15.72974639402176855, 15.80617190586768217, 101.8760903946857042 ) ) ;
#25981=CARTESIAN_POINT ( 'NONE',  ( -19.03943276465977164, 0.05219959533909376836, 81.24890960531436690 ) ) ;
#25982=CARTESIAN_POINT ( 'NONE',  ( -19.02544592524342804, 5.153800228976336051, 31.04057627198102409 ) ) ;
#25983=CARTESIAN_POINT ( 'NONE',  ( -5.719274019375665041, -21.55341960407619695, 39.79275706135235424 ) ) ;
#25984=CARTESIAN_POINT ( 'NONE',  ( 5.823673210054444382, -21.52544592524334988, 55.20942372801902565 ) ) ;
#25985=CARTESIAN_POINT ( 'NONE',  ( -19.02544592524342804, 5.153800228976336051, 51.04057627198103120 ) ) ;
#25986=CARTESIAN_POINT ( 'NONE',  ( 15.80617190586746368, 15.72974639402197994, 114.3739096053143527 ) ) ;
#25987=CARTESIAN_POINT ( 'NONE',  ( -5.049401038297874678, -19.05341960407617918, 64.79275706135233293 ) ) ;
#25988=CARTESIAN_POINT ( 'NONE',  ( 13.89961937509977652, -13.97604488694527269, 38.12390960531436690 ) ) ;
#25989=CARTESIAN_POINT ( 'NONE',  ( -8.224510206698735004, -14.34966873604973081, 24.58442372801901499 ) ) ;
#25990=CARTESIAN_POINT ( 'NONE',  ( 19.02544592524343514, -5.153800228976328945, 23.54057627198102054 ) ) ;
#25991=CARTESIAN_POINT ( 'NONE',  ( 8.224510206698742110, 14.34966873604972548, 77.08442372801901854 ) ) ;
#25992=CARTESIAN_POINT ( 'NONE',  ( -19.03943276465977164, 0.05219959533909376836, 36.24890960531436690 ) ) ;
#25994=CARTESIAN_POINT ( 'NONE',  ( 19.03943276465977164, -0.05219959533909143690, 83.74890960531436690 ) ) ;
#25995=CARTESIAN_POINT ( 'NONE',  ( 8.314922557960818139, 14.29746914071049879, 114.5822429386477097 ) ) ;
#25996=CARTESIAN_POINT ( 'NONE',  ( 21.55341960407610458, 5.719274019375980345, 73.95724293864769550 ) ) ;
#25998=CARTESIAN_POINT ( 'NONE',  ( 16.52544592524335698, 4.483927247898782831, 41.45942372801901143 ) ) ;
#25999=CARTESIAN_POINT ( 'NONE',  ( 18.62759615963255655, 10.81492255796105972, 111.6677570613523613 ) ) ;
#26000=CARTESIAN_POINT ( 'NONE',  ( 0.05219959533909260263, 19.03943276465977164, 34.99890960531435979 ) ) ;
#26001=CARTESIAN_POINT ( 'NONE',  ( 8.224510206698953496, -14.34966873604960469, 27.91557627198103830 ) ) ;
#26002=CARTESIAN_POINT ( 'NONE',  ( -14.34966873604960291, -8.224510206698953496, 71.66557627198100988 ) ) ;
#26003=CARTESIAN_POINT ( 'NONE',  ( 5.153800228976335163, 19.02544592524342804, 64.79057627198100988 ) ) ;
#26004=CARTESIAN_POINT ( 'NONE',  ( -16.46253265017146816, -9.564922557961047289, 19.16775706135233293 ) ) ;
#26005=CARTESIAN_POINT ( 'NONE',  ( -18.67979575497193778, 10.72451020669871902, 23.33442372801901499 ) ) ;
#26006=CARTESIAN_POINT ( 'NONE',  ( 9.474510206698971260, -16.51473224551069308, 77.91557627198103830 ) ) ;
#26007=CARTESIAN_POINT ( 'NONE',  ( 18.67979575497194134, -10.72451020669871369, 80.83442372801901854 ) ) ;
#26008=CARTESIAN_POINT ( 'NONE',  ( -0.05219959533934338120, 16.53943276465976808, 67.50109039468568994 ) ) ;
#26009=CARTESIAN_POINT ( 'NONE',  ( -9.564922557960796823, -16.46253265017161027, 112.0822429386476955 ) ) ;
#26010=CARTESIAN_POINT ( 'NONE',  ( 14.34966873604960469, 8.224510206698951720, 39.16557627198102409 ) ) ;
#26011=CARTESIAN_POINT ( 'NONE',  ( 19.02544592524343514, -5.153800228976328945, 33.54057627198102409 ) ) ;
#26012=CARTESIAN_POINT ( 'NONE',  ( 16.52544592524335698, 4.483927247898782831, 51.45942372801901854 ) ) ;
#26013=CARTESIAN_POINT ( 'NONE',  ( -8.314922557960811034, -14.29746914071050412, 52.08224293864768839 ) ) ;
#26014=CARTESIAN_POINT ( 'NONE',  ( -16.46253265017160317, 9.564922557960807481, 105.8322429386476955 ) ) ;
#26015=CARTESIAN_POINT ( 'NONE',  ( 10.81492255796078972, 18.62759615963270932, 34.58224293864770260 ) ) ;
#26016=CARTESIAN_POINT ( 'NONE',  ( 9.474510206698729675, 16.51473224551082808, 22.08442372801899722 ) ) ;
#26017=CARTESIAN_POINT ( 'NONE',  ( -8.314922557960811034, -14.29746914071050412, 87.08224293864769550 ) ) ;
#26018=CARTESIAN_POINT ( 'NONE',  ( -16.46253265017160317, 9.564922557960807481, 90.83224293864769550 ) ) ;
#26020=CARTESIAN_POINT ( 'NONE',  ( -16.52544592524335698, -4.483927247898792601, 43.95942372801902565 ) ) ;
#26021=CARTESIAN_POINT ( 'NONE',  ( 0.05219959533909260263, 19.03943276465977164, 59.99890960531436690 ) ) ;
#26022=CARTESIAN_POINT ( 'NONE',  ( 5.049401038297881783, 19.05341960407617563, 47.29275706135231161 ) ) ;
#26023=CARTESIAN_POINT ( 'NONE',  ( -19.03943276465977164, 0.05219959533909376836, 51.24890960531436690 ) ) ;
#26024=CARTESIAN_POINT ( 'NONE',  ( -14.29746914071037622, -8.314922557961029526, 79.16775706135234714 ) ) ;
#26025=CARTESIAN_POINT ( 'NONE',  ( -13.97604488694547697, 13.89961937509957934, 93.12609039468566152 ) ) ;
#26026=CARTESIAN_POINT ( 'NONE',  ( 15.72974639402176855, 15.80617190586768217, 61.87609039468568284 ) ) ;
#26027=CARTESIAN_POINT ( 'NONE',  ( 16.51473224551069308, 9.474510206698969483, 64.16557627198102409 ) ) ;
#26028=CARTESIAN_POINT ( 'NONE',  ( -10.81492255796078084, -18.62759615963271287, 92.08224293864769550 ) ) ;
#26029=CARTESIAN_POINT ( 'NONE',  ( -12.14591786802309592, -12.06949235617757132, 96.87390960531436690 ) ) ;
#26030=CARTESIAN_POINT ( 'NONE',  ( -5.153800228976607833, 19.02544592524334988, 67.70942372801900433 ) ) ;
#26031=CARTESIAN_POINT ( 'NONE',  ( -0.05219959533907301413, -21.53943276465977519, 67.49890960531436690 ) ) ;
#26032=CARTESIAN_POINT ( 'NONE',  ( 16.51473224551083163, -9.474510206698727899, 45.83442372801900433 ) ) ;
#26033=CARTESIAN_POINT ( 'NONE',  ( 16.51473224551069308, 9.474510206698969483, 114.1655762719810241 ) ) ;
#26034=CARTESIAN_POINT ( 'NONE',  ( 15.80617190586746368, 15.72974639402197994, 94.37390960531436690 ) ) ;
#26035=CARTESIAN_POINT ( 'NONE',  ( -18.87580814761071935, 5.500000000000041744, 55.87172394265761000 ) ) ;
#26036=CARTESIAN_POINT ( 'NONE',  ( -4.483927247898782831, 16.52544592524335698, 22.70942372801901499 ) ) ;
#26037=CARTESIAN_POINT ( 'NONE',  ( -19.36337904590691039, 5.499999999999949374, 60.41494137495623562 ) ) ;
#26038=CARTESIAN_POINT ( 'NONE',  ( -16.53943276465976808, -0.05219959533934237506, 28.75109039468567929 ) ) ;
#26039=CARTESIAN_POINT ( 'NONE',  ( -9.474510206698964154, 16.51473224551069663, 40.41557627198103120 ) ) ;
#26040=CARTESIAN_POINT ( 'NONE',  ( 9.564922557960805705, 16.46253265017160317, 104.5822429386476955 ) ) ;
#26041=CARTESIAN_POINT ( 'NONE',  ( 15.80617190586746368, 15.72974639402197994, 84.37390960531438111 ) ) ;
#26042=CARTESIAN_POINT ( 'NONE',  ( -15.72974639402176322, -15.80617190586768395, 69.37609039468567573 ) ) ;
#26043=CARTESIAN_POINT ( 'NONE',  ( 0.05219959533934541429, -16.53943276465976808, 30.00109039468568284 ) ) ;
#26044=CARTESIAN_POINT ( 'NONE',  ( -19.03943276465977164, -0.05219959533935918106, 33.75109039468566863 ) ) ;
#26045=CARTESIAN_POINT ( 'NONE',  ( -0.05219959533910754901, -16.53943276465976808, 27.49890960531435269 ) ) ;
#26046=CARTESIAN_POINT ( 'NONE',  ( -18.67979575497178146, -10.72451020669898902, 111.6655762719810525 ) ) ;
#26047=CARTESIAN_POINT ( 'NONE',  ( -14.34966873604960291, -8.224510206698953496, 51.66557627198102409 ) ) ;
#26048=CARTESIAN_POINT ( 'NONE',  ( 19.05341960407617918, -5.049401038297876454, 101.0427570613523045 ) ) ;
#26049=EDGE_CURVE ( 'NONE', #119129, #151905, #42620, .T. ) ;
#26050=CARTESIAN_POINT ( 'NONE',  ( 5.153800228976615827, -19.02544592524334988, 55.20942372801899722 ) ) ;
#26051=CARTESIAN_POINT ( 'NONE',  ( 21.55341960407619695, -5.719274019375665929, 66.04275706135236135 ) ) ;
#26052=CARTESIAN_POINT ( 'NONE',  ( 19.02544592524334988, 5.153800228976608722, 41.45942372801900433 ) ) ;
#26053=CARTESIAN_POINT ( 'NONE',  ( -13.89961937509977652, 13.97604488694528158, 25.62390960531434558 ) ) ;
#26054=CARTESIAN_POINT ( 'NONE',  ( 10.72451020669898902, -18.67979575497178502, 37.91557627198102409 ) ) ;
#26055=CARTESIAN_POINT ( 'NONE',  ( -16.53943276465976808, 0.05219959533911058130, 46.24890960531435979 ) ) ;
#26056=CARTESIAN_POINT ( 'NONE',  ( -18.22780087662121673, -5.500000000000063061, 51.48459894673893444 ) ) ;
#26057=CARTESIAN_POINT ( 'NONE',  ( -9.564922557961040184, 16.46253265017147172, 22.91775706135233648 ) ) ;
#26058=CARTESIAN_POINT ( 'NONE',  ( 8.224510206698742110, 14.34966873604972548, 77.08442372801901854 ) ) ;
#26059=CARTESIAN_POINT ( 'NONE',  ( -16.53943276465976808, 0.05219959533911058130, 41.24890960531435269 ) ) ;
#26060=CARTESIAN_POINT ( 'NONE',  ( -21.53943276465977519, -0.05219959533937600094, 73.75109039468567573 ) ) ;
#26061=CARTESIAN_POINT ( 'NONE',  ( -10.72451020669870658, -18.67979575497194134, 64.58442372801900433 ) ) ;
#26062=CARTESIAN_POINT ( 'NONE',  ( 5.719274019375991003, -21.55341960407610458, 82.70724293864770971 ) ) ;
#26063=CARTESIAN_POINT ( 'NONE',  ( -16.46253265017160317, 9.564922557960807481, 40.83224293864769550 ) ) ;
#26064=CARTESIAN_POINT ( 'NONE',  ( -0.05219959533937732626, 21.53943276465977519, 42.50109039468567573 ) ) ;
#26065=CARTESIAN_POINT ( 'NONE',  ( 13.97604488694527802, 13.89961937509977652, 29.37390960531435979 ) ) ;
#26066=CARTESIAN_POINT ( 'NONE',  ( 9.564922557960805705, 16.46253265017160317, 34.58224293864770260 ) ) ;
#26067=CARTESIAN_POINT ( 'NONE',  ( -4.379528057220328563, 16.55341960407611168, 90.20724293864770971 ) ) ;
#26068=CARTESIAN_POINT ( 'NONE',  ( 9.474510206698971260, -16.51473224551069308, 87.91557627198102409 ) ) ;
#26069=CARTESIAN_POINT ( 'NONE',  ( -0.05219959533910754901, -16.53943276465976808, 37.49890960531436690 ) ) ;
#26070=CARTESIAN_POINT ( 'NONE',  ( -14.34966873604960291, -8.224510206698953496, 96.66557627198102409 ) ) ;
#26071=CARTESIAN_POINT ( 'NONE',  ( -5.823673210054116645, -21.52544592524344225, 72.29057627198102409 ) ) ;
#26072=CARTESIAN_POINT ( 'NONE',  ( 15.80617190586746368, 15.72974639402197994, 109.3739096053143811 ) ) ;
#26073=CARTESIAN_POINT ( 'NONE',  ( 9.564922557960805705, 16.46253265017160317, 109.5822429386476955 ) ) ;
#26074=CARTESIAN_POINT ( 'NONE',  ( -9.564922557960796823, -16.46253265017161027, 67.08224293864769550 ) ) ;
#26075=CARTESIAN_POINT ( 'NONE',  ( -0.05219959533934338120, 16.53943276465976808, 22.50109039468567573 ) ) ;
#26076=CARTESIAN_POINT ( 'NONE',  ( 21.53943276465977519, -0.05219959533907433946, 68.74890960531435269 ) ) ;
#26077=CARTESIAN_POINT ( 'NONE',  ( 10.72451020669871369, 18.67979575497193778, 92.08442372801901854 ) ) ;
#26078=CARTESIAN_POINT ( 'NONE',  ( 9.474510206698971260, -16.51473224551069308, 82.91557627198103830 ) ) ;
#26079=CARTESIAN_POINT ( 'NONE',  ( 21.53943276465977519, -0.05219959533907433946, 108.7489096053143669 ) ) ;
#26080=CARTESIAN_POINT ( 'NONE',  ( -21.55341960407610458, -5.719274019375992779, 21.45724293864769550 ) ) ;
#26081=CARTESIAN_POINT ( 'NONE',  ( -16.52544592524335698, -4.483927247898792601, 83.95942372801900433 ) ) ;
#26082=CARTESIAN_POINT ( 'NONE',  ( 10.81492255796106328, -18.62759615963255655, 70.41775706135236135 ) ) ;
#26083=CARTESIAN_POINT ( 'NONE',  ( 15.72974639402176855, 15.80617190586768217, 101.8760903946857042 ) ) ;
#26084=CARTESIAN_POINT ( 'NONE',  ( -12.14591786802326823, 12.06949235617739902, 63.12609039468568994 ) ) ;
#26085=CARTESIAN_POINT ( 'NONE',  ( 15.80617190586769283, -15.72974639402175789, 25.62609039468567929 ) ) ;
#26086=CARTESIAN_POINT ( 'NONE',  ( 5.049401038298161559, -19.05341960407611168, 112.7072429386476813 ) ) ;
#26087=CARTESIAN_POINT ( 'NONE',  ( -0.05219959533937732626, 21.53943276465977519, 87.50109039468568994 ) ) ;
#26088=CARTESIAN_POINT ( 'NONE',  ( 19.02544592524343514, -5.153800228976328945, 93.54057627198102409 ) ) ;
#26089=CARTESIAN_POINT ( 'NONE',  ( -18.62759615963270932, 10.81492255796079327, 90.83224293864769550 ) ) ;
#26090=CARTESIAN_POINT ( 'NONE',  ( 0.05219959533936267826, -19.03943276465977164, 55.00109039468566863 ) ) ;
#26091=CARTESIAN_POINT ( 'NONE',  ( -21.53943276465977519, 0.05219959533907696930, 51.24890960531436690 ) ) ;
#26092=CARTESIAN_POINT ( 'NONE',  ( -9.474510206698964154, 16.51473224551069663, 100.4155762719810241 ) ) ;
#26093=CARTESIAN_POINT ( 'NONE',  ( 12.14591786802309770, 12.06949235617756955, 34.37390960531435979 ) ) ;
#26095=CARTESIAN_POINT ( 'NONE',  ( 9.474510206698729675, 16.51473224551082808, 82.08442372801899012 ) ) ;
#26097=CARTESIAN_POINT ( 'NONE',  ( -19.39056639909675894, -5.499999999999968914, 80.78948781074343799 ) ) ;
#26098=CARTESIAN_POINT ( 'NONE',  ( 19.05341960407617918, -5.049401038297876454, 106.0427570613523471 ) ) ;
#26099=CARTESIAN_POINT ( 'NONE',  ( 15.80617190586746368, 15.72974639402197994, 84.37390960531438111 ) ) ;
#26100=CARTESIAN_POINT ( 'NONE',  ( 8.314922557960818139, 14.29746914071049879, 69.58224293864769550 ) ) ;
#26101=CARTESIAN_POINT ( 'NONE',  ( 12.06949235617739724, 12.14591786802326823, 31.87609039468567929 ) ) ;
#26102=CARTESIAN_POINT ( 'NONE',  ( -5.153800228976328057, -19.02544592524343514, 42.29057627198101699 ) ) ;
#26103=CARTESIAN_POINT ( 'NONE',  ( 15.72974639402176855, 15.80617190586768217, 21.87609039468567573 ) ) ;
#26104=CARTESIAN_POINT ( 'NONE',  ( 5.049401038297881783, 19.05341960407617563, 82.29275706135229029 ) ) ;
#26105=CARTESIAN_POINT ( 'NONE',  ( -19.05341960407611168, -5.049401038298163336, 91.45724293864766707 ) ) ;
#26106=CARTESIAN_POINT ( 'NONE',  ( -16.51473224551069308, -9.474510206698971260, 76.66557627198103830 ) ) ;
#26107=CARTESIAN_POINT ( 'NONE',  ( 18.62759615963271287, -10.81492255796078972, 78.33224293864770971 ) ) ;
#26108=CARTESIAN_POINT ( 'NONE',  ( -19.05341960407611168, -5.049401038298163336, 51.45724293864770260 ) ) ;
#26110=CARTESIAN_POINT ( 'NONE',  ( -14.29746914071049879, 8.314922557960819915, 60.83224293864769550 ) ) ;
#26111=CARTESIAN_POINT ( 'NONE',  ( 9.474510206698971260, -16.51473224551069308, 87.91557627198102409 ) ) ;
#26113=CARTESIAN_POINT ( 'NONE',  ( 5.049401038297881783, 19.05341960407617563, 67.29275706135234714 ) ) ;
#26114=CARTESIAN_POINT ( 'NONE',  ( 21.52544592524344225, -5.823673210054117533, 73.54057627198102409 ) ) ;
#26115=CARTESIAN_POINT ( 'NONE',  ( -19.02544592524334988, -5.153800228976617603, 38.95942372801900433 ) ) ;
#26116=CARTESIAN_POINT ( 'NONE',  ( 13.97604488694527802, 13.89961937509977652, 104.3739096053143385 ) ) ;
#26117=CARTESIAN_POINT ( 'NONE',  ( -17.50000000000000355, 3.237210098469587738, 114.7123698737954101 ) ) ;
#26118=CARTESIAN_POINT ( 'NONE',  ( 21.55341960407610458, 5.719274019375980345, 38.95724293864768839 ) ) ;
#26119=CARTESIAN_POINT ( 'NONE',  ( -16.51473224551069308, -9.474510206698971260, 71.66557627198102409 ) ) ;
#26120=CARTESIAN_POINT ( 'NONE',  ( -5.719274019375665041, -21.55341960407619695, 64.79275706135234714 ) ) ;
#26121=CARTESIAN_POINT ( 'NONE',  ( -9.564922557960796823, -16.46253265017161027, 27.08224293864769550 ) ) ;
#26123=CARTESIAN_POINT ( 'NONE',  ( 0.05219959533907565091, 21.53943276465977519, 114.9989096053143669 ) ) ;
#26125=CARTESIAN_POINT ( 'NONE',  ( -21.55341960407619339, 5.719274019375674811, 48.54275706135234714 ) ) ;
#26128=CARTESIAN_POINT ( 'NONE',  ( -16.51473224551082808, 9.474510206698731452, 63.33442372801900433 ) ) ;
#26130=CARTESIAN_POINT ( 'NONE',  ( 15.80617190586746368, 15.72974639402197994, 109.3739096053143811 ) ) ;
#26131=CARTESIAN_POINT ( 'NONE',  ( -16.46253265017160317, 9.564922557960807481, 65.83224293864769550 ) ) ;
#26132=CARTESIAN_POINT ( 'NONE',  ( 0.05219959533934541429, -16.53943276465976808, 35.00109039468568284 ) ) ;
#26134=CARTESIAN_POINT ( 'NONE',  ( 21.53943276465977519, 0.05219959533937863772, 101.2510903946856757 ) ) ;
#26135=CARTESIAN_POINT ( 'NONE',  ( 5.153800228976335163, 19.02544592524342804, 44.79057627198103830 ) ) ;
#26136=CARTESIAN_POINT ( 'NONE',  ( -10.81492255796105439, 18.62759615963255655, 107.9177570613523471 ) ) ;
#26138=CARTESIAN_POINT ( 'NONE',  ( 19.02544592524343514, -5.153800228976328945, 83.54057627198100988 ) ) ;
#26139=CARTESIAN_POINT ( 'NONE',  ( -10.72451020669870658, -18.67979575497194134, 54.58442372801901143 ) ) ;
#26141=CARTESIAN_POINT ( 'NONE',  ( 19.03943276465977164, -0.05219959533909143690, 108.7489096053143527 ) ) ;
#26143=CARTESIAN_POINT ( 'NONE',  ( 8.224510206698742110, 14.34966873604972548, 52.08442372801901854 ) ) ;
#26144=CARTESIAN_POINT ( 'NONE',  ( -21.53943276465977519, -0.05219959533937600094, 68.75109039468568994 ) ) ;
#26145=CARTESIAN_POINT ( 'NONE',  ( -21.52544592524334988, -5.823673210054445271, 88.95942372801901854 ) ) ;
#26147=CARTESIAN_POINT ( 'NONE',  ( -8.314922557961024197, 14.29746914071037800, 22.91775706135235069 ) ) ;
#26148=CARTESIAN_POINT ( 'NONE',  ( -5.049401038298153566, 19.05341960407611168, 85.20724293864766707 ) ) ;
#26149=CARTESIAN_POINT ( 'NONE',  ( -19.05341960407611168, -5.049401038298163336, 106.4572429386476955 ) ) ;
#26150=ORIENTED_EDGE ( 'NONE', *, *, #3493, .F. ) ;
#26151=CARTESIAN_POINT ( 'NONE',  ( 17.49999999999999289, 5.500000000000063061, 41.70309617465829177 ) ) ;
#26152=CARTESIAN_POINT ( 'NONE',  ( -19.03943276465977164, 0.05219959533909376836, 21.24890960531436335 ) ) ;
#26153=CARTESIAN_POINT ( 'NONE',  ( 18.67979575497178502, 10.72451020669898547, 44.16557627198103120 ) ) ;
#26154=CARTESIAN_POINT ( 'NONE',  ( -8.224510206698735004, -14.34966873604973081, 94.58442372801901854 ) ) ;
#26155=CARTESIAN_POINT ( 'NONE',  ( -12.14591786802309592, -12.06949235617757132, 86.87390960531438111 ) ) ;
#26156=CARTESIAN_POINT ( 'NONE',  ( 5.049401038298161559, -19.05341960407611168, 72.70724293864768129 ) ) ;
#26157=CARTESIAN_POINT ( 'NONE',  ( 10.81492255796106328, -18.62759615963255655, 90.41775706135236135 ) ) ;
#26159=CARTESIAN_POINT ( 'NONE',  ( 4.483927247898790824, -16.52544592524335698, 20.20942372801900788 ) ) ;
#26160=CARTESIAN_POINT ( 'NONE',  ( 8.314922557960818139, 14.29746914071049879, 89.58224293864768129 ) ) ;
#26161=CARTESIAN_POINT ( 'NONE',  ( 21.52544592524334988, 5.823673210054432836, 41.45942372801901143 ) ) ;
#26162=CARTESIAN_POINT ( 'NONE',  ( -18.62759615963270932, 10.81492255796079327, 75.83224293864769550 ) ) ;
#26163=CARTESIAN_POINT ( 'NONE',  ( 19.02544592524334988, 5.153800228976608722, 41.45942372801900433 ) ) ;
#26165=CARTESIAN_POINT ( 'NONE',  ( 13.97604488694527802, 13.89961937509977652, 89.37390960531436690 ) ) ;
#26166=CARTESIAN_POINT ( 'NONE',  ( -4.379528057220328563, 16.55341960407611168, 65.20724293864768129 ) ) ;
#26167=CARTESIAN_POINT ( 'NONE',  ( 16.52544592524342804, -4.483927247898539470, 38.54057627198103120 ) ) ;
#26168=CARTESIAN_POINT ( 'NONE',  ( 8.224510206698953496, -14.34966873604960469, 22.91557627198102765 ) ) ;
#26169=CARTESIAN_POINT ( 'NONE',  ( 5.049401038297881783, 19.05341960407617563, 67.29275706135234714 ) ) ;
#26171=CARTESIAN_POINT ( 'NONE',  ( -13.97604488694527625, -13.89961937509977652, 111.8739096053143243 ) ) ;
#26172=CARTESIAN_POINT ( 'NONE',  ( -14.34966873604960291, -8.224510206698953496, 81.66557627198103830 ) ) ;
#26173=CARTESIAN_POINT ( 'NONE',  ( 19.27311148717739897, -5.499999999999809930, 38.03971402910765676 ) ) ;
#26174=CARTESIAN_POINT ( 'NONE',  ( 13.89961937509977652, -13.97604488694527269, 43.12390960531434558 ) ) ;
#26175=CARTESIAN_POINT ( 'NONE',  ( -18.67979575497178146, -10.72451020669898902, 51.66557627198102409 ) ) ;
#26176=CARTESIAN_POINT ( 'NONE',  ( 18.62759615963271287, -10.81492255796078972, 73.33224293864769550 ) ) ;
#26177=CARTESIAN_POINT ( 'NONE',  ( -0.05219959533910754901, -16.53943276465976808, 107.4989096053143669 ) ) ;
#26178=CARTESIAN_POINT ( 'NONE',  ( 12.14591786802327356, -12.06949235617739191, 60.62609039468567573 ) ) ;
#26179=CARTESIAN_POINT ( 'NONE',  ( 13.97604488694527802, 13.89961937509977652, 44.37390960531435269 ) ) ;
#26180=CARTESIAN_POINT ( 'NONE',  ( 5.823673210054444382, -21.52544592524334988, 60.20942372801902565 ) ) ;
#26182=CARTESIAN_POINT ( 'NONE',  ( -8.224510206698948167, 14.34966873604960824, 100.4155762719810241 ) ) ;
#26183=CARTESIAN_POINT ( 'NONE',  ( 13.97604488694548053, -13.89961937509957401, 95.62609039468563310 ) ) ;
#26186=CARTESIAN_POINT ( 'NONE',  ( 21.53943276465977519, -0.05219959533907433946, 43.74890960531435979 ) ) ;
#26187=CARTESIAN_POINT ( 'NONE',  ( 19.05341960407611168, 5.049401038298154454, 28.95724293864769550 ) ) ;
#26188=CARTESIAN_POINT ( 'NONE',  ( 18.67979575497194134, -10.72451020669871369, 85.83442372801901854 ) ) ;
#26189=CARTESIAN_POINT ( 'NONE',  ( 8.314922557960818139, 14.29746914071049879, 39.58224293864769550 ) ) ;
#26190=CARTESIAN_POINT ( 'NONE',  ( 16.55341960407618274, -4.379528057220086978, 51.04275706135234714 ) ) ;
#26191=CARTESIAN_POINT ( 'NONE',  ( 14.29746914071049879, -8.314922557960816363, 43.33224293864769550 ) ) ;
#26192=CARTESIAN_POINT ( 'NONE',  ( -0.05219959533907301413, -21.53943276465977519, 72.49890960531435269 ) ) ;
#26194=CARTESIAN_POINT ( 'NONE',  ( 10.72451020669898902, -18.67979575497178502, 77.91557627198102409 ) ) ;
#26196=CARTESIAN_POINT ( 'NONE',  ( -13.89961937509957401, -13.97604488694547875, 89.37609039468563310 ) ) ;
#26197=CARTESIAN_POINT ( 'NONE',  ( -0.05219959533907301413, -21.53943276465977519, 22.49890960531436335 ) ) ;
#26198=CARTESIAN_POINT ( 'NONE',  ( -5.153800228976328057, -19.02544592524343514, 47.29057627198102409 ) ) ;
#26199=CARTESIAN_POINT ( 'NONE',  ( 13.89961937509977652, -13.97604488694527269, 23.12390960531436335 ) ) ;
#26202=CARTESIAN_POINT ( 'NONE',  ( 4.483927247898790824, -16.52544592524335698, 80.20942372801901854 ) ) ;
#26203=CARTESIAN_POINT ( 'NONE',  ( -18.62759615963270932, 10.81492255796079327, 110.8322429386476955 ) ) ;
#26204=CARTESIAN_POINT ( 'NONE',  ( 13.89961937509977652, -13.97604488694527269, 73.12390960531436690 ) ) ;
#26205=CARTESIAN_POINT ( 'NONE',  ( -10.72451020669870658, -18.67979575497194134, 39.58442372801901143 ) ) ;
#26206=CARTESIAN_POINT ( 'NONE',  ( -16.51473224551069308, -9.474510206698971260, 101.6655762719810241 ) ) ;
#26208=VERTEX_POINT ( 'NONE', #182126 ) ;
#26209=CARTESIAN_POINT ( 'NONE',  ( 15.72974639402176855, 15.80617190586768217, 26.87609039468567218 ) ) ;
#26210=CARTESIAN_POINT ( 'NONE',  ( 19.03943276465977164, -0.05219959533909143690, 23.74890960531435269 ) ) ;
#26211=CARTESIAN_POINT ( 'NONE',  ( -13.97604488694547697, 13.89961937509957934, 88.12609039468563310 ) ) ;
#26212=CARTESIAN_POINT ( 'NONE',  ( -9.474510206698720793, -16.51473224551083518, 39.58442372801899722 ) ) ;
#26213=CARTESIAN_POINT ( 'NONE',  ( -0.05219959533907301413, -21.53943276465977519, 107.4989096053143669 ) ) ;
#26214=CARTESIAN_POINT ( 'NONE',  ( -9.474510206698720793, -16.51473224551083518, 39.58442372801899722 ) ) ;
#26215=CARTESIAN_POINT ( 'NONE',  ( 13.89961937509957401, 13.97604488694547697, 51.87609039468566863 ) ) ;
#26216=CARTESIAN_POINT ( 'NONE',  ( 4.379528057220092307, 16.55341960407617563, 92.29275706135236135 ) ) ;
#26217=CARTESIAN_POINT ( 'NONE',  ( 18.22780087662122384, -5.500000000000022204, 56.01540105326107977 ) ) ;
#26218=CARTESIAN_POINT ( 'NONE',  ( 16.51473224551069308, 9.474510206698969483, 69.16557627198102409 ) ) ;
#26219=CARTESIAN_POINT ( 'NONE',  ( 21.55341960407619695, -5.719274019375665929, 86.04275706135236135 ) ) ;
#26220=CARTESIAN_POINT ( 'NONE',  ( -10.72451020669870658, -18.67979575497194134, 94.58442372801901854 ) ) ;
#26222=CARTESIAN_POINT ( 'NONE',  ( -19.05341960407611168, -5.049401038298163336, 86.45724293864769550 ) ) ;
#26223=CARTESIAN_POINT ( 'NONE',  ( -18.67979575497193778, 10.72451020669871902, 63.33442372801900433 ) ) ;
#26224=CARTESIAN_POINT ( 'NONE',  ( 16.46253265017146816, 9.564922557961045513, 106.6677570613523471 ) ) ;
#26225=CARTESIAN_POINT ( 'NONE',  ( 19.05341960407611168, 5.049401038298154454, 63.95724293864769550 ) ) ;
#26226=CARTESIAN_POINT ( 'NONE',  ( -5.049401038298153566, 19.05341960407611168, 110.2072429386476671 ) ) ;
#26227=EDGE_CURVE ( 'NONE', #70081, #30365, #194315, .T. ) ;
#26228=CARTESIAN_POINT ( 'NONE',  ( -19.05341960407611168, -5.049401038298163336, 81.45724293864769550 ) ) ;
#26229=CARTESIAN_POINT ( 'NONE',  ( -17.26172910966779739, -6.454744622555839584, 89.19353091350777163 ) ) ;
#26230=CARTESIAN_POINT ( 'NONE',  ( 5.049401038298161559, -19.05341960407611168, 67.70724293864769550 ) ) ;
#26231=CARTESIAN_POINT ( 'NONE',  ( 5.049401038298161559, -19.05341960407611168, 47.70724293864770260 ) ) ;
#26232=CARTESIAN_POINT ( 'NONE',  ( -18.62759615963255300, -10.81492255796106328, 19.16775706135234714 ) ) ;
#26233=CARTESIAN_POINT ( 'NONE',  ( -8.224510206698735004, -14.34966873604973081, 99.58442372801900433 ) ) ;
#26235=SPHERICAL_SURFACE ( 'NONE', #78701, 2.000000000000000000 ) ;
#26236=CARTESIAN_POINT ( 'NONE',  ( -13.89961937509957401, -13.97604488694547875, 54.37609039468565442 ) ) ;
#26237=CARTESIAN_POINT ( 'NONE',  ( -19.05341960407611168, -5.049401038298163336, 81.45724293864769550 ) ) ;
#26238=CARTESIAN_POINT ( 'NONE',  ( -4.483927247898539470, -16.52544592524342804, 77.29057627198102409 ) ) ;
#26239=CARTESIAN_POINT ( 'NONE',  ( -8.314922557960811034, -14.29746914071050412, 107.0822429386476955 ) ) ;
#26240=CARTESIAN_POINT ( 'NONE',  ( 5.823673210054125526, 21.52544592524343514, 34.79057627198103120 ) ) ;
#26241=CARTESIAN_POINT ( 'NONE',  ( 19.02544592524343514, -5.153800228976328945, 108.5405762719810383 ) ) ;
#26242=CARTESIAN_POINT ( 'NONE',  ( 14.34966873604960469, 8.224510206698951720, 89.16557627198102409 ) ) ;
#26244=CARTESIAN_POINT ( 'NONE',  ( 13.97604488694548053, -13.89961937509957401, 35.62609039468567573 ) ) ;
#26245=CARTESIAN_POINT ( 'NONE',  ( 12.06949235617739724, 12.14591786802326823, 111.8760903946856615 ) ) ;
#26246=CARTESIAN_POINT ( 'NONE',  ( -9.474510206698964154, 16.51473224551069663, 90.41557627198103830 ) ) ;
#26247=CARTESIAN_POINT ( 'NONE',  ( 10.72451020669871369, 18.67979575497193778, 52.08442372801901854 ) ) ;
#26248=CARTESIAN_POINT ( 'NONE',  ( 21.52544592524344225, -5.823673210054117533, 38.54057627198103120 ) ) ;
#26249=CARTESIAN_POINT ( 'NONE',  ( -21.53943276465977519, -0.05219959533937600094, 28.75109039468567929 ) ) ;
#26250=CARTESIAN_POINT ( 'NONE',  ( -0.05219959533907301413, -21.53943276465977519, 67.49890960531436690 ) ) ;
#26251=CARTESIAN_POINT ( 'NONE',  ( -16.55341960407611168, -4.379528057220339221, 101.4572429386476955 ) ) ;
#26252=CARTESIAN_POINT ( 'NONE',  ( 5.153800228976615827, -19.02544592524334988, 55.20942372801899722 ) ) ;
#26253=CARTESIAN_POINT ( 'NONE',  ( 19.03943276465977164, -0.05219959533909143690, 33.74890960531435979 ) ) ;
#26254=CARTESIAN_POINT ( 'NONE',  ( 9.474510206698971260, -16.51473224551069308, 102.9155762719810241 ) ) ;
#26255=CARTESIAN_POINT ( 'NONE',  ( -19.02544592524342804, 5.153800228976336051, 96.04057627198103830 ) ) ;
#26256=CARTESIAN_POINT ( 'NONE',  ( -5.049401038298153566, 19.05341960407611168, 25.20724293864768484 ) ) ;
#26257=CARTESIAN_POINT ( 'NONE',  ( 14.29746914071049879, -8.314922557960816363, 33.33224293864769550 ) ) ;
#26258=CARTESIAN_POINT ( 'NONE',  ( 0.05219959533934541429, -16.53943276465976808, 35.00109039468568284 ) ) ;
#26259=CARTESIAN_POINT ( 'NONE',  ( -5.719274019375665041, -21.55341960407619695, 109.7927570613523613 ) ) ;
#26260=CARTESIAN_POINT ( 'NONE',  ( -13.97604488694527625, -13.89961937509977652, 96.87390960531433848 ) ) ;
#26261=CARTESIAN_POINT ( 'NONE',  ( -16.55341960407611168, -4.379528057220339221, 26.45724293864768839 ) ) ;
#26262=CARTESIAN_POINT ( 'NONE',  ( -10.72451020669870658, -18.67979575497194134, 34.58442372801900433 ) ) ;
#26263=CARTESIAN_POINT ( 'NONE',  ( 0.05219959533909260263, 19.03943276465977164, 39.99890960531436690 ) ) ;
#26264=CARTESIAN_POINT ( 'NONE',  ( 12.06949235617739724, 12.14591786802326823, 41.87609039468568284 ) ) ;
#26265=CARTESIAN_POINT ( 'NONE',  ( 4.483927247898790824, -16.52544592524335698, 105.2094237280190328 ) ) ;
#26266=CARTESIAN_POINT ( 'NONE',  ( 4.379528057220092307, 16.55341960407617563, 92.29275706135236135 ) ) ;
#26267=CARTESIAN_POINT ( 'NONE',  ( 5.153800228976615827, -19.02544592524334988, 110.2094237280189901 ) ) ;
#26268=CARTESIAN_POINT ( 'NONE',  ( 13.97604488694527802, 13.89961937509977652, 39.37390960531435269 ) ) ;
#26269=CARTESIAN_POINT ( 'NONE',  ( 8.314922557960818139, 14.29746914071049879, 94.58224293864769550 ) ) ;
#26270=CARTESIAN_POINT ( 'NONE',  ( 5.719274019375991003, -21.55341960407610458, 97.70724293864772392 ) ) ;
#26271=CARTESIAN_POINT ( 'NONE',  ( -13.97604488694527625, -13.89961937509977652, 36.87390960531436690 ) ) ;
#26272=CARTESIAN_POINT ( 'NONE',  ( -9.474510206698964154, 16.51473224551069663, 110.4155762719810383 ) ) ;
#26273=CARTESIAN_POINT ( 'NONE',  ( -21.52544592524334988, -5.823673210054445271, 28.95942372801902209 ) ) ;
#26275=CARTESIAN_POINT ( 'NONE',  ( 5.049401038298161559, -19.05341960407611168, 102.7072429386476955 ) ) ;
#26277=CARTESIAN_POINT ( 'NONE',  ( -9.564922557960796823, -16.46253265017161027, 82.08224293864768129 ) ) ;
#26278=CARTESIAN_POINT ( 'NONE',  ( 18.67979575497194134, -10.72451020669871369, 35.83442372801901143 ) ) ;
#26279=CARTESIAN_POINT ( 'NONE',  ( -4.379528057220328563, 16.55341960407611168, 95.20724293864769550 ) ) ;
#26280=CARTESIAN_POINT ( 'NONE',  ( -16.51473224551069308, -9.474510206698971260, 96.66557627198102409 ) ) ;
#26281=CARTESIAN_POINT ( 'NONE',  ( 19.05341960407617918, -5.049401038297876454, 21.04275706135232582 ) ) ;
#26282=CARTESIAN_POINT ( 'NONE',  ( 0.05219959533934541429, -16.53943276465976808, 60.00109039468568284 ) ) ;
#26283=CARTESIAN_POINT ( 'NONE',  ( 15.80617190586769283, -15.72974639402175789, 85.62609039468568994 ) ) ;
#26284=CARTESIAN_POINT ( 'NONE',  ( -0.05219959533934338120, 16.53943276465976808, 37.50109039468568284 ) ) ;
#26285=CARTESIAN_POINT ( 'NONE',  ( -16.51473224551069308, -9.474510206698971260, 86.66557627198102409 ) ) ;
#26287=CARTESIAN_POINT ( 'NONE',  ( -16.53943276465976808, -0.05219959533934237506, 18.75109039468568639 ) ) ;
#26288=CARTESIAN_POINT ( 'NONE',  ( -16.55341960407617563, 4.379528057220093196, 63.54275706135234003 ) ) ;
#26289=CARTESIAN_POINT ( 'NONE',  ( -13.89961937509957401, -13.97604488694547875, 19.37609039468566507 ) ) ;
#26290=CARTESIAN_POINT ( 'NONE',  ( 9.474510206698729675, 16.51473224551082808, 87.08442372801900433 ) ) ;
#26291=CARTESIAN_POINT ( 'NONE',  ( -13.97604488694527625, -13.89961937509977652, 61.87390960531435979 ) ) ;
#26292=CARTESIAN_POINT ( 'NONE',  ( 5.823673210054125526, 21.52544592524343514, 89.79057627198103830 ) ) ;
#26293=CARTESIAN_POINT ( 'NONE',  ( 4.483927247898545687, 16.52544592524342804, 89.79057627198103830 ) ) ;
#26294=CARTESIAN_POINT ( 'NONE',  ( -19.03943276465977164, -0.05219959533935918106, 88.75109039468567573 ) ) ;
#26295=CARTESIAN_POINT ( 'NONE',  ( -14.29746914071037622, -8.314922557961029526, 59.16775706135234714 ) ) ;
#26296=CARTESIAN_POINT ( 'NONE',  ( -19.26498983726236602, 5.499999999999801048, 80.55319577422004329 ) ) ;
#26297=CARTESIAN_POINT ( 'NONE',  ( -16.46253265017146816, -9.564922557961047289, 59.16775706135233293 ) ) ;
#26298=CARTESIAN_POINT ( 'NONE',  ( -16.53943276465976808, 0.05219959533911058130, 36.24890960531435979 ) ) ;
#26299=CARTESIAN_POINT ( 'NONE',  ( -16.55341960407611168, -4.379528057220339221, 86.45724293864770971 ) ) ;
#26300=CARTESIAN_POINT ( 'NONE',  ( -18.67979575497193778, 10.72451020669871902, 113.3344237280190328 ) ) ;
#26302=CARTESIAN_POINT ( 'NONE',  ( -5.823673210054431948, 21.52544592524334988, 27.70942372801901854 ) ) ;
#26303=CARTESIAN_POINT ( 'NONE',  ( 5.153800228976335163, 19.02544592524342804, 94.79057627198103830 ) ) ;
#26304=CARTESIAN_POINT ( 'NONE',  ( 16.46253265017160672, -9.564922557960803928, 73.33224293864769550 ) ) ;
#26305=CARTESIAN_POINT ( 'NONE',  ( -0.05219959533937732626, 21.53943276465977519, 102.5010903946856899 ) ) ;
#26306=CARTESIAN_POINT ( 'NONE',  ( -0.05219959533909027116, -19.03943276465977164, 62.49890960531435979 ) ) ;
#26307=ORIENTED_EDGE ( 'NONE', *, *, #120448, .F. ) ;
#26308=CARTESIAN_POINT ( 'NONE',  ( -10.72451020669898014, 18.67979575497178502, 30.41557627198101699 ) ) ;
#26309=CARTESIAN_POINT ( 'NONE',  ( 4.483927247898545687, 16.52544592524342804, 84.79057627198102409 ) ) ;
#26310=CARTESIAN_POINT ( 'NONE',  ( 19.05341960407611168, 5.049401038298154454, 43.95724293864769550 ) ) ;
#26311=CARTESIAN_POINT ( 'NONE',  ( -14.29746914071049879, 8.314922557960819915, 95.83224293864770971 ) ) ;
#26312=CARTESIAN_POINT ( 'NONE',  ( -21.52544592524343514, 5.823673210054127303, 116.0405762719810383 ) ) ;
#26313=CARTESIAN_POINT ( 'NONE',  ( 21.52544592524334988, 5.823673210054432836, 61.45942372801901854 ) ) ;
#26314=CARTESIAN_POINT ( 'NONE',  ( -0.05219959533909027116, -19.03943276465977164, 37.49890960531436690 ) ) ;
#26315=CARTESIAN_POINT ( 'NONE',  ( -4.379528057220086978, -16.55341960407618274, 64.79275706135234714 ) ) ;
#26316=EDGE_CURVE ( 'NONE', #14227, #109472, #42623, .T. ) ;
#26317=CARTESIAN_POINT ( 'NONE',  ( 15.72974639402199770, -15.80617190586745480, 103.1239096053143811 ) ) ;
#26318=CARTESIAN_POINT ( 'NONE',  ( -21.53943276465977519, 0.05219959533907696930, 111.2489096053143669 ) ) ;
#26319=CARTESIAN_POINT ( 'NONE',  ( -19.03943276465977164, -0.05219959533935918106, 38.75109039468566152 ) ) ;
#26320=CARTESIAN_POINT ( 'NONE',  ( 5.049401038298161559, -19.05341960407611168, 57.70724293864769550 ) ) ;
#26321=CARTESIAN_POINT ( 'NONE',  ( -16.46253265017160317, 9.564922557960807481, 115.8322429386477097 ) ) ;
#26322=CARTESIAN_POINT ( 'NONE',  ( 5.719274019375673035, 21.55341960407619339, 62.29275706135236845 ) ) ;
#26323=CARTESIAN_POINT ( 'NONE',  ( 5.719274019375991003, -21.55341960407610458, 57.70724293864770260 ) ) ;
#26324=CARTESIAN_POINT ( 'NONE',  ( -4.483927247898539470, -16.52544592524342804, 37.29057627198102409 ) ) ;
#26325=CARTESIAN_POINT ( 'NONE',  ( 21.55341960407619695, -5.719274019375665929, 71.04275706135234714 ) ) ;
#26326=CARTESIAN_POINT ( 'NONE',  ( 15.80617190586769283, -15.72974639402175789, 105.6260903946856899 ) ) ;
#26327=CARTESIAN_POINT ( 'NONE',  ( -8.224510206698948167, 14.34966873604960824, 60.41557627198102409 ) ) ;
#26328=CARTESIAN_POINT ( 'NONE',  ( -16.52544592524342804, 4.483927247898546575, 111.0405762719810525 ) ) ;
#26329=CARTESIAN_POINT ( 'NONE',  ( 0.05219959533936267826, -19.03943276465977164, 45.00109039468566863 ) ) ;
#26330=CARTESIAN_POINT ( 'NONE',  ( -8.224510206698735004, -14.34966873604973081, 99.58442372801900433 ) ) ;
#26331=CARTESIAN_POINT ( 'NONE',  ( -5.719274019375665041, -21.55341960407619695, 69.79275706135234714 ) ) ;
#26332=CARTESIAN_POINT ( 'NONE',  ( 19.03943276465977164, -0.05219959533909143690, 53.74890960531436690 ) ) ;
#26333=CARTESIAN_POINT ( 'NONE',  ( 19.03943276465977164, 0.05219959533936151252, 31.25109039468566863 ) ) ;
#26334=CARTESIAN_POINT ( 'NONE',  ( 10.72451020669898902, -18.67979575497178502, 37.91557627198102409 ) ) ;
#26335=CARTESIAN_POINT ( 'NONE',  ( 15.80617190586769283, -15.72974639402175789, 25.62609039468567929 ) ) ;
#26336=CARTESIAN_POINT ( 'NONE',  ( 15.80617190586746368, 15.72974639402197994, 89.37390960531435269 ) ) ;
#26337=CARTESIAN_POINT ( 'NONE',  ( -0.05219959533936034679, 19.03943276465977164, 87.50109039468567573 ) ) ;
#26338=CARTESIAN_POINT ( 'NONE',  ( 12.06949235617739724, 12.14591786802326823, 46.87609039468568994 ) ) ;
#26340=CARTESIAN_POINT ( 'NONE',  ( 5.719274019375991003, -21.55341960407610458, 92.70724293864770971 ) ) ;
#26341=CARTESIAN_POINT ( 'NONE',  ( 8.314922557960818139, 14.29746914071049879, 79.58224293864769550 ) ) ;
#26343=CARTESIAN_POINT ( 'NONE',  ( -19.05341960407617563, 5.049401038297882671, 113.5427570613523471 ) ) ;
#26344=CARTESIAN_POINT ( 'NONE',  ( -21.52544592524343514, 5.823673210054127303, 41.04057627198103120 ) ) ;
#26345=CARTESIAN_POINT ( 'NONE',  ( -0.05219959533934338120, 16.53943276465976808, 82.50109039468568994 ) ) ;
#26346=CARTESIAN_POINT ( 'NONE',  ( -15.49999999999999822, -5.500000000000000888, 22.00000000000000711 ) ) ;
#26347=CARTESIAN_POINT ( 'NONE',  ( 14.29746914071037800, 8.314922557961029526, 51.66775706135234714 ) ) ;
#26348=CARTESIAN_POINT ( 'NONE',  ( 10.72451020669871369, 18.67979575497193778, 22.08442372801901143 ) ) ;
#26349=CARTESIAN_POINT ( 'NONE',  ( 5.823673210054125526, 21.52544592524343514, 44.79057627198103120 ) ) ;
#26350=CARTESIAN_POINT ( 'NONE',  ( 12.06949235617739724, 12.14591786802326823, 71.87609039468568994 ) ) ;
#26351=CARTESIAN_POINT ( 'NONE',  ( -19.05341960407611168, -5.049401038298163336, 81.45724293864769550 ) ) ;
#26352=CARTESIAN_POINT ( 'NONE',  ( -18.62759615963255300, -10.81492255796106328, 54.16775706135235424 ) ) ;
#26353=CARTESIAN_POINT ( 'NONE',  ( -13.97604488694527625, -13.89961937509977652, 26.87390960531434558 ) ) ;
#26354=CARTESIAN_POINT ( 'NONE',  ( 15.80617190586746368, 15.72974639402197994, 44.37390960531435979 ) ) ;
#26355=CARTESIAN_POINT ( 'NONE',  ( 21.55341960407610458, 5.719274019375980345, 23.95724293864769550 ) ) ;
#26357=CARTESIAN_POINT ( 'NONE',  ( -9.474510206698720793, -16.51473224551083518, 44.58442372801900433 ) ) ;
#26358=CARTESIAN_POINT ( 'NONE',  ( -14.34966873604972548, 8.224510206698743886, 48.33442372801902565 ) ) ;
#26359=CARTESIAN_POINT ( 'NONE',  ( 19.03943276465977164, -0.05219959533909143690, 108.7489096053143527 ) ) ;
#26360=ORIENTED_EDGE ( 'NONE', *, *, #29949, .F. ) ;
#26361=CARTESIAN_POINT ( 'NONE',  ( 5.153800228976335163, 19.02544592524342804, 89.79057627198102409 ) ) ;
#26362=CARTESIAN_POINT ( 'NONE',  ( -8.314922557961024197, 14.29746914071037800, 102.9177570613523756 ) ) ;
#26364=CARTESIAN_POINT ( 'NONE',  ( 14.34966873604960469, 8.224510206698951720, 89.16557627198102409 ) ) ;
#26365=CARTESIAN_POINT ( 'NONE',  ( 15.80617190586746368, 15.72974639402197994, 44.37390960531435979 ) ) ;
#26366=CARTESIAN_POINT ( 'NONE',  ( -9.564922557960796823, -16.46253265017161027, 32.08224293864769550 ) ) ;
#26367=CARTESIAN_POINT ( 'NONE',  ( -0.05219959533934338120, 16.53943276465976808, 72.50109039468568994 ) ) ;
#26368=CARTESIAN_POINT ( 'NONE',  ( -10.81492255796105439, 18.62759615963255655, 22.91775706135235069 ) ) ;
#26369=CARTESIAN_POINT ( 'NONE',  ( -5.153800228976607833, 19.02544592524334988, 77.70942372801900433 ) ) ;
#26370=CARTESIAN_POINT ( 'NONE',  ( -9.474510206698964154, 16.51473224551069663, 35.41557627198102409 ) ) ;
#26371=CARTESIAN_POINT ( 'NONE',  ( 9.564922557960805705, 16.46253265017160317, 114.5822429386476955 ) ) ;
#26372=CARTESIAN_POINT ( 'NONE',  ( 18.62759615963255655, 10.81492255796105972, 111.6677570613523613 ) ) ;
#26373=CARTESIAN_POINT ( 'NONE',  ( -19.03943276465977164, 0.05219959533909376836, 71.24890960531435269 ) ) ;
#26374=EDGE_CURVE ( 'NONE', #133811, #144727, #93622, .T. ) ;
#26375=CARTESIAN_POINT ( 'NONE',  ( -16.53943276465976808, -0.05219959533934237506, 53.75109039468568994 ) ) ;
#26376=CARTESIAN_POINT ( 'NONE',  ( 18.67979575497194134, -10.72451020669871369, 95.83442372801903275 ) ) ;
#26377=CARTESIAN_POINT ( 'NONE',  ( -13.97604488694547697, 13.89961937509957934, 48.12609039468566863 ) ) ;
#26378=CARTESIAN_POINT ( 'NONE',  ( 19.02544592524334988, 5.153800228976608722, 51.45942372801900433 ) ) ;
#26380=CARTESIAN_POINT ( 'NONE',  ( -18.67979575497193778, 10.72451020669871902, 48.33442372801902565 ) ) ;
#26382=CARTESIAN_POINT ( 'NONE',  ( 16.51473224551083163, -9.474510206698727899, 45.83442372801900433 ) ) ;
#26383=CARTESIAN_POINT ( 'NONE',  ( 5.049401038298161559, -19.05341960407611168, 97.70724293864766707 ) ) ;
#26384=CARTESIAN_POINT ( 'NONE',  ( 0.05219959533909260263, 19.03943276465977164, 79.99890960531436690 ) ) ;
#26385=CARTESIAN_POINT ( 'NONE',  ( 8.224510206698953496, -14.34966873604960469, 42.91557627198103120 ) ) ;
#26386=CARTESIAN_POINT ( 'NONE',  ( -5.823673210054116645, -21.52544592524344225, 32.29057627198102409 ) ) ;
#26389=CARTESIAN_POINT ( 'NONE',  ( -18.62759615963255300, -10.81492255796106328, 109.1677570613523613 ) ) ;
#26391=CARTESIAN_POINT ( 'NONE',  ( 5.153800228976335163, 19.02544592524342804, 34.79057627198102409 ) ) ;
#26392=CARTESIAN_POINT ( 'NONE',  ( 9.474510206698971260, -16.51473224551069308, 22.91557627198102765 ) ) ;
#26395=CARTESIAN_POINT ( 'NONE',  ( -16.52544592524335698, -4.483927247898792601, 63.95942372801901854 ) ) ;
#26396=CARTESIAN_POINT ( 'NONE',  ( 21.53943276465977519, -0.05219959533907433946, 83.74890960531435269 ) ) ;
#26397=CARTESIAN_POINT ( 'NONE',  ( 14.34966873604960469, 8.224510206698951720, 54.16557627198103120 ) ) ;
#26398=CARTESIAN_POINT ( 'NONE',  ( 9.474510206698971260, -16.51473224551069308, 32.91557627198102409 ) ) ;
#26399=CARTESIAN_POINT ( 'NONE',  ( -13.97604488694527625, -13.89961937509977652, 101.8739096053143811 ) ) ;
#26400=CARTESIAN_POINT ( 'NONE',  ( -21.52544592524334988, -5.823673210054445271, 23.95942372801901143 ) ) ;
#26401=CARTESIAN_POINT ( 'NONE',  ( 5.049401038297881783, 19.05341960407617563, 37.29275706135232582 ) ) ;
#26402=CARTESIAN_POINT ( 'NONE',  ( -5.153800228976328057, -19.02544592524343514, 27.29057627198103120 ) ) ;
#26403=CARTESIAN_POINT ( 'NONE',  ( 10.72451020669871369, 18.67979575497193778, 82.08442372801901854 ) ) ;
#26405=CARTESIAN_POINT ( 'NONE',  ( -0.05219959533910754901, -16.53943276465976808, 22.49890960531436335 ) ) ;
#26407=CARTESIAN_POINT ( 'NONE',  ( 21.53943276465977519, -0.05219959533907433946, 43.74890960531435979 ) ) ;
#26408=CARTESIAN_POINT ( 'NONE',  ( 4.379528057220339221, -16.55341960407611168, 102.7072429386476955 ) ) ;
#26409=DIRECTION ( 'NONE',  ( 0.000000000000000000, 0.000000000000000000, -1.000000000000000000 ) ) ;
#26410=CARTESIAN_POINT ( 'NONE',  ( -5.153800228976328057, -19.02544592524343514, 92.29057627198099567 ) ) ;
#26411=CARTESIAN_POINT ( 'NONE',  ( 16.53943276465976808, -0.05219959533910856209, 93.74890960531436690 ) ) ;
#26412=CARTESIAN_POINT ( 'NONE',  ( 16.51473224551083163, -9.474510206698727899, 110.8344237280190043 ) ) ;
#26413=CARTESIAN_POINT ( 'NONE',  ( 21.55341960407610458, 5.719274019375980345, 58.95724293864770971 ) ) ;
#26415=CARTESIAN_POINT ( 'NONE',  ( 5.153800228976335163, 19.02544592524342804, 34.79057627198102409 ) ) ;
#26416=CARTESIAN_POINT ( 'NONE',  ( 5.153800228976335163, 19.02544592524342804, 89.79057627198102409 ) ) ;
#26417=CARTESIAN_POINT ( 'NONE',  ( -21.55341960407610458, -5.719274019375992779, 91.45724293864769550 ) ) ;
#26418=CARTESIAN_POINT ( 'NONE',  ( -14.29746914071037622, -8.314922557961029526, 104.1677570613523471 ) ) ;
#26419=CARTESIAN_POINT ( 'NONE',  ( -19.03943276465977164, 0.05219959533909376836, 81.24890960531436690 ) ) ;
#26420=CARTESIAN_POINT ( 'NONE',  ( 19.03943276465977164, 0.05219959533936151252, 86.25109039468567573 ) ) ;
#26421=CARTESIAN_POINT ( 'NONE',  ( 5.719274019375673035, 21.55341960407619339, 97.29275706135234714 ) ) ;
#26422=CARTESIAN_POINT ( 'NONE',  ( 10.81492255796078972, 18.62759615963270932, 74.58224293864768129 ) ) ;
#26423=CARTESIAN_POINT ( 'NONE',  ( 18.67979575497178502, 10.72451020669898547, 44.16557627198103120 ) ) ;
#26424=CARTESIAN_POINT ( 'NONE',  ( -19.05341960407611168, -5.049401038298163336, 46.45724293864768129 ) ) ;
#26425=CARTESIAN_POINT ( 'NONE',  ( -8.314922557960811034, -14.29746914071050412, 22.08224293864769194 ) ) ;
#26426=CARTESIAN_POINT ( 'NONE',  ( 19.02544592524343514, -5.153800228976328945, 68.54057627198103830 ) ) ;
#26429=CARTESIAN_POINT ( 'NONE',  ( 19.03943276465977164, 0.05219959533936151252, 26.25109039468566507 ) ) ;
#26430=CARTESIAN_POINT ( 'NONE',  ( -4.379528057220328563, 16.55341960407611168, 75.20724293864769550 ) ) ;
#26431=CARTESIAN_POINT ( 'NONE',  ( -10.81492255796105439, 18.62759615963255655, 22.91775706135235069 ) ) ;
#26433=CARTESIAN_POINT ( 'NONE',  ( 21.52544592524344225, -5.823673210054117533, 53.54057627198103120 ) ) ;
#26434=CARTESIAN_POINT ( 'NONE',  ( -0.05219959533934338120, 16.53943276465976808, 92.50109039468567573 ) ) ;
#26435=CARTESIAN_POINT ( 'NONE',  ( -8.314922557960811034, -14.29746914071050412, 102.0822429386476955 ) ) ;
#26436=CARTESIAN_POINT ( 'NONE',  ( 13.89961937509977652, -13.97604488694527269, 68.12390960531436690 ) ) ;
#26437=CARTESIAN_POINT ( 'NONE',  ( -4.483927247898539470, -16.52544592524342804, 27.29057627198103120 ) ) ;
#26438=CARTESIAN_POINT ( 'NONE',  ( 21.52544592524334988, 5.823673210054432836, 51.45942372801901854 ) ) ;
#26439=CARTESIAN_POINT ( 'NONE',  ( 5.049401038298161559, -19.05341960407611168, 107.7072429386476955 ) ) ;
#26440=CARTESIAN_POINT ( 'NONE',  ( 10.81492255796106328, -18.62759615963255655, 75.41775706135233293 ) ) ;
#26441=CARTESIAN_POINT ( 'NONE',  ( -5.049401038298153566, 19.05341960407611168, 35.20724293864768839 ) ) ;
#26442=CARTESIAN_POINT ( 'NONE',  ( -16.46253265017160317, 9.564922557960807481, 40.83224293864769550 ) ) ;
#26443=ORIENTED_EDGE ( 'NONE', *, *, #196667, .F. ) ;
#26444=CARTESIAN_POINT ( 'NONE',  ( 21.53943276465977519, 0.05219959533937863772, 101.2510903946856757 ) ) ;
#26445=CARTESIAN_POINT ( 'NONE',  ( 4.483927247898790824, -16.52544592524335698, 45.20942372801901854 ) ) ;
#26446=CARTESIAN_POINT ( 'NONE',  ( 5.719274019375673035, 21.55341960407619339, 77.29275706135234714 ) ) ;
#26447=CARTESIAN_POINT ( 'NONE',  ( -19.03943276465977164, 0.05219959533909376836, 101.2489096053143669 ) ) ;
#26448=CARTESIAN_POINT ( 'NONE',  ( 5.049401038297881783, 19.05341960407617563, 82.29275706135229029 ) ) ;
#26449=CARTESIAN_POINT ( 'NONE',  ( 10.81492255796106328, -18.62759615963255655, 55.41775706135234714 ) ) ;
#26450=CARTESIAN_POINT ( 'NONE',  ( 13.89961937509957401, 13.97604488694547697, 111.8760903946856757 ) ) ;
#26451=CARTESIAN_POINT ( 'NONE',  ( -16.51473224551082808, 9.474510206698731452, 88.33442372801900433 ) ) ;
#26452=CARTESIAN_POINT ( 'NONE',  ( -16.51473224551069308, -9.474510206698971260, 56.66557627198103120 ) ) ;
#26453=CARTESIAN_POINT ( 'NONE',  ( 19.03943276465977164, 0.05219959533936151252, 91.25109039468566152 ) ) ;
#26454=CARTESIAN_POINT ( 'NONE',  ( -4.379528057220328563, 16.55341960407611168, 25.20724293864769550 ) ) ;
#26455=CARTESIAN_POINT ( 'NONE',  ( -9.564922557961040184, 16.46253265017147172, 82.91775706135233293 ) ) ;
#26456=CARTESIAN_POINT ( 'NONE',  ( 4.379528057220339221, -16.55341960407611168, 42.70724293864770260 ) ) ;
#26457=CARTESIAN_POINT ( 'NONE',  ( -19.02544592524334988, -5.153800228976617603, 63.95942372801899012 ) ) ;
#26458=CARTESIAN_POINT ( 'NONE',  ( -0.05219959533934338120, 16.53943276465976808, 52.50109039468567573 ) ) ;
#26459=CARTESIAN_POINT ( 'NONE',  ( -5.049401038297874678, -19.05341960407617918, 24.79275706135233648 ) ) ;
#26460=CARTESIAN_POINT ( 'NONE',  ( -19.03943276465977164, 0.05219959533909376836, 31.24890960531435979 ) ) ;
#26461=CARTESIAN_POINT ( 'NONE',  ( -16.46253265017160317, 9.564922557960807481, 45.83224293864769550 ) ) ;
#26462=CARTESIAN_POINT ( 'NONE',  ( 12.14591786802327356, -12.06949235617739191, 40.62609039468567573 ) ) ;
#26464=EDGE_CURVE ( 'NONE', #78021, #111651, #28434, .T. ) ;
#26467=CARTESIAN_POINT ( 'NONE',  ( -19.05341960407611168, -5.049401038298163336, 96.45724293864769550 ) ) ;
#26468=CARTESIAN_POINT ( 'NONE',  ( 17.78954161113924926, -0.5375896797866550614, 102.5000000000000284 ) ) ;
#26469=ORIENTED_EDGE ( 'NONE', *, *, #135545, .F. ) ;
#26470=CARTESIAN_POINT ( 'NONE',  ( -19.02544592524334988, -5.153800228976617603, 93.95942372801900433 ) ) ;
#26471=CARTESIAN_POINT ( 'NONE',  ( 10.81492255796078972, 18.62759615963270932, 29.58224293864769905 ) ) ;
#26472=CARTESIAN_POINT ( 'NONE',  ( -0.05219959533936034679, 19.03943276465977164, 32.50109039468566863 ) ) ;
#26473=CARTESIAN_POINT ( 'NONE',  ( -13.97604488694547697, 13.89961937509957934, 108.1260903946856331 ) ) ;
#26474=CARTESIAN_POINT ( 'NONE',  ( -8.224510206698948167, 14.34966873604960824, 105.4155762719810383 ) ) ;
#26475=CARTESIAN_POINT ( 'NONE',  ( 13.97604488694527802, 13.89961937509977652, 34.37390960531436690 ) ) ;
#26476=CARTESIAN_POINT ( 'NONE',  ( 18.67979575497178502, 10.72451020669898547, 74.16557627198102409 ) ) ;
#26477=CARTESIAN_POINT ( 'NONE',  ( -13.97604488694527625, -13.89961937509977652, 41.87390960531435979 ) ) ;
#26479=CARTESIAN_POINT ( 'NONE',  ( 9.564922557961047289, -16.46253265017146816, 75.41775706135234714 ) ) ;
#26480=CARTESIAN_POINT ( 'NONE',  ( -0.05219959533910754901, -16.53943276465976808, 52.49890960531435979 ) ) ;
#26481=CARTESIAN_POINT ( 'NONE',  ( 15.72974639402199770, -15.80617190586745480, 38.12390960531436690 ) ) ;
#26482=CARTESIAN_POINT ( 'NONE',  ( -10.81492255796105439, 18.62759615963255655, 92.91775706135236135 ) ) ;
#26483=CARTESIAN_POINT ( 'NONE',  ( 10.81492255796078972, 18.62759615963270932, 89.58224293864768129 ) ) ;
#26484=CARTESIAN_POINT ( 'NONE',  ( -5.823673210054431948, 21.52544592524334988, 77.70942372801900433 ) ) ;
#26485=CARTESIAN_POINT ( 'NONE',  ( 21.55341960407619695, -5.719274019375665929, 66.04275706135236135 ) ) ;
#26486=CARTESIAN_POINT ( 'NONE',  ( 16.51473224551069308, 9.474510206698969483, 99.16557627198102409 ) ) ;
#26487=CARTESIAN_POINT ( 'NONE',  ( 14.29746914071037800, 8.314922557961029526, 96.66775706135234714 ) ) ;
#26488=CARTESIAN_POINT ( 'NONE',  ( 18.67979575497194134, -10.72451020669871369, 65.83442372801900433 ) ) ;
#26489=CARTESIAN_POINT ( 'NONE',  ( -19.02544592524342804, 5.153800228976336051, 56.04057627198100988 ) ) ;
#26490=CARTESIAN_POINT ( 'NONE',  ( -18.62759615963255300, -10.81492255796106328, 34.16775706135234714 ) ) ;
#26491=CARTESIAN_POINT ( 'NONE',  ( 0.05219959533909260263, 19.03943276465977164, 64.99890960531436690 ) ) ;
#26492=CARTESIAN_POINT ( 'NONE',  ( 14.34966873604960469, 8.224510206698951720, 69.16557627198102409 ) ) ;
#26493=CARTESIAN_POINT ( 'NONE',  ( 12.14591786802309770, 12.06949235617756955, 49.37390960531436690 ) ) ;
#26494=CARTESIAN_POINT ( 'NONE',  ( -10.81492255796078084, -18.62759615963271287, 62.08224293864769550 ) ) ;
#26495=CARTESIAN_POINT ( 'NONE',  ( 16.46253265017160672, -9.564922557960803928, 48.33224293864769550 ) ) ;
#26496=CARTESIAN_POINT ( 'NONE',  ( 15.80617190586746368, 15.72974639402197994, 54.37390960531435979 ) ) ;
#26497=CARTESIAN_POINT ( 'NONE',  ( 5.049401038297881783, 19.05341960407617563, 47.29275706135231161 ) ) ;
#26499=CARTESIAN_POINT ( 'NONE',  ( -14.29746914071049879, 8.314922557960819915, 65.83224293864769550 ) ) ;
#26500=CARTESIAN_POINT ( 'NONE',  ( 18.67979575497178502, 10.72451020669898547, 34.16557627198102409 ) ) ;
#26501=EDGE_LOOP ( 'NONE', ( #164706, #72706, #61298, #54216, #97504, #26469, #19584, #54993 ) ) ;
#26502=CARTESIAN_POINT ( 'NONE',  ( 17.31747979337948351, 6.344076630961057894, 103.8794486806518478 ) ) ;
#26503=CARTESIAN_POINT ( 'NONE',  ( 16.53943276465976808, 0.05219959533934440121, 91.25109039468568994 ) ) ;
#26504=CARTESIAN_POINT ( 'NONE',  ( -19.03943276465977164, -0.05219959533935918106, 83.75109039468567573 ) ) ;
#26505=CARTESIAN_POINT ( 'NONE',  ( 14.29746914071049879, -8.314922557960816363, 53.33224293864769550 ) ) ;
#26507=CARTESIAN_POINT ( 'NONE',  ( -19.03943276465977164, 0.05219959533909376836, 46.24890960531435979 ) ) ;
#26508=CARTESIAN_POINT ( 'NONE',  ( 14.34966873604960469, 8.224510206698951720, 39.16557627198102409 ) ) ;
#26509=CARTESIAN_POINT ( 'NONE',  ( 9.474510206698971260, -16.51473224551069308, 72.91557627198102409 ) ) ;
#26510=CARTESIAN_POINT ( 'NONE',  ( -19.03943276465977164, 0.05219959533909376836, 46.24890960531435979 ) ) ;
#26511=CARTESIAN_POINT ( 'NONE',  ( 21.55341960407619695, -5.719274019375665929, 61.04275706135234714 ) ) ;
#26512=CARTESIAN_POINT ( 'NONE',  ( -16.51473224551069308, -9.474510206698971260, 76.66557627198103830 ) ) ;
#26513=CARTESIAN_POINT ( 'NONE',  ( 5.049401038298161559, -19.05341960407611168, 32.70724293864768129 ) ) ;
#26514=CARTESIAN_POINT ( 'NONE',  ( 5.049401038298161559, -19.05341960407611168, 57.70724293864769550 ) ) ;
#26515=CARTESIAN_POINT ( 'NONE',  ( -10.72451020669898014, 18.67979575497178502, 55.41557627198102409 ) ) ;
#26516=CARTESIAN_POINT ( 'NONE',  ( -19.03943276465977164, 0.05219959533909376836, 41.24890960531435269 ) ) ;
#26517=CARTESIAN_POINT ( 'NONE',  ( 21.52544592524344225, -5.823673210054117533, 38.54057627198103120 ) ) ;
#26518=CARTESIAN_POINT ( 'NONE',  ( 14.34966873604972726, -8.224510206698740333, 105.8344237280190328 ) ) ;
#26519=CARTESIAN_POINT ( 'NONE',  ( -0.05219959533937732626, 21.53943276465977519, 112.5010903946857042 ) ) ;
#26520=CARTESIAN_POINT ( 'NONE',  ( 12.06949235617739724, 12.14591786802326823, 46.87609039468568994 ) ) ;
#26521=CARTESIAN_POINT ( 'NONE',  ( 0.05219959533934541429, -16.53943276465976808, 85.00109039468568994 ) ) ;
#26522=CARTESIAN_POINT ( 'NONE',  ( 30.00000000000000000, -5.510910596163089556E-15, 45.00000000000000000 ) ) ;
#26523=CARTESIAN_POINT ( 'NONE',  ( -16.52544592524335698, -4.483927247898792601, 73.95942372801901854 ) ) ;
#26524=CARTESIAN_POINT ( 'NONE',  ( -12.14591786802326823, 12.06949235617739902, 58.12609039468568994 ) ) ;
#26525=CARTESIAN_POINT ( 'NONE',  ( -19.03943276465977164, 0.05219959533909376836, 111.2489096053143669 ) ) ;
#26526=CARTESIAN_POINT ( 'NONE',  ( 16.51473224551069308, 9.474510206698969483, 29.16557627198103475 ) ) ;
#26527=CARTESIAN_POINT ( 'NONE',  ( -12.06949235617739369, -12.14591786802326823, 44.37609039468567573 ) ) ;
#26528=CARTESIAN_POINT ( 'NONE',  ( -16.46253265017160317, 9.564922557960807481, 35.83224293864768839 ) ) ;
#26529=CARTESIAN_POINT ( 'NONE',  ( -5.719274019375665041, -21.55341960407619695, 29.79275706135234358 ) ) ;
#26530=CARTESIAN_POINT ( 'NONE',  ( 12.06949235617739724, 12.14591786802326823, 36.87609039468568994 ) ) ;
#26531=CARTESIAN_POINT ( 'NONE',  ( 4.483927247898790824, -16.52544592524335698, 95.20942372801903275 ) ) ;
#26533=CARTESIAN_POINT ( 'NONE',  ( 10.72451020669871369, 18.67979575497193778, 107.0844237280190043 ) ) ;
#26534=CARTESIAN_POINT ( 'NONE',  ( -13.97604488694547697, 13.89961937509957934, 98.12609039468566152 ) ) ;
#26535=CARTESIAN_POINT ( 'NONE',  ( 4.483927247898545687, 16.52544592524342804, 54.79057627198104541 ) ) ;
#26536=CARTESIAN_POINT ( 'NONE',  ( -13.97604488694527625, -13.89961937509977652, 26.87390960531434558 ) ) ;
#26537=CARTESIAN_POINT ( 'NONE',  ( -16.46253265017146816, -9.564922557961047289, 64.16775706135233293 ) ) ;
#26538=CARTESIAN_POINT ( 'NONE',  ( 16.88567814943162304, 6.947325034625711382, 78.79001122652589117 ) ) ;
#26539=CARTESIAN_POINT ( 'NONE',  ( 10.72451020669871369, 18.67979575497193778, 67.08442372801901854 ) ) ;
#26540=CARTESIAN_POINT ( 'NONE',  ( -0.05219959533934338120, 16.53943276465976808, 22.50109039468567573 ) ) ;
#26541=CARTESIAN_POINT ( 'NONE',  ( 16.29526858892874230, 7.335722546920140807, 83.29670597800203780 ) ) ;
#26542=CARTESIAN_POINT ( 'NONE',  ( 9.564922557960805705, 16.46253265017160317, 114.5822429386476955 ) ) ;
#26543=CARTESIAN_POINT ( 'NONE',  ( 5.049401038297881783, 19.05341960407617563, 107.2927570613523187 ) ) ;
#26546=CARTESIAN_POINT ( 'NONE',  ( 13.97604488694527802, 13.89961937509977652, 29.37390960531435979 ) ) ;
#26547=CARTESIAN_POINT ( 'NONE',  ( 21.53943276465977519, 0.05219959533937863772, 101.2510903946856757 ) ) ;
#26548=CARTESIAN_POINT ( 'NONE',  ( 9.474510206698971260, -16.51473224551069308, 47.91557627198102409 ) ) ;
#26549=CARTESIAN_POINT ( 'NONE',  ( -10.81492255796105439, 18.62759615963255655, 52.91775706135235424 ) ) ;
#26550=CARTESIAN_POINT ( 'NONE',  ( -10.72451020669870658, -18.67979575497194134, 99.58442372801900433 ) ) ;
#26551=CARTESIAN_POINT ( 'NONE',  ( -0.05219959533934338120, 16.53943276465976808, 97.50109039468567573 ) ) ;
#26552=EDGE_CURVE ( 'NONE', #26208, #112608, #131887, .T. ) ;
#26553=CARTESIAN_POINT ( 'NONE',  ( 13.89961937509977652, -13.97604488694527269, 78.12390960531433848 ) ) ;
#26554=CARTESIAN_POINT ( 'NONE',  ( 21.53943276465977519, 0.05219959533937863772, 41.25109039468568284 ) ) ;
#26555=CARTESIAN_POINT ( 'NONE',  ( -10.81492255796105439, 18.62759615963255655, 52.91775706135235424 ) ) ;
#26556=CARTESIAN_POINT ( 'NONE',  ( 5.049401038297881783, 19.05341960407617563, 82.29275706135229029 ) ) ;
#26557=CARTESIAN_POINT ( 'NONE',  ( 19.05341960407611168, 5.049401038298154454, 93.95724293864769550 ) ) ;
#26558=CARTESIAN_POINT ( 'NONE',  ( 19.02544592524343514, -5.153800228976328945, 23.54057627198102054 ) ) ;
#26559=CARTESIAN_POINT ( 'NONE',  ( 5.823673210054125526, 21.52544592524343514, 99.79057627198103830 ) ) ;
#26560=CARTESIAN_POINT ( 'NONE',  ( 19.03943276465977164, 0.05219959533936151252, 26.25109039468566507 ) ) ;
#26561=CARTESIAN_POINT ( 'NONE',  ( 8.224510206698953496, -14.34966873604960469, 102.9155762719810383 ) ) ;
#26562=CARTESIAN_POINT ( 'NONE',  ( 9.474510206698971260, -16.51473224551069308, 47.91557627198102409 ) ) ;
#26563=CARTESIAN_POINT ( 'NONE',  ( -16.51473224551082808, 9.474510206698731452, 78.33442372801900433 ) ) ;
#26564=CARTESIAN_POINT ( 'NONE',  ( -12.06949235617756955, 12.14591786802309770, 45.62390960531436690 ) ) ;
#26565=CARTESIAN_POINT ( 'NONE',  ( -15.72974639402176322, -15.80617190586768395, 104.3760903946856899 ) ) ;
#26566=CARTESIAN_POINT ( 'NONE',  ( 13.89961937509977652, -13.97604488694527269, 103.1239096053143527 ) ) ;
#26567=CARTESIAN_POINT ( 'NONE',  ( -5.049401038297874678, -19.05341960407617918, 69.79275706135233293 ) ) ;
#26568=CARTESIAN_POINT ( 'NONE',  ( -0.05219959533907301413, -21.53943276465977519, 72.49890960531435269 ) ) ;
#26569=CARTESIAN_POINT ( 'NONE',  ( 10.81492255796106328, -18.62759615963255655, 30.41775706135234358 ) ) ;
#26570=CARTESIAN_POINT ( 'NONE',  ( 14.34966873604972726, -8.224510206698740333, 35.83442372801901143 ) ) ;
#26571=CARTESIAN_POINT ( 'NONE',  ( -16.55341960407617563, 4.379528057220093196, 98.54275706135234714 ) ) ;
#26572=CARTESIAN_POINT ( 'NONE',  ( -13.97604488694527625, -13.89961937509977652, 26.87390960531434558 ) ) ;
#26573=CARTESIAN_POINT ( 'NONE',  ( 5.719274019375673035, 21.55341960407619339, 37.29275706135235424 ) ) ;
#26574=CARTESIAN_POINT ( 'NONE',  ( 21.53943276465977519, -0.05219959533907433946, 38.74890960531435979 ) ) ;
#26575=CARTESIAN_POINT ( 'NONE',  ( 13.89961937509977652, -13.97604488694527269, 23.12390960531436335 ) ) ;
#26577=CARTESIAN_POINT ( 'NONE',  ( 14.34966873604972726, -8.224510206698740333, 60.83442372801901854 ) ) ;
#26578=CARTESIAN_POINT ( 'NONE',  ( 4.483927247898545687, 16.52544592524342804, 94.79057627198105251 ) ) ;
#26579=CARTESIAN_POINT ( 'NONE',  ( 10.81492255796078972, 18.62759615963270932, 84.58224293864769550 ) ) ;
#26580=CARTESIAN_POINT ( 'NONE',  ( -0.05219959533934338120, 16.53943276465976808, 112.5010903946857042 ) ) ;
#26581=CARTESIAN_POINT ( 'NONE',  ( -14.29746914071037622, -8.314922557961029526, 49.16775706135234003 ) ) ;
#26582=CARTESIAN_POINT ( 'NONE',  ( -9.474510206698964154, 16.51473224551069663, 60.41557627198102409 ) ) ;
#26583=CARTESIAN_POINT ( 'NONE',  ( -0.05219959533934338120, 16.53943276465976808, 87.50109039468568994 ) ) ;
#26584=CARTESIAN_POINT ( 'NONE',  ( 19.02544592524334988, 5.153800228976608722, 91.45942372801900433 ) ) ;
#26585=CARTESIAN_POINT ( 'NONE',  ( 5.719274019375991003, -21.55341960407610458, 82.70724293864770971 ) ) ;
#26586=CARTESIAN_POINT ( 'NONE',  ( -8.314922557960811034, -14.29746914071050412, 22.08224293864769194 ) ) ;
#26588=CARTESIAN_POINT ( 'NONE',  ( -19.03943276465977164, 0.05219959533909376836, 116.2489096053143669 ) ) ;
#26589=CARTESIAN_POINT ( 'NONE',  ( -21.53943276465977519, 0.05219959533907696930, 61.24890960531435979 ) ) ;
#26590=CARTESIAN_POINT ( 'NONE',  ( 16.53943276465976808, 0.05219959533934440121, 91.25109039468568994 ) ) ;
#26591=ORIENTED_EDGE ( 'NONE', *, *, #57096, .F. ) ;
#26592=CARTESIAN_POINT ( 'NONE',  ( 18.67979575497178502, 10.72451020669898547, 29.16557627198103120 ) ) ;
#26594=CARTESIAN_POINT ( 'NONE',  ( 15.72974639402199770, -15.80617190586745480, 88.12390960531436690 ) ) ;
#26595=CARTESIAN_POINT ( 'NONE',  ( -16.55341960407611168, -4.379528057220339221, 26.45724293864768839 ) ) ;
#26596=CARTESIAN_POINT ( 'NONE',  ( 16.53943276465976808, 0.05219959533934440121, 41.25109039468568284 ) ) ;
#26597=CARTESIAN_POINT ( 'NONE',  ( 19.02544592524343514, -5.153800228976328945, 38.54057627198103120 ) ) ;
#26598=CARTESIAN_POINT ( 'NONE',  ( 4.483927247898790824, -16.52544592524335698, 30.20942372801902565 ) ) ;
#26599=CARTESIAN_POINT ( 'NONE',  ( 16.46253265017160672, -9.564922557960803928, 48.33224293864769550 ) ) ;
#26601=CARTESIAN_POINT ( 'NONE',  ( 19.05341960407611168, 5.049401038298154454, 108.9572429386477097 ) ) ;
#26603=CARTESIAN_POINT ( 'NONE',  ( -14.34966873604972548, 8.224510206698743886, 103.3344237280190043 ) ) ;
#26604=CARTESIAN_POINT ( 'NONE',  ( 9.474510206698729675, 16.51473224551082808, 92.08442372801900433 ) ) ;
#26605=CARTESIAN_POINT ( 'NONE',  ( -9.474510206698720793, -16.51473224551083518, 39.58442372801899722 ) ) ;
#26606=CARTESIAN_POINT ( 'NONE',  ( -21.52544592524343514, 5.823673210054127303, 76.04057627198102409 ) ) ;
#26607=CARTESIAN_POINT ( 'NONE',  ( -8.314922557961024197, 14.29746914071037800, 102.9177570613523756 ) ) ;
#26608=CARTESIAN_POINT ( 'NONE',  ( 21.53943276465977519, -0.05219959533907433946, 38.74890960531435979 ) ) ;
#26609=CARTESIAN_POINT ( 'NONE',  ( -13.97604488694547697, 13.89961937509957934, 113.1260903946856757 ) ) ;
#26610=CARTESIAN_POINT ( 'NONE',  ( 13.89961937509977652, -13.97604488694527269, 108.1239096053143669 ) ) ;
#26611=CARTESIAN_POINT ( 'NONE',  ( 5.719274019375673035, 21.55341960407619339, 57.29275706135234714 ) ) ;
#26612=CARTESIAN_POINT ( 'NONE',  ( -9.474510206698964154, 16.51473224551069663, 60.41557627198102409 ) ) ;
#26613=CARTESIAN_POINT ( 'NONE',  ( 4.483927247898545687, 16.52544592524342804, 94.79057627198105251 ) ) ;
#26614=CARTESIAN_POINT ( 'NONE',  ( -17.44279575226824264, -5.990770900252441855, 84.16442432485685288 ) ) ;
#26615=CARTESIAN_POINT ( 'NONE',  ( 8.224510206698953496, -14.34966873604960469, 72.91557627198103830 ) ) ;
#26616=CARTESIAN_POINT ( 'NONE',  ( 0.05219959533907565091, 21.53943276465977519, 74.99890960531435269 ) ) ;
#26618=CARTESIAN_POINT ( 'NONE',  ( 9.474510206698729675, 16.51473224551082808, 97.08442372801900433 ) ) ;
#26620=CARTESIAN_POINT ( 'NONE',  ( 0.05219959533909260263, 19.03943276465977164, 59.99890960531436690 ) ) ;
#26621=CARTESIAN_POINT ( 'NONE',  ( 17.05116617787848554, -6.768360034955527738, 71.15675553259190167 ) ) ;
#26622=CARTESIAN_POINT ( 'NONE',  ( -19.03943276465977164, 0.05219959533909376836, 76.24890960531435269 ) ) ;
#26623=CARTESIAN_POINT ( 'NONE',  ( 0.05219959533909260263, 19.03943276465977164, 89.99890960531436690 ) ) ;
#26624=CARTESIAN_POINT ( 'NONE',  ( -8.224510206698735004, -14.34966873604973081, 69.58442372801900433 ) ) ;
#26626=CARTESIAN_POINT ( 'NONE',  ( -16.51473224551082808, 9.474510206698731452, 43.33442372801900433 ) ) ;
#26628=CARTESIAN_POINT ( 'NONE',  ( -16.51473224551069308, -9.474510206698971260, 111.6655762719810383 ) ) ;
#26629=CARTESIAN_POINT ( 'NONE',  ( 16.53943276465976808, 0.05219959533934440121, 106.2510903946856757 ) ) ;
#26631=CARTESIAN_POINT ( 'NONE',  ( -16.55341960407617563, 4.379528057220093196, 93.54275706135234714 ) ) ;
#26632=CARTESIAN_POINT ( 'NONE',  ( -16.36317988757059894, 7.306389748694930297, 29.09789608363226066 ) ) ;
#26633=CARTESIAN_POINT ( 'NONE',  ( 16.53943276465976808, 0.05219959533934440121, 66.25109039468567573 ) ) ;
#26635=CARTESIAN_POINT ( 'NONE',  ( 10.81492255796106328, -18.62759615963255655, 65.41775706135234714 ) ) ;
#26636=CARTESIAN_POINT ( 'NONE',  ( 9.474510206698729675, 16.51473224551082808, 72.08442372801900433 ) ) ;
#26637=CARTESIAN_POINT ( 'NONE',  ( 9.564922557961047289, -16.46253265017146816, 30.41775706135232937 ) ) ;
#26638=CARTESIAN_POINT ( 'NONE',  ( -13.97604488694527625, -13.89961937509977652, 66.87390960531436690 ) ) ;
#26639=CARTESIAN_POINT ( 'NONE',  ( -16.51473224551069308, -9.474510206698971260, 41.66557627198103120 ) ) ;
#26640=CARTESIAN_POINT ( 'NONE',  ( 16.17801625226016782, -7.381721853229580965, 22.13251340186824478 ) ) ;
#26641=CARTESIAN_POINT ( 'NONE',  ( 0.05219959533907565091, 21.53943276465977519, 84.99890960531436690 ) ) ;
#26642=CARTESIAN_POINT ( 'NONE',  ( 21.53943276465977519, -0.05219959533907433946, 38.74890960531435979 ) ) ;
#26643=CARTESIAN_POINT ( 'NONE',  ( -13.97604488694527625, -13.89961937509977652, 36.87390960531436690 ) ) ;
#26644=CARTESIAN_POINT ( 'NONE',  ( 8.314922557961029526, -14.29746914071037800, 50.41775706135235424 ) ) ;
#26645=B_SPLINE_CURVE_WITH_KNOTS ( 'NONE', 3,
 ( #37488, #20317, #158829, #173028, #68822, #126504, #67825, #81965, #96165, #19345, #80993, #130481, #4147, #65826, #189200, #82984, #53659, #129480, #192178, #159831, #23329, #127495 ),
 .UNSPECIFIED., .F., .F.,
 ( 4, 2, 2, 2, 2, 2, 2, 2, 2, 2, 4 ),
 ( 2.024876365526581719E-17, 0.001309639967555213495, 0.001964459951332811569, 0.002291869943221612558, 0.002455574939166013486, 0.002619279935110414414, 0.002782984931054815342, 0.002946689926999216270, 0.003274099918888017692, 0.003928919902665620537, 0.005238559870220827960 ),
 .UNSPECIFIED. ) ;
#26646=ORIENTED_EDGE ( 'NONE', *, *, #153757, .T. ) ;
#26647=CARTESIAN_POINT ( 'NONE',  ( 18.62759615963255655, 10.81492255796105972, 36.66775706135234714 ) ) ;
#26648=CARTESIAN_POINT ( 'NONE',  ( 16.53943276465976808, -0.05219959533910856209, 58.74890960531436690 ) ) ;
#26650=CARTESIAN_POINT ( 'NONE',  ( 12.14591786802327356, -12.06949235617739191, 30.62609039468567929 ) ) ;
#26651=CARTESIAN_POINT ( 'NONE',  ( 16.51473224551083163, -9.474510206698727899, 45.83442372801900433 ) ) ;
#26652=CARTESIAN_POINT ( 'NONE',  ( 16.55341960407611168, 4.379528057220329451, 63.95724293864770260 ) ) ;
#26653=CARTESIAN_POINT ( 'NONE',  ( -21.55341960407610458, -5.719274019375992779, 111.4572429386476813 ) ) ;
#26656=CARTESIAN_POINT ( 'NONE',  ( -10.72451020669898014, 18.67979575497178502, 80.41557627198103830 ) ) ;
#26657=CARTESIAN_POINT ( 'NONE',  ( 5.153800228976335163, 19.02544592524342804, 84.79057627198099567 ) ) ;
#26658=CARTESIAN_POINT ( 'NONE',  ( 4.483927247898545687, 16.52544592524342804, 54.79057627198104541 ) ) ;
#26659=CARTESIAN_POINT ( 'NONE',  ( -19.02544592524342804, 5.153800228976336051, 101.0405762719810241 ) ) ;
#26661=CARTESIAN_POINT ( 'NONE',  ( 16.46253265017146816, 9.564922557961045513, 61.66775706135234003 ) ) ;
#26662=CARTESIAN_POINT ( 'NONE',  ( 15.80617190586746368, 15.72974639402197994, 104.3739096053143669 ) ) ;
#26663=CARTESIAN_POINT ( 'NONE',  ( -19.02544592524342804, 5.153800228976336051, 51.04057627198103120 ) ) ;
#26664=CARTESIAN_POINT ( 'NONE',  ( -9.564922557961040184, 16.46253265017147172, 47.91775706135233293 ) ) ;
#26665=CARTESIAN_POINT ( 'NONE',  ( -16.55341960407611168, -4.379528057220339221, 111.4572429386476813 ) ) ;
#26666=CARTESIAN_POINT ( 'NONE',  ( -18.62759615963255300, -10.81492255796106328, 59.16775706135234714 ) ) ;
#26669=CARTESIAN_POINT ( 'NONE',  ( -0.05219959533910754901, -16.53943276465976808, 47.49890960531435979 ) ) ;
#26670=CARTESIAN_POINT ( 'NONE',  ( 13.89961937509977652, -13.97604488694527269, 53.12390960531434558 ) ) ;
#26671=CARTESIAN_POINT ( 'NONE',  ( 13.89961937509977652, -13.97604488694527269, 113.1239096053143527 ) ) ;
#26672=CARTESIAN_POINT ( 'NONE',  ( 21.53943276465977519, -0.05219959533907433946, 78.74890960531436690 ) ) ;
#26674=CARTESIAN_POINT ( 'NONE',  ( 19.05341960407611168, 5.049401038298154454, 38.95724293864767418 ) ) ;
#26676=CARTESIAN_POINT ( 'NONE',  ( -15.80617190586745835, -15.72974639402198527, 71.87390960531438111 ) ) ;
#26677=CARTESIAN_POINT ( 'NONE',  ( -21.55341960407619339, 5.719274019375674811, 83.54275706135234714 ) ) ;
#26679=CARTESIAN_POINT ( 'NONE',  ( 4.483927247898790824, -16.52544592524335698, 95.20942372801903275 ) ) ;
#26680=CARTESIAN_POINT ( 'NONE',  ( -8.314922557960811034, -14.29746914071050412, 82.08224293864768129 ) ) ;
#26681=CARTESIAN_POINT ( 'NONE',  ( -13.97604488694527625, -13.89961937509977652, 76.87390960531433848 ) ) ;
#26683=CARTESIAN_POINT ( 'NONE',  ( -19.02544592524334988, -5.153800228976617603, 38.95942372801900433 ) ) ;
#26684=CARTESIAN_POINT ( 'NONE',  ( 16.53943276465976808, 0.05219959533934440121, 86.25109039468568994 ) ) ;
#26685=CARTESIAN_POINT ( 'NONE',  ( 16.51473224551083163, -9.474510206698727899, 20.83442372801899722 ) ) ;
#26686=CARTESIAN_POINT ( 'NONE',  ( -9.564922557960796823, -16.46253265017161027, 87.08224293864769550 ) ) ;
#26687=CARTESIAN_POINT ( 'NONE',  ( 10.72451020669898902, -18.67979575497178502, 47.91557627198102409 ) ) ;
#26689=CARTESIAN_POINT ( 'NONE',  ( 18.67979575497194134, -10.72451020669871369, 90.83442372801901854 ) ) ;
#26690=CARTESIAN_POINT ( 'NONE',  ( -8.224510206698735004, -14.34966873604973081, 59.58442372801901854 ) ) ;
#26691=CARTESIAN_POINT ( 'NONE',  ( 15.72974639402199770, -15.80617190586745480, 113.1239096053143953 ) ) ;
#26692=CARTESIAN_POINT ( 'NONE',  ( 14.34966873604972726, -8.224510206698740333, 25.83442372801901499 ) ) ;
#26693=CARTESIAN_POINT ( 'NONE',  ( -13.89961937509977652, 13.97604488694528158, 90.62390960531432427 ) ) ;
#26694=CARTESIAN_POINT ( 'NONE',  ( -5.049401038298153566, 19.05341960407611168, 35.20724293864768839 ) ) ;
#26695=CARTESIAN_POINT ( 'NONE',  ( 19.03943276465977164, -0.05219959533909143690, 48.74890960531435979 ) ) ;
#26696=CARTESIAN_POINT ( 'NONE',  ( -16.53943276465976808, -0.05219959533934237506, 38.75109039468567573 ) ) ;
#26697=CARTESIAN_POINT ( 'NONE',  ( 8.224510206698953496, -14.34966873604960469, 77.91557627198102409 ) ) ;
#26698=CARTESIAN_POINT ( 'NONE',  ( 12.06949235617739724, 12.14591786802326823, 106.8760903946856899 ) ) ;
#26699=CARTESIAN_POINT ( 'NONE',  ( 18.62759615963255655, 10.81492255796105972, 46.66775706135234714 ) ) ;
#26700=CARTESIAN_POINT ( 'NONE',  ( 19.02544592524343514, -5.153800228976328945, 63.54057627198103830 ) ) ;
#26701=CARTESIAN_POINT ( 'NONE',  ( -16.46253265017160317, 9.564922557960807481, 50.83224293864770260 ) ) ;
#26702=CARTESIAN_POINT ( 'NONE',  ( -5.153800228976328057, -19.02544592524343514, 77.29057627198099567 ) ) ;
#26703=CARTESIAN_POINT ( 'NONE',  ( 4.379528057220339221, -16.55341960407611168, 32.70724293864770260 ) ) ;
#26704=CARTESIAN_POINT ( 'NONE',  ( -4.483927247898782831, 16.52544592524335698, 87.70942372801901854 ) ) ;
#26707=CARTESIAN_POINT ( 'NONE',  ( -9.474510206698720793, -16.51473224551083518, 34.58442372801899722 ) ) ;
#26709=CARTESIAN_POINT ( 'NONE',  ( 5.153800228976335163, 19.02544592524342804, 44.79057627198103830 ) ) ;
#26710=CARTESIAN_POINT ( 'NONE',  ( 19.02544592524334988, 5.153800228976608722, 21.45942372801899012 ) ) ;
#26712=CARTESIAN_POINT ( 'NONE',  ( -4.483927247898782831, 16.52544592524335698, 42.70942372801901854 ) ) ;
#26713=CARTESIAN_POINT ( 'NONE',  ( -5.153800228976607833, 19.02544592524334988, 67.70942372801900433 ) ) ;
#26714=CARTESIAN_POINT ( 'NONE',  ( 12.14591786802327356, -12.06949235617739191, 60.62609039468567573 ) ) ;
#26716=CARTESIAN_POINT ( 'NONE',  ( 19.03943276465977164, -0.05219959533909143690, 83.74890960531436690 ) ) ;
#26717=CARTESIAN_POINT ( 'NONE',  ( 18.62759615963271287, -10.81492255796078972, 113.3322429386476955 ) ) ;
#26718=CARTESIAN_POINT ( 'NONE',  ( -13.89961937509957401, -13.97604488694547875, 64.37609039468567573 ) ) ;
#26719=CARTESIAN_POINT ( 'NONE',  ( -9.564922557960796823, -16.46253265017161027, 102.0822429386477097 ) ) ;
#26720=CARTESIAN_POINT ( 'NONE',  ( -0.05219959533909027116, -19.03943276465977164, 37.49890960531436690 ) ) ;
#26721=CARTESIAN_POINT ( 'NONE',  ( -13.89961937509977652, 13.97604488694528158, 80.62390960531436690 ) ) ;
#26722=CARTESIAN_POINT ( 'NONE',  ( 4.379528057220339221, -16.55341960407611168, 32.70724293864770260 ) ) ;
#26723=CARTESIAN_POINT ( 'NONE',  ( -19.03943276465977164, 0.05219959533909376836, 41.24890960531435269 ) ) ;
#26724=CARTESIAN_POINT ( 'NONE',  ( -19.03943276465977164, -0.05219959533935918106, 33.75109039468566863 ) ) ;
#26725=CARTESIAN_POINT ( 'NONE',  ( 4.483927247898545687, 16.52544592524342804, 79.79057627198102409 ) ) ;
#26726=CARTESIAN_POINT ( 'NONE',  ( 21.53943276465977519, 0.05219959533937863772, 111.2510903946856899 ) ) ;
#26727=CARTESIAN_POINT ( 'NONE',  ( 16.46253265017160672, -9.564922557960803928, 58.33224293864769550 ) ) ;
#26728=CARTESIAN_POINT ( 'NONE',  ( -14.34966873604960291, -8.224510206698953496, 56.66557627198103830 ) ) ;
#26729=CARTESIAN_POINT ( 'NONE',  ( 18.67979575497194134, -10.72451020669871369, 105.8344237280190328 ) ) ;
#26730=CARTESIAN_POINT ( 'NONE',  ( 0.05219959533909260263, 19.03943276465977164, 94.99890960531436690 ) ) ;
#26731=CARTESIAN_POINT ( 'NONE',  ( 13.89961937509977652, -13.97604488694527269, 108.1239096053143669 ) ) ;
#26732=CARTESIAN_POINT ( 'NONE',  ( -9.474510206698964154, 16.51473224551069663, 40.41557627198103120 ) ) ;
#26733=CARTESIAN_POINT ( 'NONE',  ( 19.02544592524343514, -5.153800228976328945, 23.54057627198102054 ) ) ;
#26734=CARTESIAN_POINT ( 'NONE',  ( -16.55341960407611168, -4.379528057220339221, 86.45724293864770971 ) ) ;
#26735=CARTESIAN_POINT ( 'NONE',  ( -21.53943276465977519, 0.05219959533907696930, 96.24890960531435269 ) ) ;
#26736=CARTESIAN_POINT ( 'NONE',  ( -16.51473224551069308, -9.474510206698971260, 81.66557627198103830 ) ) ;
#26737=CARTESIAN_POINT ( 'NONE',  ( 21.55341960407610458, 5.719274019375980345, 103.9572429386476813 ) ) ;
#26738=CARTESIAN_POINT ( 'NONE',  ( 9.564922557960805705, 16.46253265017160317, 89.58224293864769550 ) ) ;
#26740=CARTESIAN_POINT ( 'NONE',  ( -0.05219959533910754901, -16.53943276465976808, 102.4989096053143811 ) ) ;
#26741=CARTESIAN_POINT ( 'NONE',  ( 13.89961937509977652, -13.97604488694527269, 73.12390960531436690 ) ) ;
#26742=CARTESIAN_POINT ( 'NONE',  ( -10.72451020669898014, 18.67979575497178502, 85.41557627198102409 ) ) ;
#26745=CARTESIAN_POINT ( 'NONE',  ( -21.53943276465977519, 0.05219959533907696930, 31.24890960531435979 ) ) ;
#26747=CARTESIAN_POINT ( 'NONE',  ( -8.224510206698735004, -14.34966873604973081, 29.58442372801901854 ) ) ;
#26748=CARTESIAN_POINT ( 'NONE',  ( -16.53943276465976808, 0.05219959533911058130, 91.24890960531436690 ) ) ;
#26749=CARTESIAN_POINT ( 'NONE',  ( -17.31728774477273447, -6.344390552232393787, 94.18093348310682700 ) ) ;
#26750=CARTESIAN_POINT ( 'NONE',  ( -19.05341960407611168, -5.049401038298163336, 91.45724293864766707 ) ) ;
#26751=CARTESIAN_POINT ( 'NONE',  ( -5.049401038298153566, 19.05341960407611168, 40.20724293864768839 ) ) ;
#26752=CARTESIAN_POINT ( 'NONE',  ( 8.314922557960818139, 14.29746914071049879, 79.58224293864769550 ) ) ;
#26753=CARTESIAN_POINT ( 'NONE',  ( 5.719274019375991003, -21.55341960407610458, 37.70724293864769550 ) ) ;
#26754=CARTESIAN_POINT ( 'NONE',  ( 12.06949235617757843, -12.14591786802309237, 48.12390960531436690 ) ) ;
#26755=CARTESIAN_POINT ( 'NONE',  ( -19.02544592524334988, -5.153800228976617603, 103.9594237280190043 ) ) ;
#26756=CARTESIAN_POINT ( 'NONE',  ( -18.62759615963255300, -10.81492255796106328, 64.16775706135234714 ) ) ;
#26758=CARTESIAN_POINT ( 'NONE',  ( 19.05341960407611168, 5.049401038298154454, 98.95724293864766707 ) ) ;
#26759=CARTESIAN_POINT ( 'NONE',  ( 14.34966873604972726, -8.224510206698740333, 85.83442372801901854 ) ) ;
#26760=CARTESIAN_POINT ( 'NONE',  ( 13.97604488694527802, 13.89961937509977652, 29.37390960531435979 ) ) ;
#26761=CARTESIAN_POINT ( 'NONE',  ( 19.03943276465977164, -0.05219959533909143690, 73.74890960531435269 ) ) ;
#26762=CARTESIAN_POINT ( 'NONE',  ( 5.823673210054125526, 21.52544592524343514, 74.79057627198105251 ) ) ;
#26763=CARTESIAN_POINT ( 'NONE',  ( -19.03943276465977164, -0.05219959533935918106, 113.7510903946856757 ) ) ;
#26764=CARTESIAN_POINT ( 'NONE',  ( 12.06949235617757843, -12.14591786802309237, 58.12390960531435979 ) ) ;
#26765=CARTESIAN_POINT ( 'NONE',  ( -21.55341960407619339, 5.719274019375674811, 63.54275706135234003 ) ) ;
#26766=CARTESIAN_POINT ( 'NONE',  ( 16.53943276465976808, 0.05219959533934440121, 81.25109039468568994 ) ) ;
#26767=CARTESIAN_POINT ( 'NONE',  ( 5.719274019375991003, -21.55341960407610458, 22.70724293864769194 ) ) ;
#26770=CARTESIAN_POINT ( 'NONE',  ( -16.55341960407617563, 4.379528057220093196, 113.5427570613523756 ) ) ;
#26771=CARTESIAN_POINT ( 'NONE',  ( 8.224510206698742110, 14.34966873604972548, 62.08442372801901143 ) ) ;
#26772=CARTESIAN_POINT ( 'NONE',  ( -9.564922557960796823, -16.46253265017161027, 77.08224293864769550 ) ) ;
#26773=CARTESIAN_POINT ( 'NONE',  ( 16.51473224551069308, 9.474510206698969483, 89.16557627198103830 ) ) ;
#26774=CARTESIAN_POINT ( 'NONE',  ( -18.62759615963255300, -10.81492255796106328, 69.16775706135234714 ) ) ;
#26775=CARTESIAN_POINT ( 'NONE',  ( 16.55341960407618274, -4.379528057220086978, 81.04275706135236135 ) ) ;
#26776=CARTESIAN_POINT ( 'NONE',  ( -8.224510206698948167, 14.34966873604960824, 50.41557627198103120 ) ) ;
#26777=CARTESIAN_POINT ( 'NONE',  ( -19.02544592524342804, 5.153800228976336051, 51.04057627198103120 ) ) ;
#26778=CARTESIAN_POINT ( 'NONE',  ( -13.97604488694527625, -13.89961937509977652, 51.87390960531436690 ) ) ;
#26779=CARTESIAN_POINT ( 'NONE',  ( -16.55341960407617563, 4.379528057220093196, 38.54275706135234714 ) ) ;
#26780=ORIENTED_EDGE ( 'NONE', *, *, #128791, .F. ) ;
#26781=CARTESIAN_POINT ( 'NONE',  ( 19.03943276465977164, 0.05219959533936151252, 101.2510903946856757 ) ) ;
#26782=CARTESIAN_POINT ( 'NONE',  ( -4.483927247898539470, -16.52544592524342804, 102.2905762719810383 ) ) ;
#26783=CARTESIAN_POINT ( 'NONE',  ( -16.46253265017160317, 9.564922557960807481, 65.83224293864769550 ) ) ;
#26784=CARTESIAN_POINT ( 'NONE',  ( -16.51473224551082808, 9.474510206698731452, 98.33442372801900433 ) ) ;
#26786=CARTESIAN_POINT ( 'NONE',  ( -15.80617190586768217, 15.72974639402176855, 103.1260903946856757 ) ) ;
#26787=CARTESIAN_POINT ( 'NONE',  ( 14.29746914071037800, 8.314922557961029526, 71.66775706135234714 ) ) ;
#26789=CARTESIAN_POINT ( 'NONE',  ( 15.72974639402199770, -15.80617190586745480, 63.12390960531435979 ) ) ;
#26790=CARTESIAN_POINT ( 'NONE',  ( 16.52544592524335698, 4.483927247898782831, 51.45942372801901854 ) ) ;
#26792=CARTESIAN_POINT ( 'NONE',  ( -5.153800228976607833, 19.02544592524334988, 57.70942372801899012 ) ) ;
#26793=CARTESIAN_POINT ( 'NONE',  ( -13.97604488694527625, -13.89961937509977652, 96.87390960531433848 ) ) ;
#26794=CARTESIAN_POINT ( 'NONE',  ( 5.049401038298161559, -19.05341960407611168, 27.70724293864769550 ) ) ;
#26795=CARTESIAN_POINT ( 'NONE',  ( 13.97604488694527802, 13.89961937509977652, 59.37390960531434558 ) ) ;
#26796=CARTESIAN_POINT ( 'NONE',  ( 4.379528057220339221, -16.55341960407611168, 52.70724293864769550 ) ) ;
#26797=EDGE_CURVE ( 'NONE', #94779, #9238, #76911, .T. ) ;
#26798=CARTESIAN_POINT ( 'NONE',  ( -18.62759615963255300, -10.81492255796106328, 79.16775706135234714 ) ) ;
#26799=CARTESIAN_POINT ( 'NONE',  ( 16.46253265017146816, 9.564922557961045513, 41.66775706135234003 ) ) ;
#26800=CARTESIAN_POINT ( 'NONE',  ( 16.46253265017146816, 9.564922557961045513, 31.66775706135232937 ) ) ;
#26801=CARTESIAN_POINT ( 'NONE',  ( -5.153800228976328057, -19.02544592524343514, 52.29057627198100988 ) ) ;
#26802=CARTESIAN_POINT ( 'NONE',  ( -16.46253265017160317, 9.564922557960807481, 115.8322429386477097 ) ) ;
#26803=CARTESIAN_POINT ( 'NONE',  ( -10.81492255796105439, 18.62759615963255655, 92.91775706135236135 ) ) ;
#26804=CARTESIAN_POINT ( 'NONE',  ( 19.03943276465977164, -0.05219959533909143690, 68.74890960531436690 ) ) ;
#26806=CARTESIAN_POINT ( 'NONE',  ( -5.719274019375665041, -21.55341960407619695, 89.79275706135236135 ) ) ;
#26807=CARTESIAN_POINT ( 'NONE',  ( 15.72974639402199770, -15.80617190586745480, 43.12390960531435269 ) ) ;
#26808=CARTESIAN_POINT ( 'NONE',  ( 19.05341960407611168, 5.049401038298154454, 78.95724293864769550 ) ) ;
#26809=CARTESIAN_POINT ( 'NONE',  ( 19.03943276465977164, 0.05219959533936151252, 56.25109039468566863 ) ) ;
#26810=CARTESIAN_POINT ( 'NONE',  ( -9.474510206698964154, 16.51473224551069663, 40.41557627198103120 ) ) ;
#26811=CARTESIAN_POINT ( 'NONE',  ( -9.564922557960796823, -16.46253265017161027, 92.08224293864769550 ) ) ;
#26812=CARTESIAN_POINT ( 'NONE',  ( 4.483927247898790824, -16.52544592524335698, 35.20942372801901854 ) ) ;
#26813=CARTESIAN_POINT ( 'NONE',  ( -14.29746914071049879, 8.314922557960819915, 100.8322429386477097 ) ) ;
#26814=CARTESIAN_POINT ( 'NONE',  ( -13.97604488694527625, -13.89961937509977652, 76.87390960531433848 ) ) ;
#26815=CARTESIAN_POINT ( 'NONE',  ( 10.81492255796078972, 18.62759615963270932, 49.58224293864769550 ) ) ;
#26816=CARTESIAN_POINT ( 'NONE',  ( 0.05219959533936267826, -19.03943276465977164, 110.0010903946856757 ) ) ;
#26817=CARTESIAN_POINT ( 'NONE',  ( 18.62759615963271287, -10.81492255796078972, 113.3322429386476955 ) ) ;
#26818=CARTESIAN_POINT ( 'NONE',  ( -5.719274019375665041, -21.55341960407619695, 64.79275706135234714 ) ) ;
#26819=CARTESIAN_POINT ( 'NONE',  ( 4.483927247898790824, -16.52544592524335698, 65.20942372801901854 ) ) ;
#26820=CARTESIAN_POINT ( 'NONE',  ( 9.474510206698971260, -16.51473224551069308, 77.91557627198103830 ) ) ;
#26821=CARTESIAN_POINT ( 'NONE',  ( -16.55341960407617563, 4.379528057220093196, 103.5427570613523613 ) ) ;
#26822=CARTESIAN_POINT ( 'NONE',  ( -19.05341960407617563, 5.049401038297882671, 38.54275706135233293 ) ) ;
#26823=CARTESIAN_POINT ( 'NONE',  ( 0.05219959533937995610, -21.53943276465977519, 35.00109039468568284 ) ) ;
#26824=CARTESIAN_POINT ( 'NONE',  ( 0.05219959533910956823, 16.53943276465976808, 64.99890960531435269 ) ) ;
#26825=CARTESIAN_POINT ( 'NONE',  ( 9.474510206698971260, -16.51473224551069308, 102.9155762719810241 ) ) ;
#26826=CARTESIAN_POINT ( 'NONE',  ( 14.34966873604972726, -8.224510206698740333, 95.83442372801903275 ) ) ;
#26827=CARTESIAN_POINT ( 'NONE',  ( -18.62759615963255300, -10.81492255796106328, 74.16775706135231871 ) ) ;
#26828=CARTESIAN_POINT ( 'NONE',  ( 8.224510206698742110, 14.34966873604972548, 27.08442372801901854 ) ) ;
#26829=CARTESIAN_POINT ( 'NONE',  ( -10.81492255796105439, 18.62759615963255655, 32.91775706135234714 ) ) ;
#26830=CARTESIAN_POINT ( 'NONE',  ( 12.14591786802309770, 12.06949235617756955, 69.37390960531436690 ) ) ;
#26831=EDGE_CURVE ( 'NONE', #69916, #33580, #79901, .T. ) ;
#26832=ORIENTED_EDGE ( 'NONE', *, *, #147658, .F. ) ;
#26833=CARTESIAN_POINT ( 'NONE',  ( -15.72974639402197994, 15.80617190586746368, 100.6239096053143811 ) ) ;
#26834=CARTESIAN_POINT ( 'NONE',  ( 8.224510206698953496, -14.34966873604960469, 47.91557627198102409 ) ) ;
#26836=CARTESIAN_POINT ( 'NONE',  ( -0.05219959533909027116, -19.03943276465977164, 27.49890960531435624 ) ) ;
#26837=CARTESIAN_POINT ( 'NONE',  ( 21.52544592524344225, -5.823673210054117533, 33.54057627198102409 ) ) ;
#26838=CARTESIAN_POINT ( 'NONE',  ( -5.823673210054431948, 21.52544592524334988, 42.70942372801901854 ) ) ;
#26839=CARTESIAN_POINT ( 'NONE',  ( 16.53943276465976808, -0.05219959533910856209, 68.74890960531435269 ) ) ;
#26841=CARTESIAN_POINT ( 'NONE',  ( -5.823673210054116645, -21.52544592524344225, 72.29057627198102409 ) ) ;
#26842=CARTESIAN_POINT ( 'NONE',  ( -16.46253265017160317, 9.564922557960807481, 75.83224293864769550 ) ) ;
#26843=CARTESIAN_POINT ( 'NONE',  ( -19.03943276465977164, 0.05219959533909376836, 26.24890960531435624 ) ) ;
#26844=CARTESIAN_POINT ( 'NONE',  ( 0.05219959533936267826, -19.03943276465977164, 80.00109039468567573 ) ) ;
#26845=CARTESIAN_POINT ( 'NONE',  ( -18.67979575497178146, -10.72451020669898902, 51.66557627198102409 ) ) ;
#26846=CARTESIAN_POINT ( 'NONE',  ( 9.474510206698971260, -16.51473224551069308, 42.91557627198103120 ) ) ;
#26847=CARTESIAN_POINT ( 'NONE',  ( -16.46253265017160317, 9.564922557960807481, 75.83224293864769550 ) ) ;
#26848=ORIENTED_EDGE ( 'NONE', *, *, #33627, .F. ) ;
#26849=CARTESIAN_POINT ( 'NONE',  ( -16.55341960407617563, 4.379528057220093196, 38.54275706135234714 ) ) ;
#26850=CARTESIAN_POINT ( 'NONE',  ( 21.53943276465977519, -0.05219959533907433946, 113.7489096053143527 ) ) ;
#26851=CARTESIAN_POINT ( 'NONE',  ( 16.52544592524342804, -4.483927247898539470, 43.54057627198103830 ) ) ;
#26852=CARTESIAN_POINT ( 'NONE',  ( 21.55341960407619695, -5.719274019375665929, 61.04275706135234714 ) ) ;
#26853=CARTESIAN_POINT ( 'NONE',  ( -5.049401038298153566, 19.05341960407611168, 105.2072429386476671 ) ) ;
#26854=CARTESIAN_POINT ( 'NONE',  ( 5.823673210054125526, 21.52544592524343514, 69.79057627198102409 ) ) ;
#26855=CARTESIAN_POINT ( 'NONE',  ( 21.52544592524344225, -5.823673210054117533, 108.5405762719810241 ) ) ;
#26856=CARTESIAN_POINT ( 'NONE',  ( -14.29746914071037622, -8.314922557961029526, 49.16775706135234003 ) ) ;
#26857=CARTESIAN_POINT ( 'NONE',  ( 10.72451020669898902, -18.67979575497178502, 47.91557627198102409 ) ) ;
#26858=CARTESIAN_POINT ( 'NONE',  ( -5.719274019375665041, -21.55341960407619695, 104.7927570613523898 ) ) ;
#26859=CARTESIAN_POINT ( 'NONE',  ( -19.03943276465977164, 0.05219959533909376836, 51.24890960531436690 ) ) ;
#26860=CARTESIAN_POINT ( 'NONE',  ( 5.153800228976335163, 19.02544592524342804, 114.7905762719810241 ) ) ;
#26861=CARTESIAN_POINT ( 'NONE',  ( -13.89961937509977652, 13.97604488694528158, 70.62390960531432427 ) ) ;
#26863=CARTESIAN_POINT ( 'NONE',  ( -19.03943276465977164, -0.05219959533935918106, 63.75109039468566863 ) ) ;
#26864=CARTESIAN_POINT ( 'NONE',  ( -15.80617190586768217, 15.72974639402176855, 113.1260903946856899 ) ) ;
#26865=CARTESIAN_POINT ( 'NONE',  ( -21.55341960407610458, -5.719274019375992779, 26.45724293864768839 ) ) ;
#26866=CARTESIAN_POINT ( 'NONE',  ( -16.55341960407617563, 4.379528057220093196, 108.5427570613523756 ) ) ;
#26867=CARTESIAN_POINT ( 'NONE',  ( 5.153800228976615827, -19.02544592524334988, 90.20942372801900433 ) ) ;
#26868=CARTESIAN_POINT ( 'NONE',  ( -17.48847506799968698, 5.747544572773787053, 60.82697437843280142 ) ) ;
#26869=CARTESIAN_POINT ( 'NONE',  ( -21.55341960407619339, 5.719274019375674811, 113.5427570613523756 ) ) ;
#26870=CARTESIAN_POINT ( 'NONE',  ( -19.05341960407617563, 5.049401038297882671, 83.54275706135233293 ) ) ;
#26871=CARTESIAN_POINT ( 'NONE',  ( -19.03943276465977164, -0.05219959533935918106, 48.75109039468566863 ) ) ;
#26872=CARTESIAN_POINT ( 'NONE',  ( 17.48853670773245028, 5.747243402303108262, 108.8332870025001142 ) ) ;
#26873=CARTESIAN_POINT ( 'NONE',  ( -19.05341960407611168, -5.049401038298163336, 41.45724293864769550 ) ) ;
#26874=CARTESIAN_POINT ( 'NONE',  ( 16.55341960407611168, 4.379528057220329451, 48.95724293864770971 ) ) ;
#26875=CARTESIAN_POINT ( 'NONE',  ( -9.474510206698964154, 16.51473224551069663, 30.41557627198102054 ) ) ;
#26876=CARTESIAN_POINT ( 'NONE',  ( 8.224510206698953496, -14.34966873604960469, 42.91557627198103120 ) ) ;
#26878=CARTESIAN_POINT ( 'NONE',  ( -14.34966873604972548, 8.224510206698743886, 113.3344237280190328 ) ) ;
#26879=CARTESIAN_POINT ( 'NONE',  ( 9.564922557960805705, 16.46253265017160317, 54.58224293864769550 ) ) ;
#26880=CARTESIAN_POINT ( 'NONE',  ( 19.05341960407617918, -5.049401038297876454, 26.04275706135233293 ) ) ;
#26881=CARTESIAN_POINT ( 'NONE',  ( -8.224510206698735004, -14.34966873604973081, 29.58442372801901854 ) ) ;
#26882=CARTESIAN_POINT ( 'NONE',  ( 5.719274019375991003, -21.55341960407610458, 42.70724293864770260 ) ) ;
#26883=CARTESIAN_POINT ( 'NONE',  ( -21.55341960407619339, 5.719274019375674811, 88.54275706135236135 ) ) ;
#26884=ORIENTED_EDGE ( 'NONE', *, *, #197067, .F. ) ;
#26885=CARTESIAN_POINT ( 'NONE',  ( -13.97604488694527625, -13.89961937509977652, 101.8739096053143811 ) ) ;
#26886=CARTESIAN_POINT ( 'NONE',  ( -5.153800228976328057, -19.02544592524343514, 82.29057627198103830 ) ) ;
#26888=CARTESIAN_POINT ( 'NONE',  ( -21.53943276465977519, 0.05219959533907696930, 116.2489096053143669 ) ) ;
#26889=CARTESIAN_POINT ( 'NONE',  ( 14.29746914071049879, -8.314922557960816363, 83.33224293864769550 ) ) ;
#26890=CARTESIAN_POINT ( 'NONE',  ( -18.62759615963270932, 10.81492255796079327, 70.83224293864770971 ) ) ;
#26891=CARTESIAN_POINT ( 'NONE',  ( 0.05219959533909260263, 19.03943276465977164, 74.99890960531435269 ) ) ;
#26892=CARTESIAN_POINT ( 'NONE',  ( 19.02544592524343514, -5.153800228976328945, 78.54057627198099567 ) ) ;
#26893=CARTESIAN_POINT ( 'NONE',  ( -15.80617190586745835, -15.72974639402198527, 96.87390960531436690 ) ) ;
#26895=CARTESIAN_POINT ( 'NONE',  ( 13.97604488694527802, 13.89961937509977652, 54.37390960531435979 ) ) ;
#26896=CARTESIAN_POINT ( 'NONE',  ( 12.14591786802309770, 12.06949235617756955, 94.37390960531436690 ) ) ;
#26897=CARTESIAN_POINT ( 'NONE',  ( -5.153800228976328057, -19.02544592524343514, 22.29057627198102765 ) ) ;
#26898=CARTESIAN_POINT ( 'NONE',  ( 16.46253265017160672, -9.564922557960803928, 58.33224293864769550 ) ) ;
#26899=CARTESIAN_POINT ( 'NONE',  ( 5.049401038297881783, 19.05341960407617563, 77.29275706135231871 ) ) ;
#26900=CARTESIAN_POINT ( 'NONE',  ( -14.34966873604960291, -8.224510206698953496, 101.6655762719810383 ) ) ;
#26901=CARTESIAN_POINT ( 'NONE',  ( -5.823673210054431948, 21.52544592524334988, 52.70942372801902565 ) ) ;
#26902=CARTESIAN_POINT ( 'NONE',  ( 16.51473224551069308, 9.474510206698969483, 49.16557627198102409 ) ) ;
#26903=CARTESIAN_POINT ( 'NONE',  ( 15.80617190586769283, -15.72974639402175789, 20.62609039468568639 ) ) ;
#26904=CARTESIAN_POINT ( 'NONE',  ( 4.379528057220339221, -16.55341960407611168, 102.7072429386476955 ) ) ;
#26906=CARTESIAN_POINT ( 'NONE',  ( -13.97604488694527625, -13.89961937509977652, 56.87390960531434558 ) ) ;
#26908=CARTESIAN_POINT ( 'NONE',  ( -19.03943276465977164, -0.05219959533935918106, 108.7510903946856615 ) ) ;
#26909=CARTESIAN_POINT ( 'NONE',  ( 19.02544592524343514, -5.153800228976328945, 113.5405762719810241 ) ) ;
#26910=CARTESIAN_POINT ( 'NONE',  ( 0.05219959533937995610, -21.53943276465977519, 55.00109039468568284 ) ) ;
#26911=CARTESIAN_POINT ( 'NONE',  ( 5.049401038298161559, -19.05341960407611168, 97.70724293864766707 ) ) ;
#26912=CARTESIAN_POINT ( 'NONE',  ( 19.02544592524334988, 5.153800228976608722, 81.45942372801897591 ) ) ;
#26913=VECTOR ( 'NONE', #29672, 1000.000000000000000 ) ;
#26914=CARTESIAN_POINT ( 'NONE',  ( 13.97604488694527802, 13.89961937509977652, 59.37390960531434558 ) ) ;
#26915=CARTESIAN_POINT ( 'NONE',  ( -8.224510206698948167, 14.34966873604960824, 75.41557627198102409 ) ) ;
#26916=CARTESIAN_POINT ( 'NONE',  ( -0.05219959533909027116, -19.03943276465977164, 107.4989096053143527 ) ) ;
#26917=CARTESIAN_POINT ( 'NONE',  ( 14.29746914071049879, -8.314922557960816363, 78.33224293864770971 ) ) ;
#26918=CARTESIAN_POINT ( 'NONE',  ( 19.02544592524343514, -5.153800228976328945, 78.54057627198099567 ) ) ;
#26919=CARTESIAN_POINT ( 'NONE',  ( 16.51473224551083163, -9.474510206698727899, 45.83442372801900433 ) ) ;
#26920=CARTESIAN_POINT ( 'NONE',  ( -13.89961937509977652, 13.97604488694528158, 55.62390960531434558 ) ) ;
#26921=CARTESIAN_POINT ( 'NONE',  ( -16.53943276465976808, 0.05219959533911058130, 46.24890960531435979 ) ) ;
#26922=( BOUNDED_CURVE ( )  B_SPLINE_CURVE ( 2, ( #39883, #101550, #163242, #24742, #198559, #46855, #105545, #167231, #170193, #122688, #92345, #60029, #43881 ),
 .UNSPECIFIED., .F., .F. ) 
 B_SPLINE_CURVE_WITH_KNOTS ( ( 3, 2, 2, 2, 2, 2, 3 ),
 ( 0.5024761162491353517, 0.5043859649122807154, 0.5087719298245614308, 0.5131578947368421462, 0.5175438596491228616, 0.5219298245614034659, 0.5238853530466391906 ),
 .UNSPECIFIED. ) 
 CURVE ( )  GEOMETRIC_REPRESENTATION_ITEM ( )  RATIONAL_B_SPLINE_CURVE ( ( 0.9832469066685285419, 0.9851625545550100060, 1.000000000000000000, 0.9659258262890683122, 1.000000000000000000, 0.9659258262890683122, 1.000000000000000000, 0.9659258262890683122, 1.000000000000000000, 0.9659258262890683122, 1.000000000000000000, 0.9848076720550078544, 0.9831626618144001517 ) ) 
 REPRESENTATION_ITEM ( '' )  );
#26923=CARTESIAN_POINT ( 'NONE',  ( -16.46253265017160317, 9.564922557960807481, 30.83224293864769550 ) ) ;
#26925=CARTESIAN_POINT ( 'NONE',  ( -21.55341960407619339, 5.719274019375674811, 43.54275706135235424 ) ) ;
#26926=CARTESIAN_POINT ( 'NONE',  ( 19.03943276465977164, 0.05219959533936151252, 81.25109039468567573 ) ) ;
#26927=CARTESIAN_POINT ( 'NONE',  ( 8.314922557960818139, 14.29746914071049879, 39.58224293864769550 ) ) ;
#26928=CARTESIAN_POINT ( 'NONE',  ( -0.05219959533907301413, -21.53943276465977519, 97.49890960531436690 ) ) ;
#26929=CARTESIAN_POINT ( 'NONE',  ( 18.62759615963271287, -10.81492255796078972, 38.33224293864768839 ) ) ;
#26930=CARTESIAN_POINT ( 'NONE',  ( 4.483927247898545687, 16.52544592524342804, 69.79057627198102409 ) ) ;
#26931=CARTESIAN_POINT ( 'NONE',  ( -16.51473224551069308, -9.474510206698971260, 36.66557627198102409 ) ) ;
#26932=CARTESIAN_POINT ( 'NONE',  ( -14.34966873604972548, 8.224510206698743886, 103.3344237280190043 ) ) ;
#26933=CARTESIAN_POINT ( 'NONE',  ( -8.314922557961024197, 14.29746914071037800, 67.91775706135234714 ) ) ;
#26934=CARTESIAN_POINT ( 'NONE',  ( -13.97604488694547697, 13.89961937509957934, 28.12609039468565797 ) ) ;
#26935=CARTESIAN_POINT ( 'NONE',  ( -16.46253265017160317, 9.564922557960807481, 95.83224293864769550 ) ) ;
#26936=CARTESIAN_POINT ( 'NONE',  ( 19.03943276465977164, -0.05219959533909143690, 83.74890960531436690 ) ) ;
#26937=CARTESIAN_POINT ( 'NONE',  ( -16.52544592524335698, -4.483927247898792601, 68.95942372801901854 ) ) ;
#26938=CARTESIAN_POINT ( 'NONE',  ( -16.46253265017160317, 9.564922557960807481, 30.83224293864769550 ) ) ;
#26939=CARTESIAN_POINT ( 'NONE',  ( 12.14591786802309770, 12.06949235617756955, 49.37390960531436690 ) ) ;
#26941=CARTESIAN_POINT ( 'NONE',  ( -16.51473224551069308, -9.474510206698971260, 91.66557627198103830 ) ) ;
#26942=CARTESIAN_POINT ( 'NONE',  ( 5.719274019375991003, -21.55341960407610458, 32.70724293864770260 ) ) ;
#26943=CARTESIAN_POINT ( 'NONE',  ( -0.05219959533910754901, -16.53943276465976808, 72.49890960531435269 ) ) ;
#26946=CARTESIAN_POINT ( 'NONE',  ( -16.52544592524342804, 4.483927247898546575, 61.04057627198103120 ) ) ;
#26947=CARTESIAN_POINT ( 'NONE',  ( -8.224510206698735004, -14.34966873604973081, 54.58442372801901143 ) ) ;
#26948=CARTESIAN_POINT ( 'NONE',  ( 17.50000000000001066, -3.209263204892516264, 32.26196825606286467 ) ) ;
#26949=CARTESIAN_POINT ( 'NONE',  ( 16.51473224551083163, -9.474510206698727899, 65.83442372801900433 ) ) ;
#26950=CARTESIAN_POINT ( 'NONE',  ( 0.05219959533909260263, 19.03943276465977164, 89.99890960531436690 ) ) ;
#26951=CARTESIAN_POINT ( 'NONE',  ( -19.03943276465977164, -0.05219959533935918106, 63.75109039468566863 ) ) ;
#26952=CARTESIAN_POINT ( 'NONE',  ( 17.59860650958994555, -7.585241751806880650, 95.92337014262491834 ) ) ;
#26953=CARTESIAN_POINT ( 'NONE',  ( 12.06949235617739724, 12.14591786802326823, 21.87609039468567573 ) ) ;
#26954=CARTESIAN_POINT ( 'NONE',  ( 12.06949235617739724, 12.14591786802326823, 101.8760903946857042 ) ) ;
#26955=CARTESIAN_POINT ( 'NONE',  ( -5.049401038298153566, 19.05341960407611168, 40.20724293864768839 ) ) ;
#26956=CARTESIAN_POINT ( 'NONE',  ( -19.02544592524342804, 5.153800228976336051, 116.0405762719810383 ) ) ;
#26957=CARTESIAN_POINT ( 'NONE',  ( -18.67979575497193778, 10.72451020669871902, 58.33442372801901143 ) ) ;
#26958=CARTESIAN_POINT ( 'NONE',  ( -8.314922557961024197, 14.29746914071037800, 27.91775706135234358 ) ) ;
#26960=CARTESIAN_POINT ( 'NONE',  ( 19.02544592524343514, -5.153800228976328945, 73.54057627198103830 ) ) ;
#26961=CARTESIAN_POINT ( 'NONE',  ( 16.51473224551069308, 9.474510206698969483, 114.1655762719810241 ) ) ;
#26962=CARTESIAN_POINT ( 'NONE',  ( 0.05219959533910956823, 16.53943276465976808, 79.99890960531435269 ) ) ;
#26963=CARTESIAN_POINT ( 'NONE',  ( 9.474510206698971260, -16.51473224551069308, 77.91557627198103830 ) ) ;
#26964=CARTESIAN_POINT ( 'NONE',  ( -19.03943276465977164, 0.05219959533909376836, 76.24890960531435269 ) ) ;
#26965=CARTESIAN_POINT ( 'NONE',  ( 0.05219959533936267826, -19.03943276465977164, 90.00109039468567573 ) ) ;
#26966=CARTESIAN_POINT ( 'NONE',  ( 15.80617190586746368, 15.72974639402197994, 64.37390960531435269 ) ) ;
#26967=CARTESIAN_POINT ( 'NONE',  ( -13.97604488694527625, -13.89961937509977652, 31.87390960531435979 ) ) ;
#26968=CARTESIAN_POINT ( 'NONE',  ( 16.51473224551083163, -9.474510206698727899, 55.83442372801899722 ) ) ;
#26969=CARTESIAN_POINT ( 'NONE',  ( 9.474510206698971260, -16.51473224551069308, 52.91557627198102409 ) ) ;
#26970=CARTESIAN_POINT ( 'NONE',  ( -13.89961937509977652, 13.97604488694528158, 90.62390960531432427 ) ) ;
#26972=CARTESIAN_POINT ( 'NONE',  ( 10.81492255796078972, 18.62759615963270932, 94.58224293864769550 ) ) ;
#26973=CARTESIAN_POINT ( 'NONE',  ( -14.29746914071049879, 8.314922557960819915, 90.83224293864769550 ) ) ;
#26974=CARTESIAN_POINT ( 'NONE',  ( -19.05341960407617563, 5.049401038297882671, 43.54275706135232582 ) ) ;
#26975=CARTESIAN_POINT ( 'NONE',  ( 0.05219959533907565091, 21.53943276465977519, 79.99890960531435269 ) ) ;
#26976=CARTESIAN_POINT ( 'NONE',  ( 10.81492255796078972, 18.62759615963270932, 64.58224293864769550 ) ) ;
#26977=CARTESIAN_POINT ( 'NONE',  ( 16.55341960407611168, 4.379528057220329451, 28.95724293864769905 ) ) ;
#26978=CARTESIAN_POINT ( 'NONE',  ( -21.52544592524334988, -5.823673210054445271, 103.9594237280190185 ) ) ;
#26979=CARTESIAN_POINT ( 'NONE',  ( 5.153800228976335163, 19.02544592524342804, 79.79057627198102409 ) ) ;
#26980=CARTESIAN_POINT ( 'NONE',  ( 9.474510206698971260, -16.51473224551069308, 37.91557627198102409 ) ) ;
#26981=CARTESIAN_POINT ( 'NONE',  ( -5.719274019375665041, -21.55341960407619695, 34.79275706135235424 ) ) ;
#26982=CARTESIAN_POINT ( 'NONE',  ( -18.62759615963255300, -10.81492255796106328, 49.16775706135234003 ) ) ;
#26983=CARTESIAN_POINT ( 'NONE',  ( 9.474510206698971260, -16.51473224551069308, 52.91557627198102409 ) ) ;
#26984=CARTESIAN_POINT ( 'NONE',  ( -18.67979575497193778, 10.72451020669871902, 28.33442372801902209 ) ) ;
#26985=CARTESIAN_POINT ( 'NONE',  ( -16.51473224551082808, 9.474510206698731452, 63.33442372801900433 ) ) ;
#26986=CARTESIAN_POINT ( 'NONE',  ( -5.153800228976328057, -19.02544592524343514, 32.29057627198102409 ) ) ;
#26987=CARTESIAN_POINT ( 'NONE',  ( 8.314922557961029526, -14.29746914071037800, 30.41775706135234358 ) ) ;
#26988=CARTESIAN_POINT ( 'NONE',  ( -5.153800228976328057, -19.02544592524343514, 27.29057627198103120 ) ) ;
#26989=CARTESIAN_POINT ( 'NONE',  ( -16.52544592524335698, -4.483927247898792601, 78.95942372801901854 ) ) ;
#26990=CARTESIAN_POINT ( 'NONE',  ( 9.474510206698971260, -16.51473224551069308, 42.91557627198103120 ) ) ;
#26992=CARTESIAN_POINT ( 'NONE',  ( 5.049401038298161559, -19.05341960407611168, 82.70724293864770971 ) ) ;
#26993=CARTESIAN_POINT ( 'NONE',  ( -9.474510206698964154, 16.51473224551069663, 25.41557627198103120 ) ) ;
#26994=CARTESIAN_POINT ( 'NONE',  ( -10.72451020669898014, 18.67979575497178502, 70.41557627198102409 ) ) ;
#26995=CARTESIAN_POINT ( 'NONE',  ( 16.52544592524335698, 4.483927247898782831, 46.45942372801901854 ) ) ;
#26996=CARTESIAN_POINT ( 'NONE',  ( 0.05219959533937995610, -21.53943276465977519, 105.0010903946856757 ) ) ;
#26997=CARTESIAN_POINT ( 'NONE',  ( -13.89961937509977652, 13.97604488694528158, 45.62390960531433848 ) ) ;
#26998=CARTESIAN_POINT ( 'NONE',  ( 16.53943276465976808, -0.05219959533910856209, 33.74890960531436690 ) ) ;
#26999=CARTESIAN_POINT ( 'NONE',  ( -8.314922557960811034, -14.29746914071050412, 67.08224293864770971 ) ) ;
#27000=CARTESIAN_POINT ( 'NONE',  ( 13.89961937509977652, -13.97604488694527269, 68.12390960531436690 ) ) ;
#27001=CARTESIAN_POINT ( 'NONE',  ( 0.05219959533937995610, -21.53943276465977519, 105.0010903946856757 ) ) ;
#27002=CARTESIAN_POINT ( 'NONE',  ( -21.53943276465977519, -0.05219959533937600094, 23.75109039468567929 ) ) ;
#27003=CARTESIAN_POINT ( 'NONE',  ( 16.46253265017160672, -9.564922557960803928, 83.33224293864768129 ) ) ;
#27005=CARTESIAN_POINT ( 'NONE',  ( -0.05219959533937732626, 21.53943276465977519, 82.50109039468568994 ) ) ;
#27006=CARTESIAN_POINT ( 'NONE',  ( -8.224510206698735004, -14.34966873604973081, 59.58442372801901854 ) ) ;
#27007=CARTESIAN_POINT ( 'NONE',  ( 16.55341960407618274, -4.379528057220086978, 26.04275706135235779 ) ) ;
#27008=CARTESIAN_POINT ( 'NONE',  ( -12.14591786802309592, -12.06949235617757132, 96.87390960531436690 ) ) ;
#27009=CARTESIAN_POINT ( 'NONE',  ( 18.62759615963255655, 10.81492255796105972, 96.66775706135234714 ) ) ;
#27010=CARTESIAN_POINT ( 'NONE',  ( -16.52544592524342804, 4.483927247898546575, 31.04057627198102409 ) ) ;
#27011=CARTESIAN_POINT ( 'NONE',  ( 16.51473224551069308, 9.474510206698969483, 34.16557627198102409 ) ) ;
#27012=CARTESIAN_POINT ( 'NONE',  ( -0.05219959533934338120, 16.53943276465976808, 47.50109039468568994 ) ) ;
#27013=CARTESIAN_POINT ( 'NONE',  ( 4.379528057220339221, -16.55341960407611168, 52.70724293864769550 ) ) ;
#27014=CARTESIAN_POINT ( 'NONE',  ( -4.379528057220086978, -16.55341960407618274, 99.79275706135234714 ) ) ;
#27015=CARTESIAN_POINT ( 'NONE',  ( -18.67979575497178146, -10.72451020669898902, 21.66557627198102409 ) ) ;
#27016=CARTESIAN_POINT ( 'NONE',  ( -18.67979575497178146, -10.72451020669898902, 26.66557627198103475 ) ) ;
#27017=CARTESIAN_POINT ( 'NONE',  ( 5.049401038297881783, 19.05341960407617563, 22.29275706135233648 ) ) ;
#27018=CARTESIAN_POINT ( 'NONE',  ( 16.53943276465976808, -0.05219959533910856209, 88.74890960531436690 ) ) ;
#27019=CARTESIAN_POINT ( 'NONE',  ( 19.02544592524343514, -5.153800228976328945, 88.54057627198102409 ) ) ;
#27021=CARTESIAN_POINT ( 'NONE',  ( -0.05219959533934338120, 16.53943276465976808, 42.50109039468567573 ) ) ;
#27022=CARTESIAN_POINT ( 'NONE',  ( -13.97604488694527625, -13.89961937509977652, 41.87390960531435979 ) ) ;
#27023=CARTESIAN_POINT ( 'NONE',  ( -14.29746914071037622, -8.314922557961029526, 39.16775706135235424 ) ) ;
#27025=CARTESIAN_POINT ( 'NONE',  ( 0.05219959533936267826, -19.03943276465977164, 55.00109039468566863 ) ) ;
#27026=CARTESIAN_POINT ( 'NONE',  ( 19.05341960407611168, 5.049401038298154454, 43.95724293864769550 ) ) ;
#27027=CARTESIAN_POINT ( 'NONE',  ( -16.55341960407617563, 4.379528057220093196, 83.54275706135234714 ) ) ;
#27028=CARTESIAN_POINT ( 'NONE',  ( 19.03943276465977164, 0.05219959533936151252, 101.2510903946856757 ) ) ;
#27029=CARTESIAN_POINT ( 'NONE',  ( -19.03943276465977164, -0.05219959533935918106, 33.75109039468566863 ) ) ;
#27030=CARTESIAN_POINT ( 'NONE',  ( -9.564922557960796823, -16.46253265017161027, 67.08224293864769550 ) ) ;
#27031=CARTESIAN_POINT ( 'NONE',  ( 16.55341960407611168, 4.379528057220329451, 93.95724293864770971 ) ) ;
#27032=B_SPLINE_CURVE_WITH_KNOTS ( 'NONE', 3,
 ( #129363, #142556, #21206, #191059, #37368, #84856 ),
 .UNSPECIFIED., .F., .F.,
 ( 4, 2, 4 ),
 ( 0.003989672132298176417, 0.004372778065220590121, 0.004755883998143003825 ),
 .UNSPECIFIED. ) ;
#27033=CARTESIAN_POINT ( 'NONE',  ( -9.474510206698720793, -16.51473224551083518, 69.58442372801901854 ) ) ;
#27034=CARTESIAN_POINT ( 'NONE',  ( 15.80617190586746368, 15.72974639402197994, 64.37390960531435269 ) ) ;
#27035=CARTESIAN_POINT ( 'NONE',  ( 19.03943276465977164, 0.05219959533936151252, 46.25109039468566863 ) ) ;
#27036=CARTESIAN_POINT ( 'NONE',  ( -19.05341960407611168, -5.049401038298163336, 106.4572429386476955 ) ) ;
#27037=CARTESIAN_POINT ( 'NONE',  ( -21.55341960407610458, -5.719274019375992779, 91.45724293864769550 ) ) ;
#27038=CARTESIAN_POINT ( 'NONE',  ( -16.21995358207302829, 7.366697692864236480, 84.93551001512155096 ) ) ;
#27039=CARTESIAN_POINT ( 'NONE',  ( -19.02544592524334988, -5.153800228976617603, 98.95942372801900433 ) ) ;
#27041=CARTESIAN_POINT ( 'NONE',  ( -4.483927247898782831, 16.52544592524335698, 32.70942372801900433 ) ) ;
#27042=CARTESIAN_POINT ( 'NONE',  ( 13.97604488694527802, 13.89961937509977652, 49.37390960531434558 ) ) ;
#27043=CARTESIAN_POINT ( 'NONE',  ( -16.51473224551069308, -9.474510206698971260, 106.6655762719810383 ) ) ;
#27044=CARTESIAN_POINT ( 'NONE',  ( -15.72974639402197994, 15.80617190586746368, 95.62390960531436690 ) ) ;
#27045=CARTESIAN_POINT ( 'NONE',  ( 15.80617190586769283, -15.72974639402175789, 60.62609039468567573 ) ) ;
#27046=CARTESIAN_POINT ( 'NONE',  ( 16.46253265017146816, 9.564922557961045513, 106.6677570613523471 ) ) ;
#27047=CARTESIAN_POINT ( 'NONE',  ( -15.72974639402176322, -15.80617190586768395, 109.3760903946857042 ) ) ;
#27048=CARTESIAN_POINT ( 'NONE',  ( 8.224510206698953496, -14.34966873604960469, 22.91557627198102765 ) ) ;
#27049=CARTESIAN_POINT ( 'NONE',  ( -5.823673210054116645, -21.52544592524344225, 97.29057627198105251 ) ) ;
#27050=CARTESIAN_POINT ( 'NONE',  ( -16.52544592524342804, 4.483927247898546575, 56.04057627198102409 ) ) ;
#27051=CARTESIAN_POINT ( 'NONE',  ( 9.474510206698729675, 16.51473224551082808, 87.08442372801900433 ) ) ;
#27052=CARTESIAN_POINT ( 'NONE',  ( -5.049401038297874678, -19.05341960407617918, 59.79275706135231871 ) ) ;
#27053=CARTESIAN_POINT ( 'NONE',  ( 15.80617190586769283, -15.72974639402175789, 70.62609039468567573 ) ) ;
#27054=CARTESIAN_POINT ( 'NONE',  ( 19.03943276465977164, 0.05219959533936151252, 36.25109039468567573 ) ) ;
#27055=CARTESIAN_POINT ( 'NONE',  ( 13.97604488694527802, 13.89961937509977652, 24.37390960531435624 ) ) ;
#27056=CARTESIAN_POINT ( 'NONE',  ( -10.72451020669898014, 18.67979575497178502, 50.41557627198103120 ) ) ;
#27057=CARTESIAN_POINT ( 'NONE',  ( 16.52544592524342804, -4.483927247898539470, 33.54057627198102409 ) ) ;
#27058=CARTESIAN_POINT ( 'NONE',  ( 18.62759615963255655, 10.81492255796105972, 111.6677570613523613 ) ) ;
#27059=CARTESIAN_POINT ( 'NONE',  ( -12.14591786802326823, 12.06949235617739902, 68.12609039468567573 ) ) ;
#27060=CARTESIAN_POINT ( 'NONE',  ( -0.05219959533910754901, -16.53943276465976808, 42.49890960531435979 ) ) ;
#27061=CARTESIAN_POINT ( 'NONE',  ( -18.67979575497193778, 10.72451020669871902, 78.33442372801901854 ) ) ;
#27062=CARTESIAN_POINT ( 'NONE',  ( 10.81492255796106328, -18.62759615963255655, 65.41775706135234714 ) ) ;
#27063=CARTESIAN_POINT ( 'NONE',  ( 21.52544592524344225, -5.823673210054117533, 73.54057627198102409 ) ) ;
#27064=EDGE_CURVE ( 'NONE', #92863, #63341, #105389, .T. ) ;
#27065=ORIENTED_EDGE ( 'NONE', *, *, #193126, .F. ) ;
#27066=CARTESIAN_POINT ( 'NONE',  ( -13.97604488694527625, -13.89961937509977830, 61.87390960531435269 ) ) ;
#27067=CARTESIAN_POINT ( 'NONE',  ( -0.05219959533937732626, 21.53943276465977519, 37.50109039468568284 ) ) ;
#27068=CARTESIAN_POINT ( 'NONE',  ( 8.314922557960818139, 14.29746914071049879, 114.5822429386477097 ) ) ;
#27069=CARTESIAN_POINT ( 'NONE',  ( -5.049401038298153566, 19.05341960407611168, 40.20724293864768839 ) ) ;
#27070=CARTESIAN_POINT ( 'NONE',  ( -8.314922557960811034, -14.29746914071050412, 97.08224293864770971 ) ) ;
#27071=CARTESIAN_POINT ( 'NONE',  ( 19.02544592524343514, -5.153800228976328945, 88.54057627198102409 ) ) ;
#27072=CARTESIAN_POINT ( 'NONE',  ( -0.05219959533910754901, -16.53943276465976808, 22.49890960531436335 ) ) ;
#27073=CARTESIAN_POINT ( 'NONE',  ( -4.379528057220328563, 16.55341960407611168, 100.2072429386476955 ) ) ;
#27074=CARTESIAN_POINT ( 'NONE',  ( -18.62759615963270932, 10.81492255796079327, 75.83224293864769550 ) ) ;
#27075=CARTESIAN_POINT ( 'NONE',  ( -18.62759615963270932, 10.81492255796079327, 100.8322429386477097 ) ) ;
#27076=CARTESIAN_POINT ( 'NONE',  ( 16.51473224551069308, 9.474510206698969483, 109.1655762719810383 ) ) ;
#27077=CARTESIAN_POINT ( 'NONE',  ( 16.51473224551069308, 9.474510206698969483, 59.16557627198102409 ) ) ;
#27078=CARTESIAN_POINT ( 'NONE',  ( 8.314922557961029526, -14.29746914071037800, 20.41775706135234714 ) ) ;
#27079=CARTESIAN_POINT ( 'NONE',  ( -15.72974639402197994, 15.80617190586746368, 55.62390960531436690 ) ) ;
#27080=CARTESIAN_POINT ( 'NONE',  ( -10.72451020669870658, -18.67979575497194134, 84.58442372801903275 ) ) ;
#27081=CARTESIAN_POINT ( 'NONE',  ( -13.89961937509977652, 13.97604488694528158, 80.62390960531436690 ) ) ;
#27083=CARTESIAN_POINT ( 'NONE',  ( -19.05341960407611168, -5.049401038298163336, 106.4572429386476955 ) ) ;
#27084=CARTESIAN_POINT ( 'NONE',  ( 0.05219959533934541429, -16.53943276465976808, 75.00109039468568994 ) ) ;
#27085=CARTESIAN_POINT ( 'NONE',  ( -5.719274019375665041, -21.55341960407619695, 69.79275706135234714 ) ) ;
#27086=CARTESIAN_POINT ( 'NONE',  ( -18.62759615963255300, -10.81492255796106328, 104.1677570613523471 ) ) ;
#27087=CARTESIAN_POINT ( 'NONE',  ( 8.224510206698742110, 14.34966873604972548, 67.08442372801901854 ) ) ;
#27088=CARTESIAN_POINT ( 'NONE',  ( 10.81492255796078972, 18.62759615963270932, 114.5822429386477097 ) ) ;
#27089=CARTESIAN_POINT ( 'NONE',  ( 9.474510206698971260, -16.51473224551069308, 112.9155762719810383 ) ) ;
#27090=CARTESIAN_POINT ( 'NONE',  ( 21.53943276465977519, 0.05219959533937863772, 91.25109039468568994 ) ) ;
#27091=CARTESIAN_POINT ( 'NONE',  ( 15.80617190586746368, 15.72974639402197994, 94.37390960531436690 ) ) ;
#27092=CARTESIAN_POINT ( 'NONE',  ( -13.97604488694547697, 13.89961937509957934, 53.12609039468565442 ) ) ;
#27093=CARTESIAN_POINT ( 'NONE',  ( 21.55341960407610458, 5.719274019375980345, 48.95724293864770971 ) ) ;
#27094=CARTESIAN_POINT ( 'NONE',  ( 5.153800228976335163, 19.02544592524342804, 94.79057627198103830 ) ) ;
#27095=CARTESIAN_POINT ( 'NONE',  ( -4.483927247898539470, -16.52544592524342804, 37.29057627198102409 ) ) ;
#27096=CARTESIAN_POINT ( 'NONE',  ( -17.49999999999999289, 5.500000000000036415, 65.79690382534171533 ) ) ;
#27097=CARTESIAN_POINT ( 'NONE',  ( 18.09867054820430710, 5.500000000000001776, 81.48393025253585620 ) ) ;
#27098=B_SPLINE_CURVE_WITH_KNOTS ( 'NONE', 3,
 ( #64626, #199167, #944, #62619, #30312, #107138, #77795, #75809, #169815, #124297, #63632, #18136, #141463, #170812, #126288, #140463, #78786, #152652, #185994, #123295, #1953, #60634, #171809, #168808, #91955, #125308, #153648, #172806, #187004, #156640, #47477, #187985 ),
 .UNSPECIFIED., .F., .F.,
 ( 4, 2, 2, 2, 2, 2, 2, 2, 2, 2, 2, 2, 2, 2, 2, 4 ),
 ( 1.262897753262582698E-17, 0.0003712461730036966984, 0.0007424923460073807116, 0.001113738519011064779, 0.001484984692014748846, 0.002227477038022110042, 0.002598723211025783918, 0.002969969384029457361, 0.003341215557033131237, 0.003712461730036805546, 0.004083707903040478988, 0.004454954076044153298, 0.004826200249047825873, 0.005197446422051500182, 0.005568692595055173625, 0.005939938768058847067 ),
 .UNSPECIFIED. ) ;
#27099=CARTESIAN_POINT ( 'NONE',  ( -14.29746914071037622, -8.314922557961029526, 19.16775706135234714 ) ) ;
#27100=CARTESIAN_POINT ( 'NONE',  ( -18.67979575497178146, -10.72451020669898902, 86.66557627198102409 ) ) ;
#27101=CARTESIAN_POINT ( 'NONE',  ( -14.29746914071049879, 8.314922557960819915, 45.83224293864769550 ) ) ;
#27102=CARTESIAN_POINT ( 'NONE',  ( 8.224510206698742110, 14.34966873604972548, 32.08442372801901854 ) ) ;
#27103=CARTESIAN_POINT ( 'NONE',  ( 19.02544592524343514, -5.153800228976328945, 38.54057627198103120 ) ) ;
#27104=CARTESIAN_POINT ( 'NONE',  ( 18.67979575497178502, 10.72451020669898547, 109.1655762719810383 ) ) ;
#27105=CARTESIAN_POINT ( 'NONE',  ( -9.564922557961040184, 16.46253265017147172, 87.91775706135233293 ) ) ;
#27106=CARTESIAN_POINT ( 'NONE',  ( 5.049401038298161559, -19.05341960407611168, 82.70724293864770971 ) ) ;
#27107=CARTESIAN_POINT ( 'NONE',  ( -0.05219959533909027116, -19.03943276465977164, 77.49890960531435269 ) ) ;
#27108=CARTESIAN_POINT ( 'NONE',  ( 21.55341960407610458, 5.719274019375980345, 73.95724293864769550 ) ) ;
#27109=CARTESIAN_POINT ( 'NONE',  ( -19.05341960407611168, -5.049401038298163336, 36.45724293864766707 ) ) ;
#27111=CARTESIAN_POINT ( 'NONE',  ( 12.14591786802309770, 12.06949235617756955, 54.37390960531435979 ) ) ;
#27112=CARTESIAN_POINT ( 'NONE',  ( 13.97604488694527802, 13.89961937509977652, 84.37390960531433848 ) ) ;
#27114=CARTESIAN_POINT ( 'NONE',  ( 9.474510206698729675, 16.51473224551082808, 72.08442372801900433 ) ) ;
#27115=CARTESIAN_POINT ( 'NONE',  ( -5.823673210054116645, -21.52544592524344225, 77.29057627198102409 ) ) ;
#27116=CARTESIAN_POINT ( 'NONE',  ( -5.049401038297874678, -19.05341960407617918, 34.79275706135233293 ) ) ;
#27117=CARTESIAN_POINT ( 'NONE',  ( -19.05341960407611168, -5.049401038298163336, 106.4572429386476955 ) ) ;
#27118=CARTESIAN_POINT ( 'NONE',  ( -17.49999999999999645, 3.189878218039174040, 114.8705143742876089 ) ) ;
#27119=CARTESIAN_POINT ( 'NONE',  ( -15.72974639402197994, 15.80617190586746368, 25.62390960531435624 ) ) ;
#27120=CARTESIAN_POINT ( 'NONE',  ( 16.51473224551069308, 9.474510206698969483, 74.16557627198103830 ) ) ;
#27121=CARTESIAN_POINT ( 'NONE',  ( 15.80617190586769283, -15.72974639402175789, 50.62609039468568994 ) ) ;
#27122=CARTESIAN_POINT ( 'NONE',  ( -16.46253265017160317, 9.564922557960807481, 25.83224293864769194 ) ) ;
#27123=CARTESIAN_POINT ( 'NONE',  ( -5.719274019375978568, 21.55341960407610458, 115.2072429386476955 ) ) ;
#27124=ORIENTED_EDGE ( 'NONE', *, *, #38220, .T. ) ;
#27125=CARTESIAN_POINT ( 'NONE',  ( 21.52544592524334988, 5.823673210054432836, 36.45942372801901143 ) ) ;
#27127=CARTESIAN_POINT ( 'NONE',  ( -13.97604488694527625, -13.89961937509977652, 106.8739096053143669 ) ) ;
#27129=CARTESIAN_POINT ( 'NONE',  ( 0.05219959533907565091, 21.53943276465977519, 109.9989096053143527 ) ) ;
#27130=CARTESIAN_POINT ( 'NONE',  ( 9.564922557960805705, 16.46253265017160317, 59.58224293864769550 ) ) ;
#27131=CARTESIAN_POINT ( 'NONE',  ( -14.34966873604972548, 8.224510206698743886, 23.33442372801901499 ) ) ;
#27133=CARTESIAN_POINT ( 'NONE',  ( -21.55341960407619339, 5.719274019375674811, 103.5427570613523613 ) ) ;
#27134=CARTESIAN_POINT ( 'NONE',  ( -9.564922557960796823, -16.46253265017161027, 47.08224293864769550 ) ) ;
#27135=CARTESIAN_POINT ( 'NONE',  ( -21.52544592524334988, -5.823673210054445271, 98.95942372801903275 ) ) ;
#27136=CARTESIAN_POINT ( 'NONE',  ( 19.03943276465977164, -0.05219959533909143690, 88.74890960531436690 ) ) ;
#27137=CARTESIAN_POINT ( 'NONE',  ( -18.67979575497193778, 10.72451020669871902, 63.33442372801900433 ) ) ;
#27139=CARTESIAN_POINT ( 'NONE',  ( -0.05219959533909027116, -19.03943276465977164, 107.4989096053143527 ) ) ;
#27140=CARTESIAN_POINT ( 'NONE',  ( -17.50000000000001421, 3.189878218039132296, 29.87051437428767287 ) ) ;
#27141=CARTESIAN_POINT ( 'NONE',  ( -0.05219959533934338120, 16.53943276465976808, 47.50109039468568994 ) ) ;
#27142=CARTESIAN_POINT ( 'NONE',  ( 16.55341960407618274, -4.379528057220086978, 66.04275706135236135 ) ) ;
#27143=CARTESIAN_POINT ( 'NONE',  ( 5.719274019375673035, 21.55341960407619339, 52.29275706135236135 ) ) ;
#27144=CARTESIAN_POINT ( 'NONE',  ( 21.53943276465977519, 0.05219959533937863772, 96.25109039468568994 ) ) ;
#27146=CARTESIAN_POINT ( 'NONE',  ( -14.34966873604972548, 8.224510206698743886, 28.33442372801902209 ) ) ;
#27147=CARTESIAN_POINT ( 'NONE',  ( 16.51473224551069308, 9.474510206698969483, 69.16557627198102409 ) ) ;
#27148=CARTESIAN_POINT ( 'NONE',  ( 0.05219959533909260263, 19.03943276465977164, 109.9989096053143669 ) ) ;
#27149=CARTESIAN_POINT ( 'NONE',  ( 17.13100169013298668, 6.664070546373162429, 41.73210164300153480 ) ) ;
#27150=CARTESIAN_POINT ( 'NONE',  ( -13.89961937509977652, 13.97604488694528158, 25.62390960531434558 ) ) ;
#27151=CARTESIAN_POINT ( 'NONE',  ( 10.72451020669898902, -18.67979575497178502, 47.91557627198102409 ) ) ;
#27152=CARTESIAN_POINT ( 'NONE',  ( 12.06949235617739724, 12.14591786802326823, 91.87609039468568994 ) ) ;
#27153=CARTESIAN_POINT ( 'NONE',  ( -0.05219959533910754901, -16.53943276465976808, 77.49890960531433848 ) ) ;
#27154=CARTESIAN_POINT ( 'NONE',  ( -9.564922557960796823, -16.46253265017161027, 62.08224293864769550 ) ) ;
#27155=CARTESIAN_POINT ( 'NONE',  ( -21.53943276465977519, -0.05219959533937600094, 93.75109039468567573 ) ) ;
#27157=CARTESIAN_POINT ( 'NONE',  ( -16.52544592524335698, -4.483927247898792601, 23.95942372801901143 ) ) ;
#27158=CARTESIAN_POINT ( 'NONE',  ( -16.52544592524342804, 4.483927247898546575, 71.04057627198103830 ) ) ;
#27159=CARTESIAN_POINT ( 'NONE',  ( 15.80617190586769283, -15.72974639402175789, 40.62609039468567573 ) ) ;
#27160=CARTESIAN_POINT ( 'NONE',  ( -10.81492255796078084, -18.62759615963271287, 72.08224293864769550 ) ) ;
#27161=CARTESIAN_POINT ( 'NONE',  ( -9.564922557961040184, 16.46253265017147172, 37.91775706135233293 ) ) ;
#27163=CARTESIAN_POINT ( 'NONE',  ( -0.05219959533909027116, -19.03943276465977164, 77.49890960531435269 ) ) ;
#27164=CARTESIAN_POINT ( 'NONE',  ( -12.14591786802309592, -12.06949235617757132, 51.87390960531437401 ) ) ;
#27166=CARTESIAN_POINT ( 'NONE',  ( -4.379528057220328563, 16.55341960407611168, 30.20724293864769550 ) ) ;
#27167=CARTESIAN_POINT ( 'NONE',  ( -14.34966873604972548, 8.224510206698743886, 108.3344237280190185 ) ) ;
#27168=CARTESIAN_POINT ( 'NONE',  ( -16.46253265017146816, -9.564922557961047289, 69.16775706135233293 ) ) ;
#27170=CARTESIAN_POINT ( 'NONE',  ( 15.72974639402199770, -15.80617190586745480, 28.12390960531435979 ) ) ;
#27171=CARTESIAN_POINT ( 'NONE',  ( -16.52544592524342804, 4.483927247898546575, 91.04057627198103830 ) ) ;
#27172=CARTESIAN_POINT ( 'NONE',  ( -18.10062525802553424, 5.500000000000031086, 58.51383468041921532 ) ) ;
#27173=CARTESIAN_POINT ( 'NONE',  ( 0.05219959533909260263, 19.03943276465977164, 39.99890960531436690 ) ) ;
#27174=CARTESIAN_POINT ( 'NONE',  ( 18.67979575497178502, 10.72451020669898547, 44.16557627198103120 ) ) ;
#27175=CARTESIAN_POINT ( 'NONE',  ( 21.52544592524344225, -5.823673210054117533, 63.54057627198103830 ) ) ;
#27176=CARTESIAN_POINT ( 'NONE',  ( 16.55341960407611168, 4.379528057220329451, 108.9572429386476955 ) ) ;
#27177=CARTESIAN_POINT ( 'NONE',  ( -8.224510206698735004, -14.34966873604973081, 64.58442372801900433 ) ) ;
#27178=CARTESIAN_POINT ( 'NONE',  ( -5.153800228976328057, -19.02544592524343514, 42.29057627198101699 ) ) ;
#27179=CARTESIAN_POINT ( 'NONE',  ( 15.80617190586769283, -15.72974639402175789, 60.62609039468567573 ) ) ;
#27180=CARTESIAN_POINT ( 'NONE',  ( 8.314922557960818139, 14.29746914071049879, 104.5822429386477097 ) ) ;
#27181=CARTESIAN_POINT ( 'NONE',  ( -16.51473224551082808, 9.474510206698731452, 93.33442372801900433 ) ) ;
#27184=CARTESIAN_POINT ( 'NONE',  ( -5.823673210054116645, -21.52544592524344225, 37.29057627198102409 ) ) ;
#27185=CARTESIAN_POINT ( 'NONE',  ( 17.48847506799968343, -5.747544572773780835, 68.32697437843283694 ) ) ;
#27186=CARTESIAN_POINT ( 'NONE',  ( -18.67979575497193778, 10.72451020669871902, 73.33442372801901854 ) ) ;
#27187=CARTESIAN_POINT ( 'NONE',  ( 16.52544592524335698, 4.483927247898782831, 56.45942372801902565 ) ) ;
#27188=CARTESIAN_POINT ( 'NONE',  ( 4.483927247898545687, 16.52544592524342804, 49.79057627198102409 ) ) ;
#27189=CARTESIAN_POINT ( 'NONE',  ( 10.72451020669898902, -18.67979575497178502, 62.91557627198102409 ) ) ;
#27190=CARTESIAN_POINT ( 'NONE',  ( -10.72451020669898014, 18.67979575497178502, 65.41557627198102409 ) ) ;
#27192=CARTESIAN_POINT ( 'NONE',  ( 19.03943276465977164, 0.05219959533936151252, 81.25109039468567573 ) ) ;
#27193=CARTESIAN_POINT ( 'NONE',  ( 13.89961937509977652, -13.97604488694527269, 108.1239096053143669 ) ) ;
#27195=CARTESIAN_POINT ( 'NONE',  ( 19.03943276465977164, -0.05219959533909143690, 43.74890960531435979 ) ) ;
#27196=CARTESIAN_POINT ( 'NONE',  ( 0.05219959533910956823, 16.53943276465976808, 109.9989096053143527 ) ) ;
#27197=CARTESIAN_POINT ( 'NONE',  ( 19.02544592524343514, -5.153800228976328945, 113.5405762719810241 ) ) ;
#27199=CARTESIAN_POINT ( 'NONE',  ( -12.06949235617739369, -12.14591786802326823, 74.37609039468568994 ) ) ;
#27200=CARTESIAN_POINT ( 'NONE',  ( -18.62759615963270932, 10.81492255796079327, 105.8322429386476955 ) ) ;
#27201=CARTESIAN_POINT ( 'NONE',  ( 16.51473224551069308, 9.474510206698969483, 74.16557627198103830 ) ) ;
#27202=CARTESIAN_POINT ( 'NONE',  ( 15.72974639402176855, 15.80617190586768217, 36.87609039468568994 ) ) ;
#27203=CARTESIAN_POINT ( 'NONE',  ( 19.05341960407611168, 5.049401038298154454, 98.95724293864766707 ) ) ;
#27205=VERTEX_POINT ( 'NONE', #110236 ) ;
#27206=CARTESIAN_POINT ( 'NONE',  ( -21.55341960407619339, 5.719274019375674811, 33.54275706135234714 ) ) ;
#27207=CARTESIAN_POINT ( 'NONE',  ( 9.474510206698971260, -16.51473224551069308, 27.91557627198103120 ) ) ;
#27208=CARTESIAN_POINT ( 'NONE',  ( -9.474510206698720793, -16.51473224551083518, 84.58442372801900433 ) ) ;
#27209=CARTESIAN_POINT ( 'NONE',  ( -19.02544592524334988, -5.153800228976617603, 33.95942372801897591 ) ) ;
#27210=CARTESIAN_POINT ( 'NONE',  ( -10.72451020669898014, 18.67979575497178502, 110.4155762719810383 ) ) ;
#27211=CARTESIAN_POINT ( 'NONE',  ( 16.46253265017146816, 9.564922557961045513, 36.66775706135233293 ) ) ;
#27212=CARTESIAN_POINT ( 'NONE',  ( 5.049401038297881783, 19.05341960407617563, 47.29275706135231161 ) ) ;
#27213=CARTESIAN_POINT ( 'NONE',  ( -12.06949235617739369, -12.14591786802326823, 94.37609039468568994 ) ) ;
#27215=CARTESIAN_POINT ( 'NONE',  ( -0.05219959533909027116, -19.03943276465977164, 67.49890960531436690 ) ) ;
#27216=CARTESIAN_POINT ( 'NONE',  ( 21.52544592524334988, 5.823673210054432836, 81.45942372801900433 ) ) ;
#27217=CARTESIAN_POINT ( 'NONE',  ( -18.62759615963255300, -10.81492255796106328, 94.16775706135237556 ) ) ;
#27219=CARTESIAN_POINT ( 'NONE',  ( -19.05341960407611168, -5.049401038298163336, 81.45724293864769550 ) ) ;
#27220=CARTESIAN_POINT ( 'NONE',  ( -21.52544592524334988, -5.823673210054445271, 58.95942372801902565 ) ) ;
#27221=CARTESIAN_POINT ( 'NONE',  ( 19.02544592524334988, 5.153800228976608722, 101.4594237280189759 ) ) ;
#27222=CARTESIAN_POINT ( 'NONE',  ( 19.02544592524343514, -5.153800228976328945, 68.54057627198103830 ) ) ;
#27223=CARTESIAN_POINT ( 'NONE',  ( -0.05219959533907301413, -21.53943276465977519, 22.49890960531436335 ) ) ;
#27224=CARTESIAN_POINT ( 'NONE',  ( 5.049401038298161559, -19.05341960407611168, 82.70724293864770971 ) ) ;
#27226=CARTESIAN_POINT ( 'NONE',  ( 13.89961937509977652, -13.97604488694527269, 63.12390960531435979 ) ) ;
#27227=CARTESIAN_POINT ( 'NONE',  ( 19.03943276465977164, -0.05219959533909143690, 48.74890960531435979 ) ) ;
#27228=CARTESIAN_POINT ( 'NONE',  ( -15.80617190586745835, -15.72974639402198527, 111.8739096053143669 ) ) ;
#27229=CARTESIAN_POINT ( 'NONE',  ( 14.34966873604972726, -8.224510206698740333, 90.83442372801901854 ) ) ;
#27231=CARTESIAN_POINT ( 'NONE',  ( -19.03943276465977164, -0.05219959533935918106, 58.75109039468566863 ) ) ;
#27232=CARTESIAN_POINT ( 'NONE',  ( 16.46253265017160672, -9.564922557960803928, 73.33224293864769550 ) ) ;
#27233=CARTESIAN_POINT ( 'NONE',  ( -4.483927247898539470, -16.52544592524342804, 72.29057627198102409 ) ) ;
#27234=CARTESIAN_POINT ( 'NONE',  ( -14.34966873604960291, -8.224510206698953496, 101.6655762719810383 ) ) ;
#27235=CARTESIAN_POINT ( 'NONE',  ( -5.049401038298153566, 19.05341960407611168, 115.2072429386477097 ) ) ;
#27236=CARTESIAN_POINT ( 'NONE',  ( 19.03943276465977164, -0.05219959533909143690, 98.74890960531436690 ) ) ;
#27237=CARTESIAN_POINT ( 'NONE',  ( -8.314922557960811034, -14.29746914071050412, 77.08224293864769550 ) ) ;
#27238=CARTESIAN_POINT ( 'NONE',  ( -5.049401038298153566, 19.05341960407611168, 115.2072429386477097 ) ) ;
#27239=CARTESIAN_POINT ( 'NONE',  ( 16.51473224551083163, -9.474510206698727899, 30.83442372801900433 ) ) ;
#27240=CARTESIAN_POINT ( 'NONE',  ( -4.379528057220086978, -16.55341960407618274, 109.7927570613523613 ) ) ;
#27241=CARTESIAN_POINT ( 'NONE',  ( -13.89961937509977652, 13.97604488694528158, 90.62390960531432427 ) ) ;
#27242=CARTESIAN_POINT ( 'NONE',  ( -18.62759615963255300, -10.81492255796106328, 54.16775706135235424 ) ) ;
#27243=CARTESIAN_POINT ( 'NONE',  ( 18.67979575497178502, 10.72451020669898547, 44.16557627198103120 ) ) ;
#27244=CARTESIAN_POINT ( 'NONE',  ( 21.52544592524344225, -5.823673210054117533, 113.5405762719810383 ) ) ;
#27245=CARTESIAN_POINT ( 'NONE',  ( 15.80617190586746368, 15.72974639402197994, 64.37390960531435269 ) ) ;
#27246=CARTESIAN_POINT ( 'NONE',  ( 16.53943276465976808, -0.05219959533910856209, 88.74890960531436690 ) ) ;
#27247=CARTESIAN_POINT ( 'NONE',  ( -16.46253265017146816, -9.564922557961047289, 54.16775706135234003 ) ) ;
#27249=CARTESIAN_POINT ( 'NONE',  ( -19.05341960407611168, -5.049401038298163336, 26.45724293864769550 ) ) ;
#27250=CARTESIAN_POINT ( 'NONE',  ( 19.02544592524343514, -5.153800228976328945, 88.54057627198102409 ) ) ;
#27251=CARTESIAN_POINT ( 'NONE',  ( -19.05341960407611168, -5.049401038298163336, 81.45724293864769550 ) ) ;
#27252=CARTESIAN_POINT ( 'NONE',  ( -12.06949235617756955, 12.14591786802309770, 100.6239096053143811 ) ) ;
#27254=CARTESIAN_POINT ( 'NONE',  ( -16.55341960407611168, -4.379528057220339221, 26.45724293864768839 ) ) ;
#27255=CARTESIAN_POINT ( 'NONE',  ( 8.224510206698742110, 14.34966873604972548, 47.08442372801901854 ) ) ;
#27256=CARTESIAN_POINT ( 'NONE',  ( 10.81492255796106328, -18.62759615963255655, 110.4177570613523756 ) ) ;
#27257=CARTESIAN_POINT ( 'NONE',  ( 5.049401038298161559, -19.05341960407611168, 97.70724293864766707 ) ) ;
#27258=CARTESIAN_POINT ( 'NONE',  ( -0.05219959533937732626, 21.53943276465977519, 27.50109039468567929 ) ) ;
#27259=CARTESIAN_POINT ( 'NONE',  ( -5.153800228976328057, -19.02544592524343514, 47.29057627198102409 ) ) ;
#27261=CARTESIAN_POINT ( 'NONE',  ( 16.53943276465976808, 0.05219959533934440121, 41.25109039468568284 ) ) ;
#27262=CARTESIAN_POINT ( 'NONE',  ( -14.29746914071037622, -8.314922557961029526, 84.16775706135234714 ) ) ;
#27263=CARTESIAN_POINT ( 'NONE',  ( -9.564922557961040184, 16.46253265017147172, 107.9177570613523471 ) ) ;
#27264=CARTESIAN_POINT ( 'NONE',  ( -5.049401038298153566, 19.05341960407611168, 35.20724293864768839 ) ) ;
#27265=CARTESIAN_POINT ( 'NONE',  ( 16.53943276465976808, -0.05219959533910856209, 93.74890960531436690 ) ) ;
#27266=CARTESIAN_POINT ( 'NONE',  ( -0.05219959533907301413, -21.53943276465977519, 97.49890960531436690 ) ) ;
#27267=CARTESIAN_POINT ( 'NONE',  ( 16.46253265017146816, 9.564922557961045513, 76.66775706135234714 ) ) ;
#27268=CARTESIAN_POINT ( 'NONE',  ( -16.46253265017160317, 9.564922557960807481, 25.83224293864769194 ) ) ;
#27269=CARTESIAN_POINT ( 'NONE',  ( 13.97604488694527802, 13.89961937509977652, 89.37390960531436690 ) ) ;
#27270=CARTESIAN_POINT ( 'NONE',  ( -5.719274019375665041, -21.55341960407619695, 34.79275706135235424 ) ) ;
#27272=CARTESIAN_POINT ( 'NONE',  ( -19.02544592524342804, 5.153800228976336051, 96.04057627198103830 ) ) ;
#27275=CARTESIAN_POINT ( 'NONE',  ( 19.02544592524343514, -5.153800228976328945, 88.54057627198102409 ) ) ;
#27276=CARTESIAN_POINT ( 'NONE',  ( 21.52544592524334988, 5.823673210054432836, 36.45942372801901143 ) ) ;
#27277=CARTESIAN_POINT ( 'NONE',  ( -14.29746914071049879, 8.314922557960819915, 85.83224293864768129 ) ) ;
#27278=CARTESIAN_POINT ( 'NONE',  ( -5.049401038298153566, 19.05341960407611168, 100.2072429386476955 ) ) ;
#27279=CARTESIAN_POINT ( 'NONE',  ( 16.46253265017146816, 9.564922557961045513, 21.66775706135233648 ) ) ;
#27281=CARTESIAN_POINT ( 'NONE',  ( -8.224510206698735004, -14.34966873604973081, 54.58442372801901143 ) ) ;
#27283=CARTESIAN_POINT ( 'NONE',  ( 5.823673210054444382, -21.52544592524334988, 75.20942372801901854 ) ) ;
#27284=CARTESIAN_POINT ( 'NONE',  ( -4.483927247898782831, 16.52544592524335698, 42.70942372801901854 ) ) ;
#27285=CARTESIAN_POINT ( 'NONE',  ( 13.89961937509977652, -13.97604488694527269, 68.12390960531436690 ) ) ;
#27286=CARTESIAN_POINT ( 'NONE',  ( -19.02544592524334988, -5.153800228976617603, 93.95942372801900433 ) ) ;
#27287=CARTESIAN_POINT ( 'NONE',  ( 16.55341960407618274, -4.379528057220086978, 71.04275706135234714 ) ) ;
#27288=CARTESIAN_POINT ( 'NONE',  ( -21.52544592524334988, -5.823673210054445271, 108.9594237280190185 ) ) ;
#27289=CARTESIAN_POINT ( 'NONE',  ( -9.474510206698720793, -16.51473224551083518, 74.58442372801900433 ) ) ;
#27290=CARTESIAN_POINT ( 'NONE',  ( -19.03943276465977164, 0.05219959533909376836, 61.24890960531436690 ) ) ;
#27291=CARTESIAN_POINT ( 'NONE',  ( -5.719274019375978568, 21.55341960407610458, 90.20724293864770971 ) ) ;
#27292=CARTESIAN_POINT ( 'NONE',  ( 12.06949235617757843, -12.14591786802309237, 83.12390960531436690 ) ) ;
#27293=CARTESIAN_POINT ( 'NONE',  ( -19.02544592524334988, -5.153800228976617603, 93.95942372801900433 ) ) ;
#27294=CARTESIAN_POINT ( 'NONE',  ( -19.35633801406908816, 5.499999999999577227, 79.13373818172760821 ) ) ;
#27295=CARTESIAN_POINT ( 'NONE',  ( 19.03943276465977164, 0.05219959533936151252, 56.25109039468566863 ) ) ;
#27296=CARTESIAN_POINT ( 'NONE',  ( 12.06949235617739724, 12.14591786802326823, 111.8760903946856615 ) ) ;
#27297=CARTESIAN_POINT ( 'NONE',  ( -12.14591786802309592, -12.06949235617757132, 76.87390960531439532 ) ) ;
#27298=CARTESIAN_POINT ( 'NONE',  ( 5.153800228976615827, -19.02544592524334988, 20.20942372801899722 ) ) ;
#27299=CARTESIAN_POINT ( 'NONE',  ( -16.31925111598407341, 7.325300261831847237, 40.16424538967169866 ) ) ;
#27300=CARTESIAN_POINT ( 'NONE',  ( -21.52544592524343514, 5.823673210054127303, 106.0405762719810525 ) ) ;
#27301=CARTESIAN_POINT ( 'NONE',  ( -5.153800228976328057, -19.02544592524343514, 102.2905762719810383 ) ) ;
#27302=CARTESIAN_POINT ( 'NONE',  ( 19.02544592524343514, -5.153800228976328945, 83.54057627198100988 ) ) ;
#27303=CARTESIAN_POINT ( 'NONE',  ( 18.62759615963255655, 10.81492255796105972, 81.66775706135236135 ) ) ;
#27304=CARTESIAN_POINT ( 'NONE',  ( 5.153800228976335163, 19.02544592524342804, 64.79057627198100988 ) ) ;
#27305=CARTESIAN_POINT ( 'NONE',  ( -16.51473224551069308, -9.474510206698971260, 41.66557627198103120 ) ) ;
#27306=CARTESIAN_POINT ( 'NONE',  ( -21.52544592524343514, 5.823673210054127303, 26.04057627198103475 ) ) ;
#27307=CARTESIAN_POINT ( 'NONE',  ( -16.53943276465976808, 0.05219959533911058130, 86.24890960531436690 ) ) ;
#27308=CARTESIAN_POINT ( 'NONE',  ( 0.05219959533909260263, 19.03943276465977164, 49.99890960531435979 ) ) ;
#27309=CARTESIAN_POINT ( 'NONE',  ( 8.314922557960818139, 14.29746914071049879, 99.58224293864770971 ) ) ;
#27311=CARTESIAN_POINT ( 'NONE',  ( 18.62759615963271287, -10.81492255796078972, 103.3322429386476955 ) ) ;
#27312=CARTESIAN_POINT ( 'NONE',  ( 15.72974639402176855, 15.80617190586768217, 46.87609039468568994 ) ) ;
#27313=CARTESIAN_POINT ( 'NONE',  ( 19.03943276465977164, -0.05219959533909143690, 33.74890960531435979 ) ) ;
#27314=CARTESIAN_POINT ( 'NONE',  ( -14.34966873604972548, 8.224510206698743886, 58.33442372801901143 ) ) ;
#27315=CARTESIAN_POINT ( 'NONE',  ( 21.53943276465977519, -0.05219959533907433946, 98.74890960531438111 ) ) ;
#27316=CARTESIAN_POINT ( 'NONE',  ( -5.823673210054116645, -21.52544592524344225, 102.2905762719810383 ) ) ;
#27317=CARTESIAN_POINT ( 'NONE',  ( -13.89961937509957401, -13.97604488694547875, 34.37609039468566863 ) ) ;
#27318=CARTESIAN_POINT ( 'NONE',  ( -9.564922557960796823, -16.46253265017161027, 47.08224293864769550 ) ) ;
#27319=CARTESIAN_POINT ( 'NONE',  ( -5.049401038298153566, 19.05341960407611168, 115.2072429386477097 ) ) ;
#27320=CARTESIAN_POINT ( 'NONE',  ( 18.67979575497194134, -10.72451020669871369, 50.83442372801901143 ) ) ;
#27321=CARTESIAN_POINT ( 'NONE',  ( -5.823673210054116645, -21.52544592524344225, 52.29057627198102409 ) ) ;
#27322=CARTESIAN_POINT ( 'NONE',  ( -14.34966873604960291, -8.224510206698953496, 41.66557627198103120 ) ) ;
#27323=CARTESIAN_POINT ( 'NONE',  ( -10.81492255796105439, 18.62759615963255655, 77.91775706135231871 ) ) ;
#27324=CARTESIAN_POINT ( 'NONE',  ( -18.67979575497193778, 10.72451020669871902, 113.3344237280190328 ) ) ;
#27325=CARTESIAN_POINT ( 'NONE',  ( 0.05219959533910956823, 16.53943276465976808, 84.99890960531436690 ) ) ;
#27326=CARTESIAN_POINT ( 'NONE',  ( -19.02544592524334988, -5.153800228976617603, 43.95942372801899012 ) ) ;
#27327=CARTESIAN_POINT ( 'NONE',  ( -14.34966873604972548, 8.224510206698743886, 103.3344237280190043 ) ) ;
#27328=CARTESIAN_POINT ( 'NONE',  ( -10.81492255796105439, 18.62759615963255655, 72.91775706135234714 ) ) ;
#27329=CARTESIAN_POINT ( 'NONE',  ( 16.51473224551069308, 9.474510206698969483, 59.16557627198102409 ) ) ;
#27330=CARTESIAN_POINT ( 'NONE',  ( 13.97604488694548053, -13.89961937509957401, 40.62609039468564731 ) ) ;
#27331=CARTESIAN_POINT ( 'NONE',  ( -18.62759615963270932, 10.81492255796079327, 35.83224293864768839 ) ) ;
#27332=CARTESIAN_POINT ( 'NONE',  ( 21.55341960407619695, -5.719274019375665929, 31.04275706135234714 ) ) ;
#27333=CARTESIAN_POINT ( 'NONE',  ( -10.81492255796078084, -18.62759615963271287, 87.08224293864769550 ) ) ;
#27334=CARTESIAN_POINT ( 'NONE',  ( 16.51473224551083163, -9.474510206698727899, 90.83442372801900433 ) ) ;
#27335=CARTESIAN_POINT ( 'NONE',  ( 12.06949235617739724, 12.14591786802326823, 51.87609039468568284 ) ) ;
#27337=CARTESIAN_POINT ( 'NONE',  ( -0.05219959533907301413, -21.53943276465977519, 87.49890960531436690 ) ) ;
#27338=CARTESIAN_POINT ( 'NONE',  ( -8.224510206698735004, -14.34966873604973081, 74.58442372801901854 ) ) ;
#27339=CARTESIAN_POINT ( 'NONE',  ( -16.55341960407611168, -4.379528057220339221, 76.45724293864769550 ) ) ;
#27341=CARTESIAN_POINT ( 'NONE',  ( 5.153800228976615827, -19.02544592524334988, 100.2094237280190043 ) ) ;
#27342=CARTESIAN_POINT ( 'NONE',  ( -21.52544592524343514, 5.823673210054127303, 31.04057627198102409 ) ) ;
#27344=CARTESIAN_POINT ( 'NONE',  ( -12.06949235617739369, -12.14591786802326823, 54.37609039468568994 ) ) ;
#27345=CARTESIAN_POINT ( 'NONE',  ( 10.72451020669871369, 18.67979575497193778, 27.08442372801901854 ) ) ;
#27346=CARTESIAN_POINT ( 'NONE',  ( -15.72974639402197994, 15.80617190586746368, 40.62390960531435269 ) ) ;
#27347=CARTESIAN_POINT ( 'NONE',  ( -12.14591786802326823, 12.06949235617739902, 68.12609039468567573 ) ) ;
#27348=CARTESIAN_POINT ( 'NONE',  ( -5.049401038298153566, 19.05341960407611168, 85.20724293864766707 ) ) ;
#27349=CARTESIAN_POINT ( 'NONE',  ( -15.80617190586768217, 15.72974639402176855, 53.12609039468568284 ) ) ;
#27350=CARTESIAN_POINT ( 'NONE',  ( -16.51473224551069308, -9.474510206698971260, 21.66557627198102765 ) ) ;
#27351=CARTESIAN_POINT ( 'NONE',  ( -5.719274019375978568, 21.55341960407610458, 40.20724293864769550 ) ) ;
#27353=CARTESIAN_POINT ( 'NONE',  ( 19.05341960407617918, -5.049401038297876454, 41.04275706135233293 ) ) ;
#27354=CARTESIAN_POINT ( 'NONE',  ( -14.34966873604972548, 8.224510206698743886, 58.33442372801901143 ) ) ;
#27355=CARTESIAN_POINT ( 'NONE',  ( -19.03943276465977164, 0.05219959533909376836, 116.2489096053143669 ) ) ;
#27357=CARTESIAN_POINT ( 'NONE',  ( -0.05219959533909027116, -19.03943276465977164, 92.49890960531436690 ) ) ;
#27358=CARTESIAN_POINT ( 'NONE',  ( 4.379528057220092307, 16.55341960407617563, 102.2927570613523613 ) ) ;
#27360=CARTESIAN_POINT ( 'NONE',  ( -14.34966873604960291, -8.224510206698953496, 101.6655762719810383 ) ) ;
#27361=CARTESIAN_POINT ( 'NONE',  ( 15.80617190586746368, 15.72974639402197994, 39.37390960531436690 ) ) ;
#27362=CARTESIAN_POINT ( 'NONE',  ( -16.46253265017160317, 9.564922557960807481, 35.83224293864768839 ) ) ;
#27363=CARTESIAN_POINT ( 'NONE',  ( 12.06949235617739724, 12.14591786802326823, 81.87609039468568994 ) ) ;
#27364=CARTESIAN_POINT ( 'NONE',  ( -21.53943276465977519, 0.05219959533907696930, 111.2489096053143669 ) ) ;
#27365=CARTESIAN_POINT ( 'NONE',  ( 13.97604488694548053, -13.89961937509957401, 70.62609039468567573 ) ) ;
#27366=CARTESIAN_POINT ( 'NONE',  ( 16.46253265017160672, -9.564922557960803928, 43.33224293864769550 ) ) ;
#27367=FACE_OUTER_BOUND ( 'NONE', #29474, .T. ) ;
#27368=CARTESIAN_POINT ( 'NONE',  ( 21.55341960407619695, -5.719274019375665929, 111.0427570613523613 ) ) ;
#27369=CARTESIAN_POINT ( 'NONE',  ( 9.564922557960805705, 16.46253265017160317, 59.58224293864769550 ) ) ;
#27370=CARTESIAN_POINT ( 'NONE',  ( 8.314922557961029526, -14.29746914071037800, 55.41775706135234714 ) ) ;
#27371=CARTESIAN_POINT ( 'NONE',  ( -5.823673210054431948, 21.52544592524334988, 97.70942372801904696 ) ) ;
#27372=CARTESIAN_POINT ( 'NONE',  ( 16.46253265017146816, 9.564922557961045513, 36.66775706135233293 ) ) ;
#27374=CARTESIAN_POINT ( 'NONE',  ( 5.049401038297881783, 19.05341960407617563, 47.29275706135231161 ) ) ;
#27376=CARTESIAN_POINT ( 'NONE',  ( -5.719274019375665041, -21.55341960407619695, 44.79275706135234714 ) ) ;
#27377=CARTESIAN_POINT ( 'NONE',  ( -0.05219959533909027116, -19.03943276465977164, 22.49890960531436690 ) ) ;
#27378=CARTESIAN_POINT ( 'NONE',  ( 19.02544592524334988, 5.153800228976608722, 46.45942372801899012 ) ) ;
#27379=CARTESIAN_POINT ( 'NONE',  ( 9.564922557960805705, 16.46253265017160317, 104.5822429386476955 ) ) ;
#27380=CARTESIAN_POINT ( 'NONE',  ( -5.049401038298153566, 19.05341960407611168, 80.20724293864769550 ) ) ;
#27381=CARTESIAN_POINT ( 'NONE',  ( 16.55341960407611168, 4.379528057220329451, 38.95724293864768839 ) ) ;
#27382=CARTESIAN_POINT ( 'NONE',  ( -0.05219959533907301413, -21.53943276465977519, 27.49890960531435269 ) ) ;
#27384=CARTESIAN_POINT ( 'NONE',  ( 15.50000000000000178, 5.499999999999998224, 22.00000000000000711 ) ) ;
#27385=CARTESIAN_POINT ( 'NONE',  ( 15.72974639402176855, 15.80617190586768217, 101.8760903946857042 ) ) ;
#27387=CARTESIAN_POINT ( 'NONE',  ( -9.474510206698964154, 16.51473224551069663, 40.41557627198103120 ) ) ;
#27388=FACE_OUTER_BOUND ( 'NONE', #124646, .T. ) ;
#27391=CARTESIAN_POINT ( 'NONE',  ( -16.55341960407617563, 4.379528057220093196, 63.54275706135234003 ) ) ;
#27392=CARTESIAN_POINT ( 'NONE',  ( -10.81492255796078084, -18.62759615963271287, 87.08224293864769550 ) ) ;
#27394=CARTESIAN_POINT ( 'NONE',  ( 16.53943276465976808, -0.05219959533910856209, 38.74890960531435979 ) ) ;
#27395=CARTESIAN_POINT ( 'NONE',  ( -0.05219959533909027116, -19.03943276465977164, 32.49890960531435979 ) ) ;
#27396=CARTESIAN_POINT ( 'NONE',  ( -5.049401038298153566, 19.05341960407611168, 110.2072429386476671 ) ) ;
#27397=CARTESIAN_POINT ( 'NONE',  ( -15.72974639402176322, -15.80617190586768395, 24.37609039468567573 ) ) ;
#27398=CARTESIAN_POINT ( 'NONE',  ( -16.51473224551082808, 9.474510206698731452, 38.33442372801899722 ) ) ;
#27399=CARTESIAN_POINT ( 'NONE',  ( 19.02544592524343514, -5.153800228976328945, 28.54057627198102409 ) ) ;
#27400=CARTESIAN_POINT ( 'NONE',  ( 18.62759615963255655, 10.81492255796105972, 76.66775706135234714 ) ) ;
#27402=CARTESIAN_POINT ( 'NONE',  ( -16.55341960407611168, -4.379528057220339221, 26.45724293864768839 ) ) ;
#27404=CARTESIAN_POINT ( 'NONE',  ( 18.67979575497178502, 10.72451020669898547, 24.16557627198103120 ) ) ;
#27405=CARTESIAN_POINT ( 'NONE',  ( 16.55341960407611168, 4.379528057220329451, 98.95724293864770971 ) ) ;
#27406=CARTESIAN_POINT ( 'NONE',  ( -17.72560187377285246, -5.500000000000055955, 39.07814504131320632 ) ) ;
#27407=CARTESIAN_POINT ( 'NONE',  ( -5.049401038298153566, 19.05341960407611168, 90.20724293864766707 ) ) ;
#27408=CARTESIAN_POINT ( 'NONE',  ( 14.29746914071049879, -8.314922557960816363, 73.33224293864769550 ) ) ;
#27409=CARTESIAN_POINT ( 'NONE',  ( 9.564922557961047289, -16.46253265017146816, 110.4177570613523471 ) ) ;
#27410=CARTESIAN_POINT ( 'NONE',  ( 0.05219959533907565091, 21.53943276465977519, 64.99890960531435269 ) ) ;
#27411=VERTEX_POINT ( 'NONE', #93069 ) ;
#27412=CARTESIAN_POINT ( 'NONE',  ( 9.474510206698971260, -16.51473224551069308, 37.91557627198102409 ) ) ;
#27413=CARTESIAN_POINT ( 'NONE',  ( 19.02544592524343514, -5.153800228976328945, 88.54057627198102409 ) ) ;
#27414=CARTESIAN_POINT ( 'NONE',  ( 21.52544592524344225, -5.823673210054117533, 93.54057627198103830 ) ) ;
#27415=CARTESIAN_POINT ( 'NONE',  ( -14.34966873604972548, 8.224510206698743886, 103.3344237280190043 ) ) ;
#27416=CARTESIAN_POINT ( 'NONE',  ( 9.564922557960805705, 16.46253265017160317, 89.58224293864769550 ) ) ;
#27417=CARTESIAN_POINT ( 'NONE',  ( 16.46253265017146816, 9.564922557961045513, 86.66775706135233293 ) ) ;
#27418=CARTESIAN_POINT ( 'NONE',  ( -18.62759615963255300, -10.81492255796106328, 94.16775706135237556 ) ) ;
#27419=CARTESIAN_POINT ( 'NONE',  ( 21.53943276465977519, -0.05219959533907433946, 78.74890960531436690 ) ) ;
#27420=CARTESIAN_POINT ( 'NONE',  ( -21.53943276465977519, 0.05219959533907696930, 31.24890960531435979 ) ) ;
#27422=CARTESIAN_POINT ( 'NONE',  ( 16.51473224551069308, 9.474510206698969483, 54.16557627198103120 ) ) ;
#27423=CARTESIAN_POINT ( 'NONE',  ( -16.55341960407611168, -4.379528057220339221, 21.45724293864769550 ) ) ;
#27424=CARTESIAN_POINT ( 'NONE',  ( 9.564922557960805705, 16.46253265017160317, 69.58224293864770971 ) ) ;
#27426=CARTESIAN_POINT ( 'NONE',  ( -21.55341960407619339, 5.719274019375674811, 113.5427570613523756 ) ) ;
#27427=CARTESIAN_POINT ( 'NONE',  ( 4.483927247898545687, 16.52544592524342804, 69.79057627198102409 ) ) ;
#27429=CARTESIAN_POINT ( 'NONE',  ( -10.81492255796078084, -18.62759615963271287, 107.0822429386476955 ) ) ;
#27430=CARTESIAN_POINT ( 'NONE',  ( 0.05219959533907565091, 21.53943276465977519, 109.9989096053143527 ) ) ;
#27432=CARTESIAN_POINT ( 'NONE',  ( 10.81492255796078972, 18.62759615963270932, 59.58224293864770260 ) ) ;
#27434=CARTESIAN_POINT ( 'NONE',  ( -4.379528057220086978, -16.55341960407618274, 94.79275706135234714 ) ) ;
#27435=CARTESIAN_POINT ( 'NONE',  ( 8.314922557960818139, 14.29746914071049879, 109.5822429386476955 ) ) ;
#27436=CARTESIAN_POINT ( 'NONE',  ( 5.049401038298161559, -19.05341960407611168, 62.70724293864769550 ) ) ;
#27438=CARTESIAN_POINT ( 'NONE',  ( 4.483927247898545687, 16.52544592524342804, 29.79057627198102409 ) ) ;
#27440=CARTESIAN_POINT ( 'NONE',  ( 15.72974639402176855, 15.80617190586768217, 41.87609039468568284 ) ) ;
#27441=CARTESIAN_POINT ( 'NONE',  ( 19.03943276465977164, -0.05219959533909143690, 103.7489096053143669 ) ) ;
#27442=CARTESIAN_POINT ( 'NONE',  ( 5.823673210054444382, -21.52544592524334988, 75.20942372801901854 ) ) ;
#27443=CARTESIAN_POINT ( 'NONE',  ( -19.02544592524342804, 5.153800228976336051, 26.04057627198103120 ) ) ;
#27444=CARTESIAN_POINT ( 'NONE',  ( 9.564922557960805705, 16.46253265017160317, 39.58224293864768839 ) ) ;
#27446=CARTESIAN_POINT ( 'NONE',  ( -5.719274019375665041, -21.55341960407619695, 79.79275706135236135 ) ) ;
#27447=CARTESIAN_POINT ( 'NONE',  ( -16.53943276465976808, -0.05219959533934237506, 43.75109039468568284 ) ) ;
#27448=CARTESIAN_POINT ( 'NONE',  ( -10.81492255796105439, 18.62759615963255655, 67.91775706135234714 ) ) ;
#27449=CARTESIAN_POINT ( 'NONE',  ( 16.51473224551069308, 9.474510206698969483, 99.16557627198102409 ) ) ;
#27450=CARTESIAN_POINT ( 'NONE',  ( 16.51473224551083163, -9.474510206698727899, 75.83442372801900433 ) ) ;
#27451=CARTESIAN_POINT ( 'NONE',  ( -21.52544592524334988, -5.823673210054445271, 53.95942372801900433 ) ) ;
#27452=CARTESIAN_POINT ( 'NONE',  ( 0.05219959533934541429, -16.53943276465976808, 25.00109039468567218 ) ) ;
#27453=CARTESIAN_POINT ( 'NONE',  ( -9.474510206698720793, -16.51473224551083518, 74.58442372801900433 ) ) ;
#27454=CARTESIAN_POINT ( 'NONE',  ( -5.153800228976328057, -19.02544592524343514, 57.29057627198103120 ) ) ;
#27455=CARTESIAN_POINT ( 'NONE',  ( -13.97604488694547697, 13.89961937509957934, 83.12609039468564731 ) ) ;
#27457=CARTESIAN_POINT ( 'NONE',  ( -16.53943276465976808, 0.05219959533911058130, 26.24890960531435624 ) ) ;
#27458=CARTESIAN_POINT ( 'NONE',  ( -13.97604488694547697, 13.89961937509957934, 93.12609039468566152 ) ) ;
#27459=CARTESIAN_POINT ( 'NONE',  ( 8.224510206698953496, -14.34966873604960469, 37.91557627198102409 ) ) ;
#27460=CARTESIAN_POINT ( 'NONE',  ( 9.564922557961047289, -16.46253265017146816, 60.41775706135233293 ) ) ;
#27461=CARTESIAN_POINT ( 'NONE',  ( -16.52544592524335698, -4.483927247898792601, 43.95942372801902565 ) ) ;
#27462=CARTESIAN_POINT ( 'NONE',  ( -19.02544592524334988, -5.153800228976617603, 28.95942372801900433 ) ) ;
#27463=CARTESIAN_POINT ( 'NONE',  ( 16.46253265017160672, -9.564922557960803928, 43.33224293864769550 ) ) ;
#27464=CARTESIAN_POINT ( 'NONE',  ( 18.87580814761075132, -5.500000000000047073, 73.37172394265759579 ) ) ;
#27465=CARTESIAN_POINT ( 'NONE',  ( -0.05219959533934338120, 16.53943276465976808, 47.50109039468568994 ) ) ;
#27468=CARTESIAN_POINT ( 'NONE',  ( 19.02544592524343514, -5.153800228976328945, 98.54057627198100988 ) ) ;
#27469=CARTESIAN_POINT ( 'NONE',  ( -16.46253265017146816, -9.564922557961047289, 84.16775706135233293 ) ) ;
#27471=CARTESIAN_POINT ( 'NONE',  ( 5.153800228976615827, -19.02544592524334988, 100.2094237280190043 ) ) ;
#27472=CARTESIAN_POINT ( 'NONE',  ( 21.53943276465977519, -0.05219959533907433946, 28.74890960531435624 ) ) ;
#27473=CARTESIAN_POINT ( 'NONE',  ( -5.823673210054431948, 21.52544592524334988, 107.7094237280190328 ) ) ;
#27474=CARTESIAN_POINT ( 'NONE',  ( 19.05341960407617918, -5.049401038297876454, 106.0427570613523471 ) ) ;
#27475=CARTESIAN_POINT ( 'NONE',  ( -16.53943276465976808, 0.05219959533911058130, 111.2489096053143669 ) ) ;
#27476=CARTESIAN_POINT ( 'NONE',  ( -19.03943276465977164, 0.05219959533909376836, 36.24890960531436690 ) ) ;
#27477=CARTESIAN_POINT ( 'NONE',  ( -18.67979575497178146, -10.72451020669898902, 71.66557627198100988 ) ) ;
#27478=CARTESIAN_POINT ( 'NONE',  ( 9.474510206698971260, -16.51473224551069308, 37.91557627198102409 ) ) ;
#27479=CARTESIAN_POINT ( 'NONE',  ( 5.049401038297881783, 19.05341960407617918, 47.29275706135232582 ) ) ;
#27480=CARTESIAN_POINT ( 'NONE',  ( 16.51473224551083163, -9.474510206698727899, 70.83442372801900433 ) ) ;
#27481=CARTESIAN_POINT ( 'NONE',  ( -0.05219959533910754901, -16.53943276465976808, 47.49890960531435979 ) ) ;
#27482=CARTESIAN_POINT ( 'NONE',  ( 5.719274019375991003, -21.55341960407610458, 32.70724293864770260 ) ) ;
#27483=CARTESIAN_POINT ( 'NONE',  ( 18.62759615963255655, 10.81492255796105972, 86.66775706135234714 ) ) ;
#27484=CARTESIAN_POINT ( 'NONE',  ( -10.72451020669898014, 18.67979575497178502, 85.41557627198102409 ) ) ;
#27485=CARTESIAN_POINT ( 'NONE',  ( 21.52544592524334988, 5.823673210054432836, 56.45942372801902565 ) ) ;
#27486=CARTESIAN_POINT ( 'NONE',  ( -10.81492255796105439, 18.62759615963255655, 57.91775706135234714 ) ) ;
#27487=CARTESIAN_POINT ( 'NONE',  ( -19.05341960407611168, -5.049401038298163336, 96.45724293864769550 ) ) ;
#27488=CARTESIAN_POINT ( 'NONE',  ( -16.55341960407617563, 4.379528057220093196, 93.54275706135234714 ) ) ;
#27489=CARTESIAN_POINT ( 'NONE',  ( 10.81492255796106328, -18.62759615963255655, 60.41775706135235424 ) ) ;
#27490=CARTESIAN_POINT ( 'NONE',  ( -16.46253265017160317, 9.564922557960807481, 55.83224293864769550 ) ) ;
#27491=CARTESIAN_POINT ( 'NONE',  ( 9.474510206698971260, -16.51473224551069308, 27.91557627198103120 ) ) ;
#27492=CARTESIAN_POINT ( 'NONE',  ( -16.51473224551069308, -9.474510206698971260, 51.66557627198102409 ) ) ;
#27494=CARTESIAN_POINT ( 'NONE',  ( 16.52544592524342804, -4.483927247898539470, 63.54057627198103830 ) ) ;
#27495=CARTESIAN_POINT ( 'NONE',  ( 12.14591786802309770, 12.06949235617756955, 34.37390960531435979 ) ) ;
#27496=CARTESIAN_POINT ( 'NONE',  ( 5.719274019375991003, -21.55341960407610458, 42.70724293864770260 ) ) ;
#27497=CARTESIAN_POINT ( 'NONE',  ( 19.03943276465977164, -0.05219959533909143690, 53.74890960531436690 ) ) ;
#27498=CARTESIAN_POINT ( 'NONE',  ( 15.80617190586746368, 15.72974639402197994, 64.37390960531435269 ) ) ;
#27499=CARTESIAN_POINT ( 'NONE',  ( 19.02544592524334988, 5.153800228976608722, 51.45942372801900433 ) ) ;
#27501=CARTESIAN_POINT ( 'NONE',  ( 12.14591786802309770, 12.06949235617756955, 49.37390960531436690 ) ) ;
#27502=CARTESIAN_POINT ( 'NONE',  ( 21.52544592524344225, -5.823673210054117533, 33.54057627198102409 ) ) ;
#27504=ORIENTED_EDGE ( 'NONE', *, *, #125615, .F. ) ;
#27505=CARTESIAN_POINT ( 'NONE',  ( 16.81555441253553340, 7.025013491695490941, 101.8631455466574494 ) ) ;
#27506=CARTESIAN_POINT ( 'NONE',  ( 14.29746914071037800, 8.314922557961029526, 91.66775706135234714 ) ) ;
#27507=EDGE_CURVE ( 'NONE', #155869, #16989, #146558, .T. ) ;
#27508=CARTESIAN_POINT ( 'NONE',  ( -13.89961937509957401, -13.97604488694547875, 69.37609039468564731 ) ) ;
#27509=CARTESIAN_POINT ( 'NONE',  ( 16.55341960407611168, 4.379528057220329451, 48.95724293864770971 ) ) ;
#27510=CARTESIAN_POINT ( 'NONE',  ( 17.44279575226827816, -5.990770900252369913, 53.33557567514319686 ) ) ;
#27511=CARTESIAN_POINT ( 'NONE',  ( -12.14591786802309592, -12.06949235617757132, 36.87390960531435979 ) ) ;
#27512=CARTESIAN_POINT ( 'NONE',  ( 13.97604488694527802, 13.89961937509977652, 49.37390960531434558 ) ) ;
#27513=CARTESIAN_POINT ( 'NONE',  ( 19.05341960407611168, 5.049401038298154454, 68.95724293864769550 ) ) ;
#27514=CARTESIAN_POINT ( 'NONE',  ( -19.02544592524342804, 5.153800228976336051, 36.04057627198100988 ) ) ;
#27515=CARTESIAN_POINT ( 'NONE',  ( -21.53943276465977519, -0.05219959533937600094, 48.75109039468568284 ) ) ;
#27516=CARTESIAN_POINT ( 'NONE',  ( -0.05219959533909027116, -19.03943276465977164, 72.49890960531435269 ) ) ;
#27517=CARTESIAN_POINT ( 'NONE',  ( 9.474510206698971260, -16.51473224551069308, 22.91557627198102765 ) ) ;
#27518=CARTESIAN_POINT ( 'NONE',  ( 19.05341960407611168, 5.049401038298154454, 53.95724293864770260 ) ) ;
#27519=CARTESIAN_POINT ( 'NONE',  ( -21.55341960407610458, -5.719274019375992779, 46.45724293864769550 ) ) ;
#27520=CARTESIAN_POINT ( 'NONE',  ( -9.564922557960796823, -16.46253265017161027, 37.08224293864768839 ) ) ;
#27521=CARTESIAN_POINT ( 'NONE',  ( -0.05219959533907301413, -21.53943276465977519, 37.49890960531436690 ) ) ;
#27522=CARTESIAN_POINT ( 'NONE',  ( 16.52544592524335698, 4.483927247898782831, 106.4594237280190328 ) ) ;
#27523=CARTESIAN_POINT ( 'NONE',  ( -18.67979575497193778, 10.72451020669871902, 113.3344237280190328 ) ) ;
#27524=CARTESIAN_POINT ( 'NONE',  ( -14.34966873604972548, 8.224510206698743886, 48.33442372801902565 ) ) ;
#27525=CARTESIAN_POINT ( 'NONE',  ( -8.224510206698735004, -14.34966873604973081, 74.58442372801901854 ) ) ;
#27527=CARTESIAN_POINT ( 'NONE',  ( -12.14591786802326823, 12.06949235617739902, 63.12609039468568994 ) ) ;
#27528=CARTESIAN_POINT ( 'NONE',  ( -4.483927247898782831, 16.52544592524335698, 37.70942372801900433 ) ) ;
#27529=CARTESIAN_POINT ( 'NONE',  ( 16.46253265017160672, -9.564922557960803928, 103.3322429386476955 ) ) ;
#27530=CARTESIAN_POINT ( 'NONE',  ( -16.53943276465976808, -0.05219959533934237506, 28.75109039468567929 ) ) ;
#27531=CARTESIAN_POINT ( 'NONE',  ( 13.97604488694527802, 13.89961937509977652, 29.37390960531435979 ) ) ;
#27532=CARTESIAN_POINT ( 'NONE',  ( 10.81492255796106328, -18.62759615963255655, 30.41775706135234358 ) ) ;
#27533=CARTESIAN_POINT ( 'NONE',  ( -16.52544592524335698, -4.483927247898792601, 33.95942372801901143 ) ) ;
#27534=CARTESIAN_POINT ( 'NONE',  ( 14.34966873604972726, -8.224510206698740333, 95.83442372801903275 ) ) ;
#27535=DIRECTION ( 'NONE',  ( 0.000000000000000000, 0.000000000000000000, -1.000000000000000000 ) ) ;
#27536=CARTESIAN_POINT ( 'NONE',  ( -15.72974639402176322, -15.80617190586768395, 99.37609039468568994 ) ) ;
#27537=CARTESIAN_POINT ( 'NONE',  ( -19.03943276465977164, -0.05219959533935918106, 93.75109039468566152 ) ) ;
#27538=CARTESIAN_POINT ( 'NONE',  ( 12.06949235617757843, -12.14591786802309237, 63.12390960531435979 ) ) ;
#27539=CARTESIAN_POINT ( 'NONE',  ( 5.049401038298161559, -19.05341960407611168, 22.70724293864769194 ) ) ;
#27540=CARTESIAN_POINT ( 'NONE',  ( 13.89961937509957401, 13.97604488694547697, 61.87609039468566863 ) ) ;
#27541=CARTESIAN_POINT ( 'NONE',  ( 16.79531203550645913, 7.028104445595632299, 78.75244988220443076 ) ) ;
#27542=CARTESIAN_POINT ( 'NONE',  ( -18.62759615963255300, -10.81492255796106328, 69.16775706135234714 ) ) ;
#27543=CARTESIAN_POINT ( 'NONE',  ( 8.314922557961029526, -14.29746914071037800, 25.41775706135235779 ) ) ;
#27545=CARTESIAN_POINT ( 'NONE',  ( 21.53943276465977519, -0.05219959533907433946, 28.74890960531435624 ) ) ;
#27546=CARTESIAN_POINT ( 'NONE',  ( -10.81492255796078084, -18.62759615963271287, 72.08224293864769550 ) ) ;
#27547=CARTESIAN_POINT ( 'NONE',  ( -19.03943276465977164, -0.05219959533935918106, 103.7510903946856757 ) ) ;
#27548=CARTESIAN_POINT ( 'NONE',  ( 19.05341960407611168, 5.049401038298154454, 103.9572429386476671 ) ) ;
#27550=CARTESIAN_POINT ( 'NONE',  ( 19.02544592524343514, -5.153800228976328945, 28.54057627198102409 ) ) ;
#27551=CARTESIAN_POINT ( 'NONE',  ( -5.823673210054431948, 21.52544592524334988, 107.7094237280190328 ) ) ;
#27552=CARTESIAN_POINT ( 'NONE',  ( -13.97604488694527625, -13.89961937509977652, 46.87390960531435979 ) ) ;
#27554=CARTESIAN_POINT ( 'NONE',  ( 0.05219959533937995610, -21.53943276465977519, 50.00109039468568994 ) ) ;
#27555=CARTESIAN_POINT ( 'NONE',  ( 21.52544592524334988, 5.823673210054432836, 91.45942372801901854 ) ) ;
#27556=CARTESIAN_POINT ( 'NONE',  ( -12.14591786802326823, 12.06949235617739902, 103.1260903946856757 ) ) ;
#27557=CARTESIAN_POINT ( 'NONE',  ( 0.05219959533909260263, 19.03943276465977164, 79.99890960531436690 ) ) ;
#27558=CARTESIAN_POINT ( 'NONE',  ( 15.80617190586769283, -15.72974639402175789, 40.62609039468567573 ) ) ;
#27559=CARTESIAN_POINT ( 'NONE',  ( -10.72451020669870658, -18.67979575497194134, 54.58442372801901143 ) ) ;
#27560=CARTESIAN_POINT ( 'NONE',  ( -5.049401038297874678, -19.05341960407617918, 74.79275706135231871 ) ) ;
#27561=CARTESIAN_POINT ( 'NONE',  ( 19.05341960407611168, 5.049401038298154454, 98.95724293864766707 ) ) ;
#27562=CARTESIAN_POINT ( 'NONE',  ( -14.29746914071049879, 8.314922557960819915, 100.8322429386477097 ) ) ;
#27563=CARTESIAN_POINT ( 'NONE',  ( -15.72974639402197994, 15.80617190586746368, 100.6239096053143811 ) ) ;
#27564=CARTESIAN_POINT ( 'NONE',  ( -16.53943276465976808, 0.05219959533911058130, 71.24890960531435269 ) ) ;
#27565=CARTESIAN_POINT ( 'NONE',  ( 5.153800228976615827, -19.02544592524334988, 25.20942372801900433 ) ) ;
#27566=CARTESIAN_POINT ( 'NONE',  ( -14.29746914071049879, 8.314922557960819915, 100.8322429386477097 ) ) ;
#27567=CARTESIAN_POINT ( 'NONE',  ( 9.564922557960805705, 16.46253265017160317, 49.58224293864770260 ) ) ;
#27568=CARTESIAN_POINT ( 'NONE',  ( 5.153800228976615827, -19.02544592524334988, 90.20942372801900433 ) ) ;
#27570=CARTESIAN_POINT ( 'NONE',  ( 8.224510206698953496, -14.34966873604960469, 47.91557627198102409 ) ) ;
#27571=CARTESIAN_POINT ( 'NONE',  ( -9.474510206698720793, -16.51473224551083518, 19.58442372801899722 ) ) ;
#27572=CARTESIAN_POINT ( 'NONE',  ( 5.049401038298161559, -19.05341960407611168, 102.7072429386476955 ) ) ;
#27573=CARTESIAN_POINT ( 'NONE',  ( -19.05341960407617563, 5.049401038297882671, 73.54275706135233293 ) ) ;
#27574=CARTESIAN_POINT ( 'NONE',  ( 21.53943276465977519, -0.05219959533907433946, 78.74890960531436690 ) ) ;
#27575=VECTOR ( 'NONE', #139496, 999.9999999999998863 ) ;
#27576=CARTESIAN_POINT ( 'NONE',  ( 0.05219959533937995610, -21.53943276465977519, 35.00109039468568284 ) ) ;
#27577=CARTESIAN_POINT ( 'NONE',  ( 16.55341960407618274, -4.379528057220086978, 26.04275706135235779 ) ) ;
#27578=CARTESIAN_POINT ( 'NONE',  ( -14.34966873604972548, 8.224510206698743886, 93.33442372801901854 ) ) ;
#27579=CARTESIAN_POINT ( 'NONE',  ( 17.13100169013300089, 6.664070546373172199, 61.73210164300152059 ) ) ;
#27580=CARTESIAN_POINT ( 'NONE',  ( 21.55341960407619695, -5.719274019375665929, 31.04275706135234714 ) ) ;
#27581=CARTESIAN_POINT ( 'NONE',  ( 14.29746914071049879, -8.314922557960816363, 113.3322429386476955 ) ) ;
#27583=CARTESIAN_POINT ( 'NONE',  ( -14.34966873604972548, 8.224510206698743886, 68.33442372801900433 ) ) ;
#27584=CARTESIAN_POINT ( 'NONE',  ( 8.314922557960818139, 14.29746914071049879, 94.58224293864769550 ) ) ;
#27585=CARTESIAN_POINT ( 'NONE',  ( 21.52544592524344225, -5.823673210054117533, 78.54057627198103830 ) ) ;
#27586=CARTESIAN_POINT ( 'NONE',  ( 16.52544592524342804, -4.483927247898539470, 23.54057627198102765 ) ) ;
#27587=CARTESIAN_POINT ( 'NONE',  ( -8.224510206698735004, -14.34966873604973081, 54.58442372801901143 ) ) ;
#27588=CARTESIAN_POINT ( 'NONE',  ( -16.51473224551069308, -9.474510206698971260, 51.66557627198102409 ) ) ;
#27589=CARTESIAN_POINT ( 'NONE',  ( 16.53943276465976808, 0.05219959533934440121, 91.25109039468568994 ) ) ;
#27590=CARTESIAN_POINT ( 'NONE',  ( -19.02544592524334988, -5.153800228976617603, 88.95942372801897591 ) ) ;
#27591=CARTESIAN_POINT ( 'NONE',  ( -15.80617190586745835, -15.72974639402198527, 91.87390960531436690 ) ) ;
#27592=CARTESIAN_POINT ( 'NONE',  ( -14.29746914071037622, -8.314922557961029526, 109.1677570613523613 ) ) ;
#27593=ORIENTED_EDGE ( 'NONE', *, *, #6630, .F. ) ;
#27595=CARTESIAN_POINT ( 'NONE',  ( 5.719274019375991003, -21.55341960407610458, 57.70724293864770260 ) ) ;
#27597=CARTESIAN_POINT ( 'NONE',  ( -12.14591786802326823, 12.06949235617739902, 88.12609039468570415 ) ) ;
#27599=CARTESIAN_POINT ( 'NONE',  ( 15.80617190586746368, 15.72974639402197994, 24.37390960531435979 ) ) ;
#27600=CARTESIAN_POINT ( 'NONE',  ( 17.50000000000000711, 5.068104630630374530, 106.7718159465997303 ) ) ;
#27601=CARTESIAN_POINT ( 'NONE',  ( 0.05219959533907565091, 21.53943276465977519, 79.99890960531435269 ) ) ;
#27602=CARTESIAN_POINT ( 'NONE',  ( 16.53943276465976808, -0.05219959533910856209, 28.74890960531435624 ) ) ;
#27603=CARTESIAN_POINT ( 'NONE',  ( 16.55341960407618274, -4.379528057220086978, 26.04275706135235779 ) ) ;
#27604=CARTESIAN_POINT ( 'NONE',  ( -9.474510206698964154, 16.51473224551069663, 40.41557627198103120 ) ) ;
#27605=CARTESIAN_POINT ( 'NONE',  ( -8.224510206698735004, -14.34966873604973081, 29.58442372801901854 ) ) ;
#27606=CARTESIAN_POINT ( 'NONE',  ( 9.474510206698971260, -16.51473224551069308, 57.91557627198103120 ) ) ;
#27608=CARTESIAN_POINT ( 'NONE',  ( -9.474510206698964154, 16.51473224551069663, 105.4155762719810383 ) ) ;
#27609=CARTESIAN_POINT ( 'NONE',  ( 5.049401038298161559, -19.05341960407611168, 107.7072429386476955 ) ) ;
#27610=CARTESIAN_POINT ( 'NONE',  ( 8.224510206698742110, 14.34966873604972548, 87.08442372801901854 ) ) ;
#27611=CARTESIAN_POINT ( 'NONE',  ( -9.474510206698720793, -16.51473224551083518, 89.58442372801900433 ) ) ;
#27612=CARTESIAN_POINT ( 'NONE',  ( 0.05219959533936267826, -19.03943276465977164, 35.00109039468566863 ) ) ;
#27613=CARTESIAN_POINT ( 'NONE',  ( -15.72974639402197994, 15.80617190586746368, 70.62390960531436690 ) ) ;
#27615=CARTESIAN_POINT ( 'NONE',  ( 8.224510206698742110, 14.34966873604972548, 97.08442372801904696 ) ) ;
#27616=CARTESIAN_POINT ( 'NONE',  ( 15.80617190586746368, 15.72974639402197994, 39.37390960531436690 ) ) ;
#27617=CARTESIAN_POINT ( 'NONE',  ( 13.89961937509957401, 13.97604488694547697, 86.87609039468567573 ) ) ;
#27618=CARTESIAN_POINT ( 'NONE',  ( -19.02544592524342804, 5.153800228976336051, 46.04057627198101699 ) ) ;
#27619=CARTESIAN_POINT ( 'NONE',  ( 19.03943276465977164, -0.05219959533909143690, 88.74890960531436690 ) ) ;
#27620=CARTESIAN_POINT ( 'NONE',  ( -10.72451020669870658, -18.67979575497194134, 64.58442372801900433 ) ) ;
#27621=CARTESIAN_POINT ( 'NONE',  ( -19.03943276465977164, 0.05219959533909376836, 56.24890960531435979 ) ) ;
#27622=CARTESIAN_POINT ( 'NONE',  ( 8.224510206698953496, -14.34966873604960469, 97.91557627198103830 ) ) ;
#27623=CARTESIAN_POINT ( 'NONE',  ( -17.05587630539786659, -6.762274262135685277, 84.25819690962686082 ) ) ;
#27624=CARTESIAN_POINT ( 'NONE',  ( 16.55341960407611168, 4.379528057220329451, 73.95724293864769550 ) ) ;
#27625=CARTESIAN_POINT ( 'NONE',  ( 5.719274019375991003, -21.55341960407610458, 67.70724293864769550 ) ) ;
#27626=CARTESIAN_POINT ( 'NONE',  ( 19.02544592524334988, 5.153800228976608722, 96.45942372801897591 ) ) ;
#27628=CARTESIAN_POINT ( 'NONE',  ( -13.97604488694527625, -13.89961937509977652, 61.87390960531435979 ) ) ;
#27630=CARTESIAN_POINT ( 'NONE',  ( -5.049401038298153566, 19.05341960407611168, 80.20724293864769550 ) ) ;
#27631=CARTESIAN_POINT ( 'NONE',  ( -19.03943276465977164, 0.05219959533909376836, 81.24890960531436690 ) ) ;
#27632=CARTESIAN_POINT ( 'NONE',  ( -4.379528057220086978, -16.55341960407618274, 69.79275706135234714 ) ) ;
#27633=CARTESIAN_POINT ( 'NONE',  ( -16.88567814943163725, -6.947325034625594142, 51.29001122652586986 ) ) ;
#27634=CARTESIAN_POINT ( 'NONE',  ( 9.564922557961047289, -16.46253265017146816, 45.41775706135232582 ) ) ;
#27636=CARTESIAN_POINT ( 'NONE',  ( 5.153800228976335163, 19.02544592524342804, 109.7905762719810099 ) ) ;
#27637=CARTESIAN_POINT ( 'NONE',  ( -14.34966873604972548, 8.224510206698743886, 108.3344237280190185 ) ) ;
#27639=CARTESIAN_POINT ( 'NONE',  ( -14.29746914071037622, -8.314922557961029526, 84.16775706135234714 ) ) ;
#27641=CARTESIAN_POINT ( 'NONE',  ( 0.05219959533934541429, -16.53943276465976808, 50.00109039468568994 ) ) ;
#27643=CARTESIAN_POINT ( 'NONE',  ( -21.52544592524334988, -5.823673210054445271, 63.95942372801901854 ) ) ;
#27644=CARTESIAN_POINT ( 'NONE',  ( -0.05219959533936034679, 19.03943276465977164, 77.50109039468566152 ) ) ;
#27645=CARTESIAN_POINT ( 'NONE',  ( 19.03943276465977164, 0.05219959533936151252, 31.25109039468566863 ) ) ;
#27647=CARTESIAN_POINT ( 'NONE',  ( 0.05219959533909260263, 19.03943276465977164, 69.99890960531435269 ) ) ;
#27648=CARTESIAN_POINT ( 'NONE',  ( 16.46253265017160672, -9.564922557960803928, 48.33224293864769550 ) ) ;
#27649=CARTESIAN_POINT ( 'NONE',  ( 17.08558671903228188, -6.726026106045698505, 23.25235570636825955 ) ) ;
#27650=CARTESIAN_POINT ( 'NONE',  ( 5.719274019375991003, -21.55341960407610458, 67.70724293864769550 ) ) ;
#27651=CARTESIAN_POINT ( 'NONE',  ( 5.719274019375991003, -21.55341960407610458, 37.70724293864769550 ) ) ;
#27652=CARTESIAN_POINT ( 'NONE',  ( 16.53943276465976808, -0.05219959533910856209, 108.7489096053143669 ) ) ;
#27653=CARTESIAN_POINT ( 'NONE',  ( 14.29746914071037800, 8.314922557961029526, 46.66775706135234714 ) ) ;
#27655=CARTESIAN_POINT ( 'NONE',  ( -5.823673210054431948, 21.52544592524334988, 37.70942372801900433 ) ) ;
#27656=CARTESIAN_POINT ( 'NONE',  ( 16.53943276465976808, -0.05219959533910856209, 48.74890960531435979 ) ) ;
#27658=CARTESIAN_POINT ( 'NONE',  ( 14.29746914071037800, 8.314922557961029526, 31.66775706135234358 ) ) ;
#27659=CARTESIAN_POINT ( 'NONE',  ( -0.05219959533936034679, 19.03943276465977164, 37.50109039468567573 ) ) ;
#27660=CARTESIAN_POINT ( 'NONE',  ( 4.483927247898545687, 16.52544592524342804, 44.79057627198103120 ) ) ;
#27661=CARTESIAN_POINT ( 'NONE',  ( -15.72974639402176322, -15.80617190586768395, 24.37609039468567573 ) ) ;
#27662=CARTESIAN_POINT ( 'NONE',  ( -16.46253265017160317, 9.564922557960807481, 100.8322429386477097 ) ) ;
#27663=CARTESIAN_POINT ( 'NONE',  ( 0.05219959533907565091, 21.53943276465977519, 79.99890960531435269 ) ) ;
#27664=CARTESIAN_POINT ( 'NONE',  ( -16.46253265017160317, 9.564922557960807481, 90.83224293864769550 ) ) ;
#27665=CARTESIAN_POINT ( 'NONE',  ( -14.29746914071049879, 8.314922557960819915, 60.83224293864769550 ) ) ;
#27666=CARTESIAN_POINT ( 'NONE',  ( -0.05219959533909027116, -19.03943276465977164, 97.49890960531436690 ) ) ;
#27668=CARTESIAN_POINT ( 'NONE',  ( -16.51473224551082808, 9.474510206698731452, 73.33442372801900433 ) ) ;
#27669=CARTESIAN_POINT ( 'NONE',  ( -21.52544592524343514, 5.823673210054127303, 101.0405762719810383 ) ) ;
#27670=CARTESIAN_POINT ( 'NONE',  ( 5.049401038298161559, -19.05341960407611168, 62.70724293864769550 ) ) ;
#27671=CARTESIAN_POINT ( 'NONE',  ( 0.05219959533910956823, 16.53943276465976808, 114.9989096053143669 ) ) ;
#27672=CARTESIAN_POINT ( 'NONE',  ( -15.80617190586768217, 15.72974639402176855, 53.12609039468568284 ) ) ;
#27674=CARTESIAN_POINT ( 'NONE',  ( -4.379528057220328563, 16.55341960407611168, 40.20724293864769550 ) ) ;
#27675=CARTESIAN_POINT ( 'NONE',  ( 0.05219959533909260263, 19.03943276465977164, 44.99890960531435979 ) ) ;
#27676=CARTESIAN_POINT ( 'NONE',  ( 9.564922557960805705, 16.46253265017160317, 99.58224293864770971 ) ) ;
#27677=CARTESIAN_POINT ( 'NONE',  ( -15.80617190586745835, -15.72974639402198527, 76.87390960531439532 ) ) ;
#27679=CARTESIAN_POINT ( 'NONE',  ( 16.46253265017160672, -9.564922557960803928, 38.33224293864768839 ) ) ;
#27680=CARTESIAN_POINT ( 'NONE',  ( -21.53943276465977519, 0.05219959533907696930, 61.24890960531435979 ) ) ;
#27681=CARTESIAN_POINT ( 'NONE',  ( 18.62759615963255655, 10.81492255796105972, 91.66775706135234714 ) ) ;
#27683=CARTESIAN_POINT ( 'NONE',  ( 8.314922557961029526, -14.29746914071037800, 85.41775706135236135 ) ) ;
#27684=CARTESIAN_POINT ( 'NONE',  ( -4.379528057220328563, 16.55341960407611168, 85.20724293864770971 ) ) ;
#27685=CARTESIAN_POINT ( 'NONE',  ( 13.89961937509977652, -13.97604488694527269, 68.12390960531436690 ) ) ;
#27687=CARTESIAN_POINT ( 'NONE',  ( 19.03943276465977164, 0.05219959533936151252, 21.25109039468565797 ) ) ;
#27688=CARTESIAN_POINT ( 'NONE',  ( -16.55341960407617563, 4.379528057220093196, 93.54275706135234714 ) ) ;
#27689=CARTESIAN_POINT ( 'NONE',  ( 15.72974639402176855, 15.80617190586768217, 106.8760903946856899 ) ) ;
#27690=CARTESIAN_POINT ( 'NONE',  ( 19.02544592524343514, -5.153800228976328945, 88.54057627198102409 ) ) ;
#27691=CARTESIAN_POINT ( 'NONE',  ( -18.62759615963270932, 10.81492255796079327, 50.83224293864770971 ) ) ;
#27692=CARTESIAN_POINT ( 'NONE',  ( 21.52544592524334988, 5.823673210054432836, 91.45942372801901854 ) ) ;
#27693=CARTESIAN_POINT ( 'NONE',  ( 8.224510206698742110, 14.34966873604972548, 57.08442372801901854 ) ) ;
#27694=CARTESIAN_POINT ( 'NONE',  ( 21.55341960407619695, -5.719274019375665929, 21.04275706135234714 ) ) ;
#27695=CARTESIAN_POINT ( 'NONE',  ( -8.224510206698735004, -14.34966873604973081, 29.58442372801901854 ) ) ;
#27696=CARTESIAN_POINT ( 'NONE',  ( -5.049401038298153566, 19.05341960407611168, 95.20724293864770971 ) ) ;
#27697=CARTESIAN_POINT ( 'NONE',  ( -8.224510206698735004, -14.34966873604973081, 34.58442372801900433 ) ) ;
#27698=CARTESIAN_POINT ( 'NONE',  ( -13.97604488694527625, -13.89961937509977652, 46.87390960531435979 ) ) ;
#27699=CARTESIAN_POINT ( 'NONE',  ( -0.05219959533934338120, 16.53943276465976808, 27.50109039468567929 ) ) ;
#27700=CARTESIAN_POINT ( 'NONE',  ( 16.52544592524342804, -4.483927247898539470, 83.54057627198102409 ) ) ;
#27701=CARTESIAN_POINT ( 'NONE',  ( 8.224510206698742110, 14.34966873604972548, 92.08442372801901854 ) ) ;
#27702=CARTESIAN_POINT ( 'NONE',  ( 10.81492255796106328, -18.62759615963255655, 45.41775706135234003 ) ) ;
#27703=CARTESIAN_POINT ( 'NONE',  ( 13.97604488694527802, 13.89961937509977652, 64.37390960531436690 ) ) ;
#27704=CARTESIAN_POINT ( 'NONE',  ( -5.153800228976328057, -19.02544592524343514, 82.29057627198103830 ) ) ;
#27706=CARTESIAN_POINT ( 'NONE',  ( 16.53943276465976808, -0.05219959533910856209, 28.74890960531435624 ) ) ;
#27707=CARTESIAN_POINT ( 'NONE',  ( -8.224510206698735004, -14.34966873604973081, 79.58442372801903275 ) ) ;
#27709=CARTESIAN_POINT ( 'NONE',  ( -5.153800228976607833, 19.02544592524334988, 32.70942372801899722 ) ) ;
#27710=CARTESIAN_POINT ( 'NONE',  ( 19.05341960407611168, 5.049401038298154454, 98.95724293864766707 ) ) ;
#27711=CARTESIAN_POINT ( 'NONE',  ( 5.153800228976335163, 19.02544592524342804, 54.79057627198103120 ) ) ;
#27713=CARTESIAN_POINT ( 'NONE',  ( -16.52544592524335698, -4.483927247898792601, 43.95942372801902565 ) ) ;
#27714=CARTESIAN_POINT ( 'NONE',  ( -13.89961937509957401, -13.97604488694547875, 64.37609039468567573 ) ) ;
#27715=CARTESIAN_POINT ( 'NONE',  ( 8.314922557961029526, -14.29746914071037800, 60.41775706135235424 ) ) ;
#27717=CARTESIAN_POINT ( 'NONE',  ( -19.02544592524342804, 5.153800228976336051, 76.04057627198102409 ) ) ;
#27718=CARTESIAN_POINT ( 'NONE',  ( 21.55341960407610458, 5.719274019375980345, 108.9572429386476955 ) ) ;
#27719=CARTESIAN_POINT ( 'NONE',  ( -0.05219959533936034679, 19.03943276465977164, 62.50109039468566863 ) ) ;
#27720=CARTESIAN_POINT ( 'NONE',  ( -13.89961937509977652, 13.97604488694528158, 100.6239096053143669 ) ) ;
#27721=CARTESIAN_POINT ( 'NONE',  ( -13.89961937509977652, 13.97604488694528158, 25.62390960531434558 ) ) ;
#27722=CARTESIAN_POINT ( 'NONE',  ( 0.05219959533909260263, 19.03943276465977164, 79.99890960531436690 ) ) ;
#27723=CARTESIAN_POINT ( 'NONE',  ( -4.483927247898539470, -16.52544592524342804, 32.29057627198102409 ) ) ;
#27724=CARTESIAN_POINT ( 'NONE',  ( 22.00000000000000000, -1.163414459189985801E-14, 95.00000000000000000 ) ) ;
#27725=CARTESIAN_POINT ( 'NONE',  ( 16.46253265017146816, 9.564922557961045513, 31.66775706135232937 ) ) ;
#27726=CARTESIAN_POINT ( 'NONE',  ( -4.379528057220328563, 16.55341960407611168, 70.20724293864769550 ) ) ;
#27727=CARTESIAN_POINT ( 'NONE',  ( -18.67979575497193778, 10.72451020669871902, 113.3344237280190328 ) ) ;
#27728=CARTESIAN_POINT ( 'NONE',  ( 19.05341960407611168, 5.049401038298154454, 33.95724293864769550 ) ) ;
#27729=CARTESIAN_POINT ( 'NONE',  ( 16.55341960407611168, 4.379528057220329451, 43.95724293864769550 ) ) ;
#27730=CARTESIAN_POINT ( 'NONE',  ( -18.62759615963255300, -10.81492255796106328, 109.1677570613523613 ) ) ;
#27731=CARTESIAN_POINT ( 'NONE',  ( 9.474510206698971260, -16.51473224551069308, 87.91557627198102409 ) ) ;
#27732=CARTESIAN_POINT ( 'NONE',  ( -13.89961937509977652, 13.97604488694528158, 110.6239096053143243 ) ) ;
#27733=CARTESIAN_POINT ( 'NONE',  ( 0.05219959533909260263, 19.03943276465977164, 39.99890960531436690 ) ) ;
#27734=CARTESIAN_POINT ( 'NONE',  ( 16.53943276465976808, -0.05219959533910856209, 113.7489096053143527 ) ) ;
#27735=CARTESIAN_POINT ( 'NONE',  ( -8.224510206698948167, 14.34966873604960824, 70.41557627198102409 ) ) ;
#27736=CARTESIAN_POINT ( 'NONE',  ( 10.81492255796078972, 18.62759615963270932, 84.58224293864769550 ) ) ;
#27737=CARTESIAN_POINT ( 'NONE',  ( -5.153800228976328057, -19.02544592524343514, 92.29057627198099567 ) ) ;
#27738=CARTESIAN_POINT ( 'NONE',  ( 10.72451020669898902, -18.67979575497178502, 92.91557627198103830 ) ) ;
#27739=CARTESIAN_POINT ( 'NONE',  ( -16.46253265017160317, 9.564922557960807481, 85.83224293864769550 ) ) ;
#27741=CARTESIAN_POINT ( 'NONE',  ( -18.39639308325438805, -5.499999999999988454, 91.48252246182197212 ) ) ;
#27742=CARTESIAN_POINT ( 'NONE',  ( -4.483927247898539470, -16.52544592524342804, 102.2905762719810383 ) ) ;
#27743=CARTESIAN_POINT ( 'NONE',  ( 16.46253265017160672, -9.564922557960803928, 68.33224293864770971 ) ) ;
#27744=CARTESIAN_POINT ( 'NONE',  ( 10.72451020669898902, -18.67979575497178502, 82.91557627198103830 ) ) ;
#27746=CARTESIAN_POINT ( 'NONE',  ( 10.81492255796078972, 18.62759615963270932, 29.58224293864769905 ) ) ;
#27747=DIRECTION ( 'NONE',  ( 1.000000000000000000, -0.000000000000000000, -0.000000000000000000 ) ) ;
#27748=CARTESIAN_POINT ( 'NONE',  ( -4.483927247898782831, 16.52544592524335698, 22.70942372801901499 ) ) ;
#27749=CARTESIAN_POINT ( 'NONE',  ( -0.05219959533910754901, -16.53943276465976808, 92.49890960531436690 ) ) ;
#27750=CARTESIAN_POINT ( 'NONE',  ( -16.19135201231365784, -7.376712067591944866, 95.18680854052031748 ) ) ;
#27751=CARTESIAN_POINT ( 'NONE',  ( -13.97604488694527625, -13.89961937509977652, 81.87390960531436690 ) ) ;
#27752=CARTESIAN_POINT ( 'NONE',  ( -19.03943276465977164, 0.05219959533909376836, 46.24890960531435979 ) ) ;
#27753=CARTESIAN_POINT ( 'NONE',  ( -12.14591786802309592, -12.06949235617757132, 86.87390960531438111 ) ) ;
#27754=CARTESIAN_POINT ( 'NONE',  ( 18.62759615963271287, -10.81492255796078972, 23.33224293864769194 ) ) ;
#27755=CARTESIAN_POINT ( 'NONE',  ( -12.06949235617756955, 12.14591786802309770, 50.62390960531435979 ) ) ;
#27756=CARTESIAN_POINT ( 'NONE',  ( 19.05341960407617918, -5.049401038297876454, 96.04275706135231871 ) ) ;
#27757=CARTESIAN_POINT ( 'NONE',  ( 21.55341960407619695, -5.719274019375665929, 66.04275706135236135 ) ) ;
#27759=CARTESIAN_POINT ( 'NONE',  ( 13.97604488694527802, 13.89961937509977652, 94.37390960531436690 ) ) ;
#27760=CARTESIAN_POINT ( 'NONE',  ( 10.81492255796078972, 18.62759615963270932, 89.58224293864768129 ) ) ;
#27761=CARTESIAN_POINT ( 'NONE',  ( -14.34966873604972548, 8.224510206698743886, 88.33442372801901854 ) ) ;
#27762=CARTESIAN_POINT ( 'NONE',  ( 19.03943276465977164, -0.05219959533909143690, 28.74890960531435624 ) ) ;
#27763=CARTESIAN_POINT ( 'NONE',  ( -5.153800228976328057, -19.02544592524343514, 82.29057627198103830 ) ) ;
#27764=CARTESIAN_POINT ( 'NONE',  ( 10.81492255796078972, 18.62759615963270932, 84.58224293864769550 ) ) ;
#27765=CARTESIAN_POINT ( 'NONE',  ( -9.474510206698720793, -16.51473224551083518, 104.5844237280190043 ) ) ;
#27766=CARTESIAN_POINT ( 'NONE',  ( -14.34966873604960291, -8.224510206698953496, 51.66557627198102409 ) ) ;
#27767=CARTESIAN_POINT ( 'NONE',  ( -5.719274019375665041, -21.55341960407619695, 59.79275706135234714 ) ) ;
#27768=CARTESIAN_POINT ( 'NONE',  ( 12.14591786802327356, -12.06949235617739191, 85.62609039468568994 ) ) ;
#27769=CARTESIAN_POINT ( 'NONE',  ( -15.80617190586745835, -15.72974639402198527, 21.87390960531436690 ) ) ;
#27770=CARTESIAN_POINT ( 'NONE',  ( 17.49999999999999289, 5.622605283950886879, 28.81207310596113302 ) ) ;
#27771=CARTESIAN_POINT ( 'NONE',  ( -16.38665767535054840, 7.295008042176047702, 80.26400864214549813 ) ) ;
#27772=CARTESIAN_POINT ( 'NONE',  ( 16.53943276465976808, 0.05219959533934440121, 106.2510903946856757 ) ) ;
#27773=CARTESIAN_POINT ( 'NONE',  ( 12.06949235617739724, 12.14591786802326823, 56.87609039468568994 ) ) ;
#27774=CARTESIAN_POINT ( 'NONE',  ( 9.474510206698971260, -16.51473224551069308, 77.91557627198103830 ) ) ;
#27775=CARTESIAN_POINT ( 'NONE',  ( 19.02544592524343514, -5.153800228976328945, 78.54057627198099567 ) ) ;
#27776=CARTESIAN_POINT ( 'NONE',  ( -15.80617190586768217, 15.72974639402176855, 78.12609039468570415 ) ) ;
#27777=CARTESIAN_POINT ( 'NONE',  ( 16.53943276465976808, 0.05219959533934440121, 81.25109039468568994 ) ) ;
#27778=CARTESIAN_POINT ( 'NONE',  ( -14.34966873604960291, -8.224510206698953496, 46.66557627198102409 ) ) ;
#27779=CARTESIAN_POINT ( 'NONE',  ( 9.474510206698971260, -16.51473224551069308, 52.91557627198102409 ) ) ;
#27780=CARTESIAN_POINT ( 'NONE',  ( 9.564922557960805705, 16.46253265017160317, 49.58224293864770260 ) ) ;
#27781=CARTESIAN_POINT ( 'NONE',  ( -16.53943276465976808, -0.05219959533934237506, 43.75109039468568284 ) ) ;
#27783=CARTESIAN_POINT ( 'NONE',  ( -13.97604488694547697, 13.89961937509957934, 98.12609039468566152 ) ) ;
#27784=CARTESIAN_POINT ( 'NONE',  ( 12.06949235617757843, -12.14591786802309237, 98.12390960531436690 ) ) ;
#27785=CARTESIAN_POINT ( 'NONE',  ( 19.02544592524343514, -5.153800228976328945, 63.54057627198103830 ) ) ;
#27786=CARTESIAN_POINT ( 'NONE',  ( 0.05219959533936267826, -19.03943276465977164, 95.00109039468567573 ) ) ;
#27788=CARTESIAN_POINT ( 'NONE',  ( -18.62759615963255300, -10.81492255796106328, 99.16775706135234714 ) ) ;
#27789=CARTESIAN_POINT ( 'NONE',  ( 4.483927247898790824, -16.52544592524335698, 70.20942372801904696 ) ) ;
#27790=LINE ( 'NONE', #154077, #127747 ) ;
#27791=CARTESIAN_POINT ( 'NONE',  ( -21.52544592524343514, 5.823673210054127303, 61.04057627198103120 ) ) ;
#27792=CARTESIAN_POINT ( 'NONE',  ( -8.224510206698735004, -14.34966873604973081, 54.58442372801901143 ) ) ;
#27793=CARTESIAN_POINT ( 'NONE',  ( 19.05341960407611168, 5.049401038298154454, 33.95724293864770260 ) ) ;
#27794=CARTESIAN_POINT ( 'NONE',  ( -5.049401038297874678, -19.05341960407617918, 39.79275706135232582 ) ) ;
#27796=CARTESIAN_POINT ( 'NONE',  ( -19.02544592524342804, 5.153800228976336051, 96.04057627198103830 ) ) ;
#27797=CARTESIAN_POINT ( 'NONE',  ( 12.14591786802309770, 12.06949235617756955, 114.3739096053143527 ) ) ;
#27798=CARTESIAN_POINT ( 'NONE',  ( 5.153800228976335163, 19.02544592524342804, 69.79057627198103830 ) ) ;
#27799=CARTESIAN_POINT ( 'NONE',  ( 5.823673210054444382, -21.52544592524334988, 70.20942372801904696 ) ) ;
#27800=CARTESIAN_POINT ( 'NONE',  ( 16.51473224551083163, -9.474510206698727899, 40.83442372801900433 ) ) ;
#27801=CARTESIAN_POINT ( 'NONE',  ( 13.89961937509957401, 13.97604488694547697, 26.87609039468566507 ) ) ;
#27802=CARTESIAN_POINT ( 'NONE',  ( -13.97604488694527625, -13.89961937509977652, 61.87390960531435979 ) ) ;
#27803=CARTESIAN_POINT ( 'NONE',  ( 16.51473224551069308, 9.474510206698969483, 114.1655762719810241 ) ) ;
#27804=B_SPLINE_CURVE_WITH_KNOTS ( 'NONE', 3,
 ( #138856, #336, #62004, #185367, #46859, #170198 ),
 .UNSPECIFIED., .F., .F.,
 ( 4, 2, 4 ),
 ( 0.003989672132298080140, 0.004372778065220498181, 0.004755883998142916222 ),
 .UNSPECIFIED. ) ;
#27805=CARTESIAN_POINT ( 'NONE',  ( -0.05219959533937732626, 21.53943276465977519, 87.50109039468568994 ) ) ;
#27806=CARTESIAN_POINT ( 'NONE',  ( 13.89961937509977652, -13.97604488694527269, 63.12390960531435979 ) ) ;
#27807=CARTESIAN_POINT ( 'NONE',  ( -21.52544592524334988, -5.823673210054445271, 93.95942372801903275 ) ) ;
#27808=CARTESIAN_POINT ( 'NONE',  ( 10.72451020669898902, -18.67979575497178502, 32.91557627198102409 ) ) ;
#27809=CARTESIAN_POINT ( 'NONE',  ( 16.46253265017160672, -9.564922557960803928, 88.33224293864769550 ) ) ;
#27810=CARTESIAN_POINT ( 'NONE',  ( 15.80617190586769283, -15.72974639402175789, 45.62609039468567573 ) ) ;
#27811=CARTESIAN_POINT ( 'NONE',  ( -0.05219959533936034679, 19.03943276465977164, 62.50109039468566863 ) ) ;
#27812=CARTESIAN_POINT ( 'NONE',  ( -13.89961937509977652, 13.97604488694528158, 40.62390960531435979 ) ) ;
#27813=CARTESIAN_POINT ( 'NONE',  ( -5.153800228976328057, -19.02544592524343514, 87.29057627198103830 ) ) ;
#27814=CARTESIAN_POINT ( 'NONE',  ( -8.224510206698735004, -14.34966873604973081, 24.58442372801901499 ) ) ;
#27815=CARTESIAN_POINT ( 'NONE',  ( 14.34966873604960469, 8.224510206698951720, 84.16557627198103830 ) ) ;
#27816=CARTESIAN_POINT ( 'NONE',  ( 19.05341960407611168, 5.049401038298154454, 68.95724293864769550 ) ) ;
#27817=CARTESIAN_POINT ( 'NONE',  ( -5.719274019375978568, 21.55341960407610458, 45.20724293864769550 ) ) ;
#27818=CARTESIAN_POINT ( 'NONE',  ( 8.224510206698742110, 14.34966873604972548, 22.08442372801901143 ) ) ;
#27819=CARTESIAN_POINT ( 'NONE',  ( -5.719274019375665041, -21.55341960407619695, 24.79275706135235779 ) ) ;
#27820=CARTESIAN_POINT ( 'NONE',  ( -5.823673210054431948, 21.52544592524334988, 72.70942372801901854 ) ) ;
#27821=CARTESIAN_POINT ( 'NONE',  ( -12.06949235617739369, -12.14591786802326823, 64.37609039468568994 ) ) ;
#27822=CARTESIAN_POINT ( 'NONE',  ( 14.29746914071037800, 8.314922557961029526, 66.66775706135234714 ) ) ;
#27823=CARTESIAN_POINT ( 'NONE',  ( -9.564922557960796823, -16.46253265017161027, 62.08224293864769550 ) ) ;
#27824=CARTESIAN_POINT ( 'NONE',  ( -14.29746914071037622, -8.314922557961029526, 104.1677570613523471 ) ) ;
#27825=CARTESIAN_POINT ( 'NONE',  ( 19.05341960407617918, -5.049401038297876454, 46.04275706135233293 ) ) ;
#27826=CARTESIAN_POINT ( 'NONE',  ( 15.80617190586746368, 15.72974639402197994, 114.3739096053143527 ) ) ;
#27828=CARTESIAN_POINT ( 'NONE',  ( -12.06949235617756955, 12.14591786802309770, 70.62390960531436690 ) ) ;
#27829=CARTESIAN_POINT ( 'NONE',  ( 0.05219959533909260263, 19.03943276465977164, 79.99890960531436690 ) ) ;
#27830=CARTESIAN_POINT ( 'NONE',  ( -12.14591786802326823, 12.06949235617739902, 83.12609039468568994 ) ) ;
#27831=CARTESIAN_POINT ( 'NONE',  ( 10.81492255796106328, -18.62759615963255655, 60.41775706135235424 ) ) ;
#27832=CARTESIAN_POINT ( 'NONE',  ( 8.224510206698742110, 14.34966873604972548, 37.08442372801901143 ) ) ;
#27833=CARTESIAN_POINT ( 'NONE',  ( 21.53943276465977519, 0.05219959533937863772, 21.25109039468567218 ) ) ;
#27834=CARTESIAN_POINT ( 'NONE',  ( 4.483927247898545687, 16.52544592524342804, 64.79057627198103830 ) ) ;
#27836=CARTESIAN_POINT ( 'NONE',  ( -5.823673210054116645, -21.52544592524344225, 107.2905762719810525 ) ) ;
#27837=CARTESIAN_POINT ( 'NONE',  ( -12.06949235617756955, 12.14591786802309770, 45.62390960531436690 ) ) ;
#27840=CARTESIAN_POINT ( 'NONE',  ( 10.72451020669898902, -18.67979575497178502, 32.91557627198102409 ) ) ;
#27841=CARTESIAN_POINT ( 'NONE',  ( 21.55341960407619695, -5.719274019375665929, 41.04275706135236135 ) ) ;
#27842=CARTESIAN_POINT ( 'NONE',  ( -14.29746914071049879, 8.314922557960819915, 70.83224293864770971 ) ) ;
#27844=CARTESIAN_POINT ( 'NONE',  ( 21.53943276465977519, -0.05219959533907433946, 68.74890960531435269 ) ) ;
#27845=CARTESIAN_POINT ( 'NONE',  ( -5.049401038298153566, 19.05341960407611168, 75.20724293864769550 ) ) ;
#27846=CARTESIAN_POINT ( 'NONE',  ( 19.05341960407611168, 5.049401038298154454, 28.95724293864769550 ) ) ;
#27847=CARTESIAN_POINT ( 'NONE',  ( -19.05341960407617563, 5.049401038297882671, 63.54275706135234003 ) ) ;
#27848=CARTESIAN_POINT ( 'NONE',  ( 5.719274019375991003, -21.55341960407610458, 52.70724293864769550 ) ) ;
#27849=CARTESIAN_POINT ( 'NONE',  ( 13.97604488694527802, 13.89961937509977652, 64.37390960531436690 ) ) ;
#27851=CARTESIAN_POINT ( 'NONE',  ( -8.314922557961024197, 14.29746914071037800, 32.91775706135234714 ) ) ;
#27852=CARTESIAN_POINT ( 'NONE',  ( -21.55341960407619339, 5.719274019375674811, 23.54275706135235424 ) ) ;
#27854=CARTESIAN_POINT ( 'NONE',  ( -16.53943276465976808, 0.05219959533911058130, 41.24890960531435269 ) ) ;
#27855=CARTESIAN_POINT ( 'NONE',  ( 19.05341960407611168, 5.049401038298154454, 98.95724293864766707 ) ) ;
#27856=CARTESIAN_POINT ( 'NONE',  ( -21.55341960407610458, -5.719274019375992779, 71.45724293864769550 ) ) ;
#27857=CARTESIAN_POINT ( 'NONE',  ( 18.67979575497178502, 10.72451020669898547, 114.1655762719810383 ) ) ;
#27858=CARTESIAN_POINT ( 'NONE',  ( 16.55341960407618274, -4.379528057220086978, 41.04275706135236135 ) ) ;
#27859=CARTESIAN_POINT ( 'NONE',  ( -21.53943276465977519, 0.05219959533907696930, 56.24890960531436690 ) ) ;
#27860=CARTESIAN_POINT ( 'NONE',  ( -18.67979575497193778, 10.72451020669871902, 108.3344237280190185 ) ) ;
#27861=CARTESIAN_POINT ( 'NONE',  ( 5.153800228976335163, 19.02544592524342804, 39.79057627198100988 ) ) ;
#27862=CARTESIAN_POINT ( 'NONE',  ( -5.049401038298153566, 19.05341960407611168, 100.2072429386476955 ) ) ;
#27863=CARTESIAN_POINT ( 'NONE',  ( -19.05341960407611168, -5.049401038298163336, 81.45724293864769550 ) ) ;
#27864=CARTESIAN_POINT ( 'NONE',  ( 16.20579543436696213, -7.371946100355082798, 86.93479165828053112 ) ) ;
#27865=CARTESIAN_POINT ( 'NONE',  ( 19.03943276465977164, 0.05219959533936151252, 56.25109039468566863 ) ) ;
#27866=CARTESIAN_POINT ( 'NONE',  ( 5.719274019375673035, 21.55341960407619339, 112.2927570613523471 ) ) ;
#27867=CARTESIAN_POINT ( 'NONE',  ( -21.55341960407610458, -5.719274019375992779, 31.45724293864769550 ) ) ;
#27868=CARTESIAN_POINT ( 'NONE',  ( -4.379528057220086978, -16.55341960407618274, 109.7927570613523613 ) ) ;
#27869=CARTESIAN_POINT ( 'NONE',  ( 0.05219959533936267826, -19.03943276465977164, 80.00109039468567573 ) ) ;
#27871=CARTESIAN_POINT ( 'NONE',  ( 19.03943276465977164, 0.05219959533936151252, 86.25109039468567573 ) ) ;
#27872=CARTESIAN_POINT ( 'NONE',  ( 19.03943276465977164, 0.05219959533936151252, 41.25109039468566152 ) ) ;
#27874=CARTESIAN_POINT ( 'NONE',  ( 13.89961937509977652, -13.97604488694527269, 43.12390960531434558 ) ) ;
#27875=CARTESIAN_POINT ( 'NONE',  ( -12.14591786802309592, -12.06949235617757132, 46.87390960531435979 ) ) ;
#27876=CARTESIAN_POINT ( 'NONE',  ( -9.474510206698964154, 16.51473224551069663, 40.41557627198103120 ) ) ;
#27877=CARTESIAN_POINT ( 'NONE',  ( 12.14591786802309770, 12.06949235617756955, 44.37390960531435979 ) ) ;
#27879=CARTESIAN_POINT ( 'NONE',  ( -4.379528057220086978, -16.55341960407618274, 104.7927570613523898 ) ) ;
#27880=CARTESIAN_POINT ( 'NONE',  ( 13.89961937509977652, -13.97604488694527269, 48.12390960531435979 ) ) ;
#27881=CARTESIAN_POINT ( 'NONE',  ( -10.81492255796105439, 18.62759615963255655, 112.9177570613523329 ) ) ;
#27882=CARTESIAN_POINT ( 'NONE',  ( 16.51473224551083163, -9.474510206698727899, 110.8344237280190043 ) ) ;
#27883=CARTESIAN_POINT ( 'NONE',  ( -18.62759615963270932, 10.81492255796079327, 35.83224293864768839 ) ) ;
#27884=CARTESIAN_POINT ( 'NONE',  ( 0.05219959533937995610, -21.53943276465977519, 95.00109039468568994 ) ) ;
#27886=CARTESIAN_POINT ( 'NONE',  ( -13.89961937509977652, 13.97604488694528158, 110.6239096053143243 ) ) ;
#27887=CARTESIAN_POINT ( 'NONE',  ( -13.89961937509977652, 13.97604488694528158, 85.62390960531433848 ) ) ;
#27889=CARTESIAN_POINT ( 'NONE',  ( -5.823673210054116645, -21.52544592524344225, 107.2905762719810525 ) ) ;
#27890=VECTOR ( 'NONE', #27535, 1000.000000000000000 ) ;
#27891=CARTESIAN_POINT ( 'NONE',  ( -14.29746914071049879, 8.314922557960819915, 75.83224293864769550 ) ) ;
#27892=CARTESIAN_POINT ( 'NONE',  ( 21.55341960407610458, 5.719274019375980345, 73.95724293864769550 ) ) ;
#27893=CARTESIAN_POINT ( 'NONE',  ( -16.51473224551069308, -9.474510206698971260, 56.66557627198103120 ) ) ;
#27894=CARTESIAN_POINT ( 'NONE',  ( -21.52544592524343514, 5.823673210054127303, 96.04057627198102409 ) ) ;
#27896=CARTESIAN_POINT ( 'NONE',  ( -16.46253265017160317, 9.564922557960807481, 60.83224293864769550 ) ) ;
#27897=CARTESIAN_POINT ( 'NONE',  ( 14.34966873604960469, 8.224510206698951720, 89.16557627198102409 ) ) ;
#27899=CARTESIAN_POINT ( 'NONE',  ( 16.46253265017160672, -9.564922557960803928, 68.33224293864770971 ) ) ;
#27900=CARTESIAN_POINT ( 'NONE',  ( -5.049401038297874678, -19.05341960407617918, 79.79275706135233293 ) ) ;
#27901=CARTESIAN_POINT ( 'NONE',  ( 14.29746914071049879, -8.314922557960816363, 88.33224293864769550 ) ) ;
#27902=CARTESIAN_POINT ( 'NONE',  ( -21.53943276465977519, -0.05219959533937600094, 53.75109039468568994 ) ) ;
#27903=CARTESIAN_POINT ( 'NONE',  ( -13.89961937509977652, 13.97604488694528158, 45.62390960531433848 ) ) ;
#27904=CARTESIAN_POINT ( 'NONE',  ( -21.52544592524334988, -5.823673210054445271, 23.95942372801901143 ) ) ;
#27905=CARTESIAN_POINT ( 'NONE',  ( -0.05219959533910754901, -16.53943276465976808, 102.4989096053143811 ) ) ;
#27907=CARTESIAN_POINT ( 'NONE',  ( 16.46253265017160672, -9.564922557960803928, 63.33224293864769550 ) ) ;
#27908=CARTESIAN_POINT ( 'NONE',  ( 16.29526858892874230, 7.335722546920135478, 113.2967059780020946 ) ) ;
#27909=CARTESIAN_POINT ( 'NONE',  ( -9.564922557961040184, 16.46253265017147172, 112.9177570613523329 ) ) ;
#27910=CARTESIAN_POINT ( 'NONE',  ( -13.89961937509977652, 13.97604488694528158, 115.6239096053143669 ) ) ;
#27911=CARTESIAN_POINT ( 'NONE',  ( 5.823673210054444382, -21.52544592524334988, 55.20942372801902565 ) ) ;
#27912=CARTESIAN_POINT ( 'NONE',  ( 9.474510206698971260, -16.51473224551069308, 97.91557627198102409 ) ) ;
#27913=CARTESIAN_POINT ( 'NONE',  ( -13.89961937509957401, -13.97604488694547875, 84.37609039468567573 ) ) ;
#27914=CARTESIAN_POINT ( 'NONE',  ( 5.049401038298161559, -19.05341960407611168, 52.70724293864767418 ) ) ;
#27915=CARTESIAN_POINT ( 'NONE',  ( -14.29746914071049879, 8.314922557960819915, 80.83224293864769550 ) ) ;
#27916=CARTESIAN_POINT ( 'NONE',  ( -12.14591786802309592, -12.06949235617757132, 81.87390960531435269 ) ) ;
#27917=CARTESIAN_POINT ( 'NONE',  ( 9.474510206698971260, -16.51473224551069308, 92.91557627198103830 ) ) ;
#27918=CARTESIAN_POINT ( 'NONE',  ( 8.314922557960818139, 14.29746914071049879, 79.58224293864769550 ) ) ;
#27919=CARTESIAN_POINT ( 'NONE',  ( 16.51473224551069308, 9.474510206698969483, 84.16557627198102409 ) ) ;
#27920=CARTESIAN_POINT ( 'NONE',  ( -19.03943276465977164, -0.05219959533935918106, 33.75109039468566863 ) ) ;
#27921=CARTESIAN_POINT ( 'NONE',  ( -5.153800228976328057, -19.02544592524343514, 52.29057627198100988 ) ) ;
#27922=CARTESIAN_POINT ( 'NONE',  ( -16.52544592524342804, 4.483927247898546575, 26.04057627198103475 ) ) ;
#27923=CARTESIAN_POINT ( 'NONE',  ( 13.89961937509977652, -13.97604488694527269, 28.12390960531435624 ) ) ;
#27925=CARTESIAN_POINT ( 'NONE',  ( -18.62759615963255300, -10.81492255796106328, 39.16775706135235424 ) ) ;
#27926=CARTESIAN_POINT ( 'NONE',  ( 5.153800228976615827, -19.02544592524334988, 80.20942372801901854 ) ) ;
#27927=CARTESIAN_POINT ( 'NONE',  ( 16.55341960407611168, 4.379528057220329451, 38.95724293864768839 ) ) ;
#27928=CARTESIAN_POINT ( 'NONE',  ( 15.80617190586746368, 15.72974639402197994, 84.37390960531438111 ) ) ;
#27929=CARTESIAN_POINT ( 'NONE',  ( 0.05219959533907565091, 21.53943276465977519, 29.99890960531435979 ) ) ;
#27930=CARTESIAN_POINT ( 'NONE',  ( 16.55341960407611168, 4.379528057220329451, 63.95724293864770260 ) ) ;
#27931=CARTESIAN_POINT ( 'NONE',  ( -5.153800228976328057, -19.02544592524343514, 42.29057627198101699 ) ) ;
#27932=CARTESIAN_POINT ( 'NONE',  ( 4.483927247898790824, -16.52544592524335698, 100.2094237280190043 ) ) ;
#27933=CARTESIAN_POINT ( 'NONE',  ( 12.06949235617739724, 12.14591786802326823, 66.87609039468568994 ) ) ;
#27934=CARTESIAN_POINT ( 'NONE',  ( 21.52544592524344225, -5.823673210054117533, 33.54057627198102409 ) ) ;
#27935=CARTESIAN_POINT ( 'NONE',  ( 19.02544592524334988, 5.153800228976608722, 21.45942372801899012 ) ) ;
#27936=CARTESIAN_POINT ( 'NONE',  ( 16.46253265017160672, -9.564922557960803928, 93.33224293864769550 ) ) ;
#27938=CARTESIAN_POINT ( 'NONE',  ( 16.52544592524335698, 4.483927247898782831, 71.45942372801901854 ) ) ;
#27939=CARTESIAN_POINT ( 'NONE',  ( -0.05219959533909027116, -19.03943276465977164, 27.49890960531435624 ) ) ;
#27940=CARTESIAN_POINT ( 'NONE',  ( 16.53943276465976808, -0.05219959533910856209, 38.74890960531435979 ) ) ;
#27941=CARTESIAN_POINT ( 'NONE',  ( 5.153800228976335163, 19.02544592524342804, 104.7905762719809957 ) ) ;
#27942=CARTESIAN_POINT ( 'NONE',  ( -19.05341960407611168, -5.049401038298163336, 96.45724293864769550 ) ) ;
#27943=CARTESIAN_POINT ( 'NONE',  ( -15.80617190586745835, -15.72974639402198527, 21.87390960531436690 ) ) ;
#27945=CARTESIAN_POINT ( 'NONE',  ( 14.29746914071049879, -8.314922557960816363, 78.33224293864770971 ) ) ;
#27946=CARTESIAN_POINT ( 'NONE',  ( -4.483927247898539470, -16.52544592524342804, 47.29057627198103120 ) ) ;
#27948=CARTESIAN_POINT ( 'NONE',  ( -14.29746914071037622, -8.314922557961029526, 49.16775706135234003 ) ) ;
#27950=CARTESIAN_POINT ( 'NONE',  ( -5.153800228976607833, 19.02544592524334988, 52.70942372801900433 ) ) ;
#27951=CARTESIAN_POINT ( 'NONE',  ( -19.05341960407611168, -5.049401038298163336, 86.45724293864769550 ) ) ;
#27952=CARTESIAN_POINT ( 'NONE',  ( 5.153800228976615827, -19.02544592524334988, 65.20942372801900433 ) ) ;
#27954=CARTESIAN_POINT ( 'NONE',  ( -16.52544592524335698, -4.483927247898792601, 18.95942372801901143 ) ) ;
#27955=CARTESIAN_POINT ( 'NONE',  ( 14.29746914071037800, 8.314922557961029526, 91.66775706135234714 ) ) ;
#27956=CARTESIAN_POINT ( 'NONE',  ( 5.153800228976335163, 19.02544592524342804, 34.79057627198102409 ) ) ;
#27957=CARTESIAN_POINT ( 'NONE',  ( 13.97604488694527802, 13.89961937509977652, 114.3739096053143669 ) ) ;
#27958=CARTESIAN_POINT ( 'NONE',  ( -18.62759615963255300, -10.81492255796106328, 49.16775706135234003 ) ) ;
#27959=CARTESIAN_POINT ( 'NONE',  ( 9.564922557961047289, -16.46253265017146816, 100.4177570613523329 ) ) ;
#27960=CARTESIAN_POINT ( 'NONE',  ( -30.00000000000000000, -1.163414459189985801E-14, 95.00000000000000000 ) ) ;
#27961=CARTESIAN_POINT ( 'NONE',  ( -9.564922557960796823, -16.46253265017161027, 72.08224293864770971 ) ) ;
#27963=CARTESIAN_POINT ( 'NONE',  ( 16.52544592524342804, -4.483927247898539470, 78.54057627198103830 ) ) ;
#27964=CARTESIAN_POINT ( 'NONE',  ( 9.474510206698971260, -16.51473224551069308, 67.91557627198102409 ) ) ;
#27966=CARTESIAN_POINT ( 'NONE',  ( -5.049401038298153566, 19.05341960407611168, 75.20724293864769550 ) ) ;
#27967=CARTESIAN_POINT ( 'NONE',  ( -9.564922557961040184, 16.46253265017147172, 72.91775706135233293 ) ) ;
#27968=CARTESIAN_POINT ( 'NONE',  ( 21.55341960407610458, 5.719274019375980345, 68.95724293864769550 ) ) ;
#27969=CARTESIAN_POINT ( 'NONE',  ( -0.05219959533910754901, -16.53943276465976808, 112.4989096053143669 ) ) ;
#27970=CARTESIAN_POINT ( 'NONE',  ( -0.05219959533936034679, 19.03943276465977164, 62.50109039468566863 ) ) ;
#27971=CARTESIAN_POINT ( 'NONE',  ( -5.153800228976328057, -19.02544592524343514, 62.29057627198100988 ) ) ;
#27972=CARTESIAN_POINT ( 'NONE',  ( -19.05341960407611168, -5.049401038298163336, 96.45724293864769550 ) ) ;
#27973=EDGE_CURVE ( 'NONE', #138021, #60866, #16219, .T. ) ;
#27974=CARTESIAN_POINT ( 'NONE',  ( -15.72974639402197994, 15.80617190586746368, 95.62390960531436690 ) ) ;
#27975=CARTESIAN_POINT ( 'NONE',  ( -8.314922557960811034, -14.29746914071050412, 77.08224293864769550 ) ) ;
#27976=CARTESIAN_POINT ( 'NONE',  ( -5.153800228976607833, 19.02544592524334988, 42.70942372801901143 ) ) ;
#27977=CARTESIAN_POINT ( 'NONE',  ( 0.05219959533907565091, 21.53943276465977519, 74.99890960531435269 ) ) ;
#27978=CARTESIAN_POINT ( 'NONE',  ( -0.05219959533907301413, -21.53943276465977519, 62.49890960531436690 ) ) ;
#27979=CARTESIAN_POINT ( 'NONE',  ( 8.224510206698953496, -14.34966873604960469, 27.91557627198103830 ) ) ;
#27980=CARTESIAN_POINT ( 'NONE',  ( 18.67979575497194134, -10.72451020669871369, 95.83442372801903275 ) ) ;
#27981=CARTESIAN_POINT ( 'NONE',  ( 13.97604488694527802, 13.89961937509977652, 79.37390960531435269 ) ) ;
#27982=CARTESIAN_POINT ( 'NONE',  ( -16.51473224551069308, -9.474510206698971260, 36.66557627198102409 ) ) ;
#27983=CARTESIAN_POINT ( 'NONE',  ( 21.55341960407619695, -5.719274019375665929, 46.04275706135234714 ) ) ;
#27985=CARTESIAN_POINT ( 'NONE',  ( 10.72451020669871369, 18.67979575497193778, 37.08442372801901143 ) ) ;
#27986=CARTESIAN_POINT ( 'NONE',  ( 19.03943276465977164, -0.05219959533909143690, 43.74890960531435979 ) ) ;
#27987=CARTESIAN_POINT ( 'NONE',  ( -15.72974639402176322, -15.80617190586768395, 19.37609039468568639 ) ) ;
#27988=CARTESIAN_POINT ( 'NONE',  ( 19.02544592524334988, 5.153800228976608722, 56.45942372801898301 ) ) ;
#27989=CARTESIAN_POINT ( 'NONE',  ( 13.89961937509977652, -13.97604488694527269, 43.12390960531434558 ) ) ;
#27990=CARTESIAN_POINT ( 'NONE',  ( -0.05219959533934338120, 16.53943276465976808, 27.50109039468567929 ) ) ;
#27991=CARTESIAN_POINT ( 'NONE',  ( -16.51473224551069308, -9.474510206698971260, 26.66557627198103120 ) ) ;
#27992=CARTESIAN_POINT ( 'NONE',  ( -8.224510206698735004, -14.34966873604973081, 69.58442372801900433 ) ) ;
#27993=CARTESIAN_POINT ( 'NONE',  ( -5.049401038298153566, 19.05341960407611168, 40.20724293864768839 ) ) ;
#27995=CARTESIAN_POINT ( 'NONE',  ( -13.89961937509977652, 13.97604488694528158, 85.62390960531433848 ) ) ;
#27996=CARTESIAN_POINT ( 'NONE',  ( -14.29746914071049879, 8.314922557960819915, 115.8322429386477097 ) ) ;
#27997=CARTESIAN_POINT ( 'NONE',  ( -18.67979575497178146, -10.72451020669898902, 61.66557627198103120 ) ) ;
#27998=CARTESIAN_POINT ( 'NONE',  ( -0.05219959533934338120, 16.53943276465976808, 42.50109039468567573 ) ) ;
#27999=CARTESIAN_POINT ( 'NONE',  ( 18.62759615963255655, 10.81492255796105972, 96.66775706135234714 ) ) ;
#28000=CARTESIAN_POINT ( 'NONE',  ( -19.02544592524342804, 5.153800228976336051, 46.04057627198101699 ) ) ;
#28001=CARTESIAN_POINT ( 'NONE',  ( -12.14591786802309592, -12.06949235617757132, 36.87390960531435979 ) ) ;
#28002=CARTESIAN_POINT ( 'NONE',  ( 4.483927247898545687, 16.52544592524342804, 64.79057627198103830 ) ) ;
#28003=CARTESIAN_POINT ( 'NONE',  ( -5.153800228976328057, -19.02544592524343514, 67.29057627198102409 ) ) ;
#28004=CARTESIAN_POINT ( 'NONE',  ( -5.049401038297874678, -19.05341960407617918, 19.79275706135233293 ) ) ;
#28005=CARTESIAN_POINT ( 'NONE',  ( 18.67979575497194134, -10.72451020669871369, 20.83442372801901143 ) ) ;
#28006=CARTESIAN_POINT ( 'NONE',  ( 0.05219959533909260263, 19.03943276465977164, 74.99890960531435269 ) ) ;
#28007=CARTESIAN_POINT ( 'NONE',  ( -5.823673210054431948, 21.52544592524334988, 87.70942372801901854 ) ) ;
#28008=CARTESIAN_POINT ( 'NONE',  ( -16.53943276465976808, -0.05219959533934237506, 58.75109039468568994 ) ) ;
#28009=CARTESIAN_POINT ( 'NONE',  ( 12.06949235617739724, 12.14591786802326823, 26.87609039468567218 ) ) ;
#28010=CARTESIAN_POINT ( 'NONE',  ( -8.314922557960811034, -14.29746914071050412, 87.08224293864769550 ) ) ;
#28011=CARTESIAN_POINT ( 'NONE',  ( 5.719274019375673035, 21.55341960407619339, 97.29275706135234714 ) ) ;
#28012=CARTESIAN_POINT ( 'NONE',  ( 16.55341960407611168, 4.379528057220329451, 33.95724293864769550 ) ) ;
#28013=CARTESIAN_POINT ( 'NONE',  ( -5.153800228976328057, -19.02544592524343514, 32.29057627198102409 ) ) ;
#28014=CARTESIAN_POINT ( 'NONE',  ( 16.53943276465976808, 0.05219959533934440121, 56.25109039468568284 ) ) ;
#28015=CARTESIAN_POINT ( 'NONE',  ( 16.53943276465976808, -0.05219959533910856209, 58.74890960531436690 ) ) ;
#28016=CARTESIAN_POINT ( 'NONE',  ( -0.05219959533934338120, 16.53943276465976808, 102.5010903946856899 ) ) ;
#28017=CARTESIAN_POINT ( 'NONE',  ( 5.153800228976335163, 19.02544592524342804, 109.7905762719810099 ) ) ;
#28018=CARTESIAN_POINT ( 'NONE',  ( 5.049401038298161559, -19.05341960407611168, 112.7072429386476813 ) ) ;
#28019=CARTESIAN_POINT ( 'NONE',  ( -21.53943276465977519, -0.05219959533937600094, 113.7510903946856757 ) ) ;
#28020=CARTESIAN_POINT ( 'NONE',  ( 14.29746914071049879, -8.314922557960816363, 83.33224293864769550 ) ) ;
#28021=CARTESIAN_POINT ( 'NONE',  ( -13.89961937509977652, 13.97604488694528158, 95.62390960531436690 ) ) ;
#28023=CARTESIAN_POINT ( 'NONE',  ( 0.05219959533934541429, -16.53943276465976808, 35.00109039468568284 ) ) ;
#28024=CARTESIAN_POINT ( 'NONE',  ( 13.97604488694527802, 13.89961937509977652, 44.37390960531435269 ) ) ;
#28025=CARTESIAN_POINT ( 'NONE',  ( 4.379528057220092307, 16.55341960407617563, 47.29275706135234003 ) ) ;
#28027=CARTESIAN_POINT ( 'NONE',  ( 19.05341960407617918, -5.049401038297876454, 51.04275706135231871 ) ) ;
#28028=CARTESIAN_POINT ( 'NONE',  ( 13.97604488694527802, 13.89961937509977652, 49.37390960531434558 ) ) ;
#28029=CARTESIAN_POINT ( 'NONE',  ( 4.379528057220092307, 16.55341960407617563, 82.29275706135234714 ) ) ;
#28030=CARTESIAN_POINT ( 'NONE',  ( 13.89961937509957401, 13.97604488694547697, 76.87609039468566152 ) ) ;
#28031=CARTESIAN_POINT ( 'NONE',  ( -13.89961937509957401, -13.97604488694547875, 24.37609039468565442 ) ) ;
#28032=CARTESIAN_POINT ( 'NONE',  ( -16.51473224551069308, -9.474510206698971260, 61.66557627198103120 ) ) ;
#28033=CARTESIAN_POINT ( 'NONE',  ( -16.52544592524342804, 4.483927247898546575, 101.0405762719810383 ) ) ;
#28035=CARTESIAN_POINT ( 'NONE',  ( -19.03943276465977164, -0.05219959533935918106, 73.75109039468566152 ) ) ;
#28036=CARTESIAN_POINT ( 'NONE',  ( -5.719274019375978568, 21.55341960407610458, 65.20724293864768129 ) ) ;
#28037=CARTESIAN_POINT ( 'NONE',  ( -13.97604488694547697, 13.89961937509957934, 33.12609039468566863 ) ) ;
#28038=CARTESIAN_POINT ( 'NONE',  ( 13.97604488694527802, 13.89961937509977652, 99.37390960531436690 ) ) ;
#28039=CARTESIAN_POINT ( 'NONE',  ( 5.719274019375991003, -21.55341960407610458, 82.70724293864770971 ) ) ;
#28040=CARTESIAN_POINT ( 'NONE',  ( -17.44270441346519007, 5.991230190322971438, 83.63664920735773478 ) ) ;
#28041=CARTESIAN_POINT ( 'NONE',  ( -19.03943276465977164, -0.05219959533935918106, 103.7510903946856757 ) ) ;
#28044=CARTESIAN_POINT ( 'NONE',  ( 12.06949235617739724, 12.14591786802326823, 21.87609039468567573 ) ) ;
#28045=CARTESIAN_POINT ( 'NONE',  ( -16.51473224551069308, -9.474510206698971260, 36.66557627198102409 ) ) ;
#28046=CARTESIAN_POINT ( 'NONE',  ( 9.474510206698971260, -16.51473224551069308, 107.9155762719810383 ) ) ;
#28047=CARTESIAN_POINT ( 'NONE',  ( -18.67979575497178146, -10.72451020669898902, 91.66557627198103830 ) ) ;
#28048=CARTESIAN_POINT ( 'NONE',  ( -5.719274019375665041, -21.55341960407619695, 54.79275706135235424 ) ) ;
#28049=CARTESIAN_POINT ( 'NONE',  ( 5.153800228976615827, -19.02544592524334988, 105.2094237280190185 ) ) ;
#28050=CARTESIAN_POINT ( 'NONE',  ( -18.67979575497193778, 10.72451020669871902, 113.3344237280190328 ) ) ;
#28051=CARTESIAN_POINT ( 'NONE',  ( -16.53943276465976808, -0.05219959533934237506, 103.7510903946857042 ) ) ;
#28052=CARTESIAN_POINT ( 'NONE',  ( 0.05219959533907565091, 21.53943276465977519, 99.99890960531436690 ) ) ;
#28053=CARTESIAN_POINT ( 'NONE',  ( -16.55341960407611168, -4.379528057220339221, 51.45724293864770260 ) ) ;
#28054=CARTESIAN_POINT ( 'NONE',  ( -13.89961937509957401, -13.97604488694547875, 84.37609039468567573 ) ) ;
#28055=CARTESIAN_POINT ( 'NONE',  ( -13.97604488694547697, 13.89961937509957934, 58.12609039468566863 ) ) ;
#28056=CARTESIAN_POINT ( 'NONE',  ( -18.67979575497193778, 10.72451020669871902, 68.33442372801900433 ) ) ;
#28057=CARTESIAN_POINT ( 'NONE',  ( -9.474510206698720793, -16.51473224551083518, 44.58442372801900433 ) ) ;
#28058=CARTESIAN_POINT ( 'NONE',  ( 0.05219959533910956823, 16.53943276465976808, 104.9989096053143669 ) ) ;
#28059=CARTESIAN_POINT ( 'NONE',  ( -18.67979575497178146, -10.72451020669898902, 41.66557627198103120 ) ) ;
#28060=CARTESIAN_POINT ( 'NONE',  ( -14.29746914071049879, 8.314922557960819915, 30.83224293864770260 ) ) ;
#28061=CARTESIAN_POINT ( 'NONE',  ( -15.72974639402176322, -15.80617190586768395, 94.37609039468568994 ) ) ;
#28062=CARTESIAN_POINT ( 'NONE',  ( -12.06949235617739369, -12.14591786802326823, 69.37609039468567573 ) ) ;
#28063=CARTESIAN_POINT ( 'NONE',  ( -14.29746914071049879, 8.314922557960819915, 25.83224293864769194 ) ) ;
#28064=CARTESIAN_POINT ( 'NONE',  ( -21.52544592524334988, -5.823673210054445271, 58.95942372801902565 ) ) ;
#28065=CARTESIAN_POINT ( 'NONE',  ( -0.05219959533937732626, 21.53943276465977519, 67.50109039468568994 ) ) ;
#28067=CARTESIAN_POINT ( 'NONE',  ( -21.52544592524343514, 5.823673210054127303, 66.04057627198103830 ) ) ;
#28069=CARTESIAN_POINT ( 'NONE',  ( -13.89961937509977652, 13.97604488694528158, 25.62390960531434558 ) ) ;
#28070=CARTESIAN_POINT ( 'NONE',  ( -21.55341960407619339, 5.719274019375674811, 43.54275706135235424 ) ) ;
#28071=CARTESIAN_POINT ( 'NONE',  ( -5.049401038298153566, 19.05341960407611168, 25.20724293864768484 ) ) ;
#28072=CARTESIAN_POINT ( 'NONE',  ( -0.05219959533909027116, -19.03943276465977164, 37.49890960531436690 ) ) ;
#28073=CARTESIAN_POINT ( 'NONE',  ( 16.53943276465976808, -0.05219959533910856209, 73.74890960531433848 ) ) ;
#28074=CARTESIAN_POINT ( 'NONE',  ( 16.51473224551069308, 9.474510206698969483, 84.16557627198102409 ) ) ;
#28075=CARTESIAN_POINT ( 'NONE',  ( -14.34966873604960291, -8.224510206698953496, 21.66557627198102409 ) ) ;
#28076=CARTESIAN_POINT ( 'NONE',  ( 14.29746914071049879, -8.314922557960816363, 103.3322429386476955 ) ) ;
#28077=CARTESIAN_POINT ( 'NONE',  ( 21.53943276465977519, -0.05219959533907433946, 73.74890960531433848 ) ) ;
#28078=VECTOR ( 'NONE', #39367, 1000.000000000000000 ) ;
#28079=CARTESIAN_POINT ( 'NONE',  ( 10.81492255796078972, 18.62759615963270932, 104.5822429386477097 ) ) ;
#28081=CARTESIAN_POINT ( 'NONE',  ( 19.03943276465977164, -0.05219959533909143690, 68.74890960531436690 ) ) ;
#28082=CARTESIAN_POINT ( 'NONE',  ( -12.06949235617739369, -12.14591786802326823, 19.37609039468568639 ) ) ;
#28083=CARTESIAN_POINT ( 'NONE',  ( -10.81492255796078084, -18.62759615963271287, 52.08224293864768839 ) ) ;
#28084=CARTESIAN_POINT ( 'NONE',  ( -5.823673210054431948, 21.52544592524334988, 77.70942372801900433 ) ) ;
#28085=CARTESIAN_POINT ( 'NONE',  ( 16.51473224551069308, 9.474510206698969483, 79.16557627198103830 ) ) ;
#28086=CARTESIAN_POINT ( 'NONE',  ( 5.153800228976335163, 19.02544592524342804, 99.79057627198102409 ) ) ;
#28087=CARTESIAN_POINT ( 'NONE',  ( -4.379528057220086978, -16.55341960407618274, 74.79275706135234714 ) ) ;
#28088=CARTESIAN_POINT ( 'NONE',  ( 5.719274019375673035, 21.55341960407619339, 57.29275706135234714 ) ) ;
#28089=CARTESIAN_POINT ( 'NONE',  ( 10.81492255796106328, -18.62759615963255655, 100.4177570613523471 ) ) ;
#28090=CARTESIAN_POINT ( 'NONE',  ( 16.52544592524335698, 4.483927247898782831, 66.45942372801903275 ) ) ;
#28091=CARTESIAN_POINT ( 'NONE',  ( -5.823673210054116645, -21.52544592524344225, 107.2905762719810525 ) ) ;
#28092=CARTESIAN_POINT ( 'NONE',  ( -9.564922557960796823, -16.46253265017161027, 112.0822429386476955 ) ) ;
#28093=CARTESIAN_POINT ( 'NONE',  ( -10.72451020669898014, 18.67979575497178502, 85.41557627198102409 ) ) ;
#28094=CARTESIAN_POINT ( 'NONE',  ( 9.474510206698729675, 16.51473224551082808, 42.08442372801900433 ) ) ;
#28095=CARTESIAN_POINT ( 'NONE',  ( 21.52544592524344225, -5.823673210054117533, 38.54057627198103120 ) ) ;
#28096=CARTESIAN_POINT ( 'NONE',  ( 9.564922557960805705, 16.46253265017160317, 79.58224293864769550 ) ) ;
#28097=CARTESIAN_POINT ( 'NONE',  ( 4.483927247898545687, 16.52544592524342804, 34.79057627198103120 ) ) ;
#28099=CARTESIAN_POINT ( 'NONE',  ( -18.87255363501902750, -5.500000000000066613, 81.32513748171831480 ) ) ;
#28100=CARTESIAN_POINT ( 'NONE',  ( -19.02544592524334988, -5.153800228976617603, 93.95942372801900433 ) ) ;
#28101=CARTESIAN_POINT ( 'NONE',  ( -5.823673210054116645, -21.52544592524344225, 67.29057627198103830 ) ) ;
#28102=CARTESIAN_POINT ( 'NONE',  ( 16.52544592524342804, -4.483927247898539470, 48.54057627198103120 ) ) ;
#28103=CARTESIAN_POINT ( 'NONE',  ( -8.224510206698735004, -14.34966873604973081, 29.58442372801901854 ) ) ;
#28104=CARTESIAN_POINT ( 'NONE',  ( -5.049401038298153566, 19.05341960407611168, 45.20724293864769550 ) ) ;
#28105=CARTESIAN_POINT ( 'NONE',  ( 5.719274019375991003, -21.55341960407610458, 112.7072429386476955 ) ) ;
#28106=CARTESIAN_POINT ( 'NONE',  ( -9.474510206698720793, -16.51473224551083518, 89.58442372801900433 ) ) ;
#28107=CARTESIAN_POINT ( 'NONE',  ( -16.51473224551069308, -9.474510206698971260, 76.66557627198103830 ) ) ;
#28108=CARTESIAN_POINT ( 'NONE',  ( -0.05219959533910754901, -16.53943276465976808, 87.49890960531436690 ) ) ;
#28110=CARTESIAN_POINT ( 'NONE',  ( 19.03943276465977164, -0.05219959533909143690, 68.74890960531436690 ) ) ;
#28111=CARTESIAN_POINT ( 'NONE',  ( -5.823673210054116645, -21.52544592524344225, 77.29057627198102409 ) ) ;
#28112=CARTESIAN_POINT ( 'NONE',  ( 16.46253265017160672, -9.564922557960803928, 33.33224293864770260 ) ) ;
#28114=CARTESIAN_POINT ( 'NONE',  ( -16.53943276465976808, 0.05219959533911058130, 56.24890960531436690 ) ) ;
#28115=CARTESIAN_POINT ( 'NONE',  ( -19.03943276465977164, 0.05219959533909376836, 91.24890960531436690 ) ) ;
#28117=CARTESIAN_POINT ( 'NONE',  ( -5.049401038297874678, -19.05341960407617918, 49.79275706135231871 ) ) ;
#28118=CARTESIAN_POINT ( 'NONE',  ( -15.80617190586745835, -15.72974639402198527, 71.87390960531438111 ) ) ;
#28119=CARTESIAN_POINT ( 'NONE',  ( -13.89961937509957401, -13.97604488694547875, 34.37609039468566863 ) ) ;
#28120=CARTESIAN_POINT ( 'NONE',  ( 19.05341960407611168, 5.049401038298154454, 83.95724293864766707 ) ) ;
#28121=CARTESIAN_POINT ( 'NONE',  ( -19.03943276465977164, -1.327063459122257427E-13, 20.00000000000001776 ) ) ;
#28122=CARTESIAN_POINT ( 'NONE',  ( -21.53943276465977519, 0.05219959533907696930, 31.24890960531435979 ) ) ;
#28123=CARTESIAN_POINT ( 'NONE',  ( 19.03943276465977164, -0.05219959533909143690, 73.74890960531435269 ) ) ;
#28124=CARTESIAN_POINT ( 'NONE',  ( -18.67979575497193778, 10.72451020669871902, 53.33442372801901854 ) ) ;
#28125=CARTESIAN_POINT ( 'NONE',  ( 14.34966873604960469, 8.224510206698951720, 114.1655762719810383 ) ) ;
#28126=CARTESIAN_POINT ( 'NONE',  ( -21.53943276465977519, 0.05219959533907696930, 116.2489096053143669 ) ) ;
#28127=CARTESIAN_POINT ( 'NONE',  ( 19.05341960407611168, 5.049401038298154454, 93.95724293864769550 ) ) ;
#28129=CARTESIAN_POINT ( 'NONE',  ( -18.62759615963255300, -10.81492255796106328, 44.16775706135234714 ) ) ;
#28131=CARTESIAN_POINT ( 'NONE',  ( 0.05219959533909260263, 19.03943276465977164, 104.9989096053143669 ) ) ;
#28133=CARTESIAN_POINT ( 'NONE',  ( 5.823673210054125526, 21.52544592524343514, 104.7905762719810241 ) ) ;
#28134=CARTESIAN_POINT ( 'NONE',  ( 9.474510206698971260, -16.51473224551069308, 42.91557627198103120 ) ) ;
#28135=CARTESIAN_POINT ( 'NONE',  ( 0.05219959533934541429, -16.53943276465976808, 30.00109039468568284 ) ) ;
#28137=CARTESIAN_POINT ( 'NONE',  ( 15.72974639402176855, 15.80617190586768217, 106.8760903946856899 ) ) ;
#28138=CARTESIAN_POINT ( 'NONE',  ( 19.03943276465977164, -0.05219959533909143690, 43.74890960531435979 ) ) ;
#28139=CARTESIAN_POINT ( 'NONE',  ( -21.53943276465977519, -0.05219959533937600094, 93.75109039468567573 ) ) ;
#28140=CARTESIAN_POINT ( 'NONE',  ( 19.02544592524343514, -5.153800228976328945, 88.54057627198102409 ) ) ;
#28141=CARTESIAN_POINT ( 'NONE',  ( 10.72451020669871369, 18.67979575497193778, 57.08442372801901854 ) ) ;
#28143=CARTESIAN_POINT ( 'NONE',  ( -0.05219959533909027116, -19.03943276465977164, 102.4989096053143669 ) ) ;
#28144=CARTESIAN_POINT ( 'NONE',  ( -17.50000000000002487, 4.658240926743135724, 28.94470417816804186 ) ) ;
#28145=CARTESIAN_POINT ( 'NONE',  ( -0.05219959533934338120, 16.53943276465976808, 57.50109039468568994 ) ) ;
#28146=CARTESIAN_POINT ( 'NONE',  ( -14.34966873604972548, 8.224510206698743886, 63.33442372801900433 ) ) ;
#28147=CARTESIAN_POINT ( 'NONE',  ( -15.72974639402176322, -15.80617190586768395, 59.37609039468568284 ) ) ;
#28148=CARTESIAN_POINT ( 'NONE',  ( 21.52544592524334988, 5.823673210054432836, 86.45942372801901854 ) ) ;
#28150=CARTESIAN_POINT ( 'NONE',  ( 4.379528057220092307, 16.55341960407617563, 27.29275706135234358 ) ) ;
#28151=CARTESIAN_POINT ( 'NONE',  ( -0.05219959533909027116, -19.03943276465977164, 67.49890960531436690 ) ) ;
#28152=CARTESIAN_POINT ( 'NONE',  ( -5.153800228976328057, -19.02544592524343514, 97.29057627198099567 ) ) ;
#28153=CARTESIAN_POINT ( 'NONE',  ( 5.153800228976335163, 19.02544592524342804, 114.7905762719810241 ) ) ;
#28154=CARTESIAN_POINT ( 'NONE',  ( -5.049401038298153566, 19.05341960407611168, 25.20724293864768484 ) ) ;
#28155=CARTESIAN_POINT ( 'NONE',  ( 10.72451020669898902, -18.67979575497178502, 27.91557627198103830 ) ) ;
#28156=CARTESIAN_POINT ( 'NONE',  ( 8.224510206698742110, 14.34966873604972548, 87.08442372801901854 ) ) ;
#28157=CARTESIAN_POINT ( 'NONE',  ( -16.53943276465976808, 0.05219959533911058130, 81.24890960531436690 ) ) ;
#28158=CARTESIAN_POINT ( 'NONE',  ( -0.05219959533909027116, -19.03943276465977164, 62.49890960531435979 ) ) ;
#28159=CARTESIAN_POINT ( 'NONE',  ( 5.719274019375673035, 21.55341960407619339, 92.29275706135236135 ) ) ;
#28160=CARTESIAN_POINT ( 'NONE',  ( 17.48941328179922294, 5.058624476862394026, 21.78938172987509247 ) ) ;
#28161=CARTESIAN_POINT ( 'NONE',  ( 12.06949235617739724, 12.14591786802326823, 21.87609039468567573 ) ) ;
#28162=CARTESIAN_POINT ( 'NONE',  ( 0.05219959533910956823, 16.53943276465976808, 69.99890960531435269 ) ) ;
#28163=CARTESIAN_POINT ( 'NONE',  ( 18.62759615963255655, 10.81492255796105972, 31.66775706135234358 ) ) ;
#28164=CARTESIAN_POINT ( 'NONE',  ( -0.05219959533907301413, -21.53943276465977519, 67.49890960531436690 ) ) ;
#28165=CARTESIAN_POINT ( 'NONE',  ( -5.153800228976607833, 19.02544592524334988, 37.70942372801899722 ) ) ;
#28167=CARTESIAN_POINT ( 'NONE',  ( 19.05341960407611168, 5.049401038298154454, 83.95724293864766707 ) ) ;
#28168=CARTESIAN_POINT ( 'NONE',  ( 8.314922557960818139, 14.29746914071049879, 44.58224293864769550 ) ) ;
#28170=CARTESIAN_POINT ( 'NONE',  ( 16.53943276465976808, -0.05219959533910856209, 33.74890960531436690 ) ) ;
#28171=CARTESIAN_POINT ( 'NONE',  ( 0.05219959533934541429, -16.53943276465976808, 105.0010903946856757 ) ) ;
#28172=CARTESIAN_POINT ( 'NONE',  ( 16.51473224551083163, -9.474510206698727899, 70.83442372801900433 ) ) ;
#28173=CARTESIAN_POINT ( 'NONE',  ( 19.53091890409952214, 5.500000000000025757, 52.56097431831423705 ) ) ;
#28174=CARTESIAN_POINT ( 'NONE',  ( -10.81492255796078084, -18.62759615963271287, 22.08224293864769194 ) ) ;
#28175=CARTESIAN_POINT ( 'NONE',  ( 16.55341960407611168, 4.379528057220329451, 73.95724293864769550 ) ) ;
#28177=CARTESIAN_POINT ( 'NONE',  ( 16.46253265017160672, -9.564922557960803928, 28.33224293864769550 ) ) ;
#28178=CARTESIAN_POINT ( 'NONE',  ( 0.05219959533907565091, 21.53943276465977519, 29.99890960531435979 ) ) ;
#28179=CARTESIAN_POINT ( 'NONE',  ( -10.81492255796078084, -18.62759615963271287, 62.08224293864769550 ) ) ;
#28180=CARTESIAN_POINT ( 'NONE',  ( -19.05341960407611168, -5.049401038298163336, 21.45724293864768839 ) ) ;
#28181=CARTESIAN_POINT ( 'NONE',  ( 8.224510206698742110, 14.34966873604972548, 67.08442372801901854 ) ) ;
#28182=CARTESIAN_POINT ( 'NONE',  ( -5.153800228976328057, -19.02544592524343514, 52.29057627198100988 ) ) ;
#28183=CARTESIAN_POINT ( 'NONE',  ( -5.823673210054431948, 21.52544592524334988, 57.70942372801901143 ) ) ;
#28185=CARTESIAN_POINT ( 'NONE',  ( -14.34966873604960291, -8.224510206698953496, 101.6655762719810383 ) ) ;
#28186=CARTESIAN_POINT ( 'NONE',  ( -5.153800228976607833, 19.02544592524334988, 87.70942372801897591 ) ) ;
#28187=CARTESIAN_POINT ( 'NONE',  ( -17.31747979337948706, 6.344076630960993057, 48.62055131934816643 ) ) ;
#28188=DIRECTION ( 'NONE',  ( 0.000000000000000000, 0.000000000000000000, -1.000000000000000000 ) ) ;
#28189=CARTESIAN_POINT ( 'NONE',  ( 10.81492255796078972, 18.62759615963270932, 39.58224293864769550 ) ) ;
#28190=CARTESIAN_POINT ( 'NONE',  ( -17.49999999999999645, 5.500000000000000888, 108.7176903769643559 ) ) ;
#28191=CARTESIAN_POINT ( 'NONE',  ( 21.52544592524334988, 5.823673210054432836, 71.45942372801901854 ) ) ;
#28192=CARTESIAN_POINT ( 'NONE',  ( 4.483927247898790824, -16.52544592524335698, 55.20942372801902565 ) ) ;
#28193=CARTESIAN_POINT ( 'NONE',  ( 8.224510206698953496, -14.34966873604960469, 42.91557627198103120 ) ) ;
#28194=CARTESIAN_POINT ( 'NONE',  ( 0.05219959533907565091, 21.53943276465977519, 74.99890960531435269 ) ) ;
#28195=CARTESIAN_POINT ( 'NONE',  ( -15.72974639402197994, 15.80617190586746368, 60.62390960531437401 ) ) ;
#28197=CARTESIAN_POINT ( 'NONE',  ( 13.97604488694548053, -13.89961937509957401, 85.62609039468568994 ) ) ;
#28198=CARTESIAN_POINT ( 'NONE',  ( 0.05219959533909260263, 19.03943276465977164, 109.9989096053143669 ) ) ;
#28199=CARTESIAN_POINT ( 'NONE',  ( -9.564922557960796823, -16.46253265017161027, 52.08224293864768839 ) ) ;
#28200=CARTESIAN_POINT ( 'NONE',  ( -12.06949235617756955, 12.14591786802309770, 110.6239096053143669 ) ) ;
#28202=FACE_OUTER_BOUND ( 'NONE', #78803, .T. ) ;
#28204=CARTESIAN_POINT ( 'NONE',  ( -4.379528057220086978, -16.55341960407618274, 64.79275706135234714 ) ) ;
#28205=CARTESIAN_POINT ( 'NONE',  ( 15.72974639402199770, -15.80617190586745480, 103.1239096053143811 ) ) ;
#28206=CARTESIAN_POINT ( 'NONE',  ( -19.05341960407611168, -5.049401038298163336, 51.45724293864770260 ) ) ;
#28207=CARTESIAN_POINT ( 'NONE',  ( 15.72974639402176855, 15.80617190586768217, 46.87609039468568994 ) ) ;
#28208=CARTESIAN_POINT ( 'NONE',  ( 19.05341960407611168, 5.049401038298154454, 93.95724293864769550 ) ) ;
#28212=CARTESIAN_POINT ( 'NONE',  ( 10.81492255796106328, -18.62759615963255655, 35.41775706135234003 ) ) ;
#28213=CARTESIAN_POINT ( 'NONE',  ( -16.51473224551069308, -9.474510206698971260, 101.6655762719810241 ) ) ;
#28214=CARTESIAN_POINT ( 'NONE',  ( 13.97604488694548053, -13.89961937509957401, 85.62609039468568994 ) ) ;
#28215=CARTESIAN_POINT ( 'NONE',  ( -5.049401038297874678, -19.05341960407617918, 39.79275706135232582 ) ) ;
#28216=CARTESIAN_POINT ( 'NONE',  ( 5.823673210054125526, 21.52544592524343514, 94.79057627198105251 ) ) ;
#28217=CARTESIAN_POINT ( 'NONE',  ( -19.05341960407617563, 5.049401038297882671, 38.54275706135233293 ) ) ;
#28218=CARTESIAN_POINT ( 'NONE',  ( -9.474510206698720793, -16.51473224551083518, 44.58442372801900433 ) ) ;
#28219=CARTESIAN_POINT ( 'NONE',  ( -16.55341960407617563, 4.379528057220093196, 93.54275706135234714 ) ) ;
#28220=CARTESIAN_POINT ( 'NONE',  ( 0.05219959533909260263, 19.03943276465977164, 114.9989096053143669 ) ) ;
#28221=CARTESIAN_POINT ( 'NONE',  ( -13.97604488694527625, -13.89961937509977652, 71.87390960531433848 ) ) ;
#28223=CARTESIAN_POINT ( 'NONE',  ( 21.53943276465977519, 0.05219959533937863772, 76.25109039468568994 ) ) ;
#28224=CARTESIAN_POINT ( 'NONE',  ( -21.53943276465977519, -0.05219959533937600094, 78.75109039468568994 ) ) ;
#28226=CARTESIAN_POINT ( 'NONE',  ( 19.05341960407611168, 5.049401038298154454, 93.95724293864769550 ) ) ;
#28227=CARTESIAN_POINT ( 'NONE',  ( -15.72974639402176322, -15.80617190586768395, 59.37609039468568284 ) ) ;
#28228=CARTESIAN_POINT ( 'NONE',  ( -19.02544592524334988, -5.153800228976617603, 98.95942372801900433 ) ) ;
#28229=CARTESIAN_POINT ( 'NONE',  ( 19.03943276465977164, -0.05219959533909143690, 68.74890960531436690 ) ) ;
#28230=CARTESIAN_POINT ( 'NONE',  ( 13.89961937509977652, -13.97604488694527269, 108.1239096053143669 ) ) ;
#28231=CARTESIAN_POINT ( 'NONE',  ( 13.89961937509977652, -13.97604488694527269, 78.12390960531433848 ) ) ;
#28232=CARTESIAN_POINT ( 'NONE',  ( 17.50000000000002487, -3.194745095267013557, 22.41015012971208265 ) ) ;
#28233=CARTESIAN_POINT ( 'NONE',  ( 16.46253265017160672, -9.564922557960803928, 63.33224293864769550 ) ) ;
#28234=CARTESIAN_POINT ( 'NONE',  ( -19.03943276465977164, 0.05219959533909376836, 56.24890960531435979 ) ) ;
#28235=CARTESIAN_POINT ( 'NONE',  ( 5.823673210054125526, 21.52544592524343514, 109.7905762719810383 ) ) ;
#28236=CARTESIAN_POINT ( 'NONE',  ( 16.53943276465976808, 0.05219959533934440121, 81.25109039468568994 ) ) ;
#28238=CARTESIAN_POINT ( 'NONE',  ( -19.05341960407617563, 5.049401038297882671, 48.54275706135233293 ) ) ;
#28239=CARTESIAN_POINT ( 'NONE',  ( -13.89961937509977652, 13.97604488694528158, 80.62390960531436690 ) ) ;
#28240=CARTESIAN_POINT ( 'NONE',  ( -14.34966873604960291, -8.224510206698953496, 71.66557627198100988 ) ) ;
#28241=CARTESIAN_POINT ( 'NONE',  ( -16.55341960407611168, -4.379528057220339221, 111.4572429386476813 ) ) ;
#28242=CARTESIAN_POINT ( 'NONE',  ( 5.153800228976335163, 19.02544592524342804, 109.7905762719810099 ) ) ;
#28243=CARTESIAN_POINT ( 'NONE',  ( -16.46253265017160317, 9.564922557960807481, 105.8322429386476955 ) ) ;
#28244=CARTESIAN_POINT ( 'NONE',  ( 8.224510206698953496, -14.34966873604960469, 72.91557627198103830 ) ) ;
#28246=CARTESIAN_POINT ( 'NONE',  ( -9.474510206698720793, -16.51473224551083518, 34.58442372801899722 ) ) ;
#28247=CARTESIAN_POINT ( 'NONE',  ( -14.34966873604972548, 8.224510206698743886, 98.33442372801901854 ) ) ;
#28248=CARTESIAN_POINT ( 'NONE',  ( -19.02544592524342804, 5.153800228976336051, 76.04057627198102409 ) ) ;
#28249=CARTESIAN_POINT ( 'NONE',  ( -21.52544592524334988, -5.823673210054445271, 53.95942372801900433 ) ) ;
#28250=CARTESIAN_POINT ( 'NONE',  ( -5.719274019375978568, 21.55341960407610458, 40.20724293864769550 ) ) ;
#28251=CARTESIAN_POINT ( 'NONE',  ( -21.52544592524334988, -5.823673210054445271, 18.95942372801901143 ) ) ;
#28253=CARTESIAN_POINT ( 'NONE',  ( -18.62759615963270932, 10.81492255796079327, 75.83224293864769550 ) ) ;
#28254=CARTESIAN_POINT ( 'NONE',  ( -12.14591786802309592, -12.06949235617757132, 96.87390960531436690 ) ) ;
#28255=CARTESIAN_POINT ( 'NONE',  ( -16.46253265017146816, -9.564922557961047289, 59.16775706135233293 ) ) ;
#28256=CARTESIAN_POINT ( 'NONE',  ( 13.97604488694527802, 13.89961937509977652, 34.37390960531436690 ) ) ;
#28257=CARTESIAN_POINT ( 'NONE',  ( 5.049401038298161559, -19.05341960407611168, 82.70724293864770971 ) ) ;
#28258=CARTESIAN_POINT ( 'NONE',  ( 9.474510206698971260, -16.51473224551069308, 87.91557627198102409 ) ) ;
#28259=CARTESIAN_POINT ( 'NONE',  ( 14.34966873604960469, 8.224510206698951720, 104.1655762719810241 ) ) ;
#28261=CARTESIAN_POINT ( 'NONE',  ( 4.483927247898545687, 16.52544592524342804, 29.79057627198102409 ) ) ;
#28262=CARTESIAN_POINT ( 'NONE',  ( 4.483927247898790824, -16.52544592524335698, 35.20942372801901854 ) ) ;
#28263=CARTESIAN_POINT ( 'NONE',  ( -15.72974639402176322, -15.80617190586768395, 104.3760903946856899 ) ) ;
#28264=CARTESIAN_POINT ( 'NONE',  ( -19.03943276465977164, 0.05219959533909376836, 106.2489096053143669 ) ) ;
#28265=CARTESIAN_POINT ( 'NONE',  ( -15.80617190586768217, 15.72974639402176855, 23.12609039468567573 ) ) ;
#28266=CARTESIAN_POINT ( 'NONE',  ( -5.049401038298153566, 19.05341960407611168, 40.20724293864768839 ) ) ;
#28267=CARTESIAN_POINT ( 'NONE',  ( -4.483927247898782831, 16.52544592524335698, 47.70942372801902565 ) ) ;
#28268=CARTESIAN_POINT ( 'NONE',  ( 13.89961937509957401, 13.97604488694547697, 101.8760903946856331 ) ) ;
#28269=CARTESIAN_POINT ( 'NONE',  ( -16.46253265017160317, 9.564922557960807481, 35.83224293864768839 ) ) ;
#28270=CARTESIAN_POINT ( 'NONE',  ( -4.483927247898539470, -16.52544592524342804, 97.29057627198105251 ) ) ;
#28271=CARTESIAN_POINT ( 'NONE',  ( -5.719274019375978568, 21.55341960407610458, 110.2072429386477239 ) ) ;
#28272=CARTESIAN_POINT ( 'NONE',  ( 0.05219959533936267826, -19.03943276465977164, 80.00109039468567573 ) ) ;
#28273=CARTESIAN_POINT ( 'NONE',  ( 9.564922557960805705, 16.46253265017160317, 24.58224293864769194 ) ) ;
#28274=CARTESIAN_POINT ( 'NONE',  ( 5.153800228976335163, 19.02544592524342804, 89.79057627198102409 ) ) ;
#28275=CARTESIAN_POINT ( 'NONE',  ( 18.67979575497194134, -10.72451020669871369, 20.83442372801901143 ) ) ;
#28276=CARTESIAN_POINT ( 'NONE',  ( 13.89961937509977652, -13.97604488694527269, 23.12390960531436335 ) ) ;
#28277=CARTESIAN_POINT ( 'NONE',  ( 5.049401038298161559, -19.05341960407611168, 87.70724293864769550 ) ) ;
#28278=DIRECTION ( 'NONE',  ( 0.000000000000000000, 0.000000000000000000, -1.000000000000000000 ) ) ;
#28279=CARTESIAN_POINT ( 'NONE',  ( -16.46253265017160317, 9.564922557960807481, 85.83224293864769550 ) ) ;
#28280=CARTESIAN_POINT ( 'NONE',  ( -21.52544592524334988, -5.823673210054445271, 28.95942372801902209 ) ) ;
#28281=CARTESIAN_POINT ( 'NONE',  ( 4.483927247898545687, 16.52544592524342804, 89.79057627198103830 ) ) ;
#28282=CARTESIAN_POINT ( 'NONE',  ( 9.474510206698971260, -16.51473224551069308, 92.91557627198103830 ) ) ;
#28283=CARTESIAN_POINT ( 'NONE',  ( -9.474510206698720793, -16.51473224551083518, 29.58442372801900433 ) ) ;
#28284=CARTESIAN_POINT ( 'NONE',  ( 12.14591786802327356, -12.06949235617739191, 45.62609039468567573 ) ) ;
#28285=CARTESIAN_POINT ( 'NONE',  ( -21.53943276465977519, -0.05219959533937600094, 63.75109039468568284 ) ) ;
#28286=CARTESIAN_POINT ( 'NONE',  ( 12.14591786802327356, -12.06949235617739191, 25.62609039468567929 ) ) ;
#28287=CARTESIAN_POINT ( 'NONE',  ( -9.474510206698964154, 16.51473224551069663, 75.41557627198103830 ) ) ;
#28288=CARTESIAN_POINT ( 'NONE',  ( 16.46253265017146816, 9.564922557961045513, 96.66775706135233293 ) ) ;
#28289=CARTESIAN_POINT ( 'NONE',  ( -14.34966873604972548, 8.224510206698743886, 68.33442372801900433 ) ) ;
#28290=CARTESIAN_POINT ( 'NONE',  ( 15.72974639402176855, 15.80617190586768217, 111.8760903946856615 ) ) ;
#28291=CARTESIAN_POINT ( 'NONE',  ( -13.89961937509957401, -13.97604488694547875, 84.37609039468567573 ) ) ;
#28292=CARTESIAN_POINT ( 'NONE',  ( 16.51473224551069308, 9.474510206698969483, 54.16557627198103120 ) ) ;
#28293=CARTESIAN_POINT ( 'NONE',  ( 21.53943276465977519, -0.05219959533907433946, 88.74890960531436690 ) ) ;
#28294=CARTESIAN_POINT ( 'NONE',  ( 8.314922557960818139, 14.29746914071049879, 79.58224293864769550 ) ) ;
#28295=CARTESIAN_POINT ( 'NONE',  ( -16.51473224551082808, 9.474510206698731452, 73.33442372801900433 ) ) ;
#28297=CARTESIAN_POINT ( 'NONE',  ( 5.049401038297881783, 19.05341960407617563, 62.29275706135234003 ) ) ;
#28298=CARTESIAN_POINT ( 'NONE',  ( -12.14591786802309592, -12.06949235617757132, 21.87390960531436690 ) ) ;
#28299=CARTESIAN_POINT ( 'NONE',  ( -8.314922557960811034, -14.29746914071050412, 67.08224293864770971 ) ) ;
#28300=CARTESIAN_POINT ( 'NONE',  ( 15.80617190586769283, -15.72974639402175789, 100.6260903946857184 ) ) ;
#28302=CARTESIAN_POINT ( 'NONE',  ( 21.53943276465977519, -0.05219959533907433946, 103.7489096053143669 ) ) ;
#28303=CARTESIAN_POINT ( 'NONE',  ( 9.474510206698971260, -16.51473224551069308, 62.91557627198102409 ) ) ;
#28304=CARTESIAN_POINT ( 'NONE',  ( -15.80617190586768217, 15.72974639402176855, 88.12609039468570415 ) ) ;
#28305=CARTESIAN_POINT ( 'NONE',  ( 16.51473224551069308, 9.474510206698969483, 69.16557627198102409 ) ) ;
#28307=CARTESIAN_POINT ( 'NONE',  ( 14.34966873604960469, 8.224510206698951720, 114.1655762719810383 ) ) ;
#28308=CARTESIAN_POINT ( 'NONE',  ( -18.62759615963270932, 10.81492255796079327, 30.83224293864770260 ) ) ;
#28309=CARTESIAN_POINT ( 'NONE',  ( -14.29746914071049879, 8.314922557960819915, 65.83224293864769550 ) ) ;
#28310=CARTESIAN_POINT ( 'NONE',  ( 13.89961937509977652, -13.97604488694527269, 48.12390960531435979 ) ) ;
#28311=CARTESIAN_POINT ( 'NONE',  ( -16.53943276465976808, 0.05219959533911058130, 96.24890960531435269 ) ) ;
#28313=CARTESIAN_POINT ( 'NONE',  ( 5.719274019375991003, -21.55341960407610458, 112.7072429386476955 ) ) ;
#28314=CARTESIAN_POINT ( 'NONE',  ( -18.62759615963255300, -10.81492255796106328, 49.16775706135234003 ) ) ;
#28315=CARTESIAN_POINT ( 'NONE',  ( -13.97604488694527625, -13.89961937509977652, 26.87390960531434558 ) ) ;
#28316=CARTESIAN_POINT ( 'NONE',  ( 4.483927247898790824, -16.52544592524335698, 65.20942372801901854 ) ) ;
#28317=CARTESIAN_POINT ( 'NONE',  ( -0.05219959533907301413, -21.53943276465977519, 102.4989096053143811 ) ) ;
#28318=CARTESIAN_POINT ( 'NONE',  ( 18.62759615963271287, -10.81492255796078972, 93.33224293864769550 ) ) ;
#28319=CARTESIAN_POINT ( 'NONE',  ( 5.153800228976615827, -19.02544592524334988, 30.20942372801900433 ) ) ;
#28320=CARTESIAN_POINT ( 'NONE',  ( 16.46253265017160672, -9.564922557960803928, 53.33224293864768839 ) ) ;
#28322=CARTESIAN_POINT ( 'NONE',  ( -0.05219959533937732626, 21.53943276465977519, 57.50109039468568994 ) ) ;
#28323=CARTESIAN_POINT ( 'NONE',  ( 21.53943276465977519, -0.05219959533907433946, 53.74890960531437401 ) ) ;
#28324=CARTESIAN_POINT ( 'NONE',  ( -12.06949235617756955, 12.14591786802309770, 30.62390960531436335 ) ) ;
#28325=CARTESIAN_POINT ( 'NONE',  ( -21.52544592524334988, -5.823673210054445271, 78.95942372801901854 ) ) ;
#28326=CARTESIAN_POINT ( 'NONE',  ( 21.52544592524334988, 5.823673210054432836, 101.4594237280190185 ) ) ;
#28327=CARTESIAN_POINT ( 'NONE',  ( 9.564922557961047289, -16.46253265017146816, 50.41775706135233293 ) ) ;
#28328=CARTESIAN_POINT ( 'NONE',  ( 8.224510206698742110, 14.34966873604972548, 107.0844237280190043 ) ) ;
#28329=CARTESIAN_POINT ( 'NONE',  ( 21.53943276465977519, 0.05219959533937863772, 61.25109039468567573 ) ) ;
#28330=CARTESIAN_POINT ( 'NONE',  ( -16.46253265017160317, 9.564922557960807481, 60.83224293864769550 ) ) ;
#28331=CARTESIAN_POINT ( 'NONE',  ( -5.049401038297874678, -19.05341960407617918, 34.79275706135233293 ) ) ;
#28332=CARTESIAN_POINT ( 'NONE',  ( -15.80617190586745835, -15.72974639402198527, 41.87390960531435979 ) ) ;
#28333=CARTESIAN_POINT ( 'NONE',  ( -21.55341960407619339, 5.719274019375674811, 28.54275706135234358 ) ) ;
#28334=CARTESIAN_POINT ( 'NONE',  ( 0.05219959533907565091, 21.53943276465977519, 84.99890960531436690 ) ) ;
#28335=CARTESIAN_POINT ( 'NONE',  ( -5.049401038297874678, -19.05341960407617918, 89.79275706135230450 ) ) ;
#28336=CARTESIAN_POINT ( 'NONE',  ( 16.55341960407618274, -4.379528057220086978, 56.04275706135235424 ) ) ;
#28337=CARTESIAN_POINT ( 'NONE',  ( 17.50000000000001066, -5.272787497354020303, 36.27284815830161335 ) ) ;
#28338=CARTESIAN_POINT ( 'NONE',  ( 21.52544592524344225, -5.823673210054117533, 98.54057627198105251 ) ) ;
#28339=CARTESIAN_POINT ( 'NONE',  ( 12.06949235617739724, 12.14591786802326823, 76.87609039468567573 ) ) ;
#28340=CARTESIAN_POINT ( 'NONE',  ( -4.379528057220328563, 16.55341960407611168, 75.20724293864769550 ) ) ;
#28342=CARTESIAN_POINT ( 'NONE',  ( 16.46253265017146816, 9.564922557961045513, 106.6677570613523471 ) ) ;
#28344=CARTESIAN_POINT ( 'NONE',  ( 10.72451020669898902, -18.67979575497178502, 32.91557627198102409 ) ) ;
#28346=CARTESIAN_POINT ( 'NONE',  ( 0.05219959533934541429, -16.53943276465976808, 55.00109039468568284 ) ) ;
#28347=CARTESIAN_POINT ( 'NONE',  ( 21.55341960407610458, 5.719274019375980345, 108.9572429386476955 ) ) ;
#28348=CARTESIAN_POINT ( 'NONE',  ( -15.72974639402197994, 15.80617190586746368, 30.62390960531436335 ) ) ;
#28349=CARTESIAN_POINT ( 'NONE',  ( 16.53943276465976808, 0.05219959533934440121, 76.25109039468568994 ) ) ;
#28350=CARTESIAN_POINT ( 'NONE',  ( -13.97604488694527625, -13.89961937509977652, 86.87390960531436690 ) ) ;
#28351=CARTESIAN_POINT ( 'NONE',  ( 18.67979575497194134, -10.72451020669871369, 55.83442372801901854 ) ) ;
#28352=CARTESIAN_POINT ( 'NONE',  ( 16.46253265017160672, -9.564922557960803928, 33.33224293864770260 ) ) ;
#28353=CARTESIAN_POINT ( 'NONE',  ( 15.72974639402199770, -15.80617190586745480, 23.12390960531436335 ) ) ;
#28354=ORIENTED_EDGE ( 'NONE', *, *, #57463, .F. ) ;
#28355=CARTESIAN_POINT ( 'NONE',  ( 9.564922557961047289, -16.46253265017146816, 40.41775706135234003 ) ) ;
#28356=CARTESIAN_POINT ( 'NONE',  ( -4.483927247898782831, 16.52544592524335698, 57.70942372801901143 ) ) ;
#28357=CARTESIAN_POINT ( 'NONE',  ( -19.05341960407611168, -5.049401038298163336, 111.4572429386476671 ) ) ;
#28358=CARTESIAN_POINT ( 'NONE',  ( -19.05341960407611168, -5.049401038298163336, 76.45724293864769550 ) ) ;
#28359=CARTESIAN_POINT ( 'NONE',  ( -8.224510206698735004, -14.34966873604973081, 104.5844237280190185 ) ) ;
#28361=CARTESIAN_POINT ( 'NONE',  ( 16.52544592524342804, -4.483927247898539470, 93.54057627198103830 ) ) ;
#28362=CARTESIAN_POINT ( 'NONE',  ( 5.823673210054125526, 21.52544592524343514, 39.79057627198103830 ) ) ;
#28363=CARTESIAN_POINT ( 'NONE',  ( 5.153800228976335163, 19.02544592524342804, 34.79057627198102409 ) ) ;
#28364=CARTESIAN_POINT ( 'NONE',  ( 14.34966873604972726, -8.224510206698740333, 70.83442372801901854 ) ) ;
#28365=CARTESIAN_POINT ( 'NONE',  ( -21.52544592524334988, -5.823673210054445271, 23.95942372801901143 ) ) ;
#28366=CARTESIAN_POINT ( 'NONE',  ( 5.153800228976615827, -19.02544592524334988, 70.20942372801899012 ) ) ;
#28367=CARTESIAN_POINT ( 'NONE',  ( -16.46253265017160317, 9.564922557960807481, 45.83224293864769550 ) ) ;
#28368=CARTESIAN_POINT ( 'NONE',  ( 5.823673210054125526, 21.52544592524343514, 74.79057627198105251 ) ) ;
#28370=CARTESIAN_POINT ( 'NONE',  ( -15.72974639402176322, -15.80617190586768395, 89.37609039468568994 ) ) ;
#28371=CARTESIAN_POINT ( 'NONE',  ( 16.46253265017160672, -9.564922557960803928, 63.33224293864769550 ) ) ;
#28372=CARTESIAN_POINT ( 'NONE',  ( 14.34966873604972726, -8.224510206698740333, 50.83442372801901143 ) ) ;
#28373=CARTESIAN_POINT ( 'NONE',  ( -15.80617190586768217, 15.72974639402176855, 73.12609039468567573 ) ) ;
#28374=CARTESIAN_POINT ( 'NONE',  ( -5.153800228976607833, 19.02544592524334988, 37.70942372801899722 ) ) ;
#28375=CARTESIAN_POINT ( 'NONE',  ( -5.049401038297874678, -19.05341960407617918, 54.79275706135234003 ) ) ;
#28377=CARTESIAN_POINT ( 'NONE',  ( -21.53943276465977519, -0.05219959533937600094, 43.75109039468568284 ) ) ;
#28379=CARTESIAN_POINT ( 'NONE',  ( -5.049401038297874678, -19.05341960407617918, 44.79275706135232582 ) ) ;
#28380=CARTESIAN_POINT ( 'NONE',  ( -16.46253265017160317, 9.564922557960807481, 105.8322429386476955 ) ) ;
#28381=CARTESIAN_POINT ( 'NONE',  ( -13.97604488694527625, -13.89961937509977652, 76.87390960531433848 ) ) ;
#28382=CARTESIAN_POINT ( 'NONE',  ( -12.06949235617756955, 12.14591786802309770, 40.62390960531435269 ) ) ;
#28383=CARTESIAN_POINT ( 'NONE',  ( -5.823673210054116645, -21.52544592524344225, 37.29057627198102409 ) ) ;
#28385=CARTESIAN_POINT ( 'NONE',  ( 17.40861289039004234, 6.110651285853276882, 58.87232470827434838 ) ) ;
#28386=CARTESIAN_POINT ( 'NONE',  ( 15.80617190586769283, -15.72974639402175789, 100.6260903946857184 ) ) ;
#28388=CARTESIAN_POINT ( 'NONE',  ( 9.474510206698971260, -16.51473224551069308, 42.91557627198103120 ) ) ;
#28391=CARTESIAN_POINT ( 'NONE',  ( 8.224510206698742110, 14.34966873604972548, 47.08442372801901854 ) ) ;
#28392=CARTESIAN_POINT ( 'NONE',  ( 15.72974639402199770, -15.80617190586745480, 63.12390960531435979 ) ) ;
#28393=CARTESIAN_POINT ( 'NONE',  ( 14.34966873604960469, 8.224510206698951720, 34.16557627198102409 ) ) ;
#28394=CARTESIAN_POINT ( 'NONE',  ( -19.03943276465977164, 0.05219959533909376836, 26.24890960531435624 ) ) ;
#28395=CARTESIAN_POINT ( 'NONE',  ( 0.05219959533909260263, 19.03943276465977164, 104.9989096053143669 ) ) ;
#28396=CARTESIAN_POINT ( 'NONE',  ( 21.53943276465977519, 0.05219959533937863772, 31.25109039468568639 ) ) ;
#28397=CARTESIAN_POINT ( 'NONE',  ( -13.89961937509957401, -13.97604488694547875, 29.37609039468565797 ) ) ;
#28398=CARTESIAN_POINT ( 'NONE',  ( -12.06949235617756955, 12.14591786802309770, 115.6239096053143669 ) ) ;
#28399=CARTESIAN_POINT ( 'NONE',  ( -10.81492255796105439, 18.62759615963255655, 82.91775706135234714 ) ) ;
#28401=CARTESIAN_POINT ( 'NONE',  ( -0.05219959533910754901, -16.53943276465976808, 32.49890960531435979 ) ) ;
#28403=CARTESIAN_POINT ( 'NONE',  ( 15.72974639402199770, -15.80617190586745480, 28.12390960531435979 ) ) ;
#28404=CARTESIAN_POINT ( 'NONE',  ( 4.483927247898545687, 16.52544592524342804, 84.79057627198102409 ) ) ;
#28406=CARTESIAN_POINT ( 'NONE',  ( 13.97604488694527802, 13.89961937509977652, 79.37390960531435269 ) ) ;
#28407=CARTESIAN_POINT ( 'NONE',  ( -12.14591786802309592, -12.06949235617757132, 71.87390960531438111 ) ) ;
#28408=CARTESIAN_POINT ( 'NONE',  ( 16.46253265017146816, 9.564922557961045513, 101.6677570613523329 ) ) ;
#28410=EDGE_CURVE ( 'NONE', #170763, #111352, #40193, .T. ) ;
#28411=CARTESIAN_POINT ( 'NONE',  ( 21.55341960407610458, 5.719274019375980345, 63.95724293864770260 ) ) ;
#28413=CARTESIAN_POINT ( 'NONE',  ( -19.03943276465977164, 0.05219959533909376836, 36.24890960531436690 ) ) ;
#28414=CARTESIAN_POINT ( 'NONE',  ( -13.89961937509977652, 13.97604488694528158, 70.62390960531432427 ) ) ;
#28415=CARTESIAN_POINT ( 'NONE',  ( -15.72974639402197994, 15.80617190586746368, 70.62390960531436690 ) ) ;
#28416=CARTESIAN_POINT ( 'NONE',  ( -16.53943276465976808, -0.05219959533934237506, 108.7510903946857042 ) ) ;
#28417=CARTESIAN_POINT ( 'NONE',  ( 16.51473224551069308, 9.474510206698969483, 89.16557627198103830 ) ) ;
#28418=CARTESIAN_POINT ( 'NONE',  ( 16.46253265017146816, 9.564922557961045513, 71.66775706135233293 ) ) ;
#28419=CARTESIAN_POINT ( 'NONE',  ( 21.55341960407619695, -5.719274019375665929, 96.04275706135236135 ) ) ;
#28420=CARTESIAN_POINT ( 'NONE',  ( 21.55341960407610458, 5.719274019375980345, 78.95724293864769550 ) ) ;
#28421=CARTESIAN_POINT ( 'NONE',  ( 19.02544592524343514, -5.153800228976328945, 113.5405762719810241 ) ) ;
#28422=CARTESIAN_POINT ( 'NONE',  ( 5.153800228976335163, 19.02544592524342804, 44.79057627198103830 ) ) ;
#28423=CARTESIAN_POINT ( 'NONE',  ( 16.53943276465976808, 0.05219959533934440121, 111.2510903946856899 ) ) ;
#28424=CARTESIAN_POINT ( 'NONE',  ( 9.474510206698971260, -16.51473224551069308, 67.91557627198102409 ) ) ;
#28425=CARTESIAN_POINT ( 'NONE',  ( -17.59860650958993844, 7.585241751806885979, 83.42337014262491834 ) ) ;
#28426=CARTESIAN_POINT ( 'NONE',  ( 18.62759615963255655, 10.81492255796105972, 106.6677570613523756 ) ) ;
#28427=CARTESIAN_POINT ( 'NONE',  ( -0.05219959533910754901, -16.53943276465976808, 67.49890960531436690 ) ) ;
#28428=CARTESIAN_POINT ( 'NONE',  ( 0.05219959533907565091, 21.53943276465977519, 114.9989096053143669 ) ) ;
#28429=CARTESIAN_POINT ( 'NONE',  ( -10.72451020669898014, 18.67979575497178502, 100.4155762719810241 ) ) ;
#28431=CARTESIAN_POINT ( 'NONE',  ( -21.52544592524343514, 5.823673210054127303, 56.04057627198102409 ) ) ;
#28432=CARTESIAN_POINT ( 'NONE',  ( 16.52544592524335698, 4.483927247898782831, 81.45942372801900433 ) ) ;
#28433=CARTESIAN_POINT ( 'NONE',  ( -8.224510206698948167, 14.34966873604960824, 105.4155762719810383 ) ) ;
#28434=B_SPLINE_CURVE_WITH_KNOTS ( 'NONE', 3,
 ( #136601, #197301, #164974, #59759, #121427, #179153 ),
 .UNSPECIFIED., .F., .F.,
 ( 4, 2, 4 ),
 ( 0.003989672132298133916, 0.004372778065220557162, 0.004755883998142979539 ),
 .UNSPECIFIED. ) ;
#28435=CARTESIAN_POINT ( 'NONE',  ( 9.474510206698971260, -16.51473224551069308, 52.91557627198102409 ) ) ;
#28436=CARTESIAN_POINT ( 'NONE',  ( 8.224510206698742110, 14.34966873604972548, 112.0844237280190185 ) ) ;
#28438=CARTESIAN_POINT ( 'NONE',  ( 10.81492255796106328, -18.62759615963255655, 45.41775706135234003 ) ) ;
#28439=CARTESIAN_POINT ( 'NONE',  ( -5.049401038298153566, 19.05341960407611168, 110.2072429386476671 ) ) ;
#28440=CARTESIAN_POINT ( 'NONE',  ( -10.81492255796105439, 18.62759615963255655, 77.91775706135231871 ) ) ;
#28441=CARTESIAN_POINT ( 'NONE',  ( 13.89961937509977652, -13.97604488694527269, 33.12390960531434558 ) ) ;
#28442=CARTESIAN_POINT ( 'NONE',  ( -5.049401038298153566, 19.05341960407611168, 35.20724293864768839 ) ) ;
#28443=ORIENTED_EDGE ( 'NONE', *, *, #54823, .F. ) ;
#28444=CARTESIAN_POINT ( 'NONE',  ( 0.05219959533937995610, -21.53943276465977519, 70.00109039468568994 ) ) ;
#28445=CARTESIAN_POINT ( 'NONE',  ( 16.51473224551069308, 9.474510206698969483, 109.1655762719810383 ) ) ;
#28446=CARTESIAN_POINT ( 'NONE',  ( -5.049401038297874678, -19.05341960407617918, 79.79275706135233293 ) ) ;
#28447=CARTESIAN_POINT ( 'NONE',  ( 21.52544592524334988, 5.823673210054432836, 41.45942372801901143 ) ) ;
#28448=CARTESIAN_POINT ( 'NONE',  ( 8.314922557961029526, -14.29746914071037800, 25.41775706135235779 ) ) ;
#28449=CARTESIAN_POINT ( 'NONE',  ( 13.97604488694548053, -13.89961937509957401, 70.62609039468567573 ) ) ;
#28450=CARTESIAN_POINT ( 'NONE',  ( -0.05219959533909027116, -19.03943276465977164, 47.49890960531435979 ) ) ;
#28451=CARTESIAN_POINT ( 'NONE',  ( -5.153800228976607833, 19.02544592524334988, 87.70942372801897591 ) ) ;
#28452=CARTESIAN_POINT ( 'NONE',  ( 14.29746914071049879, -8.314922557960816363, 28.33224293864769550 ) ) ;
#28453=CARTESIAN_POINT ( 'NONE',  ( -16.51473224551082808, 9.474510206698731452, 93.33442372801900433 ) ) ;
#28454=CARTESIAN_POINT ( 'NONE',  ( -16.53943276465976808, 0.05219959533911058130, 41.24890960531435269 ) ) ;
#28455=CARTESIAN_POINT ( 'NONE',  ( -9.564922557961040184, 16.46253265017147172, 62.91775706135233293 ) ) ;
#28456=CARTESIAN_POINT ( 'NONE',  ( 8.224510206698742110, 14.34966873604972548, 42.08442372801901854 ) ) ;
#28457=CARTESIAN_POINT ( 'NONE',  ( 9.564922557961047289, -16.46253265017146816, 25.41775706135234003 ) ) ;
#28458=CARTESIAN_POINT ( 'NONE',  ( 19.02544592524343514, -5.153800228976328945, 48.54057627198103120 ) ) ;
#28459=CARTESIAN_POINT ( 'NONE',  ( -18.22780087662121673, -5.500000000000062172, 66.48459894673892734 ) ) ;
#28460=CARTESIAN_POINT ( 'NONE',  ( 12.06949235617739724, 12.14591786802326823, 46.87609039468568994 ) ) ;
#28463=CARTESIAN_POINT ( 'NONE',  ( -16.51473224551069308, -9.474510206698971260, 91.66557627198103830 ) ) ;
#28464=CARTESIAN_POINT ( 'NONE',  ( 0.05219959533936267826, -19.03943276465977164, 85.00109039468567573 ) ) ;
#28466=CARTESIAN_POINT ( 'NONE',  ( -5.153800228976607833, 19.02544592524334988, 87.70942372801897591 ) ) ;
#28467=CARTESIAN_POINT ( 'NONE',  ( 18.62759615963271287, -10.81492255796078972, 28.33224293864769550 ) ) ;
#28468=CARTESIAN_POINT ( 'NONE',  ( -5.153800228976607833, 19.02544592524334988, 22.70942372801899012 ) ) ;
#28469=CARTESIAN_POINT ( 'NONE',  ( -16.51473224551082808, 9.474510206698731452, 98.33442372801900433 ) ) ;
#28470=CARTESIAN_POINT ( 'NONE',  ( 0.05219959533910956823, 16.53943276465976808, 109.9989096053143527 ) ) ;
#28471=CARTESIAN_POINT ( 'NONE',  ( -9.474510206698964154, 16.51473224551069663, 35.41557627198102409 ) ) ;
#28472=CARTESIAN_POINT ( 'NONE',  ( 21.52544592524344225, -5.823673210054117533, 58.54057627198103120 ) ) ;
#28473=( BOUNDED_SURFACE ( )  B_SPLINE_SURFACE ( 3, 2, ( 
 ( #138517, #94998, #141505, #123337, #30355, #40392, #64668, #61668, #156684, #126330, #113887, #140507, #79835, #175585, #17175, #83553, #1996, #60678, #2990, #122353, #160414, #46517, #21903, #108176, #169857, #77838, #988, #170855, #47520, #125350, #109176, #32346, #93999, #9742, #192755, #40057, #134083, #68392, #41075, #38071, #178594, #10742, #26916, #72406, #99727, #114903, #163422, #103742, #85561, #100724, #180605, #24920, #148248, #84549, #147247, #54238, #8738, #86565, #6714, #101734, #165422, #87564, #130044, #23907, #118920, #145232, #179603, #71406, #53227, #115909, #164427, #56232, #42078, #191744, #133070, #176597, #131066, #161411, #22903, #146227, #132075, #7714, #69399, #194760, #177599, #39067, #162405, #117914, #70407, #193764, #102739, #55232, #116901, #25920, #149251, #195773, #57246, #169365, #91515, #89560, #73418, #121872, #92520, #183565, #104730, #77360, #196765, #199725, #12735, #153201, #28902, #166422, #27917, #135089, #138044, #181586, #151246, #15699, #76367, #139028, #122863, #167406, #106708, #45050, #14706, #105719, #507, #108692, #62179, #170370, #60202, #58233, #119901, #47035, #152224, #107687, #61191, #11751, #75375, #74401, #197741, #136067, #44059, #182576, #184551, #90542, #13709, #43064, #154210, #59207, #46032, #30874, #120876, #137045, #198737, #123843, #168382, #185541, #88558, #150257, #29877, #19666, #20649, #50008, #113646, #173361, #93515, #189527, #155201, #142991, #124860, #35822, #66158, #34831, #4469, #31862, #140014, #16690, #78340, #32857, #51987, #95502, #81307, #65166, #174351, #1502, #186559, #48031, #67157, #111674, #127821, #63180, #96486, #109688, #157188, #171369, #159153, #94507, #158175, #50999, #17688, #112660, #156189, #97468, #82303, #188531, #143993, #5474, #128814, #190513, #126825, #79346, #80329, #110673, #141017, #2504, #18682, #49018, #142001, #64184, #125850, #187551, #172353, #3489, #33842, #56997, #176350, #160167, #8487, #179361, #70163, #191499, #164181, #83310, #86322, #99483, #178350, #115668, #52975, #114652, #21657, #24672, #68149, #37823, #102496, #163168, #25679, #9499, #53994, #193514, #131832, #101478, #192510, #87324, #195524, #149009, #175340, #147001, #144987, #6468, #133833, #38827, #194514, #39813, #98473, #162164, #161164, #84307, #22660, #130819, #69153, #71163, #177357, #100485, #129800, #40824, #145986, #148009, #117664, #7469, #23661, #85309, #10497, #54990, #132828, #72158, #36807, #116659, #55988, #107444, #136803, #265, #59960, #180363, #76118, #41831, #29633, #11505, #122621, #152957, #121626, #91266, #118672, #26670, #103498, #165176, #119666, #138784, #182335, #106458, #151981, #60946, #88311, #73176, #134847, #153960, #198487, #168137, #149999, #183322, #196525, #43813, #57996, #45792, #181348, #44803, #14455, #104492, #137796, #42827, #199480, #184311, #75133, #169118, #30623, #92276, #15458, #13470, #77114, #167163, #197502, #166174, #27675, #105476, #135833, #28662, #89315, #151008, #12499, #74161, #90297, #58969, #120637, #64928, #49767, #50766, #80095, #143752, #3255, #123602, #19430, #185297, #173119, #154953, #65916, #96252, #126588, #34594, #61933, #170123, #46788, #108447, #62932, #82058, #125609, #111432, #95264, #4236, #31618, #16449, #78098, #97231, #141763, #157939, #93268, #188290, #139767, #187308, #1255, #189288, #124612, #81077, #142756, #47788, #127589, #186307, #112424, #174115, #18444, #35585, #158919, #20409, #109439, #156947, #171122, #110433, #140769, #32611, #94265, #48779, #79096, #172115, #155944, #17440, #2258, #63941, #33601, #176107, #87085, #8246, #6234, #190271, #38590, #9260, #100245, #21415, #194283, #113409, #116422, #129566, #69924, #145749, #83073, #144749, #51748, #54748, #98223, #67913, #132593, #193275, #55749, #39578, #84070, #23421, #161927, #131590, #22420, #117423, #25445, #179121, #5232, #177119, #175100, #36568, #163947, #68915, #24434 ),
 ( #37577, #85069, #40589, #102260, #70926, #191264, #52739, #178110, #146751, #66913, #101237, #130577, #128577, #159926, #114406, #162926, #99240, #7230, #160929, #192272, #86082, #147773, #53754, #115428, #57762, #150769, #166932, #10259, #43580, #168883, #91041, #133590, #27435, #122386, #30388, #183090, #182096, #56763, #119432, #167911, #59727, #184075, #45559, #105245, #195281, #134606, #103260, #107213, #148770, #135599, #11265, #71919, #28433, #196292, #118435, #41596, #13245, #12266, #180128, #90070, #89078, #73930, #164942, #44572, #121397, #151752, #29411, #74908, #26435, #88076, #106227, #181116, #149762, #72937, #152728, #42590, #14218, #136572, #198252, #197271, #75887, #137562, #199245, #104253, #165936, #58733, #60712, #120403, #111196, #189065, #185064, #171885, #48551, #169893, #127351, #124378, #79871, #186073, #110205, #19204, #142530, #157714, #154724, #31387, #95031, #33373, #50536, #141540, #155713, #61702, #172888, #123371, #156721, #76880, #17209, #28, #49534, #93036, #78862, #80853, #3029, #140542, #62696, #47556, #63710, #109209, #18213, #138551, #4008, #2030, #64705, #139539, #187082, #65687, #15221, #188063, #46552, #125385, #112198, #173888, #92035, #153725, #126367, #108214, #77872, #16218, #1023, #170888, #34367, #32380, #94034, #96028, #97989, #101004, #5000, #68674, #191032, #116188, #22181, #129337, #52507, #39345, #38349, #115186, #145512, #23186, #83831, #97008, #128345, #100004, #21180, #158690, #81825, #161691, #190044, #84829, #130328, #160690, #114167, #6993, #192025, #131350, #144515, #143512, #6000, #53509, #176879, #146509, #177877, #66683, #7999, #69683, #51518, #35357, #67679, #193038, #175870, #54515, #20179, #113180, #174870, #37342, #99000, #36336, #159683, #82835, #38636, #114453, #115474, #144797, #8293, #67958, #188336, #84115, #49814, #37624, #19476, #130623, #160973, #129613, #99286, #126634, #34639, #111479, #173164, #127634, #146800, #190317, #176154, #159972, #68961, #96299, #81122, #142802, #161971, #6280, #22467, #157985, #191308, #4283, #51794, #65963, #53799, #189334, #52784, #145794, #112469, #7277, #50811, #192319, #177163, #83120, #100293, #23467, #85116, #174162, #21459, #35632, #175146, #5281, #97277, #158965, #113453, #143798, #36614, #20456, #82106, #66963, #98270, #128624, #119476, #118482, #40634, #102303, #41641, #163992, #72982, #54795, #58777, #180172, #134651, #117468, #164985, #120445, #193321, #165980, #162974, #103306, #135643, #151795, #197313, #24479, #39624, #88122, #28477, #10306, #25489, #105286, #149806, #196337, #9306, #71963, #179166, #133637, #11312, #131637, #26480, #90111, #12308, #116470, #148816, #43622, #69971, #104298, #57805, #178159, #87131, #89124, #181159, #166974, #101284, #42635, #86129, #55796, #147820, #70972, #132640, #56808, #194328, #195328, #27481, #150812, #73974, #182139, #77915, #76924, #48595, #169938, #153771, #138595, #33417, #47598, #186118, #93082, #94077, #31429, #74950, #29453, #109251, #184123, #198294, #121439, #170931, #91085, #32422, #139582, #46598, #15266, #154766, #16264, #63753, #168929, #59771, #107258, #62742, #1067, #155756, #110246, #106269, #124422, #17254, #152772, #171928, #45605, #78907, #30435, #140584, #2074, #125427, #187123, #75933, #14264, #92082, #108258, #95076, #123415, #77, #183132, #13286, #44615, #136613, #167954, #61747, #137608, #199291, #60758, #122431, #185108, #127398, #141582, #64747, #114213, #172932, #175918, #21227, #190086, #97050, #36380, #159731, #7037, #112240, #3070, #50580, #6047, #144561, #37389, #53555, #49578, #98034, #113226, #34411, #192074, #189107, #67725, #173930, #174916, #83877, #68719, #22228, #19249, #96069, #35399, #51562, #129383, #66730, #20222, #126409, #99046, #188105, #82883, #111241, #81870, #157758, #160736, #80896, #143561, #145559, #191079, #5044, #158732, #128390, #52552, #130376, #115234, #142573, #176925, #38396 ),
 ( #156764, #18258, #4052, #79911, #65729, #85894, #118245, #100052, #87884, #26245, #56571, #180927, #165746, #164750, #196103, #133399, #88889, #148579, #178927, #27240, #84877, #25253, #117234, #86895, #131397, #42402, #24245, #193085, #10069, #70738, #181909, #103068, #101052, #146554, #195088, #104065, #179936, #116233, #150581, #8050, #11068, #147582, #149572, #40397, #177924, #39392, #69729, #72746, #54560, #162737, #12080, #134417, #73743, #57573, #9068, #132405, #71729, #194098, #161738, #119243, #55560, #102068, #41403, #135415, #197086, #163753, #58553, #120219, #23233, #167726, #46360, #183890, #121210, #59532, #28247, #92849, #136389, #182901, #170703, #31198, #93850, #77689, #122198, #61520, #200051, #169704, #60523, #155528, #63522, #32192, #125197, #15034, #151570, #13059, #1840, #107028, #62511, #108018, #166744, #30202, #106040, #152542, #29224, #199053, #137375, #139357, #45375, #168700, #74725, #47369, #89887, #154534, #91843, #198066, #44385, #90857, #109024, #14030, #75695, #153537, #123189, #17023, #16031, #78676, #184878, #43388, #838, #105060, #124183, #185884, #76694, #138371, #140352, #36151, #35167, #157524, #19018, #158507, #80664, #189859, #171699, #175676, #96822, #51333, #34179, #81638, #37150, #110019, #82642, #79680, #19994, #52320, #68484, #113978, #141351, #156528, #4807, #145323, #127160, #142340, #21993, #66496, #112993, #126183, #188868, #95840, #50351, #128159, #48364, #143320, #6806, #129147, #33188, #65498, #160503, #186893, #20986, #174687, #94847, #3820, #5814, #97803, #2838, #98809, #18027, #159492, #111008, #144325, #112010, #64516, #187878, #49346, #67489, #172694, #173699, #83646, #190844, #180693, #164515, #8826, #148337, #86653, #56322, #147339, #42169, #150346, #57334, #11842, #101823, #38164, #99819, #88650, #193854, #149336, #133158, #53317, #116990, #192846, #39155, #54326, #85652, #23995, #26008, #70495, #132162, #161504, #134174, #114995, #118005, #55319, #84642, #176689, #22994, #195862, #146319, #7808, #177687, #9832, #103829, #179694, #119010, #71492, #130139, #69492, #163511, #131157, #10831, #41166, #115998, #165509, #87650, #194850, #102829, #191836, #100811, #162495, #178684, #40146, #25009, #72500, #27006, #106797, #15789, #58319, #28008, #166510, #108783, #91608, #122953, #181673, #138134, #43153, #198825, #93607, #596, #104821, #199815, #46122, #59298, #153296, #73507, #61283, #184641, #29969, #154299, #139120, #107776, #169461, #168471, #62267, #121963, #152313, #123935, #119987, #60290, #90631, #183656, #89648, #77449, #197832, #151336, #45140, #44149, #155292, #76457, #74491, #12825, #14797, #185633, #136157, #92609, #120966, #182665, #105808, #30962, #47125, #170461, #167495, #31952, #135179, #196853, #28991, #13799, #75465, #137138, #49112, #19757, #1597, #5567, #65259, #81398, #64276, #111766, #67246, #140106, #112750, #109777, #50106, #82398, #98567, #144086, #171460, #186649, #34924, #175434, #157280, #172451, #52081, #96579, #143084, #156282, #18776, #125943, #80423, #158268, #78431, #173455, #36904, #159247, #63273, #95596, #190605, #16782, #51090, #4563, #124953, #187641, #35913, #127915, #113737, #48120, #66255, #32948, #2597, #94603, #17783, #79438, #3581, #141109, #110769, #189617, #33938, #142096, #126919, #174444, #188626, #97559, #20743, #128905, #23757, #180456, #194608, #132921, #39910, #40919, #178443, #21751, #176444, #56080, #130914, #145080, #68240, #117761, #37917, #179453, #24768, #193610, #100576, #101577, #163266, #10592, #115761, #6563, #54087, #9592, #148100, #102592, #57093, #53072, #86415, #116752, #99576, #195621, #192605, #71257, #177449, #164277, #87417, #72253, #25771, #22752, #161258, #38919, #55082, #149102, #70258, #85407, #133931, #84401, #146077, #162258, #118767, #41928, #131926, #147099, #129893, #160261, #191593, #114750, #7562, #83402, #69248, #8584, #42916, #28752, #92365, #153048 ),
 ( #26763, #199568, #196615, #136896, #169209, #185386, #30718, #58085, #73268, #121719, #62023, #43904, #59059, #138873, #183411, #106551, #104582, #105567, #12588, #167253, #44894, #165269, #198583, #123687, #45879, #88403, #182426, #77204, #103594, #137887, #60051, #11600, #74253, #122709, #14550, #353, #150099, #168227, #134937, #89408, #119755, #181438, #166267, #90388, #27765, #151097, #29724, #135923, #197593, #120726, #91356, #152073, #13558, #76208, #75224, #61037, #184399, #107533, #154051, #15546, #127673, #65016, #108537, #63025, #81160, #17529, #31709, #155044, #4321, #124703, #66004, #111518, #80178, #187397, #126672, #49853, #97317, #2347, #93358, #140858, #96337, #34679, #189373, #143840, #139855, #188376, #3341, #186400, #82144, #79188, #158024, #64028, #173203, #174201, #159003, #19515, #142842, #20496, #125698, #16539, #48865, #50850, #112507, #35669, #5319, #1344, #67003, #128662, #47877, #46877, #110520, #170216, #172201, #78186, #109530, #171212, #32702, #94353, #156032, #33686, #141850, #95349, #157033, #18531, #160012, #12104, #21500, #83161, #144835, #23508, #42428, #150608, #129651, #115517, #181934, #104090, #38678, #161013, #22507, #162012, #84154, #193361, #175188, #43415, #100334, #54837, #37665, #85156, #105085, #113493, #88916, #6319, #146842, #58577, #74749, #120243, #67998, #191347, #8336, #151593, #130666, #145833, #28272, #70011, #116511, #52825, #192360, #99330, #53843, #131680, #51834, #178199, #13084, #135440, #36654, #69000, #166771, #190357, #27267, #165773, #98312, #7315, #73767, #197110, #89911, #114494, #176196, #177205, #122223, #90883, #110047, #171727, #123212, #199080, #94875, #16056, #183914, #18055, #29249, #862, #200075, #33215, #92873, #76718, #61543, #156555, #170727, #109050, #77714, #17048, #154560, #198092, #152567, #32219, #107052, #121235, #44411, #93876, #14056, #155554, #62537, #169729, #138394, #124211, #78703, #45399, #139380, #136412, #185909, #47395, #140380, #1867, #63548, #125222, #186920, #31224, #48390, #184902, #15058, #59557, #182928, #46386, #153561, #108044, #167751, #106065, #60548, #75723, #137399, #168725, #30226, #91868, #80691, #64544, #113019, #83671, #174711, #95868, #68510, #187905, #190870, #3847, #82668, #20022, #157551, #19044, #126209, #129172, #172723, #142368, #6831, #67515, #130164, #114002, #158533, #97828, #36175, #5839, #96848, #191861, #99844, #53343, #161528, #51358, #49374, #111037, #38188, #143347, #98835, #144352, #2866, #66522, #65526, #188897, #127186, #35195, #173726, #175700, #81664, #4835, #34205, #145349, #50378, #52346, #128185, #112038, #189883, #159516, #115022, #21012, #37176, #160530, #22019, #176715, #79709, #141378, #41192, #104849, #39180, #194874, #177712, #42196, #134203, #116023, #27035, #57366, #26032, #195891, #23020, #131183, #84666, #69518, #24023, #43181, #86678, #10858, #56347, #165538, #7832, #100837, #162520, #58347, #102854, #72527, #192873, #87677, #54351, #148362, #146345, #150376, #85677, #101851, #196881, #147364, #119039, #118030, #8853, #193880, #103857, #180721, #120015, #181700, #179721, #70520, #132189, #55345, #117015, #178710, #9857, #40172, #163535, #164540, #25035, #71516, #133184, #149362, #88680, #11872, #73536, #135209, #30001, #186684, #628, #139151, #46155, #47157, #184672, #28037, #182695, #62299, #137167, #151364, #74520, #123969, #44180, #185666, #30992, #199849, #106828, #107810, #169492, #16815, #121997, #12855, #60322, #15821, #154331, #108816, #63309, #59327, #92641, #122985, #105838, #1632, #198856, #77482, #183687, #170495, #93642, #78465, #31985, #29021, #167525, #45173, #61315, #155327, #76491, #91639, #136185, #140140, #197860, #120996, #90661, #124988, #48154, #166539, #152343, #153327, #89678, #13828, #14829, #168503, #138168, #75494, #142131, #112786, #94637, #98603, #158303, #174480, #157317, #4598, #160297, #32984, #5602, #2634, #143118 ),
 ( #97593, #35947, #66290, #190641, #175469, #159281, #67281, #127949, #21787, #19791, #128940, #189652, #83438, #81432, #188662, #36941, #156317, #34962, #126953, #96614, #141144, #52117, #33973, #64310, #51126, #80457, #191629, #20778, #110804, #17818, #82433, #113773, #144121, #125978, #145115, #79476, #6600, #95630, #68279, #50141, #187676, #49146, #172486, #129930, #18813, #3615, #109812, #171495, #65294, #111800, #173489, #71296, #9629, #179493, #70294, #103633, #73307, #180494, #134978, #24804, #161294, #22789, #11640, #116788, #72291, #56117, #176480, #39946, #115796, #162294, #177486, #8622, #147134, #87454, #131962, #193647, #84436, #57132, #37956, #40958, #55119, #7598, #99614, #146114, #118808, #69284, #130950, #100611, #132959, #165310, #102630, #41966, #194647, #53109, #192640, #86453, #54123, #133969, #164315, #38955, #26803, #149140, #117800, #25808, #114787, #23794, #85444, #178479, #101617, #163306, #148138, #10630, #195661, #88444, #150139, #151135, #89445, #31750, #14593, #45920, #104619, #61077, #166308, #121759, #16579, #123730, #27805, #122749, #169252, #182463, #76249, #196655, #184440, #107574, #153089, #77244, #62065, #30759, #183452, #12626, #138912, #120762, #74291, #106593, #167293, #78226, #199611, #197630, #181477, #29766, #392, #91400, #135960, #185429, #59096, #92406, #43944, #154092, #136936, #105606, #28790, #42955, #15586, #90429, #152115, #46919, #108579, #170256, #93399, #75265, #137927, #155085, #58124, #13598, #119793, #198625, #60091, #44936, #168269, #47918, #109572, #98354, #3380, #159043, #142880, #63067, #126712, #2389, #48906, #64068, #95389, #33727, #174242, #18571, #157075, #171255, #143879, #124746, #66045, #80218, #94394, #186442, #32742, #5360, #156073, #17571, #187438, #19555, #51875, #127712, #128702, #158064, #21540, #79232, #111559, #140903, #20536, #50889, #125738, #67043, #35710, #4361, #112547, #139897, #110560, #1386, #172241, #141889, #160053, #65055, #189413, #188415, #34719, #190399, #49893, #97357, #173244, #96377, #113534, #81199, #175228, #82186, #36693, #101361, #41718, #23546, #38714, #118558, #163051, #86207, #22544, #85193, #192398, #146882, #24558, #144874, #178236, #103382, #25567, #68037, #162050, #56884, #165060, #117545, #116548, #179245, #39699, #72040, #131717, #8374, #148893, #129689, #70049, #100371, #193399, #114534, #164068, #7354, #176234, #54874, #53880, #83200, #147897, #84191, #191386, #9383, #87211, #71049, #99367, #133713, #52862, #194403, #69038, #132715, #55871, #161050, #145871, #37705, #40711, #130703, #115555, #10383, #102380, #195406, #180248, #6357, #177242, #183208, #152846, #43698, #76997, #46671, #153843, #108331, #198369, #134729, #196411, #185181, #90185, #45677, #29524, #149881, #13358, #89198, #135718, #150891, #182214, #120521, #60830, #105360, #167047, #57881, #30505, #11387, #14340, #28548, #181236, #73057, #119553, #92156, #42712, #104374, #74047, #106343, #138669, #76006, #15341, #44689, #26554, #166057, #59846, #27558, #107328, #137681, #12385, #149, #122505, #91157, #199366, #88197, #197389, #58854, #151868, #75022, #136687, #121513, #168027, #184195, #169001, #61818, #123488, #62815, #5115, #188179, #19321, #77986, #34483, #139653, #95147, #190156, #97120, #1141, #96141, #142644, #155830, #49651, #170011, #157830, #80968, #126481, #50649, #35471, #4123, #140657, #141654, #2149, #173004, #154840, #3145, #63827, #65802, #124499, #64819, #158803, #93155, #127470, #186194, #111315, #20292, #51632, #81940, #47675, #109326, #189176, #128460, #110320, #125499, #66797, #112310, #174000, #171008, #172001, #78982, #33489, #143631, #31502, #16337, #32499, #94151, #17327, #48668, #187197, #156836, #18331, #79986, #21300, #83953, #132476, #24314, #86966, #148653, #146630, #159805, #99124, #67800, #10141, #71801, #100127, #175993, #133470, #193155, #160814, #195161, #6117, #177991, #177001, #113296 ),
 ( #98108, #82957, #70807, #129455, #194165, #39458, #8122, #53632, #54627, #116302, #163823, #68795, #144634, #7113, #162805, #101119, #55629, #174987, #191154, #85963, #69800, #52628, #36451, #145633, #147652, #130454, #131468, #40466, #25324, #178998, #37463, #114291, #192151, #9140, #117302, #23304, #38470, #22302, #102138, #115309, #161809, #84948, #181980, #74793, #121279, #72817, #73815, #90924, #136455, #197155, #42473, #119311, #166816, #14100, #198136, #152610, #105130, #122267, #149645, #120287, #11143, #182972, #59606, #26317, #167794, #44456, #28317, #106110, #56642, #164821, #180008, #103139, #134486, #118315, #88962, #151636, #43462, #89956, #87957, #196173, #57645, #41475, #29294, #199125, #27315, #75768, #150652, #137446, #180997, #104136, #12150, #60592, #165818, #135485, #58620, #13131, #24977, #163480, #193824, #117972, #102797, #101792, #133127, #70466, #25977, #85620, #115969, #164483, #21964, #162464, #54297, #23965, #68455, #179663, #161474, #130109, #147307, #7777, #118979, #40114, #38135, #83615, #132131, #41133, #55289, #53286, #87620, #145293, #148306, #22963, #86623, #177657, #114965, #176658, #6776, #9800, #191805, #99788, #149306, #71462, #10800, #194817, #39126, #116961, #178652, #56290, #100781, #72469, #57302, #134142, #37120, #8796, #84611, #146290, #195831, #98779, #160473, #69460, #131127, #192815, #43122, #89616, #104790, #136125, #74459, #14766, #59267, #197801, #150315, #187357, #165479, #106766, #120936, #135148, #26975, #88618, #48827, #11811, #58288, #76427, #13767, #172163, #28960, #182635, #110480, #73475, #105778, #44119, #167465, #196821, #61252, #166478, #119957, #90601, #151305, #64975, #183627, #181643, #27977, #75435, #33648, #137109, #12794, #95309, #152283, #91576, #198795, #45109, #60261, #121932, #168441, #29937, #153265, #138103, #199784, #156993, #125660, #18492, #80140, #141810, #3303, #180662, #42138, #103799, #197618, #88431, #151121, #196642, #165296, #72279, #11626, #134964, #182449, #87442, #178467, #25796, #181465, #119781, #12614, #28775, #24792, #73294, #150125, #9617, #167277, #164303, #42943, #149127, #58111, #59083, #43929, #120750, #194635, #71282, #102617, #26789, #104607, #41954, #195647, #101603, #74278, #163291, #86440, #148126, #166295, #27791, #89433, #132947, #57120, #105591, #135948, #180483, #10618, #133956, #103620, #118794, #90414, #116776, #152099, #13583, #131950, #56105, #193634, #55106, #39934, #117786, #179480, #40945, #140885, #157060, #2375, #29750, #44921, #93384, #33713, #15572, #30743, #110547, #155070, #78212, #14576, #77230, #184426, #138899, #16565, #136921, #170242, #32727, #76234, #379, #64055, #124729, #123716, #45906, #107559, #46904, #169237, #139882, #60076, #108564, #92391, #171238, #106577, #31736, #125725, #198608, #94379, #168254, #1371, #187424, #75250, #48892, #91385, #153074, #63050, #95375, #62051, #154078, #172228, #186427, #47903, #137914, #185413, #109557, #156059, #17556, #121744, #79216, #183436, #199596, #61063, #122735, #192385, #100359, #52849, #51861, #126698, #189399, #37690, #129675, #53868, #115542, #113521, #65042, #4347, #173230, #177230, #38702, #5346, #81186, #18557, #98340, #66032, #80205, #111545, #83187, #82171, #141876, #175215, #159030, #143867, #3367, #114520, #191373, #160039, #99355, #36680, #188402, #34706, #176221, #50876, #96363, #174228, #84179, #21526, #161038, #144861, #6344, #20523, #68024, #22532, #69026, #35697, #49880, #112534, #145859, #7341, #130691, #158051, #19541, #142868, #127699, #97344, #67030, #128689, #190386, #194393, #180237, #89186, #12372, #27545, #24546, #101350, #132704, #56872, #134717, #72029, #25556, #131705, #181224, #193386, #54862, #116536, #195394, #11375, #165049, #85180, #148881, #86196, #71037, #147886, #117534, #55860, #196400, #40698, #179232, #178224, #166045, #146869, #88186, #102368, #39688, #8361, #70036, #150878, #163039, #9372 ),
 ( #87200, #74035, #73045, #10372, #164057, #133702, #118547, #41706, #26542, #103371, #149870, #57869, #119541, #42700, #104361, #135706, #197377, #58842, #120509, #182200, #43685, #162038, #23534, #59831, #75010, #123477, #63817, #45666, #60819, #140647, #185169, #108319, #44677, #107317, #14329, #168990, #46660, #167034, #138, #125490, #47663, #90172, #184184, #78972, #187187, #139642, #138657, #13346, #75994, #124486, #16325, #2137, #105347, #61807, #151855, #91146, #121501, #28536, #136675, #92145, #168016, #198357, #169999, #152835, #183195, #106330, #31490, #30494, #29512, #93142, #153831, #15327, #137667, #1130, #77975, #154827, #186182, #62804, #199354, #122493, #109315, #76986, #170994, #32487, #94140, #155819, #17317, #113285, #81928, #189166, #128449, #51620, #99111, #191143, #33480, #127460, #22291, #130440, #82945, #143620, #156827, #19310, #67787, #159793, #83942, #145622, #5104, #95138, #34472, #3135, #7101, #68783, #35459, #111305, #48658, #190144, #96131, #110310, #141645, #174976, #112300, #171992, #66785, #50638, #173990, #18320, #144623, #21288, #36440, #129444, #98095, #79977, #64810, #6106, #80958, #126471, #4112, #114279, #52616, #175982, #37450, #160803, #97110, #188169, #49642, #172994, #65791, #157820, #142634, #158793, #20282, #11130, #88949, #84937, #71790, #148639, #69788, #27302, #24303, #179996, #85952, #10129, #119300, #42459, #57634, #54615, #131456, #162794, #86955, #164809, #102127, #55618, #161798, #72805, #23293, #146618, #8110, #25313, #41463, #149632, #193143, #117291, #180983, #103128, #40453, #147640, #9129, #163811, #70795, #195149, #176989, #133459, #132463, #87944, #116290, #56630, #104123, #115296, #134475, #177980, #118304, #165805, #73800, #150640, #39447, #101108, #26304, #12136, #194154, #178986, #192139, #196160, #53620, #38459, #100115, #44442, #137431, #153591, #197141, #30257, #155585, #185940, #169760, #14088, #15090, #91900, #61573, #75754, #106096, #17080, #152597, #135473, #107082, #43449, #105117, #93907, #199111, #154591, #138425, #58608, #122254, #198124, #167782, #59591, #90912, #29281, #31255, #60578, #183944, #166803, #139411, #120274, #123242, #45429, #89943, #181966, #28303, #894, #151624, #13117, #182959, #76750, #47425, #184933, #124245, #200105, #74781, #136443, #168754, #121265, #16087, #46418, #108076, #62568, #92905, #77745, #109081, #170760, #32249, #140410, #125253, #79739, #98867, #111067, #158562, #127218, #35225, #63579, #33247, #171758, #114035, #96878, #128217, #186952, #143377, #48422, #3879, #160563, #5870, #110078, #4869, #51389, #64575, #20051, #78734, #66553, #189914, #81694, #159549, #144384, #113050, #174742, #112069, #67546, #188931, #157581, #129204, #94905, #65558, #95898, #50409, #156589, #21046, #2896, #18084, #173757, #49404, #1899, #36205, #141408, #126240, #97859, #82700, #190902, #52378, #187935, #172756, #34236, #175733, #142400, #37211, #19074, #80722, #85712, #42226, #56381, #194906, #101885, #102884, #69552, #163567, #134235, #9889, #10887, #40206, #103887, #38221, #193914, #176747, #41223, #133215, #115055, #26063, #118063, #25067, #179753, #22052, #130198, #83703, #68542, #23053, #145381, #54384, #86710, #70554, #178742, #6863, #99876, #161560, #57396, #148395, #71550, #191893, #164569, #53377, #147398, #84698, #149392, #146378, #87706, #72560, #7866, #195920, #131216, #119068, #180750, #192907, #116057, #177745, #39214, #100870, #55377, #162552, #132221, #24057, #8886, #117047, #90690, #182726, #152373, #196911, #46185, #89710, #58378, #75525, #136215, #47186, #168531, #166569, #150407, #120045, #61344, #169522, #30029, #154360, #73566, #76521, #151395, #91667, #105869, #43213, #181732, #11902, #14860, #104881, #28069, #92672, #153358, #15854, #199880, #44210, #183717, #122027, #138198, #167556, #197890, #185697, #29050, #165567, #137200, #135239, #12885, #123999, #13858, #184700, #123015, #88712 ) ),
 .UNSPECIFIED., .T., .F., .F. ) 
 B_SPLINE_SURFACE_WITH_KNOTS ( ( 4, 3, 4 ),
 ( 3, 2, 2, 2, 2, 2, 2, 2, 2, 2, 2, 2, 2, 2, 2, 2, 2, 2, 2, 2, 2, 2, 2, 2, 2, 2, 2, 2, 2, 2, 2, 2, 2, 2, 2, 2, 2, 2, 2, 2, 2, 2, 2, 2, 2, 2, 2, 2, 2, 2, 2, 2, 2, 2, 2, 2, 2, 2, 2, 2, 2, 2, 2, 2, 2, 2, 2, 2, 2, 2, 2, 2, 2, 2, 2, 2, 2, 2, 2, 2, 2, 2, 2, 2, 2, 2, 2, 2, 2, 2, 2, 2, 2, 2, 2, 2, 2, 2, 2, 2, 2, 2, 2, 2, 2, 2, 2, 2, 2, 2, 2, 2, 2, 2, 2, 2, 2, 2, 2, 2, 2, 2, 2, 2, 2, 2, 2, 2, 2, 2, 2, 2, 2, 2, 2, 2, 2, 2, 2, 2, 2, 2, 2, 2, 2, 2, 2, 2, 2, 2, 2, 2, 2, 2, 2, 2, 2, 2, 2, 2, 2, 2, 2, 2, 2, 2, 2, 2, 2, 2, 2, 2, 2, 2, 2, 2, 2, 2, 2, 2, 2, 2, 2, 2, 2, 2, 2, 2, 2, 2, 2, 2, 2, 2, 2, 2, 2, 2, 2, 2, 2, 2, 2, 2, 2, 2, 2, 2, 2, 2, 2, 2, 2, 2, 2, 2, 2, 2, 2, 2, 2, 2, 2, 2, 2, 2, 2, 2, 3 ),
 ( 0.000000000000000000, 0.5000000000000000000, 1.000000000000000000 ),
 ( 0.000000000000000000, 0.004385964912280701511, 0.008771929824561403022, 0.01315789473684210453, 0.01754385964912280604, 0.02192982456140350755, 0.02631578947368420907, 0.03070175438596491058, 0.03508771929824561209, 0.03947368421052631360, 0.04385964912280701511, 0.04824561403508771662, 0.05263157894736841813, 0.05701754385964911964, 0.06140350877192982115, 0.06578947368421052266, 0.07017543859649122417, 0.07456140350877192569, 0.07894736842105262720, 0.08333333333333332871, 0.08771929824561403022, 0.09210526315789473173, 0.09649122807017543324, 0.1008771929824561348, 0.1052631578947368363, 0.1096491228070175378, 0.1140350877192982393, 0.1184210526315789408, 0.1228070175438596423, 0.1271929824561403577, 0.1315789473684210453, 0.1359649122807017607, 0.1403508771929824483, 0.1447368421052631637, 0.1491228070175438514, 0.1535087719298245668, 0.1578947368421052544, 0.1622807017543859698, 0.1666666666666666574, 0.1710526315789473728, 0.1754385964912280604, 0.1798245614035087758, 0.1842105263157894635, 0.1885964912280701788, 0.1929824561403508665, 0.1973684210526315819, 0.2017543859649122695, 0.2061403508771929849, 0.2105263157894736725, 0.2149122807017543879, 0.2192982456140350755, 0.2236842105263157909, 0.2280701754385964786, 0.2324561403508771940, 0.2368421052631578816, 0.2412280701754385970, 0.2456140350877192846, 0.2500000000000000000, 0.2543859649122807154, 0.2587719298245614308, 0.2631578947368420907, 0.2675438596491228060, 0.2719298245614035214, 0.2763157894736842368, 0.2807017543859648967, 0.2850877192982456121, 0.2894736842105263275, 0.2938596491228070429, 0.2982456140350877027, 0.3026315789473684181, 0.3070175438596491335, 0.3114035087719298489, 0.3157894736842105088, 0.3201754385964912242, 0.3245614035087719396, 0.3289473684210526550, 0.3333333333333333148, 0.3377192982456140302, 0.3421052631578947456, 0.3464912280701754610, 0.3508771929824561209, 0.3552631578947368363, 0.3596491228070175517, 0.3640350877192982670, 0.3684210526315789269, 0.3728070175438596423, 0.3771929824561403577, 0.3815789473684210731, 0.3859649122807017330, 0.3903508771929824483, 0.3947368421052631637, 0.3991228070175438791, 0.4035087719298245390, 0.4078947368421052544, 0.4122807017543859698, 0.4166666666666666852, 0.4210526315789473450, 0.4254385964912280604, 0.4298245614035087758, 0.4342105263157894912, 0.4385964912280701511, 0.4429824561403508665, 0.4473684210526315819, 0.4517543859649122973, 0.4561403508771929571, 0.4605263157894736725, 0.4649122807017543879, 0.4692982456140351033, 0.4736842105263157632, 0.4780701754385964786, 0.4824561403508771940, 0.4868421052631579093, 0.4912280701754385692, 0.4956140350877192846, 0.5000000000000000000, 0.5043859649122807154, 0.5087719298245614308, 0.5131578947368421462, 0.5175438596491228616, 0.5219298245614034659, 0.5263157894736841813, 0.5307017543859648967, 0.5350877192982456121, 0.5394736842105263275, 0.5438596491228070429, 0.5482456140350877583, 0.5526315789473684736, 0.5570175438596490780, 0.5614035087719297934, 0.5657894736842105088, 0.5701754385964912242, 0.5745614035087719396, 0.5789473684210526550, 0.5833333333333333703, 0.5877192982456140857, 0.5921052631578946901, 0.5964912280701754055, 0.6008771929824561209, 0.6052631578947368363, 0.6096491228070175517, 0.6140350877192982670, 0.6184210526315789824, 0.6228070175438596978, 0.6271929824561403022, 0.6315789473684210176, 0.6359649122807017330, 0.6403508771929824483, 0.6447368421052631637, 0.6491228070175438791, 0.6535087719298245945, 0.6578947368421053099, 0.6622807017543859143, 0.6666666666666666297, 0.6710526315789473450, 0.6754385964912280604, 0.6798245614035087758, 0.6842105263157894912, 0.6885964912280702066, 0.6929824561403509220, 0.6973684210526315264, 0.7017543859649122417, 0.7061403508771929571, 0.7105263157894736725, 0.7149122807017543879, 0.7192982456140351033, 0.7236842105263158187, 0.7280701754385965341, 0.7324561403508771384, 0.7368421052631578538, 0.7412280701754385692, 0.7456140350877192846, 0.7500000000000000000, 0.7543859649122807154, 0.7587719298245614308, 0.7631578947368421462, 0.7675438596491228616, 0.7719298245614034659, 0.7763157894736841813, 0.7807017543859648967, 0.7850877192982456121, 0.7894736842105263275, 0.7938596491228070429, 0.7982456140350877583, 0.8026315789473684736, 0.8070175438596490780, 0.8114035087719297934, 0.8157894736842105088, 0.8201754385964912242, 0.8245614035087719396, 0.8289473684210526550, 0.8333333333333333703, 0.8377192982456140857, 0.8421052631578946901, 0.8464912280701754055, 0.8508771929824561209, 0.8552631578947368363, 0.8596491228070175517, 0.8640350877192982670, 0.8684210526315789824, 0.8728070175438596978, 0.8771929824561403022, 0.8815789473684210176, 0.8859649122807017330, 0.8903508771929824483, 0.8947368421052631637, 0.8991228070175438791, 0.9035087719298245945, 0.9078947368421053099, 0.9122807017543859143, 0.9166666666666666297, 0.9210526315789473450, 0.9254385964912280604, 0.9298245614035087758, 0.9342105263157894912, 0.9385964912280702066, 0.9429824561403509220, 0.9473684210526315264, 0.9517543859649122417, 0.9561403508771929571, 0.9605263157894736725, 0.9649122807017543879, 0.9692982456140351033, 0.9736842105263158187, 0.9780701754385965341, 0.9824561403508771384, 0.9868421052631578538, 0.9912280701754385692, 0.9956140350877192846, 1.000000000000000000 ),
 .UNSPECIFIED. ) 
 GEOMETRIC_REPRESENTATION_ITEM ( )  RATIONAL_B_SPLINE_SURFACE ( (
 ( 1.000000000000000000, 0.9659258262890683122, 1.000000000000000000, 0.9659258262890683122, 1.000000000000000000, 0.9659258262890683122, 1.000000000000000000, 0.9659258262890683122, 1.000000000000000000, 0.9659258262890683122, 1.000000000000000000, 0.9659258262890683122, 1.000000000000000000, 0.9659258262890683122, 1.000000000000000000, 0.9659258262890683122, 1.000000000000000000, 0.9659258262890683122, 1.000000000000000000, 0.9659258262890683122, 1.000000000000000000, 0.9659258262890683122, 1.000000000000000000, 0.9659258262890683122, 1.000000000000000000, 0.9659258262890683122, 1.000000000000000000, 0.9659258262890683122, 1.000000000000000000, 0.9659258262890683122, 1.000000000000000000, 0.9659258262890683122, 1.000000000000000000, 0.9659258262890683122, 1.000000000000000000, 0.9659258262890683122, 1.000000000000000000, 0.9659258262890683122, 1.000000000000000000, 0.9659258262890683122, 1.000000000000000000, 0.9659258262890683122, 1.000000000000000000, 0.9659258262890683122, 1.000000000000000000, 0.9659258262890683122, 1.000000000000000000, 0.9659258262890683122, 1.000000000000000000, 0.9659258262890683122, 1.000000000000000000, 0.9659258262890683122, 1.000000000000000000, 0.9659258262890683122, 1.000000000000000000, 0.9659258262890683122, 1.000000000000000000, 0.9659258262890683122, 1.000000000000000000, 0.9659258262890683122, 1.000000000000000000, 0.9659258262890683122, 1.000000000000000000, 0.9659258262890683122, 1.000000000000000000, 0.9659258262890683122, 1.000000000000000000, 0.9659258262890683122, 1.000000000000000000, 0.9659258262890683122, 1.000000000000000000, 0.9659258262890683122, 1.000000000000000000, 0.9659258262890683122, 1.000000000000000000, 0.9659258262890683122, 1.000000000000000000, 0.9659258262890683122, 1.000000000000000000, 0.9659258262890683122, 1.000000000000000000, 0.9659258262890683122, 1.000000000000000000, 0.9659258262890683122, 1.000000000000000000, 0.9659258262890683122, 1.000000000000000000, 0.9659258262890683122, 1.000000000000000000, 0.9659258262890683122, 1.000000000000000000, 0.9659258262890683122, 1.000000000000000000, 0.9659258262890683122, 1.000000000000000000, 0.9659258262890683122, 1.000000000000000000, 0.9659258262890683122, 1.000000000000000000, 0.9659258262890683122, 1.000000000000000000, 0.9659258262890683122, 1.000000000000000000, 0.9659258262890683122, 1.000000000000000000, 0.9659258262890683122, 1.000000000000000000, 0.9659258262890683122, 1.000000000000000000, 0.9659258262890683122, 1.000000000000000000, 0.9659258262890683122, 1.000000000000000000, 0.9659258262890683122, 1.000000000000000000, 0.9659258262890683122, 1.000000000000000000, 0.9659258262890683122, 1.000000000000000000, 0.9659258262890683122, 1.000000000000000000, 0.9659258262890683122, 1.000000000000000000, 0.9659258262890683122, 1.000000000000000000, 0.9659258262890683122, 1.000000000000000000, 0.9659258262890683122, 1.000000000000000000, 0.9659258262890683122, 1.000000000000000000, 0.9659258262890683122, 1.000000000000000000, 0.9659258262890683122, 1.000000000000000000, 0.9659258262890683122, 1.000000000000000000, 0.9659258262890683122, 1.000000000000000000, 0.9659258262890683122, 1.000000000000000000, 0.9659258262890683122, 1.000000000000000000, 0.9659258262890683122, 1.000000000000000000, 0.9659258262890683122, 1.000000000000000000, 0.9659258262890683122, 1.000000000000000000, 0.9659258262890683122, 1.000000000000000000, 0.9659258262890683122, 1.000000000000000000, 0.9659258262890683122, 1.000000000000000000, 0.9659258262890683122, 1.000000000000000000, 0.9659258262890683122, 1.000000000000000000, 0.9659258262890683122, 1.000000000000000000, 0.9659258262890683122, 1.000000000000000000, 0.9659258262890683122, 1.000000000000000000, 0.9659258262890683122, 1.000000000000000000, 0.9659258262890683122, 1.000000000000000000, 0.9659258262890683122, 1.000000000000000000, 0.9659258262890683122, 1.000000000000000000, 0.9659258262890683122, 1.000000000000000000, 0.9659258262890683122, 1.000000000000000000, 0.9659258262890683122, 1.000000000000000000, 0.9659258262890683122, 1.000000000000000000, 0.9659258262890683122, 1.000000000000000000, 0.9659258262890683122, 1.000000000000000000, 0.9659258262890683122, 1.000000000000000000, 0.9659258262890683122, 1.000000000000000000, 0.9659258262890683122, 1.000000000000000000, 0.9659258262890683122, 1.000000000000000000, 0.9659258262890683122, 1.000000000000000000, 0.9659258262890683122, 1.000000000000000000, 0.9659258262890683122, 1.000000000000000000, 0.9659258262890683122, 1.000000000000000000, 0.9659258262890683122, 1.000000000000000000, 0.9659258262890683122, 1.000000000000000000, 0.9659258262890683122, 1.000000000000000000, 0.9659258262890683122, 1.000000000000000000, 0.9659258262890683122, 1.000000000000000000, 0.9659258262890683122, 1.000000000000000000, 0.9659258262890683122, 1.000000000000000000, 0.9659258262890683122, 1.000000000000000000, 0.9659258262890683122, 1.000000000000000000, 0.9659258262890683122, 1.000000000000000000, 0.9659258262890683122, 1.000000000000000000, 0.9659258262890683122, 1.000000000000000000, 0.9659258262890683122, 1.000000000000000000, 0.9659258262890683122, 1.000000000000000000, 0.9659258262890683122, 1.000000000000000000, 0.9659258262890683122, 1.000000000000000000, 0.9659258262890683122, 1.000000000000000000, 0.9659258262890683122, 1.000000000000000000, 0.9659258262890683122, 1.000000000000000000, 0.9659258262890683122, 1.000000000000000000, 0.9659258262890683122, 1.000000000000000000, 0.9659258262890683122, 1.000000000000000000, 0.9659258262890683122, 1.000000000000000000, 0.9659258262890683122, 1.000000000000000000, 0.9659258262890683122, 1.000000000000000000, 0.9659258262890683122, 1.000000000000000000, 0.9659258262890683122, 1.000000000000000000, 0.9659258262890683122, 1.000000000000000000, 0.9659258262890683122, 1.000000000000000000, 0.9659258262890683122, 1.000000000000000000, 0.9659258262890683122, 1.000000000000000000, 0.9659258262890683122, 1.000000000000000000, 0.9659258262890683122, 1.000000000000000000, 0.9659258262890683122, 1.000000000000000000, 0.9659258262890683122, 1.000000000000000000, 0.9659258262890683122, 1.000000000000000000, 0.9659258262890683122, 1.000000000000000000, 0.9659258262890683122, 1.000000000000000000, 0.9659258262890683122, 1.000000000000000000, 0.9659258262890683122, 1.000000000000000000, 0.9659258262890683122, 1.000000000000000000, 0.9659258262890683122, 1.000000000000000000, 0.9659258262890683122, 1.000000000000000000, 0.9659258262890683122, 1.000000000000000000, 0.9659258262890683122, 1.000000000000000000, 0.9659258262890683122, 1.000000000000000000, 0.9659258262890683122, 1.000000000000000000, 0.9659258262890683122, 1.000000000000000000, 0.9659258262890683122, 1.000000000000000000, 0.9659258262890683122, 1.000000000000000000, 0.9659258262890683122, 1.000000000000000000, 0.9659258262890683122, 1.000000000000000000, 0.9659258262890683122, 1.000000000000000000, 0.9659258262890683122, 1.000000000000000000, 0.9659258262890683122, 1.000000000000000000, 0.9659258262890683122, 1.000000000000000000, 0.9659258262890683122, 1.000000000000000000, 0.9659258262890683122, 1.000000000000000000, 0.9659258262890683122, 1.000000000000000000, 0.9659258262890683122, 1.000000000000000000, 0.9659258262890683122, 1.000000000000000000, 0.9659258262890683122, 1.000000000000000000, 0.9659258262890683122, 1.000000000000000000, 0.9659258262890683122, 1.000000000000000000, 0.9659258262890683122, 1.000000000000000000, 0.9659258262890683122, 1.000000000000000000, 0.9659258262890683122, 1.000000000000000000, 0.9659258262890683122, 1.000000000000000000, 0.9659258262890683122, 1.000000000000000000, 0.9659258262890683122, 1.000000000000000000, 0.9659258262890683122, 1.000000000000000000, 0.9659258262890683122, 1.000000000000000000, 0.9659258262890683122, 1.000000000000000000, 0.9659258262890683122, 1.000000000000000000, 0.9659258262890683122, 1.000000000000000000, 0.9659258262890683122, 1.000000000000000000, 0.9659258262890683122, 1.000000000000000000, 0.9659258262890683122, 1.000000000000000000, 0.9659258262890683122, 1.000000000000000000, 0.9659258262890683122, 1.000000000000000000, 0.9659258262890683122, 1.000000000000000000, 0.9659258262890683122, 1.000000000000000000, 0.9659258262890683122, 1.000000000000000000, 0.9659258262890683122, 1.000000000000000000, 0.9659258262890683122, 1.000000000000000000, 0.9659258262890683122, 1.000000000000000000, 0.9659258262890683122, 1.000000000000000000, 0.9659258262890683122, 1.000000000000000000, 0.9659258262890683122, 1.000000000000000000, 0.9659258262890683122, 1.000000000000000000, 0.9659258262890683122, 1.000000000000000000, 0.9659258262890683122, 1.000000000000000000, 0.9659258262890683122, 1.000000000000000000, 0.9659258262890683122, 1.000000000000000000, 0.9659258262890683122, 1.000000000000000000, 0.9659258262890683122, 1.000000000000000000, 0.9659258262890683122, 1.000000000000000000, 0.9659258262890683122, 1.000000000000000000, 0.9659258262890683122, 1.000000000000000000, 0.9659258262890683122, 1.000000000000000000, 0.9659258262890683122, 1.000000000000000000, 0.9659258262890683122, 1.000000000000000000, 0.9659258262890683122, 1.000000000000000000, 0.9659258262890683122, 1.000000000000000000, 0.9659258262890683122, 1.000000000000000000, 0.9659258262890683122, 1.000000000000000000, 0.9659258262890683122, 1.000000000000000000, 0.9659258262890683122, 1.000000000000000000, 0.9659258262890683122, 1.000000000000000000, 0.9659258262890683122, 1.000000000000000000, 0.9659258262890683122, 1.000000000000000000, 0.9659258262890683122, 1.000000000000000000, 0.9659258262890683122, 1.000000000000000000, 0.9659258262890683122, 1.000000000000000000, 0.9659258262890683122, 1.000000000000000000, 0.9659258262890683122, 1.000000000000000000, 0.9659258262890683122, 1.000000000000000000, 0.9659258262890683122, 1.000000000000000000, 0.9659258262890683122, 1.000000000000000000, 0.9659258262890683122, 1.000000000000000000, 0.9659258262890683122, 1.000000000000000000, 0.9659258262890683122, 1.000000000000000000, 0.9659258262890683122, 1.000000000000000000, 0.9659258262890683122, 1.000000000000000000, 0.9659258262890683122, 1.000000000000000000, 0.9659258262890683122, 1.000000000000000000, 0.9659258262890683122, 1.000000000000000000, 0.9659258262890683122, 1.000000000000000000),
 ( 0.3333333333333333703, 0.3219752754296894559, 0.3333333333333333703, 0.3219752754296894559, 0.3333333333333333703, 0.3219752754296894559, 0.3333333333333333703, 0.3219752754296894559, 0.3333333333333333703, 0.3219752754296894559, 0.3333333333333333703, 0.3219752754296894559, 0.3333333333333333703, 0.3219752754296894559, 0.3333333333333333703, 0.3219752754296894559, 0.3333333333333333703, 0.3219752754296894559, 0.3333333333333333703, 0.3219752754296894559, 0.3333333333333333703, 0.3219752754296894559, 0.3333333333333333703, 0.3219752754296894559, 0.3333333333333333703, 0.3219752754296894559, 0.3333333333333333703, 0.3219752754296894559, 0.3333333333333333703, 0.3219752754296894559, 0.3333333333333333703, 0.3219752754296894559, 0.3333333333333333703, 0.3219752754296894559, 0.3333333333333333703, 0.3219752754296894559, 0.3333333333333333703, 0.3219752754296894559, 0.3333333333333333703, 0.3219752754296894559, 0.3333333333333333703, 0.3219752754296894559, 0.3333333333333333703, 0.3219752754296894559, 0.3333333333333333703, 0.3219752754296894559, 0.3333333333333333703, 0.3219752754296894559, 0.3333333333333333703, 0.3219752754296894559, 0.3333333333333333703, 0.3219752754296894559, 0.3333333333333333703, 0.3219752754296894559, 0.3333333333333333703, 0.3219752754296894559, 0.3333333333333333703, 0.3219752754296894559, 0.3333333333333333703, 0.3219752754296894559, 0.3333333333333333703, 0.3219752754296894559, 0.3333333333333333703, 0.3219752754296894559, 0.3333333333333333703, 0.3219752754296894559, 0.3333333333333333703, 0.3219752754296894559, 0.3333333333333333703, 0.3219752754296894559, 0.3333333333333333703, 0.3219752754296894559, 0.3333333333333333703, 0.3219752754296894559, 0.3333333333333333703, 0.3219752754296894559, 0.3333333333333333703, 0.3219752754296894559, 0.3333333333333333703, 0.3219752754296894559, 0.3333333333333333703, 0.3219752754296894559, 0.3333333333333333703, 0.3219752754296894559, 0.3333333333333333703, 0.3219752754296894559, 0.3333333333333333703, 0.3219752754296894559, 0.3333333333333333703, 0.3219752754296894559, 0.3333333333333333703, 0.3219752754296894559, 0.3333333333333333703, 0.3219752754296894559, 0.3333333333333333703, 0.3219752754296894559, 0.3333333333333333703, 0.3219752754296894559, 0.3333333333333333703, 0.3219752754296894559, 0.3333333333333333703, 0.3219752754296894559, 0.3333333333333333703, 0.3219752754296894559, 0.3333333333333333703, 0.3219752754296894559, 0.3333333333333333703, 0.3219752754296894559, 0.3333333333333333703, 0.3219752754296894559, 0.3333333333333333703, 0.3219752754296894559, 0.3333333333333333703, 0.3219752754296894559, 0.3333333333333333703, 0.3219752754296894559, 0.3333333333333333703, 0.3219752754296894559, 0.3333333333333333703, 0.3219752754296894559, 0.3333333333333333703, 0.3219752754296894559, 0.3333333333333333703, 0.3219752754296894559, 0.3333333333333333703, 0.3219752754296894559, 0.3333333333333333703, 0.3219752754296894559, 0.3333333333333333703, 0.3219752754296894559, 0.3333333333333333703, 0.3219752754296894559, 0.3333333333333333703, 0.3219752754296894559, 0.3333333333333333703, 0.3219752754296894559, 0.3333333333333333703, 0.3219752754296894559, 0.3333333333333333703, 0.3219752754296894559, 0.3333333333333333703, 0.3219752754296894559, 0.3333333333333333703, 0.3219752754296894559, 0.3333333333333333703, 0.3219752754296894559, 0.3333333333333333703, 0.3219752754296894559, 0.3333333333333333703, 0.3219752754296894559, 0.3333333333333333703, 0.3219752754296894559, 0.3333333333333333703, 0.3219752754296894559, 0.3333333333333333703, 0.3219752754296894559, 0.3333333333333333703, 0.3219752754296894559, 0.3333333333333333703, 0.3219752754296894559, 0.3333333333333333703, 0.3219752754296894559, 0.3333333333333333703, 0.3219752754296894559, 0.3333333333333333703, 0.3219752754296894559, 0.3333333333333333703, 0.3219752754296894559, 0.3333333333333333703, 0.3219752754296894559, 0.3333333333333333703, 0.3219752754296894559, 0.3333333333333333703, 0.3219752754296894559, 0.3333333333333333703, 0.3219752754296894559, 0.3333333333333333703, 0.3219752754296894559, 0.3333333333333333703, 0.3219752754296894559, 0.3333333333333333703, 0.3219752754296894559, 0.3333333333333333703, 0.3219752754296894559, 0.3333333333333333703, 0.3219752754296894559, 0.3333333333333333703, 0.3219752754296894559, 0.3333333333333333703, 0.3219752754296894559, 0.3333333333333333703, 0.3219752754296894559, 0.3333333333333333703, 0.3219752754296894559, 0.3333333333333333703, 0.3219752754296894559, 0.3333333333333333703, 0.3219752754296894559, 0.3333333333333333703, 0.3219752754296894559, 0.3333333333333333703, 0.3219752754296894559, 0.3333333333333333703, 0.3219752754296894559, 0.3333333333333333703, 0.3219752754296894559, 0.3333333333333333703, 0.3219752754296894559, 0.3333333333333333703, 0.3219752754296894559, 0.3333333333333333703, 0.3219752754296894559, 0.3333333333333333703, 0.3219752754296894559, 0.3333333333333333703, 0.3219752754296894559, 0.3333333333333333703, 0.3219752754296894559, 0.3333333333333333703, 0.3219752754296894559, 0.3333333333333333703, 0.3219752754296894559, 0.3333333333333333703, 0.3219752754296894559, 0.3333333333333333703, 0.3219752754296894559, 0.3333333333333333703, 0.3219752754296894559, 0.3333333333333333703, 0.3219752754296894559, 0.3333333333333333703, 0.3219752754296894559, 0.3333333333333333703, 0.3219752754296894559, 0.3333333333333333703, 0.3219752754296894559, 0.3333333333333333703, 0.3219752754296894559, 0.3333333333333333703, 0.3219752754296894559, 0.3333333333333333703, 0.3219752754296894559, 0.3333333333333333703, 0.3219752754296894559, 0.3333333333333333703, 0.3219752754296894559, 0.3333333333333333703, 0.3219752754296894559, 0.3333333333333333703, 0.3219752754296894559, 0.3333333333333333703, 0.3219752754296894559, 0.3333333333333333703, 0.3219752754296894559, 0.3333333333333333703, 0.3219752754296894559, 0.3333333333333333703, 0.3219752754296894559, 0.3333333333333333703, 0.3219752754296894559, 0.3333333333333333703, 0.3219752754296894559, 0.3333333333333333703, 0.3219752754296894559, 0.3333333333333333703, 0.3219752754296894559, 0.3333333333333333703, 0.3219752754296894559, 0.3333333333333333703, 0.3219752754296894559, 0.3333333333333333703, 0.3219752754296894559, 0.3333333333333333703, 0.3219752754296894559, 0.3333333333333333703, 0.3219752754296894559, 0.3333333333333333703, 0.3219752754296894559, 0.3333333333333333703, 0.3219752754296894559, 0.3333333333333333703, 0.3219752754296894559, 0.3333333333333333703, 0.3219752754296894559, 0.3333333333333333703, 0.3219752754296894559, 0.3333333333333333703, 0.3219752754296894559, 0.3333333333333333703, 0.3219752754296894559, 0.3333333333333333703, 0.3219752754296894559, 0.3333333333333333703, 0.3219752754296894559, 0.3333333333333333703, 0.3219752754296894559, 0.3333333333333333703, 0.3219752754296894559, 0.3333333333333333703, 0.3219752754296894559, 0.3333333333333333703, 0.3219752754296894559, 0.3333333333333333703, 0.3219752754296894559, 0.3333333333333333703, 0.3219752754296894559, 0.3333333333333333703, 0.3219752754296894559, 0.3333333333333333703, 0.3219752754296894559, 0.3333333333333333703, 0.3219752754296894559, 0.3333333333333333703, 0.3219752754296894559, 0.3333333333333333703, 0.3219752754296894559, 0.3333333333333333703, 0.3219752754296894559, 0.3333333333333333703, 0.3219752754296894559, 0.3333333333333333703, 0.3219752754296894559, 0.3333333333333333703, 0.3219752754296894559, 0.3333333333333333703, 0.3219752754296894559, 0.3333333333333333703, 0.3219752754296894559, 0.3333333333333333703, 0.3219752754296894559, 0.3333333333333333703, 0.3219752754296894559, 0.3333333333333333703, 0.3219752754296894559, 0.3333333333333333703, 0.3219752754296894559, 0.3333333333333333703, 0.3219752754296894559, 0.3333333333333333703, 0.3219752754296894559, 0.3333333333333333703, 0.3219752754296894559, 0.3333333333333333703, 0.3219752754296894559, 0.3333333333333333703, 0.3219752754296894559, 0.3333333333333333703, 0.3219752754296894559, 0.3333333333333333703, 0.3219752754296894559, 0.3333333333333333703, 0.3219752754296894559, 0.3333333333333333703, 0.3219752754296894559, 0.3333333333333333703, 0.3219752754296894559, 0.3333333333333333703, 0.3219752754296894559, 0.3333333333333333703, 0.3219752754296894559, 0.3333333333333333703, 0.3219752754296894559, 0.3333333333333333703, 0.3219752754296894559, 0.3333333333333333703, 0.3219752754296894559, 0.3333333333333333703, 0.3219752754296894559, 0.3333333333333333703, 0.3219752754296894559, 0.3333333333333333703, 0.3219752754296894559, 0.3333333333333333703, 0.3219752754296894559, 0.3333333333333333703, 0.3219752754296894559, 0.3333333333333333703, 0.3219752754296894559, 0.3333333333333333703, 0.3219752754296894559, 0.3333333333333333703, 0.3219752754296894559, 0.3333333333333333703, 0.3219752754296894559, 0.3333333333333333703, 0.3219752754296894559, 0.3333333333333333703, 0.3219752754296894559, 0.3333333333333333703, 0.3219752754296894559, 0.3333333333333333703, 0.3219752754296894559, 0.3333333333333333703, 0.3219752754296894559, 0.3333333333333333703, 0.3219752754296894559, 0.3333333333333333703, 0.3219752754296894559, 0.3333333333333333703, 0.3219752754296894559, 0.3333333333333333703, 0.3219752754296894559, 0.3333333333333333703, 0.3219752754296894559, 0.3333333333333333703, 0.3219752754296894559, 0.3333333333333333703, 0.3219752754296894559, 0.3333333333333333703, 0.3219752754296894559, 0.3333333333333333703, 0.3219752754296894559, 0.3333333333333333703, 0.3219752754296894559, 0.3333333333333333703, 0.3219752754296894559, 0.3333333333333333703, 0.3219752754296894559, 0.3333333333333333703, 0.3219752754296894559, 0.3333333333333333703, 0.3219752754296894559, 0.3333333333333333703, 0.3219752754296894559, 0.3333333333333333703, 0.3219752754296894559, 0.3333333333333333703, 0.3219752754296894559, 0.3333333333333333703, 0.3219752754296894559, 0.3333333333333333703, 0.3219752754296894559, 0.3333333333333333703, 0.3219752754296894559, 0.3333333333333333703, 0.3219752754296894559, 0.3333333333333333703, 0.3219752754296894559, 0.3333333333333333703, 0.3219752754296894559, 0.3333333333333333703, 0.3219752754296894559, 0.3333333333333333703, 0.3219752754296894559, 0.3333333333333333703, 0.3219752754296894559, 0.3333333333333333703, 0.3219752754296894559, 0.3333333333333333703, 0.3219752754296894559, 0.3333333333333333703, 0.3219752754296894559, 0.3333333333333333703, 0.3219752754296894559, 0.3333333333333333703, 0.3219752754296894559, 0.3333333333333333703),
 ( 0.3333333333333333703, 0.3219752754296894559, 0.3333333333333333703, 0.3219752754296894559, 0.3333333333333333703, 0.3219752754296894559, 0.3333333333333333703, 0.3219752754296894559, 0.3333333333333333703, 0.3219752754296894559, 0.3333333333333333703, 0.3219752754296894559, 0.3333333333333333703, 0.3219752754296894559, 0.3333333333333333703, 0.3219752754296894559, 0.3333333333333333703, 0.3219752754296894559, 0.3333333333333333703, 0.3219752754296894559, 0.3333333333333333703, 0.3219752754296894559, 0.3333333333333333703, 0.3219752754296894559, 0.3333333333333333703, 0.3219752754296894559, 0.3333333333333333703, 0.3219752754296894559, 0.3333333333333333703, 0.3219752754296894559, 0.3333333333333333703, 0.3219752754296894559, 0.3333333333333333703, 0.3219752754296894559, 0.3333333333333333703, 0.3219752754296894559, 0.3333333333333333703, 0.3219752754296894559, 0.3333333333333333703, 0.3219752754296894559, 0.3333333333333333703, 0.3219752754296894559, 0.3333333333333333703, 0.3219752754296894559, 0.3333333333333333703, 0.3219752754296894559, 0.3333333333333333703, 0.3219752754296894559, 0.3333333333333333703, 0.3219752754296894559, 0.3333333333333333703, 0.3219752754296894559, 0.3333333333333333703, 0.3219752754296894559, 0.3333333333333333703, 0.3219752754296894559, 0.3333333333333333703, 0.3219752754296894559, 0.3333333333333333703, 0.3219752754296894559, 0.3333333333333333703, 0.3219752754296894559, 0.3333333333333333703, 0.3219752754296894559, 0.3333333333333333703, 0.3219752754296894559, 0.3333333333333333703, 0.3219752754296894559, 0.3333333333333333703, 0.3219752754296894559, 0.3333333333333333703, 0.3219752754296894559, 0.3333333333333333703, 0.3219752754296894559, 0.3333333333333333703, 0.3219752754296894559, 0.3333333333333333703, 0.3219752754296894559, 0.3333333333333333703, 0.3219752754296894559, 0.3333333333333333703, 0.3219752754296894559, 0.3333333333333333703, 0.3219752754296894559, 0.3333333333333333703, 0.3219752754296894559, 0.3333333333333333703, 0.3219752754296894559, 0.3333333333333333703, 0.3219752754296894559, 0.3333333333333333703, 0.3219752754296894559, 0.3333333333333333703, 0.3219752754296894559, 0.3333333333333333703, 0.3219752754296894559, 0.3333333333333333703, 0.3219752754296894559, 0.3333333333333333703, 0.3219752754296894559, 0.3333333333333333703, 0.3219752754296894559, 0.3333333333333333703, 0.3219752754296894559, 0.3333333333333333703, 0.3219752754296894559, 0.3333333333333333703, 0.3219752754296894559, 0.3333333333333333703, 0.3219752754296894559, 0.3333333333333333703, 0.3219752754296894559, 0.3333333333333333703, 0.3219752754296894559, 0.3333333333333333703, 0.3219752754296894559, 0.3333333333333333703, 0.3219752754296894559, 0.3333333333333333703, 0.3219752754296894559, 0.3333333333333333703, 0.3219752754296894559, 0.3333333333333333703, 0.3219752754296894559, 0.3333333333333333703, 0.3219752754296894559, 0.3333333333333333703, 0.3219752754296894559, 0.3333333333333333703, 0.3219752754296894559, 0.3333333333333333703, 0.3219752754296894559, 0.3333333333333333703, 0.3219752754296894559, 0.3333333333333333703, 0.3219752754296894559, 0.3333333333333333703, 0.3219752754296894559, 0.3333333333333333703, 0.3219752754296894559, 0.3333333333333333703, 0.3219752754296894559, 0.3333333333333333703, 0.3219752754296894559, 0.3333333333333333703, 0.3219752754296894559, 0.3333333333333333703, 0.3219752754296894559, 0.3333333333333333703, 0.3219752754296894559, 0.3333333333333333703, 0.3219752754296894559, 0.3333333333333333703, 0.3219752754296894559, 0.3333333333333333703, 0.3219752754296894559, 0.3333333333333333703, 0.3219752754296894559, 0.3333333333333333703, 0.3219752754296894559, 0.3333333333333333703, 0.3219752754296894559, 0.3333333333333333703, 0.3219752754296894559, 0.3333333333333333703, 0.3219752754296894559, 0.3333333333333333703, 0.3219752754296894559, 0.3333333333333333703, 0.3219752754296894559, 0.3333333333333333703, 0.3219752754296894559, 0.3333333333333333703, 0.3219752754296894559, 0.3333333333333333703, 0.3219752754296894559, 0.3333333333333333703, 0.3219752754296894559, 0.3333333333333333703, 0.3219752754296894559, 0.3333333333333333703, 0.3219752754296894559, 0.3333333333333333703, 0.3219752754296894559, 0.3333333333333333703, 0.3219752754296894559, 0.3333333333333333703, 0.3219752754296894559, 0.3333333333333333703, 0.3219752754296894559, 0.3333333333333333703, 0.3219752754296894559, 0.3333333333333333703, 0.3219752754296894559, 0.3333333333333333703, 0.3219752754296894559, 0.3333333333333333703, 0.3219752754296894559, 0.3333333333333333703, 0.3219752754296894559, 0.3333333333333333703, 0.3219752754296894559, 0.3333333333333333703, 0.3219752754296894559, 0.3333333333333333703, 0.3219752754296894559, 0.3333333333333333703, 0.3219752754296894559, 0.3333333333333333703, 0.3219752754296894559, 0.3333333333333333703, 0.3219752754296894559, 0.3333333333333333703, 0.3219752754296894559, 0.3333333333333333703, 0.3219752754296894559, 0.3333333333333333703, 0.3219752754296894559, 0.3333333333333333703, 0.3219752754296894559, 0.3333333333333333703, 0.3219752754296894559, 0.3333333333333333703, 0.3219752754296894559, 0.3333333333333333703, 0.3219752754296894559, 0.3333333333333333703, 0.3219752754296894559, 0.3333333333333333703, 0.3219752754296894559, 0.3333333333333333703, 0.3219752754296894559, 0.3333333333333333703, 0.3219752754296894559, 0.3333333333333333703, 0.3219752754296894559, 0.3333333333333333703, 0.3219752754296894559, 0.3333333333333333703, 0.3219752754296894559, 0.3333333333333333703, 0.3219752754296894559, 0.3333333333333333703, 0.3219752754296894559, 0.3333333333333333703, 0.3219752754296894559, 0.3333333333333333703, 0.3219752754296894559, 0.3333333333333333703, 0.3219752754296894559, 0.3333333333333333703, 0.3219752754296894559, 0.3333333333333333703, 0.3219752754296894559, 0.3333333333333333703, 0.3219752754296894559, 0.3333333333333333703, 0.3219752754296894559, 0.3333333333333333703, 0.3219752754296894559, 0.3333333333333333703, 0.3219752754296894559, 0.3333333333333333703, 0.3219752754296894559, 0.3333333333333333703, 0.3219752754296894559, 0.3333333333333333703, 0.3219752754296894559, 0.3333333333333333703, 0.3219752754296894559, 0.3333333333333333703, 0.3219752754296894559, 0.3333333333333333703, 0.3219752754296894559, 0.3333333333333333703, 0.3219752754296894559, 0.3333333333333333703, 0.3219752754296894559, 0.3333333333333333703, 0.3219752754296894559, 0.3333333333333333703, 0.3219752754296894559, 0.3333333333333333703, 0.3219752754296894559, 0.3333333333333333703, 0.3219752754296894559, 0.3333333333333333703, 0.3219752754296894559, 0.3333333333333333703, 0.3219752754296894559, 0.3333333333333333703, 0.3219752754296894559, 0.3333333333333333703, 0.3219752754296894559, 0.3333333333333333703, 0.3219752754296894559, 0.3333333333333333703, 0.3219752754296894559, 0.3333333333333333703, 0.3219752754296894559, 0.3333333333333333703, 0.3219752754296894559, 0.3333333333333333703, 0.3219752754296894559, 0.3333333333333333703, 0.3219752754296894559, 0.3333333333333333703, 0.3219752754296894559, 0.3333333333333333703, 0.3219752754296894559, 0.3333333333333333703, 0.3219752754296894559, 0.3333333333333333703, 0.3219752754296894559, 0.3333333333333333703, 0.3219752754296894559, 0.3333333333333333703, 0.3219752754296894559, 0.3333333333333333703, 0.3219752754296894559, 0.3333333333333333703, 0.3219752754296894559, 0.3333333333333333703, 0.3219752754296894559, 0.3333333333333333703, 0.3219752754296894559, 0.3333333333333333703, 0.3219752754296894559, 0.3333333333333333703, 0.3219752754296894559, 0.3333333333333333703, 0.3219752754296894559, 0.3333333333333333703, 0.3219752754296894559, 0.3333333333333333703, 0.3219752754296894559, 0.3333333333333333703, 0.3219752754296894559, 0.3333333333333333703, 0.3219752754296894559, 0.3333333333333333703, 0.3219752754296894559, 0.3333333333333333703, 0.3219752754296894559, 0.3333333333333333703, 0.3219752754296894559, 0.3333333333333333703, 0.3219752754296894559, 0.3333333333333333703, 0.3219752754296894559, 0.3333333333333333703, 0.3219752754296894559, 0.3333333333333333703, 0.3219752754296894559, 0.3333333333333333703, 0.3219752754296894559, 0.3333333333333333703, 0.3219752754296894559, 0.3333333333333333703, 0.3219752754296894559, 0.3333333333333333703, 0.3219752754296894559, 0.3333333333333333703, 0.3219752754296894559, 0.3333333333333333703, 0.3219752754296894559, 0.3333333333333333703, 0.3219752754296894559, 0.3333333333333333703, 0.3219752754296894559, 0.3333333333333333703, 0.3219752754296894559, 0.3333333333333333703, 0.3219752754296894559, 0.3333333333333333703, 0.3219752754296894559, 0.3333333333333333703, 0.3219752754296894559, 0.3333333333333333703, 0.3219752754296894559, 0.3333333333333333703, 0.3219752754296894559, 0.3333333333333333703, 0.3219752754296894559, 0.3333333333333333703, 0.3219752754296894559, 0.3333333333333333703, 0.3219752754296894559, 0.3333333333333333703, 0.3219752754296894559, 0.3333333333333333703, 0.3219752754296894559, 0.3333333333333333703, 0.3219752754296894559, 0.3333333333333333703, 0.3219752754296894559, 0.3333333333333333703, 0.3219752754296894559, 0.3333333333333333703, 0.3219752754296894559, 0.3333333333333333703, 0.3219752754296894559, 0.3333333333333333703, 0.3219752754296894559, 0.3333333333333333703, 0.3219752754296894559, 0.3333333333333333703, 0.3219752754296894559, 0.3333333333333333703, 0.3219752754296894559, 0.3333333333333333703, 0.3219752754296894559, 0.3333333333333333703, 0.3219752754296894559, 0.3333333333333333703, 0.3219752754296894559, 0.3333333333333333703, 0.3219752754296894559, 0.3333333333333333703, 0.3219752754296894559, 0.3333333333333333703, 0.3219752754296894559, 0.3333333333333333703, 0.3219752754296894559, 0.3333333333333333703, 0.3219752754296894559, 0.3333333333333333703, 0.3219752754296894559, 0.3333333333333333703, 0.3219752754296894559, 0.3333333333333333703, 0.3219752754296894559, 0.3333333333333333703, 0.3219752754296894559, 0.3333333333333333703, 0.3219752754296894559, 0.3333333333333333703, 0.3219752754296894559, 0.3333333333333333703, 0.3219752754296894559, 0.3333333333333333703, 0.3219752754296894559, 0.3333333333333333703, 0.3219752754296894559, 0.3333333333333333703, 0.3219752754296894559, 0.3333333333333333703, 0.3219752754296894559, 0.3333333333333333703, 0.3219752754296894559, 0.3333333333333333703, 0.3219752754296894559, 0.3333333333333333703, 0.3219752754296894559, 0.3333333333333333703, 0.3219752754296894559, 0.3333333333333333703),
 ( 1.000000000000000000, 0.9659258262890683122, 1.000000000000000000, 0.9659258262890683122, 1.000000000000000000, 0.9659258262890683122, 1.000000000000000000, 0.9659258262890683122, 1.000000000000000000, 0.9659258262890683122, 1.000000000000000000, 0.9659258262890683122, 1.000000000000000000, 0.9659258262890683122, 1.000000000000000000, 0.9659258262890683122, 1.000000000000000000, 0.9659258262890683122, 1.000000000000000000, 0.9659258262890683122, 1.000000000000000000, 0.9659258262890683122, 1.000000000000000000, 0.9659258262890683122, 1.000000000000000000, 0.9659258262890683122, 1.000000000000000000, 0.9659258262890683122, 1.000000000000000000, 0.9659258262890683122, 1.000000000000000000, 0.9659258262890683122, 1.000000000000000000, 0.9659258262890683122, 1.000000000000000000, 0.9659258262890683122, 1.000000000000000000, 0.9659258262890683122, 1.000000000000000000, 0.9659258262890683122, 1.000000000000000000, 0.9659258262890683122, 1.000000000000000000, 0.9659258262890683122, 1.000000000000000000, 0.9659258262890683122, 1.000000000000000000, 0.9659258262890683122, 1.000000000000000000, 0.9659258262890683122, 1.000000000000000000, 0.9659258262890683122, 1.000000000000000000, 0.9659258262890683122, 1.000000000000000000, 0.9659258262890683122, 1.000000000000000000, 0.9659258262890683122, 1.000000000000000000, 0.9659258262890683122, 1.000000000000000000, 0.9659258262890683122, 1.000000000000000000, 0.9659258262890683122, 1.000000000000000000, 0.9659258262890683122, 1.000000000000000000, 0.9659258262890683122, 1.000000000000000000, 0.9659258262890683122, 1.000000000000000000, 0.9659258262890683122, 1.000000000000000000, 0.9659258262890683122, 1.000000000000000000, 0.9659258262890683122, 1.000000000000000000, 0.9659258262890683122, 1.000000000000000000, 0.9659258262890683122, 1.000000000000000000, 0.9659258262890683122, 1.000000000000000000, 0.9659258262890683122, 1.000000000000000000, 0.9659258262890683122, 1.000000000000000000, 0.9659258262890683122, 1.000000000000000000, 0.9659258262890683122, 1.000000000000000000, 0.9659258262890683122, 1.000000000000000000, 0.9659258262890683122, 1.000000000000000000, 0.9659258262890683122, 1.000000000000000000, 0.9659258262890683122, 1.000000000000000000, 0.9659258262890683122, 1.000000000000000000, 0.9659258262890683122, 1.000000000000000000, 0.9659258262890683122, 1.000000000000000000, 0.9659258262890683122, 1.000000000000000000, 0.9659258262890683122, 1.000000000000000000, 0.9659258262890683122, 1.000000000000000000, 0.9659258262890683122, 1.000000000000000000, 0.9659258262890683122, 1.000000000000000000, 0.9659258262890683122, 1.000000000000000000, 0.9659258262890683122, 1.000000000000000000, 0.9659258262890683122, 1.000000000000000000, 0.9659258262890683122, 1.000000000000000000, 0.9659258262890683122, 1.000000000000000000, 0.9659258262890683122, 1.000000000000000000, 0.9659258262890683122, 1.000000000000000000, 0.9659258262890683122, 1.000000000000000000, 0.9659258262890683122, 1.000000000000000000, 0.9659258262890683122, 1.000000000000000000, 0.9659258262890683122, 1.000000000000000000, 0.9659258262890683122, 1.000000000000000000, 0.9659258262890683122, 1.000000000000000000, 0.9659258262890683122, 1.000000000000000000, 0.9659258262890683122, 1.000000000000000000, 0.9659258262890683122, 1.000000000000000000, 0.9659258262890683122, 1.000000000000000000, 0.9659258262890683122, 1.000000000000000000, 0.9659258262890683122, 1.000000000000000000, 0.9659258262890683122, 1.000000000000000000, 0.9659258262890683122, 1.000000000000000000, 0.9659258262890683122, 1.000000000000000000, 0.9659258262890683122, 1.000000000000000000, 0.9659258262890683122, 1.000000000000000000, 0.9659258262890683122, 1.000000000000000000, 0.9659258262890683122, 1.000000000000000000, 0.9659258262890683122, 1.000000000000000000, 0.9659258262890683122, 1.000000000000000000, 0.9659258262890683122, 1.000000000000000000, 0.9659258262890683122, 1.000000000000000000, 0.9659258262890683122, 1.000000000000000000, 0.9659258262890683122, 1.000000000000000000, 0.9659258262890683122, 1.000000000000000000, 0.9659258262890683122, 1.000000000000000000, 0.9659258262890683122, 1.000000000000000000, 0.9659258262890683122, 1.000000000000000000, 0.9659258262890683122, 1.000000000000000000, 0.9659258262890683122, 1.000000000000000000, 0.9659258262890683122, 1.000000000000000000, 0.9659258262890683122, 1.000000000000000000, 0.9659258262890683122, 1.000000000000000000, 0.9659258262890683122, 1.000000000000000000, 0.9659258262890683122, 1.000000000000000000, 0.9659258262890683122, 1.000000000000000000, 0.9659258262890683122, 1.000000000000000000, 0.9659258262890683122, 1.000000000000000000, 0.9659258262890683122, 1.000000000000000000, 0.9659258262890683122, 1.000000000000000000, 0.9659258262890683122, 1.000000000000000000, 0.9659258262890683122, 1.000000000000000000, 0.9659258262890683122, 1.000000000000000000, 0.9659258262890683122, 1.000000000000000000, 0.9659258262890683122, 1.000000000000000000, 0.9659258262890683122, 1.000000000000000000, 0.9659258262890683122, 1.000000000000000000, 0.9659258262890683122, 1.000000000000000000, 0.9659258262890683122, 1.000000000000000000, 0.9659258262890683122, 1.000000000000000000, 0.9659258262890683122, 1.000000000000000000, 0.9659258262890683122, 1.000000000000000000, 0.9659258262890683122, 1.000000000000000000, 0.9659258262890683122, 1.000000000000000000, 0.9659258262890683122, 1.000000000000000000, 0.9659258262890683122, 1.000000000000000000, 0.9659258262890683122, 1.000000000000000000, 0.9659258262890683122, 1.000000000000000000, 0.9659258262890683122, 1.000000000000000000, 0.9659258262890683122, 1.000000000000000000, 0.9659258262890683122, 1.000000000000000000, 0.9659258262890683122, 1.000000000000000000, 0.9659258262890683122, 1.000000000000000000, 0.9659258262890683122, 1.000000000000000000, 0.9659258262890683122, 1.000000000000000000, 0.9659258262890683122, 1.000000000000000000, 0.9659258262890683122, 1.000000000000000000, 0.9659258262890683122, 1.000000000000000000, 0.9659258262890683122, 1.000000000000000000, 0.9659258262890683122, 1.000000000000000000, 0.9659258262890683122, 1.000000000000000000, 0.9659258262890683122, 1.000000000000000000, 0.9659258262890683122, 1.000000000000000000, 0.9659258262890683122, 1.000000000000000000, 0.9659258262890683122, 1.000000000000000000, 0.9659258262890683122, 1.000000000000000000, 0.9659258262890683122, 1.000000000000000000, 0.9659258262890683122, 1.000000000000000000, 0.9659258262890683122, 1.000000000000000000, 0.9659258262890683122, 1.000000000000000000, 0.9659258262890683122, 1.000000000000000000, 0.9659258262890683122, 1.000000000000000000, 0.9659258262890683122, 1.000000000000000000, 0.9659258262890683122, 1.000000000000000000, 0.9659258262890683122, 1.000000000000000000, 0.9659258262890683122, 1.000000000000000000, 0.9659258262890683122, 1.000000000000000000, 0.9659258262890683122, 1.000000000000000000, 0.9659258262890683122, 1.000000000000000000, 0.9659258262890683122, 1.000000000000000000, 0.9659258262890683122, 1.000000000000000000, 0.9659258262890683122, 1.000000000000000000, 0.9659258262890683122, 1.000000000000000000, 0.9659258262890683122, 1.000000000000000000, 0.9659258262890683122, 1.000000000000000000, 0.9659258262890683122, 1.000000000000000000, 0.9659258262890683122, 1.000000000000000000, 0.9659258262890683122, 1.000000000000000000, 0.9659258262890683122, 1.000000000000000000, 0.9659258262890683122, 1.000000000000000000, 0.9659258262890683122, 1.000000000000000000, 0.9659258262890683122, 1.000000000000000000, 0.9659258262890683122, 1.000000000000000000, 0.9659258262890683122, 1.000000000000000000, 0.9659258262890683122, 1.000000000000000000, 0.9659258262890683122, 1.000000000000000000, 0.9659258262890683122, 1.000000000000000000, 0.9659258262890683122, 1.000000000000000000, 0.9659258262890683122, 1.000000000000000000, 0.9659258262890683122, 1.000000000000000000, 0.9659258262890683122, 1.000000000000000000, 0.9659258262890683122, 1.000000000000000000, 0.9659258262890683122, 1.000000000000000000, 0.9659258262890683122, 1.000000000000000000, 0.9659258262890683122, 1.000000000000000000, 0.9659258262890683122, 1.000000000000000000, 0.9659258262890683122, 1.000000000000000000, 0.9659258262890683122, 1.000000000000000000, 0.9659258262890683122, 1.000000000000000000, 0.9659258262890683122, 1.000000000000000000, 0.9659258262890683122, 1.000000000000000000, 0.9659258262890683122, 1.000000000000000000, 0.9659258262890683122, 1.000000000000000000, 0.9659258262890683122, 1.000000000000000000, 0.9659258262890683122, 1.000000000000000000, 0.9659258262890683122, 1.000000000000000000, 0.9659258262890683122, 1.000000000000000000, 0.9659258262890683122, 1.000000000000000000, 0.9659258262890683122, 1.000000000000000000, 0.9659258262890683122, 1.000000000000000000, 0.9659258262890683122, 1.000000000000000000, 0.9659258262890683122, 1.000000000000000000, 0.9659258262890683122, 1.000000000000000000, 0.9659258262890683122, 1.000000000000000000, 0.9659258262890683122, 1.000000000000000000, 0.9659258262890683122, 1.000000000000000000, 0.9659258262890683122, 1.000000000000000000, 0.9659258262890683122, 1.000000000000000000, 0.9659258262890683122, 1.000000000000000000, 0.9659258262890683122, 1.000000000000000000, 0.9659258262890683122, 1.000000000000000000, 0.9659258262890683122, 1.000000000000000000, 0.9659258262890683122, 1.000000000000000000, 0.9659258262890683122, 1.000000000000000000, 0.9659258262890683122, 1.000000000000000000, 0.9659258262890683122, 1.000000000000000000, 0.9659258262890683122, 1.000000000000000000, 0.9659258262890683122, 1.000000000000000000, 0.9659258262890683122, 1.000000000000000000, 0.9659258262890683122, 1.000000000000000000, 0.9659258262890683122, 1.000000000000000000, 0.9659258262890683122, 1.000000000000000000, 0.9659258262890683122, 1.000000000000000000, 0.9659258262890683122, 1.000000000000000000, 0.9659258262890683122, 1.000000000000000000, 0.9659258262890683122, 1.000000000000000000, 0.9659258262890683122, 1.000000000000000000, 0.9659258262890683122, 1.000000000000000000, 0.9659258262890683122, 1.000000000000000000, 0.9659258262890683122, 1.000000000000000000, 0.9659258262890683122, 1.000000000000000000, 0.9659258262890683122, 1.000000000000000000, 0.9659258262890683122, 1.000000000000000000),
 ( 0.3333333333333333703, 0.3219752754296894559, 0.3333333333333333703, 0.3219752754296894559, 0.3333333333333333703, 0.3219752754296894559, 0.3333333333333333703, 0.3219752754296894559, 0.3333333333333333703, 0.3219752754296894559, 0.3333333333333333703, 0.3219752754296894559, 0.3333333333333333703, 0.3219752754296894559, 0.3333333333333333703, 0.3219752754296894559, 0.3333333333333333703, 0.3219752754296894559, 0.3333333333333333703, 0.3219752754296894559, 0.3333333333333333703, 0.3219752754296894559, 0.3333333333333333703, 0.3219752754296894559, 0.3333333333333333703, 0.3219752754296894559, 0.3333333333333333703, 0.3219752754296894559, 0.3333333333333333703, 0.3219752754296894559, 0.3333333333333333703, 0.3219752754296894559, 0.3333333333333333703, 0.3219752754296894559, 0.3333333333333333703, 0.3219752754296894559, 0.3333333333333333703, 0.3219752754296894559, 0.3333333333333333703, 0.3219752754296894559, 0.3333333333333333703, 0.3219752754296894559, 0.3333333333333333703, 0.3219752754296894559, 0.3333333333333333703, 0.3219752754296894559, 0.3333333333333333703, 0.3219752754296894559, 0.3333333333333333703, 0.3219752754296894559, 0.3333333333333333703, 0.3219752754296894559, 0.3333333333333333703, 0.3219752754296894559, 0.3333333333333333703, 0.3219752754296894559, 0.3333333333333333703, 0.3219752754296894559, 0.3333333333333333703, 0.3219752754296894559, 0.3333333333333333703, 0.3219752754296894559, 0.3333333333333333703, 0.3219752754296894559, 0.3333333333333333703, 0.3219752754296894559, 0.3333333333333333703, 0.3219752754296894559, 0.3333333333333333703, 0.3219752754296894559, 0.3333333333333333703, 0.3219752754296894559, 0.3333333333333333703, 0.3219752754296894559, 0.3333333333333333703, 0.3219752754296894559, 0.3333333333333333703, 0.3219752754296894559, 0.3333333333333333703, 0.3219752754296894559, 0.3333333333333333703, 0.3219752754296894559, 0.3333333333333333703, 0.3219752754296894559, 0.3333333333333333703, 0.3219752754296894559, 0.3333333333333333703, 0.3219752754296894559, 0.3333333333333333703, 0.3219752754296894559, 0.3333333333333333703, 0.3219752754296894559, 0.3333333333333333703, 0.3219752754296894559, 0.3333333333333333703, 0.3219752754296894559, 0.3333333333333333703, 0.3219752754296894559, 0.3333333333333333703, 0.3219752754296894559, 0.3333333333333333703, 0.3219752754296894559, 0.3333333333333333703, 0.3219752754296894559, 0.3333333333333333703, 0.3219752754296894559, 0.3333333333333333703, 0.3219752754296894559, 0.3333333333333333703, 0.3219752754296894559, 0.3333333333333333703, 0.3219752754296894559, 0.3333333333333333703, 0.3219752754296894559, 0.3333333333333333703, 0.3219752754296894559, 0.3333333333333333703, 0.3219752754296894559, 0.3333333333333333703, 0.3219752754296894559, 0.3333333333333333703, 0.3219752754296894559, 0.3333333333333333703, 0.3219752754296894559, 0.3333333333333333703, 0.3219752754296894559, 0.3333333333333333703, 0.3219752754296894559, 0.3333333333333333703, 0.3219752754296894559, 0.3333333333333333703, 0.3219752754296894559, 0.3333333333333333703, 0.3219752754296894559, 0.3333333333333333703, 0.3219752754296894559, 0.3333333333333333703, 0.3219752754296894559, 0.3333333333333333703, 0.3219752754296894559, 0.3333333333333333703, 0.3219752754296894559, 0.3333333333333333703, 0.3219752754296894559, 0.3333333333333333703, 0.3219752754296894559, 0.3333333333333333703, 0.3219752754296894559, 0.3333333333333333703, 0.3219752754296894559, 0.3333333333333333703, 0.3219752754296894559, 0.3333333333333333703, 0.3219752754296894559, 0.3333333333333333703, 0.3219752754296894559, 0.3333333333333333703, 0.3219752754296894559, 0.3333333333333333703, 0.3219752754296894559, 0.3333333333333333703, 0.3219752754296894559, 0.3333333333333333703, 0.3219752754296894559, 0.3333333333333333703, 0.3219752754296894559, 0.3333333333333333703, 0.3219752754296894559, 0.3333333333333333703, 0.3219752754296894559, 0.3333333333333333703, 0.3219752754296894559, 0.3333333333333333703, 0.3219752754296894559, 0.3333333333333333703, 0.3219752754296894559, 0.3333333333333333703, 0.3219752754296894559, 0.3333333333333333703, 0.3219752754296894559, 0.3333333333333333703, 0.3219752754296894559, 0.3333333333333333703, 0.3219752754296894559, 0.3333333333333333703, 0.3219752754296894559, 0.3333333333333333703, 0.3219752754296894559, 0.3333333333333333703, 0.3219752754296894559, 0.3333333333333333703, 0.3219752754296894559, 0.3333333333333333703, 0.3219752754296894559, 0.3333333333333333703, 0.3219752754296894559, 0.3333333333333333703, 0.3219752754296894559, 0.3333333333333333703, 0.3219752754296894559, 0.3333333333333333703, 0.3219752754296894559, 0.3333333333333333703, 0.3219752754296894559, 0.3333333333333333703, 0.3219752754296894559, 0.3333333333333333703, 0.3219752754296894559, 0.3333333333333333703, 0.3219752754296894559, 0.3333333333333333703, 0.3219752754296894559, 0.3333333333333333703, 0.3219752754296894559, 0.3333333333333333703, 0.3219752754296894559, 0.3333333333333333703, 0.3219752754296894559, 0.3333333333333333703, 0.3219752754296894559, 0.3333333333333333703, 0.3219752754296894559, 0.3333333333333333703, 0.3219752754296894559, 0.3333333333333333703, 0.3219752754296894559, 0.3333333333333333703, 0.3219752754296894559, 0.3333333333333333703, 0.3219752754296894559, 0.3333333333333333703, 0.3219752754296894559, 0.3333333333333333703, 0.3219752754296894559, 0.3333333333333333703, 0.3219752754296894559, 0.3333333333333333703, 0.3219752754296894559, 0.3333333333333333703, 0.3219752754296894559, 0.3333333333333333703, 0.3219752754296894559, 0.3333333333333333703, 0.3219752754296894559, 0.3333333333333333703, 0.3219752754296894559, 0.3333333333333333703, 0.3219752754296894559, 0.3333333333333333703, 0.3219752754296894559, 0.3333333333333333703, 0.3219752754296894559, 0.3333333333333333703, 0.3219752754296894559, 0.3333333333333333703, 0.3219752754296894559, 0.3333333333333333703, 0.3219752754296894559, 0.3333333333333333703, 0.3219752754296894559, 0.3333333333333333703, 0.3219752754296894559, 0.3333333333333333703, 0.3219752754296894559, 0.3333333333333333703, 0.3219752754296894559, 0.3333333333333333703, 0.3219752754296894559, 0.3333333333333333703, 0.3219752754296894559, 0.3333333333333333703, 0.3219752754296894559, 0.3333333333333333703, 0.3219752754296894559, 0.3333333333333333703, 0.3219752754296894559, 0.3333333333333333703, 0.3219752754296894559, 0.3333333333333333703, 0.3219752754296894559, 0.3333333333333333703, 0.3219752754296894559, 0.3333333333333333703, 0.3219752754296894559, 0.3333333333333333703, 0.3219752754296894559, 0.3333333333333333703, 0.3219752754296894559, 0.3333333333333333703, 0.3219752754296894559, 0.3333333333333333703, 0.3219752754296894559, 0.3333333333333333703, 0.3219752754296894559, 0.3333333333333333703, 0.3219752754296894559, 0.3333333333333333703, 0.3219752754296894559, 0.3333333333333333703, 0.3219752754296894559, 0.3333333333333333703, 0.3219752754296894559, 0.3333333333333333703, 0.3219752754296894559, 0.3333333333333333703, 0.3219752754296894559, 0.3333333333333333703, 0.3219752754296894559, 0.3333333333333333703, 0.3219752754296894559, 0.3333333333333333703, 0.3219752754296894559, 0.3333333333333333703, 0.3219752754296894559, 0.3333333333333333703, 0.3219752754296894559, 0.3333333333333333703, 0.3219752754296894559, 0.3333333333333333703, 0.3219752754296894559, 0.3333333333333333703, 0.3219752754296894559, 0.3333333333333333703, 0.3219752754296894559, 0.3333333333333333703, 0.3219752754296894559, 0.3333333333333333703, 0.3219752754296894559, 0.3333333333333333703, 0.3219752754296894559, 0.3333333333333333703, 0.3219752754296894559, 0.3333333333333333703, 0.3219752754296894559, 0.3333333333333333703, 0.3219752754296894559, 0.3333333333333333703, 0.3219752754296894559, 0.3333333333333333703, 0.3219752754296894559, 0.3333333333333333703, 0.3219752754296894559, 0.3333333333333333703, 0.3219752754296894559, 0.3333333333333333703, 0.3219752754296894559, 0.3333333333333333703, 0.3219752754296894559, 0.3333333333333333703, 0.3219752754296894559, 0.3333333333333333703, 0.3219752754296894559, 0.3333333333333333703, 0.3219752754296894559, 0.3333333333333333703, 0.3219752754296894559, 0.3333333333333333703, 0.3219752754296894559, 0.3333333333333333703, 0.3219752754296894559, 0.3333333333333333703, 0.3219752754296894559, 0.3333333333333333703, 0.3219752754296894559, 0.3333333333333333703, 0.3219752754296894559, 0.3333333333333333703, 0.3219752754296894559, 0.3333333333333333703, 0.3219752754296894559, 0.3333333333333333703, 0.3219752754296894559, 0.3333333333333333703, 0.3219752754296894559, 0.3333333333333333703, 0.3219752754296894559, 0.3333333333333333703, 0.3219752754296894559, 0.3333333333333333703, 0.3219752754296894559, 0.3333333333333333703, 0.3219752754296894559, 0.3333333333333333703, 0.3219752754296894559, 0.3333333333333333703, 0.3219752754296894559, 0.3333333333333333703, 0.3219752754296894559, 0.3333333333333333703, 0.3219752754296894559, 0.3333333333333333703, 0.3219752754296894559, 0.3333333333333333703, 0.3219752754296894559, 0.3333333333333333703, 0.3219752754296894559, 0.3333333333333333703, 0.3219752754296894559, 0.3333333333333333703, 0.3219752754296894559, 0.3333333333333333703, 0.3219752754296894559, 0.3333333333333333703, 0.3219752754296894559, 0.3333333333333333703, 0.3219752754296894559, 0.3333333333333333703, 0.3219752754296894559, 0.3333333333333333703, 0.3219752754296894559, 0.3333333333333333703, 0.3219752754296894559, 0.3333333333333333703, 0.3219752754296894559, 0.3333333333333333703, 0.3219752754296894559, 0.3333333333333333703, 0.3219752754296894559, 0.3333333333333333703, 0.3219752754296894559, 0.3333333333333333703, 0.3219752754296894559, 0.3333333333333333703, 0.3219752754296894559, 0.3333333333333333703, 0.3219752754296894559, 0.3333333333333333703, 0.3219752754296894559, 0.3333333333333333703, 0.3219752754296894559, 0.3333333333333333703, 0.3219752754296894559, 0.3333333333333333703, 0.3219752754296894559, 0.3333333333333333703, 0.3219752754296894559, 0.3333333333333333703, 0.3219752754296894559, 0.3333333333333333703, 0.3219752754296894559, 0.3333333333333333703, 0.3219752754296894559, 0.3333333333333333703, 0.3219752754296894559, 0.3333333333333333703, 0.3219752754296894559, 0.3333333333333333703, 0.3219752754296894559, 0.3333333333333333703, 0.3219752754296894559, 0.3333333333333333703, 0.3219752754296894559, 0.3333333333333333703, 0.3219752754296894559, 0.3333333333333333703, 0.3219752754296894559, 0.3333333333333333703),
 ( 0.3333333333333333703, 0.3219752754296894559, 0.3333333333333333703, 0.3219752754296894559, 0.3333333333333333703, 0.3219752754296894559, 0.3333333333333333703, 0.3219752754296894559, 0.3333333333333333703, 0.3219752754296894559, 0.3333333333333333703, 0.3219752754296894559, 0.3333333333333333703, 0.3219752754296894559, 0.3333333333333333703, 0.3219752754296894559, 0.3333333333333333703, 0.3219752754296894559, 0.3333333333333333703, 0.3219752754296894559, 0.3333333333333333703, 0.3219752754296894559, 0.3333333333333333703, 0.3219752754296894559, 0.3333333333333333703, 0.3219752754296894559, 0.3333333333333333703, 0.3219752754296894559, 0.3333333333333333703, 0.3219752754296894559, 0.3333333333333333703, 0.3219752754296894559, 0.3333333333333333703, 0.3219752754296894559, 0.3333333333333333703, 0.3219752754296894559, 0.3333333333333333703, 0.3219752754296894559, 0.3333333333333333703, 0.3219752754296894559, 0.3333333333333333703, 0.3219752754296894559, 0.3333333333333333703, 0.3219752754296894559, 0.3333333333333333703, 0.3219752754296894559, 0.3333333333333333703, 0.3219752754296894559, 0.3333333333333333703, 0.3219752754296894559, 0.3333333333333333703, 0.3219752754296894559, 0.3333333333333333703, 0.3219752754296894559, 0.3333333333333333703, 0.3219752754296894559, 0.3333333333333333703, 0.3219752754296894559, 0.3333333333333333703, 0.3219752754296894559, 0.3333333333333333703, 0.3219752754296894559, 0.3333333333333333703, 0.3219752754296894559, 0.3333333333333333703, 0.3219752754296894559, 0.3333333333333333703, 0.3219752754296894559, 0.3333333333333333703, 0.3219752754296894559, 0.3333333333333333703, 0.3219752754296894559, 0.3333333333333333703, 0.3219752754296894559, 0.3333333333333333703, 0.3219752754296894559, 0.3333333333333333703, 0.3219752754296894559, 0.3333333333333333703, 0.3219752754296894559, 0.3333333333333333703, 0.3219752754296894559, 0.3333333333333333703, 0.3219752754296894559, 0.3333333333333333703, 0.3219752754296894559, 0.3333333333333333703, 0.3219752754296894559, 0.3333333333333333703, 0.3219752754296894559, 0.3333333333333333703, 0.3219752754296894559, 0.3333333333333333703, 0.3219752754296894559, 0.3333333333333333703, 0.3219752754296894559, 0.3333333333333333703, 0.3219752754296894559, 0.3333333333333333703, 0.3219752754296894559, 0.3333333333333333703, 0.3219752754296894559, 0.3333333333333333703, 0.3219752754296894559, 0.3333333333333333703, 0.3219752754296894559, 0.3333333333333333703, 0.3219752754296894559, 0.3333333333333333703, 0.3219752754296894559, 0.3333333333333333703, 0.3219752754296894559, 0.3333333333333333703, 0.3219752754296894559, 0.3333333333333333703, 0.3219752754296894559, 0.3333333333333333703, 0.3219752754296894559, 0.3333333333333333703, 0.3219752754296894559, 0.3333333333333333703, 0.3219752754296894559, 0.3333333333333333703, 0.3219752754296894559, 0.3333333333333333703, 0.3219752754296894559, 0.3333333333333333703, 0.3219752754296894559, 0.3333333333333333703, 0.3219752754296894559, 0.3333333333333333703, 0.3219752754296894559, 0.3333333333333333703, 0.3219752754296894559, 0.3333333333333333703, 0.3219752754296894559, 0.3333333333333333703, 0.3219752754296894559, 0.3333333333333333703, 0.3219752754296894559, 0.3333333333333333703, 0.3219752754296894559, 0.3333333333333333703, 0.3219752754296894559, 0.3333333333333333703, 0.3219752754296894559, 0.3333333333333333703, 0.3219752754296894559, 0.3333333333333333703, 0.3219752754296894559, 0.3333333333333333703, 0.3219752754296894559, 0.3333333333333333703, 0.3219752754296894559, 0.3333333333333333703, 0.3219752754296894559, 0.3333333333333333703, 0.3219752754296894559, 0.3333333333333333703, 0.3219752754296894559, 0.3333333333333333703, 0.3219752754296894559, 0.3333333333333333703, 0.3219752754296894559, 0.3333333333333333703, 0.3219752754296894559, 0.3333333333333333703, 0.3219752754296894559, 0.3333333333333333703, 0.3219752754296894559, 0.3333333333333333703, 0.3219752754296894559, 0.3333333333333333703, 0.3219752754296894559, 0.3333333333333333703, 0.3219752754296894559, 0.3333333333333333703, 0.3219752754296894559, 0.3333333333333333703, 0.3219752754296894559, 0.3333333333333333703, 0.3219752754296894559, 0.3333333333333333703, 0.3219752754296894559, 0.3333333333333333703, 0.3219752754296894559, 0.3333333333333333703, 0.3219752754296894559, 0.3333333333333333703, 0.3219752754296894559, 0.3333333333333333703, 0.3219752754296894559, 0.3333333333333333703, 0.3219752754296894559, 0.3333333333333333703, 0.3219752754296894559, 0.3333333333333333703, 0.3219752754296894559, 0.3333333333333333703, 0.3219752754296894559, 0.3333333333333333703, 0.3219752754296894559, 0.3333333333333333703, 0.3219752754296894559, 0.3333333333333333703, 0.3219752754296894559, 0.3333333333333333703, 0.3219752754296894559, 0.3333333333333333703, 0.3219752754296894559, 0.3333333333333333703, 0.3219752754296894559, 0.3333333333333333703, 0.3219752754296894559, 0.3333333333333333703, 0.3219752754296894559, 0.3333333333333333703, 0.3219752754296894559, 0.3333333333333333703, 0.3219752754296894559, 0.3333333333333333703, 0.3219752754296894559, 0.3333333333333333703, 0.3219752754296894559, 0.3333333333333333703, 0.3219752754296894559, 0.3333333333333333703, 0.3219752754296894559, 0.3333333333333333703, 0.3219752754296894559, 0.3333333333333333703, 0.3219752754296894559, 0.3333333333333333703, 0.3219752754296894559, 0.3333333333333333703, 0.3219752754296894559, 0.3333333333333333703, 0.3219752754296894559, 0.3333333333333333703, 0.3219752754296894559, 0.3333333333333333703, 0.3219752754296894559, 0.3333333333333333703, 0.3219752754296894559, 0.3333333333333333703, 0.3219752754296894559, 0.3333333333333333703, 0.3219752754296894559, 0.3333333333333333703, 0.3219752754296894559, 0.3333333333333333703, 0.3219752754296894559, 0.3333333333333333703, 0.3219752754296894559, 0.3333333333333333703, 0.3219752754296894559, 0.3333333333333333703, 0.3219752754296894559, 0.3333333333333333703, 0.3219752754296894559, 0.3333333333333333703, 0.3219752754296894559, 0.3333333333333333703, 0.3219752754296894559, 0.3333333333333333703, 0.3219752754296894559, 0.3333333333333333703, 0.3219752754296894559, 0.3333333333333333703, 0.3219752754296894559, 0.3333333333333333703, 0.3219752754296894559, 0.3333333333333333703, 0.3219752754296894559, 0.3333333333333333703, 0.3219752754296894559, 0.3333333333333333703, 0.3219752754296894559, 0.3333333333333333703, 0.3219752754296894559, 0.3333333333333333703, 0.3219752754296894559, 0.3333333333333333703, 0.3219752754296894559, 0.3333333333333333703, 0.3219752754296894559, 0.3333333333333333703, 0.3219752754296894559, 0.3333333333333333703, 0.3219752754296894559, 0.3333333333333333703, 0.3219752754296894559, 0.3333333333333333703, 0.3219752754296894559, 0.3333333333333333703, 0.3219752754296894559, 0.3333333333333333703, 0.3219752754296894559, 0.3333333333333333703, 0.3219752754296894559, 0.3333333333333333703, 0.3219752754296894559, 0.3333333333333333703, 0.3219752754296894559, 0.3333333333333333703, 0.3219752754296894559, 0.3333333333333333703, 0.3219752754296894559, 0.3333333333333333703, 0.3219752754296894559, 0.3333333333333333703, 0.3219752754296894559, 0.3333333333333333703, 0.3219752754296894559, 0.3333333333333333703, 0.3219752754296894559, 0.3333333333333333703, 0.3219752754296894559, 0.3333333333333333703, 0.3219752754296894559, 0.3333333333333333703, 0.3219752754296894559, 0.3333333333333333703, 0.3219752754296894559, 0.3333333333333333703, 0.3219752754296894559, 0.3333333333333333703, 0.3219752754296894559, 0.3333333333333333703, 0.3219752754296894559, 0.3333333333333333703, 0.3219752754296894559, 0.3333333333333333703, 0.3219752754296894559, 0.3333333333333333703, 0.3219752754296894559, 0.3333333333333333703, 0.3219752754296894559, 0.3333333333333333703, 0.3219752754296894559, 0.3333333333333333703, 0.3219752754296894559, 0.3333333333333333703, 0.3219752754296894559, 0.3333333333333333703, 0.3219752754296894559, 0.3333333333333333703, 0.3219752754296894559, 0.3333333333333333703, 0.3219752754296894559, 0.3333333333333333703, 0.3219752754296894559, 0.3333333333333333703, 0.3219752754296894559, 0.3333333333333333703, 0.3219752754296894559, 0.3333333333333333703, 0.3219752754296894559, 0.3333333333333333703, 0.3219752754296894559, 0.3333333333333333703, 0.3219752754296894559, 0.3333333333333333703, 0.3219752754296894559, 0.3333333333333333703, 0.3219752754296894559, 0.3333333333333333703, 0.3219752754296894559, 0.3333333333333333703, 0.3219752754296894559, 0.3333333333333333703, 0.3219752754296894559, 0.3333333333333333703, 0.3219752754296894559, 0.3333333333333333703, 0.3219752754296894559, 0.3333333333333333703, 0.3219752754296894559, 0.3333333333333333703, 0.3219752754296894559, 0.3333333333333333703, 0.3219752754296894559, 0.3333333333333333703, 0.3219752754296894559, 0.3333333333333333703, 0.3219752754296894559, 0.3333333333333333703, 0.3219752754296894559, 0.3333333333333333703, 0.3219752754296894559, 0.3333333333333333703, 0.3219752754296894559, 0.3333333333333333703, 0.3219752754296894559, 0.3333333333333333703, 0.3219752754296894559, 0.3333333333333333703, 0.3219752754296894559, 0.3333333333333333703, 0.3219752754296894559, 0.3333333333333333703, 0.3219752754296894559, 0.3333333333333333703, 0.3219752754296894559, 0.3333333333333333703, 0.3219752754296894559, 0.3333333333333333703, 0.3219752754296894559, 0.3333333333333333703, 0.3219752754296894559, 0.3333333333333333703, 0.3219752754296894559, 0.3333333333333333703, 0.3219752754296894559, 0.3333333333333333703, 0.3219752754296894559, 0.3333333333333333703, 0.3219752754296894559, 0.3333333333333333703, 0.3219752754296894559, 0.3333333333333333703, 0.3219752754296894559, 0.3333333333333333703, 0.3219752754296894559, 0.3333333333333333703, 0.3219752754296894559, 0.3333333333333333703, 0.3219752754296894559, 0.3333333333333333703, 0.3219752754296894559, 0.3333333333333333703, 0.3219752754296894559, 0.3333333333333333703, 0.3219752754296894559, 0.3333333333333333703, 0.3219752754296894559, 0.3333333333333333703, 0.3219752754296894559, 0.3333333333333333703, 0.3219752754296894559, 0.3333333333333333703, 0.3219752754296894559, 0.3333333333333333703, 0.3219752754296894559, 0.3333333333333333703, 0.3219752754296894559, 0.3333333333333333703, 0.3219752754296894559, 0.3333333333333333703, 0.3219752754296894559, 0.3333333333333333703, 0.3219752754296894559, 0.3333333333333333703, 0.3219752754296894559, 0.3333333333333333703, 0.3219752754296894559, 0.3333333333333333703),
 ( 1.000000000000000000, 0.9659258262890683122, 1.000000000000000000, 0.9659258262890683122, 1.000000000000000000, 0.9659258262890683122, 1.000000000000000000, 0.9659258262890683122, 1.000000000000000000, 0.9659258262890683122, 1.000000000000000000, 0.9659258262890683122, 1.000000000000000000, 0.9659258262890683122, 1.000000000000000000, 0.9659258262890683122, 1.000000000000000000, 0.9659258262890683122, 1.000000000000000000, 0.9659258262890683122, 1.000000000000000000, 0.9659258262890683122, 1.000000000000000000, 0.9659258262890683122, 1.000000000000000000, 0.9659258262890683122, 1.000000000000000000, 0.9659258262890683122, 1.000000000000000000, 0.9659258262890683122, 1.000000000000000000, 0.9659258262890683122, 1.000000000000000000, 0.9659258262890683122, 1.000000000000000000, 0.9659258262890683122, 1.000000000000000000, 0.9659258262890683122, 1.000000000000000000, 0.9659258262890683122, 1.000000000000000000, 0.9659258262890683122, 1.000000000000000000, 0.9659258262890683122, 1.000000000000000000, 0.9659258262890683122, 1.000000000000000000, 0.9659258262890683122, 1.000000000000000000, 0.9659258262890683122, 1.000000000000000000, 0.9659258262890683122, 1.000000000000000000, 0.9659258262890683122, 1.000000000000000000, 0.9659258262890683122, 1.000000000000000000, 0.9659258262890683122, 1.000000000000000000, 0.9659258262890683122, 1.000000000000000000, 0.9659258262890683122, 1.000000000000000000, 0.9659258262890683122, 1.000000000000000000, 0.9659258262890683122, 1.000000000000000000, 0.9659258262890683122, 1.000000000000000000, 0.9659258262890683122, 1.000000000000000000, 0.9659258262890683122, 1.000000000000000000, 0.9659258262890683122, 1.000000000000000000, 0.9659258262890683122, 1.000000000000000000, 0.9659258262890683122, 1.000000000000000000, 0.9659258262890683122, 1.000000000000000000, 0.9659258262890683122, 1.000000000000000000, 0.9659258262890683122, 1.000000000000000000, 0.9659258262890683122, 1.000000000000000000, 0.9659258262890683122, 1.000000000000000000, 0.9659258262890683122, 1.000000000000000000, 0.9659258262890683122, 1.000000000000000000, 0.9659258262890683122, 1.000000000000000000, 0.9659258262890683122, 1.000000000000000000, 0.9659258262890683122, 1.000000000000000000, 0.9659258262890683122, 1.000000000000000000, 0.9659258262890683122, 1.000000000000000000, 0.9659258262890683122, 1.000000000000000000, 0.9659258262890683122, 1.000000000000000000, 0.9659258262890683122, 1.000000000000000000, 0.9659258262890683122, 1.000000000000000000, 0.9659258262890683122, 1.000000000000000000, 0.9659258262890683122, 1.000000000000000000, 0.9659258262890683122, 1.000000000000000000, 0.9659258262890683122, 1.000000000000000000, 0.9659258262890683122, 1.000000000000000000, 0.9659258262890683122, 1.000000000000000000, 0.9659258262890683122, 1.000000000000000000, 0.9659258262890683122, 1.000000000000000000, 0.9659258262890683122, 1.000000000000000000, 0.9659258262890683122, 1.000000000000000000, 0.9659258262890683122, 1.000000000000000000, 0.9659258262890683122, 1.000000000000000000, 0.9659258262890683122, 1.000000000000000000, 0.9659258262890683122, 1.000000000000000000, 0.9659258262890683122, 1.000000000000000000, 0.9659258262890683122, 1.000000000000000000, 0.9659258262890683122, 1.000000000000000000, 0.9659258262890683122, 1.000000000000000000, 0.9659258262890683122, 1.000000000000000000, 0.9659258262890683122, 1.000000000000000000, 0.9659258262890683122, 1.000000000000000000, 0.9659258262890683122, 1.000000000000000000, 0.9659258262890683122, 1.000000000000000000, 0.9659258262890683122, 1.000000000000000000, 0.9659258262890683122, 1.000000000000000000, 0.9659258262890683122, 1.000000000000000000, 0.9659258262890683122, 1.000000000000000000, 0.9659258262890683122, 1.000000000000000000, 0.9659258262890683122, 1.000000000000000000, 0.9659258262890683122, 1.000000000000000000, 0.9659258262890683122, 1.000000000000000000, 0.9659258262890683122, 1.000000000000000000, 0.9659258262890683122, 1.000000000000000000, 0.9659258262890683122, 1.000000000000000000, 0.9659258262890683122, 1.000000000000000000, 0.9659258262890683122, 1.000000000000000000, 0.9659258262890683122, 1.000000000000000000, 0.9659258262890683122, 1.000000000000000000, 0.9659258262890683122, 1.000000000000000000, 0.9659258262890683122, 1.000000000000000000, 0.9659258262890683122, 1.000000000000000000, 0.9659258262890683122, 1.000000000000000000, 0.9659258262890683122, 1.000000000000000000, 0.9659258262890683122, 1.000000000000000000, 0.9659258262890683122, 1.000000000000000000, 0.9659258262890683122, 1.000000000000000000, 0.9659258262890683122, 1.000000000000000000, 0.9659258262890683122, 1.000000000000000000, 0.9659258262890683122, 1.000000000000000000, 0.9659258262890683122, 1.000000000000000000, 0.9659258262890683122, 1.000000000000000000, 0.9659258262890683122, 1.000000000000000000, 0.9659258262890683122, 1.000000000000000000, 0.9659258262890683122, 1.000000000000000000, 0.9659258262890683122, 1.000000000000000000, 0.9659258262890683122, 1.000000000000000000, 0.9659258262890683122, 1.000000000000000000, 0.9659258262890683122, 1.000000000000000000, 0.9659258262890683122, 1.000000000000000000, 0.9659258262890683122, 1.000000000000000000, 0.9659258262890683122, 1.000000000000000000, 0.9659258262890683122, 1.000000000000000000, 0.9659258262890683122, 1.000000000000000000, 0.9659258262890683122, 1.000000000000000000, 0.9659258262890683122, 1.000000000000000000, 0.9659258262890683122, 1.000000000000000000, 0.9659258262890683122, 1.000000000000000000, 0.9659258262890683122, 1.000000000000000000, 0.9659258262890683122, 1.000000000000000000, 0.9659258262890683122, 1.000000000000000000, 0.9659258262890683122, 1.000000000000000000, 0.9659258262890683122, 1.000000000000000000, 0.9659258262890683122, 1.000000000000000000, 0.9659258262890683122, 1.000000000000000000, 0.9659258262890683122, 1.000000000000000000, 0.9659258262890683122, 1.000000000000000000, 0.9659258262890683122, 1.000000000000000000, 0.9659258262890683122, 1.000000000000000000, 0.9659258262890683122, 1.000000000000000000, 0.9659258262890683122, 1.000000000000000000, 0.9659258262890683122, 1.000000000000000000, 0.9659258262890683122, 1.000000000000000000, 0.9659258262890683122, 1.000000000000000000, 0.9659258262890683122, 1.000000000000000000, 0.9659258262890683122, 1.000000000000000000, 0.9659258262890683122, 1.000000000000000000, 0.9659258262890683122, 1.000000000000000000, 0.9659258262890683122, 1.000000000000000000, 0.9659258262890683122, 1.000000000000000000, 0.9659258262890683122, 1.000000000000000000, 0.9659258262890683122, 1.000000000000000000, 0.9659258262890683122, 1.000000000000000000, 0.9659258262890683122, 1.000000000000000000, 0.9659258262890683122, 1.000000000000000000, 0.9659258262890683122, 1.000000000000000000, 0.9659258262890683122, 1.000000000000000000, 0.9659258262890683122, 1.000000000000000000, 0.9659258262890683122, 1.000000000000000000, 0.9659258262890683122, 1.000000000000000000, 0.9659258262890683122, 1.000000000000000000, 0.9659258262890683122, 1.000000000000000000, 0.9659258262890683122, 1.000000000000000000, 0.9659258262890683122, 1.000000000000000000, 0.9659258262890683122, 1.000000000000000000, 0.9659258262890683122, 1.000000000000000000, 0.9659258262890683122, 1.000000000000000000, 0.9659258262890683122, 1.000000000000000000, 0.9659258262890683122, 1.000000000000000000, 0.9659258262890683122, 1.000000000000000000, 0.9659258262890683122, 1.000000000000000000, 0.9659258262890683122, 1.000000000000000000, 0.9659258262890683122, 1.000000000000000000, 0.9659258262890683122, 1.000000000000000000, 0.9659258262890683122, 1.000000000000000000, 0.9659258262890683122, 1.000000000000000000, 0.9659258262890683122, 1.000000000000000000, 0.9659258262890683122, 1.000000000000000000, 0.9659258262890683122, 1.000000000000000000, 0.9659258262890683122, 1.000000000000000000, 0.9659258262890683122, 1.000000000000000000, 0.9659258262890683122, 1.000000000000000000, 0.9659258262890683122, 1.000000000000000000, 0.9659258262890683122, 1.000000000000000000, 0.9659258262890683122, 1.000000000000000000, 0.9659258262890683122, 1.000000000000000000, 0.9659258262890683122, 1.000000000000000000, 0.9659258262890683122, 1.000000000000000000, 0.9659258262890683122, 1.000000000000000000, 0.9659258262890683122, 1.000000000000000000, 0.9659258262890683122, 1.000000000000000000, 0.9659258262890683122, 1.000000000000000000, 0.9659258262890683122, 1.000000000000000000, 0.9659258262890683122, 1.000000000000000000, 0.9659258262890683122, 1.000000000000000000, 0.9659258262890683122, 1.000000000000000000, 0.9659258262890683122, 1.000000000000000000, 0.9659258262890683122, 1.000000000000000000, 0.9659258262890683122, 1.000000000000000000, 0.9659258262890683122, 1.000000000000000000, 0.9659258262890683122, 1.000000000000000000, 0.9659258262890683122, 1.000000000000000000, 0.9659258262890683122, 1.000000000000000000, 0.9659258262890683122, 1.000000000000000000, 0.9659258262890683122, 1.000000000000000000, 0.9659258262890683122, 1.000000000000000000, 0.9659258262890683122, 1.000000000000000000, 0.9659258262890683122, 1.000000000000000000, 0.9659258262890683122, 1.000000000000000000, 0.9659258262890683122, 1.000000000000000000, 0.9659258262890683122, 1.000000000000000000, 0.9659258262890683122, 1.000000000000000000, 0.9659258262890683122, 1.000000000000000000, 0.9659258262890683122, 1.000000000000000000, 0.9659258262890683122, 1.000000000000000000, 0.9659258262890683122, 1.000000000000000000, 0.9659258262890683122, 1.000000000000000000, 0.9659258262890683122, 1.000000000000000000, 0.9659258262890683122, 1.000000000000000000, 0.9659258262890683122, 1.000000000000000000, 0.9659258262890683122, 1.000000000000000000, 0.9659258262890683122, 1.000000000000000000, 0.9659258262890683122, 1.000000000000000000, 0.9659258262890683122, 1.000000000000000000, 0.9659258262890683122, 1.000000000000000000, 0.9659258262890683122, 1.000000000000000000, 0.9659258262890683122, 1.000000000000000000, 0.9659258262890683122, 1.000000000000000000, 0.9659258262890683122, 1.000000000000000000, 0.9659258262890683122, 1.000000000000000000, 0.9659258262890683122, 1.000000000000000000, 0.9659258262890683122, 1.000000000000000000, 0.9659258262890683122, 1.000000000000000000, 0.9659258262890683122, 1.000000000000000000) ) ) 
 REPRESENTATION_ITEM ( '' )  SURFACE ( )  );
#28474=CARTESIAN_POINT ( 'NONE',  ( 5.049401038298161559, -19.05341960407611168, 22.70724293864769194 ) ) ;
#28476=CARTESIAN_POINT ( 'NONE',  ( -16.51473224551082808, 9.474510206698731452, 68.33442372801900433 ) ) ;
#28477=CARTESIAN_POINT ( 'NONE',  ( 0.05219959533910956823, 16.53943276465976808, 54.99890960531435269 ) ) ;
#28478=CARTESIAN_POINT ( 'NONE',  ( -21.52544592524343514, 5.823673210054127303, 31.04057627198102409 ) ) ;
#28479=CARTESIAN_POINT ( 'NONE',  ( 10.72451020669871369, 18.67979575497193778, 92.08442372801901854 ) ) ;
#28480=CARTESIAN_POINT ( 'NONE',  ( -10.72451020669898014, 18.67979575497178502, 90.41557627198103830 ) ) ;
#28481=CARTESIAN_POINT ( 'NONE',  ( 10.81492255796106328, -18.62759615963255655, 60.41775706135235424 ) ) ;
#28482=CARTESIAN_POINT ( 'NONE',  ( -0.05219959533937732626, 21.53943276465977519, 67.50109039468568994 ) ) ;
#28483=CARTESIAN_POINT ( 'NONE',  ( -13.89961937509977652, 13.97604488694528158, 100.6239096053143669 ) ) ;
#28484=CARTESIAN_POINT ( 'NONE',  ( -4.379528057220086978, -16.55341960407618274, 94.79275706135234714 ) ) ;
#28485=CARTESIAN_POINT ( 'NONE',  ( -21.55341960407619339, 5.719274019375674811, 63.54275706135234003 ) ) ;
#28486=CARTESIAN_POINT ( 'NONE',  ( -16.52544592524342804, 4.483927247898546575, 116.0405762719810383 ) ) ;
#28487=CARTESIAN_POINT ( 'NONE',  ( 14.29746914071049879, -8.314922557960816363, 68.33224293864769550 ) ) ;
#28488=CARTESIAN_POINT ( 'NONE',  ( -16.52544592524342804, 4.483927247898546575, 36.04057627198102409 ) ) ;
#28489=CARTESIAN_POINT ( 'NONE',  ( 10.81492255796078972, 18.62759615963270932, 49.58224293864769550 ) ) ;
#28490=CARTESIAN_POINT ( 'NONE',  ( 9.564922557960805705, 16.46253265017160317, 44.58224293864769550 ) ) ;
#28491=CARTESIAN_POINT ( 'NONE',  ( 10.81492255796078972, 18.62759615963270932, 64.58224293864769550 ) ) ;
#28492=CARTESIAN_POINT ( 'NONE',  ( -16.46253265017146816, -9.564922557961047289, 54.16775706135234003 ) ) ;
#28494=CARTESIAN_POINT ( 'NONE',  ( 16.55341960407611168, 4.379528057220329451, 43.95724293864769550 ) ) ;
#28495=CARTESIAN_POINT ( 'NONE',  ( 0.05219959533907565091, 21.53943276465977519, 24.99890960531435624 ) ) ;
#28499=CARTESIAN_POINT ( 'NONE',  ( 14.29746914071037800, 8.314922557961029526, 76.66775706135234714 ) ) ;
#28500=CARTESIAN_POINT ( 'NONE',  ( 13.89961937509957401, 13.97604488694547697, 81.87609039468564731 ) ) ;
#28501=CARTESIAN_POINT ( 'NONE',  ( -14.29746914071049879, 8.314922557960819915, 45.83224293864769550 ) ) ;
#28502=CARTESIAN_POINT ( 'NONE',  ( 17.50000000000002487, -5.499999999999880984, 53.29690382534172244 ) ) ;
#28503=CARTESIAN_POINT ( 'NONE',  ( -4.483927247898539470, -16.52544592524342804, 27.29057627198103120 ) ) ;
#28504=CARTESIAN_POINT ( 'NONE',  ( -19.05341960407611168, -5.049401038298163336, 46.45724293864768129 ) ) ;
#28505=CARTESIAN_POINT ( 'NONE',  ( -16.46253265017160317, 9.564922557960807481, 70.83224293864770971 ) ) ;
#28506=CARTESIAN_POINT ( 'NONE',  ( -5.049401038298153566, 19.05341960407611168, 45.20724293864769550 ) ) ;
#28507=CARTESIAN_POINT ( 'NONE',  ( -15.80617190586768217, 15.72974639402176855, 48.12609039468568284 ) ) ;
#28508=CARTESIAN_POINT ( 'NONE',  ( -9.474510206698964154, 16.51473224551069663, 60.41557627198102409 ) ) ;
#28510=CARTESIAN_POINT ( 'NONE',  ( -19.03943276465977164, 0.05219959533909376836, 61.24890960531436690 ) ) ;
#28511=CARTESIAN_POINT ( 'NONE',  ( -18.67979575497178146, -10.72451020669898902, 36.66557627198103120 ) ) ;
#28512=CARTESIAN_POINT ( 'NONE',  ( -19.05341960407611168, -5.049401038298163336, 36.45724293864766707 ) ) ;
#28513=CARTESIAN_POINT ( 'NONE',  ( 18.67979575497178502, 10.72451020669898547, 39.16557627198102409 ) ) ;
#28514=CARTESIAN_POINT ( 'NONE',  ( -8.224510206698735004, -14.34966873604973081, 89.58442372801901854 ) ) ;
#28515=CARTESIAN_POINT ( 'NONE',  ( -16.51473224551082808, 9.474510206698731452, 23.33442372801900078 ) ) ;
#28516=CARTESIAN_POINT ( 'NONE',  ( -16.52544592524335698, -4.483927247898792601, 68.95942372801901854 ) ) ;
#28517=CARTESIAN_POINT ( 'NONE',  ( 5.049401038298161559, -19.05341960407611168, 102.7072429386476955 ) ) ;
#28518=CARTESIAN_POINT ( 'NONE',  ( -14.34966873604972548, 8.224510206698743886, 58.33442372801901143 ) ) ;
#28519=CARTESIAN_POINT ( 'NONE',  ( -4.379528057220086978, -16.55341960407618274, 34.79275706135235424 ) ) ;
#28520=CARTESIAN_POINT ( 'NONE',  ( 19.03943276465977164, -0.05219959533909143690, 103.7489096053143669 ) ) ;
#28521=CARTESIAN_POINT ( 'NONE',  ( 16.52544592524335698, 4.483927247898782831, 21.45942372801901499 ) ) ;
#28522=CARTESIAN_POINT ( 'NONE',  ( 19.02544592524343514, -5.153800228976328945, 33.54057627198102409 ) ) ;
#28523=CARTESIAN_POINT ( 'NONE',  ( -18.67979575497193778, 10.72451020669871902, 23.33442372801901499 ) ) ;
#28524=CARTESIAN_POINT ( 'NONE',  ( 12.06949235617739724, 12.14591786802326823, 26.87609039468567218 ) ) ;
#28525=CARTESIAN_POINT ( 'NONE',  ( 16.55341960407618274, -4.379528057220086978, 106.0427570613523471 ) ) ;
#28527=CARTESIAN_POINT ( 'NONE',  ( -15.72974639402176322, -15.80617190586768395, 104.3760903946856899 ) ) ;
#28528=CARTESIAN_POINT ( 'NONE',  ( 19.02544592524334988, 5.153800228976608722, 91.45942372801900433 ) ) ;
#28529=CARTESIAN_POINT ( 'NONE',  ( 12.14591786802309770, 12.06949235617756955, 54.37390960531435979 ) ) ;
#28530=CARTESIAN_POINT ( 'NONE',  ( -12.06949235617756955, 12.14591786802309770, 115.6239096053143669 ) ) ;
#28531=CARTESIAN_POINT ( 'NONE',  ( -13.89961937509957401, -13.97604488694547875, 49.37609039468567573 ) ) ;
#28533=CARTESIAN_POINT ( 'NONE',  ( 21.53943276465977519, 0.05219959533937863772, 46.25109039468567573 ) ) ;
#28534=CARTESIAN_POINT ( 'NONE',  ( -16.53943276465976808, -0.05219959533934237506, 23.75109039468567929 ) ) ;
#28535=CARTESIAN_POINT ( 'NONE',  ( 17.49999999999999645, 5.624438216177598981, 81.68329655085356933 ) ) ;
#28536=CARTESIAN_POINT ( 'NONE',  ( 13.97604488694527802, 13.89961937509977652, 104.3739096053143385 ) ) ;
#28537=CARTESIAN_POINT ( 'NONE',  ( -18.62759615963270932, 10.81492255796079327, 75.83224293864769550 ) ) ;
#28538=CARTESIAN_POINT ( 'NONE',  ( -13.89961937509957401, -13.97604488694547875, 104.3760903946856757 ) ) ;
#28539=CARTESIAN_POINT ( 'NONE',  ( -19.03943276465977164, 0.05219959533909376836, 101.2489096053143669 ) ) ;
#28541=CARTESIAN_POINT ( 'NONE',  ( -16.52544592524342804, 4.483927247898546575, 111.0405762719810525 ) ) ;
#28542=CARTESIAN_POINT ( 'NONE',  ( -15.80617190586768217, 15.72974639402176855, 98.12609039468570415 ) ) ;
#28543=CARTESIAN_POINT ( 'NONE',  ( -9.474510206698964154, 16.51473224551069663, 40.41557627198103120 ) ) ;
#28544=CARTESIAN_POINT ( 'NONE',  ( 5.719274019375673035, 21.55341960407619339, 52.29275706135236135 ) ) ;
#28545=CARTESIAN_POINT ( 'NONE',  ( -21.52544592524334988, -5.823673210054445271, 88.95942372801901854 ) ) ;
#28546=CARTESIAN_POINT ( 'NONE',  ( -16.55341960407617563, 4.379528057220093196, 103.5427570613523613 ) ) ;
#28547=CARTESIAN_POINT ( 'NONE',  ( -19.03943276465977164, 0.05219959533909376836, 76.24890960531435269 ) ) ;
#28548=CARTESIAN_POINT ( 'NONE',  ( -21.52544592524334988, -5.823673210054445271, 43.95942372801902565 ) ) ;
#28549=CARTESIAN_POINT ( 'NONE',  ( -5.719274019375665041, -21.55341960407619695, 44.79275706135234714 ) ) ;
#28550=CARTESIAN_POINT ( 'NONE',  ( -13.89961937509957401, -13.97604488694547875, 64.37609039468567573 ) ) ;
#28551=CARTESIAN_POINT ( 'NONE',  ( -19.02544592524342804, 5.153800228976336051, 86.04057627198103830 ) ) ;
#28552=CARTESIAN_POINT ( 'NONE',  ( -12.14591786802309592, -12.06949235617757132, 101.8739096053143811 ) ) ;
#28553=CARTESIAN_POINT ( 'NONE',  ( -0.05219959533907301413, -21.53943276465977519, 92.49890960531436690 ) ) ;
#28554=CARTESIAN_POINT ( 'NONE',  ( -0.05219959533910754901, -16.53943276465976808, 67.49890960531436690 ) ) ;
#28555=CARTESIAN_POINT ( 'NONE',  ( -16.46253265017146816, -9.564922557961047289, 24.16775706135233648 ) ) ;
#28556=CARTESIAN_POINT ( 'NONE',  ( -4.379528057220328563, 16.55341960407611168, 90.20724293864770971 ) ) ;
#28557=CARTESIAN_POINT ( 'NONE',  ( -0.05219959533909027116, -19.03943276465977164, 37.49890960531436690 ) ) ;
#28558=CARTESIAN_POINT ( 'NONE',  ( 16.51473224551083163, -9.474510206698727899, 85.83442372801900433 ) ) ;
#28559=CARTESIAN_POINT ( 'NONE',  ( -4.379528057220328563, 16.55341960407611168, 55.20724293864770260 ) ) ;
#28560=CARTESIAN_POINT ( 'NONE',  ( 10.72451020669871369, 18.67979575497193778, 97.08442372801904696 ) ) ;
#28561=CARTESIAN_POINT ( 'NONE',  ( -19.03943276465977164, 0.05219959533909376836, 101.2489096053143669 ) ) ;
#28562=CARTESIAN_POINT ( 'NONE',  ( -13.97604488694547697, 13.89961937509957934, 78.12609039468567573 ) ) ;
#28563=CARTESIAN_POINT ( 'NONE',  ( -21.52544592524343514, 5.823673210054127303, 81.04057627198102409 ) ) ;
#28564=CARTESIAN_POINT ( 'NONE',  ( 5.823673210054444382, -21.52544592524334988, 30.20942372801902565 ) ) ;
#28565=CARTESIAN_POINT ( 'NONE',  ( -4.483927247898782831, 16.52544592524335698, 32.70942372801900433 ) ) ;
#28566=CARTESIAN_POINT ( 'NONE',  ( 0.05219959533934541429, -16.53943276465976808, 90.00109039468567573 ) ) ;
#28567=CARTESIAN_POINT ( 'NONE',  ( -19.03943276465977164, 0.05219959533909376836, 26.24890960531435624 ) ) ;
#28568=CARTESIAN_POINT ( 'NONE',  ( 21.55341960407619695, -5.719274019375665929, 36.04275706135234714 ) ) ;
#28569=CARTESIAN_POINT ( 'NONE',  ( -16.52544592524342804, 4.483927247898546575, 116.0405762719810383 ) ) ;
#28571=CARTESIAN_POINT ( 'NONE',  ( 14.29746914071037800, 8.314922557961029526, 46.66775706135234714 ) ) ;
#28573=CARTESIAN_POINT ( 'NONE',  ( -16.53943276465976808, 0.05219959533911058130, 76.24890960531435269 ) ) ;
#28574=CARTESIAN_POINT ( 'NONE',  ( -10.72451020669898014, 18.67979575497178502, 70.41557627198102409 ) ) ;
#28575=CARTESIAN_POINT ( 'NONE',  ( 4.379528057220339221, -16.55341960407611168, 27.70724293864769905 ) ) ;
#28576=CARTESIAN_POINT ( 'NONE',  ( 14.34966873604972726, -8.224510206698740333, 55.83442372801901854 ) ) ;
#28577=CARTESIAN_POINT ( 'NONE',  ( 5.153800228976335163, 19.02544592524342804, 49.79057627198100988 ) ) ;
#28578=CARTESIAN_POINT ( 'NONE',  ( -16.52544592524335698, -4.483927247898792601, 88.95942372801901854 ) ) ;
#28579=CARTESIAN_POINT ( 'NONE',  ( 19.02544592524334988, 5.153800228976608722, 86.45942372801900433 ) ) ;
#28580=CARTESIAN_POINT ( 'NONE',  ( 5.823673210054125526, 21.52544592524343514, 74.79057627198105251 ) ) ;
#28581=CARTESIAN_POINT ( 'NONE',  ( -4.483927247898782831, 16.52544592524335698, 112.7094237280190328 ) ) ;
#28584=CARTESIAN_POINT ( 'NONE',  ( -15.72974639402197994, 15.80617190586746368, 65.62390960531436690 ) ) ;
#28586=CARTESIAN_POINT ( 'NONE',  ( -4.379528057220086978, -16.55341960407618274, 94.79275706135234714 ) ) ;
#28588=CARTESIAN_POINT ( 'NONE',  ( -16.46253265017160317, 9.564922557960807481, 110.8322429386476955 ) ) ;
#28589=CARTESIAN_POINT ( 'NONE',  ( 5.823673210054125526, 21.52544592524343514, 74.79057627198105251 ) ) ;
#28590=CARTESIAN_POINT ( 'NONE',  ( 14.34966873604960469, 8.224510206698951720, 24.16557627198103120 ) ) ;
#28591=CARTESIAN_POINT ( 'NONE',  ( -16.53943276465976808, -0.05219959533934237506, 23.75109039468567929 ) ) ;
#28592=CARTESIAN_POINT ( 'NONE',  ( -19.05341960407611168, -5.049401038298163336, 21.45724293864768839 ) ) ;
#28593=CARTESIAN_POINT ( 'NONE',  ( -16.53943276465976808, -0.05219959533934237506, 33.75109039468568284 ) ) ;
#28594=CARTESIAN_POINT ( 'NONE',  ( -13.89961937509977652, 13.97604488694528158, 55.62390960531434558 ) ) ;
#28596=CARTESIAN_POINT ( 'NONE',  ( -5.049401038298153566, 19.05341960407611168, 100.2072429386476955 ) ) ;
#28597=CARTESIAN_POINT ( 'NONE',  ( 0.05219959533934541429, -16.53943276465976808, 95.00109039468568994 ) ) ;
#28598=CARTESIAN_POINT ( 'NONE',  ( 19.02544592524334988, 5.153800228976608722, 91.45942372801900433 ) ) ;
#28599=CARTESIAN_POINT ( 'NONE',  ( -13.97604488694547697, 13.89961937509957934, 28.12609039468565797 ) ) ;
#28600=CARTESIAN_POINT ( 'NONE',  ( -18.67979575497178146, -10.72451020669898902, 81.66557627198103830 ) ) ;
#28601=CARTESIAN_POINT ( 'NONE',  ( -14.29746914071037622, -8.314922557961029526, 94.16775706135237556 ) ) ;
#28602=CARTESIAN_POINT ( 'NONE',  ( 5.049401038297881783, 19.05341960407617563, 92.29275706135234714 ) ) ;
#28603=CARTESIAN_POINT ( 'NONE',  ( -13.89961937509977652, 13.97604488694528158, 55.62390960531434558 ) ) ;
#28604=CARTESIAN_POINT ( 'NONE',  ( -19.03943276465977164, 0.05219959533909376836, 91.24890960531436690 ) ) ;
#28605=CARTESIAN_POINT ( 'NONE',  ( 10.72451020669871369, 18.67979575497193778, 57.08442372801901854 ) ) ;
#28606=CARTESIAN_POINT ( 'NONE',  ( -19.05341960407611168, -5.049401038298163336, 61.45724293864769550 ) ) ;
#28607=CARTESIAN_POINT ( 'NONE',  ( -16.53943276465976808, 0.05219959533911058130, 86.24890960531436690 ) ) ;
#28608=CARTESIAN_POINT ( 'NONE',  ( -17.31747979337950838, -6.344076630960981511, 86.37944868065183357 ) ) ;
#28609=CARTESIAN_POINT ( 'NONE',  ( 8.224510206698953496, -14.34966873604960469, 77.91557627198102409 ) ) ;
#28610=CARTESIAN_POINT ( 'NONE',  ( 21.53943276465977519, -0.05219959533907433946, 73.74890960531433848 ) ) ;
#28611=CARTESIAN_POINT ( 'NONE',  ( -16.51473224551082808, 9.474510206698731452, 93.33442372801900433 ) ) ;
#28612=CARTESIAN_POINT ( 'NONE',  ( 16.79531203550648044, -7.028104445595602989, 81.24755011779561187 ) ) ;
#28613=CARTESIAN_POINT ( 'NONE',  ( 16.46253265017146816, 9.564922557961045513, 41.66775706135234003 ) ) ;
#28616=CARTESIAN_POINT ( 'NONE',  ( 19.03943276465977164, -0.05219959533909143690, 83.74890960531436690 ) ) ;
#28617=CARTESIAN_POINT ( 'NONE',  ( 13.89961937509977652, -13.97604488694527269, 93.12390960531436690 ) ) ;
#28618=CARTESIAN_POINT ( 'NONE',  ( -16.53943276465976808, -0.05219959533934237506, 63.75109039468568284 ) ) ;
#28620=CARTESIAN_POINT ( 'NONE',  ( 19.05341960407617918, -5.049401038297876454, 46.04275706135233293 ) ) ;
#28622=CARTESIAN_POINT ( 'NONE',  ( 0.05219959533909260263, 19.03943276465977164, 109.9989096053143669 ) ) ;
#28623=CARTESIAN_POINT ( 'NONE',  ( -16.53943276465976808, -0.05219959533934237506, 108.7510903946857042 ) ) ;
#28625=CARTESIAN_POINT ( 'NONE',  ( -8.224510206698735004, -14.34966873604973081, 74.58442372801901854 ) ) ;
#28626=CARTESIAN_POINT ( 'NONE',  ( -16.20579543436675252, 7.371946100355233789, 29.43479165828123101 ) ) ;
#28627=CARTESIAN_POINT ( 'NONE',  ( 16.55341960407618274, -4.379528057220086978, 51.04275706135234714 ) ) ;
#28628=CARTESIAN_POINT ( 'NONE',  ( 0.05219959533909260263, 19.03943276465977164, 74.99890960531435269 ) ) ;
#28629=CARTESIAN_POINT ( 'NONE',  ( 21.53943276465977519, 0.05219959533937863772, 66.25109039468567573 ) ) ;
#28630=CARTESIAN_POINT ( 'NONE',  ( -16.46253265017146816, -9.564922557961047289, 69.16775706135233293 ) ) ;
#28631=CARTESIAN_POINT ( 'NONE',  ( 19.05341960407617918, -5.049401038297876454, 26.04275706135233293 ) ) ;
#28632=CARTESIAN_POINT ( 'NONE',  ( -13.97604488694527625, -13.89961937509977652, 56.87390960531434558 ) ) ;
#28633=CARTESIAN_POINT ( 'NONE',  ( 19.03943276465977164, -0.05219959533909143690, 48.74890960531435979 ) ) ;
#28635=CARTESIAN_POINT ( 'NONE',  ( -18.62759615963270932, 10.81492255796079327, 65.83224293864769550 ) ) ;
#28636=CARTESIAN_POINT ( 'NONE',  ( -0.05219959533907301413, -21.53943276465977519, 32.49890960531435979 ) ) ;
#28637=CARTESIAN_POINT ( 'NONE',  ( -8.224510206698948167, 14.34966873604960824, 115.4155762719810241 ) ) ;
#28638=CARTESIAN_POINT ( 'NONE',  ( -14.34966873604972548, 8.224510206698743886, 48.33442372801902565 ) ) ;
#28641=CARTESIAN_POINT ( 'NONE',  ( 21.52544592524344225, -5.823673210054117533, 113.5405762719810383 ) ) ;
#28642=CARTESIAN_POINT ( 'NONE',  ( -14.34966873604960291, -8.224510206698953496, 51.66557627198102409 ) ) ;
#28644=CARTESIAN_POINT ( 'NONE',  ( -5.153800228976607833, 19.02544592524334988, 112.7094237280190043 ) ) ;
#28645=CARTESIAN_POINT ( 'NONE',  ( 19.03943276465977164, 0.05219959533936151252, 46.25109039468566863 ) ) ;
#28646=CARTESIAN_POINT ( 'NONE',  ( -8.314922557960811034, -14.29746914071050412, 42.08224293864769550 ) ) ;
#28647=CARTESIAN_POINT ( 'NONE',  ( 18.67979575497194134, -10.72451020669871369, 20.83442372801901143 ) ) ;
#28649=CARTESIAN_POINT ( 'NONE',  ( -15.72974639402197994, 15.80617190586746368, 70.62390960531436690 ) ) ;
#28650=CARTESIAN_POINT ( 'NONE',  ( -19.02544592524342804, 5.153800228976336051, 91.04057627198100988 ) ) ;
#28651=CARTESIAN_POINT ( 'NONE',  ( -8.224510206698948167, 14.34966873604960824, 65.41557627198102409 ) ) ;
#28652=CARTESIAN_POINT ( 'NONE',  ( 19.02544592524343514, -5.153800228976328945, 108.5405762719810383 ) ) ;
#28653=EDGE_CURVE ( 'NONE', #91449, #137808, #101042, .T. ) ;
#28654=CARTESIAN_POINT ( 'NONE',  ( -16.46253265017160317, 9.564922557960807481, 80.83224293864769550 ) ) ;
#28655=CARTESIAN_POINT ( 'NONE',  ( -13.89961937509957401, -13.97604488694547875, 49.37609039468567573 ) ) ;
#28656=CARTESIAN_POINT ( 'NONE',  ( 18.62759615963271287, -10.81492255796078972, 113.3322429386476955 ) ) ;
#28657=CARTESIAN_POINT ( 'NONE',  ( 5.153800228976335163, 19.02544592524342804, 39.79057627198100988 ) ) ;
#28658=CARTESIAN_POINT ( 'NONE',  ( -0.05219959533910754901, -16.53943276465976808, 112.4989096053143669 ) ) ;
#28659=CARTESIAN_POINT ( 'NONE',  ( -15.80617190586768217, 15.72974639402176855, 48.12609039468568284 ) ) ;
#28661=CARTESIAN_POINT ( 'NONE',  ( 8.224510206698953496, -14.34966873604960469, 22.91557627198102765 ) ) ;
#28662=CARTESIAN_POINT ( 'NONE',  ( 13.97604488694527802, 13.89961937509977652, 44.37390960531435269 ) ) ;
#28663=CARTESIAN_POINT ( 'NONE',  ( 9.564922557960805705, 16.46253265017160317, 94.58224293864769550 ) ) ;
#28664=CARTESIAN_POINT ( 'NONE',  ( 0.05219959533907565091, 21.53943276465977519, 74.99890960531435269 ) ) ;
#28666=CARTESIAN_POINT ( 'NONE',  ( 16.51473224551069308, 9.474510206698969483, 49.16557627198102409 ) ) ;
#28667=CARTESIAN_POINT ( 'NONE',  ( -21.52544592524343514, 5.823673210054127303, 56.04057627198102409 ) ) ;
#28668=CARTESIAN_POINT ( 'NONE',  ( 15.72974639402176855, 15.80617190586768217, 81.87609039468568994 ) ) ;
#28669=CARTESIAN_POINT ( 'NONE',  ( 17.97214573761831957, 5.500000000000083489, 53.96970049038659312 ) ) ;
#28670=CARTESIAN_POINT ( 'NONE',  ( -0.05219959533934338120, 16.53943276465976808, 82.50109039468568994 ) ) ;
#28671=CARTESIAN_POINT ( 'NONE',  ( 14.34966873604960469, 8.224510206698951720, 64.16557627198102409 ) ) ;
#28672=CARTESIAN_POINT ( 'NONE',  ( -19.02544592524342804, 5.153800228976336051, 76.04057627198102409 ) ) ;
#28674=CARTESIAN_POINT ( 'NONE',  ( 5.049401038297881783, 19.05341960407617563, 27.29275706135232937 ) ) ;
#28675=CARTESIAN_POINT ( 'NONE',  ( 12.06949235617739724, 12.14591786802326823, 91.87609039468568994 ) ) ;
#28676=CARTESIAN_POINT ( 'NONE',  ( -9.564922557961040184, 16.46253265017147172, 22.91775706135233648 ) ) ;
#28677=CARTESIAN_POINT ( 'NONE',  ( -13.89961937509977652, 13.97604488694528158, 80.62390960531436690 ) ) ;
#28678=CARTESIAN_POINT ( 'NONE',  ( -5.823673210054116645, -21.52544592524344225, 42.29057627198103120 ) ) ;
#28679=CARTESIAN_POINT ( 'NONE',  ( -16.52544592524335698, -4.483927247898792601, 23.95942372801901143 ) ) ;
#28680=CARTESIAN_POINT ( 'NONE',  ( 18.62759615963255655, 10.81492255796105972, 96.66775706135234714 ) ) ;
#28681=CARTESIAN_POINT ( 'NONE',  ( 16.53943276465976808, 0.05219959533934440121, 66.25109039468567573 ) ) ;
#28682=CARTESIAN_POINT ( 'NONE',  ( -10.72451020669898014, 18.67979575497178502, 110.4155762719810383 ) ) ;
#28683=CARTESIAN_POINT ( 'NONE',  ( -14.29746914071037622, -8.314922557961029526, 19.16775706135234714 ) ) ;
#28684=CARTESIAN_POINT ( 'NONE',  ( -16.46253265017160317, 9.564922557960807481, 90.83224293864769550 ) ) ;
#28685=CARTESIAN_POINT ( 'NONE',  ( -0.05219959533934338120, 16.53943276465976808, 22.50109039468567573 ) ) ;
#28686=CARTESIAN_POINT ( 'NONE',  ( 19.02544592524343514, -5.153800228976328945, 48.54057627198103120 ) ) ;
#28687=CARTESIAN_POINT ( 'NONE',  ( -4.379528057220086978, -16.55341960407618274, 34.79275706135235424 ) ) ;
#28688=CARTESIAN_POINT ( 'NONE',  ( 16.53943276465976808, -0.05219959533910856209, 78.74890960531436690 ) ) ;
#28689=CARTESIAN_POINT ( 'NONE',  ( 12.06949235617739724, 12.14591786802326823, 91.87609039468568994 ) ) ;
#28690=CARTESIAN_POINT ( 'NONE',  ( 21.53943276465977519, 0.05219959533937863772, 31.25109039468568639 ) ) ;
#28691=CARTESIAN_POINT ( 'NONE',  ( 9.474510206698971260, -16.51473224551069308, 67.91557627198102409 ) ) ;
#28692=CARTESIAN_POINT ( 'NONE',  ( -9.474510206698964154, 16.51473224551069663, 80.41557627198103830 ) ) ;
#28693=CARTESIAN_POINT ( 'NONE',  ( 16.52544592524335698, 4.483927247898782831, 81.45942372801900433 ) ) ;
#28696=ORIENTED_EDGE ( 'NONE', *, *, #136135, .F. ) ;
#28697=CARTESIAN_POINT ( 'NONE',  ( -5.049401038297874678, -19.05341960407617918, 34.79275706135233293 ) ) ;
#28698=CARTESIAN_POINT ( 'NONE',  ( 16.51473224551069308, 9.474510206698969483, 104.1655762719810241 ) ) ;
#28699=CARTESIAN_POINT ( 'NONE',  ( -9.564922557960796823, -16.46253265017161027, 47.08224293864769550 ) ) ;
#28701=CARTESIAN_POINT ( 'NONE',  ( 14.29746914071037800, 8.314922557961029526, 36.66775706135234714 ) ) ;
#28702=CARTESIAN_POINT ( 'NONE',  ( 5.049401038297881783, 19.05341960407617563, 57.29275706135231871 ) ) ;
#28703=CARTESIAN_POINT ( 'NONE',  ( -8.314922557961024197, 14.29746914071037800, 47.91775706135234714 ) ) ;
#28704=CARTESIAN_POINT ( 'NONE',  ( 19.02544592524343514, -5.153800228976328945, 103.5405762719809957 ) ) ;
#28705=CARTESIAN_POINT ( 'NONE',  ( -5.049401038298153566, 19.05341960407611168, 75.20724293864769550 ) ) ;
#28706=CARTESIAN_POINT ( 'NONE',  ( -0.05219959533907301413, -21.53943276465977519, 97.49890960531436690 ) ) ;
#28707=CARTESIAN_POINT ( 'NONE',  ( 19.03943276465977164, 0.05219959533936151252, 66.25109039468567573 ) ) ;
#28708=CARTESIAN_POINT ( 'NONE',  ( -5.153800228976328057, -19.02544592524343514, 87.29057627198103830 ) ) ;
#28709=CARTESIAN_POINT ( 'NONE',  ( 17.43360820948602097, -4.799606864746338353, 21.47765276293580428 ) ) ;
#28710=CARTESIAN_POINT ( 'NONE',  ( 13.89961937509977652, -13.97604488694527269, 63.12390960531435979 ) ) ;
#28711=CARTESIAN_POINT ( 'NONE',  ( -16.52544592524342804, 4.483927247898546575, 36.04057627198102409 ) ) ;
#28712=CARTESIAN_POINT ( 'NONE',  ( -9.474510206698964154, 16.51473224551069663, 70.41557627198102409 ) ) ;
#28713=CARTESIAN_POINT ( 'NONE',  ( 13.97604488694548053, -13.89961937509957401, 40.62609039468564731 ) ) ;
#28714=CARTESIAN_POINT ( 'NONE',  ( 4.379528057220339221, -16.55341960407611168, 77.70724293864770971 ) ) ;
#28715=CARTESIAN_POINT ( 'NONE',  ( -15.80617190586768217, 15.72974639402176855, 103.1260903946856757 ) ) ;
#28716=CARTESIAN_POINT ( 'NONE',  ( -16.46253265017160317, 9.564922557960807481, 35.83224293864768839 ) ) ;
#28717=CARTESIAN_POINT ( 'NONE',  ( 12.14591786802327356, -12.06949235617739191, 55.62609039468568284 ) ) ;
#28718=CARTESIAN_POINT ( 'NONE',  ( 16.53943276465976808, -0.05219959533910856209, 33.74890960531436690 ) ) ;
#28719=CARTESIAN_POINT ( 'NONE',  ( -10.81492255796105439, 18.62759615963255655, 107.9177570613523471 ) ) ;
#28720=CARTESIAN_POINT ( 'NONE',  ( -5.049401038298153566, 19.05341960407611168, 90.20724293864766707 ) ) ;
#28721=CARTESIAN_POINT ( 'NONE',  ( 9.564922557960805705, 16.46253265017160317, 94.58224293864769550 ) ) ;
#28722=CARTESIAN_POINT ( 'NONE',  ( 9.474510206698971260, -16.51473224551069308, 22.91557627198102765 ) ) ;
#28723=CARTESIAN_POINT ( 'NONE',  ( -16.55341960407611168, -4.379528057220339221, 111.4572429386476813 ) ) ;
#28724=CARTESIAN_POINT ( 'NONE',  ( -4.483927247898539470, -16.52544592524342804, 77.29057627198102409 ) ) ;
#28725=CARTESIAN_POINT ( 'NONE',  ( -10.72451020669898014, 18.67979575497178502, 85.41557627198102409 ) ) ;
#28726=CARTESIAN_POINT ( 'NONE',  ( 16.46253265017160672, -9.564922557960803928, 88.33224293864769550 ) ) ;
#28727=CARTESIAN_POINT ( 'NONE',  ( -21.55341960407610458, -5.719274019375992779, 101.4572429386476955 ) ) ;
#28728=CARTESIAN_POINT ( 'NONE',  ( 5.049401038298161559, -19.05341960407611168, 92.70724293864769550 ) ) ;
#28729=CARTESIAN_POINT ( 'NONE',  ( 18.22780087662122384, -5.500000000000022204, 46.01540105326107266 ) ) ;
#28730=CARTESIAN_POINT ( 'NONE',  ( -8.224510206698948167, 14.34966873604960824, 95.41557627198102409 ) ) ;
#28731=CARTESIAN_POINT ( 'NONE',  ( 16.46253265017160672, -9.564922557960803928, 58.33224293864769550 ) ) ;
#28732=CARTESIAN_POINT ( 'NONE',  ( -18.62759615963270932, 10.81492255796079327, 60.83224293864769550 ) ) ;
#28734=CARTESIAN_POINT ( 'NONE',  ( 16.52544592524335698, 4.483927247898782831, 111.4594237280190328 ) ) ;
#28736=CARTESIAN_POINT ( 'NONE',  ( -8.314922557961024197, 14.29746914071037800, 22.91775706135235069 ) ) ;
#28737=CARTESIAN_POINT ( 'NONE',  ( 4.379528057220339221, -16.55341960407611168, 92.70724293864770971 ) ) ;
#28738=CARTESIAN_POINT ( 'NONE',  ( 19.26498983726236247, -5.499999999999801936, 53.05319577422001487 ) ) ;
#28739=CARTESIAN_POINT ( 'NONE',  ( 9.474510206698971260, -16.51473224551069308, 82.91557627198103830 ) ) ;
#28740=CARTESIAN_POINT ( 'NONE',  ( 9.474510206698971260, -16.51473224551069308, 47.91557627198102409 ) ) ;
#28741=CARTESIAN_POINT ( 'NONE',  ( -16.55341960407611168, -4.379528057220339221, 61.45724293864770260 ) ) ;
#28743=CARTESIAN_POINT ( 'NONE',  ( 19.02544592524343514, -5.153800228976328945, 108.5405762719810383 ) ) ;
#28744=CARTESIAN_POINT ( 'NONE',  ( -9.564922557961040184, 16.46253265017147172, 102.9177570613523329 ) ) ;
#28745=CARTESIAN_POINT ( 'NONE',  ( 5.823673210054444382, -21.52544592524334988, 60.20942372801902565 ) ) ;
#28746=CARTESIAN_POINT ( 'NONE',  ( 16.46253265017160672, -9.564922557960803928, 103.3322429386476955 ) ) ;
#28747=CARTESIAN_POINT ( 'NONE',  ( 18.62759615963271287, -10.81492255796078972, 78.33224293864770971 ) ) ;
#28748=CARTESIAN_POINT ( 'NONE',  ( -4.379528057220086978, -16.55341960407618274, 64.79275706135234714 ) ) ;
#28749=CARTESIAN_POINT ( 'NONE',  ( -5.049401038298153566, 19.05341960407611168, 30.20724293864768839 ) ) ;
#28750=CARTESIAN_POINT ( 'NONE',  ( 19.02544592524343514, -5.153800228976328945, 78.54057627198099567 ) ) ;
#28751=CARTESIAN_POINT ( 'NONE',  ( -18.67979575497178146, -10.72451020669898902, 76.66557627198103830 ) ) ;
#28752=CARTESIAN_POINT ( 'NONE',  ( -14.29746914071037622, -8.314922557961029526, 19.16775706135234714 ) ) ;
#28753=CARTESIAN_POINT ( 'NONE',  ( 12.06949235617757843, -12.14591786802309237, 38.12390960531436690 ) ) ;
#28754=CARTESIAN_POINT ( 'NONE',  ( -0.05219959533937732626, 21.53943276465977519, 57.50109039468568994 ) ) ;
#28755=CARTESIAN_POINT ( 'NONE',  ( -16.55341960407617563, 4.379528057220093196, 88.54275706135236135 ) ) ;
#28756=CARTESIAN_POINT ( 'NONE',  ( 0.05219959533907565091, 21.53943276465977519, 24.99890960531435624 ) ) ;
#28757=CARTESIAN_POINT ( 'NONE',  ( -19.02544592524342804, 5.153800228976336939, 106.0405762719810383 ) ) ;
#28759=CARTESIAN_POINT ( 'NONE',  ( -12.14591786802326823, 12.06949235617739902, 113.1260903946856899 ) ) ;
#28760=CARTESIAN_POINT ( 'NONE',  ( -12.14591786802326823, 12.06949235617739902, 43.12609039468568284 ) ) ;
#28761=CARTESIAN_POINT ( 'NONE',  ( 13.97604488694527802, 13.89961937509977652, 59.37390960531434558 ) ) ;
#28762=CARTESIAN_POINT ( 'NONE',  ( 9.474510206698971260, -16.51473224551069308, 67.91557627198102409 ) ) ;
#28763=CARTESIAN_POINT ( 'NONE',  ( 12.06949235617739724, 12.14591786802326823, 56.87609039468568994 ) ) ;
#28764=CARTESIAN_POINT ( 'NONE',  ( -14.34966873604960291, -8.224510206698953496, 51.66557627198102409 ) ) ;
#28765=CARTESIAN_POINT ( 'NONE',  ( 19.03943276465977164, -0.05219959533909143690, 53.74890960531436690 ) ) ;
#28766=CARTESIAN_POINT ( 'NONE',  ( -19.03943276465977164, 0.05219959533909376836, 46.24890960531435979 ) ) ;
#28767=CARTESIAN_POINT ( 'NONE',  ( 8.224510206698742110, 14.34966873604972548, 47.08442372801901854 ) ) ;
#28768=CARTESIAN_POINT ( 'NONE',  ( 19.05341960407617918, -5.049401038297876454, 96.04275706135231871 ) ) ;
#28769=CARTESIAN_POINT ( 'NONE',  ( 4.483927247898545687, 16.52544592524342804, 94.79057627198105251 ) ) ;
#28770=CARTESIAN_POINT ( 'NONE',  ( 0.05219959533909260263, 19.03943276465977164, 69.99890960531435269 ) ) ;
#28771=CARTESIAN_POINT ( 'NONE',  ( -19.02544592524334988, -5.153800228976617603, 98.95942372801900433 ) ) ;
#28773=CARTESIAN_POINT ( 'NONE',  ( 18.62759615963255655, 10.81492255796105972, 91.66775706135234714 ) ) ;
#28774=CARTESIAN_POINT ( 'NONE',  ( -16.52544592524335698, -4.483927247898792601, 73.95942372801901854 ) ) ;
#28775=CARTESIAN_POINT ( 'NONE',  ( -21.55341960407610458, -5.719274019375992779, 66.45724293864768129 ) ) ;
#28776=CARTESIAN_POINT ( 'NONE',  ( 4.483927247898790824, -16.52544592524335698, 50.20942372801901854 ) ) ;
#28777=CARTESIAN_POINT ( 'NONE',  ( 5.049401038298163336, -19.05341960407611168, 32.70724293864768839 ) ) ;
#28778=CARTESIAN_POINT ( 'NONE',  ( -16.51473224551082808, 9.474510206698731452, 43.33442372801900433 ) ) ;
#28779=CARTESIAN_POINT ( 'NONE',  ( 0.05219959533909260263, 19.03943276465977164, 94.99890960531436690 ) ) ;
#28780=CARTESIAN_POINT ( 'NONE',  ( -0.05219959533910754901, -16.53943276465976808, 112.4989096053143669 ) ) ;
#28781=CARTESIAN_POINT ( 'NONE',  ( 13.89961937509977652, -13.97604488694527269, 63.12390960531435979 ) ) ;
#28783=CARTESIAN_POINT ( 'NONE',  ( 18.67979575497194134, -10.72451020669871369, 80.83442372801901854 ) ) ;
#28785=CARTESIAN_POINT ( 'NONE',  ( 13.97604488694548053, -13.89961937509957401, 30.62609039468566863 ) ) ;
#28786=CARTESIAN_POINT ( 'NONE',  ( 19.05341960407617918, -5.049401038297876454, 31.04275706135232227 ) ) ;
#28787=CARTESIAN_POINT ( 'NONE',  ( -14.34966873604960291, -8.224510206698953496, 56.66557627198103830 ) ) ;
#28788=CARTESIAN_POINT ( 'NONE',  ( 9.474510206698971260, -16.51473224551069308, 62.91557627198102409 ) ) ;
#28789=CARTESIAN_POINT ( 'NONE',  ( 15.80617190586746368, 15.72974639402197994, 29.37390960531435269 ) ) ;
#28790=CARTESIAN_POINT ( 'NONE',  ( 10.81492255796106328, -18.62759615963255655, 80.41775706135234714 ) ) ;
#28791=CARTESIAN_POINT ( 'NONE',  ( 19.05341960407611168, 5.049401038298154454, 63.95724293864769550 ) ) ;
#28792=CARTESIAN_POINT ( 'NONE',  ( -5.719274019375665041, -21.55341960407619695, 79.79275706135236135 ) ) ;
#28793=CARTESIAN_POINT ( 'NONE',  ( -21.55341960407610458, -5.719274019375992779, 31.45724293864769550 ) ) ;
#28794=CARTESIAN_POINT ( 'NONE',  ( 13.89961937509977652, -13.97604488694527269, 73.12390960531436690 ) ) ;
#28795=CARTESIAN_POINT ( 'NONE',  ( -18.62759615963255300, -10.81492255796106328, 44.16775706135234714 ) ) ;
#28796=CARTESIAN_POINT ( 'NONE',  ( -16.51473224551082808, 9.474510206698731452, 58.33442372801900433 ) ) ;
#28797=CARTESIAN_POINT ( 'NONE',  ( 9.474510206698971260, -16.51473224551069308, 37.91557627198102409 ) ) ;
#28798=CARTESIAN_POINT ( 'NONE',  ( 9.564922557960805705, 16.46253265017160317, 79.58224293864769550 ) ) ;
#28799=CARTESIAN_POINT ( 'NONE',  ( -12.06949235617739369, -12.14591786802326823, 29.37609039468568284 ) ) ;
#28800=CARTESIAN_POINT ( 'NONE',  ( -8.224510206698948167, 14.34966873604960824, 85.41557627198102409 ) ) ;
#28801=CARTESIAN_POINT ( 'NONE',  ( 19.03943276465977164, -0.05219959533909143690, 53.74890960531436690 ) ) ;
#28802=CARTESIAN_POINT ( 'NONE',  ( -21.53943276465977519, 0.05219959533907696930, 51.24890960531436690 ) ) ;
#28803=CARTESIAN_POINT ( 'NONE',  ( 12.14591786802327356, -12.06949235617739191, 25.62609039468567929 ) ) ;
#28804=CARTESIAN_POINT ( 'NONE',  ( -18.62759615963255300, -10.81492255796106328, 24.16775706135235424 ) ) ;
#28805=CARTESIAN_POINT ( 'NONE',  ( -18.62759615963255300, -10.81492255796106328, 64.16775706135234714 ) ) ;
#28806=CARTESIAN_POINT ( 'NONE',  ( -14.29746914071037622, -8.314922557961029526, 69.16775706135234714 ) ) ;
#28807=CARTESIAN_POINT ( 'NONE',  ( 14.29746914071037800, 8.314922557961029526, 71.66775706135234714 ) ) ;
#28808=CARTESIAN_POINT ( 'NONE',  ( -9.474510206698964154, 16.51473224551069663, 55.41557627198103120 ) ) ;
#28809=CARTESIAN_POINT ( 'NONE',  ( 12.06949235617739724, 12.14591786802326823, 91.87609039468568994 ) ) ;
#28810=CARTESIAN_POINT ( 'NONE',  ( -5.049401038297874678, -19.05341960407617918, 44.79275706135232582 ) ) ;
#28812=CARTESIAN_POINT ( 'NONE',  ( 15.80617190586746368, 15.72974639402197994, 109.3739096053143811 ) ) ;
#28813=CARTESIAN_POINT ( 'NONE',  ( 14.34966873604960469, 8.224510206698951720, 69.16557627198102409 ) ) ;
#28814=CARTESIAN_POINT ( 'NONE',  ( 19.05341960407611168, 5.049401038298154454, 83.95724293864766707 ) ) ;
#28815=CARTESIAN_POINT ( 'NONE',  ( -8.314922557961024197, 14.29746914071037800, 87.91775706135234714 ) ) ;
#28816=CARTESIAN_POINT ( 'NONE',  ( -18.62759615963255300, -10.81492255796106328, 64.16775706135234714 ) ) ;
#28817=CARTESIAN_POINT ( 'NONE',  ( 16.52544592524335698, 4.483927247898782831, 31.45942372801901854 ) ) ;
#28818=CARTESIAN_POINT ( 'NONE',  ( -0.05219959533937732626, 21.53943276465977519, 22.50109039468567573 ) ) ;
#28819=CARTESIAN_POINT ( 'NONE',  ( -12.06949235617756955, 12.14591786802309770, 55.62390960531436690 ) ) ;
#28821=CARTESIAN_POINT ( 'NONE',  ( 10.81492255796078972, 18.62759615963270932, 99.58224293864770971 ) ) ;
#28822=CARTESIAN_POINT ( 'NONE',  ( -0.05219959533910754901, -16.53943276465976808, 37.49890960531436690 ) ) ;
#28825=CARTESIAN_POINT ( 'NONE',  ( 15.80617190586746368, 15.72974639402197994, 34.37390960531435979 ) ) ;
#28826=CARTESIAN_POINT ( 'NONE',  ( -5.719274019375665041, -21.55341960407619695, 34.79275706135235424 ) ) ;
#28827=CARTESIAN_POINT ( 'NONE',  ( 16.52544592524342804, -4.483927247898539470, 68.54057627198103830 ) ) ;
#28828=CARTESIAN_POINT ( 'NONE',  ( 16.46253265017160672, -9.564922557960803928, 78.33224293864769550 ) ) ;
#28829=CARTESIAN_POINT ( 'NONE',  ( 19.03943276465977164, -0.05219959533909143690, 23.74890960531435269 ) ) ;
#28830=CARTESIAN_POINT ( 'NONE',  ( 5.153800228976615827, -19.02544592524334988, 65.20942372801900433 ) ) ;
#28832=CARTESIAN_POINT ( 'NONE',  ( 21.52544592524344225, -5.823673210054117533, 48.54057627198103120 ) ) ;
#28834=CARTESIAN_POINT ( 'NONE',  ( -5.049401038298153566, 19.05341960407611168, 55.20724293864769550 ) ) ;
#28835=CARTESIAN_POINT ( 'NONE',  ( 14.29746914071037800, 8.314922557961029526, 41.66775706135235424 ) ) ;
#28836=CARTESIAN_POINT ( 'NONE',  ( -5.823673210054116645, -21.52544592524344225, 112.2905762719810241 ) ) ;
#28837=CARTESIAN_POINT ( 'NONE',  ( 12.14591786802309770, 12.06949235617756955, 49.37390960531436690 ) ) ;
#28839=CARTESIAN_POINT ( 'NONE',  ( -9.474510206698964154, 16.51473224551069663, 95.41557627198102409 ) ) ;
#28840=CARTESIAN_POINT ( 'NONE',  ( -21.55341960407610458, -5.719274019375992779, 76.45724293864769550 ) ) ;
#28841=CARTESIAN_POINT ( 'NONE',  ( 18.62759615963271287, -10.81492255796078972, 113.3322429386476955 ) ) ;
#28842=CARTESIAN_POINT ( 'NONE',  ( 14.29746914071037800, 8.314922557961029526, 31.66775706135234358 ) ) ;
#28843=CARTESIAN_POINT ( 'NONE',  ( 5.719274019375991003, -21.55341960407610458, 32.70724293864770260 ) ) ;
#28844=CARTESIAN_POINT ( 'NONE',  ( -0.05219959533937732626, 21.53943276465977519, 107.5010903946856899 ) ) ;
#28845=CARTESIAN_POINT ( 'NONE',  ( 0.05219959533909260263, 19.03943276465977164, 99.99890960531436690 ) ) ;
#28847=CARTESIAN_POINT ( 'NONE',  ( -13.89961937509977652, 13.97604488694528158, 35.62390960531435269 ) ) ;
#28848=CARTESIAN_POINT ( 'NONE',  ( -9.564922557960796823, -16.46253265017161027, 97.08224293864769550 ) ) ;
#28849=CARTESIAN_POINT ( 'NONE',  ( 19.03943276465977164, -0.05219959533909143690, 73.74890960531435269 ) ) ;
#28851=CARTESIAN_POINT ( 'NONE',  ( 5.153800228976615827, -19.02544592524334988, 60.20942372801899012 ) ) ;
#28852=CARTESIAN_POINT ( 'NONE',  ( 15.72974639402176855, 15.80617190586768217, 106.8760903946856899 ) ) ;
#28853=CARTESIAN_POINT ( 'NONE',  ( 21.52544592524344225, -5.823673210054117533, 33.54057627198102409 ) ) ;
#28854=CARTESIAN_POINT ( 'NONE',  ( -14.29746914071037622, -8.314922557961029526, 104.1677570613523471 ) ) ;
#28855=CARTESIAN_POINT ( 'NONE',  ( 9.474510206698729675, 16.51473224551082808, 87.08442372801900433 ) ) ;
#28857=CARTESIAN_POINT ( 'NONE',  ( -16.51473224551082808, 9.474510206698731452, 78.33442372801900433 ) ) ;
#28858=CARTESIAN_POINT ( 'NONE',  ( 19.03943276465977164, 0.05219959533936151252, 31.25109039468566863 ) ) ;
#28859=CARTESIAN_POINT ( 'NONE',  ( -16.20579543436681291, -7.371946100354976217, 45.56520834171876544 ) ) ;
#28860=CARTESIAN_POINT ( 'NONE',  ( 13.89961937509977652, -13.97604488694527269, 48.12390960531435979 ) ) ;
#28861=CARTESIAN_POINT ( 'NONE',  ( 16.55341960407611168, 4.379528057220329451, 53.95724293864770260 ) ) ;
#28862=CARTESIAN_POINT ( 'NONE',  ( -16.36317988757057762, -7.306389748694935626, 110.9021039163677784 ) ) ;
#28863=CARTESIAN_POINT ( 'NONE',  ( -12.14591786802309592, -12.06949235617757132, 21.87390960531436690 ) ) ;
#28865=CARTESIAN_POINT ( 'NONE',  ( -14.29746914071037622, -8.314922557961029526, 89.16775706135236135 ) ) ;
#28866=CARTESIAN_POINT ( 'NONE',  ( -9.474510206698964154, 16.51473224551069663, 45.41557627198103120 ) ) ;
#28867=CARTESIAN_POINT ( 'NONE',  ( 10.81492255796106328, -18.62759615963255655, 110.4177570613523756 ) ) ;
#28868=CARTESIAN_POINT ( 'NONE',  ( -9.564922557961040184, 16.46253265017147172, 112.9177570613523329 ) ) ;
#28869=CARTESIAN_POINT ( 'NONE',  ( -10.81492255796105439, 18.62759615963255655, 92.91775706135236135 ) ) ;
#28870=CARTESIAN_POINT ( 'NONE',  ( -19.05341960407611168, -5.049401038298163336, 86.45724293864769550 ) ) ;
#28871=CARTESIAN_POINT ( 'NONE',  ( 16.51473224551069308, 9.474510206698969483, 89.16557627198103830 ) ) ;
#28873=CARTESIAN_POINT ( 'NONE',  ( -21.52544592524343514, 5.823673210054127303, 116.0405762719810383 ) ) ;
#28874=VECTOR ( 'NONE', #149367, 1000.000000000000000 ) ;
#28875=CARTESIAN_POINT ( 'NONE',  ( -16.52544592524342804, 4.483927247898546575, 86.04057627198102409 ) ) ;
#28876=CARTESIAN_POINT ( 'NONE',  ( 10.81492255796078972, 18.62759615963270932, 69.58224293864769550 ) ) ;
#28877=CARTESIAN_POINT ( 'NONE',  ( -16.46253265017160317, 9.564922557960807481, 55.83224293864769550 ) ) ;
#28878=CARTESIAN_POINT ( 'NONE',  ( 18.62759615963271287, -10.81492255796078972, 103.3322429386476955 ) ) ;
#28879=CARTESIAN_POINT ( 'NONE',  ( 14.34966873604972726, -8.224510206698740333, 95.83442372801903275 ) ) ;
#28881=CARTESIAN_POINT ( 'NONE',  ( -16.51473224551069308, -9.474510206698971260, 61.66557627198103120 ) ) ;
#28882=CARTESIAN_POINT ( 'NONE',  ( -14.34966873604960291, -8.224510206698953496, 86.66557627198102409 ) ) ;
#28884=CARTESIAN_POINT ( 'NONE',  ( 9.474510206698971260, -16.51473224551069308, 62.91557627198102409 ) ) ;
#28885=CARTESIAN_POINT ( 'NONE',  ( 9.564922557961047289, -16.46253265017146816, 80.41775706135234714 ) ) ;
#28886=CARTESIAN_POINT ( 'NONE',  ( -12.06949235617756955, 12.14591786802309770, 85.62390960531436690 ) ) ;
#28887=CARTESIAN_POINT ( 'NONE',  ( -10.72451020669870658, -18.67979575497194134, 59.58442372801901854 ) ) ;
#28888=CARTESIAN_POINT ( 'NONE',  ( -13.97604488694527625, -13.89961937509977652, 51.87390960531436690 ) ) ;
#28889=CARTESIAN_POINT ( 'NONE',  ( 18.67979575497178502, 10.72451020669898547, 114.1655762719810383 ) ) ;
#28890=CARTESIAN_POINT ( 'NONE',  ( -0.05219959533910754901, -16.53943276465976808, 107.4989096053143669 ) ) ;
#28892=CARTESIAN_POINT ( 'NONE',  ( 16.46253265017160672, -9.564922557960803928, 53.33224293864768839 ) ) ;
#28893=CARTESIAN_POINT ( 'NONE',  ( 30.00000000000000000, -1.163414459189985801E-14, 95.00000000000000000 ) ) ;
#28894=CARTESIAN_POINT ( 'NONE',  ( -19.05341960407617563, 5.049401038297882671, 98.54275706135233293 ) ) ;
#28895=CARTESIAN_POINT ( 'NONE',  ( -16.51473224551069308, -9.474510206698971260, 111.6655762719810383 ) ) ;
#28896=CARTESIAN_POINT ( 'NONE',  ( 18.67979575497194134, -10.72451020669871369, 45.83442372801901854 ) ) ;
#28897=CARTESIAN_POINT ( 'NONE',  ( -5.049401038298153566, 19.05341960407611168, 85.20724293864766707 ) ) ;
#28898=CARTESIAN_POINT ( 'NONE',  ( 9.564922557961047289, -16.46253265017146816, 75.41775706135234714 ) ) ;
#28899=CARTESIAN_POINT ( 'NONE',  ( -16.46253265017160317, 9.564922557960807481, 60.83224293864769550 ) ) ;
#28900=CARTESIAN_POINT ( 'NONE',  ( 12.06949235617757843, -12.14591786802309237, 78.12390960531436690 ) ) ;
#28901=CARTESIAN_POINT ( 'NONE',  ( 8.314922557960818139, 14.29746914071049879, 74.58224293864768129 ) ) ;
#28902=CARTESIAN_POINT ( 'NONE',  ( 16.46253265017160672, -9.564922557960803928, 93.33224293864769550 ) ) ;
#28903=CARTESIAN_POINT ( 'NONE',  ( 16.53943276465976808, -0.05219959533910856209, 83.74890960531435269 ) ) ;
#28904=CARTESIAN_POINT ( 'NONE',  ( -9.564922557960796823, -16.46253265017161027, 82.08224293864768129 ) ) ;
#28905=CARTESIAN_POINT ( 'NONE',  ( -13.97604488694547697, 13.89961937509957934, 38.12609039468566152 ) ) ;
#28906=CARTESIAN_POINT ( 'NONE',  ( 19.02544592524343514, -5.153800228976328945, 53.54057627198102409 ) ) ;
#28907=CARTESIAN_POINT ( 'NONE',  ( 14.34966873604960469, 8.224510206698951720, 34.16557627198102409 ) ) ;
#28908=CARTESIAN_POINT ( 'NONE',  ( -14.29746914071049879, 8.314922557960819915, 110.8322429386476955 ) ) ;
#28910=CARTESIAN_POINT ( 'NONE',  ( -18.67979575497193778, 10.72451020669871902, 43.33442372801901143 ) ) ;
#28911=CARTESIAN_POINT ( 'NONE',  ( -16.46253265017146816, -9.564922557961047289, 64.16775706135233293 ) ) ;
#28912=CARTESIAN_POINT ( 'NONE',  ( 4.379528057220339221, -16.55341960407611168, 37.70724293864769550 ) ) ;
#28913=CARTESIAN_POINT ( 'NONE',  ( -21.52544592524343514, 5.823673210054127303, 81.04057627198102409 ) ) ;
#28914=CARTESIAN_POINT ( 'NONE',  ( -19.05341960407611168, -5.049401038298163336, 111.4572429386476671 ) ) ;
#28915=CARTESIAN_POINT ( 'NONE',  ( 8.224510206698953496, -14.34966873604960469, 72.91557627198103830 ) ) ;
#28916=CARTESIAN_POINT ( 'NONE',  ( -13.89961937509977652, 13.97604488694528158, 40.62390960531435979 ) ) ;
#28917=CARTESIAN_POINT ( 'NONE',  ( -19.05341960407617563, 5.049401038297882671, 43.54275706135232582 ) ) ;
#28918=CARTESIAN_POINT ( 'NONE',  ( -12.06949235617739369, -12.14591786802326823, 99.37609039468568994 ) ) ;
#28919=CARTESIAN_POINT ( 'NONE',  ( -14.34966873604972548, 8.224510206698743886, 53.33442372801901854 ) ) ;
#28920=CARTESIAN_POINT ( 'NONE',  ( 21.53943276465977519, -0.05219959533907433946, 33.74890960531436690 ) ) ;
#28921=CARTESIAN_POINT ( 'NONE',  ( 10.81492255796106328, -18.62759615963255655, 105.4177570613523613 ) ) ;
#28922=CARTESIAN_POINT ( 'NONE',  ( 9.474510206698971260, -16.51473224551069308, 87.91557627198102409 ) ) ;
#28923=CARTESIAN_POINT ( 'NONE',  ( 16.55341960407618274, -4.379528057220086978, 71.04275706135234714 ) ) ;
#28924=CARTESIAN_POINT ( 'NONE',  ( -9.474510206698964154, 16.51473224551069663, 25.41557627198103120 ) ) ;
#28925=CARTESIAN_POINT ( 'NONE',  ( 16.53943276465976808, -0.05219959533910856209, 33.74890960531436690 ) ) ;
#28926=CARTESIAN_POINT ( 'NONE',  ( 19.02544592524343514, -5.153800228976328945, 108.5405762719810383 ) ) ;
#28927=CARTESIAN_POINT ( 'NONE',  ( 9.564922557960805705, 16.46253265017160317, 94.58224293864769550 ) ) ;
#28928=CARTESIAN_POINT ( 'NONE',  ( 10.72451020669898902, -18.67979575497178502, 32.91557627198102409 ) ) ;
#28929=CARTESIAN_POINT ( 'NONE',  ( 4.379528057220339221, -16.55341960407611168, 67.70724293864769550 ) ) ;
#28930=CARTESIAN_POINT ( 'NONE',  ( -16.55341960407611168, -4.379528057220339221, 46.45724293864769550 ) ) ;
#28931=ORIENTED_EDGE ( 'NONE', *, *, #142282, .F. ) ;
#28932=CARTESIAN_POINT ( 'NONE',  ( 12.06949235617739724, 12.14591786802326823, 56.87609039468568994 ) ) ;
#28934=CARTESIAN_POINT ( 'NONE',  ( -19.03943276465977164, -0.05219959533935918106, 53.75109039468566863 ) ) ;
#28935=CARTESIAN_POINT ( 'NONE',  ( 16.46253265017160672, -9.564922557960803928, 83.33224293864768129 ) ) ;
#28936=CARTESIAN_POINT ( 'NONE',  ( -19.02544592524334988, -5.153800228976617603, 63.95942372801899012 ) ) ;
#28938=CARTESIAN_POINT ( 'NONE',  ( 13.89961937509957401, 13.97604488694547697, 51.87609039468566863 ) ) ;
#28939=CARTESIAN_POINT ( 'NONE',  ( 19.02544592524334988, 5.153800228976608722, 101.4594237280189759 ) ) ;
#28940=CARTESIAN_POINT ( 'NONE',  ( -0.05219959533934338120, 16.53943276465976808, 102.5010903946856899 ) ) ;
#28942=CARTESIAN_POINT ( 'NONE',  ( 19.02544592524343514, -5.153800228976328945, 43.54057627198103120 ) ) ;
#28943=CARTESIAN_POINT ( 'NONE',  ( -5.719274019375978568, 21.55341960407610458, 25.20724293864769550 ) ) ;
#28944=CARTESIAN_POINT ( 'NONE',  ( -18.67979575497193778, 10.72451020669871902, 48.33442372801902565 ) ) ;
#28945=CARTESIAN_POINT ( 'NONE',  ( 19.05341960407617918, -5.049401038297876454, 101.0427570613523045 ) ) ;
#28946=FACE_OUTER_BOUND ( 'NONE', #55332, .T. ) ;
#28947=CARTESIAN_POINT ( 'NONE',  ( -16.51473224551069308, -9.474510206698971260, 66.66557627198102409 ) ) ;
#28949=CARTESIAN_POINT ( 'NONE',  ( -16.55341960407611168, -4.379528057220339221, 71.45724293864769550 ) ) ;
#28950=CARTESIAN_POINT ( 'NONE',  ( 19.03943276465977164, -0.05219959533909143690, 58.74890960531435979 ) ) ;
#28951=CARTESIAN_POINT ( 'NONE',  ( 19.05341960407611168, 5.049401038298154454, 73.95724293864768129 ) ) ;
#28952=CARTESIAN_POINT ( 'NONE',  ( 9.474510206698729675, 16.51473224551082808, 82.08442372801899012 ) ) ;
#28953=CARTESIAN_POINT ( 'NONE',  ( 18.67979575497178502, 10.72451020669898547, 64.16557627198102409 ) ) ;
#28954=CARTESIAN_POINT ( 'NONE',  ( 16.53943276465976808, -0.05219959533910856209, 113.7489096053143527 ) ) ;
#28955=CARTESIAN_POINT ( 'NONE',  ( 0.05219959533936267826, -19.03943276465977164, 45.00109039468566863 ) ) ;
#28956=CARTESIAN_POINT ( 'NONE',  ( 19.02544592524343514, -5.153800228976328945, 78.54057627198099567 ) ) ;
#28957=CARTESIAN_POINT ( 'NONE',  ( 5.823673210054125526, 21.52544592524343514, 84.79057627198102409 ) ) ;
#28958=CARTESIAN_POINT ( 'NONE',  ( 16.53943276465976808, -0.05219959533910856209, 73.74890960531433848 ) ) ;
#28959=CARTESIAN_POINT ( 'NONE',  ( 19.03943276465977164, 0.05219959533936151252, 51.25109039468567573 ) ) ;
#28960=CARTESIAN_POINT ( 'NONE',  ( 18.62759615963271287, -10.81492255796078972, 78.33224293864770971 ) ) ;
#28961=CARTESIAN_POINT ( 'NONE',  ( -15.72974639402197994, 15.80617190586746368, 60.62390960531437401 ) ) ;
#28962=CARTESIAN_POINT ( 'NONE',  ( 21.53943276465977519, -0.05219959533907433946, 38.74890960531435979 ) ) ;
#28963=CARTESIAN_POINT ( 'NONE',  ( -10.81492255796105439, 18.62759615963255655, 87.91775706135234714 ) ) ;
#28964=CARTESIAN_POINT ( 'NONE',  ( 16.51473224551069308, 9.474510206698969483, 79.16557627198103830 ) ) ;
#28965=CARTESIAN_POINT ( 'NONE',  ( 13.89961937509977652, -13.97604488694527269, 23.12390960531436335 ) ) ;
#28966=CARTESIAN_POINT ( 'NONE',  ( -5.823673210054431948, 21.52544592524334988, 32.70942372801900433 ) ) ;
#28967=CARTESIAN_POINT ( 'NONE',  ( -0.05219959533937732626, 21.53943276465977519, 47.50109039468568994 ) ) ;
#28968=CARTESIAN_POINT ( 'NONE',  ( -5.049401038298153566, 19.05341960407611168, 40.20724293864768839 ) ) ;
#28969=CARTESIAN_POINT ( 'NONE',  ( -21.55341960407619339, 5.719274019375674811, 28.54275706135234358 ) ) ;
#28970=CARTESIAN_POINT ( 'NONE',  ( 19.02544592524334988, 5.153800228976608722, 61.45942372801900433 ) ) ;
#28971=CARTESIAN_POINT ( 'NONE',  ( 0.05219959533909260263, 19.03943276465977164, 34.99890960531435979 ) ) ;
#28972=CARTESIAN_POINT ( 'NONE',  ( -16.52544592524335698, -4.483927247898792601, 33.95942372801901143 ) ) ;
#28974=CARTESIAN_POINT ( 'NONE',  ( 16.52544592524335698, 4.483927247898782831, 61.45942372801901854 ) ) ;
#28975=CARTESIAN_POINT ( 'NONE',  ( 13.89961937509977652, -13.97604488694527269, 38.12390960531436690 ) ) ;
#28977=CARTESIAN_POINT ( 'NONE',  ( 5.153800228976335163, 19.02544592524342804, 84.79057627198099567 ) ) ;
#28978=CARTESIAN_POINT ( 'NONE',  ( 0.05219959533909260263, 19.03943276465977164, 24.99890960531435269 ) ) ;
#28980=CARTESIAN_POINT ( 'NONE',  ( -18.62759615963270932, 10.81492255796079327, 55.83224293864770260 ) ) ;
#28981=CARTESIAN_POINT ( 'NONE',  ( -12.14591786802326823, 12.06949235617739902, 53.12609039468568284 ) ) ;
#28982=CARTESIAN_POINT ( 'NONE',  ( -21.52544592524334988, -5.823673210054445271, 103.9594237280190185 ) ) ;
#28983=CARTESIAN_POINT ( 'NONE',  ( -13.89961937509977652, 13.97604488694528158, 40.62390960531435979 ) ) ;
#28984=CARTESIAN_POINT ( 'NONE',  ( -0.05219959533910754901, -16.53943276465976808, 27.49890960531435269 ) ) ;
#28985=CARTESIAN_POINT ( 'NONE',  ( -8.224510206698948167, 14.34966873604960824, 60.41557627198102409 ) ) ;
#28987=CARTESIAN_POINT ( 'NONE',  ( 16.51473224551069308, 9.474510206698969483, 59.16557627198102409 ) ) ;
#28988=CARTESIAN_POINT ( 'NONE',  ( 21.52544592524334988, 5.823673210054432836, 106.4594237280190328 ) ) ;
#28989=CARTESIAN_POINT ( 'NONE',  ( -5.719274019375665041, -21.55341960407619695, 19.79275706135235069 ) ) ;
#28990=CARTESIAN_POINT ( 'NONE',  ( -0.05219959533937732626, 21.53943276465977519, 87.50109039468568994 ) ) ;
#28991=CARTESIAN_POINT ( 'NONE',  ( 12.06949235617739724, 12.14591786802326823, 46.87609039468568994 ) ) ;
#28992=CARTESIAN_POINT ( 'NONE',  ( 4.483927247898790824, -16.52544592524335698, 30.20942372801902565 ) ) ;
#28993=CARTESIAN_POINT ( 'NONE',  ( -8.224510206698948167, 14.34966873604960824, 95.41557627198102409 ) ) ;
#28994=CARTESIAN_POINT ( 'NONE',  ( -21.53943276465977519, -0.05219959533937600094, 103.7510903946857042 ) ) ;
#28995=CARTESIAN_POINT ( 'NONE',  ( -16.53943276465976808, 0.05219959533911058130, 31.24890960531435979 ) ) ;
#28996=CARTESIAN_POINT ( 'NONE',  ( -5.049401038298153566, 19.05341960407611168, 25.20724293864768484 ) ) ;
#28997=CARTESIAN_POINT ( 'NONE',  ( -8.224510206698735004, -14.34966873604973081, 44.58442372801901854 ) ) ;
#28998=CARTESIAN_POINT ( 'NONE',  ( -16.55341960407611168, -4.379528057220339221, 56.45724293864768839 ) ) ;
#28999=CARTESIAN_POINT ( 'NONE',  ( 8.224510206698742110, 14.34966873604972548, 92.08442372801901854 ) ) ;
#29000=CARTESIAN_POINT ( 'NONE',  ( 9.564922557960805705, 16.46253265017160317, 94.58224293864769550 ) ) ;
#29001=CARTESIAN_POINT ( 'NONE',  ( -21.55341960407610458, -5.719274019375992779, 21.45724293864769550 ) ) ;
#29002=CARTESIAN_POINT ( 'NONE',  ( -15.80617190586768217, 15.72974639402176855, 108.1260903946856757 ) ) ;
#29003=CARTESIAN_POINT ( 'NONE',  ( 16.55341960407611168, 4.379528057220329451, 88.95724293864769550 ) ) ;
#29004=CARTESIAN_POINT ( 'NONE',  ( -5.049401038298153566, 19.05341960407611168, 100.2072429386476955 ) ) ;
#29007=CARTESIAN_POINT ( 'NONE',  ( 8.224510206698742110, 14.34966873604972548, 42.08442372801901854 ) ) ;
#29008=CARTESIAN_POINT ( 'NONE',  ( 0.05219959533909260263, 19.03943276465977164, 44.99890960531435979 ) ) ;
#29009=CARTESIAN_POINT ( 'NONE',  ( 5.153800228976335163, 19.02544592524342804, 109.7905762719810099 ) ) ;
#29010=CARTESIAN_POINT ( 'NONE',  ( 14.29746914071037800, 8.314922557961029526, 46.66775706135234714 ) ) ;
#29011=CARTESIAN_POINT ( 'NONE',  ( -16.46253265017146816, -9.564922557961047289, 29.16775706135232937 ) ) ;
#29012=CARTESIAN_POINT ( 'NONE',  ( 19.02544592524343514, -5.153800228976328945, 43.54057627198103120 ) ) ;
#29013=CARTESIAN_POINT ( 'NONE',  ( 14.29746914071037800, 8.314922557961029526, 76.66775706135234714 ) ) ;
#29014=CARTESIAN_POINT ( 'NONE',  ( 19.05341960407617918, -5.049401038297876454, 81.04275706135231871 ) ) ;
#29015=CARTESIAN_POINT ( 'NONE',  ( -16.46253265017146816, -9.564922557961047289, 24.16775706135233648 ) ) ;
#29016=CARTESIAN_POINT ( 'NONE',  ( -13.97604488694527625, -13.89961937509977652, 56.87390960531434558 ) ) ;
#29017=CARTESIAN_POINT ( 'NONE',  ( 16.55341960407611168, 4.379528057220329451, 103.9572429386476813 ) ) ;
#29019=CARTESIAN_POINT ( 'NONE',  ( -16.46253265017146816, -9.564922557961047289, 74.16775706135234714 ) ) ;
#29020=CARTESIAN_POINT ( 'NONE',  ( -10.81492255796078084, -18.62759615963271287, 62.08224293864769550 ) ) ;
#29021=CARTESIAN_POINT ( 'NONE',  ( 19.05341960407617918, -5.049401038297876454, 26.04275706135233293 ) ) ;
#29022=CARTESIAN_POINT ( 'NONE',  ( 9.564922557960805705, 16.46253265017160317, 99.58224293864770971 ) ) ;
#29023=CARTESIAN_POINT ( 'NONE',  ( -21.55341960407610458, -5.719274019375992779, 76.45724293864769550 ) ) ;
#29024=CARTESIAN_POINT ( 'NONE',  ( -18.39443945427639093, 5.500000000000031974, 53.51745347608652992 ) ) ;
#29025=CARTESIAN_POINT ( 'NONE',  ( 19.05341960407617918, -5.049401038297876454, 96.04275706135231871 ) ) ;
#29026=CARTESIAN_POINT ( 'NONE',  ( -19.49149378614658445, 5.499999999999785949, 59.43757513605363840 ) ) ;
#29027=CARTESIAN_POINT ( 'NONE',  ( -16.55341960407617563, 4.379528057220093196, 23.54275706135235424 ) ) ;
#29028=CARTESIAN_POINT ( 'NONE',  ( 16.51473224551069308, 9.474510206698969483, 34.16557627198102409 ) ) ;
#29029=CARTESIAN_POINT ( 'NONE',  ( 19.02544592524343514, -5.153800228976328945, 103.5405762719809957 ) ) ;
#29030=CARTESIAN_POINT ( 'NONE',  ( 5.823673210054125526, 21.52544592524343514, 89.79057627198103830 ) ) ;
#29031=CARTESIAN_POINT ( 'NONE',  ( 18.67979575497194134, -10.72451020669871369, 65.83442372801900433 ) ) ;
#29032=CARTESIAN_POINT ( 'NONE',  ( -19.05341960407617563, 5.049401038297882671, 103.5427570613523329 ) ) ;
#29033=CARTESIAN_POINT ( 'NONE',  ( -15.72974639402176322, -15.80617190586768395, 104.3760903946856899 ) ) ;
#29034=CARTESIAN_POINT ( 'NONE',  ( -8.224510206698735004, -14.34966873604973081, 109.5844237280190328 ) ) ;
#29035=CARTESIAN_POINT ( 'NONE',  ( 15.80617190586746368, 15.72974639402197994, 104.3739096053143669 ) ) ;
#29036=CARTESIAN_POINT ( 'NONE',  ( -4.379528057220328563, 16.55341960407611168, 50.20724293864769550 ) ) ;
#29037=CARTESIAN_POINT ( 'NONE',  ( 16.51473224551083163, -9.474510206698727899, 85.83442372801900433 ) ) ;
#29038=CARTESIAN_POINT ( 'NONE',  ( 5.153800228976615827, -19.02544592524334988, 60.20942372801899012 ) ) ;
#29039=CARTESIAN_POINT ( 'NONE',  ( -5.823673210054431948, 21.52544592524334988, 57.70942372801901143 ) ) ;
#29040=CARTESIAN_POINT ( 'NONE',  ( -19.05341960407617563, 5.049401038297882671, 43.54275706135232582 ) ) ;
#29041=CARTESIAN_POINT ( 'NONE',  ( 12.14591786802309770, 12.06949235617756955, 109.3739096053143811 ) ) ;
#29042=CARTESIAN_POINT ( 'NONE',  ( -21.55341960407610458, -5.719274019375992779, 36.45724293864768839 ) ) ;
#29043=CARTESIAN_POINT ( 'NONE',  ( 0.05219959533910956823, 16.53943276465976808, 34.99890960531435979 ) ) ;
#29044=CARTESIAN_POINT ( 'NONE',  ( -21.55341960407619339, 5.719274019375674811, 93.54275706135234714 ) ) ;
#29045=CARTESIAN_POINT ( 'NONE',  ( 14.29746914071037800, 8.314922557961029526, 76.66775706135234714 ) ) ;
#29046=CARTESIAN_POINT ( 'NONE',  ( 12.14591786802309770, 12.06949235617756955, 29.37390960531435269 ) ) ;
#29047=CARTESIAN_POINT ( 'NONE',  ( -18.62759615963255300, -10.81492255796106328, 59.16775706135234714 ) ) ;
#29048=CARTESIAN_POINT ( 'NONE',  ( 21.53943276465977519, 0.05219959533937863772, 61.25109039468567573 ) ) ;
#29049=CARTESIAN_POINT ( 'NONE',  ( -21.53943276465977519, 0.05219959533907696930, 71.24890960531435269 ) ) ;
#29050=CARTESIAN_POINT ( 'NONE',  ( 13.89961937509977652, -13.97604488694527269, 23.12390960531436335 ) ) ;
#29051=CARTESIAN_POINT ( 'NONE',  ( 10.72451020669871369, 18.67979575497193778, 42.08442372801901854 ) ) ;
#29052=CARTESIAN_POINT ( 'NONE',  ( 19.05341960407611168, 5.049401038298154454, 23.95724293864769194 ) ) ;
#29053=CARTESIAN_POINT ( 'NONE',  ( -13.89961937509977652, 13.97604488694528158, 40.62390960531435979 ) ) ;
#29054=CARTESIAN_POINT ( 'NONE',  ( -16.52544592524342804, 4.483927247898546575, 86.04057627198102409 ) ) ;
#29055=CARTESIAN_POINT ( 'NONE',  ( 9.474510206698971260, -16.51473224551069308, 82.91557627198103830 ) ) ;
#29056=CARTESIAN_POINT ( 'NONE',  ( 12.06949235617757843, -12.14591786802309237, 33.12390960531435979 ) ) ;
#29057=CARTESIAN_POINT ( 'NONE',  ( -10.72451020669898014, 18.67979575497178502, 65.41557627198102409 ) ) ;
#29058=CARTESIAN_POINT ( 'NONE',  ( 15.72974639402199770, -15.80617190586745480, 108.1239096053143811 ) ) ;
#29059=CARTESIAN_POINT ( 'NONE',  ( 5.049401038298161559, -19.05341960407611168, 112.7072429386476813 ) ) ;
#29060=CARTESIAN_POINT ( 'NONE',  ( -16.51473224551069308, -9.474510206698971260, 71.66557627198102409 ) ) ;
#29061=CARTESIAN_POINT ( 'NONE',  ( 9.474510206698729675, 16.51473224551082808, 107.0844237280190043 ) ) ;
#29063=CARTESIAN_POINT ( 'NONE',  ( -10.72451020669898014, 18.67979575497178502, 60.41557627198102409 ) ) ;
#29064=CARTESIAN_POINT ( 'NONE',  ( -21.55341960407619339, 5.719274019375674811, 78.54275706135236135 ) ) ;
#29065=CARTESIAN_POINT ( 'NONE',  ( 16.46253265017160672, -9.564922557960803928, 73.33224293864769550 ) ) ;
#29066=CARTESIAN_POINT ( 'NONE',  ( 5.049401038298161559, -19.05341960407611168, 97.70724293864766707 ) ) ;
#29067=CARTESIAN_POINT ( 'NONE',  ( -16.52544592524335698, -4.483927247898792601, 73.95942372801901854 ) ) ;
#29068=CARTESIAN_POINT ( 'NONE',  ( 0.05219959533937995610, -21.53943276465977519, 55.00109039468568284 ) ) ;
#29069=CARTESIAN_POINT ( 'NONE',  ( 15.72974639402176855, 15.80617190586768217, 96.87609039468568994 ) ) ;
#29070=CARTESIAN_POINT ( 'NONE',  ( 18.67979575497178502, 10.72451020669898547, 109.1655762719810383 ) ) ;
#29071=CARTESIAN_POINT ( 'NONE',  ( -5.823673210054116645, -21.52544592524344225, 77.29057627198102409 ) ) ;
#29072=CARTESIAN_POINT ( 'NONE',  ( 16.46253265017146816, 9.564922557961045513, 41.66775706135234003 ) ) ;
#29073=CARTESIAN_POINT ( 'NONE',  ( 21.53943276465977519, -0.05219959533907433946, 38.74890960531435979 ) ) ;
#29074=CARTESIAN_POINT ( 'NONE',  ( -5.049401038298153566, 19.05341960407611168, 75.20724293864769550 ) ) ;
#29075=CARTESIAN_POINT ( 'NONE',  ( 16.53943276465976808, -0.05219959533910856209, 33.74890960531436690 ) ) ;
#29076=CARTESIAN_POINT ( 'NONE',  ( -17.26172910966778673, 6.454744622555848466, 65.80646908649227100 ) ) ;
#29078=CARTESIAN_POINT ( 'NONE',  ( 13.97604488694548053, -13.89961937509957401, 90.62609039468567573 ) ) ;
#29079=CARTESIAN_POINT ( 'NONE',  ( 18.67979575497178502, 10.72451020669898547, 74.16557627198102409 ) ) ;
#29080=CARTESIAN_POINT ( 'NONE',  ( -8.224510206698948167, 14.34966873604960824, 50.41557627198103120 ) ) ;
#29081=CARTESIAN_POINT ( 'NONE',  ( 4.379528057220092307, 16.55341960407617563, 27.29275706135234358 ) ) ;
#29082=CARTESIAN_POINT ( 'NONE',  ( -19.05341960407611168, -5.049401038298163336, 41.45724293864769550 ) ) ;
#29083=CARTESIAN_POINT ( 'NONE',  ( 18.62759615963271287, -10.81492255796078972, 103.3322429386476955 ) ) ;
#29084=CARTESIAN_POINT ( 'NONE',  ( -19.05341960407617563, 5.049401038297882671, 88.54275706135230450 ) ) ;
#29085=CARTESIAN_POINT ( 'NONE',  ( 16.46253265017160672, -9.564922557960803928, 83.33224293864768129 ) ) ;
#29086=CARTESIAN_POINT ( 'NONE',  ( -16.55341960407611168, -4.379528057220339221, 96.45724293864770971 ) ) ;
#29087=CARTESIAN_POINT ( 'NONE',  ( -13.89961937509977652, 13.97604488694528158, 65.62390960531436690 ) ) ;
#29088=CARTESIAN_POINT ( 'NONE',  ( -4.379528057220328563, 16.55341960407611168, 65.20724293864768129 ) ) ;
#29089=CARTESIAN_POINT ( 'NONE',  ( 9.564922557960805705, 16.46253265017160317, 34.58224293864770260 ) ) ;
#29091=CARTESIAN_POINT ( 'NONE',  ( -16.55341960407611168, -4.379528057220339221, 36.45724293864768839 ) ) ;
#29092=CARTESIAN_POINT ( 'NONE',  ( 13.89961937509977652, -13.97604488694527269, 88.12390960531438111 ) ) ;
#29094=CARTESIAN_POINT ( 'NONE',  ( -9.474510206698720793, -16.51473224551083518, 54.58442372801899722 ) ) ;
#29095=CARTESIAN_POINT ( 'NONE',  ( -4.379528057220086978, -16.55341960407618274, 54.79275706135235424 ) ) ;
#29096=CARTESIAN_POINT ( 'NONE',  ( -0.05219959533907301413, -21.53943276465977519, 82.49890960531436690 ) ) ;
#29097=CARTESIAN_POINT ( 'NONE',  ( 19.02544592524334988, 5.153800228976608722, 36.45942372801900433 ) ) ;
#29098=CARTESIAN_POINT ( 'NONE',  ( 16.51473224551069308, 9.474510206698969483, 89.16557627198103830 ) ) ;
#29099=CARTESIAN_POINT ( 'NONE',  ( -17.50000000000002487, 4.049696124445873124, 114.1803967066594652 ) ) ;
#29100=CARTESIAN_POINT ( 'NONE',  ( -5.823673210054116645, -21.52544592524344225, 32.29057627198102409 ) ) ;
#29101=CARTESIAN_POINT ( 'NONE',  ( -5.049401038298153566, 19.05341960407611168, 55.20724293864769550 ) ) ;
#29102=CARTESIAN_POINT ( 'NONE',  ( -15.80617190586768217, 15.72974639402176855, 48.12609039468568284 ) ) ;
#29104=CARTESIAN_POINT ( 'NONE',  ( -9.564922557960796823, -16.46253265017161027, 22.08224293864768839 ) ) ;
#29105=CARTESIAN_POINT ( 'NONE',  ( 15.72974639402176855, 15.80617190586768217, 21.87609039468567573 ) ) ;
#29106=CARTESIAN_POINT ( 'NONE',  ( 0.05219959533909260263, 19.03943276465977164, 89.99890960531436690 ) ) ;
#29108=CARTESIAN_POINT ( 'NONE',  ( 10.72451020669871369, 18.67979575497193778, 42.08442372801901854 ) ) ;
#29109=ORIENTED_EDGE ( 'NONE', *, *, #155151, .T. ) ;
#29110=CARTESIAN_POINT ( 'NONE',  ( -19.03943276465977164, 0.05219959533909376836, 96.24890960531436690 ) ) ;
#29112=CARTESIAN_POINT ( 'NONE',  ( -21.53943276465977519, 0.05219959533907696930, 111.2489096053143669 ) ) ;
#29113=CARTESIAN_POINT ( 'NONE',  ( 19.03943276465977164, -0.05219959533909143690, 43.74890960531435979 ) ) ;
#29114=CARTESIAN_POINT ( 'NONE',  ( -14.29746914071037622, -8.314922557961029526, 24.16775706135235424 ) ) ;
#29116=CARTESIAN_POINT ( 'NONE',  ( -21.55341960407619339, 5.719274019375674811, 98.54275706135234714 ) ) ;
#29117=CARTESIAN_POINT ( 'NONE',  ( 19.05341960407611168, 5.049401038298154454, 28.95724293864769550 ) ) ;
#29118=CARTESIAN_POINT ( 'NONE',  ( -18.67979575497193778, 10.72451020669871902, 98.33442372801901854 ) ) ;
#29119=CARTESIAN_POINT ( 'NONE',  ( -0.05219959533909027116, -19.03943276465977164, 87.49890960531436690 ) ) ;
#29120=CARTESIAN_POINT ( 'NONE',  ( 5.719274019375673035, 21.55341960407619339, 57.29275706135234714 ) ) ;
#29123=CARTESIAN_POINT ( 'NONE',  ( -9.474510206698964154, 16.51473224551069663, 95.41557627198102409 ) ) ;
#29124=CARTESIAN_POINT ( 'NONE',  ( -17.49999999999999645, 3.237210098469573083, 29.71236987379550598 ) ) ;
#29125=CARTESIAN_POINT ( 'NONE',  ( 16.52544592524335698, 4.483927247898782831, 51.45942372801901854 ) ) ;
#29126=CARTESIAN_POINT ( 'NONE',  ( -0.05219959533934338120, 16.53943276465976808, 67.50109039468568994 ) ) ;
#29127=CARTESIAN_POINT ( 'NONE',  ( 15.80617190586769283, -15.72974639402175789, 60.62609039468567573 ) ) ;
#29128=CARTESIAN_POINT ( 'NONE',  ( 18.67979575497194134, -10.72451020669871369, 85.83442372801901854 ) ) ;
#29130=CARTESIAN_POINT ( 'NONE',  ( -8.314922557961024197, 14.29746914071037800, 27.91775706135234358 ) ) ;
#29131=CARTESIAN_POINT ( 'NONE',  ( 0.05219959533909260263, 19.03943276465977164, 74.99890960531435269 ) ) ;
#29132=CARTESIAN_POINT ( 'NONE',  ( -13.89961937509977652, 13.97604488694528158, 95.62390960531436690 ) ) ;
#29133=CARTESIAN_POINT ( 'NONE',  ( 18.22780087662123805, 5.499999999999960032, 91.48236817873106475 ) ) ;
#29134=CARTESIAN_POINT ( 'NONE',  ( 19.05341960407611168, 5.049401038298154454, 28.95724293864769550 ) ) ;
#29135=CARTESIAN_POINT ( 'NONE',  ( 15.72974639402199770, -15.80617190586745480, 28.12390960531435979 ) ) ;
#29136=CARTESIAN_POINT ( 'NONE',  ( -16.53943276465976808, -0.05219959533934237506, 98.75109039468568994 ) ) ;
#29137=CARTESIAN_POINT ( 'NONE',  ( 16.52544592524342804, -4.483927247898539470, 73.54057627198102409 ) ) ;
#29138=CARTESIAN_POINT ( 'NONE',  ( -19.03943276465977164, 0.05219959533909376836, 71.24890960531435269 ) ) ;
#29139=CARTESIAN_POINT ( 'NONE',  ( 21.55341960407619695, -5.719274019375665929, 91.04275706135236135 ) ) ;
#29141=CARTESIAN_POINT ( 'NONE',  ( -13.89961937509957401, -13.97604488694547875, 104.3760903946856757 ) ) ;
#29142=CARTESIAN_POINT ( 'NONE',  ( -8.314922557960811034, -14.29746914071050412, 82.08224293864768129 ) ) ;
#29143=CARTESIAN_POINT ( 'NONE',  ( -5.823673210054431948, 21.52544592524334988, 27.70942372801901854 ) ) ;
#29144=CARTESIAN_POINT ( 'NONE',  ( 0.05219959533907565091, 21.53943276465977519, 74.99890960531435269 ) ) ;
#29145=CARTESIAN_POINT ( 'NONE',  ( -19.02544592524334988, -5.153800228976617603, 43.95942372801899012 ) ) ;
#29147=CARTESIAN_POINT ( 'NONE',  ( 19.03943276465977164, -0.05219959533909143690, 78.74890960531436690 ) ) ;
#29148=CARTESIAN_POINT ( 'NONE',  ( 8.314922557960818139, 14.29746914071049879, 54.58224293864769550 ) ) ;
#29149=CARTESIAN_POINT ( 'NONE',  ( 14.34966873604960469, 8.224510206698951720, 29.16557627198103120 ) ) ;
#29150=CARTESIAN_POINT ( 'NONE',  ( 12.14591786802327356, -12.06949235617739191, 95.62609039468568994 ) ) ;
#29151=CARTESIAN_POINT ( 'NONE',  ( 13.97604488694548053, -13.89961937509957401, 50.62609039468566152 ) ) ;
#29152=CARTESIAN_POINT ( 'NONE',  ( 5.049401038297881783, 19.05341960407617918, 77.29275706135233293 ) ) ;
#29153=CARTESIAN_POINT ( 'NONE',  ( -16.46253265017160317, 9.564922557960807481, 105.8322429386476955 ) ) ;
#29154=CARTESIAN_POINT ( 'NONE',  ( 0.05219959533910956823, 16.53943276465976808, 69.99890960531435269 ) ) ;
#29155=DIRECTION ( 'NONE',  ( -0.000000000000000000, -0.000000000000000000, 1.000000000000000000 ) ) ;
#29156=CARTESIAN_POINT ( 'NONE',  ( -9.564922557960796823, -16.46253265017161027, 37.08224293864768839 ) ) ;
#29157=CARTESIAN_POINT ( 'NONE',  ( 5.823673210054125526, 21.52544592524343514, 29.79057627198102409 ) ) ;
#29158=CARTESIAN_POINT ( 'NONE',  ( 18.67979575497178502, 10.72451020669898547, 64.16557627198102409 ) ) ;
#29159=CARTESIAN_POINT ( 'NONE',  ( 4.379528057220339221, -16.55341960407611168, 107.7072429386476955 ) ) ;
#29160=CARTESIAN_POINT ( 'NONE',  ( 16.55341960407618274, -4.379528057220086978, 71.04275706135234714 ) ) ;
#29161=CARTESIAN_POINT ( 'NONE',  ( -9.474510206698964154, 16.51473224551069663, 45.41557627198103120 ) ) ;
#29162=CARTESIAN_POINT ( 'NONE',  ( 21.55341960407619695, -5.719274019375665929, 36.04275706135234714 ) ) ;
#29164=CARTESIAN_POINT ( 'NONE',  ( -8.314922557960811034, -14.29746914071050412, 87.08224293864769550 ) ) ;
#29168=CARTESIAN_POINT ( 'NONE',  ( -21.52544592524343514, 5.823673210054127303, 36.04057627198102409 ) ) ;
#29169=CARTESIAN_POINT ( 'NONE',  ( 17.50000000000000711, -5.622605283950866450, 66.18792689403889540 ) ) ;
#29171=CARTESIAN_POINT ( 'NONE',  ( 8.314922557961029526, -14.29746914071037800, 40.41775706135234714 ) ) ;
#29172=CARTESIAN_POINT ( 'NONE',  ( -0.05219959533910754901, -16.53943276465976808, 47.49890960531435979 ) ) ;
#29173=CARTESIAN_POINT ( 'NONE',  ( 21.52544592524344225, -5.823673210054117533, 73.54057627198102409 ) ) ;
#29174=CARTESIAN_POINT ( 'NONE',  ( 10.81492255796078972, 18.62759615963270932, 59.58224293864770260 ) ) ;
#29176=CARTESIAN_POINT ( 'NONE',  ( -9.474510206698720793, -16.51473224551083518, 79.58442372801899012 ) ) ;
#29177=CARTESIAN_POINT ( 'NONE',  ( 19.05341960407611168, 5.049401038298154454, 98.95724293864766707 ) ) ;
#29178=CARTESIAN_POINT ( 'NONE',  ( 13.97604488694527802, 13.89961937509977652, 44.37390960531435269 ) ) ;
#29179=CARTESIAN_POINT ( 'NONE',  ( 16.52544592524342804, -4.483927247898539470, 113.5405762719810383 ) ) ;
#29180=ADVANCED_FACE ( 'NONE', ( #127889 ), #58787, .T. ) ;
#29182=FACE_BOUND ( 'NONE', #8465, .T. ) ;
#29184=CARTESIAN_POINT ( 'NONE',  ( 14.34966873604972726, -8.224510206698740333, 70.83442372801901854 ) ) ;
#29185=CARTESIAN_POINT ( 'NONE',  ( -21.52544592524343514, 5.823673210054127303, 101.0405762719810383 ) ) ;
#29186=CARTESIAN_POINT ( 'NONE',  ( -5.049401038298153566, 19.05341960407611168, 50.20724293864770260 ) ) ;
#29187=CARTESIAN_POINT ( 'NONE',  ( -21.52544592524334988, -5.823673210054445271, 38.95942372801901854 ) ) ;
#29188=CARTESIAN_POINT ( 'NONE',  ( -9.474510206698964154, 16.51473224551069663, 90.41557627198103830 ) ) ;
#29191=CARTESIAN_POINT ( 'NONE',  ( -21.55341960407619339, 5.719274019375674811, 28.54275706135234358 ) ) ;
#29192=CARTESIAN_POINT ( 'NONE',  ( 16.46253265017160672, -9.564922557960803928, 108.3322429386476955 ) ) ;
#29193=CARTESIAN_POINT ( 'NONE',  ( 5.153800228976615827, -19.02544592524334988, 90.20942372801900433 ) ) ;
#29194=CARTESIAN_POINT ( 'NONE',  ( 5.049401038297881783, 19.05341960407617563, 42.29275706135234003 ) ) ;
#29195=CARTESIAN_POINT ( 'NONE',  ( -21.53943276465977519, 0.05219959533907696930, 106.2489096053143811 ) ) ;
#29196=CARTESIAN_POINT ( 'NONE',  ( 0.05219959533936267826, -19.03943276465977164, 35.00109039468566863 ) ) ;
#29197=CARTESIAN_POINT ( 'NONE',  ( 19.05341960407617918, -5.049401038297876454, 36.04275706135234003 ) ) ;
#29198=CARTESIAN_POINT ( 'NONE',  ( -4.483927247898782831, 16.52544592524335698, 92.70942372801901854 ) ) ;
#29200=CARTESIAN_POINT ( 'NONE',  ( -16.51473224551069308, -9.474510206698971260, 56.66557627198103120 ) ) ;
#29201=CARTESIAN_POINT ( 'NONE',  ( -15.72974639402176322, -15.80617190586768395, 69.37609039468567573 ) ) ;
#29202=CARTESIAN_POINT ( 'NONE',  ( 18.67979575497194134, -10.72451020669871369, 80.83442372801901854 ) ) ;
#29204=CARTESIAN_POINT ( 'NONE',  ( 13.97604488694527802, 13.89961937509977652, 84.37390960531433848 ) ) ;
#29205=CARTESIAN_POINT ( 'NONE',  ( -0.05219959533937732626, 21.53943276465977519, 67.50109039468568994 ) ) ;
#29206=CARTESIAN_POINT ( 'NONE',  ( 5.153800228976615827, -19.02544592524334988, 100.2094237280190043 ) ) ;
#29207=CARTESIAN_POINT ( 'NONE',  ( -5.153800228976328057, -19.02544592524343514, 72.29057627198102409 ) ) ;
#29208=CARTESIAN_POINT ( 'NONE',  ( -0.05219959533909027116, -19.03943276465977164, 97.49890960531436690 ) ) ;
#29209=CARTESIAN_POINT ( 'NONE',  ( 5.153800228976335163, 19.02544592524342804, 74.79057627198103830 ) ) ;
#29210=CARTESIAN_POINT ( 'NONE',  ( 18.22780087662123805, -5.499999999999976019, 78.51763182126894947 ) ) ;
#29211=CARTESIAN_POINT ( 'NONE',  ( -9.564922557960796823, -16.46253265017161027, 62.08224293864769550 ) ) ;
#29212=EDGE_CURVE ( 'NONE', #105512, #73939, #66461, .T. ) ;
#29213=CARTESIAN_POINT ( 'NONE',  ( 10.81492255796078972, 18.62759615963270932, 99.58224293864770971 ) ) ;
#29214=CARTESIAN_POINT ( 'NONE',  ( 14.29746914071037800, 8.314922557961029526, 91.66775706135234714 ) ) ;
#29216=CARTESIAN_POINT ( 'NONE',  ( -19.02544592524334988, -5.153800228976617603, 43.95942372801899012 ) ) ;
#29217=CARTESIAN_POINT ( 'NONE',  ( 19.02544592524343514, -5.153800228976328945, 78.54057627198099567 ) ) ;
#29218=CARTESIAN_POINT ( 'NONE',  ( -8.224510206698948167, 14.34966873604960824, 70.41557627198102409 ) ) ;
#29219=CARTESIAN_POINT ( 'NONE',  ( 12.06949235617757843, -12.14591786802309237, 108.1239096053143811 ) ) ;
#29220=CARTESIAN_POINT ( 'NONE',  ( 19.02544592524343514, -5.153800228976328945, 113.5405762719810241 ) ) ;
#29221=CARTESIAN_POINT ( 'NONE',  ( 0.05219959533909260263, 19.03943276465977164, 109.9989096053143669 ) ) ;
#29222=CARTESIAN_POINT ( 'NONE',  ( -0.05219959533909027116, -19.03943276465977164, 82.49890960531436690 ) ) ;
#29223=CARTESIAN_POINT ( 'NONE',  ( -19.05341960407617563, 5.049401038297882671, 28.54275706135232937 ) ) ;
#29224=CARTESIAN_POINT ( 'NONE',  ( -0.05219959533934338120, 16.53943276465976808, 92.50109039468567573 ) ) ;
#29225=CARTESIAN_POINT ( 'NONE',  ( -19.03943276465977164, 0.05219959533909376836, 76.24890960531435269 ) ) ;
#29226=CARTESIAN_POINT ( 'NONE',  ( 21.53943276465977519, 0.05219959533937863772, 56.25109039468568284 ) ) ;
#29227=CARTESIAN_POINT ( 'NONE',  ( 21.55341960407610458, 5.719274019375980345, 28.95724293864769905 ) ) ;
#29228=CARTESIAN_POINT ( 'NONE',  ( -5.719274019375978568, 21.55341960407610458, 115.2072429386476955 ) ) ;
#29229=CARTESIAN_POINT ( 'NONE',  ( -15.80617190586745835, -15.72974639402198527, 66.87390960531436690 ) ) ;
#29230=CARTESIAN_POINT ( 'NONE',  ( -14.29746914071049879, 8.314922557960819915, 90.83224293864769550 ) ) ;
#29231=CARTESIAN_POINT ( 'NONE',  ( -9.564922557961040184, 16.46253265017147172, 57.91775706135233293 ) ) ;
#29232=CARTESIAN_POINT ( 'NONE',  ( 19.03943276465977164, -0.05219959533909143690, 28.74890960531435624 ) ) ;
#29233=CARTESIAN_POINT ( 'NONE',  ( -0.05219959533909027116, -19.03943276465977164, 82.49890960531436690 ) ) ;
#29234=CARTESIAN_POINT ( 'NONE',  ( -19.03943276465977164, 0.05219959533909376836, 81.24890960531436690 ) ) ;
#29236=CARTESIAN_POINT ( 'NONE',  ( 14.29746914071049879, -8.314922557960816363, 103.3322429386476955 ) ) ;
#29238=CARTESIAN_POINT ( 'NONE',  ( 14.29746914071049879, -8.314922557960816363, 23.33224293864769194 ) ) ;
#29239=CARTESIAN_POINT ( 'NONE',  ( -16.55341960407617563, 4.379528057220093196, 28.54275706135234358 ) ) ;
#29240=CARTESIAN_POINT ( 'NONE',  ( 10.72451020669871369, 18.67979575497193778, 92.08442372801901854 ) ) ;
#29241=CARTESIAN_POINT ( 'NONE',  ( -5.153800228976328057, -19.02544592524343514, 107.2905762719810383 ) ) ;
#29242=CARTESIAN_POINT ( 'NONE',  ( -21.53943276465977519, -0.05219959533937600094, 18.75109039468568639 ) ) ;
#29243=CARTESIAN_POINT ( 'NONE',  ( 19.05341960407611168, 5.049401038298154454, 38.95724293864767418 ) ) ;
#29244=CARTESIAN_POINT ( 'NONE',  ( -14.34966873604972548, 8.224510206698743886, 43.33442372801901143 ) ) ;
#29245=CARTESIAN_POINT ( 'NONE',  ( 9.474510206698729675, 16.51473224551082808, 112.0844237280190043 ) ) ;
#29246=CARTESIAN_POINT ( 'NONE',  ( -9.564922557960796823, -16.46253265017161027, 32.08224293864769550 ) ) ;
#29247=CARTESIAN_POINT ( 'NONE',  ( 12.06949235617757843, -12.14591786802309237, 93.12390960531436690 ) ) ;
#29248=CARTESIAN_POINT ( 'NONE',  ( 21.52544592524344225, -5.823673210054117533, 98.54057627198105251 ) ) ;
#29249=CARTESIAN_POINT ( 'NONE',  ( -0.05219959533936034679, 19.03943276465977164, 72.50109039468566152 ) ) ;
#29251=CARTESIAN_POINT ( 'NONE',  ( -0.05219959533937732626, 21.53943276465977519, 22.50109039468567573 ) ) ;
#29252=CARTESIAN_POINT ( 'NONE',  ( -9.564922557960796823, -16.46253265017161027, 22.08224293864768839 ) ) ;
#29253=CARTESIAN_POINT ( 'NONE',  ( -0.05219959533909027116, -19.03943276465977164, 92.49890960531436690 ) ) ;
#29254=CARTESIAN_POINT ( 'NONE',  ( 17.31747979337949772, -6.344076630961069441, 111.1205513193481949 ) ) ;
#29255=CARTESIAN_POINT ( 'NONE',  ( 13.97604488694527802, 13.89961937509977652, 84.37390960531433848 ) ) ;
#29256=CARTESIAN_POINT ( 'NONE',  ( -5.823673210054431948, 21.52544592524334988, 27.70942372801901854 ) ) ;
#29257=CARTESIAN_POINT ( 'NONE',  ( -12.14591786802309592, -12.06949235617757132, 81.87390960531435269 ) ) ;
#29258=CARTESIAN_POINT ( 'NONE',  ( -5.153800228976328057, -19.02544592524343514, 77.29057627198099567 ) ) ;
#29259=CARTESIAN_POINT ( 'NONE',  ( 13.97604488694548053, -13.89961937509957401, 30.62609039468566863 ) ) ;
#29260=CARTESIAN_POINT ( 'NONE',  ( -16.52544592524335698, -4.483927247898792601, 48.95942372801902565 ) ) ;
#29261=CARTESIAN_POINT ( 'NONE',  ( 5.049401038297881783, 19.05341960407617563, 52.29275706135234003 ) ) ;
#29262=CARTESIAN_POINT ( 'NONE',  ( 21.52544592524334988, 5.823673210054432836, 71.45942372801901854 ) ) ;
#29263=CARTESIAN_POINT ( 'NONE',  ( -4.483927247898782831, 16.52544592524335698, 32.70942372801900433 ) ) ;
#29264=CARTESIAN_POINT ( 'NONE',  ( -0.05219959533909027116, -19.03943276465977164, 62.49890960531435979 ) ) ;
#29265=CARTESIAN_POINT ( 'NONE',  ( 16.51473224551083163, -9.474510206698727899, 95.83442372801900433 ) ) ;
#29266=CARTESIAN_POINT ( 'NONE',  ( 16.55341960407618274, -4.379528057220086978, 66.04275706135236135 ) ) ;
#29267=CARTESIAN_POINT ( 'NONE',  ( -15.80617190586768217, 15.72974639402176855, 93.12609039468568994 ) ) ;
#29268=CARTESIAN_POINT ( 'NONE',  ( 16.51473224551083163, -9.474510206698727899, 85.83442372801900433 ) ) ;
#29269=CARTESIAN_POINT ( 'NONE',  ( -5.153800228976328057, -19.02544592524343514, 52.29057627198100988 ) ) ;
#29270=CARTESIAN_POINT ( 'NONE',  ( 15.80617190586746368, 15.72974639402197994, 69.37390960531436690 ) ) ;
#29271=CARTESIAN_POINT ( 'NONE',  ( -16.55341960407611168, -4.379528057220339221, 76.45724293864769550 ) ) ;
#29272=CARTESIAN_POINT ( 'NONE',  ( 5.153800228976615827, -19.02544592524334988, 80.20942372801901854 ) ) ;
#29273=CARTESIAN_POINT ( 'NONE',  ( 17.50000000000000000, -5.499999999999992895, 61.21769037696436300 ) ) ;
#29274=CARTESIAN_POINT ( 'NONE',  ( 5.049401038297881783, 19.05341960407617563, 47.29275706135231161 ) ) ;
#29275=CARTESIAN_POINT ( 'NONE',  ( -8.224510206698735004, -14.34966873604973081, 109.5844237280190328 ) ) ;
#29276=CARTESIAN_POINT ( 'NONE',  ( 16.53943276465976808, -0.05219959533910856209, 68.74890960531435269 ) ) ;
#29277=CARTESIAN_POINT ( 'NONE',  ( -21.52544592524334988, -5.823673210054445271, 108.9594237280190185 ) ) ;
#29279=CARTESIAN_POINT ( 'NONE',  ( 10.72451020669898902, -18.67979575497178502, 112.9155762719810383 ) ) ;
#29280=( BOUNDED_SURFACE ( )  B_SPLINE_SURFACE ( 3, 2, ( 
 ( #178204, #132685, #55840, #117514, #122473, #90153, #43666, #77955, #109295, #106311, #107297, #121482, #108299, #91126, #16305, #14308, #61787, #168969, #76966, #137648, #118, #32467, #29493, #153812, #31470, #199335, #139622, #198336, #1110, #184164, #47643, #17297, #15307, #167997, #183176, #59812, #44658, #152816, #94120, #93122, #62784, #138637, #151836, #124465, #155799, #186162, #45646, #182181, #60800, #75975, #74991, #123457, #170974, #167016, #154807, #135686, #30474, #197358, #92124, #185149, #46639, #169978, #58822, #120490, #105328, #28517, #13326, #136655, #129425, #37432, #50620, #140626, #2116, #160784, #143602, #156808, #158774, #4093, #18300, #99092, #78951, #36420, #190126, #63798, #175963, #189147, #6089, #65772, #67768, #191123, #66768, #35439, #82926, #21269, #81909, #49622, #19291, #97091, #51601, #112281, #159774, #111284, #110290, #113265, #127441, #5086, #173971, #141625, #95118, #172974, #144604, #125470, #3114, #52597, #114258, #174957, #20263, #48638, #34453, #171972, #128429, #33460, #98076, #96112, #187167, #79956, #64790, #157800, #80938, #126451, #188149, #142614, #103110, #54599, #53602, #195131, #147623, #86937, #117275, #84920, #38441, #116273, #26285, #42442, #146600, #72787, #57614, #118286, #194137, #192120, #177963, #115278, #148620, #176972, #71771, #193125, #7083, #55601, #104105, #180965, #22272, #163793, #83923, #145604, #9111, #100097, #130422, #164791, #196142, #39431, #178969, #8093, #56612, #101091, #87927, #162777, #10111, #40436, #25295, #24285, #133441, #119282, #85934, #102108, #179977, #70777, #149614, #69771, #11112, #132446, #134457, #68764, #41445, #161781, #131439, #23276, #28287, #89927, #124228, #123226, #31239, #45413, #181948, #92888, #62552, #154575, #14071, #12119, #167766, #13100, #105100, #168737, #16071, #197124, #184917, #77729, #44426, #165788, #137414, #121249, #91884, #75738, #107066, #88931, #139395, #152581, #74765, #108060, #877, #185924, #199095, #27285, #150623, #47409, #30241, #43431, #153575, #90895, #166786, #73783, #135455, #46401, #76733, #58591, #120257, #60562, #151608, #122238, #136427, #198108, #15072, #183928, #169744, #59574, #182943, #106080, #138409, #200089, #29264, #61557, #97845, #155569, #93891, #17064, #157566, #143362, #113036, #50393, #129190, #95883, #142384, #66539, #1882, #79724, #170743, #78718, #65542, #141393, #32233, #127201, #158547, #33231, #19059, #140394, #112053, #188915, #80706, #3862, #48405, #125237, #173741, #189900, #94890, #110062, #63563, #156574, #35210, #96863, #67532, #171742, #186935, #81679, #20037, #18069, #2881, #144369, #4854, #128203, #51375, #109065, #174728, #36191, #159533, #5856, #64560, #21032, #82685, #190888, #126224, #187920, #49389, #111052, #34221, #172740, #90436, #196662, #114021, #181485, #152122, #175718, #89453, #39952, #25814, #40964, #86459, #165317, #197638, #101623, #13604, #87460, #9635, #75272, #120769, #57138, #150145, #136942, #24810, #180500, #149147, #134984, #182470, #58131, #11647, #164321, #43951, #10637, #72297, #166315, #52364, #71302, #195667, #163312, #119800, #27812, #26810, #148144, #42963, #104626, #151142, #132965, #41972, #105613, #73313, #167301, #12633, #194654, #28797, #88450, #56124, #117806, #133976, #179499, #102636, #118814, #103639, #74298, #135967, #59104, #60097, #16585, #47925, #122756, #46925, #44944, #1393, #78233, #108585, #170262, #137933, #14599, #185435, #79239, #184446, #199617, #121765, #45926, #139904, #155091, #157082, #61083, #183458, #171262, #109579, #106599, #168275, #33735, #93405, #31756, #156082, #198631, #63074, #32750, #94401, #95396, #91407, #124753, #186449, #17578, #140910, #2396, #64075, #172248, #123736, #125745, #18578, #187445, #29772, #48913, #80225, #153095, #110567, #76255, #169258, #107581, #30765, #92412, #154098, #15592, #77250, #138918, #399, #62071, #7362, #143887, #36701, #100380, #111567 ),
 ( #82194, #49900, #83208, #52871, #113542, #141896, #144883, #191394, #37713, #177250, #67052, #69047, #160061, #130712, #68045, #188423, #192406, #175236, #173251, #34726, #159051, #96384, #112555, #19562, #114542, #98362, #35718, #142887, #53888, #158071, #126719, #81206, #190407, #176242, #145879, #6365, #162058, #128710, #21548, #99375, #161058, #174250, #4369, #129697, #23554, #3387, #65062, #22553, #66052, #127720, #51883, #189422, #50897, #84199, #115563, #97365, #38722, #20545, #5368, #40718, #166065, #164075, #11394, #118565, #26561, #87218, #149888, #182222, #179252, #103389, #181243, #148900, #89206, #147904, #27566, #72047, #197397, #167055, #165067, #55880, #71056, #9390, #132722, #194410, #43706, #42720, #150899, #88204, #101369, #12393, #105368, #74055, #133721, #131725, #10390, #117553, #24565, #73064, #135726, #116556, #104382, #58863, #25574, #85202, #56891, #102387, #134736, #195413, #196418, #8382, #120529, #180255, #146890, #70057, #193407, #41725, #57888, #119560, #54882, #39706, #178245, #163058, #86214, #139661, #157, #28556, #31510, #77994, #124507, #63835, #153851, #94159, #46680, #17335, #154848, #75030, #155838, #61826, #59854, #121521, #45685, #136696, #199374, #106351, #1149, #123496, #122513, #29532, #78991, #198377, #13366, #183216, #77005, #62824, #32507, #170020, #48676, #15349, #185189, #186202, #44697, #60838, #90193, #168035, #108339, #184203, #151876, #47684, #93163, #91165, #16345, #109334, #171016, #125508, #138677, #140665, #2157, #187205, #110328, #152854, #14349, #76014, #137689, #107336, #169009, #30513, #92165, #49660, #82968, #5125, #65812, #173014, #160825, #18340, #156845, #79995, #20302, #6128, #176005, #113306, #192163, #158814, #66807, #129466, #64828, #142654, #33498, #141663, #128470, #4133, #95157, #190166, #21311, #96151, #81950, #3155, #174997, #51642, #143642, #36462, #111324, #188188, #98119, #52638, #157840, #34493, #126490, #19331, #159816, #144645, #130465, #80979, #127481, #67811, #191165, #189186, #50659, #7124, #114303, #37474, #99135, #172009, #22313, #83964, #145644, #68806, #112320, #53643, #174010, #35481, #97130, #103150, #164831, #134496, #132486, #55639, #196183, #86976, #177012, #10151, #57655, #38481, #56652, #100138, #101129, #116312, #23314, #117312, #26327, #161819, #119321, #162815, #8133, #181008, #87967, #70817, #102148, #115320, #193165, #163833, #194175, #195171, #25335, #180018, #149655, #146640, #84958, #179008, #40476, #11153, #69811, #24324, #148663, #178001, #72827, #131478, #54637, #39468, #85973, #147663, #9150, #71811, #133479, #118325, #41485, #161476, #67459, #127133, #188839, #112964, #142313, #66467, #173671, #6778, #129117, #189831, #96790, #84613, #3793, #80636, #65470, #144295, #130111, #99790, #37122, #115971, #82614, #190816, #53289, #50324, #128129, #157497, #111979, #52291, #51303, #18990, #113948, #145295, #19967, #5785, #35138, #98781, #175647, #160475, #21966, #158479, #81609, #83617, #176660, #143293, #4779, #174657, #36122, #68457, #191807, #54299, #97774, #159461, #114967, #38137, #20957, #22965, #131129, #146292, #7779, #69463, #95811, #192817, #177659, #73477, #74461, #132134, #134145, #195833, #57305, #72471, #119959, #43124, #12796, #164485, #25979, #136127, #180664, #100783, #165481, #197803, #162466, #135150, #23967, #9802, #24979, #70468, #149308, #181645, #85623, #59269, #71464, #193826, #120938, #104792, #41135, #118981, #39128, #8798, #87622, #133129, #42140, #10802, #103801, #196823, #147309, #166481, #148308, #194820, #150318, #55291, #116963, #179665, #178654, #26977, #11813, #88620, #40116, #58290, #27979, #89618, #151307, #101795, #163482, #86625, #56292, #117975, #102799, #29708, #45863, #62005, #78170, #77187, #186382, #137872, #136878, #139838, #30699, #170199, #337, #168211, #121701, #199551, #109513, #125680, #91340, #156015, #140841, #1327, #138857, #75207, #61021 ),
 ( #183396, #92350, #47860, #153031, #44878, #167236, #14531, #46860, #123671, #64011, #106534, #28734, #63007, #155026, #90371, #13542, #2330, #185368, #154036, #124686, #105551, #15530, #16522, #171195, #187378, #198564, #108520, #31692, #93341, #32684, #94337, #17512, #79170, #152056, #60034, #76192, #122693, #184382, #107516, #169192, #110501, #83143, #33668, #19498, #34662, #80160, #158986, #191330, #172183, #84138, #81143, #3324, #145817, #114475, #50833, #143821, #7300, #18513, #174184, #142824, #128645, #35652, #113476, #6302, #95330, #176178, #158007, #4304, #159995, #48847, #64997, #189356, #157015, #190340, #21482, #20478, #141832, #51816, #98293, #144818, #68985, #126655, #188358, #130649, #5302, #97300, #67980, #49836, #82128, #129634, #52808, #111500, #173186, #66986, #175170, #36636, #37648, #99312, #160996, #22491, #96320, #65986, #127656, #112490, #53825, #118506, #27506, #115500, #26503, #177187, #162998, #178183, #23491, #102327, #134675, #38660, #89148, #24504, #146825, #150837, #57829, #194352, #87158, #12333, #161995, #117493, #86155, #71986, #179190, #56831, #149830, #100316, #119502, #101309, #147845, #103330, #192343, #8319, #132664, #85140, #133661, #165009, #164017, #69995, #195351, #41666, #88145, #73997, #40658, #181183, #10330, #42660, #180196, #131663, #104322, #25513, #9331, #70997, #55820, #148840, #11335, #193345, #73006, #196361, #166006, #54820, #116494, #39648, #120470, #182162, #184146, #169958, #139603, #76946, #155780, #122453, #168950, #93103, #28499, #106292, #197339, #105309, #92104, #167978, #58802, #153792, #185128, #59794, #45627, #43646, #138615, #15287, #107279, #30456, #74973, #151818, #98, #16285, #121463, #136635, #166997, #183155, #61767, #123435, #94100, #198317, #90133, #108280, #46619, #31450, #77936, #13307, #170954, #29476, #44640, #32447, #1089, #137630, #154787, #17277, #91107, #60781, #152796, #62765, #124446, #186142, #47621, #14288, #109275, #75956, #199315, #135667, #78931, #33440, #19272, #187146, #20243, #190108, #50602, #140607, #81891, #128412, #174938, #114236, #4075, #144583, #97073, #67747, #5066, #125450, #6069, #112261, #34433, #49600, #111264, #96093, #172955, #156788, #51583, #173953, #157782, #79936, #129405, #48619, #63778, #110270, #127421, #113248, #82904, #143584, #99071, #65752, #35420, #36401, #171951, #80919, #2097, #95099, #158754, #142595, #18281, #66751, #98055, #3093, #189130, #141606, #159755, #21250, #191102, #52576, #64770, #126432, #175942, #37412, #188129, #160760, #83900, #69749, #166528, #181690, #183675, #23256, #145583, #197849, #74508, #7061, #130400, #60309, #120004, #11860, #182683, #22251, #73525, #136174, #59316, #121985, #115257, #43171, #104838, #28025, #58336, #105827, #29010, #198845, #150364, #135196, #45160, #89667, #68742, #151353, #106816, #192098, #120985, #53580, #195879, #8073, #176950, #38419, #100076, #165527, #161761, #12842, #44168, #196870, #84899, #167514, #90649, #152331, #146578, #13817, #75483, #137156, #131418, #57352, #119027, #180710, #42186, #103846, #27023, #88668, #185651, #139138, #46141, #79458, #1615, #62285, #169479, #157299, #14816, #153315, #76477, #16800, #2617, #172469, #109795, #188645, #155311, #63291, #125961, #61302, #615, #29988, #138154, #124971, #123953, #91627, #186668, #17801, #92627, #78450, #199835, #171478, #48138, #140124, #32967, #107795, #184659, #94621, #49130, #154318, #30980, #122972, #15807, #156300, #141127, #126937, #77468, #47143, #64294, #187659, #108801, #170480, #3599, #110788, #33956, #95614, #168490, #18796, #80441, #142114, #65278, #31970, #50124, #93626, #68260, #145098, #192623, #115779, #85426, #36923, #98585, #147117, #53090, #173472, #37935, #8604, #34945, #146096, #96597, #82416, #97577, #143102, #21770, #54105, #158286, #70277, #144105, #66274, #131945, #177468, #113756, #6581, #193629, #81416, #160279, #5585, #191611 ),
 ( #35931, #162276, #111784, #7580, #83421, #4581, #67265, #127933, #176462, #189635, #161276, #128923, #19775, #129911, #51110, #112769, #174462, #114768, #159265, #20761, #99596, #190624, #52099, #38937, #175452, #22771, #84419, #69266, #130932, #100594, #23776, #133951, #181460, #88426, #196637, #57115, #119776, #152094, #149122, #73289, #151117, #118789, #59078, #117781, #135943, #41949, #167272, #136916, #134959, #25791, #40940, #179475, #102612, #164298, #13578, #12609, #120745, #58106, #71277, #182444, #75245, #43924, #103615, #101598, #180478, #87437, #194630, #42938, #105586, #86435, #74273, #28771, #195642, #55101, #26784, #10613, #104602, #165291, #166290, #178462, #132942, #116771, #39929, #150120, #90409, #163286, #11621, #24787, #148121, #9612, #27786, #56100, #89428, #197613, #72274, #157055, #198603, #156054, #109552, #18552, #95370, #108559, #125720, #185408, #187419, #48887, #186422, #155065, #80200, #60071, #46899, #122730, #138894, #16560, #171233, #170237, #79211, #30739, #29745, #32722, #123711, #63045, #93379, #110542, #91380, #17551, #172223, #77225, #121739, #31731, #154073, #124724, #78207, #139877, #183431, #76229, #44916, #106572, #374, #33708, #168249, #1366, #153069, #14571, #137909, #47898, #199591, #94374, #140880, #61058, #184421, #45901, #2370, #64050, #107554, #169232, #92386, #15567, #62046, #130686, #192380, #129671, #98335, #38698, #3362, #190381, #66027, #82166, #160034, #114515, #113516, #22527, #174223, #173225, #176216, #67025, #6339, #36675, #4342, #158046, #35692, #145854, #162033, #127694, #53863, #177225, #37685, #175210, #111540, #97339, #34701, #68019, #96358, #191368, #112529, #126693, #21521, #23529, #100354, #141871, #83182, #65037, #188397, #128684, #19536, #49875, #84174, #115537, #159025, #144856, #189394, #99350, #20518, #7336, #143862, #81181, #52845, #142863, #161033, #69021, #51856, #50871, #5341, #133697, #196395, #119536, #120504, #178219, #180232, #41701, #103366, #118542, #166040, #89181, #58837, #10367, #72024, #182195, #26537, #146864, #11370, #43680, #8356, #181219, #70031, #55855, #71032, #116531, #195389, #27540, #131700, #117529, #179227, #102363, #40693, #163034, #57864, #165044, #164052, #86191, #74030, #193381, #54857, #39683, #56867, #42695, #150873, #88181, #105342, #149865, #73040, #104356, #101345, #25551, #24541, #147881, #134712, #87195, #9367, #12367, #135701, #132699, #197372, #194388, #167029, #85175, #148876, #138652, #168011, #44672, #15322, #109310, #152830, #29507, #90167, #75989, #169994, #185164, #187182, #91141, #151850, #1125, #63813, #139637, #110305, #46655, #123472, #76981, #186177, #28531, #133, #62799, #124481, #125486, #121496, #108314, #31485, #93137, #61802, #170989, #32482, #2132, #153827, #154822, #48653, #16320, #13341, #77970, #75005, #136670, #47659, #198352, #199349, #14324, #59826, #94135, #155814, #183190, #106325, #60814, #137662, #122488, #17312, #30489, #78967, #184179, #45661, #140642, #107312, #168985, #92140, #36435, #129439, #95133, #37446, #80953, #65786, #82940, #171987, #126466, #112295, #79972, #113280, #144618, #143615, #33475, #174971, #21283, #67782, #7097, #97105, #99106, #190140, #160798, #98090, #18315, #22286, #5099, #127455, #158789, #111300, #130436, #156823, #191138, #6102, #192135, #68779, #81923, #83937, #20277, #145618, #53616, #159788, #128443, #141640, #3130, #66782, #96126, #173985, #51615, #52611, #114273, #175977, #4107, #64805, #188164, #49637, #172989, #34467, #157815, #19305, #189161, #142628, #50634, #35454, #165801, #150636, #11126, #86951, #84933, #70791, #8106, #179992, #69784, #164805, #85947, #100110, #148635, #197137, #73796, #115292, #56626, #176985, #38455, #102123, #131452, #23289, #57629, #88945, #147636, #10125, #101104, #87941, #132459, #196156, #194150, #118300, #161794, #134471, #27298, #41459, #12132, #9125, #133455, #72801, #117288, #119296 ),
 ( #103124, #146614, #26300, #135469, #193139, #149628, #54612, #55614, #162790, #116286, #25309, #180979, #177976, #39444, #178982, #24299, #40449, #42455, #163807, #71785, #195145, #104119, #183941, #29277, #138422, #45426, #123239, #16084, #181962, #124242, #167779, #152594, #169757, #58604, #13114, #199108, #166799, #105113, #61570, #76747, #107079, #168751, #198121, #74778, #30254, #139408, #182956, #59588, #120270, #106093, #200102, #15086, #17077, #121262, #43444, #31252, #93904, #92902, #140407, #184930, #153588, #91897, #77742, #28300, #46415, #154588, #890, #155582, #151621, #108073, #62565, #185937, #47422, #109078, #170757, #32246, #78731, #89940, #136440, #44439, #90909, #14085, #75751, #137428, #60575, #122251, #172752, #187932, #33244, #112065, #144380, #63576, #37208, #34233, #156586, #98864, #67543, #3875, #96874, #160559, #171755, #127213, #95895, #81691, #188927, #66550, #159545, #125250, #129201, #111064, #157578, #113047, #1896, #18081, #142396, #110075, #143373, #174739, #173753, #186948, #4865, #51386, #97856, #22049, #50405, #190899, #20048, #52375, #128214, #48419, #114032, #35221, #19071, #80718, #65554, #158558, #189911, #79736, #36202, #21043, #82696, #2893, #175729, #94902, #141405, #64572, #5867, #83700, #126237, #49401, #165564, #132218, #178739, #102881, #38217, #116053, #6860, #115052, #101882, #177742, #68539, #163564, #194903, #69549, #193910, #191890, #55374, #179750, #149388, #86707, #27061, #117044, #40202, #164566, #99873, #39211, #130194, #176744, #25064, #100867, #53374, #148392, #56377, #131213, #9886, #161557, #71546, #133212, #118060, #41220, #84695, #23050, #26060, #87703, #192904, #146375, #7862, #54381, #10884, #72554, #103884, #162549, #24053, #134232, #180747, #195917, #145378, #57392, #119065, #42223, #85709, #147395, #8883, #70551, #123012, #123996, #181728, #183714, #45200, #106854, #122023, #169519, #92669, #62326, #13854, #75521, #185694, #30027, #150403, #14857, #47184, #11899, #184698, #73562, #59355, #74546, #120041, #198882, #31019, #135235, #108843, #121024, #43209, #170524, #154357, #90687, #168529, #88707, #58374, #137196, #182721, #91665, #60349, #153355, #46182, #196907, #15850, #197886, #44206, #199877, #104876, #166565, #29047, #28064, #76518, #61341, #138194, #89705, #107835, #77509, #139180, #151391, #656, #12881, #136211, #105865, #167552, #152369, #100392, #6375, #190417, #5378, #67062, #51893, #128720, #112565, #145891, #68055, #113552, #35728, #23566, #78495, #16845, #115575, #175246, #63339, #7374, #160071, #99387, #129709, #97375, #50907, #36711, #38734, #54894, #159061, #85214, #70069, #130726, #191405, #1661, #98373, #125016, #161070, #186712, #84211, #21558, #140168, #52882, #116568, #193419, #32013, #176254, #93670, #155355, #83218, #174260, #20555, #177262, #8394, #144893, #114556, #82205, #69059, #37725, #162070, #22565, #192418, #143897, #53900, #146904, #131737, #75042, #72059, #196430, #74067, #180267, #182234, #40730, #58875, #165079, #90205, #59866, #57900, #148912, #164087, #102400, #25586, #87230, #136708, #135738, #43719, #119572, #194422, #105380, #198389, #167067, #26573, #24577, #41737, #10402, #117565, #181255, #28568, #9402, #197409, #151888, #56903, #178257, #149900, #133733, #104394, #88216, #42732, #101381, #55892, #39718, #163072, #118577, #13378, #86226, #11407, #147916, #71068, #132734, #166077, #179265, #27580, #103401, #195426, #73076, #134748, #120541, #89218, #150911, #12405, #31522, #48687, #108353, #110340, #172021, #109346, #78006, #18352, #183228, #170032, #45697, #61838, #139673, #94171, #93175, #95169, #92178, #154860, #107348, #155850, #77017, #2169, #170, #62836, #121533, #140677, #33510, #186215, #80007, #15361, #1161, #17347, #123508, #125520, #184215, #63848, #16358, #156857, #3167, #124520, #153863, #169021, #30526, #138689, #185201, #141676, #79003, #187217, #47696, #137701, #44709 ),
 ( #106363, #171028, #46692, #32519, #168047, #29544, #91177, #199386, #152866, #14361, #76026, #60850, #122525, #36475, #126502, #188200, #146653, #129478, #142666, #144658, #190180, #4145, #23327, #64840, #22326, #176017, #84970, #161832, #175011, #192176, #51655, #53657, #115334, #52651, #21324, #49672, #111336, #113319, #189198, #5139, #82982, #37486, #98132, #145656, #97144, #96163, #99148, #159829, #191177, #6141, #127493, #80991, #158827, #68820, #173026, #50673, #177025, #100151, #160837, #67823, #34505, #20315, #157852, #114315, #19343, #83976, #35494, #65824, #7137, #112333, #174023, #81963, #130479, #143655, #66821, #38495, #128484, #116325, #150673, #131491, #85987, #166837, #193178, #86989, #58642, #28338, #180031, #69824, #54651, #89977, #72840, #147676, #87980, #133492, #9164, #8147, #178014, #165840, #119335, #39481, #105151, #118338, #135507, #195184, #197177, #120308, #196196, #164844, #101142, #162828, #56665, #132499, #148676, #26340, #181021, #41500, #88983, #40489, #24337, #42495, #103164, #134510, #149668, #70831, #194188, #102161, #12171, #55653, #117325, #182001, #43484, #104159, #11166, #179021, #163847, #25348, #57668, #10164, #27337, #71824, #73836, #123274, #33277, #110111, #151658, #92937, #13152, #74815, #138455, #106131, #59627, #93939, #125286, #122287, #184965, #137466, #124277, #107116, #32284, #30289, #154625, #136477, #170792, #63611, #16119, #48454, #45462, #169793, #47457, #153626, #155618, #14121, #17114, #200136, #186983, #198157, #31286, #183976, #199146, #75788, #60612, #168787, #171789, #109113, #78765, #77775, #167815, #140442, #121301, #1932, #61605, #182993, #15122, #91934, #90944, #139443, #44476, #29314, #152631, #76784, #46449, #108109, #925, #62599, #185973, #4899, #36236, #21077, #141441, #160591, #66581, #50439, #65590, #127250, #112098, #188963, #172788, #5900, #128246, #173788, #95928, #83731, #2928, #79771, #64607, #143411, #129235, #98897, #97888, #115084, #81726, #189943, #52408, #187967, #35255, #156621, #126270, #51418, #96909, #18116, #113078, #144414, #19104, #174770, #49437, #159580, #82733, #67577, #190931, #34269, #111098, #114067, #175765, #80754, #157613, #142431, #3910, #37241, #22080, #53406, #158592, #20081, #145410, #130227, #6892, #176776, #68570, #191922, #94936, #195950, #38248, #86739, #149420, #72589, #73592, #131246, #133244, #194936, #56412, #71578, #119096, #42253, #11928, #163596, #25097, #135265, #179782, #99903, #164597, #196936, #161588, #134263, #23082, #8915, #24086, #69580, #148424, #180778, #84727, #58404, #70583, #192935, #120070, #103915, #40238, #118092, #146405, #7895, #9919, #132252, #41251, #102913, #26091, #57423, #54412, #165595, #147428, #193943, #116084, #177772, #87735, #39242, #10916, #27093, #100898, #162582, #85741, #88739, #150433, #55406, #117076, #178772, #101914, #60377, #15879, #136239, #91693, #198909, #197913, #124025, #181758, #107863, #123039, #185723, #47213, #45227, #77537, #122049, #139209, #684, #61368, #153384, #43240, #104907, #106881, #167579, #183740, #14885, #169548, #30052, #154384, #13881, #59383, #31047, #168554, #199904, #76546, #44235, #121056, #75548, #62355, #166595, #29073, #28095, #89734, #151420, #138222, #182751, #184725, #105892, #92696, #90712, #12907, #46209, #152395, #74571, #137223, #120708, #43886, #103576, #162239, #23739, #149084, #116736, #70241, #104563, #135903, #132902, #133911, #148082, #134919, #117740, #42898, #40901, #165251, #85388, #181420, #74234, #26745, #59041, #56061, #180438, #58067, #164258, #166245, #24750, #27746, #10572, #197574, #147082, #41910, #194591, #9573, #86397, #71239, #179435, #182407, #119737, #89389, #88383, #178425, #151077, #8566, #12568, #72235, #131909, #25753, #102574, #101556, #150077, #193593, #55064, #39889, #163248, #87399, #195602, #57075, #118749, #11582, #73249, #196596, #117024, #149370, #88689, #181708, #147373, #55354 ),
 ( #194883, #71525, #85686, #105847, #150385, #101860, #103865, #10866, #163544, #182703, #24032, #43189, #135217, #44188, #121005, #134212, #151372, #72536, #12863, #74528, #11881, #180729, #8862, #70529, #195899, #148371, #164547, #42205, #196889, #57374, #104858, #56357, #178719, #58356, #119047, #73544, #165546, #86687, #40181, #118039, #28046, #132198, #9866, #136193, #59335, #120023, #27043, #193889, #179730, #25044, #166547, #133192, #89687, #41200, #102862, #197868, #26040, #87685, #49155, #108824, #167534, #29029, #154338, #122005, #75502, #109821, #141154, #138176, #139160, #153336, #140149, #122994, #48163, #46163, #170503, #90669, #186693, #79485, #31993, #64319, #61323, #185675, #63318, #169501, #171504, #30009, #32993, #15830, #2643, #152351, #47165, #199857, #14837, #91647, #76500, #184680, #125987, #124998, #94647, #93651, #183696, #156327, #187685, #17827, #77490, #13836, #31000, #107817, #106836, #155336, #137176, #198864, #60331, #45182, #92649, #168511, #637, #62307, #123977, #16825, #78476, #1641, #192650, #190651, #81441, #96623, #34971, #173498, #158312, #69294, #68289, #176490, #52127, #126962, #37966, #7608, #99624, #159291, #157327, #112795, #19800, #50151, #113783, #161305, #142140, #129940, #22800, #189662, #110813, #82443, #66299, #143127, #144131, #51135, #175479, #188671, #130960, #33983, #174489, #65303, #36951, #4607, #127959, #172496, #95639, #98613, #111810, #160307, #35956, #97603, #18822, #80466, #191639, #21797, #3624, #20788, #5613, #84446, #67292, #146124, #128950, #83449, #145126, #6610, #53119, #114797, #178490, #194660, #10642, #26814, #25819, #134988, #86464, #85454, #88454, #179504, #118819, #149152, #116799, #70304, #148149, #58135, #74302, #39957, #104630, #89457, #150150, #87465, #23804, #9640, #147144, #180505, #8632, #103644, #24815, #38966, #72303, #135971, #12637, #54133, #195672, #115806, #177496, #40970, #131973, #162304, #196666, #27816, #71307, #133981, #101628, #11651, #132970, #119804, #56129, #57143, #100622, #73317, #166319, #41977, #151146, #117811, #165322, #181489, #102641, #42967, #163317, #193657, #55129, #164326, #197642, #184450, #152126, #105617, #142642, #173998, #168279, #169263, #183462, #173002, #153099, #80966, #76259, #138922, #59108, #19319, #112308, #62075, #97118, #91411, #15596, #96139, #199621, #4120, #60101, #65799, #45930, #35469, #81937, #77254, #29776, #44948, #121769, #106603, #14603, #158801, #157828, #127468, #403, #13608, #189174, #20290, #50647, #107585, #43955, #61088, #137937, #136946, #123740, #120773, #28801, #182474, #167305, #122760, #90440, #30769, #92416, #154102, #185439, #46929, #111313, #75276, #198635, #34481, #22300, #98106, #23302, #114289, #191152, #5113, #25322, #8120, #21297, #84946, #68793, #82955, #102136, #143628, #101117, #54624, #163821, #40464, #53630, #70804, #130451, #132473, #194163, #131466, #100125, #66795, #128458, #192149, #67798, #83951, #161807, #116300, #115306, #24312, #175991, #174985, #177989, #176998, #69798, #38468, #6115, #159802, #37460, #147650, #190154, #129453, #55627, #178996, #39456, #146628, #113294, #99121, #36449, #193152, #144632, #162803, #160812, #51630, #85961, #52626, #145631, #7111, #9138, #117300, #26314, #45441, #86964, #44454, #198134, #107094, #183954, #197153, #14098, #73813, #75766, #137443, #74791, #43459, #168764, #148650, #135483, #11141, #27313, #105128, #59603, #58618, #167792, #119309, #118313, #121276, #12148, #151634, #181977, #149643, #103137, #180994, #90922, #10138, #72815, #199122, #122265, #182970, #120285, #56640, #42471, #180006, #13129, #41473, #136453, #57643, #71799, #166814, #133468, #195159, #164819, #28315, #87954, #134484, #89954, #196171, #104133, #29292, #60590, #165815, #106107, #88960, #152608, #150650, #111079, #109093, #171769, #30267, #49417, #142412, #94916, #127229, #124257, #48434, #126251, #32261, #34249, #92917, #172769 ) ),
 .UNSPECIFIED., .T., .F., .F. ) 
 B_SPLINE_SURFACE_WITH_KNOTS ( ( 4, 3, 4 ),
 ( 3, 2, 2, 2, 2, 2, 2, 2, 2, 2, 2, 2, 2, 2, 2, 2, 2, 2, 2, 2, 2, 2, 2, 2, 2, 2, 2, 2, 2, 2, 2, 2, 2, 2, 2, 2, 2, 2, 2, 2, 2, 2, 2, 2, 2, 2, 2, 2, 2, 2, 2, 2, 2, 2, 2, 2, 2, 2, 2, 2, 2, 2, 2, 2, 2, 2, 2, 2, 2, 2, 2, 2, 2, 2, 2, 2, 2, 2, 2, 2, 2, 2, 2, 2, 2, 2, 2, 2, 2, 2, 2, 2, 2, 2, 2, 2, 2, 2, 2, 2, 2, 2, 2, 2, 2, 2, 2, 2, 2, 2, 2, 2, 2, 2, 2, 2, 2, 2, 2, 2, 2, 2, 2, 2, 2, 2, 2, 2, 2, 2, 2, 2, 2, 2, 2, 2, 2, 2, 2, 2, 2, 2, 2, 2, 2, 2, 2, 2, 2, 2, 2, 2, 2, 2, 2, 2, 2, 2, 2, 2, 2, 2, 2, 2, 2, 2, 2, 2, 2, 2, 2, 2, 2, 2, 2, 2, 2, 2, 2, 2, 2, 2, 2, 2, 2, 2, 2, 2, 2, 2, 2, 2, 2, 2, 2, 2, 2, 2, 2, 2, 2, 2, 2, 2, 2, 2, 2, 2, 2, 2, 2, 2, 2, 2, 2, 2, 2, 2, 2, 2, 2, 2, 2, 2, 2, 2, 2, 2, 3 ),
 ( 0.000000000000000000, 0.5000000000000000000, 1.000000000000000000 ),
 ( 0.000000000000000000, 0.004385964912280701511, 0.008771929824561403022, 0.01315789473684210453, 0.01754385964912280604, 0.02192982456140350755, 0.02631578947368420907, 0.03070175438596491058, 0.03508771929824561209, 0.03947368421052631360, 0.04385964912280701511, 0.04824561403508771662, 0.05263157894736841813, 0.05701754385964911964, 0.06140350877192982115, 0.06578947368421052266, 0.07017543859649122417, 0.07456140350877192569, 0.07894736842105262720, 0.08333333333333332871, 0.08771929824561403022, 0.09210526315789473173, 0.09649122807017543324, 0.1008771929824561348, 0.1052631578947368363, 0.1096491228070175378, 0.1140350877192982393, 0.1184210526315789408, 0.1228070175438596423, 0.1271929824561403577, 0.1315789473684210453, 0.1359649122807017607, 0.1403508771929824483, 0.1447368421052631637, 0.1491228070175438514, 0.1535087719298245668, 0.1578947368421052544, 0.1622807017543859698, 0.1666666666666666574, 0.1710526315789473728, 0.1754385964912280604, 0.1798245614035087758, 0.1842105263157894635, 0.1885964912280701788, 0.1929824561403508665, 0.1973684210526315819, 0.2017543859649122695, 0.2061403508771929849, 0.2105263157894736725, 0.2149122807017543879, 0.2192982456140350755, 0.2236842105263157909, 0.2280701754385964786, 0.2324561403508771940, 0.2368421052631578816, 0.2412280701754385970, 0.2456140350877192846, 0.2500000000000000000, 0.2543859649122807154, 0.2587719298245614308, 0.2631578947368420907, 0.2675438596491228060, 0.2719298245614035214, 0.2763157894736842368, 0.2807017543859648967, 0.2850877192982456121, 0.2894736842105263275, 0.2938596491228070429, 0.2982456140350877027, 0.3026315789473684181, 0.3070175438596491335, 0.3114035087719298489, 0.3157894736842105088, 0.3201754385964912242, 0.3245614035087719396, 0.3289473684210526550, 0.3333333333333333148, 0.3377192982456140302, 0.3421052631578947456, 0.3464912280701754610, 0.3508771929824561209, 0.3552631578947368363, 0.3596491228070175517, 0.3640350877192982670, 0.3684210526315789269, 0.3728070175438596423, 0.3771929824561403577, 0.3815789473684210731, 0.3859649122807017330, 0.3903508771929824483, 0.3947368421052631637, 0.3991228070175438791, 0.4035087719298245390, 0.4078947368421052544, 0.4122807017543859698, 0.4166666666666666852, 0.4210526315789473450, 0.4254385964912280604, 0.4298245614035087758, 0.4342105263157894912, 0.4385964912280701511, 0.4429824561403508665, 0.4473684210526315819, 0.4517543859649122973, 0.4561403508771929571, 0.4605263157894736725, 0.4649122807017543879, 0.4692982456140351033, 0.4736842105263157632, 0.4780701754385964786, 0.4824561403508771940, 0.4868421052631579093, 0.4912280701754385692, 0.4956140350877192846, 0.5000000000000000000, 0.5043859649122807154, 0.5087719298245614308, 0.5131578947368421462, 0.5175438596491228616, 0.5219298245614034659, 0.5263157894736841813, 0.5307017543859648967, 0.5350877192982456121, 0.5394736842105263275, 0.5438596491228070429, 0.5482456140350877583, 0.5526315789473684736, 0.5570175438596490780, 0.5614035087719297934, 0.5657894736842105088, 0.5701754385964912242, 0.5745614035087719396, 0.5789473684210526550, 0.5833333333333333703, 0.5877192982456140857, 0.5921052631578946901, 0.5964912280701754055, 0.6008771929824561209, 0.6052631578947368363, 0.6096491228070175517, 0.6140350877192982670, 0.6184210526315789824, 0.6228070175438596978, 0.6271929824561403022, 0.6315789473684210176, 0.6359649122807017330, 0.6403508771929824483, 0.6447368421052631637, 0.6491228070175438791, 0.6535087719298245945, 0.6578947368421053099, 0.6622807017543859143, 0.6666666666666666297, 0.6710526315789473450, 0.6754385964912280604, 0.6798245614035087758, 0.6842105263157894912, 0.6885964912280702066, 0.6929824561403509220, 0.6973684210526315264, 0.7017543859649122417, 0.7061403508771929571, 0.7105263157894736725, 0.7149122807017543879, 0.7192982456140351033, 0.7236842105263158187, 0.7280701754385965341, 0.7324561403508771384, 0.7368421052631578538, 0.7412280701754385692, 0.7456140350877192846, 0.7500000000000000000, 0.7543859649122807154, 0.7587719298245614308, 0.7631578947368421462, 0.7675438596491228616, 0.7719298245614034659, 0.7763157894736841813, 0.7807017543859648967, 0.7850877192982456121, 0.7894736842105263275, 0.7938596491228070429, 0.7982456140350877583, 0.8026315789473684736, 0.8070175438596490780, 0.8114035087719297934, 0.8157894736842105088, 0.8201754385964912242, 0.8245614035087719396, 0.8289473684210526550, 0.8333333333333333703, 0.8377192982456140857, 0.8421052631578946901, 0.8464912280701754055, 0.8508771929824561209, 0.8552631578947368363, 0.8596491228070175517, 0.8640350877192982670, 0.8684210526315789824, 0.8728070175438596978, 0.8771929824561403022, 0.8815789473684210176, 0.8859649122807017330, 0.8903508771929824483, 0.8947368421052631637, 0.8991228070175438791, 0.9035087719298245945, 0.9078947368421053099, 0.9122807017543859143, 0.9166666666666666297, 0.9210526315789473450, 0.9254385964912280604, 0.9298245614035087758, 0.9342105263157894912, 0.9385964912280702066, 0.9429824561403509220, 0.9473684210526315264, 0.9517543859649122417, 0.9561403508771929571, 0.9605263157894736725, 0.9649122807017543879, 0.9692982456140351033, 0.9736842105263158187, 0.9780701754385965341, 0.9824561403508771384, 0.9868421052631578538, 0.9912280701754385692, 0.9956140350877192846, 1.000000000000000000 ),
 .UNSPECIFIED. ) 
 GEOMETRIC_REPRESENTATION_ITEM ( )  RATIONAL_B_SPLINE_SURFACE ( (
 ( 1.000000000000000000, 0.9659258262890683122, 1.000000000000000000, 0.9659258262890683122, 1.000000000000000000, 0.9659258262890683122, 1.000000000000000000, 0.9659258262890683122, 1.000000000000000000, 0.9659258262890683122, 1.000000000000000000, 0.9659258262890683122, 1.000000000000000000, 0.9659258262890683122, 1.000000000000000000, 0.9659258262890683122, 1.000000000000000000, 0.9659258262890683122, 1.000000000000000000, 0.9659258262890683122, 1.000000000000000000, 0.9659258262890683122, 1.000000000000000000, 0.9659258262890683122, 1.000000000000000000, 0.9659258262890683122, 1.000000000000000000, 0.9659258262890683122, 1.000000000000000000, 0.9659258262890683122, 1.000000000000000000, 0.9659258262890683122, 1.000000000000000000, 0.9659258262890683122, 1.000000000000000000, 0.9659258262890683122, 1.000000000000000000, 0.9659258262890683122, 1.000000000000000000, 0.9659258262890683122, 1.000000000000000000, 0.9659258262890683122, 1.000000000000000000, 0.9659258262890683122, 1.000000000000000000, 0.9659258262890683122, 1.000000000000000000, 0.9659258262890683122, 1.000000000000000000, 0.9659258262890683122, 1.000000000000000000, 0.9659258262890683122, 1.000000000000000000, 0.9659258262890683122, 1.000000000000000000, 0.9659258262890683122, 1.000000000000000000, 0.9659258262890683122, 1.000000000000000000, 0.9659258262890683122, 1.000000000000000000, 0.9659258262890683122, 1.000000000000000000, 0.9659258262890683122, 1.000000000000000000, 0.9659258262890683122, 1.000000000000000000, 0.9659258262890683122, 1.000000000000000000, 0.9659258262890683122, 1.000000000000000000, 0.9659258262890683122, 1.000000000000000000, 0.9659258262890683122, 1.000000000000000000, 0.9659258262890683122, 1.000000000000000000, 0.9659258262890683122, 1.000000000000000000, 0.9659258262890683122, 1.000000000000000000, 0.9659258262890683122, 1.000000000000000000, 0.9659258262890683122, 1.000000000000000000, 0.9659258262890683122, 1.000000000000000000, 0.9659258262890683122, 1.000000000000000000, 0.9659258262890683122, 1.000000000000000000, 0.9659258262890683122, 1.000000000000000000, 0.9659258262890683122, 1.000000000000000000, 0.9659258262890683122, 1.000000000000000000, 0.9659258262890683122, 1.000000000000000000, 0.9659258262890683122, 1.000000000000000000, 0.9659258262890683122, 1.000000000000000000, 0.9659258262890683122, 1.000000000000000000, 0.9659258262890683122, 1.000000000000000000, 0.9659258262890683122, 1.000000000000000000, 0.9659258262890683122, 1.000000000000000000, 0.9659258262890683122, 1.000000000000000000, 0.9659258262890683122, 1.000000000000000000, 0.9659258262890683122, 1.000000000000000000, 0.9659258262890683122, 1.000000000000000000, 0.9659258262890683122, 1.000000000000000000, 0.9659258262890683122, 1.000000000000000000, 0.9659258262890683122, 1.000000000000000000, 0.9659258262890683122, 1.000000000000000000, 0.9659258262890683122, 1.000000000000000000, 0.9659258262890683122, 1.000000000000000000, 0.9659258262890683122, 1.000000000000000000, 0.9659258262890683122, 1.000000000000000000, 0.9659258262890683122, 1.000000000000000000, 0.9659258262890683122, 1.000000000000000000, 0.9659258262890683122, 1.000000000000000000, 0.9659258262890683122, 1.000000000000000000, 0.9659258262890683122, 1.000000000000000000, 0.9659258262890683122, 1.000000000000000000, 0.9659258262890683122, 1.000000000000000000, 0.9659258262890683122, 1.000000000000000000, 0.9659258262890683122, 1.000000000000000000, 0.9659258262890683122, 1.000000000000000000, 0.9659258262890683122, 1.000000000000000000, 0.9659258262890683122, 1.000000000000000000, 0.9659258262890683122, 1.000000000000000000, 0.9659258262890683122, 1.000000000000000000, 0.9659258262890683122, 1.000000000000000000, 0.9659258262890683122, 1.000000000000000000, 0.9659258262890683122, 1.000000000000000000, 0.9659258262890683122, 1.000000000000000000, 0.9659258262890683122, 1.000000000000000000, 0.9659258262890683122, 1.000000000000000000, 0.9659258262890683122, 1.000000000000000000, 0.9659258262890683122, 1.000000000000000000, 0.9659258262890683122, 1.000000000000000000, 0.9659258262890683122, 1.000000000000000000, 0.9659258262890683122, 1.000000000000000000, 0.9659258262890683122, 1.000000000000000000, 0.9659258262890683122, 1.000000000000000000, 0.9659258262890683122, 1.000000000000000000, 0.9659258262890683122, 1.000000000000000000, 0.9659258262890683122, 1.000000000000000000, 0.9659258262890683122, 1.000000000000000000, 0.9659258262890683122, 1.000000000000000000, 0.9659258262890683122, 1.000000000000000000, 0.9659258262890683122, 1.000000000000000000, 0.9659258262890683122, 1.000000000000000000, 0.9659258262890683122, 1.000000000000000000, 0.9659258262890683122, 1.000000000000000000, 0.9659258262890683122, 1.000000000000000000, 0.9659258262890683122, 1.000000000000000000, 0.9659258262890683122, 1.000000000000000000, 0.9659258262890683122, 1.000000000000000000, 0.9659258262890683122, 1.000000000000000000, 0.9659258262890683122, 1.000000000000000000, 0.9659258262890683122, 1.000000000000000000, 0.9659258262890683122, 1.000000000000000000, 0.9659258262890683122, 1.000000000000000000, 0.9659258262890683122, 1.000000000000000000, 0.9659258262890683122, 1.000000000000000000, 0.9659258262890683122, 1.000000000000000000, 0.9659258262890683122, 1.000000000000000000, 0.9659258262890683122, 1.000000000000000000, 0.9659258262890683122, 1.000000000000000000, 0.9659258262890683122, 1.000000000000000000, 0.9659258262890683122, 1.000000000000000000, 0.9659258262890683122, 1.000000000000000000, 0.9659258262890683122, 1.000000000000000000, 0.9659258262890683122, 1.000000000000000000, 0.9659258262890683122, 1.000000000000000000, 0.9659258262890683122, 1.000000000000000000, 0.9659258262890683122, 1.000000000000000000, 0.9659258262890683122, 1.000000000000000000, 0.9659258262890683122, 1.000000000000000000, 0.9659258262890683122, 1.000000000000000000, 0.9659258262890683122, 1.000000000000000000, 0.9659258262890683122, 1.000000000000000000, 0.9659258262890683122, 1.000000000000000000, 0.9659258262890683122, 1.000000000000000000, 0.9659258262890683122, 1.000000000000000000, 0.9659258262890683122, 1.000000000000000000, 0.9659258262890683122, 1.000000000000000000, 0.9659258262890683122, 1.000000000000000000, 0.9659258262890683122, 1.000000000000000000, 0.9659258262890683122, 1.000000000000000000, 0.9659258262890683122, 1.000000000000000000, 0.9659258262890683122, 1.000000000000000000, 0.9659258262890683122, 1.000000000000000000, 0.9659258262890683122, 1.000000000000000000, 0.9659258262890683122, 1.000000000000000000, 0.9659258262890683122, 1.000000000000000000, 0.9659258262890683122, 1.000000000000000000, 0.9659258262890683122, 1.000000000000000000, 0.9659258262890683122, 1.000000000000000000, 0.9659258262890683122, 1.000000000000000000, 0.9659258262890683122, 1.000000000000000000, 0.9659258262890683122, 1.000000000000000000, 0.9659258262890683122, 1.000000000000000000, 0.9659258262890683122, 1.000000000000000000, 0.9659258262890683122, 1.000000000000000000, 0.9659258262890683122, 1.000000000000000000, 0.9659258262890683122, 1.000000000000000000, 0.9659258262890683122, 1.000000000000000000, 0.9659258262890683122, 1.000000000000000000, 0.9659258262890683122, 1.000000000000000000, 0.9659258262890683122, 1.000000000000000000, 0.9659258262890683122, 1.000000000000000000, 0.9659258262890683122, 1.000000000000000000, 0.9659258262890683122, 1.000000000000000000, 0.9659258262890683122, 1.000000000000000000, 0.9659258262890683122, 1.000000000000000000, 0.9659258262890683122, 1.000000000000000000, 0.9659258262890683122, 1.000000000000000000, 0.9659258262890683122, 1.000000000000000000, 0.9659258262890683122, 1.000000000000000000, 0.9659258262890683122, 1.000000000000000000, 0.9659258262890683122, 1.000000000000000000, 0.9659258262890683122, 1.000000000000000000, 0.9659258262890683122, 1.000000000000000000, 0.9659258262890683122, 1.000000000000000000, 0.9659258262890683122, 1.000000000000000000, 0.9659258262890683122, 1.000000000000000000, 0.9659258262890683122, 1.000000000000000000, 0.9659258262890683122, 1.000000000000000000, 0.9659258262890683122, 1.000000000000000000, 0.9659258262890683122, 1.000000000000000000, 0.9659258262890683122, 1.000000000000000000, 0.9659258262890683122, 1.000000000000000000, 0.9659258262890683122, 1.000000000000000000, 0.9659258262890683122, 1.000000000000000000, 0.9659258262890683122, 1.000000000000000000, 0.9659258262890683122, 1.000000000000000000, 0.9659258262890683122, 1.000000000000000000, 0.9659258262890683122, 1.000000000000000000, 0.9659258262890683122, 1.000000000000000000, 0.9659258262890683122, 1.000000000000000000, 0.9659258262890683122, 1.000000000000000000, 0.9659258262890683122, 1.000000000000000000, 0.9659258262890683122, 1.000000000000000000, 0.9659258262890683122, 1.000000000000000000, 0.9659258262890683122, 1.000000000000000000, 0.9659258262890683122, 1.000000000000000000, 0.9659258262890683122, 1.000000000000000000, 0.9659258262890683122, 1.000000000000000000, 0.9659258262890683122, 1.000000000000000000, 0.9659258262890683122, 1.000000000000000000, 0.9659258262890683122, 1.000000000000000000, 0.9659258262890683122, 1.000000000000000000, 0.9659258262890683122, 1.000000000000000000, 0.9659258262890683122, 1.000000000000000000, 0.9659258262890683122, 1.000000000000000000, 0.9659258262890683122, 1.000000000000000000, 0.9659258262890683122, 1.000000000000000000, 0.9659258262890683122, 1.000000000000000000, 0.9659258262890683122, 1.000000000000000000, 0.9659258262890683122, 1.000000000000000000, 0.9659258262890683122, 1.000000000000000000, 0.9659258262890683122, 1.000000000000000000, 0.9659258262890683122, 1.000000000000000000, 0.9659258262890683122, 1.000000000000000000, 0.9659258262890683122, 1.000000000000000000, 0.9659258262890683122, 1.000000000000000000, 0.9659258262890683122, 1.000000000000000000, 0.9659258262890683122, 1.000000000000000000, 0.9659258262890683122, 1.000000000000000000, 0.9659258262890683122, 1.000000000000000000, 0.9659258262890683122, 1.000000000000000000, 0.9659258262890683122, 1.000000000000000000, 0.9659258262890683122, 1.000000000000000000, 0.9659258262890683122, 1.000000000000000000, 0.9659258262890683122, 1.000000000000000000, 0.9659258262890683122, 1.000000000000000000, 0.9659258262890683122, 1.000000000000000000),
 ( 0.3333333333333333703, 0.3219752754296894559, 0.3333333333333333703, 0.3219752754296894559, 0.3333333333333333703, 0.3219752754296894559, 0.3333333333333333703, 0.3219752754296894559, 0.3333333333333333703, 0.3219752754296894559, 0.3333333333333333703, 0.3219752754296894559, 0.3333333333333333703, 0.3219752754296894559, 0.3333333333333333703, 0.3219752754296894559, 0.3333333333333333703, 0.3219752754296894559, 0.3333333333333333703, 0.3219752754296894559, 0.3333333333333333703, 0.3219752754296894559, 0.3333333333333333703, 0.3219752754296894559, 0.3333333333333333703, 0.3219752754296894559, 0.3333333333333333703, 0.3219752754296894559, 0.3333333333333333703, 0.3219752754296894559, 0.3333333333333333703, 0.3219752754296894559, 0.3333333333333333703, 0.3219752754296894559, 0.3333333333333333703, 0.3219752754296894559, 0.3333333333333333703, 0.3219752754296894559, 0.3333333333333333703, 0.3219752754296894559, 0.3333333333333333703, 0.3219752754296894559, 0.3333333333333333703, 0.3219752754296894559, 0.3333333333333333703, 0.3219752754296894559, 0.3333333333333333703, 0.3219752754296894559, 0.3333333333333333703, 0.3219752754296894559, 0.3333333333333333703, 0.3219752754296894559, 0.3333333333333333703, 0.3219752754296894559, 0.3333333333333333703, 0.3219752754296894559, 0.3333333333333333703, 0.3219752754296894559, 0.3333333333333333703, 0.3219752754296894559, 0.3333333333333333703, 0.3219752754296894559, 0.3333333333333333703, 0.3219752754296894559, 0.3333333333333333703, 0.3219752754296894559, 0.3333333333333333703, 0.3219752754296894559, 0.3333333333333333703, 0.3219752754296894559, 0.3333333333333333703, 0.3219752754296894559, 0.3333333333333333703, 0.3219752754296894559, 0.3333333333333333703, 0.3219752754296894559, 0.3333333333333333703, 0.3219752754296894559, 0.3333333333333333703, 0.3219752754296894559, 0.3333333333333333703, 0.3219752754296894559, 0.3333333333333333703, 0.3219752754296894559, 0.3333333333333333703, 0.3219752754296894559, 0.3333333333333333703, 0.3219752754296894559, 0.3333333333333333703, 0.3219752754296894559, 0.3333333333333333703, 0.3219752754296894559, 0.3333333333333333703, 0.3219752754296894559, 0.3333333333333333703, 0.3219752754296894559, 0.3333333333333333703, 0.3219752754296894559, 0.3333333333333333703, 0.3219752754296894559, 0.3333333333333333703, 0.3219752754296894559, 0.3333333333333333703, 0.3219752754296894559, 0.3333333333333333703, 0.3219752754296894559, 0.3333333333333333703, 0.3219752754296894559, 0.3333333333333333703, 0.3219752754296894559, 0.3333333333333333703, 0.3219752754296894559, 0.3333333333333333703, 0.3219752754296894559, 0.3333333333333333703, 0.3219752754296894559, 0.3333333333333333703, 0.3219752754296894559, 0.3333333333333333703, 0.3219752754296894559, 0.3333333333333333703, 0.3219752754296894559, 0.3333333333333333703, 0.3219752754296894559, 0.3333333333333333703, 0.3219752754296894559, 0.3333333333333333703, 0.3219752754296894559, 0.3333333333333333703, 0.3219752754296894559, 0.3333333333333333703, 0.3219752754296894559, 0.3333333333333333703, 0.3219752754296894559, 0.3333333333333333703, 0.3219752754296894559, 0.3333333333333333703, 0.3219752754296894559, 0.3333333333333333703, 0.3219752754296894559, 0.3333333333333333703, 0.3219752754296894559, 0.3333333333333333703, 0.3219752754296894559, 0.3333333333333333703, 0.3219752754296894559, 0.3333333333333333703, 0.3219752754296894559, 0.3333333333333333703, 0.3219752754296894559, 0.3333333333333333703, 0.3219752754296894559, 0.3333333333333333703, 0.3219752754296894559, 0.3333333333333333703, 0.3219752754296894559, 0.3333333333333333703, 0.3219752754296894559, 0.3333333333333333703, 0.3219752754296894559, 0.3333333333333333703, 0.3219752754296894559, 0.3333333333333333703, 0.3219752754296894559, 0.3333333333333333703, 0.3219752754296894559, 0.3333333333333333703, 0.3219752754296894559, 0.3333333333333333703, 0.3219752754296894559, 0.3333333333333333703, 0.3219752754296894559, 0.3333333333333333703, 0.3219752754296894559, 0.3333333333333333703, 0.3219752754296894559, 0.3333333333333333703, 0.3219752754296894559, 0.3333333333333333703, 0.3219752754296894559, 0.3333333333333333703, 0.3219752754296894559, 0.3333333333333333703, 0.3219752754296894559, 0.3333333333333333703, 0.3219752754296894559, 0.3333333333333333703, 0.3219752754296894559, 0.3333333333333333703, 0.3219752754296894559, 0.3333333333333333703, 0.3219752754296894559, 0.3333333333333333703, 0.3219752754296894559, 0.3333333333333333703, 0.3219752754296894559, 0.3333333333333333703, 0.3219752754296894559, 0.3333333333333333703, 0.3219752754296894559, 0.3333333333333333703, 0.3219752754296894559, 0.3333333333333333703, 0.3219752754296894559, 0.3333333333333333703, 0.3219752754296894559, 0.3333333333333333703, 0.3219752754296894559, 0.3333333333333333703, 0.3219752754296894559, 0.3333333333333333703, 0.3219752754296894559, 0.3333333333333333703, 0.3219752754296894559, 0.3333333333333333703, 0.3219752754296894559, 0.3333333333333333703, 0.3219752754296894559, 0.3333333333333333703, 0.3219752754296894559, 0.3333333333333333703, 0.3219752754296894559, 0.3333333333333333703, 0.3219752754296894559, 0.3333333333333333703, 0.3219752754296894559, 0.3333333333333333703, 0.3219752754296894559, 0.3333333333333333703, 0.3219752754296894559, 0.3333333333333333703, 0.3219752754296894559, 0.3333333333333333703, 0.3219752754296894559, 0.3333333333333333703, 0.3219752754296894559, 0.3333333333333333703, 0.3219752754296894559, 0.3333333333333333703, 0.3219752754296894559, 0.3333333333333333703, 0.3219752754296894559, 0.3333333333333333703, 0.3219752754296894559, 0.3333333333333333703, 0.3219752754296894559, 0.3333333333333333703, 0.3219752754296894559, 0.3333333333333333703, 0.3219752754296894559, 0.3333333333333333703, 0.3219752754296894559, 0.3333333333333333703, 0.3219752754296894559, 0.3333333333333333703, 0.3219752754296894559, 0.3333333333333333703, 0.3219752754296894559, 0.3333333333333333703, 0.3219752754296894559, 0.3333333333333333703, 0.3219752754296894559, 0.3333333333333333703, 0.3219752754296894559, 0.3333333333333333703, 0.3219752754296894559, 0.3333333333333333703, 0.3219752754296894559, 0.3333333333333333703, 0.3219752754296894559, 0.3333333333333333703, 0.3219752754296894559, 0.3333333333333333703, 0.3219752754296894559, 0.3333333333333333703, 0.3219752754296894559, 0.3333333333333333703, 0.3219752754296894559, 0.3333333333333333703, 0.3219752754296894559, 0.3333333333333333703, 0.3219752754296894559, 0.3333333333333333703, 0.3219752754296894559, 0.3333333333333333703, 0.3219752754296894559, 0.3333333333333333703, 0.3219752754296894559, 0.3333333333333333703, 0.3219752754296894559, 0.3333333333333333703, 0.3219752754296894559, 0.3333333333333333703, 0.3219752754296894559, 0.3333333333333333703, 0.3219752754296894559, 0.3333333333333333703, 0.3219752754296894559, 0.3333333333333333703, 0.3219752754296894559, 0.3333333333333333703, 0.3219752754296894559, 0.3333333333333333703, 0.3219752754296894559, 0.3333333333333333703, 0.3219752754296894559, 0.3333333333333333703, 0.3219752754296894559, 0.3333333333333333703, 0.3219752754296894559, 0.3333333333333333703, 0.3219752754296894559, 0.3333333333333333703, 0.3219752754296894559, 0.3333333333333333703, 0.3219752754296894559, 0.3333333333333333703, 0.3219752754296894559, 0.3333333333333333703, 0.3219752754296894559, 0.3333333333333333703, 0.3219752754296894559, 0.3333333333333333703, 0.3219752754296894559, 0.3333333333333333703, 0.3219752754296894559, 0.3333333333333333703, 0.3219752754296894559, 0.3333333333333333703, 0.3219752754296894559, 0.3333333333333333703, 0.3219752754296894559, 0.3333333333333333703, 0.3219752754296894559, 0.3333333333333333703, 0.3219752754296894559, 0.3333333333333333703, 0.3219752754296894559, 0.3333333333333333703, 0.3219752754296894559, 0.3333333333333333703, 0.3219752754296894559, 0.3333333333333333703, 0.3219752754296894559, 0.3333333333333333703, 0.3219752754296894559, 0.3333333333333333703, 0.3219752754296894559, 0.3333333333333333703, 0.3219752754296894559, 0.3333333333333333703, 0.3219752754296894559, 0.3333333333333333703, 0.3219752754296894559, 0.3333333333333333703, 0.3219752754296894559, 0.3333333333333333703, 0.3219752754296894559, 0.3333333333333333703, 0.3219752754296894559, 0.3333333333333333703, 0.3219752754296894559, 0.3333333333333333703, 0.3219752754296894559, 0.3333333333333333703, 0.3219752754296894559, 0.3333333333333333703, 0.3219752754296894559, 0.3333333333333333703, 0.3219752754296894559, 0.3333333333333333703, 0.3219752754296894559, 0.3333333333333333703, 0.3219752754296894559, 0.3333333333333333703, 0.3219752754296894559, 0.3333333333333333703, 0.3219752754296894559, 0.3333333333333333703, 0.3219752754296894559, 0.3333333333333333703, 0.3219752754296894559, 0.3333333333333333703, 0.3219752754296894559, 0.3333333333333333703, 0.3219752754296894559, 0.3333333333333333703, 0.3219752754296894559, 0.3333333333333333703, 0.3219752754296894559, 0.3333333333333333703, 0.3219752754296894559, 0.3333333333333333703, 0.3219752754296894559, 0.3333333333333333703, 0.3219752754296894559, 0.3333333333333333703, 0.3219752754296894559, 0.3333333333333333703, 0.3219752754296894559, 0.3333333333333333703, 0.3219752754296894559, 0.3333333333333333703, 0.3219752754296894559, 0.3333333333333333703, 0.3219752754296894559, 0.3333333333333333703, 0.3219752754296894559, 0.3333333333333333703, 0.3219752754296894559, 0.3333333333333333703, 0.3219752754296894559, 0.3333333333333333703, 0.3219752754296894559, 0.3333333333333333703, 0.3219752754296894559, 0.3333333333333333703, 0.3219752754296894559, 0.3333333333333333703, 0.3219752754296894559, 0.3333333333333333703, 0.3219752754296894559, 0.3333333333333333703, 0.3219752754296894559, 0.3333333333333333703, 0.3219752754296894559, 0.3333333333333333703, 0.3219752754296894559, 0.3333333333333333703, 0.3219752754296894559, 0.3333333333333333703, 0.3219752754296894559, 0.3333333333333333703, 0.3219752754296894559, 0.3333333333333333703, 0.3219752754296894559, 0.3333333333333333703, 0.3219752754296894559, 0.3333333333333333703, 0.3219752754296894559, 0.3333333333333333703, 0.3219752754296894559, 0.3333333333333333703, 0.3219752754296894559, 0.3333333333333333703, 0.3219752754296894559, 0.3333333333333333703, 0.3219752754296894559, 0.3333333333333333703, 0.3219752754296894559, 0.3333333333333333703, 0.3219752754296894559, 0.3333333333333333703, 0.3219752754296894559, 0.3333333333333333703, 0.3219752754296894559, 0.3333333333333333703),
 ( 0.3333333333333333703, 0.3219752754296894559, 0.3333333333333333703, 0.3219752754296894559, 0.3333333333333333703, 0.3219752754296894559, 0.3333333333333333703, 0.3219752754296894559, 0.3333333333333333703, 0.3219752754296894559, 0.3333333333333333703, 0.3219752754296894559, 0.3333333333333333703, 0.3219752754296894559, 0.3333333333333333703, 0.3219752754296894559, 0.3333333333333333703, 0.3219752754296894559, 0.3333333333333333703, 0.3219752754296894559, 0.3333333333333333703, 0.3219752754296894559, 0.3333333333333333703, 0.3219752754296894559, 0.3333333333333333703, 0.3219752754296894559, 0.3333333333333333703, 0.3219752754296894559, 0.3333333333333333703, 0.3219752754296894559, 0.3333333333333333703, 0.3219752754296894559, 0.3333333333333333703, 0.3219752754296894559, 0.3333333333333333703, 0.3219752754296894559, 0.3333333333333333703, 0.3219752754296894559, 0.3333333333333333703, 0.3219752754296894559, 0.3333333333333333703, 0.3219752754296894559, 0.3333333333333333703, 0.3219752754296894559, 0.3333333333333333703, 0.3219752754296894559, 0.3333333333333333703, 0.3219752754296894559, 0.3333333333333333703, 0.3219752754296894559, 0.3333333333333333703, 0.3219752754296894559, 0.3333333333333333703, 0.3219752754296894559, 0.3333333333333333703, 0.3219752754296894559, 0.3333333333333333703, 0.3219752754296894559, 0.3333333333333333703, 0.3219752754296894559, 0.3333333333333333703, 0.3219752754296894559, 0.3333333333333333703, 0.3219752754296894559, 0.3333333333333333703, 0.3219752754296894559, 0.3333333333333333703, 0.3219752754296894559, 0.3333333333333333703, 0.3219752754296894559, 0.3333333333333333703, 0.3219752754296894559, 0.3333333333333333703, 0.3219752754296894559, 0.3333333333333333703, 0.3219752754296894559, 0.3333333333333333703, 0.3219752754296894559, 0.3333333333333333703, 0.3219752754296894559, 0.3333333333333333703, 0.3219752754296894559, 0.3333333333333333703, 0.3219752754296894559, 0.3333333333333333703, 0.3219752754296894559, 0.3333333333333333703, 0.3219752754296894559, 0.3333333333333333703, 0.3219752754296894559, 0.3333333333333333703, 0.3219752754296894559, 0.3333333333333333703, 0.3219752754296894559, 0.3333333333333333703, 0.3219752754296894559, 0.3333333333333333703, 0.3219752754296894559, 0.3333333333333333703, 0.3219752754296894559, 0.3333333333333333703, 0.3219752754296894559, 0.3333333333333333703, 0.3219752754296894559, 0.3333333333333333703, 0.3219752754296894559, 0.3333333333333333703, 0.3219752754296894559, 0.3333333333333333703, 0.3219752754296894559, 0.3333333333333333703, 0.3219752754296894559, 0.3333333333333333703, 0.3219752754296894559, 0.3333333333333333703, 0.3219752754296894559, 0.3333333333333333703, 0.3219752754296894559, 0.3333333333333333703, 0.3219752754296894559, 0.3333333333333333703, 0.3219752754296894559, 0.3333333333333333703, 0.3219752754296894559, 0.3333333333333333703, 0.3219752754296894559, 0.3333333333333333703, 0.3219752754296894559, 0.3333333333333333703, 0.3219752754296894559, 0.3333333333333333703, 0.3219752754296894559, 0.3333333333333333703, 0.3219752754296894559, 0.3333333333333333703, 0.3219752754296894559, 0.3333333333333333703, 0.3219752754296894559, 0.3333333333333333703, 0.3219752754296894559, 0.3333333333333333703, 0.3219752754296894559, 0.3333333333333333703, 0.3219752754296894559, 0.3333333333333333703, 0.3219752754296894559, 0.3333333333333333703, 0.3219752754296894559, 0.3333333333333333703, 0.3219752754296894559, 0.3333333333333333703, 0.3219752754296894559, 0.3333333333333333703, 0.3219752754296894559, 0.3333333333333333703, 0.3219752754296894559, 0.3333333333333333703, 0.3219752754296894559, 0.3333333333333333703, 0.3219752754296894559, 0.3333333333333333703, 0.3219752754296894559, 0.3333333333333333703, 0.3219752754296894559, 0.3333333333333333703, 0.3219752754296894559, 0.3333333333333333703, 0.3219752754296894559, 0.3333333333333333703, 0.3219752754296894559, 0.3333333333333333703, 0.3219752754296894559, 0.3333333333333333703, 0.3219752754296894559, 0.3333333333333333703, 0.3219752754296894559, 0.3333333333333333703, 0.3219752754296894559, 0.3333333333333333703, 0.3219752754296894559, 0.3333333333333333703, 0.3219752754296894559, 0.3333333333333333703, 0.3219752754296894559, 0.3333333333333333703, 0.3219752754296894559, 0.3333333333333333703, 0.3219752754296894559, 0.3333333333333333703, 0.3219752754296894559, 0.3333333333333333703, 0.3219752754296894559, 0.3333333333333333703, 0.3219752754296894559, 0.3333333333333333703, 0.3219752754296894559, 0.3333333333333333703, 0.3219752754296894559, 0.3333333333333333703, 0.3219752754296894559, 0.3333333333333333703, 0.3219752754296894559, 0.3333333333333333703, 0.3219752754296894559, 0.3333333333333333703, 0.3219752754296894559, 0.3333333333333333703, 0.3219752754296894559, 0.3333333333333333703, 0.3219752754296894559, 0.3333333333333333703, 0.3219752754296894559, 0.3333333333333333703, 0.3219752754296894559, 0.3333333333333333703, 0.3219752754296894559, 0.3333333333333333703, 0.3219752754296894559, 0.3333333333333333703, 0.3219752754296894559, 0.3333333333333333703, 0.3219752754296894559, 0.3333333333333333703, 0.3219752754296894559, 0.3333333333333333703, 0.3219752754296894559, 0.3333333333333333703, 0.3219752754296894559, 0.3333333333333333703, 0.3219752754296894559, 0.3333333333333333703, 0.3219752754296894559, 0.3333333333333333703, 0.3219752754296894559, 0.3333333333333333703, 0.3219752754296894559, 0.3333333333333333703, 0.3219752754296894559, 0.3333333333333333703, 0.3219752754296894559, 0.3333333333333333703, 0.3219752754296894559, 0.3333333333333333703, 0.3219752754296894559, 0.3333333333333333703, 0.3219752754296894559, 0.3333333333333333703, 0.3219752754296894559, 0.3333333333333333703, 0.3219752754296894559, 0.3333333333333333703, 0.3219752754296894559, 0.3333333333333333703, 0.3219752754296894559, 0.3333333333333333703, 0.3219752754296894559, 0.3333333333333333703, 0.3219752754296894559, 0.3333333333333333703, 0.3219752754296894559, 0.3333333333333333703, 0.3219752754296894559, 0.3333333333333333703, 0.3219752754296894559, 0.3333333333333333703, 0.3219752754296894559, 0.3333333333333333703, 0.3219752754296894559, 0.3333333333333333703, 0.3219752754296894559, 0.3333333333333333703, 0.3219752754296894559, 0.3333333333333333703, 0.3219752754296894559, 0.3333333333333333703, 0.3219752754296894559, 0.3333333333333333703, 0.3219752754296894559, 0.3333333333333333703, 0.3219752754296894559, 0.3333333333333333703, 0.3219752754296894559, 0.3333333333333333703, 0.3219752754296894559, 0.3333333333333333703, 0.3219752754296894559, 0.3333333333333333703, 0.3219752754296894559, 0.3333333333333333703, 0.3219752754296894559, 0.3333333333333333703, 0.3219752754296894559, 0.3333333333333333703, 0.3219752754296894559, 0.3333333333333333703, 0.3219752754296894559, 0.3333333333333333703, 0.3219752754296894559, 0.3333333333333333703, 0.3219752754296894559, 0.3333333333333333703, 0.3219752754296894559, 0.3333333333333333703, 0.3219752754296894559, 0.3333333333333333703, 0.3219752754296894559, 0.3333333333333333703, 0.3219752754296894559, 0.3333333333333333703, 0.3219752754296894559, 0.3333333333333333703, 0.3219752754296894559, 0.3333333333333333703, 0.3219752754296894559, 0.3333333333333333703, 0.3219752754296894559, 0.3333333333333333703, 0.3219752754296894559, 0.3333333333333333703, 0.3219752754296894559, 0.3333333333333333703, 0.3219752754296894559, 0.3333333333333333703, 0.3219752754296894559, 0.3333333333333333703, 0.3219752754296894559, 0.3333333333333333703, 0.3219752754296894559, 0.3333333333333333703, 0.3219752754296894559, 0.3333333333333333703, 0.3219752754296894559, 0.3333333333333333703, 0.3219752754296894559, 0.3333333333333333703, 0.3219752754296894559, 0.3333333333333333703, 0.3219752754296894559, 0.3333333333333333703, 0.3219752754296894559, 0.3333333333333333703, 0.3219752754296894559, 0.3333333333333333703, 0.3219752754296894559, 0.3333333333333333703, 0.3219752754296894559, 0.3333333333333333703, 0.3219752754296894559, 0.3333333333333333703, 0.3219752754296894559, 0.3333333333333333703, 0.3219752754296894559, 0.3333333333333333703, 0.3219752754296894559, 0.3333333333333333703, 0.3219752754296894559, 0.3333333333333333703, 0.3219752754296894559, 0.3333333333333333703, 0.3219752754296894559, 0.3333333333333333703, 0.3219752754296894559, 0.3333333333333333703, 0.3219752754296894559, 0.3333333333333333703, 0.3219752754296894559, 0.3333333333333333703, 0.3219752754296894559, 0.3333333333333333703, 0.3219752754296894559, 0.3333333333333333703, 0.3219752754296894559, 0.3333333333333333703, 0.3219752754296894559, 0.3333333333333333703, 0.3219752754296894559, 0.3333333333333333703, 0.3219752754296894559, 0.3333333333333333703, 0.3219752754296894559, 0.3333333333333333703, 0.3219752754296894559, 0.3333333333333333703, 0.3219752754296894559, 0.3333333333333333703, 0.3219752754296894559, 0.3333333333333333703, 0.3219752754296894559, 0.3333333333333333703, 0.3219752754296894559, 0.3333333333333333703, 0.3219752754296894559, 0.3333333333333333703, 0.3219752754296894559, 0.3333333333333333703, 0.3219752754296894559, 0.3333333333333333703, 0.3219752754296894559, 0.3333333333333333703, 0.3219752754296894559, 0.3333333333333333703, 0.3219752754296894559, 0.3333333333333333703, 0.3219752754296894559, 0.3333333333333333703, 0.3219752754296894559, 0.3333333333333333703, 0.3219752754296894559, 0.3333333333333333703, 0.3219752754296894559, 0.3333333333333333703, 0.3219752754296894559, 0.3333333333333333703, 0.3219752754296894559, 0.3333333333333333703, 0.3219752754296894559, 0.3333333333333333703, 0.3219752754296894559, 0.3333333333333333703, 0.3219752754296894559, 0.3333333333333333703, 0.3219752754296894559, 0.3333333333333333703, 0.3219752754296894559, 0.3333333333333333703, 0.3219752754296894559, 0.3333333333333333703, 0.3219752754296894559, 0.3333333333333333703, 0.3219752754296894559, 0.3333333333333333703, 0.3219752754296894559, 0.3333333333333333703, 0.3219752754296894559, 0.3333333333333333703, 0.3219752754296894559, 0.3333333333333333703, 0.3219752754296894559, 0.3333333333333333703, 0.3219752754296894559, 0.3333333333333333703, 0.3219752754296894559, 0.3333333333333333703, 0.3219752754296894559, 0.3333333333333333703, 0.3219752754296894559, 0.3333333333333333703, 0.3219752754296894559, 0.3333333333333333703, 0.3219752754296894559, 0.3333333333333333703, 0.3219752754296894559, 0.3333333333333333703, 0.3219752754296894559, 0.3333333333333333703, 0.3219752754296894559, 0.3333333333333333703),
 ( 1.000000000000000000, 0.9659258262890683122, 1.000000000000000000, 0.9659258262890683122, 1.000000000000000000, 0.9659258262890683122, 1.000000000000000000, 0.9659258262890683122, 1.000000000000000000, 0.9659258262890683122, 1.000000000000000000, 0.9659258262890683122, 1.000000000000000000, 0.9659258262890683122, 1.000000000000000000, 0.9659258262890683122, 1.000000000000000000, 0.9659258262890683122, 1.000000000000000000, 0.9659258262890683122, 1.000000000000000000, 0.9659258262890683122, 1.000000000000000000, 0.9659258262890683122, 1.000000000000000000, 0.9659258262890683122, 1.000000000000000000, 0.9659258262890683122, 1.000000000000000000, 0.9659258262890683122, 1.000000000000000000, 0.9659258262890683122, 1.000000000000000000, 0.9659258262890683122, 1.000000000000000000, 0.9659258262890683122, 1.000000000000000000, 0.9659258262890683122, 1.000000000000000000, 0.9659258262890683122, 1.000000000000000000, 0.9659258262890683122, 1.000000000000000000, 0.9659258262890683122, 1.000000000000000000, 0.9659258262890683122, 1.000000000000000000, 0.9659258262890683122, 1.000000000000000000, 0.9659258262890683122, 1.000000000000000000, 0.9659258262890683122, 1.000000000000000000, 0.9659258262890683122, 1.000000000000000000, 0.9659258262890683122, 1.000000000000000000, 0.9659258262890683122, 1.000000000000000000, 0.9659258262890683122, 1.000000000000000000, 0.9659258262890683122, 1.000000000000000000, 0.9659258262890683122, 1.000000000000000000, 0.9659258262890683122, 1.000000000000000000, 0.9659258262890683122, 1.000000000000000000, 0.9659258262890683122, 1.000000000000000000, 0.9659258262890683122, 1.000000000000000000, 0.9659258262890683122, 1.000000000000000000, 0.9659258262890683122, 1.000000000000000000, 0.9659258262890683122, 1.000000000000000000, 0.9659258262890683122, 1.000000000000000000, 0.9659258262890683122, 1.000000000000000000, 0.9659258262890683122, 1.000000000000000000, 0.9659258262890683122, 1.000000000000000000, 0.9659258262890683122, 1.000000000000000000, 0.9659258262890683122, 1.000000000000000000, 0.9659258262890683122, 1.000000000000000000, 0.9659258262890683122, 1.000000000000000000, 0.9659258262890683122, 1.000000000000000000, 0.9659258262890683122, 1.000000000000000000, 0.9659258262890683122, 1.000000000000000000, 0.9659258262890683122, 1.000000000000000000, 0.9659258262890683122, 1.000000000000000000, 0.9659258262890683122, 1.000000000000000000, 0.9659258262890683122, 1.000000000000000000, 0.9659258262890683122, 1.000000000000000000, 0.9659258262890683122, 1.000000000000000000, 0.9659258262890683122, 1.000000000000000000, 0.9659258262890683122, 1.000000000000000000, 0.9659258262890683122, 1.000000000000000000, 0.9659258262890683122, 1.000000000000000000, 0.9659258262890683122, 1.000000000000000000, 0.9659258262890683122, 1.000000000000000000, 0.9659258262890683122, 1.000000000000000000, 0.9659258262890683122, 1.000000000000000000, 0.9659258262890683122, 1.000000000000000000, 0.9659258262890683122, 1.000000000000000000, 0.9659258262890683122, 1.000000000000000000, 0.9659258262890683122, 1.000000000000000000, 0.9659258262890683122, 1.000000000000000000, 0.9659258262890683122, 1.000000000000000000, 0.9659258262890683122, 1.000000000000000000, 0.9659258262890683122, 1.000000000000000000, 0.9659258262890683122, 1.000000000000000000, 0.9659258262890683122, 1.000000000000000000, 0.9659258262890683122, 1.000000000000000000, 0.9659258262890683122, 1.000000000000000000, 0.9659258262890683122, 1.000000000000000000, 0.9659258262890683122, 1.000000000000000000, 0.9659258262890683122, 1.000000000000000000, 0.9659258262890683122, 1.000000000000000000, 0.9659258262890683122, 1.000000000000000000, 0.9659258262890683122, 1.000000000000000000, 0.9659258262890683122, 1.000000000000000000, 0.9659258262890683122, 1.000000000000000000, 0.9659258262890683122, 1.000000000000000000, 0.9659258262890683122, 1.000000000000000000, 0.9659258262890683122, 1.000000000000000000, 0.9659258262890683122, 1.000000000000000000, 0.9659258262890683122, 1.000000000000000000, 0.9659258262890683122, 1.000000000000000000, 0.9659258262890683122, 1.000000000000000000, 0.9659258262890683122, 1.000000000000000000, 0.9659258262890683122, 1.000000000000000000, 0.9659258262890683122, 1.000000000000000000, 0.9659258262890683122, 1.000000000000000000, 0.9659258262890683122, 1.000000000000000000, 0.9659258262890683122, 1.000000000000000000, 0.9659258262890683122, 1.000000000000000000, 0.9659258262890683122, 1.000000000000000000, 0.9659258262890683122, 1.000000000000000000, 0.9659258262890683122, 1.000000000000000000, 0.9659258262890683122, 1.000000000000000000, 0.9659258262890683122, 1.000000000000000000, 0.9659258262890683122, 1.000000000000000000, 0.9659258262890683122, 1.000000000000000000, 0.9659258262890683122, 1.000000000000000000, 0.9659258262890683122, 1.000000000000000000, 0.9659258262890683122, 1.000000000000000000, 0.9659258262890683122, 1.000000000000000000, 0.9659258262890683122, 1.000000000000000000, 0.9659258262890683122, 1.000000000000000000, 0.9659258262890683122, 1.000000000000000000, 0.9659258262890683122, 1.000000000000000000, 0.9659258262890683122, 1.000000000000000000, 0.9659258262890683122, 1.000000000000000000, 0.9659258262890683122, 1.000000000000000000, 0.9659258262890683122, 1.000000000000000000, 0.9659258262890683122, 1.000000000000000000, 0.9659258262890683122, 1.000000000000000000, 0.9659258262890683122, 1.000000000000000000, 0.9659258262890683122, 1.000000000000000000, 0.9659258262890683122, 1.000000000000000000, 0.9659258262890683122, 1.000000000000000000, 0.9659258262890683122, 1.000000000000000000, 0.9659258262890683122, 1.000000000000000000, 0.9659258262890683122, 1.000000000000000000, 0.9659258262890683122, 1.000000000000000000, 0.9659258262890683122, 1.000000000000000000, 0.9659258262890683122, 1.000000000000000000, 0.9659258262890683122, 1.000000000000000000, 0.9659258262890683122, 1.000000000000000000, 0.9659258262890683122, 1.000000000000000000, 0.9659258262890683122, 1.000000000000000000, 0.9659258262890683122, 1.000000000000000000, 0.9659258262890683122, 1.000000000000000000, 0.9659258262890683122, 1.000000000000000000, 0.9659258262890683122, 1.000000000000000000, 0.9659258262890683122, 1.000000000000000000, 0.9659258262890683122, 1.000000000000000000, 0.9659258262890683122, 1.000000000000000000, 0.9659258262890683122, 1.000000000000000000, 0.9659258262890683122, 1.000000000000000000, 0.9659258262890683122, 1.000000000000000000, 0.9659258262890683122, 1.000000000000000000, 0.9659258262890683122, 1.000000000000000000, 0.9659258262890683122, 1.000000000000000000, 0.9659258262890683122, 1.000000000000000000, 0.9659258262890683122, 1.000000000000000000, 0.9659258262890683122, 1.000000000000000000, 0.9659258262890683122, 1.000000000000000000, 0.9659258262890683122, 1.000000000000000000, 0.9659258262890683122, 1.000000000000000000, 0.9659258262890683122, 1.000000000000000000, 0.9659258262890683122, 1.000000000000000000, 0.9659258262890683122, 1.000000000000000000, 0.9659258262890683122, 1.000000000000000000, 0.9659258262890683122, 1.000000000000000000, 0.9659258262890683122, 1.000000000000000000, 0.9659258262890683122, 1.000000000000000000, 0.9659258262890683122, 1.000000000000000000, 0.9659258262890683122, 1.000000000000000000, 0.9659258262890683122, 1.000000000000000000, 0.9659258262890683122, 1.000000000000000000, 0.9659258262890683122, 1.000000000000000000, 0.9659258262890683122, 1.000000000000000000, 0.9659258262890683122, 1.000000000000000000, 0.9659258262890683122, 1.000000000000000000, 0.9659258262890683122, 1.000000000000000000, 0.9659258262890683122, 1.000000000000000000, 0.9659258262890683122, 1.000000000000000000, 0.9659258262890683122, 1.000000000000000000, 0.9659258262890683122, 1.000000000000000000, 0.9659258262890683122, 1.000000000000000000, 0.9659258262890683122, 1.000000000000000000, 0.9659258262890683122, 1.000000000000000000, 0.9659258262890683122, 1.000000000000000000, 0.9659258262890683122, 1.000000000000000000, 0.9659258262890683122, 1.000000000000000000, 0.9659258262890683122, 1.000000000000000000, 0.9659258262890683122, 1.000000000000000000, 0.9659258262890683122, 1.000000000000000000, 0.9659258262890683122, 1.000000000000000000, 0.9659258262890683122, 1.000000000000000000, 0.9659258262890683122, 1.000000000000000000, 0.9659258262890683122, 1.000000000000000000, 0.9659258262890683122, 1.000000000000000000, 0.9659258262890683122, 1.000000000000000000, 0.9659258262890683122, 1.000000000000000000, 0.9659258262890683122, 1.000000000000000000, 0.9659258262890683122, 1.000000000000000000, 0.9659258262890683122, 1.000000000000000000, 0.9659258262890683122, 1.000000000000000000, 0.9659258262890683122, 1.000000000000000000, 0.9659258262890683122, 1.000000000000000000, 0.9659258262890683122, 1.000000000000000000, 0.9659258262890683122, 1.000000000000000000, 0.9659258262890683122, 1.000000000000000000, 0.9659258262890683122, 1.000000000000000000, 0.9659258262890683122, 1.000000000000000000, 0.9659258262890683122, 1.000000000000000000, 0.9659258262890683122, 1.000000000000000000, 0.9659258262890683122, 1.000000000000000000, 0.9659258262890683122, 1.000000000000000000, 0.9659258262890683122, 1.000000000000000000, 0.9659258262890683122, 1.000000000000000000, 0.9659258262890683122, 1.000000000000000000, 0.9659258262890683122, 1.000000000000000000, 0.9659258262890683122, 1.000000000000000000, 0.9659258262890683122, 1.000000000000000000, 0.9659258262890683122, 1.000000000000000000, 0.9659258262890683122, 1.000000000000000000, 0.9659258262890683122, 1.000000000000000000, 0.9659258262890683122, 1.000000000000000000, 0.9659258262890683122, 1.000000000000000000, 0.9659258262890683122, 1.000000000000000000, 0.9659258262890683122, 1.000000000000000000, 0.9659258262890683122, 1.000000000000000000, 0.9659258262890683122, 1.000000000000000000, 0.9659258262890683122, 1.000000000000000000, 0.9659258262890683122, 1.000000000000000000, 0.9659258262890683122, 1.000000000000000000, 0.9659258262890683122, 1.000000000000000000, 0.9659258262890683122, 1.000000000000000000, 0.9659258262890683122, 1.000000000000000000, 0.9659258262890683122, 1.000000000000000000, 0.9659258262890683122, 1.000000000000000000, 0.9659258262890683122, 1.000000000000000000, 0.9659258262890683122, 1.000000000000000000),
 ( 0.3333333333333333703, 0.3219752754296894559, 0.3333333333333333703, 0.3219752754296894559, 0.3333333333333333703, 0.3219752754296894559, 0.3333333333333333703, 0.3219752754296894559, 0.3333333333333333703, 0.3219752754296894559, 0.3333333333333333703, 0.3219752754296894559, 0.3333333333333333703, 0.3219752754296894559, 0.3333333333333333703, 0.3219752754296894559, 0.3333333333333333703, 0.3219752754296894559, 0.3333333333333333703, 0.3219752754296894559, 0.3333333333333333703, 0.3219752754296894559, 0.3333333333333333703, 0.3219752754296894559, 0.3333333333333333703, 0.3219752754296894559, 0.3333333333333333703, 0.3219752754296894559, 0.3333333333333333703, 0.3219752754296894559, 0.3333333333333333703, 0.3219752754296894559, 0.3333333333333333703, 0.3219752754296894559, 0.3333333333333333703, 0.3219752754296894559, 0.3333333333333333703, 0.3219752754296894559, 0.3333333333333333703, 0.3219752754296894559, 0.3333333333333333703, 0.3219752754296894559, 0.3333333333333333703, 0.3219752754296894559, 0.3333333333333333703, 0.3219752754296894559, 0.3333333333333333703, 0.3219752754296894559, 0.3333333333333333703, 0.3219752754296894559, 0.3333333333333333703, 0.3219752754296894559, 0.3333333333333333703, 0.3219752754296894559, 0.3333333333333333703, 0.3219752754296894559, 0.3333333333333333703, 0.3219752754296894559, 0.3333333333333333703, 0.3219752754296894559, 0.3333333333333333703, 0.3219752754296894559, 0.3333333333333333703, 0.3219752754296894559, 0.3333333333333333703, 0.3219752754296894559, 0.3333333333333333703, 0.3219752754296894559, 0.3333333333333333703, 0.3219752754296894559, 0.3333333333333333703, 0.3219752754296894559, 0.3333333333333333703, 0.3219752754296894559, 0.3333333333333333703, 0.3219752754296894559, 0.3333333333333333703, 0.3219752754296894559, 0.3333333333333333703, 0.3219752754296894559, 0.3333333333333333703, 0.3219752754296894559, 0.3333333333333333703, 0.3219752754296894559, 0.3333333333333333703, 0.3219752754296894559, 0.3333333333333333703, 0.3219752754296894559, 0.3333333333333333703, 0.3219752754296894559, 0.3333333333333333703, 0.3219752754296894559, 0.3333333333333333703, 0.3219752754296894559, 0.3333333333333333703, 0.3219752754296894559, 0.3333333333333333703, 0.3219752754296894559, 0.3333333333333333703, 0.3219752754296894559, 0.3333333333333333703, 0.3219752754296894559, 0.3333333333333333703, 0.3219752754296894559, 0.3333333333333333703, 0.3219752754296894559, 0.3333333333333333703, 0.3219752754296894559, 0.3333333333333333703, 0.3219752754296894559, 0.3333333333333333703, 0.3219752754296894559, 0.3333333333333333703, 0.3219752754296894559, 0.3333333333333333703, 0.3219752754296894559, 0.3333333333333333703, 0.3219752754296894559, 0.3333333333333333703, 0.3219752754296894559, 0.3333333333333333703, 0.3219752754296894559, 0.3333333333333333703, 0.3219752754296894559, 0.3333333333333333703, 0.3219752754296894559, 0.3333333333333333703, 0.3219752754296894559, 0.3333333333333333703, 0.3219752754296894559, 0.3333333333333333703, 0.3219752754296894559, 0.3333333333333333703, 0.3219752754296894559, 0.3333333333333333703, 0.3219752754296894559, 0.3333333333333333703, 0.3219752754296894559, 0.3333333333333333703, 0.3219752754296894559, 0.3333333333333333703, 0.3219752754296894559, 0.3333333333333333703, 0.3219752754296894559, 0.3333333333333333703, 0.3219752754296894559, 0.3333333333333333703, 0.3219752754296894559, 0.3333333333333333703, 0.3219752754296894559, 0.3333333333333333703, 0.3219752754296894559, 0.3333333333333333703, 0.3219752754296894559, 0.3333333333333333703, 0.3219752754296894559, 0.3333333333333333703, 0.3219752754296894559, 0.3333333333333333703, 0.3219752754296894559, 0.3333333333333333703, 0.3219752754296894559, 0.3333333333333333703, 0.3219752754296894559, 0.3333333333333333703, 0.3219752754296894559, 0.3333333333333333703, 0.3219752754296894559, 0.3333333333333333703, 0.3219752754296894559, 0.3333333333333333703, 0.3219752754296894559, 0.3333333333333333703, 0.3219752754296894559, 0.3333333333333333703, 0.3219752754296894559, 0.3333333333333333703, 0.3219752754296894559, 0.3333333333333333703, 0.3219752754296894559, 0.3333333333333333703, 0.3219752754296894559, 0.3333333333333333703, 0.3219752754296894559, 0.3333333333333333703, 0.3219752754296894559, 0.3333333333333333703, 0.3219752754296894559, 0.3333333333333333703, 0.3219752754296894559, 0.3333333333333333703, 0.3219752754296894559, 0.3333333333333333703, 0.3219752754296894559, 0.3333333333333333703, 0.3219752754296894559, 0.3333333333333333703, 0.3219752754296894559, 0.3333333333333333703, 0.3219752754296894559, 0.3333333333333333703, 0.3219752754296894559, 0.3333333333333333703, 0.3219752754296894559, 0.3333333333333333703, 0.3219752754296894559, 0.3333333333333333703, 0.3219752754296894559, 0.3333333333333333703, 0.3219752754296894559, 0.3333333333333333703, 0.3219752754296894559, 0.3333333333333333703, 0.3219752754296894559, 0.3333333333333333703, 0.3219752754296894559, 0.3333333333333333703, 0.3219752754296894559, 0.3333333333333333703, 0.3219752754296894559, 0.3333333333333333703, 0.3219752754296894559, 0.3333333333333333703, 0.3219752754296894559, 0.3333333333333333703, 0.3219752754296894559, 0.3333333333333333703, 0.3219752754296894559, 0.3333333333333333703, 0.3219752754296894559, 0.3333333333333333703, 0.3219752754296894559, 0.3333333333333333703, 0.3219752754296894559, 0.3333333333333333703, 0.3219752754296894559, 0.3333333333333333703, 0.3219752754296894559, 0.3333333333333333703, 0.3219752754296894559, 0.3333333333333333703, 0.3219752754296894559, 0.3333333333333333703, 0.3219752754296894559, 0.3333333333333333703, 0.3219752754296894559, 0.3333333333333333703, 0.3219752754296894559, 0.3333333333333333703, 0.3219752754296894559, 0.3333333333333333703, 0.3219752754296894559, 0.3333333333333333703, 0.3219752754296894559, 0.3333333333333333703, 0.3219752754296894559, 0.3333333333333333703, 0.3219752754296894559, 0.3333333333333333703, 0.3219752754296894559, 0.3333333333333333703, 0.3219752754296894559, 0.3333333333333333703, 0.3219752754296894559, 0.3333333333333333703, 0.3219752754296894559, 0.3333333333333333703, 0.3219752754296894559, 0.3333333333333333703, 0.3219752754296894559, 0.3333333333333333703, 0.3219752754296894559, 0.3333333333333333703, 0.3219752754296894559, 0.3333333333333333703, 0.3219752754296894559, 0.3333333333333333703, 0.3219752754296894559, 0.3333333333333333703, 0.3219752754296894559, 0.3333333333333333703, 0.3219752754296894559, 0.3333333333333333703, 0.3219752754296894559, 0.3333333333333333703, 0.3219752754296894559, 0.3333333333333333703, 0.3219752754296894559, 0.3333333333333333703, 0.3219752754296894559, 0.3333333333333333703, 0.3219752754296894559, 0.3333333333333333703, 0.3219752754296894559, 0.3333333333333333703, 0.3219752754296894559, 0.3333333333333333703, 0.3219752754296894559, 0.3333333333333333703, 0.3219752754296894559, 0.3333333333333333703, 0.3219752754296894559, 0.3333333333333333703, 0.3219752754296894559, 0.3333333333333333703, 0.3219752754296894559, 0.3333333333333333703, 0.3219752754296894559, 0.3333333333333333703, 0.3219752754296894559, 0.3333333333333333703, 0.3219752754296894559, 0.3333333333333333703, 0.3219752754296894559, 0.3333333333333333703, 0.3219752754296894559, 0.3333333333333333703, 0.3219752754296894559, 0.3333333333333333703, 0.3219752754296894559, 0.3333333333333333703, 0.3219752754296894559, 0.3333333333333333703, 0.3219752754296894559, 0.3333333333333333703, 0.3219752754296894559, 0.3333333333333333703, 0.3219752754296894559, 0.3333333333333333703, 0.3219752754296894559, 0.3333333333333333703, 0.3219752754296894559, 0.3333333333333333703, 0.3219752754296894559, 0.3333333333333333703, 0.3219752754296894559, 0.3333333333333333703, 0.3219752754296894559, 0.3333333333333333703, 0.3219752754296894559, 0.3333333333333333703, 0.3219752754296894559, 0.3333333333333333703, 0.3219752754296894559, 0.3333333333333333703, 0.3219752754296894559, 0.3333333333333333703, 0.3219752754296894559, 0.3333333333333333703, 0.3219752754296894559, 0.3333333333333333703, 0.3219752754296894559, 0.3333333333333333703, 0.3219752754296894559, 0.3333333333333333703, 0.3219752754296894559, 0.3333333333333333703, 0.3219752754296894559, 0.3333333333333333703, 0.3219752754296894559, 0.3333333333333333703, 0.3219752754296894559, 0.3333333333333333703, 0.3219752754296894559, 0.3333333333333333703, 0.3219752754296894559, 0.3333333333333333703, 0.3219752754296894559, 0.3333333333333333703, 0.3219752754296894559, 0.3333333333333333703, 0.3219752754296894559, 0.3333333333333333703, 0.3219752754296894559, 0.3333333333333333703, 0.3219752754296894559, 0.3333333333333333703, 0.3219752754296894559, 0.3333333333333333703, 0.3219752754296894559, 0.3333333333333333703, 0.3219752754296894559, 0.3333333333333333703, 0.3219752754296894559, 0.3333333333333333703, 0.3219752754296894559, 0.3333333333333333703, 0.3219752754296894559, 0.3333333333333333703, 0.3219752754296894559, 0.3333333333333333703, 0.3219752754296894559, 0.3333333333333333703, 0.3219752754296894559, 0.3333333333333333703, 0.3219752754296894559, 0.3333333333333333703, 0.3219752754296894559, 0.3333333333333333703, 0.3219752754296894559, 0.3333333333333333703, 0.3219752754296894559, 0.3333333333333333703, 0.3219752754296894559, 0.3333333333333333703, 0.3219752754296894559, 0.3333333333333333703, 0.3219752754296894559, 0.3333333333333333703, 0.3219752754296894559, 0.3333333333333333703, 0.3219752754296894559, 0.3333333333333333703, 0.3219752754296894559, 0.3333333333333333703, 0.3219752754296894559, 0.3333333333333333703, 0.3219752754296894559, 0.3333333333333333703, 0.3219752754296894559, 0.3333333333333333703, 0.3219752754296894559, 0.3333333333333333703, 0.3219752754296894559, 0.3333333333333333703, 0.3219752754296894559, 0.3333333333333333703, 0.3219752754296894559, 0.3333333333333333703, 0.3219752754296894559, 0.3333333333333333703, 0.3219752754296894559, 0.3333333333333333703, 0.3219752754296894559, 0.3333333333333333703, 0.3219752754296894559, 0.3333333333333333703, 0.3219752754296894559, 0.3333333333333333703, 0.3219752754296894559, 0.3333333333333333703, 0.3219752754296894559, 0.3333333333333333703, 0.3219752754296894559, 0.3333333333333333703, 0.3219752754296894559, 0.3333333333333333703, 0.3219752754296894559, 0.3333333333333333703, 0.3219752754296894559, 0.3333333333333333703, 0.3219752754296894559, 0.3333333333333333703, 0.3219752754296894559, 0.3333333333333333703, 0.3219752754296894559, 0.3333333333333333703),
 ( 0.3333333333333333703, 0.3219752754296894559, 0.3333333333333333703, 0.3219752754296894559, 0.3333333333333333703, 0.3219752754296894559, 0.3333333333333333703, 0.3219752754296894559, 0.3333333333333333703, 0.3219752754296894559, 0.3333333333333333703, 0.3219752754296894559, 0.3333333333333333703, 0.3219752754296894559, 0.3333333333333333703, 0.3219752754296894559, 0.3333333333333333703, 0.3219752754296894559, 0.3333333333333333703, 0.3219752754296894559, 0.3333333333333333703, 0.3219752754296894559, 0.3333333333333333703, 0.3219752754296894559, 0.3333333333333333703, 0.3219752754296894559, 0.3333333333333333703, 0.3219752754296894559, 0.3333333333333333703, 0.3219752754296894559, 0.3333333333333333703, 0.3219752754296894559, 0.3333333333333333703, 0.3219752754296894559, 0.3333333333333333703, 0.3219752754296894559, 0.3333333333333333703, 0.3219752754296894559, 0.3333333333333333703, 0.3219752754296894559, 0.3333333333333333703, 0.3219752754296894559, 0.3333333333333333703, 0.3219752754296894559, 0.3333333333333333703, 0.3219752754296894559, 0.3333333333333333703, 0.3219752754296894559, 0.3333333333333333703, 0.3219752754296894559, 0.3333333333333333703, 0.3219752754296894559, 0.3333333333333333703, 0.3219752754296894559, 0.3333333333333333703, 0.3219752754296894559, 0.3333333333333333703, 0.3219752754296894559, 0.3333333333333333703, 0.3219752754296894559, 0.3333333333333333703, 0.3219752754296894559, 0.3333333333333333703, 0.3219752754296894559, 0.3333333333333333703, 0.3219752754296894559, 0.3333333333333333703, 0.3219752754296894559, 0.3333333333333333703, 0.3219752754296894559, 0.3333333333333333703, 0.3219752754296894559, 0.3333333333333333703, 0.3219752754296894559, 0.3333333333333333703, 0.3219752754296894559, 0.3333333333333333703, 0.3219752754296894559, 0.3333333333333333703, 0.3219752754296894559, 0.3333333333333333703, 0.3219752754296894559, 0.3333333333333333703, 0.3219752754296894559, 0.3333333333333333703, 0.3219752754296894559, 0.3333333333333333703, 0.3219752754296894559, 0.3333333333333333703, 0.3219752754296894559, 0.3333333333333333703, 0.3219752754296894559, 0.3333333333333333703, 0.3219752754296894559, 0.3333333333333333703, 0.3219752754296894559, 0.3333333333333333703, 0.3219752754296894559, 0.3333333333333333703, 0.3219752754296894559, 0.3333333333333333703, 0.3219752754296894559, 0.3333333333333333703, 0.3219752754296894559, 0.3333333333333333703, 0.3219752754296894559, 0.3333333333333333703, 0.3219752754296894559, 0.3333333333333333703, 0.3219752754296894559, 0.3333333333333333703, 0.3219752754296894559, 0.3333333333333333703, 0.3219752754296894559, 0.3333333333333333703, 0.3219752754296894559, 0.3333333333333333703, 0.3219752754296894559, 0.3333333333333333703, 0.3219752754296894559, 0.3333333333333333703, 0.3219752754296894559, 0.3333333333333333703, 0.3219752754296894559, 0.3333333333333333703, 0.3219752754296894559, 0.3333333333333333703, 0.3219752754296894559, 0.3333333333333333703, 0.3219752754296894559, 0.3333333333333333703, 0.3219752754296894559, 0.3333333333333333703, 0.3219752754296894559, 0.3333333333333333703, 0.3219752754296894559, 0.3333333333333333703, 0.3219752754296894559, 0.3333333333333333703, 0.3219752754296894559, 0.3333333333333333703, 0.3219752754296894559, 0.3333333333333333703, 0.3219752754296894559, 0.3333333333333333703, 0.3219752754296894559, 0.3333333333333333703, 0.3219752754296894559, 0.3333333333333333703, 0.3219752754296894559, 0.3333333333333333703, 0.3219752754296894559, 0.3333333333333333703, 0.3219752754296894559, 0.3333333333333333703, 0.3219752754296894559, 0.3333333333333333703, 0.3219752754296894559, 0.3333333333333333703, 0.3219752754296894559, 0.3333333333333333703, 0.3219752754296894559, 0.3333333333333333703, 0.3219752754296894559, 0.3333333333333333703, 0.3219752754296894559, 0.3333333333333333703, 0.3219752754296894559, 0.3333333333333333703, 0.3219752754296894559, 0.3333333333333333703, 0.3219752754296894559, 0.3333333333333333703, 0.3219752754296894559, 0.3333333333333333703, 0.3219752754296894559, 0.3333333333333333703, 0.3219752754296894559, 0.3333333333333333703, 0.3219752754296894559, 0.3333333333333333703, 0.3219752754296894559, 0.3333333333333333703, 0.3219752754296894559, 0.3333333333333333703, 0.3219752754296894559, 0.3333333333333333703, 0.3219752754296894559, 0.3333333333333333703, 0.3219752754296894559, 0.3333333333333333703, 0.3219752754296894559, 0.3333333333333333703, 0.3219752754296894559, 0.3333333333333333703, 0.3219752754296894559, 0.3333333333333333703, 0.3219752754296894559, 0.3333333333333333703, 0.3219752754296894559, 0.3333333333333333703, 0.3219752754296894559, 0.3333333333333333703, 0.3219752754296894559, 0.3333333333333333703, 0.3219752754296894559, 0.3333333333333333703, 0.3219752754296894559, 0.3333333333333333703, 0.3219752754296894559, 0.3333333333333333703, 0.3219752754296894559, 0.3333333333333333703, 0.3219752754296894559, 0.3333333333333333703, 0.3219752754296894559, 0.3333333333333333703, 0.3219752754296894559, 0.3333333333333333703, 0.3219752754296894559, 0.3333333333333333703, 0.3219752754296894559, 0.3333333333333333703, 0.3219752754296894559, 0.3333333333333333703, 0.3219752754296894559, 0.3333333333333333703, 0.3219752754296894559, 0.3333333333333333703, 0.3219752754296894559, 0.3333333333333333703, 0.3219752754296894559, 0.3333333333333333703, 0.3219752754296894559, 0.3333333333333333703, 0.3219752754296894559, 0.3333333333333333703, 0.3219752754296894559, 0.3333333333333333703, 0.3219752754296894559, 0.3333333333333333703, 0.3219752754296894559, 0.3333333333333333703, 0.3219752754296894559, 0.3333333333333333703, 0.3219752754296894559, 0.3333333333333333703, 0.3219752754296894559, 0.3333333333333333703, 0.3219752754296894559, 0.3333333333333333703, 0.3219752754296894559, 0.3333333333333333703, 0.3219752754296894559, 0.3333333333333333703, 0.3219752754296894559, 0.3333333333333333703, 0.3219752754296894559, 0.3333333333333333703, 0.3219752754296894559, 0.3333333333333333703, 0.3219752754296894559, 0.3333333333333333703, 0.3219752754296894559, 0.3333333333333333703, 0.3219752754296894559, 0.3333333333333333703, 0.3219752754296894559, 0.3333333333333333703, 0.3219752754296894559, 0.3333333333333333703, 0.3219752754296894559, 0.3333333333333333703, 0.3219752754296894559, 0.3333333333333333703, 0.3219752754296894559, 0.3333333333333333703, 0.3219752754296894559, 0.3333333333333333703, 0.3219752754296894559, 0.3333333333333333703, 0.3219752754296894559, 0.3333333333333333703, 0.3219752754296894559, 0.3333333333333333703, 0.3219752754296894559, 0.3333333333333333703, 0.3219752754296894559, 0.3333333333333333703, 0.3219752754296894559, 0.3333333333333333703, 0.3219752754296894559, 0.3333333333333333703, 0.3219752754296894559, 0.3333333333333333703, 0.3219752754296894559, 0.3333333333333333703, 0.3219752754296894559, 0.3333333333333333703, 0.3219752754296894559, 0.3333333333333333703, 0.3219752754296894559, 0.3333333333333333703, 0.3219752754296894559, 0.3333333333333333703, 0.3219752754296894559, 0.3333333333333333703, 0.3219752754296894559, 0.3333333333333333703, 0.3219752754296894559, 0.3333333333333333703, 0.3219752754296894559, 0.3333333333333333703, 0.3219752754296894559, 0.3333333333333333703, 0.3219752754296894559, 0.3333333333333333703, 0.3219752754296894559, 0.3333333333333333703, 0.3219752754296894559, 0.3333333333333333703, 0.3219752754296894559, 0.3333333333333333703, 0.3219752754296894559, 0.3333333333333333703, 0.3219752754296894559, 0.3333333333333333703, 0.3219752754296894559, 0.3333333333333333703, 0.3219752754296894559, 0.3333333333333333703, 0.3219752754296894559, 0.3333333333333333703, 0.3219752754296894559, 0.3333333333333333703, 0.3219752754296894559, 0.3333333333333333703, 0.3219752754296894559, 0.3333333333333333703, 0.3219752754296894559, 0.3333333333333333703, 0.3219752754296894559, 0.3333333333333333703, 0.3219752754296894559, 0.3333333333333333703, 0.3219752754296894559, 0.3333333333333333703, 0.3219752754296894559, 0.3333333333333333703, 0.3219752754296894559, 0.3333333333333333703, 0.3219752754296894559, 0.3333333333333333703, 0.3219752754296894559, 0.3333333333333333703, 0.3219752754296894559, 0.3333333333333333703, 0.3219752754296894559, 0.3333333333333333703, 0.3219752754296894559, 0.3333333333333333703, 0.3219752754296894559, 0.3333333333333333703, 0.3219752754296894559, 0.3333333333333333703, 0.3219752754296894559, 0.3333333333333333703, 0.3219752754296894559, 0.3333333333333333703, 0.3219752754296894559, 0.3333333333333333703, 0.3219752754296894559, 0.3333333333333333703, 0.3219752754296894559, 0.3333333333333333703, 0.3219752754296894559, 0.3333333333333333703, 0.3219752754296894559, 0.3333333333333333703, 0.3219752754296894559, 0.3333333333333333703, 0.3219752754296894559, 0.3333333333333333703, 0.3219752754296894559, 0.3333333333333333703, 0.3219752754296894559, 0.3333333333333333703, 0.3219752754296894559, 0.3333333333333333703, 0.3219752754296894559, 0.3333333333333333703, 0.3219752754296894559, 0.3333333333333333703, 0.3219752754296894559, 0.3333333333333333703, 0.3219752754296894559, 0.3333333333333333703, 0.3219752754296894559, 0.3333333333333333703, 0.3219752754296894559, 0.3333333333333333703, 0.3219752754296894559, 0.3333333333333333703, 0.3219752754296894559, 0.3333333333333333703, 0.3219752754296894559, 0.3333333333333333703, 0.3219752754296894559, 0.3333333333333333703, 0.3219752754296894559, 0.3333333333333333703, 0.3219752754296894559, 0.3333333333333333703, 0.3219752754296894559, 0.3333333333333333703, 0.3219752754296894559, 0.3333333333333333703, 0.3219752754296894559, 0.3333333333333333703, 0.3219752754296894559, 0.3333333333333333703, 0.3219752754296894559, 0.3333333333333333703, 0.3219752754296894559, 0.3333333333333333703, 0.3219752754296894559, 0.3333333333333333703, 0.3219752754296894559, 0.3333333333333333703, 0.3219752754296894559, 0.3333333333333333703, 0.3219752754296894559, 0.3333333333333333703, 0.3219752754296894559, 0.3333333333333333703, 0.3219752754296894559, 0.3333333333333333703, 0.3219752754296894559, 0.3333333333333333703, 0.3219752754296894559, 0.3333333333333333703, 0.3219752754296894559, 0.3333333333333333703, 0.3219752754296894559, 0.3333333333333333703, 0.3219752754296894559, 0.3333333333333333703, 0.3219752754296894559, 0.3333333333333333703, 0.3219752754296894559, 0.3333333333333333703, 0.3219752754296894559, 0.3333333333333333703, 0.3219752754296894559, 0.3333333333333333703, 0.3219752754296894559, 0.3333333333333333703),
 ( 1.000000000000000000, 0.9659258262890683122, 1.000000000000000000, 0.9659258262890683122, 1.000000000000000000, 0.9659258262890683122, 1.000000000000000000, 0.9659258262890683122, 1.000000000000000000, 0.9659258262890683122, 1.000000000000000000, 0.9659258262890683122, 1.000000000000000000, 0.9659258262890683122, 1.000000000000000000, 0.9659258262890683122, 1.000000000000000000, 0.9659258262890683122, 1.000000000000000000, 0.9659258262890683122, 1.000000000000000000, 0.9659258262890683122, 1.000000000000000000, 0.9659258262890683122, 1.000000000000000000, 0.9659258262890683122, 1.000000000000000000, 0.9659258262890683122, 1.000000000000000000, 0.9659258262890683122, 1.000000000000000000, 0.9659258262890683122, 1.000000000000000000, 0.9659258262890683122, 1.000000000000000000, 0.9659258262890683122, 1.000000000000000000, 0.9659258262890683122, 1.000000000000000000, 0.9659258262890683122, 1.000000000000000000, 0.9659258262890683122, 1.000000000000000000, 0.9659258262890683122, 1.000000000000000000, 0.9659258262890683122, 1.000000000000000000, 0.9659258262890683122, 1.000000000000000000, 0.9659258262890683122, 1.000000000000000000, 0.9659258262890683122, 1.000000000000000000, 0.9659258262890683122, 1.000000000000000000, 0.9659258262890683122, 1.000000000000000000, 0.9659258262890683122, 1.000000000000000000, 0.9659258262890683122, 1.000000000000000000, 0.9659258262890683122, 1.000000000000000000, 0.9659258262890683122, 1.000000000000000000, 0.9659258262890683122, 1.000000000000000000, 0.9659258262890683122, 1.000000000000000000, 0.9659258262890683122, 1.000000000000000000, 0.9659258262890683122, 1.000000000000000000, 0.9659258262890683122, 1.000000000000000000, 0.9659258262890683122, 1.000000000000000000, 0.9659258262890683122, 1.000000000000000000, 0.9659258262890683122, 1.000000000000000000, 0.9659258262890683122, 1.000000000000000000, 0.9659258262890683122, 1.000000000000000000, 0.9659258262890683122, 1.000000000000000000, 0.9659258262890683122, 1.000000000000000000, 0.9659258262890683122, 1.000000000000000000, 0.9659258262890683122, 1.000000000000000000, 0.9659258262890683122, 1.000000000000000000, 0.9659258262890683122, 1.000000000000000000, 0.9659258262890683122, 1.000000000000000000, 0.9659258262890683122, 1.000000000000000000, 0.9659258262890683122, 1.000000000000000000, 0.9659258262890683122, 1.000000000000000000, 0.9659258262890683122, 1.000000000000000000, 0.9659258262890683122, 1.000000000000000000, 0.9659258262890683122, 1.000000000000000000, 0.9659258262890683122, 1.000000000000000000, 0.9659258262890683122, 1.000000000000000000, 0.9659258262890683122, 1.000000000000000000, 0.9659258262890683122, 1.000000000000000000, 0.9659258262890683122, 1.000000000000000000, 0.9659258262890683122, 1.000000000000000000, 0.9659258262890683122, 1.000000000000000000, 0.9659258262890683122, 1.000000000000000000, 0.9659258262890683122, 1.000000000000000000, 0.9659258262890683122, 1.000000000000000000, 0.9659258262890683122, 1.000000000000000000, 0.9659258262890683122, 1.000000000000000000, 0.9659258262890683122, 1.000000000000000000, 0.9659258262890683122, 1.000000000000000000, 0.9659258262890683122, 1.000000000000000000, 0.9659258262890683122, 1.000000000000000000, 0.9659258262890683122, 1.000000000000000000, 0.9659258262890683122, 1.000000000000000000, 0.9659258262890683122, 1.000000000000000000, 0.9659258262890683122, 1.000000000000000000, 0.9659258262890683122, 1.000000000000000000, 0.9659258262890683122, 1.000000000000000000, 0.9659258262890683122, 1.000000000000000000, 0.9659258262890683122, 1.000000000000000000, 0.9659258262890683122, 1.000000000000000000, 0.9659258262890683122, 1.000000000000000000, 0.9659258262890683122, 1.000000000000000000, 0.9659258262890683122, 1.000000000000000000, 0.9659258262890683122, 1.000000000000000000, 0.9659258262890683122, 1.000000000000000000, 0.9659258262890683122, 1.000000000000000000, 0.9659258262890683122, 1.000000000000000000, 0.9659258262890683122, 1.000000000000000000, 0.9659258262890683122, 1.000000000000000000, 0.9659258262890683122, 1.000000000000000000, 0.9659258262890683122, 1.000000000000000000, 0.9659258262890683122, 1.000000000000000000, 0.9659258262890683122, 1.000000000000000000, 0.9659258262890683122, 1.000000000000000000, 0.9659258262890683122, 1.000000000000000000, 0.9659258262890683122, 1.000000000000000000, 0.9659258262890683122, 1.000000000000000000, 0.9659258262890683122, 1.000000000000000000, 0.9659258262890683122, 1.000000000000000000, 0.9659258262890683122, 1.000000000000000000, 0.9659258262890683122, 1.000000000000000000, 0.9659258262890683122, 1.000000000000000000, 0.9659258262890683122, 1.000000000000000000, 0.9659258262890683122, 1.000000000000000000, 0.9659258262890683122, 1.000000000000000000, 0.9659258262890683122, 1.000000000000000000, 0.9659258262890683122, 1.000000000000000000, 0.9659258262890683122, 1.000000000000000000, 0.9659258262890683122, 1.000000000000000000, 0.9659258262890683122, 1.000000000000000000, 0.9659258262890683122, 1.000000000000000000, 0.9659258262890683122, 1.000000000000000000, 0.9659258262890683122, 1.000000000000000000, 0.9659258262890683122, 1.000000000000000000, 0.9659258262890683122, 1.000000000000000000, 0.9659258262890683122, 1.000000000000000000, 0.9659258262890683122, 1.000000000000000000, 0.9659258262890683122, 1.000000000000000000, 0.9659258262890683122, 1.000000000000000000, 0.9659258262890683122, 1.000000000000000000, 0.9659258262890683122, 1.000000000000000000, 0.9659258262890683122, 1.000000000000000000, 0.9659258262890683122, 1.000000000000000000, 0.9659258262890683122, 1.000000000000000000, 0.9659258262890683122, 1.000000000000000000, 0.9659258262890683122, 1.000000000000000000, 0.9659258262890683122, 1.000000000000000000, 0.9659258262890683122, 1.000000000000000000, 0.9659258262890683122, 1.000000000000000000, 0.9659258262890683122, 1.000000000000000000, 0.9659258262890683122, 1.000000000000000000, 0.9659258262890683122, 1.000000000000000000, 0.9659258262890683122, 1.000000000000000000, 0.9659258262890683122, 1.000000000000000000, 0.9659258262890683122, 1.000000000000000000, 0.9659258262890683122, 1.000000000000000000, 0.9659258262890683122, 1.000000000000000000, 0.9659258262890683122, 1.000000000000000000, 0.9659258262890683122, 1.000000000000000000, 0.9659258262890683122, 1.000000000000000000, 0.9659258262890683122, 1.000000000000000000, 0.9659258262890683122, 1.000000000000000000, 0.9659258262890683122, 1.000000000000000000, 0.9659258262890683122, 1.000000000000000000, 0.9659258262890683122, 1.000000000000000000, 0.9659258262890683122, 1.000000000000000000, 0.9659258262890683122, 1.000000000000000000, 0.9659258262890683122, 1.000000000000000000, 0.9659258262890683122, 1.000000000000000000, 0.9659258262890683122, 1.000000000000000000, 0.9659258262890683122, 1.000000000000000000, 0.9659258262890683122, 1.000000000000000000, 0.9659258262890683122, 1.000000000000000000, 0.9659258262890683122, 1.000000000000000000, 0.9659258262890683122, 1.000000000000000000, 0.9659258262890683122, 1.000000000000000000, 0.9659258262890683122, 1.000000000000000000, 0.9659258262890683122, 1.000000000000000000, 0.9659258262890683122, 1.000000000000000000, 0.9659258262890683122, 1.000000000000000000, 0.9659258262890683122, 1.000000000000000000, 0.9659258262890683122, 1.000000000000000000, 0.9659258262890683122, 1.000000000000000000, 0.9659258262890683122, 1.000000000000000000, 0.9659258262890683122, 1.000000000000000000, 0.9659258262890683122, 1.000000000000000000, 0.9659258262890683122, 1.000000000000000000, 0.9659258262890683122, 1.000000000000000000, 0.9659258262890683122, 1.000000000000000000, 0.9659258262890683122, 1.000000000000000000, 0.9659258262890683122, 1.000000000000000000, 0.9659258262890683122, 1.000000000000000000, 0.9659258262890683122, 1.000000000000000000, 0.9659258262890683122, 1.000000000000000000, 0.9659258262890683122, 1.000000000000000000, 0.9659258262890683122, 1.000000000000000000, 0.9659258262890683122, 1.000000000000000000, 0.9659258262890683122, 1.000000000000000000, 0.9659258262890683122, 1.000000000000000000, 0.9659258262890683122, 1.000000000000000000, 0.9659258262890683122, 1.000000000000000000, 0.9659258262890683122, 1.000000000000000000, 0.9659258262890683122, 1.000000000000000000, 0.9659258262890683122, 1.000000000000000000, 0.9659258262890683122, 1.000000000000000000, 0.9659258262890683122, 1.000000000000000000, 0.9659258262890683122, 1.000000000000000000, 0.9659258262890683122, 1.000000000000000000, 0.9659258262890683122, 1.000000000000000000, 0.9659258262890683122, 1.000000000000000000, 0.9659258262890683122, 1.000000000000000000, 0.9659258262890683122, 1.000000000000000000, 0.9659258262890683122, 1.000000000000000000, 0.9659258262890683122, 1.000000000000000000, 0.9659258262890683122, 1.000000000000000000, 0.9659258262890683122, 1.000000000000000000, 0.9659258262890683122, 1.000000000000000000, 0.9659258262890683122, 1.000000000000000000, 0.9659258262890683122, 1.000000000000000000, 0.9659258262890683122, 1.000000000000000000, 0.9659258262890683122, 1.000000000000000000, 0.9659258262890683122, 1.000000000000000000, 0.9659258262890683122, 1.000000000000000000, 0.9659258262890683122, 1.000000000000000000, 0.9659258262890683122, 1.000000000000000000, 0.9659258262890683122, 1.000000000000000000, 0.9659258262890683122, 1.000000000000000000, 0.9659258262890683122, 1.000000000000000000, 0.9659258262890683122, 1.000000000000000000, 0.9659258262890683122, 1.000000000000000000, 0.9659258262890683122, 1.000000000000000000, 0.9659258262890683122, 1.000000000000000000, 0.9659258262890683122, 1.000000000000000000, 0.9659258262890683122, 1.000000000000000000, 0.9659258262890683122, 1.000000000000000000, 0.9659258262890683122, 1.000000000000000000, 0.9659258262890683122, 1.000000000000000000, 0.9659258262890683122, 1.000000000000000000, 0.9659258262890683122, 1.000000000000000000, 0.9659258262890683122, 1.000000000000000000, 0.9659258262890683122, 1.000000000000000000, 0.9659258262890683122, 1.000000000000000000, 0.9659258262890683122, 1.000000000000000000, 0.9659258262890683122, 1.000000000000000000, 0.9659258262890683122, 1.000000000000000000, 0.9659258262890683122, 1.000000000000000000, 0.9659258262890683122, 1.000000000000000000, 0.9659258262890683122, 1.000000000000000000) ) ) 
 REPRESENTATION_ITEM ( '' )  SURFACE ( )  );
#29281=CARTESIAN_POINT ( 'NONE',  ( -5.049401038298153566, 19.05341960407611168, 65.20724293864765286 ) ) ;
#29282=CARTESIAN_POINT ( 'NONE',  ( 15.72974639402176855, 15.80617190586768217, 76.87609039468567573 ) ) ;
#29283=CARTESIAN_POINT ( 'NONE',  ( -16.46253265017160317, 9.564922557960807481, 60.83224293864769550 ) ) ;
#29284=CARTESIAN_POINT ( 'NONE',  ( 16.46253265017160672, -9.564922557960803928, 23.33224293864769194 ) ) ;
#29285=CARTESIAN_POINT ( 'NONE',  ( -5.823673210054116645, -21.52544592524344225, 32.29057627198102409 ) ) ;
#29286=CARTESIAN_POINT ( 'NONE',  ( 12.06949235617757843, -12.14591786802309237, 63.12390960531435979 ) ) ;
#29287=CARTESIAN_POINT ( 'NONE',  ( 16.46253265017160672, -9.564922557960803928, 43.33224293864769550 ) ) ;
#29288=CARTESIAN_POINT ( 'NONE',  ( 12.06949235617757843, -12.14591786802309237, 98.12390960531436690 ) ) ;
#29289=CARTESIAN_POINT ( 'NONE',  ( -10.81492255796078084, -18.62759615963271287, 107.0822429386476955 ) ) ;
#29291=CARTESIAN_POINT ( 'NONE',  ( 0.05219959533937995610, -21.53943276465977519, 50.00109039468568994 ) ) ;
#29292=CARTESIAN_POINT ( 'NONE',  ( -13.89961937509977652, 13.97604488694528158, 25.62390960531434558 ) ) ;
#29293=CARTESIAN_POINT ( 'NONE',  ( 14.29746914071037800, 8.314922557961029526, 51.66775706135234714 ) ) ;
#29294=CARTESIAN_POINT ( 'NONE',  ( 18.67979575497178502, 10.72451020669898547, 99.16557627198100988 ) ) ;
#29295=CARTESIAN_POINT ( 'NONE',  ( -21.53943276465977519, 0.05219959533907696930, 91.24890960531436690 ) ) ;
#29296=CARTESIAN_POINT ( 'NONE',  ( 0.05219959533936267826, -19.03943276465977164, 25.00109039468566152 ) ) ;
#29297=CARTESIAN_POINT ( 'NONE',  ( 5.049401038298161559, -19.05341960407611168, 52.70724293864767418 ) ) ;
#29298=CARTESIAN_POINT ( 'NONE',  ( -13.97604488694527625, -13.89961937509977652, 106.8739096053143669 ) ) ;
#29299=CARTESIAN_POINT ( 'NONE',  ( -10.81492255796105439, 18.62759615963255655, 62.91775706135236135 ) ) ;
#29300=CARTESIAN_POINT ( 'NONE',  ( -21.55341960407610458, -5.719274019375992779, 46.45724293864769550 ) ) ;
#29301=CARTESIAN_POINT ( 'NONE',  ( 8.224510206698742110, 14.34966873604972548, 112.0844237280190185 ) ) ;
#29302=CARTESIAN_POINT ( 'NONE',  ( 10.81492255796106328, -18.62759615963255655, 65.41775706135234714 ) ) ;
#29303=CARTESIAN_POINT ( 'NONE',  ( 5.823673210054444382, -21.52544592524334988, 95.20942372801903275 ) ) ;
#29304=CARTESIAN_POINT ( 'NONE',  ( 9.474510206698729675, 16.51473224551082808, 47.08442372801900433 ) ) ;
#29305=CARTESIAN_POINT ( 'NONE',  ( 14.34966873604972726, -8.224510206698740333, 105.8344237280190328 ) ) ;
#29306=CARTESIAN_POINT ( 'NONE',  ( -21.53943276465977519, -0.05219959533937600094, 48.75109039468568284 ) ) ;
#29307=CARTESIAN_POINT ( 'NONE',  ( -19.03943276465977164, 0.05219959533909376836, 56.24890960531435979 ) ) ;
#29308=CARTESIAN_POINT ( 'NONE',  ( 15.80617190586769283, -15.72974639402175789, 110.6260903946857042 ) ) ;
#29309=CARTESIAN_POINT ( 'NONE',  ( -13.89961937509977652, 13.97604488694528158, 115.6239096053143669 ) ) ;
#29310=CARTESIAN_POINT ( 'NONE',  ( -0.05219959533907301413, -21.53943276465977519, 112.4989096053143669 ) ) ;
#29311=CARTESIAN_POINT ( 'NONE',  ( -5.823673210054116645, -21.52544592524344225, 82.29057627198103830 ) ) ;
#29312=CARTESIAN_POINT ( 'NONE',  ( -0.05219959533934338120, 16.53943276465976808, 37.50109039468568284 ) ) ;
#29314=CARTESIAN_POINT ( 'NONE',  ( -5.719274019375978568, 21.55341960407610458, 75.20724293864769550 ) ) ;
#29315=CARTESIAN_POINT ( 'NONE',  ( -16.52544592524335698, -4.483927247898792601, 58.95942372801902565 ) ) ;
#29316=CARTESIAN_POINT ( 'NONE',  ( 8.314922557960818139, 14.29746914071049879, 74.58224293864768129 ) ) ;
#29318=CARTESIAN_POINT ( 'NONE',  ( 19.02544592524334988, 5.153800228976608722, 106.4594237280190185 ) ) ;
#29319=CARTESIAN_POINT ( 'NONE',  ( -15.80617190586745835, -15.72974639402198527, 31.87390960531435979 ) ) ;
#29321=CARTESIAN_POINT ( 'NONE',  ( 16.53943276465976808, 0.05219959533934440121, 36.25109039468567573 ) ) ;
#29322=CARTESIAN_POINT ( 'NONE',  ( -18.62759615963270932, 10.81492255796079327, 105.8322429386476955 ) ) ;
#29323=CARTESIAN_POINT ( 'NONE',  ( -21.53943276465977519, 0.05219959533907696930, 31.24890960531435979 ) ) ;
#29324=CARTESIAN_POINT ( 'NONE',  ( 14.29746914071037800, 8.314922557961029526, 66.66775706135234714 ) ) ;
#29325=B_SPLINE_CURVE_WITH_KNOTS ( 'NONE', 3,
 ( #194899, #102877, #161553, #162545, #71542, #26056 ),
 .UNSPECIFIED., .F., .F.,
 ( 4, 2, 4 ),
 ( 0.007228050697041544029, 0.007608510107495010041, 0.007988969517948476054 ),
 .UNSPECIFIED. ) ;
#29326=CARTESIAN_POINT ( 'NONE',  ( -16.51473224551069308, -9.474510206698971260, 86.66557627198102409 ) ) ;
#29327=CARTESIAN_POINT ( 'NONE',  ( 21.55341960407619695, -5.719274019375665929, 61.04275706135234714 ) ) ;
#29328=CARTESIAN_POINT ( 'NONE',  ( 13.97604488694527802, 13.89961937509977652, 24.37390960531435624 ) ) ;
#29330=CARTESIAN_POINT ( 'NONE',  ( 10.72451020669898902, -18.67979575497178502, 22.91557627198102765 ) ) ;
#29331=ORIENTED_EDGE ( 'NONE', *, *, #187522, .T. ) ;
#29332=CARTESIAN_POINT ( 'NONE',  ( 0.05219959533936267826, -19.03943276465977164, 35.00109039468566863 ) ) ;
#29333=CARTESIAN_POINT ( 'NONE',  ( -16.55341960407617563, 4.379528057220093196, 58.54275706135235424 ) ) ;
#29334=CARTESIAN_POINT ( 'NONE',  ( 19.05341960407611168, 5.049401038298154454, 108.9572429386477097 ) ) ;
#29335=CARTESIAN_POINT ( 'NONE',  ( 19.03943276465977164, -0.05219959533909143690, 73.74890960531435269 ) ) ;
#29336=CARTESIAN_POINT ( 'NONE',  ( -16.53943276465976808, -0.05219959533934237506, 93.75109039468567573 ) ) ;
#29338=CARTESIAN_POINT ( 'NONE',  ( -14.34966873604960291, -8.224510206698953496, 91.66557627198103830 ) ) ;
#29339=CARTESIAN_POINT ( 'NONE',  ( -15.80617190586745835, -15.72974639402198527, 31.87390960531435979 ) ) ;
#29340=CARTESIAN_POINT ( 'NONE',  ( 19.03943276465977164, -0.05219959533909143690, 33.74890960531435979 ) ) ;
#29341=CARTESIAN_POINT ( 'NONE',  ( -8.314922557961024197, 14.29746914071037800, 67.91775706135234714 ) ) ;
#29342=CARTESIAN_POINT ( 'NONE',  ( -18.67979575497193778, 10.72451020669871902, 23.33442372801901499 ) ) ;
#29343=CARTESIAN_POINT ( 'NONE',  ( 0.05219959533936267826, -19.03943276465977164, 75.00109039468566152 ) ) ;
#29344=CARTESIAN_POINT ( 'NONE',  ( 9.474510206698971260, -16.51473224551069308, 37.91557627198102409 ) ) ;
#29345=CARTESIAN_POINT ( 'NONE',  ( 15.72974639402199770, -15.80617190586745480, 73.12390960531436690 ) ) ;
#29346=CARTESIAN_POINT ( 'NONE',  ( 5.153800228976335163, 19.02544592524342804, 109.7905762719810099 ) ) ;
#29347=CARTESIAN_POINT ( 'NONE',  ( 18.62759615963255655, 10.81492255796105972, 86.66775706135234714 ) ) ;
#29348=CARTESIAN_POINT ( 'NONE',  ( -16.51473224551069308, -9.474510206698971260, 61.66557627198103120 ) ) ;
#29349=CARTESIAN_POINT ( 'NONE',  ( -4.379528057220086978, -16.55341960407618274, 44.79275706135234714 ) ) ;
#29350=CARTESIAN_POINT ( 'NONE',  ( 16.51473224551069308, 9.474510206698969483, 54.16557627198103120 ) ) ;
#29351=CARTESIAN_POINT ( 'NONE',  ( 10.72451020669871369, 18.67979575497193778, 82.08442372801901854 ) ) ;
#29352=CARTESIAN_POINT ( 'NONE',  ( -0.05219959533936034679, 19.03943276465977164, 37.50109039468567573 ) ) ;
#29353=CARTESIAN_POINT ( 'NONE',  ( -13.97604488694547697, 13.89961937509957934, 48.12609039468566863 ) ) ;
#29354=CARTESIAN_POINT ( 'NONE',  ( 21.53943276465977519, 0.05219959533937863772, 51.25109039468568994 ) ) ;
#29356=CARTESIAN_POINT ( 'NONE',  ( -19.05341960407617563, 5.049401038297882671, 48.54275706135233293 ) ) ;
#29357=CARTESIAN_POINT ( 'NONE',  ( 5.153800228976335163, 19.02544592524342804, 104.7905762719809957 ) ) ;
#29358=CARTESIAN_POINT ( 'NONE',  ( -19.05341960407611168, -5.049401038298163336, 66.45724293864769550 ) ) ;
#29359=CARTESIAN_POINT ( 'NONE',  ( -16.55341960407611168, -4.379528057220339221, 26.45724293864768839 ) ) ;
#29360=CARTESIAN_POINT ( 'NONE',  ( 5.719274019375991003, -21.55341960407610458, 32.70724293864770260 ) ) ;
#29361=CARTESIAN_POINT ( 'NONE',  ( -18.62759615963255300, -10.81492255796106328, 99.16775706135234714 ) ) ;
#29364=CARTESIAN_POINT ( 'NONE',  ( 15.72974639402176855, 15.80617190586768217, 91.87609039468568994 ) ) ;
#29366=CARTESIAN_POINT ( 'NONE',  ( 0.05219959533909260263, 19.03943276465977164, 39.99890960531436690 ) ) ;
#29367=CARTESIAN_POINT ( 'NONE',  ( 19.02544592524343514, -5.153800228976328945, 108.5405762719810383 ) ) ;
#29369=CARTESIAN_POINT ( 'NONE',  ( 16.53943276465976808, 0.05219959533934440121, 46.25109039468567573 ) ) ;
#29370=CARTESIAN_POINT ( 'NONE',  ( -21.53943276465977519, 0.05219959533907696930, 66.24890960531436690 ) ) ;
#29371=CARTESIAN_POINT ( 'NONE',  ( -14.34966873604960291, -8.224510206698953496, 46.66557627198102409 ) ) ;
#29372=CARTESIAN_POINT ( 'NONE',  ( -4.483927247898539470, -16.52544592524342804, 107.2905762719810525 ) ) ;
#29373=CARTESIAN_POINT ( 'NONE',  ( 0.05219959533909260263, 19.03943276465977164, 109.9989096053143669 ) ) ;
#29374=CARTESIAN_POINT ( 'NONE',  ( -10.81492255796105439, 18.62759615963255655, 27.91775706135234358 ) ) ;
#29375=CARTESIAN_POINT ( 'NONE',  ( -16.46253265017146816, -9.564922557961047289, 39.16775706135234003 ) ) ;
#29376=CARTESIAN_POINT ( 'NONE',  ( -9.564922557960796823, -16.46253265017161027, 27.08224293864769550 ) ) ;
#29377=CARTESIAN_POINT ( 'NONE',  ( -21.53943276465977519, -0.05219959533937600094, 68.75109039468568994 ) ) ;
#29378=CARTESIAN_POINT ( 'NONE',  ( 17.50000000000000355, -5.622605283950867339, 31.18792689403888829 ) ) ;
#29379=CARTESIAN_POINT ( 'NONE',  ( -14.34966873604960291, -8.224510206698953496, 31.66557627198102054 ) ) ;
#29381=CARTESIAN_POINT ( 'NONE',  ( -21.55341960407610458, -5.719274019375992779, 21.45724293864769550 ) ) ;
#29382=CARTESIAN_POINT ( 'NONE',  ( -16.53943276465976808, 0.05219959533911058130, 86.24890960531436690 ) ) ;
#29384=CARTESIAN_POINT ( 'NONE',  ( 9.564922557960805705, 16.46253265017160317, 79.58224293864769550 ) ) ;
#29385=CARTESIAN_POINT ( 'NONE',  ( -8.224510206698948167, 14.34966873604960824, 75.41557627198102409 ) ) ;
#29386=CARTESIAN_POINT ( 'NONE',  ( -13.97604488694547697, 13.89961937509957934, 108.1260903946856331 ) ) ;
#29387=CARTESIAN_POINT ( 'NONE',  ( 15.80617190586746368, 15.72974639402197994, 54.37390960531435979 ) ) ;
#29389=CARTESIAN_POINT ( 'NONE',  ( -16.53943276465976808, 0.05219959533911058130, 111.2489096053143669 ) ) ;
#29390=CARTESIAN_POINT ( 'NONE',  ( -19.05341960407611168, -5.049401038298163336, 66.45724293864769550 ) ) ;
#29391=B_SPLINE_CURVE_WITH_KNOTS ( 'NONE', 3,
 ( #74814, #198156, #42494, #180030, #167814, #136476 ),
 .UNSPECIFIED., .F., .F.,
 ( 4, 2, 4 ),
 ( 0.007228050697041449486, 0.007608510107494925040, 0.007988969517948399726 ),
 .UNSPECIFIED. ) ;
#29392=CARTESIAN_POINT ( 'NONE',  ( 0.05219959533907565091, 21.53943276465977519, 79.99890960531435269 ) ) ;
#29393=CARTESIAN_POINT ( 'NONE',  ( -16.55341960407617563, 4.379528057220093196, 108.5427570613523756 ) ) ;
#29394=CARTESIAN_POINT ( 'NONE',  ( 0.05219959533909260263, 19.03943276465977164, 84.99890960531436690 ) ) ;
#29395=CARTESIAN_POINT ( 'NONE',  ( -9.564922557961040184, 16.46253265017147172, 67.91775706135233293 ) ) ;
#29396=CARTESIAN_POINT ( 'NONE',  ( -0.05219959533937732626, 21.53943276465977519, 97.50109039468567573 ) ) ;
#29397=CARTESIAN_POINT ( 'NONE',  ( -21.53943276465977519, 0.05219959533907696930, 66.24890960531436690 ) ) ;
#29398=CARTESIAN_POINT ( 'NONE',  ( -10.81492255796078084, -18.62759615963271287, 27.08224293864769550 ) ) ;
#29399=CARTESIAN_POINT ( 'NONE',  ( -5.153800228976328057, -19.02544592524343514, 32.29057627198102409 ) ) ;
#29400=CARTESIAN_POINT ( 'NONE',  ( 16.52544592524335698, 4.483927247898782831, 101.4594237280190185 ) ) ;
#29401=CARTESIAN_POINT ( 'NONE',  ( -9.474510206698964154, 16.51473224551069663, 60.41557627198102409 ) ) ;
#29402=CARTESIAN_POINT ( 'NONE',  ( 0.05219959533934541429, -16.53943276465976808, 20.00109039468568639 ) ) ;
#29403=CARTESIAN_POINT ( 'NONE',  ( 16.31925111598457079, 7.325300261831481308, 52.33575461032751974 ) ) ;
#29404=CARTESIAN_POINT ( 'NONE',  ( 10.81492255796106328, -18.62759615963255655, 110.4177570613523756 ) ) ;
#29405=CARTESIAN_POINT ( 'NONE',  ( 12.14591786802309770, 12.06949235617756955, 74.37390960531436690 ) ) ;
#29406=CARTESIAN_POINT ( 'NONE',  ( -21.53943276465977519, 0.05219959533907696930, 106.2489096053143811 ) ) ;
#29407=CARTESIAN_POINT ( 'NONE',  ( -10.81492255796078084, -18.62759615963271287, 97.08224293864770971 ) ) ;
#29409=CARTESIAN_POINT ( 'NONE',  ( -5.823673210054116645, -21.52544592524344225, 62.29057627198102409 ) ) ;
#29410=CARTESIAN_POINT ( 'NONE',  ( -12.06949235617739369, -12.14591786802326823, 84.37609039468570415 ) ) ;
#29411=CARTESIAN_POINT ( 'NONE',  ( -0.05219959533910754901, -16.53943276465976808, 102.4989096053143811 ) ) ;
#29412=CARTESIAN_POINT ( 'NONE',  ( 9.474510206698971260, -16.51473224551069308, 57.91557627198103120 ) ) ;
#29413=CARTESIAN_POINT ( 'NONE',  ( 12.06949235617739724, 12.14591786802326823, 106.8760903946856899 ) ) ;
#29414=CARTESIAN_POINT ( 'NONE',  ( 15.72974639402176855, 15.80617190586768217, 46.87609039468568994 ) ) ;
#29415=CARTESIAN_POINT ( 'NONE',  ( 9.474510206698971260, -16.51473224551069308, 97.91557627198102409 ) ) ;
#29416=CARTESIAN_POINT ( 'NONE',  ( -21.55341960407619339, 5.719274019375674811, 78.54275706135236135 ) ) ;
#29417=CARTESIAN_POINT ( 'NONE',  ( 16.46253265017160672, -9.564922557960803928, 28.33224293864769550 ) ) ;
#29418=CARTESIAN_POINT ( 'NONE',  ( 19.05341960407611168, 5.049401038298154454, 38.95724293864767418 ) ) ;
#29420=CARTESIAN_POINT ( 'NONE',  ( -21.52544592524334988, -5.823673210054445271, 78.95942372801901854 ) ) ;
#29421=CARTESIAN_POINT ( 'NONE',  ( -13.97604488694527625, -13.89961937509977652, 106.8739096053143669 ) ) ;
#29422=CARTESIAN_POINT ( 'NONE',  ( -16.46253265017146816, -9.564922557961047289, 79.16775706135234714 ) ) ;
#29423=CARTESIAN_POINT ( 'NONE',  ( -5.823673210054431948, 21.52544592524334988, 37.70942372801900433 ) ) ;
#29424=CARTESIAN_POINT ( 'NONE',  ( -4.483927247898782831, 16.52544592524335698, 27.70942372801901854 ) ) ;
#29425=CARTESIAN_POINT ( 'NONE',  ( 9.474510206698729675, 16.51473224551082808, 67.08442372801900433 ) ) ;
#29426=CARTESIAN_POINT ( 'NONE',  ( 19.03943276465977164, -0.05219959533909143690, 48.74890960531435979 ) ) ;
#29427=CARTESIAN_POINT ( 'NONE',  ( -13.89961937509957401, -13.97604488694547875, 79.37609039468567573 ) ) ;
#29428=CARTESIAN_POINT ( 'NONE',  ( 14.29746914071049879, -8.314922557960816363, 23.33224293864769194 ) ) ;
#29429=CARTESIAN_POINT ( 'NONE',  ( 19.03943276465977164, 0.05219959533936151252, 81.25109039468567573 ) ) ;
#29430=CARTESIAN_POINT ( 'NONE',  ( -8.224510206698948167, 14.34966873604960824, 40.41557627198103120 ) ) ;
#29431=CARTESIAN_POINT ( 'NONE',  ( -16.51473224551082808, 9.474510206698731452, 63.33442372801900433 ) ) ;
#29432=CARTESIAN_POINT ( 'NONE',  ( 16.53943276465976808, 0.05219959533934440121, 51.25109039468568994 ) ) ;
#29433=CARTESIAN_POINT ( 'NONE',  ( -16.46253265017146816, -9.564922557961047289, 29.16775706135232937 ) ) ;
#29434=CARTESIAN_POINT ( 'NONE',  ( 9.564922557960805705, 16.46253265017160317, 34.58224293864770260 ) ) ;
#29435=CARTESIAN_POINT ( 'NONE',  ( -17.48847506799969054, -5.747544572773811034, 64.17302562156720569 ) ) ;
#29436=CARTESIAN_POINT ( 'NONE',  ( -16.55341960407617563, 4.379528057220093196, 48.54275706135234714 ) ) ;
#29439=CARTESIAN_POINT ( 'NONE',  ( 19.03943276465977164, -0.05219959533909143690, 93.74890960531435269 ) ) ;
#29442=CARTESIAN_POINT ( 'NONE',  ( -9.474510206698720793, -16.51473224551083518, 84.58442372801900433 ) ) ;
#29443=CARTESIAN_POINT ( 'NONE',  ( -5.823673210054116645, -21.52544592524344225, 22.29057627198102765 ) ) ;
#29444=CARTESIAN_POINT ( 'NONE',  ( -16.46253265017146816, -9.564922557961047289, 19.16775706135233293 ) ) ;
#29445=CARTESIAN_POINT ( 'NONE',  ( -16.46253265017146816, -9.564922557961047289, 104.1677570613523329 ) ) ;
#29446=CARTESIAN_POINT ( 'NONE',  ( 4.379528057220339221, -16.55341960407611168, 107.7072429386476955 ) ) ;
#29447=CARTESIAN_POINT ( 'NONE',  ( -16.46253265017160317, 9.564922557960807481, 40.83224293864769550 ) ) ;
#29448=CARTESIAN_POINT ( 'NONE',  ( 15.72974639402199770, -15.80617190586745480, 53.12390960531436690 ) ) ;
#29449=CARTESIAN_POINT ( 'NONE',  ( -21.53943276465977519, 0.05219959533907696930, 56.24890960531436690 ) ) ;
#29450=CARTESIAN_POINT ( 'NONE',  ( -9.564922557960796823, -16.46253265017161027, 27.08224293864769550 ) ) ;
#29451=FACE_OUTER_BOUND ( 'NONE', #110681, .T. ) ;
#29452=CARTESIAN_POINT ( 'NONE',  ( 19.03943276465977164, 0.05219959533936151252, 66.25109039468567573 ) ) ;
#29453=CARTESIAN_POINT ( 'NONE',  ( 16.55341960407611168, 4.379528057220329451, 43.95724293864769550 ) ) ;
#29454=CARTESIAN_POINT ( 'NONE',  ( -18.62759615963270932, 10.81492255796079327, 25.83224293864769194 ) ) ;
#29455=CARTESIAN_POINT ( 'NONE',  ( -18.62759615963255300, -10.81492255796106328, 99.16775706135234714 ) ) ;
#29456=CARTESIAN_POINT ( 'NONE',  ( -5.719274019375978568, 21.55341960407610458, 90.20724293864770971 ) ) ;
#29457=CARTESIAN_POINT ( 'NONE',  ( -5.823673210054431948, 21.52544592524334988, 57.70942372801901143 ) ) ;
#29458=CARTESIAN_POINT ( 'NONE',  ( 21.55341960407619695, -5.719274019375665929, 71.04275706135234714 ) ) ;
#29459=CARTESIAN_POINT ( 'NONE',  ( -19.05341960407611168, -5.049401038298163336, 91.45724293864766707 ) ) ;
#29460=CARTESIAN_POINT ( 'NONE',  ( -8.314922557961024197, 14.29746914071037800, 92.91775706135236135 ) ) ;
#29461=CARTESIAN_POINT ( 'NONE',  ( -0.05219959533937732626, 21.53943276465977519, 47.50109039468568994 ) ) ;
#29462=CARTESIAN_POINT ( 'NONE',  ( -4.483927247898539470, -16.52544592524342804, 112.2905762719810241 ) ) ;
#29463=CARTESIAN_POINT ( 'NONE',  ( 12.14591786802309770, 12.06949235617756955, 69.37390960531436690 ) ) ;
#29464=CARTESIAN_POINT ( 'NONE',  ( -8.224510206698948167, 14.34966873604960824, 30.41557627198101699 ) ) ;
#29465=CARTESIAN_POINT ( 'NONE',  ( -21.53943276465977519, 0.05219959533907696930, 41.24890960531435269 ) ) ;
#29466=CARTESIAN_POINT ( 'NONE',  ( -16.46253265017160317, 9.564922557960807481, 70.83224293864770971 ) ) ;
#29467=CARTESIAN_POINT ( 'NONE',  ( -5.153800228976328057, -19.02544592524343514, 52.29057627198100988 ) ) ;
#29468=CARTESIAN_POINT ( 'NONE',  ( -5.823673210054116645, -21.52544592524344225, 62.29057627198102409 ) ) ;
#29469=CARTESIAN_POINT ( 'NONE',  ( 19.05341960407617918, -5.049401038297876454, 41.04275706135233293 ) ) ;
#29471=CARTESIAN_POINT ( 'NONE',  ( -16.55341960407611168, -4.379528057220339221, 46.45724293864769550 ) ) ;
#29472=CARTESIAN_POINT ( 'NONE',  ( -15.72974639402197994, 15.80617190586746368, 25.62390960531435624 ) ) ;
#29473=ORIENTED_EDGE ( 'NONE', *, *, #36295, .F. ) ;
#29474=EDGE_LOOP ( 'NONE', ( #122212, #62042, #7298, #67452, #164950, #5265, #111171, #42746 ) ) ;
#29476=CARTESIAN_POINT ( 'NONE',  ( -12.06949235617739369, -12.14591786802326823, 69.37609039468567573 ) ) ;
#29477=CARTESIAN_POINT ( 'NONE',  ( -19.05341960407617563, 5.049401038297882671, 73.54275706135233293 ) ) ;
#29478=CARTESIAN_POINT ( 'NONE',  ( 0.05219959533910956823, 16.53943276465976808, 34.99890960531435979 ) ) ;
#29480=CARTESIAN_POINT ( 'NONE',  ( -16.55341960407611168, -4.379528057220339221, 21.45724293864769550 ) ) ;
#29481=CARTESIAN_POINT ( 'NONE',  ( -5.049401038298153566, 19.05341960407611168, 45.20724293864769550 ) ) ;
#29482=CARTESIAN_POINT ( 'NONE',  ( 19.03943276465977164, -0.05219959533909143690, 78.74890960531436690 ) ) ;
#29483=CARTESIAN_POINT ( 'NONE',  ( 13.97604488694527802, 13.89961937509977652, 44.37390960531435269 ) ) ;
#29484=CARTESIAN_POINT ( 'NONE',  ( 5.719274019375673035, 21.55341960407619339, 52.29275706135236135 ) ) ;
#29485=CARTESIAN_POINT ( 'NONE',  ( -5.153800228976328057, -19.02544592524343514, 52.29057627198100988 ) ) ;
#29486=CARTESIAN_POINT ( 'NONE',  ( -0.05219959533909027116, -19.03943276465977164, 57.49890960531435979 ) ) ;
#29487=CARTESIAN_POINT ( 'NONE',  ( -15.72974639402197994, 15.80617190586746368, 30.62390960531436335 ) ) ;
#29488=CARTESIAN_POINT ( 'NONE',  ( -5.049401038298153566, 19.05341960407611168, 25.20724293864768484 ) ) ;
#29489=CARTESIAN_POINT ( 'NONE',  ( -18.67979575497178146, -10.72451020669898902, 31.66557627198102054 ) ) ;
#29490=CARTESIAN_POINT ( 'NONE',  ( 14.34966873604972726, -8.224510206698740333, 85.83442372801901854 ) ) ;
#29491=CARTESIAN_POINT ( 'NONE',  ( 10.81492255796106328, -18.62759615963255655, 105.4177570613523613 ) ) ;
#29492=CARTESIAN_POINT ( 'NONE',  ( -8.224510206698735004, -14.34966873604973081, 64.58442372801900433 ) ) ;
#29493=CARTESIAN_POINT ( 'NONE',  ( -16.51473224551069308, -9.474510206698971260, 111.6655762719810383 ) ) ;
#29494=CARTESIAN_POINT ( 'NONE',  ( -4.483927247898782831, 16.52544592524335698, 57.70942372801901143 ) ) ;
#29495=CARTESIAN_POINT ( 'NONE',  ( -14.29746914071037622, -8.314922557961029526, 44.16775706135234714 ) ) ;
#29496=CARTESIAN_POINT ( 'NONE',  ( 0.05219959533909260263, 19.03943276465977164, 109.9989096053143669 ) ) ;
#29497=CARTESIAN_POINT ( 'NONE',  ( -19.05341960407617563, 5.049401038297882671, 113.5427570613523471 ) ) ;
#29498=CARTESIAN_POINT ( 'NONE',  ( -19.02544592524342804, 5.153800228976336051, 36.04057627198100988 ) ) ;
#29499=CARTESIAN_POINT ( 'NONE',  ( 21.55341960407619695, -5.719274019375665929, 26.04275706135235779 ) ) ;
#29500=CARTESIAN_POINT ( 'NONE',  ( -4.483927247898782831, 16.52544592524335698, 22.70942372801901499 ) ) ;
#29501=CARTESIAN_POINT ( 'NONE',  ( 14.29746914071037800, 8.314922557961029526, 91.66775706135234714 ) ) ;
#29503=CARTESIAN_POINT ( 'NONE',  ( -10.81492255796105439, 18.62759615963255655, 87.91775706135234714 ) ) ;
#29504=CARTESIAN_POINT ( 'NONE',  ( -0.05219959533936034679, 19.03943276465977164, 87.50109039468567573 ) ) ;
#29505=CARTESIAN_POINT ( 'NONE',  ( -8.314922557960811034, -14.29746914071050412, 52.08224293864768839 ) ) ;
#29506=CARTESIAN_POINT ( 'NONE',  ( -0.05219959533910754901, -16.53943276465976808, 107.4989096053143669 ) ) ;
#29507=CARTESIAN_POINT ( 'NONE',  ( -5.153800228976607833, 19.02544592524334988, 52.70942372801900433 ) ) ;
#29509=CARTESIAN_POINT ( 'NONE',  ( -21.55341960407619339, 5.719274019375674811, 48.54275706135234714 ) ) ;
#29510=CARTESIAN_POINT ( 'NONE',  ( 5.049401038297881783, 19.05341960407617563, 107.2927570613523187 ) ) ;
#29511=CARTESIAN_POINT ( 'NONE',  ( 16.61371651742599553, 7.165104196376154810, 83.64584930007004004 ) ) ;
#29512=CARTESIAN_POINT ( 'NONE',  ( -9.564922557960796823, -16.46253265017161027, 102.0822429386477097 ) ) ;
#29513=CARTESIAN_POINT ( 'NONE',  ( 15.72974639402199770, -15.80617190586745480, 73.12390960531436690 ) ) ;
#29514=CARTESIAN_POINT ( 'NONE',  ( 19.02544592524334988, 5.153800228976608722, 91.45942372801900433 ) ) ;
#29515=CARTESIAN_POINT ( 'NONE',  ( 0.05219959533909260263, 19.03943276465977164, 99.99890960531436690 ) ) ;
#29517=CARTESIAN_POINT ( 'NONE',  ( 16.55341960407611168, 4.379528057220329451, 103.9572429386476813 ) ) ;
#29518=CARTESIAN_POINT ( 'NONE',  ( -15.72974639402176322, -15.80617190586768395, 99.37609039468568994 ) ) ;
#29519=CARTESIAN_POINT ( 'NONE',  ( 16.51473224551069308, 9.474510206698969483, 39.16557627198103120 ) ) ;
#29520=CARTESIAN_POINT ( 'NONE',  ( -0.05219959533937732626, 21.53943276465977519, 57.50109039468568994 ) ) ;
#29521=CARTESIAN_POINT ( 'NONE',  ( -0.05219959533937732626, 21.53943276465977519, 82.50109039468568994 ) ) ;
#29522=CARTESIAN_POINT ( 'NONE',  ( -12.06949235617739369, -12.14591786802326823, 99.37609039468568994 ) ) ;
#29524=CARTESIAN_POINT ( 'NONE',  ( 10.72451020669871369, 18.67979575497193778, 47.08442372801901854 ) ) ;
#29525=CARTESIAN_POINT ( 'NONE',  ( -5.719274019375665041, -21.55341960407619695, 34.79275706135235424 ) ) ;
#29526=CARTESIAN_POINT ( 'NONE',  ( -19.02544592524334988, -5.153800228976617603, 63.95942372801899012 ) ) ;
#29527=CARTESIAN_POINT ( 'NONE',  ( 16.51473224551069308, 9.474510206698969483, 94.16557627198103830 ) ) ;
#29528=CARTESIAN_POINT ( 'NONE',  ( -16.53943276465976808, 0.05219959533911058130, 106.2489096053143811 ) ) ;
#29529=CARTESIAN_POINT ( 'NONE',  ( 15.72974639402199770, -15.80617190586745480, 88.12390960531436690 ) ) ;
#29530=CARTESIAN_POINT ( 'NONE',  ( -16.52544592524342804, 4.483927247898546575, 61.04057627198103120 ) ) ;
#29531=CARTESIAN_POINT ( 'NONE',  ( -19.02544592524334988, -5.153800228976617603, 18.95942372801899722 ) ) ;
#29532=CARTESIAN_POINT ( 'NONE',  ( -12.06949235617756955, 12.14591786802309770, 85.62390960531436690 ) ) ;
#29533=CARTESIAN_POINT ( 'NONE',  ( 16.51473224551069308, 9.474510206698969483, 39.16557627198103120 ) ) ;
#29534=CARTESIAN_POINT ( 'NONE',  ( -19.03943276465977164, -0.05219959533935918106, 83.75109039468567573 ) ) ;
#29535=CARTESIAN_POINT ( 'NONE',  ( -4.379528057220328563, 16.55341960407611168, 45.20724293864769550 ) ) ;
#29536=CARTESIAN_POINT ( 'NONE',  ( 18.67979575497194134, -10.72451020669871369, 95.83442372801903275 ) ) ;
#29537=CARTESIAN_POINT ( 'NONE',  ( -0.05219959533909027116, -19.03943276465977164, 87.49890960531436690 ) ) ;
#29538=CARTESIAN_POINT ( 'NONE',  ( 13.89961937509957401, 13.97604488694547697, 61.87609039468566863 ) ) ;
#29539=CARTESIAN_POINT ( 'NONE',  ( 18.62759615963271287, -10.81492255796078972, 73.33224293864769550 ) ) ;
#29540=CARTESIAN_POINT ( 'NONE',  ( -18.62759615963255300, -10.81492255796106328, 34.16775706135234714 ) ) ;
#29541=CARTESIAN_POINT ( 'NONE',  ( 12.14591786802327356, -12.06949235617739191, 30.62609039468567929 ) ) ;
#29542=CARTESIAN_POINT ( 'NONE',  ( -4.379528057220086978, -16.55341960407618274, 84.79275706135234714 ) ) ;
#29543=CARTESIAN_POINT ( 'NONE',  ( -13.97604488694527625, -13.89961937509977652, 21.87390960531435979 ) ) ;
#29544=CARTESIAN_POINT ( 'NONE',  ( -5.719274019375978568, 21.55341960407610458, 115.2072429386476955 ) ) ;
#29545=CARTESIAN_POINT ( 'NONE',  ( 16.52544592524342804, -4.483927247898539470, 113.5405762719810383 ) ) ;
#29547=CARTESIAN_POINT ( 'NONE',  ( -4.379528057220086978, -16.55341960407618274, 44.79275706135234714 ) ) ;
#29548=CARTESIAN_POINT ( 'NONE',  ( 14.34966873604960469, 8.224510206698951720, 74.16557627198102409 ) ) ;
#29549=CARTESIAN_POINT ( 'NONE',  ( -10.81492255796078084, -18.62759615963271287, 72.08224293864769550 ) ) ;
#29550=CARTESIAN_POINT ( 'NONE',  ( 8.314922557960818139, 14.29746914071049879, 24.58224293864768839 ) ) ;
#29551=CARTESIAN_POINT ( 'NONE',  ( -12.14591786802326823, 12.06949235617739902, 53.12609039468568284 ) ) ;
#29552=CARTESIAN_POINT ( 'NONE',  ( 13.89961937509977652, -13.97604488694527269, 43.12390960531434558 ) ) ;
#29553=CARTESIAN_POINT ( 'NONE',  ( -14.34966873604972548, 8.224510206698743886, 78.33442372801901854 ) ) ;
#29554=CARTESIAN_POINT ( 'NONE',  ( 13.89961937509957401, 13.97604488694547697, 71.87609039468567573 ) ) ;
#29555=CARTESIAN_POINT ( 'NONE',  ( 15.72974639402199770, -15.80617190586745480, 73.12390960531436690 ) ) ;
#29556=CARTESIAN_POINT ( 'NONE',  ( -12.14591786802326823, 12.06949235617739902, 108.1260903946856757 ) ) ;
#29558=CARTESIAN_POINT ( 'NONE',  ( -13.89961937509977652, 13.97604488694528158, 115.6239096053143669 ) ) ;
#29559=ADVANCED_FACE ( 'NONE', ( #42877 ), #130798, .F. ) ;
#29560=CARTESIAN_POINT ( 'NONE',  ( -10.81492255796078084, -18.62759615963271287, 52.08224293864768839 ) ) ;
#29562=CARTESIAN_POINT ( 'NONE',  ( -16.55341960407617563, 4.379528057220093196, 88.54275706135236135 ) ) ;
#29564=CARTESIAN_POINT ( 'NONE',  ( -9.564922557960796823, -16.46253265017161027, 107.0822429386476955 ) ) ;
#29565=CARTESIAN_POINT ( 'NONE',  ( -18.39635199886969730, 5.499999999999980460, 76.01967076360001840 ) ) ;
#29566=CARTESIAN_POINT ( 'NONE',  ( 15.80617190586746368, 15.72974639402197994, 69.37390960531436690 ) ) ;
#29567=CARTESIAN_POINT ( 'NONE',  ( -16.55341960407617563, 4.379528057220093196, 103.5427570613523613 ) ) ;
#29568=CARTESIAN_POINT ( 'NONE',  ( 13.89961937509957401, 13.97604488694547697, 111.8760903946856757 ) ) ;
#29569=CARTESIAN_POINT ( 'NONE',  ( -16.52544592524342804, 4.483927247898546575, 111.0405762719810525 ) ) ;
#29570=CARTESIAN_POINT ( 'NONE',  ( 0.05219959533934541429, -16.53943276465976808, 30.00109039468568284 ) ) ;
#29571=CARTESIAN_POINT ( 'NONE',  ( -16.51473224551069308, -9.474510206698971260, 56.66557627198103120 ) ) ;
#29573=CARTESIAN_POINT ( 'NONE',  ( 19.02544592524343514, -5.153800228976328945, 98.54057627198100988 ) ) ;
#29574=CARTESIAN_POINT ( 'NONE',  ( -4.483927247898782831, 16.52544592524335698, 92.70942372801901854 ) ) ;
#29575=CARTESIAN_POINT ( 'NONE',  ( 13.97604488694548053, -13.89961937509957401, 85.62609039468568994 ) ) ;
#29576=CARTESIAN_POINT ( 'NONE',  ( 0.05219959533936267826, -19.03943276465977164, 30.00109039468566863 ) ) ;
#29577=CARTESIAN_POINT ( 'NONE',  ( -5.823673210054116645, -21.52544592524344225, 77.29057627198102409 ) ) ;
#29578=CARTESIAN_POINT ( 'NONE',  ( 12.14591786802327356, -12.06949235617739191, 105.6260903946856899 ) ) ;
#29579=CARTESIAN_POINT ( 'NONE',  ( -13.97604488694547697, 13.89961937509957934, 98.12609039468566152 ) ) ;
#29580=CARTESIAN_POINT ( 'NONE',  ( -5.153800228976328057, -19.02544592524343514, 52.29057627198100988 ) ) ;
#29581=CARTESIAN_POINT ( 'NONE',  ( 19.02544592524343514, -5.153800228976328945, 93.54057627198102409 ) ) ;
#29582=CARTESIAN_POINT ( 'NONE',  ( 15.72974639402176855, 15.80617190586768217, 61.87609039468568284 ) ) ;
#29583=CARTESIAN_POINT ( 'NONE',  ( -13.89961937509977652, 13.97604488694528158, 50.62390960531435979 ) ) ;
#29585=CARTESIAN_POINT ( 'NONE',  ( 16.53943276465976808, -0.05219959533910856209, 73.74890960531433848 ) ) ;
#29586=CARTESIAN_POINT ( 'NONE',  ( -21.53943276465977519, 0.05219959533907696930, 76.24890960531435269 ) ) ;
#29589=CARTESIAN_POINT ( 'NONE',  ( -16.51473224551082808, 9.474510206698731452, 38.33442372801899722 ) ) ;
#29590=CARTESIAN_POINT ( 'NONE',  ( 17.40861289039006365, -6.110651285853166748, 71.12767529172569425 ) ) ;
#29591=CARTESIAN_POINT ( 'NONE',  ( 9.474510206698971260, -16.51473224551069308, 82.91557627198103830 ) ) ;
#29592=CARTESIAN_POINT ( 'NONE',  ( 5.049401038298161559, -19.05341960407611168, 82.70724293864770971 ) ) ;
#29593=CARTESIAN_POINT ( 'NONE',  ( -4.483927247898782831, 16.52544592524335698, 62.70942372801902565 ) ) ;
#29595=CARTESIAN_POINT ( 'NONE',  ( -0.05219959533936034679, 19.03943276465977164, 32.50109039468566863 ) ) ;
#29597=CARTESIAN_POINT ( 'NONE',  ( -4.379528057220086978, -16.55341960407618274, 89.79275706135236135 ) ) ;
#29599=CARTESIAN_POINT ( 'NONE',  ( -16.55341960407617563, 4.379528057220093196, 83.54275706135234714 ) ) ;
#29600=CARTESIAN_POINT ( 'NONE',  ( -16.55341960407617563, 4.379528057220093196, 53.54275706135234714 ) ) ;
#29601=CARTESIAN_POINT ( 'NONE',  ( -17.97058386085787163, -5.500000000000058620, 59.00390968646216550 ) ) ;
#29602=CARTESIAN_POINT ( 'NONE',  ( 18.67979575497194134, -10.72451020669871369, 65.83442372801900433 ) ) ;
#29603=CARTESIAN_POINT ( 'NONE',  ( -5.153800228976607833, 19.02544592524334988, 77.70942372801900433 ) ) ;
#29604=CARTESIAN_POINT ( 'NONE',  ( -18.62759615963255300, -10.81492255796106328, 104.1677570613523471 ) ) ;
#29605=CARTESIAN_POINT ( 'NONE',  ( -19.02544592524342804, 5.153800228976336051, 51.04057627198103120 ) ) ;
#29606=CARTESIAN_POINT ( 'NONE',  ( 19.02544592524343514, -5.153800228976328945, 38.54057627198103120 ) ) ;
#29608=CARTESIAN_POINT ( 'NONE',  ( -5.823673210054116645, -21.52544592524344225, 62.29057627198102409 ) ) ;
#29609=CARTESIAN_POINT ( 'NONE',  ( 21.55341960407610458, 5.719274019375980345, 23.95724293864769550 ) ) ;
#29610=CARTESIAN_POINT ( 'NONE',  ( -16.52544592524342804, 4.483927247898546575, 111.0405762719810525 ) ) ;
#29611=CARTESIAN_POINT ( 'NONE',  ( -16.53943276465976808, -0.05219959533934237506, 53.75109039468568994 ) ) ;
#29613=CARTESIAN_POINT ( 'NONE',  ( -0.05219959533907301413, -21.53943276465977519, 112.4989096053143669 ) ) ;
#29614=CARTESIAN_POINT ( 'NONE',  ( -14.29746914071049879, 8.314922557960819915, 50.83224293864770971 ) ) ;
#29616=CARTESIAN_POINT ( 'NONE',  ( -5.049401038297874678, -19.05341960407617918, 104.7927570613523471 ) ) ;
#29617=CARTESIAN_POINT ( 'NONE',  ( 0.05219959533936267826, -19.03943276465977164, 40.00109039468566152 ) ) ;
#29618=CARTESIAN_POINT ( 'NONE',  ( -12.14591786802309592, -12.06949235617757132, 46.87390960531435979 ) ) ;
#29619=CARTESIAN_POINT ( 'NONE',  ( -15.80617190586768217, 15.72974639402176855, 23.12609039468567573 ) ) ;
#29621=CARTESIAN_POINT ( 'NONE',  ( -18.62759615963270932, 10.81492255796079327, 70.83224293864770971 ) ) ;
#29622=CARTESIAN_POINT ( 'NONE',  ( 5.049401038298161559, -19.05341960407611168, 87.70724293864769550 ) ) ;
#29623=CARTESIAN_POINT ( 'NONE',  ( 16.55341960407611168, 4.379528057220329451, 48.95724293864770971 ) ) ;
#29624=CARTESIAN_POINT ( 'NONE',  ( -16.46253265017160317, 9.564922557960807481, 100.8322429386477097 ) ) ;
#29626=CARTESIAN_POINT ( 'NONE',  ( -19.03943276465977164, -0.05219959533935918106, 53.75109039468566863 ) ) ;
#29627=CARTESIAN_POINT ( 'NONE',  ( -5.719274019375978568, 21.55341960407610458, 100.2072429386476955 ) ) ;
#29628=CARTESIAN_POINT ( 'NONE',  ( 13.97604488694527802, 13.89961937509977652, 39.37390960531435269 ) ) ;
#29629=CARTESIAN_POINT ( 'NONE',  ( 19.02544592524343514, -5.153800228976328945, 23.54057627198102054 ) ) ;
#29630=CARTESIAN_POINT ( 'NONE',  ( -0.05219959533937732626, 21.53943276465977519, 47.50109039468568994 ) ) ;
#29632=CARTESIAN_POINT ( 'NONE',  ( -4.483927247898539470, -16.52544592524342804, 22.29057627198102765 ) ) ;
#29633=CARTESIAN_POINT ( 'NONE',  ( 9.564922557960805705, 16.46253265017160317, 54.58224293864769550 ) ) ;
#29634=CARTESIAN_POINT ( 'NONE',  ( 0.05219959533909260263, 19.03943276465977164, 99.99890960531436690 ) ) ;
#29635=CARTESIAN_POINT ( 'NONE',  ( -10.72451020669898014, 18.67979575497178502, 65.41557627198102409 ) ) ;
#29637=CARTESIAN_POINT ( 'NONE',  ( 16.46253265017160672, -9.564922557960803928, 43.33224293864769550 ) ) ;
#29638=CARTESIAN_POINT ( 'NONE',  ( 5.823673210054125526, 21.52544592524343514, 49.79057627198102409 ) ) ;
#29640=CARTESIAN_POINT ( 'NONE',  ( 5.823673210054444382, -21.52544592524334988, 85.20942372801901854 ) ) ;
#29642=CARTESIAN_POINT ( 'NONE',  ( -4.483927247898782831, 16.52544592524335698, 87.70942372801901854 ) ) ;
#29643=CARTESIAN_POINT ( 'NONE',  ( 12.14591786802309770, 12.06949235617756955, 74.37390960531436690 ) ) ;
#29644=CARTESIAN_POINT ( 'NONE',  ( -12.06949235617739369, -12.14591786802326823, 94.37609039468568994 ) ) ;
#29645=CARTESIAN_POINT ( 'NONE',  ( -19.03943276465977164, 0.05219959533909376836, 76.24890960531435269 ) ) ;
#29646=VERTEX_POINT ( 'NONE', #93320 ) ;
#29647=CARTESIAN_POINT ( 'NONE',  ( -16.46253265017146816, -9.564922557961047289, 29.16775706135232937 ) ) ;
#29648=CARTESIAN_POINT ( 'NONE',  ( -12.06949235617739369, -12.14591786802326823, 84.37609039468570415 ) ) ;
#29649=CARTESIAN_POINT ( 'NONE',  ( 5.719274019375673035, 21.55341960407619339, 112.2927570613523471 ) ) ;
#29650=CARTESIAN_POINT ( 'NONE',  ( -9.564922557960796823, -16.46253265017161027, 77.08224293864769550 ) ) ;
#29651=CARTESIAN_POINT ( 'NONE',  ( -15.80617190586745835, -15.72974639402198527, 41.87390960531435979 ) ) ;
#29652=CARTESIAN_POINT ( 'NONE',  ( -16.55341960407617563, 4.379528057220093196, 23.54275706135235424 ) ) ;
#29653=CARTESIAN_POINT ( 'NONE',  ( 15.72974639402176855, 15.80617190586768217, 86.87609039468568994 ) ) ;
#29654=CARTESIAN_POINT ( 'NONE',  ( -12.06949235617739369, -12.14591786802326823, 64.37609039468568994 ) ) ;
#29655=CARTESIAN_POINT ( 'NONE',  ( 21.55341960407610458, 5.719274019375980345, 113.9572429386477239 ) ) ;
#29656=CARTESIAN_POINT ( 'NONE',  ( -13.97604488694547697, 13.89961937509957934, 113.1260903946856757 ) ) ;
#29657=CARTESIAN_POINT ( 'NONE',  ( 5.153800228976335163, 19.02544592524342804, 94.79057627198103830 ) ) ;
#29658=CARTESIAN_POINT ( 'NONE',  ( 16.52544592524335698, 4.483927247898782831, 26.45942372801901854 ) ) ;
#29659=CARTESIAN_POINT ( 'NONE',  ( 19.05341960407611168, 5.049401038298154454, 38.95724293864767418 ) ) ;
#29660=CARTESIAN_POINT ( 'NONE',  ( 8.314922557961029526, -14.29746914071037800, 40.41775706135234714 ) ) ;
#29661=CARTESIAN_POINT ( 'NONE',  ( -8.224510206698948167, 14.34966873604960824, 85.41557627198102409 ) ) ;
#29662=CARTESIAN_POINT ( 'NONE',  ( 14.34966873604972726, -8.224510206698740333, 80.83442372801901854 ) ) ;
#29663=CARTESIAN_POINT ( 'NONE',  ( -18.62759615963255300, -10.81492255796106328, 24.16775706135235424 ) ) ;
#29664=CARTESIAN_POINT ( 'NONE',  ( 19.03943276465977164, -0.05219959533909143690, 63.74890960531435979 ) ) ;
#29665=CARTESIAN_POINT ( 'NONE',  ( -16.46253265017160317, 9.564922557960807481, 75.83224293864769550 ) ) ;
#29666=CARTESIAN_POINT ( 'NONE',  ( -0.05219959533934338120, 16.53943276465976808, 92.50109039468567573 ) ) ;
#29668=ORIENTED_EDGE ( 'NONE', *, *, #148562, .F. ) ;
#29670=CARTESIAN_POINT ( 'NONE',  ( 9.474510206698729675, 16.51473224551082808, 32.08442372801900433 ) ) ;
#29671=CARTESIAN_POINT ( 'NONE',  ( 13.89961937509977652, -13.97604488694527269, 53.12390960531434558 ) ) ;
#29672=DIRECTION ( 'NONE',  ( 0.000000000000000000, 0.000000000000000000, -1.000000000000000000 ) ) ;
#29674=CARTESIAN_POINT ( 'NONE',  ( -16.52544592524335698, -4.483927247898792601, 23.95942372801901143 ) ) ;
#29675=CARTESIAN_POINT ( 'NONE',  ( -13.97604488694547697, 13.89961937509957934, 53.12609039468565442 ) ) ;
#29676=CARTESIAN_POINT ( 'NONE',  ( 12.14591786802327356, -12.06949235617739191, 45.62609039468567573 ) ) ;
#29677=CARTESIAN_POINT ( 'NONE',  ( -19.03943276465977164, 0.05219959533909376836, 101.2489096053143669 ) ) ;
#29678=CARTESIAN_POINT ( 'NONE',  ( -5.049401038298153566, 19.05341960407611168, 80.20724293864769550 ) ) ;
#29679=CARTESIAN_POINT ( 'NONE',  ( 18.62759615963271287, -10.81492255796078972, 93.33224293864769550 ) ) ;
#29680=CARTESIAN_POINT ( 'NONE',  ( 16.51473224551083163, -9.474510206698727899, 65.83442372801900433 ) ) ;
#29681=CARTESIAN_POINT ( 'NONE',  ( 16.46253265017160672, -9.564922557960803928, 98.33224293864769550 ) ) ;
#29682=CARTESIAN_POINT ( 'NONE',  ( 17.40593841890343896, -5.148608847476693562, 21.38766112942987974 ) ) ;
#29684=CARTESIAN_POINT ( 'NONE',  ( 9.474510206698971260, -16.51473224551069308, 57.91557627198103120 ) ) ;
#29685=CARTESIAN_POINT ( 'NONE',  ( -8.224510206698735004, -14.34966873604973081, 109.5844237280190328 ) ) ;
#29686=CARTESIAN_POINT ( 'NONE',  ( 13.97604488694527802, 13.89961937509977652, 24.37390960531435624 ) ) ;
#29687=CARTESIAN_POINT ( 'NONE',  ( 5.049401038297881783, 19.05341960407617563, 37.29275706135232582 ) ) ;
#29689=CARTESIAN_POINT ( 'NONE',  ( -14.29746914071049879, 8.314922557960819915, 80.83224293864769550 ) ) ;
#29690=CARTESIAN_POINT ( 'NONE',  ( 10.81492255796106328, -18.62759615963255655, 95.41775706135234714 ) ) ;
#29691=CARTESIAN_POINT ( 'NONE',  ( -19.02544592524342804, 5.153800228976336051, 41.04057627198103120 ) ) ;
#29692=CARTESIAN_POINT ( 'NONE',  ( 4.483927247898790824, -16.52544592524335698, 55.20942372801902565 ) ) ;
#29693=CARTESIAN_POINT ( 'NONE',  ( -0.05219959533910754901, -16.53943276465976808, 42.49890960531435979 ) ) ;
#29694=CARTESIAN_POINT ( 'NONE',  ( 10.81492255796106328, -18.62759615963255655, 90.41775706135236135 ) ) ;
#29695=CARTESIAN_POINT ( 'NONE',  ( -16.51473224551069308, -9.474510206698971260, 86.66557627198102409 ) ) ;
#29696=CARTESIAN_POINT ( 'NONE',  ( -13.89961937509977652, 13.97604488694528158, 95.62390960531436690 ) ) ;
#29697=CARTESIAN_POINT ( 'NONE',  ( 16.53943276465976808, -0.05219959533910856209, 108.7489096053143669 ) ) ;
#29698=CARTESIAN_POINT ( 'NONE',  ( 16.52544592524342804, -4.483927247898539470, 73.54057627198102409 ) ) ;
#29699=CARTESIAN_POINT ( 'NONE',  ( 5.719274019375991003, -21.55341960407610458, 87.70724293864769550 ) ) ;
#29700=CARTESIAN_POINT ( 'NONE',  ( 13.89961937509977652, -13.97604488694527269, 83.12390960531436690 ) ) ;
#29701=CARTESIAN_POINT ( 'NONE',  ( 0.05219959533907565091, 21.53943276465977519, 99.99890960531436690 ) ) ;
#29702=CARTESIAN_POINT ( 'NONE',  ( 9.474510206698971260, -16.51473224551069308, 87.91557627198102409 ) ) ;
#29703=CARTESIAN_POINT ( 'NONE',  ( 19.25663599770063072, -5.499999999999451106, 46.49419308057203182 ) ) ;
#29704=CARTESIAN_POINT ( 'NONE',  ( -4.379528057220328563, 16.55341960407611168, 90.20724293864770971 ) ) ;
#29705=CARTESIAN_POINT ( 'NONE',  ( 16.51473224551069308, 9.474510206698969483, 54.16557627198103120 ) ) ;
#29706=CARTESIAN_POINT ( 'NONE',  ( -21.53943276465977519, 0.05219959533907696930, 66.24890960531436690 ) ) ;
#29708=CARTESIAN_POINT ( 'NONE',  ( -16.52544592524342804, 4.483927247898546575, 26.04057627198103475 ) ) ;
#29709=DIRECTION ( 'NONE',  ( 0.000000000000000000, 0.000000000000000000, -1.000000000000000000 ) ) ;
#29710=CARTESIAN_POINT ( 'NONE',  ( 19.05341960407617918, -5.049401038297876454, 111.0427570613523329 ) ) ;
#29711=CARTESIAN_POINT ( 'NONE',  ( -12.14591786802309592, -12.06949235617757132, 76.87390960531439532 ) ) ;
#29712=CARTESIAN_POINT ( 'NONE',  ( -16.29526858892875296, -7.335722546920131926, 95.79670597800208043 ) ) ;
#29713=CARTESIAN_POINT ( 'NONE',  ( 9.474510206698971260, -16.51473224551069308, 72.91557627198102409 ) ) ;
#29714=CARTESIAN_POINT ( 'NONE',  ( 13.97604488694527802, 13.89961937509977652, 49.37390960531434558 ) ) ;
#29715=CARTESIAN_POINT ( 'NONE',  ( -16.55341960407611168, -4.379528057220339221, 71.45724293864769550 ) ) ;
#29716=CARTESIAN_POINT ( 'NONE',  ( -19.02544592524342804, 5.153800228976336051, 116.0405762719810383 ) ) ;
#29717=CARTESIAN_POINT ( 'NONE',  ( 19.05341960407617918, -5.049401038297876454, 101.0427570613523045 ) ) ;
#29718=CARTESIAN_POINT ( 'NONE',  ( -19.03943276465977164, 0.05219959533909376836, 101.2489096053143669 ) ) ;
#29719=CARTESIAN_POINT ( 'NONE',  ( 21.52544592524344225, -5.823673210054117533, 73.54057627198102409 ) ) ;
#29720=CARTESIAN_POINT ( 'NONE',  ( 4.379528057220092307, 16.55341960407617563, 67.29275706135234714 ) ) ;
#29721=CARTESIAN_POINT ( 'NONE',  ( -16.38665767534994089, 7.295008042176404750, 95.26400864214467390 ) ) ;
#29722=CARTESIAN_POINT ( 'NONE',  ( 13.97604488694527802, 13.89961937509977652, 74.37390960531436690 ) ) ;
#29723=CARTESIAN_POINT ( 'NONE',  ( -21.55341960407610458, -5.719274019375992779, 81.45724293864769550 ) ) ;
#29724=CARTESIAN_POINT ( 'NONE',  ( -16.46253265017146816, -9.564922557961047289, 104.1677570613523329 ) ) ;
#29725=CARTESIAN_POINT ( 'NONE',  ( -12.06949235617756955, 12.14591786802309770, 40.62390960531435269 ) ) ;
#29726=CARTESIAN_POINT ( 'NONE',  ( -15.80617190586768217, 15.72974639402176855, 53.12609039468568284 ) ) ;
#29728=CARTESIAN_POINT ( 'NONE',  ( -14.29746914071037622, -8.314922557961029526, 69.16775706135234714 ) ) ;
#29729=CARTESIAN_POINT ( 'NONE',  ( -19.03943276465977164, 0.05219959533909376836, 106.2489096053143669 ) ) ;
#29731=CARTESIAN_POINT ( 'NONE',  ( -17.05116617787825106, 6.768360034955815507, 78.65675553259198693 ) ) ;
#29732=CARTESIAN_POINT ( 'NONE',  ( 16.53943276465976808, 0.05219959533934440121, 96.25109039468568994 ) ) ;
#29733=CARTESIAN_POINT ( 'NONE',  ( -0.05219959533934338120, 16.53943276465976808, 52.50109039468567573 ) ) ;
#29734=CARTESIAN_POINT ( 'NONE',  ( 13.97604488694527802, 13.89961937509977652, 54.37390960531435979 ) ) ;
#29735=CARTESIAN_POINT ( 'NONE',  ( 0.05219959533909260263, 19.03943276465977164, 74.99890960531435269 ) ) ;
#29736=CARTESIAN_POINT ( 'NONE',  ( -21.52544592524334988, -5.823673210054445271, 68.95942372801901854 ) ) ;
#29737=CARTESIAN_POINT ( 'NONE',  ( -4.483927247898782831, 16.52544592524335698, 57.70942372801901143 ) ) ;
#29738=CARTESIAN_POINT ( 'NONE',  ( -14.29746914071049879, 8.314922557960819915, 35.83224293864768839 ) ) ;
#29739=CARTESIAN_POINT ( 'NONE',  ( -19.05341960407611168, -5.049401038298163336, 41.45724293864769550 ) ) ;
#29740=CARTESIAN_POINT ( 'NONE',  ( 16.46253265017160672, -9.564922557960803928, 38.33224293864768839 ) ) ;
#29741=CARTESIAN_POINT ( 'NONE',  ( 4.483927247898790824, -16.52544592524335698, 35.20942372801901854 ) ) ;
#29742=CARTESIAN_POINT ( 'NONE',  ( -16.46253265017146816, -9.564922557961047289, 89.16775706135234714 ) ) ;
#29743=CARTESIAN_POINT ( 'NONE',  ( 8.314922557960818139, 14.29746914071049879, 99.58224293864770971 ) ) ;
#29744=CARTESIAN_POINT ( 'NONE',  ( 13.89961937509977652, -13.97604488694527269, 53.12390960531434558 ) ) ;
#29745=CARTESIAN_POINT ( 'NONE',  ( -16.46253265017146816, -9.564922557961047289, 89.16775706135234714 ) ) ;
#29747=CARTESIAN_POINT ( 'NONE',  ( -10.81492255796105439, 18.62759615963255655, 92.91775706135236135 ) ) ;
#29748=CARTESIAN_POINT ( 'NONE',  ( 4.379528057220092307, 16.55341960407617563, 57.29275706135234714 ) ) ;
#29750=CARTESIAN_POINT ( 'NONE',  ( -15.72974639402197994, 15.80617190586746368, 55.62390960531436690 ) ) ;
#29751=CARTESIAN_POINT ( 'NONE',  ( 0.05219959533934541429, -16.53943276465976808, 45.00109039468568284 ) ) ;
#29752=CARTESIAN_POINT ( 'NONE',  ( -19.48894818550245844, 5.499999999999919176, 70.10307310435241845 ) ) ;
#29753=CARTESIAN_POINT ( 'NONE',  ( 19.02544592524334988, 5.153800228976608722, 41.45942372801900433 ) ) ;
#29754=CARTESIAN_POINT ( 'NONE',  ( 0.05219959533909260263, 19.03943276465977164, 89.99890960531436690 ) ) ;
#29755=CARTESIAN_POINT ( 'NONE',  ( -8.314922557960811034, -14.29746914071050412, 102.0822429386476955 ) ) ;
#29756=CARTESIAN_POINT ( 'NONE',  ( 5.153800228976335163, 19.02544592524342804, 54.79057627198103120 ) ) ;
#29758=CARTESIAN_POINT ( 'NONE',  ( -5.719274019375665041, -21.55341960407619695, 79.79275706135236135 ) ) ;
#29759=CARTESIAN_POINT ( 'NONE',  ( -18.22780087662124160, -5.499999999999927169, 88.98236817873107896 ) ) ;
#29760=ADVANCED_FACE ( 'NONE', ( #33646 ), #137169, .F. ) ;
#29761=CARTESIAN_POINT ( 'NONE',  ( 5.049401038297881783, 19.05341960407617563, 32.29275706135233293 ) ) ;
#29762=CARTESIAN_POINT ( 'NONE',  ( -21.53943276465977519, -0.05219959533937600094, 113.7510903946856757 ) ) ;
#29763=CARTESIAN_POINT ( 'NONE',  ( -16.55341960407611168, -4.379528057220339221, 56.45724293864768839 ) ) ;
#29764=CARTESIAN_POINT ( 'NONE',  ( 16.46253265017160672, -9.564922557960803928, 58.33224293864769550 ) ) ;
#29765=CARTESIAN_POINT ( 'NONE',  ( -19.02544592524342804, 5.153800228976336051, 106.0405762719810241 ) ) ;
#29766=CARTESIAN_POINT ( 'NONE',  ( -5.823673210054431948, 21.52544592524334988, 82.70942372801900433 ) ) ;
#29767=CARTESIAN_POINT ( 'NONE',  ( 13.97604488694527802, 13.89961937509977652, 69.37390960531436690 ) ) ;
#29768=CARTESIAN_POINT ( 'NONE',  ( -21.55341960407619339, 5.719274019375674811, 73.54275706135234714 ) ) ;
#29769=CARTESIAN_POINT ( 'NONE',  ( -21.52544592524343514, 5.823673210054127303, 36.04057627198102409 ) ) ;
#29770=CARTESIAN_POINT ( 'NONE',  ( 15.80617190586769283, -15.72974639402175789, 35.62609039468568994 ) ) ;
#29771=CARTESIAN_POINT ( 'NONE',  ( 13.89961937509957401, 13.97604488694547697, 56.87609039468564731 ) ) ;
#29772=CARTESIAN_POINT ( 'NONE',  ( -9.474510206698964154, 16.51473224551069663, 25.41557627198103120 ) ) ;
#29773=CARTESIAN_POINT ( 'NONE',  ( 16.46253265017160672, -9.564922557960803928, 73.33224293864769550 ) ) ;
#29774=CARTESIAN_POINT ( 'NONE',  ( -16.53943276465976808, -0.05219959533934237506, 28.75109039468567929 ) ) ;
#29775=CARTESIAN_POINT ( 'NONE',  ( -0.05219959533910754901, -16.53943276465976808, 92.49890960531436690 ) ) ;
#29776=CARTESIAN_POINT ( 'NONE',  ( 9.474510206698971260, -16.51473224551069308, 57.91557627198103120 ) ) ;
#29777=CARTESIAN_POINT ( 'NONE',  ( -10.72451020669898014, 18.67979575497178502, 30.41557627198101699 ) ) ;
#29778=CARTESIAN_POINT ( 'NONE',  ( -16.52544592524335698, -4.483927247898792601, 18.95942372801901143 ) ) ;
#29779=CARTESIAN_POINT ( 'NONE',  ( 15.80617190586769283, -15.72974639402175789, 20.62609039468568639 ) ) ;
#29780=CARTESIAN_POINT ( 'NONE',  ( 15.80617190586769283, -15.72974639402175789, 65.62609039468568994 ) ) ;
#29781=CARTESIAN_POINT ( 'NONE',  ( -0.05219959533934338120, 16.53943276465976808, 72.50109039468568994 ) ) ;
#29782=CARTESIAN_POINT ( 'NONE',  ( -4.483927247898782831, 16.52544592524335698, 72.70942372801901854 ) ) ;
#29783=CARTESIAN_POINT ( 'NONE',  ( 13.89961937509977652, -13.97604488694527269, 63.12390960531435979 ) ) ;
#29784=CARTESIAN_POINT ( 'NONE',  ( -16.55341960407617563, 4.379528057220093196, 88.54275706135236135 ) ) ;
#29785=CARTESIAN_POINT ( 'NONE',  ( 19.05341960407617918, -5.049401038297876454, 36.04275706135234003 ) ) ;
#29786=CARTESIAN_POINT ( 'NONE',  ( 15.80617190586769283, -15.72974639402175789, 20.62609039468568639 ) ) ;
#29787=CARTESIAN_POINT ( 'NONE',  ( 14.34966873604960469, 8.224510206698951720, 64.16557627198102409 ) ) ;
#29788=CARTESIAN_POINT ( 'NONE',  ( -16.51473224551069308, -9.474510206698971260, 91.66557627198103830 ) ) ;
#29789=CARTESIAN_POINT ( 'NONE',  ( 16.52544592524335698, 4.483927247898782831, 91.45942372801901854 ) ) ;
#29790=CARTESIAN_POINT ( 'NONE',  ( 21.55341960407619695, -5.719274019375665929, 61.04275706135234714 ) ) ;
#29791=CARTESIAN_POINT ( 'NONE',  ( -16.55341960407617563, 4.379528057220093196, 33.54275706135234714 ) ) ;
#29792=CARTESIAN_POINT ( 'NONE',  ( -21.52544592524343514, 5.823673210054127303, 116.0405762719810383 ) ) ;
#29793=CARTESIAN_POINT ( 'NONE',  ( -12.06949235617756955, 12.14591786802309770, 60.62390960531437401 ) ) ;
#29794=EDGE_LOOP ( 'NONE', ( #87485, #63464, #136171, #43735 ) ) ;
#29795=CARTESIAN_POINT ( 'NONE',  ( -21.53943276465977519, 0.05219959533907696930, 106.2489096053143811 ) ) ;
#29796=CARTESIAN_POINT ( 'NONE',  ( 8.314922557960818139, 14.29746914071049879, 44.58224293864769550 ) ) ;
#29797=ORIENTED_EDGE ( 'NONE', *, *, #84815, .T. ) ;
#29799=CARTESIAN_POINT ( 'NONE',  ( 18.62759615963271287, -10.81492255796078972, 113.3322429386476955 ) ) ;
#29800=CARTESIAN_POINT ( 'NONE',  ( 9.564922557960805705, 16.46253265017160317, 109.5822429386476955 ) ) ;
#29801=CARTESIAN_POINT ( 'NONE',  ( 21.55341960407619695, -5.719274019375665929, 36.04275706135234714 ) ) ;
#29802=CARTESIAN_POINT ( 'NONE',  ( 0.05219959533910956823, 16.53943276465976808, 49.99890960531437401 ) ) ;
#29803=CARTESIAN_POINT ( 'NONE',  ( 5.049401038298161559, -19.05341960407611168, 67.70724293864769550 ) ) ;
#29804=CARTESIAN_POINT ( 'NONE',  ( 5.049401038297881783, 19.05341960407617563, 72.29275706135234714 ) ) ;
#29805=CARTESIAN_POINT ( 'NONE',  ( 16.51473224551069308, 9.474510206698969483, 99.16557627198102409 ) ) ;
#29806=CARTESIAN_POINT ( 'NONE',  ( -10.81492255796078084, -18.62759615963271287, 47.08224293864770260 ) ) ;
#29808=CARTESIAN_POINT ( 'NONE',  ( 19.02544592524343514, -5.153800228976328945, 53.54057627198102409 ) ) ;
#29809=CARTESIAN_POINT ( 'NONE',  ( 12.14591786802327356, -12.06949235617739191, 35.62609039468568994 ) ) ;
#29810=CARTESIAN_POINT ( 'NONE',  ( -13.97604488694547697, 13.89961937509957934, 63.12609039468566152 ) ) ;
#29811=CARTESIAN_POINT ( 'NONE',  ( -21.53943276465977519, 0.05219959533907696930, 116.2489096053143669 ) ) ;
#29812=CARTESIAN_POINT ( 'NONE',  ( -16.52544592524342804, 4.483927247898546575, 46.04057627198103830 ) ) ;
#29814=CARTESIAN_POINT ( 'NONE',  ( -16.51473224551069308, -9.474510206698971260, 86.66557627198102409 ) ) ;
#29815=CARTESIAN_POINT ( 'NONE',  ( -5.823673210054116645, -21.52544592524344225, 77.29057627198102409 ) ) ;
#29816=CARTESIAN_POINT ( 'NONE',  ( 21.53943276465977519, -0.05219959533907433946, 113.7489096053143527 ) ) ;
#29817=CARTESIAN_POINT ( 'NONE',  ( 14.29746914071037800, 8.314922557961029526, 36.66775706135234714 ) ) ;
#29818=CARTESIAN_POINT ( 'NONE',  ( 21.52544592524344225, -5.823673210054117533, 33.54057627198102409 ) ) ;
#29819=CARTESIAN_POINT ( 'NONE',  ( -10.81492255796105439, 18.62759615963255655, 107.9177570613523471 ) ) ;
#29820=CARTESIAN_POINT ( 'NONE',  ( 16.46253265017160672, -9.564922557960803928, 88.33224293864769550 ) ) ;
#29821=CARTESIAN_POINT ( 'NONE',  ( -16.46253265017160317, 9.564922557960807481, 40.83224293864769550 ) ) ;
#29822=CARTESIAN_POINT ( 'NONE',  ( 5.049401038298161559, -19.05341960407611168, 97.70724293864766707 ) ) ;
#29823=CARTESIAN_POINT ( 'NONE',  ( 13.89961937509977652, -13.97604488694527269, 73.12390960531436690 ) ) ;
#29824=CARTESIAN_POINT ( 'NONE',  ( -16.53943276465976808, -0.05219959533934237506, 23.75109039468567929 ) ) ;
#29825=CARTESIAN_POINT ( 'NONE',  ( 16.52216118717250382, -7.221426719304220754, 86.42400978952974810 ) ) ;
#29826=CARTESIAN_POINT ( 'NONE',  ( -5.153800228976607833, 19.02544592524334988, 57.70942372801899012 ) ) ;
#29827=CARTESIAN_POINT ( 'NONE',  ( -9.474510206698720793, -16.51473224551083518, 19.58442372801899722 ) ) ;
#29828=CARTESIAN_POINT ( 'NONE',  ( -15.72974639402197994, 15.80617190586746368, 35.62390960531437401 ) ) ;
#29829=CARTESIAN_POINT ( 'NONE',  ( 14.34966873604972726, -8.224510206698740333, 100.8344237280190185 ) ) ;
#29831=CARTESIAN_POINT ( 'NONE',  ( -9.474510206698720793, -16.51473224551083518, 69.58442372801901854 ) ) ;
#29832=CARTESIAN_POINT ( 'NONE',  ( -0.05219959533936034679, 19.03943276465977164, 27.50109039468566507 ) ) ;
#29834=CARTESIAN_POINT ( 'NONE',  ( -19.02544592524342804, 5.153800228976336051, 36.04057627198100988 ) ) ;
#29835=CARTESIAN_POINT ( 'NONE',  ( -8.224510206698948167, 14.34966873604960824, 40.41557627198103120 ) ) ;
#29836=CARTESIAN_POINT ( 'NONE',  ( -19.02544592524342804, 5.153800228976336051, 26.04057627198103120 ) ) ;
#29837=CARTESIAN_POINT ( 'NONE',  ( -12.14591786802326823, 12.06949235617739902, 113.1260903946856899 ) ) ;
#29839=CARTESIAN_POINT ( 'NONE',  ( 14.29746914071037800, 8.314922557961029526, 96.66775706135234714 ) ) ;
#29840=CARTESIAN_POINT ( 'NONE',  ( 19.03943276465977164, -0.05219959533909143690, 53.74890960531436690 ) ) ;
#29841=CARTESIAN_POINT ( 'NONE',  ( 0.05219959533937995610, -21.53943276465977519, 110.0010903946856757 ) ) ;
#29842=CARTESIAN_POINT ( 'NONE',  ( 14.29746914071037800, 8.314922557961029526, 26.66775706135235424 ) ) ;
#29843=CARTESIAN_POINT ( 'NONE',  ( -21.55341960407619339, 5.719274019375674811, 83.54275706135234714 ) ) ;
#29845=CARTESIAN_POINT ( 'NONE',  ( 19.05341960407617918, -5.049401038297876454, 61.04275706135232582 ) ) ;
#29846=CARTESIAN_POINT ( 'NONE',  ( -19.02544592524342804, 5.153800228976336051, 86.04057627198103830 ) ) ;
#29847=CARTESIAN_POINT ( 'NONE',  ( -9.564922557960796823, -16.46253265017161027, 82.08224293864768129 ) ) ;
#29849=CARTESIAN_POINT ( 'NONE',  ( -18.67979575497178146, -10.72451020669898902, 111.6655762719810525 ) ) ;
#29850=CARTESIAN_POINT ( 'NONE',  ( -4.379528057220328563, 16.55341960407611168, 70.20724293864769550 ) ) ;
#29851=CARTESIAN_POINT ( 'NONE',  ( -18.62759615963270932, 10.81492255796079327, 65.83224293864769550 ) ) ;
#29852=CARTESIAN_POINT ( 'NONE',  ( 19.03943276465977164, -0.05219959533909143690, 53.74890960531436690 ) ) ;
#29853=CARTESIAN_POINT ( 'NONE',  ( -0.05219959533907301413, -21.53943276465977519, 92.49890960531436690 ) ) ;
#29854=CARTESIAN_POINT ( 'NONE',  ( -4.483927247898782831, 16.52544592524335698, 92.70942372801901854 ) ) ;
#29855=ORIENTED_EDGE ( 'NONE', *, *, #111391, .F. ) ;
#29856=CARTESIAN_POINT ( 'NONE',  ( -9.564922557960796823, -16.46253265017161027, 57.08224293864769550 ) ) ;
#29857=CARTESIAN_POINT ( 'NONE',  ( -16.52544592524342804, 4.483927247898546575, 91.04057627198103830 ) ) ;
#29859=CARTESIAN_POINT ( 'NONE',  ( 5.153800228976335163, 19.02544592524342804, 49.79057627198100988 ) ) ;
#29860=CARTESIAN_POINT ( 'NONE',  ( -19.05341960407617563, 5.049401038297882671, 78.54275706135233293 ) ) ;
#29861=CARTESIAN_POINT ( 'NONE',  ( -4.379528057220328563, 16.55341960407611168, 85.20724293864770971 ) ) ;
#29862=CARTESIAN_POINT ( 'NONE',  ( -15.80617190586768217, 15.72974639402176855, 63.12609039468568994 ) ) ;
#29863=CARTESIAN_POINT ( 'NONE',  ( 19.02544592524343514, -5.153800228976328945, 38.54057627198103120 ) ) ;
#29864=CARTESIAN_POINT ( 'NONE',  ( 0.05219959533907565091, 21.53943276465977519, 109.9989096053143527 ) ) ;
#29865=CARTESIAN_POINT ( 'NONE',  ( 8.224510206698953496, -14.34966873604960469, 97.91557627198103830 ) ) ;
#29867=CARTESIAN_POINT ( 'NONE',  ( 19.02544592524343514, -5.153800228976328945, 63.54057627198103830 ) ) ;
#29869=CARTESIAN_POINT ( 'NONE',  ( -16.51473224551082808, 9.474510206698731452, 88.33442372801900433 ) ) ;
#29870=CARTESIAN_POINT ( 'NONE',  ( 16.51473224551069308, 9.474510206698969483, 114.1655762719810241 ) ) ;
#29871=CARTESIAN_POINT ( 'NONE',  ( -21.52544592524334988, -5.823673210054445271, 38.95942372801901854 ) ) ;
#29872=CARTESIAN_POINT ( 'NONE',  ( -16.51473224551069308, -9.474510206698971260, 81.66557627198103830 ) ) ;
#29873=CARTESIAN_POINT ( 'NONE',  ( 19.03943276465977164, 0.05219959533936151252, 66.25109039468567573 ) ) ;
#29874=CARTESIAN_POINT ( 'NONE',  ( 5.153800228976335163, 19.02544592524342804, 59.79057627198100988 ) ) ;
#29875=CARTESIAN_POINT ( 'NONE',  ( 8.224510206698953496, -14.34966873604960469, 82.91557627198103830 ) ) ;
#29876=CARTESIAN_POINT ( 'NONE',  ( -4.379528057220328563, 16.55341960407611168, 65.20724293864768129 ) ) ;
#29877=CARTESIAN_POINT ( 'NONE',  ( 9.474510206698971260, -16.51473224551069308, 82.91557627198103830 ) ) ;
#29878=CARTESIAN_POINT ( 'NONE',  ( 8.224510206698953496, -14.34966873604960469, 82.91557627198103830 ) ) ;
#29879=CARTESIAN_POINT ( 'NONE',  ( -16.46253265017160317, 9.564922557960807481, 90.83224293864769550 ) ) ;
#29880=CARTESIAN_POINT ( 'NONE',  ( 16.46253265017146816, 9.564922557961045513, 36.66775706135233293 ) ) ;
#29881=CARTESIAN_POINT ( 'NONE',  ( 16.46253265017160672, -9.564922557960803928, 48.33224293864769550 ) ) ;
#29882=CARTESIAN_POINT ( 'NONE',  ( 16.55341960407611168, 4.379528057220329451, 28.95724293864769905 ) ) ;
#29883=CARTESIAN_POINT ( 'NONE',  ( -16.52544592524342804, 4.483927247898546575, 106.0405762719810525 ) ) ;
#29884=ORIENTED_EDGE ( 'NONE', *, *, #12228, .T. ) ;
#29885=CARTESIAN_POINT ( 'NONE',  ( 15.80617190586769283, -15.72974639402175789, 45.62609039468567573 ) ) ;
#29886=CARTESIAN_POINT ( 'NONE',  ( -19.03943276465977164, -0.05219959533935918106, 63.75109039468566863 ) ) ;
#29887=CARTESIAN_POINT ( 'NONE',  ( 14.34966873604960469, 8.224510206698951720, 39.16557627198102409 ) ) ;
#29888=CARTESIAN_POINT ( 'NONE',  ( -10.72451020669898014, 18.67979575497178502, 90.41557627198103830 ) ) ;
#29889=CARTESIAN_POINT ( 'NONE',  ( -19.02544592524342804, 5.153800228976336051, 111.0405762719810099 ) ) ;
#29890=CARTESIAN_POINT ( 'NONE',  ( -16.53943276465976808, 0.05219959533911058130, 71.24890960531435269 ) ) ;
#29891=CARTESIAN_POINT ( 'NONE',  ( 19.02544592524343514, -5.153800228976328945, 48.54057627198103120 ) ) ;
#29892=CARTESIAN_POINT ( 'NONE',  ( -19.03943276465977164, -0.05219959533935918106, 28.75109039468566507 ) ) ;
#29893=CARTESIAN_POINT ( 'NONE',  ( 12.14591786802327356, -12.06949235617739191, 105.6260903946856899 ) ) ;
#29894=CARTESIAN_POINT ( 'NONE',  ( -4.379528057220086978, -16.55341960407618274, 54.79275706135235424 ) ) ;
#29895=CARTESIAN_POINT ( 'NONE',  ( 0.05219959533907565091, 21.53943276465977519, 39.99890960531436690 ) ) ;
#29896=CARTESIAN_POINT ( 'NONE',  ( -19.03943276465977164, -0.05219959533935918106, 18.75109039468567218 ) ) ;
#29897=CARTESIAN_POINT ( 'NONE',  ( -19.02544592524342804, 5.153800228976336051, 86.04057627198103830 ) ) ;
#29898=CARTESIAN_POINT ( 'NONE',  ( -12.06949235617739369, -12.14591786802326823, 69.37609039468567573 ) ) ;
#29899=CARTESIAN_POINT ( 'NONE',  ( -16.46253265017160317, 9.564922557960807481, 25.83224293864769194 ) ) ;
#29900=CARTESIAN_POINT ( 'NONE',  ( 14.29746914071049879, -8.314922557960816363, 28.33224293864769550 ) ) ;
#29901=CARTESIAN_POINT ( 'NONE',  ( 0.05219959533909260263, 19.03943276465977164, 99.99890960531436690 ) ) ;
#29902=CARTESIAN_POINT ( 'NONE',  ( 13.97604488694527802, 13.89961937509977652, 94.37390960531436690 ) ) ;
#29903=CARTESIAN_POINT ( 'NONE',  ( -10.72451020669898014, 18.67979575497178502, 25.41557627198103120 ) ) ;
#29904=CARTESIAN_POINT ( 'NONE',  ( -0.05219959533910754901, -16.53943276465976808, 57.49890960531435979 ) ) ;
#29905=CARTESIAN_POINT ( 'NONE',  ( 12.06949235617757843, -12.14591786802309237, 38.12390960531436690 ) ) ;
#29907=CARTESIAN_POINT ( 'NONE',  ( -14.29746914071049879, 8.314922557960819915, 45.83224293864769550 ) ) ;
#29908=CARTESIAN_POINT ( 'NONE',  ( 16.53943276465976808, 0.05219959533934440121, 41.25109039468568284 ) ) ;
#29909=CARTESIAN_POINT ( 'NONE',  ( 17.50000000000001776, -4.049696124445805623, 31.68039670665950780 ) ) ;
#29910=CARTESIAN_POINT ( 'NONE',  ( -13.97604488694547697, 13.89961937509957934, 53.12609039468565442 ) ) ;
#29911=CARTESIAN_POINT ( 'NONE',  ( -13.89961937509977652, 13.97604488694528158, 95.62390960531436690 ) ) ;
#29912=CARTESIAN_POINT ( 'NONE',  ( -0.05219959533936034679, 19.03943276465977164, 62.50109039468566863 ) ) ;
#29914=CARTESIAN_POINT ( 'NONE',  ( 5.153800228976615827, -19.02544592524334988, 55.20942372801899722 ) ) ;
#29915=CARTESIAN_POINT ( 'NONE',  ( -19.03943276465977164, -0.05219959533935918106, 98.75109039468567573 ) ) ;
#29916=CARTESIAN_POINT ( 'NONE',  ( 12.06949235617739724, 12.14591786802326823, 81.87609039468568994 ) ) ;
#29918=CARTESIAN_POINT ( 'NONE',  ( 9.474510206698971260, -16.51473224551069308, 22.91557627198102765 ) ) ;
#29919=CARTESIAN_POINT ( 'NONE',  ( -16.51473224551069308, -9.474510206698971260, 111.6655762719810383 ) ) ;
#29920=CARTESIAN_POINT ( 'NONE',  ( -18.62759615963255300, -10.81492255796106328, 39.16775706135235424 ) ) ;
#29921=CARTESIAN_POINT ( 'NONE',  ( 13.97604488694548053, -13.89961937509957401, 100.6260903946856615 ) ) ;
#29922=CARTESIAN_POINT ( 'NONE',  ( 17.50000000000000000, -5.500000000000000888, 108.2969038253417153 ) ) ;
#29923=CARTESIAN_POINT ( 'NONE',  ( 0.05219959533909260263, 19.03943276465977164, 64.99890960531436690 ) ) ;
#29925=CARTESIAN_POINT ( 'NONE',  ( 16.51473224551069308, 9.474510206698969483, 104.1655762719810241 ) ) ;
#29926=CARTESIAN_POINT ( 'NONE',  ( 8.314922557960818139, 14.29746914071049879, 69.58224293864769550 ) ) ;
#29927=CARTESIAN_POINT ( 'NONE',  ( 16.46253265017160672, -9.564922557960803928, 58.33224293864769550 ) ) ;
#29928=CARTESIAN_POINT ( 'NONE',  ( -9.474510206698964154, 16.51473224551069663, 70.41557627198102409 ) ) ;
#29929=CARTESIAN_POINT ( 'NONE',  ( -9.564922557961040184, 16.46253265017147172, 82.91775706135233293 ) ) ;
#29930=CARTESIAN_POINT ( 'NONE',  ( -10.81492255796078084, -18.62759615963271287, 52.08224293864768839 ) ) ;
#29931=CARTESIAN_POINT ( 'NONE',  ( -5.153800228976328057, -19.02544592524343514, 22.29057627198102765 ) ) ;
#29932=CARTESIAN_POINT ( 'NONE',  ( 9.474510206698729675, 16.51473224551082808, 37.08442372801899722 ) ) ;
#29933=CARTESIAN_POINT ( 'NONE',  ( 13.97604488694527802, 13.89961937509977652, 74.37390960531436690 ) ) ;
#29934=CARTESIAN_POINT ( 'NONE',  ( -21.55341960407610458, -5.719274019375992779, 71.45724293864769550 ) ) ;
#29935=CARTESIAN_POINT ( 'NONE',  ( -16.52544592524342804, 4.483927247898546575, 81.04057627198102409 ) ) ;
#29936=CARTESIAN_POINT ( 'NONE',  ( -5.153800228976607833, 19.02544592524334988, 47.70942372801900433 ) ) ;
#29937=CARTESIAN_POINT ( 'NONE',  ( -5.823673210054116645, -21.52544592524344225, 72.29057627198102409 ) ) ;
#29938=CARTESIAN_POINT ( 'NONE',  ( -10.72451020669898014, 18.67979575497178502, 60.41557627198102409 ) ) ;
#29939=CARTESIAN_POINT ( 'NONE',  ( 15.72974639402199770, -15.80617190586745480, 33.12390960531435979 ) ) ;
#29940=CARTESIAN_POINT ( 'NONE',  ( -18.67979575497193778, 10.72451020669871902, 93.33442372801901854 ) ) ;
#29941=CARTESIAN_POINT ( 'NONE',  ( 19.02544592524343514, -5.153800228976328945, 63.54057627198103830 ) ) ;
#29942=CARTESIAN_POINT ( 'NONE',  ( 9.564922557960805705, 16.46253265017160317, 24.58224293864769194 ) ) ;
#29943=CARTESIAN_POINT ( 'NONE',  ( -15.80617190586768217, 15.72974639402176855, 28.12609039468568284 ) ) ;
#29945=CARTESIAN_POINT ( 'NONE',  ( 21.53943276465977519, 0.05219959533937863772, 46.25109039468567573 ) ) ;
#29946=CARTESIAN_POINT ( 'NONE',  ( -13.89961937509977652, 13.97604488694528158, 35.62390960531435269 ) ) ;
#29947=CARTESIAN_POINT ( 'NONE',  ( -18.67979575497178146, -10.72451020669898902, 106.6655762719810383 ) ) ;
#29948=CARTESIAN_POINT ( 'NONE',  ( -13.89961937509957401, -13.97604488694547875, 54.37609039468565442 ) ) ;
#29949=EDGE_CURVE ( 'NONE', #11857, #161202, #199201, .T. ) ;
#29950=CARTESIAN_POINT ( 'NONE',  ( 13.89961937509977652, -13.97604488694527269, 33.12390960531434558 ) ) ;
#29951=CARTESIAN_POINT ( 'NONE',  ( 13.97604488694527802, 13.89961937509977652, 29.37390960531435979 ) ) ;
#29953=CARTESIAN_POINT ( 'NONE',  ( -16.52544592524335698, -4.483927247898792601, 63.95942372801901854 ) ) ;
#29954=CARTESIAN_POINT ( 'NONE',  ( 9.474510206698971260, -16.51473224551069308, 22.91557627198102765 ) ) ;
#29956=CARTESIAN_POINT ( 'NONE',  ( 5.049401038298161559, -19.05341960407611168, 87.70724293864769550 ) ) ;
#29957=CARTESIAN_POINT ( 'NONE',  ( -8.224510206698948167, 14.34966873604960824, 110.4155762719810383 ) ) ;
#29959=CARTESIAN_POINT ( 'NONE',  ( 21.53943276465977519, -0.05219959533907433946, 53.74890960531437401 ) ) ;
#29960=CARTESIAN_POINT ( 'NONE',  ( -8.314922557961024197, 14.29746914071037800, 42.91775706135235424 ) ) ;
#29961=CARTESIAN_POINT ( 'NONE',  ( -15.80617190586768217, 15.72974639402176855, 98.12609039468570415 ) ) ;
#29962=CARTESIAN_POINT ( 'NONE',  ( 16.46253265017160672, -9.564922557960803928, 23.33224293864769194 ) ) ;
#29963=CARTESIAN_POINT ( 'NONE',  ( 8.314922557961029526, -14.29746914071037800, 105.4177570613523613 ) ) ;
#29964=CARTESIAN_POINT ( 'NONE',  ( 8.224510206698953496, -14.34966873604960469, 52.91557627198103830 ) ) ;
#29965=CARTESIAN_POINT ( 'NONE',  ( 16.46253265017160672, -9.564922557960803928, 58.33224293864769550 ) ) ;
#29966=CARTESIAN_POINT ( 'NONE',  ( -10.81492255796105439, 18.62759615963255655, 112.9177570613523329 ) ) ;
#29967=CARTESIAN_POINT ( 'NONE',  ( 10.81492255796106328, -18.62759615963255655, 25.41775706135235779 ) ) ;
#29968=CARTESIAN_POINT ( 'NONE',  ( -10.81492255796105439, 18.62759615963255655, 72.91775706135234714 ) ) ;
#29969=CARTESIAN_POINT ( 'NONE',  ( -4.379528057220086978, -16.55341960407618274, 54.79275706135235424 ) ) ;
#29970=CARTESIAN_POINT ( 'NONE',  ( -4.483927247898782831, 16.52544592524335698, 32.70942372801900433 ) ) ;
#29971=CARTESIAN_POINT ( 'NONE',  ( 8.224510206698953496, -14.34966873604960469, 72.91557627198103830 ) ) ;
#29972=CARTESIAN_POINT ( 'NONE',  ( 18.67979575497194134, -10.72451020669871369, 100.8344237280190185 ) ) ;
#29973=CARTESIAN_POINT ( 'NONE',  ( 16.53943276465976808, -0.05219959533910856209, 28.74890960531435624 ) ) ;
#29974=CARTESIAN_POINT ( 'NONE',  ( -17.31747979337947285, 6.344076630961062335, 113.6205513193481522 ) ) ;
#29975=CARTESIAN_POINT ( 'NONE',  ( -12.06949235617739369, -12.14591786802326823, 44.37609039468567573 ) ) ;
#29976=CARTESIAN_POINT ( 'NONE',  ( 12.14591786802309770, 12.06949235617756955, 44.37390960531435979 ) ) ;
#29977=CARTESIAN_POINT ( 'NONE',  ( 8.314922557961029526, -14.29746914071037800, 85.41775706135236135 ) ) ;
#29978=CARTESIAN_POINT ( 'NONE',  ( 9.474510206698971260, -16.51473224551069308, 92.91557627198103830 ) ) ;
#29979=CARTESIAN_POINT ( 'NONE',  ( 21.52544592524344225, -5.823673210054117533, 23.54057627198102765 ) ) ;
#29980=CARTESIAN_POINT ( 'NONE',  ( 10.81492255796106328, -18.62759615963255655, 100.4177570613523471 ) ) ;
#29981=CARTESIAN_POINT ( 'NONE',  ( -12.14591786802326823, 12.06949235617739902, 98.12609039468570415 ) ) ;
#29982=CARTESIAN_POINT ( 'NONE',  ( -16.52544592524342804, 4.483927247898546575, 91.04057627198103830 ) ) ;
#29983=CARTESIAN_POINT ( 'NONE',  ( 5.049401038298161559, -19.05341960407611168, 87.70724293864769550 ) ) ;
#29984=VERTEX_POINT ( 'NONE', #189332 ) ;
#29985=CARTESIAN_POINT ( 'NONE',  ( 16.52544592524335698, 4.483927247898782831, 36.45942372801901143 ) ) ;
#29986=CARTESIAN_POINT ( 'NONE',  ( 13.89961937509977652, -13.97604488694527269, 43.12390960531434558 ) ) ;
#29987=CARTESIAN_POINT ( 'NONE',  ( -9.474510206698964154, 16.51473224551069663, 110.4155762719810383 ) ) ;
#29988=CARTESIAN_POINT ( 'NONE',  ( -12.06949235617739369, -12.14591786802326823, 34.37609039468568284 ) ) ;
#29990=CARTESIAN_POINT ( 'NONE',  ( -16.51473224551082808, 9.474510206698731452, 38.33442372801899722 ) ) ;
#29991=CARTESIAN_POINT ( 'NONE',  ( -16.53943276465976808, -0.05219959533934237506, 108.7510903946857042 ) ) ;
#29992=CARTESIAN_POINT ( 'NONE',  ( -13.97604488694527625, -13.89961937509977652, 36.87390960531436690 ) ) ;
#29993=CARTESIAN_POINT ( 'NONE',  ( -4.483927247898782831, 16.52544592524335698, 72.70942372801901854 ) ) ;
#29994=CARTESIAN_POINT ( 'NONE',  ( 19.05341960407617918, -5.049401038297876454, 76.04275706135230450 ) ) ;
#29995=CARTESIAN_POINT ( 'NONE',  ( 16.51473224551083163, -9.474510206698727899, 30.83442372801900433 ) ) ;
#29996=CARTESIAN_POINT ( 'NONE',  ( 9.474510206698971260, -16.51473224551069308, 62.91557627198102409 ) ) ;
#29997=CARTESIAN_POINT ( 'NONE',  ( -12.14591786802309592, -12.06949235617757132, 81.87390960531435269 ) ) ;
#29998=EDGE_CURVE ( 'NONE', #64402, #12092, #51792, .T. ) ;
#29999=CARTESIAN_POINT ( 'NONE',  ( 5.049401038297881783, 19.05341960407617563, 62.29275706135234003 ) ) ;
#30000=CARTESIAN_POINT ( 'NONE',  ( 21.53943276465977519, -0.05219959533907433946, 58.74890960531436690 ) ) ;
#30001=CARTESIAN_POINT ( 'NONE',  ( -9.474510206698720793, -16.51473224551083518, 34.58442372801899722 ) ) ;
#30002=CARTESIAN_POINT ( 'NONE',  ( 5.153800228976335163, 19.02544592524342804, 109.7905762719810099 ) ) ;
#30003=CARTESIAN_POINT ( 'NONE',  ( 5.719274019375991003, -21.55341960407610458, 77.70724293864770971 ) ) ;
#30004=CARTESIAN_POINT ( 'NONE',  ( -9.474510206698964154, 16.51473224551069663, 105.4155762719810383 ) ) ;
#30005=CARTESIAN_POINT ( 'NONE',  ( -16.46253265017146816, -9.564922557961047289, 104.1677570613523329 ) ) ;
#30006=CARTESIAN_POINT ( 'NONE',  ( -17.50000000000000355, 5.076555817581250629, 108.8204850795023049 ) ) ;
#30007=CARTESIAN_POINT ( 'NONE',  ( 12.06949235617739724, 12.14591786802326823, 31.87609039468567929 ) ) ;
#30008=CARTESIAN_POINT ( 'NONE',  ( 19.03943276465977164, -0.05219959533909143690, 38.74890960531436690 ) ) ;
#30009=CARTESIAN_POINT ( 'NONE',  ( 19.02544592524343514, -5.153800228976328945, 98.54057627198100988 ) ) ;
#30010=CARTESIAN_POINT ( 'NONE',  ( -15.80617190586745835, -15.72974639402198527, 81.87390960531435269 ) ) ;
#30011=CARTESIAN_POINT ( 'NONE',  ( 14.34966873604972726, -8.224510206698740333, 55.83442372801901854 ) ) ;
#30012=CARTESIAN_POINT ( 'NONE',  ( -10.72451020669870658, -18.67979575497194134, 59.58442372801901854 ) ) ;
#30013=CARTESIAN_POINT ( 'NONE',  ( -16.46253265017146816, -9.564922557961047289, 109.1677570613523471 ) ) ;
#30014=CARTESIAN_POINT ( 'NONE',  ( 21.53943276465977519, 0.05219959533937863772, 106.2510903946856757 ) ) ;
#30015=CARTESIAN_POINT ( 'NONE',  ( -16.53943276465976808, 0.05219959533911058130, 21.24890960531436690 ) ) ;
#30016=CARTESIAN_POINT ( 'NONE',  ( 10.81492255796078972, 18.62759615963270932, 94.58224293864769550 ) ) ;
#30017=CARTESIAN_POINT ( 'NONE',  ( -16.55341960407611168, -4.379528057220339221, 41.45724293864769550 ) ) ;
#30018=CARTESIAN_POINT ( 'NONE',  ( 16.46253265017146816, 9.564922557961045513, 81.66775706135233293 ) ) ;
#30019=CARTESIAN_POINT ( 'NONE',  ( -15.80617190586768217, 15.72974639402176855, 53.12609039468568284 ) ) ;
#30020=CARTESIAN_POINT ( 'NONE',  ( -19.02544592524334988, -5.153800228976617603, 43.95942372801899012 ) ) ;
#30021=CARTESIAN_POINT ( 'NONE',  ( -16.53943276465976808, 0.05219959533911058130, 106.2489096053143811 ) ) ;
#30022=CARTESIAN_POINT ( 'NONE',  ( 10.72451020669898902, -18.67979575497178502, 27.91557627198103830 ) ) ;
#30023=CARTESIAN_POINT ( 'NONE',  ( 14.34966873604960469, 8.224510206698951720, 34.16557627198102409 ) ) ;
#30024=CARTESIAN_POINT ( 'NONE',  ( 18.67979575497194134, -10.72451020669871369, 95.83442372801903275 ) ) ;
#30025=CARTESIAN_POINT ( 'NONE',  ( -0.05219959533934338120, 16.53943276465976808, 77.50109039468567573 ) ) ;
#30026=CARTESIAN_POINT ( 'NONE',  ( -4.483927247898539470, -16.52544592524342804, 27.29057627198103120 ) ) ;
#30027=CARTESIAN_POINT ( 'NONE',  ( 21.52544592524334988, 5.823673210054432836, 66.45942372801903275 ) ) ;
#30028=CARTESIAN_POINT ( 'NONE',  ( 5.719274019375673035, 21.55341960407619339, 52.29275706135236135 ) ) ;
#30029=CARTESIAN_POINT ( 'NONE',  ( 13.89961937509977652, -13.97604488694527269, 28.12390960531435624 ) ) ;
#30030=CARTESIAN_POINT ( 'NONE',  ( -5.719274019375665041, -21.55341960407619695, 39.79275706135235424 ) ) ;
#30031=CARTESIAN_POINT ( 'NONE',  ( 8.224510206698953496, -14.34966873604960469, 112.9155762719810383 ) ) ;
#30032=CARTESIAN_POINT ( 'NONE',  ( 5.153800228976335163, 19.02544592524342804, 39.79057627198100988 ) ) ;
#30033=CARTESIAN_POINT ( 'NONE',  ( 16.55341960407611168, 4.379528057220329451, 78.95724293864769550 ) ) ;
#30034=CARTESIAN_POINT ( 'NONE',  ( -5.153800228976328057, -19.02544592524343514, 77.29057627198099567 ) ) ;
#30035=CARTESIAN_POINT ( 'NONE',  ( -8.314922557960811034, -14.29746914071050412, 32.08224293864769550 ) ) ;
#30036=CARTESIAN_POINT ( 'NONE',  ( -0.05219959533907301413, -21.53943276465977519, 62.49890960531436690 ) ) ;
#30037=CARTESIAN_POINT ( 'NONE',  ( -15.72974639402197994, 15.80617190586746368, 110.6239096053143669 ) ) ;
#30038=CARTESIAN_POINT ( 'NONE',  ( 16.51473224551069308, 9.474510206698969483, 99.16557627198102409 ) ) ;
#30039=CARTESIAN_POINT ( 'NONE',  ( -0.05219959533909027116, -19.03943276465977164, 62.49890960531435979 ) ) ;
#30040=CARTESIAN_POINT ( 'NONE',  ( -13.89961937509957401, -13.97604488694547875, 99.37609039468567573 ) ) ;
#30041=CARTESIAN_POINT ( 'NONE',  ( 15.72974639402199770, -15.80617190586745480, 58.12390960531435979 ) ) ;
#30042=CARTESIAN_POINT ( 'NONE',  ( 15.72974639402176855, 15.80617190586768217, 81.87609039468568994 ) ) ;
#30043=CARTESIAN_POINT ( 'NONE',  ( 16.46253265017160672, -9.564922557960803928, 68.33224293864770971 ) ) ;
#30044=CARTESIAN_POINT ( 'NONE',  ( -13.89961937509977652, 13.97604488694528158, 100.6239096053143669 ) ) ;
#30045=CARTESIAN_POINT ( 'NONE',  ( -12.14591786802326823, 12.06949235617739902, 78.12609039468570415 ) ) ;
#30046=CARTESIAN_POINT ( 'NONE',  ( -15.72974639402176322, -15.80617190586768395, 54.37609039468568994 ) ) ;
#30047=CARTESIAN_POINT ( 'NONE',  ( -10.81492255796105439, 18.62759615963255655, 87.91775706135234714 ) ) ;
#30048=CARTESIAN_POINT ( 'NONE',  ( 5.719274019375991003, -21.55341960407610458, 112.7072429386476955 ) ) ;
#30049=CARTESIAN_POINT ( 'NONE',  ( -16.55341960407617563, 4.379528057220093196, 83.54275706135234714 ) ) ;
#30050=CARTESIAN_POINT ( 'NONE',  ( 5.719274019375991003, -21.55341960407610458, 72.70724293864769550 ) ) ;
#30051=CARTESIAN_POINT ( 'NONE',  ( 13.89961937509957401, 13.97604488694547697, 46.87609039468565442 ) ) ;
#30052=CARTESIAN_POINT ( 'NONE',  ( -21.55341960407610458, -5.719274019375992779, 41.45724293864769550 ) ) ;
#30053=CARTESIAN_POINT ( 'NONE',  ( 16.51473224551069308, 9.474510206698969483, 84.16557627198102409 ) ) ;
#30054=CARTESIAN_POINT ( 'NONE',  ( 4.483927247898545687, 16.52544592524342804, 29.79057627198102409 ) ) ;
#30055=CARTESIAN_POINT ( 'NONE',  ( 5.719274019375991003, -21.55341960407610458, 27.70724293864769905 ) ) ;
#30058=CARTESIAN_POINT ( 'NONE',  ( -9.564922557961040184, 16.46253265017147172, 92.91775706135233293 ) ) ;
#30059=CARTESIAN_POINT ( 'NONE',  ( -18.62759615963270932, 10.81492255796079327, 70.83224293864770971 ) ) ;
#30060=CARTESIAN_POINT ( 'NONE',  ( 16.55341960407611168, 4.379528057220329451, 48.95724293864770971 ) ) ;
#30061=CARTESIAN_POINT ( 'NONE',  ( 16.46253265017146816, 9.564922557961045513, 106.6677570613523471 ) ) ;
#30062=CARTESIAN_POINT ( 'NONE',  ( 16.51473224551069308, 9.474510206698969483, 39.16557627198103120 ) ) ;
#30063=CARTESIAN_POINT ( 'NONE',  ( 21.55341960407610458, 5.719274019375980345, 98.95724293864770971 ) ) ;
#30064=CARTESIAN_POINT ( 'NONE',  ( 19.03943276465977164, 0.05219959533936151252, 71.25109039468566152 ) ) ;
#30065=CARTESIAN_POINT ( 'NONE',  ( 16.46253265017160672, -9.564922557960803928, 88.33224293864769550 ) ) ;
#30066=CARTESIAN_POINT ( 'NONE',  ( -16.53943276465976808, 0.05219959533911058130, 91.24890960531436690 ) ) ;
#30067=CARTESIAN_POINT ( 'NONE',  ( -19.05341960407611168, -5.049401038298163336, 61.45724293864769550 ) ) ;
#30068=CARTESIAN_POINT ( 'NONE',  ( -8.314922557960811034, -14.29746914071050412, 67.08224293864770971 ) ) ;
#30069=CARTESIAN_POINT ( 'NONE',  ( -9.564922557960796823, -16.46253265017161027, 37.08224293864768839 ) ) ;
#30071=CARTESIAN_POINT ( 'NONE',  ( 16.55341960407611168, 4.379528057220329451, 43.95724293864769550 ) ) ;
#30072=CARTESIAN_POINT ( 'NONE',  ( -19.02544592524342804, 5.153800228976336051, 86.04057627198103830 ) ) ;
#30074=CARTESIAN_POINT ( 'NONE',  ( -9.564922557961040184, 16.46253265017147172, 57.91775706135233293 ) ) ;
#30075=CARTESIAN_POINT ( 'NONE',  ( 8.314922557961029526, -14.29746914071037800, 65.41775706135234714 ) ) ;
#30076=CARTESIAN_POINT ( 'NONE',  ( 10.72451020669898902, -18.67979575497178502, 67.91557627198102409 ) ) ;
#30077=CARTESIAN_POINT ( 'NONE',  ( -16.51473224551082808, 9.474510206698731452, 33.33442372801899722 ) ) ;
#30078=CARTESIAN_POINT ( 'NONE',  ( -19.02544592524342804, 5.153800228976336051, 91.04057627198100988 ) ) ;
#30080=CARTESIAN_POINT ( 'NONE',  ( -18.62759615963270932, 10.81492255796079327, 25.83224293864769194 ) ) ;
#30081=CARTESIAN_POINT ( 'NONE',  ( -9.474510206698964154, 16.51473224551069663, 60.41557627198102409 ) ) ;
#30082=CARTESIAN_POINT ( 'NONE',  ( 18.67979575497194134, -10.72451020669871369, 45.83442372801901854 ) ) ;
#30083=CARTESIAN_POINT ( 'NONE',  ( 19.05341960407611168, 5.049401038298154454, 28.95724293864769550 ) ) ;
#30084=CARTESIAN_POINT ( 'NONE',  ( -18.67979575497178146, -10.72451020669898902, 101.6655762719810383 ) ) ;
#30085=CARTESIAN_POINT ( 'NONE',  ( 19.05341960407611168, 5.049401038298154454, 88.95724293864769550 ) ) ;
#30086=ORIENTED_EDGE ( 'NONE', *, *, #85875, .T. ) ;
#30087=CARTESIAN_POINT ( 'NONE',  ( 15.72974639402176855, 15.80617190586768217, 41.87609039468568284 ) ) ;
#30089=CARTESIAN_POINT ( 'NONE',  ( -13.89961937509977652, 13.97604488694528158, 100.6239096053143669 ) ) ;
#30092=CARTESIAN_POINT ( 'NONE',  ( -17.49999999999999645, -5.500000000000000888, 109.2030961746582847 ) ) ;
#30093=CARTESIAN_POINT ( 'NONE',  ( -0.05219959533907301413, -21.53943276465977519, 112.4989096053143669 ) ) ;
#30094=CARTESIAN_POINT ( 'NONE',  ( -13.97604488694527625, -13.89961937509977652, 41.87390960531435979 ) ) ;
#30095=CARTESIAN_POINT ( 'NONE',  ( -16.52544592524335698, -4.483927247898792601, 23.95942372801901143 ) ) ;
#30097=CARTESIAN_POINT ( 'NONE',  ( 13.97604488694527802, 13.89961937509977652, 34.37390960531436690 ) ) ;
#30098=CARTESIAN_POINT ( 'NONE',  ( -21.55341960407619339, 5.719274019375674811, 98.54275706135234714 ) ) ;
#30099=CARTESIAN_POINT ( 'NONE',  ( -5.153800228976328057, -19.02544592524343514, 77.29057627198099567 ) ) ;
#30100=CARTESIAN_POINT ( 'NONE',  ( -21.52544592524334988, -5.823673210054445271, 43.95942372801902565 ) ) ;
#30102=CARTESIAN_POINT ( 'NONE',  ( 9.564922557960805705, 16.46253265017160317, 94.58224293864769550 ) ) ;
#30103=CARTESIAN_POINT ( 'NONE',  ( 19.49190055781010145, 5.500000000000047962, 63.06116087098784107 ) ) ;
#30104=CARTESIAN_POINT ( 'NONE',  ( 14.34966873604972726, -8.224510206698740333, 45.83442372801901854 ) ) ;
#30105=CARTESIAN_POINT ( 'NONE',  ( -16.53943276465976808, -0.05219959533934237506, 73.75109039468567573 ) ) ;
#30106=CARTESIAN_POINT ( 'NONE',  ( -0.05219959533937732626, 21.53943276465977519, 57.50109039468568994 ) ) ;
#30107=CARTESIAN_POINT ( 'NONE',  ( 15.72974639402176855, 15.80617190586768217, 91.87609039468568994 ) ) ;
#30109=CARTESIAN_POINT ( 'NONE',  ( -5.049401038297874678, -19.05341960407617918, 104.7927570613523471 ) ) ;
#30110=CARTESIAN_POINT ( 'NONE',  ( -9.564922557960796823, -16.46253265017161027, 72.08224293864770971 ) ) ;
#30111=CARTESIAN_POINT ( 'NONE',  ( 19.03943276465977164, -0.05219959533909143690, 98.74890960531436690 ) ) ;
#30112=CARTESIAN_POINT ( 'NONE',  ( -16.55341960407611168, -4.379528057220339221, 111.4572429386476813 ) ) ;
#30113=CARTESIAN_POINT ( 'NONE',  ( 21.55341960407610458, 5.719274019375980345, 28.95724293864769905 ) ) ;
#30114=CARTESIAN_POINT ( 'NONE',  ( 16.52544592524335698, 4.483927247898782831, 91.45942372801901854 ) ) ;
#30115=CARTESIAN_POINT ( 'NONE',  ( -12.06949235617756955, 12.14591786802309770, 75.62390960531439532 ) ) ;
#30116=CARTESIAN_POINT ( 'NONE',  ( 19.05341960407611168, 5.049401038298154454, 53.95724293864770260 ) ) ;
#30117=CARTESIAN_POINT ( 'NONE',  ( 10.81492255796106328, -18.62759615963255655, 75.41775706135233293 ) ) ;
#30119=CARTESIAN_POINT ( 'NONE',  ( 16.46253265017146816, 9.564922557961045513, 101.6677570613523329 ) ) ;
#30120=CARTESIAN_POINT ( 'NONE',  ( -12.14591786802309592, -12.06949235617757132, 76.87390960531439532 ) ) ;
#30121=CARTESIAN_POINT ( 'NONE',  ( 15.72974639402176855, 15.80617190586768217, 31.87609039468567929 ) ) ;
#30122=CARTESIAN_POINT ( 'NONE',  ( 5.719274019375991003, -21.55341960407610458, 57.70724293864770260 ) ) ;
#30123=CARTESIAN_POINT ( 'NONE',  ( -13.97604488694547697, 13.89961937509957934, 33.12609039468566863 ) ) ;
#30125=CARTESIAN_POINT ( 'NONE',  ( 13.89961937509977652, -13.97604488694527269, 88.12390960531438111 ) ) ;
#30126=CARTESIAN_POINT ( 'NONE',  ( -16.53943276465976808, 0.05219959533911058130, 51.24890960531436690 ) ) ;
#30127=CARTESIAN_POINT ( 'NONE',  ( 0.05219959533910956823, 16.53943276465976808, 39.99890960531436690 ) ) ;
#30128=CARTESIAN_POINT ( 'NONE',  ( -14.29746914071037622, -8.314922557961029526, 94.16775706135237556 ) ) ;
#30129=CARTESIAN_POINT ( 'NONE',  ( -0.05219959533936034679, 19.03943276465977164, 47.50109039468566863 ) ) ;
#30130=CARTESIAN_POINT ( 'NONE',  ( 9.474510206698729675, 16.51473224551082808, 77.08442372801900433 ) ) ;
#30131=CARTESIAN_POINT ( 'NONE',  ( 19.05341960407611168, 5.049401038298154454, 98.95724293864766707 ) ) ;
#30132=CARTESIAN_POINT ( 'NONE',  ( 16.53943276465976808, -0.05219959533910856209, 68.74890960531435269 ) ) ;
#30133=CARTESIAN_POINT ( 'NONE',  ( -16.46253265017146816, -9.564922557961047289, 49.16775706135233293 ) ) ;
#30134=CARTESIAN_POINT ( 'NONE',  ( 19.05341960407611168, 5.049401038298154454, 28.95724293864769550 ) ) ;
#30135=CARTESIAN_POINT ( 'NONE',  ( -21.53943276465977519, 0.05219959533907696930, 36.24890960531435979 ) ) ;
#30136=CARTESIAN_POINT ( 'NONE',  ( -5.823673210054116645, -21.52544592524344225, 62.29057627198102409 ) ) ;
#30137=CARTESIAN_POINT ( 'NONE',  ( 14.29746914071049879, -8.314922557960816363, 98.33224293864769550 ) ) ;
#30138=CARTESIAN_POINT ( 'NONE',  ( 4.379528057220092307, 16.55341960407617563, 52.29275706135236135 ) ) ;
#30139=CARTESIAN_POINT ( 'NONE',  ( 5.823673210054444382, -21.52544592524334988, 35.20942372801901854 ) ) ;
#30140=CARTESIAN_POINT ( 'NONE',  ( -12.06949235617756955, 12.14591786802309770, 85.62390960531436690 ) ) ;
#30143=CARTESIAN_POINT ( 'NONE',  ( 18.62759615963271287, -10.81492255796078972, 38.33224293864768839 ) ) ;
#30146=CARTESIAN_POINT ( 'NONE',  ( -14.29746914071037622, -8.314922557961029526, 39.16775706135235424 ) ) ;
#30147=CARTESIAN_POINT ( 'NONE',  ( 8.314922557960818139, 14.29746914071049879, 29.58224293864769905 ) ) ;
#30148=CARTESIAN_POINT ( 'NONE',  ( 21.55341960407610458, 5.719274019375980345, 68.95724293864769550 ) ) ;
#30150=CARTESIAN_POINT ( 'NONE',  ( 13.97604488694548053, -13.89961937509957401, 90.62609039468567573 ) ) ;
#30151=CARTESIAN_POINT ( 'NONE',  ( 21.53943276465977519, -0.05219959533907433946, 68.74890960531435269 ) ) ;
#30153=CARTESIAN_POINT ( 'NONE',  ( -0.05219959533909027116, -19.03943276465977164, 42.49890960531435269 ) ) ;
#30154=CARTESIAN_POINT ( 'NONE',  ( -19.02544592524342804, 5.153800228976336051, 96.04057627198103830 ) ) ;
#30155=CARTESIAN_POINT ( 'NONE',  ( -13.97604488694527625, -13.89961937509977652, 41.87390960531435979 ) ) ;
#30156=CARTESIAN_POINT ( 'NONE',  ( 9.474510206698971260, -16.51473224551069308, 22.91557627198102765 ) ) ;
#30158=CARTESIAN_POINT ( 'NONE',  ( 0.05219959533909260263, 19.03943276465977164, 109.9989096053143669 ) ) ;
#30160=CARTESIAN_POINT ( 'NONE',  ( -16.55341960407617563, 4.379528057220093196, 68.54275706135234714 ) ) ;
#30161=CARTESIAN_POINT ( 'NONE',  ( 5.823673210054125526, 21.52544592524343514, 94.79057627198105251 ) ) ;
#30162=CARTESIAN_POINT ( 'NONE',  ( -5.049401038298153566, 19.05341960407611168, 60.20724293864768129 ) ) ;
#30163=CARTESIAN_POINT ( 'NONE',  ( 0.05219959533937995610, -21.53943276465977519, 30.00109039468568284 ) ) ;
#30164=CARTESIAN_POINT ( 'NONE',  ( -19.02544592524342804, 5.153800228976336051, 81.04057627198103830 ) ) ;
#30165=CARTESIAN_POINT ( 'NONE',  ( -13.89961937509977652, 13.97604488694528158, 115.6239096053143669 ) ) ;
#30166=VERTEX_POINT ( 'NONE', #158963 ) ;
#30167=CARTESIAN_POINT ( 'NONE',  ( 5.823673210054444382, -21.52544592524334988, 20.20942372801900788 ) ) ;
#30168=CARTESIAN_POINT ( 'NONE',  ( -19.05341960407611168, -5.049401038298163336, 21.45724293864768839 ) ) ;
#30169=CARTESIAN_POINT ( 'NONE',  ( -13.89961937509977652, 13.97604488694528158, 100.6239096053143669 ) ) ;
#30170=CARTESIAN_POINT ( 'NONE',  ( 0.05219959533936267826, -19.03943276465977164, 90.00109039468567573 ) ) ;
#30172=CARTESIAN_POINT ( 'NONE',  ( -5.049401038297874678, -19.05341960407617918, 24.79275706135233648 ) ) ;
#30173=CARTESIAN_POINT ( 'NONE',  ( -5.719274019375978568, 21.55341960407610458, 95.20724293864769550 ) ) ;
#30174=CARTESIAN_POINT ( 'NONE',  ( 19.02544592524334988, 5.153800228976608722, 31.45942372801900433 ) ) ;
#30175=CARTESIAN_POINT ( 'NONE',  ( -8.224510206698735004, -14.34966873604973081, 84.58442372801903275 ) ) ;
#30176=CARTESIAN_POINT ( 'NONE',  ( 5.153800228976335163, 19.02544592524342804, 104.7905762719809957 ) ) ;
#30177=CARTESIAN_POINT ( 'NONE',  ( -0.05219959533909027116, -19.03943276465977164, 57.49890960531435979 ) ) ;
#30178=CARTESIAN_POINT ( 'NONE',  ( 5.823673210054444382, -21.52544592524334988, 65.20942372801901854 ) ) ;
#30179=CARTESIAN_POINT ( 'NONE',  ( -18.67979575497193778, 10.72451020669871902, 78.33442372801901854 ) ) ;
#30181=CARTESIAN_POINT ( 'NONE',  ( 13.89961937509977652, -13.97604488694527269, 78.12390960531433848 ) ) ;
#30182=CARTESIAN_POINT ( 'NONE',  ( -18.62759615963255300, -10.81492255796106328, 54.16775706135235424 ) ) ;
#30183=CARTESIAN_POINT ( 'NONE',  ( 13.89961937509957401, 13.97604488694547697, 81.87609039468564731 ) ) ;
#30185=CARTESIAN_POINT ( 'NONE',  ( -13.89961937509977652, 13.97604488694528158, 55.62390960531434558 ) ) ;
#30186=CARTESIAN_POINT ( 'NONE',  ( 9.474510206698971260, -16.51473224551069308, 102.9155762719810241 ) ) ;
#30187=CARTESIAN_POINT ( 'NONE',  ( -5.153800228976328057, -19.02544592524343514, 77.29057627198099567 ) ) ;
#30188=CARTESIAN_POINT ( 'NONE',  ( 17.49999999999999645, -5.249764055310042643, 23.25708826289255882 ) ) ;
#30189=CARTESIAN_POINT ( 'NONE',  ( -13.97604488694527625, -13.89961937509977652, 51.87390960531436690 ) ) ;
#30190=CARTESIAN_POINT ( 'NONE',  ( 18.62759615963271287, -10.81492255796078972, 93.33224293864769550 ) ) ;
#30191=CARTESIAN_POINT ( 'NONE',  ( 16.55341960407618274, -4.379528057220086978, 91.04275706135236135 ) ) ;
#30192=DIRECTION ( 'NONE',  ( 1.000000000000000000, 0.000000000000000000, -0.000000000000000000 ) ) ;
#30193=CARTESIAN_POINT ( 'NONE',  ( -19.03943276465977164, -0.05219959533935918106, 43.75109039468566863 ) ) ;
#30194=CARTESIAN_POINT ( 'NONE',  ( 0.05219959533909260263, 19.03943276465977164, 84.99890960531436690 ) ) ;
#30195=CARTESIAN_POINT ( 'NONE',  ( -14.34966873604960291, -8.224510206698953496, 56.66557627198103830 ) ) ;
#30196=CARTESIAN_POINT ( 'NONE',  ( -14.34966873604960291, -8.224510206698953496, 96.66557627198102409 ) ) ;
#30197=CARTESIAN_POINT ( 'NONE',  ( -21.53943276465977519, 0.05219959533907696930, 21.24890960531436690 ) ) ;
#30198=( BOUNDED_CURVE ( )  B_SPLINE_CURVE ( 2, ( #119378, #150714, #12213, #197218, #58680, #198198, #187026, #77815, #186017, #32326, #15165, #48497, #45502 ),
 .UNSPECIFIED., .F., .F. ) 
 B_SPLINE_CURVE_WITH_KNOTS ( ( 3, 2, 2, 2, 2, 2, 3 ),
 ( 0.6340093837954662304, 0.6359649122807017330, 0.6403508771929824483, 0.6447368421052631637, 0.6491228070175438791, 0.6535087719298245945, 0.6554186205929700693 ),
 .UNSPECIFIED. ) 
 CURVE ( )  GEOMETRIC_REPRESENTATION_ITEM ( )  RATIONAL_B_SPLINE_CURVE ( ( 0.9831626618144007068, 0.9848076720550096308, 1.000000000000000000, 0.9659258262890683122, 1.000000000000000000, 0.9659258262890683122, 1.000000000000000000, 0.9659258262890683122, 1.000000000000000000, 0.9659258262890683122, 1.000000000000000000, 0.9851625545550091179, 0.9832469066685282089 ) ) 
 REPRESENTATION_ITEM ( '' )  );
#30199=CARTESIAN_POINT ( 'NONE',  ( -0.05219959533909027116, -19.03943276465977164, 107.4989096053143527 ) ) ;
#30200=CARTESIAN_POINT ( 'NONE',  ( -9.474510206698964154, 16.51473224551069663, 115.4155762719810241 ) ) ;
#30201=CARTESIAN_POINT ( 'NONE',  ( 16.46253265017146816, 9.564922557961045513, 21.66775706135233648 ) ) ;
#30202=CARTESIAN_POINT ( 'NONE',  ( -12.14591786802326823, 12.06949235617739902, 93.12609039468568994 ) ) ;
#30203=CARTESIAN_POINT ( 'NONE',  ( 13.97604488694527802, 13.89961937509977652, 79.37390960531435269 ) ) ;
#30204=CARTESIAN_POINT ( 'NONE',  ( -15.72974639402176322, -15.80617190586768395, 44.37609039468567573 ) ) ;
#30205=CARTESIAN_POINT ( 'NONE',  ( 5.823673210054125526, 21.52544592524343514, 34.79057627198103120 ) ) ;
#30206=CARTESIAN_POINT ( 'NONE',  ( 5.719274019375991003, -21.55341960407610458, 112.7072429386476955 ) ) ;
#30207=CARTESIAN_POINT ( 'NONE',  ( -21.52544592524343514, 5.823673210054127303, 66.04057627198103830 ) ) ;
#30208=CARTESIAN_POINT ( 'NONE',  ( 14.29746914071049879, -8.314922557960816363, 93.33224293864769550 ) ) ;
#30209=CARTESIAN_POINT ( 'NONE',  ( -13.97604488694547697, 13.89961937509957934, 38.12609039468566152 ) ) ;
#30210=CARTESIAN_POINT ( 'NONE',  ( 5.049401038298161559, -19.05341960407611168, 27.70724293864769550 ) ) ;
#30211=CARTESIAN_POINT ( 'NONE',  ( -16.46253265017160317, 9.564922557960807481, 85.83224293864769550 ) ) ;
#30212=CARTESIAN_POINT ( 'NONE',  ( -13.89961937509977652, 13.97604488694528158, 80.62390960531436690 ) ) ;
#30214=CARTESIAN_POINT ( 'NONE',  ( -16.55341960407611168, -4.379528057220339221, 106.4572429386477097 ) ) ;
#30216=CARTESIAN_POINT ( 'NONE',  ( -4.483927247898539470, -16.52544592524342804, 22.29057627198102765 ) ) ;
#30217=CARTESIAN_POINT ( 'NONE',  ( -0.05219959533934338120, 16.53943276465976808, 32.50109039468568284 ) ) ;
#30218=CARTESIAN_POINT ( 'NONE',  ( -21.53943276465977519, -0.05219959533937600094, 93.75109039468567573 ) ) ;
#30219=CARTESIAN_POINT ( 'NONE',  ( -19.05341960407611168, -5.049401038298163336, 106.4572429386476955 ) ) ;
#30220=CARTESIAN_POINT ( 'NONE',  ( -21.52544592524343514, 5.823673210054127303, 111.0405762719810525 ) ) ;
#30221=CARTESIAN_POINT ( 'NONE',  ( 5.153800228976335163, 19.02544592524342804, 49.79057627198100988 ) ) ;
#30222=CARTESIAN_POINT ( 'NONE',  ( -4.379528057220086978, -16.55341960407618274, 49.79275706135234714 ) ) ;
#30223=CARTESIAN_POINT ( 'NONE',  ( -19.05341960407617563, 5.049401038297882671, 108.5427570613523187 ) ) ;
#30225=CARTESIAN_POINT ( 'NONE',  ( -21.53943276465977519, 0.05219959533907696930, 101.2489096053143669 ) ) ;
#30226=CARTESIAN_POINT ( 'NONE',  ( 16.46253265017146816, 9.564922557961045513, 61.66775706135234003 ) ) ;
#30228=B_SPLINE_CURVE_WITH_KNOTS ( 'NONE', 3,
 ( #2223, #173081, #171083, #64893, #98948, #161637 ),
 .UNSPECIFIED., .F., .F.,
 ( 4, 2, 4 ),
 ( 0.003239945802372284651, 0.003620412082092146384, 0.004000878361812008552 ),
 .UNSPECIFIED. ) ;
#30229=CARTESIAN_POINT ( 'NONE',  ( -21.55341960407610458, -5.719274019375992779, 111.4572429386476813 ) ) ;
#30231=CARTESIAN_POINT ( 'NONE',  ( 9.564922557960805705, 16.46253265017160317, 89.58224293864769550 ) ) ;
#30232=CARTESIAN_POINT ( 'NONE',  ( 18.22780087662123805, 5.499999999999960032, 91.48236817873106475 ) ) ;
#30233=CARTESIAN_POINT ( 'NONE',  ( -13.97604488694527625, -13.89961937509977652, 86.87390960531436690 ) ) ;
#30234=CARTESIAN_POINT ( 'NONE',  ( 10.72451020669871369, 18.67979575497193778, 27.08442372801901854 ) ) ;
#30235=CARTESIAN_POINT ( 'NONE',  ( -4.379528057220328563, 16.55341960407611168, 80.20724293864769550 ) ) ;
#30236=CARTESIAN_POINT ( 'NONE',  ( -13.89961937509977652, 13.97604488694528158, 80.62390960531436690 ) ) ;
#30237=CARTESIAN_POINT ( 'NONE',  ( 14.29746914071037800, 8.314922557961029526, 56.66775706135235424 ) ) ;
#30238=CARTESIAN_POINT ( 'NONE',  ( 13.89961937509957401, 13.97604488694547697, 61.87609039468566863 ) ) ;
#30239=CARTESIAN_POINT ( 'NONE',  ( -15.72974639402176322, -15.80617190586768395, 69.37609039468567573 ) ) ;
#30240=CARTESIAN_POINT ( 'NONE',  ( -14.29746914071037622, -8.314922557961029526, 24.16775706135235424 ) ) ;
#30241=CARTESIAN_POINT ( 'NONE',  ( -0.05219959533909027116, -19.03943276465977164, 67.49890960531436690 ) ) ;
#30242=CARTESIAN_POINT ( 'NONE',  ( 5.049401038297881783, 19.05341960407617563, 92.29275706135234714 ) ) ;
#30243=CARTESIAN_POINT ( 'NONE',  ( 14.29746914071037800, 8.314922557961029526, 56.66775706135235424 ) ) ;
#30244=CARTESIAN_POINT ( 'NONE',  ( 21.52544592524334988, 5.823673210054432836, 96.45942372801901854 ) ) ;
#30245=CARTESIAN_POINT ( 'NONE',  ( 16.46253265017146816, 9.564922557961045513, 76.66775706135234714 ) ) ;
#30246=CARTESIAN_POINT ( 'NONE',  ( 9.564922557960805705, 16.46253265017160317, 44.58224293864769550 ) ) ;
#30247=CARTESIAN_POINT ( 'NONE',  ( 10.72451020669898902, -18.67979575497178502, 72.91557627198103830 ) ) ;
#30248=CARTESIAN_POINT ( 'NONE',  ( 16.52544592524342804, -4.483927247898539470, 78.54057627198103830 ) ) ;
#30249=CARTESIAN_POINT ( 'NONE',  ( -0.05219959533936034679, 19.03943276465977164, 77.50109039468566152 ) ) ;
#30250=DIRECTION ( 'NONE',  ( 0.000000000000000000, 0.000000000000000000, -1.000000000000000000 ) ) ;
#30251=CARTESIAN_POINT ( 'NONE',  ( 5.153800228976615827, -19.02544592524334988, 45.20942372801901143 ) ) ;
#30252=CARTESIAN_POINT ( 'NONE',  ( 0.05219959533934541429, -16.53943276465976808, 110.0010903946856757 ) ) ;
#30253=CARTESIAN_POINT ( 'NONE',  ( -16.55341960407611168, -4.379528057220339221, 66.45724293864768129 ) ) ;
#30254=CARTESIAN_POINT ( 'NONE',  ( -10.72451020669870658, -18.67979575497194134, 104.5844237280190185 ) ) ;
#30256=CARTESIAN_POINT ( 'NONE',  ( -15.72974639402197994, 15.80617190586746368, 105.6239096053143669 ) ) ;
#30257=CARTESIAN_POINT ( 'NONE',  ( -13.89961937509977652, 13.97604488694528158, 70.62390960531432427 ) ) ;
#30258=CARTESIAN_POINT ( 'NONE',  ( -21.53943276465977519, -0.05219959533937600094, 88.75109039468567573 ) ) ;
#30259=CARTESIAN_POINT ( 'NONE',  ( 0.05219959533909260263, 19.03943276465977164, 64.99890960531436690 ) ) ;
#30260=CARTESIAN_POINT ( 'NONE',  ( -19.03943276465977164, 0.05219959533909376836, 26.24890960531435624 ) ) ;
#30261=CARTESIAN_POINT ( 'NONE',  ( -18.67979575497178146, -10.72451020669898902, 26.66557627198103475 ) ) ;
#30262=CARTESIAN_POINT ( 'NONE',  ( -16.53943276465976808, 0.05219959533911058130, 61.24890960531435979 ) ) ;
#30263=CARTESIAN_POINT ( 'NONE',  ( -19.05341960407611168, -5.049401038298163336, 41.45724293864769550 ) ) ;
#30264=CARTESIAN_POINT ( 'NONE',  ( 12.14591786802309770, 12.06949235617756955, 89.37390960531435269 ) ) ;
#30265=CARTESIAN_POINT ( 'NONE',  ( 21.53943276465977519, -0.05219959533907433946, 108.7489096053143669 ) ) ;
#30266=CARTESIAN_POINT ( 'NONE',  ( 21.52544592524334988, 5.823673210054432836, 46.45942372801901854 ) ) ;
#30267=CARTESIAN_POINT ( 'NONE',  ( 19.02544592524343514, -5.153800228976328945, 23.54057627198102054 ) ) ;
#30268=CARTESIAN_POINT ( 'NONE',  ( 12.14591786802327356, -12.06949235617739191, 45.62609039468567573 ) ) ;
#30269=CARTESIAN_POINT ( 'NONE',  ( 21.53943276465977519, -0.05219959533907433946, 98.74890960531438111 ) ) ;
#30270=CARTESIAN_POINT ( 'NONE',  ( 13.89961937509957401, 13.97604488694547697, 26.87609039468566507 ) ) ;
#30271=CARTESIAN_POINT ( 'NONE',  ( 5.049401038298161559, -19.05341960407611168, 37.70724293864768839 ) ) ;
#30272=CARTESIAN_POINT ( 'NONE',  ( -9.474510206698964154, 16.51473224551069663, 105.4155762719810383 ) ) ;
#30273=CARTESIAN_POINT ( 'NONE',  ( 18.62759615963255655, 10.81492255796105972, 56.66775706135235424 ) ) ;
#30274=CARTESIAN_POINT ( 'NONE',  ( -18.67979575497178146, -10.72451020669898902, 41.66557627198103120 ) ) ;
#30275=CARTESIAN_POINT ( 'NONE',  ( -4.483927247898539470, -16.52544592524342804, 22.29057627198102765 ) ) ;
#30276=CARTESIAN_POINT ( 'NONE',  ( -21.52544592524334988, -5.823673210054445271, 68.95942372801901854 ) ) ;
#30277=CARTESIAN_POINT ( 'NONE',  ( -15.80617190586768217, 15.72974639402176855, 93.12609039468568994 ) ) ;
#30278=CARTESIAN_POINT ( 'NONE',  ( -5.153800228976607833, 19.02544592524334988, 37.70942372801899722 ) ) ;
#30279=CARTESIAN_POINT ( 'NONE',  ( -4.483927247898782831, 16.52544592524335698, 97.70942372801904696 ) ) ;
#30280=CARTESIAN_POINT ( 'NONE',  ( -10.72451020669870658, -18.67979575497194134, 59.58442372801901854 ) ) ;
#30282=CARTESIAN_POINT ( 'NONE',  ( -13.89961937509977652, 13.97604488694528158, 50.62390960531435979 ) ) ;
#30283=CARTESIAN_POINT ( 'NONE',  ( 5.049401038297881783, 19.05341960407617563, 27.29275706135232937 ) ) ;
#30284=CARTESIAN_POINT ( 'NONE',  ( 13.97604488694527802, 13.89961937509977652, 114.3739096053143669 ) ) ;
#30285=CARTESIAN_POINT ( 'NONE',  ( 10.72451020669871369, 18.67979575497193778, 22.08442372801901143 ) ) ;
#30286=CARTESIAN_POINT ( 'NONE',  ( -15.72974639402197994, 15.80617190586746368, 80.62390960531438111 ) ) ;
#30287=CARTESIAN_POINT ( 'NONE',  ( 8.314922557961029526, -14.29746914071037800, 35.41775706135234003 ) ) ;
#30289=CARTESIAN_POINT ( 'NONE',  ( 15.72974639402199770, -15.80617190586745480, 83.12390960531436690 ) ) ;
#30290=CARTESIAN_POINT ( 'NONE',  ( 14.29746914071037800, 8.314922557961029526, 66.66775706135234714 ) ) ;
#30291=CARTESIAN_POINT ( 'NONE',  ( -4.379528057220328563, 16.55341960407611168, 70.20724293864769550 ) ) ;
#30293=CARTESIAN_POINT ( 'NONE',  ( 19.05341960407617918, -5.049401038297876454, 101.0427570613523045 ) ) ;
#30295=CARTESIAN_POINT ( 'NONE',  ( -15.72974639402197994, 15.80617190586746368, 35.62390960531437401 ) ) ;
#30296=CARTESIAN_POINT ( 'NONE',  ( 17.59860650958990647, 7.585241751807016541, 94.07662985737508166 ) ) ;
#30297=ADVANCED_FACE ( 'NONE', ( #29451 ), #74948, .F. ) ;
#30298=CARTESIAN_POINT ( 'NONE',  ( 4.379528057220092307, 16.55341960407617563, 37.29275706135235424 ) ) ;
#30299=CARTESIAN_POINT ( 'NONE',  ( -21.52544592524334988, -5.823673210054445271, 18.95942372801901143 ) ) ;
#30300=CARTESIAN_POINT ( 'NONE',  ( 18.67979575497178502, 10.72451020669898547, 34.16557627198102409 ) ) ;
#30301=CARTESIAN_POINT ( 'NONE',  ( -12.06949235617739369, -12.14591786802326823, 69.37609039468567573 ) ) ;
#30302=CARTESIAN_POINT ( 'NONE',  ( -13.89961937509977652, 13.97604488694528158, 90.62390960531432427 ) ) ;
#30303=CARTESIAN_POINT ( 'NONE',  ( 21.55341960407619695, -5.719274019375665929, 46.04275706135234714 ) ) ;
#30304=CARTESIAN_POINT ( 'NONE',  ( -16.53943276465976808, -0.05219959533934237506, 18.75109039468568639 ) ) ;
#30305=CARTESIAN_POINT ( 'NONE',  ( -5.719274019375978568, 21.55341960407610458, 30.20724293864769550 ) ) ;
#30307=CARTESIAN_POINT ( 'NONE',  ( 13.97604488694548053, -13.89961937509957401, 30.62609039468566863 ) ) ;
#30308=CARTESIAN_POINT ( 'NONE',  ( -16.53943276465976808, -0.05219959533934237506, 48.75109039468568284 ) ) ;
#30309=CARTESIAN_POINT ( 'NONE',  ( -0.05219959533909027116, -19.03943276465977164, 102.4989096053143669 ) ) ;
#30310=CARTESIAN_POINT ( 'NONE',  ( 21.52544592524344225, -5.823673210054117533, 103.5405762719810383 ) ) ;
#30311=CARTESIAN_POINT ( 'NONE',  ( 13.89961937509977652, -13.97604488694527269, 68.12390960531436690 ) ) ;
#30312=CARTESIAN_POINT ( 'NONE',  ( -17.40805194822030089, 6.112264579159337963, 25.83371272510612116 ) ) ;
#30313=CARTESIAN_POINT ( 'NONE',  ( -8.314922557960811034, -14.29746914071050412, 82.08224293864768129 ) ) ;
#30314=CARTESIAN_POINT ( 'NONE',  ( 21.53943276465977519, -0.05219959533907433946, 33.74890960531436690 ) ) ;
#30315=CARTESIAN_POINT ( 'NONE',  ( -9.564922557960796823, -16.46253265017161027, 22.08224293864768839 ) ) ;
#30316=CARTESIAN_POINT ( 'NONE',  ( 4.379528057220092307, 16.55341960407617563, 67.29275706135234714 ) ) ;
#30317=CARTESIAN_POINT ( 'NONE',  ( 18.62759615963271287, -10.81492255796078972, 113.3322429386476955 ) ) ;
#30318=CARTESIAN_POINT ( 'NONE',  ( -16.51473224551082808, 9.474510206698731452, 73.33442372801900433 ) ) ;
#30319=CARTESIAN_POINT ( 'NONE',  ( 5.049401038298161559, -19.05341960407611168, 32.70724293864768129 ) ) ;
#30320=CARTESIAN_POINT ( 'NONE',  ( -10.72451020669898014, 18.67979575497178502, 65.41557627198102409 ) ) ;
#30322=CARTESIAN_POINT ( 'NONE',  ( 16.51473224551069308, 9.474510206698969483, 104.1655762719810241 ) ) ;
#30323=CARTESIAN_POINT ( 'NONE',  ( -21.52544592524334988, -5.823673210054445271, 88.95942372801901854 ) ) ;
#30324=CARTESIAN_POINT ( 'NONE',  ( -16.46253265017160317, 9.564922557960807481, 65.83224293864769550 ) ) ;
#30325=CARTESIAN_POINT ( 'NONE',  ( -16.53943276465976808, -0.05219959533934237506, 43.75109039468568284 ) ) ;
#30326=CARTESIAN_POINT ( 'NONE',  ( -19.05341960407611168, -5.049401038298163336, 56.45724293864768129 ) ) ;
#30327=CARTESIAN_POINT ( 'NONE',  ( -15.80617190586768217, 15.72974639402176855, 83.12609039468568994 ) ) ;
#30329=CARTESIAN_POINT ( 'NONE',  ( -19.02544592524334988, -5.153800228976617603, 33.95942372801897591 ) ) ;
#30331=CARTESIAN_POINT ( 'NONE',  ( 19.02544592524334988, 5.153800228976608722, 56.45942372801898301 ) ) ;
#30332=CARTESIAN_POINT ( 'NONE',  ( 5.719274019375673035, 21.55341960407619339, 52.29275706135236135 ) ) ;
#30334=CARTESIAN_POINT ( 'NONE',  ( 13.97604488694548053, -13.89961937509957401, 50.62609039468566152 ) ) ;
#30335=CARTESIAN_POINT ( 'NONE',  ( -13.97604488694527625, -13.89961937509977652, 101.8739096053143811 ) ) ;
#30336=CARTESIAN_POINT ( 'NONE',  ( -0.05219959533909027116, -19.03943276465977164, 67.49890960531436690 ) ) ;
#30337=CARTESIAN_POINT ( 'NONE',  ( 14.34966873604960469, 8.224510206698951720, 29.16557627198103120 ) ) ;
#30338=CARTESIAN_POINT ( 'NONE',  ( 13.97604488694527802, 13.89961937509977652, 114.3739096053143669 ) ) ;
#30339=CARTESIAN_POINT ( 'NONE',  ( -10.72451020669870658, -18.67979575497194134, 94.58442372801901854 ) ) ;
#30342=CARTESIAN_POINT ( 'NONE',  ( -10.72451020669870658, -18.67979575497194134, 99.58442372801900433 ) ) ;
#30344=CARTESIAN_POINT ( 'NONE',  ( -13.97604488694527625, -13.89961937509977652, 26.87390960531434558 ) ) ;
#30347=CARTESIAN_POINT ( 'NONE',  ( 16.52544592524335698, 4.483927247898782831, 51.45942372801901854 ) ) ;
#30348=CARTESIAN_POINT ( 'NONE',  ( 5.823673210054125526, 21.52544592524343514, 69.79057627198102409 ) ) ;
#30349=CARTESIAN_POINT ( 'NONE',  ( -16.55341960407611168, -4.379528057220339221, 46.45724293864769550 ) ) ;
#30350=CARTESIAN_POINT ( 'NONE',  ( -12.06949235617756955, 12.14591786802309770, 105.6239096053143669 ) ) ;
#30351=CARTESIAN_POINT ( 'NONE',  ( -13.97604488694527625, -13.89961937509977652, 96.87390960531433848 ) ) ;
#30352=CARTESIAN_POINT ( 'NONE',  ( -19.02544592524334988, -5.153800228976617603, 38.95942372801900433 ) ) ;
#30353=CARTESIAN_POINT ( 'NONE',  ( 0.05219959533910956823, 16.53943276465976808, 114.9989096053143669 ) ) ;
#30354=CARTESIAN_POINT ( 'NONE',  ( 18.67979575497194134, -10.72451020669871369, 70.83442372801901854 ) ) ;
#30355=CARTESIAN_POINT ( 'NONE',  ( -9.474510206698964154, 16.51473224551069663, 115.4155762719810241 ) ) ;
#30356=CARTESIAN_POINT ( 'NONE',  ( -14.34966873604972548, 8.224510206698743886, 103.3344237280190043 ) ) ;
#30358=CARTESIAN_POINT ( 'NONE',  ( 5.823673210054125526, 21.52544592524343514, 24.79057627198103120 ) ) ;
#30359=CARTESIAN_POINT ( 'NONE',  ( -14.34966873604960291, -8.224510206698953496, 96.66557627198102409 ) ) ;
#30360=CARTESIAN_POINT ( 'NONE',  ( -9.564922557961040184, 16.46253265017147172, 62.91775706135233293 ) ) ;
#30361=CARTESIAN_POINT ( 'NONE',  ( -5.153800228976328057, -19.02544592524343514, 82.29057627198103830 ) ) ;
#30362=CARTESIAN_POINT ( 'NONE',  ( 4.483927247898545687, 16.52544592524342804, 74.79057627198105251 ) ) ;
#30363=CARTESIAN_POINT ( 'NONE',  ( 19.02544592524334988, 5.153800228976608722, 86.45942372801900433 ) ) ;
#30364=CARTESIAN_POINT ( 'NONE',  ( -21.55341960407610458, -5.719274019375992779, 46.45724293864769550 ) ) ;
#30365=VERTEX_POINT ( 'NONE', #90109 ) ;
#30366=CARTESIAN_POINT ( 'NONE',  ( 16.52544592524342804, -4.483927247898539470, 113.5405762719810383 ) ) ;
#30367=CARTESIAN_POINT ( 'NONE',  ( -16.62475595723695676, -7.163666690055260133, 29.47286648189535896 ) ) ;
#30368=CARTESIAN_POINT ( 'NONE',  ( 16.46253265017160672, -9.564922557960803928, 78.33224293864769550 ) ) ;
#30369=CARTESIAN_POINT ( 'NONE',  ( -0.05219959533907301413, -21.53943276465977519, 82.49890960531436690 ) ) ;
#30370=CARTESIAN_POINT ( 'NONE',  ( 16.55341960407618274, -4.379528057220086978, 96.04275706135236135 ) ) ;
#30371=CARTESIAN_POINT ( 'NONE',  ( -13.97604488694527625, -13.89961937509977652, 86.87390960531436690 ) ) ;
#30372=CARTESIAN_POINT ( 'NONE',  ( 16.51473224551083163, -9.474510206698727899, 70.83442372801900433 ) ) ;
#30373=CARTESIAN_POINT ( 'NONE',  ( -21.53943276465977519, -0.05219959533937600094, 78.75109039468568994 ) ) ;
#30374=CARTESIAN_POINT ( 'NONE',  ( 18.62759615963271287, -10.81492255796078972, 58.33224293864768839 ) ) ;
#30375=CARTESIAN_POINT ( 'NONE',  ( -16.46253265017160317, 9.564922557960807481, 115.8322429386477097 ) ) ;
#30376=CARTESIAN_POINT ( 'NONE',  ( 19.05341960407611168, 5.049401038298154454, 38.95724293864767418 ) ) ;
#30377=CARTESIAN_POINT ( 'NONE',  ( -14.34966873604972548, 8.224510206698743886, 103.3344237280190043 ) ) ;
#30378=CARTESIAN_POINT ( 'NONE',  ( 16.46253265017160672, -9.564922557960803928, 53.33224293864768839 ) ) ;
#30379=CARTESIAN_POINT ( 'NONE',  ( 19.03943276465977164, 0.05219959533936151252, 111.2510903946856757 ) ) ;
#30381=CARTESIAN_POINT ( 'NONE',  ( 5.153800228976615827, -19.02544592524334988, 20.20942372801899722 ) ) ;
#30382=CARTESIAN_POINT ( 'NONE',  ( -16.55341960407611168, -4.379528057220339221, 61.45724293864770260 ) ) ;
#30383=CARTESIAN_POINT ( 'NONE',  ( -5.719274019375978568, 21.55341960407610458, 105.2072429386477097 ) ) ;
#30384=CARTESIAN_POINT ( 'NONE',  ( 21.53943276465977519, -0.05219959533907433946, 103.7489096053143669 ) ) ;
#30385=CARTESIAN_POINT ( 'NONE',  ( 17.48847506799968698, -5.747544572773782612, 98.32697437843285115 ) ) ;
#30386=CARTESIAN_POINT ( 'NONE',  ( 21.55341960407610458, 5.719274019375980345, 48.95724293864770971 ) ) ;
#30387=CARTESIAN_POINT ( 'NONE',  ( 8.314922557961029526, -14.29746914071037800, 75.41775706135233293 ) ) ;
#30388=CARTESIAN_POINT ( 'NONE',  ( 14.34966873604960469, 8.224510206698951720, 109.1655762719810383 ) ) ;
#30389=CARTESIAN_POINT ( 'NONE',  ( 9.564922557960805705, 16.46253265017160317, 64.58224293864769550 ) ) ;
#30390=FILL_AREA_STYLE_COLOUR ( '', #36903 ) ;
#30392=CARTESIAN_POINT ( 'NONE',  ( -12.14591786802326823, 12.06949235617739902, 108.1260903946856757 ) ) ;
#30393=CARTESIAN_POINT ( 'NONE',  ( -18.62759615963255300, -10.81492255796106328, 49.16775706135234003 ) ) ;
#30394=CARTESIAN_POINT ( 'NONE',  ( 19.03943276465977164, -0.05219959533909143690, 93.74890960531435269 ) ) ;
#30395=CARTESIAN_POINT ( 'NONE',  ( 18.62759615963255655, 10.81492255796105972, 81.66775706135236135 ) ) ;
#30397=CARTESIAN_POINT ( 'NONE',  ( -9.474510206698964154, 16.51473224551069663, 30.41557627198102054 ) ) ;
#30399=ORIENTED_EDGE ( 'NONE', *, *, #52038, .F. ) ;
#30400=CARTESIAN_POINT ( 'NONE',  ( -21.55341960407619339, 5.719274019375674811, 78.54275706135236135 ) ) ;
#30401=CARTESIAN_POINT ( 'NONE',  ( 9.474510206698971260, -16.51473224551069308, 52.91557627198102409 ) ) ;
#30402=CARTESIAN_POINT ( 'NONE',  ( -9.474510206698964154, 16.51473224551069663, 85.41557627198102409 ) ) ;
#30403=CARTESIAN_POINT ( 'NONE',  ( 5.153800228976615827, -19.02544592524334988, 85.20942372801900433 ) ) ;
#30404=CARTESIAN_POINT ( 'NONE',  ( -15.72974639402176322, -15.80617190586768395, 44.37609039468567573 ) ) ;
#30405=CARTESIAN_POINT ( 'NONE',  ( -13.89961937509957401, -13.97604488694547875, 109.3760903946856331 ) ) ;
#30406=CARTESIAN_POINT ( 'NONE',  ( -9.564922557961040184, 16.46253265017147172, 77.91775706135234714 ) ) ;
#30407=CARTESIAN_POINT ( 'NONE',  ( 9.474510206698971260, -16.51473224551069308, 37.91557627198102409 ) ) ;
#30408=CARTESIAN_POINT ( 'NONE',  ( -0.05219959533936034679, 19.03943276465977164, 82.50109039468567573 ) ) ;
#30409=CARTESIAN_POINT ( 'NONE',  ( 14.34966873604972726, -8.224510206698740333, 110.8344237280190043 ) ) ;
#30410=CARTESIAN_POINT ( 'NONE',  ( 9.564922557961047289, -16.46253265017146816, 80.41775706135234714 ) ) ;
#30411=CARTESIAN_POINT ( 'NONE',  ( -0.05219959533910754901, -16.53943276465976808, 42.49890960531435979 ) ) ;
#30412=CARTESIAN_POINT ( 'NONE',  ( 5.049401038297881783, 19.05341960407617563, 47.29275706135231161 ) ) ;
#30413=CARTESIAN_POINT ( 'NONE',  ( -5.719274019375665041, -21.55341960407619695, 109.7927570613523613 ) ) ;
#30414=CARTESIAN_POINT ( 'NONE',  ( -19.02544592524334988, -5.153800228976617603, 23.95942372801900078 ) ) ;
#30415=CARTESIAN_POINT ( 'NONE',  ( 19.02544592524343514, -5.153800228976328945, 28.54057627198102409 ) ) ;
#30416=CARTESIAN_POINT ( 'NONE',  ( 10.72451020669871369, 18.67979575497193778, 87.08442372801901854 ) ) ;
#30417=CARTESIAN_POINT ( 'NONE',  ( 4.379528057220092307, 16.55341960407617563, 52.29275706135236135 ) ) ;
#30418=CARTESIAN_POINT ( 'NONE',  ( 9.564922557960805705, 16.46253265017160317, 94.58224293864769550 ) ) ;
#30420=CARTESIAN_POINT ( 'NONE',  ( -19.03943276465977164, 0.05219959533909376836, 91.24890960531436690 ) ) ;
#30421=CARTESIAN_POINT ( 'NONE',  ( -17.26172910966711882, 6.454744622557081257, 100.8064690864920863 ) ) ;
#30424=CARTESIAN_POINT ( 'NONE',  ( 19.05341960407617918, -5.049401038297876454, 86.04275706135233293 ) ) ;
#30425=CARTESIAN_POINT ( 'NONE',  ( 10.72451020669898902, -18.67979575497178502, 22.91557627198102765 ) ) ;
#30426=CARTESIAN_POINT ( 'NONE',  ( 15.80617190586769283, -15.72974639402175789, 110.6260903946857042 ) ) ;
#30427=CARTESIAN_POINT ( 'NONE',  ( -13.89961937509957401, -13.97604488694547875, 99.37609039468567573 ) ) ;
#30428=CARTESIAN_POINT ( 'NONE',  ( -12.06949235617756955, 12.14591786802309770, 115.6239096053143669 ) ) ;
#30429=CARTESIAN_POINT ( 'NONE',  ( 19.02544592524343514, -5.153800228976328945, 23.54057627198102054 ) ) ;
#30430=CARTESIAN_POINT ( 'NONE',  ( -15.72974639402197994, 15.80617190586746368, 60.62390960531437401 ) ) ;
#30431=CARTESIAN_POINT ( 'NONE',  ( 21.52544592524344225, -5.823673210054117533, 43.54057627198103830 ) ) ;
#30432=CARTESIAN_POINT ( 'NONE',  ( 19.05341960407611168, 5.049401038298154454, 23.95724293864769194 ) ) ;
#30434=CARTESIAN_POINT ( 'NONE',  ( 19.03943276465977164, 0.05219959533936151252, 76.25109039468566152 ) ) ;
#30435=CARTESIAN_POINT ( 'NONE',  ( 12.06949235617757843, -12.14591786802309237, 38.12390960531436690 ) ) ;
#30436=CARTESIAN_POINT ( 'NONE',  ( 21.55341960407610458, 5.719274019375980345, 23.95724293864769550 ) ) ;
#30437=CARTESIAN_POINT ( 'NONE',  ( -18.62759615963255300, -10.81492255796106328, 89.16775706135236135 ) ) ;
#30438=CARTESIAN_POINT ( 'NONE',  ( -10.72451020669898014, 18.67979575497178502, 70.41557627198102409 ) ) ;
#30439=CARTESIAN_POINT ( 'NONE',  ( -21.52544592524334988, -5.823673210054445271, 63.95942372801901854 ) ) ;
#30440=CARTESIAN_POINT ( 'NONE',  ( 21.52544592524334988, 5.823673210054432836, 46.45942372801901854 ) ) ;
#30442=CARTESIAN_POINT ( 'NONE',  ( -5.153800228976328057, -19.02544592524343514, 92.29057627198099567 ) ) ;
#30443=CARTESIAN_POINT ( 'NONE',  ( 16.53943276465976808, 0.05219959533934440121, 91.25109039468568994 ) ) ;
#30444=CARTESIAN_POINT ( 'NONE',  ( 5.153800228976335163, 19.02544592524342804, 29.79057627198102409 ) ) ;
#30446=CARTESIAN_POINT ( 'NONE',  ( -16.53943276465976808, 0.05219959533911058130, 66.24890960531436690 ) ) ;
#30447=CARTESIAN_POINT ( 'NONE',  ( -4.483927247898539470, -16.52544592524342804, 32.29057627198102409 ) ) ;
#30448=CARTESIAN_POINT ( 'NONE',  ( 16.46253265017160672, -9.564922557960803928, 63.33224293864769550 ) ) ;
#30449=CARTESIAN_POINT ( 'NONE',  ( 5.153800228976335163, 19.02544592524342804, 39.79057627198100988 ) ) ;
#30450=CARTESIAN_POINT ( 'NONE',  ( -18.62759615963270932, 10.81492255796079327, 60.83224293864769550 ) ) ;
#30451=CARTESIAN_POINT ( 'NONE',  ( -16.51473224551082808, 9.474510206698731452, 33.33442372801899722 ) ) ;
#30453=CARTESIAN_POINT ( 'NONE',  ( -12.14591786802309592, -12.06949235617757132, 51.87390960531437401 ) ) ;
#30454=CARTESIAN_POINT ( 'NONE',  ( -18.67979575497178146, -10.72451020669898902, 31.66557627198102054 ) ) ;
#30456=CARTESIAN_POINT ( 'NONE',  ( -16.55341960407617563, 4.379528057220093196, 73.54275706135234714 ) ) ;
#30457=CARTESIAN_POINT ( 'NONE',  ( 19.03943276465977164, 0.05219959533936151252, 71.25109039468566152 ) ) ;
#30458=CARTESIAN_POINT ( 'NONE',  ( 4.379528057220339221, -16.55341960407611168, 37.70724293864769550 ) ) ;
#30459=DIRECTION ( 'NONE',  ( 0.000000000000000000, 0.000000000000000000, -1.000000000000000000 ) ) ;
#30460=CARTESIAN_POINT ( 'NONE',  ( -4.483927247898539470, -16.52544592524342804, 32.29057627198102409 ) ) ;
#30461=CARTESIAN_POINT ( 'NONE',  ( 19.02544592524343514, -5.153800228976328945, 53.54057627198102409 ) ) ;
#30462=CARTESIAN_POINT ( 'NONE',  ( 9.564922557960805705, 16.46253265017160317, 74.58224293864769550 ) ) ;
#30463=CARTESIAN_POINT ( 'NONE',  ( 9.564922557960805705, 16.46253265017160317, 34.58224293864770260 ) ) ;
#30464=CARTESIAN_POINT ( 'NONE',  ( -21.55341960407619339, 5.719274019375674811, 48.54275706135234714 ) ) ;
#30465=CARTESIAN_POINT ( 'NONE',  ( -13.97604488694527625, -13.89961937509977652, 61.87390960531435979 ) ) ;
#30467=CARTESIAN_POINT ( 'NONE',  ( 13.89961937509977652, -13.97604488694527269, 63.12390960531435979 ) ) ;
#30468=CARTESIAN_POINT ( 'NONE',  ( 0.05219959533907565091, 21.53943276465977519, 29.99890960531435979 ) ) ;
#30469=CARTESIAN_POINT ( 'NONE',  ( 16.52544592524342804, -4.483927247898539470, 113.5405762719810383 ) ) ;
#30470=CARTESIAN_POINT ( 'NONE',  ( 21.55341960407610458, 5.719274019375980345, 33.95724293864769550 ) ) ;
#30471=CARTESIAN_POINT ( 'NONE',  ( -4.379528057220086978, -16.55341960407618274, 94.79275706135234714 ) ) ;
#30472=CARTESIAN_POINT ( 'NONE',  ( -5.823673210054431948, 21.52544592524334988, 102.7094237280190185 ) ) ;
#30473=CARTESIAN_POINT ( 'NONE',  ( -14.29746914071037622, -8.314922557961029526, 69.16775706135234714 ) ) ;
#30474=CARTESIAN_POINT ( 'NONE',  ( 9.564922557960805705, 16.46253265017160317, 104.5822429386476955 ) ) ;
#30475=CARTESIAN_POINT ( 'NONE',  ( -12.06949235617739369, -12.14591786802326823, 59.37609039468568284 ) ) ;
#30476=CARTESIAN_POINT ( 'NONE',  ( 8.224510206698742110, 14.34966873604972548, 42.08442372801901854 ) ) ;
#30477=CARTESIAN_POINT ( 'NONE',  ( 16.53943276465976808, 0.05219959533934440121, 96.25109039468568994 ) ) ;
#30478=CARTESIAN_POINT ( 'NONE',  ( -14.34966873604972548, 8.224510206698743886, 28.33442372801902209 ) ) ;
#30479=CARTESIAN_POINT ( 'NONE',  ( 19.03943276465977164, -0.05219959533909143690, 33.74890960531435979 ) ) ;
#30480=CARTESIAN_POINT ( 'NONE',  ( -0.05219959533907301413, -21.53943276465977519, 112.4989096053143669 ) ) ;
#30481=CARTESIAN_POINT ( 'NONE',  ( -16.53943276465976808, -0.05219959533934237506, 23.75109039468567929 ) ) ;
#30482=CARTESIAN_POINT ( 'NONE',  ( 16.52544592524335698, 4.483927247898782831, 81.45942372801900433 ) ) ;
#30483=CARTESIAN_POINT ( 'NONE',  ( -17.05587630539706723, 6.762274262136762637, 45.74180309037284786 ) ) ;
#30484=CARTESIAN_POINT ( 'NONE',  ( -18.67979575497193778, 10.72451020669871902, 83.33442372801903275 ) ) ;
#30485=CARTESIAN_POINT ( 'NONE',  ( -0.05219959533936034679, 19.03943276465977164, 77.50109039468566152 ) ) ;
#30486=CARTESIAN_POINT ( 'NONE',  ( -12.06949235617756955, 12.14591786802309770, 65.62390960531436690 ) ) ;
#30487=CARTESIAN_POINT ( 'NONE',  ( -14.29746914071049879, 8.314922557960819915, 40.83224293864769550 ) ) ;
#30488=CARTESIAN_POINT ( 'NONE',  ( 4.483927247898545687, 16.52544592524342804, 104.7905762719810241 ) ) ;
#30489=CARTESIAN_POINT ( 'NONE',  ( 5.049401038297881783, 19.05341960407617563, 42.29275706135234003 ) ) ;
#30491=CARTESIAN_POINT ( 'NONE',  ( -15.72974639402176322, -15.80617190586768395, 54.37609039468568994 ) ) ;
#30492=CARTESIAN_POINT ( 'NONE',  ( 12.14591786802327356, -12.06949235617739191, 20.62609039468568639 ) ) ;
#30493=CARTESIAN_POINT ( 'NONE',  ( 16.81555441253551564, 7.025013491695493606, 81.86314554665740673 ) ) ;
#30494=CARTESIAN_POINT ( 'NONE',  ( -5.153800228976328057, -19.02544592524343514, 102.2905762719810383 ) ) ;
#30495=CARTESIAN_POINT ( 'NONE',  ( -21.55341960407610458, -5.719274019375992779, 71.45724293864769550 ) ) ;
#30496=CARTESIAN_POINT ( 'NONE',  ( 0.05219959533936267826, -19.03943276465977164, 95.00109039468567573 ) ) ;
#30497=CARTESIAN_POINT ( 'NONE',  ( -0.05219959533909027116, -19.03943276465977164, 107.4989096053143527 ) ) ;
#30499=CARTESIAN_POINT ( 'NONE',  ( 8.314922557960818139, 14.29746914071049879, 109.5822429386476955 ) ) ;
#30500=CARTESIAN_POINT ( 'NONE',  ( 5.719274019375673035, 21.55341960407619339, 97.29275706135234714 ) ) ;
#30501=CARTESIAN_POINT ( 'NONE',  ( -9.564922557960796823, -16.46253265017161027, 27.08224293864769550 ) ) ;
#30502=CARTESIAN_POINT ( 'NONE',  ( -15.80617190586768217, 15.72974639402176855, 53.12609039468568284 ) ) ;
#30503=CARTESIAN_POINT ( 'NONE',  ( 10.81492255796106328, -18.62759615963255655, 85.41775706135236135 ) ) ;
#30504=CARTESIAN_POINT ( 'NONE',  ( -8.224510206698735004, -14.34966873604973081, 94.58442372801901854 ) ) ;
#30505=CARTESIAN_POINT ( 'NONE',  ( -10.72451020669870658, -18.67979575497194134, 44.58442372801901854 ) ) ;
#30506=CARTESIAN_POINT ( 'NONE',  ( 5.823673210054444382, -21.52544592524334988, 40.20942372801901854 ) ) ;
#30507=CARTESIAN_POINT ( 'NONE',  ( 13.89961937509957401, 13.97604488694547697, 61.87609039468566863 ) ) ;
#30508=CARTESIAN_POINT ( 'NONE',  ( -16.51473224551069308, -9.474510206698971260, 91.66557627198103830 ) ) ;
#30509=CARTESIAN_POINT ( 'NONE',  ( 12.06949235617757843, -12.14591786802309237, 103.1239096053143811 ) ) ;
#30510=CARTESIAN_POINT ( 'NONE',  ( -15.72974639402197994, 15.80617190586746368, 85.62390960531436690 ) ) ;
#30511=CARTESIAN_POINT ( 'NONE',  ( -4.379528057220328563, 16.55341960407611168, 65.20724293864768129 ) ) ;
#30512=CARTESIAN_POINT ( 'NONE',  ( 21.55341960407619695, -5.719274019375665929, 101.0427570613523756 ) ) ;
#30513=CARTESIAN_POINT ( 'NONE',  ( 4.379528057220339221, -16.55341960407611168, 77.70724293864770971 ) ) ;
#30514=CARTESIAN_POINT ( 'NONE',  ( 5.153800228976335163, 19.02544592524342804, 34.79057627198102409 ) ) ;
#30515=CARTESIAN_POINT ( 'NONE',  ( -13.97604488694547697, 13.89961937509957934, 83.12609039468564731 ) ) ;
#30516=CARTESIAN_POINT ( 'NONE',  ( -4.379528057220328563, 16.55341960407611168, 50.20724293864769550 ) ) ;
#30517=CARTESIAN_POINT ( 'NONE',  ( 18.67979575497194134, -10.72451020669871369, 100.8344237280190185 ) ) ;
#30518=CARTESIAN_POINT ( 'NONE',  ( -5.049401038298153566, 19.05341960407611168, 90.20724293864766707 ) ) ;
#30519=B_SPLINE_CURVE_WITH_KNOTS ( 'NONE', 3,
 ( #136774, #195496, #118643, #168110, #14426, #95236, #110405, #141738, #186281, #199450, #126563, #49737, #185270, #31590, #80068, #184281, #30595, #155918, #237, #122593 ),
 .UNSPECIFIED., .F., .F.,
 ( 4, 2, 2, 2, 2, 2, 2, 2, 2, 4 ),
 ( 4.982613841084487634E-18, 0.0002490660040300066245, 0.0004981320080600082616, 0.0009962640161200063318, 0.001494396024180004402, 0.001992528032240002255, 0.002490660040300000759, 0.002988792048359998395, 0.003486924056419996899, 0.003985056064479994969 ),
 .UNSPECIFIED. ) ;
#30520=CARTESIAN_POINT ( 'NONE',  ( 5.049401038297881783, 19.05341960407617563, 67.29275706135234714 ) ) ;
#30521=CARTESIAN_POINT ( 'NONE',  ( -5.719274019375978568, 21.55341960407610458, 65.20724293864768129 ) ) ;
#30522=CARTESIAN_POINT ( 'NONE',  ( -18.67979575497193778, 10.72451020669871902, 23.33442372801901499 ) ) ;
#30523=CARTESIAN_POINT ( 'NONE',  ( 19.02544592524334988, 5.153800228976608722, 111.4594237280190043 ) ) ;
#30524=CARTESIAN_POINT ( 'NONE',  ( -14.34966873604972548, 8.224510206698743886, 78.33442372801901854 ) ) ;
#30525=CARTESIAN_POINT ( 'NONE',  ( -13.89961937509977652, 13.97604488694528158, 25.62390960531434558 ) ) ;
#30526=CARTESIAN_POINT ( 'NONE',  ( 10.81492255796106328, -18.62759615963255655, 20.41775706135234714 ) ) ;
#30527=CARTESIAN_POINT ( 'NONE',  ( -4.483927247898539470, -16.52544592524342804, 112.2905762719810241 ) ) ;
#30529=CARTESIAN_POINT ( 'NONE',  ( -0.05219959533934338120, 16.53943276465976808, 52.50109039468567573 ) ) ;
#30530=CARTESIAN_POINT ( 'NONE',  ( -14.34966873604960291, -8.224510206698953496, 76.66557627198103830 ) ) ;
#30531=CARTESIAN_POINT ( 'NONE',  ( 5.823673210054125526, 21.52544592524343514, 79.79057627198102409 ) ) ;
#30532=CARTESIAN_POINT ( 'NONE',  ( -8.224510206698948167, 14.34966873604960824, 25.41557627198103120 ) ) ;
#30533=CARTESIAN_POINT ( 'NONE',  ( -4.379528057220086978, -16.55341960407618274, 34.79275706135235424 ) ) ;
#30534=CARTESIAN_POINT ( 'NONE',  ( 5.153800228976335163, 19.02544592524342804, 39.79057627198100988 ) ) ;
#30535=B_SPLINE_CURVE_WITH_KNOTS ( 'NONE', 3,
 ( #20502, #130671, #7321, #48871, #51840, #110526, #172207, #35675, #3347, #157040, #191352, #22512, #19521, #82150, #34686, #21505, #4327, #52830, #127679, #175194 ),
 .UNSPECIFIED., .F., .F.,
 ( 4, 2, 2, 2, 2, 2, 2, 2, 2, 4 ),
 ( 0.004000878361811823804, 0.004499404418915833696, 0.004997930476019843589, 0.005496456533123854349, 0.005994982590227864241, 0.006244245618779868320, 0.006493508647331874134, 0.006992034704435884027, 0.007490560761539893919, 0.007989086818643903812 ),
 .UNSPECIFIED. ) ;
#30536=CARTESIAN_POINT ( 'NONE',  ( 12.14591786802327356, -12.06949235617739191, 75.62609039468567573 ) ) ;
#30537=CARTESIAN_POINT ( 'NONE',  ( -13.89961937509957401, -13.97604488694547875, 74.37609039468566152 ) ) ;
#30538=CARTESIAN_POINT ( 'NONE',  ( -10.81492255796078084, -18.62759615963271287, 77.08224293864769550 ) ) ;
#30539=CARTESIAN_POINT ( 'NONE',  ( 16.52544592524342804, -4.483927247898539470, 23.54057627198102765 ) ) ;
#30541=CARTESIAN_POINT ( 'NONE',  ( -21.55341960407619339, 5.719274019375674811, 78.54275706135236135 ) ) ;
#30543=CARTESIAN_POINT ( 'NONE',  ( 5.719274019375991003, -21.55341960407610458, 42.70724293864770260 ) ) ;
#30545=CARTESIAN_POINT ( 'NONE',  ( -16.55341960407617563, 4.379528057220093196, 98.54275706135234714 ) ) ;
#30546=CARTESIAN_POINT ( 'NONE',  ( 5.823673210054125526, 21.52544592524343514, 39.79057627198103830 ) ) ;
#30548=CARTESIAN_POINT ( 'NONE',  ( 16.51473224551069308, 9.474510206698969483, 109.1655762719810383 ) ) ;
#30549=CARTESIAN_POINT ( 'NONE',  ( 17.49999999999999289, 3.189878218039149615, 107.6294856257125048 ) ) ;
#30550=CARTESIAN_POINT ( 'NONE',  ( -12.06949235617756955, 12.14591786802309770, 115.6239096053143669 ) ) ;
#30551=CARTESIAN_POINT ( 'NONE',  ( 10.81492255796078972, 18.62759615963270932, 69.58224293864769550 ) ) ;
#30552=CARTESIAN_POINT ( 'NONE',  ( -12.14591786802326823, 12.06949235617739902, 103.1260903946856757 ) ) ;
#30553=CARTESIAN_POINT ( 'NONE',  ( 10.72451020669871369, 18.67979575497193778, 57.08442372801901854 ) ) ;
#30554=CARTESIAN_POINT ( 'NONE',  ( 16.53943276465976808, 0.05219959533934440121, 21.25109039468567218 ) ) ;
#30555=CARTESIAN_POINT ( 'NONE',  ( 16.52544592524342804, -4.483927247898539470, 113.5405762719810383 ) ) ;
#30556=CARTESIAN_POINT ( 'NONE',  ( -16.55341960407617563, 4.379528057220093196, 28.54275706135234358 ) ) ;
#30557=CARTESIAN_POINT ( 'NONE',  ( 16.51473224551069308, 9.474510206698969483, 39.16557627198103120 ) ) ;
#30559=CARTESIAN_POINT ( 'NONE',  ( 13.97604488694527802, 13.89961937509977652, 109.3739096053143669 ) ) ;
#30561=CARTESIAN_POINT ( 'NONE',  ( 8.314922557961029526, -14.29746914071037800, 85.41775706135236135 ) ) ;
#30562=CARTESIAN_POINT ( 'NONE',  ( 19.05341960407617918, -5.049401038297876454, 81.04275706135231871 ) ) ;
#30563=CARTESIAN_POINT ( 'NONE',  ( -16.51473224551082808, 9.474510206698731452, 28.33442372801900433 ) ) ;
#30564=CARTESIAN_POINT ( 'NONE',  ( 0.05219959533907565091, 21.53943276465977519, 74.99890960531435269 ) ) ;
#30565=CARTESIAN_POINT ( 'NONE',  ( -4.379528057220086978, -16.55341960407618274, 94.79275706135234714 ) ) ;
#30566=CARTESIAN_POINT ( 'NONE',  ( -19.03943276465977164, -0.05219959533935918106, 93.75109039468566152 ) ) ;
#30567=CARTESIAN_POINT ( 'NONE',  ( 19.02544592524343514, -5.153800228976328945, 53.54057627198102409 ) ) ;
#30568=CARTESIAN_POINT ( 'NONE',  ( 9.474510206698971260, -16.51473224551069308, 87.91557627198102409 ) ) ;
#30569=CARTESIAN_POINT ( 'NONE',  ( 21.55341960407619695, -5.719274019375665929, 51.04275706135234714 ) ) ;
#30570=CARTESIAN_POINT ( 'NONE',  ( -0.05219959533909027116, -19.03943276465977164, 42.49890960531435269 ) ) ;
#30572=CARTESIAN_POINT ( 'NONE',  ( 9.474510206698971260, -16.51473224551069308, 107.9155762719810383 ) ) ;
#30573=CARTESIAN_POINT ( 'NONE',  ( 16.53943276465976808, -0.05219959533910856209, 63.74890960531435979 ) ) ;
#30574=CARTESIAN_POINT ( 'NONE',  ( -5.719274019375978568, 21.55341960407610458, 75.20724293864769550 ) ) ;
#30576=CARTESIAN_POINT ( 'NONE',  ( -5.049401038297874678, -19.05341960407617918, 44.79275706135232582 ) ) ;
#30577=CARTESIAN_POINT ( 'NONE',  ( 16.21995358207278670, -7.366697692864217828, 72.43551001512068410 ) ) ;
#30578=CARTESIAN_POINT ( 'NONE',  ( -19.03943276465977164, 0.05219959533909376836, 66.24890960531436690 ) ) ;
#30579=CARTESIAN_POINT ( 'NONE',  ( -0.05219959533909027116, -19.03943276465977164, 92.49890960531436690 ) ) ;
#30580=CARTESIAN_POINT ( 'NONE',  ( 8.224510206698742110, 14.34966873604972548, 47.08442372801901854 ) ) ;
#30581=CARTESIAN_POINT ( 'NONE',  ( -17.58332526062526213, -7.635886036038624702, 79.07665040441536064 ) ) ;
#30582=CARTESIAN_POINT ( 'NONE',  ( 19.02544592524334988, 5.153800228976608722, 36.45942372801900433 ) ) ;
#30583=CARTESIAN_POINT ( 'NONE',  ( -17.49999999999999645, 5.499999999999992006, 28.71769037696435234 ) ) ;
#30584=CARTESIAN_POINT ( 'NONE',  ( 16.53943276465976808, 0.05219959533934440121, 86.25109039468568994 ) ) ;
#30586=CARTESIAN_POINT ( 'NONE',  ( -8.314922557961024197, 14.29746914071037800, 82.91775706135234714 ) ) ;
#30587=CARTESIAN_POINT ( 'NONE',  ( -12.14591786802326823, 12.06949235617739902, 53.12609039468568284 ) ) ;
#30588=CARTESIAN_POINT ( 'NONE',  ( -21.53943276465977519, -0.05219959533937600094, 113.7510903946856757 ) ) ;
#30589=CARTESIAN_POINT ( 'NONE',  ( 13.97604488694527802, 13.89961937509977652, 54.37390960531435979 ) ) ;
#30591=CARTESIAN_POINT ( 'NONE',  ( -0.05219959533937732626, 21.53943276465977519, 67.50109039468568994 ) ) ;
#30592=CARTESIAN_POINT ( 'NONE',  ( 9.564922557961047289, -16.46253265017146816, 80.41775706135234714 ) ) ;
#30593=CARTESIAN_POINT ( 'NONE',  ( 15.80617190586769283, -15.72974639402175789, 105.6260903946856899 ) ) ;
#30594=CARTESIAN_POINT ( 'NONE',  ( 9.564922557960805705, 16.46253265017160317, 24.58224293864769194 ) ) ;
#30595=CARTESIAN_POINT ( 'NONE',  ( 17.39952324805926409, 6.147335277187066183, 23.87583945527051910 ) ) ;
#30596=CARTESIAN_POINT ( 'NONE',  ( -15.80617190586745835, -15.72974639402198527, 66.87390960531436690 ) ) ;
#30598=CARTESIAN_POINT ( 'NONE',  ( 10.81492255796078972, 18.62759615963270932, 24.58224293864768839 ) ) ;
#30599=CARTESIAN_POINT ( 'NONE',  ( 16.51473224551069308, 9.474510206698969483, 24.16557627198102765 ) ) ;
#30600=CARTESIAN_POINT ( 'NONE',  ( -16.52544592524335698, -4.483927247898792601, 38.95942372801901854 ) ) ;
#30601=CARTESIAN_POINT ( 'NONE',  ( -8.224510206698948167, 14.34966873604960824, 35.41557627198102409 ) ) ;
#30603=CARTESIAN_POINT ( 'NONE',  ( 10.72451020669871369, 18.67979575497193778, 22.08442372801901143 ) ) ;
#30604=CARTESIAN_POINT ( 'NONE',  ( 14.34966873604960469, 8.224510206698951720, 59.16557627198103120 ) ) ;
#30606=CARTESIAN_POINT ( 'NONE',  ( 9.474510206698729675, 16.51473224551082808, 112.0844237280190043 ) ) ;
#30607=CARTESIAN_POINT ( 'NONE',  ( 5.049401038297881783, 19.05341960407617563, 32.29275706135233293 ) ) ;
#30608=CARTESIAN_POINT ( 'NONE',  ( 14.34966873604960469, 8.224510206698951720, 49.16557627198102409 ) ) ;
#30609=CARTESIAN_POINT ( 'NONE',  ( 15.80617190586746368, 15.72974639402197994, 109.3739096053143811 ) ) ;
#30611=CARTESIAN_POINT ( 'NONE',  ( 5.719274019375991003, -21.55341960407610458, 67.70724293864769550 ) ) ;
#30612=CARTESIAN_POINT ( 'NONE',  ( 19.02544592524343514, -5.153800228976328945, 83.54057627198100988 ) ) ;
#30613=CARTESIAN_POINT ( 'NONE',  ( -8.314922557960811034, -14.29746914071050412, 47.08224293864770260 ) ) ;
#30614=CARTESIAN_POINT ( 'NONE',  ( 19.03943276465977164, -0.05219959533909143690, 98.74890960531436690 ) ) ;
#30616=CARTESIAN_POINT ( 'NONE',  ( 16.51473224551083163, -9.474510206698727899, 60.83442372801900433 ) ) ;
#30617=CARTESIAN_POINT ( 'NONE',  ( 21.55341960407610458, 5.719274019375980345, 93.95724293864770971 ) ) ;
#30618=CARTESIAN_POINT ( 'NONE',  ( -9.474510206698964154, 16.51473224551069663, 40.41557627198103120 ) ) ;
#30619=CARTESIAN_POINT ( 'NONE',  ( -4.379528057220328563, 16.55341960407611168, 115.2072429386476955 ) ) ;
#30620=CARTESIAN_POINT ( 'NONE',  ( -10.81492255796105439, 18.62759615963255655, 52.91775706135235424 ) ) ;
#30622=CARTESIAN_POINT ( 'NONE',  ( -14.29746914071049879, 8.314922557960819915, 30.83224293864770260 ) ) ;
#30623=CARTESIAN_POINT ( 'NONE',  ( -16.51473224551069308, -9.474510206698971260, 46.66557627198102409 ) ) ;
#30624=CARTESIAN_POINT ( 'NONE',  ( -19.02544592524342804, 5.153800228976336051, 106.0405762719810241 ) ) ;
#30625=CARTESIAN_POINT ( 'NONE',  ( -15.72974639402197994, 15.80617190586746368, 55.62390960531436690 ) ) ;
#30627=CARTESIAN_POINT ( 'NONE',  ( -5.049401038298153566, 19.05341960407611168, 45.20724293864769550 ) ) ;
#30628=CARTESIAN_POINT ( 'NONE',  ( 5.719274019375991003, -21.55341960407610458, 47.70724293864770260 ) ) ;
#30630=CARTESIAN_POINT ( 'NONE',  ( -5.823673210054431948, 21.52544592524334988, 92.70942372801901854 ) ) ;
#30632=CARTESIAN_POINT ( 'NONE',  ( -8.224510206698735004, -14.34966873604973081, 84.58442372801903275 ) ) ;
#30633=CARTESIAN_POINT ( 'NONE',  ( -16.55341960407617563, 4.379528057220093196, 93.54275706135234714 ) ) ;
#30634=CARTESIAN_POINT ( 'NONE',  ( 9.474510206698971260, -16.51473224551069308, 52.91557627198102409 ) ) ;
#30635=CARTESIAN_POINT ( 'NONE',  ( 16.46253265017160672, -9.564922557960803928, 68.33224293864770971 ) ) ;
#30637=CARTESIAN_POINT ( 'NONE',  ( -5.049401038297874678, -19.05341960407617918, 29.79275706135232227 ) ) ;
#30638=CARTESIAN_POINT ( 'NONE',  ( -16.53943276465976808, -0.05219959533934237506, 73.75109039468567573 ) ) ;
#30639=CARTESIAN_POINT ( 'NONE',  ( 16.46253265017146816, 9.564922557961045513, 21.66775706135233648 ) ) ;
#30640=CARTESIAN_POINT ( 'NONE',  ( -16.46253265017160317, 9.564922557960807481, 75.83224293864769550 ) ) ;
#30641=CARTESIAN_POINT ( 'NONE',  ( 15.72974639402199770, -15.80617190586745480, 53.12390960531436690 ) ) ;
#30642=CARTESIAN_POINT ( 'NONE',  ( -8.314922557961024197, 14.29746914071037800, 27.91775706135234358 ) ) ;
#30643=CARTESIAN_POINT ( 'NONE',  ( -21.52544592524334988, -5.823673210054445271, 78.95942372801901854 ) ) ;
#30644=CARTESIAN_POINT ( 'NONE',  ( 12.14591786802327356, -12.06949235617739191, 50.62609039468568994 ) ) ;
#30645=CARTESIAN_POINT ( 'NONE',  ( 15.72974639402199770, -15.80617190586745480, 108.1239096053143811 ) ) ;
#30646=CARTESIAN_POINT ( 'NONE',  ( -16.53943276465976808, -0.05219959533934237506, 18.75109039468568639 ) ) ;
#30647=CARTESIAN_POINT ( 'NONE',  ( -19.05341960407611168, -5.049401038298163336, 76.45724293864769550 ) ) ;
#30648=CARTESIAN_POINT ( 'NONE',  ( 4.379528057220092307, 16.55341960407617563, 32.29275706135235424 ) ) ;
#30649=CARTESIAN_POINT ( 'NONE',  ( 9.474510206698971260, -16.51473224551069308, 37.91557627198102409 ) ) ;
#30650=CARTESIAN_POINT ( 'NONE',  ( -16.55341960407617563, 4.379528057220093196, 23.54275706135235424 ) ) ;
#30651=CARTESIAN_POINT ( 'NONE',  ( -16.53943276465976808, 0.05219959533911058130, 76.24890960531435269 ) ) ;
#30652=CARTESIAN_POINT ( 'NONE',  ( -16.53943276465976808, -0.05219959533934237506, 83.75109039468568994 ) ) ;
#30653=CARTESIAN_POINT ( 'NONE',  ( 5.823673210054444382, -21.52544592524334988, 30.20942372801902565 ) ) ;
#30654=CARTESIAN_POINT ( 'NONE',  ( -5.049401038298153566, 19.05341960407611168, 60.20724293864768129 ) ) ;
#30655=CARTESIAN_POINT ( 'NONE',  ( -19.05341960407611168, -5.049401038298163336, 71.45724293864766707 ) ) ;
#30656=CARTESIAN_POINT ( 'NONE',  ( -14.34966873604972548, 8.224510206698743886, 88.33442372801901854 ) ) ;
#30657=AXIS2_PLACEMENT_3D ( 'NONE', #199289, #134649, #150810 ) ;
#30660=ORIENTED_EDGE ( 'NONE', *, *, #23111, .T. ) ;
#30661=CARTESIAN_POINT ( 'NONE',  ( 13.89961937509957401, 13.97604488694547697, 36.87609039468565442 ) ) ;
#30662=CARTESIAN_POINT ( 'NONE',  ( 19.03943276465977164, -0.05219959533909143690, 38.74890960531436690 ) ) ;
#30663=CARTESIAN_POINT ( 'NONE',  ( -5.049401038298153566, 19.05341960407611168, 115.2072429386477097 ) ) ;
#30665=CARTESIAN_POINT ( 'NONE',  ( -14.29746914071037622, -8.314922557961029526, 24.16775706135235424 ) ) ;
#30666=CARTESIAN_POINT ( 'NONE',  ( -5.153800228976607833, 19.02544592524334988, 57.70942372801899012 ) ) ;
#30667=CARTESIAN_POINT ( 'NONE',  ( 16.52544592524335698, 4.483927247898782831, 41.45942372801901143 ) ) ;
#30668=CARTESIAN_POINT ( 'NONE',  ( -16.46253265017160317, 9.564922557960807481, 110.8322429386476955 ) ) ;
#30669=CARTESIAN_POINT ( 'NONE',  ( -13.97604488694527625, -13.89961937509977652, 66.87390960531436690 ) ) ;
#30670=CARTESIAN_POINT ( 'NONE',  ( 10.81492255796078972, 18.62759615963270932, 104.5822429386477097 ) ) ;
#30671=CARTESIAN_POINT ( 'NONE',  ( -5.153800228976328057, -19.02544592524343514, 92.29057627198099567 ) ) ;
#30672=CARTESIAN_POINT ( 'NONE',  ( 0.05219959533909260263, 19.03943276465977164, 24.99890960531435269 ) ) ;
#30673=CARTESIAN_POINT ( 'NONE',  ( -19.02544592524342804, 5.153800228976336051, 66.04057627198103830 ) ) ;
#30674=CARTESIAN_POINT ( 'NONE',  ( -4.483927247898539470, -16.52544592524342804, 27.29057627198103120 ) ) ;
#30675=CARTESIAN_POINT ( 'NONE',  ( 17.59860650958989936, 7.585241751807028088, 69.07662985737508166 ) ) ;
#30676=CARTESIAN_POINT ( 'NONE',  ( -5.153800228976607833, 19.02544592524334988, 42.70942372801901143 ) ) ;
#30678=CARTESIAN_POINT ( 'NONE',  ( 14.29746914071049879, -8.314922557960816363, 58.33224293864768839 ) ) ;
#30679=CARTESIAN_POINT ( 'NONE',  ( -5.719274019375665041, -21.55341960407619695, 94.79275706135234714 ) ) ;
#30680=CARTESIAN_POINT ( 'NONE',  ( -9.474510206698964154, 16.51473224551069663, 35.41557627198102409 ) ) ;
#30681=CARTESIAN_POINT ( 'NONE',  ( -4.379528057220086978, -16.55341960407618274, 54.79275706135235424 ) ) ;
#30683=CARTESIAN_POINT ( 'NONE',  ( -12.14591786802309592, -12.06949235617757132, 36.87390960531435979 ) ) ;
#30684=CARTESIAN_POINT ( 'NONE',  ( -21.53943276465977519, -0.05219959533937600094, 88.75109039468567573 ) ) ;
#30685=CARTESIAN_POINT ( 'NONE',  ( 16.51473224551069308, 9.474510206698969483, 84.16557627198102409 ) ) ;
#30686=CARTESIAN_POINT ( 'NONE',  ( 19.02544592524343514, -5.153800228976328945, 98.54057627198100988 ) ) ;
#30687=CARTESIAN_POINT ( 'NONE',  ( -8.224510206698948167, 14.34966873604960824, 105.4155762719810383 ) ) ;
#30688=CARTESIAN_POINT ( 'NONE',  ( 0.05219959533910956823, 16.53943276465976808, 74.99890960531435269 ) ) ;
#30689=CARTESIAN_POINT ( 'NONE',  ( 18.62759615963271287, -10.81492255796078972, 83.33224293864769550 ) ) ;
#30690=CARTESIAN_POINT ( 'NONE',  ( -0.05219959533909027116, -19.03943276465977164, 92.49890960531436690 ) ) ;
#30691=CARTESIAN_POINT ( 'NONE',  ( -10.81492255796078084, -18.62759615963271287, 102.0822429386476955 ) ) ;
#30693=CARTESIAN_POINT ( 'NONE',  ( -0.05219959533936034679, 19.03943276465977164, 77.50109039468566152 ) ) ;
#30695=CARTESIAN_POINT ( 'NONE',  ( 16.55341960407611168, 4.379528057220329451, 83.95724293864770971 ) ) ;
#30696=CARTESIAN_POINT ( 'NONE',  ( -19.02544592524342804, 5.153800228976336051, 56.04057627198100988 ) ) ;
#30697=CARTESIAN_POINT ( 'NONE',  ( -15.80617190586745835, -15.72974639402198527, 71.87390960531438111 ) ) ;
#30698=CARTESIAN_POINT ( 'NONE',  ( 17.48853670773243252, -5.747243402303153559, 26.16671299749992130 ) ) ;
#30699=CARTESIAN_POINT ( 'NONE',  ( 14.34966873604960469, 8.224510206698951720, 24.16557627198103120 ) ) ;
#30701=CARTESIAN_POINT ( 'NONE',  ( 16.55341960407618274, -4.379528057220086978, 21.04275706135234714 ) ) ;
#30702=CARTESIAN_POINT ( 'NONE',  ( -8.314922557960811034, -14.29746914071050412, 82.08224293864768129 ) ) ;
#30704=CARTESIAN_POINT ( 'NONE',  ( -13.89961937509977652, 13.97604488694528158, 80.62390960531436690 ) ) ;
#30705=CARTESIAN_POINT ( 'NONE',  ( 13.97604488694527802, 13.89961937509977652, 34.37390960531436690 ) ) ;
#30706=CARTESIAN_POINT ( 'NONE',  ( 14.29746914071049879, -8.314922557960816363, 63.33224293864770260 ) ) ;
#30707=CARTESIAN_POINT ( 'NONE',  ( -13.89961937509977652, 13.97604488694528158, 110.6239096053143243 ) ) ;
#30708=CARTESIAN_POINT ( 'NONE',  ( -19.02544592524334988, -5.153800228976617603, 93.95942372801900433 ) ) ;
#30710=CARTESIAN_POINT ( 'NONE',  ( 19.03943276465977164, -0.05219959533909143690, 98.74890960531436690 ) ) ;
#30711=CARTESIAN_POINT ( 'NONE',  ( 21.53943276465977519, -0.05219959533907433946, 73.74890960531433848 ) ) ;
#30712=CARTESIAN_POINT ( 'NONE',  ( 12.06949235617739724, 12.14591786802326823, 76.87609039468567573 ) ) ;
#30713=AXIS2_PLACEMENT_3D ( 'NONE', #154163, #62135, #123799 ) ;
#30714=CARTESIAN_POINT ( 'NONE',  ( 5.153800228976617603, -19.02544592524335343, 110.2094237280189901 ) ) ;
#30715=CARTESIAN_POINT ( 'NONE',  ( 13.97604488694527802, 13.89961937509977652, 59.37390960531434558 ) ) ;
#30716=CARTESIAN_POINT ( 'NONE',  ( 10.81492255796078972, 18.62759615963270932, 69.58224293864769550 ) ) ;
#30717=CARTESIAN_POINT ( 'NONE',  ( 4.379528057220092307, 16.55341960407617563, 107.2927570613523471 ) ) ;
#30718=CARTESIAN_POINT ( 'NONE',  ( -0.05219959533936034679, 19.03943276465977164, 112.5010903946856757 ) ) ;
#30719=CARTESIAN_POINT ( 'NONE',  ( 4.379528057220339221, -16.55341960407611168, 32.70724293864770260 ) ) ;
#30720=CARTESIAN_POINT ( 'NONE',  ( -18.67979575497193778, 10.72451020669871902, 63.33442372801900433 ) ) ;
#30722=CARTESIAN_POINT ( 'NONE',  ( -16.53943276465976808, -0.05219959533934237506, 73.75109039468567573 ) ) ;
#30723=CARTESIAN_POINT ( 'NONE',  ( 16.51473224551069308, 9.474510206698969483, 104.1655762719810241 ) ) ;
#30724=CARTESIAN_POINT ( 'NONE',  ( 19.05341960407611168, 5.049401038298154454, 103.9572429386476813 ) ) ;
#30725=CARTESIAN_POINT ( 'NONE',  ( -17.44270441346519007, 5.991230190322968774, 78.63664920735773478 ) ) ;
#30726=CARTESIAN_POINT ( 'NONE',  ( -8.314922557961024197, 14.29746914071037800, 97.91775706135236135 ) ) ;
#30727=CARTESIAN_POINT ( 'NONE',  ( 14.34966873604972726, -8.224510206698740333, 45.83442372801901854 ) ) ;
#30728=CARTESIAN_POINT ( 'NONE',  ( 13.89961937509977652, -13.97604488694527269, 53.12390960531434558 ) ) ;
#30729=CARTESIAN_POINT ( 'NONE',  ( -16.46253265017160317, 9.564922557960807481, 75.83224293864769550 ) ) ;
#30730=CARTESIAN_POINT ( 'NONE',  ( 10.72451020669871369, 18.67979575497193778, 57.08442372801901854 ) ) ;
#30731=CARTESIAN_POINT ( 'NONE',  ( 16.53943276465976808, 0.05219959533934440121, 56.25109039468568284 ) ) ;
#30732=CARTESIAN_POINT ( 'NONE',  ( 14.29746914071049879, -8.314922557960816363, 28.33224293864769550 ) ) ;
#30733=CARTESIAN_POINT ( 'NONE',  ( -13.97604488694527625, -13.89961937509977652, 36.87390960531436690 ) ) ;
#30734=CARTESIAN_POINT ( 'NONE',  ( -5.153800228976328057, -19.02544592524343514, 32.29057627198102409 ) ) ;
#30735=CARTESIAN_POINT ( 'NONE',  ( -16.55341960407617563, 4.379528057220093196, 33.54275706135234714 ) ) ;
#30736=CARTESIAN_POINT ( 'NONE',  ( -19.03943276465977164, -0.05219959533935918106, 83.75109039468567573 ) ) ;
#30737=CARTESIAN_POINT ( 'NONE',  ( 12.14591786802309770, 12.06949235617756955, 79.37390960531436690 ) ) ;
#30738=CARTESIAN_POINT ( 'NONE',  ( 5.049401038298161559, -19.05341960407611168, 47.70724293864770260 ) ) ;
#30739=CARTESIAN_POINT ( 'NONE',  ( -13.89961937509957401, -13.97604488694547875, 89.37609039468563310 ) ) ;
#30740=CARTESIAN_POINT ( 'NONE',  ( -18.67979575497193778, 10.72451020669871902, 93.33442372801901854 ) ) ;
#30741=CARTESIAN_POINT ( 'NONE',  ( -8.224510206698735004, -14.34966873604973081, 54.58442372801901143 ) ) ;
#30742=CARTESIAN_POINT ( 'NONE',  ( -17.50000000000000000, 5.068104630630428709, 25.72818405340030523 ) ) ;
#30743=CARTESIAN_POINT ( 'NONE',  ( 10.81492255796078972, 18.62759615963270932, 54.58224293864769550 ) ) ;
#30744=CARTESIAN_POINT ( 'NONE',  ( -16.55341960407617563, 4.379528057220093196, 38.54275706135234714 ) ) ;
#30745=CARTESIAN_POINT ( 'NONE',  ( 18.22780087662119897, -5.500000000000146549, 38.51763182126893525 ) ) ;
#30746=CARTESIAN_POINT ( 'NONE',  ( 5.049401038297881783, 19.05341960407617563, 37.29275706135232582 ) ) ;
#30747=CARTESIAN_POINT ( 'NONE',  ( -9.474510206698964154, 16.51473224551069663, 95.41557627198102409 ) ) ;
#30748=CARTESIAN_POINT ( 'NONE',  ( 16.46253265017160672, -9.564922557960803928, 48.33224293864769550 ) ) ;
#30751=CARTESIAN_POINT ( 'NONE',  ( 15.72974639402176855, 15.80617190586768217, 76.87609039468567573 ) ) ;
#30752=CARTESIAN_POINT ( 'NONE',  ( -17.49999999999999645, 5.500000000000037303, 50.79690382534172244 ) ) ;
#30754=CARTESIAN_POINT ( 'NONE',  ( -9.564922557961040184, 16.46253265017147172, 32.91775706135233293 ) ) ;
#30755=CARTESIAN_POINT ( 'NONE',  ( -10.72451020669870658, -18.67979575497194134, 104.5844237280190185 ) ) ;
#30756=CARTESIAN_POINT ( 'NONE',  ( -0.05219959533910754901, -16.53943276465976808, 32.49890960531435979 ) ) ;
#30757=CARTESIAN_POINT ( 'NONE',  ( -19.05341960407611168, -5.049401038298163336, 46.45724293864768129 ) ) ;
#30758=CARTESIAN_POINT ( 'NONE',  ( -19.03943276465977164, 0.05219959533909376836, 101.2489096053143669 ) ) ;
#30759=CARTESIAN_POINT ( 'NONE',  ( 5.823673210054444382, -21.52544592524334988, 85.20942372801901854 ) ) ;
#30760=CARTESIAN_POINT ( 'NONE',  ( -5.049401038298153566, 19.05341960407611168, 60.20724293864768129 ) ) ;
#30761=CARTESIAN_POINT ( 'NONE',  ( 15.72974639402176855, 15.80617190586768217, 81.87609039468568994 ) ) ;
#30762=CARTESIAN_POINT ( 'NONE',  ( -18.67979575497178146, -10.72451020669898902, 36.66557627198103120 ) ) ;
#30763=CARTESIAN_POINT ( 'NONE',  ( -5.823673210054431948, 21.52544592524334988, 27.70942372801901854 ) ) ;
#30764=CARTESIAN_POINT ( 'NONE',  ( 13.89961937509957401, 13.97604488694547697, 41.87609039468566152 ) ) ;
#30765=CARTESIAN_POINT ( 'NONE',  ( 19.03943276465977164, -0.05219959533909143690, 23.74890960531435269 ) ) ;
#30766=CARTESIAN_POINT ( 'NONE',  ( 16.51473224551069308, 9.474510206698969483, 74.16557627198103830 ) ) ;
#30767=CARTESIAN_POINT ( 'NONE',  ( -4.379528057220086978, -16.55341960407618274, 29.79275706135234358 ) ) ;
#30768=CARTESIAN_POINT ( 'NONE',  ( 16.53943276465976808, -0.05219959533910856209, 83.74890960531435269 ) ) ;
#30769=CARTESIAN_POINT ( 'NONE',  ( 5.049401038298161559, -19.05341960407611168, 52.70724293864767418 ) ) ;
#30770=CARTESIAN_POINT ( 'NONE',  ( -21.52544592524343514, 5.823673210054127303, 31.04057627198102409 ) ) ;
#30771=CARTESIAN_POINT ( 'NONE',  ( 13.89961937509957401, 13.97604488694547697, 101.8760903946856331 ) ) ;
#30772=CARTESIAN_POINT ( 'NONE',  ( -5.823673210054116645, -21.52544592524344225, 107.2905762719810525 ) ) ;
#30773=CARTESIAN_POINT ( 'NONE',  ( 5.719274019375673035, 21.55341960407619339, 72.29275706135236135 ) ) ;
#30774=CARTESIAN_POINT ( 'NONE',  ( 12.06949235617739724, 12.14591786802326823, 66.87609039468568994 ) ) ;
#30775=CARTESIAN_POINT ( 'NONE',  ( 8.314922557961029526, -14.29746914071037800, 65.41775706135234714 ) ) ;
#30776=VERTEX_POINT ( 'NONE', #136611 ) ;
#30777=CARTESIAN_POINT ( 'NONE',  ( 13.97604488694527802, 13.89961937509977652, 59.37390960531434558 ) ) ;
#30778=CARTESIAN_POINT ( 'NONE',  ( -16.55341960407617563, 4.379528057220093196, 93.54275706135234714 ) ) ;
#30779=CARTESIAN_POINT ( 'NONE',  ( -15.72974639402176322, -15.80617190586768395, 19.37609039468568639 ) ) ;
#30780=CARTESIAN_POINT ( 'NONE',  ( -4.379528057220328563, 16.55341960407611168, 65.20724293864768129 ) ) ;
#30781=CARTESIAN_POINT ( 'NONE',  ( -9.564922557960796823, -16.46253265017161027, 92.08224293864769550 ) ) ;
#30782=CARTESIAN_POINT ( 'NONE',  ( 12.06949235617739724, 12.14591786802326823, 81.87609039468568994 ) ) ;
#30783=CARTESIAN_POINT ( 'NONE',  ( 5.823673210054444382, -21.52544592524334988, 55.20942372801902565 ) ) ;
#30784=CARTESIAN_POINT ( 'NONE',  ( 19.02544592524334988, 5.153800228976608722, 111.4594237280190043 ) ) ;
#30785=CARTESIAN_POINT ( 'NONE',  ( 18.67979575497178502, 10.72451020669898547, 114.1655762719810383 ) ) ;
#30786=CARTESIAN_POINT ( 'NONE',  ( -0.05219959533910754901, -16.53943276465976808, 62.49890960531436690 ) ) ;
#30788=CARTESIAN_POINT ( 'NONE',  ( -0.05219959533907301413, -21.53943276465977519, 87.49890960531436690 ) ) ;
#30789=CARTESIAN_POINT ( 'NONE',  ( 16.53943276465976808, -0.05219959533910856209, 38.74890960531435979 ) ) ;
#30790=ORIENTED_EDGE ( 'NONE', *, *, #131008, .F. ) ;
#30792=CARTESIAN_POINT ( 'NONE',  ( 5.823673210054444382, -21.52544592524334988, 20.20942372801900788 ) ) ;
#30793=CARTESIAN_POINT ( 'NONE',  ( 19.03943276465977164, -0.05219959533909143690, 113.7489096053143669 ) ) ;
#30794=CARTESIAN_POINT ( 'NONE',  ( 5.823673210054444382, -21.52544592524334988, 35.20942372801901854 ) ) ;
#30795=CARTESIAN_POINT ( 'NONE',  ( -4.379528057220328563, 16.55341960407611168, 45.20724293864769550 ) ) ;
#30796=CARTESIAN_POINT ( 'NONE',  ( -16.51473224551069308, -9.474510206698971260, 66.66557627198102409 ) ) ;
#30797=CARTESIAN_POINT ( 'NONE',  ( 19.05341960407617918, -5.049401038297876454, 61.04275706135232582 ) ) ;
#30798=CARTESIAN_POINT ( 'NONE',  ( -0.05219959533909027116, -19.03943276465977164, 92.49890960531436690 ) ) ;
#30799=CARTESIAN_POINT ( 'NONE',  ( 18.67979575497178502, 10.72451020669898547, 49.16557627198102409 ) ) ;
#30801=CARTESIAN_POINT ( 'NONE',  ( -0.05219959533909027116, -19.03943276465977164, 52.49890960531436690 ) ) ;
#30802=CARTESIAN_POINT ( 'NONE',  ( 12.06949235617739724, 12.14591786802326823, 36.87609039468568994 ) ) ;
#30803=CARTESIAN_POINT ( 'NONE',  ( -19.05341960407617563, 5.049401038297882671, 58.54275706135234003 ) ) ;
#30804=CARTESIAN_POINT ( 'NONE',  ( -5.823673210054431948, 21.52544592524334988, 22.70942372801901499 ) ) ;
#30805=CARTESIAN_POINT ( 'NONE',  ( 16.53943276465976808, -0.05219959533910856209, 43.74890960531435979 ) ) ;
#30806=CARTESIAN_POINT ( 'NONE',  ( 9.564922557960805705, 16.46253265017160317, 84.58224293864769550 ) ) ;
#30807=CARTESIAN_POINT ( 'NONE',  ( -18.67979575497178146, -10.72451020669898902, 76.66557627198103830 ) ) ;
#30808=CARTESIAN_POINT ( 'NONE',  ( -18.67979575497178146, -10.72451020669898902, 96.66557627198102409 ) ) ;
#30809=CARTESIAN_POINT ( 'NONE',  ( -16.55341960407617563, 4.379528057220093196, 43.54275706135235424 ) ) ;
#30810=CARTESIAN_POINT ( 'NONE',  ( -21.53943276465977519, 0.05219959533907696930, 31.24890960531435979 ) ) ;
#30811=CARTESIAN_POINT ( 'NONE',  ( 18.62759615963255655, 10.81492255796105972, 91.66775706135234714 ) ) ;
#30812=CARTESIAN_POINT ( 'NONE',  ( -9.474510206698964154, 16.51473224551069663, 90.41557627198103830 ) ) ;
#30813=CARTESIAN_POINT ( 'NONE',  ( -19.05341960407611168, -5.049401038298163336, 41.45724293864769550 ) ) ;
#30814=CARTESIAN_POINT ( 'NONE',  ( -13.97604488694527625, -13.89961937509977652, 91.87390960531432427 ) ) ;
#30815=CARTESIAN_POINT ( 'NONE',  ( -14.34966873604960291, -8.224510206698953496, 101.6655762719810383 ) ) ;
#30816=CARTESIAN_POINT ( 'NONE',  ( 13.97604488694527802, 13.89961937509977652, 59.37390960531434558 ) ) ;
#30817=CARTESIAN_POINT ( 'NONE',  ( -13.97604488694547697, 13.89961937509957934, 113.1260903946856757 ) ) ;
#30818=CARTESIAN_POINT ( 'NONE',  ( 17.44270441346519007, -5.991230190322930582, 86.13664920735777741 ) ) ;
#30820=CARTESIAN_POINT ( 'NONE',  ( 0.05219959533936267826, -19.03943276465977164, 60.00109039468566863 ) ) ;
#30821=CARTESIAN_POINT ( 'NONE',  ( -21.53943276465977519, -0.05219959533937600094, 93.75109039468567573 ) ) ;
#30822=CARTESIAN_POINT ( 'NONE',  ( -21.53943276465977519, 0.05219959533907696930, 36.24890960531435979 ) ) ;
#30823=CARTESIAN_POINT ( 'NONE',  ( 0.05219959533934541429, -16.53943276465976808, 90.00109039468567573 ) ) ;
#30824=DIRECTION ( 'NONE',  ( -0.000000000000000000, -0.000000000000000000, 1.000000000000000000 ) ) ;
#30825=CARTESIAN_POINT ( 'NONE',  ( 16.46253265017146816, 9.564922557961045513, 76.66775706135234714 ) ) ;
#30826=CARTESIAN_POINT ( 'NONE',  ( -5.049401038297874678, -19.05341960407617918, 34.79275706135233293 ) ) ;
#30828=CARTESIAN_POINT ( 'NONE',  ( 16.46253265017160672, -9.564922557960803928, 48.33224293864769550 ) ) ;
#30829=CARTESIAN_POINT ( 'NONE',  ( 4.379528057220339221, -16.55341960407611168, 32.70724293864770260 ) ) ;
#30830=CARTESIAN_POINT ( 'NONE',  ( -16.81555441253553340, -7.025013491695469625, 109.3631455466574209 ) ) ;
#30831=CARTESIAN_POINT ( 'NONE',  ( 12.06949235617757843, -12.14591786802309237, 23.12390960531436335 ) ) ;
#30832=DIRECTION ( 'NONE',  ( 0.000000000000000000, 0.000000000000000000, -1.000000000000000000 ) ) ;
#30833=CARTESIAN_POINT ( 'NONE',  ( -4.483927247898782831, 16.52544592524335698, 97.70942372801904696 ) ) ;
#30834=CARTESIAN_POINT ( 'NONE',  ( -0.05219959533909027116, -19.03943276465977164, 32.49890960531435979 ) ) ;
#30835=CARTESIAN_POINT ( 'NONE',  ( -21.55341960407619339, 5.719274019375674811, 108.5427570613523756 ) ) ;
#30836=CARTESIAN_POINT ( 'NONE',  ( 14.34966873604972726, -8.224510206698740333, 20.83442372801901143 ) ) ;
#30837=CARTESIAN_POINT ( 'NONE',  ( -21.52544592524334988, -5.823673210054445271, 78.95942372801901854 ) ) ;
#30839=CARTESIAN_POINT ( 'NONE',  ( -5.049401038297874678, -19.05341960407617918, 54.79275706135234003 ) ) ;
#30840=CARTESIAN_POINT ( 'NONE',  ( 19.02544592524343514, -5.153800228976328945, 88.54057627198102409 ) ) ;
#30841=CARTESIAN_POINT ( 'NONE',  ( -16.46253265017160317, 9.564922557960807481, 85.83224293864769550 ) ) ;
#30842=CARTESIAN_POINT ( 'NONE',  ( 16.20579543436676673, 7.371946100355104114, 73.06520834171871570 ) ) ;
#30843=CARTESIAN_POINT ( 'NONE',  ( 18.62759615963271287, -10.81492255796078972, 113.3322429386476955 ) ) ;
#30845=CARTESIAN_POINT ( 'NONE',  ( -12.14591786802309592, -12.06949235617757132, 61.87390960531436690 ) ) ;
#30846=CARTESIAN_POINT ( 'NONE',  ( -21.55341960407610458, -5.719274019375992779, 66.45724293864768129 ) ) ;
#30847=CARTESIAN_POINT ( 'NONE',  ( -16.46253265017160317, 9.564922557960807481, 60.83224293864769550 ) ) ;
#30848=CARTESIAN_POINT ( 'NONE',  ( -15.80617190586745835, -15.72974639402198527, 91.87390960531436690 ) ) ;
#30849=CARTESIAN_POINT ( 'NONE',  ( 16.55341960407618274, -4.379528057220086978, 96.04275706135236135 ) ) ;
#30851=CARTESIAN_POINT ( 'NONE',  ( 13.97604488694527802, 13.89961937509977652, 49.37390960531434558 ) ) ;
#30852=CARTESIAN_POINT ( 'NONE',  ( -14.29746914071049879, 8.314922557960819915, 95.83224293864770971 ) ) ;
#30854=CARTESIAN_POINT ( 'NONE',  ( -19.02544592524342804, 5.153800228976336051, 51.04057627198103120 ) ) ;
#30855=CARTESIAN_POINT ( 'NONE',  ( -8.224510206698948167, 14.34966873604960824, 115.4155762719810241 ) ) ;
#30856=CARTESIAN_POINT ( 'NONE',  ( -5.153800228976607833, 19.02544592524334988, 77.70942372801900433 ) ) ;
#30857=CARTESIAN_POINT ( 'NONE',  ( -4.483927247898539470, -16.52544592524342804, 82.29057627198103830 ) ) ;
#30858=CARTESIAN_POINT ( 'NONE',  ( 21.55341960407619695, -5.719274019375665929, 46.04275706135234714 ) ) ;
#30859=CARTESIAN_POINT ( 'NONE',  ( -9.564922557960796823, -16.46253265017161027, 32.08224293864769550 ) ) ;
#30860=CARTESIAN_POINT ( 'NONE',  ( 5.823673210054125526, 21.52544592524343514, 109.7905762719810383 ) ) ;
#30861=CARTESIAN_POINT ( 'NONE',  ( -8.224510206698948167, 14.34966873604960824, 85.41557627198102409 ) ) ;
#30863=CARTESIAN_POINT ( 'NONE',  ( -19.02544592524342804, 5.153800228976336051, 66.04057627198103830 ) ) ;
#30866=CARTESIAN_POINT ( 'NONE',  ( 13.97604488694548053, -13.89961937509957401, 90.62609039468567573 ) ) ;
#30867=CARTESIAN_POINT ( 'NONE',  ( 5.049401038298161559, -19.05341960407611168, 107.7072429386476955 ) ) ;
#30868=CARTESIAN_POINT ( 'NONE',  ( 21.53943276465977519, 0.05219959533937863772, 41.25109039468568284 ) ) ;
#30869=CARTESIAN_POINT ( 'NONE',  ( 13.89961937509977652, -13.97604488694527269, 83.12390960531436690 ) ) ;
#30870=CARTESIAN_POINT ( 'NONE',  ( 16.46253265017146816, 9.564922557961045513, 71.66775706135233293 ) ) ;
#30871=CARTESIAN_POINT ( 'NONE',  ( 19.05341960407611168, 5.049401038298154454, 53.95724293864770260 ) ) ;
#30872=CARTESIAN_POINT ( 'NONE',  ( -8.314922557960811034, -14.29746914071050412, 82.08224293864768129 ) ) ;
#30873=CARTESIAN_POINT ( 'NONE',  ( -16.53943276465976808, 0.05219959533911058130, 66.24890960531436690 ) ) ;
#30874=CARTESIAN_POINT ( 'NONE',  ( 5.153800228976335163, 19.02544592524342804, 84.79057627198099567 ) ) ;
#30875=CARTESIAN_POINT ( 'NONE',  ( -15.72974639402197994, 15.80617190586746368, 95.62390960531436690 ) ) ;
#30876=CARTESIAN_POINT ( 'NONE',  ( -9.474510206698964154, 16.51473224551069663, 90.41557627198103830 ) ) ;
#30877=CARTESIAN_POINT ( 'NONE',  ( 5.153800228976615827, -19.02544592524334988, 35.20942372801899722 ) ) ;
#30878=CARTESIAN_POINT ( 'NONE',  ( -9.564922557960796823, -16.46253265017161027, 42.08224293864769550 ) ) ;
#30879=CARTESIAN_POINT ( 'NONE',  ( -4.483927247898539470, -16.52544592524342804, 32.29057627198102409 ) ) ;
#30880=CARTESIAN_POINT ( 'NONE',  ( -12.06949235617756955, 12.14591786802309770, 115.6239096053143669 ) ) ;
#30882=CARTESIAN_POINT ( 'NONE',  ( 18.62759615963255655, 10.81492255796105972, 31.66775706135234358 ) ) ;
#30883=CARTESIAN_POINT ( 'NONE',  ( -19.05341960407617563, 5.049401038297882671, 63.54275706135234003 ) ) ;
#30884=CARTESIAN_POINT ( 'NONE',  ( -16.53943276465976808, 0.05219959533911058130, 31.24890960531435979 ) ) ;
#30885=CARTESIAN_POINT ( 'NONE',  ( -0.05219959533907301413, -21.53943276465977519, 87.49890960531436690 ) ) ;
#30886=CARTESIAN_POINT ( 'NONE',  ( 5.153800228976335163, 19.02544592524342804, 114.7905762719810241 ) ) ;
#30887=CARTESIAN_POINT ( 'NONE',  ( -14.34966873604960291, -8.224510206698953496, 66.66557627198102409 ) ) ;
#30888=CARTESIAN_POINT ( 'NONE',  ( 0.05219959533909260263, 19.03943276465977164, 24.99890960531435269 ) ) ;
#30889=CARTESIAN_POINT ( 'NONE',  ( 5.049401038297881783, 19.05341960407617563, 22.29275706135233648 ) ) ;
#30890=CARTESIAN_POINT ( 'NONE',  ( -0.05219959533934338120, 16.53943276465976808, 102.5010903946856899 ) ) ;
#30891=CARTESIAN_POINT ( 'NONE',  ( -8.224510206698735004, -14.34966873604973081, 54.58442372801901143 ) ) ;
#30892=CARTESIAN_POINT ( 'NONE',  ( -18.67979575497178146, -10.72451020669898902, 41.66557627198103120 ) ) ;
#30893=CARTESIAN_POINT ( 'NONE',  ( 18.62759615963255655, 10.81492255796105972, 111.6677570613523613 ) ) ;
#30894=CARTESIAN_POINT ( 'NONE',  ( 9.474510206698971260, -16.51473224551069308, 82.91557627198103830 ) ) ;
#30895=CARTESIAN_POINT ( 'NONE',  ( 12.06949235617739724, 12.14591786802326823, 56.87609039468568994 ) ) ;
#30896=CARTESIAN_POINT ( 'NONE',  ( 0.05219959533910956823, 16.53943276465976808, 114.9989096053143669 ) ) ;
#30898=CARTESIAN_POINT ( 'NONE',  ( -14.29746914071049879, 8.314922557960819915, 30.83224293864770260 ) ) ;
#30899=CARTESIAN_POINT ( 'NONE',  ( 9.564922557960805705, 16.46253265017160317, 104.5822429386476955 ) ) ;
#30900=CARTESIAN_POINT ( 'NONE',  ( 0.05219959533909260263, 19.03943276465977164, 89.99890960531436690 ) ) ;
#30901=CARTESIAN_POINT ( 'NONE',  ( -13.89961937509977652, 13.97604488694528158, 115.6239096053143669 ) ) ;
#30902=CARTESIAN_POINT ( 'NONE',  ( 14.29746914071049879, -8.314922557960816363, 63.33224293864770260 ) ) ;
#30903=CARTESIAN_POINT ( 'NONE',  ( 4.379528057220339221, -16.55341960407611168, 37.70724293864769550 ) ) ;
#30904=CARTESIAN_POINT ( 'NONE',  ( -16.55341960407611168, -4.379528057220339221, 56.45724293864768839 ) ) ;
#30905=CARTESIAN_POINT ( 'NONE',  ( 4.483927247898790824, -16.52544592524335698, 45.20942372801901854 ) ) ;
#30906=CARTESIAN_POINT ( 'NONE',  ( -5.049401038297874678, -19.05341960407618274, 59.79275706135232582 ) ) ;
#30907=CARTESIAN_POINT ( 'NONE',  ( -13.89961937509957401, -13.97604488694547875, 49.37609039468567573 ) ) ;
#30908=CARTESIAN_POINT ( 'NONE',  ( -19.02544592524342804, 5.153800228976336051, 71.04057627198099567 ) ) ;
#30909=CARTESIAN_POINT ( 'NONE',  ( 19.05341960407617918, -5.049401038297876454, 71.04275706135234714 ) ) ;
#30911=CARTESIAN_POINT ( 'NONE',  ( -9.474510206698720793, -16.51473224551083518, 54.58442372801899722 ) ) ;
#30912=CARTESIAN_POINT ( 'NONE',  ( -0.05219959533936034679, 19.03943276465977164, 102.5010903946856757 ) ) ;
#30913=CARTESIAN_POINT ( 'NONE',  ( 12.06949235617739724, 12.14591786802326823, 76.87609039468567573 ) ) ;
#30916=CARTESIAN_POINT ( 'NONE',  ( 19.05341960407611168, 5.049401038298154454, 113.9572429386477097 ) ) ;
#30917=CARTESIAN_POINT ( 'NONE',  ( 15.80617190586769283, -15.72974639402175789, 35.62609039468568994 ) ) ;
#30918=CARTESIAN_POINT ( 'NONE',  ( -5.049401038297874678, -19.05341960407617918, 109.7927570613523187 ) ) ;
#30919=DIRECTION ( 'NONE',  ( -1.000000000000000000, 8.673617379884036458E-16, -0.000000000000000000 ) ) ;
#30920=CARTESIAN_POINT ( 'NONE',  ( -13.89961937509977652, 13.97604488694528158, 65.62390960531436690 ) ) ;
#30921=CARTESIAN_POINT ( 'NONE',  ( -19.05341960407611168, -5.049401038298163336, 101.4572429386476955 ) ) ;
#30922=CARTESIAN_POINT ( 'NONE',  ( 4.483927247898545687, 16.52544592524342804, 64.79057627198103830 ) ) ;
#30923=CARTESIAN_POINT ( 'NONE',  ( 5.049401038298161559, -19.05341960407611168, 57.70724293864769550 ) ) ;
#30924=CARTESIAN_POINT ( 'NONE',  ( 9.564922557960805705, 16.46253265017160317, 59.58224293864769550 ) ) ;
#30925=CARTESIAN_POINT ( 'NONE',  ( 0.05219959533936267826, -19.03943276465977164, 75.00109039468566152 ) ) ;
#30926=CARTESIAN_POINT ( 'NONE',  ( 10.81492255796078972, 18.62759615963270932, 49.58224293864769550 ) ) ;
#30927=CARTESIAN_POINT ( 'NONE',  ( 0.05219959533910956823, 16.53943276465976808, 114.9989096053143669 ) ) ;
#30928=CARTESIAN_POINT ( 'NONE',  ( -13.89961937509957401, -13.97604488694547875, 39.37609039468566152 ) ) ;
#30929=CARTESIAN_POINT ( 'NONE',  ( -0.05219959533909027116, -19.03943276465977164, 77.49890960531435269 ) ) ;
#30930=CARTESIAN_POINT ( 'NONE',  ( 18.62759615963271287, -10.81492255796078972, 73.33224293864769550 ) ) ;
#30931=CARTESIAN_POINT ( 'NONE',  ( 4.379528057220339221, -16.55341960407611168, 82.70724293864770971 ) ) ;
#30932=CARTESIAN_POINT ( 'NONE',  ( -19.05341960407617563, 5.049401038297882671, 28.54275706135232937 ) ) ;
#30933=CARTESIAN_POINT ( 'NONE',  ( -5.719274019375978568, 21.55341960407610458, 55.20724293864770260 ) ) ;
#30935=CARTESIAN_POINT ( 'NONE',  ( -5.719274019375978568, 21.55341960407610458, 35.20724293864768839 ) ) ;
#30936=CARTESIAN_POINT ( 'NONE',  ( -5.719274019375665041, -21.55341960407619695, 89.79275706135236135 ) ) ;
#30937=CARTESIAN_POINT ( 'NONE',  ( 5.153800228976335163, 19.02544592524342804, 69.79057627198103830 ) ) ;
#30938=CARTESIAN_POINT ( 'NONE',  ( 14.34966873604960469, 8.224510206698951720, 109.1655762719810383 ) ) ;
#30939=CARTESIAN_POINT ( 'NONE',  ( -0.05219959533937732626, 21.53943276465977519, 22.50109039468567573 ) ) ;
#30941=CARTESIAN_POINT ( 'NONE',  ( -0.05219959533937732626, 21.53943276465977519, 42.50109039468567573 ) ) ;
#30942=CARTESIAN_POINT ( 'NONE',  ( -9.564922557960796823, -16.46253265017161027, 32.08224293864769550 ) ) ;
#30943=CARTESIAN_POINT ( 'NONE',  ( -0.05219959533907301413, -21.53943276465977519, 107.4989096053143669 ) ) ;
#30944=CARTESIAN_POINT ( 'NONE',  ( -16.46253265017146816, -9.564922557961047289, 54.16775706135234003 ) ) ;
#30945=CARTESIAN_POINT ( 'NONE',  ( 13.97604488694527802, 13.89961937509977652, 29.37390960531435979 ) ) ;
#30946=CARTESIAN_POINT ( 'NONE',  ( -0.05219959533909027116, -19.03943276465977164, 27.49890960531435624 ) ) ;
#30947=CARTESIAN_POINT ( 'NONE',  ( 16.52544592524335698, 4.483927247898782831, 56.45942372801902565 ) ) ;
#30948=CARTESIAN_POINT ( 'NONE',  ( 16.51473224551069308, 9.474510206698969483, 29.16557627198103475 ) ) ;
#30950=CARTESIAN_POINT ( 'NONE',  ( -19.03943276465977164, 0.05219959533909376836, 71.24890960531435269 ) ) ;
#30951=CARTESIAN_POINT ( 'NONE',  ( -16.55341960407611168, -4.379528057220339221, 111.4572429386476813 ) ) ;
#30952=CARTESIAN_POINT ( 'NONE',  ( 10.81492255796078972, 18.62759615963270932, 64.58224293864769550 ) ) ;
#30953=CARTESIAN_POINT ( 'NONE',  ( -16.53943276465976808, -0.05219959533934237506, 38.75109039468567573 ) ) ;
#30954=CARTESIAN_POINT ( 'NONE',  ( 10.72451020669871369, 18.67979575497193778, 102.0844237280190185 ) ) ;
#30955=CARTESIAN_POINT ( 'NONE',  ( -9.564922557960796823, -16.46253265017161027, 22.08224293864768839 ) ) ;
#30956=CARTESIAN_POINT ( 'NONE',  ( -16.53943276465976808, -0.05219959533934237506, 108.7510903946857042 ) ) ;
#30957=CARTESIAN_POINT ( 'NONE',  ( 8.314922557960818139, 14.29746914071049879, 49.58224293864769550 ) ) ;
#30958=CARTESIAN_POINT ( 'NONE',  ( -19.03943276465977164, 0.05219959533909376836, 46.24890960531435979 ) ) ;
#30959=CARTESIAN_POINT ( 'NONE',  ( 0.05219959533937995610, -21.53943276465977519, 100.0010903946857042 ) ) ;
#30960=CARTESIAN_POINT ( 'NONE',  ( -0.05219959533907301413, -21.53943276465977519, 107.4989096053143669 ) ) ;
#30961=CARTESIAN_POINT ( 'NONE',  ( -18.67979575497193778, 10.72451020669871902, 68.33442372801900433 ) ) ;
#30962=CARTESIAN_POINT ( 'NONE',  ( -14.34966873604972548, 8.224510206698743886, 48.33442372801902565 ) ) ;
#30963=CARTESIAN_POINT ( 'NONE',  ( 0.05219959533910956823, 16.53943276465976808, 74.99890960531435269 ) ) ;
#30964=CARTESIAN_POINT ( 'NONE',  ( 5.823673210054444382, -21.52544592524334988, 100.2094237280190043 ) ) ;
#30965=CARTESIAN_POINT ( 'NONE',  ( 16.55341960407611168, 4.379528057220329451, 23.95724293864769550 ) ) ;
#30967=CARTESIAN_POINT ( 'NONE',  ( -16.53943276465976808, -0.05219959533934237506, 33.75109039468568284 ) ) ;
#30968=CARTESIAN_POINT ( 'NONE',  ( 16.53943276465976808, -0.05219959533910856209, 43.74890960531435979 ) ) ;
#30969=CARTESIAN_POINT ( 'NONE',  ( 16.52544592524335698, 4.483927247898782831, 86.45942372801901854 ) ) ;
#30970=CARTESIAN_POINT ( 'NONE',  ( 13.89961937509977652, -13.97604488694527269, 103.1239096053143527 ) ) ;
#30971=CARTESIAN_POINT ( 'NONE',  ( 18.62759615963271287, -10.81492255796078972, 23.33224293864769194 ) ) ;
#30972=CARTESIAN_POINT ( 'NONE',  ( 5.823673210054444382, -21.52544592524334988, 95.20942372801903275 ) ) ;
#30973=CARTESIAN_POINT ( 'NONE',  ( 14.29746914071037800, 8.314922557961029526, 96.66775706135234714 ) ) ;
#30974=CARTESIAN_POINT ( 'NONE',  ( -4.483927247898539470, -16.52544592524342804, 77.29057627198102409 ) ) ;
#30975=CARTESIAN_POINT ( 'NONE',  ( 16.46253265017160672, -9.564922557960803928, 78.33224293864769550 ) ) ;
#30977=CARTESIAN_POINT ( 'NONE',  ( 12.06949235617739724, 12.14591786802326823, 26.87609039468567218 ) ) ;
#30978=CARTESIAN_POINT ( 'NONE',  ( 9.474510206698971260, -16.51473224551069308, 47.91557627198102409 ) ) ;
#30979=CARTESIAN_POINT ( 'NONE',  ( -16.46253265017160317, 9.564922557960807481, 90.83224293864769550 ) ) ;
#30980=CARTESIAN_POINT ( 'NONE',  ( 8.314922557961029526, -14.29746914071037800, 30.41775706135234358 ) ) ;
#30981=CARTESIAN_POINT ( 'NONE',  ( -19.05341960407617563, 5.049401038297882671, 38.54275706135233293 ) ) ;
#30982=CARTESIAN_POINT ( 'NONE',  ( -8.224510206698735004, -14.34966873604973081, 89.58442372801901854 ) ) ;
#30983=CARTESIAN_POINT ( 'NONE',  ( -5.049401038298153566, 19.05341960407611168, 35.20724293864768839 ) ) ;
#30984=CARTESIAN_POINT ( 'NONE',  ( -16.55341960407617563, 4.379528057220093196, 83.54275706135234714 ) ) ;
#30985=CARTESIAN_POINT ( 'NONE',  ( 4.379528057220092307, 16.55341960407617563, 62.29275706135236845 ) ) ;
#30986=CARTESIAN_POINT ( 'NONE',  ( -19.03943276465977164, -0.05219959533935918106, 78.75109039468567573 ) ) ;
#30987=CARTESIAN_POINT ( 'NONE',  ( 5.049401038297881783, 19.05341960407617563, 22.29275706135233648 ) ) ;
#30988=CARTESIAN_POINT ( 'NONE',  ( -13.89961937509977652, 13.97604488694528158, 50.62390960531435979 ) ) ;
#30989=CARTESIAN_POINT ( 'NONE',  ( 12.06949235617757843, -12.14591786802309237, 88.12390960531436690 ) ) ;
#30990=CARTESIAN_POINT ( 'NONE',  ( -5.153800228976607833, 19.02544592524334988, 52.70942372801900433 ) ) ;
#30991=CARTESIAN_POINT ( 'NONE',  ( 0.05219959533907565091, 21.53943276465977519, 54.99890960531435269 ) ) ;
#30992=CARTESIAN_POINT ( 'NONE',  ( 19.03943276465977164, 0.05219959533936151252, 31.25109039468566863 ) ) ;
#30993=CARTESIAN_POINT ( 'NONE',  ( -19.03943276465977164, 0.05219959533909376836, 106.2489096053143669 ) ) ;
#30994=CARTESIAN_POINT ( 'NONE',  ( -10.81492255796078084, -18.62759615963271287, 82.08224293864768129 ) ) ;
#30995=CARTESIAN_POINT ( 'NONE',  ( -13.89961937509977652, 13.97604488694528158, 110.6239096053143243 ) ) ;
#30996=CARTESIAN_POINT ( 'NONE',  ( 19.02544592524334988, 5.153800228976608722, 91.45942372801900433 ) ) ;
#30997=CARTESIAN_POINT ( 'NONE',  ( -19.03943276465977164, 0.05219959533909376836, 111.2489096053143669 ) ) ;
#30998=CARTESIAN_POINT ( 'NONE',  ( 14.34966873604972726, -8.224510206698740333, 20.83442372801901143 ) ) ;
#30999=CARTESIAN_POINT ( 'NONE',  ( -5.153800228976328057, -19.02544592524343514, 37.29057627198102409 ) ) ;
#31000=CARTESIAN_POINT ( 'NONE',  ( 16.51473224551069308, 9.474510206698969483, 94.16557627198103830 ) ) ;
#31001=CARTESIAN_POINT ( 'NONE',  ( 15.72974639402199770, -15.80617190586745480, 83.12390960531436690 ) ) ;
#31002=CARTESIAN_POINT ( 'NONE',  ( 16.53943276465976808, 0.05219959533934440121, 51.25109039468568994 ) ) ;
#31003=CARTESIAN_POINT ( 'NONE',  ( -5.823673210054431948, 21.52544592524334988, 57.70942372801901143 ) ) ;
#31004=CARTESIAN_POINT ( 'NONE',  ( -5.153800228976607833, 19.02544592524334988, 112.7094237280190043 ) ) ;
#31005=CARTESIAN_POINT ( 'NONE',  ( -0.05219959533937732626, 21.53943276465977519, 112.5010903946857042 ) ) ;
#31006=CARTESIAN_POINT ( 'NONE',  ( 14.29746914071037800, 8.314922557961029526, 106.6677570613523756 ) ) ;
#31007=CARTESIAN_POINT ( 'NONE',  ( 19.05341960407611168, 5.049401038298154454, 103.9572429386476671 ) ) ;
#31008=CARTESIAN_POINT ( 'NONE',  ( 18.67979575497178502, 10.72451020669898547, 99.16557627198100988 ) ) ;
#31009=CARTESIAN_POINT ( 'NONE',  ( -8.314922557960811034, -14.29746914071050412, 32.08224293864769550 ) ) ;
#31010=CARTESIAN_POINT ( 'NONE',  ( 16.46253265017146816, 9.564922557961045513, 76.66775706135234714 ) ) ;
#31011=CARTESIAN_POINT ( 'NONE',  ( 15.72974639402176855, 15.80617190586768217, 61.87609039468568284 ) ) ;
#31012=CARTESIAN_POINT ( 'NONE',  ( 5.049401038297881783, 19.05341960407617563, 32.29275706135233293 ) ) ;
#31013=CARTESIAN_POINT ( 'NONE',  ( -14.29746914071049879, 8.314922557960819915, 105.8322429386476955 ) ) ;
#31014=CARTESIAN_POINT ( 'NONE',  ( 21.52544592524344225, -5.823673210054117533, 28.54057627198103120 ) ) ;
#31015=CARTESIAN_POINT ( 'NONE',  ( -14.34966873604960291, -8.224510206698953496, 31.66557627198102054 ) ) ;
#31016=CARTESIAN_POINT ( 'NONE',  ( -0.05219959533937732626, 21.53943276465977519, 102.5010903946856899 ) ) ;
#31017=CARTESIAN_POINT ( 'NONE',  ( -16.53943276465976808, -0.05219959533934237506, 58.75109039468568994 ) ) ;
#31018=CARTESIAN_POINT ( 'NONE',  ( -12.14591786802326823, 12.06949235617739902, 113.1260903946856899 ) ) ;
#31019=CARTESIAN_POINT ( 'NONE',  ( -18.62759615963255300, -10.81492255796106328, 64.16775706135234714 ) ) ;
#31020=CARTESIAN_POINT ( 'NONE',  ( -10.72451020669870658, -18.67979575497194134, 54.58442372801901143 ) ) ;
#31022=CARTESIAN_POINT ( 'NONE',  ( -0.05219959533909027116, -19.03943276465977164, 62.49890960531435979 ) ) ;
#31023=CARTESIAN_POINT ( 'NONE',  ( -21.52544592524334988, -5.823673210054445271, 33.95942372801901143 ) ) ;
#31024=CARTESIAN_POINT ( 'NONE',  ( 4.379528057220339221, -16.55341960407611168, 107.7072429386476955 ) ) ;
#31025=CARTESIAN_POINT ( 'NONE',  ( -19.03943276465977164, 0.05219959533909376836, 31.24890960531435979 ) ) ;
#31026=CARTESIAN_POINT ( 'NONE',  ( -8.224510206698948167, 14.34966873604960824, 75.41557627198102409 ) ) ;
#31027=CARTESIAN_POINT ( 'NONE',  ( 9.474510206698971260, -16.51473224551069308, 72.91557627198102409 ) ) ;
#31028=CARTESIAN_POINT ( 'NONE',  ( -16.53943276465976808, 0.05219959533911058130, 31.24890960531435979 ) ) ;
#31029=CARTESIAN_POINT ( 'NONE',  ( -5.823673210054116645, -21.52544592524344225, 52.29057627198102409 ) ) ;
#31030=CARTESIAN_POINT ( 'NONE',  ( -8.314922557960811034, -14.29746914071050412, 92.08224293864769550 ) ) ;
#31032=CARTESIAN_POINT ( 'NONE',  ( 5.823673210054125526, 21.52544592524343514, 94.79057627198105251 ) ) ;
#31033=CARTESIAN_POINT ( 'NONE',  ( -9.564922557960796823, -16.46253265017161027, 102.0822429386477097 ) ) ;
#31034=CARTESIAN_POINT ( 'NONE',  ( 5.049401038298161559, -19.05341960407611168, 57.70724293864769550 ) ) ;
#31035=CARTESIAN_POINT ( 'NONE',  ( -9.474510206698720793, -16.51473224551083518, 104.5844237280190043 ) ) ;
#31036=CARTESIAN_POINT ( 'NONE',  ( 5.823673210054125526, 21.52544592524343514, 59.79057627198103120 ) ) ;
#31037=CARTESIAN_POINT ( 'NONE',  ( 10.81492255796106328, -18.62759615963255655, 80.41775706135234714 ) ) ;
#31038=CARTESIAN_POINT ( 'NONE',  ( -19.02544592524342804, 5.153800228976336051, 71.04057627198099567 ) ) ;
#31039=CARTESIAN_POINT ( 'NONE',  ( 19.02544592524343514, -5.153800228976328945, 98.54057627198100988 ) ) ;
#31040=CARTESIAN_POINT ( 'NONE',  ( 14.29746914071037800, 8.314922557961029526, 76.66775706135234714 ) ) ;
#31041=CARTESIAN_POINT ( 'NONE',  ( 21.55341960407619695, -5.719274019375665929, 56.04275706135235424 ) ) ;
#31042=CARTESIAN_POINT ( 'NONE',  ( 21.55341960407619695, -5.719274019375665929, 81.04275706135236135 ) ) ;
#31043=CARTESIAN_POINT ( 'NONE',  ( -15.80617190586745835, -15.72974639402198527, 111.8739096053143669 ) ) ;
#31044=CARTESIAN_POINT ( 'NONE',  ( 12.06949235617739724, 12.14591786802326823, 81.87609039468568994 ) ) ;
#31045=CARTESIAN_POINT ( 'NONE',  ( 18.67979575497178502, 10.72451020669898547, 74.16557627198102409 ) ) ;
#31046=CARTESIAN_POINT ( 'NONE',  ( 9.564922557961047289, -16.46253265017146816, 40.41775706135234003 ) ) ;
#31047=CARTESIAN_POINT ( 'NONE',  ( -15.72974639402197994, 15.80617190586746368, 40.62390960531435269 ) ) ;
#31048=CARTESIAN_POINT ( 'NONE',  ( -9.564922557960796823, -16.46253265017161027, 82.08224293864768129 ) ) ;
#31049=CARTESIAN_POINT ( 'NONE',  ( 4.379528057220092307, 16.55341960407617563, 112.2927570613523471 ) ) ;
#31050=CARTESIAN_POINT ( 'NONE',  ( -17.31747979337949772, 6.344076630960997498, 63.62055131934819485 ) ) ;
#31051=CARTESIAN_POINT ( 'NONE',  ( -16.46253265017160317, 9.564922557960807481, 115.8322429386477097 ) ) ;
#31054=CARTESIAN_POINT ( 'NONE',  ( 0.05219959533936267826, -19.03943276465977164, 95.00109039468567573 ) ) ;
#31055=CARTESIAN_POINT ( 'NONE',  ( -0.05219959533907301413, -21.53943276465977519, 72.49890960531435269 ) ) ;
#31056=CARTESIAN_POINT ( 'NONE',  ( -8.314922557960811034, -14.29746914071050412, 47.08224293864770260 ) ) ;
#31057=CARTESIAN_POINT ( 'NONE',  ( 16.52544592524335698, 4.483927247898782831, 21.45942372801901499 ) ) ;
#31058=CARTESIAN_POINT ( 'NONE',  ( -13.89961937509977652, 13.97604488694528158, 25.62390960531434558 ) ) ;
#31059=CARTESIAN_POINT ( 'NONE',  ( -5.049401038297874678, -19.05341960407617918, 104.7927570613523471 ) ) ;
#31060=CARTESIAN_POINT ( 'NONE',  ( 5.719274019375991003, -21.55341960407610458, 102.7072429386476955 ) ) ;
#31061=CARTESIAN_POINT ( 'NONE',  ( 13.89961937509957401, 13.97604488694547697, 76.87609039468566152 ) ) ;
#31062=CARTESIAN_POINT ( 'NONE',  ( 14.34966873604972726, -8.224510206698740333, 80.83442372801901854 ) ) ;
#31063=CARTESIAN_POINT ( 'NONE',  ( 16.51473224551069308, 9.474510206698969483, 79.16557627198103830 ) ) ;
#31064=CARTESIAN_POINT ( 'NONE',  ( -4.483927247898539470, -16.52544592524342804, 72.29057627198102409 ) ) ;
#31065=CARTESIAN_POINT ( 'NONE',  ( 19.02544592524343514, -5.153800228976328945, 58.54057627198102409 ) ) ;
#31066=CARTESIAN_POINT ( 'NONE',  ( -4.379528057220328563, 16.55341960407611168, 70.20724293864769550 ) ) ;
#31067=CARTESIAN_POINT ( 'NONE',  ( 13.97604488694527802, 13.89961937509977652, 39.37390960531435269 ) ) ;
#31069=CARTESIAN_POINT ( 'NONE',  ( 16.52544592524342804, -4.483927247898539470, 38.54057627198103120 ) ) ;
#31070=CARTESIAN_POINT ( 'NONE',  ( 5.153800228976335163, 19.02544592524342804, 74.79057627198103830 ) ) ;
#31072=CARTESIAN_POINT ( 'NONE',  ( -9.564922557961040184, 16.46253265017147172, 52.91775706135233293 ) ) ;
#31073=CARTESIAN_POINT ( 'NONE',  ( -0.05219959533934338120, 16.53943276465976808, 62.50109039468568284 ) ) ;
#31075=CARTESIAN_POINT ( 'NONE',  ( -21.52544592524343514, 5.823673210054127303, 61.04057627198103120 ) ) ;
#31076=CARTESIAN_POINT ( 'NONE',  ( -5.049401038297874678, -19.05341960407617918, 29.79275706135232227 ) ) ;
#31077=CARTESIAN_POINT ( 'NONE',  ( -9.474510206698964154, 16.51473224551069663, 85.41557627198102409 ) ) ;
#31079=CARTESIAN_POINT ( 'NONE',  ( 10.72451020669898902, -18.67979575497178502, 27.91557627198103830 ) ) ;
#31080=CARTESIAN_POINT ( 'NONE',  ( -19.02544592524342804, 5.153800228976336051, 66.04057627198103830 ) ) ;
#31081=CARTESIAN_POINT ( 'NONE',  ( 10.72451020669871369, 18.67979575497193778, 52.08442372801901854 ) ) ;
#31082=CARTESIAN_POINT ( 'NONE',  ( 4.483927247898545687, 16.52544592524342804, 109.7905762719810383 ) ) ;
#31083=CARTESIAN_POINT ( 'NONE',  ( -21.52544592524343514, 5.823673210054127303, 101.0405762719810383 ) ) ;
#31084=CARTESIAN_POINT ( 'NONE',  ( -5.049401038298153566, 19.05341960407611168, 95.20724293864770971 ) ) ;
#31086=CARTESIAN_POINT ( 'NONE',  ( 18.67979575497194134, -10.72451020669871369, 45.83442372801901854 ) ) ;
#31088=CARTESIAN_POINT ( 'NONE',  ( -13.97604488694527625, -13.89961937509977652, 101.8739096053143811 ) ) ;
#31089=CARTESIAN_POINT ( 'NONE',  ( 17.59860650958989936, 7.585241751807028088, 89.07662985737509587 ) ) ;
#31090=CARTESIAN_POINT ( 'NONE',  ( 15.80617190586746368, 15.72974639402197994, 94.37390960531436690 ) ) ;
#31091=CARTESIAN_POINT ( 'NONE',  ( -9.564922557960796823, -16.46253265017161027, 52.08224293864768839 ) ) ;
#31092=CARTESIAN_POINT ( 'NONE',  ( -12.14591786802326823, 12.06949235617739902, 23.12609039468567573 ) ) ;
#31094=CARTESIAN_POINT ( 'NONE',  ( 0.05219959533909260263, 19.03943276465977164, 34.99890960531435979 ) ) ;
#31095=CARTESIAN_POINT ( 'NONE',  ( 5.719274019375673035, 21.55341960407619339, 102.2927570613523613 ) ) ;
#31096=CARTESIAN_POINT ( 'NONE',  ( 19.02544592524343514, -5.153800228976328945, 78.54057627198099567 ) ) ;
#31097=CARTESIAN_POINT ( 'NONE',  ( 15.80617190586769283, -15.72974639402175789, 45.62609039468567573 ) ) ;
#31098=CARTESIAN_POINT ( 'NONE',  ( 10.81492255796106328, -18.62759615963255655, 25.41775706135235779 ) ) ;
#31100=CARTESIAN_POINT ( 'NONE',  ( -16.51473224551069308, -9.474510206698971260, 96.66557627198102409 ) ) ;
#31102=CARTESIAN_POINT ( 'NONE',  ( -0.05219959533934338120, 16.53943276465976808, 37.50109039468568284 ) ) ;
#31103=CARTESIAN_POINT ( 'NONE',  ( -16.52544592524335698, -4.483927247898792601, 73.95942372801901854 ) ) ;
#31104=CARTESIAN_POINT ( 'NONE',  ( 18.67979575497194134, -10.72451020669871369, 60.83442372801901854 ) ) ;
#31105=CARTESIAN_POINT ( 'NONE',  ( 15.72974639402176855, 15.80617190586768217, 81.87609039468568994 ) ) ;
#31106=DIRECTION ( 'NONE',  ( 0.000000000000000000, 0.000000000000000000, -1.000000000000000000 ) ) ;
#31107=CARTESIAN_POINT ( 'NONE',  ( -5.153800228976607833, 19.02544592524334988, 112.7094237280190043 ) ) ;
#31108=CARTESIAN_POINT ( 'NONE',  ( -9.564922557960796823, -16.46253265017161027, 77.08224293864769550 ) ) ;
#31109=CARTESIAN_POINT ( 'NONE',  ( -16.51473224551069308, -9.474510206698971260, 101.6655762719810241 ) ) ;
#31110=CARTESIAN_POINT ( 'NONE',  ( 16.55341960407611168, 4.379528057220329451, 103.9572429386476813 ) ) ;
#31111=CARTESIAN_POINT ( 'NONE',  ( 16.52544592524342804, -4.483927247898539470, 108.5405762719810241 ) ) ;
#31112=CARTESIAN_POINT ( 'NONE',  ( 5.719274019375991003, -21.55341960407610458, 27.70724293864769905 ) ) ;
#31113=CARTESIAN_POINT ( 'NONE',  ( 4.483927247898790824, -16.52544592524335698, 80.20942372801901854 ) ) ;
#31114=CARTESIAN_POINT ( 'NONE',  ( 16.53943276465976808, -0.05219959533910856209, 68.74890960531435269 ) ) ;
#31115=CARTESIAN_POINT ( 'NONE',  ( -19.02544592524342804, 5.153800228976336051, 61.04057627198103120 ) ) ;
#31116=CARTESIAN_POINT ( 'NONE',  ( -21.52544592524334988, -5.823673210054445271, 78.95942372801901854 ) ) ;
#31118=CARTESIAN_POINT ( 'NONE',  ( 9.474510206698729675, 16.51473224551082808, 112.0844237280190043 ) ) ;
#31119=CARTESIAN_POINT ( 'NONE',  ( 14.29746914071049879, -8.314922557960816363, 73.33224293864769550 ) ) ;
#31120=CARTESIAN_POINT ( 'NONE',  ( 5.823673210054444382, -21.52544592524334988, 25.20942372801901854 ) ) ;
#31121=CARTESIAN_POINT ( 'NONE',  ( 18.67979575497178502, 10.72451020669898547, 64.16557627198102409 ) ) ;
#31124=CARTESIAN_POINT ( 'NONE',  ( -16.46253265017160317, 9.564922557960807481, 75.83224293864769550 ) ) ;
#31125=CARTESIAN_POINT ( 'NONE',  ( -14.34966873604960291, -8.224510206698953496, 46.66557627198102409 ) ) ;
#31126=CARTESIAN_POINT ( 'NONE',  ( -14.34966873604960291, -8.224510206698953496, 26.66557627198103475 ) ) ;
#31127=CARTESIAN_POINT ( 'NONE',  ( 16.52544592524335698, 4.483927247898782831, 91.45942372801901854 ) ) ;
#31128=CARTESIAN_POINT ( 'NONE',  ( -13.97604488694547697, 13.89961937509957934, 58.12609039468566863 ) ) ;
#31129=CARTESIAN_POINT ( 'NONE',  ( 17.50000000000001421, 5.622605283950889543, 48.81207310596114013 ) ) ;
#31130=CARTESIAN_POINT ( 'NONE',  ( -19.02544592524342804, 5.153800228976336051, 111.0405762719810099 ) ) ;
#31131=EDGE_CURVE ( 'NONE', #59793, #74699, #44625, .T. ) ;
#31132=CARTESIAN_POINT ( 'NONE',  ( -14.34966873604960291, -8.224510206698953496, 71.66557627198100988 ) ) ;
#31133=CARTESIAN_POINT ( 'NONE',  ( -9.474510206698720793, -16.51473224551083518, 44.58442372801900433 ) ) ;
#31134=CARTESIAN_POINT ( 'NONE',  ( -5.049401038298153566, 19.05341960407611168, 30.20724293864768839 ) ) ;
#31135=CARTESIAN_POINT ( 'NONE',  ( -5.823673210054116645, -21.52544592524344225, 37.29057627198102409 ) ) ;
#31136=CARTESIAN_POINT ( 'NONE',  ( 21.52544592524344225, -5.823673210054117533, 48.54057627198103120 ) ) ;
#31138=CARTESIAN_POINT ( 'NONE',  ( -4.379528057220328563, 16.55341960407611168, 105.2072429386477097 ) ) ;
#31139=CARTESIAN_POINT ( 'NONE',  ( 14.29746914071037800, 8.314922557961029526, 46.66775706135234714 ) ) ;
#31140=CARTESIAN_POINT ( 'NONE',  ( -12.06949235617756955, 12.14591786802309770, 95.62390960531436690 ) ) ;
#31141=CARTESIAN_POINT ( 'NONE',  ( 16.21995358207306026, -7.366697692864082825, 37.43551001512158649 ) ) ;
#31143=CARTESIAN_POINT ( 'NONE',  ( -21.55341960407610458, -5.719274019375992779, 36.45724293864768839 ) ) ;
#31144=CARTESIAN_POINT ( 'NONE',  ( 18.22780087662123805, -5.499999999999976019, 78.51763182126894947 ) ) ;
#31146=CARTESIAN_POINT ( 'NONE',  ( 14.29746914071037800, 8.314922557961029526, 36.66775706135234714 ) ) ;
#31147=CARTESIAN_POINT ( 'NONE',  ( 16.55341960407611168, 4.379528057220329451, 28.95724293864769905 ) ) ;
#31148=CARTESIAN_POINT ( 'NONE',  ( -21.55341960407610458, -5.719274019375992779, 56.45724293864768839 ) ) ;
#31149=CARTESIAN_POINT ( 'NONE',  ( -19.03943276465977164, -0.05219959533935918106, 78.75109039468567573 ) ) ;
#31150=CARTESIAN_POINT ( 'NONE',  ( 21.52544592524344225, -5.823673210054117533, 68.54057627198103830 ) ) ;
#31151=CARTESIAN_POINT ( 'NONE',  ( 21.55341960407619695, -5.719274019375665929, 81.04275706135236135 ) ) ;
#31153=CARTESIAN_POINT ( 'NONE',  ( -8.314922557961024197, 14.29746914071037800, 42.91775706135235424 ) ) ;
#31154=CARTESIAN_POINT ( 'NONE',  ( 16.51473224551069308, 9.474510206698969483, 34.16557627198102409 ) ) ;
#31155=CARTESIAN_POINT ( 'NONE',  ( -9.564922557960796823, -16.46253265017161027, 102.0822429386477097 ) ) ;
#31156=CARTESIAN_POINT ( 'NONE',  ( -9.564922557960796823, -16.46253265017161027, 32.08224293864769550 ) ) ;
#31157=CARTESIAN_POINT ( 'NONE',  ( 14.29746914071049879, -8.314922557960816363, 103.3322429386476955 ) ) ;
#31158=CARTESIAN_POINT ( 'NONE',  ( -16.46253265017160317, 9.564922557960807481, 110.8322429386476955 ) ) ;
#31160=CARTESIAN_POINT ( 'NONE',  ( 16.52544592524335698, 4.483927247898782831, 71.45942372801901854 ) ) ;
#31161=CARTESIAN_POINT ( 'NONE',  ( -15.72974639402197994, 15.80617190586746368, 85.62390960531436690 ) ) ;
#31162=CARTESIAN_POINT ( 'NONE',  ( 5.153800228976335163, 19.02544592524342804, 54.79057627198103120 ) ) ;
#31163=CARTESIAN_POINT ( 'NONE',  ( -21.55341960407619339, 5.719274019375674811, 23.54275706135235424 ) ) ;
#31164=CARTESIAN_POINT ( 'NONE',  ( 9.564922557960805705, 16.46253265017160317, 84.58224293864769550 ) ) ;
#31167=CARTESIAN_POINT ( 'NONE',  ( -5.719274019375978568, 21.55341960407610458, 115.2072429386476955 ) ) ;
#31168=CARTESIAN_POINT ( 'NONE',  ( -16.51473224551069308, -9.474510206698971260, 31.66557627198102054 ) ) ;
#31169=CARTESIAN_POINT ( 'NONE',  ( 19.03943276465977164, -0.05219959533909143690, 108.7489096053143527 ) ) ;
#31170=CARTESIAN_POINT ( 'NONE',  ( -13.97604488694547697, 13.89961937509957934, 73.12609039468568994 ) ) ;
#31171=CARTESIAN_POINT ( 'NONE',  ( -9.474510206698720793, -16.51473224551083518, 24.58442372801900078 ) ) ;
#31172=CARTESIAN_POINT ( 'NONE',  ( -21.55341960407610458, -5.719274019375992779, 96.45724293864770971 ) ) ;
#31173=CARTESIAN_POINT ( 'NONE',  ( 19.02544592524334988, 5.153800228976608722, 36.45942372801900433 ) ) ;
#31174=CARTESIAN_POINT ( 'NONE',  ( -16.55341960407617563, 4.379528057220093196, 83.54275706135234714 ) ) ;
#31175=CARTESIAN_POINT ( 'NONE',  ( -5.049401038298153566, 19.05341960407611168, 110.2072429386476671 ) ) ;
#31176=CARTESIAN_POINT ( 'NONE',  ( -9.474510206698964154, 16.51473224551069663, 65.41557627198102409 ) ) ;
#31177=CARTESIAN_POINT ( 'NONE',  ( 5.823673210054444382, -21.52544592524334988, 60.20942372801902565 ) ) ;
#31178=CARTESIAN_POINT ( 'NONE',  ( -5.823673210054431948, 21.52544592524334988, 77.70942372801900433 ) ) ;
#31179=CARTESIAN_POINT ( 'NONE',  ( 13.97604488694527802, 13.89961937509977652, 69.37390960531436690 ) ) ;
#31180=CARTESIAN_POINT ( 'NONE',  ( -5.823673210054431948, 21.52544592524334988, 42.70942372801901854 ) ) ;
#31181=CARTESIAN_POINT ( 'NONE',  ( 0.05219959533936267826, -19.03943276465977164, 85.00109039468567573 ) ) ;
#31182=CARTESIAN_POINT ( 'NONE',  ( 19.02544592524343514, -5.153800228976328945, 48.54057627198103120 ) ) ;
#31183=CARTESIAN_POINT ( 'NONE',  ( 5.049401038298161559, -19.05341960407611168, 92.70724293864769550 ) ) ;
#31184=CARTESIAN_POINT ( 'NONE',  ( 9.564922557960805705, 16.46253265017160317, 69.58224293864770971 ) ) ;
#31185=CARTESIAN_POINT ( 'NONE',  ( 9.564922557960805705, 16.46253265017160317, 54.58224293864769550 ) ) ;
#31186=CARTESIAN_POINT ( 'NONE',  ( 18.67979575497178502, 10.72451020669898547, 104.1655762719810241 ) ) ;
#31187=CARTESIAN_POINT ( 'NONE',  ( -8.314922557961024197, 14.29746914071037800, 87.91775706135234714 ) ) ;
#31189=CARTESIAN_POINT ( 'NONE',  ( -16.46253265017146816, -9.564922557961047289, 39.16775706135234003 ) ) ;
#31190=CARTESIAN_POINT ( 'NONE',  ( 16.46253265017160672, -9.564922557960803928, 63.33224293864769550 ) ) ;
#31191=CARTESIAN_POINT ( 'NONE',  ( 14.29746914071049879, -8.314922557960816363, 53.33224293864769550 ) ) ;
#31192=CARTESIAN_POINT ( 'NONE',  ( -4.483927247898539470, -16.52544592524342804, 97.29057627198105251 ) ) ;
#31193=CARTESIAN_POINT ( 'NONE',  ( -13.89961937509977652, 13.97604488694528158, 110.6239096053143243 ) ) ;
#31195=CARTESIAN_POINT ( 'NONE',  ( 19.03943276465977164, -0.05219959533909143690, 88.74890960531436690 ) ) ;
#31196=CARTESIAN_POINT ( 'NONE',  ( -9.474510206698964154, 16.51473224551069663, 100.4155762719810241 ) ) ;
#31197=CARTESIAN_POINT ( 'NONE',  ( 19.05341960407617918, -5.049401038297876454, 21.04275706135232582 ) ) ;
#31198=CARTESIAN_POINT ( 'NONE',  ( 4.379528057220092307, 16.55341960407617563, 97.29275706135234714 ) ) ;
#31199=CARTESIAN_POINT ( 'NONE',  ( -9.564922557960796823, -16.46253265017161027, 77.08224293864769550 ) ) ;
#31200=CARTESIAN_POINT ( 'NONE',  ( 21.52544592524334988, 5.823673210054432836, 41.45942372801901143 ) ) ;
#31201=CARTESIAN_POINT ( 'NONE',  ( -15.72974639402197994, 15.80617190586746368, 25.62390960531435624 ) ) ;
#31202=CARTESIAN_POINT ( 'NONE',  ( -18.62759615963270932, 10.81492255796079327, 115.8322429386477097 ) ) ;
#31203=CARTESIAN_POINT ( 'NONE',  ( 8.224510206698953496, -14.34966873604960469, 62.91557627198102409 ) ) ;
#31204=CARTESIAN_POINT ( 'NONE',  ( 13.97604488694527802, 13.89961937509977652, 59.37390960531434558 ) ) ;
#31205=CARTESIAN_POINT ( 'NONE',  ( 14.34966873604960469, 8.224510206698951720, 84.16557627198103830 ) ) ;
#31206=CARTESIAN_POINT ( 'NONE',  ( 9.564922557961047289, -16.46253265017146816, 45.41775706135232582 ) ) ;
#31207=CARTESIAN_POINT ( 'NONE',  ( 12.06949235617757843, -12.14591786802309237, 113.1239096053143953 ) ) ;
#31208=CARTESIAN_POINT ( 'NONE',  ( 16.51473224551069308, 9.474510206698969483, 84.16557627198102409 ) ) ;
#31209=CARTESIAN_POINT ( 'NONE',  ( -19.03943276465977164, 0.05219959533909376836, 86.24890960531436690 ) ) ;
#31211=CARTESIAN_POINT ( 'NONE',  ( -16.55341960407611168, -4.379528057220339221, 101.4572429386476955 ) ) ;
#31213=CARTESIAN_POINT ( 'NONE',  ( 16.52544592524335698, 4.483927247898782831, 101.4594237280190185 ) ) ;
#31214=CARTESIAN_POINT ( 'NONE',  ( 8.314922557961029526, -14.29746914071037800, 30.41775706135234358 ) ) ;
#31215=CARTESIAN_POINT ( 'NONE',  ( 21.55341960407619695, -5.719274019375665929, 96.04275706135236135 ) ) ;
#31216=CARTESIAN_POINT ( 'NONE',  ( 5.153800228976335163, 19.02544592524342804, 84.79057627198099567 ) ) ;
#31217=CARTESIAN_POINT ( 'NONE',  ( 21.53943276465977519, 0.05219959533937863772, 21.25109039468567218 ) ) ;
#31218=CARTESIAN_POINT ( 'NONE',  ( 5.153800228976335163, 19.02544592524342804, 24.79057627198102765 ) ) ;
#31219=VECTOR ( 'NONE', #15448, 1000.000000000000000 ) ;
#31220=CARTESIAN_POINT ( 'NONE',  ( -12.14591786802326823, 12.06949235617739902, 33.12609039468569705 ) ) ;
#31221=CARTESIAN_POINT ( 'NONE',  ( 9.564922557961047289, -16.46253265017146816, 95.41775706135233293 ) ) ;
#31222=EDGE_CURVE ( 'NONE', #176653, #179099, #110244, .T. ) ;
#31223=CARTESIAN_POINT ( 'NONE',  ( -21.52544592524343514, 5.823673210054127303, 96.04057627198102409 ) ) ;
#31224=CARTESIAN_POINT ( 'NONE',  ( -5.049401038297874678, -19.05341960407617918, 64.79275706135233293 ) ) ;
#31225=CARTESIAN_POINT ( 'NONE',  ( -19.03943276465977164, 0.05219959533909376836, 21.24890960531436335 ) ) ;
#31226=CARTESIAN_POINT ( 'NONE',  ( 0.05219959533937995610, -21.53943276465977519, 20.00109039468568639 ) ) ;
#31228=CARTESIAN_POINT ( 'NONE',  ( 19.03943276465977164, -0.05219959533909143690, 93.74890960531435269 ) ) ;
#31229=CARTESIAN_POINT ( 'NONE',  ( 4.379528057220092307, 16.55341960407617563, 42.29275706135235424 ) ) ;
#31230=CARTESIAN_POINT ( 'NONE',  ( -17.60728821187777271, 5.499999999999950262, 100.8669092774361076 ) ) ;
#31231=CARTESIAN_POINT ( 'NONE',  ( -9.474510206698720793, -16.51473224551083518, 54.58442372801899722 ) ) ;
#31232=CARTESIAN_POINT ( 'NONE',  ( 10.81492255796106328, -18.62759615963255655, 25.41775706135235779 ) ) ;
#31233=CARTESIAN_POINT ( 'NONE',  ( -14.29746914071049879, 8.314922557960819915, 80.83224293864769550 ) ) ;
#31234=CARTESIAN_POINT ( 'NONE',  ( 9.564922557960805705, 16.46253265017160317, 84.58224293864769550 ) ) ;
#31235=CARTESIAN_POINT ( 'NONE',  ( -4.483927247898782831, 16.52544592524335698, 57.70942372801901143 ) ) ;
#31236=CARTESIAN_POINT ( 'NONE',  ( 9.474510206698729675, 16.51473224551082808, 62.08442372801899722 ) ) ;
#31237=CARTESIAN_POINT ( 'NONE',  ( 5.719274019375673035, 21.55341960407619339, 72.29275706135236135 ) ) ;
#31238=CARTESIAN_POINT ( 'NONE',  ( 12.14591786802327356, -12.06949235617739191, 30.62609039468567929 ) ) ;
#31239=CARTESIAN_POINT ( 'NONE',  ( 9.564922557960805705, 16.46253265017160317, 74.58224293864769550 ) ) ;
#31240=CARTESIAN_POINT ( 'NONE',  ( 5.049401038297881783, 19.05341960407617563, 87.29275706135234714 ) ) ;
#31241=CARTESIAN_POINT ( 'NONE',  ( 12.14591786802327356, -12.06949235617739191, 60.62609039468567573 ) ) ;
#31242=CARTESIAN_POINT ( 'NONE',  ( -18.67979575497193778, 10.72451020669871902, 103.3344237280190043 ) ) ;
#31243=CARTESIAN_POINT ( 'NONE',  ( -16.46253265017146816, -9.564922557961047289, 79.16775706135234714 ) ) ;
#31244=CARTESIAN_POINT ( 'NONE',  ( -9.564922557960796823, -16.46253265017161027, 52.08224293864768839 ) ) ;
#31245=CARTESIAN_POINT ( 'NONE',  ( 21.52544592524344225, -5.823673210054117533, 73.54057627198102409 ) ) ;
#31246=CARTESIAN_POINT ( 'NONE',  ( -16.55341960407611168, -4.379528057220339221, 71.45724293864769550 ) ) ;
#31247=CARTESIAN_POINT ( 'NONE',  ( 9.564922557961047289, -16.46253265017146816, 75.41775706135234714 ) ) ;
#31248=CARTESIAN_POINT ( 'NONE',  ( 16.52216118717208815, -7.221426719304427699, 61.42400978953011759 ) ) ;
#31249=CARTESIAN_POINT ( 'NONE',  ( 13.97604488694548053, -13.89961937509957401, 45.62609039468566863 ) ) ;
#31250=CARTESIAN_POINT ( 'NONE',  ( -16.55341960407617563, 4.379528057220093196, 108.5427570613523756 ) ) ;
#31251=CARTESIAN_POINT ( 'NONE',  ( 14.34966873604960469, 8.224510206698951720, 69.16557627198102409 ) ) ;
#31252=CARTESIAN_POINT ( 'NONE',  ( 5.719274019375673035, 21.55341960407619339, 102.2927570613523613 ) ) ;
#31254=CARTESIAN_POINT ( 'NONE',  ( 15.80617190586746368, 15.72974639402197994, 104.3739096053143669 ) ) ;
#31255=CARTESIAN_POINT ( 'NONE',  ( 0.05219959533909260263, 19.03943276465977164, 64.99890960531436690 ) ) ;
#31256=CARTESIAN_POINT ( 'NONE',  ( -5.823673210054431948, 21.52544592524334988, 82.70942372801900433 ) ) ;
#31257=CARTESIAN_POINT ( 'NONE',  ( 16.46253265017160672, -9.564922557960803928, 53.33224293864768839 ) ) ;
#31258=CARTESIAN_POINT ( 'NONE',  ( -16.46253265017160317, 9.564922557960807481, 30.83224293864769550 ) ) ;
#31259=CARTESIAN_POINT ( 'NONE',  ( -9.474510206698964154, 16.51473224551069663, 115.4155762719810241 ) ) ;
#31260=CARTESIAN_POINT ( 'NONE',  ( 16.52544592524342804, -4.483927247898539470, 73.54057627198102409 ) ) ;
#31261=CARTESIAN_POINT ( 'NONE',  ( -13.97604488694527625, -13.89961937509977652, 26.87390960531434558 ) ) ;
#31262=CARTESIAN_POINT ( 'NONE',  ( -0.05219959533910754901, -16.53943276465976808, 87.49890960531436690 ) ) ;
#31264=CARTESIAN_POINT ( 'NONE',  ( 21.53943276465977519, -0.05219959533907433946, 98.74890960531438111 ) ) ;
#31265=CARTESIAN_POINT ( 'NONE',  ( 21.52544592524334988, 5.823673210054432836, 51.45942372801901854 ) ) ;
#31267=CARTESIAN_POINT ( 'NONE',  ( -12.06949235617739369, -12.14591786802326823, 49.37609039468569705 ) ) ;
#31268=CARTESIAN_POINT ( 'NONE',  ( -5.719274019375978568, 21.55341960407610458, 95.20724293864769550 ) ) ;
#31269=CARTESIAN_POINT ( 'NONE',  ( -16.46253265017146816, -9.564922557961047289, 24.16775706135233648 ) ) ;
#31270=CARTESIAN_POINT ( 'NONE',  ( -13.89961937509977652, 13.97604488694528158, 100.6239096053143669 ) ) ;
#31271=CARTESIAN_POINT ( 'NONE',  ( 10.81492255796106328, -18.62759615963255655, 40.41775706135234714 ) ) ;
#31272=CARTESIAN_POINT ( 'NONE',  ( -21.52544592524343514, 5.823673210054127303, 46.04057627198103830 ) ) ;
#31273=CARTESIAN_POINT ( 'NONE',  ( -8.314922557961024197, 14.29746914071037800, 112.9177570613523329 ) ) ;
#31274=CARTESIAN_POINT ( 'NONE',  ( 0.05219959533937995610, -21.53943276465977519, 70.00109039468568994 ) ) ;
#31275=CARTESIAN_POINT ( 'NONE',  ( -5.719274019375665041, -21.55341960407619695, 99.79275706135234714 ) ) ;
#31276=CARTESIAN_POINT ( 'NONE',  ( 16.46253265017146816, 9.564922557961045513, 26.66775706135234003 ) ) ;
#31277=CARTESIAN_POINT ( 'NONE',  ( -0.05219959533934338120, 16.53943276465976808, 82.50109039468568994 ) ) ;
#31278=CARTESIAN_POINT ( 'NONE',  ( -15.80617190586768217, 15.72974639402176855, 53.12609039468568284 ) ) ;
#31279=CARTESIAN_POINT ( 'NONE',  ( 19.02544592524343514, -5.153800228976328945, 43.54057627198103120 ) ) ;
#31280=CARTESIAN_POINT ( 'NONE',  ( 9.564922557961047289, -16.46253265017146816, 25.41775706135234003 ) ) ;
#31281=CARTESIAN_POINT ( 'NONE',  ( 21.55341960407610458, 5.719274019375980345, 28.95724293864769905 ) ) ;
#31282=CARTESIAN_POINT ( 'NONE',  ( -5.823673210054431948, 21.52544592524334988, 22.70942372801901499 ) ) ;
#31283=CARTESIAN_POINT ( 'NONE',  ( 5.719274019375991003, -21.55341960407610458, 72.70724293864769550 ) ) ;
#31284=CARTESIAN_POINT ( 'NONE',  ( 16.55341960407618274, -4.379528057220086978, 46.04275706135234714 ) ) ;
#31286=CARTESIAN_POINT ( 'NONE',  ( 10.81492255796078972, 18.62759615963270932, 79.58224293864769550 ) ) ;
#31287=CARTESIAN_POINT ( 'NONE',  ( 8.314922557961029526, -14.29746914071037800, 60.41775706135235424 ) ) ;
#31288=CARTESIAN_POINT ( 'NONE',  ( -4.483927247898539470, -16.52544592524342804, 62.29057627198102409 ) ) ;
#31290=CARTESIAN_POINT ( 'NONE',  ( -13.89961937509957401, -13.97604488694547875, 104.3760903946856757 ) ) ;
#31291=CARTESIAN_POINT ( 'NONE',  ( 21.55341960407610458, 5.719274019375980345, 23.95724293864769550 ) ) ;
#31293=CARTESIAN_POINT ( 'NONE',  ( -12.06949235617739369, -12.14591786802326823, 44.37609039468567573 ) ) ;
#31294=CARTESIAN_POINT ( 'NONE',  ( 15.72974639402199770, -15.80617190586745480, 108.1239096053143811 ) ) ;
#31295=CARTESIAN_POINT ( 'NONE',  ( -18.62759615963270932, 10.81492255796079327, 25.83224293864769194 ) ) ;
#31296=CARTESIAN_POINT ( 'NONE',  ( 12.06949235617739724, 12.14591786802326823, 51.87609039468568284 ) ) ;
#31297=CARTESIAN_POINT ( 'NONE',  ( -5.153800228976328057, -19.02544592524343514, 67.29057627198102409 ) ) ;
#31298=CARTESIAN_POINT ( 'NONE',  ( -18.62759615963255300, -10.81492255796106328, 44.16775706135234714 ) ) ;
#31299=CARTESIAN_POINT ( 'NONE',  ( 0.05219959533934541429, -16.53943276465976808, 20.00109039468568639 ) ) ;
#31300=CARTESIAN_POINT ( 'NONE',  ( 10.72451020669898902, -18.67979575497178502, 27.91557627198103830 ) ) ;
#31301=CARTESIAN_POINT ( 'NONE',  ( -16.51473224551082808, 9.474510206698731452, 28.33442372801900433 ) ) ;
#31302=CARTESIAN_POINT ( 'NONE',  ( 12.06949235617739724, 12.14591786802326823, 41.87609039468568284 ) ) ;
#31303=CARTESIAN_POINT ( 'NONE',  ( -16.46253265017160317, 9.564922557960807481, 105.8322429386476955 ) ) ;
#31304=CARTESIAN_POINT ( 'NONE',  ( 18.67979575497178502, 10.72451020669898547, 104.1655762719810241 ) ) ;
#31305=CARTESIAN_POINT ( 'NONE',  ( -19.02544592524342804, 5.153800228976336051, 76.04057627198102409 ) ) ;
#31307=CARTESIAN_POINT ( 'NONE',  ( 14.34966873604960469, 8.224510206698951720, 84.16557627198103830 ) ) ;
#31308=CARTESIAN_POINT ( 'NONE',  ( 18.67979575497178502, 10.72451020669898547, 39.16557627198102409 ) ) ;
#31309=CARTESIAN_POINT ( 'NONE',  ( -16.21995358207306737, 7.366697692864094371, 34.93551001512157939 ) ) ;
#31310=CARTESIAN_POINT ( 'NONE',  ( -16.53943276465976808, -0.05219959533934237506, 68.75109039468568994 ) ) ;
#31311=CARTESIAN_POINT ( 'NONE',  ( -5.719274019375978568, 21.55341960407610458, 110.2072429386477239 ) ) ;
#31312=CARTESIAN_POINT ( 'NONE',  ( -9.474510206698720793, -16.51473224551083518, 59.58442372801900433 ) ) ;
#31313=CARTESIAN_POINT ( 'NONE',  ( -21.55341960407610458, -5.719274019375992779, 31.45724293864769550 ) ) ;
#31314=CARTESIAN_POINT ( 'NONE',  ( -16.51473224551069308, -9.474510206698971260, 21.66557627198102765 ) ) ;
#31315=CARTESIAN_POINT ( 'NONE',  ( 0.05219959533907565091, 21.53943276465977519, 74.99890960531435269 ) ) ;
#31317=CARTESIAN_POINT ( 'NONE',  ( 16.51473224551069308, 9.474510206698969483, 94.16557627198103830 ) ) ;
#31318=CARTESIAN_POINT ( 'NONE',  ( 21.55341960407619695, -5.719274019375665929, 96.04275706135236135 ) ) ;
#31319=CARTESIAN_POINT ( 'NONE',  ( -19.03943276465977164, 0.05219959533909376836, 51.24890960531436690 ) ) ;
#31321=CARTESIAN_POINT ( 'NONE',  ( 4.379528057220092307, 16.55341960407617563, 32.29275706135235424 ) ) ;
#31322=CARTESIAN_POINT ( 'NONE',  ( -19.05341960407611168, -5.049401038298163336, 61.45724293864769550 ) ) ;
#31323=CARTESIAN_POINT ( 'NONE',  ( 0.05219959533937995610, -21.53943276465977519, 85.00109039468568994 ) ) ;
#31325=CARTESIAN_POINT ( 'NONE',  ( -5.049401038297874678, -19.05341960407617918, 44.79275706135232582 ) ) ;
#31326=CARTESIAN_POINT ( 'NONE',  ( 9.474510206698729675, 16.51473224551082808, 42.08442372801900433 ) ) ;
#31327=CARTESIAN_POINT ( 'NONE',  ( 10.81492255796106328, -18.62759615963255655, 35.41775706135234003 ) ) ;
#31330=CARTESIAN_POINT ( 'NONE',  ( 13.97604488694548053, -13.89961937509957401, 35.62609039468567573 ) ) ;
#31331=CARTESIAN_POINT ( 'NONE',  ( -16.46253265017160317, 9.564922557960807481, 90.83224293864769550 ) ) ;
#31332=CARTESIAN_POINT ( 'NONE',  ( 13.97604488694527802, 13.89961937509977652, 69.37390960531436690 ) ) ;
#31333=CARTESIAN_POINT ( 'NONE',  ( 14.34966873604972726, -8.224510206698740333, 110.8344237280190043 ) ) ;
#31334=CARTESIAN_POINT ( 'NONE',  ( 15.72974639402199770, -15.80617190586745480, 23.12390960531436335 ) ) ;
#31335=CARTESIAN_POINT ( 'NONE',  ( 5.719274019375673035, 21.55341960407619339, 92.29275706135236135 ) ) ;
#31338=CARTESIAN_POINT ( 'NONE',  ( 5.719274019375673035, 21.55341960407619339, 97.29275706135234714 ) ) ;
#31340=CARTESIAN_POINT ( 'NONE',  ( -16.46253265017160317, 9.564922557960807481, 25.83224293864769194 ) ) ;
#31341=CARTESIAN_POINT ( 'NONE',  ( -13.89961937509977652, 13.97604488694528158, 115.6239096053143669 ) ) ;
#31343=CARTESIAN_POINT ( 'NONE',  ( -16.55341960407617563, 4.379528057220093196, 48.54275706135234714 ) ) ;
#31344=CARTESIAN_POINT ( 'NONE',  ( -5.719274019375978568, 21.55341960407610458, 75.20724293864769550 ) ) ;
#31345=CARTESIAN_POINT ( 'NONE',  ( -16.53943276465976808, 0.05219959533911058130, 36.24890960531435979 ) ) ;
#31346=CARTESIAN_POINT ( 'NONE',  ( 16.53943276465976808, -0.05219959533910856209, 103.7489096053143669 ) ) ;
#31347=CARTESIAN_POINT ( 'NONE',  ( 0.05219959533909260263, 19.03943276465977164, 89.99890960531436690 ) ) ;
#31348=CARTESIAN_POINT ( 'NONE',  ( -9.474510206698720793, -16.51473224551083518, 19.58442372801899722 ) ) ;
#31349=CARTESIAN_POINT ( 'NONE',  ( 16.46253265017160672, -9.564922557960803928, 23.33224293864769194 ) ) ;
#31350=CARTESIAN_POINT ( 'NONE',  ( -5.719274019375665041, -21.55341960407619695, 69.79275706135234714 ) ) ;
#31351=CARTESIAN_POINT ( 'NONE',  ( -17.59860650958990647, -7.585241751807021870, 96.57662985737508166 ) ) ;
#31352=CARTESIAN_POINT ( 'NONE',  ( 14.34966873604972726, -8.224510206698740333, 100.8344237280190185 ) ) ;
#31353=CARTESIAN_POINT ( 'NONE',  ( -16.46253265017146816, -9.564922557961047289, 59.16775706135233293 ) ) ;
#31355=CARTESIAN_POINT ( 'NONE',  ( -0.05219959533907301413, -21.53943276465977519, 32.49890960531435979 ) ) ;
#31356=CARTESIAN_POINT ( 'NONE',  ( -12.06949235617756955, 12.14591786802309770, 95.62390960531436690 ) ) ;
#31357=CARTESIAN_POINT ( 'NONE',  ( -0.05219959533936034679, 19.03943276465977164, 52.50109039468566863 ) ) ;
#31359=CARTESIAN_POINT ( 'NONE',  ( 19.02544592524343514, -5.153800228976328945, 73.54057627198103830 ) ) ;
#31360=CARTESIAN_POINT ( 'NONE',  ( 12.06949235617757843, -12.14591786802309237, 63.12390960531435979 ) ) ;
#31361=CARTESIAN_POINT ( 'NONE',  ( -13.97604488694547697, 13.89961937509957934, 88.12609039468563310 ) ) ;
#31362=CARTESIAN_POINT ( 'NONE',  ( 21.52544592524344225, -5.823673210054117533, 48.54057627198103120 ) ) ;
#31364=CARTESIAN_POINT ( 'NONE',  ( 16.53943276465976808, -0.05219959533910856209, 113.7489096053143527 ) ) ;
#31366=CARTESIAN_POINT ( 'NONE',  ( -9.474510206698964154, 16.51473224551069663, 70.41557627198102409 ) ) ;
#31367=CARTESIAN_POINT ( 'NONE',  ( 15.72974639402199770, -15.80617190586745480, 73.12390960531436690 ) ) ;
#31368=CARTESIAN_POINT ( 'NONE',  ( -16.55341960407617563, 4.379528057220093196, 88.54275706135236135 ) ) ;
#31369=CARTESIAN_POINT ( 'NONE',  ( 16.51473224551069308, 9.474510206698969483, 69.16557627198102409 ) ) ;
#31370=CARTESIAN_POINT ( 'NONE',  ( -16.46253265017146816, -9.564922557961047289, 64.16775706135233293 ) ) ;
#31371=CARTESIAN_POINT ( 'NONE',  ( 18.67979575497194134, -10.72451020669871369, 75.83442372801900433 ) ) ;
#31372=CARTESIAN_POINT ( 'NONE',  ( -18.67979575497178146, -10.72451020669898902, 66.66557627198102409 ) ) ;
#31373=CARTESIAN_POINT ( 'NONE',  ( 0.05219959533909260263, 19.03943276465977164, 114.9989096053143669 ) ) ;
#31374=CARTESIAN_POINT ( 'NONE',  ( -16.51473224551069308, -9.474510206698971260, 31.66557627198102054 ) ) ;
#31375=CARTESIAN_POINT ( 'NONE',  ( -8.224510206698735004, -14.34966873604973081, 104.5844237280190185 ) ) ;
#31376=CARTESIAN_POINT ( 'NONE',  ( 16.51473224551069308, 9.474510206698969483, 54.16557627198103120 ) ) ;
#31377=CARTESIAN_POINT ( 'NONE',  ( 14.29746914071037800, 8.314922557961029526, 21.66775706135235069 ) ) ;
#31378=FACE_OUTER_BOUND ( 'NONE', #112348, .T. ) ;
#31379=CARTESIAN_POINT ( 'NONE',  ( -10.81492255796105439, 18.62759615963255655, 112.9177570613523329 ) ) ;
#31380=CARTESIAN_POINT ( 'NONE',  ( 8.224510206698953496, -14.34966873604960469, 57.91557627198103120 ) ) ;
#31382=CARTESIAN_POINT ( 'NONE',  ( 18.62759615963271287, -10.81492255796078972, 113.3322429386476955 ) ) ;
#31383=CARTESIAN_POINT ( 'NONE',  ( 21.53943276465977519, -0.05219959533907433946, 98.74890960531438111 ) ) ;
#31384=CARTESIAN_POINT ( 'NONE',  ( 16.38665767535052709, -7.295008042176097440, 97.76400864214549813 ) ) ;
#31385=CARTESIAN_POINT ( 'NONE',  ( 10.81492255796078972, 18.62759615963270932, 49.58224293864769550 ) ) ;
#31386=CARTESIAN_POINT ( 'NONE',  ( -16.52544592524335698, -4.483927247898792601, 78.95942372801901854 ) ) ;
#31387=CARTESIAN_POINT ( 'NONE',  ( 4.483927247898545687, 16.52544592524342804, 94.79057627198105251 ) ) ;
#31388=CARTESIAN_POINT ( 'NONE',  ( -13.97604488694527625, -13.89961937509977652, 56.87390960531434558 ) ) ;
#31390=CARTESIAN_POINT ( 'NONE',  ( 14.29746914071037800, 8.314922557961029526, 111.6677570613523613 ) ) ;
#31391=CARTESIAN_POINT ( 'NONE',  ( -10.81492255796105439, 18.62759615963255655, 37.91775706135235424 ) ) ;
#31392=CARTESIAN_POINT ( 'NONE',  ( -13.89961937509977652, 13.97604488694528158, 90.62390960531432427 ) ) ;
#31393=CARTESIAN_POINT ( 'NONE',  ( -21.55341960407619339, 5.719274019375674811, 73.54275706135234714 ) ) ;
#31394=CARTESIAN_POINT ( 'NONE',  ( -5.153800228976328057, -19.02544592524343514, 22.29057627198102765 ) ) ;
#31397=CARTESIAN_POINT ( 'NONE',  ( 5.719274019375673035, 21.55341960407619339, 62.29275706135236845 ) ) ;
#31398=CARTESIAN_POINT ( 'NONE',  ( -19.05341960407611168, -5.049401038298163336, 56.45724293864768129 ) ) ;
#31399=CARTESIAN_POINT ( 'NONE',  ( 19.02544592524343514, -5.153800228976328945, 83.54057627198100988 ) ) ;
#31400=CARTESIAN_POINT ( 'NONE',  ( 19.05341960407617918, -5.049401038297876454, 71.04275706135234714 ) ) ;
#31401=CARTESIAN_POINT ( 'NONE',  ( -21.55341960407619339, 5.719274019375674811, 43.54275706135235424 ) ) ;
#31402=CARTESIAN_POINT ( 'NONE',  ( 16.46253265017146816, 9.564922557961045513, 101.6677570613523329 ) ) ;
#31403=CARTESIAN_POINT ( 'NONE',  ( -13.89961937509957401, -13.97604488694547875, 69.37609039468564731 ) ) ;
#31404=CARTESIAN_POINT ( 'NONE',  ( 5.153800228976335163, 19.02544592524342804, 34.79057627198102409 ) ) ;
#31405=CARTESIAN_POINT ( 'NONE',  ( 14.29746914071037800, 8.314922557961029526, 106.6677570613523756 ) ) ;
#31406=CARTESIAN_POINT ( 'NONE',  ( 19.05341960407617918, -5.049401038297876454, 71.04275706135234714 ) ) ;
#31407=CARTESIAN_POINT ( 'NONE',  ( 4.483927247898545687, 16.52544592524342804, 24.79057627198103120 ) ) ;
#31408=CARTESIAN_POINT ( 'NONE',  ( 13.97604488694548053, -13.89961937509957401, 45.62609039468566863 ) ) ;
#31409=CARTESIAN_POINT ( 'NONE',  ( -5.719274019375665041, -21.55341960407619695, 99.79275706135234714 ) ) ;
#31410=CARTESIAN_POINT ( 'NONE',  ( -5.153800228976607833, 19.02544592524334988, 27.70942372801899722 ) ) ;
#31411=CARTESIAN_POINT ( 'NONE',  ( 13.89961937509977652, -13.97604488694527269, 23.12390960531436335 ) ) ;
#31412=CARTESIAN_POINT ( 'NONE',  ( 0.05219959533937995610, -21.53943276465977519, 85.00109039468568994 ) ) ;
#31413=CARTESIAN_POINT ( 'NONE',  ( -4.483927247898782831, 16.52544592524335698, 27.70942372801901854 ) ) ;
#31414=CARTESIAN_POINT ( 'NONE',  ( 19.03943276465977164, -0.05219959533909143690, 93.74890960531435269 ) ) ;
#31416=CARTESIAN_POINT ( 'NONE',  ( -5.153800228976328057, -19.02544592524343514, 82.29057627198103830 ) ) ;
#31418=ORIENTED_EDGE ( 'NONE', *, *, #78315, .T. ) ;
#31419=CARTESIAN_POINT ( 'NONE',  ( -13.97604488694547697, 13.89961937509957934, 83.12609039468564731 ) ) ;
#31420=CARTESIAN_POINT ( 'NONE',  ( -0.05219959533909027116, -19.03943276465977164, 112.4989096053143669 ) ) ;
#31421=CARTESIAN_POINT ( 'NONE',  ( -21.53943276465977519, -0.05219959533937600094, 113.7510903946856757 ) ) ;
#31422=CARTESIAN_POINT ( 'NONE',  ( -0.05219959533910754901, -16.53943276465976808, 92.49890960531436690 ) ) ;
#31424=CARTESIAN_POINT ( 'NONE',  ( 15.80617190586746368, 15.72974639402197994, 54.37390960531435979 ) ) ;
#31425=CARTESIAN_POINT ( 'NONE',  ( -15.80617190586745835, -15.72974639402198527, 41.87390960531435979 ) ) ;
#31426=CARTESIAN_POINT ( 'NONE',  ( 19.02544592524343514, -5.153800228976328945, 23.54057627198102054 ) ) ;
#31428=CARTESIAN_POINT ( 'NONE',  ( -13.97604488694547697, 13.89961937509957934, 58.12609039468566863 ) ) ;
#31429=CARTESIAN_POINT ( 'NONE',  ( 12.14591786802309770, 12.06949235617756955, 44.37390960531435979 ) ) ;
#31430=CARTESIAN_POINT ( 'NONE',  ( 18.67979575497178502, 10.72451020669898547, 24.16557627198103120 ) ) ;
#31431=CARTESIAN_POINT ( 'NONE',  ( 18.67979575497194134, -10.72451020669871369, 85.83442372801901854 ) ) ;
#31432=CARTESIAN_POINT ( 'NONE',  ( 21.53943276465977519, -0.05219959533907433946, 73.74890960531433848 ) ) ;
#31433=CARTESIAN_POINT ( 'NONE',  ( -15.72974639402176322, -15.80617190586768395, 59.37609039468568284 ) ) ;
#31434=CARTESIAN_POINT ( 'NONE',  ( -5.823673210054431948, 21.52544592524334988, 47.70942372801902565 ) ) ;
#31435=CARTESIAN_POINT ( 'NONE',  ( 9.474510206698971260, -16.51473224551069308, 87.91557627198102409 ) ) ;
#31436=CARTESIAN_POINT ( 'NONE',  ( 14.29746914071037800, 8.314922557961029526, 76.66775706135234714 ) ) ;
#31437=CARTESIAN_POINT ( 'NONE',  ( 19.05341960407611168, 5.049401038298154454, 28.95724293864769550 ) ) ;
#31439=CARTESIAN_POINT ( 'NONE',  ( -8.224510206698948167, 14.34966873604960824, 55.41557627198102409 ) ) ;
#31440=CARTESIAN_POINT ( 'NONE',  ( 16.52544592524342804, -4.483927247898539470, 28.54057627198103120 ) ) ;
#31441=CARTESIAN_POINT ( 'NONE',  ( 16.46253265017160672, -9.564922557960803928, 68.33224293864770971 ) ) ;
#31442=CARTESIAN_POINT ( 'NONE',  ( 5.049401038298161559, -19.05341960407611168, 32.70724293864768129 ) ) ;
#31443=CARTESIAN_POINT ( 'NONE',  ( 18.67979575497178502, 10.72451020669898547, 39.16557627198102409 ) ) ;
#31444=CARTESIAN_POINT ( 'NONE',  ( 19.02544592524334988, 5.153800228976608722, 31.45942372801900433 ) ) ;
#31447=CARTESIAN_POINT ( 'NONE',  ( -16.52544592524342804, 4.483927247898546575, 56.04057627198102409 ) ) ;
#31448=CARTESIAN_POINT ( 'NONE',  ( -21.55341960407610458, -5.719274019375992779, 21.45724293864769550 ) ) ;
#31450=CARTESIAN_POINT ( 'NONE',  ( 4.483927247898790824, -16.52544592524335698, 70.20942372801904696 ) ) ;
#31451=CARTESIAN_POINT ( 'NONE',  ( -9.474510206698720793, -16.51473224551083518, 69.58442372801901854 ) ) ;
#31452=CARTESIAN_POINT ( 'NONE',  ( -8.224510206698948167, 14.34966873604960824, 40.41557627198103120 ) ) ;
#31453=CARTESIAN_POINT ( 'NONE',  ( 17.44270441346517941, -5.991230190323000748, 51.13664920735774899 ) ) ;
#31454=CARTESIAN_POINT ( 'NONE',  ( 8.224510206698953496, -14.34966873604960469, 27.91557627198103830 ) ) ;
#31455=CARTESIAN_POINT ( 'NONE',  ( -13.97604488694527625, -13.89961937509977652, 31.87390960531435979 ) ) ;
#31457=CARTESIAN_POINT ( 'NONE',  ( 9.474510206698971260, -16.51473224551069308, 62.91557627198102409 ) ) ;
#31458=CARTESIAN_POINT ( 'NONE',  ( -19.02544592524342804, 5.153800228976336051, 46.04057627198101699 ) ) ;
#31459=CARTESIAN_POINT ( 'NONE',  ( 15.80617190586769283, -15.72974639402175789, 45.62609039468567573 ) ) ;
#31460=CARTESIAN_POINT ( 'NONE',  ( -16.46253265017160317, 9.564922557960807481, 60.83224293864769550 ) ) ;
#31462=CARTESIAN_POINT ( 'NONE',  ( 9.564922557960805705, 16.46253265017160317, 39.58224293864768839 ) ) ;
#31463=CARTESIAN_POINT ( 'NONE',  ( -10.81492255796078084, -18.62759615963271287, 37.08224293864768129 ) ) ;
#31464=CARTESIAN_POINT ( 'NONE',  ( 5.823673210054444382, -21.52544592524334988, 60.20942372801902565 ) ) ;
#31465=CARTESIAN_POINT ( 'NONE',  ( -19.03943276465977164, 0.05219959533909376836, 21.24890960531436335 ) ) ;
#31466=CARTESIAN_POINT ( 'NONE',  ( -5.823673210054116645, -21.52544592524344225, 22.29057627198102765 ) ) ;
#31467=CARTESIAN_POINT ( 'NONE',  ( 16.55341960407618274, -4.379528057220086978, 96.04275706135236135 ) ) ;
#31468=CARTESIAN_POINT ( 'NONE',  ( 18.67979575497194134, -10.72451020669871369, 105.8344237280190328 ) ) ;
#31469=CARTESIAN_POINT ( 'NONE',  ( -16.55341960407617563, 4.379528057220093196, 68.54275706135234714 ) ) ;
#31470=CARTESIAN_POINT ( 'NONE',  ( -19.03943276465977164, 0.05219959533909376836, 111.2489096053143669 ) ) ;
#31471=CARTESIAN_POINT ( 'NONE',  ( 8.224510206698742110, 14.34966873604972548, 52.08442372801901854 ) ) ;
#31472=CARTESIAN_POINT ( 'NONE',  ( 12.06949235617739724, 12.14591786802326823, 41.87609039468568284 ) ) ;
#31473=CARTESIAN_POINT ( 'NONE',  ( 14.29746914071037800, 8.314922557961029526, 96.66775706135234714 ) ) ;
#31474=CARTESIAN_POINT ( 'NONE',  ( 15.80617190586769283, -15.72974639402175789, 55.62609039468568284 ) ) ;
#31475=CARTESIAN_POINT ( 'NONE',  ( -19.03943276465977164, -0.05219959533935918106, 113.7510903946856757 ) ) ;
#31476=CARTESIAN_POINT ( 'NONE',  ( 15.72974639402199770, -15.80617190586745480, 108.1239096053143811 ) ) ;
#31477=CARTESIAN_POINT ( 'NONE',  ( 12.14591786802327356, -12.06949235617739191, 25.62609039468567929 ) ) ;
#31478=CARTESIAN_POINT ( 'NONE',  ( -8.224510206698735004, -14.34966873604973081, 84.58442372801903275 ) ) ;
#31480=CARTESIAN_POINT ( 'NONE',  ( 18.67979575497194134, -10.72451020669871369, 80.83442372801901854 ) ) ;
#31481=CARTESIAN_POINT ( 'NONE',  ( -19.05341960407617563, 5.049401038297882671, 83.54275706135233293 ) ) ;
#31482=CARTESIAN_POINT ( 'NONE',  ( 8.224510206698953496, -14.34966873604960469, 52.91557627198103830 ) ) ;
#31483=CARTESIAN_POINT ( 'NONE',  ( 16.53943276465976808, -0.05219959533910856209, 43.74890960531435979 ) ) ;
#31484=CARTESIAN_POINT ( 'NONE',  ( -16.53943276465976808, 0.05219959533911058130, 106.2489096053143811 ) ) ;
#31485=CARTESIAN_POINT ( 'NONE',  ( -9.564922557961040184, 16.46253265017147172, 47.91775706135233293 ) ) ;
#31487=CARTESIAN_POINT ( 'NONE',  ( -21.53943276465977519, -0.05219959533937600094, 53.75109039468568994 ) ) ;
#31488=CARTESIAN_POINT ( 'NONE',  ( -16.51473224551082808, 9.474510206698731452, 108.3344237280190043 ) ) ;
#31490=CARTESIAN_POINT ( 'NONE',  ( -0.05219959533909027116, -19.03943276465977164, 102.4989096053143669 ) ) ;
#31491=CARTESIAN_POINT ( 'NONE',  ( 21.53943276465977519, -0.05219959533907433946, 68.74890960531435269 ) ) ;
#31492=CARTESIAN_POINT ( 'NONE',  ( 19.03943276465977164, 0.05219959533936151252, 101.2510903946856757 ) ) ;
#31493=CARTESIAN_POINT ( 'NONE',  ( 16.51473224551069308, 9.474510206698969483, 99.16557627198102409 ) ) ;
#31494=CARTESIAN_POINT ( 'NONE',  ( 15.72974639402199770, -15.80617190586745480, 58.12390960531435979 ) ) ;
#31495=CARTESIAN_POINT ( 'NONE',  ( 16.53943276465976808, -0.05219959533910856209, 103.7489096053143669 ) ) ;
#31496=CARTESIAN_POINT ( 'NONE',  ( 10.81492255796106328, -18.62759615963255655, 90.41775706135236135 ) ) ;
#31497=CARTESIAN_POINT ( 'NONE',  ( 16.51473224551069308, 9.474510206698969483, 24.16557627198102765 ) ) ;
#31499=CARTESIAN_POINT ( 'NONE',  ( 10.72451020669871369, 18.67979575497193778, 37.08442372801901143 ) ) ;
#31500=CARTESIAN_POINT ( 'NONE',  ( -18.62759615963255300, -10.81492255796106328, 84.16775706135234714 ) ) ;
#31501=CARTESIAN_POINT ( 'NONE',  ( 4.379528057220092307, 16.55341960407617563, 92.29275706135236135 ) ) ;
#31502=CARTESIAN_POINT ( 'NONE',  ( 5.823673210054444382, -21.52544592524334988, 25.20942372801901854 ) ) ;
#31503=CARTESIAN_POINT ( 'NONE',  ( -18.67979575497193778, 10.72451020669871902, 33.33442372801900433 ) ) ;
#31504=CARTESIAN_POINT ( 'NONE',  ( 19.05341960407617918, -5.049401038297876454, 71.04275706135234714 ) ) ;
#31505=CARTESIAN_POINT ( 'NONE',  ( -19.05341960407611168, -5.049401038298163336, 81.45724293864769550 ) ) ;
#31506=CARTESIAN_POINT ( 'NONE',  ( -0.05219959533937732626, 21.53943276465977519, 82.50109039468568994 ) ) ;
#31507=CARTESIAN_POINT ( 'NONE',  ( -15.80617190586745835, -15.72974639402198527, 76.87390960531439532 ) ) ;
#31508=CARTESIAN_POINT ( 'NONE',  ( 4.483927247898545687, 16.52544592524342804, 59.79057627198103120 ) ) ;
#31509=CARTESIAN_POINT ( 'NONE',  ( 15.80617190586769283, -15.72974639402175789, 105.6260903946856899 ) ) ;
#31510=CARTESIAN_POINT ( 'NONE',  ( 0.05219959533910956823, 16.53943276465976808, 89.99890960531438111 ) ) ;
#31511=CARTESIAN_POINT ( 'NONE',  ( 19.05341960407611168, 5.049401038298154454, 38.95724293864767418 ) ) ;
#31512=CARTESIAN_POINT ( 'NONE',  ( 5.153800228976615827, -19.02544592524334988, 75.20942372801896170 ) ) ;
#31513=CARTESIAN_POINT ( 'NONE',  ( -14.29746914071049879, 8.314922557960819915, 30.83224293864770260 ) ) ;
#31514=CARTESIAN_POINT ( 'NONE',  ( 21.55341960407619695, -5.719274019375665929, 101.0427570613523756 ) ) ;
#31515=CARTESIAN_POINT ( 'NONE',  ( 5.049401038298161559, -19.05341960407611168, 92.70724293864769550 ) ) ;
#31516=CARTESIAN_POINT ( 'NONE',  ( 13.89961937509957401, 13.97604488694547697, 66.87609039468567573 ) ) ;
#31517=CARTESIAN_POINT ( 'NONE',  ( -18.67979575497178146, -10.72451020669898902, 66.66557627198102409 ) ) ;
#31518=CARTESIAN_POINT ( 'NONE',  ( -21.53943276465977519, 0.05219959533907696930, 111.2489096053143669 ) ) ;
#31519=CARTESIAN_POINT ( 'NONE',  ( 9.564922557961047289, -16.46253265017146816, 110.4177570613523471 ) ) ;
#31520=CARTESIAN_POINT ( 'NONE',  ( 8.314922557961029526, -14.29746914071037800, 75.41775706135233293 ) ) ;
#31521=CARTESIAN_POINT ( 'NONE',  ( 16.81555441253551209, 7.025013491695494494, 61.86314554665744936 ) ) ;
#31522=CARTESIAN_POINT ( 'NONE',  ( -18.62759615963255300, -10.81492255796106328, 29.16775706135234003 ) ) ;
#31523=CARTESIAN_POINT ( 'NONE',  ( -12.06949235617756955, 12.14591786802309770, 100.6239096053143811 ) ) ;
#31525=CARTESIAN_POINT ( 'NONE',  ( -8.224510206698735004, -14.34966873604973081, 44.58442372801901854 ) ) ;
#31526=CARTESIAN_POINT ( 'NONE',  ( -16.55341960407611168, -4.379528057220339221, 76.45724293864769550 ) ) ;
#31527=CARTESIAN_POINT ( 'NONE',  ( 21.55341960407610458, 5.719274019375980345, 68.95724293864769550 ) ) ;
#31528=CARTESIAN_POINT ( 'NONE',  ( 12.06949235617739724, 12.14591786802326823, 106.8760903946856899 ) ) ;
#31529=CARTESIAN_POINT ( 'NONE',  ( 8.224510206698742110, 14.34966873604972548, 42.08442372801901854 ) ) ;
#31530=CARTESIAN_POINT ( 'NONE',  ( 5.049401038298161559, -19.05341960407611168, 42.70724293864767418 ) ) ;
#31531=CARTESIAN_POINT ( 'NONE',  ( 4.379528057220092307, 16.55341960407617563, 77.29275706135234714 ) ) ;
#31532=CARTESIAN_POINT ( 'NONE',  ( -5.153800228976607833, 19.02544592524334988, 67.70942372801900433 ) ) ;
#31533=CARTESIAN_POINT ( 'NONE',  ( 18.67979575497178502, 10.72451020669898547, 74.16557627198102409 ) ) ;
#31534=CARTESIAN_POINT ( 'NONE',  ( -16.55341960407617563, 4.379528057220093196, 93.54275706135234714 ) ) ;
#31535=CARTESIAN_POINT ( 'NONE',  ( -10.72451020669870658, -18.67979575497194134, 84.58442372801903275 ) ) ;
#31536=CARTESIAN_POINT ( 'NONE',  ( 10.72451020669898902, -18.67979575497178502, 67.91557627198102409 ) ) ;
#31537=CARTESIAN_POINT ( 'NONE',  ( 15.72974639402199770, -15.80617190586745480, 53.12390960531436690 ) ) ;
#31539=ORIENTED_EDGE ( 'NONE', *, *, #141448, .T. ) ;
#31540=CARTESIAN_POINT ( 'NONE',  ( -4.379528057220086978, -16.55341960407618274, 74.79275706135234714 ) ) ;
#31541=CARTESIAN_POINT ( 'NONE',  ( 5.823673210054125526, 21.52544592524343514, 44.79057627198103120 ) ) ;
#31543=CARTESIAN_POINT ( 'NONE',  ( -9.564922557960796823, -16.46253265017161027, 112.0822429386476955 ) ) ;
#31544=CARTESIAN_POINT ( 'NONE',  ( -19.35633801406909171, 5.499999999999578115, 74.13373818172760821 ) ) ;
#31545=CARTESIAN_POINT ( 'NONE',  ( -9.564922557960796823, -16.46253265017161027, 27.08224293864769550 ) ) ;
#31546=CARTESIAN_POINT ( 'NONE',  ( 18.62759615963271287, -10.81492255796078972, 73.33224293864769550 ) ) ;
#31547=CARTESIAN_POINT ( 'NONE',  ( 16.52544592524335698, 4.483927247898782831, 106.4594237280190328 ) ) ;
#31548=CARTESIAN_POINT ( 'NONE',  ( 10.81492255796106328, -18.62759615963255655, 45.41775706135234003 ) ) ;
#31549=CARTESIAN_POINT ( 'NONE',  ( 16.55341960407618274, -4.379528057220086978, 21.04275706135234714 ) ) ;
#31550=CARTESIAN_POINT ( 'NONE',  ( 0.05219959533910956823, 16.53943276465976808, 114.9989096053143669 ) ) ;
#31551=CARTESIAN_POINT ( 'NONE',  ( -0.05219959533936034679, 19.03943276465977164, 107.5010903946856615 ) ) ;
#31552=CARTESIAN_POINT ( 'NONE',  ( -19.05341960407611168, -5.049401038298163336, 41.45724293864769550 ) ) ;
#31554=CARTESIAN_POINT ( 'NONE',  ( 19.05341960407611168, 5.049401038298154454, 108.9572429386477097 ) ) ;
#31556=CARTESIAN_POINT ( 'NONE',  ( -4.483927247898782831, 16.52544592524335698, 87.70942372801901854 ) ) ;
#31557=CARTESIAN_POINT ( 'NONE',  ( -13.89961937509957401, -13.97604488694547875, 74.37609039468566152 ) ) ;
#31558=CARTESIAN_POINT ( 'NONE',  ( 19.03943276465977164, 0.05219959533936151252, 26.25109039468566507 ) ) ;
#31559=CARTESIAN_POINT ( 'NONE',  ( 18.62759615963271287, -10.81492255796078972, 63.33224293864770260 ) ) ;
#31560=CARTESIAN_POINT ( 'NONE',  ( -4.379528057220086978, -16.55341960407618274, 89.79275706135236135 ) ) ;
#31561=CARTESIAN_POINT ( 'NONE',  ( -13.97604488694547697, 13.89961937509957934, 88.12609039468563310 ) ) ;
#31562=CARTESIAN_POINT ( 'NONE',  ( 16.46253265017160672, -9.564922557960803928, 48.33224293864769550 ) ) ;
#31563=CARTESIAN_POINT ( 'NONE',  ( -5.049401038298153566, 19.05341960407611168, 95.20724293864770971 ) ) ;
#31564=CARTESIAN_POINT ( 'NONE',  ( 18.67979575497194134, -10.72451020669871369, 45.83442372801901854 ) ) ;
#31565=CARTESIAN_POINT ( 'NONE',  ( -19.03943276465977164, 0.05219959533909376836, 41.24890960531435269 ) ) ;
#31567=CARTESIAN_POINT ( 'NONE',  ( -16.46253265017160317, 9.564922557960807481, 105.8322429386476955 ) ) ;
#31568=CARTESIAN_POINT ( 'NONE',  ( -16.52544592524342804, 4.483927247898546575, 66.04057627198103830 ) ) ;
#31569=CARTESIAN_POINT ( 'NONE',  ( 21.55341960407610458, 5.719274019375980345, 63.95724293864770260 ) ) ;
#31571=CARTESIAN_POINT ( 'NONE',  ( -9.564922557961040184, 16.46253265017147172, 42.91775706135234003 ) ) ;
#31573=CARTESIAN_POINT ( 'NONE',  ( 5.153800228976335163, 19.02544592524342804, 69.79057627198103830 ) ) ;
#31574=CARTESIAN_POINT ( 'NONE',  ( -16.46253265017160317, 9.564922557960807481, 75.83224293864769550 ) ) ;
#31575=CARTESIAN_POINT ( 'NONE',  ( 14.34966873604972726, -8.224510206698740333, 50.83442372801901143 ) ) ;
#31577=CARTESIAN_POINT ( 'NONE',  ( -17.31728774477274868, 6.344390552232366254, 110.8190665168931872 ) ) ;
#31578=CARTESIAN_POINT ( 'NONE',  ( -16.53943276465976808, -0.05219959533934237506, 93.75109039468567573 ) ) ;
#31581=CARTESIAN_POINT ( 'NONE',  ( 14.34966873604972726, -8.224510206698740333, 85.83442372801901854 ) ) ;
#31582=CARTESIAN_POINT ( 'NONE',  ( 4.483927247898790824, -16.52544592524335698, 55.20942372801902565 ) ) ;
#31583=CARTESIAN_POINT ( 'NONE',  ( -0.05219959533937732626, 21.53943276465977519, 112.5010903946857042 ) ) ;
#31584=CARTESIAN_POINT ( 'NONE',  ( 9.564922557960805705, 16.46253265017160317, 49.58224293864770260 ) ) ;
#31586=CARTESIAN_POINT ( 'NONE',  ( -18.67979575497193778, 10.72451020669871902, 48.33442372801902565 ) ) ;
#31587=CARTESIAN_POINT ( 'NONE',  ( -5.153800228976607833, 19.02544592524334988, 57.70942372801899012 ) ) ;
#31588=CARTESIAN_POINT ( 'NONE',  ( 21.55341960407619695, -5.719274019375665929, 111.0427570613523613 ) ) ;
#31589=CARTESIAN_POINT ( 'NONE',  ( -19.02544592524342804, 5.153800228976336051, 31.04057627198102409 ) ) ;
#31590=CARTESIAN_POINT ( 'NONE',  ( 17.08218171090884141, 6.734076229372654154, 23.85283434757613819 ) ) ;
#31591=CARTESIAN_POINT ( 'NONE',  ( -21.55341960407610458, -5.719274019375992779, 66.45724293864768129 ) ) ;
#31593=CARTESIAN_POINT ( 'NONE',  ( 16.46253265017160672, -9.564922557960803928, 113.3322429386476955 ) ) ;
#31594=CARTESIAN_POINT ( 'NONE',  ( 16.53943276465976808, -0.05219959533910856209, 113.7489096053143527 ) ) ;
#31595=CARTESIAN_POINT ( 'NONE',  ( -8.314922557961024197, 14.29746914071037800, 32.91775706135234714 ) ) ;
#31596=CARTESIAN_POINT ( 'NONE',  ( -14.29746914071049879, 8.314922557960819915, 25.83224293864769194 ) ) ;
#31598=CARTESIAN_POINT ( 'NONE',  ( -0.05219959533937732626, 21.53943276465977519, 22.50109039468567573 ) ) ;
#31599=CARTESIAN_POINT ( 'NONE',  ( -4.483927247898539470, -16.52544592524342804, 37.29057627198102409 ) ) ;
#31600=CARTESIAN_POINT ( 'NONE',  ( -19.03943276465977164, 0.05219959533909376836, 111.2489096053143669 ) ) ;
#31601=CARTESIAN_POINT ( 'NONE',  ( 19.02544592524334988, 5.153800228976608722, 111.4594237280190043 ) ) ;
#31602=CARTESIAN_POINT ( 'NONE',  ( -13.97604488694547697, 13.89961937509957934, 33.12609039468566863 ) ) ;
#31603=CARTESIAN_POINT ( 'NONE',  ( -14.29746914071049879, 8.314922557960819915, 45.83224293864769550 ) ) ;
#31604=CARTESIAN_POINT ( 'NONE',  ( -5.823673210054116645, -21.52544592524344225, 97.29057627198105251 ) ) ;
#31606=CARTESIAN_POINT ( 'NONE',  ( 5.719274019375991003, -21.55341960407610458, 62.70724293864769550 ) ) ;
#31607=CARTESIAN_POINT ( 'NONE',  ( 19.03943276465977164, -0.05219959533909143690, 73.74890960531435269 ) ) ;
#31608=CARTESIAN_POINT ( 'NONE',  ( 4.379528057220339221, -16.55341960407611168, 42.70724293864770260 ) ) ;
#31609=CARTESIAN_POINT ( 'NONE',  ( -16.51473224551069308, -9.474510206698971260, 91.66557627198103830 ) ) ;
#31611=CARTESIAN_POINT ( 'NONE',  ( 19.05341960407617918, -5.049401038297876454, 56.04275706135234714 ) ) ;
#31612=CARTESIAN_POINT ( 'NONE',  ( 5.719274019375991003, -21.55341960407610458, 87.70724293864769550 ) ) ;
#31613=CARTESIAN_POINT ( 'NONE',  ( -4.379528057220328563, 16.55341960407611168, 95.20724293864769550 ) ) ;
#31614=CARTESIAN_POINT ( 'NONE',  ( -18.62759615963255300, -10.81492255796106328, 49.16775706135234003 ) ) ;
#31617=CARTESIAN_POINT ( 'NONE',  ( 4.483927247898545687, 16.52544592524342804, 29.79057627198102409 ) ) ;
#31618=CARTESIAN_POINT ( 'NONE',  ( -0.05219959533909027116, -19.03943276465977164, 37.49890960531436690 ) ) ;
#31619=CARTESIAN_POINT ( 'NONE',  ( 19.02544592524343514, -5.153800228976328945, 103.5405762719809957 ) ) ;
#31620=CARTESIAN_POINT ( 'NONE',  ( -18.67979575497178146, -10.72451020669898902, 56.66557627198103830 ) ) ;
#31621=CARTESIAN_POINT ( 'NONE',  ( -17.59860650958993844, 7.585241751806885979, 93.42337014262493256 ) ) ;
#31622=CARTESIAN_POINT ( 'NONE',  ( -19.03943276465977164, 0.05219959533909376836, 31.24890960531435979 ) ) ;
#31623=CARTESIAN_POINT ( 'NONE',  ( 15.72974639402199770, -15.80617190586745480, 53.12390960531436690 ) ) ;
#31624=CARTESIAN_POINT ( 'NONE',  ( -21.55341960407619339, 5.719274019375674811, 68.54275706135234714 ) ) ;
#31626=CARTESIAN_POINT ( 'NONE',  ( 4.379528057220092307, 16.55341960407617563, 87.29275706135236135 ) ) ;
#31627=CARTESIAN_POINT ( 'NONE',  ( -13.97604488694527625, -13.89961937509977652, 61.87390960531435979 ) ) ;
#31628=CARTESIAN_POINT ( 'NONE',  ( -19.02544592524342804, 5.153800228976336051, 66.04057627198103830 ) ) ;
#31629=( BOUNDED_CURVE ( )  B_SPLINE_CURVE ( 2, ( #190588, #96562, #158250, #97543, #159230, #20725, #52064, #6545, #68224, #129877, #191576, #53054, #37902 ),
 .UNSPECIFIED., .F., .T. ) 
 B_SPLINE_CURVE_WITH_KNOTS ( ( 3, 2, 2, 2, 2, 2, 3 ),
 ( 0.5813778048480978677, 0.5833333333333333703, 0.5877192982456140857, 0.5921052631578946901, 0.5964912280701754055, 0.6008771929824561209, 0.6027870416456015956 ),
 .UNSPECIFIED. ) 
 CURVE ( )  GEOMETRIC_REPRESENTATION_ITEM ( )  RATIONAL_B_SPLINE_CURVE ( ( 0.9831626618144007068, 0.9848076720550096308, 1.000000000000000000, 0.9659258262890683122, 1.000000000000000000, 0.9659258262890683122, 1.000000000000000000, 0.9659258262890683122, 1.000000000000000000, 0.9659258262890683122, 1.000000000000000000, 0.9851625545550091179, 0.9832469066685282089 ) ) 
 REPRESENTATION_ITEM ( '' )  );
#31631=CARTESIAN_POINT ( 'NONE',  ( 19.03943276465977164, 0.05219959533936151252, 31.25109039468566863 ) ) ;
#31632=CARTESIAN_POINT ( 'NONE',  ( 16.53943276465976808, 0.05219959533934440121, 71.25109039468568994 ) ) ;
#31633=CARTESIAN_POINT ( 'NONE',  ( -10.72451020669870658, -18.67979575497194134, 104.5844237280190185 ) ) ;
#31634=CARTESIAN_POINT ( 'NONE',  ( -5.049401038298153566, 19.05341960407611168, 70.20724293864769550 ) ) ;
#31635=CARTESIAN_POINT ( 'NONE',  ( -10.81492255796078084, -18.62759615963271287, 32.08224293864769550 ) ) ;
#31636=CARTESIAN_POINT ( 'NONE',  ( -13.97604488694547697, 13.89961937509957934, 108.1260903946856331 ) ) ;
#31637=CARTESIAN_POINT ( 'NONE',  ( 15.72974639402176855, 15.80617190586768217, 76.87609039468567573 ) ) ;
#31638=CARTESIAN_POINT ( 'NONE',  ( 14.34966873604972726, -8.224510206698740333, 45.83442372801901854 ) ) ;
#31639=CARTESIAN_POINT ( 'NONE',  ( -5.719274019375978568, 21.55341960407610458, 95.20724293864769550 ) ) ;
#31640=CARTESIAN_POINT ( 'NONE',  ( 16.51473224551083163, -9.474510206698727899, 105.8344237280190043 ) ) ;
#31641=CARTESIAN_POINT ( 'NONE',  ( -13.89961937509977652, 13.97604488694528158, 75.62390960531438111 ) ) ;
#31642=CARTESIAN_POINT ( 'NONE',  ( -14.34966873604972548, 8.224510206698743886, 23.33442372801901499 ) ) ;
#31643=CARTESIAN_POINT ( 'NONE',  ( -5.153800228976328057, -19.02544592524343514, 42.29057627198101699 ) ) ;
#31644=CARTESIAN_POINT ( 'NONE',  ( 9.564922557961047289, -16.46253265017146816, 110.4177570613523471 ) ) ;
#31645=CARTESIAN_POINT ( 'NONE',  ( -16.55341960407611168, -4.379528057220339221, 66.45724293864768129 ) ) ;
#31646=CARTESIAN_POINT ( 'NONE',  ( 4.379528057220092307, 16.55341960407617563, 72.29275706135236135 ) ) ;
#31647=CARTESIAN_POINT ( 'NONE',  ( -5.823673210054431948, 21.52544592524334988, 27.70942372801901854 ) ) ;
#31648=CARTESIAN_POINT ( 'NONE',  ( 13.97604488694527802, 13.89961937509977652, 49.37390960531434558 ) ) ;
#31649=CARTESIAN_POINT ( 'NONE',  ( -9.564922557960796823, -16.46253265017161027, 67.08224293864769550 ) ) ;
#31650=CARTESIAN_POINT ( 'NONE',  ( -14.34966873604972548, 8.224510206698743886, 78.33442372801901854 ) ) ;
#31654=CARTESIAN_POINT ( 'NONE',  ( -15.80617190586768217, 15.72974639402176855, 108.1260903946856757 ) ) ;
#31656=CARTESIAN_POINT ( 'NONE',  ( -16.51473224551069308, -9.474510206698971260, 41.66557627198103120 ) ) ;
#31657=CARTESIAN_POINT ( 'NONE',  ( 19.05341960407611168, 5.049401038298154454, 108.9572429386477097 ) ) ;
#31659=CARTESIAN_POINT ( 'NONE',  ( -12.06949235617739369, -12.14591786802326823, 34.37609039468568284 ) ) ;
#31660=CARTESIAN_POINT ( 'NONE',  ( 16.46253265017146816, 9.564922557961045513, 61.66775706135234003 ) ) ;
#31661=CARTESIAN_POINT ( 'NONE',  ( -14.34966873604972548, 8.224510206698743886, 38.33442372801900433 ) ) ;
#31662=CARTESIAN_POINT ( 'NONE',  ( -9.564922557960796823, -16.46253265017161027, 42.08224293864769550 ) ) ;
#31663=CARTESIAN_POINT ( 'NONE',  ( 19.03943276465977164, -0.05219959533909143690, 103.7489096053143669 ) ) ;
#31664=CARTESIAN_POINT ( 'NONE',  ( -9.564922557960796823, -16.46253265017161027, 62.08224293864769550 ) ) ;
#31665=CARTESIAN_POINT ( 'NONE',  ( 21.53943276465977519, -0.05219959533907433946, 98.74890960531438111 ) ) ;
#31666=CARTESIAN_POINT ( 'NONE',  ( 5.049401038298161559, -19.05341960407611168, 92.70724293864769550 ) ) ;
#31667=CARTESIAN_POINT ( 'NONE',  ( -5.153800228976328057, -19.02544592524343514, 22.29057627198102765 ) ) ;
#31668=CARTESIAN_POINT ( 'NONE',  ( -13.89961937509977652, 13.97604488694528158, 65.62390960531436690 ) ) ;
#31669=CARTESIAN_POINT ( 'NONE',  ( -16.52544592524335698, -4.483927247898792601, 108.9594237280190185 ) ) ;
#31670=CARTESIAN_POINT ( 'NONE',  ( 5.153800228976335163, 19.02544592524342804, 24.79057627198102765 ) ) ;
#31671=CARTESIAN_POINT ( 'NONE',  ( -16.46253265017146816, -9.564922557961047289, 104.1677570613523329 ) ) ;
#31672=CARTESIAN_POINT ( 'NONE',  ( -18.67979575497193778, 10.72451020669871902, 113.3344237280190328 ) ) ;
#31674=CARTESIAN_POINT ( 'NONE',  ( -16.55341960407611168, -4.379528057220339221, 56.45724293864768839 ) ) ;
#31675=CARTESIAN_POINT ( 'NONE',  ( -18.67979575497193778, 10.72451020669871902, 98.33442372801901854 ) ) ;
#31676=CARTESIAN_POINT ( 'NONE',  ( 9.474510206698971260, -16.51473224551069308, 37.91557627198102409 ) ) ;
#31677=CARTESIAN_POINT ( 'NONE',  ( 8.224510206698953496, -14.34966873604960469, 42.91557627198103120 ) ) ;
#31678=CARTESIAN_POINT ( 'NONE',  ( -5.719274019375665041, -21.55341960407619695, 84.79275706135234714 ) ) ;
#31679=CARTESIAN_POINT ( 'NONE',  ( -5.153800228976328057, -19.02544592524343514, 77.29057627198099567 ) ) ;
#31680=CARTESIAN_POINT ( 'NONE',  ( -9.564922557960796823, -16.46253265017161027, 92.08224293864769550 ) ) ;
#31681=CARTESIAN_POINT ( 'NONE',  ( 16.55341960407611168, 4.379528057220329451, 113.9572429386477239 ) ) ;
#31682=CARTESIAN_POINT ( 'NONE',  ( 8.314922557960818139, 14.29746914071049879, 79.58224293864769550 ) ) ;
#31683=CARTESIAN_POINT ( 'NONE',  ( -5.823673210054116645, -21.52544592524344225, 82.29057627198103830 ) ) ;
#31684=CARTESIAN_POINT ( 'NONE',  ( 19.03943276465977164, -0.05219959533909143690, 68.74890960531436690 ) ) ;
#31685=CARTESIAN_POINT ( 'NONE',  ( -15.72974639402197994, 15.80617190586746368, 85.62390960531436690 ) ) ;
#31686=CARTESIAN_POINT ( 'NONE',  ( -0.05219959533936034679, 19.03943276465977164, 82.50109039468567573 ) ) ;
#31688=CARTESIAN_POINT ( 'NONE',  ( 16.55341960407611168, 4.379528057220329451, 88.95724293864769550 ) ) ;
#31689=CARTESIAN_POINT ( 'NONE',  ( 19.03943276465977164, -0.05219959533909143690, 58.74890960531435979 ) ) ;
#31690=CARTESIAN_POINT ( 'NONE',  ( 21.55341960407610458, 5.719274019375980345, 63.95724293864770260 ) ) ;
#31692=CARTESIAN_POINT ( 'NONE',  ( -12.14591786802326823, 12.06949235617739902, 108.1260903946856757 ) ) ;
#31694=CARTESIAN_POINT ( 'NONE',  ( -5.153800228976607833, 19.02544592524334988, 112.7094237280190043 ) ) ;
#31695=CARTESIAN_POINT ( 'NONE',  ( 16.53943276465976808, -0.05219959533910856209, 83.74890960531435269 ) ) ;
#31697=CARTESIAN_POINT ( 'NONE',  ( 9.564922557960805705, 16.46253265017160317, 79.58224293864769550 ) ) ;
#31698=CARTESIAN_POINT ( 'NONE',  ( 0.05219959533909260263, 19.03943276465977164, 29.99890960531435979 ) ) ;
#31699=CARTESIAN_POINT ( 'NONE',  ( -16.52544592524342804, 4.483927247898546575, 71.04057627198103830 ) ) ;
#31700=CARTESIAN_POINT ( 'NONE',  ( -16.46253265017160317, 9.564922557960807481, 115.8322429386477097 ) ) ;
#31701=CARTESIAN_POINT ( 'NONE',  ( 19.05341960407617918, -5.049401038297876454, 86.04275706135233293 ) ) ;
#31702=CARTESIAN_POINT ( 'NONE',  ( 5.153800228976335163, 19.02544592524342804, 74.79057627198103830 ) ) ;
#31703=CARTESIAN_POINT ( 'NONE',  ( -9.474510206698964154, 16.51473224551069663, 90.41557627198103830 ) ) ;
#31704=CARTESIAN_POINT ( 'NONE',  ( 15.80617190586746368, 15.72974639402197994, 74.37390960531436690 ) ) ;
#31705=CARTESIAN_POINT ( 'NONE',  ( -8.314922557961024197, 14.29746914071037800, 67.91775706135234714 ) ) ;
#31706=CARTESIAN_POINT ( 'NONE',  ( -17.31747979337959009, 6.344076630960794994, 93.62055131934819485 ) ) ;
#31707=CARTESIAN_POINT ( 'NONE',  ( 0.05219959533909260263, 19.03943276465977164, 59.99890960531436690 ) ) ;
#31708=CARTESIAN_POINT ( 'NONE',  ( -21.53943276465977519, 0.05219959533907696930, 71.24890960531435269 ) ) ;
#31709=CARTESIAN_POINT ( 'NONE',  ( 0.05219959533936267826, -19.03943276465977164, 100.0010903946856757 ) ) ;
#31710=CARTESIAN_POINT ( 'NONE',  ( 16.52544592524342804, -4.483927247898539470, 33.54057627198102409 ) ) ;
#31711=CARTESIAN_POINT ( 'NONE',  ( -18.62759615963255300, -10.81492255796106328, 44.16775706135234714 ) ) ;
#31713=CARTESIAN_POINT ( 'NONE',  ( 12.14591786802327356, -12.06949235617739191, 70.62609039468567573 ) ) ;
#31714=CARTESIAN_POINT ( 'NONE',  ( 5.153800228976335163, 19.02544592524342804, 99.79057627198102409 ) ) ;
#31717=CARTESIAN_POINT ( 'NONE',  ( -16.55341960407617563, 4.379528057220093196, 93.54275706135234714 ) ) ;
#31718=CARTESIAN_POINT ( 'NONE',  ( 14.34966873604972726, -8.224510206698740333, 50.83442372801901143 ) ) ;
#31719=CARTESIAN_POINT ( 'NONE',  ( 9.474510206698971260, -16.51473224551069308, 57.91557627198103120 ) ) ;
#31720=CARTESIAN_POINT ( 'NONE',  ( 19.05341960407611168, 5.049401038298154454, 68.95724293864769550 ) ) ;
#31721=CARTESIAN_POINT ( 'NONE',  ( -18.62759615963255300, -10.81492255796106328, 59.16775706135234714 ) ) ;
#31722=CARTESIAN_POINT ( 'NONE',  ( -14.34966873604972548, 8.224510206698743886, 63.33442372801900433 ) ) ;
#31723=CARTESIAN_POINT ( 'NONE',  ( 14.29746914071049879, -8.314922557960816363, 38.33224293864768839 ) ) ;
#31724=CARTESIAN_POINT ( 'NONE',  ( -16.46253265017160317, 9.564922557960807481, 45.83224293864769550 ) ) ;
#31725=CARTESIAN_POINT ( 'NONE',  ( 16.51473224551069308, 9.474510206698969483, 29.16557627198103475 ) ) ;
#31726=CARTESIAN_POINT ( 'NONE',  ( -8.224510206698735004, -14.34966873604973081, 24.58442372801901499 ) ) ;
#31727=ORIENTED_EDGE ( 'NONE', *, *, #198449, .T. ) ;
#31728=CARTESIAN_POINT ( 'NONE',  ( 0.05219959533936267826, -19.03943276465977164, 85.00109039468567573 ) ) ;
#31729=CARTESIAN_POINT ( 'NONE',  ( -14.29746914071049879, 8.314922557960819915, 85.83224293864768129 ) ) ;
#31730=CARTESIAN_POINT ( 'NONE',  ( 9.474510206698971260, -16.51473224551069308, 47.91557627198102409 ) ) ;
#31731=CARTESIAN_POINT ( 'NONE',  ( 13.89961937509957401, 13.97604488694547697, 86.87609039468567573 ) ) ;
#31732=CARTESIAN_POINT ( 'NONE',  ( -18.22780087662119541, 5.500000000000102141, 56.01763182126894947 ) ) ;
#31733=CARTESIAN_POINT ( 'NONE',  ( 5.719274019375673035, 21.55341960407619339, 87.29275706135236135 ) ) ;
#31734=CARTESIAN_POINT ( 'NONE',  ( -0.05219959533934338120, 16.53943276465976808, 47.50109039468568994 ) ) ;
#31735=CARTESIAN_POINT ( 'NONE',  ( -17.50000000000013145, 3.292511757969945663, 25.06520270210549839 ) ) ;
#31736=CARTESIAN_POINT ( 'NONE',  ( 21.55341960407610458, 5.719274019375980345, 48.95724293864770971 ) ) ;
#31737=CARTESIAN_POINT ( 'NONE',  ( -16.55341960407617563, 4.379528057220093196, 43.54275706135235424 ) ) ;
#31738=CARTESIAN_POINT ( 'NONE',  ( 9.474510206698971260, -16.51473224551069308, 32.91557627198102409 ) ) ;
#31739=CARTESIAN_POINT ( 'NONE',  ( -19.02544592524334988, -5.153800228976617603, 43.95942372801899012 ) ) ;
#31740=CARTESIAN_POINT ( 'NONE',  ( -5.153800228976328057, -19.02544592524343514, 82.29057627198103830 ) ) ;
#31741=CARTESIAN_POINT ( 'NONE',  ( 19.03943276465977164, -0.05219959533909143690, 53.74890960531436690 ) ) ;
#31742=CARTESIAN_POINT ( 'NONE',  ( 20.49784845243110709, -5.510910596163089556E-15, 45.00000000000000000 ) ) ;
#31743=CARTESIAN_POINT ( 'NONE',  ( 19.02544592524343514, -5.153800228976328945, 63.54057627198103830 ) ) ;
#31744=CARTESIAN_POINT ( 'NONE',  ( -0.05219959533909027116, -19.03943276465977164, 92.49890960531436690 ) ) ;
#31745=CARTESIAN_POINT ( 'NONE',  ( 19.05341960407617918, -5.049401038297876454, 31.04275706135232227 ) ) ;
#31746=CARTESIAN_POINT ( 'NONE',  ( 5.153800228976615827, -19.02544592524334988, 20.20942372801899722 ) ) ;
#31747=CARTESIAN_POINT ( 'NONE',  ( -16.55341960407611168, -4.379528057220339221, 36.45724293864768839 ) ) ;
#31748=CARTESIAN_POINT ( 'NONE',  ( 19.05341960407611168, 5.049401038298154454, 48.95724293864768129 ) ) ;
#31749=CARTESIAN_POINT ( 'NONE',  ( -9.564922557960796823, -16.46253265017161027, 102.0822429386477097 ) ) ;
#31750=CARTESIAN_POINT ( 'NONE',  ( -15.72974639402176322, -15.80617190586768395, 89.37609039468568994 ) ) ;
#31751=CARTESIAN_POINT ( 'NONE',  ( 16.46253265017160672, -9.564922557960803928, 48.33224293864769550 ) ) ;
#31752=CARTESIAN_POINT ( 'NONE',  ( -21.55341960407619339, 5.719274019375674811, 83.54275706135234714 ) ) ;
#31753=CARTESIAN_POINT ( 'NONE',  ( -5.823673210054116645, -21.52544592524344225, 27.29057627198103120 ) ) ;
#31754=CARTESIAN_POINT ( 'NONE',  ( -10.72451020669870658, -18.67979575497194134, 19.58442372801901143 ) ) ;
#31755=CARTESIAN_POINT ( 'NONE',  ( 5.153800228976615827, -19.02544592524334988, 45.20942372801901143 ) ) ;
#31756=CARTESIAN_POINT ( 'NONE',  ( 13.97604488694527802, 13.89961937509977652, 29.37390960531435979 ) ) ;
#31757=CARTESIAN_POINT ( 'NONE',  ( -19.03943276465977164, 0.05219959533909376836, 76.24890960531435269 ) ) ;
#31758=CARTESIAN_POINT ( 'NONE',  ( 8.224510206698742110, 14.34966873604972548, 22.08442372801901143 ) ) ;
#31759=CARTESIAN_POINT ( 'NONE',  ( 12.14591786802309770, 12.06949235617756955, 89.37390960531435269 ) ) ;
#31760=CARTESIAN_POINT ( 'NONE',  ( 10.72451020669898902, -18.67979575497178502, 42.91557627198103120 ) ) ;
#31761=CARTESIAN_POINT ( 'NONE',  ( 13.97604488694548053, -13.89961937509957401, 95.62609039468563310 ) ) ;
#31762=CARTESIAN_POINT ( 'NONE',  ( 21.52544592524344225, -5.823673210054117533, 103.5405762719810383 ) ) ;
#31763=CARTESIAN_POINT ( 'NONE',  ( -10.81492255796105439, 18.62759615963255655, 62.91775706135236135 ) ) ;
#31764=CARTESIAN_POINT ( 'NONE',  ( 8.224510206698742110, 14.34966873604972548, 52.08442372801901854 ) ) ;
#31765=CARTESIAN_POINT ( 'NONE',  ( -14.29746914071037622, -8.314922557961029526, 69.16775706135234714 ) ) ;
#31766=CARTESIAN_POINT ( 'NONE',  ( -19.05341960407611168, -5.049401038298163336, 56.45724293864768129 ) ) ;
#31767=CARTESIAN_POINT ( 'NONE',  ( 12.06949235617739724, 12.14591786802326823, 86.87609039468568994 ) ) ;
#31769=CARTESIAN_POINT ( 'NONE',  ( -10.81492255796105439, 18.62759615963255655, 22.91775706135235069 ) ) ;
#31770=CARTESIAN_POINT ( 'NONE',  ( -8.224510206698948167, 14.34966873604960824, 55.41557627198102409 ) ) ;
#31771=CARTESIAN_POINT ( 'NONE',  ( -13.89961937509977652, 13.97604488694528158, 90.62390960531432427 ) ) ;
#31772=CARTESIAN_POINT ( 'NONE',  ( 4.483927247898790824, -16.52544592524335698, 70.20942372801904696 ) ) ;
#31773=CARTESIAN_POINT ( 'NONE',  ( -15.72974639402176322, -15.80617190586768395, 64.37609039468568994 ) ) ;
#31774=CARTESIAN_POINT ( 'NONE',  ( -16.51473224551082808, 9.474510206698731452, 108.3344237280190043 ) ) ;
#31775=CARTESIAN_POINT ( 'NONE',  ( -21.55341960407610458, -5.719274019375992779, 106.4572429386477097 ) ) ;
#31776=CARTESIAN_POINT ( 'NONE',  ( 16.53943276465976808, -0.05219959533910856209, 48.74890960531435979 ) ) ;
#31778=CARTESIAN_POINT ( 'NONE',  ( -17.05587630539787014, 6.762274262135696823, 75.74180309037312497 ) ) ;
#31779=CARTESIAN_POINT ( 'NONE',  ( 5.823673210054125526, 21.52544592524343514, 89.79057627198103830 ) ) ;
#31780=CARTESIAN_POINT ( 'NONE',  ( -16.53943276465976808, 0.05219959533911058130, 21.24890960531436690 ) ) ;
#31783=CARTESIAN_POINT ( 'NONE',  ( -21.53943276465977519, 0.05219959533907696930, 116.2489096053143669 ) ) ;
#31784=CARTESIAN_POINT ( 'NONE',  ( -13.97604488694527625, -13.89961937509977652, 111.8739096053143243 ) ) ;
#31785=CARTESIAN_POINT ( 'NONE',  ( 5.823673210054444382, -21.52544592524334988, 30.20942372801902565 ) ) ;
#31786=CARTESIAN_POINT ( 'NONE',  ( -16.52544592524342804, 4.483927247898546575, 51.04057627198103120 ) ) ;
#31787=CARTESIAN_POINT ( 'NONE',  ( 12.14591786802327356, -12.06949235617739191, 65.62609039468568994 ) ) ;
#31788=CARTESIAN_POINT ( 'NONE',  ( -19.03943276465977164, 0.05219959533909376836, 66.24890960531436690 ) ) ;
#31789=CARTESIAN_POINT ( 'NONE',  ( -5.153800228976607833, 19.02544592524334988, 62.70942372801899722 ) ) ;
#31790=CARTESIAN_POINT ( 'NONE',  ( -19.02544592524342804, 5.153800228976336051, 86.04057627198103830 ) ) ;
#31791=CARTESIAN_POINT ( 'NONE',  ( 18.62759615963271287, -10.81492255796078972, 33.33224293864769550 ) ) ;
#31793=CARTESIAN_POINT ( 'NONE',  ( -9.474510206698964154, 16.51473224551069663, 55.41557627198103120 ) ) ;
#31794=CARTESIAN_POINT ( 'NONE',  ( 0.05219959533934541429, -16.53943276465976808, 30.00109039468568284 ) ) ;
#31795=CARTESIAN_POINT ( 'NONE',  ( 16.51473224551083163, -9.474510206698727899, 60.83442372801900433 ) ) ;
#31796=CARTESIAN_POINT ( 'NONE',  ( 0.05219959533907565091, 21.53943276465977519, 99.99890960531436690 ) ) ;
#31797=CARTESIAN_POINT ( 'NONE',  ( 16.55341960407611168, 4.379528057220329451, 28.95724293864769905 ) ) ;
#31798=CARTESIAN_POINT ( 'NONE',  ( 9.564922557960805705, 16.46253265017160317, 94.58224293864769550 ) ) ;
#31799=CARTESIAN_POINT ( 'NONE',  ( 0.05219959533907565091, 21.53943276465977519, 59.99890960531436690 ) ) ;
#31800=CARTESIAN_POINT ( 'NONE',  ( 21.53943276465977519, -0.05219959533907433946, 93.74890960531436690 ) ) ;
#31801=CARTESIAN_POINT ( 'NONE',  ( 8.314922557961029526, -14.29746914071037800, 35.41775706135234003 ) ) ;
#31802=CARTESIAN_POINT ( 'NONE',  ( 21.53943276465977519, -0.05219959533907433946, 33.74890960531436690 ) ) ;
#31803=CARTESIAN_POINT ( 'NONE',  ( -5.719274019375665041, -21.55341960407619695, 94.79275706135234714 ) ) ;
#31804=CARTESIAN_POINT ( 'NONE',  ( -13.97604488694527625, -13.89961937509977652, 91.87390960531432427 ) ) ;
#31805=CARTESIAN_POINT ( 'NONE',  ( 9.564922557960805705, 16.46253265017160317, 39.58224293864768839 ) ) ;
#31806=CARTESIAN_POINT ( 'NONE',  ( -16.51473224551069308, -9.474510206698971260, 86.66557627198102409 ) ) ;
#31807=CARTESIAN_POINT ( 'NONE',  ( -12.14591786802309592, -12.06949235617757132, 101.8739096053143811 ) ) ;
#31808=CARTESIAN_POINT ( 'NONE',  ( 19.02544592524343514, -5.153800228976328945, 58.54057627198102409 ) ) ;
#31809=CARTESIAN_POINT ( 'NONE',  ( 4.379528057220092307, 16.55341960407617563, 27.29275706135234358 ) ) ;
#31810=CARTESIAN_POINT ( 'NONE',  ( -16.51473224551082808, 9.474510206698731452, 43.33442372801900433 ) ) ;
#31811=CARTESIAN_POINT ( 'NONE',  ( -0.05219959533937732626, 21.53943276465977519, 97.50109039468567573 ) ) ;
#31812=CARTESIAN_POINT ( 'NONE',  ( 16.51473224551069308, 9.474510206698969483, 109.1655762719810383 ) ) ;
#31813=CARTESIAN_POINT ( 'NONE',  ( 12.14591786802327356, -12.06949235617739191, 95.62609039468568994 ) ) ;
#31815=CARTESIAN_POINT ( 'NONE',  ( -13.89961937509957401, -13.97604488694547875, 74.37609039468566152 ) ) ;
#31816=CARTESIAN_POINT ( 'NONE',  ( 16.51473224551083163, -9.474510206698727899, 30.83442372801900433 ) ) ;
#31818=CARTESIAN_POINT ( 'NONE',  ( -9.474510206698964154, 16.51473224551069663, 25.41557627198103120 ) ) ;
#31819=CARTESIAN_POINT ( 'NONE',  ( 16.55341960407611168, 4.379528057220329451, 38.95724293864768839 ) ) ;
#31821=CARTESIAN_POINT ( 'NONE',  ( -16.31925111598457434, -7.325300261831539039, 109.8357546103274700 ) ) ;
#31822=CARTESIAN_POINT ( 'NONE',  ( 12.06949235617757843, -12.14591786802309237, 28.12390960531435979 ) ) ;
#31824=CARTESIAN_POINT ( 'NONE',  ( -16.55341960407617563, 4.379528057220093196, 98.54275706135234714 ) ) ;
#31825=CARTESIAN_POINT ( 'NONE',  ( 19.03943276465977164, -0.05219959533909143690, 38.74890960531436690 ) ) ;
#31826=CARTESIAN_POINT ( 'NONE',  ( -5.823673210054431948, 21.52544592524334988, 92.70942372801901854 ) ) ;
#31827=CARTESIAN_POINT ( 'NONE',  ( -13.97604488694547697, 13.89961937509957934, 113.1260903946856757 ) ) ;
#31828=CARTESIAN_POINT ( 'NONE',  ( -10.72451020669870658, -18.67979575497194134, 74.58442372801901854 ) ) ;
#31829=CARTESIAN_POINT ( 'NONE',  ( -19.05341960407617563, 5.049401038297882671, 48.54275706135233293 ) ) ;
#31830=CARTESIAN_POINT ( 'NONE',  ( -5.049401038298153566, 19.05341960407611168, 90.20724293864766707 ) ) ;
#31831=CARTESIAN_POINT ( 'NONE',  ( -9.564922557960796823, -16.46253265017161027, 77.08224293864769550 ) ) ;
#31832=LINE ( 'NONE', #3461, #7749 ) ;
#31833=CARTESIAN_POINT ( 'NONE',  ( -21.52544592524343514, 5.823673210054127303, 91.04057627198103830 ) ) ;
#31834=CARTESIAN_POINT ( 'NONE',  ( -4.379528057220328563, 16.55341960407611168, 60.20724293864768839 ) ) ;
#31835=CARTESIAN_POINT ( 'NONE',  ( -5.823673210054116645, -21.52544592524344225, 62.29057627198102409 ) ) ;
#31836=CARTESIAN_POINT ( 'NONE',  ( 13.89961937509977652, -13.97604488694527269, 63.12390960531435979 ) ) ;
#31837=CARTESIAN_POINT ( 'NONE',  ( -5.823673210054116645, -21.52544592524344225, 87.29057627198103830 ) ) ;
#31838=CARTESIAN_POINT ( 'NONE',  ( 16.53943276465976808, 0.05219959533934440121, 81.25109039468568994 ) ) ;
#31840=CARTESIAN_POINT ( 'NONE',  ( -16.46253265017160317, 9.564922557960807481, 40.83224293864769550 ) ) ;
#31841=CARTESIAN_POINT ( 'NONE',  ( 16.52544592524342804, -4.483927247898539470, 78.54057627198103830 ) ) ;
#31843=CARTESIAN_POINT ( 'NONE',  ( -13.89961937509977652, 13.97604488694528158, 50.62390960531435979 ) ) ;
#31844=CARTESIAN_POINT ( 'NONE',  ( -4.483927247898539470, -16.52544592524342804, 112.2905762719810241 ) ) ;
#31845=CARTESIAN_POINT ( 'NONE',  ( 9.564922557961047289, -16.46253265017146816, 60.41775706135233293 ) ) ;
#31846=CARTESIAN_POINT ( 'NONE',  ( -12.06949235617756955, 12.14591786802309770, 90.62390960531436690 ) ) ;
#31847=CARTESIAN_POINT ( 'NONE',  ( 10.72451020669871369, 18.67979575497193778, 42.08442372801901854 ) ) ;
#31848=CARTESIAN_POINT ( 'NONE',  ( -19.03943276465977164, 0.05219959533909376836, 36.24890960531436690 ) ) ;
#31849=CARTESIAN_POINT ( 'NONE',  ( 0.05219959533907565091, 21.53943276465977519, 99.99890960531436690 ) ) ;
#31850=CARTESIAN_POINT ( 'NONE',  ( -16.55341960407611168, -4.379528057220339221, 86.45724293864770971 ) ) ;
#31852=CARTESIAN_POINT ( 'NONE',  ( -0.05219959533909027116, -19.03943276465977164, 47.49890960531435979 ) ) ;
#31853=CARTESIAN_POINT ( 'NONE',  ( 17.49999999999998224, 5.622605283950877109, 113.8120731059611188 ) ) ;
#31854=CARTESIAN_POINT ( 'NONE',  ( 16.46253265017146816, 9.564922557961045513, 91.66775706135234714 ) ) ;
#31855=CARTESIAN_POINT ( 'NONE',  ( -5.153800228976328057, -19.02544592524343514, 97.29057627198099567 ) ) ;
#31856=CARTESIAN_POINT ( 'NONE',  ( 5.719274019375673035, 21.55341960407619339, 42.29275706135235424 ) ) ;
#31857=CARTESIAN_POINT ( 'NONE',  ( -5.153800228976328057, -19.02544592524343514, 87.29057627198103830 ) ) ;
#31858=CARTESIAN_POINT ( 'NONE',  ( -5.153800228976607833, 19.02544592524334988, 67.70942372801900433 ) ) ;
#31859=CARTESIAN_POINT ( 'NONE',  ( 9.564922557960805705, 16.46253265017160317, 49.58224293864770260 ) ) ;
#31860=CARTESIAN_POINT ( 'NONE',  ( -14.29746914071049879, 8.314922557960819915, 75.83224293864769550 ) ) ;
#31861=CARTESIAN_POINT ( 'NONE',  ( -4.379528057220328563, 16.55341960407611168, 70.20724293864769550 ) ) ;
#31862=CARTESIAN_POINT ( 'NONE',  ( 5.153800228976335163, 19.02544592524342804, 79.79057627198102409 ) ) ;
#31863=CARTESIAN_POINT ( 'NONE',  ( 5.823673210054125526, 21.52544592524343514, 94.79057627198105251 ) ) ;
#31864=CARTESIAN_POINT ( 'NONE',  ( 19.05341960407611168, 5.049401038298154454, 68.95724293864769550 ) ) ;
#31865=CARTESIAN_POINT ( 'NONE',  ( 13.97604488694548053, -13.89961937509957401, 35.62609039468567573 ) ) ;
#31866=CARTESIAN_POINT ( 'NONE',  ( 5.049401038298161559, -19.05341960407611168, 32.70724293864768129 ) ) ;
#31867=CARTESIAN_POINT ( 'NONE',  ( 14.29746914071049879, -8.314922557960816363, 33.33224293864769550 ) ) ;
#31868=CARTESIAN_POINT ( 'NONE',  ( -16.52544592524342804, 4.483927247898546575, 111.0405762719810525 ) ) ;
#31869=CARTESIAN_POINT ( 'NONE',  ( -16.46253265017146816, -9.564922557961047289, 104.1677570613523329 ) ) ;
#31871=CARTESIAN_POINT ( 'NONE',  ( 5.719274019375673035, 21.55341960407619339, 27.29275706135234358 ) ) ;
#31872=CARTESIAN_POINT ( 'NONE',  ( 16.46253265017146816, 9.564922557961045513, 66.66775706135233293 ) ) ;
#31873=CARTESIAN_POINT ( 'NONE',  ( -4.483927247898539470, -16.52544592524342804, 22.29057627198102765 ) ) ;
#31874=CARTESIAN_POINT ( 'NONE',  ( -5.823673210054116645, -21.52544592524344225, 82.29057627198103830 ) ) ;
#31875=CARTESIAN_POINT ( 'NONE',  ( -21.55341960407610458, -5.719274019375992779, 26.45724293864768839 ) ) ;
#31876=CARTESIAN_POINT ( 'NONE',  ( 12.14591786802309770, 12.06949235617756955, 59.37390960531436690 ) ) ;
#31877=CARTESIAN_POINT ( 'NONE',  ( -9.474510206698964154, 16.51473224551069663, 35.41557627198102409 ) ) ;
#31878=CARTESIAN_POINT ( 'NONE',  ( 19.05341960407617918, -5.049401038297876454, 31.04275706135232227 ) ) ;
#31879=CARTESIAN_POINT ( 'NONE',  ( -12.06949235617739369, -12.14591786802326823, 84.37609039468570415 ) ) ;
#31880=CARTESIAN_POINT ( 'NONE',  ( 12.14591786802327356, -12.06949235617739191, 55.62609039468568284 ) ) ;
#31881=CARTESIAN_POINT ( 'NONE',  ( -18.67979575497178146, -10.72451020669898902, 26.66557627198103475 ) ) ;
#31882=CARTESIAN_POINT ( 'NONE',  ( 18.62759615963255655, 10.81492255796105972, 106.6677570613523756 ) ) ;
#31883=CARTESIAN_POINT ( 'NONE',  ( 0.05219959533909260263, 19.03943276465977164, 84.99890960531436690 ) ) ;
#31884=CARTESIAN_POINT ( 'NONE',  ( -8.224510206698735004, -14.34966873604973081, 54.58442372801901143 ) ) ;
#31885=CARTESIAN_POINT ( 'NONE',  ( 0.05219959533909260263, 19.03943276465977164, 24.99890960531435269 ) ) ;
#31886=CARTESIAN_POINT ( 'NONE',  ( 12.06949235617757843, -12.14591786802309237, 33.12390960531435979 ) ) ;
#31888=CARTESIAN_POINT ( 'NONE',  ( -5.719274019375665041, -21.55341960407619695, 69.79275706135234714 ) ) ;
#31889=CARTESIAN_POINT ( 'NONE',  ( -19.02544592524342804, 5.153800228976336051, 96.04057627198103830 ) ) ;
#31890=CARTESIAN_POINT ( 'NONE',  ( 9.564922557960805705, 16.46253265017160317, 74.58224293864769550 ) ) ;
#31891=CARTESIAN_POINT ( 'NONE',  ( -13.89961937509977652, 13.97604488694528158, 105.6239096053143527 ) ) ;
#31892=CARTESIAN_POINT ( 'NONE',  ( -4.483927247898539470, -16.52544592524342804, 52.29057627198102409 ) ) ;
#31893=CARTESIAN_POINT ( 'NONE',  ( -12.14591786802309592, -12.06949235617757132, 31.87390960531435979 ) ) ;
#31895=CARTESIAN_POINT ( 'NONE',  ( -16.53943276465976808, 0.05219959533911058130, 51.24890960531436690 ) ) ;
#31896=CARTESIAN_POINT ( 'NONE',  ( 8.224510206698742110, 14.34966873604972548, 37.08442372801901143 ) ) ;
#31898=CARTESIAN_POINT ( 'NONE',  ( 9.564922557961047289, -16.46253265017146816, 45.41775706135232582 ) ) ;
#31899=CARTESIAN_POINT ( 'NONE',  ( -5.049401038298153566, 19.05341960407611168, 70.20724293864769550 ) ) ;
#31900=CARTESIAN_POINT ( 'NONE',  ( 5.049401038297881783, 19.05341960407617563, 47.29275706135231161 ) ) ;
#31901=CARTESIAN_POINT ( 'NONE',  ( 19.02544592524334988, 5.153800228976608722, 51.45942372801900433 ) ) ;
#31902=CARTESIAN_POINT ( 'NONE',  ( 16.46253265017146816, 9.564922557961045513, 91.66775706135234714 ) ) ;
#31903=CARTESIAN_POINT ( 'NONE',  ( 14.29746914071037800, 8.314922557961029526, 86.66775706135234714 ) ) ;
#31905=CARTESIAN_POINT ( 'NONE',  ( 13.89961937509977652, -13.97604488694527269, 28.12390960531435624 ) ) ;
#31906=CARTESIAN_POINT ( 'NONE',  ( -13.89961937509977652, 13.97604488694528158, 110.6239096053143243 ) ) ;
#31907=CARTESIAN_POINT ( 'NONE',  ( -18.67979575497193778, 10.72451020669871902, 38.33442372801900433 ) ) ;
#31908=CARTESIAN_POINT ( 'NONE',  ( 19.05341960407617918, -5.049401038297876454, 86.04275706135233293 ) ) ;
#31910=CARTESIAN_POINT ( 'NONE',  ( -0.05219959533909027116, -19.03943276465977164, 67.49890960531436690 ) ) ;
#31911=CARTESIAN_POINT ( 'NONE',  ( 19.02544592524343514, -5.153800228976328945, 103.5405762719809957 ) ) ;
#31912=CARTESIAN_POINT ( 'NONE',  ( -8.314922557960811034, -14.29746914071050412, 62.08224293864769550 ) ) ;
#31913=CARTESIAN_POINT ( 'NONE',  ( -19.03943276465977164, 0.05219959533909376836, 61.24890960531436690 ) ) ;
#31914=CARTESIAN_POINT ( 'NONE',  ( 19.03943276465977164, -0.05219959533909143690, 58.74890960531435979 ) ) ;
#31915=CARTESIAN_POINT ( 'NONE',  ( 16.46253265017146816, 9.564922557961045513, 81.66775706135233293 ) ) ;
#31916=CARTESIAN_POINT ( 'NONE',  ( -18.67979575497178146, -10.72451020669898902, 46.66557627198102409 ) ) ;
#31917=CARTESIAN_POINT ( 'NONE',  ( -19.03943276465977164, -0.05219959533935918106, 48.75109039468566863 ) ) ;
#31918=CARTESIAN_POINT ( 'NONE',  ( -9.564922557960796823, -16.46253265017161027, 77.08224293864769550 ) ) ;
#31919=CARTESIAN_POINT ( 'NONE',  ( 10.72451020669898902, -18.67979575497178502, 82.91557627198103830 ) ) ;
#31920=CARTESIAN_POINT ( 'NONE',  ( -14.29746914071049879, 8.314922557960819915, 80.83224293864769550 ) ) ;
#31921=CARTESIAN_POINT ( 'NONE',  ( 16.51473224551083163, -9.474510206698727899, 35.83442372801899722 ) ) ;
#31922=CARTESIAN_POINT ( 'NONE',  ( -18.67979575497178146, -10.72451020669898902, 41.66557627198103120 ) ) ;
#31923=CARTESIAN_POINT ( 'NONE',  ( -10.72451020669898014, 18.67979575497178502, 40.41557627198103120 ) ) ;
#31924=CARTESIAN_POINT ( 'NONE',  ( 16.46253265017160672, -9.564922557960803928, 68.33224293864770971 ) ) ;
#31925=CARTESIAN_POINT ( 'NONE',  ( 5.153800228976335163, 19.02544592524342804, 54.79057627198103120 ) ) ;
#31926=CARTESIAN_POINT ( 'NONE',  ( 16.55341960407611168, 4.379528057220329451, 108.9572429386476955 ) ) ;
#31927=CARTESIAN_POINT ( 'NONE',  ( 10.81492255796106328, -18.62759615963255655, 30.41775706135234358 ) ) ;
#31928=CARTESIAN_POINT ( 'NONE',  ( -16.46253265017160317, 9.564922557960807481, 110.8322429386476955 ) ) ;
#31929=CARTESIAN_POINT ( 'NONE',  ( 18.62759615963255655, 10.81492255796105972, 36.66775706135234714 ) ) ;
#31930=CARTESIAN_POINT ( 'NONE',  ( 16.51473224551069308, 9.474510206698969483, 34.16557627198102409 ) ) ;
#31931=CARTESIAN_POINT ( 'NONE',  ( -21.52544592524343514, 5.823673210054127303, 111.0405762719810525 ) ) ;
#31932=CARTESIAN_POINT ( 'NONE',  ( -9.564922557961040184, 16.46253265017147172, 52.91775706135233293 ) ) ;
#31933=CARTESIAN_POINT ( 'NONE',  ( 17.97182807773871360, -5.500000000000043521, 76.03038844047287625 ) ) ;
#31936=CARTESIAN_POINT ( 'NONE',  ( -16.52544592524335698, -4.483927247898792601, 53.95942372801900433 ) ) ;
#31937=CARTESIAN_POINT ( 'NONE',  ( -0.05219959533909027116, -19.03943276465977164, 32.49890960531435979 ) ) ;
#31939=CARTESIAN_POINT ( 'NONE',  ( -9.564922557960796823, -16.46253265017161027, 67.08224293864769550 ) ) ;
#31940=CARTESIAN_POINT ( 'NONE',  ( 14.29746914071049879, -8.314922557960816363, 108.3322429386477097 ) ) ;
#31941=CARTESIAN_POINT ( 'NONE',  ( -15.72974639402197994, 15.80617190586746368, 65.62390960531436690 ) ) ;
#31942=CARTESIAN_POINT ( 'NONE',  ( -16.53943276465976808, 0.05219959533911058130, 81.24890960531436690 ) ) ;
#31943=CARTESIAN_POINT ( 'NONE',  ( 16.53943276465976808, 0.05219959533934440121, 31.25109039468568639 ) ) ;
#31944=CARTESIAN_POINT ( 'NONE',  ( 15.80617190586769283, -15.72974639402175789, 85.62609039468568994 ) ) ;
#31945=CARTESIAN_POINT ( 'NONE',  ( -16.51473224551069308, -9.474510206698971260, 31.66557627198102054 ) ) ;
#31946=CARTESIAN_POINT ( 'NONE',  ( -8.314922557960811034, -14.29746914071050412, 22.08224293864769194 ) ) ;
#31947=CARTESIAN_POINT ( 'NONE',  ( -4.483927247898539470, -16.52544592524342804, 52.29057627198102409 ) ) ;
#31948=CARTESIAN_POINT ( 'NONE',  ( -19.05341960407611168, -5.049401038298163336, 56.45724293864768129 ) ) ;
#31949=CARTESIAN_POINT ( 'NONE',  ( 10.81492255796106328, -18.62759615963255655, 95.41775706135234714 ) ) ;
#31950=CARTESIAN_POINT ( 'NONE',  ( 10.72451020669898902, -18.67979575497178502, 102.9155762719810383 ) ) ;
#31951=CARTESIAN_POINT ( 'NONE',  ( -15.72974639402176322, -15.80617190586768395, 79.37609039468567573 ) ) ;
#31952=CARTESIAN_POINT ( 'NONE',  ( -0.05219959533934338120, 16.53943276465976808, 47.50109039468568994 ) ) ;
#31953=CARTESIAN_POINT ( 'NONE',  ( -4.483927247898539470, -16.52544592524342804, 72.29057627198102409 ) ) ;
#31954=CARTESIAN_POINT ( 'NONE',  ( -10.72451020669870658, -18.67979575497194134, 79.58442372801903275 ) ) ;
#31955=CARTESIAN_POINT ( 'NONE',  ( -4.379528057220328563, 16.55341960407611168, 25.20724293864769550 ) ) ;
#31956=CARTESIAN_POINT ( 'NONE',  ( -17.49999999999999645, 5.499999999999996447, 113.7176903769643417 ) ) ;
#31957=CARTESIAN_POINT ( 'NONE',  ( -16.55341960407617563, 4.379528057220093196, 43.54275706135235424 ) ) ;
#31958=CARTESIAN_POINT ( 'NONE',  ( -14.34966873604960291, -8.224510206698953496, 41.66557627198103120 ) ) ;
#31959=CARTESIAN_POINT ( 'NONE',  ( -0.05219959533934338120, 16.53943276465976808, 92.50109039468567573 ) ) ;
#31960=CARTESIAN_POINT ( 'NONE',  ( 5.153800228976335163, 19.02544592524342804, 104.7905762719809957 ) ) ;
#31961=CARTESIAN_POINT ( 'NONE',  ( 16.51473224551069308, 9.474510206698969483, 109.1655762719810383 ) ) ;
#31962=CARTESIAN_POINT ( 'NONE',  ( -21.52544592524334988, -5.823673210054445271, 103.9594237280190185 ) ) ;
#31963=CARTESIAN_POINT ( 'NONE',  ( -14.34966873604972548, 8.224510206698743886, 98.33442372801901854 ) ) ;
#31964=CARTESIAN_POINT ( 'NONE',  ( 4.483927247898545687, 16.52544592524342804, 74.79057627198105251 ) ) ;
#31965=CARTESIAN_POINT ( 'NONE',  ( -9.474510206698964154, 16.51473224551069663, 75.41557627198103830 ) ) ;
#31967=CARTESIAN_POINT ( 'NONE',  ( 4.379528057220092307, 16.55341960407617563, 22.29275706135235069 ) ) ;
#31968=CARTESIAN_POINT ( 'NONE',  ( 19.05341960407611168, 5.049401038298154454, 23.95724293864769194 ) ) ;
#31969=CARTESIAN_POINT ( 'NONE',  ( -13.89961937509977652, 13.97604488694528158, 85.62390960531433848 ) ) ;
#31970=CARTESIAN_POINT ( 'NONE',  ( 16.55341960407618274, -4.379528057220086978, 26.04275706135235779 ) ) ;
#31972=CARTESIAN_POINT ( 'NONE',  ( 19.03943276465977164, 0.05219959533936151252, 31.25109039468566863 ) ) ;
#31973=CARTESIAN_POINT ( 'NONE',  ( 16.52544592524335698, 4.483927247898782831, 91.45942372801901854 ) ) ;
#31974=CARTESIAN_POINT ( 'NONE',  ( -16.51473224551082808, 9.474510206698731452, 103.3344237280190043 ) ) ;
#31975=CARTESIAN_POINT ( 'NONE',  ( 19.05341960407611168, 5.049401038298154454, 28.95724293864769550 ) ) ;
#31976=CARTESIAN_POINT ( 'NONE',  ( 12.06949235617739724, 12.14591786802326823, 76.87609039468567573 ) ) ;
#31977=CARTESIAN_POINT ( 'NONE',  ( -12.06949235617739369, -12.14591786802326823, 64.37609039468568994 ) ) ;
#31978=CARTESIAN_POINT ( 'NONE',  ( 9.474510206698729675, 16.51473224551082808, 82.08442372801899012 ) ) ;
#31979=CARTESIAN_POINT ( 'NONE',  ( -21.55341960407619339, 5.719274019375674811, 113.5427570613523756 ) ) ;
#31980=CARTESIAN_POINT ( 'NONE',  ( -19.03943276465977164, 0.05219959533909376836, 46.24890960531435979 ) ) ;
#31981=CARTESIAN_POINT ( 'NONE',  ( 0.05219959533909260263, 19.03943276465977164, 89.99890960531436690 ) ) ;
#31982=CARTESIAN_POINT ( 'NONE',  ( 16.52544592524342804, -4.483927247898539470, 83.54057627198102409 ) ) ;
#31983=CARTESIAN_POINT ( 'NONE',  ( -13.89961937509957401, -13.97604488694547875, 49.37609039468567573 ) ) ;
#31984=CARTESIAN_POINT ( 'NONE',  ( 15.80617190586746368, 15.72974639402197994, 44.37390960531435979 ) ) ;
#31985=CARTESIAN_POINT ( 'NONE',  ( 19.03943276465977164, 0.05219959533936151252, 26.25109039468566507 ) ) ;
#31986=CARTESIAN_POINT ( 'NONE',  ( 13.89961937509977652, -13.97604488694527269, 93.12390960531436690 ) ) ;
#31987=CARTESIAN_POINT ( 'NONE',  ( 18.67979575497178502, 10.72451020669898547, 74.16557627198102409 ) ) ;
#31988=CARTESIAN_POINT ( 'NONE',  ( 9.564922557960805705, 16.46253265017160317, 109.5822429386476955 ) ) ;
#31989=CARTESIAN_POINT ( 'NONE',  ( -9.564922557961040184, 16.46253265017147172, 87.91775706135233293 ) ) ;
#31990=CARTESIAN_POINT ( 'NONE',  ( 16.51473224551069308, 9.474510206698969483, 114.1655762719810241 ) ) ;
#31991=CARTESIAN_POINT ( 'NONE',  ( 13.89961937509957401, 13.97604488694547697, 106.8760903946856757 ) ) ;
#31992=CARTESIAN_POINT ( 'NONE',  ( 19.05341960407611168, 5.049401038298154454, 28.95724293864769550 ) ) ;
#31993=CARTESIAN_POINT ( 'NONE',  ( 0.05219959533909260263, 19.03943276465977164, 99.99890960531436690 ) ) ;
#31994=CARTESIAN_POINT ( 'NONE',  ( -10.72451020669898014, 18.67979575497178502, 70.41557627198102409 ) ) ;
#31996=CARTESIAN_POINT ( 'NONE',  ( 0.05219959533934541429, -16.53943276465976808, 45.00109039468568284 ) ) ;
#31997=CARTESIAN_POINT ( 'NONE',  ( 10.72451020669871369, 18.67979575497193778, 52.08442372801901854 ) ) ;
#31998=CARTESIAN_POINT ( 'NONE',  ( -0.05219959533936034679, 19.03943276465977164, 87.50109039468567573 ) ) ;
#31999=CARTESIAN_POINT ( 'NONE',  ( 15.72974639402176855, 15.80617190586768217, 96.87609039468568994 ) ) ;
#32000=CARTESIAN_POINT ( 'NONE',  ( 4.379528057220092307, 16.55341960407617563, 102.2927570613523613 ) ) ;
#32001=CARTESIAN_POINT ( 'NONE',  ( -9.564922557960796823, -16.46253265017161027, 102.0822429386477097 ) ) ;
#32002=CARTESIAN_POINT ( 'NONE',  ( 0.05219959533910956823, 16.53943276465976808, 89.99890960531438111 ) ) ;
#32003=CARTESIAN_POINT ( 'NONE',  ( -12.14591786802309592, -12.06949235617757132, 36.87390960531435979 ) ) ;
#32004=CARTESIAN_POINT ( 'NONE',  ( -13.97604488694547697, 13.89961937509957934, 68.12609039468563310 ) ) ;
#32005=CARTESIAN_POINT ( 'NONE',  ( -15.80617190586768217, 15.72974639402176855, 63.12609039468568994 ) ) ;
#32006=CARTESIAN_POINT ( 'NONE',  ( -9.564922557961040184, 16.46253265017147172, 22.91775706135233648 ) ) ;
#32007=CARTESIAN_POINT ( 'NONE',  ( -0.05219959533910754901, -16.53943276465976808, 102.4989096053143811 ) ) ;
#32008=CARTESIAN_POINT ( 'NONE',  ( 15.72974639402199770, -15.80617190586745480, 28.12390960531435979 ) ) ;
#32009=CARTESIAN_POINT ( 'NONE',  ( -12.14591786802309592, -12.06949235617757132, 21.87390960531436690 ) ) ;
#32010=CARTESIAN_POINT ( 'NONE',  ( -15.72974639402176322, -15.80617190586768395, 99.37609039468568994 ) ) ;
#32011=CARTESIAN_POINT ( 'NONE',  ( -16.52544592524335698, -4.483927247898792601, 53.95942372801900433 ) ) ;
#32012=CARTESIAN_POINT ( 'NONE',  ( 16.52544592524342804, -4.483927247898539470, 33.54057627198102409 ) ) ;
#32013=CARTESIAN_POINT ( 'NONE',  ( 15.72974639402176855, 15.80617190586768217, 46.87609039468568994 ) ) ;
#32014=CARTESIAN_POINT ( 'NONE',  ( -15.72974639402176322, -15.80617190586768395, 54.37609039468568994 ) ) ;
#32017=CARTESIAN_POINT ( 'NONE',  ( -21.53943276465977519, -0.05219959533937600094, 23.75109039468567929 ) ) ;
#32018=CARTESIAN_POINT ( 'NONE',  ( 14.29746914071049879, -8.314922557960816363, 108.3322429386477097 ) ) ;
#32019=CARTESIAN_POINT ( 'NONE',  ( 19.96322699617727636, 3.697860406115289322, 37.49999999999999289 ) ) ;
#32020=CARTESIAN_POINT ( 'NONE',  ( 12.14591786802309770, 12.06949235617756955, 79.37390960531436690 ) ) ;
#32021=CARTESIAN_POINT ( 'NONE',  ( -16.51473224551069308, -9.474510206698971260, 66.66557627198102409 ) ) ;
#32022=CARTESIAN_POINT ( 'NONE',  ( 8.314922557961029526, -14.29746914071037800, 105.4177570613523613 ) ) ;
#32023=CARTESIAN_POINT ( 'NONE',  ( -15.80617190586745835, -15.72974639402198527, 61.87390960531436690 ) ) ;
#32024=CARTESIAN_POINT ( 'NONE',  ( 14.29746914071049879, -8.314922557960816363, 88.33224293864769550 ) ) ;
#32025=CARTESIAN_POINT ( 'NONE',  ( 21.52544592524344225, -5.823673210054117533, 93.54057627198103830 ) ) ;
#32026=CARTESIAN_POINT ( 'NONE',  ( 9.564922557960805705, 16.46253265017160317, 104.5822429386476955 ) ) ;
#32027=CARTESIAN_POINT ( 'NONE',  ( 19.05341960407611168, 5.049401038298154454, 53.95724293864770260 ) ) ;
#32028=CARTESIAN_POINT ( 'NONE',  ( 0.05219959533936267826, -19.03943276465977164, 105.0010903946856615 ) ) ;
#32029=CARTESIAN_POINT ( 'NONE',  ( 0.05219959533907565091, 21.53943276465977519, 49.99890960531437401 ) ) ;
#32030=CARTESIAN_POINT ( 'NONE',  ( -21.52544592524334988, -5.823673210054445271, 63.95942372801901854 ) ) ;
#32031=B_SPLINE_CURVE_WITH_KNOTS ( 'NONE', 3,
 ( #9577, #147086, #87403, #177436, #54074, #83390, #25757, #69235, #38906, #6548, #132907, #37905, #68227, #23743, #22739, #133916, #55069, #53058, #36889, #85393, #56065, #72239 ),
 .UNSPECIFIED., .F., .F.,
 ( 4, 2, 2, 2, 2, 2, 2, 2, 2, 2, 4 ),
 ( 0.000000000000000000, 0.001309639967555296328, 0.001964459951332936903, 0.002291869943221747433, 0.002455574939166153131, 0.002619279935110557962, 0.002782984931054963227, 0.002946689926999368058, 0.003274099918888177720, 0.003928919902665816560, 0.005238559870221097710 ),
 .UNSPECIFIED. ) ;
#32032=CARTESIAN_POINT ( 'NONE',  ( -0.05219959533909027116, -19.03943276465977164, 62.49890960531435979 ) ) ;
#32033=CARTESIAN_POINT ( 'NONE',  ( -9.474510206698964154, 16.51473224551069663, 95.41557627198102409 ) ) ;
#32034=CARTESIAN_POINT ( 'NONE',  ( -12.14591786802326823, 12.06949235617739902, 63.12609039468568994 ) ) ;
#32035=CARTESIAN_POINT ( 'NONE',  ( -10.81492255796105439, 18.62759615963255655, 52.91775706135235424 ) ) ;
#32036=CARTESIAN_POINT ( 'NONE',  ( 5.719274019375673035, 21.55341960407619339, 87.29275706135236135 ) ) ;
#32037=CARTESIAN_POINT ( 'NONE',  ( 5.823673210054125526, 21.52544592524343514, 94.79057627198105251 ) ) ;
#32038=CARTESIAN_POINT ( 'NONE',  ( 5.719274019375673035, 21.55341960407619339, 37.29275706135235424 ) ) ;
#32039=CARTESIAN_POINT ( 'NONE',  ( -4.379528057220086978, -16.55341960407618274, 84.79275706135234714 ) ) ;
#32040=CARTESIAN_POINT ( 'NONE',  ( -18.62759615963270932, 10.81492255796079327, 80.83224293864769550 ) ) ;
#32041=CARTESIAN_POINT ( 'NONE',  ( -13.89961937509957401, -13.97604488694547875, 39.37609039468566152 ) ) ;
#32042=CARTESIAN_POINT ( 'NONE',  ( 13.89961937509977652, -13.97604488694527269, 83.12390960531436690 ) ) ;
#32043=CARTESIAN_POINT ( 'NONE',  ( 14.29746914071049879, -8.314922557960816363, 28.33224293864769550 ) ) ;
#32045=CARTESIAN_POINT ( 'NONE',  ( -5.153800228976328057, -19.02544592524343514, 107.2905762719810383 ) ) ;
#32047=CARTESIAN_POINT ( 'NONE',  ( 19.02544592524334988, 5.153800228976608722, 91.45942372801900433 ) ) ;
#32048=CARTESIAN_POINT ( 'NONE',  ( 0.05219959533907565091, 21.53943276465977519, 74.99890960531435269 ) ) ;
#32049=CARTESIAN_POINT ( 'NONE',  ( -4.483927247898539470, -16.52544592524342804, 42.29057627198103120 ) ) ;
#32050=CARTESIAN_POINT ( 'NONE',  ( 5.049401038297881783, 19.05341960407617563, 107.2927570613523187 ) ) ;
#32051=CARTESIAN_POINT ( 'NONE',  ( -16.46253265017160317, 9.564922557960807481, 30.83224293864769550 ) ) ;
#32052=CARTESIAN_POINT ( 'NONE',  ( -5.153800228976607833, 19.02544592524334988, 107.7094237280189759 ) ) ;
#32053=CARTESIAN_POINT ( 'NONE',  ( 10.81492255796078972, 18.62759615963270932, 104.5822429386477097 ) ) ;
#32054=CARTESIAN_POINT ( 'NONE',  ( 5.153800228976615827, -19.02544592524334988, 75.20942372801896170 ) ) ;
#32055=CARTESIAN_POINT ( 'NONE',  ( -14.29746914071037622, -8.314922557961029526, 84.16775706135234714 ) ) ;
#32056=CARTESIAN_POINT ( 'NONE',  ( -9.564922557960796823, -16.46253265017161027, 67.08224293864769550 ) ) ;
#32057=CARTESIAN_POINT ( 'NONE',  ( 8.224510206698953496, -14.34966873604960469, 77.91557627198102409 ) ) ;
#32059=CARTESIAN_POINT ( 'NONE',  ( 19.05341960407611168, 5.049401038298154454, 58.95724293864768129 ) ) ;
#32060=CARTESIAN_POINT ( 'NONE',  ( -12.06949235617756955, 12.14591786802309770, 70.62390960531436690 ) ) ;
#32063=CARTESIAN_POINT ( 'NONE',  ( 4.379528057220339221, -16.55341960407611168, 37.70724293864769550 ) ) ;
#32064=CARTESIAN_POINT ( 'NONE',  ( -19.05341960407611168, -5.049401038298163336, 71.45724293864766707 ) ) ;
#32066=CARTESIAN_POINT ( 'NONE',  ( 16.51473224551083163, -9.474510206698727899, 55.83442372801899722 ) ) ;
#32067=CARTESIAN_POINT ( 'NONE',  ( 16.55341960407618274, -4.379528057220086978, 56.04275706135235424 ) ) ;
#32068=CARTESIAN_POINT ( 'NONE',  ( -0.05219959533907301413, -21.53943276465977519, 62.49890960531436690 ) ) ;
#32069=CARTESIAN_POINT ( 'NONE',  ( -16.46253265017146816, -9.564922557961047289, 29.16775706135232937 ) ) ;
#32070=CARTESIAN_POINT ( 'NONE',  ( -19.02544592524342804, 5.153800228976336051, 86.04057627198103830 ) ) ;
#32072=CARTESIAN_POINT ( 'NONE',  ( 9.474510206698971260, -16.51473224551069308, 112.9155762719810383 ) ) ;
#32073=CARTESIAN_POINT ( 'NONE',  ( 13.97604488694527802, 13.89961937509977652, 64.37390960531436690 ) ) ;
#32074=CARTESIAN_POINT ( 'NONE',  ( 18.62759615963255655, 10.81492255796105972, 36.66775706135234714 ) ) ;
#32075=CARTESIAN_POINT ( 'NONE',  ( -4.483927247898539470, -16.52544592524342804, 107.2905762719810525 ) ) ;
#32076=CARTESIAN_POINT ( 'NONE',  ( 10.81492255796078972, 18.62759615963270932, 99.58224293864770971 ) ) ;
#32077=CARTESIAN_POINT ( 'NONE',  ( -19.02544592524342804, 5.153800228976336051, 101.0405762719810241 ) ) ;
#32078=ORIENTED_EDGE ( 'NONE', *, *, #80571, .T. ) ;
#32079=CARTESIAN_POINT ( 'NONE',  ( -18.67979575497193778, 10.72451020669871902, 23.33442372801901499 ) ) ;
#32081=CARTESIAN_POINT ( 'NONE',  ( 5.049401038298161559, -19.05341960407611168, 92.70724293864769550 ) ) ;
#32082=CARTESIAN_POINT ( 'NONE',  ( 19.52217212775662247, -5.499999999999912959, 82.43993709005258097 ) ) ;
#32083=CARTESIAN_POINT ( 'NONE',  ( 5.719274019375991003, -21.55341960407610458, 92.70724293864770971 ) ) ;
#32084=CARTESIAN_POINT ( 'NONE',  ( -9.564922557960796823, -16.46253265017161027, 47.08224293864769550 ) ) ;
#32085=CARTESIAN_POINT ( 'NONE',  ( -13.97604488694547697, 13.89961937509957934, 108.1260903946856331 ) ) ;
#32087=CARTESIAN_POINT ( 'NONE',  ( 0.05219959533909260263, 19.03943276465977164, 24.99890960531435269 ) ) ;
#32088=CARTESIAN_POINT ( 'NONE',  ( 0.05219959533937995610, -21.53943276465977519, 90.00109039468567573 ) ) ;
#32089=CARTESIAN_POINT ( 'NONE',  ( 16.46253265017160672, -9.564922557960803928, 73.33224293864769550 ) ) ;
#32090=CARTESIAN_POINT ( 'NONE',  ( -5.823673210054431948, 21.52544592524334988, 47.70942372801902565 ) ) ;
#32091=CARTESIAN_POINT ( 'NONE',  ( -10.72451020669870658, -18.67979575497194134, 29.58442372801901854 ) ) ;
#32093=CARTESIAN_POINT ( 'NONE',  ( 9.474510206698971260, -16.51473224551069308, 97.91557627198102409 ) ) ;
#32095=CARTESIAN_POINT ( 'NONE',  ( 16.53943276465976808, 0.05219959533934440121, 41.25109039468568284 ) ) ;
#32096=CARTESIAN_POINT ( 'NONE',  ( -10.72451020669898014, 18.67979575497178502, 40.41557627198103120 ) ) ;
#32097=CARTESIAN_POINT ( 'NONE',  ( 21.53943276465977519, 0.05219959533937863772, 41.25109039468568284 ) ) ;
#32098=CARTESIAN_POINT ( 'NONE',  ( 21.52544592524334988, 5.823673210054432836, 71.45942372801901854 ) ) ;
#32099=CARTESIAN_POINT ( 'NONE',  ( 17.97035753253448576, -5.500000000000063949, 38.49602986858894127 ) ) ;
#32100=CARTESIAN_POINT ( 'NONE',  ( -13.89961937509957401, -13.97604488694547875, 109.3760903946856331 ) ) ;
#32101=CARTESIAN_POINT ( 'NONE',  ( -0.05219959533909027116, -19.03943276465977164, 57.49890960531435979 ) ) ;
#32102=CARTESIAN_POINT ( 'NONE',  ( 13.97604488694527802, 13.89961937509977652, 94.37390960531436690 ) ) ;
#32103=CARTESIAN_POINT ( 'NONE',  ( -8.224510206698948167, 14.34966873604960824, 105.4155762719810383 ) ) ;
#32104=CARTESIAN_POINT ( 'NONE',  ( -16.53943276465976808, 0.05219959533911058130, 111.2489096053143669 ) ) ;
#32105=CARTESIAN_POINT ( 'NONE',  ( 21.53943276465977519, -0.05219959533907433946, 33.74890960531436690 ) ) ;
#32106=CARTESIAN_POINT ( 'NONE',  ( -16.53943276465976808, -0.05219959533934237506, 83.75109039468568994 ) ) ;
#32107=CARTESIAN_POINT ( 'NONE',  ( -14.29746914071049879, 8.314922557960819915, 65.83224293864769550 ) ) ;
#32108=CARTESIAN_POINT ( 'NONE',  ( -9.474510206698964154, 16.51473224551069663, 50.41557627198102409 ) ) ;
#32109=CARTESIAN_POINT ( 'NONE',  ( 21.52544592524334988, 5.823673210054432836, 71.45942372801901854 ) ) ;
#32110=CARTESIAN_POINT ( 'NONE',  ( -21.52544592524334988, -5.823673210054445271, 73.95942372801901854 ) ) ;
#32111=CARTESIAN_POINT ( 'NONE',  ( 5.049401038297881783, 19.05341960407617563, 102.2927570613523045 ) ) ;
#32112=CARTESIAN_POINT ( 'NONE',  ( -12.14591786802309592, -12.06949235617757132, 56.87390960531436690 ) ) ;
#32113=CARTESIAN_POINT ( 'NONE',  ( -18.67979575497193778, 10.72451020669871902, 33.33442372801900433 ) ) ;
#32114=CARTESIAN_POINT ( 'NONE',  ( 5.823673210054125526, 21.52544592524343514, 54.79057627198104541 ) ) ;
#32117=CARTESIAN_POINT ( 'NONE',  ( 9.564922557960805705, 16.46253265017160317, 64.58224293864769550 ) ) ;
#32118=CARTESIAN_POINT ( 'NONE',  ( -12.14591786802309592, -12.06949235617757132, 31.87390960531435979 ) ) ;
#32119=CARTESIAN_POINT ( 'NONE',  ( -14.29746914071049879, 8.314922557960819915, 25.83224293864769194 ) ) ;
#32120=CARTESIAN_POINT ( 'NONE',  ( 8.314922557961029526, -14.29746914071037800, 95.41775706135234714 ) ) ;
#32121=CARTESIAN_POINT ( 'NONE',  ( 19.02544592524334988, 5.153800228976608722, 51.45942372801900433 ) ) ;
#32122=CARTESIAN_POINT ( 'NONE',  ( 17.05116617787827238, 6.768360034955707150, 48.84324446740802728 ) ) ;
#32123=CARTESIAN_POINT ( 'NONE',  ( -16.51473224551069308, -9.474510206698971260, 106.6655762719810383 ) ) ;
#32124=CARTESIAN_POINT ( 'NONE',  ( -16.52544592524342804, 4.483927247898546575, 76.04057627198102409 ) ) ;
#32125=CARTESIAN_POINT ( 'NONE',  ( 9.564922557961047289, -16.46253265017146816, 40.41775706135234003 ) ) ;
#32126=CARTESIAN_POINT ( 'NONE',  ( 9.564922557960805705, 16.46253265017160317, 29.58224293864769550 ) ) ;
#32127=CARTESIAN_POINT ( 'NONE',  ( 18.67979575497178502, 10.72451020669898547, 24.16557627198103120 ) ) ;
#32128=CARTESIAN_POINT ( 'NONE',  ( -21.55341960407610458, -5.719274019375992779, 56.45724293864768839 ) ) ;
#32129=CARTESIAN_POINT ( 'NONE',  ( 16.55341960407611168, 4.379528057220329451, 98.95724293864770971 ) ) ;
#32130=CARTESIAN_POINT ( 'NONE',  ( 12.06949235617739724, 12.14591786802326823, 51.87609039468568284 ) ) ;
#32131=CARTESIAN_POINT ( 'NONE',  ( -0.05219959533910754901, -16.53943276465976808, 92.49890960531436690 ) ) ;
#32132=CARTESIAN_POINT ( 'NONE',  ( 16.81555441253552274, -7.025013491695476731, 38.13685445334257906 ) ) ;
#32134=CARTESIAN_POINT ( 'NONE',  ( 9.564922557960805705, 16.46253265017160317, 114.5822429386476955 ) ) ;
#32138=CARTESIAN_POINT ( 'NONE',  ( 14.29746914071037800, 8.314922557961029526, 41.66775706135235424 ) ) ;
#32139=CARTESIAN_POINT ( 'NONE',  ( 12.06949235617757843, -12.14591786802309237, 33.12390960531435979 ) ) ;
#32140=CARTESIAN_POINT ( 'NONE',  ( 5.823673210054125526, 21.52544592524343514, 59.79057627198103120 ) ) ;
#32141=CARTESIAN_POINT ( 'NONE',  ( 5.049401038297881783, 19.05341960407617563, 87.29275706135234714 ) ) ;
#32142=CARTESIAN_POINT ( 'NONE',  ( -15.80617190586745835, -15.72974639402198527, 51.87390960531437401 ) ) ;
#32143=CARTESIAN_POINT ( 'NONE',  ( -18.67979575497193778, 10.72451020669871902, 83.33442372801903275 ) ) ;
#32145=CARTESIAN_POINT ( 'NONE',  ( 4.379528057220092307, 16.55341960407617563, 52.29275706135236135 ) ) ;
#32146=CARTESIAN_POINT ( 'NONE',  ( -9.564922557960796823, -16.46253265017161027, 32.08224293864769550 ) ) ;
#32147=CARTESIAN_POINT ( 'NONE',  ( 19.05341960407611168, 5.049401038298154454, 103.9572429386476671 ) ) ;
#32148=CARTESIAN_POINT ( 'NONE',  ( 16.51473224551069308, 9.474510206698969483, 29.16557627198103475 ) ) ;
#32149=CARTESIAN_POINT ( 'NONE',  ( -4.379528057220328563, 16.55341960407611168, 95.20724293864769550 ) ) ;
#32151=CARTESIAN_POINT ( 'NONE',  ( 16.46253265017160672, -9.564922557960803928, 98.33224293864769550 ) ) ;
#32153=CARTESIAN_POINT ( 'NONE',  ( -0.05219959533934338120, 16.53943276465976808, 62.50109039468568284 ) ) ;
#32154=CARTESIAN_POINT ( 'NONE',  ( -18.67979575497178146, -10.72451020669898902, 96.66557627198102409 ) ) ;
#32155=CARTESIAN_POINT ( 'NONE',  ( 9.564922557960805705, 16.46253265017160317, 54.58224293864769550 ) ) ;
#32156=CARTESIAN_POINT ( 'NONE',  ( 15.72974639402176855, 15.80617190586768217, 21.87609039468567573 ) ) ;
#32157=CARTESIAN_POINT ( 'NONE',  ( -19.05341960407611168, -5.049401038298163336, 86.45724293864769550 ) ) ;
#32160=CARTESIAN_POINT ( 'NONE',  ( -21.52544592524334988, -5.823673210054445271, 23.95942372801901143 ) ) ;
#32161=CARTESIAN_POINT ( 'NONE',  ( -19.05341960407611168, -5.049401038298163336, 26.45724293864769550 ) ) ;
#32162=CARTESIAN_POINT ( 'NONE',  ( 16.51473224551069308, 9.474510206698969483, 109.1655762719810383 ) ) ;
#32163=CARTESIAN_POINT ( 'NONE',  ( 13.97604488694548053, -13.89961937509957401, 70.62609039468567573 ) ) ;
#32164=CARTESIAN_POINT ( 'NONE',  ( -19.05341960407617563, 5.049401038297882671, 23.54275706135233648 ) ) ;
#32165=CARTESIAN_POINT ( 'NONE',  ( -5.823673210054116645, -21.52544592524344225, 97.29057627198105251 ) ) ;
#32166=CARTESIAN_POINT ( 'NONE',  ( -19.03943276465977164, -0.05219959533935918106, 38.75109039468566152 ) ) ;
#32167=CARTESIAN_POINT ( 'NONE',  ( 0.05219959533934541429, -16.53943276465976808, 85.00109039468568994 ) ) ;
#32168=CARTESIAN_POINT ( 'NONE',  ( -19.05341960407611168, -5.049401038298163336, 101.4572429386476955 ) ) ;
#32169=CARTESIAN_POINT ( 'NONE',  ( -5.049401038298153566, 19.05341960407611168, 55.20724293864769550 ) ) ;
#32171=CARTESIAN_POINT ( 'NONE',  ( 5.823673210054444382, -21.52544592524334988, 70.20942372801904696 ) ) ;
#32172=CARTESIAN_POINT ( 'NONE',  ( 0.05219959533937995610, -21.53943276465977519, 85.00109039468568994 ) ) ;
#32173=CARTESIAN_POINT ( 'NONE',  ( -5.049401038298153566, 19.05341960407611168, 80.20724293864769550 ) ) ;
#32174=CARTESIAN_POINT ( 'NONE',  ( -21.55341960407619339, 5.719274019375674811, 48.54275706135234714 ) ) ;
#32175=CARTESIAN_POINT ( 'NONE',  ( -0.05219959533936034679, 19.03943276465977164, 82.50109039468567573 ) ) ;
#32176=CARTESIAN_POINT ( 'NONE',  ( -19.03943276465977164, 0.05219959533909376836, 56.24890960531435979 ) ) ;
#32177=CARTESIAN_POINT ( 'NONE',  ( 19.03943276465977164, -0.05219959533909143690, 103.7489096053143669 ) ) ;
#32178=CARTESIAN_POINT ( 'NONE',  ( 0.05219959533909260263, 19.03943276465977164, 64.99890960531436690 ) ) ;
#32180=CARTESIAN_POINT ( 'NONE',  ( 5.153800228976335163, 19.02544592524342804, 54.79057627198103120 ) ) ;
#32181=CARTESIAN_POINT ( 'NONE',  ( -5.823673210054116645, -21.52544592524344225, 97.29057627198105251 ) ) ;
#32182=CARTESIAN_POINT ( 'NONE',  ( 8.314922557961029526, -14.29746914071037800, 80.41775706135234714 ) ) ;
#32184=CARTESIAN_POINT ( 'NONE',  ( -5.049401038297874678, -19.05341960407617918, 49.79275706135231871 ) ) ;
#32185=CARTESIAN_POINT ( 'NONE',  ( -19.05341960407611168, -5.049401038298163336, 66.45724293864769550 ) ) ;
#32186=CARTESIAN_POINT ( 'NONE',  ( 16.53943276465976808, -0.05219959533910856209, 58.74890960531436690 ) ) ;
#32187=CARTESIAN_POINT ( 'NONE',  ( 14.29746914071049879, -8.314922557960816363, 88.33224293864769550 ) ) ;
#32188=CARTESIAN_POINT ( 'NONE',  ( 13.97604488694527802, 13.89961937509977652, 99.37390960531436690 ) ) ;
#32189=CARTESIAN_POINT ( 'NONE',  ( -19.03943276465977164, 0.05219959533909376836, 91.24890960531436690 ) ) ;
#32190=CARTESIAN_POINT ( 'NONE',  ( -13.89961937509977652, 13.97604488694528158, 100.6239096053143669 ) ) ;
#32191=CARTESIAN_POINT ( 'NONE',  ( -19.03943276465977164, -0.05219959533935918106, 23.75109039468566152 ) ) ;
#32192=CARTESIAN_POINT ( 'NONE',  ( 4.483927247898790824, -16.52544592524335698, 95.20942372801903275 ) ) ;
#32193=CARTESIAN_POINT ( 'NONE',  ( 16.51473224551069308, 9.474510206698969483, 74.16557627198103830 ) ) ;
#32195=CARTESIAN_POINT ( 'NONE',  ( -10.72451020669870658, -18.67979575497194134, 44.58442372801901854 ) ) ;
#32196=CARTESIAN_POINT ( 'NONE',  ( 0.05219959533907565091, 21.53943276465977519, 34.99890960531435979 ) ) ;
#32197=CARTESIAN_POINT ( 'NONE',  ( 15.72974639402199770, -15.80617190586745480, 108.1239096053143811 ) ) ;
#32198=CARTESIAN_POINT ( 'NONE',  ( 8.224510206698953496, -14.34966873604960469, 57.91557627198103120 ) ) ;
#32199=CARTESIAN_POINT ( 'NONE',  ( -9.474510206698964154, 16.51473224551069663, 60.41557627198102409 ) ) ;
#32200=CARTESIAN_POINT ( 'NONE',  ( 8.224510206698953496, -14.34966873604960469, 87.91557627198103830 ) ) ;
#32201=B_SPLINE_CURVE_WITH_KNOTS ( 'NONE', 3,
 ( #179284, #70086, #131755, #116585, #40749, #102418, #178274, #164105, #87248, #148932, #10422, #44730 ),
 .UNSPECIFIED., .F., .F.,
 ( 4, 2, 2, 2, 2, 4 ),
 ( 7.806255641895631925E-18, 0.001213821615221375490, 0.001820732422832063453, 0.002124187826637407434, 0.002275915528540080075, 0.002427643230442752716 ),
 .UNSPECIFIED. ) ;
#32202=CARTESIAN_POINT ( 'NONE',  ( -5.049401038297874678, -19.05341960407617918, 39.79275706135232582 ) ) ;
#32203=CARTESIAN_POINT ( 'NONE',  ( 9.564922557960805705, 16.46253265017160317, 24.58224293864769194 ) ) ;
#32204=CARTESIAN_POINT ( 'NONE',  ( -12.06949235617739369, -12.14591786802326823, 69.37609039468567573 ) ) ;
#32205=CARTESIAN_POINT ( 'NONE',  ( -13.89961937509977652, 13.97604488694528158, 70.62390960531432427 ) ) ;
#32207=CARTESIAN_POINT ( 'NONE',  ( -12.06949235617756955, 12.14591786802309770, 90.62390960531436690 ) ) ;
#32208=CARTESIAN_POINT ( 'NONE',  ( 21.55341960407610458, 5.719274019375980345, 43.95724293864769550 ) ) ;
#32209=ORIENTED_EDGE ( 'NONE', *, *, #126426, .T. ) ;
#32210=CARTESIAN_POINT ( 'NONE',  ( -16.53943276465976808, -0.05219959533934237506, 108.7510903946857042 ) ) ;
#32211=CARTESIAN_POINT ( 'NONE',  ( 8.224510206698742110, 14.34966873604972548, 27.08442372801901854 ) ) ;
#32212=CARTESIAN_POINT ( 'NONE',  ( -18.62759615963255300, -10.81492255796106328, 94.16775706135237556 ) ) ;
#32213=CARTESIAN_POINT ( 'NONE',  ( -5.049401038298153566, 19.05341960407611168, 90.20724293864766707 ) ) ;
#32214=CARTESIAN_POINT ( 'NONE',  ( -21.52544592524334988, -5.823673210054445271, 23.95942372801901143 ) ) ;
#32215=CARTESIAN_POINT ( 'NONE',  ( -5.049401038298153566, 19.05341960407611168, 35.20724293864768839 ) ) ;
#32216=CARTESIAN_POINT ( 'NONE',  ( 0.05219959533934541429, -16.53943276465976808, 25.00109039468567218 ) ) ;
#32217=CARTESIAN_POINT ( 'NONE',  ( -5.153800228976607833, 19.02544592524334988, 92.70942372801901854 ) ) ;
#32218=CARTESIAN_POINT ( 'NONE',  ( 15.80617190586746368, 15.72974639402197994, 84.37390960531438111 ) ) ;
#32219=CARTESIAN_POINT ( 'NONE',  ( -13.89961937509957401, -13.97604488694547875, 69.37609039468564731 ) ) ;
#32220=CARTESIAN_POINT ( 'NONE',  ( -21.52544592524334988, -5.823673210054445271, 18.95942372801901143 ) ) ;
#32221=FACE_OUTER_BOUND ( 'NONE', #159072, .T. ) ;
#32222=CARTESIAN_POINT ( 'NONE',  ( -13.97604488694527625, -13.89961937509977652, 76.87390960531433848 ) ) ;
#32223=CARTESIAN_POINT ( 'NONE',  ( 0.05219959533934541429, -16.53943276465976808, 35.00109039468568284 ) ) ;
#32225=CARTESIAN_POINT ( 'NONE',  ( 19.05341960407617918, -5.049401038297876454, 61.04275706135232582 ) ) ;
#32226=CARTESIAN_POINT ( 'NONE',  ( -21.55341960407619339, 5.719274019375674811, 23.54275706135235424 ) ) ;
#32227=CARTESIAN_POINT ( 'NONE',  ( 4.379528057220339221, -16.55341960407611168, 82.70724293864770971 ) ) ;
#32228=CARTESIAN_POINT ( 'NONE',  ( 13.89961937509977652, -13.97604488694527269, 88.12390960531438111 ) ) ;
#32229=CARTESIAN_POINT ( 'NONE',  ( -12.06949235617739369, -12.14591786802326823, 39.37609039468567573 ) ) ;
#32230=CARTESIAN_POINT ( 'NONE',  ( -19.02544592524334988, -5.153800228976617603, 38.95942372801900433 ) ) ;
#32231=CARTESIAN_POINT ( 'NONE',  ( -0.05219959533937732626, 21.53943276465977519, 62.50109039468568284 ) ) ;
#32232=CARTESIAN_POINT ( 'NONE',  ( -16.53943276465976808, -0.05219959533934237506, 33.75109039468568284 ) ) ;
#32233=CARTESIAN_POINT ( 'NONE',  ( 16.46253265017160672, -9.564922557960803928, 58.33224293864769550 ) ) ;
#32234=CARTESIAN_POINT ( 'NONE',  ( -9.564922557961040184, 16.46253265017147172, 77.91775706135234714 ) ) ;
#32235=CARTESIAN_POINT ( 'NONE',  ( 8.224510206698742110, 14.34966873604972548, 52.08442372801901854 ) ) ;
#32236=CARTESIAN_POINT ( 'NONE',  ( 15.72974639402176855, 15.80617190586768217, 101.8760903946857042 ) ) ;
#32237=CARTESIAN_POINT ( 'NONE',  ( -19.05341960407617563, 5.049401038297882671, 63.54275706135234003 ) ) ;
#32238=CARTESIAN_POINT ( 'NONE',  ( -9.564922557960796823, -16.46253265017161027, 47.08224293864769550 ) ) ;
#32239=CARTESIAN_POINT ( 'NONE',  ( 18.67979575497178502, 10.72451020669898547, 74.16557627198102409 ) ) ;
#32240=CARTESIAN_POINT ( 'NONE',  ( -12.06949235617756955, 12.14591786802309770, 65.62390960531436690 ) ) ;
#32241=CARTESIAN_POINT ( 'NONE',  ( 9.474510206698729675, 16.51473224551082808, 67.08442372801900433 ) ) ;
#32242=CARTESIAN_POINT ( 'NONE',  ( 16.21995358207300697, -7.366697692864327074, 62.43551001512160781 ) ) ;
#32243=CARTESIAN_POINT ( 'NONE',  ( 9.564922557961047289, -16.46253265017146816, 45.41775706135232582 ) ) ;
#32244=CARTESIAN_POINT ( 'NONE',  ( 12.06949235617739724, 12.14591786802326823, 96.87609039468568994 ) ) ;
#32245=CARTESIAN_POINT ( 'NONE',  ( 4.379528057220339221, -16.55341960407611168, 67.70724293864769550 ) ) ;
#32246=CARTESIAN_POINT ( 'NONE',  ( -15.80617190586768217, 15.72974639402176855, 98.12609039468570415 ) ) ;
#32248=CARTESIAN_POINT ( 'NONE',  ( -0.05219959533907301413, -21.53943276465977519, 97.49890960531436690 ) ) ;
#32249=CARTESIAN_POINT ( 'NONE',  ( 16.46253265017160672, -9.564922557960803928, 58.33224293864769550 ) ) ;
#32250=CARTESIAN_POINT ( 'NONE',  ( -15.80617190586768217, 15.72974639402176855, 68.12609039468567573 ) ) ;
#32251=CARTESIAN_POINT ( 'NONE',  ( -19.03943276465977164, 0.05219959533909376836, 46.24890960531435979 ) ) ;
#32253=CARTESIAN_POINT ( 'NONE',  ( -19.05341960407611168, -5.049401038298163336, 71.45724293864766707 ) ) ;
#32254=CARTESIAN_POINT ( 'NONE',  ( -4.379528057220328563, 16.55341960407611168, 115.2072429386476955 ) ) ;
#32255=CARTESIAN_POINT ( 'NONE',  ( -0.05219959533909027116, -19.03943276465977164, 107.4989096053143527 ) ) ;
#32256=CARTESIAN_POINT ( 'NONE',  ( 0.05219959533910956823, 16.53943276465976808, 64.99890960531435269 ) ) ;
#32257=CARTESIAN_POINT ( 'NONE',  ( 13.89961937509977652, -13.97604488694527269, 33.12390960531434558 ) ) ;
#32258=CARTESIAN_POINT ( 'NONE',  ( 4.379528057220339221, -16.55341960407611168, 87.70724293864769550 ) ) ;
#32259=CARTESIAN_POINT ( 'NONE',  ( 0.05219959533907565091, 21.53943276465977519, 89.99890960531438111 ) ) ;
#32260=CARTESIAN_POINT ( 'NONE',  ( -5.719274019375665041, -21.55341960407619695, 39.79275706135235424 ) ) ;
#32261=CARTESIAN_POINT ( 'NONE',  ( -13.97604488694527625, -13.89961937509977652, 21.87390960531435979 ) ) ;
#32263=CARTESIAN_POINT ( 'NONE',  ( -14.34966873604972548, 8.224510206698743886, 53.33442372801901854 ) ) ;
#32264=CARTESIAN_POINT ( 'NONE',  ( -0.05219959533907301413, -21.53943276465977519, 87.49890960531436690 ) ) ;
#32265=CARTESIAN_POINT ( 'NONE',  ( 0.05219959533936267826, -19.03943276465977164, 30.00109039468566863 ) ) ;
#32266=CARTESIAN_POINT ( 'NONE',  ( 16.51473224551069308, 9.474510206698969483, 109.1655762719810383 ) ) ;
#32267=CARTESIAN_POINT ( 'NONE',  ( -21.53943276465977519, -0.05219959533937600094, 48.75109039468568284 ) ) ;
#32268=CARTESIAN_POINT ( 'NONE',  ( -10.81492255796078084, -18.62759615963271287, 47.08224293864770260 ) ) ;
#32269=CARTESIAN_POINT ( 'NONE',  ( -14.34966873604960291, -8.224510206698953496, 21.66557627198102409 ) ) ;
#32270=CARTESIAN_POINT ( 'NONE',  ( 10.81492255796106328, -18.62759615963255655, 60.41775706135235424 ) ) ;
#32271=CARTESIAN_POINT ( 'NONE',  ( -5.823673210054431948, 21.52544592524334988, 92.70942372801901854 ) ) ;
#32272=CARTESIAN_POINT ( 'NONE',  ( -13.97604488694547697, 13.89961937509957934, 28.12609039468565797 ) ) ;
#32273=CARTESIAN_POINT ( 'NONE',  ( 8.314922557961029526, -14.29746914071037800, 90.41775706135236135 ) ) ;
#32274=CARTESIAN_POINT ( 'NONE',  ( 18.62759615963255655, 10.81492255796105972, 46.66775706135234714 ) ) ;
#32275=CARTESIAN_POINT ( 'NONE',  ( -16.46253265017160317, 9.564922557960807481, 50.83224293864770260 ) ) ;
#32276=CARTESIAN_POINT ( 'NONE',  ( 5.719274019375673035, 21.55341960407619339, 112.2927570613523471 ) ) ;
#32277=CARTESIAN_POINT ( 'NONE',  ( -18.62759615963270932, 10.81492255796079327, 25.83224293864769194 ) ) ;
#32278=EDGE_CURVE ( 'NONE', #165187, #194003, #54516, .T. ) ;
#32279=CARTESIAN_POINT ( 'NONE',  ( 5.719274019375673035, 21.55341960407619339, 22.29275706135235069 ) ) ;
#32280=AXIS2_PLACEMENT_3D ( 'NONE', #5065, #97072, #22250 ) ;
#32281=CARTESIAN_POINT ( 'NONE',  ( 5.823673210054125526, 21.52544592524343514, 69.79057627198102409 ) ) ;
#32282=CARTESIAN_POINT ( 'NONE',  ( 8.224510206698742110, 14.34966873604972548, 42.08442372801901854 ) ) ;
#32284=CARTESIAN_POINT ( 'NONE',  ( 18.62759615963271287, -10.81492255796078972, 83.33224293864769550 ) ) ;
#32285=CARTESIAN_POINT ( 'NONE',  ( -14.29746914071037622, -8.314922557961029526, 69.16775706135234714 ) ) ;
#32286=CARTESIAN_POINT ( 'NONE',  ( 0.05219959533910956823, 16.53943276465976808, 64.99890960531435269 ) ) ;
#32288=CARTESIAN_POINT ( 'NONE',  ( -9.474510206698720793, -16.51473224551083518, 89.58442372801900433 ) ) ;
#32290=CARTESIAN_POINT ( 'NONE',  ( -8.224510206698735004, -14.34966873604973081, 34.58442372801900433 ) ) ;
#32291=CARTESIAN_POINT ( 'NONE',  ( 15.72974639402199770, -15.80617190586745480, 113.1239096053143953 ) ) ;
#32292=CARTESIAN_POINT ( 'NONE',  ( -18.67979575497178146, -10.72451020669898902, 76.66557627198103830 ) ) ;
#32293=CARTESIAN_POINT ( 'NONE',  ( -5.719274019375978568, 21.55341960407610458, 35.20724293864768839 ) ) ;
#32294=CARTESIAN_POINT ( 'NONE',  ( -4.483927247898782831, 16.52544592524335698, 62.70942372801902565 ) ) ;
#32295=CARTESIAN_POINT ( 'NONE',  ( 16.51473224551069308, 9.474510206698969483, 74.16557627198103830 ) ) ;
#32296=CARTESIAN_POINT ( 'NONE',  ( -15.72974639402176322, -15.80617190586768395, 49.37609039468569705 ) ) ;
#32297=CARTESIAN_POINT ( 'NONE',  ( 16.53943276465976808, 0.05219959533934440121, 21.25109039468567218 ) ) ;
#32298=CARTESIAN_POINT ( 'NONE',  ( 16.51473224551069308, 9.474510206698969483, 109.1655762719810383 ) ) ;
#32300=CARTESIAN_POINT ( 'NONE',  ( -9.564922557961040184, 16.46253265017147172, 22.91775706135233648 ) ) ;
#32301=CARTESIAN_POINT ( 'NONE',  ( -4.379528057220086978, -16.55341960407618274, 39.79275706135235424 ) ) ;
#32302=CARTESIAN_POINT ( 'NONE',  ( 5.153800228976335163, 19.02544592524342804, 104.7905762719809957 ) ) ;
#32303=CARTESIAN_POINT ( 'NONE',  ( 5.719274019375991003, -21.55341960407610458, 107.7072429386476955 ) ) ;
#32304=CARTESIAN_POINT ( 'NONE',  ( 9.474510206698971260, -16.51473224551069308, 67.91557627198102409 ) ) ;
#32306=CARTESIAN_POINT ( 'NONE',  ( -16.55341960407611168, -4.379528057220339221, 86.45724293864770971 ) ) ;
#32307=CARTESIAN_POINT ( 'NONE',  ( 5.719274019375991003, -21.55341960407610458, 22.70724293864769194 ) ) ;
#32308=CARTESIAN_POINT ( 'NONE',  ( -16.61371651742598132, 7.165104196376278267, 33.85415069992996706 ) ) ;
#32309=CARTESIAN_POINT ( 'NONE',  ( 5.719274019375991003, -21.55341960407610458, 102.7072429386476955 ) ) ;
#32310=CARTESIAN_POINT ( 'NONE',  ( 5.153800228976615827, -19.02544592524334988, 60.20942372801899012 ) ) ;
#32311=CARTESIAN_POINT ( 'NONE',  ( 18.62759615963271287, -10.81492255796078972, 33.33224293864769550 ) ) ;
#32312=CARTESIAN_POINT ( 'NONE',  ( 5.049401038298161559, -19.05341960407611168, 22.70724293864769194 ) ) ;
#32313=CARTESIAN_POINT ( 'NONE',  ( -15.72974639402197994, 15.80617190586746368, 65.62390960531436690 ) ) ;
#32315=CARTESIAN_POINT ( 'NONE',  ( -16.46253265017160317, 9.564922557960807481, 105.8322429386476955 ) ) ;
#32316=CARTESIAN_POINT ( 'NONE',  ( 10.81492255796106328, -18.62759615963255655, 90.41775706135236135 ) ) ;
#32317=CARTESIAN_POINT ( 'NONE',  ( -16.46253265017160317, 9.564922557960807481, 45.83224293864769550 ) ) ;
#32318=CARTESIAN_POINT ( 'NONE',  ( 8.224510206698953496, -14.34966873604960469, 82.91557627198103830 ) ) ;
#32319=CARTESIAN_POINT ( 'NONE',  ( 16.55341960407618274, -4.379528057220086978, 31.04275706135234714 ) ) ;
#32320=CARTESIAN_POINT ( 'NONE',  ( 13.97604488694527802, 13.89961937509977652, 59.37390960531434558 ) ) ;
#32321=CARTESIAN_POINT ( 'NONE',  ( -18.67979575497193778, 10.72451020669871902, 73.33442372801901854 ) ) ;
#32322=ORIENTED_EDGE ( 'NONE', *, *, #96372, .F. ) ;
#32323=CARTESIAN_POINT ( 'NONE',  ( -5.049401038297874678, -19.05341960407617918, 29.79275706135232227 ) ) ;
#32324=CARTESIAN_POINT ( 'NONE',  ( -19.02544592524334988, -5.153800228976617603, 43.95942372801899012 ) ) ;
#32325=CARTESIAN_POINT ( 'NONE',  ( 10.81492255796106328, -18.62759615963255655, 30.41775706135234358 ) ) ;
#32326=CARTESIAN_POINT ( 'NONE',  ( 13.97604488694527802, 13.89961937509977830, 54.37390960531435979 ) ) ;
#32327=CARTESIAN_POINT ( 'NONE',  ( -13.89961937509957401, -13.97604488694547875, 29.37609039468565797 ) ) ;
#32328=CARTESIAN_POINT ( 'NONE',  ( -13.89961937509977652, 13.97604488694528158, 85.62390960531433848 ) ) ;
#32329=CARTESIAN_POINT ( 'NONE',  ( 16.46253265017160672, -9.564922557960803928, 63.33224293864769550 ) ) ;
#32330=CARTESIAN_POINT ( 'NONE',  ( 14.34966873604960469, 8.224510206698951720, 24.16557627198103120 ) ) ;
#32331=CARTESIAN_POINT ( 'NONE',  ( -19.02544592524342804, 5.153800228976336051, 111.0405762719810099 ) ) ;
#32332=CARTESIAN_POINT ( 'NONE',  ( 10.81492255796106328, -18.62759615963255655, 85.41775706135236135 ) ) ;
#32334=CARTESIAN_POINT ( 'NONE',  ( 17.48853670773242186, 5.747243402303175763, 58.83328700250011423 ) ) ;
#32335=CARTESIAN_POINT ( 'NONE',  ( -21.52544592524334988, -5.823673210054445271, 78.95942372801901854 ) ) ;
#32337=CARTESIAN_POINT ( 'NONE',  ( -19.05341960407611168, -5.049401038298163336, 96.45724293864769550 ) ) ;
#32339=CARTESIAN_POINT ( 'NONE',  ( 21.55341960407610458, 5.719274019375980345, 68.95724293864769550 ) ) ;
#32340=CARTESIAN_POINT ( 'NONE',  ( -8.224510206698948167, 14.34966873604960824, 30.41557627198101699 ) ) ;
#32341=CARTESIAN_POINT ( 'NONE',  ( 12.06949235617757843, -12.14591786802309237, 113.1239096053143953 ) ) ;
#32342=CARTESIAN_POINT ( 'NONE',  ( -5.049401038298153566, 19.05341960407611168, 95.20724293864770971 ) ) ;
#32343=CARTESIAN_POINT ( 'NONE',  ( -5.823673210054431948, 21.52544592524334988, 112.7094237280190328 ) ) ;
#32344=CARTESIAN_POINT ( 'NONE',  ( 19.03943276465977164, -0.05219959533909143690, 23.74890960531435269 ) ) ;
#32345=CARTESIAN_POINT ( 'NONE',  ( -0.05219959533937732626, 21.53943276465977519, 62.50109039468568284 ) ) ;
#32346=CARTESIAN_POINT ( 'NONE',  ( 5.153800228976335163, 19.02544592524342804, 109.7905762719810099 ) ) ;
#32347=CARTESIAN_POINT ( 'NONE',  ( 14.29746914071037800, 8.314922557961029526, 106.6677570613523756 ) ) ;
#32348=CARTESIAN_POINT ( 'NONE',  ( 16.51473224551083163, -9.474510206698727899, 70.83442372801900433 ) ) ;
#32349=CARTESIAN_POINT ( 'NONE',  ( 13.89961937509957579, 13.97604488694547520, 66.87609039468567573 ) ) ;
#32350=CARTESIAN_POINT ( 'NONE',  ( 19.05341960407611168, 5.049401038298154454, 103.9572429386476671 ) ) ;
#32351=CARTESIAN_POINT ( 'NONE',  ( -12.06949235617756955, 12.14591786802309770, 90.62390960531436690 ) ) ;
#32352=CARTESIAN_POINT ( 'NONE',  ( 9.564922557961047289, -16.46253265017146816, 55.41775706135234003 ) ) ;
#32353=CARTESIAN_POINT ( 'NONE',  ( 19.02544592524343514, -5.153800228976328945, 78.54057627198099567 ) ) ;
#32354=CARTESIAN_POINT ( 'NONE',  ( -14.34966873604960291, -8.224510206698953496, 66.66557627198102409 ) ) ;
#32355=CARTESIAN_POINT ( 'NONE',  ( -16.51473224551082808, 9.474510206698731452, 93.33442372801900433 ) ) ;
#32356=CARTESIAN_POINT ( 'NONE',  ( 10.72451020669898902, -18.67979575497178502, 47.91557627198102409 ) ) ;
#32358=CARTESIAN_POINT ( 'NONE',  ( -16.52544592524342804, 4.483927247898546575, 111.0405762719810525 ) ) ;
#32360=CARTESIAN_POINT ( 'NONE',  ( -19.05341960407611168, -5.049401038298163336, 71.45724293864766707 ) ) ;
#32361=CARTESIAN_POINT ( 'NONE',  ( -5.719274019375978568, 21.55341960407610458, 80.20724293864769550 ) ) ;
#32362=CARTESIAN_POINT ( 'NONE',  ( 14.29746914071037800, 8.314922557961029526, 86.66775706135234714 ) ) ;
#32363=CARTESIAN_POINT ( 'NONE',  ( -0.05219959533909027116, -19.03943276465977164, 67.49890960531436690 ) ) ;
#32364=CARTESIAN_POINT ( 'NONE',  ( -5.153800228976607833, 19.02544592524334988, 62.70942372801899722 ) ) ;
#32365=CARTESIAN_POINT ( 'NONE',  ( -21.52544592524334988, -5.823673210054445271, 83.95942372801900433 ) ) ;
#32366=CARTESIAN_POINT ( 'NONE',  ( 15.80617190586746368, 15.72974639402197994, 64.37390960531435269 ) ) ;
#32367=CARTESIAN_POINT ( 'NONE',  ( -21.55341960407610458, -5.719274019375992779, 21.45724293864769550 ) ) ;
#32368=CARTESIAN_POINT ( 'NONE',  ( -16.46253265017160317, 9.564922557960807481, 30.83224293864769550 ) ) ;
#32369=CARTESIAN_POINT ( 'NONE',  ( 8.224510206698742110, 14.34966873604972548, 102.0844237280190185 ) ) ;
#32370=CARTESIAN_POINT ( 'NONE',  ( 14.34966873604972726, -8.224510206698740333, 25.83442372801901499 ) ) ;
#32371=CARTESIAN_POINT ( 'NONE',  ( 18.22780087662122739, 5.500000000000000888, 76.48236817873106475 ) ) ;
#32372=CARTESIAN_POINT ( 'NONE',  ( 21.55341960407619695, -5.719274019375665929, 91.04275706135236135 ) ) ;
#32373=ORIENTED_EDGE ( 'NONE', *, *, #61610, .T. ) ;
#32374=CARTESIAN_POINT ( 'NONE',  ( 14.29746914071049879, -8.314922557960816363, 53.33224293864769550 ) ) ;
#32375=CARTESIAN_POINT ( 'NONE',  ( -18.62759615963270932, 10.81492255796079327, 90.83224293864769550 ) ) ;
#32376=CARTESIAN_POINT ( 'NONE',  ( 5.719274019375991003, -21.55341960407610458, 107.7072429386476955 ) ) ;
#32378=CARTESIAN_POINT ( 'NONE',  ( -21.55341960407610458, -5.719274019375992779, 41.45724293864769550 ) ) ;
#32379=CARTESIAN_POINT ( 'NONE',  ( -16.52544592524335698, -4.483927247898792601, 73.95942372801901854 ) ) ;
#32380=CARTESIAN_POINT ( 'NONE',  ( -4.379528057220328563, 16.55341960407611168, 85.20724293864770971 ) ) ;
#32381=CARTESIAN_POINT ( 'NONE',  ( -5.049401038298153566, 19.05341960407611168, 45.20724293864769550 ) ) ;
#32383=CARTESIAN_POINT ( 'NONE',  ( 12.06949235617757843, -12.14591786802309237, 23.12390960531436335 ) ) ;
#32384=CARTESIAN_POINT ( 'NONE',  ( -5.719274019375665041, -21.55341960407619695, 29.79275706135234358 ) ) ;
#32385=CARTESIAN_POINT ( 'NONE',  ( -5.049401038298153566, 19.05341960407611168, 90.20724293864766707 ) ) ;
#32386=CARTESIAN_POINT ( 'NONE',  ( 18.62759615963255655, 10.81492255796105972, 61.66775706135235424 ) ) ;
#32388=CARTESIAN_POINT ( 'NONE',  ( 19.02544592524343514, -5.153800228976328945, 28.54057627198102409 ) ) ;
#32390=CARTESIAN_POINT ( 'NONE',  ( -5.823673210054431948, 21.52544592524334988, 57.70942372801901143 ) ) ;
#32391=CARTESIAN_POINT ( 'NONE',  ( -13.89961937509977652, 13.97604488694528158, 55.62390960531434558 ) ) ;
#32392=CARTESIAN_POINT ( 'NONE',  ( 5.153800228976335163, 19.02544592524342804, 24.79057627198102765 ) ) ;
#32393=CARTESIAN_POINT ( 'NONE',  ( 16.51473224551069308, 9.474510206698969483, 89.16557627198103830 ) ) ;
#32394=CARTESIAN_POINT ( 'NONE',  ( -9.564922557961040184, 16.46253265017147172, 62.91775706135233293 ) ) ;
#32395=CARTESIAN_POINT ( 'NONE',  ( -21.53943276465977519, -0.05219959533937600094, 43.75109039468568284 ) ) ;
#32396=CARTESIAN_POINT ( 'NONE',  ( -5.153800228976607833, 19.02544592524334988, 62.70942372801899722 ) ) ;
#32397=CARTESIAN_POINT ( 'NONE',  ( -19.02544592524342804, 5.153800228976336051, 36.04057627198100988 ) ) ;
#32398=CARTESIAN_POINT ( 'NONE',  ( 16.55341960407618274, -4.379528057220086978, 101.0427570613523756 ) ) ;
#32399=CARTESIAN_POINT ( 'NONE',  ( -19.05341960407617563, 5.049401038297882671, 78.54275706135233293 ) ) ;
#32400=CARTESIAN_POINT ( 'NONE',  ( 14.29746914071049879, -8.314922557960816363, 28.33224293864769550 ) ) ;
#32401=CARTESIAN_POINT ( 'NONE',  ( -19.02544592524334988, -5.153800228976617603, 43.95942372801899012 ) ) ;
#32402=CARTESIAN_POINT ( 'NONE',  ( 13.89961937509977652, -13.97604488694527269, 103.1239096053143527 ) ) ;
#32403=CARTESIAN_POINT ( 'NONE',  ( 5.719274019375673035, 21.55341960407619339, 112.2927570613523471 ) ) ;
#32404=CARTESIAN_POINT ( 'NONE',  ( 16.51473224551083163, -9.474510206698727899, 25.83442372801900078 ) ) ;
#32405=CARTESIAN_POINT ( 'NONE',  ( -0.05219959533909027116, -19.03943276465977164, 32.49890960531435979 ) ) ;
#32406=CARTESIAN_POINT ( 'NONE',  ( -15.80617190586768217, 15.72974639402176855, 93.12609039468568994 ) ) ;
#32407=CARTESIAN_POINT ( 'NONE',  ( 12.14591786802327356, -12.06949235617739191, 30.62609039468567929 ) ) ;
#32408=CARTESIAN_POINT ( 'NONE',  ( -19.03943276465977164, 0.05219959533909376836, 86.24890960531436690 ) ) ;
#32410=CARTESIAN_POINT ( 'NONE',  ( 19.02544592524343514, -5.153800228976328945, 78.54057627198099567 ) ) ;
#32412=CARTESIAN_POINT ( 'NONE',  ( -13.97604488694547697, 13.89961937509957934, 78.12609039468567573 ) ) ;
#32413=CARTESIAN_POINT ( 'NONE',  ( 13.97604488694527802, 13.89961937509977652, 104.3739096053143385 ) ) ;
#32414=CARTESIAN_POINT ( 'NONE',  ( -18.62759615963255300, -10.81492255796106328, 104.1677570613523471 ) ) ;
#32415=CARTESIAN_POINT ( 'NONE',  ( 14.29746914071049879, -8.314922557960816363, 98.33224293864769550 ) ) ;
#32416=CARTESIAN_POINT ( 'NONE',  ( 13.97604488694527802, 13.89961937509977652, 29.37390960531435979 ) ) ;
#32417=CARTESIAN_POINT ( 'NONE',  ( 0.05219959533907565091, 21.53943276465977519, 39.99890960531436690 ) ) ;
#32418=CARTESIAN_POINT ( 'NONE',  ( -18.67979575497178146, -10.72451020669898902, 31.66557627198102054 ) ) ;
#32419=CARTESIAN_POINT ( 'NONE',  ( -4.379528057220328563, 16.55341960407611168, 115.2072429386476955 ) ) ;
#32421=CARTESIAN_POINT ( 'NONE',  ( 9.474510206698729675, 16.51473224551082808, 62.08442372801899722 ) ) ;
#32422=CARTESIAN_POINT ( 'NONE',  ( -0.05219959533910754901, -16.53943276465976808, 42.49890960531435979 ) ) ;
#32423=CARTESIAN_POINT ( 'NONE',  ( 16.46253265017160672, -9.564922557960803928, 113.3322429386476955 ) ) ;
#32425=CARTESIAN_POINT ( 'NONE',  ( -21.53943276465977519, -0.05219959533937600094, 73.75109039468567573 ) ) ;
#32426=CARTESIAN_POINT ( 'NONE',  ( -5.823673210054116645, -21.52544592524344225, 77.29057627198102409 ) ) ;
#32427=CARTESIAN_POINT ( 'NONE',  ( 5.823673210054444382, -21.52544592524334988, 50.20942372801901854 ) ) ;
#32428=CARTESIAN_POINT ( 'NONE',  ( 21.52544592524344225, -5.823673210054117533, 93.54057627198103830 ) ) ;
#32429=CARTESIAN_POINT ( 'NONE',  ( 15.72974639402176855, 15.80617190586768217, 56.87609039468568994 ) ) ;
#32430=CARTESIAN_POINT ( 'NONE',  ( -16.46253265017160317, 9.564922557960807481, 30.83224293864769550 ) ) ;
#32431=CARTESIAN_POINT ( 'NONE',  ( 0.05219959533909260263, 19.03943276465977164, 79.99890960531436690 ) ) ;
#32432=CARTESIAN_POINT ( 'NONE',  ( 14.34966873604972726, -8.224510206698740333, 75.83442372801900433 ) ) ;
#32433=CARTESIAN_POINT ( 'NONE',  ( -4.379528057220328563, 16.55341960407611168, 105.2072429386477097 ) ) ;
#32435=CARTESIAN_POINT ( 'NONE',  ( 12.06949235617757843, -12.14591786802309237, 48.12390960531436690 ) ) ;
#32436=CARTESIAN_POINT ( 'NONE',  ( -16.53943276465976808, 0.05219959533911058130, 21.24890960531436690 ) ) ;
#32437=CARTESIAN_POINT ( 'NONE',  ( -5.153800228976328057, -19.02544592524343514, 62.29057627198100988 ) ) ;
#32438=CARTESIAN_POINT ( 'NONE',  ( -19.02544592524342804, 5.153800228976336051, 36.04057627198100988 ) ) ;
#32439=CARTESIAN_POINT ( 'NONE',  ( 15.72974639402199770, -15.80617190586745480, 48.12390960531436690 ) ) ;
#32440=CARTESIAN_POINT ( 'NONE',  ( 9.564922557961047289, -16.46253265017146816, 35.41775706135233293 ) ) ;
#32441=CARTESIAN_POINT ( 'NONE',  ( -17.12812012977023812, -6.668231424566066323, 41.35948759323144230 ) ) ;
#32442=CARTESIAN_POINT ( 'NONE',  ( -14.34966873604960291, -8.224510206698953496, 41.66557627198103120 ) ) ;
#32443=CARTESIAN_POINT ( 'NONE',  ( -15.80617190586745835, -15.72974639402198527, 31.87390960531435979 ) ) ;
#32445=CARTESIAN_POINT ( 'NONE',  ( -15.80617190586768217, 15.72974639402176855, 58.12609039468568994 ) ) ;
#32447=CARTESIAN_POINT ( 'NONE',  ( -16.52544592524335698, -4.483927247898792601, 68.95942372801901854 ) ) ;
#32448=CARTESIAN_POINT ( 'NONE',  ( -9.564922557961040184, 16.46253265017147172, 67.91775706135233293 ) ) ;
#32450=CARTESIAN_POINT ( 'NONE',  ( 14.29746914071049879, -8.314922557960816363, 43.33224293864769550 ) ) ;
#32451=CARTESIAN_POINT ( 'NONE',  ( -19.35543954521082455, -5.499999999999491074, 74.58901960356450900 ) ) ;
#32452=CARTESIAN_POINT ( 'NONE',  ( -12.14591786802309592, -12.06949235617757132, 31.87390960531435979 ) ) ;
#32453=CARTESIAN_POINT ( 'NONE',  ( 16.51473224551069308, 9.474510206698969483, 44.16557627198103120 ) ) ;
#32454=CARTESIAN_POINT ( 'NONE',  ( 16.46253265017160672, -9.564922557960803928, 58.33224293864769550 ) ) ;
#32455=CARTESIAN_POINT ( 'NONE',  ( 9.474510206698971260, -16.51473224551069308, 27.91557627198103120 ) ) ;
#32456=CARTESIAN_POINT ( 'NONE',  ( -21.55341960407619339, 5.719274019375674811, 28.54275706135234358 ) ) ;
#32457=CARTESIAN_POINT ( 'NONE',  ( 5.153800228976335163, 19.02544592524342804, 54.79057627198103120 ) ) ;
#32458=DIRECTION ( 'NONE',  ( 1.000000000000000000, 0.000000000000000000, 0.000000000000000000 ) ) ;
#32459=CARTESIAN_POINT ( 'NONE',  ( 19.05341960407611168, 5.049401038298154454, 48.95724293864768129 ) ) ;
#32460=CARTESIAN_POINT ( 'NONE',  ( 15.72974639402199770, -15.80617190586745480, 33.12390960531435979 ) ) ;
#32461=CARTESIAN_POINT ( 'NONE',  ( -5.719274019375665041, -21.55341960407619695, 54.79275706135235424 ) ) ;
#32462=CARTESIAN_POINT ( 'NONE',  ( 0.05219959533910956823, 16.53943276465976808, 114.9989096053143669 ) ) ;
#32463=CARTESIAN_POINT ( 'NONE',  ( 15.72974639402199770, -15.80617190586745480, 23.12390960531436335 ) ) ;
#32464=CARTESIAN_POINT ( 'NONE',  ( 14.34966873604972726, -8.224510206698740333, 90.83442372801901854 ) ) ;
#32465=CARTESIAN_POINT ( 'NONE',  ( 15.72974639402176855, 15.80617190586768217, 106.8760903946856899 ) ) ;
#32466=CARTESIAN_POINT ( 'NONE',  ( 12.14591786802327356, -12.06949235617739191, 60.62609039468567573 ) ) ;
#32467=CARTESIAN_POINT ( 'NONE',  ( -13.97604488694527625, -13.89961937509977652, 111.8739096053143243 ) ) ;
#32468=CARTESIAN_POINT ( 'NONE',  ( 14.29746914071037800, 8.314922557961029526, 56.66775706135235424 ) ) ;
#32469=CARTESIAN_POINT ( 'NONE',  ( 16.53943276465976808, 0.05219959533934440121, 31.25109039468568639 ) ) ;
#32470=CARTESIAN_POINT ( 'NONE',  ( -4.379528057220086978, -16.55341960407618274, 89.79275706135236135 ) ) ;
#32471=CARTESIAN_POINT ( 'NONE',  ( -0.05219959533937732626, 21.53943276465977519, 47.50109039468568994 ) ) ;
#32472=CARTESIAN_POINT ( 'NONE',  ( 13.89961937509957401, 13.97604488694547697, 111.8760903946856757 ) ) ;
#32473=CARTESIAN_POINT ( 'NONE',  ( -21.52544592524343514, 5.823673210054127303, 111.0405762719810525 ) ) ;
#32474=CARTESIAN_POINT ( 'NONE',  ( 14.34966873604972726, -8.224510206698740333, 20.83442372801901143 ) ) ;
#32475=CARTESIAN_POINT ( 'NONE',  ( 4.379528057220092307, 16.55341960407617563, 87.29275706135236135 ) ) ;
#32477=CARTESIAN_POINT ( 'NONE',  ( 5.823673210054444382, -21.52544592524334988, 90.20942372801903275 ) ) ;
#32478=CARTESIAN_POINT ( 'NONE',  ( 9.474510206698729675, 16.51473224551082808, 82.08442372801899012 ) ) ;
#32479=CARTESIAN_POINT ( 'NONE',  ( 12.14591786802309770, 12.06949235617756955, 49.37390960531436690 ) ) ;
#32480=CARTESIAN_POINT ( 'NONE',  ( -16.53943276465976808, 0.05219959533911058130, 41.24890960531435269 ) ) ;
#32481=CARTESIAN_POINT ( 'NONE',  ( 0.05219959533910956823, 16.53943276465976808, 104.9989096053143669 ) ) ;
#32482=CARTESIAN_POINT ( 'NONE',  ( 9.474510206698729675, 16.51473224551082808, 47.08442372801900433 ) ) ;
#32484=CARTESIAN_POINT ( 'NONE',  ( 21.53943276465977519, 0.05219959533937863772, 31.25109039468568639 ) ) ;
#32485=CARTESIAN_POINT ( 'NONE',  ( -14.29746914071037622, -8.314922557961029526, 19.16775706135234714 ) ) ;
#32486=CARTESIAN_POINT ( 'NONE',  ( 17.50000000000000000, -5.500000000000000888, 120.0000000000000142 ) ) ;
#32487=CARTESIAN_POINT ( 'NONE',  ( 19.05341960407611168, 5.049401038298154454, 98.95724293864766707 ) ) ;
#32488=CARTESIAN_POINT ( 'NONE',  ( -5.719274019375978568, 21.55341960407610458, 55.20724293864770260 ) ) ;
#32489=CARTESIAN_POINT ( 'NONE',  ( 5.049401038297881783, 19.05341960407617563, 92.29275706135234714 ) ) ;
#32490=CARTESIAN_POINT ( 'NONE',  ( 9.474510206698971260, -16.51473224551069308, 87.91557627198102409 ) ) ;
#32491=CARTESIAN_POINT ( 'NONE',  ( 15.80617190586746368, 15.72974639402197994, 59.37390960531436690 ) ) ;
#32492=CARTESIAN_POINT ( 'NONE',  ( 14.29746914071049879, -8.314922557960816363, 103.3322429386476955 ) ) ;
#32493=CARTESIAN_POINT ( 'NONE',  ( 19.05341960407611168, 5.049401038298154454, 63.95724293864769550 ) ) ;
#32494=CARTESIAN_POINT ( 'NONE',  ( -9.474510206698964154, 16.51473224551069663, 35.41557627198102409 ) ) ;
#32495=CARTESIAN_POINT ( 'NONE',  ( -21.55341960407619339, 5.719274019375674811, 33.54275706135234714 ) ) ;
#32496=CARTESIAN_POINT ( 'NONE',  ( 10.81492255796106328, -18.62759615963255655, 80.41775706135234714 ) ) ;
#32498=CARTESIAN_POINT ( 'NONE',  ( 12.06949235617739724, 12.14591786802326823, 96.87609039468568994 ) ) ;
#32499=CARTESIAN_POINT ( 'NONE',  ( -5.719274019375665041, -21.55341960407619695, 24.79275706135235779 ) ) ;
#32500=CARTESIAN_POINT ( 'NONE',  ( 15.72974639402176855, 15.80617190586768217, 26.87609039468567218 ) ) ;
#32501=CARTESIAN_POINT ( 'NONE',  ( -19.05341960407617563, 5.049401038297882671, 68.54275706135230450 ) ) ;
#32502=CARTESIAN_POINT ( 'NONE',  ( 19.03943276465977164, -0.05219959533909143690, 83.74890960531436690 ) ) ;
#32503=CARTESIAN_POINT ( 'NONE',  ( -18.67979575497193778, 10.72451020669871902, 78.33442372801901854 ) ) ;
#32504=CARTESIAN_POINT ( 'NONE',  ( 0.05219959533907565091, 21.53943276465977519, 79.99890960531435269 ) ) ;
#32505=CARTESIAN_POINT ( 'NONE',  ( -8.314922557960811034, -14.29746914071050412, 67.08224293864770971 ) ) ;
#32506=CARTESIAN_POINT ( 'NONE',  ( 5.823673210054444382, -21.52544592524334988, 105.2094237280190328 ) ) ;
#32507=CARTESIAN_POINT ( 'NONE',  ( 14.34966873604960469, 8.224510206698951720, 84.16557627198103830 ) ) ;
#32508=CARTESIAN_POINT ( 'NONE',  ( -19.03943276465977164, 0.05219959533909376836, 31.24890960531435979 ) ) ;
#32509=CARTESIAN_POINT ( 'NONE',  ( 19.02544592524334988, 5.153800228976608722, 76.45942372801897591 ) ) ;
#32510=CARTESIAN_POINT ( 'NONE',  ( 8.224510206698953496, -14.34966873604960469, 37.91557627198102409 ) ) ;
#32511=CARTESIAN_POINT ( 'NONE',  ( -21.53943276465977519, -0.05219959533937600094, 88.75109039468567573 ) ) ;
#32512=CARTESIAN_POINT ( 'NONE',  ( -19.05341960407611168, -5.049401038298163336, 96.45724293864769550 ) ) ;
#32513=CARTESIAN_POINT ( 'NONE',  ( -9.474510206698720793, -16.51473224551083518, 59.58442372801900433 ) ) ;
#32514=CARTESIAN_POINT ( 'NONE',  ( 21.55341960407610458, 5.719274019375980345, 68.95724293864769550 ) ) ;
#32515=CARTESIAN_POINT ( 'NONE',  ( 15.72974639402199770, -15.80617190586745480, 113.1239096053143953 ) ) ;
#32516=CARTESIAN_POINT ( 'NONE',  ( 16.46253265017146816, 9.564922557961045513, 106.6677570613523471 ) ) ;
#32517=CARTESIAN_POINT ( 'NONE',  ( 16.55341960407618274, -4.379528057220086978, 86.04275706135236135 ) ) ;
#32519=CARTESIAN_POINT ( 'NONE',  ( -15.72974639402197994, 15.80617190586746368, 115.6239096053143669 ) ) ;
#32520=CARTESIAN_POINT ( 'NONE',  ( -4.483927247898539470, -16.52544592524342804, 97.29057627198105251 ) ) ;
#32522=CARTESIAN_POINT ( 'NONE',  ( -12.06949235617739369, -12.14591786802326823, 49.37609039468569705 ) ) ;
#32523=CARTESIAN_POINT ( 'NONE',  ( 15.80617190586746368, 15.72974639402197994, 64.37390960531435269 ) ) ;
#32524=CARTESIAN_POINT ( 'NONE',  ( 16.52544592524335698, 4.483927247898782831, 111.4594237280190328 ) ) ;
#32525=CARTESIAN_POINT ( 'NONE',  ( -16.55341960407617563, 4.379528057220093196, 38.54275706135234714 ) ) ;
#32526=CARTESIAN_POINT ( 'NONE',  ( 19.05341960407611168, 5.049401038298154454, 33.95724293864769550 ) ) ;
#32527=CARTESIAN_POINT ( 'NONE',  ( -14.34966873604972548, 8.224510206698743886, 83.33442372801903275 ) ) ;
#32528=CARTESIAN_POINT ( 'NONE',  ( -16.46253265017146816, -9.564922557961047289, 79.16775706135234714 ) ) ;
#32529=CARTESIAN_POINT ( 'NONE',  ( 18.62759615963271287, -10.81492255796078972, 68.33224293864769550 ) ) ;
#32530=CARTESIAN_POINT ( 'NONE',  ( -4.483927247898782831, 16.52544592524335698, 102.7094237280190185 ) ) ;
#32531=CARTESIAN_POINT ( 'NONE',  ( 0.05219959533937995610, -21.53943276465977519, 80.00109039468568994 ) ) ;
#32532=CARTESIAN_POINT ( 'NONE',  ( -10.81492255796078084, -18.62759615963271287, 62.08224293864769550 ) ) ;
#32533=CARTESIAN_POINT ( 'NONE',  ( 10.72451020669898902, -18.67979575497178502, 47.91557627198102409 ) ) ;
#32534=CARTESIAN_POINT ( 'NONE',  ( -16.52544592524335698, -4.483927247898792601, 78.95942372801901854 ) ) ;
#32535=CARTESIAN_POINT ( 'NONE',  ( 15.72974639402199770, -15.80617190586745480, 48.12390960531436690 ) ) ;
#32537=CARTESIAN_POINT ( 'NONE',  ( 9.564922557960805705, 16.46253265017160317, 109.5822429386476955 ) ) ;
#32539=CARTESIAN_POINT ( 'NONE',  ( 5.049401038298161559, -19.05341960407611168, 22.70724293864769194 ) ) ;
#32540=CARTESIAN_POINT ( 'NONE',  ( -15.80617190586745835, -15.72974639402198527, 56.87390960531436690 ) ) ;
#32541=CARTESIAN_POINT ( 'NONE',  ( 12.06949235617739724, 12.14591786802326823, 106.8760903946856899 ) ) ;
#32542=CARTESIAN_POINT ( 'NONE',  ( 15.80617190586769283, -15.72974639402175789, 50.62609039468568994 ) ) ;
#32543=CARTESIAN_POINT ( 'NONE',  ( -19.02544592524334988, -5.153800228976617603, 98.95942372801900433 ) ) ;
#32544=CARTESIAN_POINT ( 'NONE',  ( -14.34966873604960291, -8.224510206698953496, 111.6655762719810525 ) ) ;
#32545=CARTESIAN_POINT ( 'NONE',  ( -5.049401038297874678, -19.05341960407617918, 109.7927570613523187 ) ) ;
#32546=CARTESIAN_POINT ( 'NONE',  ( 19.02544592524343514, -5.153800228976328945, 43.54057627198103120 ) ) ;
#32548=CARTESIAN_POINT ( 'NONE',  ( 19.05341960407611168, 5.049401038298154454, 88.95724293864769550 ) ) ;
#32549=CARTESIAN_POINT ( 'NONE',  ( 14.34966873604972726, -8.224510206698740333, 75.83442372801900433 ) ) ;
#32550=CARTESIAN_POINT ( 'NONE',  ( -13.97604488694547697, 13.89961937509957934, 73.12609039468568994 ) ) ;
#32551=CARTESIAN_POINT ( 'NONE',  ( -19.03943276465977164, -0.05219959533935918106, 18.75109039468567218 ) ) ;
#32552=CARTESIAN_POINT ( 'NONE',  ( -21.52544592524343514, 5.823673210054127303, 61.04057627198103120 ) ) ;
#32553=CARTESIAN_POINT ( 'NONE',  ( 16.53943276465976808, 0.05219959533934440121, 81.25109039468568994 ) ) ;
#32554=CARTESIAN_POINT ( 'NONE',  ( -9.564922557961040184, 16.46253265017147172, 77.91775706135234714 ) ) ;
#32555=CARTESIAN_POINT ( 'NONE',  ( 5.049401038298161559, -19.05341960407611168, 37.70724293864768839 ) ) ;
#32556=CARTESIAN_POINT ( 'NONE',  ( -0.05219959533909027116, -19.03943276465977164, 72.49890960531435269 ) ) ;
#32557=CARTESIAN_POINT ( 'NONE',  ( -10.81492255796105439, 18.62759615963255655, 47.91775706135234714 ) ) ;
#32558=CARTESIAN_POINT ( 'NONE',  ( -13.89961937509977652, 13.97604488694528158, 40.62390960531435979 ) ) ;
#32559=CARTESIAN_POINT ( 'NONE',  ( 9.474510206698729675, 16.51473224551082808, 72.08442372801900433 ) ) ;
#32561=CARTESIAN_POINT ( 'NONE',  ( 16.51473224551069308, 9.474510206698969483, 104.1655762719810241 ) ) ;
#32562=CARTESIAN_POINT ( 'NONE',  ( 4.483927247898545687, 16.52544592524342804, 69.79057627198102409 ) ) ;
#32563=CARTESIAN_POINT ( 'NONE',  ( -21.53943276465977519, 0.05219959533907696930, 61.24890960531435979 ) ) ;
#32566=CARTESIAN_POINT ( 'NONE',  ( -16.46253265017146816, -9.564922557961047289, 44.16775706135232582 ) ) ;
#32568=CARTESIAN_POINT ( 'NONE',  ( -13.97604488694527625, -13.89961937509977652, 61.87390960531435979 ) ) ;
#32569=CARTESIAN_POINT ( 'NONE',  ( -5.049401038298153566, 19.05341960407611168, 70.20724293864769550 ) ) ;
#32570=CARTESIAN_POINT ( 'NONE',  ( 16.53943276465976808, 0.05219959533934440121, 56.25109039468568284 ) ) ;
#32573=CARTESIAN_POINT ( 'NONE',  ( -4.379528057220086978, -16.55341960407618274, 94.79275706135234714 ) ) ;
#32575=CARTESIAN_POINT ( 'NONE',  ( 14.29746914071037800, 8.314922557961029526, 71.66775706135234714 ) ) ;
#32576=CARTESIAN_POINT ( 'NONE',  ( -4.483927247898782831, 16.52544592524335698, 37.70942372801900433 ) ) ;
#32577=CARTESIAN_POINT ( 'NONE',  ( -16.51473224551082808, 9.474510206698731452, 28.33442372801900433 ) ) ;
#32578=CARTESIAN_POINT ( 'NONE',  ( -19.02544592524342804, 5.153800228976336051, 61.04057627198103120 ) ) ;
#32580=CARTESIAN_POINT ( 'NONE',  ( -18.67979575497193778, 10.72451020669871902, 58.33442372801901143 ) ) ;
#32581=CARTESIAN_POINT ( 'NONE',  ( 19.02544592524334988, 5.153800228976608722, 61.45942372801900433 ) ) ;
#32582=CARTESIAN_POINT ( 'NONE',  ( -21.55341960407619339, 5.719274019375674811, 108.5427570613523756 ) ) ;
#32583=CARTESIAN_POINT ( 'NONE',  ( -9.564922557960796823, -16.46253265017161027, 32.08224293864769550 ) ) ;
#32585=CARTESIAN_POINT ( 'NONE',  ( 15.80617190586746368, 15.72974639402197994, 54.37390960531435979 ) ) ;
#32586=B_SPLINE_CURVE_WITH_KNOTS ( 'NONE', 3,
 ( #155226, #165685, #156216, #95531, #12022, #78365 ),
 .UNSPECIFIED., .F., .F.,
 ( 4, 2, 4 ),
 ( 0.003239945802372214394, 0.003620412082092060516, 0.004000878361811907070 ),
 .UNSPECIFIED. ) ;
#32587=CARTESIAN_POINT ( 'NONE',  ( 19.02544592524343514, -5.153800228976328945, 113.5405762719810241 ) ) ;
#32588=CARTESIAN_POINT ( 'NONE',  ( -12.14591786802309592, -12.06949235617757132, 96.87390960531436690 ) ) ;
#32589=CARTESIAN_POINT ( 'NONE',  ( 12.14591786802327356, -12.06949235617739191, 40.62609039468567573 ) ) ;
#32590=CARTESIAN_POINT ( 'NONE',  ( 4.483927247898545687, 16.52544592524342804, 29.79057627198102409 ) ) ;
#32593=CARTESIAN_POINT ( 'NONE',  ( -21.55341960407619339, 5.719274019375674811, 23.54275706135235424 ) ) ;
#32594=CARTESIAN_POINT ( 'NONE',  ( 12.14591786802309770, 12.06949235617756955, 34.37390960531435979 ) ) ;
#32595=CARTESIAN_POINT ( 'NONE',  ( 19.03943276465977164, -0.05219959533909143690, 108.7489096053143527 ) ) ;
#32596=CARTESIAN_POINT ( 'NONE',  ( -9.564922557961040184, 16.46253265017147172, 102.9177570613523329 ) ) ;
#32597=CARTESIAN_POINT ( 'NONE',  ( -5.049401038297874678, -19.05341960407617918, 29.79275706135232227 ) ) ;
#32598=CARTESIAN_POINT ( 'NONE',  ( -12.14591786802309592, -12.06949235617757132, 26.87390960531435979 ) ) ;
#32599=CARTESIAN_POINT ( 'NONE',  ( 18.62759615963271287, -10.81492255796078972, 103.3322429386476955 ) ) ;
#32600=CARTESIAN_POINT ( 'NONE',  ( -18.67979575497178146, -10.72451020669898902, 61.66557627198103120 ) ) ;
#32601=CARTESIAN_POINT ( 'NONE',  ( 19.05341960407611168, 5.049401038298154454, 73.95724293864768129 ) ) ;
#32602=CARTESIAN_POINT ( 'NONE',  ( -16.55341960407611168, -4.379528057220339221, 46.45724293864769550 ) ) ;
#32603=CARTESIAN_POINT ( 'NONE',  ( -19.05341960407611168, -5.049401038298163336, 96.45724293864769550 ) ) ;
#32605=CARTESIAN_POINT ( 'NONE',  ( -5.153800228976607833, 19.02544592524334988, 52.70942372801900433 ) ) ;
#32606=CARTESIAN_POINT ( 'NONE',  ( -0.05219959533907301413, -21.53943276465977519, 92.49890960531436690 ) ) ;
#32607=CARTESIAN_POINT ( 'NONE',  ( -12.06949235617756955, 12.14591786802309770, 100.6239096053143811 ) ) ;
#32608=CARTESIAN_POINT ( 'NONE',  ( 15.72974639402176855, 15.80617190586768217, 41.87609039468568284 ) ) ;
#32610=CARTESIAN_POINT ( 'NONE',  ( 14.34966873604960469, 8.224510206698951720, 34.16557627198102409 ) ) ;
#32611=CARTESIAN_POINT ( 'NONE',  ( -19.05341960407611168, -5.049401038298163336, 31.45724293864769550 ) ) ;
#32612=CARTESIAN_POINT ( 'NONE',  ( 9.564922557960805705, 16.46253265017160317, 79.58224293864769550 ) ) ;
#32613=CARTESIAN_POINT ( 'NONE',  ( -21.52544592524343514, 5.823673210054127303, 61.04057627198103120 ) ) ;
#32614=CARTESIAN_POINT ( 'NONE',  ( -16.51473224551082808, 9.474510206698731452, 93.33442372801900433 ) ) ;
#32615=CARTESIAN_POINT ( 'NONE',  ( -9.474510206698964154, 16.51473224551069663, 25.41557627198103120 ) ) ;
#32616=CARTESIAN_POINT ( 'NONE',  ( -21.52544592524343514, 5.823673210054127303, 51.04057627198103120 ) ) ;
#32617=CARTESIAN_POINT ( 'NONE',  ( -21.53943276465977519, -0.05219959533937600094, 73.75109039468567573 ) ) ;
#32619=CARTESIAN_POINT ( 'NONE',  ( 4.379528057220092307, 16.55341960407617563, 67.29275706135234714 ) ) ;
#32620=CARTESIAN_POINT ( 'NONE',  ( 13.89961937509977652, -13.97604488694527269, 53.12390960531434558 ) ) ;
#32621=CARTESIAN_POINT ( 'NONE',  ( -13.97604488694527625, -13.89961937509977652, 66.87390960531436690 ) ) ;
#32622=ORIENTED_EDGE ( 'NONE', *, *, #91774, .T. ) ;
#32623=CARTESIAN_POINT ( 'NONE',  ( 18.62759615963255655, 10.81492255796105972, 106.6677570613523756 ) ) ;
#32624=CARTESIAN_POINT ( 'NONE',  ( 14.34966873604972726, -8.224510206698740333, 75.83442372801900433 ) ) ;
#32625=CARTESIAN_POINT ( 'NONE',  ( -10.81492255796105439, 18.62759615963255655, 92.91775706135236135 ) ) ;
#32626=CARTESIAN_POINT ( 'NONE',  ( 19.05341960407611168, 5.049401038298154454, 78.95724293864769550 ) ) ;
#32627=CARTESIAN_POINT ( 'NONE',  ( -21.52544592524343514, 5.823673210054127303, 31.04057627198102409 ) ) ;
#32628=CARTESIAN_POINT ( 'NONE',  ( 5.153800228976615827, -19.02544592524334988, 105.2094237280190185 ) ) ;
#32629=CARTESIAN_POINT ( 'NONE',  ( 10.81492255796106328, -18.62759615963255655, 85.41775706135236135 ) ) ;
#32630=CARTESIAN_POINT ( 'NONE',  ( -16.55341960407617563, 4.379528057220093196, 48.54275706135234714 ) ) ;
#32631=CARTESIAN_POINT ( 'NONE',  ( -0.05219959533907301413, -21.53943276465977519, 102.4989096053143811 ) ) ;
#32632=CARTESIAN_POINT ( 'NONE',  ( 13.97604488694548053, -13.89961937509957401, 100.6260903946856615 ) ) ;
#32633=CARTESIAN_POINT ( 'NONE',  ( -5.153800228976328057, -19.02544592524343514, 72.29057627198102409 ) ) ;
#32634=CARTESIAN_POINT ( 'NONE',  ( 19.02544592524334988, 5.153800228976608722, 111.4594237280190043 ) ) ;
#32635=CARTESIAN_POINT ( 'NONE',  ( -9.564922557960796823, -16.46253265017161027, 37.08224293864768839 ) ) ;
#32636=CARTESIAN_POINT ( 'NONE',  ( 4.379528057220092307, 16.55341960407617563, 27.29275706135234358 ) ) ;
#32637=CARTESIAN_POINT ( 'NONE',  ( 4.483927247898545687, 16.52544592524342804, 64.79057627198103830 ) ) ;
#32638=CARTESIAN_POINT ( 'NONE',  ( 0.05219959533934541429, -16.53943276465976808, 80.00109039468568994 ) ) ;
#32639=CARTESIAN_POINT ( 'NONE',  ( 5.823673210054444382, -21.52544592524334988, 25.20942372801901854 ) ) ;
#32640=CARTESIAN_POINT ( 'NONE',  ( 5.049401038298161559, -19.05341960407611168, 57.70724293864769550 ) ) ;
#32641=CARTESIAN_POINT ( 'NONE',  ( 16.51473224551069308, 9.474510206698969483, 74.16557627198103830 ) ) ;
#32642=CARTESIAN_POINT ( 'NONE',  ( -0.05219959533934338120, 16.53943276465976808, 67.50109039468568994 ) ) ;
#32645=CARTESIAN_POINT ( 'NONE',  ( -0.05219959533937732626, 21.53943276465977519, 107.5010903946856899 ) ) ;
#32646=CARTESIAN_POINT ( 'NONE',  ( -16.51473224551069308, -9.474510206698971260, 31.66557627198102054 ) ) ;
#32648=CARTESIAN_POINT ( 'NONE',  ( 19.03943276465977164, -0.05219959533909143690, 103.7489096053143669 ) ) ;
#32649=ORIENTED_EDGE ( 'NONE', *, *, #62981, .T. ) ;
#32650=CARTESIAN_POINT ( 'NONE',  ( 12.06949235617739724, 12.14591786802326823, 26.87609039468567218 ) ) ;
#32651=CARTESIAN_POINT ( 'NONE',  ( 9.564922557961047289, -16.46253265017146816, 45.41775706135232582 ) ) ;
#32652=CARTESIAN_POINT ( 'NONE',  ( 14.29746914071037800, 8.314922557961029526, 36.66775706135234714 ) ) ;
#32653=CARTESIAN_POINT ( 'NONE',  ( -16.51473224551069308, -9.474510206698971260, 36.66557627198102409 ) ) ;
#32654=CARTESIAN_POINT ( 'NONE',  ( 5.153800228976335163, 19.02544592524342804, 109.7905762719810099 ) ) ;
#32655=CARTESIAN_POINT ( 'NONE',  ( -19.02544592524342804, 5.153800228976336051, 61.04057627198103120 ) ) ;
#32656=CARTESIAN_POINT ( 'NONE',  ( -21.52544592524343514, 5.823673210054127303, 106.0405762719810525 ) ) ;
#32657=CARTESIAN_POINT ( 'NONE',  ( -9.564922557960796823, -16.46253265017161027, 97.08224293864769550 ) ) ;
#32658=CARTESIAN_POINT ( 'NONE',  ( -19.02544592524342804, 5.153800228976336051, 116.0405762719810383 ) ) ;
#32659=CARTESIAN_POINT ( 'NONE',  ( 5.153800228976335163, 19.02544592524342804, 69.79057627198103830 ) ) ;
#32660=CARTESIAN_POINT ( 'NONE',  ( -14.34966873604960291, -8.224510206698953496, 21.66557627198102409 ) ) ;
#32662=CARTESIAN_POINT ( 'NONE',  ( 9.474510206698729675, 16.51473224551082808, 97.08442372801900433 ) ) ;
#32663=CARTESIAN_POINT ( 'NONE',  ( 16.51473224551083163, -9.474510206698727899, 25.83442372801900078 ) ) ;
#32664=B_SPLINE_CURVE_WITH_KNOTS ( 'NONE', 3,
 ( #176201, #145839, #87179, #179211, #149851, #192365 ),
 .UNSPECIFIED., .F., .F.,
 ( 4, 2, 4 ),
 ( 0.003989672132298143457, 0.004372778065220561498, 0.004755883998142979539 ),
 .UNSPECIFIED. ) ;
#32665=CARTESIAN_POINT ( 'NONE',  ( 12.14591786802309770, 12.06949235617756955, 54.37390960531435979 ) ) ;
#32666=CARTESIAN_POINT ( 'NONE',  ( -15.72974639402176322, -15.80617190586768395, 104.3760903946856899 ) ) ;
#32667=CARTESIAN_POINT ( 'NONE',  ( 16.51473224551069308, 9.474510206698969483, 29.16557627198103475 ) ) ;
#32668=CARTESIAN_POINT ( 'NONE',  ( 14.34966873604960469, 8.224510206698951720, 29.16557627198103120 ) ) ;
#32669=CARTESIAN_POINT ( 'NONE',  ( 18.62759615963255655, 10.81492255796105972, 96.66775706135234714 ) ) ;
#32670=CARTESIAN_POINT ( 'NONE',  ( -19.05341960407611168, -5.049401038298163336, 86.45724293864769550 ) ) ;
#32671=CARTESIAN_POINT ( 'NONE',  ( -15.72974639402176322, -15.80617190586768395, 49.37609039468569705 ) ) ;
#32672=CARTESIAN_POINT ( 'NONE',  ( 16.51473224551069308, 9.474510206698969483, 94.16557627198103830 ) ) ;
#32673=CARTESIAN_POINT ( 'NONE',  ( 12.14591786802309770, 12.06949235617756955, 94.37390960531436690 ) ) ;
#32674=CARTESIAN_POINT ( 'NONE',  ( -16.53943276465976808, 0.05219959533911058130, 66.24890960531436690 ) ) ;
#32675=CARTESIAN_POINT ( 'NONE',  ( -10.72451020669898014, 18.67979575497178502, 75.41557627198102409 ) ) ;
#32676=CARTESIAN_POINT ( 'NONE',  ( -5.049401038298153566, 19.05341960407611168, 70.20724293864769550 ) ) ;
#32677=CARTESIAN_POINT ( 'NONE',  ( 18.67979575497178502, 10.72451020669898547, 84.16557627198103830 ) ) ;
#32678=CARTESIAN_POINT ( 'NONE',  ( -9.474510206698720793, -16.51473224551083518, 84.58442372801900433 ) ) ;
#32679=CARTESIAN_POINT ( 'NONE',  ( 5.049401038297881783, 19.05341960407617918, 32.29275706135233293 ) ) ;
#32680=CARTESIAN_POINT ( 'NONE',  ( -8.224510206698948167, 14.34966873604960824, 85.41557627198102409 ) ) ;
#32681=CARTESIAN_POINT ( 'NONE',  ( -16.46253265017160317, 9.564922557960807481, 60.83224293864769550 ) ) ;
#32682=CARTESIAN_POINT ( 'NONE',  ( 21.52544592524344225, -5.823673210054117533, 68.54057627198103830 ) ) ;
#32683=CARTESIAN_POINT ( 'NONE',  ( 16.36317988757059183, -7.306389748694916975, 26.59789608363226421 ) ) ;
#32684=CARTESIAN_POINT ( 'NONE',  ( -4.483927247898782831, 16.52544592524335698, 107.7094237280190328 ) ) ;
#32686=CARTESIAN_POINT ( 'NONE',  ( -5.049401038297874678, -19.05341960407617918, 104.7927570613523471 ) ) ;
#32688=CARTESIAN_POINT ( 'NONE',  ( 0.05219959533910956823, 16.53943276465976808, 84.99890960531436690 ) ) ;
#32690=CARTESIAN_POINT ( 'NONE',  ( 9.564922557960805705, 16.46253265017160317, 74.58224293864769550 ) ) ;
#32691=CARTESIAN_POINT ( 'NONE',  ( 16.46253265017160672, -9.564922557960803928, 33.33224293864770260 ) ) ;
#32692=CARTESIAN_POINT ( 'NONE',  ( 4.379528057220339221, -16.55341960407611168, 62.70724293864769550 ) ) ;
#32693=CARTESIAN_POINT ( 'NONE',  ( 9.474510206698971260, -16.51473224551069308, 97.91557627198102409 ) ) ;
#32694=CARTESIAN_POINT ( 'NONE',  ( -0.05219959533936034679, 19.03943276465977164, 92.50109039468566152 ) ) ;
#32695=CARTESIAN_POINT ( 'NONE',  ( -19.05341960407611168, -5.049401038298163336, 66.45724293864769550 ) ) ;
#32696=CARTESIAN_POINT ( 'NONE',  ( 13.89961937509977652, -13.97604488694527269, 88.12390960531438111 ) ) ;
#32697=CARTESIAN_POINT ( 'NONE',  ( 21.55341960407610458, 5.719274019375980345, 73.95724293864769550 ) ) ;
#32698=CARTESIAN_POINT ( 'NONE',  ( 12.06949235617739724, 12.14591786802326823, 71.87609039468568994 ) ) ;
#32699=CARTESIAN_POINT ( 'NONE',  ( -17.05587630539708854, 6.762274262136623193, 95.74180309037286918 ) ) ;
#32700=CARTESIAN_POINT ( 'NONE',  ( -5.153800228976328057, -19.02544592524343514, 62.29057627198100988 ) ) ;
#32701=CARTESIAN_POINT ( 'NONE',  ( 0.05219959533907565091, 21.53943276465977519, 64.99890960531435269 ) ) ;
#32702=CARTESIAN_POINT ( 'NONE',  ( -9.474510206698720793, -16.51473224551083518, 89.58442372801900433 ) ) ;
#32703=CARTESIAN_POINT ( 'NONE',  ( 12.14591786802309770, 12.06949235617756955, 44.37390960531435979 ) ) ;
#32704=CARTESIAN_POINT ( 'NONE',  ( -0.05219959533937732626, 21.53943276465977519, 47.50109039468568994 ) ) ;
#32705=CARTESIAN_POINT ( 'NONE',  ( 14.34966873604972726, -8.224510206698740333, 75.83442372801900433 ) ) ;
#32706=CARTESIAN_POINT ( 'NONE',  ( 9.474510206698971260, -16.51473224551069308, 107.9155762719810383 ) ) ;
#32707=CARTESIAN_POINT ( 'NONE',  ( 0.05219959533909260263, 19.03943276465977164, 104.9989096053143669 ) ) ;
#32709=CARTESIAN_POINT ( 'NONE',  ( -4.379528057220086978, -16.55341960407618274, 89.79275706135236135 ) ) ;
#32710=CARTESIAN_POINT ( 'NONE',  ( 14.29746914071037800, 8.314922557961029526, 51.66775706135234714 ) ) ;
#32711=CARTESIAN_POINT ( 'NONE',  ( 9.564922557960805705, 16.46253265017160317, 64.58224293864769550 ) ) ;
#32712=CARTESIAN_POINT ( 'NONE',  ( 19.02544592524343514, -5.153800228976328945, 58.54057627198102409 ) ) ;
#32713=CARTESIAN_POINT ( 'NONE',  ( 5.719274019375673035, 21.55341960407619339, 47.29275706135234003 ) ) ;
#32714=CARTESIAN_POINT ( 'NONE',  ( -16.55341960407617563, 4.379528057220093196, 68.54275706135234714 ) ) ;
#32715=CARTESIAN_POINT ( 'NONE',  ( -4.379528057220328563, 16.55341960407611168, 30.20724293864769550 ) ) ;
#32716=CARTESIAN_POINT ( 'NONE',  ( 19.03943276465977164, -0.05219959533909143690, 43.74890960531435979 ) ) ;
#32717=CARTESIAN_POINT ( 'NONE',  ( -19.05341960407611168, -5.049401038298163336, 41.45724293864769550 ) ) ;
#32718=CARTESIAN_POINT ( 'NONE',  ( 0.05219959533934541429, -16.53943276465976808, 30.00109039468568284 ) ) ;
#32719=CARTESIAN_POINT ( 'NONE',  ( -0.05219959533936034679, 19.03943276465977164, 82.50109039468567573 ) ) ;
#32720=CARTESIAN_POINT ( 'NONE',  ( 12.06949235617757843, -12.14591786802309237, 83.12390960531436690 ) ) ;
#32721=CARTESIAN_POINT ( 'NONE',  ( 9.564922557960805705, 16.46253265017160317, 54.58224293864769550 ) ) ;
#32722=CARTESIAN_POINT ( 'NONE',  ( -19.02544592524334988, -5.153800228976617603, 88.95942372801897591 ) ) ;
#32724=CARTESIAN_POINT ( 'NONE',  ( 5.823673210054444382, -21.52544592524334988, 90.20942372801903275 ) ) ;
#32725=CARTESIAN_POINT ( 'NONE',  ( 16.52544592524335698, 4.483927247898782831, 56.45942372801902565 ) ) ;
#32726=CARTESIAN_POINT ( 'NONE',  ( 17.05116617787827593, 6.768360034955705373, 38.84324446740802017 ) ) ;
#32727=CARTESIAN_POINT ( 'NONE',  ( -5.823673210054116645, -21.52544592524344225, 52.29057627198102409 ) ) ;
#32728=CARTESIAN_POINT ( 'NONE',  ( 14.29746914071037800, 8.314922557961029526, 41.66775706135235424 ) ) ;
#32729=CARTESIAN_POINT ( 'NONE',  ( 17.60779699588838909, 5.500000000000005329, 88.84981316670105400 ) ) ;
#32730=CARTESIAN_POINT ( 'NONE',  ( 5.153800228976615827, -19.02544592524334988, 25.20942372801900433 ) ) ;
#32731=CARTESIAN_POINT ( 'NONE',  ( -5.049401038298153566, 19.05341960407611168, 80.20724293864769550 ) ) ;
#32733=CARTESIAN_POINT ( 'NONE',  ( -19.03943276465977164, 0.05219959533909376836, 56.24890960531435979 ) ) ;
#32735=CARTESIAN_POINT ( 'NONE',  ( 9.474510206698971260, -16.51473224551069308, 72.91557627198102409 ) ) ;
#32736=CARTESIAN_POINT ( 'NONE',  ( -19.52851543214742236, -5.500000000000035527, 55.39357721762581122 ) ) ;
#32737=CARTESIAN_POINT ( 'NONE',  ( -0.05219959533936034679, 19.03943276465977164, 37.50109039468567573 ) ) ;
#32738=CARTESIAN_POINT ( 'NONE',  ( 5.719274019375673035, 21.55341960407619339, 107.2927570613523471 ) ) ;
#32739=CARTESIAN_POINT ( 'NONE',  ( -14.34966873604960291, -8.224510206698953496, 36.66557627198103120 ) ) ;
#32740=CARTESIAN_POINT ( 'NONE',  ( 5.049401038298161559, -19.05341960407611168, 42.70724293864767418 ) ) ;
#32741=CARTESIAN_POINT ( 'NONE',  ( 9.564922557960805705, 16.46253265017160317, 109.5822429386476955 ) ) ;
#32742=CARTESIAN_POINT ( 'NONE',  ( 18.62759615963255655, 10.81492255796105972, 71.66775706135234714 ) ) ;
#32743=CARTESIAN_POINT ( 'NONE',  ( -19.03943276465977164, 0.05219959533909376836, 56.24890960531435979 ) ) ;
#32744=CARTESIAN_POINT ( 'NONE',  ( -21.55341960407619339, 5.719274019375674811, 78.54275706135236135 ) ) ;
#32745=CARTESIAN_POINT ( 'NONE',  ( 13.97604488694527802, 13.89961937509977652, 114.3739096053143669 ) ) ;
#32746=CARTESIAN_POINT ( 'NONE',  ( -9.564922557960796823, -16.46253265017161027, 42.08224293864769550 ) ) ;
#32748=CARTESIAN_POINT ( 'NONE',  ( -5.719274019375665041, -21.55341960407619695, 19.79275706135235069 ) ) ;
#32749=CARTESIAN_POINT ( 'NONE',  ( 19.02544592524334988, 5.153800228976608722, 46.45942372801899012 ) ) ;
#32750=CARTESIAN_POINT ( 'NONE',  ( 19.02544592524343514, -5.153800228976328945, 28.54057627198102409 ) ) ;
#32751=CARTESIAN_POINT ( 'NONE',  ( 19.03943276465977164, -0.05219959533909143690, 73.74890960531435269 ) ) ;
#32752=CARTESIAN_POINT ( 'NONE',  ( -0.05219959533936034679, 19.03943276465977164, 107.5010903946856615 ) ) ;
#32753=CARTESIAN_POINT ( 'NONE',  ( -8.314922557960811034, -14.29746914071050412, 72.08224293864769550 ) ) ;
#32754=CARTESIAN_POINT ( 'NONE',  ( -21.53943276465977519, 0.05219959533907696930, 41.24890960531435269 ) ) ;
#32755=CARTESIAN_POINT ( 'NONE',  ( -19.05341960407617563, 5.049401038297882671, 98.54275706135233293 ) ) ;
#32756=CARTESIAN_POINT ( 'NONE',  ( 10.81492255796078972, 18.62759615963270932, 104.5822429386477097 ) ) ;
#32757=CARTESIAN_POINT ( 'NONE',  ( -5.823673210054431948, 21.52544592524334988, 57.70942372801901143 ) ) ;
#32758=CARTESIAN_POINT ( 'NONE',  ( 14.34966873604972726, -8.224510206698740333, 50.83442372801901143 ) ) ;
#32759=CARTESIAN_POINT ( 'NONE',  ( 14.29746914071037800, 8.314922557961029526, 51.66775706135234714 ) ) ;
#32760=CARTESIAN_POINT ( 'NONE',  ( 15.72974639402199770, -15.80617190586745480, 73.12390960531436690 ) ) ;
#32761=CARTESIAN_POINT ( 'NONE',  ( 16.46253265017160672, -9.564922557960803928, 48.33224293864769550 ) ) ;
#32762=CARTESIAN_POINT ( 'NONE',  ( 4.483927247898790824, -16.52544592524335698, 85.20942372801901854 ) ) ;
#32763=CARTESIAN_POINT ( 'NONE',  ( 21.52544592524344225, -5.823673210054117533, 108.5405762719810241 ) ) ;
#32764=CARTESIAN_POINT ( 'NONE',  ( 8.224510206698953496, -14.34966873604960469, 57.91557627198103120 ) ) ;
#32765=CARTESIAN_POINT ( 'NONE',  ( 16.51473224551069308, 9.474510206698969483, 69.16557627198102409 ) ) ;
#32766=CARTESIAN_POINT ( 'NONE',  ( 16.53943276465976808, 0.05219959533934440121, 76.25109039468568994 ) ) ;
#32767=CARTESIAN_POINT ( 'NONE',  ( -4.483927247898782831, 16.52544592524335698, 22.70942372801901499 ) ) ;
#32768=CARTESIAN_POINT ( 'NONE',  ( 5.823673210054125526, 21.52544592524343514, 109.7905762719810383 ) ) ;
#32769=CARTESIAN_POINT ( 'NONE',  ( 12.06949235617757843, -12.14591786802309237, 48.12390960531436690 ) ) ;
#32771=CARTESIAN_POINT ( 'NONE',  ( -17.26172910966778673, 6.454744622555849354, 75.80646908649225679 ) ) ;
#32772=CARTESIAN_POINT ( 'NONE',  ( 10.72451020669898902, -18.67979575497178502, 92.91557627198103830 ) ) ;
#32773=CARTESIAN_POINT ( 'NONE',  ( -4.483927247898539470, -16.52544592524342804, 32.29057627198102409 ) ) ;
#32775=CARTESIAN_POINT ( 'NONE',  ( -16.61371651742604172, -7.165104196376049117, 56.14584930007003294 ) ) ;
#32776=CARTESIAN_POINT ( 'NONE',  ( 5.719274019375991003, -21.55341960407610458, 112.7072429386476955 ) ) ;
#32777=CARTESIAN_POINT ( 'NONE',  ( -5.153800228976328057, -19.02544592524343514, 107.2905762719810383 ) ) ;
#32778=CARTESIAN_POINT ( 'NONE',  ( 18.62759615963255655, 10.81492255796105972, 21.66775706135235069 ) ) ;
#32779=CARTESIAN_POINT ( 'NONE',  ( -16.53943276465976808, 0.05219959533911058130, 51.24890960531436690 ) ) ;
#32780=CARTESIAN_POINT ( 'NONE',  ( 12.06949235617739724, 12.14591786802326823, 51.87609039468568284 ) ) ;
#32781=CARTESIAN_POINT ( 'NONE',  ( -16.46253265017160317, 9.564922557960807481, 55.83224293864769550 ) ) ;
#32782=CARTESIAN_POINT ( 'NONE',  ( 5.049401038297881783, 19.05341960407617563, 57.29275706135231871 ) ) ;
#32783=CARTESIAN_POINT ( 'NONE',  ( 16.51473224551069308, 9.474510206698969483, 84.16557627198102409 ) ) ;
#32784=CARTESIAN_POINT ( 'NONE',  ( 21.53943276465977519, -0.05219959533907433946, 33.74890960531436690 ) ) ;
#32786=CARTESIAN_POINT ( 'NONE',  ( 19.03943276465977164, -0.05219959533909143690, 48.74890960531435979 ) ) ;
#32787=CARTESIAN_POINT ( 'NONE',  ( 0.05219959533934541429, -16.53943276465976808, 20.00109039468568639 ) ) ;
#32788=CARTESIAN_POINT ( 'NONE',  ( -9.564922557961040184, 16.46253265017147172, 57.91775706135233293 ) ) ;
#32789=CARTESIAN_POINT ( 'NONE',  ( -0.05219959533907301413, -21.53943276465977519, 97.49890960531436690 ) ) ;
#32790=CARTESIAN_POINT ( 'NONE',  ( 8.224510206698953496, -14.34966873604960469, 27.91557627198103830 ) ) ;
#32791=CARTESIAN_POINT ( 'NONE',  ( 5.153800228976335163, 19.02544592524342804, 89.79057627198102409 ) ) ;
#32792=CARTESIAN_POINT ( 'NONE',  ( 15.72974639402199770, -15.80617190586745480, 63.12390960531435979 ) ) ;
#32793=CARTESIAN_POINT ( 'NONE',  ( 10.72451020669898902, -18.67979575497178502, 92.91557627198103830 ) ) ;
#32794=CARTESIAN_POINT ( 'NONE',  ( 4.483927247898790824, -16.52544592524335698, 30.20942372801902565 ) ) ;
#32796=CARTESIAN_POINT ( 'NONE',  ( -18.67979575497178146, -10.72451020669898902, 21.66557627198102409 ) ) ;
#32797=CARTESIAN_POINT ( 'NONE',  ( 21.55341960407619695, -5.719274019375665929, 91.04275706135236135 ) ) ;
#32798=CARTESIAN_POINT ( 'NONE',  ( -16.51473224551069308, -9.474510206698971260, 81.66557627198103830 ) ) ;
#32799=CARTESIAN_POINT ( 'NONE',  ( 5.153800228976335163, 19.02544592524342804, 29.79057627198102409 ) ) ;
#32800=CARTESIAN_POINT ( 'NONE',  ( -16.46253265017160317, 9.564922557960807481, 85.83224293864769550 ) ) ;
#32801=CARTESIAN_POINT ( 'NONE',  ( -8.314922557960811034, -14.29746914071050412, 107.0822429386476955 ) ) ;
#32802=CARTESIAN_POINT ( 'NONE',  ( 16.51473224551069308, 9.474510206698969483, 64.16557627198102409 ) ) ;
#32803=CARTESIAN_POINT ( 'NONE',  ( -0.05219959533934338120, 16.53943276465976808, 22.50109039468567573 ) ) ;
#32805=CARTESIAN_POINT ( 'NONE',  ( 5.719274019375673035, 21.55341960407619339, 92.29275706135236135 ) ) ;
#32806=CARTESIAN_POINT ( 'NONE',  ( 9.564922557960805705, 16.46253265017160317, 109.5822429386476955 ) ) ;
#32807=CARTESIAN_POINT ( 'NONE',  ( -16.53943276465976808, -0.05219959533934237506, 93.75109039468567573 ) ) ;
#32810=CARTESIAN_POINT ( 'NONE',  ( -16.46253265017146816, -9.564922557961047289, 69.16775706135233293 ) ) ;
#32811=CARTESIAN_POINT ( 'NONE',  ( 9.474510206698729675, 16.51473224551082808, 37.08442372801899722 ) ) ;
#32813=CARTESIAN_POINT ( 'NONE',  ( 5.153800228976335163, 19.02544592524342804, 34.79057627198102409 ) ) ;
#32814=CARTESIAN_POINT ( 'NONE',  ( -16.52544592524342804, 4.483927247898546575, 41.04057627198103120 ) ) ;
#32815=CARTESIAN_POINT ( 'NONE',  ( 19.03943276465977164, -0.05219959533909143690, 23.74890960531435269 ) ) ;
#32816=CARTESIAN_POINT ( 'NONE',  ( 0.05219959533910956823, 16.53943276465976808, 24.99890960531435624 ) ) ;
#32817=CARTESIAN_POINT ( 'NONE',  ( 17.13100169013299734, 6.664070546373170423, 66.73210164300152769 ) ) ;
#32818=CARTESIAN_POINT ( 'NONE',  ( -8.314922557961024197, 14.29746914071037800, 92.91775706135236135 ) ) ;
#32819=CARTESIAN_POINT ( 'NONE',  ( -9.474510206698964154, 16.51473224551069663, 30.41557627198102054 ) ) ;
#32820=CARTESIAN_POINT ( 'NONE',  ( -21.52544592524334988, -5.823673210054445271, 88.95942372801901854 ) ) ;
#32821=CARTESIAN_POINT ( 'NONE',  ( 19.05341960407617918, -5.049401038297876454, 106.0427570613523471 ) ) ;
#32822=CARTESIAN_POINT ( 'NONE',  ( 18.62759615963255655, 10.81492255796105972, 81.66775706135236135 ) ) ;
#32823=CARTESIAN_POINT ( 'NONE',  ( 13.89961937509957401, 13.97604488694547697, 46.87609039468565442 ) ) ;
#32824=CARTESIAN_POINT ( 'NONE',  ( 9.564922557960805705, 16.46253265017160317, 89.58224293864769550 ) ) ;
#32825=CARTESIAN_POINT ( 'NONE',  ( -16.51473224551069308, -9.474510206698971260, 66.66557627198102409 ) ) ;
#32827=CARTESIAN_POINT ( 'NONE',  ( 16.55341960407611168, 4.379528057220329451, 68.95724293864769550 ) ) ;
#32828=CARTESIAN_POINT ( 'NONE',  ( -18.62759615963270932, 10.81492255796079327, 55.83224293864770260 ) ) ;
#32829=CARTESIAN_POINT ( 'NONE',  ( 19.05341960407611168, 5.049401038298154454, 43.95724293864769550 ) ) ;
#32830=CARTESIAN_POINT ( 'NONE',  ( 10.72451020669898902, -18.67979575497178502, 87.91557627198103830 ) ) ;
#32831=CARTESIAN_POINT ( 'NONE',  ( 4.483927247898790824, -16.52544592524335698, 75.20942372801901854 ) ) ;
#32833=CARTESIAN_POINT ( 'NONE',  ( -13.89961937509977652, 13.97604488694528158, 50.62390960531435979 ) ) ;
#32834=EDGE_CURVE ( 'NONE', #141234, #72646, #42269, .T. ) ;
#32835=CARTESIAN_POINT ( 'NONE',  ( 16.55341960407611168, 4.379528057220329451, 73.95724293864769550 ) ) ;
#32837=CARTESIAN_POINT ( 'NONE',  ( 16.46253265017160672, -9.564922557960803928, 53.33224293864768839 ) ) ;
#32838=CARTESIAN_POINT ( 'NONE',  ( 9.474510206698971260, -16.51473224551069308, 27.91557627198103120 ) ) ;
#32839=CARTESIAN_POINT ( 'NONE',  ( -0.05219959533936034679, 19.03943276465977164, 67.50109039468566152 ) ) ;
#32840=CARTESIAN_POINT ( 'NONE',  ( -16.53943276465976808, 0.05219959533911058130, 71.24890960531435269 ) ) ;
#32841=CARTESIAN_POINT ( 'NONE',  ( -21.52544592524334988, -5.823673210054445271, 43.95942372801902565 ) ) ;
#32842=CARTESIAN_POINT ( 'NONE',  ( -19.03943276465977164, 0.05219959533909376836, 41.24890960531435269 ) ) ;
#32843=CARTESIAN_POINT ( 'NONE',  ( 21.52544592524344225, -5.823673210054117533, 103.5405762719810383 ) ) ;
#32845=CARTESIAN_POINT ( 'NONE',  ( -8.314922557960811034, -14.29746914071050412, 92.08224293864769550 ) ) ;
#32847=CARTESIAN_POINT ( 'NONE',  ( 13.97604488694527802, 13.89961937509977652, 44.37390960531435269 ) ) ;
#32848=CARTESIAN_POINT ( 'NONE',  ( 19.49671883438229258, 5.499999999999973355, 47.39279849105685827 ) ) ;
#32849=CARTESIAN_POINT ( 'NONE',  ( -0.05219959533936034679, 19.03943276465977164, 92.50109039468566152 ) ) ;
#32850=CARTESIAN_POINT ( 'NONE',  ( -16.51473224551069308, -9.474510206698971260, 101.6655762719810241 ) ) ;
#32851=CARTESIAN_POINT ( 'NONE',  ( 10.81492255796106328, -18.62759615963255655, 35.41775706135234003 ) ) ;
#32852=CARTESIAN_POINT ( 'NONE',  ( 5.153800228976335163, 19.02544592524342804, 79.79057627198102409 ) ) ;
#32853=CARTESIAN_POINT ( 'NONE',  ( -13.97604488694547697, 13.89961937509957934, 68.12609039468563310 ) ) ;
#32854=CARTESIAN_POINT ( 'NONE',  ( -19.03943276465977164, 0.05219959533909376836, 51.24890960531436690 ) ) ;
#32855=CARTESIAN_POINT ( 'NONE',  ( 16.52544592524342804, -4.483927247898539470, 68.54057627198103830 ) ) ;
#32856=CARTESIAN_POINT ( 'NONE',  ( -8.314922557960811034, -14.29746914071050412, 72.08224293864769550 ) ) ;
#32857=CARTESIAN_POINT ( 'NONE',  ( 19.05341960407611168, 5.049401038298154454, 78.95724293864769550 ) ) ;
#32858=CARTESIAN_POINT ( 'NONE',  ( 21.52544592524344225, -5.823673210054117533, 103.5405762719810383 ) ) ;
#32859=CARTESIAN_POINT ( 'NONE',  ( -13.89961937509977652, 13.97604488694528158, 65.62390960531436690 ) ) ;
#32860=CARTESIAN_POINT ( 'NONE',  ( 15.80617190586769283, -15.72974639402175789, 110.6260903946857042 ) ) ;
#32861=CARTESIAN_POINT ( 'NONE',  ( -16.51473224551069308, -9.474510206698971260, 41.66557627198103120 ) ) ;
#32862=CARTESIAN_POINT ( 'NONE',  ( 8.314922557961029526, -14.29746914071037800, 105.4177570613523613 ) ) ;
#32863=CARTESIAN_POINT ( 'NONE',  ( -14.29746914071049879, 8.314922557960819915, 115.8322429386477097 ) ) ;
#32864=CARTESIAN_POINT ( 'NONE',  ( -0.05219959533936034679, 19.03943276465977164, 107.5010903946856615 ) ) ;
#32866=CARTESIAN_POINT ( 'NONE',  ( 0.05219959533937995610, -21.53943276465977519, 25.00109039468567218 ) ) ;
#32867=CARTESIAN_POINT ( 'NONE',  ( 5.049401038297881783, 19.05341960407617563, 67.29275706135234714 ) ) ;
#32868=CARTESIAN_POINT ( 'NONE',  ( 16.53943276465976808, -0.05219959533910856209, 23.74890960531435269 ) ) ;
#32869=CARTESIAN_POINT ( 'NONE',  ( -15.80617190586745835, -15.72974639402198527, 76.87390960531439532 ) ) ;
#32870=CARTESIAN_POINT ( 'NONE',  ( -5.049401038298153566, 19.05341960407611168, 115.2072429386477097 ) ) ;
#32871=CARTESIAN_POINT ( 'NONE',  ( -16.52544592524342804, 4.483927247898546575, 51.04057627198103120 ) ) ;
#32872=CARTESIAN_POINT ( 'NONE',  ( 13.97604488694527802, 13.89961937509977652, 24.37390960531435624 ) ) ;
#32873=CARTESIAN_POINT ( 'NONE',  ( 19.05341960407611168, 5.049401038298154454, 28.95724293864769550 ) ) ;
#32874=CARTESIAN_POINT ( 'NONE',  ( -19.05341960407617563, 5.049401038297882671, 28.54275706135232937 ) ) ;
#32875=CARTESIAN_POINT ( 'NONE',  ( -8.314922557961024197, 14.29746914071037800, 82.91775706135234714 ) ) ;
#32876=CARTESIAN_POINT ( 'NONE',  ( 4.379528057220092307, 16.55341960407617563, 57.29275706135234714 ) ) ;
#32877=CARTESIAN_POINT ( 'NONE',  ( -9.564922557960796823, -16.46253265017161027, 112.0822429386476955 ) ) ;
#32878=CARTESIAN_POINT ( 'NONE',  ( -5.049401038298153566, 19.05341960407611168, 55.20724293864769550 ) ) ;
#32879=CARTESIAN_POINT ( 'NONE',  ( -5.719274019375665041, -21.55341960407619695, 109.7927570613523613 ) ) ;
#32880=CARTESIAN_POINT ( 'NONE',  ( 19.03943276465977164, -0.05219959533909143690, 83.74890960531436690 ) ) ;
#32881=CARTESIAN_POINT ( 'NONE',  ( 16.52544592524335698, 4.483927247898782831, 56.45942372801902565 ) ) ;
#32882=CARTESIAN_POINT ( 'NONE',  ( -16.53943276465976808, 0.05219959533911058130, 111.2489096053143669 ) ) ;
#32883=CARTESIAN_POINT ( 'NONE',  ( -14.34966873604960291, -8.224510206698953496, 26.66557627198103475 ) ) ;
#32885=CARTESIAN_POINT ( 'NONE',  ( -21.55341960407619339, 5.719274019375674811, 63.54275706135234003 ) ) ;
#32886=CARTESIAN_POINT ( 'NONE',  ( 19.02544592524343514, -5.153800228976328945, 93.54057627198102409 ) ) ;
#32887=CARTESIAN_POINT ( 'NONE',  ( -9.564922557960796823, -16.46253265017161027, 82.08224293864768129 ) ) ;
#32888=CARTESIAN_POINT ( 'NONE',  ( 19.02544592524343514, -5.153800228976328945, 113.5405762719810241 ) ) ;
#32889=CARTESIAN_POINT ( 'NONE',  ( -8.314922557960811034, -14.29746914071050412, 52.08224293864768839 ) ) ;
#32890=CARTESIAN_POINT ( 'NONE',  ( -4.379528057220328563, 16.55341960407611168, 25.20724293864769550 ) ) ;
#32891=CARTESIAN_POINT ( 'NONE',  ( 14.34966873604960469, 8.224510206698951720, 34.16557627198102409 ) ) ;
#32892=CARTESIAN_POINT ( 'NONE',  ( -8.224510206698735004, -14.34966873604973081, 44.58442372801901854 ) ) ;
#32894=CARTESIAN_POINT ( 'NONE',  ( -13.97604488694547697, 13.89961937509957934, 38.12609039468566152 ) ) ;
#32895=CARTESIAN_POINT ( 'NONE',  ( 13.97604488694527802, 13.89961937509977652, 79.37390960531435269 ) ) ;
#32896=CARTESIAN_POINT ( 'NONE',  ( -9.564922557961040184, 16.46253265017147172, 57.91775706135233293 ) ) ;
#32897=CARTESIAN_POINT ( 'NONE',  ( 9.474510206698729675, 16.51473224551082808, 62.08442372801899722 ) ) ;
#32898=CARTESIAN_POINT ( 'NONE',  ( 13.89961937509957401, 13.97604488694547697, 96.87609039468566152 ) ) ;
#32899=CARTESIAN_POINT ( 'NONE',  ( -16.53943276465976808, -0.05219959533934237506, 88.75109039468567573 ) ) ;
#32900=CARTESIAN_POINT ( 'NONE',  ( -5.153800228976328057, -19.02544592524343514, 32.29057627198102409 ) ) ;
#32901=CARTESIAN_POINT ( 'NONE',  ( 9.474510206698971260, -16.51473224551069308, 107.9155762719810383 ) ) ;
#32902=CARTESIAN_POINT ( 'NONE',  ( 5.823673210054444382, -21.52544592524334988, 35.20942372801901854 ) ) ;
#32903=CARTESIAN_POINT ( 'NONE',  ( 9.564922557961047289, -16.46253265017146816, 85.41775706135233293 ) ) ;
#32904=CARTESIAN_POINT ( 'NONE',  ( 17.50000000000003197, 3.964703510696900413, 23.28111287675285368 ) ) ;
#32905=CARTESIAN_POINT ( 'NONE',  ( 0.05219959533909260263, 19.03943276465977164, 59.99890960531436690 ) ) ;
#32906=CARTESIAN_POINT ( 'NONE',  ( 0.05219959533909260263, 19.03943276465977164, 104.9989096053143669 ) ) ;
#32907=CARTESIAN_POINT ( 'NONE',  ( 8.224510206698953496, -14.34966873604960469, 67.91557627198102409 ) ) ;
#32908=CARTESIAN_POINT ( 'NONE',  ( -19.05341960407611168, -5.049401038298163336, 46.45724293864768129 ) ) ;
#32909=CARTESIAN_POINT ( 'NONE',  ( -9.564922557960796823, -16.46253265017161027, 67.08224293864769550 ) ) ;
#32910=CARTESIAN_POINT ( 'NONE',  ( -9.564922557961040184, 16.46253265017147172, 67.91775706135233293 ) ) ;
#32911=CARTESIAN_POINT ( 'NONE',  ( 13.97604488694548053, -13.89961937509957401, 30.62609039468566863 ) ) ;
#32912=CARTESIAN_POINT ( 'NONE',  ( -9.474510206698720793, -16.51473224551083518, 44.58442372801900433 ) ) ;
#32913=CARTESIAN_POINT ( 'NONE',  ( 16.46253265017160672, -9.564922557960803928, 78.33224293864769550 ) ) ;
#32914=CARTESIAN_POINT ( 'NONE',  ( 5.719274019375991003, -21.55341960407610458, 77.70724293864770971 ) ) ;
#32915=CARTESIAN_POINT ( 'NONE',  ( -4.379528057220328563, 16.55341960407611168, 65.20724293864768129 ) ) ;
#32916=CARTESIAN_POINT ( 'NONE',  ( 19.05341960407617918, -5.049401038297876454, 31.04275706135232227 ) ) ;
#32917=CARTESIAN_POINT ( 'NONE',  ( -5.719274019375978568, 21.55341960407610458, 40.20724293864769550 ) ) ;
#32918=CARTESIAN_POINT ( 'NONE',  ( 10.81492255796078972, 18.62759615963270932, 39.58224293864769550 ) ) ;
#32919=CARTESIAN_POINT ( 'NONE',  ( -16.51473224551069308, -9.474510206698971260, 61.66557627198103120 ) ) ;
#32920=CARTESIAN_POINT ( 'NONE',  ( -16.46253265017160317, 9.564922557960807481, 40.83224293864769550 ) ) ;
#32921=CARTESIAN_POINT ( 'NONE',  ( -13.97604488694527625, -13.89961937509977652, 21.87390960531435979 ) ) ;
#32922=CARTESIAN_POINT ( 'NONE',  ( -10.72451020669870658, -18.67979575497194134, 24.58442372801901499 ) ) ;
#32923=CARTESIAN_POINT ( 'NONE',  ( 19.05341960407611168, 5.049401038298154454, 113.9572429386477097 ) ) ;
#32924=CARTESIAN_POINT ( 'NONE',  ( -15.80617190586768217, 15.72974639402176855, 33.12609039468569705 ) ) ;
#32925=CARTESIAN_POINT ( 'NONE',  ( 19.05341960407611168, 5.049401038298154454, 33.95724293864769550 ) ) ;
#32926=CARTESIAN_POINT ( 'NONE',  ( 18.67979575497178502, 10.72451020669898547, 104.1655762719810241 ) ) ;
#32927=CARTESIAN_POINT ( 'NONE',  ( 5.049401038297881783, 19.05341960407617563, 52.29275706135234003 ) ) ;
#32928=CARTESIAN_POINT ( 'NONE',  ( 9.564922557960805705, 16.46253265017160317, 24.58224293864769194 ) ) ;
#32929=CARTESIAN_POINT ( 'NONE',  ( 0.05219959533909260263, 19.03943276465977164, 24.99890960531435269 ) ) ;
#32931=CARTESIAN_POINT ( 'NONE',  ( -4.379528057220086978, -16.55341960407618274, 59.79275706135234714 ) ) ;
#32932=CARTESIAN_POINT ( 'NONE',  ( -16.51473224551069308, -9.474510206698971260, 31.66557627198102054 ) ) ;
#32934=CARTESIAN_POINT ( 'NONE',  ( 19.03943276465977164, -0.05219959533909143690, 78.74890960531436690 ) ) ;
#32935=CARTESIAN_POINT ( 'NONE',  ( -16.53943276465976808, 0.05219959533911058130, 106.2489096053143811 ) ) ;
#32936=VECTOR ( 'NONE', #3060, 1000.000000000000000 ) ;
#32937=CARTESIAN_POINT ( 'NONE',  ( -18.67979575497178146, -10.72451020669898902, 41.66557627198103120 ) ) ;
#32938=CARTESIAN_POINT ( 'NONE',  ( 8.224510206698953496, -14.34966873604960469, 77.91557627198102409 ) ) ;
#32939=CARTESIAN_POINT ( 'NONE',  ( -0.05219959533934338120, 16.53943276465976808, 37.50109039468568284 ) ) ;
#32940=CARTESIAN_POINT ( 'NONE',  ( 21.52544592524334988, 5.823673210054432836, 81.45942372801900433 ) ) ;
#32941=CARTESIAN_POINT ( 'NONE',  ( 5.049401038298161559, -19.05341960407611168, 22.70724293864769194 ) ) ;
#32942=CARTESIAN_POINT ( 'NONE',  ( 14.34966873604972726, -8.224510206698740333, 110.8344237280190043 ) ) ;
#32943=CARTESIAN_POINT ( 'NONE',  ( -14.34966873604960291, -8.224510206698953496, 51.66557627198102409 ) ) ;
#32944=CARTESIAN_POINT ( 'NONE',  ( -13.97604488694527625, -13.89961937509977652, 56.87390960531434558 ) ) ;
#32945=CARTESIAN_POINT ( 'NONE',  ( -10.81492255796105439, 18.62759615963255655, 92.91775706135236135 ) ) ;
#32946=CARTESIAN_POINT ( 'NONE',  ( 5.823673210054125526, 21.52544592524343514, 109.7905762719810383 ) ) ;
#32947=CARTESIAN_POINT ( 'NONE',  ( 21.52544592524334988, 5.823673210054432836, 76.45942372801901854 ) ) ;
#32948=CARTESIAN_POINT ( 'NONE',  ( 16.53943276465976808, 0.05219959533934440121, 36.25109039468567573 ) ) ;
#32949=CARTESIAN_POINT ( 'NONE',  ( -12.14591786802309592, -12.06949235617757132, 71.87390960531438111 ) ) ;
#32950=CARTESIAN_POINT ( 'NONE',  ( 21.53943276465977519, 0.05219959533937863772, 86.25109039468568994 ) ) ;
#32951=CARTESIAN_POINT ( 'NONE',  ( -16.52544592524335698, -4.483927247898792601, 108.9594237280190185 ) ) ;
#32952=CARTESIAN_POINT ( 'NONE',  ( -19.03943276465977164, 0.05219959533909376836, 21.24890960531436335 ) ) ;
#32953=CARTESIAN_POINT ( 'NONE',  ( -4.483927247898782831, 16.52544592524335698, 37.70942372801900433 ) ) ;
#32954=CARTESIAN_POINT ( 'NONE',  ( 14.29746914071049879, -8.314922557960816363, 43.33224293864769550 ) ) ;
#32955=CARTESIAN_POINT ( 'NONE',  ( 14.29746914071037800, 8.314922557961029526, 86.66775706135234714 ) ) ;
#32956=CARTESIAN_POINT ( 'NONE',  ( 9.564922557960805705, 16.46253265017160317, 104.5822429386476955 ) ) ;
#32957=CARTESIAN_POINT ( 'NONE',  ( 16.46253265017160672, -9.564922557960803928, 103.3322429386476955 ) ) ;
#32958=CARTESIAN_POINT ( 'NONE',  ( -15.72974639402176322, -15.80617190586768395, 94.37609039468568994 ) ) ;
#32960=CARTESIAN_POINT ( 'NONE',  ( 4.379528057220092307, 16.55341960407617563, 107.2927570613523471 ) ) ;
#32961=CARTESIAN_POINT ( 'NONE',  ( 8.314922557960818139, 14.29746914071049879, 74.58224293864768129 ) ) ;
#32962=CARTESIAN_POINT ( 'NONE',  ( -16.46253265017160317, 9.564922557960807481, 75.83224293864769550 ) ) ;
#32964=CARTESIAN_POINT ( 'NONE',  ( 8.314922557961029526, -14.29746914071037800, 20.41775706135234714 ) ) ;
#32965=CARTESIAN_POINT ( 'NONE',  ( 13.89961937509977652, -13.97604488694527269, 28.12390960531435624 ) ) ;
#32966=CARTESIAN_POINT ( 'NONE',  ( -13.89961937509977652, 13.97604488694528158, 95.62390960531436690 ) ) ;
#32967=CARTESIAN_POINT ( 'NONE',  ( 14.29746914071037800, 8.314922557961029526, 31.66775706135234358 ) ) ;
#32969=CARTESIAN_POINT ( 'NONE',  ( -16.46253265017146816, -9.564922557961047289, 34.16775706135233293 ) ) ;
#32970=CARTESIAN_POINT ( 'NONE',  ( -12.06949235617739369, -12.14591786802326823, 99.37609039468568994 ) ) ;
#32971=CARTESIAN_POINT ( 'NONE',  ( -9.564922557961040184, 16.46253265017147172, 107.9177570613523471 ) ) ;
#32972=CARTESIAN_POINT ( 'NONE',  ( 13.89961937509977652, -13.97604488694527269, 33.12390960531434558 ) ) ;
#32973=CARTESIAN_POINT ( 'NONE',  ( 12.14591786802327356, -12.06949235617739191, 80.62609039468567573 ) ) ;
#32974=CARTESIAN_POINT ( 'NONE',  ( -12.14591786802326823, 12.06949235617739902, 63.12609039468568994 ) ) ;
#32975=CARTESIAN_POINT ( 'NONE',  ( 16.46253265017160672, -9.564922557960803928, 33.33224293864770260 ) ) ;
#32976=CARTESIAN_POINT ( 'NONE',  ( 19.03943276465977164, 0.05219959533936151252, 71.25109039468566152 ) ) ;
#32977=CARTESIAN_POINT ( 'NONE',  ( 15.80617190586769283, -15.72974639402175789, 110.6260903946857042 ) ) ;
#32978=CARTESIAN_POINT ( 'NONE',  ( 16.46253265017160672, -9.564922557960803928, 43.33224293864769550 ) ) ;
#32979=CARTESIAN_POINT ( 'NONE',  ( -13.97604488694527625, -13.89961937509977652, 91.87390960531432427 ) ) ;
#32980=CARTESIAN_POINT ( 'NONE',  ( 14.29746914071049879, -8.314922557960816363, 88.33224293864769550 ) ) ;
#32981=B_SPLINE_CURVE_WITH_KNOTS ( 'NONE', 3,
 ( #157932, #50759, #51741, #6227, #129559, #158911, #191258, #128569, #190264, #140762, #34587, #111425, #173111, #96244, #110426, #112416, #83065, #113402, #79089, #97224 ),
 .UNSPECIFIED., .F., .F.,
 ( 4, 2, 2, 2, 2, 2, 2, 2, 2, 4 ),
 ( 0.000000000000000000, 0.0004987090165372478744, 0.0009974180330744957489, 0.001246772541343130420, 0.001496127049611765090, 0.001994836066149034866, 0.002493545082686304207, 0.002742899590954927386, 0.002992254099223550130, 0.003989672132298028098 ),
 .UNSPECIFIED. ) ;
#32982=CARTESIAN_POINT ( 'NONE',  ( -16.51473224551082808, 9.474510206698731452, 48.33442372801900433 ) ) ;
#32983=CARTESIAN_POINT ( 'NONE',  ( -21.55341960407610458, -5.719274019375992779, 51.45724293864770260 ) ) ;
#32984=CARTESIAN_POINT ( 'NONE',  ( -13.89961937509957401, -13.97604488694547875, 19.37609039468566507 ) ) ;
#32985=CARTESIAN_POINT ( 'NONE',  ( 13.97604488694527802, 13.89961937509977652, 84.37390960531433848 ) ) ;
#32986=CARTESIAN_POINT ( 'NONE',  ( -5.049401038297874678, -19.05341960407617918, 29.79275706135232227 ) ) ;
#32987=CARTESIAN_POINT ( 'NONE',  ( 15.72974639402199770, -15.80617190586745480, 68.12390960531436690 ) ) ;
#32988=CARTESIAN_POINT ( 'NONE',  ( -16.46253265017160317, 9.564922557960807481, 105.8322429386476955 ) ) ;
#32989=CARTESIAN_POINT ( 'NONE',  ( -5.153800228976607833, 19.02544592524334988, 87.70942372801897591 ) ) ;
#32990=CARTESIAN_POINT ( 'NONE',  ( -5.049401038298153566, 19.05341960407611168, 110.2072429386476671 ) ) ;
#32991=CARTESIAN_POINT ( 'NONE',  ( 5.049401038297881783, 19.05341960407617563, 107.2927570613523187 ) ) ;
#32992=CARTESIAN_POINT ( 'NONE',  ( 14.29746914071049879, -8.314922557960816363, 113.3322429386476955 ) ) ;
#32993=CARTESIAN_POINT ( 'NONE',  ( 16.46253265017160672, -9.564922557960803928, 98.33224293864769550 ) ) ;
#32994=CARTESIAN_POINT ( 'NONE',  ( -5.719274019375978568, 21.55341960407610458, 80.20724293864769550 ) ) ;
#32995=CARTESIAN_POINT ( 'NONE',  ( -16.52544592524335698, -4.483927247898792601, 43.95942372801902565 ) ) ;
#32996=CARTESIAN_POINT ( 'NONE',  ( -5.823673210054431948, 21.52544592524334988, 52.70942372801902565 ) ) ;
#32997=CARTESIAN_POINT ( 'NONE',  ( 18.62759615963255655, 10.81492255796105972, 101.6677570613523613 ) ) ;
#32998=CARTESIAN_POINT ( 'NONE',  ( 4.379528057220092307, 16.55341960407617563, 97.29275706135234714 ) ) ;
#32999=CARTESIAN_POINT ( 'NONE',  ( -19.05341960407611168, -5.049401038298163336, 86.45724293864769550 ) ) ;
#33000=CARTESIAN_POINT ( 'NONE',  ( -8.314922557960811034, -14.29746914071050412, 97.08224293864770971 ) ) ;
#33001=CARTESIAN_POINT ( 'NONE',  ( 16.52544592524342804, -4.483927247898539470, 33.54057627198102409 ) ) ;
#33002=CARTESIAN_POINT ( 'NONE',  ( 13.97604488694548053, -13.89961937509957401, 75.62609039468564731 ) ) ;
#33003=CARTESIAN_POINT ( 'NONE',  ( 10.81492255796106328, -18.62759615963255655, 60.41775706135235424 ) ) ;
#33004=CARTESIAN_POINT ( 'NONE',  ( 5.153800228976615827, -19.02544592524334988, 20.20942372801899722 ) ) ;
#33005=CARTESIAN_POINT ( 'NONE',  ( -4.483927247898539470, -16.52544592524342804, 92.29057627198103830 ) ) ;
#33006=CARTESIAN_POINT ( 'NONE',  ( -15.80617190586745835, -15.72974639402198527, 31.87390960531435979 ) ) ;
#33007=CARTESIAN_POINT ( 'NONE',  ( 8.314922557960818139, 14.29746914071049879, 24.58224293864768839 ) ) ;
#33008=CARTESIAN_POINT ( 'NONE',  ( -5.823673210054431948, 21.52544592524334988, 82.70942372801900433 ) ) ;
#33009=CARTESIAN_POINT ( 'NONE',  ( -16.55341960407617563, 4.379528057220093196, 53.54275706135234714 ) ) ;
#33010=CARTESIAN_POINT ( 'NONE',  ( -8.314922557961024197, 14.29746914071037800, 107.9177570613523471 ) ) ;
#33011=CARTESIAN_POINT ( 'NONE',  ( 18.67979575497194134, -10.72451020669871369, 50.83442372801901143 ) ) ;
#33013=CARTESIAN_POINT ( 'NONE',  ( -18.67979575497193778, 10.72451020669871902, 33.33442372801900433 ) ) ;
#33014=CARTESIAN_POINT ( 'NONE',  ( 14.29746914071049879, -8.314922557960816363, 98.33224293864769550 ) ) ;
#33015=CARTESIAN_POINT ( 'NONE',  ( 5.049401038298161559, -19.05341960407611168, 22.70724293864769194 ) ) ;
#33016=CARTESIAN_POINT ( 'NONE',  ( 8.224510206698953496, -14.34966873604960469, 62.91557627198102409 ) ) ;
#33017=CARTESIAN_POINT ( 'NONE',  ( -9.474510206698964154, 16.51473224551069663, 65.41557627198102409 ) ) ;
#33018=CARTESIAN_POINT ( 'NONE',  ( 12.14591786802327356, -12.06949235617739191, 105.6260903946856899 ) ) ;
#33019=CARTESIAN_POINT ( 'NONE',  ( 5.823673210054125526, 21.52544592524343514, 59.79057627198103120 ) ) ;
#33020=CARTESIAN_POINT ( 'NONE',  ( -16.52544592524342804, 4.483927247898546575, 86.04057627198102409 ) ) ;
#33021=CARTESIAN_POINT ( 'NONE',  ( -18.62759615963270932, 10.81492255796079327, 95.83224293864770971 ) ) ;
#33022=CARTESIAN_POINT ( 'NONE',  ( -19.03943276465977164, 0.05219959533909376836, 96.24890960531436690 ) ) ;
#33023=CARTESIAN_POINT ( 'NONE',  ( -16.51473224551069308, -9.474510206698971260, 56.66557627198103120 ) ) ;
#33024=CARTESIAN_POINT ( 'NONE',  ( 19.03943276465977164, 0.05219959533936151252, 101.2510903946856757 ) ) ;
#33025=CARTESIAN_POINT ( 'NONE',  ( 5.719274019375991003, -21.55341960407610458, 37.70724293864769550 ) ) ;
#33026=CARTESIAN_POINT ( 'NONE',  ( -5.823673210054431948, 21.52544592524334988, 62.70942372801902565 ) ) ;
#33027=CARTESIAN_POINT ( 'NONE',  ( 19.03943276465977164, -0.05219959533909143690, 48.74890960531435979 ) ) ;
#33028=CARTESIAN_POINT ( 'NONE',  ( 19.03943276465977164, -0.05219959533909143690, 88.74890960531436690 ) ) ;
#33029=CARTESIAN_POINT ( 'NONE',  ( 8.314922557961029526, -14.29746914071037800, 60.41775706135235424 ) ) ;
#33030=CARTESIAN_POINT ( 'NONE',  ( 21.55341960407619695, -5.719274019375665929, 46.04275706135234714 ) ) ;
#33031=CARTESIAN_POINT ( 'NONE',  ( -18.62759615963255300, -10.81492255796106328, 89.16775706135236135 ) ) ;
#33032=CARTESIAN_POINT ( 'NONE',  ( 5.823673210054125526, 21.52544592524343514, 104.7905762719810241 ) ) ;
#33033=CARTESIAN_POINT ( 'NONE',  ( -0.05219959533937732626, 21.53943276465977519, 32.50109039468568284 ) ) ;
#33034=CARTESIAN_POINT ( 'NONE',  ( 16.53943276465976808, 0.05219959533934440121, 61.25109039468567573 ) ) ;
#33035=B_SPLINE_CURVE_WITH_KNOTS ( 'NONE', 3,
 ( #6438, #129772, #22630, #144957, #160138, #114621 ),
 .UNSPECIFIED., .F., .F.,
 ( 4, 2, 4 ),
 ( 0.003239945802372206588, 0.003620412082092015413, 0.004000878361811823804 ),
 .UNSPECIFIED. ) ;
#33036=CARTESIAN_POINT ( 'NONE',  ( 21.53943276465977519, -0.05219959533907433946, 73.74890960531433848 ) ) ;
#33037=CARTESIAN_POINT ( 'NONE',  ( 16.46253265017146816, 9.564922557961045513, 36.66775706135233293 ) ) ;
#33038=CARTESIAN_POINT ( 'NONE',  ( -5.049401038298153566, 19.05341960407611168, 65.20724293864765286 ) ) ;
#33039=CARTESIAN_POINT ( 'NONE',  ( 4.379528057220339221, -16.55341960407611168, 22.70724293864769194 ) ) ;
#33041=CARTESIAN_POINT ( 'NONE',  ( -9.564922557960796823, -16.46253265017161027, 97.08224293864769550 ) ) ;
#33043=CARTESIAN_POINT ( 'NONE',  ( 5.049401038297881783, 19.05341960407617563, 87.29275706135234714 ) ) ;
#33044=CARTESIAN_POINT ( 'NONE',  ( -18.67979575497178146, -10.72451020669898902, 56.66557627198103830 ) ) ;
#33045=CARTESIAN_POINT ( 'NONE',  ( 12.14591786802309770, 12.06949235617756955, 44.37390960531435979 ) ) ;
#33046=CARTESIAN_POINT ( 'NONE',  ( 19.03943276465977164, 0.05219959533936151252, 111.2510903946856757 ) ) ;
#33047=CARTESIAN_POINT ( 'NONE',  ( 19.05341960407611168, 5.049401038298154454, 33.95724293864769550 ) ) ;
#33048=CARTESIAN_POINT ( 'NONE',  ( 12.14591786802327356, -12.06949235617739191, 20.62609039468568639 ) ) ;
#33049=CARTESIAN_POINT ( 'NONE',  ( -18.62759615963270932, 10.81492255796079327, 95.83224293864770971 ) ) ;
#33050=CARTESIAN_POINT ( 'NONE',  ( 13.89961937509957401, 13.97604488694547697, 71.87609039468567573 ) ) ;
#33051=CARTESIAN_POINT ( 'NONE',  ( 12.06949235617739724, 12.14591786802326823, 76.87609039468567573 ) ) ;
#33052=CARTESIAN_POINT ( 'NONE',  ( 5.049401038298161559, -19.05341960407611168, 67.70724293864769550 ) ) ;
#33053=CARTESIAN_POINT ( 'NONE',  ( 12.14591786802309770, 12.06949235617756955, 74.37390960531436690 ) ) ;
#33054=CARTESIAN_POINT ( 'NONE',  ( -5.049401038298153566, 19.05341960407611168, 55.20724293864769550 ) ) ;
#33055=CARTESIAN_POINT ( 'NONE',  ( 8.224510206698953496, -14.34966873604960469, 72.91557627198103830 ) ) ;
#33056=FACE_BOUND ( 'NONE', #183865, .T. ) ;
#33058=CARTESIAN_POINT ( 'NONE',  ( 4.379528057220339221, -16.55341960407611168, 47.70724293864770260 ) ) ;
#33059=CARTESIAN_POINT ( 'NONE',  ( 9.564922557960805705, 16.46253265017160317, 74.58224293864769550 ) ) ;
#33061=CARTESIAN_POINT ( 'NONE',  ( 5.049401038297881783, 19.05341960407617563, 32.29275706135233293 ) ) ;
#33062=CARTESIAN_POINT ( 'NONE',  ( 16.53943276465976808, 0.05219959533934440121, 46.25109039468567573 ) ) ;
#33063=CARTESIAN_POINT ( 'NONE',  ( -21.53943276465977519, 0.05219959533907696930, 66.24890960531436690 ) ) ;
#33064=CARTESIAN_POINT ( 'NONE',  ( -19.03943276465977164, -0.05219959533935918106, 23.75109039468566152 ) ) ;
#33065=CARTESIAN_POINT ( 'NONE',  ( -13.89961937509977652, 13.97604488694528158, 70.62390960531432427 ) ) ;
#33067=CARTESIAN_POINT ( 'NONE',  ( -9.564922557960796823, -16.46253265017161027, 112.0822429386476955 ) ) ;
#33068=CARTESIAN_POINT ( 'NONE',  ( -5.823673210054431948, 21.52544592524334988, 32.70942372801900433 ) ) ;
#33069=CARTESIAN_POINT ( 'NONE',  ( -0.05219959533910754901, -16.53943276465976808, 102.4989096053143811 ) ) ;
#33070=CARTESIAN_POINT ( 'NONE',  ( -21.55341960407610458, -5.719274019375992779, 106.4572429386477097 ) ) ;
#33071=CARTESIAN_POINT ( 'NONE',  ( -9.474510206698964154, 16.51473224551069663, 85.41557627198102409 ) ) ;
#33073=CARTESIAN_POINT ( 'NONE',  ( -15.72974639402176322, -15.80617190586768395, 29.37609039468568284 ) ) ;
#33075=CARTESIAN_POINT ( 'NONE',  ( 9.474510206698971260, -16.51473224551069308, 87.91557627198102409 ) ) ;
#33077=CARTESIAN_POINT ( 'NONE',  ( 15.80617190586746368, 15.72974639402197994, 99.37390960531436690 ) ) ;
#33078=CARTESIAN_POINT ( 'NONE',  ( -5.153800228976328057, -19.02544592524343514, 32.29057627198102409 ) ) ;
#33079=CARTESIAN_POINT ( 'NONE',  ( -5.153800228976607833, 19.02544592524334988, 107.7094237280189759 ) ) ;
#33081=CARTESIAN_POINT ( 'NONE',  ( -0.05219959533909027116, -19.03943276465977164, 32.49890960531435979 ) ) ;
#33082=CARTESIAN_POINT ( 'NONE',  ( 15.80617190586769283, -15.72974639402175789, 85.62609039468568994 ) ) ;
#33083=CARTESIAN_POINT ( 'NONE',  ( -13.97604488694527625, -13.89961937509977652, 76.87390960531433848 ) ) ;
#33084=CARTESIAN_POINT ( 'NONE',  ( 21.53943276465977519, 0.05219959533937863772, 46.25109039468567573 ) ) ;
#33085=CARTESIAN_POINT ( 'NONE',  ( 15.72974639402176855, 15.80617190586768217, 21.87609039468567573 ) ) ;
#33087=CARTESIAN_POINT ( 'NONE',  ( -5.153800228976328057, -19.02544592524343514, 92.29057627198099567 ) ) ;
#33089=CARTESIAN_POINT ( 'NONE',  ( 8.314922557961029526, -14.29746914071037800, 45.41775706135234003 ) ) ;
#33090=CARTESIAN_POINT ( 'NONE',  ( 10.72451020669898902, -18.67979575497178502, 47.91557627198102409 ) ) ;
#33091=CARTESIAN_POINT ( 'NONE',  ( 15.80617190586769283, -15.72974639402175789, 40.62609039468567573 ) ) ;
#33092=CARTESIAN_POINT ( 'NONE',  ( 0.05219959533937995610, -21.53943276465977519, 70.00109039468568994 ) ) ;
#33094=CARTESIAN_POINT ( 'NONE',  ( 19.03943276465977164, 0.05219959533936151252, 111.2510903946856757 ) ) ;
#33095=CARTESIAN_POINT ( 'NONE',  ( 16.51473224551069308, 9.474510206698969483, 64.16557627198102409 ) ) ;
#33096=CARTESIAN_POINT ( 'NONE',  ( 16.51473224551069308, 9.474510206698969483, 89.16557627198103830 ) ) ;
#33097=CARTESIAN_POINT ( 'NONE',  ( 0.05219959533910956823, 16.53943276465976808, 109.9989096053143527 ) ) ;
#33098=CARTESIAN_POINT ( 'NONE',  ( -12.14591786802309592, -12.06949235617757132, 101.8739096053143811 ) ) ;
#33099=CARTESIAN_POINT ( 'NONE',  ( 13.97604488694527802, 13.89961937509977652, 114.3739096053143669 ) ) ;
#33100=CARTESIAN_POINT ( 'NONE',  ( 4.379528057220092307, 16.55341960407617563, 77.29275706135234714 ) ) ;
#33101=CARTESIAN_POINT ( 'NONE',  ( 16.52544592524342804, -4.483927247898539470, 68.54057627198103830 ) ) ;
#33102=CARTESIAN_POINT ( 'NONE',  ( 19.03943276465977164, -0.05219959533909143690, 48.74890960531435979 ) ) ;
#33103=CARTESIAN_POINT ( 'NONE',  ( -18.62759615963255300, -10.81492255796106328, 79.16775706135234714 ) ) ;
#33104=CARTESIAN_POINT ( 'NONE',  ( 15.80617190586769283, -15.72974639402175789, 70.62609039468567573 ) ) ;
#33105=CARTESIAN_POINT ( 'NONE',  ( -16.46253265017146816, -9.564922557961047289, 109.1677570613523471 ) ) ;
#33106=CARTESIAN_POINT ( 'NONE',  ( 8.314922557960818139, 14.29746914071049879, 59.58224293864770260 ) ) ;
#33107=CARTESIAN_POINT ( 'NONE',  ( 21.52544592524334988, 5.823673210054432836, 21.45942372801901499 ) ) ;
#33108=CARTESIAN_POINT ( 'NONE',  ( 21.53943276465977519, -0.05219959533907433946, 58.74890960531436690 ) ) ;
#33109=CARTESIAN_POINT ( 'NONE',  ( -16.21995358207304605, -7.366697692864190294, 105.0644899848784490 ) ) ;
#33111=CARTESIAN_POINT ( 'NONE',  ( 16.46253265017160672, -9.564922557960803928, 73.33224293864769550 ) ) ;
#33112=CARTESIAN_POINT ( 'NONE',  ( 16.53943276465976808, -0.05219959533910856209, 33.74890960531436690 ) ) ;
#33113=CARTESIAN_POINT ( 'NONE',  ( -12.14591786802326823, 12.06949235617739902, 113.1260903946856899 ) ) ;
#33114=CARTESIAN_POINT ( 'NONE',  ( 14.29746914071037800, 8.314922557961029526, 91.66775706135234714 ) ) ;
#33115=CARTESIAN_POINT ( 'NONE',  ( 0.05219959533936267826, -19.03943276465977164, 50.00109039468566863 ) ) ;
#33116=CARTESIAN_POINT ( 'NONE',  ( 16.21995358207306381, 7.366697692864114799, 47.56448998487843483 ) ) ;
#33117=CARTESIAN_POINT ( 'NONE',  ( 5.153800228976335163, 19.02544592524342804, 104.7905762719809957 ) ) ;
#33118=CARTESIAN_POINT ( 'NONE',  ( 4.483927247898545687, 16.52544592524342804, 64.79057627198103830 ) ) ;
#33119=CARTESIAN_POINT ( 'NONE',  ( 16.46253265017160672, -9.564922557960803928, 23.33224293864769194 ) ) ;
#33120=CARTESIAN_POINT ( 'NONE',  ( -5.153800228976328057, -19.02544592524343514, 112.2905762719810099 ) ) ;
#33121=CARTESIAN_POINT ( 'NONE',  ( -0.05219959533907301413, -21.53943276465977519, 57.49890960531435979 ) ) ;
#33123=CARTESIAN_POINT ( 'NONE',  ( -14.34966873604960291, -8.224510206698953496, 101.6655762719810383 ) ) ;
#33124=CARTESIAN_POINT ( 'NONE',  ( -16.52544592524335698, -4.483927247898792601, 48.95942372801902565 ) ) ;
#33125=B_SPLINE_CURVE_WITH_KNOTS ( 'NONE', 3,
 ( #132826, #164179, #25677, #24670, #7467, #85307, #53992, #87322, #148007, #54988, #115665, #165174, #69151, #130817, #177355, #9497, #149006, #118670, #10495, #134845, #72156, #88309, #11503, #133831, #73174, #38825, #56995, #180361, #100483, #41829, #162162, #116657 ),
 .UNSPECIFIED., .F., .F.,
 ( 4, 2, 2, 2, 2, 2, 2, 2, 2, 2, 2, 2, 2, 2, 2, 4 ),
 ( 5.204170427930422054E-18, 0.0003712461730036866695, 0.0007424923460073681349, 0.001113738519011049600, 0.001484984692014731066, 0.002227477038022093996, 0.002598723211025772209, 0.002969969384029450422, 0.003341215557033128634, 0.003712461730036806414, 0.004083707903040484193, 0.004454954076044162839, 0.004826200249047841485, 0.005197446422051519264, 0.005568692595055197911, 0.005939938768058875690 ),
 .UNSPECIFIED. ) ;
#33126=CARTESIAN_POINT ( 'NONE',  ( -0.05219959533910754901, -16.53943276465976808, 87.49890960531436690 ) ) ;
#33127=CARTESIAN_POINT ( 'NONE',  ( -19.01533133064925352, 5.499999999999452882, 63.76586590595741200 ) ) ;
#33128=CARTESIAN_POINT ( 'NONE',  ( 5.153800228976615827, -19.02544592524334988, 80.20942372801901854 ) ) ;
#33129=CARTESIAN_POINT ( 'NONE',  ( -9.474510206698964154, 16.51473224551069663, 110.4155762719810383 ) ) ;
#33132=CARTESIAN_POINT ( 'NONE',  ( -4.379528057220086978, -16.55341960407618274, 44.79275706135234714 ) ) ;
#33133=CARTESIAN_POINT ( 'NONE',  ( 0.05219959533910956823, 16.53943276465976808, 34.99890960531435979 ) ) ;
#33134=CARTESIAN_POINT ( 'NONE',  ( -0.05219959533907301413, -21.53943276465977519, 57.49890960531435979 ) ) ;
#33135=CARTESIAN_POINT ( 'NONE',  ( 9.474510206698729675, 16.51473224551082808, 87.08442372801900433 ) ) ;
#33136=CARTESIAN_POINT ( 'NONE',  ( 10.72451020669898902, -18.67979575497178502, 47.91557627198102409 ) ) ;
#33137=CARTESIAN_POINT ( 'NONE',  ( -5.823673210054431948, 21.52544592524334988, 87.70942372801901854 ) ) ;
#33139=CARTESIAN_POINT ( 'NONE',  ( -14.34966873604972548, 8.224510206698743886, 33.33442372801900433 ) ) ;
#33140=CARTESIAN_POINT ( 'NONE',  ( -9.564922557960796823, -16.46253265017161027, 42.08224293864769550 ) ) ;
#33141=CARTESIAN_POINT ( 'NONE',  ( -16.46253265017160317, 9.564922557960807481, 100.8322429386477097 ) ) ;
#33142=CARTESIAN_POINT ( 'NONE',  ( 16.46253265017160672, -9.564922557960803928, 33.33224293864770260 ) ) ;
#33143=CARTESIAN_POINT ( 'NONE',  ( -12.06949235617756955, 12.14591786802309770, 95.62390960531436690 ) ) ;
#33145=CARTESIAN_POINT ( 'NONE',  ( 19.03943276465977164, -0.05219959533909143690, 98.74890960531436690 ) ) ;
#33147=CARTESIAN_POINT ( 'NONE',  ( -16.55341960407617563, 4.379528057220093196, 53.54275706135234714 ) ) ;
#33148=CARTESIAN_POINT ( 'NONE',  ( -21.53943276465977519, 0.05219959533907696930, 86.24890960531436690 ) ) ;
#33149=CARTESIAN_POINT ( 'NONE',  ( 19.05341960407611168, 5.049401038298154454, 48.95724293864768129 ) ) ;
#33150=CARTESIAN_POINT ( 'NONE',  ( 21.52544592524334988, 5.823673210054432836, 21.45942372801901499 ) ) ;
#33151=CARTESIAN_POINT ( 'NONE',  ( -9.564922557960796823, -16.46253265017161027, 82.08224293864768129 ) ) ;
#33152=CARTESIAN_POINT ( 'NONE',  ( 0.05219959533909260263, 19.03943276465977164, 114.9989096053143669 ) ) ;
#33154=CARTESIAN_POINT ( 'NONE',  ( 4.379528057220092307, 16.55341960407617563, 47.29275706135234003 ) ) ;
#33155=CARTESIAN_POINT ( 'NONE',  ( -0.05219959533937732626, 21.53943276465977519, 22.50109039468567573 ) ) ;
#33156=CARTESIAN_POINT ( 'NONE',  ( -9.474510206698964154, 16.51473224551069663, 25.41557627198103120 ) ) ;
#33157=CARTESIAN_POINT ( 'NONE',  ( 19.05341960407611168, 5.049401038298154454, 98.95724293864766707 ) ) ;
#33158=CARTESIAN_POINT ( 'NONE',  ( -13.89961937509957401, -13.97604488694547875, 69.37609039468564731 ) ) ;
#33159=CARTESIAN_POINT ( 'NONE',  ( -13.97604488694547697, 13.89961937509957934, 23.12609039468565442 ) ) ;
#33160=CARTESIAN_POINT ( 'NONE',  ( 21.55341960407610458, 5.719274019375980345, 83.95724293864770971 ) ) ;
#33161=CARTESIAN_POINT ( 'NONE',  ( 19.05341960407617918, -5.049401038297876454, 31.04275706135232227 ) ) ;
#33162=CARTESIAN_POINT ( 'NONE',  ( -4.483927247898782831, 16.52544592524335698, 82.70942372801900433 ) ) ;
#33163=CARTESIAN_POINT ( 'NONE',  ( 16.46253265017160672, -9.564922557960803928, 108.3322429386476955 ) ) ;
#33164=CARTESIAN_POINT ( 'NONE',  ( 16.46253265017160672, -9.564922557960803928, 63.33224293864769550 ) ) ;
#33165=CARTESIAN_POINT ( 'NONE',  ( -18.62759615963255300, -10.81492255796106328, 64.16775706135234714 ) ) ;
#33166=ADVANCED_FACE ( 'NONE', ( #88887 ), #158561, .T. ) ;
#33167=CARTESIAN_POINT ( 'NONE',  ( -18.67979575497193778, 10.72451020669871902, 68.33442372801900433 ) ) ;
#33168=CARTESIAN_POINT ( 'NONE',  ( -5.049401038298153566, 19.05341960407611168, 75.20724293864769550 ) ) ;
#33169=CARTESIAN_POINT ( 'NONE',  ( -15.72974639402176322, -15.80617190586768395, 44.37609039468567573 ) ) ;
#33170=CARTESIAN_POINT ( 'NONE',  ( -5.153800228976607833, 19.02544592524334988, 82.70942372801897591 ) ) ;
#33171=CARTESIAN_POINT ( 'NONE',  ( 13.97604488694527802, 13.89961937509977652, 54.37390960531435979 ) ) ;
#33172=CARTESIAN_POINT ( 'NONE',  ( 9.564922557960805705, 16.46253265017160317, 104.5822429386476955 ) ) ;
#33173=CARTESIAN_POINT ( 'NONE',  ( 9.474510206698971260, -16.51473224551069308, 67.91557627198102409 ) ) ;
#33174=CARTESIAN_POINT ( 'NONE',  ( 13.89961937509977652, -13.97604488694527269, 113.1239096053143527 ) ) ;
#33175=CARTESIAN_POINT ( 'NONE',  ( -13.89961937509977652, 13.97604488694528158, 50.62390960531435979 ) ) ;
#33176=CARTESIAN_POINT ( 'NONE',  ( -18.67979575497178146, -10.72451020669898902, 96.66557627198102409 ) ) ;
#33177=CARTESIAN_POINT ( 'NONE',  ( 14.34966873604972726, -8.224510206698740333, 70.83442372801901854 ) ) ;
#33179=CARTESIAN_POINT ( 'NONE',  ( 9.474510206698729675, 16.51473224551082808, 37.08442372801899722 ) ) ;
#33180=CARTESIAN_POINT ( 'NONE',  ( -16.51473224551069308, -9.474510206698971260, 71.66557627198102409 ) ) ;
#33181=CARTESIAN_POINT ( 'NONE',  ( 4.483927247898545687, 16.52544592524342804, 64.79057627198103830 ) ) ;
#33182=CARTESIAN_POINT ( 'NONE',  ( 14.29746914071049879, -8.314922557960816363, 98.33224293864769550 ) ) ;
#33183=CARTESIAN_POINT ( 'NONE',  ( -13.89961937509977652, 13.97604488694528158, 105.6239096053143527 ) ) ;
#33184=CARTESIAN_POINT ( 'NONE',  ( -0.05219959533909027116, -19.03943276465977164, 92.49890960531436690 ) ) ;
#33185=CARTESIAN_POINT ( 'NONE',  ( 10.72451020669871369, 18.67979575497193778, 47.08442372801901854 ) ) ;
#33186=CARTESIAN_POINT ( 'NONE',  ( -5.049401038298153566, 19.05341960407611168, 105.2072429386476671 ) ) ;
#33187=CARTESIAN_POINT ( 'NONE',  ( -21.55341960407619339, 5.719274019375674811, 108.5427570613523756 ) ) ;
#33188=CARTESIAN_POINT ( 'NONE',  ( -8.314922557961024197, 14.29746914071037800, 77.91775706135231871 ) ) ;
#33189=CARTESIAN_POINT ( 'NONE',  ( -15.80617190586768217, 15.72974639402176855, 38.12609039468567573 ) ) ;
#33190=CARTESIAN_POINT ( 'NONE',  ( 21.55341960407610458, 5.719274019375980345, 33.95724293864769550 ) ) ;
#33191=CARTESIAN_POINT ( 'NONE',  ( 21.55341960407610458, 5.719274019375980345, 103.9572429386476813 ) ) ;
#33192=CARTESIAN_POINT ( 'NONE',  ( -8.314922557960811034, -14.29746914071050412, 57.08224293864769550 ) ) ;
#33193=CARTESIAN_POINT ( 'NONE',  ( -19.02544592524342804, 5.153800228976336051, 51.04057627198103120 ) ) ;
#33194=CARTESIAN_POINT ( 'NONE',  ( -4.483927247898539470, -16.52544592524342804, 87.29057627198103830 ) ) ;
#33195=CARTESIAN_POINT ( 'NONE',  ( -15.72974639402197994, 15.80617190586746368, 45.62390960531436690 ) ) ;
#33196=CARTESIAN_POINT ( 'NONE',  ( -16.46253265017146816, -9.564922557961047289, 49.16775706135233293 ) ) ;
#33198=CARTESIAN_POINT ( 'NONE',  ( -0.05219959533910754901, -16.53943276465976808, 112.4989096053143669 ) ) ;
#33199=EDGE_LOOP ( 'NONE', ( #80621, #173709 ) ) ;
#33200=CARTESIAN_POINT ( 'NONE',  ( -12.06949235617739369, -12.14591786802326823, 64.37609039468568994 ) ) ;
#33201=CARTESIAN_POINT ( 'NONE',  ( -19.05341960407611168, -5.049401038298163336, 66.45724293864769550 ) ) ;
#33203=CARTESIAN_POINT ( 'NONE',  ( 8.314922557960818139, 14.29746914071049879, 84.58224293864769550 ) ) ;
#33204=CARTESIAN_POINT ( 'NONE',  ( -21.53943276465977519, 0.05219959533907696930, 41.24890960531435269 ) ) ;
#33205=CARTESIAN_POINT ( 'NONE',  ( -12.06949235617739369, -12.14591786802326823, 104.3760903946856899 ) ) ;
#33206=CARTESIAN_POINT ( 'NONE',  ( -16.46253265017146816, -9.564922557961047289, 109.1677570613523471 ) ) ;
#33207=CARTESIAN_POINT ( 'NONE',  ( -5.823673210054431948, 21.52544592524334988, 92.70942372801901854 ) ) ;
#33208=CARTESIAN_POINT ( 'NONE',  ( -9.474510206698964154, 16.51473224551069663, 90.41557627198103830 ) ) ;
#33209=CARTESIAN_POINT ( 'NONE',  ( 21.55341960407610458, 5.719274019375980345, 103.9572429386476813 ) ) ;
#33210=CARTESIAN_POINT ( 'NONE',  ( -12.06949235617739369, -12.14591786802326823, 54.37609039468568994 ) ) ;
#33211=CARTESIAN_POINT ( 'NONE',  ( 5.049401038298161559, -19.05341960407611168, 32.70724293864768129 ) ) ;
#33212=CARTESIAN_POINT ( 'NONE',  ( 4.483927247898790824, -16.52544592524335698, 35.20942372801901854 ) ) ;
#33213=CARTESIAN_POINT ( 'NONE',  ( 5.153800228976615827, -19.02544592524334988, 90.20942372801900433 ) ) ;
#33214=CARTESIAN_POINT ( 'NONE',  ( -18.67979575497178146, -10.72451020669898902, 96.66557627198102409 ) ) ;
#33215=CARTESIAN_POINT ( 'NONE',  ( 13.89961937509957401, 13.97604488694547697, 71.87609039468567573 ) ) ;
#33216=CARTESIAN_POINT ( 'NONE',  ( 19.25663599770061296, -5.499999999999443112, 86.49419308057204603 ) ) ;
#33217=CARTESIAN_POINT ( 'NONE',  ( 10.72451020669898902, -18.67979575497178502, 102.9155762719810383 ) ) ;
#33219=CARTESIAN_POINT ( 'NONE',  ( -13.89961937509977652, 13.97604488694528158, 75.62390960531438111 ) ) ;
#33220=CARTESIAN_POINT ( 'NONE',  ( -12.06949235617739369, -12.14591786802326823, 34.37609039468568284 ) ) ;
#33221=CARTESIAN_POINT ( 'NONE',  ( -18.22780087662123805, 5.499999999999981348, 101.0176318212689495 ) ) ;
#33222=CARTESIAN_POINT ( 'NONE',  ( 9.474510206698729675, 16.51473224551082808, 62.08442372801899722 ) ) ;
#33223=CARTESIAN_POINT ( 'NONE',  ( -21.53943276465977519, -0.05219959533937600094, 23.75109039468567929 ) ) ;
#33224=CARTESIAN_POINT ( 'NONE',  ( -12.14591786802309592, -12.06949235617757132, 76.87390960531439532 ) ) ;
#33225=CARTESIAN_POINT ( 'NONE',  ( 16.51473224551069308, 9.474510206698969483, 84.16557627198102409 ) ) ;
#33226=CARTESIAN_POINT ( 'NONE',  ( -0.05219959533934338120, 16.53943276465976808, 32.50109039468568284 ) ) ;
#33227=CARTESIAN_POINT ( 'NONE',  ( 19.05341960407617918, -5.049401038297876454, 46.04275706135233293 ) ) ;
#33229=CARTESIAN_POINT ( 'NONE',  ( 5.823673210054444382, -21.52544592524334988, 50.20942372801901854 ) ) ;
#33230=CARTESIAN_POINT ( 'NONE',  ( -5.153800228976607833, 19.02544592524334988, 107.7094237280189759 ) ) ;
#33231=CARTESIAN_POINT ( 'NONE',  ( 5.049401038298161559, -19.05341960407611168, 57.70724293864769550 ) ) ;
#33232=CARTESIAN_POINT ( 'NONE',  ( 5.049401038297881783, 19.05341960407617563, 77.29275706135231871 ) ) ;
#33233=CARTESIAN_POINT ( 'NONE',  ( 12.06949235617739724, 12.14591786802326823, 51.87609039468568284 ) ) ;
#33234=CARTESIAN_POINT ( 'NONE',  ( 5.823673210054444382, -21.52544592524334988, 95.20942372801903275 ) ) ;
#33235=CARTESIAN_POINT ( 'NONE',  ( 16.46253265017146816, 9.564922557961045513, 61.66775706135234003 ) ) ;
#33236=CARTESIAN_POINT ( 'NONE',  ( 13.89961937509977652, -13.97604488694527269, 43.12390960531434558 ) ) ;
#33237=CARTESIAN_POINT ( 'NONE',  ( 10.72451020669898902, -18.67979575497178502, 67.91557627198102409 ) ) ;
#33238=CARTESIAN_POINT ( 'NONE',  ( -4.483927247898539470, -16.52544592524342804, 62.29057627198102409 ) ) ;
#33239=CARTESIAN_POINT ( 'NONE',  ( 0.05219959533936267826, -19.03943276465977164, 70.00109039468566152 ) ) ;
#33240=CARTESIAN_POINT ( 'NONE',  ( -17.60779699588839620, -5.499999999999975131, 101.3498131667010256 ) ) ;
#33241=CARTESIAN_POINT ( 'NONE',  ( -13.97604488694547697, 13.89961937509957934, 38.12609039468566152 ) ) ;
#33242=CARTESIAN_POINT ( 'NONE',  ( 14.34966873604972726, -8.224510206698740333, 95.83442372801903275 ) ) ;
#33243=CARTESIAN_POINT ( 'NONE',  ( 16.55341960407611168, 4.379528057220329451, 53.95724293864770260 ) ) ;
#33244=CARTESIAN_POINT ( 'NONE',  ( 10.81492255796106328, -18.62759615963255655, 95.41775706135234714 ) ) ;
#33246=CARTESIAN_POINT ( 'NONE',  ( 21.55341960407610458, 5.719274019375980345, 88.95724293864769550 ) ) ;
#33247=CARTESIAN_POINT ( 'NONE',  ( -19.03943276465977164, 0.05219959533909376836, 56.24890960531435979 ) ) ;
#33248=CARTESIAN_POINT ( 'NONE',  ( 5.823673210054444382, -21.52544592524334988, 70.20942372801904696 ) ) ;
#33249=CARTESIAN_POINT ( 'NONE',  ( 9.564922557960805705, 16.46253265017160317, 54.58224293864769550 ) ) ;
#33250=CARTESIAN_POINT ( 'NONE',  ( -5.153800228976328057, -19.02544592524343514, 72.29057627198102409 ) ) ;
#33251=CARTESIAN_POINT ( 'NONE',  ( 14.29746914071049879, -8.314922557960816363, 108.3322429386477097 ) ) ;
#33252=CARTESIAN_POINT ( 'NONE',  ( -19.02544592524342804, 5.153800228976336051, 106.0405762719810241 ) ) ;
#33253=CARTESIAN_POINT ( 'NONE',  ( 16.52544592524342804, -4.483927247898539470, 58.54057627198103120 ) ) ;
#33254=CARTESIAN_POINT ( 'NONE',  ( -5.049401038298153566, 19.05341960407611168, 35.20724293864768839 ) ) ;
#33255=CARTESIAN_POINT ( 'NONE',  ( 4.483927247898545687, 16.52544592524342804, 79.79057627198102409 ) ) ;
#33256=CARTESIAN_POINT ( 'NONE',  ( -18.67979575497178146, -10.72451020669898902, 91.66557627198103830 ) ) ;
#33257=CARTESIAN_POINT ( 'NONE',  ( -5.719274019375665041, -21.55341960407619695, 29.79275706135234358 ) ) ;
#33259=CARTESIAN_POINT ( 'NONE',  ( -16.55341960407617563, 4.379528057220093196, 48.54275706135234714 ) ) ;
#33260=CARTESIAN_POINT ( 'NONE',  ( 15.72974639402199770, -15.80617190586745480, 83.12390960531436690 ) ) ;
#33261=CARTESIAN_POINT ( 'NONE',  ( 5.823673210054444382, -21.52544592524334988, 110.2094237280190185 ) ) ;
#33262=CARTESIAN_POINT ( 'NONE',  ( 9.474510206698971260, -16.51473224551069308, 107.9155762719810383 ) ) ;
#33263=CARTESIAN_POINT ( 'NONE',  ( -10.72451020669870658, -18.67979575497194134, 49.58442372801901143 ) ) ;
#33264=CARTESIAN_POINT ( 'NONE',  ( 5.719274019375991003, -21.55341960407610458, 37.70724293864769550 ) ) ;
#33265=CARTESIAN_POINT ( 'NONE',  ( -0.05219959533934338120, 16.53943276465976808, 107.5010903946856899 ) ) ;
#33266=CARTESIAN_POINT ( 'NONE',  ( -10.81492255796105439, 18.62759615963255655, 57.91775706135234714 ) ) ;
#33267=CARTESIAN_POINT ( 'NONE',  ( -21.53943276465977519, -0.05219959533937600094, 83.75109039468568994 ) ) ;
#33268=CARTESIAN_POINT ( 'NONE',  ( -19.02544592524334988, -5.153800228976617603, 28.95942372801900433 ) ) ;
#33269=CARTESIAN_POINT ( 'NONE',  ( -12.06949235617739369, -12.14591786802326823, 94.37609039468568994 ) ) ;
#33270=CARTESIAN_POINT ( 'NONE',  ( 21.55341960407619695, -5.719274019375665929, 36.04275706135234714 ) ) ;
#33271=CARTESIAN_POINT ( 'NONE',  ( -5.049401038298153566, 19.05341960407611168, 45.20724293864769550 ) ) ;
#33272=CARTESIAN_POINT ( 'NONE',  ( 19.02544592524334988, 5.153800228976608722, 26.45942372801899722 ) ) ;
#33273=CARTESIAN_POINT ( 'NONE',  ( 5.719274019375991003, -21.55341960407610458, 27.70724293864769905 ) ) ;
#33274=CARTESIAN_POINT ( 'NONE',  ( 0.05219959533937995610, -21.53943276465977519, 25.00109039468567218 ) ) ;
#33275=CARTESIAN_POINT ( 'NONE',  ( -21.55341960407610458, -5.719274019375992779, 76.45724293864769550 ) ) ;
#33277=CARTESIAN_POINT ( 'NONE',  ( -18.67979575497178146, -10.72451020669898902, 86.66557627198102409 ) ) ;
#33278=CARTESIAN_POINT ( 'NONE',  ( 8.314922557961029526, -14.29746914071037800, 65.41775706135234714 ) ) ;
#33279=CARTESIAN_POINT ( 'NONE',  ( 12.14591786802309770, 12.06949235617756955, 69.37390960531436690 ) ) ;
#33281=CARTESIAN_POINT ( 'NONE',  ( 19.03943276465977164, 0.05219959533936151252, 91.25109039468566152 ) ) ;
#33283=CARTESIAN_POINT ( 'NONE',  ( 16.53943276465976808, 0.05219959533934440121, 21.25109039468567218 ) ) ;
#33284=CARTESIAN_POINT ( 'NONE',  ( -5.823673210054116645, -21.52544592524344225, 97.29057627198105251 ) ) ;
#33285=CARTESIAN_POINT ( 'NONE',  ( 5.823673210054125526, 21.52544592524343514, 74.79057627198105251 ) ) ;
#33286=CARTESIAN_POINT ( 'NONE',  ( -19.02544592524342804, 5.153800228976336051, 111.0405762719810099 ) ) ;
#33287=CARTESIAN_POINT ( 'NONE',  ( 14.29746914071037800, 8.314922557961029526, 56.66775706135235424 ) ) ;
#33288=CARTESIAN_POINT ( 'NONE',  ( -16.46253265017160317, 9.564922557960807481, 75.83224293864769550 ) ) ;
#33289=CARTESIAN_POINT ( 'NONE',  ( 5.719274019375673035, 21.55341960407619339, 47.29275706135234003 ) ) ;
#33290=CARTESIAN_POINT ( 'NONE',  ( 5.049401038297881783, 19.05341960407617563, 107.2927570613523187 ) ) ;
#33291=CARTESIAN_POINT ( 'NONE',  ( 9.564922557960805705, 16.46253265017160317, 104.5822429386476955 ) ) ;
#33292=CARTESIAN_POINT ( 'NONE',  ( -5.153800228976607833, 19.02544592524334988, 22.70942372801899012 ) ) ;
#33293=CARTESIAN_POINT ( 'NONE',  ( -16.52544592524335698, -4.483927247898792601, 43.95942372801902565 ) ) ;
#33294=CARTESIAN_POINT ( 'NONE',  ( -0.05219959533909027116, -19.03943276465977164, 107.4989096053143527 ) ) ;
#33295=CARTESIAN_POINT ( 'NONE',  ( 5.719274019375991003, -21.55341960407610458, 102.7072429386476955 ) ) ;
#33296=CARTESIAN_POINT ( 'NONE',  ( -13.89961937509977652, 13.97604488694528158, 60.62390960531436690 ) ) ;
#33298=CARTESIAN_POINT ( 'NONE',  ( -12.14591786802309592, -12.06949235617757132, 76.87390960531439532 ) ) ;
#33299=CARTESIAN_POINT ( 'NONE',  ( 21.55341960407610458, 5.719274019375980345, 23.95724293864769550 ) ) ;
#33300=CARTESIAN_POINT ( 'NONE',  ( -17.31728774477272381, 6.344390552232388458, 35.81906651689320142 ) ) ;
#33301=CARTESIAN_POINT ( 'NONE',  ( -15.80617190586745835, -15.72974639402198527, 106.8739096053143811 ) ) ;
#33302=CARTESIAN_POINT ( 'NONE',  ( 13.89961937509957401, 13.97604488694547697, 56.87609039468564731 ) ) ;
#33303=CARTESIAN_POINT ( 'NONE',  ( -0.05219959533909027116, -19.03943276465977164, 112.4989096053143669 ) ) ;
#33304=CARTESIAN_POINT ( 'NONE',  ( -0.05219959533909027116, -19.03943276465977164, 32.49890960531435979 ) ) ;
#33305=CARTESIAN_POINT ( 'NONE',  ( 10.72451020669898902, -18.67979575497178502, 52.91557627198103830 ) ) ;
#33306=CARTESIAN_POINT ( 'NONE',  ( -19.03943276465977164, 0.05219959533909376836, 96.24890960531436690 ) ) ;
#33307=CARTESIAN_POINT ( 'NONE',  ( -0.05219959533937732626, 21.53943276465977519, 82.50109039468568994 ) ) ;
#33308=CARTESIAN_POINT ( 'NONE',  ( -19.02544592524342804, 5.153800228976336051, 46.04057627198101699 ) ) ;
#33309=CARTESIAN_POINT ( 'NONE',  ( 0.05219959533910956823, 16.53943276465976808, 84.99890960531436690 ) ) ;
#33310=CARTESIAN_POINT ( 'NONE',  ( 4.379528057220092307, 16.55341960407617563, 37.29275706135235424 ) ) ;
#33311=CARTESIAN_POINT ( 'NONE',  ( -10.72451020669870658, -18.67979575497194134, 69.58442372801900433 ) ) ;
#33312=VERTEX_POINT ( 'NONE', #31956 ) ;
#33313=CARTESIAN_POINT ( 'NONE',  ( 16.51473224551083163, -9.474510206698727899, 30.83442372801900433 ) ) ;
#33314=CARTESIAN_POINT ( 'NONE',  ( -9.474510206698720793, -16.51473224551083518, 74.58442372801900433 ) ) ;
#33315=CARTESIAN_POINT ( 'NONE',  ( -13.89961937509957401, -13.97604488694547875, 39.37609039468566152 ) ) ;
#33316=CARTESIAN_POINT ( 'NONE',  ( 10.72451020669871369, 18.67979575497193778, 37.08442372801901143 ) ) ;
#33318=CARTESIAN_POINT ( 'NONE',  ( -13.97604488694547697, 13.89961937509957934, 28.12609039468565797 ) ) ;
#33319=CARTESIAN_POINT ( 'NONE',  ( 9.474510206698971260, -16.51473224551069308, 62.91557627198102409 ) ) ;
#33320=CARTESIAN_POINT ( 'NONE',  ( -16.55341960407611168, -4.379528057220339221, 21.45724293864769550 ) ) ;
#33321=CARTESIAN_POINT ( 'NONE',  ( 5.049401038298161559, -19.05341960407611168, 112.7072429386476813 ) ) ;
#33322=CARTESIAN_POINT ( 'NONE',  ( 0.05219959533937995610, -21.53943276465977519, 90.00109039468567573 ) ) ;
#33324=CARTESIAN_POINT ( 'NONE',  ( -18.22780087662122028, 5.500000000000031086, 98.51540105326105845 ) ) ;
#33325=CARTESIAN_POINT ( 'NONE',  ( -15.80617190586768217, 15.72974639402176855, 83.12609039468568994 ) ) ;
#33326=CARTESIAN_POINT ( 'NONE',  ( 16.81555441253550143, -7.025013491695467849, 43.13685445334256485 ) ) ;
#33327=CARTESIAN_POINT ( 'NONE',  ( 19.02544592524343514, -5.153800228976328945, 98.54057627198100988 ) ) ;
#33328=EDGE_CURVE ( 'NONE', #115197, #33312, #44858, .T. ) ;
#33330=CARTESIAN_POINT ( 'NONE',  ( 9.474510206698971260, -16.51473224551069308, 52.91557627198102409 ) ) ;
#33331=CARTESIAN_POINT ( 'NONE',  ( -21.53943276465977519, 0.05219959533907696930, 61.24890960531435979 ) ) ;
#33332=CARTESIAN_POINT ( 'NONE',  ( -8.314922557960811034, -14.29746914071050412, 32.08224293864769550 ) ) ;
#33333=CARTESIAN_POINT ( 'NONE',  ( -4.379528057220328563, 16.55341960407611168, 115.2072429386476955 ) ) ;
#33334=CARTESIAN_POINT ( 'NONE',  ( -16.46253265017160317, 9.564922557960807481, 95.83224293864769550 ) ) ;
#33335=CARTESIAN_POINT ( 'NONE',  ( -5.153800228976607833, 19.02544592524334988, 27.70942372801899722 ) ) ;
#33336=CARTESIAN_POINT ( 'NONE',  ( 16.53943276465976808, -0.05219959533910856209, 103.7489096053143669 ) ) ;
#33337=CARTESIAN_POINT ( 'NONE',  ( -10.72451020669870658, -18.67979575497194134, 69.58442372801900433 ) ) ;
#33339=CARTESIAN_POINT ( 'NONE',  ( -4.483927247898782831, 16.52544592524335698, 112.7094237280190328 ) ) ;
#33340=CARTESIAN_POINT ( 'NONE',  ( -5.049401038297874678, -19.05341960407617918, 59.79275706135231871 ) ) ;
#33342=CARTESIAN_POINT ( 'NONE',  ( -5.049401038298153566, 19.05341960407611168, 110.2072429386476671 ) ) ;
#33343=CARTESIAN_POINT ( 'NONE',  ( -0.05219959533910754901, -16.53943276465976808, 82.49890960531436690 ) ) ;
#33344=CARTESIAN_POINT ( 'NONE',  ( 0.05219959533936267826, -19.03943276465977164, 55.00109039468566863 ) ) ;
#33345=CARTESIAN_POINT ( 'NONE',  ( 16.46253265017160672, -9.564922557960803928, 63.33224293864769550 ) ) ;
#33346=CARTESIAN_POINT ( 'NONE',  ( -14.29746914071049879, 8.314922557960819915, 65.83224293864769550 ) ) ;
#33347=CARTESIAN_POINT ( 'NONE',  ( 19.03943276465977164, 0.05219959533936151252, 96.25109039468567573 ) ) ;
#33348=CARTESIAN_POINT ( 'NONE',  ( 10.72451020669898902, -18.67979575497178502, 52.91557627198103830 ) ) ;
#33350=CARTESIAN_POINT ( 'NONE',  ( -12.14591786802309592, -12.06949235617757132, 111.8739096053143669 ) ) ;
#33351=CARTESIAN_POINT ( 'NONE',  ( 5.153800228976617603, -19.02544592524335343, 100.2094237280190043 ) ) ;
#33352=CARTESIAN_POINT ( 'NONE',  ( -16.46253265017160317, 9.564922557960807481, 55.83224293864769550 ) ) ;
#33353=CARTESIAN_POINT ( 'NONE',  ( -5.719274019375978568, 21.55341960407610458, 60.20724293864768839 ) ) ;
#33354=CARTESIAN_POINT ( 'NONE',  ( 12.14591786802327356, -12.06949235617739191, 95.62609039468568994 ) ) ;
#33355=CARTESIAN_POINT ( 'NONE',  ( 9.474510206698971260, -16.51473224551069308, 72.91557627198102409 ) ) ;
#33356=CARTESIAN_POINT ( 'NONE',  ( -9.474510206698720793, -16.51473224551083518, 49.58442372801899722 ) ) ;
#33357=CARTESIAN_POINT ( 'NONE',  ( -21.52544592524334988, -5.823673210054445271, 78.95942372801901854 ) ) ;
#33358=CARTESIAN_POINT ( 'NONE',  ( 5.823673210054125526, 21.52544592524343514, 69.79057627198102409 ) ) ;
#33359=CARTESIAN_POINT ( 'NONE',  ( -19.02544592524342804, 5.153800228976336051, 111.0405762719810099 ) ) ;
#33360=CARTESIAN_POINT ( 'NONE',  ( -9.474510206698964154, 16.51473224551069663, 40.41557627198103120 ) ) ;
#33361=CARTESIAN_POINT ( 'NONE',  ( 14.34966873604972726, -8.224510206698740333, 95.83442372801903275 ) ) ;
#33362=CARTESIAN_POINT ( 'NONE',  ( -9.564922557961040184, 16.46253265017147172, 112.9177570613523329 ) ) ;
#33363=CARTESIAN_POINT ( 'NONE',  ( 17.12812012977023812, 6.668231424566061882, 53.85948759323142809 ) ) ;
#33364=CARTESIAN_POINT ( 'NONE',  ( -21.52544592524334988, -5.823673210054445271, 98.95942372801903275 ) ) ;
#33366=CARTESIAN_POINT ( 'NONE',  ( 16.55341960407611168, 4.379528057220329451, 63.95724293864770260 ) ) ;
#33367=CARTESIAN_POINT ( 'NONE',  ( 14.29746914071049879, -8.314922557960816363, 73.33224293864769550 ) ) ;
#33368=CARTESIAN_POINT ( 'NONE',  ( -5.719274019375978568, 21.55341960407610458, 90.20724293864770971 ) ) ;
#33369=CARTESIAN_POINT ( 'NONE',  ( -21.53943276465977519, 0.05219959533907696930, 86.24890960531436690 ) ) ;
#33370=CARTESIAN_POINT ( 'NONE',  ( 16.52216118717208460, -7.221426719304491648, 96.42400978953010338 ) ) ;
#33371=CARTESIAN_POINT ( 'NONE',  ( -21.55341960407610458, -5.719274019375992779, 46.45724293864769550 ) ) ;
#33372=CARTESIAN_POINT ( 'NONE',  ( 16.52544592524335698, 4.483927247898782831, 66.45942372801903275 ) ) ;
#33373=CARTESIAN_POINT ( 'NONE',  ( 12.14591786802309770, 12.06949235617756955, 94.37390960531436690 ) ) ;
#33374=CARTESIAN_POINT ( 'NONE',  ( -16.46253265017160317, 9.564922557960807481, 40.83224293864769550 ) ) ;
#33376=CARTESIAN_POINT ( 'NONE',  ( 4.483927247898790824, -16.52544592524335698, 95.20942372801903275 ) ) ;
#33377=CARTESIAN_POINT ( 'NONE',  ( -18.67979575497193778, 10.72451020669871902, 28.33442372801902209 ) ) ;
#33378=CARTESIAN_POINT ( 'NONE',  ( 19.02544592524343514, -5.153800228976328945, 98.54057627198100988 ) ) ;
#33379=CARTESIAN_POINT ( 'NONE',  ( -15.80617190586768217, 15.72974639402176855, 68.12609039468567573 ) ) ;
#33380=CARTESIAN_POINT ( 'NONE',  ( 5.049401038298161559, -19.05341960407611168, 22.70724293864769194 ) ) ;
#33381=CARTESIAN_POINT ( 'NONE',  ( 19.05341960407611168, 5.049401038298154454, 28.95724293864769550 ) ) ;
#33384=CARTESIAN_POINT ( 'NONE',  ( -0.05219959533937732626, 21.53943276465977519, 52.50109039468567573 ) ) ;
#33385=CARTESIAN_POINT ( 'NONE',  ( 9.564922557960805705, 16.46253265017160317, 44.58224293864769550 ) ) ;
#33386=CARTESIAN_POINT ( 'NONE',  ( 18.09805431107521301, -5.500000000000095923, 58.51606229291888894 ) ) ;
#33387=CARTESIAN_POINT ( 'NONE',  ( 5.049401038298161559, -19.05341960407611168, 92.70724293864769550 ) ) ;
#33388=CARTESIAN_POINT ( 'NONE',  ( 16.51473224551083163, -9.474510206698727899, 60.83442372801900433 ) ) ;
#33389=CARTESIAN_POINT ( 'NONE',  ( 5.823673210054444382, -21.52544592524334988, 25.20942372801901854 ) ) ;
#33390=CARTESIAN_POINT ( 'NONE',  ( 0.05219959533936267826, -19.03943276465977164, 60.00109039468566863 ) ) ;
#33391=CARTESIAN_POINT ( 'NONE',  ( 9.564922557960805705, 16.46253265017160317, 34.58224293864770260 ) ) ;
#33392=CARTESIAN_POINT ( 'NONE',  ( 12.06949235617739724, 12.14591786802326823, 101.8760903946857042 ) ) ;
#33393=CARTESIAN_POINT ( 'NONE',  ( 0.05219959533936267826, -19.03943276465977164, 70.00109039468566152 ) ) ;
#33394=CARTESIAN_POINT ( 'NONE',  ( -14.34966873604960291, -8.224510206698953496, 31.66557627198102054 ) ) ;
#33395=CARTESIAN_POINT ( 'NONE',  ( 13.89961937509957401, 13.97604488694547697, 56.87609039468564731 ) ) ;
#33396=CARTESIAN_POINT ( 'NONE',  ( -16.46253265017160317, 9.564922557960807481, 100.8322429386477097 ) ) ;
#33397=CARTESIAN_POINT ( 'NONE',  ( 10.72451020669871369, 18.67979575497193778, 102.0844237280190185 ) ) ;
#33398=CARTESIAN_POINT ( 'NONE',  ( 5.153800228976615827, -19.02544592524334988, 20.20942372801899722 ) ) ;
#33400=CARTESIAN_POINT ( 'NONE',  ( -13.97604488694527625, -13.89961937509977652, 26.87390960531434558 ) ) ;
#33401=CARTESIAN_POINT ( 'NONE',  ( 15.80617190586769283, -15.72974639402175789, 90.62609039468567573 ) ) ;
#33402=CARTESIAN_POINT ( 'NONE',  ( -14.34966873604972548, 8.224510206698743886, 33.33442372801900433 ) ) ;
#33403=CARTESIAN_POINT ( 'NONE',  ( 5.049401038298161559, -19.05341960407611168, 97.70724293864766707 ) ) ;
#33405=CARTESIAN_POINT ( 'NONE',  ( 30.00000000000000000, -1.132798289211302014E-14, 97.50000000000000000 ) ) ;
#33406=CARTESIAN_POINT ( 'NONE',  ( -9.564922557960796823, -16.46253265017161027, 77.08224293864769550 ) ) ;
#33408=CARTESIAN_POINT ( 'NONE',  ( 9.474510206698729675, 16.51473224551082808, 77.08442372801900433 ) ) ;
#33409=CARTESIAN_POINT ( 'NONE',  ( -5.049401038298153566, 19.05341960407611168, 110.2072429386476671 ) ) ;
#33410=CARTESIAN_POINT ( 'NONE',  ( 21.53943276465977519, 0.05219959533937863772, 96.25109039468568994 ) ) ;
#33411=CARTESIAN_POINT ( 'NONE',  ( 16.52544592524342804, -4.483927247898539470, 93.54057627198103830 ) ) ;
#33412=CARTESIAN_POINT ( 'NONE',  ( 10.81492255796078972, 18.62759615963270932, 39.58224293864769550 ) ) ;
#33413=CARTESIAN_POINT ( 'NONE',  ( 18.62759615963271287, -10.81492255796078972, 33.33224293864769550 ) ) ;
#33414=CARTESIAN_POINT ( 'NONE',  ( 12.14591786802309770, 12.06949235617756955, 104.3739096053143669 ) ) ;
#33416=CARTESIAN_POINT ( 'NONE',  ( 9.564922557961047289, -16.46253265017146816, 60.41775706135233293 ) ) ;
#33417=CARTESIAN_POINT ( 'NONE',  ( -8.224510206698948167, 14.34966873604960824, 45.41557627198103830 ) ) ;
#33418=CARTESIAN_POINT ( 'NONE',  ( -13.89961937509977652, 13.97604488694528158, 110.6239096053143243 ) ) ;
#33419=CARTESIAN_POINT ( 'NONE',  ( 5.823673210054444382, -21.52544592524334988, 80.20942372801901854 ) ) ;
#33420=CARTESIAN_POINT ( 'NONE',  ( -5.823673210054116645, -21.52544592524344225, 72.29057627198102409 ) ) ;
#33421=CARTESIAN_POINT ( 'NONE',  ( 18.67979575497194134, -10.72451020669871369, 40.83442372801901854 ) ) ;
#33422=CARTESIAN_POINT ( 'NONE',  ( -0.05219959533907301413, -21.53943276465977519, 102.4989096053143811 ) ) ;
#33423=CARTESIAN_POINT ( 'NONE',  ( -15.72974639402176322, -15.80617190586768395, 54.37609039468568994 ) ) ;
#33424=CARTESIAN_POINT ( 'NONE',  ( -19.03943276465977164, 0.05219959533909376836, 31.24890960531435979 ) ) ;
#33425=CARTESIAN_POINT ( 'NONE',  ( -19.05341960407611168, -5.049401038298163336, 81.45724293864769550 ) ) ;
#33426=CARTESIAN_POINT ( 'NONE',  ( 16.52544592524335698, 4.483927247898782831, 81.45942372801900433 ) ) ;
#33427=CARTESIAN_POINT ( 'NONE',  ( 14.34966873604960469, 8.224510206698951720, 99.16557627198100988 ) ) ;
#33428=CARTESIAN_POINT ( 'NONE',  ( 16.46253265017160672, -9.564922557960803928, 113.3322429386476955 ) ) ;
#33429=CARTESIAN_POINT ( 'NONE',  ( -14.29746914071049879, 8.314922557960819915, 50.83224293864770971 ) ) ;
#33430=CARTESIAN_POINT ( 'NONE',  ( -8.314922557960811034, -14.29746914071050412, 27.08224293864769550 ) ) ;
#33431=CARTESIAN_POINT ( 'NONE',  ( 13.89961937509977652, -13.97604488694527269, 68.12390960531436690 ) ) ;
#33432=CARTESIAN_POINT ( 'NONE',  ( -19.03943276465977164, 0.05219959533909376836, 41.24890960531435269 ) ) ;
#33433=CARTESIAN_POINT ( 'NONE',  ( -5.823673210054116645, -21.52544592524344225, 47.29057627198103120 ) ) ;
#33434=CARTESIAN_POINT ( 'NONE',  ( -9.564922557961040184, 16.46253265017147172, 42.91775706135234003 ) ) ;
#33436=CARTESIAN_POINT ( 'NONE',  ( -16.52544592524342804, 4.483927247898546575, 31.04057627198102409 ) ) ;
#33437=CARTESIAN_POINT ( 'NONE',  ( -9.564922557960796823, -16.46253265017161027, 107.0822429386476955 ) ) ;
#33438=CARTESIAN_POINT ( 'NONE',  ( -18.62759615963255300, -10.81492255796106328, 54.16775706135235424 ) ) ;
#33440=CARTESIAN_POINT ( 'NONE',  ( 4.483927247898790824, -16.52544592524335698, 65.20942372801901854 ) ) ;
#33441=CARTESIAN_POINT ( 'NONE',  ( 19.05341960407617918, -5.049401038297876454, 56.04275706135234714 ) ) ;
#33442=CARTESIAN_POINT ( 'NONE',  ( 4.379528057220339221, -16.55341960407611168, 27.70724293864769905 ) ) ;
#33443=CARTESIAN_POINT ( 'NONE',  ( -18.89770734986047884, -5.500000000000005329, 74.10214472496639360 ) ) ;
#33444=CARTESIAN_POINT ( 'NONE',  ( -4.483927247898782831, 16.52544592524335698, 107.7094237280190328 ) ) ;
#33445=CARTESIAN_POINT ( 'NONE',  ( -9.474510206698964154, 16.51473224551069663, 40.41557627198103120 ) ) ;
#33446=CARTESIAN_POINT ( 'NONE',  ( -19.05341960407611168, -5.049401038298163336, 61.45724293864769550 ) ) ;
#33447=CARTESIAN_POINT ( 'NONE',  ( 9.474510206698971260, -16.51473224551069308, 22.91557627198102765 ) ) ;
#33448=CARTESIAN_POINT ( 'NONE',  ( 10.72451020669871369, 18.67979575497193778, 37.08442372801901143 ) ) ;
#33449=CARTESIAN_POINT ( 'NONE',  ( 9.564922557960805705, 16.46253265017160317, 44.58224293864769550 ) ) ;
#33451=CARTESIAN_POINT ( 'NONE',  ( 19.03943276465977164, -0.05219959533909143690, 48.74890960531435979 ) ) ;
#33452=CARTESIAN_POINT ( 'NONE',  ( -15.80617190586745835, -15.72974639402198527, 21.87390960531436690 ) ) ;
#33453=CARTESIAN_POINT ( 'NONE',  ( 15.72974639402176855, 15.80617190586768217, 61.87609039468568284 ) ) ;
#33454=CARTESIAN_POINT ( 'NONE',  ( -8.314922557960811034, -14.29746914071050412, 112.0822429386477097 ) ) ;
#33455=CARTESIAN_POINT ( 'NONE',  ( 15.80617190586746368, 15.72974639402197994, 34.37390960531435979 ) ) ;
#33457=CARTESIAN_POINT ( 'NONE',  ( 4.379528057220092307, 16.55341960407617563, 82.29275706135234714 ) ) ;
#33458=CARTESIAN_POINT ( 'NONE',  ( 18.67979575497194134, -10.72451020669871369, 100.8344237280190185 ) ) ;
#33459=CARTESIAN_POINT ( 'NONE',  ( -8.314922557961024197, 14.29746914071037800, 52.91775706135235424 ) ) ;
#33460=CARTESIAN_POINT ( 'NONE',  ( -19.02544592524342804, 5.153800228976336051, 91.04057627198100988 ) ) ;
#33461=CARTESIAN_POINT ( 'NONE',  ( 14.29746914071037800, 8.314922557961029526, 36.66775706135234714 ) ) ;
#33462=CARTESIAN_POINT ( 'NONE',  ( 8.314922557961029526, -14.29746914071037800, 30.41775706135234358 ) ) ;
#33463=CARTESIAN_POINT ( 'NONE',  ( -4.379528057220086978, -16.55341960407618274, 99.79275706135234714 ) ) ;
#33464=CARTESIAN_POINT ( 'NONE',  ( -5.719274019375665041, -21.55341960407619695, 49.79275706135234714 ) ) ;
#33465=CARTESIAN_POINT ( 'NONE',  ( 13.89961937509957401, 13.97604488694547697, 101.8760903946856331 ) ) ;
#33466=CARTESIAN_POINT ( 'NONE',  ( -21.55341960407610458, -5.719274019375992779, 106.4572429386477097 ) ) ;
#33467=CARTESIAN_POINT ( 'NONE',  ( -0.05219959533910754901, -16.53943276465976808, 102.4989096053143811 ) ) ;
#33468=CARTESIAN_POINT ( 'NONE',  ( 19.05341960407617918, -5.049401038297876454, 101.0427570613523045 ) ) ;
#33469=CARTESIAN_POINT ( 'NONE',  ( 14.29746914071037800, 8.314922557961029526, 86.66775706135234714 ) ) ;
#33470=CARTESIAN_POINT ( 'NONE',  ( -17.31747979337961851, 6.344076630960740815, 43.62055131934818064 ) ) ;
#33471=CARTESIAN_POINT ( 'NONE',  ( -5.153800228976607833, 19.02544592524334988, 77.70942372801900433 ) ) ;
#33472=CARTESIAN_POINT ( 'NONE',  ( -8.224510206698948167, 14.34966873604960824, 40.41557627198103120 ) ) ;
#33473=CARTESIAN_POINT ( 'NONE',  ( -12.14591786802309592, -12.06949235617757132, 41.87390960531435979 ) ) ;
#33474=CARTESIAN_POINT ( 'NONE',  ( -16.52544592524342804, 4.483927247898546575, 106.0405762719810525 ) ) ;
#33475=CARTESIAN_POINT ( 'NONE',  ( -5.153800228976607833, 19.02544592524334988, 37.70942372801899722 ) ) ;
#33476=CARTESIAN_POINT ( 'NONE',  ( -18.22780087662122028, 5.500000000000031086, 88.51540105326107266 ) ) ;
#33477=CARTESIAN_POINT ( 'NONE',  ( -21.55341960407619339, 5.719274019375674811, 33.54275706135234714 ) ) ;
#33478=CARTESIAN_POINT ( 'NONE',  ( 4.483927247898790824, -16.52544592524335698, 20.20942372801900788 ) ) ;
#33480=CARTESIAN_POINT ( 'NONE',  ( -16.51473224551069308, -9.474510206698971260, 96.66557627198102409 ) ) ;
#33481=CARTESIAN_POINT ( 'NONE',  ( 13.89961937509977652, -13.97604488694527269, 83.12390960531436690 ) ) ;
#33482=CARTESIAN_POINT ( 'NONE',  ( -5.719274019375978568, 21.55341960407610458, 55.20724293864770260 ) ) ;
#33483=CARTESIAN_POINT ( 'NONE',  ( -4.379528057220328563, 16.55341960407611168, 100.2072429386476955 ) ) ;
#33484=CARTESIAN_POINT ( 'NONE',  ( -9.474510206698964154, 16.51473224551069663, 65.41557627198102409 ) ) ;
#33485=CARTESIAN_POINT ( 'NONE',  ( 9.474510206698971260, -16.51473224551069308, 32.91557627198102409 ) ) ;
#33486=CARTESIAN_POINT ( 'NONE',  ( 0.05219959533937995610, -21.53943276465977519, 40.00109039468567573 ) ) ;
#33487=CARTESIAN_POINT ( 'NONE',  ( 21.55341960407619695, -5.719274019375665929, 71.04275706135234714 ) ) ;
#33488=CARTESIAN_POINT ( 'NONE',  ( 14.29746914071037800, 8.314922557961029526, 91.66775706135234714 ) ) ;
#33489=CARTESIAN_POINT ( 'NONE',  ( 15.80617190586769283, -15.72974639402175789, 25.62609039468567929 ) ) ;
#33490=CARTESIAN_POINT ( 'NONE',  ( -21.55341960407619339, 5.719274019375674811, 28.54275706135234358 ) ) ;
#33491=CARTESIAN_POINT ( 'NONE',  ( 5.049401038297881783, 19.05341960407617563, 57.29275706135231871 ) ) ;
#33492=CARTESIAN_POINT ( 'NONE',  ( -5.049401038298153566, 19.05341960407611168, 85.20724293864766707 ) ) ;
#33493=CARTESIAN_POINT ( 'NONE',  ( 5.719274019375673035, 21.55341960407619339, 82.29275706135234714 ) ) ;
#33494=CARTESIAN_POINT ( 'NONE',  ( -21.53943276465977519, 0.05219959533907696930, 81.24890960531436690 ) ) ;
#33495=CARTESIAN_POINT ( 'NONE',  ( 16.52544592524342804, -4.483927247898539470, 48.54057627198103120 ) ) ;
#33496=CARTESIAN_POINT ( 'NONE',  ( 5.823673210054444382, -21.52544592524334988, 100.2094237280190043 ) ) ;
#33497=CARTESIAN_POINT ( 'NONE',  ( 5.049401038297881783, 19.05341960407617563, 37.29275706135232582 ) ) ;
#33498=CARTESIAN_POINT ( 'NONE',  ( 14.29746914071049879, -8.314922557960816363, 73.33224293864769550 ) ) ;
#33499=CARTESIAN_POINT ( 'NONE',  ( 14.29746914071049879, -8.314922557960816363, 113.3322429386476955 ) ) ;
#33500=CARTESIAN_POINT ( 'NONE',  ( 19.05341960407617918, -5.049401038297876454, 76.04275706135230450 ) ) ;
#33501=CARTESIAN_POINT ( 'NONE',  ( 8.314922557960818139, 14.29746914071049879, 29.58224293864769905 ) ) ;
#33502=CARTESIAN_POINT ( 'NONE',  ( 21.52544592524334988, 5.823673210054432836, 81.45942372801900433 ) ) ;
#33503=CARTESIAN_POINT ( 'NONE',  ( 19.03943276465977164, -0.05219959533909143690, 83.74890960531436690 ) ) ;
#33504=CARTESIAN_POINT ( 'NONE',  ( -9.564922557961040184, 16.46253265017147172, 57.91775706135233293 ) ) ;
#33505=CARTESIAN_POINT ( 'NONE',  ( -21.52544592524343514, 5.823673210054127303, 61.04057627198103120 ) ) ;
#33506=CARTESIAN_POINT ( 'NONE',  ( -10.72451020669898014, 18.67979575497178502, 110.4155762719810383 ) ) ;
#33507=CARTESIAN_POINT ( 'NONE',  ( -19.05341960407617563, 5.049401038297882671, 113.5427570613523471 ) ) ;
#33508=CARTESIAN_POINT ( 'NONE',  ( 14.34966873604972726, -8.224510206698740333, 75.83442372801900433 ) ) ;
#33510=CARTESIAN_POINT ( 'NONE',  ( -21.53943276465977519, -0.05219959533937600094, 23.75109039468567929 ) ) ;
#33511=CARTESIAN_POINT ( 'NONE',  ( 16.55341960407611168, 4.379528057220329451, 103.9572429386476813 ) ) ;
#33513=CARTESIAN_POINT ( 'NONE',  ( 16.55341960407618274, -4.379528057220086978, 41.04275706135236135 ) ) ;
#33514=CARTESIAN_POINT ( 'NONE',  ( 5.823673210054125526, 21.52544592524343514, 59.79057627198103120 ) ) ;
#33515=CARTESIAN_POINT ( 'NONE',  ( 12.14591786802327356, -12.06949235617739191, 105.6260903946856899 ) ) ;
#33516=CARTESIAN_POINT ( 'NONE',  ( 4.483927247898790824, -16.52544592524335698, 40.20942372801901854 ) ) ;
#33517=CARTESIAN_POINT ( 'NONE',  ( 5.153800228976335163, 19.02544592524342804, 29.79057627198102409 ) ) ;
#33518=CARTESIAN_POINT ( 'NONE',  ( 12.06949235617739724, 12.14591786802326823, 76.87609039468567573 ) ) ;
#33519=CARTESIAN_POINT ( 'NONE',  ( -19.02544592524334988, -5.153800228976617603, 78.95942372801900433 ) ) ;
#33520=CARTESIAN_POINT ( 'NONE',  ( -5.719274019375978568, 21.55341960407610458, 60.20724293864768839 ) ) ;
#33521=CARTESIAN_POINT ( 'NONE',  ( -12.06949235617739369, -12.14591786802326823, 94.37609039468568994 ) ) ;
#33522=CARTESIAN_POINT ( 'NONE',  ( 18.62759615963255655, 10.81492255796105972, 76.66775706135234714 ) ) ;
#33523=CARTESIAN_POINT ( 'NONE',  ( 18.67979575497178502, 10.72451020669898547, 54.16557627198103120 ) ) ;
#33524=CARTESIAN_POINT ( 'NONE',  ( 5.823673210054125526, 21.52544592524343514, 44.79057627198103120 ) ) ;
#33525=CARTESIAN_POINT ( 'NONE',  ( 16.53943276465976808, 0.05219959533934440121, 81.25109039468568994 ) ) ;
#33526=CARTESIAN_POINT ( 'NONE',  ( -10.72451020669898014, 18.67979575497178502, 45.41557627198103830 ) ) ;
#33528=CARTESIAN_POINT ( 'NONE',  ( 19.02544592524343514, -5.153800228976328945, 98.54057627198100988 ) ) ;
#33530=CARTESIAN_POINT ( 'NONE',  ( 13.89961937509977652, -13.97604488694527269, 23.12390960531436335 ) ) ;
#33531=CARTESIAN_POINT ( 'NONE',  ( 21.52544592524344225, -5.823673210054117533, 63.54057627198103830 ) ) ;
#33532=CARTESIAN_POINT ( 'NONE',  ( 16.55341960407618274, -4.379528057220086978, 86.04275706135236135 ) ) ;
#33533=CARTESIAN_POINT ( 'NONE',  ( -10.72451020669870658, -18.67979575497194134, 49.58442372801901143 ) ) ;
#33534=CARTESIAN_POINT ( 'NONE',  ( 13.97604488694548053, -13.89961937509957401, 105.6260903946856757 ) ) ;
#33535=CARTESIAN_POINT ( 'NONE',  ( 8.224510206698953496, -14.34966873604960469, 102.9155762719810383 ) ) ;
#33536=CARTESIAN_POINT ( 'NONE',  ( -9.474510206698720793, -16.51473224551083518, 104.5844237280190043 ) ) ;
#33537=CARTESIAN_POINT ( 'NONE',  ( -16.46253265017160317, 9.564922557960807481, 40.83224293864769550 ) ) ;
#33539=CARTESIAN_POINT ( 'NONE',  ( -16.46253265017160317, 9.564922557960807481, 95.83224293864769550 ) ) ;
#33540=CARTESIAN_POINT ( 'NONE',  ( -14.29746914071037622, -8.314922557961029526, 79.16775706135234714 ) ) ;
#33541=CARTESIAN_POINT ( 'NONE',  ( -19.02544592524334988, -5.153800228976617603, 73.95942372801900433 ) ) ;
#33542=CARTESIAN_POINT ( 'NONE',  ( -5.719274019375665041, -21.55341960407619695, 109.7927570613523613 ) ) ;
#33543=CARTESIAN_POINT ( 'NONE',  ( -5.719274019375978568, 21.55341960407610458, 60.20724293864768839 ) ) ;
#33544=CARTESIAN_POINT ( 'NONE',  ( 4.483927247898790824, -16.52544592524335698, 90.20942372801903275 ) ) ;
#33546=CARTESIAN_POINT ( 'NONE',  ( 19.03943276465977164, 0.05219959533936151252, 86.25109039468567573 ) ) ;
#33547=CARTESIAN_POINT ( 'NONE',  ( -16.51473224551069308, -9.474510206698971260, 36.66557627198102409 ) ) ;
#33548=CARTESIAN_POINT ( 'NONE',  ( -19.05341960407611168, -5.049401038298163336, 81.45724293864769550 ) ) ;
#33549=CARTESIAN_POINT ( 'NONE',  ( 15.80617190586769283, -15.72974639402175789, 45.62609039468567573 ) ) ;
#33550=CARTESIAN_POINT ( 'NONE',  ( -5.153800228976328057, -19.02544592524343514, 42.29057627198101699 ) ) ;
#33551=CARTESIAN_POINT ( 'NONE',  ( 19.05341960407617918, -5.049401038297876454, 71.04275706135234714 ) ) ;
#33553=CARTESIAN_POINT ( 'NONE',  ( -9.564922557960796823, -16.46253265017161027, 112.0822429386476955 ) ) ;
#33554=CARTESIAN_POINT ( 'NONE',  ( 16.52544592524342804, -4.483927247898539470, 68.54057627198103830 ) ) ;
#33555=CARTESIAN_POINT ( 'NONE',  ( 10.81492255796078972, 18.62759615963270932, 64.58224293864769550 ) ) ;
#33557=CARTESIAN_POINT ( 'NONE',  ( -19.05341960407617563, 5.049401038297882671, 23.54275706135233648 ) ) ;
#33558=CARTESIAN_POINT ( 'NONE',  ( 0.05219959533909260263, 19.03943276465977164, 69.99890960531435269 ) ) ;
#33559=CARTESIAN_POINT ( 'NONE',  ( 0.05219959533909260263, 19.03943276465977164, 79.99890960531436690 ) ) ;
#33561=CARTESIAN_POINT ( 'NONE',  ( -12.14591786802326823, 12.06949235617739902, 53.12609039468568284 ) ) ;
#33563=CARTESIAN_POINT ( 'NONE',  ( -17.49999999999999645, 5.499999999999997335, 110.7969038253417295 ) ) ;
#33564=CARTESIAN_POINT ( 'NONE',  ( -12.06949235617739369, -12.14591786802326823, 89.37609039468568994 ) ) ;
#33565=CARTESIAN_POINT ( 'NONE',  ( 17.72560187377285956, 5.500000000000005329, 96.57814504131322053 ) ) ;
#33566=CARTESIAN_POINT ( 'NONE',  ( -8.314922557961024197, 14.29746914071037800, 72.91775706135234714 ) ) ;
#33567=CARTESIAN_POINT ( 'NONE',  ( 16.52544592524335698, 4.483927247898782831, 36.45942372801901143 ) ) ;
#33568=CARTESIAN_POINT ( 'NONE',  ( -13.97604488694527625, -13.89961937509977652, 56.87390960531434558 ) ) ;
#33570=CARTESIAN_POINT ( 'NONE',  ( -15.80617190586768217, 15.72974639402176855, 58.12609039468568994 ) ) ;
#33571=CARTESIAN_POINT ( 'NONE',  ( -16.51473224551082808, 9.474510206698731452, 58.33442372801900433 ) ) ;
#33572=CARTESIAN_POINT ( 'NONE',  ( 5.719274019375673035, 21.55341960407619339, 102.2927570613523613 ) ) ;
#33573=CARTESIAN_POINT ( 'NONE',  ( -19.03943276465977164, 0.05219959533909376836, 36.24890960531436690 ) ) ;
#33575=CARTESIAN_POINT ( 'NONE',  ( 15.72974639402199770, -15.80617190586745480, 48.12390960531436690 ) ) ;
#33576=CARTESIAN_POINT ( 'NONE',  ( -0.05219959533909027116, -19.03943276465977164, 107.4989096053143527 ) ) ;
#33577=CARTESIAN_POINT ( 'NONE',  ( -8.224510206698948167, 14.34966873604960824, 95.41557627198102409 ) ) ;
#33578=CARTESIAN_POINT ( 'NONE',  ( 4.483927247898790824, -16.52544592524335698, 35.20942372801901854 ) ) ;
#33579=CARTESIAN_POINT ( 'NONE',  ( 0.05219959533910956823, 16.53943276465976808, 29.99890960531435979 ) ) ;
#33580=VERTEX_POINT ( 'NONE', #92613 ) ;
#33581=CARTESIAN_POINT ( 'NONE',  ( -18.67979575497178146, -10.72451020669898902, 106.6655762719810383 ) ) ;
#33582=CARTESIAN_POINT ( 'NONE',  ( -14.29746914071049879, 8.314922557960819915, 35.83224293864768839 ) ) ;
#33583=CARTESIAN_POINT ( 'NONE',  ( 9.474510206698971260, -16.51473224551069308, 107.9155762719810383 ) ) ;
#33584=CARTESIAN_POINT ( 'NONE',  ( 19.05341960407617918, -5.049401038297876454, 96.04275706135231871 ) ) ;
#33585=CARTESIAN_POINT ( 'NONE',  ( -9.564922557961040184, 16.46253265017147172, 32.91775706135233293 ) ) ;
#33586=CARTESIAN_POINT ( 'NONE',  ( 8.314922557960818139, 14.29746914071049879, 29.58224293864769905 ) ) ;
#33587=CARTESIAN_POINT ( 'NONE',  ( 21.53943276465977519, -0.05219959533907433946, 108.7489096053143669 ) ) ;
#33588=CARTESIAN_POINT ( 'NONE',  ( 0.05219959533907565091, 21.53943276465977519, 54.99890960531435269 ) ) ;
#33589=CARTESIAN_POINT ( 'NONE',  ( -19.05341960407611168, -5.049401038298163336, 76.45724293864769550 ) ) ;
#33590=CARTESIAN_POINT ( 'NONE',  ( -12.14591786802309592, -12.06949235617757132, 41.87390960531435979 ) ) ;
#33591=CARTESIAN_POINT ( 'NONE',  ( 9.564922557960805705, 16.46253265017160317, 94.58224293864769550 ) ) ;
#33594=CARTESIAN_POINT ( 'NONE',  ( 9.564922557961047289, -16.46253265017146816, 45.41775706135232582 ) ) ;
#33595=CARTESIAN_POINT ( 'NONE',  ( -10.81492255796078084, -18.62759615963271287, 92.08224293864769550 ) ) ;
#33596=CARTESIAN_POINT ( 'NONE',  ( -4.379528057220328563, 16.55341960407611168, 105.2072429386477097 ) ) ;
#33598=CARTESIAN_POINT ( 'NONE',  ( 5.719274019375673035, 21.55341960407619339, 37.29275706135235424 ) ) ;
#33600=CARTESIAN_POINT ( 'NONE',  ( 4.379528057220092307, 16.55341960407617563, 107.2927570613523471 ) ) ;
#33601=CARTESIAN_POINT ( 'NONE',  ( 9.564922557960805705, 16.46253265017160317, 29.58224293864769550 ) ) ;
#33602=CARTESIAN_POINT ( 'NONE',  ( 13.89961937509977652, -13.97604488694527269, 83.12390960531436690 ) ) ;
#33604=CARTESIAN_POINT ( 'NONE',  ( -5.049401038298153566, 19.05341960407611168, 30.20724293864768839 ) ) ;
#33605=CARTESIAN_POINT ( 'NONE',  ( -12.06949235617756955, 12.14591786802309770, 40.62390960531435269 ) ) ;
#33606=CARTESIAN_POINT ( 'NONE',  ( 15.80617190586769283, -15.72974639402175789, 70.62609039468567573 ) ) ;
#33608=CARTESIAN_POINT ( 'NONE',  ( 12.14591786802327356, -12.06949235617739191, 70.62609039468567573 ) ) ;
#33609=CARTESIAN_POINT ( 'NONE',  ( 19.02544592524343514, -5.153800228976328945, 53.54057627198102409 ) ) ;
#33610=CARTESIAN_POINT ( 'NONE',  ( 13.97604488694527802, 13.89961937509977652, 64.37390960531436690 ) ) ;
#33611=ORIENTED_EDGE ( 'NONE', *, *, #158579, .T. ) ;
#33612=CARTESIAN_POINT ( 'NONE',  ( -16.46253265017146816, -9.564922557961047289, 19.16775706135233293 ) ) ;
#33613=CARTESIAN_POINT ( 'NONE',  ( 8.224510206698742110, 14.34966873604972548, 77.08442372801901854 ) ) ;
#33614=CARTESIAN_POINT ( 'NONE',  ( -21.52544592524334988, -5.823673210054445271, 103.9594237280190185 ) ) ;
#33615=CARTESIAN_POINT ( 'NONE',  ( -5.153800228976328057, -19.02544592524343514, 67.29057627198102409 ) ) ;
#33616=CARTESIAN_POINT ( 'NONE',  ( 18.67979575497178502, 10.72451020669898547, 34.16557627198102409 ) ) ;
#33617=CARTESIAN_POINT ( 'NONE',  ( 5.049401038297881783, 19.05341960407617563, 102.2927570613523045 ) ) ;
#33618=CARTESIAN_POINT ( 'NONE',  ( 18.67979575497194134, -10.72451020669871369, 85.83442372801901854 ) ) ;
#33619=CARTESIAN_POINT ( 'NONE',  ( -14.34966873604972548, 8.224510206698743886, 48.33442372801902565 ) ) ;
#33620=CARTESIAN_POINT ( 'NONE',  ( -5.823673210054116645, -21.52544592524344225, 102.2905762719810383 ) ) ;
#33621=CARTESIAN_POINT ( 'NONE',  ( 19.03943276465977164, 0.05219959533936151252, 96.25109039468567573 ) ) ;
#33622=CARTESIAN_POINT ( 'NONE',  ( 13.97604488694527802, 13.89961937509977652, 84.37390960531433848 ) ) ;
#33623=CARTESIAN_POINT ( 'NONE',  ( 19.03943276465977164, 0.05219959533936151252, 111.2510903946856757 ) ) ;
#33624=CARTESIAN_POINT ( 'NONE',  ( 16.55341960407618274, -4.379528057220086978, 26.04275706135235779 ) ) ;
#33625=CARTESIAN_POINT ( 'NONE',  ( -8.224510206698948167, 14.34966873604960824, 60.41557627198102409 ) ) ;
#33626=CARTESIAN_POINT ( 'NONE',  ( -12.14591786802326823, 12.06949235617739902, 78.12609039468570415 ) ) ;
#33627=EDGE_CURVE ( 'NONE', #192458, #83484, #139026, .T. ) ;
#33628=CARTESIAN_POINT ( 'NONE',  ( 18.62759615963255655, 10.81492255796105972, 21.66775706135235069 ) ) ;
#33629=CARTESIAN_POINT ( 'NONE',  ( -0.05219959533909027116, -19.03943276465977164, 52.49890960531436690 ) ) ;
#33630=CARTESIAN_POINT ( 'NONE',  ( -5.049401038298153566, 19.05341960407611168, 75.20724293864769550 ) ) ;
#33631=CARTESIAN_POINT ( 'NONE',  ( 8.224510206698742110, 14.34966873604972548, 77.08442372801901854 ) ) ;
#33632=CARTESIAN_POINT ( 'NONE',  ( 15.50000000000000355, 5.499999999999998224, 120.0000000000000142 ) ) ;
#33634=CARTESIAN_POINT ( 'NONE',  ( -5.049401038297874678, -19.05341960407617918, 19.79275706135233293 ) ) ;
#33635=CARTESIAN_POINT ( 'NONE',  ( 5.153800228976335163, 19.02544592524342804, 34.79057627198102409 ) ) ;
#33637=CARTESIAN_POINT ( 'NONE',  ( -14.29746914071037622, -8.314922557961029526, 29.16775706135234003 ) ) ;
#33638=CARTESIAN_POINT ( 'NONE',  ( 13.97604488694548053, -13.89961937509957401, 40.62609039468564731 ) ) ;
#33639=CARTESIAN_POINT ( 'NONE',  ( 16.53943276465976808, 0.05219959533934440121, 31.25109039468568639 ) ) ;
#33640=CARTESIAN_POINT ( 'NONE',  ( 0.05219959533909260263, 19.03943276465977164, 39.99890960531436690 ) ) ;
#33641=CARTESIAN_POINT ( 'NONE',  ( -5.049401038298153566, 19.05341960407611168, 70.20724293864769550 ) ) ;
#33642=CARTESIAN_POINT ( 'NONE',  ( -10.72451020669898014, 18.67979575497178502, 80.41557627198103830 ) ) ;
#33643=CARTESIAN_POINT ( 'NONE',  ( -16.46253265017160317, 9.564922557960807481, 75.83224293864769550 ) ) ;
#33645=CARTESIAN_POINT ( 'NONE',  ( -19.05341960407611168, -5.049401038298163336, 51.45724293864770260 ) ) ;
#33646=FACE_OUTER_BOUND ( 'NONE', #187559, .T. ) ;
#33647=CARTESIAN_POINT ( 'NONE',  ( -5.153800228976607833, 19.02544592524334988, 102.7094237280189759 ) ) ;
#33648=CARTESIAN_POINT ( 'NONE',  ( 10.81492255796078972, 18.62759615963270932, 74.58224293864768129 ) ) ;
#33649=CARTESIAN_POINT ( 'NONE',  ( 19.02544592524334988, 5.153800228976608722, 21.45942372801899012 ) ) ;
#33650=CARTESIAN_POINT ( 'NONE',  ( -16.52544592524342804, 4.483927247898546575, 61.04057627198103120 ) ) ;
#33651=CARTESIAN_POINT ( 'NONE',  ( 18.62759615963255655, 10.81492255796105972, 86.66775706135234714 ) ) ;
#33652=CARTESIAN_POINT ( 'NONE',  ( -5.153800228976328057, -19.02544592524343514, 22.29057627198102765 ) ) ;
#33653=CARTESIAN_POINT ( 'NONE',  ( 16.52544592524342804, -4.483927247898539470, 28.54057627198103120 ) ) ;
#33654=CARTESIAN_POINT ( 'NONE',  ( -21.52544592524334988, -5.823673210054445271, 93.95942372801903275 ) ) ;
#33655=CARTESIAN_POINT ( 'NONE',  ( 19.05341960407611168, 5.049401038298154454, 83.95724293864766707 ) ) ;
#33656=CARTESIAN_POINT ( 'NONE',  ( -21.53943276465977519, -0.05219959533937600094, 48.75109039468568284 ) ) ;
#33657=CARTESIAN_POINT ( 'NONE',  ( 5.049401038298161559, -19.05341960407611168, 87.70724293864769550 ) ) ;
#33658=CARTESIAN_POINT ( 'NONE',  ( 16.55341960407611168, 4.379528057220329451, 93.95724293864770971 ) ) ;
#33659=CARTESIAN_POINT ( 'NONE',  ( -8.224510206698948167, 14.34966873604960824, 65.41557627198102409 ) ) ;
#33660=CARTESIAN_POINT ( 'NONE',  ( -21.55341960407610458, -5.719274019375992779, 76.45724293864769550 ) ) ;
#33661=CARTESIAN_POINT ( 'NONE',  ( 13.89961937509977652, -13.97604488694527269, 68.12390960531436690 ) ) ;
#33662=CARTESIAN_POINT ( 'NONE',  ( -18.67979575497178146, -10.72451020669898902, 81.66557627198103830 ) ) ;
#33663=CARTESIAN_POINT ( 'NONE',  ( 13.89961937509957401, 13.97604488694547697, 76.87609039468566152 ) ) ;
#33664=CARTESIAN_POINT ( 'NONE',  ( 5.153800228976617603, -19.02544592524335343, 30.20942372801900433 ) ) ;
#33665=CARTESIAN_POINT ( 'NONE',  ( -8.224510206698948167, 14.34966873604960824, 70.41557627198102409 ) ) ;
#33666=CARTESIAN_POINT ( 'NONE',  ( 5.823673210054125526, 21.52544592524343514, 54.79057627198104541 ) ) ;
#33667=CARTESIAN_POINT ( 'NONE',  ( 16.21995358207307092, -7.366697692864084601, 27.43551001512161136 ) ) ;
#33668=CARTESIAN_POINT ( 'NONE',  ( 0.05219959533934541429, -16.53943276465976808, 105.0010903946856757 ) ) ;
#33670=CARTESIAN_POINT ( 'NONE',  ( 19.05341960407617918, -5.049401038297876454, 101.0427570613523045 ) ) ;
#33671=CARTESIAN_POINT ( 'NONE',  ( -16.52544592524342804, 4.483927247898546575, 76.04057627198102409 ) ) ;
#33673=CARTESIAN_POINT ( 'NONE',  ( -13.89961937509977652, 13.97604488694528158, 70.62390960531432427 ) ) ;
#33674=CARTESIAN_POINT ( 'NONE',  ( -13.89961937509977652, 13.97604488694528158, 35.62390960531435269 ) ) ;
#33675=CARTESIAN_POINT ( 'NONE',  ( 12.14591786802309770, 12.06949235617756955, 49.37390960531436690 ) ) ;
#33676=CARTESIAN_POINT ( 'NONE',  ( 9.474510206698971260, -16.51473224551069308, 107.9155762719810383 ) ) ;
#33677=CARTESIAN_POINT ( 'NONE',  ( 16.51473224551083163, -9.474510206698727899, 85.83442372801900433 ) ) ;
#33678=CARTESIAN_POINT ( 'NONE',  ( 0.05219959533909260263, 19.03943276465977164, 59.99890960531436690 ) ) ;
#33679=CARTESIAN_POINT ( 'NONE',  ( -16.55341960407617563, 4.379528057220093196, 23.54275706135235424 ) ) ;
#33680=CARTESIAN_POINT ( 'NONE',  ( 19.02544592524343514, -5.153800228976328945, 88.54057627198102409 ) ) ;
#33681=CARTESIAN_POINT ( 'NONE',  ( -0.05219959533907301413, -21.53943276465977519, 62.49890960531436690 ) ) ;
#33682=CARTESIAN_POINT ( 'NONE',  ( -12.06949235617739369, -12.14591786802326823, 59.37609039468568284 ) ) ;
#33683=CARTESIAN_POINT ( 'NONE',  ( -16.51473224551082808, 9.474510206698731452, 108.3344237280190043 ) ) ;
#33684=CARTESIAN_POINT ( 'NONE',  ( -5.049401038298153566, 19.05341960407611168, 65.20724293864765286 ) ) ;
#33685=CARTESIAN_POINT ( 'NONE',  ( 21.52544592524344225, -5.823673210054117533, 63.54057627198103830 ) ) ;
#33686=CARTESIAN_POINT ( 'NONE',  ( -19.02544592524334988, -5.153800228976617603, 88.95942372801897591 ) ) ;
#33687=CARTESIAN_POINT ( 'NONE',  ( 12.06949235617757843, -12.14591786802309237, 23.12390960531436335 ) ) ;
#33688=CARTESIAN_POINT ( 'NONE',  ( 18.67979575497194134, -10.72451020669871369, 50.83442372801901143 ) ) ;
#33690=CARTESIAN_POINT ( 'NONE',  ( -14.34966873604972548, 8.224510206698743886, 68.33442372801900433 ) ) ;
#33691=CARTESIAN_POINT ( 'NONE',  ( -9.564922557960796823, -16.46253265017161027, 107.0822429386476955 ) ) ;
#33692=CARTESIAN_POINT ( 'NONE',  ( -17.97182807773872071, 5.500000000000055955, 73.53038844047289047 ) ) ;
#33693=CARTESIAN_POINT ( 'NONE',  ( -14.29746914071037622, -8.314922557961029526, 94.16775706135237556 ) ) ;
#33694=CARTESIAN_POINT ( 'NONE',  ( -4.483927247898782831, 16.52544592524335698, 32.70942372801900433 ) ) ;
#33695=CARTESIAN_POINT ( 'NONE',  ( -9.564922557960796823, -16.46253265017161027, 47.08224293864769550 ) ) ;
#33696=CARTESIAN_POINT ( 'NONE',  ( 13.97604488694527802, 13.89961937509977652, 49.37390960531434558 ) ) ;
#33697=CARTESIAN_POINT ( 'NONE',  ( 5.153800228976335163, 19.02544592524342804, 64.79057627198100988 ) ) ;
#33698=CARTESIAN_POINT ( 'NONE',  ( -10.72451020669870658, -18.67979575497194134, 49.58442372801901143 ) ) ;
#33699=CARTESIAN_POINT ( 'NONE',  ( 4.483927247898790824, -16.52544592524335698, 45.20942372801901854 ) ) ;
#33700=CARTESIAN_POINT ( 'NONE',  ( -4.379528057220328563, 16.55341960407611168, 35.20724293864768839 ) ) ;
#33701=CARTESIAN_POINT ( 'NONE',  ( 5.153800228976335163, 19.02544592524342804, 39.79057627198100988 ) ) ;
#33702=CARTESIAN_POINT ( 'NONE',  ( -5.049401038298153566, 19.05341960407611168, 40.20724293864768839 ) ) ;
#33703=CARTESIAN_POINT ( 'NONE',  ( 8.224510206698742110, 14.34966873604972548, 32.08442372801901854 ) ) ;
#33705=CARTESIAN_POINT ( 'NONE',  ( -13.89961937509957401, -13.97604488694547875, 84.37609039468567573 ) ) ;
#33706=CARTESIAN_POINT ( 'NONE',  ( -0.05219959533910754901, -16.53943276465976808, 82.49890960531436690 ) ) ;
#33707=CARTESIAN_POINT ( 'NONE',  ( -9.474510206698964154, 16.51473224551069663, 55.41557627198103120 ) ) ;
#33708=CARTESIAN_POINT ( 'NONE',  ( -5.049401038297874678, -19.05341960407617918, 84.79275706135233293 ) ) ;
#33709=CARTESIAN_POINT ( 'NONE',  ( 16.31925111598456013, -7.325300261831516835, 92.66424538967251578 ) ) ;
#33710=CARTESIAN_POINT ( 'NONE',  ( 21.55341960407619695, -5.719274019375665929, 76.04275706135237556 ) ) ;
#33711=CARTESIAN_POINT ( 'NONE',  ( -14.29746914071037622, -8.314922557961029526, 59.16775706135234714 ) ) ;
#33713=CARTESIAN_POINT ( 'NONE',  ( 0.05219959533907565091, 21.53943276465977519, 54.99890960531435269 ) ) ;
#33714=CARTESIAN_POINT ( 'NONE',  ( 4.379528057220092307, 16.55341960407617563, 37.29275706135235424 ) ) ;
#33716=CARTESIAN_POINT ( 'NONE',  ( -19.02544592524334988, -5.153800228976617603, 28.95942372801900433 ) ) ;
#33718=CARTESIAN_POINT ( 'NONE',  ( -16.51473224551069308, -9.474510206698971260, 46.66557627198102409 ) ) ;
#33719=CARTESIAN_POINT ( 'NONE',  ( -17.59860650958993844, 7.585241751806885979, 58.42337014262493256 ) ) ;
#33720=CARTESIAN_POINT ( 'NONE',  ( -16.51473224551069308, -9.474510206698971260, 71.66557627198102409 ) ) ;
#33721=CARTESIAN_POINT ( 'NONE',  ( -19.01529144963332740, -5.500000000000168754, 56.23431955728440101 ) ) ;
#33722=CARTESIAN_POINT ( 'NONE',  ( 21.53943276465977519, 0.05219959533937863772, 111.2510903946856899 ) ) ;
#33723=CARTESIAN_POINT ( 'NONE',  ( -4.483927247898539470, -16.52544592524342804, 32.29057627198102409 ) ) ;
#33724=CARTESIAN_POINT ( 'NONE',  ( 19.02544592524343514, -5.153800228976328945, 43.54057627198103120 ) ) ;
#33726=CARTESIAN_POINT ( 'NONE',  ( 13.97604488694527802, 13.89961937509977652, 99.37390960531436690 ) ) ;
#33727=CARTESIAN_POINT ( 'NONE',  ( -21.52544592524334988, -5.823673210054445271, 73.95942372801901854 ) ) ;
#33728=CARTESIAN_POINT ( 'NONE',  ( 0.05219959533909260263, 19.03943276465977164, 44.99890960531435979 ) ) ;
#33730=CARTESIAN_POINT ( 'NONE',  ( -21.55341960407619339, 5.719274019375674811, 63.54275706135234003 ) ) ;
#33731=CARTESIAN_POINT ( 'NONE',  ( -21.53943276465977519, 0.05219959533907696930, 26.24890960531435624 ) ) ;
#33732=CARTESIAN_POINT ( 'NONE',  ( -19.05341960407611168, -5.049401038298163336, 36.45724293864766707 ) ) ;
#33733=CARTESIAN_POINT ( 'NONE',  ( 21.53943276465977519, 0.05219959533937863772, 31.25109039468568639 ) ) ;
#33734=CARTESIAN_POINT ( 'NONE',  ( -16.51473224551082808, 9.474510206698731452, 43.33442372801900433 ) ) ;
#33735=CARTESIAN_POINT ( 'NONE',  ( 5.153800228976335163, 19.02544592524342804, 29.79057627198102409 ) ) ;
#33736=CARTESIAN_POINT ( 'NONE',  ( -9.474510206698964154, 16.51473224551069663, 60.41557627198102409 ) ) ;
#33737=CARTESIAN_POINT ( 'NONE',  ( 8.314922557961029526, -14.29746914071037800, 20.41775706135234714 ) ) ;
#33739=CARTESIAN_POINT ( 'NONE',  ( 16.55341960407611168, 4.379528057220329451, 68.95724293864769550 ) ) ;
#33740=CARTESIAN_POINT ( 'NONE',  ( 5.823673210054125526, 21.52544592524343514, 34.79057627198103120 ) ) ;
#33741=CARTESIAN_POINT ( 'NONE',  ( -13.97604488694547697, 13.89961937509957934, 103.1260903946856473 ) ) ;
#33742=CARTESIAN_POINT ( 'NONE',  ( 10.81492255796078972, 18.62759615963270932, 109.5822429386476955 ) ) ;
#33743=CARTESIAN_POINT ( 'NONE',  ( -5.719274019375665041, -21.55341960407619695, 54.79275706135235424 ) ) ;
#33744=CARTESIAN_POINT ( 'NONE',  ( -16.55341960407617563, 4.379528057220093196, 53.54275706135234714 ) ) ;
#33745=CARTESIAN_POINT ( 'NONE',  ( 12.14591786802327356, -12.06949235617739191, 60.62609039468567573 ) ) ;
#33746=CARTESIAN_POINT ( 'NONE',  ( -5.823673210054116645, -21.52544592524344225, 62.29057627198102409 ) ) ;
#33748=( BOUNDED_SURFACE ( )  B_SPLINE_SURFACE ( 3, 2, ( 
 ( #26588, #168061, #198403, #29558, #59881, #88231, #149915, #57915, #90219, #11422, #196445, #181270, #42747, #104409, #166091, #74081, #135752, #151902, #13392, #55781, #68946, #145780, #115460, #113439, #54781, #7261, #83106, #99272, #84101, #130609, #177149, #69957, #114439, #117453, #40620, #116456, #179152, #146786, #10293, #86115, #192305, #53784, #193307, #24465, #38621, #178144, #21445, #8279, #102290, #85100, #161957, #160959, #51779, #131622, #100278, #159958, #6265, #147806, #163979, #23453, #39610, #144782, #101269, #162959, #9291, #70957, #132626, #194314, #25476, #87116, #148803, #175132, #128610, #22452, #36599, #190302, #98255, #67945, #129598, #191294, #52770, #176140, #37610, #199277, #196324, #27468, #165966, #106257, #60744, #12296, #89110, #58764, #56795, #198280, #150800, #26467, #42621, #73961, #135629, #120433, #13274, #57792, #122417, #184109, #59758, #45590, #90099, #153756, #29439, #197300, #182125, #136600, #167940, #43609, #121426, #164972, #151781, #107244, #28463, #168915, #30420, #105274, #92068, #44602, #104286, #74937, #166961, #183119, #118467, #88109, #149793, #71950, #91071, #152758, #180159, #14247, #75919, #137594, #41628, #133621, #195314, #103292, #72969, #11298, #134638, #119462, #181146, #156753, #109239, #3059, #18247, #80885, #15252, #142562, #157746, #1055, #19237, #34400, #65718, #110235, #35388, #186105, #140572, #31416, #155744, #4041, #108245, #154754, #46583, #97039, #76910, #16251, #170918, #138581, #61, #169924, #62728, #127385, #96058, #93068, #124411, #32410, #171916, #126398, #189096, #188094, #50569, #112229, #33406, #95064, #173919, #61734, #123402, #17242, #94065, #77903, #48583, #47586, #111229, #139570, #79900, #185095, #78893, #172921, #2062, #141571, #63741, #125415, #187112, #64736, #49567, #174905, #191068, #52541, #23222, #113215, #145548, #178914, #175906, #68708, #144550, #130365, #40381, #190075, #129372, #161727, #54548, #193073, #176914, #99035, #114202, #192062, #147569, #100041, #128379, #146543, #67714, #51551, #7026, #131384, #116221, #37378, #98023, #84865, #82872, #36369, #117220, #8036, #177912, #38385, #39380, #69717, #101039, #132392, #70725, #158720, #21215, #160725, #159718, #162725, #6035, #53544, #24230, #85881, #20210, #22217, #9054, #83866, #115222, #81858, #194085, #55547, #143546, #5032, #66718, #186621, #196089, #166730, #182889, #63245, #140078, #13046, #93579, #102055, #121196, #1569, #195075, #181896, #28234, #11054, #74713, #71716, #89874, #134402, #120206, #31925, #16754, #57559, #58540, #163740, #133384, #25240, #78402, #86881, #165731, #56554, #43374, #155264, #124924, #104051, #148566, #136376, #119229, #105046, #150568, #151557, #10056, #118231, #179922, #41389, #198053, #59519, #103054, #44372, #27227, #88875, #164736, #108757, #170433, #26231, #87870, #149558, #72729, #180913, #42388, #12067, #73729, #135402, #197073, #113709, #48093, #175406, #190577, #33910, #52053, #67219, #98539, #143054, #68214, #18748, #173426, #64249, #188597, #36874, #141082, #187614, #79412, #129866, #109749, #49084, #3553, #171433, #32920, #2567, #95568, #160233, #81370, #80395, #94575, #127886, #50078, #125916, #110741, #5540, #83376, #19729, #159219, #172422, #158238, #4533, #126891, #66225, #189589, #174416, #21723, #20714, #145053, #156253, #6534, #142067, #17755, #157254, #51061, #65231, #112723, #111739, #34895, #96551, #35885, #97532, #82370, #144059, #128877, #25741, #118737, #131897, #8553, #178413, #176416, #117728, #70229, #146050, #162228, #147069, #193581, #39877, #132890, #177421, #180425, #103564, #179423, #41898, #9561, #73237, #149072, #55053, #116724, #56049, #87387, #101544, #40888, #84373, #71227, #165239, #7534, #130887, #22725, #191564, #53043, #192577, #163236, #114723, #37891, #69219, #38892, #26733, #24736, #23727, #99549, #194579, #86386, #54060, #115734, #10560, #88372, #148070, #102561 ),
 ( #161231, #100549, #85376, #164246, #72224, #150066, #11571, #133899, #195590, #57062, #154024, #31681, #27734, #14519, #199540, #43874, #45852, #104552, #122682, #167225, #153020, #61994, #46848, #28723, #91328, #196585, #166234, #134908, #108508, #16511, #198552, #89377, #15519, #151066, #105539, #90360, #29697, #107505, #77176, #169181, #138846, #123660, #76180, #137860, #93330, #185357, #170187, #75196, #152045, #135891, #168200, #13530, #30687, #12557, #61010, #155015, #58055, #92338, #74223, #184371, #326, #119726, #136867, #44867, #181409, #197563, #60022, #121689, #42887, #59030, #183385, #120697, #106523, #182396, #64000, #188348, #98283, #109502, #48837, #81133, #174173, #112480, #96310, #18502, #172173, #49826, #66975, #19488, #47849, #65976, #187368, #171184, #126645, #186370, #142814, #3314, #64987, #124673, #20468, #35643, #139827, #79158, #94326, #113465, #128635, #32673, #4294, #33658, #127645, #189345, #143810, #78159, #5292, #82118, #125670, #190329, #97289, #51806, #173175, #159984, #110491, #111490, #156004, #80150, #175159, #17501, #140829, #2318, #1316, #62995, #95319, #157004, #141821, #34651, #157996, #50823, #36626, #158976, #53813, #144808, #101298, #161984, #52796, #99300, #179179, #56820, #193334, #132653, #37636, #131652, #178172, #100306, #39637, #162987, #147834, #25502, #194341, #133649, #6291, #195340, #115488, #67970, #87146, #54808, #21471, #24492, #177176, #83132, #10319, #23480, #148829, #145806, #38649, #85129, #55809, #71975, #146813, #8307, #69984, #129624, #9320, #116483, #176166, #192332, #86143, #70985, #117481, #40647, #7289, #118494, #180185, #102316, #41654, #164006, #103318, #191319, #114464, #160985, #22479, #84127, #68973, #130637, #57817, #183142, #92093, #121450, #153781, #15276, #166984, #123425, #137619, #197326, #44627, #13296, #106279, #149818, #119489, #181171, #87, #167964, #14275, #60770, #134663, #198304, #184134, #29463, #26492, #42648, #199303, #135655, #28487, #46608, #45616, #122442, #168939, #107268, #164998, #88134, #58790, #91096, #30446, #185118, #61757, #75945, #76936, #11324, #138605, #72994, #104310, #152784, #196349, #73986, #165993, #27494, #89136, #120458, #150824, #12321, #182149, #43634, #105296, #90121, #151805, #74961, #136623, #59782, #171940, #77926, #127410, #139593, #17266, #2086, #3083, #19262, #189120, #80908, #50592, #97062, #64759, #126421, #5056, #158744, #20233, #48607, #63766, #109264, #141596, #78919, #4064, #1079, #188119, #81881, #31439, #65742, #62754, #49590, #173943, #190099, #187135, #18270, #154777, #124435, #140596, #125439, #172945, #186131, #95088, #128402, #110259, #79923, #94089, #111253, #108270, #47610, #33429, #34423, #112251, #142585, #96082, #156777, #157771, #35410, #143573, #66741, #170943, #169948, #93093, #32435, #16274, #155768, #24257, #160750, #191092, #54573, #175932, #144573, #10083, #39404, #70750, #131410, #9080, #69741, #101064, #25265, #163765, #71741, #114227, #68733, #82895, #6060, #147595, #21241, #84891, #132418, #193097, #113238, #67738, #85908, #22242, #53571, #133412, #194110, #55573, #117247, #178939, #51574, #174929, #145574, #116245, #40409, #36392, #86908, #162749, #102081, #98046, #148591, #159744, #129396, #177937, #52567, #83891, #37404, #99062, #7051, #130391, #192088, #115248, #176940, #38410, #8064, #100067, #161752, #23247, #146570, #76709, #58566, #164762, #14044, #26257, #104078, #88904, #89899, #106054, #75710, #167740, #137388, #183904, #151582, #13071, #91858, #45389, #107042, #135428, #150595, #196115, #28261, #165760, #90871, #87898, #74738, #168714, #118258, #152555, #149584, #136401, #60537, #195101, #73756, #105073, #41415, #11082, #27254, #12093, #59546, #72758, #181922, #15048, #197099, #166759, #180939, #198079, #56583, #134429, #120231, #121224, #199068, #29238, #182915, #43403, #44400, #122213, #30216, #153551, #57585, #179948, #103081, #119255 ),
 ( #42415, #187895, #112027, #50367, #158523, #853, #155545, #16046, #95857, #173716, #110037, #49362, #154551, #48380, #94864, #17039, #156545, #18044, #64533, #142357, #111026, #35184, #123203, #96838, #32210, #184893, #3837, #171716, #138384, #79697, #93866, #200066, #127176, #78693, #65516, #62527, #140370, #1857, #172712, #188886, #63539, #125213, #186909, #46375, #126199, #33205, #92864, #109040, #141368, #2855, #34195, #157540, #124200, #20011, #61534, #19034, #108034, #80681, #169720, #31213, #77705, #139371, #185900, #47385, #170718, #131174, #174701, #99835, #8844, #38179, #70512, #132180, #83661, #40164, #54343, #113992, #161519, #130154, #23011, #66512, #36165, #97817, #117007, #84657, #192864, #189873, #146335, #6821, #68499, #128174, #24014, #39171, #143337, #82657, #159506, #178702, #193871, #21002, #7823, #175690, #69508, #116014, #147356, #81654, #55337, #85669, #67505, #101840, #100829, #163526, #176705, #4824, #52336, #191851, #144341, #22009, #51348, #5829, #129162, #113008, #190859, #37165, #98824, #160518, #145339, #53332, #115011, #177704, #162512, #58340, #57357, #148353, #104841, #165531, #56339, #89670, #120989, #135201, #74512, #118021, #43174, #152335, #181693, #13821, #75487, #27027, #183680, #197853, #119031, #166532, #73529, #28029, #9849, #179711, #41183, #60313, #151357, #136178, #133176, #12846, #150368, #11864, #71508, #167518, #182687, #86670, #26024, #102846, #121989, #137160, #164531, #59320, #180714, #44172, #105831, #90653, #25026, #198849, #29013, #10851, #45165, #106821, #194866, #120008, #87669, #195883, #196873, #149354, #88672, #72520, #134195, #42190, #103850, #50131, #168495, #169485, #123959, #29993, #153320, #199841, #15813, #80448, #1622, #621, #91632, #48145, #108807, #61308, #46147, #125968, #3606, #140131, #79465, #184665, #78457, #124978, #47149, #186675, #109802, #94628, #172476, #141134, #142121, #14822, #65285, #62292, #76483, #33963, #63298, #138160, #171485, #185657, #122978, #157306, #170486, #95621, #92633, #31977, #93633, #2624, #18803, #155318, #16807, #32974, #107801, #156307, #17808, #30985, #139144, #64301, #187667, #49137, #110795, #154324, #126944, #188652, #77474, #103353, #129918, #196383, #72010, #175459, #190631, #191618, #41688, #68267, #165031, #26524, #113763, #73028, #87181, #144112, #53097, #160286, #114775, #96604, #66281, #4588, #149853, #176469, #161283, #19782, #37943, #36930, #98592, #158293, #56854, #133683, #173479, #112776, #127940, #11357, #88169, #189642, #99603, #5592, #25537, #148862, #180218, #111791, #134700, #118529, #97584, #34952, #195375, #81423, #6588, #143109, #82423, #21777, #51117, #52106, #174469, #35938, #159272, #20768, #67272, #128930, #83428, #145105, #10353, #42683, #89169, #105330, #169981, #91128, #90155, #181207, #137650, #198338, #150861, #135688, #15309, #93124, #29495, #168971, #74018, #167999, #14311, #136658, #75977, #199337, #184166, #61789, #30476, #31472, #123459, #153814, #57852, #139624, #151838, #122475, #138639, #16307, #154809, #92127, #46641, #119524, #76968, #77957, #12355, #60802, #45648, #167018, #120, #27528, #107299, #13328, #185151, #108301, #104344, #74993, #166028, #197360, #58825, #120492, #182183, #43668, #121484, #28519, #59814, #183178, #44660, #106313, #152818, #112283, #81911, #173973, #143604, #190128, #82928, #1112, #2118, #156810, #62786, #186164, #32469, #48640, #113267, #34455, #33462, #124467, #80941, #141627, #94122, #78953, #158777, #36423, #172976, #35441, #17299, #111286, #157802, #79958, #19293, #142616, #127443, #63800, #4095, #18302, #155801, #174959, #95120, #47646, #66770, #96114, #109297, #65774, #3117, #170976, #51603, #64792, #128431, #125473, #126453, #188151, #97093, #98078, #49624, #189149, #50622, #140628, #20265, #5088, #187169, #171974, #159776, #21271, #110292, #85935, #130424, #71772, #56613, #132447, #133442, #162778, #26287 ),
 ( #84921, #100098, #145606, #177964, #115280, #40437, #175965, #39432, #195132, #67770, #102109, #37434, #101092, #10112, #144606, #23277, #54600, #191125, #160786, #176973, #38442, #9112, #99094, #131440, #164792, #161782, #116274, #192123, #24286, #6091, #22274, #146601, #147624, #163794, #178970, #70779, #8094, #69772, #194138, #118287, #55602, #114261, #117276, #53604, #83925, #193127, #25296, #86938, #148622, #179978, #41446, #103111, #7085, #129427, #52599, #68766, #183929, #180966, #121250, #153576, #169745, #166787, #198109, #134458, #104107, #120258, #181950, #152582, #42443, #74766, #108061, #105101, #59576, #73784, #182944, #87928, #119283, #58592, #90896, #45414, #122239, #106081, #28288, #43432, #44427, #76734, #29265, #57615, #75739, #197125, #165789, #136428, #60563, #107067, #89928, #27286, #14072, #12120, #88932, #46402, #137416, #168738, #167767, #30242, #199096, #91885, #61558, #200090, #149615, #150624, #151609, #135456, #15074, #13101, #138410, #123227, #184918, #11113, #72788, #196143, #1883, #34222, #79725, #47410, #81681, #35211, #127202, #31240, #113037, #125238, #95884, #112054, #189901, #66540, #142385, #20038, #92890, #50394, #128204, #124229, #111053, #157567, #140395, #3864, #878, #19060, #63564, #49390, #158548, #143363, #186936, #187921, #154576, #62553, #16072, #4855, #77730, #94891, #185925, #173742, #109066, #48407, #110063, #126226, #65543, #96864, #188916, #51376, #139396, #172741, #80707, #170745, #32234, #93892, #171743, #33232, #155570, #17065, #78719, #156575, #18070, #141394, #2882, #64561, #116043, #144370, #162539, #83690, #5857, #23040, #147385, #8873, #145368, #114022, #177732, #98854, #67533, #133202, #24043, #193900, #54371, #132209, #192894, #85698, #148382, #86697, #194893, #37198, #191880, #129191, #70541, #190889, #7852, #55364, #39201, #36192, #52365, #117034, #6850, #100857, #84685, #175719, #25054, #178729, #40191, #174729, #56367, #68529, #101871, #163554, #97846, #9876, #71536, #159535, #21033, #82686, #160549, #22039, #130184, #53364, #115042, #176734, #38207, #99863, #161547, #146365, #69539, #131203, #165555, #166556, #179740, #87694, #118050, #198873, #41210, #120032, #10875, #29038, #72545, #27052, #11890, #89696, #182712, #90678, #44197, #152360, #60340, #28055, #151382, #183705, #122014, #137186, #196898, #73553, #180738, #12872, #88698, #167543, #134222, #74537, #102871, #26050, #13845, #195908, #136202, #75512, #164556, #181718, #197877, #57383, #103875, #58365, #43200, #105856, #42214, #59346, #149379, #121014, #119056, #150394, #135226, #104867, #129838, #69190, #101515, #149045, #53014, #39849, #192548, #86358, #163205, #164217, #98510, #25714, #40860, #84345, #102534, #117700, #10533, #193553, #118708, #130856, #23698, #114693, #38865, #87359, #191537, #37862, #176388, #180398, #160205, #99521, #54031, #21695, #83349, #161203, #146023, #72197, #131868, #115705, #145025, #178385, #100521, #22698, #7506, #56022, #133871, #70201, #9533, #177393, #8523, #55025, #162200, #116696, #24709, #148043, #85346, #71200, #147039, #132863, #195561, #194552, #6506, #57035, #179397, #68186, #121663, #135866, #103536, #30661, #120671, #169157, #166208, #197537, #59005, #76154, #92314, #182371, #43848, #28697, #26707, #168173, #105514, #196559, #12532, #167199, #90333, #152018, #183358, #27709, #153997, #15495, #29670, #77151, #59996, #123636, #199516, #13504, #75169, #106496, #137834, #136841, #91302, #134883, #44840, #138822, #198525, #302, #61970, #152993, #41870, #14493, #74197, #60983, #122658, #184346, #88346, #58030, #119700, #165211, #45828, #107479, #150039, #11544, #73212, #181383, #42861, #104527, #89352, #151042, #186343, #1290, #20440, #3290, #34626, #158951, #97263, #5266, #47824, #2293, #16485, #81109, #154989, #18477, #4270, #64961, #46823, #62968, #19464, #155978, #188322, #33634, #124648, #35618, #189320, #142788, #185333 ),
 ( #49801, #94300, #96285, #78134, #173151, #17475, #126621, #112456, #82092, #79132, #141796, #108483, #139802, #170161, #143784, #66948, #48813, #109474, #65949, #171159, #140804, #63975, #80127, #157971, #127620, #50797, #174146, #31654, #111466, #93304, #32645, #125645, #187342, #110466, #172148, #95296, #156980, #137141, #45143, #139122, #88653, #58322, #196856, #598, #121966, #153299, #11845, #168474, #28994, #90634, #150349, #46124, #61286, #165513, #104824, #119990, #62269, #154302, #181676, #106800, #197835, #91611, #29972, #169463, #103832, #30964, #107778, #89651, #92611, #122955, #15791, #198829, #123937, #74494, #152316, #43157, #44152, #77451, #166513, #28011, #135182, #185635, #27009, #151339, #59301, #73510, #12828, #136160, #120970, #182668, #184643, #105811, #167498, #13802, #60293, #14800, #75468, #76461, #183659, #138137, #199818, #3583, #144088, #97561, #35915, #187643, #2599, #48122, #155294, #66257, #108785, #16784, #142098, #159249, #170463, #143086, #140108, #80425, #112752, #128907, #125945, #157282, #93609, #63275, #79440, #141111, #111768, #1599, #33940, #67248, #64278, #18778, #32950, #65261, #47127, #78433, #17785, #50108, #4565, #81400, #126921, #49114, #110771, #188628, #20745, #173457, #124955, #34926, #156284, #186651, #95598, #19759, #127917, #172453, #109779, #96581, #171462, #94605, #5569, #158270, #189619, #51092, #174446, #82400, #31954, #164279, #102594, #10594, #53074, #7564, #21753, #86417, #160263, #23759, #9594, #8586, #52083, #6565, #24770, #161260, #193612, #38921, #68242, #40921, #194610, #148102, #190607, #72255, #84403, #55084, #71259, #149104, #25773, #101579, #179455, #113739, #132923, #87419, #83404, #70260, #116754, #99578, #163268, #145082, #178445, #22754, #131928, #117763, #175436, #146079, #147101, #36906, #129895, #98569, #191595, #114752, #54089, #176446, #37919, #56082, #115763, #69250, #39912, #130916, #100578, #192607, #177451, #162260, #85409, #90390, #61039, #122711, #135925, #92367, #106553, #73270, #167255, #75227, #169211, #118769, #88405, #26765, #30720, #152075, #183413, #41930, #198585, #59061, #120728, #180458, #76210, #91359, #195623, #134939, #150101, #154053, #184401, #11602, #136898, #27767, #121721, #60053, #199570, #133933, #45881, #137889, #119757, #107535, #153050, #15548, #28754, #57095, #104584, #182428, #196617, #74255, #103596, #58087, #181440, #165271, #42919, #166269, #89410, #151099, #12590, #197595, #43906, #105569, #13560, #44896, #168229, #29726, #14552, #17531, #108539, #155046, #34681, #112509, #48867, #188378, #93360, #187399, #33688, #156034, #95351, #157035, #3343, #139858, #18533, #94355, #170218, #189375, #171214, #62025, #142844, #110522, #77206, #80180, #32704, #138875, #66007, #79190, #4323, #1346, #140860, #2349, #111520, #127675, #64030, #125700, #172203, #123689, #65018, #141852, #31711, #47879, #126674, #49855, #173206, #96339, #63027, #50852, #174203, #158026, #35671, #19517, #81162, #109532, #97319, #159005, #355, #185388, #46879, #16541, #78188, #124705, #186402, #105088, #86925, #190359, #42431, #51836, #132433, #117263, #118274, #134445, #104093, #196130, #165776, #12107, #179965, #41431, #120245, #73770, #135443, #163781, #178955, #24273, #128664, #27270, #82146, #113495, #103097, #197112, #143842, #119270, #175190, #56600, #88919, #20498, #102096, #133429, #67005, #36656, #55588, #40425, #87915, #98314, #10099, #43418, #25282, #195117, #9098, #164779, #5321, #160014, #194125, #26273, #180953, #57601, #149602, #148607, #71759, #11099, #58579, #72775, #85922, #150611, #181936, #147610, #70765, #139382, #864, #75725, #106067, #169731, #90884, #59560, #125224, #154562, #185911, #46388, #124213, #184904, #16058, #140382, #78705, #186922, #29251, #183916, #198095, #62539, #136415, #200077, #47396, #108046, #28275, #182930, #109052, #137401, #31226, #15060, #44413, #17050, #170729, #32220, #166774 ),
 ( #93878, #155556, #107054, #45401, #153563, #199082, #92875, #76720, #167753, #1869, #63550, #48392, #89914, #151596, #60550, #77716, #13087, #74752, #121236, #152569, #14058, #122225, #168726, #30229, #91870, #138396, #61545, #123214, #21014, #79711, #97830, #142370, #128187, #37178, #22021, #3849, #66524, #171729, #141380, #110049, #83673, #191863, #173728, #2868, #129174, #64546, #19046, #65528, #4837, #82670, #190872, #144354, #52348, #98837, #189885, #51360, #6833, #160532, #145351, #50380, #127188, #111039, #18057, #114004, #33217, #126211, #113021, #68512, #94877, #5841, #187907, #143349, #175702, #156557, #188899, #20024, #49376, #172725, #112040, #35197, #174713, #34207, #96850, #130166, #158535, #81666, #95870, #36177, #157553, #80693, #159518, #67517, #149364, #87679, #71518, #193882, #147366, #163537, #42198, #194876, #23023, #41194, #162522, #84668, #101853, #26034, #10860, #24025, #192875, #56350, #177714, #146347, #11875, #102856, #72529, #133185, #134206, #118032, #164542, #27037, #165540, #73538, #116025, #70522, #7834, #195893, #69520, #86680, #57368, #179723, #115024, #131185, #119041, #25037, #99846, #54353, #85679, #8855, #180723, #39182, #40174, #135211, #132191, #148364, #100840, #9859, #53345, #55347, #117017, #103859, #88683, #150378, #176717, #178713, #38190, #161530, #185668, #138170, #166541, #184674, #105840, #28039, #45176, #169495, #30994, #167528, #136187, #199851, #120999, #89681, #155330, #46157, #15823, #76493, #154333, #14831, #107812, #170497, #108818, #16818, #59329, #13830, #151366, #92643, #12857, #30003, #77484, #61317, #58349, #74522, #139153, #29023, #122988, #106830, #197862, #47159, #631, #62301, #196883, #78469, #90663, #123971, #31987, #120017, #93645, #181702, #43183, #104852, #182697, #44182, #152345, #75496, #137170, #198858, #60324, #121999, #183689, #168505, #91641, #153330, #52120, #172489, #96617, #1635, #171498, #140143, #113776, #21790, #3618, #109815, #159284, #32987, #49149, #33977, #34965, #51129, #20781, #112789, #82436, #128943, #158306, #19794, #36944, #190644, #175472, #80460, #95633, #141147, #48157, #144124, #63312, #94640, #81435, #98606, #124991, #35950, #156321, #173492, #5605, #186687, #18816, #142134, #157320, #2637, #17821, #67285, #79479, #64313, #143121, #160300, #125981, #97596, #187679, #4601, #110807, #65297, #126956, #50144, #188665, #111804, #66293, #127952, #189656, #174483, #70297, #103636, #100615, #193650, #69287, #55122, #165313, #114790, #54126, #86456, #179496, #117803, #101620, #23797, #177489, #116791, #72294, #24807, #53112, #71299, #192643, #176483, #131965, #56121, #40961, #115799, #22793, #148141, #7601, #37959, #41969, #132962, #102633, #163309, #164318, #9632, #194651, #57135, #195664, #83441, #146117, #162297, #99617, #25811, #161297, #178483, #87457, #149143, #145119, #84439, #10634, #38958, #133973, #39949, #130953, #118811, #180497, #6603, #68282, #129933, #85447, #191632, #147137, #8625, #62068, #137930, #15589, #26807, #45923, #123733, #119796, #106596, #91404, #135963, #199614, #196658, #14596, #59100, #44940, #154095, #138915, #120765, #183455, #88447, #58127, #150142, #396, #108582, #90432, #181480, #107577, #42959, #197633, #182466, #121762, #61080, #169255, #122753, #30762, #77247, #168272, #29769, #185432, #46922, #11644, #60094, #92409, #153092, #73310, #104622, #184443, #43947, #76252, #75269, #166311, #134981, #27808, #89449, #151138, #12629, #105609, #74294, #167297, #28793, #152118, #13601, #136939, #198628, #189418, #67048, #63070, #49896, #34722, #79235, #81202, #139901, #158067, #2392, #188419, #97361, #82190, #64071, #126715, #31753, #1389, #170259, #143883, #51879, #33731, #124749, #50893, #186445, #140906, #125741, #65058, #142883, #112551, #4365, #174246, #159047, #111563, #173247, #128706, #20541, #5364, #110563, #187441, #171258, #78230, #35714, #93402, #47921, #96380 ),
 ( #19558, #109575, #157078, #190403, #48909, #80221, #156078, #141892, #155088, #32745, #172244, #66048, #127716, #16582, #94397, #95392, #18574, #3383, #17574, #54878, #83204, #101365, #22549, #144879, #162054, #86210, #147900, #84195, #52867, #116552, #37709, #6361, #72043, #163054, #132718, #193403, #71052, #131721, #24561, #87214, #25570, #133717, #176238, #130708, #68041, #9386, #129693, #23550, #102383, #178241, #191390, #194406, #145875, #114538, #85198, #55876, #117549, #7358, #99371, #39702, #161054, #69043, #195409, #179248, #40714, #164071, #148896, #10386, #113538, #175232, #36697, #98358, #192402, #53884, #115559, #160057, #177246, #146886, #21544, #38718, #100376, #8378, #70053, #27561, #59849, #105363, #73060, #107331, #60833, #152849, #56887, #138672, #150894, #121516, #137684, #15344, #92159, #168030, #45680, #118561, #76009, #153846, #149884, #136690, #183211, #166060, #29527, #26557, #44692, #89201, #75025, #184198, #169004, #12388, #13361, #180251, #88200, #41721, #30508, #103385, #120524, #11390, #199369, #134732, #74050, #135721, #151871, #91160, #122508, #14343, #77000, #165063, #198372, #106346, #196414, #57884, #119556, #197392, #58857, #181239, #42715, #104377, #182217, #43701, #167050, #28551, #90188, #96144, #93158, #33492, #65805, #81943, #78985, #110323, #46674, #16340, #32502, #94154, #64822, #154843, #187200, #20295, #17330, #172004, #186197, #95150, #152, #31505, #171011, #3148, #157833, #34486, #18334, #140660, #155833, #61821, #77989, #19324, #2152, #126484, #48671, #139656, #50652, #4126, #80971, #123491, #185184, #63830, #188182, #142647, #158806, #35474, #111318, #189179, #108334, #127473, #97123, #1144, #79989, #49654, #109329, #173007, #170014, #112313, #125502, #141657, #174003, #62818, #156839, #124502, #47678, #174990, #143634, #55632, #25327, #7117, #113299, #162808, #36454, #52631, #37467, #38474, #54630, #24317, #116305, #85966, #132479, #100131, #161812, #40469, #194168, #117305, #83957, #99128, #144638, #51635, #147655, #5118, #98112, #23307, #179001, #66800, #39461, #159809, #177005, #9143, #128463, #22306, #53636, #190159, #21304, #175997, #160818, #8125, #82961, #130458, #163826, #145637, #115313, #129459, #84951, #6121, #67804, #114295, #146633, #101122, #177994, #69803, #68799, #192155, #131471, #102141, #193158, #191158, #70810, #196176, #56645, #135488, #59609, #121282, #57648, #26320, #89959, #11146, #180011, #45445, #74796, #106113, #166819, #44459, #105133, #136458, #60595, #199128, #107098, #149648, #104139, #118318, #182975, #41478, #120290, #167797, #28320, #181000, #151639, #29297, #168768, #122270, #198139, #75771, #86969, #90927, #183958, #103142, #13134, #152613, #119314, #14103, #164824, #137449, #42476, #148656, #10144, #71804, #165821, #43465, #133473, #87960, #195164, #72820, #134489, #150655, #27318, #88965, #12153, #73818, #197158, #181983, #58623, #113807, #144153, #175502, #21821, #127984, #189687, #129963, #83473, #145150, #173523, #188696, #34009, #141179, #52150, #91916, #2669, #51160, #6634, #153609, #128975, #126015, #66323, #98636, #114821, #111834, #143152, #76766, #49182, #65329, #126989, #97627, #187710, #19825, #53142, #50177, #4633, #18848, #112820, #30271, #64346, #3651, #35980, #190674, #67315, #174513, #34994, #96648, #159316, #68312, #20811, #110840, #82467, #142167, #172524, #81466, #5638, #36975, #158336, #95666, #160331, #157353, #80493, #191663, #15105, #195693, #56150, #134002, #194681, #25842, #150173, #88476, #196689, #38989, #193681, #7633, #72326, #146146, #9661, #57164, #117832, #37990, #192674, #10663, #147166, #179525, #24835, #54157, #26836, #180526, #118843, #176513, #58158, #69317, #99646, #11673, #161329, #39978, #130983, #41999, #115830, #85477, #70328, #71328, #87486, #103665, #149174, #165343, #73339, #132990, #40994, #135012, #22822, #84468, #116821, #131995, #177519, #100645, #162326 ) ),
 .UNSPECIFIED., .T., .F., .F. ) 
 B_SPLINE_SURFACE_WITH_KNOTS ( ( 4, 3, 4 ),
 ( 3, 2, 2, 2, 2, 2, 2, 2, 2, 2, 2, 2, 2, 2, 2, 2, 2, 2, 2, 2, 2, 2, 2, 2, 2, 2, 2, 2, 2, 2, 2, 2, 2, 2, 2, 2, 2, 2, 2, 2, 2, 2, 2, 2, 2, 2, 2, 2, 2, 2, 2, 2, 2, 2, 2, 2, 2, 2, 2, 2, 2, 2, 2, 2, 2, 2, 2, 2, 2, 2, 2, 2, 2, 2, 2, 2, 2, 2, 2, 2, 2, 2, 2, 2, 2, 2, 2, 2, 2, 2, 2, 2, 2, 2, 2, 2, 2, 2, 2, 2, 2, 2, 2, 2, 2, 2, 2, 2, 2, 2, 2, 2, 2, 2, 2, 2, 2, 2, 2, 2, 2, 2, 2, 2, 2, 2, 2, 2, 2, 2, 2, 2, 2, 2, 2, 2, 2, 2, 2, 2, 2, 2, 2, 2, 2, 2, 2, 2, 2, 2, 2, 2, 2, 2, 2, 2, 2, 2, 2, 2, 2, 2, 2, 2, 2, 2, 2, 2, 2, 2, 2, 2, 2, 2, 2, 2, 2, 2, 2, 2, 2, 2, 2, 2, 2, 2, 2, 2, 2, 2, 2, 2, 2, 2, 2, 2, 2, 2, 2, 2, 2, 2, 2, 2, 2, 2, 2, 2, 2, 2, 2, 2, 2, 2, 2, 2, 2, 2, 2, 2, 2, 2, 2, 2, 2, 2, 2, 2, 3 ),
 ( 0.000000000000000000, 0.5000000000000000000, 1.000000000000000000 ),
 ( 0.000000000000000000, 0.004385964912280701511, 0.008771929824561403022, 0.01315789473684210453, 0.01754385964912280604, 0.02192982456140350755, 0.02631578947368420907, 0.03070175438596491058, 0.03508771929824561209, 0.03947368421052631360, 0.04385964912280701511, 0.04824561403508771662, 0.05263157894736841813, 0.05701754385964911964, 0.06140350877192982115, 0.06578947368421052266, 0.07017543859649122417, 0.07456140350877192569, 0.07894736842105262720, 0.08333333333333332871, 0.08771929824561403022, 0.09210526315789473173, 0.09649122807017543324, 0.1008771929824561348, 0.1052631578947368363, 0.1096491228070175378, 0.1140350877192982393, 0.1184210526315789408, 0.1228070175438596423, 0.1271929824561403577, 0.1315789473684210453, 0.1359649122807017607, 0.1403508771929824483, 0.1447368421052631637, 0.1491228070175438514, 0.1535087719298245668, 0.1578947368421052544, 0.1622807017543859698, 0.1666666666666666574, 0.1710526315789473728, 0.1754385964912280604, 0.1798245614035087758, 0.1842105263157894635, 0.1885964912280701788, 0.1929824561403508665, 0.1973684210526315819, 0.2017543859649122695, 0.2061403508771929849, 0.2105263157894736725, 0.2149122807017543879, 0.2192982456140350755, 0.2236842105263157909, 0.2280701754385964786, 0.2324561403508771940, 0.2368421052631578816, 0.2412280701754385970, 0.2456140350877192846, 0.2500000000000000000, 0.2543859649122807154, 0.2587719298245614308, 0.2631578947368420907, 0.2675438596491228060, 0.2719298245614035214, 0.2763157894736842368, 0.2807017543859648967, 0.2850877192982456121, 0.2894736842105263275, 0.2938596491228070429, 0.2982456140350877027, 0.3026315789473684181, 0.3070175438596491335, 0.3114035087719298489, 0.3157894736842105088, 0.3201754385964912242, 0.3245614035087719396, 0.3289473684210526550, 0.3333333333333333148, 0.3377192982456140302, 0.3421052631578947456, 0.3464912280701754610, 0.3508771929824561209, 0.3552631578947368363, 0.3596491228070175517, 0.3640350877192982670, 0.3684210526315789269, 0.3728070175438596423, 0.3771929824561403577, 0.3815789473684210731, 0.3859649122807017330, 0.3903508771929824483, 0.3947368421052631637, 0.3991228070175438791, 0.4035087719298245390, 0.4078947368421052544, 0.4122807017543859698, 0.4166666666666666852, 0.4210526315789473450, 0.4254385964912280604, 0.4298245614035087758, 0.4342105263157894912, 0.4385964912280701511, 0.4429824561403508665, 0.4473684210526315819, 0.4517543859649122973, 0.4561403508771929571, 0.4605263157894736725, 0.4649122807017543879, 0.4692982456140351033, 0.4736842105263157632, 0.4780701754385964786, 0.4824561403508771940, 0.4868421052631579093, 0.4912280701754385692, 0.4956140350877192846, 0.5000000000000000000, 0.5043859649122807154, 0.5087719298245614308, 0.5131578947368421462, 0.5175438596491228616, 0.5219298245614034659, 0.5263157894736841813, 0.5307017543859648967, 0.5350877192982456121, 0.5394736842105263275, 0.5438596491228070429, 0.5482456140350877583, 0.5526315789473684736, 0.5570175438596490780, 0.5614035087719297934, 0.5657894736842105088, 0.5701754385964912242, 0.5745614035087719396, 0.5789473684210526550, 0.5833333333333333703, 0.5877192982456140857, 0.5921052631578946901, 0.5964912280701754055, 0.6008771929824561209, 0.6052631578947368363, 0.6096491228070175517, 0.6140350877192982670, 0.6184210526315789824, 0.6228070175438596978, 0.6271929824561403022, 0.6315789473684210176, 0.6359649122807017330, 0.6403508771929824483, 0.6447368421052631637, 0.6491228070175438791, 0.6535087719298245945, 0.6578947368421053099, 0.6622807017543859143, 0.6666666666666666297, 0.6710526315789473450, 0.6754385964912280604, 0.6798245614035087758, 0.6842105263157894912, 0.6885964912280702066, 0.6929824561403509220, 0.6973684210526315264, 0.7017543859649122417, 0.7061403508771929571, 0.7105263157894736725, 0.7149122807017543879, 0.7192982456140351033, 0.7236842105263158187, 0.7280701754385965341, 0.7324561403508771384, 0.7368421052631578538, 0.7412280701754385692, 0.7456140350877192846, 0.7500000000000000000, 0.7543859649122807154, 0.7587719298245614308, 0.7631578947368421462, 0.7675438596491228616, 0.7719298245614034659, 0.7763157894736841813, 0.7807017543859648967, 0.7850877192982456121, 0.7894736842105263275, 0.7938596491228070429, 0.7982456140350877583, 0.8026315789473684736, 0.8070175438596490780, 0.8114035087719297934, 0.8157894736842105088, 0.8201754385964912242, 0.8245614035087719396, 0.8289473684210526550, 0.8333333333333333703, 0.8377192982456140857, 0.8421052631578946901, 0.8464912280701754055, 0.8508771929824561209, 0.8552631578947368363, 0.8596491228070175517, 0.8640350877192982670, 0.8684210526315789824, 0.8728070175438596978, 0.8771929824561403022, 0.8815789473684210176, 0.8859649122807017330, 0.8903508771929824483, 0.8947368421052631637, 0.8991228070175438791, 0.9035087719298245945, 0.9078947368421053099, 0.9122807017543859143, 0.9166666666666666297, 0.9210526315789473450, 0.9254385964912280604, 0.9298245614035087758, 0.9342105263157894912, 0.9385964912280702066, 0.9429824561403509220, 0.9473684210526315264, 0.9517543859649122417, 0.9561403508771929571, 0.9605263157894736725, 0.9649122807017543879, 0.9692982456140351033, 0.9736842105263158187, 0.9780701754385965341, 0.9824561403508771384, 0.9868421052631578538, 0.9912280701754385692, 0.9956140350877192846, 1.000000000000000000 ),
 .UNSPECIFIED. ) 
 GEOMETRIC_REPRESENTATION_ITEM ( )  RATIONAL_B_SPLINE_SURFACE ( (
 ( 1.000000000000000000, 0.9659258262890683122, 1.000000000000000000, 0.9659258262890683122, 1.000000000000000000, 0.9659258262890683122, 1.000000000000000000, 0.9659258262890683122, 1.000000000000000000, 0.9659258262890683122, 1.000000000000000000, 0.9659258262890683122, 1.000000000000000000, 0.9659258262890683122, 1.000000000000000000, 0.9659258262890683122, 1.000000000000000000, 0.9659258262890683122, 1.000000000000000000, 0.9659258262890683122, 1.000000000000000000, 0.9659258262890683122, 1.000000000000000000, 0.9659258262890683122, 1.000000000000000000, 0.9659258262890683122, 1.000000000000000000, 0.9659258262890683122, 1.000000000000000000, 0.9659258262890683122, 1.000000000000000000, 0.9659258262890683122, 1.000000000000000000, 0.9659258262890683122, 1.000000000000000000, 0.9659258262890683122, 1.000000000000000000, 0.9659258262890683122, 1.000000000000000000, 0.9659258262890683122, 1.000000000000000000, 0.9659258262890683122, 1.000000000000000000, 0.9659258262890683122, 1.000000000000000000, 0.9659258262890683122, 1.000000000000000000, 0.9659258262890683122, 1.000000000000000000, 0.9659258262890683122, 1.000000000000000000, 0.9659258262890683122, 1.000000000000000000, 0.9659258262890683122, 1.000000000000000000, 0.9659258262890683122, 1.000000000000000000, 0.9659258262890683122, 1.000000000000000000, 0.9659258262890683122, 1.000000000000000000, 0.9659258262890683122, 1.000000000000000000, 0.9659258262890683122, 1.000000000000000000, 0.9659258262890683122, 1.000000000000000000, 0.9659258262890683122, 1.000000000000000000, 0.9659258262890683122, 1.000000000000000000, 0.9659258262890683122, 1.000000000000000000, 0.9659258262890683122, 1.000000000000000000, 0.9659258262890683122, 1.000000000000000000, 0.9659258262890683122, 1.000000000000000000, 0.9659258262890683122, 1.000000000000000000, 0.9659258262890683122, 1.000000000000000000, 0.9659258262890683122, 1.000000000000000000, 0.9659258262890683122, 1.000000000000000000, 0.9659258262890683122, 1.000000000000000000, 0.9659258262890683122, 1.000000000000000000, 0.9659258262890683122, 1.000000000000000000, 0.9659258262890683122, 1.000000000000000000, 0.9659258262890683122, 1.000000000000000000, 0.9659258262890683122, 1.000000000000000000, 0.9659258262890683122, 1.000000000000000000, 0.9659258262890683122, 1.000000000000000000, 0.9659258262890683122, 1.000000000000000000, 0.9659258262890683122, 1.000000000000000000, 0.9659258262890683122, 1.000000000000000000, 0.9659258262890683122, 1.000000000000000000, 0.9659258262890683122, 1.000000000000000000, 0.9659258262890683122, 1.000000000000000000, 0.9659258262890683122, 1.000000000000000000, 0.9659258262890683122, 1.000000000000000000, 0.9659258262890683122, 1.000000000000000000, 0.9659258262890683122, 1.000000000000000000, 0.9659258262890683122, 1.000000000000000000, 0.9659258262890683122, 1.000000000000000000, 0.9659258262890683122, 1.000000000000000000, 0.9659258262890683122, 1.000000000000000000, 0.9659258262890683122, 1.000000000000000000, 0.9659258262890683122, 1.000000000000000000, 0.9659258262890683122, 1.000000000000000000, 0.9659258262890683122, 1.000000000000000000, 0.9659258262890683122, 1.000000000000000000, 0.9659258262890683122, 1.000000000000000000, 0.9659258262890683122, 1.000000000000000000, 0.9659258262890683122, 1.000000000000000000, 0.9659258262890683122, 1.000000000000000000, 0.9659258262890683122, 1.000000000000000000, 0.9659258262890683122, 1.000000000000000000, 0.9659258262890683122, 1.000000000000000000, 0.9659258262890683122, 1.000000000000000000, 0.9659258262890683122, 1.000000000000000000, 0.9659258262890683122, 1.000000000000000000, 0.9659258262890683122, 1.000000000000000000, 0.9659258262890683122, 1.000000000000000000, 0.9659258262890683122, 1.000000000000000000, 0.9659258262890683122, 1.000000000000000000, 0.9659258262890683122, 1.000000000000000000, 0.9659258262890683122, 1.000000000000000000, 0.9659258262890683122, 1.000000000000000000, 0.9659258262890683122, 1.000000000000000000, 0.9659258262890683122, 1.000000000000000000, 0.9659258262890683122, 1.000000000000000000, 0.9659258262890683122, 1.000000000000000000, 0.9659258262890683122, 1.000000000000000000, 0.9659258262890683122, 1.000000000000000000, 0.9659258262890683122, 1.000000000000000000, 0.9659258262890683122, 1.000000000000000000, 0.9659258262890683122, 1.000000000000000000, 0.9659258262890683122, 1.000000000000000000, 0.9659258262890683122, 1.000000000000000000, 0.9659258262890683122, 1.000000000000000000, 0.9659258262890683122, 1.000000000000000000, 0.9659258262890683122, 1.000000000000000000, 0.9659258262890683122, 1.000000000000000000, 0.9659258262890683122, 1.000000000000000000, 0.9659258262890683122, 1.000000000000000000, 0.9659258262890683122, 1.000000000000000000, 0.9659258262890683122, 1.000000000000000000, 0.9659258262890683122, 1.000000000000000000, 0.9659258262890683122, 1.000000000000000000, 0.9659258262890683122, 1.000000000000000000, 0.9659258262890683122, 1.000000000000000000, 0.9659258262890683122, 1.000000000000000000, 0.9659258262890683122, 1.000000000000000000, 0.9659258262890683122, 1.000000000000000000, 0.9659258262890683122, 1.000000000000000000, 0.9659258262890683122, 1.000000000000000000, 0.9659258262890683122, 1.000000000000000000, 0.9659258262890683122, 1.000000000000000000, 0.9659258262890683122, 1.000000000000000000, 0.9659258262890683122, 1.000000000000000000, 0.9659258262890683122, 1.000000000000000000, 0.9659258262890683122, 1.000000000000000000, 0.9659258262890683122, 1.000000000000000000, 0.9659258262890683122, 1.000000000000000000, 0.9659258262890683122, 1.000000000000000000, 0.9659258262890683122, 1.000000000000000000, 0.9659258262890683122, 1.000000000000000000, 0.9659258262890683122, 1.000000000000000000, 0.9659258262890683122, 1.000000000000000000, 0.9659258262890683122, 1.000000000000000000, 0.9659258262890683122, 1.000000000000000000, 0.9659258262890683122, 1.000000000000000000, 0.9659258262890683122, 1.000000000000000000, 0.9659258262890683122, 1.000000000000000000, 0.9659258262890683122, 1.000000000000000000, 0.9659258262890683122, 1.000000000000000000, 0.9659258262890683122, 1.000000000000000000, 0.9659258262890683122, 1.000000000000000000, 0.9659258262890683122, 1.000000000000000000, 0.9659258262890683122, 1.000000000000000000, 0.9659258262890683122, 1.000000000000000000, 0.9659258262890683122, 1.000000000000000000, 0.9659258262890683122, 1.000000000000000000, 0.9659258262890683122, 1.000000000000000000, 0.9659258262890683122, 1.000000000000000000, 0.9659258262890683122, 1.000000000000000000, 0.9659258262890683122, 1.000000000000000000, 0.9659258262890683122, 1.000000000000000000, 0.9659258262890683122, 1.000000000000000000, 0.9659258262890683122, 1.000000000000000000, 0.9659258262890683122, 1.000000000000000000, 0.9659258262890683122, 1.000000000000000000, 0.9659258262890683122, 1.000000000000000000, 0.9659258262890683122, 1.000000000000000000, 0.9659258262890683122, 1.000000000000000000, 0.9659258262890683122, 1.000000000000000000, 0.9659258262890683122, 1.000000000000000000, 0.9659258262890683122, 1.000000000000000000, 0.9659258262890683122, 1.000000000000000000, 0.9659258262890683122, 1.000000000000000000, 0.9659258262890683122, 1.000000000000000000, 0.9659258262890683122, 1.000000000000000000, 0.9659258262890683122, 1.000000000000000000, 0.9659258262890683122, 1.000000000000000000, 0.9659258262890683122, 1.000000000000000000, 0.9659258262890683122, 1.000000000000000000, 0.9659258262890683122, 1.000000000000000000, 0.9659258262890683122, 1.000000000000000000, 0.9659258262890683122, 1.000000000000000000, 0.9659258262890683122, 1.000000000000000000, 0.9659258262890683122, 1.000000000000000000, 0.9659258262890683122, 1.000000000000000000, 0.9659258262890683122, 1.000000000000000000, 0.9659258262890683122, 1.000000000000000000, 0.9659258262890683122, 1.000000000000000000, 0.9659258262890683122, 1.000000000000000000, 0.9659258262890683122, 1.000000000000000000, 0.9659258262890683122, 1.000000000000000000, 0.9659258262890683122, 1.000000000000000000, 0.9659258262890683122, 1.000000000000000000, 0.9659258262890683122, 1.000000000000000000, 0.9659258262890683122, 1.000000000000000000, 0.9659258262890683122, 1.000000000000000000, 0.9659258262890683122, 1.000000000000000000, 0.9659258262890683122, 1.000000000000000000, 0.9659258262890683122, 1.000000000000000000, 0.9659258262890683122, 1.000000000000000000, 0.9659258262890683122, 1.000000000000000000, 0.9659258262890683122, 1.000000000000000000, 0.9659258262890683122, 1.000000000000000000, 0.9659258262890683122, 1.000000000000000000, 0.9659258262890683122, 1.000000000000000000, 0.9659258262890683122, 1.000000000000000000, 0.9659258262890683122, 1.000000000000000000, 0.9659258262890683122, 1.000000000000000000, 0.9659258262890683122, 1.000000000000000000, 0.9659258262890683122, 1.000000000000000000, 0.9659258262890683122, 1.000000000000000000, 0.9659258262890683122, 1.000000000000000000, 0.9659258262890683122, 1.000000000000000000, 0.9659258262890683122, 1.000000000000000000, 0.9659258262890683122, 1.000000000000000000, 0.9659258262890683122, 1.000000000000000000, 0.9659258262890683122, 1.000000000000000000, 0.9659258262890683122, 1.000000000000000000, 0.9659258262890683122, 1.000000000000000000, 0.9659258262890683122, 1.000000000000000000, 0.9659258262890683122, 1.000000000000000000, 0.9659258262890683122, 1.000000000000000000, 0.9659258262890683122, 1.000000000000000000, 0.9659258262890683122, 1.000000000000000000, 0.9659258262890683122, 1.000000000000000000, 0.9659258262890683122, 1.000000000000000000, 0.9659258262890683122, 1.000000000000000000, 0.9659258262890683122, 1.000000000000000000, 0.9659258262890683122, 1.000000000000000000, 0.9659258262890683122, 1.000000000000000000, 0.9659258262890683122, 1.000000000000000000, 0.9659258262890683122, 1.000000000000000000, 0.9659258262890683122, 1.000000000000000000, 0.9659258262890683122, 1.000000000000000000, 0.9659258262890683122, 1.000000000000000000, 0.9659258262890683122, 1.000000000000000000, 0.9659258262890683122, 1.000000000000000000, 0.9659258262890683122, 1.000000000000000000, 0.9659258262890683122, 1.000000000000000000, 0.9659258262890683122, 1.000000000000000000, 0.9659258262890683122, 1.000000000000000000, 0.9659258262890683122, 1.000000000000000000),
 ( 0.3333333333333333703, 0.3219752754296894559, 0.3333333333333333703, 0.3219752754296894559, 0.3333333333333333703, 0.3219752754296894559, 0.3333333333333333703, 0.3219752754296894559, 0.3333333333333333703, 0.3219752754296894559, 0.3333333333333333703, 0.3219752754296894559, 0.3333333333333333703, 0.3219752754296894559, 0.3333333333333333703, 0.3219752754296894559, 0.3333333333333333703, 0.3219752754296894559, 0.3333333333333333703, 0.3219752754296894559, 0.3333333333333333703, 0.3219752754296894559, 0.3333333333333333703, 0.3219752754296894559, 0.3333333333333333703, 0.3219752754296894559, 0.3333333333333333703, 0.3219752754296894559, 0.3333333333333333703, 0.3219752754296894559, 0.3333333333333333703, 0.3219752754296894559, 0.3333333333333333703, 0.3219752754296894559, 0.3333333333333333703, 0.3219752754296894559, 0.3333333333333333703, 0.3219752754296894559, 0.3333333333333333703, 0.3219752754296894559, 0.3333333333333333703, 0.3219752754296894559, 0.3333333333333333703, 0.3219752754296894559, 0.3333333333333333703, 0.3219752754296894559, 0.3333333333333333703, 0.3219752754296894559, 0.3333333333333333703, 0.3219752754296894559, 0.3333333333333333703, 0.3219752754296894559, 0.3333333333333333703, 0.3219752754296894559, 0.3333333333333333703, 0.3219752754296894559, 0.3333333333333333703, 0.3219752754296894559, 0.3333333333333333703, 0.3219752754296894559, 0.3333333333333333703, 0.3219752754296894559, 0.3333333333333333703, 0.3219752754296894559, 0.3333333333333333703, 0.3219752754296894559, 0.3333333333333333703, 0.3219752754296894559, 0.3333333333333333703, 0.3219752754296894559, 0.3333333333333333703, 0.3219752754296894559, 0.3333333333333333703, 0.3219752754296894559, 0.3333333333333333703, 0.3219752754296894559, 0.3333333333333333703, 0.3219752754296894559, 0.3333333333333333703, 0.3219752754296894559, 0.3333333333333333703, 0.3219752754296894559, 0.3333333333333333703, 0.3219752754296894559, 0.3333333333333333703, 0.3219752754296894559, 0.3333333333333333703, 0.3219752754296894559, 0.3333333333333333703, 0.3219752754296894559, 0.3333333333333333703, 0.3219752754296894559, 0.3333333333333333703, 0.3219752754296894559, 0.3333333333333333703, 0.3219752754296894559, 0.3333333333333333703, 0.3219752754296894559, 0.3333333333333333703, 0.3219752754296894559, 0.3333333333333333703, 0.3219752754296894559, 0.3333333333333333703, 0.3219752754296894559, 0.3333333333333333703, 0.3219752754296894559, 0.3333333333333333703, 0.3219752754296894559, 0.3333333333333333703, 0.3219752754296894559, 0.3333333333333333703, 0.3219752754296894559, 0.3333333333333333703, 0.3219752754296894559, 0.3333333333333333703, 0.3219752754296894559, 0.3333333333333333703, 0.3219752754296894559, 0.3333333333333333703, 0.3219752754296894559, 0.3333333333333333703, 0.3219752754296894559, 0.3333333333333333703, 0.3219752754296894559, 0.3333333333333333703, 0.3219752754296894559, 0.3333333333333333703, 0.3219752754296894559, 0.3333333333333333703, 0.3219752754296894559, 0.3333333333333333703, 0.3219752754296894559, 0.3333333333333333703, 0.3219752754296894559, 0.3333333333333333703, 0.3219752754296894559, 0.3333333333333333703, 0.3219752754296894559, 0.3333333333333333703, 0.3219752754296894559, 0.3333333333333333703, 0.3219752754296894559, 0.3333333333333333703, 0.3219752754296894559, 0.3333333333333333703, 0.3219752754296894559, 0.3333333333333333703, 0.3219752754296894559, 0.3333333333333333703, 0.3219752754296894559, 0.3333333333333333703, 0.3219752754296894559, 0.3333333333333333703, 0.3219752754296894559, 0.3333333333333333703, 0.3219752754296894559, 0.3333333333333333703, 0.3219752754296894559, 0.3333333333333333703, 0.3219752754296894559, 0.3333333333333333703, 0.3219752754296894559, 0.3333333333333333703, 0.3219752754296894559, 0.3333333333333333703, 0.3219752754296894559, 0.3333333333333333703, 0.3219752754296894559, 0.3333333333333333703, 0.3219752754296894559, 0.3333333333333333703, 0.3219752754296894559, 0.3333333333333333703, 0.3219752754296894559, 0.3333333333333333703, 0.3219752754296894559, 0.3333333333333333703, 0.3219752754296894559, 0.3333333333333333703, 0.3219752754296894559, 0.3333333333333333703, 0.3219752754296894559, 0.3333333333333333703, 0.3219752754296894559, 0.3333333333333333703, 0.3219752754296894559, 0.3333333333333333703, 0.3219752754296894559, 0.3333333333333333703, 0.3219752754296894559, 0.3333333333333333703, 0.3219752754296894559, 0.3333333333333333703, 0.3219752754296894559, 0.3333333333333333703, 0.3219752754296894559, 0.3333333333333333703, 0.3219752754296894559, 0.3333333333333333703, 0.3219752754296894559, 0.3333333333333333703, 0.3219752754296894559, 0.3333333333333333703, 0.3219752754296894559, 0.3333333333333333703, 0.3219752754296894559, 0.3333333333333333703, 0.3219752754296894559, 0.3333333333333333703, 0.3219752754296894559, 0.3333333333333333703, 0.3219752754296894559, 0.3333333333333333703, 0.3219752754296894559, 0.3333333333333333703, 0.3219752754296894559, 0.3333333333333333703, 0.3219752754296894559, 0.3333333333333333703, 0.3219752754296894559, 0.3333333333333333703, 0.3219752754296894559, 0.3333333333333333703, 0.3219752754296894559, 0.3333333333333333703, 0.3219752754296894559, 0.3333333333333333703, 0.3219752754296894559, 0.3333333333333333703, 0.3219752754296894559, 0.3333333333333333703, 0.3219752754296894559, 0.3333333333333333703, 0.3219752754296894559, 0.3333333333333333703, 0.3219752754296894559, 0.3333333333333333703, 0.3219752754296894559, 0.3333333333333333703, 0.3219752754296894559, 0.3333333333333333703, 0.3219752754296894559, 0.3333333333333333703, 0.3219752754296894559, 0.3333333333333333703, 0.3219752754296894559, 0.3333333333333333703, 0.3219752754296894559, 0.3333333333333333703, 0.3219752754296894559, 0.3333333333333333703, 0.3219752754296894559, 0.3333333333333333703, 0.3219752754296894559, 0.3333333333333333703, 0.3219752754296894559, 0.3333333333333333703, 0.3219752754296894559, 0.3333333333333333703, 0.3219752754296894559, 0.3333333333333333703, 0.3219752754296894559, 0.3333333333333333703, 0.3219752754296894559, 0.3333333333333333703, 0.3219752754296894559, 0.3333333333333333703, 0.3219752754296894559, 0.3333333333333333703, 0.3219752754296894559, 0.3333333333333333703, 0.3219752754296894559, 0.3333333333333333703, 0.3219752754296894559, 0.3333333333333333703, 0.3219752754296894559, 0.3333333333333333703, 0.3219752754296894559, 0.3333333333333333703, 0.3219752754296894559, 0.3333333333333333703, 0.3219752754296894559, 0.3333333333333333703, 0.3219752754296894559, 0.3333333333333333703, 0.3219752754296894559, 0.3333333333333333703, 0.3219752754296894559, 0.3333333333333333703, 0.3219752754296894559, 0.3333333333333333703, 0.3219752754296894559, 0.3333333333333333703, 0.3219752754296894559, 0.3333333333333333703, 0.3219752754296894559, 0.3333333333333333703, 0.3219752754296894559, 0.3333333333333333703, 0.3219752754296894559, 0.3333333333333333703, 0.3219752754296894559, 0.3333333333333333703, 0.3219752754296894559, 0.3333333333333333703, 0.3219752754296894559, 0.3333333333333333703, 0.3219752754296894559, 0.3333333333333333703, 0.3219752754296894559, 0.3333333333333333703, 0.3219752754296894559, 0.3333333333333333703, 0.3219752754296894559, 0.3333333333333333703, 0.3219752754296894559, 0.3333333333333333703, 0.3219752754296894559, 0.3333333333333333703, 0.3219752754296894559, 0.3333333333333333703, 0.3219752754296894559, 0.3333333333333333703, 0.3219752754296894559, 0.3333333333333333703, 0.3219752754296894559, 0.3333333333333333703, 0.3219752754296894559, 0.3333333333333333703, 0.3219752754296894559, 0.3333333333333333703, 0.3219752754296894559, 0.3333333333333333703, 0.3219752754296894559, 0.3333333333333333703, 0.3219752754296894559, 0.3333333333333333703, 0.3219752754296894559, 0.3333333333333333703, 0.3219752754296894559, 0.3333333333333333703, 0.3219752754296894559, 0.3333333333333333703, 0.3219752754296894559, 0.3333333333333333703, 0.3219752754296894559, 0.3333333333333333703, 0.3219752754296894559, 0.3333333333333333703, 0.3219752754296894559, 0.3333333333333333703, 0.3219752754296894559, 0.3333333333333333703, 0.3219752754296894559, 0.3333333333333333703, 0.3219752754296894559, 0.3333333333333333703, 0.3219752754296894559, 0.3333333333333333703, 0.3219752754296894559, 0.3333333333333333703, 0.3219752754296894559, 0.3333333333333333703, 0.3219752754296894559, 0.3333333333333333703, 0.3219752754296894559, 0.3333333333333333703, 0.3219752754296894559, 0.3333333333333333703, 0.3219752754296894559, 0.3333333333333333703, 0.3219752754296894559, 0.3333333333333333703, 0.3219752754296894559, 0.3333333333333333703, 0.3219752754296894559, 0.3333333333333333703, 0.3219752754296894559, 0.3333333333333333703, 0.3219752754296894559, 0.3333333333333333703, 0.3219752754296894559, 0.3333333333333333703, 0.3219752754296894559, 0.3333333333333333703, 0.3219752754296894559, 0.3333333333333333703, 0.3219752754296894559, 0.3333333333333333703, 0.3219752754296894559, 0.3333333333333333703, 0.3219752754296894559, 0.3333333333333333703, 0.3219752754296894559, 0.3333333333333333703, 0.3219752754296894559, 0.3333333333333333703, 0.3219752754296894559, 0.3333333333333333703, 0.3219752754296894559, 0.3333333333333333703, 0.3219752754296894559, 0.3333333333333333703, 0.3219752754296894559, 0.3333333333333333703, 0.3219752754296894559, 0.3333333333333333703, 0.3219752754296894559, 0.3333333333333333703, 0.3219752754296894559, 0.3333333333333333703, 0.3219752754296894559, 0.3333333333333333703, 0.3219752754296894559, 0.3333333333333333703, 0.3219752754296894559, 0.3333333333333333703, 0.3219752754296894559, 0.3333333333333333703, 0.3219752754296894559, 0.3333333333333333703, 0.3219752754296894559, 0.3333333333333333703, 0.3219752754296894559, 0.3333333333333333703, 0.3219752754296894559, 0.3333333333333333703, 0.3219752754296894559, 0.3333333333333333703, 0.3219752754296894559, 0.3333333333333333703, 0.3219752754296894559, 0.3333333333333333703, 0.3219752754296894559, 0.3333333333333333703, 0.3219752754296894559, 0.3333333333333333703, 0.3219752754296894559, 0.3333333333333333703, 0.3219752754296894559, 0.3333333333333333703, 0.3219752754296894559, 0.3333333333333333703, 0.3219752754296894559, 0.3333333333333333703, 0.3219752754296894559, 0.3333333333333333703, 0.3219752754296894559, 0.3333333333333333703, 0.3219752754296894559, 0.3333333333333333703, 0.3219752754296894559, 0.3333333333333333703, 0.3219752754296894559, 0.3333333333333333703, 0.3219752754296894559, 0.3333333333333333703),
 ( 0.3333333333333333703, 0.3219752754296894559, 0.3333333333333333703, 0.3219752754296894559, 0.3333333333333333703, 0.3219752754296894559, 0.3333333333333333703, 0.3219752754296894559, 0.3333333333333333703, 0.3219752754296894559, 0.3333333333333333703, 0.3219752754296894559, 0.3333333333333333703, 0.3219752754296894559, 0.3333333333333333703, 0.3219752754296894559, 0.3333333333333333703, 0.3219752754296894559, 0.3333333333333333703, 0.3219752754296894559, 0.3333333333333333703, 0.3219752754296894559, 0.3333333333333333703, 0.3219752754296894559, 0.3333333333333333703, 0.3219752754296894559, 0.3333333333333333703, 0.3219752754296894559, 0.3333333333333333703, 0.3219752754296894559, 0.3333333333333333703, 0.3219752754296894559, 0.3333333333333333703, 0.3219752754296894559, 0.3333333333333333703, 0.3219752754296894559, 0.3333333333333333703, 0.3219752754296894559, 0.3333333333333333703, 0.3219752754296894559, 0.3333333333333333703, 0.3219752754296894559, 0.3333333333333333703, 0.3219752754296894559, 0.3333333333333333703, 0.3219752754296894559, 0.3333333333333333703, 0.3219752754296894559, 0.3333333333333333703, 0.3219752754296894559, 0.3333333333333333703, 0.3219752754296894559, 0.3333333333333333703, 0.3219752754296894559, 0.3333333333333333703, 0.3219752754296894559, 0.3333333333333333703, 0.3219752754296894559, 0.3333333333333333703, 0.3219752754296894559, 0.3333333333333333703, 0.3219752754296894559, 0.3333333333333333703, 0.3219752754296894559, 0.3333333333333333703, 0.3219752754296894559, 0.3333333333333333703, 0.3219752754296894559, 0.3333333333333333703, 0.3219752754296894559, 0.3333333333333333703, 0.3219752754296894559, 0.3333333333333333703, 0.3219752754296894559, 0.3333333333333333703, 0.3219752754296894559, 0.3333333333333333703, 0.3219752754296894559, 0.3333333333333333703, 0.3219752754296894559, 0.3333333333333333703, 0.3219752754296894559, 0.3333333333333333703, 0.3219752754296894559, 0.3333333333333333703, 0.3219752754296894559, 0.3333333333333333703, 0.3219752754296894559, 0.3333333333333333703, 0.3219752754296894559, 0.3333333333333333703, 0.3219752754296894559, 0.3333333333333333703, 0.3219752754296894559, 0.3333333333333333703, 0.3219752754296894559, 0.3333333333333333703, 0.3219752754296894559, 0.3333333333333333703, 0.3219752754296894559, 0.3333333333333333703, 0.3219752754296894559, 0.3333333333333333703, 0.3219752754296894559, 0.3333333333333333703, 0.3219752754296894559, 0.3333333333333333703, 0.3219752754296894559, 0.3333333333333333703, 0.3219752754296894559, 0.3333333333333333703, 0.3219752754296894559, 0.3333333333333333703, 0.3219752754296894559, 0.3333333333333333703, 0.3219752754296894559, 0.3333333333333333703, 0.3219752754296894559, 0.3333333333333333703, 0.3219752754296894559, 0.3333333333333333703, 0.3219752754296894559, 0.3333333333333333703, 0.3219752754296894559, 0.3333333333333333703, 0.3219752754296894559, 0.3333333333333333703, 0.3219752754296894559, 0.3333333333333333703, 0.3219752754296894559, 0.3333333333333333703, 0.3219752754296894559, 0.3333333333333333703, 0.3219752754296894559, 0.3333333333333333703, 0.3219752754296894559, 0.3333333333333333703, 0.3219752754296894559, 0.3333333333333333703, 0.3219752754296894559, 0.3333333333333333703, 0.3219752754296894559, 0.3333333333333333703, 0.3219752754296894559, 0.3333333333333333703, 0.3219752754296894559, 0.3333333333333333703, 0.3219752754296894559, 0.3333333333333333703, 0.3219752754296894559, 0.3333333333333333703, 0.3219752754296894559, 0.3333333333333333703, 0.3219752754296894559, 0.3333333333333333703, 0.3219752754296894559, 0.3333333333333333703, 0.3219752754296894559, 0.3333333333333333703, 0.3219752754296894559, 0.3333333333333333703, 0.3219752754296894559, 0.3333333333333333703, 0.3219752754296894559, 0.3333333333333333703, 0.3219752754296894559, 0.3333333333333333703, 0.3219752754296894559, 0.3333333333333333703, 0.3219752754296894559, 0.3333333333333333703, 0.3219752754296894559, 0.3333333333333333703, 0.3219752754296894559, 0.3333333333333333703, 0.3219752754296894559, 0.3333333333333333703, 0.3219752754296894559, 0.3333333333333333703, 0.3219752754296894559, 0.3333333333333333703, 0.3219752754296894559, 0.3333333333333333703, 0.3219752754296894559, 0.3333333333333333703, 0.3219752754296894559, 0.3333333333333333703, 0.3219752754296894559, 0.3333333333333333703, 0.3219752754296894559, 0.3333333333333333703, 0.3219752754296894559, 0.3333333333333333703, 0.3219752754296894559, 0.3333333333333333703, 0.3219752754296894559, 0.3333333333333333703, 0.3219752754296894559, 0.3333333333333333703, 0.3219752754296894559, 0.3333333333333333703, 0.3219752754296894559, 0.3333333333333333703, 0.3219752754296894559, 0.3333333333333333703, 0.3219752754296894559, 0.3333333333333333703, 0.3219752754296894559, 0.3333333333333333703, 0.3219752754296894559, 0.3333333333333333703, 0.3219752754296894559, 0.3333333333333333703, 0.3219752754296894559, 0.3333333333333333703, 0.3219752754296894559, 0.3333333333333333703, 0.3219752754296894559, 0.3333333333333333703, 0.3219752754296894559, 0.3333333333333333703, 0.3219752754296894559, 0.3333333333333333703, 0.3219752754296894559, 0.3333333333333333703, 0.3219752754296894559, 0.3333333333333333703, 0.3219752754296894559, 0.3333333333333333703, 0.3219752754296894559, 0.3333333333333333703, 0.3219752754296894559, 0.3333333333333333703, 0.3219752754296894559, 0.3333333333333333703, 0.3219752754296894559, 0.3333333333333333703, 0.3219752754296894559, 0.3333333333333333703, 0.3219752754296894559, 0.3333333333333333703, 0.3219752754296894559, 0.3333333333333333703, 0.3219752754296894559, 0.3333333333333333703, 0.3219752754296894559, 0.3333333333333333703, 0.3219752754296894559, 0.3333333333333333703, 0.3219752754296894559, 0.3333333333333333703, 0.3219752754296894559, 0.3333333333333333703, 0.3219752754296894559, 0.3333333333333333703, 0.3219752754296894559, 0.3333333333333333703, 0.3219752754296894559, 0.3333333333333333703, 0.3219752754296894559, 0.3333333333333333703, 0.3219752754296894559, 0.3333333333333333703, 0.3219752754296894559, 0.3333333333333333703, 0.3219752754296894559, 0.3333333333333333703, 0.3219752754296894559, 0.3333333333333333703, 0.3219752754296894559, 0.3333333333333333703, 0.3219752754296894559, 0.3333333333333333703, 0.3219752754296894559, 0.3333333333333333703, 0.3219752754296894559, 0.3333333333333333703, 0.3219752754296894559, 0.3333333333333333703, 0.3219752754296894559, 0.3333333333333333703, 0.3219752754296894559, 0.3333333333333333703, 0.3219752754296894559, 0.3333333333333333703, 0.3219752754296894559, 0.3333333333333333703, 0.3219752754296894559, 0.3333333333333333703, 0.3219752754296894559, 0.3333333333333333703, 0.3219752754296894559, 0.3333333333333333703, 0.3219752754296894559, 0.3333333333333333703, 0.3219752754296894559, 0.3333333333333333703, 0.3219752754296894559, 0.3333333333333333703, 0.3219752754296894559, 0.3333333333333333703, 0.3219752754296894559, 0.3333333333333333703, 0.3219752754296894559, 0.3333333333333333703, 0.3219752754296894559, 0.3333333333333333703, 0.3219752754296894559, 0.3333333333333333703, 0.3219752754296894559, 0.3333333333333333703, 0.3219752754296894559, 0.3333333333333333703, 0.3219752754296894559, 0.3333333333333333703, 0.3219752754296894559, 0.3333333333333333703, 0.3219752754296894559, 0.3333333333333333703, 0.3219752754296894559, 0.3333333333333333703, 0.3219752754296894559, 0.3333333333333333703, 0.3219752754296894559, 0.3333333333333333703, 0.3219752754296894559, 0.3333333333333333703, 0.3219752754296894559, 0.3333333333333333703, 0.3219752754296894559, 0.3333333333333333703, 0.3219752754296894559, 0.3333333333333333703, 0.3219752754296894559, 0.3333333333333333703, 0.3219752754296894559, 0.3333333333333333703, 0.3219752754296894559, 0.3333333333333333703, 0.3219752754296894559, 0.3333333333333333703, 0.3219752754296894559, 0.3333333333333333703, 0.3219752754296894559, 0.3333333333333333703, 0.3219752754296894559, 0.3333333333333333703, 0.3219752754296894559, 0.3333333333333333703, 0.3219752754296894559, 0.3333333333333333703, 0.3219752754296894559, 0.3333333333333333703, 0.3219752754296894559, 0.3333333333333333703, 0.3219752754296894559, 0.3333333333333333703, 0.3219752754296894559, 0.3333333333333333703, 0.3219752754296894559, 0.3333333333333333703, 0.3219752754296894559, 0.3333333333333333703, 0.3219752754296894559, 0.3333333333333333703, 0.3219752754296894559, 0.3333333333333333703, 0.3219752754296894559, 0.3333333333333333703, 0.3219752754296894559, 0.3333333333333333703, 0.3219752754296894559, 0.3333333333333333703, 0.3219752754296894559, 0.3333333333333333703, 0.3219752754296894559, 0.3333333333333333703, 0.3219752754296894559, 0.3333333333333333703, 0.3219752754296894559, 0.3333333333333333703, 0.3219752754296894559, 0.3333333333333333703, 0.3219752754296894559, 0.3333333333333333703, 0.3219752754296894559, 0.3333333333333333703, 0.3219752754296894559, 0.3333333333333333703, 0.3219752754296894559, 0.3333333333333333703, 0.3219752754296894559, 0.3333333333333333703, 0.3219752754296894559, 0.3333333333333333703, 0.3219752754296894559, 0.3333333333333333703, 0.3219752754296894559, 0.3333333333333333703, 0.3219752754296894559, 0.3333333333333333703, 0.3219752754296894559, 0.3333333333333333703, 0.3219752754296894559, 0.3333333333333333703, 0.3219752754296894559, 0.3333333333333333703, 0.3219752754296894559, 0.3333333333333333703, 0.3219752754296894559, 0.3333333333333333703, 0.3219752754296894559, 0.3333333333333333703, 0.3219752754296894559, 0.3333333333333333703, 0.3219752754296894559, 0.3333333333333333703, 0.3219752754296894559, 0.3333333333333333703, 0.3219752754296894559, 0.3333333333333333703, 0.3219752754296894559, 0.3333333333333333703, 0.3219752754296894559, 0.3333333333333333703, 0.3219752754296894559, 0.3333333333333333703, 0.3219752754296894559, 0.3333333333333333703, 0.3219752754296894559, 0.3333333333333333703, 0.3219752754296894559, 0.3333333333333333703, 0.3219752754296894559, 0.3333333333333333703, 0.3219752754296894559, 0.3333333333333333703, 0.3219752754296894559, 0.3333333333333333703, 0.3219752754296894559, 0.3333333333333333703, 0.3219752754296894559, 0.3333333333333333703, 0.3219752754296894559, 0.3333333333333333703, 0.3219752754296894559, 0.3333333333333333703, 0.3219752754296894559, 0.3333333333333333703, 0.3219752754296894559, 0.3333333333333333703, 0.3219752754296894559, 0.3333333333333333703, 0.3219752754296894559, 0.3333333333333333703, 0.3219752754296894559, 0.3333333333333333703),
 ( 1.000000000000000000, 0.9659258262890683122, 1.000000000000000000, 0.9659258262890683122, 1.000000000000000000, 0.9659258262890683122, 1.000000000000000000, 0.9659258262890683122, 1.000000000000000000, 0.9659258262890683122, 1.000000000000000000, 0.9659258262890683122, 1.000000000000000000, 0.9659258262890683122, 1.000000000000000000, 0.9659258262890683122, 1.000000000000000000, 0.9659258262890683122, 1.000000000000000000, 0.9659258262890683122, 1.000000000000000000, 0.9659258262890683122, 1.000000000000000000, 0.9659258262890683122, 1.000000000000000000, 0.9659258262890683122, 1.000000000000000000, 0.9659258262890683122, 1.000000000000000000, 0.9659258262890683122, 1.000000000000000000, 0.9659258262890683122, 1.000000000000000000, 0.9659258262890683122, 1.000000000000000000, 0.9659258262890683122, 1.000000000000000000, 0.9659258262890683122, 1.000000000000000000, 0.9659258262890683122, 1.000000000000000000, 0.9659258262890683122, 1.000000000000000000, 0.9659258262890683122, 1.000000000000000000, 0.9659258262890683122, 1.000000000000000000, 0.9659258262890683122, 1.000000000000000000, 0.9659258262890683122, 1.000000000000000000, 0.9659258262890683122, 1.000000000000000000, 0.9659258262890683122, 1.000000000000000000, 0.9659258262890683122, 1.000000000000000000, 0.9659258262890683122, 1.000000000000000000, 0.9659258262890683122, 1.000000000000000000, 0.9659258262890683122, 1.000000000000000000, 0.9659258262890683122, 1.000000000000000000, 0.9659258262890683122, 1.000000000000000000, 0.9659258262890683122, 1.000000000000000000, 0.9659258262890683122, 1.000000000000000000, 0.9659258262890683122, 1.000000000000000000, 0.9659258262890683122, 1.000000000000000000, 0.9659258262890683122, 1.000000000000000000, 0.9659258262890683122, 1.000000000000000000, 0.9659258262890683122, 1.000000000000000000, 0.9659258262890683122, 1.000000000000000000, 0.9659258262890683122, 1.000000000000000000, 0.9659258262890683122, 1.000000000000000000, 0.9659258262890683122, 1.000000000000000000, 0.9659258262890683122, 1.000000000000000000, 0.9659258262890683122, 1.000000000000000000, 0.9659258262890683122, 1.000000000000000000, 0.9659258262890683122, 1.000000000000000000, 0.9659258262890683122, 1.000000000000000000, 0.9659258262890683122, 1.000000000000000000, 0.9659258262890683122, 1.000000000000000000, 0.9659258262890683122, 1.000000000000000000, 0.9659258262890683122, 1.000000000000000000, 0.9659258262890683122, 1.000000000000000000, 0.9659258262890683122, 1.000000000000000000, 0.9659258262890683122, 1.000000000000000000, 0.9659258262890683122, 1.000000000000000000, 0.9659258262890683122, 1.000000000000000000, 0.9659258262890683122, 1.000000000000000000, 0.9659258262890683122, 1.000000000000000000, 0.9659258262890683122, 1.000000000000000000, 0.9659258262890683122, 1.000000000000000000, 0.9659258262890683122, 1.000000000000000000, 0.9659258262890683122, 1.000000000000000000, 0.9659258262890683122, 1.000000000000000000, 0.9659258262890683122, 1.000000000000000000, 0.9659258262890683122, 1.000000000000000000, 0.9659258262890683122, 1.000000000000000000, 0.9659258262890683122, 1.000000000000000000, 0.9659258262890683122, 1.000000000000000000, 0.9659258262890683122, 1.000000000000000000, 0.9659258262890683122, 1.000000000000000000, 0.9659258262890683122, 1.000000000000000000, 0.9659258262890683122, 1.000000000000000000, 0.9659258262890683122, 1.000000000000000000, 0.9659258262890683122, 1.000000000000000000, 0.9659258262890683122, 1.000000000000000000, 0.9659258262890683122, 1.000000000000000000, 0.9659258262890683122, 1.000000000000000000, 0.9659258262890683122, 1.000000000000000000, 0.9659258262890683122, 1.000000000000000000, 0.9659258262890683122, 1.000000000000000000, 0.9659258262890683122, 1.000000000000000000, 0.9659258262890683122, 1.000000000000000000, 0.9659258262890683122, 1.000000000000000000, 0.9659258262890683122, 1.000000000000000000, 0.9659258262890683122, 1.000000000000000000, 0.9659258262890683122, 1.000000000000000000, 0.9659258262890683122, 1.000000000000000000, 0.9659258262890683122, 1.000000000000000000, 0.9659258262890683122, 1.000000000000000000, 0.9659258262890683122, 1.000000000000000000, 0.9659258262890683122, 1.000000000000000000, 0.9659258262890683122, 1.000000000000000000, 0.9659258262890683122, 1.000000000000000000, 0.9659258262890683122, 1.000000000000000000, 0.9659258262890683122, 1.000000000000000000, 0.9659258262890683122, 1.000000000000000000, 0.9659258262890683122, 1.000000000000000000, 0.9659258262890683122, 1.000000000000000000, 0.9659258262890683122, 1.000000000000000000, 0.9659258262890683122, 1.000000000000000000, 0.9659258262890683122, 1.000000000000000000, 0.9659258262890683122, 1.000000000000000000, 0.9659258262890683122, 1.000000000000000000, 0.9659258262890683122, 1.000000000000000000, 0.9659258262890683122, 1.000000000000000000, 0.9659258262890683122, 1.000000000000000000, 0.9659258262890683122, 1.000000000000000000, 0.9659258262890683122, 1.000000000000000000, 0.9659258262890683122, 1.000000000000000000, 0.9659258262890683122, 1.000000000000000000, 0.9659258262890683122, 1.000000000000000000, 0.9659258262890683122, 1.000000000000000000, 0.9659258262890683122, 1.000000000000000000, 0.9659258262890683122, 1.000000000000000000, 0.9659258262890683122, 1.000000000000000000, 0.9659258262890683122, 1.000000000000000000, 0.9659258262890683122, 1.000000000000000000, 0.9659258262890683122, 1.000000000000000000, 0.9659258262890683122, 1.000000000000000000, 0.9659258262890683122, 1.000000000000000000, 0.9659258262890683122, 1.000000000000000000, 0.9659258262890683122, 1.000000000000000000, 0.9659258262890683122, 1.000000000000000000, 0.9659258262890683122, 1.000000000000000000, 0.9659258262890683122, 1.000000000000000000, 0.9659258262890683122, 1.000000000000000000, 0.9659258262890683122, 1.000000000000000000, 0.9659258262890683122, 1.000000000000000000, 0.9659258262890683122, 1.000000000000000000, 0.9659258262890683122, 1.000000000000000000, 0.9659258262890683122, 1.000000000000000000, 0.9659258262890683122, 1.000000000000000000, 0.9659258262890683122, 1.000000000000000000, 0.9659258262890683122, 1.000000000000000000, 0.9659258262890683122, 1.000000000000000000, 0.9659258262890683122, 1.000000000000000000, 0.9659258262890683122, 1.000000000000000000, 0.9659258262890683122, 1.000000000000000000, 0.9659258262890683122, 1.000000000000000000, 0.9659258262890683122, 1.000000000000000000, 0.9659258262890683122, 1.000000000000000000, 0.9659258262890683122, 1.000000000000000000, 0.9659258262890683122, 1.000000000000000000, 0.9659258262890683122, 1.000000000000000000, 0.9659258262890683122, 1.000000000000000000, 0.9659258262890683122, 1.000000000000000000, 0.9659258262890683122, 1.000000000000000000, 0.9659258262890683122, 1.000000000000000000, 0.9659258262890683122, 1.000000000000000000, 0.9659258262890683122, 1.000000000000000000, 0.9659258262890683122, 1.000000000000000000, 0.9659258262890683122, 1.000000000000000000, 0.9659258262890683122, 1.000000000000000000, 0.9659258262890683122, 1.000000000000000000, 0.9659258262890683122, 1.000000000000000000, 0.9659258262890683122, 1.000000000000000000, 0.9659258262890683122, 1.000000000000000000, 0.9659258262890683122, 1.000000000000000000, 0.9659258262890683122, 1.000000000000000000, 0.9659258262890683122, 1.000000000000000000, 0.9659258262890683122, 1.000000000000000000, 0.9659258262890683122, 1.000000000000000000, 0.9659258262890683122, 1.000000000000000000, 0.9659258262890683122, 1.000000000000000000, 0.9659258262890683122, 1.000000000000000000, 0.9659258262890683122, 1.000000000000000000, 0.9659258262890683122, 1.000000000000000000, 0.9659258262890683122, 1.000000000000000000, 0.9659258262890683122, 1.000000000000000000, 0.9659258262890683122, 1.000000000000000000, 0.9659258262890683122, 1.000000000000000000, 0.9659258262890683122, 1.000000000000000000, 0.9659258262890683122, 1.000000000000000000, 0.9659258262890683122, 1.000000000000000000, 0.9659258262890683122, 1.000000000000000000, 0.9659258262890683122, 1.000000000000000000, 0.9659258262890683122, 1.000000000000000000, 0.9659258262890683122, 1.000000000000000000, 0.9659258262890683122, 1.000000000000000000, 0.9659258262890683122, 1.000000000000000000, 0.9659258262890683122, 1.000000000000000000, 0.9659258262890683122, 1.000000000000000000, 0.9659258262890683122, 1.000000000000000000, 0.9659258262890683122, 1.000000000000000000, 0.9659258262890683122, 1.000000000000000000, 0.9659258262890683122, 1.000000000000000000, 0.9659258262890683122, 1.000000000000000000, 0.9659258262890683122, 1.000000000000000000, 0.9659258262890683122, 1.000000000000000000, 0.9659258262890683122, 1.000000000000000000, 0.9659258262890683122, 1.000000000000000000, 0.9659258262890683122, 1.000000000000000000, 0.9659258262890683122, 1.000000000000000000, 0.9659258262890683122, 1.000000000000000000, 0.9659258262890683122, 1.000000000000000000, 0.9659258262890683122, 1.000000000000000000, 0.9659258262890683122, 1.000000000000000000, 0.9659258262890683122, 1.000000000000000000, 0.9659258262890683122, 1.000000000000000000, 0.9659258262890683122, 1.000000000000000000, 0.9659258262890683122, 1.000000000000000000, 0.9659258262890683122, 1.000000000000000000, 0.9659258262890683122, 1.000000000000000000, 0.9659258262890683122, 1.000000000000000000, 0.9659258262890683122, 1.000000000000000000, 0.9659258262890683122, 1.000000000000000000, 0.9659258262890683122, 1.000000000000000000, 0.9659258262890683122, 1.000000000000000000, 0.9659258262890683122, 1.000000000000000000, 0.9659258262890683122, 1.000000000000000000, 0.9659258262890683122, 1.000000000000000000, 0.9659258262890683122, 1.000000000000000000, 0.9659258262890683122, 1.000000000000000000, 0.9659258262890683122, 1.000000000000000000, 0.9659258262890683122, 1.000000000000000000, 0.9659258262890683122, 1.000000000000000000, 0.9659258262890683122, 1.000000000000000000, 0.9659258262890683122, 1.000000000000000000, 0.9659258262890683122, 1.000000000000000000, 0.9659258262890683122, 1.000000000000000000, 0.9659258262890683122, 1.000000000000000000, 0.9659258262890683122, 1.000000000000000000, 0.9659258262890683122, 1.000000000000000000, 0.9659258262890683122, 1.000000000000000000, 0.9659258262890683122, 1.000000000000000000, 0.9659258262890683122, 1.000000000000000000),
 ( 0.3333333333333333703, 0.3219752754296894559, 0.3333333333333333703, 0.3219752754296894559, 0.3333333333333333703, 0.3219752754296894559, 0.3333333333333333703, 0.3219752754296894559, 0.3333333333333333703, 0.3219752754296894559, 0.3333333333333333703, 0.3219752754296894559, 0.3333333333333333703, 0.3219752754296894559, 0.3333333333333333703, 0.3219752754296894559, 0.3333333333333333703, 0.3219752754296894559, 0.3333333333333333703, 0.3219752754296894559, 0.3333333333333333703, 0.3219752754296894559, 0.3333333333333333703, 0.3219752754296894559, 0.3333333333333333703, 0.3219752754296894559, 0.3333333333333333703, 0.3219752754296894559, 0.3333333333333333703, 0.3219752754296894559, 0.3333333333333333703, 0.3219752754296894559, 0.3333333333333333703, 0.3219752754296894559, 0.3333333333333333703, 0.3219752754296894559, 0.3333333333333333703, 0.3219752754296894559, 0.3333333333333333703, 0.3219752754296894559, 0.3333333333333333703, 0.3219752754296894559, 0.3333333333333333703, 0.3219752754296894559, 0.3333333333333333703, 0.3219752754296894559, 0.3333333333333333703, 0.3219752754296894559, 0.3333333333333333703, 0.3219752754296894559, 0.3333333333333333703, 0.3219752754296894559, 0.3333333333333333703, 0.3219752754296894559, 0.3333333333333333703, 0.3219752754296894559, 0.3333333333333333703, 0.3219752754296894559, 0.3333333333333333703, 0.3219752754296894559, 0.3333333333333333703, 0.3219752754296894559, 0.3333333333333333703, 0.3219752754296894559, 0.3333333333333333703, 0.3219752754296894559, 0.3333333333333333703, 0.3219752754296894559, 0.3333333333333333703, 0.3219752754296894559, 0.3333333333333333703, 0.3219752754296894559, 0.3333333333333333703, 0.3219752754296894559, 0.3333333333333333703, 0.3219752754296894559, 0.3333333333333333703, 0.3219752754296894559, 0.3333333333333333703, 0.3219752754296894559, 0.3333333333333333703, 0.3219752754296894559, 0.3333333333333333703, 0.3219752754296894559, 0.3333333333333333703, 0.3219752754296894559, 0.3333333333333333703, 0.3219752754296894559, 0.3333333333333333703, 0.3219752754296894559, 0.3333333333333333703, 0.3219752754296894559, 0.3333333333333333703, 0.3219752754296894559, 0.3333333333333333703, 0.3219752754296894559, 0.3333333333333333703, 0.3219752754296894559, 0.3333333333333333703, 0.3219752754296894559, 0.3333333333333333703, 0.3219752754296894559, 0.3333333333333333703, 0.3219752754296894559, 0.3333333333333333703, 0.3219752754296894559, 0.3333333333333333703, 0.3219752754296894559, 0.3333333333333333703, 0.3219752754296894559, 0.3333333333333333703, 0.3219752754296894559, 0.3333333333333333703, 0.3219752754296894559, 0.3333333333333333703, 0.3219752754296894559, 0.3333333333333333703, 0.3219752754296894559, 0.3333333333333333703, 0.3219752754296894559, 0.3333333333333333703, 0.3219752754296894559, 0.3333333333333333703, 0.3219752754296894559, 0.3333333333333333703, 0.3219752754296894559, 0.3333333333333333703, 0.3219752754296894559, 0.3333333333333333703, 0.3219752754296894559, 0.3333333333333333703, 0.3219752754296894559, 0.3333333333333333703, 0.3219752754296894559, 0.3333333333333333703, 0.3219752754296894559, 0.3333333333333333703, 0.3219752754296894559, 0.3333333333333333703, 0.3219752754296894559, 0.3333333333333333703, 0.3219752754296894559, 0.3333333333333333703, 0.3219752754296894559, 0.3333333333333333703, 0.3219752754296894559, 0.3333333333333333703, 0.3219752754296894559, 0.3333333333333333703, 0.3219752754296894559, 0.3333333333333333703, 0.3219752754296894559, 0.3333333333333333703, 0.3219752754296894559, 0.3333333333333333703, 0.3219752754296894559, 0.3333333333333333703, 0.3219752754296894559, 0.3333333333333333703, 0.3219752754296894559, 0.3333333333333333703, 0.3219752754296894559, 0.3333333333333333703, 0.3219752754296894559, 0.3333333333333333703, 0.3219752754296894559, 0.3333333333333333703, 0.3219752754296894559, 0.3333333333333333703, 0.3219752754296894559, 0.3333333333333333703, 0.3219752754296894559, 0.3333333333333333703, 0.3219752754296894559, 0.3333333333333333703, 0.3219752754296894559, 0.3333333333333333703, 0.3219752754296894559, 0.3333333333333333703, 0.3219752754296894559, 0.3333333333333333703, 0.3219752754296894559, 0.3333333333333333703, 0.3219752754296894559, 0.3333333333333333703, 0.3219752754296894559, 0.3333333333333333703, 0.3219752754296894559, 0.3333333333333333703, 0.3219752754296894559, 0.3333333333333333703, 0.3219752754296894559, 0.3333333333333333703, 0.3219752754296894559, 0.3333333333333333703, 0.3219752754296894559, 0.3333333333333333703, 0.3219752754296894559, 0.3333333333333333703, 0.3219752754296894559, 0.3333333333333333703, 0.3219752754296894559, 0.3333333333333333703, 0.3219752754296894559, 0.3333333333333333703, 0.3219752754296894559, 0.3333333333333333703, 0.3219752754296894559, 0.3333333333333333703, 0.3219752754296894559, 0.3333333333333333703, 0.3219752754296894559, 0.3333333333333333703, 0.3219752754296894559, 0.3333333333333333703, 0.3219752754296894559, 0.3333333333333333703, 0.3219752754296894559, 0.3333333333333333703, 0.3219752754296894559, 0.3333333333333333703, 0.3219752754296894559, 0.3333333333333333703, 0.3219752754296894559, 0.3333333333333333703, 0.3219752754296894559, 0.3333333333333333703, 0.3219752754296894559, 0.3333333333333333703, 0.3219752754296894559, 0.3333333333333333703, 0.3219752754296894559, 0.3333333333333333703, 0.3219752754296894559, 0.3333333333333333703, 0.3219752754296894559, 0.3333333333333333703, 0.3219752754296894559, 0.3333333333333333703, 0.3219752754296894559, 0.3333333333333333703, 0.3219752754296894559, 0.3333333333333333703, 0.3219752754296894559, 0.3333333333333333703, 0.3219752754296894559, 0.3333333333333333703, 0.3219752754296894559, 0.3333333333333333703, 0.3219752754296894559, 0.3333333333333333703, 0.3219752754296894559, 0.3333333333333333703, 0.3219752754296894559, 0.3333333333333333703, 0.3219752754296894559, 0.3333333333333333703, 0.3219752754296894559, 0.3333333333333333703, 0.3219752754296894559, 0.3333333333333333703, 0.3219752754296894559, 0.3333333333333333703, 0.3219752754296894559, 0.3333333333333333703, 0.3219752754296894559, 0.3333333333333333703, 0.3219752754296894559, 0.3333333333333333703, 0.3219752754296894559, 0.3333333333333333703, 0.3219752754296894559, 0.3333333333333333703, 0.3219752754296894559, 0.3333333333333333703, 0.3219752754296894559, 0.3333333333333333703, 0.3219752754296894559, 0.3333333333333333703, 0.3219752754296894559, 0.3333333333333333703, 0.3219752754296894559, 0.3333333333333333703, 0.3219752754296894559, 0.3333333333333333703, 0.3219752754296894559, 0.3333333333333333703, 0.3219752754296894559, 0.3333333333333333703, 0.3219752754296894559, 0.3333333333333333703, 0.3219752754296894559, 0.3333333333333333703, 0.3219752754296894559, 0.3333333333333333703, 0.3219752754296894559, 0.3333333333333333703, 0.3219752754296894559, 0.3333333333333333703, 0.3219752754296894559, 0.3333333333333333703, 0.3219752754296894559, 0.3333333333333333703, 0.3219752754296894559, 0.3333333333333333703, 0.3219752754296894559, 0.3333333333333333703, 0.3219752754296894559, 0.3333333333333333703, 0.3219752754296894559, 0.3333333333333333703, 0.3219752754296894559, 0.3333333333333333703, 0.3219752754296894559, 0.3333333333333333703, 0.3219752754296894559, 0.3333333333333333703, 0.3219752754296894559, 0.3333333333333333703, 0.3219752754296894559, 0.3333333333333333703, 0.3219752754296894559, 0.3333333333333333703, 0.3219752754296894559, 0.3333333333333333703, 0.3219752754296894559, 0.3333333333333333703, 0.3219752754296894559, 0.3333333333333333703, 0.3219752754296894559, 0.3333333333333333703, 0.3219752754296894559, 0.3333333333333333703, 0.3219752754296894559, 0.3333333333333333703, 0.3219752754296894559, 0.3333333333333333703, 0.3219752754296894559, 0.3333333333333333703, 0.3219752754296894559, 0.3333333333333333703, 0.3219752754296894559, 0.3333333333333333703, 0.3219752754296894559, 0.3333333333333333703, 0.3219752754296894559, 0.3333333333333333703, 0.3219752754296894559, 0.3333333333333333703, 0.3219752754296894559, 0.3333333333333333703, 0.3219752754296894559, 0.3333333333333333703, 0.3219752754296894559, 0.3333333333333333703, 0.3219752754296894559, 0.3333333333333333703, 0.3219752754296894559, 0.3333333333333333703, 0.3219752754296894559, 0.3333333333333333703, 0.3219752754296894559, 0.3333333333333333703, 0.3219752754296894559, 0.3333333333333333703, 0.3219752754296894559, 0.3333333333333333703, 0.3219752754296894559, 0.3333333333333333703, 0.3219752754296894559, 0.3333333333333333703, 0.3219752754296894559, 0.3333333333333333703, 0.3219752754296894559, 0.3333333333333333703, 0.3219752754296894559, 0.3333333333333333703, 0.3219752754296894559, 0.3333333333333333703, 0.3219752754296894559, 0.3333333333333333703, 0.3219752754296894559, 0.3333333333333333703, 0.3219752754296894559, 0.3333333333333333703, 0.3219752754296894559, 0.3333333333333333703, 0.3219752754296894559, 0.3333333333333333703, 0.3219752754296894559, 0.3333333333333333703, 0.3219752754296894559, 0.3333333333333333703, 0.3219752754296894559, 0.3333333333333333703, 0.3219752754296894559, 0.3333333333333333703, 0.3219752754296894559, 0.3333333333333333703, 0.3219752754296894559, 0.3333333333333333703, 0.3219752754296894559, 0.3333333333333333703, 0.3219752754296894559, 0.3333333333333333703, 0.3219752754296894559, 0.3333333333333333703, 0.3219752754296894559, 0.3333333333333333703, 0.3219752754296894559, 0.3333333333333333703, 0.3219752754296894559, 0.3333333333333333703, 0.3219752754296894559, 0.3333333333333333703, 0.3219752754296894559, 0.3333333333333333703, 0.3219752754296894559, 0.3333333333333333703, 0.3219752754296894559, 0.3333333333333333703, 0.3219752754296894559, 0.3333333333333333703, 0.3219752754296894559, 0.3333333333333333703, 0.3219752754296894559, 0.3333333333333333703, 0.3219752754296894559, 0.3333333333333333703, 0.3219752754296894559, 0.3333333333333333703, 0.3219752754296894559, 0.3333333333333333703, 0.3219752754296894559, 0.3333333333333333703, 0.3219752754296894559, 0.3333333333333333703, 0.3219752754296894559, 0.3333333333333333703, 0.3219752754296894559, 0.3333333333333333703, 0.3219752754296894559, 0.3333333333333333703, 0.3219752754296894559, 0.3333333333333333703, 0.3219752754296894559, 0.3333333333333333703, 0.3219752754296894559, 0.3333333333333333703, 0.3219752754296894559, 0.3333333333333333703, 0.3219752754296894559, 0.3333333333333333703, 0.3219752754296894559, 0.3333333333333333703, 0.3219752754296894559, 0.3333333333333333703),
 ( 0.3333333333333333703, 0.3219752754296894559, 0.3333333333333333703, 0.3219752754296894559, 0.3333333333333333703, 0.3219752754296894559, 0.3333333333333333703, 0.3219752754296894559, 0.3333333333333333703, 0.3219752754296894559, 0.3333333333333333703, 0.3219752754296894559, 0.3333333333333333703, 0.3219752754296894559, 0.3333333333333333703, 0.3219752754296894559, 0.3333333333333333703, 0.3219752754296894559, 0.3333333333333333703, 0.3219752754296894559, 0.3333333333333333703, 0.3219752754296894559, 0.3333333333333333703, 0.3219752754296894559, 0.3333333333333333703, 0.3219752754296894559, 0.3333333333333333703, 0.3219752754296894559, 0.3333333333333333703, 0.3219752754296894559, 0.3333333333333333703, 0.3219752754296894559, 0.3333333333333333703, 0.3219752754296894559, 0.3333333333333333703, 0.3219752754296894559, 0.3333333333333333703, 0.3219752754296894559, 0.3333333333333333703, 0.3219752754296894559, 0.3333333333333333703, 0.3219752754296894559, 0.3333333333333333703, 0.3219752754296894559, 0.3333333333333333703, 0.3219752754296894559, 0.3333333333333333703, 0.3219752754296894559, 0.3333333333333333703, 0.3219752754296894559, 0.3333333333333333703, 0.3219752754296894559, 0.3333333333333333703, 0.3219752754296894559, 0.3333333333333333703, 0.3219752754296894559, 0.3333333333333333703, 0.3219752754296894559, 0.3333333333333333703, 0.3219752754296894559, 0.3333333333333333703, 0.3219752754296894559, 0.3333333333333333703, 0.3219752754296894559, 0.3333333333333333703, 0.3219752754296894559, 0.3333333333333333703, 0.3219752754296894559, 0.3333333333333333703, 0.3219752754296894559, 0.3333333333333333703, 0.3219752754296894559, 0.3333333333333333703, 0.3219752754296894559, 0.3333333333333333703, 0.3219752754296894559, 0.3333333333333333703, 0.3219752754296894559, 0.3333333333333333703, 0.3219752754296894559, 0.3333333333333333703, 0.3219752754296894559, 0.3333333333333333703, 0.3219752754296894559, 0.3333333333333333703, 0.3219752754296894559, 0.3333333333333333703, 0.3219752754296894559, 0.3333333333333333703, 0.3219752754296894559, 0.3333333333333333703, 0.3219752754296894559, 0.3333333333333333703, 0.3219752754296894559, 0.3333333333333333703, 0.3219752754296894559, 0.3333333333333333703, 0.3219752754296894559, 0.3333333333333333703, 0.3219752754296894559, 0.3333333333333333703, 0.3219752754296894559, 0.3333333333333333703, 0.3219752754296894559, 0.3333333333333333703, 0.3219752754296894559, 0.3333333333333333703, 0.3219752754296894559, 0.3333333333333333703, 0.3219752754296894559, 0.3333333333333333703, 0.3219752754296894559, 0.3333333333333333703, 0.3219752754296894559, 0.3333333333333333703, 0.3219752754296894559, 0.3333333333333333703, 0.3219752754296894559, 0.3333333333333333703, 0.3219752754296894559, 0.3333333333333333703, 0.3219752754296894559, 0.3333333333333333703, 0.3219752754296894559, 0.3333333333333333703, 0.3219752754296894559, 0.3333333333333333703, 0.3219752754296894559, 0.3333333333333333703, 0.3219752754296894559, 0.3333333333333333703, 0.3219752754296894559, 0.3333333333333333703, 0.3219752754296894559, 0.3333333333333333703, 0.3219752754296894559, 0.3333333333333333703, 0.3219752754296894559, 0.3333333333333333703, 0.3219752754296894559, 0.3333333333333333703, 0.3219752754296894559, 0.3333333333333333703, 0.3219752754296894559, 0.3333333333333333703, 0.3219752754296894559, 0.3333333333333333703, 0.3219752754296894559, 0.3333333333333333703, 0.3219752754296894559, 0.3333333333333333703, 0.3219752754296894559, 0.3333333333333333703, 0.3219752754296894559, 0.3333333333333333703, 0.3219752754296894559, 0.3333333333333333703, 0.3219752754296894559, 0.3333333333333333703, 0.3219752754296894559, 0.3333333333333333703, 0.3219752754296894559, 0.3333333333333333703, 0.3219752754296894559, 0.3333333333333333703, 0.3219752754296894559, 0.3333333333333333703, 0.3219752754296894559, 0.3333333333333333703, 0.3219752754296894559, 0.3333333333333333703, 0.3219752754296894559, 0.3333333333333333703, 0.3219752754296894559, 0.3333333333333333703, 0.3219752754296894559, 0.3333333333333333703, 0.3219752754296894559, 0.3333333333333333703, 0.3219752754296894559, 0.3333333333333333703, 0.3219752754296894559, 0.3333333333333333703, 0.3219752754296894559, 0.3333333333333333703, 0.3219752754296894559, 0.3333333333333333703, 0.3219752754296894559, 0.3333333333333333703, 0.3219752754296894559, 0.3333333333333333703, 0.3219752754296894559, 0.3333333333333333703, 0.3219752754296894559, 0.3333333333333333703, 0.3219752754296894559, 0.3333333333333333703, 0.3219752754296894559, 0.3333333333333333703, 0.3219752754296894559, 0.3333333333333333703, 0.3219752754296894559, 0.3333333333333333703, 0.3219752754296894559, 0.3333333333333333703, 0.3219752754296894559, 0.3333333333333333703, 0.3219752754296894559, 0.3333333333333333703, 0.3219752754296894559, 0.3333333333333333703, 0.3219752754296894559, 0.3333333333333333703, 0.3219752754296894559, 0.3333333333333333703, 0.3219752754296894559, 0.3333333333333333703, 0.3219752754296894559, 0.3333333333333333703, 0.3219752754296894559, 0.3333333333333333703, 0.3219752754296894559, 0.3333333333333333703, 0.3219752754296894559, 0.3333333333333333703, 0.3219752754296894559, 0.3333333333333333703, 0.3219752754296894559, 0.3333333333333333703, 0.3219752754296894559, 0.3333333333333333703, 0.3219752754296894559, 0.3333333333333333703, 0.3219752754296894559, 0.3333333333333333703, 0.3219752754296894559, 0.3333333333333333703, 0.3219752754296894559, 0.3333333333333333703, 0.3219752754296894559, 0.3333333333333333703, 0.3219752754296894559, 0.3333333333333333703, 0.3219752754296894559, 0.3333333333333333703, 0.3219752754296894559, 0.3333333333333333703, 0.3219752754296894559, 0.3333333333333333703, 0.3219752754296894559, 0.3333333333333333703, 0.3219752754296894559, 0.3333333333333333703, 0.3219752754296894559, 0.3333333333333333703, 0.3219752754296894559, 0.3333333333333333703, 0.3219752754296894559, 0.3333333333333333703, 0.3219752754296894559, 0.3333333333333333703, 0.3219752754296894559, 0.3333333333333333703, 0.3219752754296894559, 0.3333333333333333703, 0.3219752754296894559, 0.3333333333333333703, 0.3219752754296894559, 0.3333333333333333703, 0.3219752754296894559, 0.3333333333333333703, 0.3219752754296894559, 0.3333333333333333703, 0.3219752754296894559, 0.3333333333333333703, 0.3219752754296894559, 0.3333333333333333703, 0.3219752754296894559, 0.3333333333333333703, 0.3219752754296894559, 0.3333333333333333703, 0.3219752754296894559, 0.3333333333333333703, 0.3219752754296894559, 0.3333333333333333703, 0.3219752754296894559, 0.3333333333333333703, 0.3219752754296894559, 0.3333333333333333703, 0.3219752754296894559, 0.3333333333333333703, 0.3219752754296894559, 0.3333333333333333703, 0.3219752754296894559, 0.3333333333333333703, 0.3219752754296894559, 0.3333333333333333703, 0.3219752754296894559, 0.3333333333333333703, 0.3219752754296894559, 0.3333333333333333703, 0.3219752754296894559, 0.3333333333333333703, 0.3219752754296894559, 0.3333333333333333703, 0.3219752754296894559, 0.3333333333333333703, 0.3219752754296894559, 0.3333333333333333703, 0.3219752754296894559, 0.3333333333333333703, 0.3219752754296894559, 0.3333333333333333703, 0.3219752754296894559, 0.3333333333333333703, 0.3219752754296894559, 0.3333333333333333703, 0.3219752754296894559, 0.3333333333333333703, 0.3219752754296894559, 0.3333333333333333703, 0.3219752754296894559, 0.3333333333333333703, 0.3219752754296894559, 0.3333333333333333703, 0.3219752754296894559, 0.3333333333333333703, 0.3219752754296894559, 0.3333333333333333703, 0.3219752754296894559, 0.3333333333333333703, 0.3219752754296894559, 0.3333333333333333703, 0.3219752754296894559, 0.3333333333333333703, 0.3219752754296894559, 0.3333333333333333703, 0.3219752754296894559, 0.3333333333333333703, 0.3219752754296894559, 0.3333333333333333703, 0.3219752754296894559, 0.3333333333333333703, 0.3219752754296894559, 0.3333333333333333703, 0.3219752754296894559, 0.3333333333333333703, 0.3219752754296894559, 0.3333333333333333703, 0.3219752754296894559, 0.3333333333333333703, 0.3219752754296894559, 0.3333333333333333703, 0.3219752754296894559, 0.3333333333333333703, 0.3219752754296894559, 0.3333333333333333703, 0.3219752754296894559, 0.3333333333333333703, 0.3219752754296894559, 0.3333333333333333703, 0.3219752754296894559, 0.3333333333333333703, 0.3219752754296894559, 0.3333333333333333703, 0.3219752754296894559, 0.3333333333333333703, 0.3219752754296894559, 0.3333333333333333703, 0.3219752754296894559, 0.3333333333333333703, 0.3219752754296894559, 0.3333333333333333703, 0.3219752754296894559, 0.3333333333333333703, 0.3219752754296894559, 0.3333333333333333703, 0.3219752754296894559, 0.3333333333333333703, 0.3219752754296894559, 0.3333333333333333703, 0.3219752754296894559, 0.3333333333333333703, 0.3219752754296894559, 0.3333333333333333703, 0.3219752754296894559, 0.3333333333333333703, 0.3219752754296894559, 0.3333333333333333703, 0.3219752754296894559, 0.3333333333333333703, 0.3219752754296894559, 0.3333333333333333703, 0.3219752754296894559, 0.3333333333333333703, 0.3219752754296894559, 0.3333333333333333703, 0.3219752754296894559, 0.3333333333333333703, 0.3219752754296894559, 0.3333333333333333703, 0.3219752754296894559, 0.3333333333333333703, 0.3219752754296894559, 0.3333333333333333703, 0.3219752754296894559, 0.3333333333333333703, 0.3219752754296894559, 0.3333333333333333703, 0.3219752754296894559, 0.3333333333333333703, 0.3219752754296894559, 0.3333333333333333703, 0.3219752754296894559, 0.3333333333333333703, 0.3219752754296894559, 0.3333333333333333703, 0.3219752754296894559, 0.3333333333333333703, 0.3219752754296894559, 0.3333333333333333703, 0.3219752754296894559, 0.3333333333333333703, 0.3219752754296894559, 0.3333333333333333703, 0.3219752754296894559, 0.3333333333333333703, 0.3219752754296894559, 0.3333333333333333703, 0.3219752754296894559, 0.3333333333333333703, 0.3219752754296894559, 0.3333333333333333703, 0.3219752754296894559, 0.3333333333333333703, 0.3219752754296894559, 0.3333333333333333703, 0.3219752754296894559, 0.3333333333333333703, 0.3219752754296894559, 0.3333333333333333703, 0.3219752754296894559, 0.3333333333333333703, 0.3219752754296894559, 0.3333333333333333703, 0.3219752754296894559, 0.3333333333333333703, 0.3219752754296894559, 0.3333333333333333703, 0.3219752754296894559, 0.3333333333333333703, 0.3219752754296894559, 0.3333333333333333703, 0.3219752754296894559, 0.3333333333333333703, 0.3219752754296894559, 0.3333333333333333703),
 ( 1.000000000000000000, 0.9659258262890683122, 1.000000000000000000, 0.9659258262890683122, 1.000000000000000000, 0.9659258262890683122, 1.000000000000000000, 0.9659258262890683122, 1.000000000000000000, 0.9659258262890683122, 1.000000000000000000, 0.9659258262890683122, 1.000000000000000000, 0.9659258262890683122, 1.000000000000000000, 0.9659258262890683122, 1.000000000000000000, 0.9659258262890683122, 1.000000000000000000, 0.9659258262890683122, 1.000000000000000000, 0.9659258262890683122, 1.000000000000000000, 0.9659258262890683122, 1.000000000000000000, 0.9659258262890683122, 1.000000000000000000, 0.9659258262890683122, 1.000000000000000000, 0.9659258262890683122, 1.000000000000000000, 0.9659258262890683122, 1.000000000000000000, 0.9659258262890683122, 1.000000000000000000, 0.9659258262890683122, 1.000000000000000000, 0.9659258262890683122, 1.000000000000000000, 0.9659258262890683122, 1.000000000000000000, 0.9659258262890683122, 1.000000000000000000, 0.9659258262890683122, 1.000000000000000000, 0.9659258262890683122, 1.000000000000000000, 0.9659258262890683122, 1.000000000000000000, 0.9659258262890683122, 1.000000000000000000, 0.9659258262890683122, 1.000000000000000000, 0.9659258262890683122, 1.000000000000000000, 0.9659258262890683122, 1.000000000000000000, 0.9659258262890683122, 1.000000000000000000, 0.9659258262890683122, 1.000000000000000000, 0.9659258262890683122, 1.000000000000000000, 0.9659258262890683122, 1.000000000000000000, 0.9659258262890683122, 1.000000000000000000, 0.9659258262890683122, 1.000000000000000000, 0.9659258262890683122, 1.000000000000000000, 0.9659258262890683122, 1.000000000000000000, 0.9659258262890683122, 1.000000000000000000, 0.9659258262890683122, 1.000000000000000000, 0.9659258262890683122, 1.000000000000000000, 0.9659258262890683122, 1.000000000000000000, 0.9659258262890683122, 1.000000000000000000, 0.9659258262890683122, 1.000000000000000000, 0.9659258262890683122, 1.000000000000000000, 0.9659258262890683122, 1.000000000000000000, 0.9659258262890683122, 1.000000000000000000, 0.9659258262890683122, 1.000000000000000000, 0.9659258262890683122, 1.000000000000000000, 0.9659258262890683122, 1.000000000000000000, 0.9659258262890683122, 1.000000000000000000, 0.9659258262890683122, 1.000000000000000000, 0.9659258262890683122, 1.000000000000000000, 0.9659258262890683122, 1.000000000000000000, 0.9659258262890683122, 1.000000000000000000, 0.9659258262890683122, 1.000000000000000000, 0.9659258262890683122, 1.000000000000000000, 0.9659258262890683122, 1.000000000000000000, 0.9659258262890683122, 1.000000000000000000, 0.9659258262890683122, 1.000000000000000000, 0.9659258262890683122, 1.000000000000000000, 0.9659258262890683122, 1.000000000000000000, 0.9659258262890683122, 1.000000000000000000, 0.9659258262890683122, 1.000000000000000000, 0.9659258262890683122, 1.000000000000000000, 0.9659258262890683122, 1.000000000000000000, 0.9659258262890683122, 1.000000000000000000, 0.9659258262890683122, 1.000000000000000000, 0.9659258262890683122, 1.000000000000000000, 0.9659258262890683122, 1.000000000000000000, 0.9659258262890683122, 1.000000000000000000, 0.9659258262890683122, 1.000000000000000000, 0.9659258262890683122, 1.000000000000000000, 0.9659258262890683122, 1.000000000000000000, 0.9659258262890683122, 1.000000000000000000, 0.9659258262890683122, 1.000000000000000000, 0.9659258262890683122, 1.000000000000000000, 0.9659258262890683122, 1.000000000000000000, 0.9659258262890683122, 1.000000000000000000, 0.9659258262890683122, 1.000000000000000000, 0.9659258262890683122, 1.000000000000000000, 0.9659258262890683122, 1.000000000000000000, 0.9659258262890683122, 1.000000000000000000, 0.9659258262890683122, 1.000000000000000000, 0.9659258262890683122, 1.000000000000000000, 0.9659258262890683122, 1.000000000000000000, 0.9659258262890683122, 1.000000000000000000, 0.9659258262890683122, 1.000000000000000000, 0.9659258262890683122, 1.000000000000000000, 0.9659258262890683122, 1.000000000000000000, 0.9659258262890683122, 1.000000000000000000, 0.9659258262890683122, 1.000000000000000000, 0.9659258262890683122, 1.000000000000000000, 0.9659258262890683122, 1.000000000000000000, 0.9659258262890683122, 1.000000000000000000, 0.9659258262890683122, 1.000000000000000000, 0.9659258262890683122, 1.000000000000000000, 0.9659258262890683122, 1.000000000000000000, 0.9659258262890683122, 1.000000000000000000, 0.9659258262890683122, 1.000000000000000000, 0.9659258262890683122, 1.000000000000000000, 0.9659258262890683122, 1.000000000000000000, 0.9659258262890683122, 1.000000000000000000, 0.9659258262890683122, 1.000000000000000000, 0.9659258262890683122, 1.000000000000000000, 0.9659258262890683122, 1.000000000000000000, 0.9659258262890683122, 1.000000000000000000, 0.9659258262890683122, 1.000000000000000000, 0.9659258262890683122, 1.000000000000000000, 0.9659258262890683122, 1.000000000000000000, 0.9659258262890683122, 1.000000000000000000, 0.9659258262890683122, 1.000000000000000000, 0.9659258262890683122, 1.000000000000000000, 0.9659258262890683122, 1.000000000000000000, 0.9659258262890683122, 1.000000000000000000, 0.9659258262890683122, 1.000000000000000000, 0.9659258262890683122, 1.000000000000000000, 0.9659258262890683122, 1.000000000000000000, 0.9659258262890683122, 1.000000000000000000, 0.9659258262890683122, 1.000000000000000000, 0.9659258262890683122, 1.000000000000000000, 0.9659258262890683122, 1.000000000000000000, 0.9659258262890683122, 1.000000000000000000, 0.9659258262890683122, 1.000000000000000000, 0.9659258262890683122, 1.000000000000000000, 0.9659258262890683122, 1.000000000000000000, 0.9659258262890683122, 1.000000000000000000, 0.9659258262890683122, 1.000000000000000000, 0.9659258262890683122, 1.000000000000000000, 0.9659258262890683122, 1.000000000000000000, 0.9659258262890683122, 1.000000000000000000, 0.9659258262890683122, 1.000000000000000000, 0.9659258262890683122, 1.000000000000000000, 0.9659258262890683122, 1.000000000000000000, 0.9659258262890683122, 1.000000000000000000, 0.9659258262890683122, 1.000000000000000000, 0.9659258262890683122, 1.000000000000000000, 0.9659258262890683122, 1.000000000000000000, 0.9659258262890683122, 1.000000000000000000, 0.9659258262890683122, 1.000000000000000000, 0.9659258262890683122, 1.000000000000000000, 0.9659258262890683122, 1.000000000000000000, 0.9659258262890683122, 1.000000000000000000, 0.9659258262890683122, 1.000000000000000000, 0.9659258262890683122, 1.000000000000000000, 0.9659258262890683122, 1.000000000000000000, 0.9659258262890683122, 1.000000000000000000, 0.9659258262890683122, 1.000000000000000000, 0.9659258262890683122, 1.000000000000000000, 0.9659258262890683122, 1.000000000000000000, 0.9659258262890683122, 1.000000000000000000, 0.9659258262890683122, 1.000000000000000000, 0.9659258262890683122, 1.000000000000000000, 0.9659258262890683122, 1.000000000000000000, 0.9659258262890683122, 1.000000000000000000, 0.9659258262890683122, 1.000000000000000000, 0.9659258262890683122, 1.000000000000000000, 0.9659258262890683122, 1.000000000000000000, 0.9659258262890683122, 1.000000000000000000, 0.9659258262890683122, 1.000000000000000000, 0.9659258262890683122, 1.000000000000000000, 0.9659258262890683122, 1.000000000000000000, 0.9659258262890683122, 1.000000000000000000, 0.9659258262890683122, 1.000000000000000000, 0.9659258262890683122, 1.000000000000000000, 0.9659258262890683122, 1.000000000000000000, 0.9659258262890683122, 1.000000000000000000, 0.9659258262890683122, 1.000000000000000000, 0.9659258262890683122, 1.000000000000000000, 0.9659258262890683122, 1.000000000000000000, 0.9659258262890683122, 1.000000000000000000, 0.9659258262890683122, 1.000000000000000000, 0.9659258262890683122, 1.000000000000000000, 0.9659258262890683122, 1.000000000000000000, 0.9659258262890683122, 1.000000000000000000, 0.9659258262890683122, 1.000000000000000000, 0.9659258262890683122, 1.000000000000000000, 0.9659258262890683122, 1.000000000000000000, 0.9659258262890683122, 1.000000000000000000, 0.9659258262890683122, 1.000000000000000000, 0.9659258262890683122, 1.000000000000000000, 0.9659258262890683122, 1.000000000000000000, 0.9659258262890683122, 1.000000000000000000, 0.9659258262890683122, 1.000000000000000000, 0.9659258262890683122, 1.000000000000000000, 0.9659258262890683122, 1.000000000000000000, 0.9659258262890683122, 1.000000000000000000, 0.9659258262890683122, 1.000000000000000000, 0.9659258262890683122, 1.000000000000000000, 0.9659258262890683122, 1.000000000000000000, 0.9659258262890683122, 1.000000000000000000, 0.9659258262890683122, 1.000000000000000000, 0.9659258262890683122, 1.000000000000000000, 0.9659258262890683122, 1.000000000000000000, 0.9659258262890683122, 1.000000000000000000, 0.9659258262890683122, 1.000000000000000000, 0.9659258262890683122, 1.000000000000000000, 0.9659258262890683122, 1.000000000000000000, 0.9659258262890683122, 1.000000000000000000, 0.9659258262890683122, 1.000000000000000000, 0.9659258262890683122, 1.000000000000000000, 0.9659258262890683122, 1.000000000000000000, 0.9659258262890683122, 1.000000000000000000, 0.9659258262890683122, 1.000000000000000000, 0.9659258262890683122, 1.000000000000000000, 0.9659258262890683122, 1.000000000000000000, 0.9659258262890683122, 1.000000000000000000, 0.9659258262890683122, 1.000000000000000000, 0.9659258262890683122, 1.000000000000000000, 0.9659258262890683122, 1.000000000000000000, 0.9659258262890683122, 1.000000000000000000, 0.9659258262890683122, 1.000000000000000000, 0.9659258262890683122, 1.000000000000000000, 0.9659258262890683122, 1.000000000000000000, 0.9659258262890683122, 1.000000000000000000, 0.9659258262890683122, 1.000000000000000000, 0.9659258262890683122, 1.000000000000000000, 0.9659258262890683122, 1.000000000000000000, 0.9659258262890683122, 1.000000000000000000, 0.9659258262890683122, 1.000000000000000000, 0.9659258262890683122, 1.000000000000000000, 0.9659258262890683122, 1.000000000000000000, 0.9659258262890683122, 1.000000000000000000, 0.9659258262890683122, 1.000000000000000000, 0.9659258262890683122, 1.000000000000000000, 0.9659258262890683122, 1.000000000000000000, 0.9659258262890683122, 1.000000000000000000, 0.9659258262890683122, 1.000000000000000000, 0.9659258262890683122, 1.000000000000000000, 0.9659258262890683122, 1.000000000000000000) ) ) 
 REPRESENTATION_ITEM ( '' )  SURFACE ( )  );
#33749=CARTESIAN_POINT ( 'NONE',  ( -0.05219959533909027116, -19.03943276465977164, 42.49890960531435269 ) ) ;
#33750=CARTESIAN_POINT ( 'NONE',  ( 4.379528057220092307, 16.55341960407617563, 82.29275706135234714 ) ) ;
#33751=CARTESIAN_POINT ( 'NONE',  ( 5.823673210054125526, 21.52544592524343514, 104.7905762719810241 ) ) ;
#33752=CARTESIAN_POINT ( 'NONE',  ( -14.34966873604960291, -8.224510206698953496, 51.66557627198102409 ) ) ;
#33753=CARTESIAN_POINT ( 'NONE',  ( -9.474510206698964154, 16.51473224551069663, 70.41557627198102409 ) ) ;
#33754=CARTESIAN_POINT ( 'NONE',  ( -8.224510206698735004, -14.34966873604973081, 74.58442372801901854 ) ) ;
#33755=CARTESIAN_POINT ( 'NONE',  ( -4.379528057220086978, -16.55341960407618274, 19.79275706135235069 ) ) ;
#33756=CARTESIAN_POINT ( 'NONE',  ( -21.52544592524343514, 5.823673210054127303, 111.0405762719810525 ) ) ;
#33757=CARTESIAN_POINT ( 'NONE',  ( -16.55341960407611168, -4.379528057220339221, 41.45724293864769550 ) ) ;
#33759=CARTESIAN_POINT ( 'NONE',  ( -17.12812012977028431, 6.668231424565926879, 73.64051240676856480 ) ) ;
#33760=CARTESIAN_POINT ( 'NONE',  ( -5.823673210054116645, -21.52544592524344225, 87.29057627198103830 ) ) ;
#33761=CARTESIAN_POINT ( 'NONE',  ( 4.379528057220339221, -16.55341960407611168, 27.70724293864769905 ) ) ;
#33764=CARTESIAN_POINT ( 'NONE',  ( -21.52544592524343514, 5.823673210054127303, 106.0405762719810525 ) ) ;
#33765=CARTESIAN_POINT ( 'NONE',  ( 5.153800228976335163, 19.02544592524342804, 114.7905762719810241 ) ) ;
#33766=CARTESIAN_POINT ( 'NONE',  ( 21.52544592524334988, 5.823673210054432836, 26.45942372801901854 ) ) ;
#33767=CARTESIAN_POINT ( 'NONE',  ( -0.05219959533910754901, -16.53943276465976808, 47.49890960531435979 ) ) ;
#33768=CARTESIAN_POINT ( 'NONE',  ( 8.224510206698742110, 14.34966873604972548, 52.08442372801901854 ) ) ;
#33769=CARTESIAN_POINT ( 'NONE',  ( -9.564922557960796823, -16.46253265017161027, 52.08224293864768839 ) ) ;
#33770=CARTESIAN_POINT ( 'NONE',  ( -19.05341960407617563, 5.049401038297882671, 48.54275706135233293 ) ) ;
#33771=CARTESIAN_POINT ( 'NONE',  ( -5.049401038298153566, 19.05341960407611168, 85.20724293864766707 ) ) ;
#33773=CARTESIAN_POINT ( 'NONE',  ( -0.05219959533907301413, -21.53943276465977519, 37.49890960531436690 ) ) ;
#33775=CARTESIAN_POINT ( 'NONE',  ( -13.97604488694547697, 13.89961937509957934, 113.1260903946856757 ) ) ;
#33776=CARTESIAN_POINT ( 'NONE',  ( -16.46253265017146816, -9.564922557961047289, 69.16775706135233293 ) ) ;
#33777=CARTESIAN_POINT ( 'NONE',  ( 5.823673210054125526, 21.52544592524343514, 99.79057627198103830 ) ) ;
#33778=CARTESIAN_POINT ( 'NONE',  ( -14.34966873604960291, -8.224510206698953496, 31.66557627198102054 ) ) ;
#33779=CARTESIAN_POINT ( 'NONE',  ( -0.05219959533909027116, -19.03943276465977164, 77.49890960531435269 ) ) ;
#33780=CARTESIAN_POINT ( 'NONE',  ( 5.823673210054125526, 21.52544592524343514, 59.79057627198103120 ) ) ;
#33781=CARTESIAN_POINT ( 'NONE',  ( 18.67979575497178502, 10.72451020669898547, 94.16557627198103830 ) ) ;
#33782=CARTESIAN_POINT ( 'NONE',  ( 12.14591786802327356, -12.06949235617739191, 20.62609039468568639 ) ) ;
#33783=CARTESIAN_POINT ( 'NONE',  ( -19.03943276465977164, 0.05219959533909376836, 116.2489096053143669 ) ) ;
#33784=CARTESIAN_POINT ( 'NONE',  ( -18.62759615963255300, -10.81492255796106328, 94.16775706135237556 ) ) ;
#33785=CARTESIAN_POINT ( 'NONE',  ( 5.049401038298161559, -19.05341960407611168, 92.70724293864769550 ) ) ;
#33786=CARTESIAN_POINT ( 'NONE',  ( 9.474510206698971260, -16.51473224551069308, 27.91557627198103120 ) ) ;
#33787=CARTESIAN_POINT ( 'NONE',  ( 5.049401038298161559, -19.05341960407611168, 77.70724293864765286 ) ) ;
#33788=CARTESIAN_POINT ( 'NONE',  ( 0.05219959533910956823, 16.53943276465976808, 99.99890960531436690 ) ) ;
#33789=CARTESIAN_POINT ( 'NONE',  ( -16.46253265017160317, 9.564922557960807481, 60.83224293864769550 ) ) ;
#33790=CARTESIAN_POINT ( 'NONE',  ( 4.379528057220092307, 16.55341960407617563, 22.29275706135235069 ) ) ;
#33791=CARTESIAN_POINT ( 'NONE',  ( 17.50000000000000000, -5.499999999999992895, 86.21769037696435589 ) ) ;
#33792=CARTESIAN_POINT ( 'NONE',  ( -9.474510206698964154, 16.51473224551069663, 70.41557627198102409 ) ) ;
#33793=CARTESIAN_POINT ( 'NONE',  ( -18.62759615963255300, -10.81492255796106328, 94.16775706135237556 ) ) ;
#33794=CARTESIAN_POINT ( 'NONE',  ( -0.05219959533907301413, -21.53943276465977519, 22.49890960531436335 ) ) ;
#33795=CARTESIAN_POINT ( 'NONE',  ( 8.314922557961029526, -14.29746914071037800, 95.41775706135234714 ) ) ;
#33797=CARTESIAN_POINT ( 'NONE',  ( 16.46253265017146816, 9.564922557961045513, 66.66775706135233293 ) ) ;
#33798=CARTESIAN_POINT ( 'NONE',  ( -19.03943276465977164, -0.05219959533935918106, 18.75109039468567218 ) ) ;
#33799=CARTESIAN_POINT ( 'NONE',  ( -16.52216118717206328, -7.221426719304521846, 46.07599021046992505 ) ) ;
#33800=CARTESIAN_POINT ( 'NONE',  ( 9.474510206698971260, -16.51473224551069308, 27.91557627198103120 ) ) ;
#33801=CARTESIAN_POINT ( 'NONE',  ( 8.224510206698953496, -14.34966873604960469, 42.91557627198103120 ) ) ;
#33803=CARTESIAN_POINT ( 'NONE',  ( 4.483927247898790824, -16.52544592524335698, 105.2094237280190328 ) ) ;
#33805=CARTESIAN_POINT ( 'NONE',  ( 14.34966873604972726, -8.224510206698740333, 80.83442372801901854 ) ) ;
#33806=CARTESIAN_POINT ( 'NONE',  ( 5.049401038298161559, -19.05341960407611168, 32.70724293864768129 ) ) ;
#33807=CARTESIAN_POINT ( 'NONE',  ( 10.81492255796106328, -18.62759615963255655, 95.41775706135234714 ) ) ;
#33808=CARTESIAN_POINT ( 'NONE',  ( -19.05341960407617563, 5.049401038297882671, 98.54275706135233293 ) ) ;
#33809=CARTESIAN_POINT ( 'NONE',  ( 21.52544592524334988, 5.823673210054432836, 76.45942372801901854 ) ) ;
#33810=CARTESIAN_POINT ( 'NONE',  ( 9.564922557961047289, -16.46253265017146816, 55.41775706135234003 ) ) ;
#33811=CARTESIAN_POINT ( 'NONE',  ( -0.05219959533909027116, -19.03943276465977164, 77.49890960531435269 ) ) ;
#33812=CARTESIAN_POINT ( 'NONE',  ( 9.474510206698971260, -16.51473224551069308, 72.91557627198102409 ) ) ;
#33813=CARTESIAN_POINT ( 'NONE',  ( 16.88567814943160883, 6.947325034625710494, 73.79001122652587696 ) ) ;
#33814=CARTESIAN_POINT ( 'NONE',  ( 16.55341960407611168, 4.379528057220329451, 63.95724293864770260 ) ) ;
#33815=CARTESIAN_POINT ( 'NONE',  ( -21.55341960407610458, -5.719274019375992779, 61.45724293864770260 ) ) ;
#33816=CARTESIAN_POINT ( 'NONE',  ( 9.474510206698971260, -16.51473224551069308, 42.91557627198103120 ) ) ;
#33817=CARTESIAN_POINT ( 'NONE',  ( -21.53943276465977519, 0.05219959533907696930, 86.24890960531436690 ) ) ;
#33818=CARTESIAN_POINT ( 'NONE',  ( -4.483927247898782831, 16.52544592524335698, 77.70942372801900433 ) ) ;
#33819=EDGE_CURVE ( 'NONE', #190522, #188457, #179887, .T. ) ;
#33821=CARTESIAN_POINT ( 'NONE',  ( 12.06949235617757843, -12.14591786802309237, 73.12390960531436690 ) ) ;
#33823=CARTESIAN_POINT ( 'NONE',  ( -13.97604488694527625, -13.89961937509977652, 46.87390960531435979 ) ) ;
#33824=CARTESIAN_POINT ( 'NONE',  ( -12.14591786802309592, -12.06949235617757132, 111.8739096053143669 ) ) ;
#33825=CARTESIAN_POINT ( 'NONE',  ( 0.05219959533936267826, -19.03943276465977164, 70.00109039468566152 ) ) ;
#33826=CARTESIAN_POINT ( 'NONE',  ( 16.52544592524342804, -4.483927247898539470, 73.54057627198102409 ) ) ;
#33827=CARTESIAN_POINT ( 'NONE',  ( 5.823673210054444382, -21.52544592524334988, 40.20942372801901854 ) ) ;
#33828=CARTESIAN_POINT ( 'NONE',  ( -19.05341960407611168, -5.049401038298163336, 21.45724293864768839 ) ) ;
#33829=CARTESIAN_POINT ( 'NONE',  ( 21.53943276465977519, -0.05219959533907433946, 98.74890960531438111 ) ) ;
#33830=CARTESIAN_POINT ( 'NONE',  ( 16.51473224551069308, 9.474510206698969483, 114.1655762719810241 ) ) ;
#33831=CARTESIAN_POINT ( 'NONE',  ( -4.379528057220328563, 16.55341960407611168, 85.20724293864770971 ) ) ;
#33833=CARTESIAN_POINT ( 'NONE',  ( -19.03943276465977164, 0.05219959533909376836, 41.24890960531435269 ) ) ;
#33835=CARTESIAN_POINT ( 'NONE',  ( 19.05341960407617918, -5.049401038297876454, 86.04275706135233293 ) ) ;
#33836=CARTESIAN_POINT ( 'NONE',  ( -5.823673210054431948, 21.52544592524334988, 37.70942372801900433 ) ) ;
#33837=CARTESIAN_POINT ( 'NONE',  ( 5.153800228976335163, 19.02544592524342804, 69.79057627198103830 ) ) ;
#33838=CARTESIAN_POINT ( 'NONE',  ( 5.049401038297881783, 19.05341960407617563, 57.29275706135231871 ) ) ;
#33839=CARTESIAN_POINT ( 'NONE',  ( 5.049401038298161559, -19.05341960407611168, 47.70724293864770260 ) ) ;
#33840=CARTESIAN_POINT ( 'NONE',  ( 14.34966873604960469, 8.224510206698951720, 59.16557627198103120 ) ) ;
#33841=CARTESIAN_POINT ( 'NONE',  ( -16.53943276465976808, 0.05219959533911058130, 61.24890960531435979 ) ) ;
#33842=CARTESIAN_POINT ( 'NONE',  ( 9.564922557960805705, 16.46253265017160317, 69.58224293864770971 ) ) ;
#33843=CARTESIAN_POINT ( 'NONE',  ( -18.62759615963270932, 10.81492255796079327, 100.8322429386477097 ) ) ;
#33844=CARTESIAN_POINT ( 'NONE',  ( -19.02544592524342804, 5.153800228976336051, 76.04057627198102409 ) ) ;
#33845=CARTESIAN_POINT ( 'NONE',  ( -10.72451020669898014, 18.67979575497178502, 85.41557627198102409 ) ) ;
#33846=CARTESIAN_POINT ( 'NONE',  ( -13.89961937509957401, -13.97604488694547875, 19.37609039468566507 ) ) ;
#33847=CARTESIAN_POINT ( 'NONE',  ( -13.97604488694527625, -13.89961937509977652, 36.87390960531436690 ) ) ;
#33848=CARTESIAN_POINT ( 'NONE',  ( 14.34966873604972726, -8.224510206698740333, 105.8344237280190328 ) ) ;
#33849=CARTESIAN_POINT ( 'NONE',  ( -0.05219959533910754901, -16.53943276465976808, 102.4989096053143811 ) ) ;
#33850=CARTESIAN_POINT ( 'NONE',  ( -19.02544592524334988, -5.153800228976617603, 103.9594237280190043 ) ) ;
#33852=CARTESIAN_POINT ( 'NONE',  ( 5.823673210054444382, -21.52544592524334988, 35.20942372801901854 ) ) ;
#33853=CARTESIAN_POINT ( 'NONE',  ( -19.05341960407617563, 5.049401038297882671, 48.54275706135233293 ) ) ;
#33854=CARTESIAN_POINT ( 'NONE',  ( 0.05219959533910956823, 16.53943276465976808, 24.99890960531435624 ) ) ;
#33855=CARTESIAN_POINT ( 'NONE',  ( -5.719274019375978568, 21.55341960407610458, 75.20724293864769550 ) ) ;
#33856=CARTESIAN_POINT ( 'NONE',  ( 9.474510206698971260, -16.51473224551069308, 97.91557627198102409 ) ) ;
#33857=CARTESIAN_POINT ( 'NONE',  ( -4.379528057220328563, 16.55341960407611168, 50.20724293864769550 ) ) ;
#33858=CARTESIAN_POINT ( 'NONE',  ( -19.02544592524342804, 5.153800228976336051, 26.04057627198103120 ) ) ;
#33859=CARTESIAN_POINT ( 'NONE',  ( 19.02544592524343514, -5.153800228976328945, 28.54057627198102409 ) ) ;
#33860=CARTESIAN_POINT ( 'NONE',  ( -9.474510206698720793, -16.51473224551083518, 29.58442372801900433 ) ) ;
#33861=CARTESIAN_POINT ( 'NONE',  ( -8.314922557961024197, 14.29746914071037800, 92.91775706135236135 ) ) ;
#33862=CARTESIAN_POINT ( 'NONE',  ( 15.72974639402176855, 15.80617190586768217, 36.87609039468568994 ) ) ;
#33863=CARTESIAN_POINT ( 'NONE',  ( 12.14591786802327356, -12.06949235617739191, 45.62609039468567573 ) ) ;
#33864=CARTESIAN_POINT ( 'NONE',  ( 15.80617190586746368, 15.72974639402197994, 29.37390960531435269 ) ) ;
#33865=CARTESIAN_POINT ( 'NONE',  ( -0.05219959533909027116, -19.03943276465977164, 52.49890960531436690 ) ) ;
#33866=CARTESIAN_POINT ( 'NONE',  ( 10.72451020669871369, 18.67979575497193778, 92.08442372801901854 ) ) ;
#33867=CARTESIAN_POINT ( 'NONE',  ( -19.02544592524342804, 5.153800228976336051, 76.04057627198102409 ) ) ;
#33868=AXIS2_PLACEMENT_3D ( 'NONE', #28121, #73617, #42281 ) ;
#33869=CARTESIAN_POINT ( 'NONE',  ( 4.483927247898790824, -16.52544592524335698, 65.20942372801901854 ) ) ;
#33870=CARTESIAN_POINT ( 'NONE',  ( 4.483927247898545687, 16.52544592524342804, 109.7905762719810383 ) ) ;
#33871=CARTESIAN_POINT ( 'NONE',  ( -14.34966873604960291, -8.224510206698953496, 21.66557627198102409 ) ) ;
#33873=CARTESIAN_POINT ( 'NONE',  ( -18.67979575497193778, 10.72451020669871902, 68.33442372801900433 ) ) ;
#33874=CARTESIAN_POINT ( 'NONE',  ( -9.474510206698964154, 16.51473224551069663, 95.41557627198102409 ) ) ;
#33875=CARTESIAN_POINT ( 'NONE',  ( 16.46253265017160672, -9.564922557960803928, 78.33224293864769550 ) ) ;
#33876=CARTESIAN_POINT ( 'NONE',  ( 9.564922557960805705, 16.46253265017160317, 109.5822429386476955 ) ) ;
#33877=CARTESIAN_POINT ( 'NONE',  ( 14.34966873604960469, 8.224510206698951720, 59.16557627198103120 ) ) ;
#33878=CARTESIAN_POINT ( 'NONE',  ( 0.05219959533910956823, 16.53943276465976808, 24.99890960531435624 ) ) ;
#33879=CARTESIAN_POINT ( 'NONE',  ( 12.14591786802309770, 12.06949235617756955, 44.37390960531435979 ) ) ;
#33880=CARTESIAN_POINT ( 'NONE',  ( 16.55341960407618274, -4.379528057220086978, 46.04275706135234714 ) ) ;
#33883=CARTESIAN_POINT ( 'NONE',  ( 16.46253265017146816, 9.564922557961045513, 36.66775706135233293 ) ) ;
#33884=CARTESIAN_POINT ( 'NONE',  ( 19.03943276465977164, -0.05219959533909143690, 73.74890960531435269 ) ) ;
#33885=CARTESIAN_POINT ( 'NONE',  ( 19.03943276465977164, 0.05219959533936151252, 56.25109039468566863 ) ) ;
#33889=CARTESIAN_POINT ( 'NONE',  ( -19.03943276465977164, -0.05219959533935918106, 88.75109039468567573 ) ) ;
#33890=CARTESIAN_POINT ( 'NONE',  ( 16.53943276465976808, 0.05219959533934440121, 86.25109039468568994 ) ) ;
#33891=CARTESIAN_POINT ( 'NONE',  ( -19.02544592524342804, 5.153800228976336051, 101.0405762719810241 ) ) ;
#33892=CARTESIAN_POINT ( 'NONE',  ( -21.53943276465977519, -0.05219959533937600094, 23.75109039468567929 ) ) ;
#33893=CARTESIAN_POINT ( 'NONE',  ( 0.05219959533936267826, -19.03943276465977164, 95.00109039468567573 ) ) ;
#33894=CARTESIAN_POINT ( 'NONE',  ( -17.49999999999999645, 5.499999999999997335, 35.79690382534171533 ) ) ;
#33895=CARTESIAN_POINT ( 'NONE',  ( -19.02544592524342804, 5.153800228976336051, 51.04057627198103120 ) ) ;
#33896=CARTESIAN_POINT ( 'NONE',  ( -9.474510206698964154, 16.51473224551069663, 100.4155762719810241 ) ) ;
#33897=CARTESIAN_POINT ( 'NONE',  ( 12.14591786802309770, 12.06949235617756955, 64.37390960531435269 ) ) ;
#33898=CARTESIAN_POINT ( 'NONE',  ( -13.89961937509977652, 13.97604488694528158, 50.62390960531435979 ) ) ;
#33899=CARTESIAN_POINT ( 'NONE',  ( 9.474510206698971260, -16.51473224551069308, 62.91557627198102409 ) ) ;
#33900=CARTESIAN_POINT ( 'NONE',  ( -19.03943276465977164, -0.05219959533935918106, 68.75109039468566152 ) ) ;
#33901=CARTESIAN_POINT ( 'NONE',  ( -19.05341960407617563, 5.049401038297882671, 33.54275706135231871 ) ) ;
#33902=CARTESIAN_POINT ( 'NONE',  ( -16.51473224551069308, -9.474510206698971260, 66.66557627198102409 ) ) ;
#33903=CARTESIAN_POINT ( 'NONE',  ( 10.72451020669898902, -18.67979575497178502, 72.91557627198103830 ) ) ;
#33904=CARTESIAN_POINT ( 'NONE',  ( 16.55341960407611168, 4.379528057220329451, 68.95724293864769550 ) ) ;
#33905=CARTESIAN_POINT ( 'NONE',  ( -19.03943276465977164, -0.05219959533935918106, 38.75109039468566152 ) ) ;
#33907=CARTESIAN_POINT ( 'NONE',  ( 5.823673210054125526, 21.52544592524343514, 49.79057627198102409 ) ) ;
#33908=CARTESIAN_POINT ( 'NONE',  ( 5.719274019375991003, -21.55341960407610458, 27.70724293864769905 ) ) ;
#33909=CARTESIAN_POINT ( 'NONE',  ( -9.564922557960796823, -16.46253265017161027, 57.08224293864769550 ) ) ;
#33910=CARTESIAN_POINT ( 'NONE',  ( 5.153800228976335163, 19.02544592524342804, 44.79057627198103830 ) ) ;
#33911=CARTESIAN_POINT ( 'NONE',  ( 0.05219959533910956823, 16.53943276465976808, 104.9989096053143669 ) ) ;
#33913=CARTESIAN_POINT ( 'NONE',  ( -10.72451020669898014, 18.67979575497178502, 115.4155762719810241 ) ) ;
#33915=CARTESIAN_POINT ( 'NONE',  ( 0.05219959533937995610, -21.53943276465977519, 25.00109039468567218 ) ) ;
#33916=CARTESIAN_POINT ( 'NONE',  ( 5.153800228976335163, 19.02544592524342804, 24.79057627198102765 ) ) ;
#33917=CARTESIAN_POINT ( 'NONE',  ( -10.81492255796078084, -18.62759615963271287, 97.08224293864770971 ) ) ;
#33918=CARTESIAN_POINT ( 'NONE',  ( -5.153800228976607833, 19.02544592524334988, 42.70942372801901143 ) ) ;
#33919=CARTESIAN_POINT ( 'NONE',  ( 18.22780087662122384, -5.500000000000022204, 76.01540105326107266 ) ) ;
#33920=CARTESIAN_POINT ( 'NONE',  ( 19.25663599770060586, -5.499999999999438671, 76.49419308057197497 ) ) ;
#33922=CARTESIAN_POINT ( 'NONE',  ( -4.483927247898782831, 16.52544592524335698, 42.70942372801901854 ) ) ;
#33923=CARTESIAN_POINT ( 'NONE',  ( -12.06949235617756955, 12.14591786802309770, 115.6239096053143669 ) ) ;
#33924=LINE ( 'NONE', #95581, #106449 ) ;
#33925=CARTESIAN_POINT ( 'NONE',  ( 19.03943276465977164, -0.05219959533909143690, 68.74890960531436690 ) ) ;
#33926=CARTESIAN_POINT ( 'NONE',  ( 16.55341960407611168, 4.379528057220329451, 103.9572429386476813 ) ) ;
#33927=CARTESIAN_POINT ( 'NONE',  ( -5.719274019375978568, 21.55341960407610458, 40.20724293864769550 ) ) ;
#33928=CARTESIAN_POINT ( 'NONE',  ( -4.483927247898539470, -16.52544592524342804, 77.29057627198102409 ) ) ;
#33929=CARTESIAN_POINT ( 'NONE',  ( -0.05219959533934338120, 16.53943276465976808, 32.50109039468568284 ) ) ;
#33930=CARTESIAN_POINT ( 'NONE',  ( -0.05219959533937732626, 21.53943276465977519, 92.50109039468567573 ) ) ;
#33931=CARTESIAN_POINT ( 'NONE',  ( -19.05341960407611168, -5.049401038298163336, 21.45724293864768839 ) ) ;
#33932=CARTESIAN_POINT ( 'NONE',  ( 16.52544592524335698, 4.483927247898782831, 106.4594237280190328 ) ) ;
#33933=CARTESIAN_POINT ( 'NONE',  ( -16.52544592524342804, 4.483927247898546575, 46.04057627198103830 ) ) ;
#33934=CARTESIAN_POINT ( 'NONE',  ( -13.97604488694527625, -13.89961937509977652, 51.87390960531436690 ) ) ;
#33935=CARTESIAN_POINT ( 'NONE',  ( -18.67979575497193778, 10.72451020669871902, 98.33442372801901854 ) ) ;
#33936=CARTESIAN_POINT ( 'NONE',  ( -21.55341960407610458, -5.719274019375992779, 106.4572429386477097 ) ) ;
#33937=CARTESIAN_POINT ( 'NONE',  ( -5.823673210054431948, 21.52544592524334988, 67.70942372801901854 ) ) ;
#33938=CARTESIAN_POINT ( 'NONE',  ( -12.06949235617739369, -12.14591786802326823, 34.37609039468568284 ) ) ;
#33939=CARTESIAN_POINT ( 'NONE',  ( 0.05219959533910956823, 16.53943276465976808, 79.99890960531435269 ) ) ;
#33940=CARTESIAN_POINT ( 'NONE',  ( 10.72451020669871369, 18.67979575497193778, 87.08442372801901854 ) ) ;
#33941=CARTESIAN_POINT ( 'NONE',  ( -12.14591786802326823, 12.06949235617739902, 108.1260903946856757 ) ) ;
#33942=CARTESIAN_POINT ( 'NONE',  ( -19.05341960407611168, -5.049401038298163336, 21.45724293864768839 ) ) ;
#33944=CARTESIAN_POINT ( 'NONE',  ( -8.314922557960811034, -14.29746914071050412, 37.08224293864768129 ) ) ;
#33945=CARTESIAN_POINT ( 'NONE',  ( -14.34966873604972548, 8.224510206698743886, 73.33442372801901854 ) ) ;
#33946=CARTESIAN_POINT ( 'NONE',  ( 5.153800228976335163, 19.02544592524342804, 84.79057627198099567 ) ) ;
#33947=CARTESIAN_POINT ( 'NONE',  ( 19.05341960407611168, 5.049401038298154454, 93.95724293864769550 ) ) ;
#33948=CARTESIAN_POINT ( 'NONE',  ( -15.72974639402176322, -15.80617190586768395, 104.3760903946856899 ) ) ;
#33949=CARTESIAN_POINT ( 'NONE',  ( -8.224510206698735004, -14.34966873604973081, 104.5844237280190185 ) ) ;
#33950=CARTESIAN_POINT ( 'NONE',  ( -0.05219959533910754901, -16.53943276465976808, 67.49890960531436690 ) ) ;
#33951=CARTESIAN_POINT ( 'NONE',  ( -19.05341960407611168, -5.049401038298163336, 81.45724293864769550 ) ) ;
#33953=CARTESIAN_POINT ( 'NONE',  ( 4.379528057220092307, 16.55341960407617563, 32.29275706135235424 ) ) ;
#33954=CARTESIAN_POINT ( 'NONE',  ( -16.46253265017160317, 9.564922557960807481, 30.83224293864769550 ) ) ;
#33955=CARTESIAN_POINT ( 'NONE',  ( 19.03943276465977164, -0.05219959533909143690, 93.74890960531435269 ) ) ;
#33956=CARTESIAN_POINT ( 'NONE',  ( -0.05219959533934338120, 16.53943276465976808, 27.50109039468567929 ) ) ;
#33958=CARTESIAN_POINT ( 'NONE',  ( -19.02544592524334988, -5.153800228976617603, 23.95942372801900078 ) ) ;
#33959=CARTESIAN_POINT ( 'NONE',  ( 16.55341960407618274, -4.379528057220086978, 91.04275706135236135 ) ) ;
#33960=CARTESIAN_POINT ( 'NONE',  ( -19.05341960407617563, 5.049401038297882671, 108.5427570613523187 ) ) ;
#33961=CARTESIAN_POINT ( 'NONE',  ( -16.46253265017160317, 9.564922557960807481, 35.83224293864768839 ) ) ;
#33962=CARTESIAN_POINT ( 'NONE',  ( -14.29746914071037622, -8.314922557961029526, 79.16775706135234714 ) ) ;
#33963=CARTESIAN_POINT ( 'NONE',  ( 16.52544592524335698, 4.483927247898782831, 66.45942372801903275 ) ) ;
#33964=CARTESIAN_POINT ( 'NONE',  ( 5.153800228976335163, 19.02544592524342804, 24.79057627198102765 ) ) ;
#33965=CARTESIAN_POINT ( 'NONE',  ( -5.153800228976607833, 19.02544592524334988, 62.70942372801899722 ) ) ;
#33966=VECTOR ( 'NONE', #8413, 1000.000000000000000 ) ;
#33967=CARTESIAN_POINT ( 'NONE',  ( 19.02544592524334988, 5.153800228976608722, 21.45942372801899012 ) ) ;
#33968=CARTESIAN_POINT ( 'NONE',  ( 19.02544592524343514, -5.153800228976328945, 48.54057627198103120 ) ) ;
#33969=CARTESIAN_POINT ( 'NONE',  ( 5.049401038298161559, -19.05341960407611168, 97.70724293864766707 ) ) ;
#33970=CARTESIAN_POINT ( 'NONE',  ( -0.05219959533910754901, -16.53943276465976808, 87.49890960531436690 ) ) ;
#33971=CARTESIAN_POINT ( 'NONE',  ( -9.564922557961040184, 16.46253265017147172, 57.91775706135233293 ) ) ;
#33972=CARTESIAN_POINT ( 'NONE',  ( 10.72451020669898902, -18.67979575497178502, 47.91557627198102409 ) ) ;
#33973=CARTESIAN_POINT ( 'NONE',  ( -18.62759615963255300, -10.81492255796106328, 109.1677570613523613 ) ) ;
#33974=CARTESIAN_POINT ( 'NONE',  ( 0.05219959533909260263, 19.03943276465977164, 94.99890960531436690 ) ) ;
#33976=CARTESIAN_POINT ( 'NONE',  ( -21.53943276465977519, -0.05219959533937600094, 108.7510903946857042 ) ) ;
#33977=CARTESIAN_POINT ( 'NONE',  ( 5.719274019375991003, -21.55341960407610458, 67.70724293864769550 ) ) ;
#33978=CARTESIAN_POINT ( 'NONE',  ( -19.03943276465977164, 0.05219959533909376836, 116.2489096053143669 ) ) ;
#33979=CARTESIAN_POINT ( 'NONE',  ( -0.05219959533936034679, 19.03943276465977164, 82.50109039468567573 ) ) ;
#33980=CARTESIAN_POINT ( 'NONE',  ( -13.97604488694527625, -13.89961937509977652, 111.8739096053143243 ) ) ;
#33981=CARTESIAN_POINT ( 'NONE',  ( -16.53943276465976808, -0.05219959533934237506, 18.75109039468568639 ) ) ;
#33982=CARTESIAN_POINT ( 'NONE',  ( -16.53943276465976808, 0.05219959533911058130, 116.2489096053143669 ) ) ;
#33983=CARTESIAN_POINT ( 'NONE',  ( 19.02544592524343514, -5.153800228976328945, 83.54057627198100988 ) ) ;
#33984=CARTESIAN_POINT ( 'NONE',  ( 21.53943276465977519, -0.05219959533907433946, 78.74890960531436690 ) ) ;
#33985=CARTESIAN_POINT ( 'NONE',  ( -14.29746914071037622, -8.314922557961029526, 49.16775706135234003 ) ) ;
#33986=CARTESIAN_POINT ( 'NONE',  ( 18.62759615963255655, 10.81492255796105972, 46.66775706135234714 ) ) ;
#33987=CARTESIAN_POINT ( 'NONE',  ( 0.05219959533937995610, -21.53943276465977519, 100.0010903946857042 ) ) ;
#33988=CARTESIAN_POINT ( 'NONE',  ( -12.14591786802326823, 12.06949235617739902, 93.12609039468568994 ) ) ;
#33989=CARTESIAN_POINT ( 'NONE',  ( -0.05219959533909027116, -19.03943276465977164, 92.49890960531436690 ) ) ;
#33990=CARTESIAN_POINT ( 'NONE',  ( -16.52544592524342804, 4.483927247898546575, 91.04057627198103830 ) ) ;
#33991=CARTESIAN_POINT ( 'NONE',  ( 0.05219959533934541429, -16.53943276465976808, 110.0010903946856757 ) ) ;
#33992=CARTESIAN_POINT ( 'NONE',  ( 9.474510206698729675, 16.51473224551082808, 67.08442372801900433 ) ) ;
#33993=CARTESIAN_POINT ( 'NONE',  ( 21.52544592524334988, 5.823673210054432836, 46.45942372801901854 ) ) ;
#33994=CARTESIAN_POINT ( 'NONE',  ( 16.51473224551083163, -9.474510206698727899, 25.83442372801900078 ) ) ;
#33995=CARTESIAN_POINT ( 'NONE',  ( -14.34966873604960291, -8.224510206698953496, 91.66557627198103830 ) ) ;
#33996=CARTESIAN_POINT ( 'NONE',  ( 10.72451020669898902, -18.67979575497178502, 22.91557627198102765 ) ) ;
#33997=CARTESIAN_POINT ( 'NONE',  ( -16.52544592524342804, 4.483927247898546575, 26.04057627198103475 ) ) ;
#33998=CARTESIAN_POINT ( 'NONE',  ( -5.719274019375665041, -21.55341960407619695, 79.79275706135236135 ) ) ;
#33999=CARTESIAN_POINT ( 'NONE',  ( -12.14591786802326823, 12.06949235617739902, 58.12609039468568994 ) ) ;
#34000=CARTESIAN_POINT ( 'NONE',  ( 4.483927247898790824, -16.52544592524335698, 105.2094237280190328 ) ) ;
#34001=CARTESIAN_POINT ( 'NONE',  ( 21.52544592524334988, 5.823673210054432836, 56.45942372801902565 ) ) ;
#34003=CARTESIAN_POINT ( 'NONE',  ( -21.55341960407619339, 5.719274019375674811, 28.54275706135234358 ) ) ;
#34004=CARTESIAN_POINT ( 'NONE',  ( 12.14591786802309770, 12.06949235617756955, 109.3739096053143811 ) ) ;
#34005=CARTESIAN_POINT ( 'NONE',  ( -19.02544592524342804, 5.153800228976336051, 31.04057627198102409 ) ) ;
#34006=CARTESIAN_POINT ( 'NONE',  ( -14.29746914071049879, 8.314922557960819915, 70.83224293864770971 ) ) ;
#34007=CARTESIAN_POINT ( 'NONE',  ( -9.474510206698964154, 16.51473224551069663, 70.41557627198102409 ) ) ;
#34008=CARTESIAN_POINT ( 'NONE',  ( -14.34966873604972548, 8.224510206698743886, 108.3344237280190185 ) ) ;
#34009=CARTESIAN_POINT ( 'NONE',  ( 16.46253265017160672, -9.564922557960803928, 43.33224293864769550 ) ) ;
#34010=CARTESIAN_POINT ( 'NONE',  ( -10.72451020669898014, 18.67979575497178502, 55.41557627198102409 ) ) ;
#34011=CARTESIAN_POINT ( 'NONE',  ( -16.52544592524342804, 4.483927247898546575, 91.04057627198103830 ) ) ;
#34013=CARTESIAN_POINT ( 'NONE',  ( 15.80617190586746368, 15.72974639402197994, 94.37390960531436690 ) ) ;
#34014=CARTESIAN_POINT ( 'NONE',  ( 16.46253265017160672, -9.564922557960803928, 98.33224293864769550 ) ) ;
#34015=CARTESIAN_POINT ( 'NONE',  ( 16.46253265017160672, -9.564922557960803928, 48.33224293864769550 ) ) ;
#34016=CARTESIAN_POINT ( 'NONE',  ( 19.02544592524334988, 5.153800228976608722, 96.45942372801897591 ) ) ;
#34017=CARTESIAN_POINT ( 'NONE',  ( -10.72451020669898014, 18.67979575497178502, 45.41557627198103830 ) ) ;
#34018=CARTESIAN_POINT ( 'NONE',  ( 18.67979575497194134, -10.72451020669871369, 65.83442372801900433 ) ) ;
#34019=CARTESIAN_POINT ( 'NONE',  ( 5.049401038298161559, -19.05341960407611168, 52.70724293864767418 ) ) ;
#34020=CARTESIAN_POINT ( 'NONE',  ( -19.05341960407611168, -5.049401038298163336, 86.45724293864769550 ) ) ;
#34021=CARTESIAN_POINT ( 'NONE',  ( 4.379528057220092307, 16.55341960407617563, 62.29275706135236845 ) ) ;
#34022=CARTESIAN_POINT ( 'NONE',  ( 21.53943276465977519, 0.05219959533937863772, 46.25109039468567573 ) ) ;
#34023=CARTESIAN_POINT ( 'NONE',  ( 0.05219959533937995610, -21.53943276465977519, 85.00109039468568994 ) ) ;
#34024=CARTESIAN_POINT ( 'NONE',  ( 10.81492255796078972, 18.62759615963270932, 104.5822429386477097 ) ) ;
#34025=CARTESIAN_POINT ( 'NONE',  ( -0.05219959533937732626, 21.53943276465977519, 37.50109039468568284 ) ) ;
#34026=CARTESIAN_POINT ( 'NONE',  ( -14.29746914071037622, -8.314922557961029526, 64.16775706135234714 ) ) ;
#34027=CARTESIAN_POINT ( 'NONE',  ( 15.80617190586746368, 15.72974639402197994, 64.37390960531435269 ) ) ;
#34028=CARTESIAN_POINT ( 'NONE',  ( 5.049401038297881783, 19.05341960407617563, 37.29275706135232582 ) ) ;
#34029=CARTESIAN_POINT ( 'NONE',  ( 9.474510206698971260, -16.51473224551069308, 67.91557627198102409 ) ) ;
#34030=CARTESIAN_POINT ( 'NONE',  ( 4.483927247898790824, -16.52544592524335698, 110.2094237280190185 ) ) ;
#34031=CARTESIAN_POINT ( 'NONE',  ( 17.72517630440434644, -5.499999999999968026, 83.42175719257211597 ) ) ;
#34032=CARTESIAN_POINT ( 'NONE',  ( 19.02544592524343514, -5.153800228976328945, 108.5405762719810383 ) ) ;
#34034=CARTESIAN_POINT ( 'NONE',  ( -13.89961937509957401, -13.97604488694547875, 79.37609039468567573 ) ) ;
#34036=CARTESIAN_POINT ( 'NONE',  ( -15.80617190586745835, -15.72974639402198527, 56.87390960531436690 ) ) ;
#34037=CARTESIAN_POINT ( 'NONE',  ( -16.52544592524342804, 4.483927247898546575, 36.04057627198102409 ) ) ;
#34038=CARTESIAN_POINT ( 'NONE',  ( -4.379528057220086978, -16.55341960407618274, 19.79275706135235069 ) ) ;
#34039=CARTESIAN_POINT ( 'NONE',  ( 19.03943276465977164, -0.05219959533909143690, 33.74890960531435979 ) ) ;
#34040=CARTESIAN_POINT ( 'NONE',  ( 19.03943276465977164, 0.05219959533936151252, 111.2510903946856757 ) ) ;
#34041=CARTESIAN_POINT ( 'NONE',  ( 18.62759615963271287, -10.81492255796078972, 88.33224293864769550 ) ) ;
#34042=CARTESIAN_POINT ( 'NONE',  ( 5.049401038297881783, 19.05341960407617563, 77.29275706135231871 ) ) ;
#34043=CARTESIAN_POINT ( 'NONE',  ( -12.14591786802326823, 12.06949235617739902, 83.12609039468568994 ) ) ;
#34044=CARTESIAN_POINT ( 'NONE',  ( 5.049401038298161559, -19.05341960407611168, 72.70724293864768129 ) ) ;
#34045=CARTESIAN_POINT ( 'NONE',  ( 12.06949235617757843, -12.14591786802309237, 78.12390960531436690 ) ) ;
#34046=CARTESIAN_POINT ( 'NONE',  ( -13.89961937509977652, 13.97604488694528158, 45.62390960531433848 ) ) ;
#34047=CARTESIAN_POINT ( 'NONE',  ( -12.06949235617756955, 12.14591786802309770, 55.62390960531436690 ) ) ;
#34050=CARTESIAN_POINT ( 'NONE',  ( 14.29746914071049879, -8.314922557960816363, 23.33224293864769194 ) ) ;
#34051=CARTESIAN_POINT ( 'NONE',  ( -16.51473224551069308, -9.474510206698971260, 81.66557627198103830 ) ) ;
#34053=CARTESIAN_POINT ( 'NONE',  ( -5.049401038297874678, -19.05341960407617918, 44.79275706135232582 ) ) ;
#34054=CARTESIAN_POINT ( 'NONE',  ( 16.55341960407618274, -4.379528057220086978, 41.04275706135236135 ) ) ;
#34055=CARTESIAN_POINT ( 'NONE',  ( 10.81492255796078972, 18.62759615963270932, 69.58224293864769550 ) ) ;
#34056=CARTESIAN_POINT ( 'NONE',  ( 16.51473224551083163, -9.474510206698727899, 25.83442372801900078 ) ) ;
#34057=CARTESIAN_POINT ( 'NONE',  ( -19.02544592524342804, 5.153800228976336051, 81.04057627198103830 ) ) ;
#34059=CARTESIAN_POINT ( 'NONE',  ( 5.153800228976335163, 19.02544592524342804, 104.7905762719809957 ) ) ;
#34060=CARTESIAN_POINT ( 'NONE',  ( -5.823673210054431948, 21.52544592524334988, 37.70942372801900433 ) ) ;
#34061=CARTESIAN_POINT ( 'NONE',  ( -16.53943276465976808, 0.05219959533911058130, 106.2489096053143811 ) ) ;
#34062=CARTESIAN_POINT ( 'NONE',  ( 10.72451020669898902, -18.67979575497178502, 102.9155762719810383 ) ) ;
#34063=CARTESIAN_POINT ( 'NONE',  ( -9.564922557960796823, -16.46253265017161027, 77.08224293864769550 ) ) ;
#34065=CARTESIAN_POINT ( 'NONE',  ( 21.55341960407619695, -5.719274019375665929, 31.04275706135234714 ) ) ;
#34066=EDGE_CURVE ( 'NONE', #133123, #126008, #143663, .T. ) ;
#34068=CARTESIAN_POINT ( 'NONE',  ( -19.02544592524342804, 5.153800228976336051, 86.04057627198103830 ) ) ;
#34069=CARTESIAN_POINT ( 'NONE',  ( 19.35633801406909882, -5.499999999999572786, 81.63373818172763663 ) ) ;
#34070=CARTESIAN_POINT ( 'NONE',  ( 0.05219959533909260263, 19.03943276465977164, 39.99890960531436690 ) ) ;
#34071=CARTESIAN_POINT ( 'NONE',  ( -13.97604488694547697, 13.89961937509957934, 113.1260903946856757 ) ) ;
#34073=CARTESIAN_POINT ( 'NONE',  ( 16.53943276465976808, -0.05219959533910856209, 113.7489096053143527 ) ) ;
#34074=CARTESIAN_POINT ( 'NONE',  ( -18.67979575497193778, 10.72451020669871902, 88.33442372801901854 ) ) ;
#34075=CARTESIAN_POINT ( 'NONE',  ( 13.89961937509977652, -13.97604488694527269, 73.12390960531436690 ) ) ;
#34076=CARTESIAN_POINT ( 'NONE',  ( -18.67979575497193778, 10.72451020669871902, 48.33442372801902565 ) ) ;
#34077=CARTESIAN_POINT ( 'NONE',  ( 21.53943276465977519, 0.05219959533937863772, 26.25109039468567573 ) ) ;
#34079=CARTESIAN_POINT ( 'NONE',  ( -5.153800228976328057, -19.02544592524343514, 82.29057627198103830 ) ) ;
#34081=CARTESIAN_POINT ( 'NONE',  ( -14.34966873604972548, 8.224510206698743886, 43.33442372801901143 ) ) ;
#34082=CARTESIAN_POINT ( 'NONE',  ( -0.05219959533907301413, -21.53943276465977519, 37.49890960531436690 ) ) ;
#34083=CARTESIAN_POINT ( 'NONE',  ( 10.81492255796106328, -18.62759615963255655, 75.41775706135233293 ) ) ;
#34085=CARTESIAN_POINT ( 'NONE',  ( -5.153800228976607833, 19.02544592524334988, 107.7094237280189759 ) ) ;
#34086=CARTESIAN_POINT ( 'NONE',  ( 16.51473224551069308, 9.474510206698969483, 54.16557627198103120 ) ) ;
#34087=CARTESIAN_POINT ( 'NONE',  ( 13.89961937509977652, -13.97604488694527269, 78.12390960531433848 ) ) ;
#34088=CARTESIAN_POINT ( 'NONE',  ( 16.53943276465976808, -0.05219959533910856209, 108.7489096053143669 ) ) ;
#34089=CARTESIAN_POINT ( 'NONE',  ( -12.14591786802309592, -12.06949235617757132, 106.8739096053143811 ) ) ;
#34090=CARTESIAN_POINT ( 'NONE',  ( -21.53943276465977519, 0.05219959533907696930, 21.24890960531436690 ) ) ;
#34092=CARTESIAN_POINT ( 'NONE',  ( -14.34966873604972548, 8.224510206698743886, 83.33442372801903275 ) ) ;
#34093=CARTESIAN_POINT ( 'NONE',  ( 16.52544592524342804, -4.483927247898539470, 63.54057627198103830 ) ) ;
#34094=CARTESIAN_POINT ( 'NONE',  ( -9.564922557960796823, -16.46253265017161027, 57.08224293864769550 ) ) ;
#34095=CARTESIAN_POINT ( 'NONE',  ( 15.72974639402176855, 15.80617190586768217, 81.87609039468568994 ) ) ;
#34096=CARTESIAN_POINT ( 'NONE',  ( -0.05219959533937732626, 21.53943276465977519, 67.50109039468568994 ) ) ;
#34097=CARTESIAN_POINT ( 'NONE',  ( -19.03943276465977164, -0.05219959533935918106, 98.75109039468567573 ) ) ;
#34098=CARTESIAN_POINT ( 'NONE',  ( 4.379528057220339221, -16.55341960407611168, 62.70724293864769550 ) ) ;
#34099=CARTESIAN_POINT ( 'NONE',  ( -18.67979575497178146, -10.72451020669898902, 111.6655762719810525 ) ) ;
#34100=CARTESIAN_POINT ( 'NONE',  ( -15.80617190586745835, -15.72974639402198527, 66.87390960531436690 ) ) ;
#34102=CARTESIAN_POINT ( 'NONE',  ( 22.00000000000000000, -1.163414459189985801E-14, 95.00000000000000000 ) ) ;
#34104=CARTESIAN_POINT ( 'NONE',  ( -9.474510206698964154, 16.51473224551069663, 70.41557627198102409 ) ) ;
#34105=CARTESIAN_POINT ( 'NONE',  ( -16.53943276465976808, 0.05219959533911058130, 36.24890960531435979 ) ) ;
#34106=CARTESIAN_POINT ( 'NONE',  ( -8.314922557961024197, 14.29746914071037800, 112.9177570613523329 ) ) ;
#34107=CARTESIAN_POINT ( 'NONE',  ( 4.379528057220092307, 16.55341960407617563, 77.29275706135234714 ) ) ;
#34108=CARTESIAN_POINT ( 'NONE',  ( -13.97604488694547697, 13.89961937509957934, 33.12609039468566863 ) ) ;
#34110=CARTESIAN_POINT ( 'NONE',  ( 19.02544592524343514, -5.153800228976328945, 93.54057627198102409 ) ) ;
#34111=CARTESIAN_POINT ( 'NONE',  ( 0.05219959533910956823, 16.53943276465976808, 59.99890960531436690 ) ) ;
#34113=CARTESIAN_POINT ( 'NONE',  ( 19.02544592524343514, -5.153800228976328945, 113.5405762719810241 ) ) ;
#34114=CARTESIAN_POINT ( 'NONE',  ( 15.80617190586746368, 15.72974639402197994, 54.37390960531435979 ) ) ;
#34115=CARTESIAN_POINT ( 'NONE',  ( 12.06949235617757843, -12.14591786802309237, 103.1239096053143811 ) ) ;
#34116=CARTESIAN_POINT ( 'NONE',  ( -16.55341960407617563, 4.379528057220093196, 48.54275706135234714 ) ) ;
#34117=CARTESIAN_POINT ( 'NONE',  ( -14.34966873604960291, -8.224510206698953496, 81.66557627198103830 ) ) ;
#34118=CARTESIAN_POINT ( 'NONE',  ( -19.53037848336980531, 5.499999999999902300, 64.85532783611449759 ) ) ;
#34119=CARTESIAN_POINT ( 'NONE',  ( -16.46253265017146816, -9.564922557961047289, 84.16775706135233293 ) ) ;
#34120=CARTESIAN_POINT ( 'NONE',  ( 21.52544592524344225, -5.823673210054117533, 23.54057627198102765 ) ) ;
#34122=CARTESIAN_POINT ( 'NONE',  ( -17.59860650958989936, -7.585241751807033417, 41.57662985737508166 ) ) ;
#34123=CARTESIAN_POINT ( 'NONE',  ( 14.34966873604972726, -8.224510206698740333, 30.83442372801902209 ) ) ;
#34124=CARTESIAN_POINT ( 'NONE',  ( -14.34966873604960291, -8.224510206698953496, 31.66557627198102054 ) ) ;
#34125=CARTESIAN_POINT ( 'NONE',  ( -5.823673210054116645, -21.52544592524344225, 57.29057627198103120 ) ) ;
#34126=CARTESIAN_POINT ( 'NONE',  ( -16.46253265017146816, -9.564922557961047289, 89.16775706135234714 ) ) ;
#34127=CARTESIAN_POINT ( 'NONE',  ( -0.05219959533907301413, -21.53943276465977519, 42.49890960531435979 ) ) ;
#34128=CARTESIAN_POINT ( 'NONE',  ( -5.719274019375665041, -21.55341960407619695, 84.79275706135234714 ) ) ;
#34130=CARTESIAN_POINT ( 'NONE',  ( -8.224510206698735004, -14.34966873604973081, 29.58442372801901854 ) ) ;
#34131=CARTESIAN_POINT ( 'NONE',  ( -16.51473224551069308, -9.474510206698971260, 36.66557627198102409 ) ) ;
#34132=CARTESIAN_POINT ( 'NONE',  ( -13.89961937509977652, 13.97604488694528158, 90.62390960531432427 ) ) ;
#34133=CARTESIAN_POINT ( 'NONE',  ( -19.03943276465977164, 0.05219959533909376836, 41.24890960531435269 ) ) ;
#34134=CARTESIAN_POINT ( 'NONE',  ( 8.224510206698953496, -14.34966873604960469, 102.9155762719810383 ) ) ;
#34136=CARTESIAN_POINT ( 'NONE',  ( -19.02544592524342804, 5.153800228976336051, 101.0405762719810241 ) ) ;
#34138=CARTESIAN_POINT ( 'NONE',  ( -16.55341960407617563, 4.379528057220093196, 58.54275706135235424 ) ) ;
#34139=CARTESIAN_POINT ( 'NONE',  ( 15.80617190586746368, 15.72974639402197994, 94.37390960531436690 ) ) ;
#34140=CARTESIAN_POINT ( 'NONE',  ( 19.03943276465977164, -0.05219959533909143690, 38.74890960531436690 ) ) ;
#34141=CARTESIAN_POINT ( 'NONE',  ( 13.89961937509957401, 13.97604488694547697, 71.87609039468567573 ) ) ;
#34142=CARTESIAN_POINT ( 'NONE',  ( -15.80617190586768217, 15.72974639402176855, 33.12609039468569705 ) ) ;
#34143=CARTESIAN_POINT ( 'NONE',  ( -16.46253265017160317, 9.564922557960807481, 65.83224293864769550 ) ) ;
#34144=CARTESIAN_POINT ( 'NONE',  ( -16.51473224551069308, -9.474510206698971260, 101.6655762719810241 ) ) ;
#34146=CARTESIAN_POINT ( 'NONE',  ( 12.14591786802327356, -12.06949235617739191, 35.62609039468568994 ) ) ;
#34147=CARTESIAN_POINT ( 'NONE',  ( -5.719274019375978568, 21.55341960407610458, 110.2072429386477239 ) ) ;
#34148=CARTESIAN_POINT ( 'NONE',  ( -12.06949235617756955, 12.14591786802309770, 105.6239096053143669 ) ) ;
#34149=CARTESIAN_POINT ( 'NONE',  ( -13.89961937509977652, 13.97604488694528158, 90.62390960531432427 ) ) ;
#34150=CARTESIAN_POINT ( 'NONE',  ( -5.049401038297874678, -19.05341960407617918, 79.79275706135233293 ) ) ;
#34151=CARTESIAN_POINT ( 'NONE',  ( 10.81492255796078972, 18.62759615963270932, 84.58224293864769550 ) ) ;
#34152=CARTESIAN_POINT ( 'NONE',  ( -19.02544592524334988, -5.153800228976617603, 23.95942372801900078 ) ) ;
#34153=CARTESIAN_POINT ( 'NONE',  ( 12.14591786802327356, -12.06949235617739191, 80.62609039468567573 ) ) ;
#34154=CARTESIAN_POINT ( 'NONE',  ( -19.02544592524342804, 5.153800228976336051, 101.0405762719810241 ) ) ;
#34155=CARTESIAN_POINT ( 'NONE',  ( -19.05341960407611168, -5.049401038298163336, 51.45724293864770260 ) ) ;
#34156=CARTESIAN_POINT ( 'NONE',  ( 5.823673210054444382, -21.52544592524334988, 55.20942372801902565 ) ) ;
#34157=CARTESIAN_POINT ( 'NONE',  ( -21.52544592524334988, -5.823673210054445271, 68.95942372801901854 ) ) ;
#34158=CARTESIAN_POINT ( 'NONE',  ( 19.03943276465977164, -0.05219959533909143690, 68.74890960531436690 ) ) ;
#34159=CARTESIAN_POINT ( 'NONE',  ( 5.719274019375673035, 21.55341960407619339, 47.29275706135234003 ) ) ;
#34160=CARTESIAN_POINT ( 'NONE',  ( 19.05341960407617918, -5.049401038297876454, 91.04275706135234714 ) ) ;
#34161=CARTESIAN_POINT ( 'NONE',  ( -0.05219959533909027116, -19.03943276465977164, 47.49890960531435979 ) ) ;
#34162=CARTESIAN_POINT ( 'NONE',  ( -8.314922557961024197, 14.29746914071037800, 92.91775706135236135 ) ) ;
#34163=CARTESIAN_POINT ( 'NONE',  ( 5.049401038298161559, -19.05341960407611168, 67.70724293864769550 ) ) ;
#34165=CARTESIAN_POINT ( 'NONE',  ( -16.51473224551069308, -9.474510206698971260, 46.66557627198102409 ) ) ;
#34166=CARTESIAN_POINT ( 'NONE',  ( -5.823673210054116645, -21.52544592524344225, 87.29057627198103830 ) ) ;
#34167=CARTESIAN_POINT ( 'NONE',  ( 16.55341960407618274, -4.379528057220086978, 71.04275706135234714 ) ) ;
#34169=CARTESIAN_POINT ( 'NONE',  ( -5.049401038297874678, -19.05341960407617918, 24.79275706135233648 ) ) ;
#34171=CARTESIAN_POINT ( 'NONE',  ( -16.46253265017160317, 9.564922557960807481, 70.83224293864770971 ) ) ;
#34172=CARTESIAN_POINT ( 'NONE',  ( 14.29746914071049879, -8.314922557960816363, 63.33224293864770260 ) ) ;
#34173=CARTESIAN_POINT ( 'NONE',  ( -14.29746914071049879, 8.314922557960819915, 100.8322429386477097 ) ) ;
#34174=CARTESIAN_POINT ( 'NONE',  ( 5.049401038298161559, -19.05341960407611168, 107.7072429386476955 ) ) ;
#34175=CARTESIAN_POINT ( 'NONE',  ( -19.02544592524342804, 5.153800228976336051, 96.04057627198103830 ) ) ;
#34176=CARTESIAN_POINT ( 'NONE',  ( -18.62759615963255300, -10.81492255796106328, 44.16775706135234714 ) ) ;
#34177=CARTESIAN_POINT ( 'NONE',  ( -19.02544592524342804, 5.153800228976336051, 106.0405762719810241 ) ) ;
#34178=CARTESIAN_POINT ( 'NONE',  ( -10.81492255796105439, 18.62759615963255655, 112.9177570613523329 ) ) ;
#34179=CARTESIAN_POINT ( 'NONE',  ( -16.53943276465976808, -0.05219959533934237506, 83.75109039468568994 ) ) ;
#34180=CARTESIAN_POINT ( 'NONE',  ( -10.81492255796105439, 18.62759615963255655, 42.91775706135235424 ) ) ;
#34181=CARTESIAN_POINT ( 'NONE',  ( -19.05341960407611168, -5.049401038298163336, 111.4572429386476671 ) ) ;
#34182=CARTESIAN_POINT ( 'NONE',  ( 18.62759615963271287, -10.81492255796078972, 103.3322429386476955 ) ) ;
#34183=CARTESIAN_POINT ( 'NONE',  ( 14.29746914071049879, -8.314922557960816363, 58.33224293864768839 ) ) ;
#34184=CARTESIAN_POINT ( 'NONE',  ( -9.564922557960796823, -16.46253265017161027, 57.08224293864769550 ) ) ;
#34185=CARTESIAN_POINT ( 'NONE',  ( 4.379528057220339221, -16.55341960407611168, 87.70724293864769550 ) ) ;
#34186=CARTESIAN_POINT ( 'NONE',  ( -5.823673210054116645, -21.52544592524344225, 37.29057627198102409 ) ) ;
#34187=CARTESIAN_POINT ( 'NONE',  ( 5.153800228976615827, -19.02544592524334988, 50.20942372801897591 ) ) ;
#34188=CARTESIAN_POINT ( 'NONE',  ( -16.53943276465976808, 0.05219959533911058130, 111.2489096053143669 ) ) ;
#34190=CARTESIAN_POINT ( 'NONE',  ( 12.06949235617739724, 12.14591786802326823, 66.87609039468568994 ) ) ;
#34191=CARTESIAN_POINT ( 'NONE',  ( 16.51473224551069308, 9.474510206698969483, 69.16557627198102409 ) ) ;
#34193=CARTESIAN_POINT ( 'NONE',  ( -16.52544592524342804, 4.483927247898546575, 86.04057627198102409 ) ) ;
#34194=CARTESIAN_POINT ( 'NONE',  ( -10.81492255796078084, -18.62759615963271287, 42.08224293864769550 ) ) ;
#34195=CARTESIAN_POINT ( 'NONE',  ( -14.34966873604972548, 8.224510206698743886, 103.3344237280190043 ) ) ;
#34196=CARTESIAN_POINT ( 'NONE',  ( -9.564922557961040184, 16.46253265017147172, 102.9177570613523329 ) ) ;
#34197=CARTESIAN_POINT ( 'NONE',  ( 21.55341960407619695, -5.719274019375665929, 81.04275706135236135 ) ) ;
#34198=CARTESIAN_POINT ( 'NONE',  ( 9.474510206698971260, -16.51473224551069308, 87.91557627198102409 ) ) ;
#34199=CARTESIAN_POINT ( 'NONE',  ( 21.53943276465977519, -0.05219959533907433946, 103.7489096053143669 ) ) ;
#34200=CARTESIAN_POINT ( 'NONE',  ( 0.05219959533934541429, -16.53943276465976808, 50.00109039468568994 ) ) ;
#34201=CARTESIAN_POINT ( 'NONE',  ( -5.153800228976328057, -19.02544592524343514, 27.29057627198103120 ) ) ;
#34202=CARTESIAN_POINT ( 'NONE',  ( -0.05219959533934338120, 16.53943276465976808, 37.50109039468568284 ) ) ;
#34203=CARTESIAN_POINT ( 'NONE',  ( 9.564922557961047289, -16.46253265017146816, 100.4177570613523329 ) ) ;
#34204=CARTESIAN_POINT ( 'NONE',  ( 21.52544592524344225, -5.823673210054117533, 93.54057627198103830 ) ) ;
#34205=CARTESIAN_POINT ( 'NONE',  ( 19.03943276465977164, 0.05219959533936151252, 51.25109039468567573 ) ) ;
#34206=CARTESIAN_POINT ( 'NONE',  ( 18.39443945427638738, -5.500000000000021316, 86.01745347608655834 ) ) ;
#34207=CARTESIAN_POINT ( 'NONE',  ( 15.80617190586746368, 15.72974639402197994, 99.37390960531436690 ) ) ;
#34209=CARTESIAN_POINT ( 'NONE',  ( 16.46253265017160672, -9.564922557960803928, 73.33224293864769550 ) ) ;
#34210=CARTESIAN_POINT ( 'NONE',  ( 14.34966873604972726, -8.224510206698740333, 35.83442372801901143 ) ) ;
#34212=CARTESIAN_POINT ( 'NONE',  ( 16.51473224551083163, -9.474510206698727899, 65.83442372801900433 ) ) ;
#34213=CARTESIAN_POINT ( 'NONE',  ( -10.72451020669898014, 18.67979575497178502, 115.4155762719810241 ) ) ;
#34214=CARTESIAN_POINT ( 'NONE',  ( 14.29746914071049879, -8.314922557960816363, 63.33224293864770260 ) ) ;
#34215=CARTESIAN_POINT ( 'NONE',  ( -0.05219959533909027116, -19.03943276465977164, 67.49890960531436690 ) ) ;
#34216=CARTESIAN_POINT ( 'NONE',  ( -16.52544592524335698, -4.483927247898792601, 33.95942372801901143 ) ) ;
#34217=CARTESIAN_POINT ( 'NONE',  ( -9.564922557961040184, 16.46253265017147172, 37.91775706135233293 ) ) ;
#34218=CARTESIAN_POINT ( 'NONE',  ( 18.62759615963255655, 10.81492255796105972, 56.66775706135235424 ) ) ;
#34220=CARTESIAN_POINT ( 'NONE',  ( 5.153800228976615827, -19.02544592524334988, 110.2094237280189901 ) ) ;
#34221=CARTESIAN_POINT ( 'NONE',  ( 16.51473224551069308, 9.474510206698969483, 49.16557627198102409 ) ) ;
#34222=CARTESIAN_POINT ( 'NONE',  ( -19.05341960407617563, 5.049401038297882671, 88.54275706135230450 ) ) ;
#34223=CARTESIAN_POINT ( 'NONE',  ( 10.72451020669871369, 18.67979575497193778, 82.08442372801901854 ) ) ;
#34224=CARTESIAN_POINT ( 'NONE',  ( -5.153800228976607833, 19.02544592524334988, 62.70942372801899722 ) ) ;
#34225=CARTESIAN_POINT ( 'NONE',  ( 19.03943276465977164, -0.05219959533909143690, 33.74890960531435979 ) ) ;
#34226=CARTESIAN_POINT ( 'NONE',  ( 10.72451020669898902, -18.67979575497178502, 57.91557627198103120 ) ) ;
#34227=CARTESIAN_POINT ( 'NONE',  ( 14.29746914071049879, -8.314922557960816363, 68.33224293864769550 ) ) ;
#34228=CARTESIAN_POINT ( 'NONE',  ( -16.46253265017146816, -9.564922557961047289, 69.16775706135233293 ) ) ;
#34230=CARTESIAN_POINT ( 'NONE',  ( 16.51473224551083163, -9.474510206698727899, 30.83442372801900433 ) ) ;
#34231=CARTESIAN_POINT ( 'NONE',  ( 12.14591786802327356, -12.06949235617739191, 100.6260903946857184 ) ) ;
#34232=CARTESIAN_POINT ( 'NONE',  ( 16.55341960407611168, 4.379528057220329451, 48.95724293864770971 ) ) ;
#34233=CARTESIAN_POINT ( 'NONE',  ( -15.72974639402176322, -15.80617190586768395, 94.37609039468568994 ) ) ;
#34235=CARTESIAN_POINT ( 'NONE',  ( 5.719274019375991003, -21.55341960407610458, 92.70724293864770971 ) ) ;
#34236=CARTESIAN_POINT ( 'NONE',  ( -19.02544592524342804, 5.153800228976336051, 46.04057627198101699 ) ) ;
#34237=CARTESIAN_POINT ( 'NONE',  ( -15.72974639402176322, -15.80617190586768395, 74.37609039468568994 ) ) ;
#34238=CARTESIAN_POINT ( 'NONE',  ( -13.89961937509977652, 13.97604488694528158, 55.62390960531434558 ) ) ;
#34240=CARTESIAN_POINT ( 'NONE',  ( 5.153800228976335163, 19.02544592524342804, 69.79057627198103830 ) ) ;
#34241=CARTESIAN_POINT ( 'NONE',  ( -14.29746914071049879, 8.314922557960819915, 105.8322429386476955 ) ) ;
#34242=CARTESIAN_POINT ( 'NONE',  ( -9.474510206698964154, 16.51473224551069663, 105.4155762719810383 ) ) ;
#34244=CARTESIAN_POINT ( 'NONE',  ( -14.34966873604960291, -8.224510206698953496, 51.66557627198102409 ) ) ;
#34245=CARTESIAN_POINT ( 'NONE',  ( 9.564922557960805705, 16.46253265017160317, 34.58224293864770260 ) ) ;
#34246=CARTESIAN_POINT ( 'NONE',  ( 16.52544592524342804, -4.483927247898539470, 83.54057627198102409 ) ) ;
#34247=CARTESIAN_POINT ( 'NONE',  ( 15.80617190586746368, 15.72974639402197994, 94.37390960531436690 ) ) ;
#34248=CARTESIAN_POINT ( 'NONE',  ( -10.72451020669870658, -18.67979575497194134, 39.58442372801901143 ) ) ;
#34249=CARTESIAN_POINT ( 'NONE',  ( -16.51473224551069308, -9.474510206698971260, 21.66557627198102765 ) ) ;
#34250=CARTESIAN_POINT ( 'NONE',  ( 16.52544592524335698, 4.483927247898782831, 36.45942372801901143 ) ) ;
#34251=CARTESIAN_POINT ( 'NONE',  ( -5.719274019375978568, 21.55341960407610458, 90.20724293864770971 ) ) ;
#34253=CARTESIAN_POINT ( 'NONE',  ( -21.55341960407619339, 5.719274019375674811, 108.5427570613523756 ) ) ;
#34254=CARTESIAN_POINT ( 'NONE',  ( 16.46253265017160672, -9.564922557960803928, 88.33224293864769550 ) ) ;
#34255=CARTESIAN_POINT ( 'NONE',  ( -0.05219959533937732626, 21.53943276465977519, 42.50109039468567573 ) ) ;
#34256=CARTESIAN_POINT ( 'NONE',  ( 15.72974639402199770, -15.80617190586745480, 33.12390960531435979 ) ) ;
#34257=CARTESIAN_POINT ( 'NONE',  ( -14.29746914071037622, -8.314922557961029526, 109.1677570613523613 ) ) ;
#34258=CARTESIAN_POINT ( 'NONE',  ( -18.62759615963255300, -10.81492255796106328, 54.16775706135235424 ) ) ;
#34259=CARTESIAN_POINT ( 'NONE',  ( -10.81492255796105439, 18.62759615963255655, 77.91775706135231871 ) ) ;
#34260=CARTESIAN_POINT ( 'NONE',  ( 5.153800228976615827, -19.02544592524334988, 35.20942372801899722 ) ) ;
#34261=CARTESIAN_POINT ( 'NONE',  ( 16.55341960407618274, -4.379528057220086978, 86.04275706135236135 ) ) ;
#34262=CARTESIAN_POINT ( 'NONE',  ( 21.53943276465977519, 0.05219959533937863772, 41.25109039468568284 ) ) ;
#34263=CARTESIAN_POINT ( 'NONE',  ( -13.97604488694527625, -13.89961937509977652, 51.87390960531436690 ) ) ;
#34264=CARTESIAN_POINT ( 'NONE',  ( -18.62759615963255300, -10.81492255796106328, 99.16775706135234714 ) ) ;
#34265=CARTESIAN_POINT ( 'NONE',  ( -16.46253265017160317, 9.564922557960807481, 100.8322429386477097 ) ) ;
#34266=CARTESIAN_POINT ( 'NONE',  ( 5.719274019375991003, -21.55341960407610458, 102.7072429386476955 ) ) ;
#34267=CARTESIAN_POINT ( 'NONE',  ( -18.67979575497178146, -10.72451020669898902, 76.66557627198103830 ) ) ;
#34269=CARTESIAN_POINT ( 'NONE',  ( 15.80617190586746368, 15.72974639402197994, 64.37390960531435269 ) ) ;
#34270=CARTESIAN_POINT ( 'NONE',  ( -14.34966873604972548, 8.224510206698743886, 58.33442372801901143 ) ) ;
#34271=CARTESIAN_POINT ( 'NONE',  ( -12.06949235617756955, 12.14591786802309770, 60.62390960531437401 ) ) ;
#34273=CARTESIAN_POINT ( 'NONE',  ( -5.049401038297874678, -19.05341960407617918, 94.79275706135230450 ) ) ;
#34275=CARTESIAN_POINT ( 'NONE',  ( 16.55341960407618274, -4.379528057220086978, 21.04275706135234714 ) ) ;
#34276=CARTESIAN_POINT ( 'NONE',  ( 5.823673210054125526, 21.52544592524343514, 104.7905762719810241 ) ) ;
#34277=CARTESIAN_POINT ( 'NONE',  ( -15.80617190586745835, -15.72974639402198527, 76.87390960531439532 ) ) ;
#34278=CARTESIAN_POINT ( 'NONE',  ( -15.80617190586745835, -15.72974639402198527, 21.87390960531436690 ) ) ;
#34279=CARTESIAN_POINT ( 'NONE',  ( 12.06949235617739724, 12.14591786802326823, 56.87609039468568994 ) ) ;
#34280=CARTESIAN_POINT ( 'NONE',  ( -5.049401038298153566, 19.05341960407611168, 65.20724293864765286 ) ) ;
#34281=CARTESIAN_POINT ( 'NONE',  ( -21.52544592524334988, -5.823673210054445271, 48.95942372801902565 ) ) ;
#34282=CARTESIAN_POINT ( 'NONE',  ( 16.46253265017146816, 9.564922557961045513, 106.6677570613523471 ) ) ;
#34283=CARTESIAN_POINT ( 'NONE',  ( -9.564922557960796823, -16.46253265017161027, 102.0822429386477097 ) ) ;
#34284=CARTESIAN_POINT ( 'NONE',  ( -0.05219959533909027116, -19.03943276465977164, 97.49890960531436690 ) ) ;
#34285=CARTESIAN_POINT ( 'NONE',  ( -15.72974639402197994, 15.80617190586746368, 95.62390960531436690 ) ) ;
#34286=CARTESIAN_POINT ( 'NONE',  ( -9.564922557960796823, -16.46253265017161027, 62.08224293864769550 ) ) ;
#34287=CARTESIAN_POINT ( 'NONE',  ( -16.81555441253550853, -7.025013491695501600, 59.36314554665745646 ) ) ;
#34288=CARTESIAN_POINT ( 'NONE',  ( 12.06949235617757843, -12.14591786802309237, 88.12390960531436690 ) ) ;
#34289=CARTESIAN_POINT ( 'NONE',  ( 9.474510206698971260, -16.51473224551069308, 112.9155762719810383 ) ) ;
#34291=CARTESIAN_POINT ( 'NONE',  ( -10.81492255796078084, -18.62759615963271287, 102.0822429386476955 ) ) ;
#34292=CARTESIAN_POINT ( 'NONE',  ( -16.46253265017146816, -9.564922557961047289, 69.16775706135233293 ) ) ;
#34293=CARTESIAN_POINT ( 'NONE',  ( -0.05219959533907301413, -21.53943276465977519, 22.49890960531436335 ) ) ;
#34294=CARTESIAN_POINT ( 'NONE',  ( 16.46253265017160672, -9.564922557960803928, 28.33224293864769550 ) ) ;
#34295=CARTESIAN_POINT ( 'NONE',  ( 21.53943276465977519, -0.05219959533907433946, 48.74890960531435979 ) ) ;
#34296=CARTESIAN_POINT ( 'NONE',  ( 16.46253265017160672, -9.564922557960803928, 98.33224293864769550 ) ) ;
#34297=CARTESIAN_POINT ( 'NONE',  ( 10.72451020669871369, 18.67979575497193778, 72.08442372801899012 ) ) ;
#34298=CARTESIAN_POINT ( 'NONE',  ( -5.049401038298153566, 19.05341960407611168, 50.20724293864770260 ) ) ;
#34299=CARTESIAN_POINT ( 'NONE',  ( -14.34966873604960291, -8.224510206698953496, 91.66557627198103830 ) ) ;
#34300=CARTESIAN_POINT ( 'NONE',  ( 0.05219959533934541429, -16.53943276465976808, 35.00109039468568284 ) ) ;
#34301=CARTESIAN_POINT ( 'NONE',  ( 5.823673210054444382, -21.52544592524334988, 60.20942372801902565 ) ) ;
#34303=CARTESIAN_POINT ( 'NONE',  ( 16.46253265017146816, 9.564922557961045513, 31.66775706135232937 ) ) ;
#34304=CARTESIAN_POINT ( 'NONE',  ( -9.564922557961040184, 16.46253265017147172, 77.91775706135234714 ) ) ;
#34305=CARTESIAN_POINT ( 'NONE',  ( 13.97604488694548053, -13.89961937509957401, 45.62609039468566863 ) ) ;
#34306=DIRECTION ( 'NONE',  ( 1.000000000000000000, 0.000000000000000000, 0.000000000000000000 ) ) ;
#34307=CARTESIAN_POINT ( 'NONE',  ( 0.05219959533937995610, -21.53943276465977519, 40.00109039468567573 ) ) ;
#34309=CARTESIAN_POINT ( 'NONE',  ( 19.03943276465977164, 0.05219959533936151252, 31.25109039468566863 ) ) ;
#34310=CARTESIAN_POINT ( 'NONE',  ( -9.564922557960796823, -16.46253265017161027, 62.08224293864769550 ) ) ;
#34311=CARTESIAN_POINT ( 'NONE',  ( 5.153800228976615827, -19.02544592524334988, 35.20942372801899722 ) ) ;
#34312=CARTESIAN_POINT ( 'NONE',  ( 16.52544592524335698, 4.483927247898782831, 106.4594237280190328 ) ) ;
#34313=CARTESIAN_POINT ( 'NONE',  ( 5.719274019375991003, -21.55341960407610458, 22.70724293864769194 ) ) ;
#34314=CARTESIAN_POINT ( 'NONE',  ( 21.55341960407619695, -5.719274019375665929, 91.04275706135236135 ) ) ;
#34316=CARTESIAN_POINT ( 'NONE',  ( -17.50000000000000355, -5.068104630630324792, 34.27181594659972319 ) ) ;
#34317=CARTESIAN_POINT ( 'NONE',  ( 18.67979575497194134, -10.72451020669871369, 80.83442372801901854 ) ) ;
#34319=CARTESIAN_POINT ( 'NONE',  ( 16.51473224551069308, 9.474510206698969483, 94.16557627198103830 ) ) ;
#34321=B_SPLINE_CURVE_WITH_KNOTS ( 'NONE', 3,
 ( #54377, #24049, #163560, #86703, #177738, #116049, #69545, #192900, #39207, #147391, #55370, #84691, #118056, #83696, #25060, #6856, #117040, #68535, #133208, #100863 ),
 .UNSPECIFIED., .F., .F.,
 ( 4, 2, 2, 2, 2, 2, 2, 2, 2, 4 ),
 ( 0.004000878361811936561, 0.004499404418915928239, 0.004997930476019919917, 0.005496456533123911595, 0.005994982590227904140, 0.006244245618779899545, 0.006493508647331894951, 0.006992034704435887496, 0.007490560761539879174, 0.007989086818643870852 ),
 .UNSPECIFIED. ) ;
#34322=CARTESIAN_POINT ( 'NONE',  ( -0.05219959533909027116, -19.03943276465977164, 57.49890960531435979 ) ) ;
#34323=CARTESIAN_POINT ( 'NONE',  ( 0.05219959533907565091, 21.53943276465977519, 49.99890960531437401 ) ) ;
#34324=EDGE_CURVE ( 'NONE', #22766, #155866, #110733, .T. ) ;
#34325=CARTESIAN_POINT ( 'NONE',  ( 12.06949235617757843, -12.14591786802309237, 28.12390960531435979 ) ) ;
#34326=CARTESIAN_POINT ( 'NONE',  ( 4.483927247898545687, 16.52544592524342804, 94.79057627198105251 ) ) ;
#34327=CARTESIAN_POINT ( 'NONE',  ( -0.05219959533909027116, -19.03943276465977164, 97.49890960531436690 ) ) ;
#34328=CARTESIAN_POINT ( 'NONE',  ( 13.89961937509957401, 13.97604488694547697, 21.87609039468566152 ) ) ;
#34329=CARTESIAN_POINT ( 'NONE',  ( 12.14591786802309770, 12.06949235617756955, 104.3739096053143669 ) ) ;
#34330=CARTESIAN_POINT ( 'NONE',  ( -10.81492255796105439, 18.62759615963255655, 52.91775706135235424 ) ) ;
#34331=CARTESIAN_POINT ( 'NONE',  ( -14.34966873604972548, 8.224510206698743886, 108.3344237280190185 ) ) ;
#34332=CARTESIAN_POINT ( 'NONE',  ( -16.51473224551082808, 9.474510206698731452, 63.33442372801900433 ) ) ;
#34334=CARTESIAN_POINT ( 'NONE',  ( -19.03943276465977164, 0.05219959533909376836, 111.2489096053143669 ) ) ;
#34335=CARTESIAN_POINT ( 'NONE',  ( 16.55341960407611168, 4.379528057220329451, 73.95724293864769550 ) ) ;
#34337=CARTESIAN_POINT ( 'NONE',  ( 13.97604488694548053, -13.89961937509957401, 55.62609039468566863 ) ) ;
#34338=CARTESIAN_POINT ( 'NONE',  ( 16.51473224551069308, 9.474510206698969483, 59.16557627198102409 ) ) ;
#34339=CARTESIAN_POINT ( 'NONE',  ( 4.379528057220339221, -16.55341960407611168, 62.70724293864769550 ) ) ;
#34340=CARTESIAN_POINT ( 'NONE',  ( -9.474510206698720793, -16.51473224551083518, 89.58442372801900433 ) ) ;
#34341=CARTESIAN_POINT ( 'NONE',  ( 0.05219959533907565091, 21.53943276465977519, 29.99890960531435979 ) ) ;
#34343=CARTESIAN_POINT ( 'NONE',  ( -12.14591786802309592, -12.06949235617757132, 106.8739096053143811 ) ) ;
#34344=CARTESIAN_POINT ( 'NONE',  ( -17.58332526062525147, -7.635886036038636249, 99.07665040441534643 ) ) ;
#34345=CARTESIAN_POINT ( 'NONE',  ( -9.564922557960796823, -16.46253265017161027, 62.08224293864769550 ) ) ;
#34346=CARTESIAN_POINT ( 'NONE',  ( -15.80617190586745835, -15.72974639402198527, 61.87390960531436690 ) ) ;
#34347=CARTESIAN_POINT ( 'NONE',  ( -13.89961937509977652, 13.97604488694528158, 45.62390960531433848 ) ) ;
#34348=CARTESIAN_POINT ( 'NONE',  ( -16.53943276465976808, -0.05219959533934237506, 88.75109039468567573 ) ) ;
#34349=CARTESIAN_POINT ( 'NONE',  ( 5.153800228976335163, 19.02544592524342804, 79.79057627198102409 ) ) ;
#34350=CARTESIAN_POINT ( 'NONE',  ( -5.153800228976607833, 19.02544592524334988, 47.70942372801900433 ) ) ;
#34351=CARTESIAN_POINT ( 'NONE',  ( 10.81492255796106328, -18.62759615963255655, 85.41775706135236135 ) ) ;
#34352=CARTESIAN_POINT ( 'NONE',  ( -5.719274019375978568, 21.55341960407610458, 55.20724293864770260 ) ) ;
#34353=CARTESIAN_POINT ( 'NONE',  ( 13.97604488694527802, 13.89961937509977652, 104.3739096053143385 ) ) ;
#34354=CARTESIAN_POINT ( 'NONE',  ( -5.153800228976328057, -19.02544592524343514, 22.29057627198102765 ) ) ;
#34355=CARTESIAN_POINT ( 'NONE',  ( 12.14591786802327356, -12.06949235617739191, 90.62609039468567573 ) ) ;
#34356=CARTESIAN_POINT ( 'NONE',  ( 9.564922557961047289, -16.46253265017146816, 105.4177570613523471 ) ) ;
#34357=CARTESIAN_POINT ( 'NONE',  ( 16.46253265017160672, -9.564922557960803928, 23.33224293864769194 ) ) ;
#34359=CARTESIAN_POINT ( 'NONE',  ( 15.72974639402176855, 15.80617190586768217, 101.8760903946857042 ) ) ;
#34360=CARTESIAN_POINT ( 'NONE',  ( 4.379528057220339221, -16.55341960407611168, 57.70724293864770260 ) ) ;
#34361=CARTESIAN_POINT ( 'NONE',  ( 14.29746914071049879, -8.314922557960816363, 68.33224293864769550 ) ) ;
#34362=CARTESIAN_POINT ( 'NONE',  ( 21.55341960407610458, 5.719274019375980345, 93.95724293864770971 ) ) ;
#34363=CARTESIAN_POINT ( 'NONE',  ( 5.719274019375991003, -21.55341960407610458, 92.70724293864770971 ) ) ;
#34364=CARTESIAN_POINT ( 'NONE',  ( 16.88567814943162304, -6.947325034625687401, 96.20998877347413725 ) ) ;
#34365=CARTESIAN_POINT ( 'NONE',  ( -21.55341960407610458, -5.719274019375992779, 26.45724293864768839 ) ) ;
#34366=CARTESIAN_POINT ( 'NONE',  ( 8.314922557961029526, -14.29746914071037800, 60.41775706135235424 ) ) ;
#34367=CARTESIAN_POINT ( 'NONE',  ( -8.224510206698948167, 14.34966873604960824, 85.41557627198102409 ) ) ;
#34368=CARTESIAN_POINT ( 'NONE',  ( 5.153800228976335163, 19.02544592524342804, 44.79057627198103830 ) ) ;
#34371=CARTESIAN_POINT ( 'NONE',  ( 16.52544592524335698, 4.483927247898782831, 91.45942372801901854 ) ) ;
#34372=CARTESIAN_POINT ( 'NONE',  ( -15.72974639402176322, -15.80617190586768395, 39.37609039468567573 ) ) ;
#34373=CARTESIAN_POINT ( 'NONE',  ( 5.049401038298161559, -19.05341960407611168, 82.70724293864770971 ) ) ;
#34374=CARTESIAN_POINT ( 'NONE',  ( -18.62759615963255300, -10.81492255796106328, 74.16775706135231871 ) ) ;
#34375=CARTESIAN_POINT ( 'NONE',  ( 19.02544592524343514, -5.153800228976328945, 23.54057627198102054 ) ) ;
#34376=CARTESIAN_POINT ( 'NONE',  ( -5.153800228976328057, -19.02544592524343514, 27.29057627198103120 ) ) ;
#34378=CARTESIAN_POINT ( 'NONE',  ( -18.62759615963255300, -10.81492255796106328, 64.16775706135234714 ) ) ;
#34379=CARTESIAN_POINT ( 'NONE',  ( 9.474510206698971260, -16.51473224551069308, 42.91557627198103120 ) ) ;
#34380=CARTESIAN_POINT ( 'NONE',  ( -16.46253265017160317, 9.564922557960807481, 110.8322429386476955 ) ) ;
#34381=CARTESIAN_POINT ( 'NONE',  ( -19.05341960407611168, -5.049401038298163336, 96.45724293864769550 ) ) ;
#34382=CARTESIAN_POINT ( 'NONE',  ( 13.89961937509957401, 13.97604488694547697, 66.87609039468567573 ) ) ;
#34383=CARTESIAN_POINT ( 'NONE',  ( -5.719274019375665041, -21.55341960407619695, 29.79275706135234358 ) ) ;
#34384=CARTESIAN_POINT ( 'NONE',  ( -9.564922557961040184, 16.46253265017147172, 52.91775706135233293 ) ) ;
#34385=CARTESIAN_POINT ( 'NONE',  ( 9.474510206698971260, -16.51473224551069308, 42.91557627198103120 ) ) ;
#34386=CARTESIAN_POINT ( 'NONE',  ( 4.483927247898790824, -16.52544592524335698, 100.2094237280190043 ) ) ;
#34387=CARTESIAN_POINT ( 'NONE',  ( -19.02544592524334988, -5.153800228976617603, 68.95942372801896170 ) ) ;
#34388=CARTESIAN_POINT ( 'NONE',  ( -14.29746914071049879, 8.314922557960819915, 30.83224293864770260 ) ) ;
#34389=CARTESIAN_POINT ( 'NONE',  ( 9.564922557961047289, -16.46253265017146816, 50.41775706135233293 ) ) ;
#34390=ORIENTED_EDGE ( 'NONE', *, *, #125103, .T. ) ;
#34391=CARTESIAN_POINT ( 'NONE',  ( -5.049401038298153566, 19.05341960407611168, 95.20724293864770971 ) ) ;
#34393=CARTESIAN_POINT ( 'NONE',  ( -18.67979575497193778, 10.72451020669871902, 93.33442372801901854 ) ) ;
#34394=CARTESIAN_POINT ( 'NONE',  ( -10.72451020669870658, -18.67979575497194134, 109.5844237280190328 ) ) ;
#34396=CARTESIAN_POINT ( 'NONE',  ( -21.55341960407619339, 5.719274019375674811, 83.54275706135234714 ) ) ;
#34397=CARTESIAN_POINT ( 'NONE',  ( 16.53943276465976808, 0.05219959533934440121, 26.25109039468567573 ) ) ;
#34398=CARTESIAN_POINT ( 'NONE',  ( 19.05341960407611168, 5.049401038298154454, 88.95724293864769550 ) ) ;
#34400=CARTESIAN_POINT ( 'NONE',  ( 19.02544592524343514, -5.153800228976328945, 83.54057627198100988 ) ) ;
#34402=CARTESIAN_POINT ( 'NONE',  ( 16.46253265017146816, 9.564922557961045513, 76.66775706135234714 ) ) ;
#34403=CARTESIAN_POINT ( 'NONE',  ( -16.51473224551069308, -9.474510206698971260, 106.6655762719810383 ) ) ;
#34404=CARTESIAN_POINT ( 'NONE',  ( 21.52544592524334988, 5.823673210054432836, 101.4594237280190185 ) ) ;
#34405=CARTESIAN_POINT ( 'NONE',  ( 16.53943276465976808, -0.05219959533910856209, 103.7489096053143669 ) ) ;
#34406=CARTESIAN_POINT ( 'NONE',  ( -10.81492255796078084, -18.62759615963271287, 42.08224293864769550 ) ) ;
#34407=CARTESIAN_POINT ( 'NONE',  ( 5.823673210054125526, 21.52544592524343514, 39.79057627198103830 ) ) ;
#34408=CARTESIAN_POINT ( 'NONE',  ( 16.53943276465976808, -0.05219959533910856209, 103.7489096053143669 ) ) ;
#34410=CARTESIAN_POINT ( 'NONE',  ( 19.02544592524334988, 5.153800228976608722, 56.45942372801898301 ) ) ;
#34411=CARTESIAN_POINT ( 'NONE',  ( 16.53943276465976808, -0.05219959533910856209, 28.74890960531435624 ) ) ;
#34412=CARTESIAN_POINT ( 'NONE',  ( 9.564922557960805705, 16.46253265017160317, 104.5822429386476955 ) ) ;
#34413=CARTESIAN_POINT ( 'NONE',  ( 15.80617190586769283, -15.72974639402175789, 80.62609039468567573 ) ) ;
#34414=CARTESIAN_POINT ( 'NONE',  ( 21.55341960407610458, 5.719274019375980345, 73.95724293864769550 ) ) ;
#34415=CARTESIAN_POINT ( 'NONE',  ( 15.80617190586769283, -15.72974639402175789, 40.62609039468567573 ) ) ;
#34416=CARTESIAN_POINT ( 'NONE',  ( 15.72974639402199770, -15.80617190586745480, 98.12390960531436690 ) ) ;
#34417=CARTESIAN_POINT ( 'NONE',  ( 10.81492255796106328, -18.62759615963255655, 55.41775706135234714 ) ) ;
#34418=CARTESIAN_POINT ( 'NONE',  ( 19.03943276465977164, -0.05219959533909143690, 28.74890960531435624 ) ) ;
#34419=CARTESIAN_POINT ( 'NONE',  ( -19.05341960407611168, -5.049401038298163336, 86.45724293864769550 ) ) ;
#34420=CARTESIAN_POINT ( 'NONE',  ( -0.05219959533934338120, 16.53943276465976808, 82.50109039468568994 ) ) ;
#34421=CARTESIAN_POINT ( 'NONE',  ( -4.379528057220328563, 16.55341960407611168, 110.2072429386477239 ) ) ;
#34422=CARTESIAN_POINT ( 'NONE',  ( 5.049401038298161559, -19.05341960407611168, 102.7072429386476955 ) ) ;
#34423=CARTESIAN_POINT ( 'NONE',  ( -12.06949235617756955, 12.14591786802309770, 50.62390960531435979 ) ) ;
#34424=CARTESIAN_POINT ( 'NONE',  ( 14.29746914071049879, -8.314922557960816363, 23.33224293864769194 ) ) ;
#34425=CARTESIAN_POINT ( 'NONE',  ( 16.51473224551069308, 9.474510206698969483, 59.16557627198102409 ) ) ;
#34426=CARTESIAN_POINT ( 'NONE',  ( -5.153800228976328057, -19.02544592524343514, 32.29057627198102409 ) ) ;
#34427=CARTESIAN_POINT ( 'NONE',  ( 15.80617190586746368, 15.72974639402197994, 39.37390960531436690 ) ) ;
#34428=CARTESIAN_POINT ( 'NONE',  ( -5.049401038297874678, -19.05341960407617918, 24.79275706135233648 ) ) ;
#34429=CARTESIAN_POINT ( 'NONE',  ( 17.50000000000000000, 5.499999999999997335, 120.0000000000000142 ) ) ;
#34430=CARTESIAN_POINT ( 'NONE',  ( 8.224510206698953496, -14.34966873604960469, 42.91557627198103120 ) ) ;
#34431=CARTESIAN_POINT ( 'NONE',  ( 0.05219959533937995610, -21.53943276465977519, 40.00109039468567573 ) ) ;
#34432=CARTESIAN_POINT ( 'NONE',  ( -13.89961937509977652, 13.97604488694528158, 115.6239096053143669 ) ) ;
#34433=CARTESIAN_POINT ( 'NONE',  ( 16.53943276465976808, 0.05219959533934440121, 61.25109039468567573 ) ) ;
#34434=CARTESIAN_POINT ( 'NONE',  ( 19.05341960407617918, -5.049401038297876454, 61.04275706135232582 ) ) ;
#34435=CARTESIAN_POINT ( 'NONE',  ( -4.483927247898539470, -16.52544592524342804, 22.29057627198102765 ) ) ;
#34436=CARTESIAN_POINT ( 'NONE',  ( 17.48853670773245739, -5.747243402303059412, 51.16671299749991420 ) ) ;
#34437=CARTESIAN_POINT ( 'NONE',  ( 0.05219959533934541429, -16.53943276465976808, 105.0010903946856757 ) ) ;
#34438=CARTESIAN_POINT ( 'NONE',  ( 13.89961937509977652, -13.97604488694527269, 38.12390960531436690 ) ) ;
#34439=CARTESIAN_POINT ( 'NONE',  ( -5.049401038298153566, 19.05341960407611168, 60.20724293864768129 ) ) ;
#34440=CARTESIAN_POINT ( 'NONE',  ( -13.97604488694527625, -13.89961937509977652, 31.87390960531435979 ) ) ;
#34441=CARTESIAN_POINT ( 'NONE',  ( 0.05219959533937995610, -21.53943276465977519, 30.00109039468568284 ) ) ;
#34442=CARTESIAN_POINT ( 'NONE',  ( -13.89961937509977652, 13.97604488694528158, 50.62390960531435979 ) ) ;
#34444=CARTESIAN_POINT ( 'NONE',  ( 9.564922557960805705, 16.46253265017160317, 49.58224293864770260 ) ) ;
#34445=CARTESIAN_POINT ( 'NONE',  ( -0.05219959533907301413, -21.53943276465977519, 22.49890960531436335 ) ) ;
#34446=CARTESIAN_POINT ( 'NONE',  ( 5.823673210054444382, -21.52544592524334988, 65.20942372801901854 ) ) ;
#34447=CARTESIAN_POINT ( 'NONE',  ( -16.52544592524342804, 4.483927247898546575, 111.0405762719810525 ) ) ;
#34448=CARTESIAN_POINT ( 'NONE',  ( -19.02544592524342804, 5.153800228976336051, 116.0405762719810383 ) ) ;
#34449=CARTESIAN_POINT ( 'NONE',  ( -0.05219959533934338120, 16.53943276465976808, 72.50109039468568994 ) ) ;
#34451=CARTESIAN_POINT ( 'NONE',  ( 10.72451020669871369, 18.67979575497193778, 92.08442372801901854 ) ) ;
#34452=CARTESIAN_POINT ( 'NONE',  ( 4.483927247898790824, -16.52544592524335698, 55.20942372801902565 ) ) ;
#34453=CARTESIAN_POINT ( 'NONE',  ( -16.51473224551069308, -9.474510206698971260, 91.66557627198103830 ) ) ;
#34454=CARTESIAN_POINT ( 'NONE',  ( 12.14591786802327356, -12.06949235617739191, 35.62609039468568994 ) ) ;
#34455=CARTESIAN_POINT ( 'NONE',  ( 12.14591786802327356, -12.06949235617739191, 30.62609039468567929 ) ) ;
#34456=CARTESIAN_POINT ( 'NONE',  ( 8.314922557961029526, -14.29746914071037800, 95.41775706135234714 ) ) ;
#34457=CARTESIAN_POINT ( 'NONE',  ( 5.049401038297881783, 19.05341960407617563, 107.2927570613523187 ) ) ;
#34458=CARTESIAN_POINT ( 'NONE',  ( -5.823673210054116645, -21.52544592524344225, 107.2905762719810525 ) ) ;
#34459=CARTESIAN_POINT ( 'NONE',  ( -12.14591786802309592, -12.06949235617757132, 96.87390960531436690 ) ) ;
#34460=CARTESIAN_POINT ( 'NONE',  ( 0.05219959533936267826, -19.03943276465977164, 105.0010903946856615 ) ) ;
#34461=CARTESIAN_POINT ( 'NONE',  ( 0.05219959533934541429, -16.53943276465976808, 75.00109039468568994 ) ) ;
#34463=CARTESIAN_POINT ( 'NONE',  ( 13.89961937509957401, 13.97604488694547697, 66.87609039468567573 ) ) ;
#34464=CARTESIAN_POINT ( 'NONE',  ( 4.483927247898545687, 16.52544592524342804, 49.79057627198102409 ) ) ;
#34465=CARTESIAN_POINT ( 'NONE',  ( -8.314922557960811034, -14.29746914071050412, 47.08224293864770260 ) ) ;
#34466=CARTESIAN_POINT ( 'NONE',  ( 12.14591786802309770, 12.06949235617756955, 94.37390960531436690 ) ) ;
#34467=CARTESIAN_POINT ( 'NONE',  ( -19.03943276465977164, -0.05219959533935918106, 28.75109039468566507 ) ) ;
#34468=CARTESIAN_POINT ( 'NONE',  ( -16.36317988757057407, 7.306389748694917863, 89.09789608363227842 ) ) ;
#34469=CARTESIAN_POINT ( 'NONE',  ( 21.52544592524334988, 5.823673210054432836, 41.45942372801901143 ) ) ;
#34470=CARTESIAN_POINT ( 'NONE',  ( -5.153800228976607833, 19.02544592524334988, 97.70942372801900433 ) ) ;
#34472=CARTESIAN_POINT ( 'NONE',  ( 19.03943276465977164, -0.05219959533909143690, 93.74890960531435269 ) ) ;
#34473=CARTESIAN_POINT ( 'NONE',  ( -19.05341960407611168, -5.049401038298163336, 91.45724293864766707 ) ) ;
#34474=CARTESIAN_POINT ( 'NONE',  ( -15.80617190586745835, -15.72974639402198527, 51.87390960531437401 ) ) ;
#34475=CARTESIAN_POINT ( 'NONE',  ( 4.483927247898545687, 16.52544592524342804, 89.79057627198103830 ) ) ;
#34476=CARTESIAN_POINT ( 'NONE',  ( 5.049401038298161559, -19.05341960407611168, 72.70724293864768129 ) ) ;
#34477=CARTESIAN_POINT ( 'NONE',  ( -19.02544592524342804, 5.153800228976336051, 31.04057627198102409 ) ) ;
#34478=AXIS2_PLACEMENT_3D ( 'NONE', #78214, #89435, #43931 ) ;
#34479=CARTESIAN_POINT ( 'NONE',  ( -18.62759615963255300, -10.81492255796106328, 44.16775706135234714 ) ) ;
#34480=CARTESIAN_POINT ( 'NONE',  ( 15.72974639402176855, 15.80617190586768217, 81.87609039468568994 ) ) ;
#34481=CARTESIAN_POINT ( 'NONE',  ( -19.02544592524342804, 5.153800228976336051, 51.04057627198103120 ) ) ;
#34482=CARTESIAN_POINT ( 'NONE',  ( 14.34966873604972726, -8.224510206698740333, 90.83442372801901854 ) ) ;
#34483=CARTESIAN_POINT ( 'NONE',  ( 10.81492255796106328, -18.62759615963255655, 35.41775706135234003 ) ) ;
#34484=CARTESIAN_POINT ( 'NONE',  ( 18.62759615963255655, 10.81492255796105972, 26.66775706135235424 ) ) ;
#34485=CARTESIAN_POINT ( 'NONE',  ( -9.474510206698720793, -16.51473224551083518, 49.58442372801899722 ) ) ;
#34486=CARTESIAN_POINT ( 'NONE',  ( -13.89961937509977652, 13.97604488694528158, 80.62390960531436690 ) ) ;
#34487=CARTESIAN_POINT ( 'NONE',  ( 19.02544592524334988, 5.153800228976608722, 36.45942372801900433 ) ) ;
#34488=CARTESIAN_POINT ( 'NONE',  ( 21.55341960407619695, -5.719274019375665929, 86.04275706135236135 ) ) ;
#34489=CARTESIAN_POINT ( 'NONE',  ( 15.80617190586746368, 15.72974639402197994, 74.37390960531436690 ) ) ;
#34490=CARTESIAN_POINT ( 'NONE',  ( 0.05219959533910956823, 16.53943276465976808, 44.99890960531435979 ) ) ;
#34491=CARTESIAN_POINT ( 'NONE',  ( -15.80617190586768217, 15.72974639402176855, 93.12609039468568994 ) ) ;
#34492=CARTESIAN_POINT ( 'NONE',  ( 5.049401038297881783, 19.05341960407617563, 27.29275706135232937 ) ) ;
#34493=CARTESIAN_POINT ( 'NONE',  ( 12.14591786802309770, 12.06949235617756955, 69.37390960531436690 ) ) ;
#34494=CARTESIAN_POINT ( 'NONE',  ( 13.97604488694527802, 13.89961937509977652, 29.37390960531435979 ) ) ;
#34495=CARTESIAN_POINT ( 'NONE',  ( -0.05219959533936034679, 19.03943276465977164, 67.50109039468566152 ) ) ;
#34496=CARTESIAN_POINT ( 'NONE',  ( 14.34966873604960469, 8.224510206698951720, 39.16557627198102409 ) ) ;
#34497=CARTESIAN_POINT ( 'NONE',  ( -21.53943276465977519, -0.05219959533937600094, 83.75109039468568994 ) ) ;
#34498=CARTESIAN_POINT ( 'NONE',  ( 13.97604488694527802, 13.89961937509977652, 79.37390960531435269 ) ) ;
#34499=CARTESIAN_POINT ( 'NONE',  ( 5.153800228976615827, -19.02544592524334988, 50.20942372801897591 ) ) ;
#34500=CARTESIAN_POINT ( 'NONE',  ( -0.05219959533907301413, -21.53943276465977519, 62.49890960531436690 ) ) ;
#34501=CARTESIAN_POINT ( 'NONE',  ( 18.62759615963271287, -10.81492255796078972, 113.3322429386476955 ) ) ;
#34502=CARTESIAN_POINT ( 'NONE',  ( 14.29746914071037800, 8.314922557961029526, 21.66775706135235069 ) ) ;
#34503=CARTESIAN_POINT ( 'NONE',  ( 14.29746914071037800, 8.314922557961029526, 71.66775706135234714 ) ) ;
#34504=CARTESIAN_POINT ( 'NONE',  ( 17.26058549869090442, 6.457015423128627418, 63.87745837476070676 ) ) ;
#34505=CARTESIAN_POINT ( 'NONE',  ( 21.53943276465977519, -0.05219959533907433946, 103.7489096053143669 ) ) ;
#34506=CARTESIAN_POINT ( 'NONE',  ( -12.06949235617756955, 12.14591786802309770, 105.6239096053143669 ) ) ;
#34508=CARTESIAN_POINT ( 'NONE',  ( 4.379528057220092307, 16.55341960407617563, 42.29275706135235424 ) ) ;
#34509=CARTESIAN_POINT ( 'NONE',  ( -21.52544592524343514, 5.823673210054127303, 56.04057627198102409 ) ) ;
#34510=CARTESIAN_POINT ( 'NONE',  ( -16.52544592524335698, -4.483927247898792601, 108.9594237280190185 ) ) ;
#34511=CARTESIAN_POINT ( 'NONE',  ( 5.153800228976335163, 19.02544592524342804, 34.79057627198102409 ) ) ;
#34512=CARTESIAN_POINT ( 'NONE',  ( 16.53943276465976808, 0.05219959533934440121, 66.25109039468567573 ) ) ;
#34513=CARTESIAN_POINT ( 'NONE',  ( -19.02544592524334988, -5.153800228976617603, 63.95942372801899012 ) ) ;
#34514=CARTESIAN_POINT ( 'NONE',  ( 5.823673210054444382, -21.52544592524334988, 45.20942372801901854 ) ) ;
#34515=CARTESIAN_POINT ( 'NONE',  ( 10.81492255796078972, 18.62759615963270932, 54.58224293864769550 ) ) ;
#34516=CARTESIAN_POINT ( 'NONE',  ( 4.379528057220092307, 16.55341960407617563, 97.29275706135234714 ) ) ;
#34517=CARTESIAN_POINT ( 'NONE',  ( -18.62759615963255300, -10.81492255796106328, 84.16775706135234714 ) ) ;
#34518=CARTESIAN_POINT ( 'NONE',  ( -21.52544592524343514, 5.823673210054127303, 51.04057627198103120 ) ) ;
#34519=CARTESIAN_POINT ( 'NONE',  ( 21.52544592524344225, -5.823673210054117533, 33.54057627198102409 ) ) ;
#34520=CARTESIAN_POINT ( 'NONE',  ( -12.06949235617739369, -12.14591786802326823, 74.37609039468568994 ) ) ;
#34521=CARTESIAN_POINT ( 'NONE',  ( -15.80617190586745835, -15.72974639402198527, 51.87390960531437401 ) ) ;
#34523=CARTESIAN_POINT ( 'NONE',  ( 19.03943276465977164, -0.05219959533909143690, 103.7489096053143669 ) ) ;
#34524=CARTESIAN_POINT ( 'NONE',  ( 17.50000000000000000, 4.189786006557876696, 22.00000000000000711 ) ) ;
#34525=CARTESIAN_POINT ( 'NONE',  ( -19.03943276465977164, 0.05219959533909376836, 31.24890960531435979 ) ) ;
#34526=CARTESIAN_POINT ( 'NONE',  ( -21.55341960407610458, -5.719274019375992779, 56.45724293864768839 ) ) ;
#34527=CARTESIAN_POINT ( 'NONE',  ( -0.05219959533934338120, 16.53943276465976808, 87.50109039468568994 ) ) ;
#34528=CARTESIAN_POINT ( 'NONE',  ( 15.72974639402176855, 15.80617190586768217, 41.87609039468568284 ) ) ;
#34529=CARTESIAN_POINT ( 'NONE',  ( 5.049401038297881783, 19.05341960407617563, 102.2927570613523045 ) ) ;
#34530=CARTESIAN_POINT ( 'NONE',  ( 16.55341960407611168, 4.379528057220329451, 108.9572429386476955 ) ) ;
#34531=CARTESIAN_POINT ( 'NONE',  ( -9.564922557961040184, 16.46253265017147172, 112.9177570613523329 ) ) ;
#34533=CARTESIAN_POINT ( 'NONE',  ( -13.89961937509977652, 13.97604488694528158, 45.62390960531433848 ) ) ;
#34535=CARTESIAN_POINT ( 'NONE',  ( 16.46253265017160672, -9.564922557960803928, 93.33224293864769550 ) ) ;
#34536=CARTESIAN_POINT ( 'NONE',  ( -0.05219959533934338120, 16.53943276465976808, 72.50109039468568994 ) ) ;
#34537=CARTESIAN_POINT ( 'NONE',  ( -21.53943276465977519, -0.05219959533937600094, 103.7510903946857042 ) ) ;
#34538=CARTESIAN_POINT ( 'NONE',  ( -10.81492255796078084, -18.62759615963271287, 62.08224293864769550 ) ) ;
#34539=CARTESIAN_POINT ( 'NONE',  ( 4.379528057220092307, 16.55341960407617563, 92.29275706135236135 ) ) ;
#34540=CARTESIAN_POINT ( 'NONE',  ( -16.51473224551082808, 9.474510206698731452, 83.33442372801899012 ) ) ;
#34541=CARTESIAN_POINT ( 'NONE',  ( 19.03943276465977164, -0.05219959533909143690, 33.74890960531435979 ) ) ;
#34542=CARTESIAN_POINT ( 'NONE',  ( 5.049401038298161559, -19.05341960407611168, 82.70724293864770971 ) ) ;
#34543=CARTESIAN_POINT ( 'NONE',  ( 19.03943276465977164, -0.05219959533909143690, 28.74890960531435624 ) ) ;
#34544=CARTESIAN_POINT ( 'NONE',  ( 13.97604488694548053, -13.89961937509957401, 70.62609039468567573 ) ) ;
#34546=CARTESIAN_POINT ( 'NONE',  ( -19.03943276465977164, 0.05219959533909376836, 106.2489096053143669 ) ) ;
#34547=CARTESIAN_POINT ( 'NONE',  ( 0.05219959533910956823, 16.53943276465976808, 59.99890960531436690 ) ) ;
#34548=CARTESIAN_POINT ( 'NONE',  ( 15.72974639402199770, -15.80617190586745480, 58.12390960531435979 ) ) ;
#34550=CARTESIAN_POINT ( 'NONE',  ( 0.05219959533936267826, -19.03943276465977164, 30.00109039468566863 ) ) ;
#34552=CARTESIAN_POINT ( 'NONE',  ( -0.05219959533909027116, -19.03943276465977164, 62.49890960531435979 ) ) ;
#34553=CARTESIAN_POINT ( 'NONE',  ( 13.97604488694527802, 13.89961937509977652, 69.37390960531436690 ) ) ;
#34554=CARTESIAN_POINT ( 'NONE',  ( 4.379528057220092307, 16.55341960407617563, 47.29275706135234003 ) ) ;
#34555=CARTESIAN_POINT ( 'NONE',  ( -19.25176906914649777, -5.499999999999800160, 100.9992726424227669 ) ) ;
#34557=CARTESIAN_POINT ( 'NONE',  ( 16.52544592524335698, 4.483927247898782831, 71.45942372801901854 ) ) ;
#34559=CARTESIAN_POINT ( 'NONE',  ( -8.314922557961024197, 14.29746914071037800, 62.91775706135236135 ) ) ;
#34561=( BOUNDED_CURVE ( )  B_SPLINE_CURVE ( 2, ( #196798, #85593, #58266, #165455, #22936, #84582, #73451, #57279, #40089, #118953, #24952, #70439, #147280 ),
 .UNSPECIFIED., .F., .T. ) 
 B_SPLINE_CURVE_WITH_KNOTS ( ( 3, 2, 2, 2, 2, 2, 3 ),
 ( 0.7656340109859774978, 0.7675438596491228616, 0.7719298245614034659, 0.7763157894736841813, 0.7807017543859648967, 0.7850877192982456121, 0.7870432477834813367 ),
 .UNSPECIFIED. ) 
 CURVE ( )  GEOMETRIC_REPRESENTATION_ITEM ( )  RATIONAL_B_SPLINE_CURVE ( ( 0.9832469066685285419, 0.9851625545550100060, 1.000000000000000000, 0.9659258262890683122, 1.000000000000000000, 0.9659258262890683122, 1.000000000000000000, 0.9659258262890683122, 1.000000000000000000, 0.9659258262890683122, 1.000000000000000000, 0.9848076720550078544, 0.9831626618144001517 ) ) 
 REPRESENTATION_ITEM ( '' )  );
#34562=CARTESIAN_POINT ( 'NONE',  ( -8.224510206698735004, -14.34966873604973081, 44.58442372801901854 ) ) ;
#34563=CARTESIAN_POINT ( 'NONE',  ( -9.474510206698964154, 16.51473224551069663, 55.41557627198103120 ) ) ;
#34565=CARTESIAN_POINT ( 'NONE',  ( 15.72974639402176855, 15.80617190586768217, 56.87609039468568994 ) ) ;
#34566=CARTESIAN_POINT ( 'NONE',  ( -13.97604488694547697, 13.89961937509957934, 58.12609039468566863 ) ) ;
#34567=CARTESIAN_POINT ( 'NONE',  ( -18.67979575497193778, 10.72451020669871902, 98.33442372801901854 ) ) ;
#34568=CARTESIAN_POINT ( 'NONE',  ( -19.03943276465977164, 0.05219959533909376836, 31.24890960531435979 ) ) ;
#34570=CARTESIAN_POINT ( 'NONE',  ( -15.72974639402197994, 15.80617190586746368, 55.62390960531436690 ) ) ;
#34571=CARTESIAN_POINT ( 'NONE',  ( -13.97604488694527625, -13.89961937509977652, 106.8739096053143669 ) ) ;
#34572=CARTESIAN_POINT ( 'NONE',  ( 12.06949235617757843, -12.14591786802309237, 108.1239096053143811 ) ) ;
#34573=CARTESIAN_POINT ( 'NONE',  ( 14.29746914071037800, 8.314922557961029526, 41.66775706135235424 ) ) ;
#34574=CARTESIAN_POINT ( 'NONE',  ( 12.06949235617757843, -12.14591786802309237, 33.12390960531435979 ) ) ;
#34575=ORIENTED_EDGE ( 'NONE', *, *, #196054, .T. ) ;
#34576=CARTESIAN_POINT ( 'NONE',  ( -10.72451020669898014, 18.67979575497178502, 105.4155762719810383 ) ) ;
#34577=CARTESIAN_POINT ( 'NONE',  ( 4.483927247898545687, 16.52544592524342804, 39.79057627198103830 ) ) ;
#34578=CARTESIAN_POINT ( 'NONE',  ( 5.153800228976335163, 19.02544592524342804, 114.7905762719810241 ) ) ;
#34579=CARTESIAN_POINT ( 'NONE',  ( -19.03943276465977164, -0.05219959533935918106, 88.75109039468567573 ) ) ;
#34580=CARTESIAN_POINT ( 'NONE',  ( 9.474510206698729675, 16.51473224551082808, 32.08442372801900433 ) ) ;
#34581=CARTESIAN_POINT ( 'NONE',  ( -12.14591786802309592, -12.06949235617757132, 36.87390960531435979 ) ) ;
#34582=CARTESIAN_POINT ( 'NONE',  ( 5.823673210054125526, 21.52544592524343514, 99.79057627198103830 ) ) ;
#34583=CARTESIAN_POINT ( 'NONE',  ( -10.81492255796078084, -18.62759615963271287, 57.08224293864769550 ) ) ;
#34584=CARTESIAN_POINT ( 'NONE',  ( -13.97604488694527625, -13.89961937509977652, 81.87390960531436690 ) ) ;
#34585=CARTESIAN_POINT ( 'NONE',  ( -4.379528057220328563, 16.55341960407611168, 40.20724293864769550 ) ) ;
#34586=CARTESIAN_POINT ( 'NONE',  ( 5.049401038298161559, -19.05341960407611168, 87.70724293864769550 ) ) ;
#34587=CARTESIAN_POINT ( 'NONE',  ( 19.52851543214743302, 5.500000000000026645, 57.89357721762583964 ) ) ;
#34588=CARTESIAN_POINT ( 'NONE',  ( 0.05219959533936267826, -19.03943276465977164, 40.00109039468566152 ) ) ;
#34589=CARTESIAN_POINT ( 'NONE',  ( 18.62759615963271287, -10.81492255796078972, 83.33224293864769550 ) ) ;
#34590=CARTESIAN_POINT ( 'NONE',  ( -16.53943276465976808, 0.05219959533911058130, 106.2489096053143811 ) ) ;
#34591=CARTESIAN_POINT ( 'NONE',  ( 21.53943276465977519, 0.05219959533937863772, 36.25109039468567573 ) ) ;
#34593=CARTESIAN_POINT ( 'NONE',  ( -8.224510206698735004, -14.34966873604973081, 104.5844237280190185 ) ) ;
#34594=CARTESIAN_POINT ( 'NONE',  ( 5.153800228976335163, 19.02544592524342804, 39.79057627198100988 ) ) ;
#34595=CARTESIAN_POINT ( 'NONE',  ( -5.049401038298153566, 19.05341960407611168, 90.20724293864766707 ) ) ;
#34597=CARTESIAN_POINT ( 'NONE',  ( -19.03943276465977164, 0.05219959533909376836, 26.24890960531435624 ) ) ;
#34598=CARTESIAN_POINT ( 'NONE',  ( 12.06949235617757843, -12.14591786802309237, 48.12390960531436690 ) ) ;
#34599=CARTESIAN_POINT ( 'NONE',  ( 18.62759615963255655, 10.81492255796105972, 76.66775706135234714 ) ) ;
#34601=CARTESIAN_POINT ( 'NONE',  ( -16.52544592524335698, -4.483927247898792601, 73.95942372801901854 ) ) ;
#34602=CARTESIAN_POINT ( 'NONE',  ( 5.049401038298161559, -19.05341960407611168, 62.70724293864769550 ) ) ;
#34603=CARTESIAN_POINT ( 'NONE',  ( -5.049401038298153566, 19.05341960407611168, 70.20724293864769550 ) ) ;
#34605=CARTESIAN_POINT ( 'NONE',  ( -21.53943276465977519, -0.05219959533937600094, 108.7510903946857042 ) ) ;
#34606=CARTESIAN_POINT ( 'NONE',  ( -14.34966873604972548, 8.224510206698743886, 73.33442372801901854 ) ) ;
#34607=CARTESIAN_POINT ( 'NONE',  ( 10.72451020669871369, 18.67979575497193778, 97.08442372801904696 ) ) ;
#34608=CARTESIAN_POINT ( 'NONE',  ( 5.049401038298161559, -19.05341960407611168, 67.70724293864769550 ) ) ;
#34609=CARTESIAN_POINT ( 'NONE',  ( -10.72451020669898014, 18.67979575497178502, 35.41557627198102409 ) ) ;
#34610=CARTESIAN_POINT ( 'NONE',  ( 19.02544592524334988, 5.153800228976608722, 111.4594237280190043 ) ) ;
#34611=CARTESIAN_POINT ( 'NONE',  ( -5.719274019375665041, -21.55341960407619695, 74.79275706135234714 ) ) ;
#34612=CARTESIAN_POINT ( 'NONE',  ( 4.483927247898790824, -16.52544592524335698, 55.20942372801902565 ) ) ;
#34613=CARTESIAN_POINT ( 'NONE',  ( -5.823673210054116645, -21.52544592524344225, 97.29057627198105251 ) ) ;
#34614=CARTESIAN_POINT ( 'NONE',  ( -19.05341960407617563, 5.049401038297882671, 93.54275706135234714 ) ) ;
#34615=CARTESIAN_POINT ( 'NONE',  ( 13.89961937509977652, -13.97604488694527269, 83.12390960531436690 ) ) ;
#34616=CARTESIAN_POINT ( 'NONE',  ( -16.51473224551082808, 9.474510206698731452, 108.3344237280190043 ) ) ;
#34617=CARTESIAN_POINT ( 'NONE',  ( -9.564922557961040184, 16.46253265017147172, 112.9177570613523329 ) ) ;
#34618=CARTESIAN_POINT ( 'NONE',  ( 16.55341960407611168, 4.379528057220329451, 68.95724293864769550 ) ) ;
#34619=CARTESIAN_POINT ( 'NONE',  ( -14.29746914071037622, -8.314922557961029526, 74.16775706135231871 ) ) ;
#34620=CARTESIAN_POINT ( 'NONE',  ( -15.72974639402176322, -15.80617190586768395, 19.37609039468568639 ) ) ;
#34621=CARTESIAN_POINT ( 'NONE',  ( -9.474510206698964154, 16.51473224551069663, 50.41557627198102409 ) ) ;
#34622=CARTESIAN_POINT ( 'NONE',  ( 5.049401038298161559, -19.05341960407611168, 57.70724293864769550 ) ) ;
#34623=CARTESIAN_POINT ( 'NONE',  ( -8.224510206698735004, -14.34966873604973081, 74.58442372801901854 ) ) ;
#34626=CARTESIAN_POINT ( 'NONE',  ( -16.51473224551082808, 9.474510206698731452, 23.33442372801900078 ) ) ;
#34627=CARTESIAN_POINT ( 'NONE',  ( 16.51473224551069308, 9.474510206698969483, 34.16557627198102409 ) ) ;
#34629=CARTESIAN_POINT ( 'NONE',  ( 9.564922557961047289, -16.46253265017146816, 105.4177570613523471 ) ) ;
#34630=CARTESIAN_POINT ( 'NONE',  ( -19.03943276465977164, -0.05219959533935918106, 38.75109039468566152 ) ) ;
#34631=CARTESIAN_POINT ( 'NONE',  ( 4.483927247898790824, -16.52544592524335698, 35.20942372801901854 ) ) ;
#34632=CARTESIAN_POINT ( 'NONE',  ( 9.564922557960805705, 16.46253265017160317, 44.58224293864769550 ) ) ;
#34633=CARTESIAN_POINT ( 'NONE',  ( 0.05219959533909260263, 19.03943276465977164, 69.99890960531435269 ) ) ;
#34634=CARTESIAN_POINT ( 'NONE',  ( -5.823673210054116645, -21.52544592524344225, 87.29057627198103830 ) ) ;
#34636=CARTESIAN_POINT ( 'NONE',  ( -13.89961937509977652, 13.97604488694528158, 50.62390960531435979 ) ) ;
#34637=CARTESIAN_POINT ( 'NONE',  ( -17.49999999999999645, 5.499999999999992895, 93.71769037696437010 ) ) ;
#34638=CARTESIAN_POINT ( 'NONE',  ( -19.02544592524334988, -5.153800228976617603, 103.9594237280190043 ) ) ;
#34639=CARTESIAN_POINT ( 'NONE',  ( 0.05219959533910956823, 16.53943276465976808, 69.99890960531435269 ) ) ;
#34641=CARTESIAN_POINT ( 'NONE',  ( 13.89961937509957401, 13.97604488694547697, 21.87609039468566152 ) ) ;
#34642=CARTESIAN_POINT ( 'NONE',  ( 12.06949235617757843, -12.14591786802309237, 58.12390960531435979 ) ) ;
#34643=CARTESIAN_POINT ( 'NONE',  ( -10.81492255796105439, 18.62759615963255655, 82.91775706135234714 ) ) ;
#34644=CARTESIAN_POINT ( 'NONE',  ( -19.03943276465977164, 0.05219959533909376836, 26.24890960531435624 ) ) ;
#34645=CARTESIAN_POINT ( 'NONE',  ( 10.81492255796106328, -18.62759615963255655, 85.41775706135236135 ) ) ;
#34646=CARTESIAN_POINT ( 'NONE',  ( 4.379528057220339221, -16.55341960407611168, 32.70724293864770260 ) ) ;
#34647=CARTESIAN_POINT ( 'NONE',  ( 21.52544592524334988, 5.823673210054432836, 71.45942372801901854 ) ) ;
#34648=CARTESIAN_POINT ( 'NONE',  ( 0.05219959533909260263, 19.03943276465977164, 79.99890960531436690 ) ) ;
#34649=CARTESIAN_POINT ( 'NONE',  ( -21.52544592524334988, -5.823673210054445271, 38.95942372801901854 ) ) ;
#34650=CARTESIAN_POINT ( 'NONE',  ( -5.049401038298153566, 19.05341960407611168, 75.20724293864769550 ) ) ;
#34651=CARTESIAN_POINT ( 'NONE',  ( 16.52544592524342804, -4.483927247898539470, 88.54057627198103830 ) ) ;
#34652=CARTESIAN_POINT ( 'NONE',  ( -4.483927247898539470, -16.52544592524342804, 57.29057627198103120 ) ) ;
#34653=CARTESIAN_POINT ( 'NONE',  ( -18.62759615963270932, 10.81492255796079327, 75.83224293864769550 ) ) ;
#34654=CARTESIAN_POINT ( 'NONE',  ( -16.46253265017160317, 9.564922557960807481, 70.83224293864770971 ) ) ;
#34655=CARTESIAN_POINT ( 'NONE',  ( 5.719274019375991003, -21.55341960407610458, 82.70724293864770971 ) ) ;
#34656=CARTESIAN_POINT ( 'NONE',  ( -9.474510206698720793, -16.51473224551083518, 79.58442372801899012 ) ) ;
#34657=CARTESIAN_POINT ( 'NONE',  ( -18.22780087662122028, 5.500000000000031086, 38.51540105326107266 ) ) ;
#34658=CARTESIAN_POINT ( 'NONE',  ( 16.52544592524342804, -4.483927247898539470, 78.54057627198103830 ) ) ;
#34660=CARTESIAN_POINT ( 'NONE',  ( 5.823673210054125526, 21.52544592524343514, 59.79057627198103120 ) ) ;
#34661=DIRECTION ( 'NONE',  ( -0.000000000000000000, -0.000000000000000000, 1.000000000000000000 ) ) ;
#34662=CARTESIAN_POINT ( 'NONE',  ( -8.224510206698735004, -14.34966873604973081, 104.5844237280190185 ) ) ;
#34664=CARTESIAN_POINT ( 'NONE',  ( -16.46253265017146816, -9.564922557961047289, 99.16775706135233293 ) ) ;
#34665=CARTESIAN_POINT ( 'NONE',  ( -16.53943276465976808, 0.05219959533911058130, 66.24890960531436690 ) ) ;
#34667=CARTESIAN_POINT ( 'NONE',  ( 9.564922557960805705, 16.46253265017160317, 64.58224293864769550 ) ) ;
#34668=CARTESIAN_POINT ( 'NONE',  ( 16.55341960407611168, 4.379528057220329451, 48.95724293864770971 ) ) ;
#34669=CARTESIAN_POINT ( 'NONE',  ( -5.049401038298153566, 19.05341960407611168, 95.20724293864770971 ) ) ;
#34670=CARTESIAN_POINT ( 'NONE',  ( 5.049401038297881783, 19.05341960407617563, 87.29275706135234714 ) ) ;
#34671=CARTESIAN_POINT ( 'NONE',  ( -9.564922557960796823, -16.46253265017161027, 72.08224293864770971 ) ) ;
#34672=CARTESIAN_POINT ( 'NONE',  ( -9.474510206698964154, 16.51473224551069663, 85.41557627198102409 ) ) ;
#34673=CARTESIAN_POINT ( 'NONE',  ( 5.153800228976335163, 19.02544592524342804, 84.79057627198099567 ) ) ;
#34674=CARTESIAN_POINT ( 'NONE',  ( 15.72974639402199770, -15.80617190586745480, 58.12390960531435979 ) ) ;
#34675=CARTESIAN_POINT ( 'NONE',  ( -8.224510206698735004, -14.34966873604973081, 54.58442372801901143 ) ) ;
#34677=CARTESIAN_POINT ( 'NONE',  ( -13.89961937509977652, 13.97604488694528158, 50.62390960531435979 ) ) ;
#34678=CARTESIAN_POINT ( 'NONE',  ( 10.72451020669898902, -18.67979575497178502, 72.91557627198103830 ) ) ;
#34679=CARTESIAN_POINT ( 'NONE',  ( 13.89961937509957401, 13.97604488694547697, 96.87609039468566152 ) ) ;
#34680=CARTESIAN_POINT ( 'NONE',  ( -16.55341960407611168, -4.379528057220339221, 21.45724293864769550 ) ) ;
#34681=CARTESIAN_POINT ( 'NONE',  ( 10.72451020669871369, 18.67979575497193778, 52.08442372801901854 ) ) ;
#34683=CARTESIAN_POINT ( 'NONE',  ( -13.89961937509957401, -13.97604488694547875, 39.37609039468566152 ) ) ;
#34684=CARTESIAN_POINT ( 'NONE',  ( 12.14591786802327356, -12.06949235617739191, 55.62609039468568284 ) ) ;
#34685=CARTESIAN_POINT ( 'NONE',  ( 16.52544592524335698, 4.483927247898782831, 91.45942372801901854 ) ) ;
#34686=CARTESIAN_POINT ( 'NONE',  ( 19.26498983726239800, -5.499999999999598543, 43.05319577422001487 ) ) ;
#34687=CARTESIAN_POINT ( 'NONE',  ( 16.52544592524335698, 4.483927247898782831, 86.45942372801901854 ) ) ;
#34688=CARTESIAN_POINT ( 'NONE',  ( -8.224510206698735004, -14.34966873604973081, 34.58442372801900433 ) ) ;
#34689=CARTESIAN_POINT ( 'NONE',  ( -0.05219959533909027116, -19.03943276465977164, 42.49890960531435269 ) ) ;
#34690=CARTESIAN_POINT ( 'NONE',  ( 19.05341960407611168, 5.049401038298154454, 53.95724293864770260 ) ) ;
#34691=CARTESIAN_POINT ( 'NONE',  ( 13.97604488694527802, 13.89961937509977652, 64.37390960531436690 ) ) ;
#34692=CARTESIAN_POINT ( 'NONE',  ( 15.72974639402176855, 15.80617190586768217, 56.87609039468568994 ) ) ;
#34693=CARTESIAN_POINT ( 'NONE',  ( 8.314922557961029526, -14.29746914071037800, 45.41775706135234003 ) ) ;
#34694=CARTESIAN_POINT ( 'NONE',  ( -4.483927247898539470, -16.52544592524342804, 22.29057627198102765 ) ) ;
#34695=CARTESIAN_POINT ( 'NONE',  ( -5.049401038298153566, 19.05341960407611168, 30.20724293864768839 ) ) ;
#34696=CARTESIAN_POINT ( 'NONE',  ( -19.03943276465977164, -0.05219959533935918106, 18.75109039468567218 ) ) ;
#34697=CARTESIAN_POINT ( 'NONE',  ( 16.55341960407618274, -4.379528057220086978, 31.04275706135234714 ) ) ;
#34698=CARTESIAN_POINT ( 'NONE',  ( -16.46253265017146816, -9.564922557961047289, 84.16775706135233293 ) ) ;
#34699=CARTESIAN_POINT ( 'NONE',  ( 14.34966873604960469, 8.224510206698951720, 84.16557627198103830 ) ) ;
#34700=CARTESIAN_POINT ( 'NONE',  ( 19.02544592524343514, -5.153800228976328945, 33.54057627198102409 ) ) ;
#34701=CARTESIAN_POINT ( 'NONE',  ( -16.46253265017146816, -9.564922557961047289, 74.16775706135234714 ) ) ;
#34702=CARTESIAN_POINT ( 'NONE',  ( 16.88567814943163015, -6.947325034625690954, 91.20998877347419409 ) ) ;
#34703=CARTESIAN_POINT ( 'NONE',  ( -15.80617190586768217, 15.72974639402176855, 83.12609039468568994 ) ) ;
#34704=CARTESIAN_POINT ( 'NONE',  ( 16.52544592524335698, 4.483927247898782831, 41.45942372801901143 ) ) ;
#34705=CARTESIAN_POINT ( 'NONE',  ( 16.31925111598457434, 7.325300261831481308, 37.33575461032752685 ) ) ;
#34706=CARTESIAN_POINT ( 'NONE',  ( -10.72451020669898014, 18.67979575497178502, 35.41557627198102409 ) ) ;
#34707=CARTESIAN_POINT ( 'NONE',  ( -8.314922557961024197, 14.29746914071037800, 22.91775706135235069 ) ) ;
#34708=CARTESIAN_POINT ( 'NONE',  ( -0.05219959533909027116, -19.03943276465977164, 27.49890960531435624 ) ) ;
#34709=CARTESIAN_POINT ( 'NONE',  ( -19.05341960407617563, 5.049401038297882671, 28.54275706135232937 ) ) ;
#34711=CARTESIAN_POINT ( 'NONE',  ( 0.05219959533909260263, 19.03943276465977164, 39.99890960531436690 ) ) ;
#34713=CARTESIAN_POINT ( 'NONE',  ( 16.51473224551069308, 9.474510206698969483, 69.16557627198102409 ) ) ;
#34714=CARTESIAN_POINT ( 'NONE',  ( -19.52217212775660116, 5.499999999999917399, 99.93993709005258097 ) ) ;
#34715=CARTESIAN_POINT ( 'NONE',  ( 13.97604488694548053, -13.89961937509957401, 25.62609039468566507 ) ) ;
#34716=CARTESIAN_POINT ( 'NONE',  ( -14.34966873604960291, -8.224510206698953496, 31.66557627198102054 ) ) ;
#34717=CARTESIAN_POINT ( 'NONE',  ( -16.46253265017160317, 9.564922557960807481, 40.83224293864769550 ) ) ;
#34718=CARTESIAN_POINT ( 'NONE',  ( -9.564922557960796823, -16.46253265017161027, 87.08224293864769550 ) ) ;
#34719=CARTESIAN_POINT ( 'NONE',  ( 10.81492255796106328, -18.62759615963255655, 65.41775706135234714 ) ) ;
#34720=CARTESIAN_POINT ( 'NONE',  ( 5.153800228976335163, 19.02544592524342804, 44.79057627198103830 ) ) ;
#34721=CARTESIAN_POINT ( 'NONE',  ( 18.67979575497194134, -10.72451020669871369, 60.83442372801901854 ) ) ;
#34722=CARTESIAN_POINT ( 'NONE',  ( 10.81492255796078972, 18.62759615963270932, 29.58224293864769905 ) ) ;
#34723=CARTESIAN_POINT ( 'NONE',  ( -13.97604488694527625, -13.89961937509977652, 36.87390960531436690 ) ) ;
#34724=CARTESIAN_POINT ( 'NONE',  ( 21.52544592524334988, 5.823673210054432836, 21.45942372801901499 ) ) ;
#34725=CARTESIAN_POINT ( 'NONE',  ( 9.564922557961047289, -16.46253265017146816, 45.41775706135232582 ) ) ;
#34726=CARTESIAN_POINT ( 'NONE',  ( -4.483927247898539470, -16.52544592524342804, 112.2905762719810241 ) ) ;
#34727=CARTESIAN_POINT ( 'NONE',  ( -19.02544592524342804, 5.153800228976336051, 61.04057627198103120 ) ) ;
#34728=CARTESIAN_POINT ( 'NONE',  ( -9.564922557961040184, 16.46253265017147172, 112.9177570613523329 ) ) ;
#34729=CARTESIAN_POINT ( 'NONE',  ( -8.224510206698948167, 14.34966873604960824, 80.41557627198103830 ) ) ;
#34730=CARTESIAN_POINT ( 'NONE',  ( 9.564922557960805705, 16.46253265017160317, 114.5822429386476955 ) ) ;
#34731=CARTESIAN_POINT ( 'NONE',  ( 19.03943276465977164, 0.05219959533936151252, 106.2510903946856615 ) ) ;
#34732=CARTESIAN_POINT ( 'NONE',  ( -21.53943276465977519, 0.05219959533907696930, 106.2489096053143811 ) ) ;
#34733=CARTESIAN_POINT ( 'NONE',  ( -5.823673210054431948, 21.52544592524334988, 62.70942372801902565 ) ) ;
#34734=CARTESIAN_POINT ( 'NONE',  ( -16.55341960407617563, 4.379528057220093196, 58.54275706135235424 ) ) ;
#34735=CARTESIAN_POINT ( 'NONE',  ( 8.314922557961029526, -14.29746914071037800, 60.41775706135235424 ) ) ;
#34736=CARTESIAN_POINT ( 'NONE',  ( -10.72451020669898014, 18.67979575497178502, 50.41557627198103120 ) ) ;
#34737=CARTESIAN_POINT ( 'NONE',  ( 19.02544592524343514, -5.153800228976328945, 48.54057627198103120 ) ) ;
#34738=CARTESIAN_POINT ( 'NONE',  ( -14.29746914071037622, -8.314922557961029526, 69.16775706135234714 ) ) ;
#34739=CARTESIAN_POINT ( 'NONE',  ( -10.81492255796078084, -18.62759615963271287, 102.0822429386476955 ) ) ;
#34740=CARTESIAN_POINT ( 'NONE',  ( -14.34966873604960291, -8.224510206698953496, 56.66557627198103830 ) ) ;
#34741=CARTESIAN_POINT ( 'NONE',  ( -13.97604488694527625, -13.89961937509977652, 66.87390960531436690 ) ) ;
#34742=CARTESIAN_POINT ( 'NONE',  ( 16.52544592524335698, 4.483927247898782831, 71.45942372801901854 ) ) ;
#34743=CARTESIAN_POINT ( 'NONE',  ( 4.379528057220092307, 16.55341960407617563, 22.29275706135235069 ) ) ;
#34744=CARTESIAN_POINT ( 'NONE',  ( -15.80617190586745835, -15.72974639402198527, 101.8739096053143811 ) ) ;
#34745=CARTESIAN_POINT ( 'NONE',  ( -4.379528057220328563, 16.55341960407611168, 45.20724293864769550 ) ) ;
#34747=CARTESIAN_POINT ( 'NONE',  ( 19.48894818550245844, -5.499999999999908518, 92.60307310435240424 ) ) ;
#34748=CARTESIAN_POINT ( 'NONE',  ( 15.80617190586746368, 15.72974639402197994, 84.37390960531438111 ) ) ;
#34749=CARTESIAN_POINT ( 'NONE',  ( 0.05219959533910956823, 16.53943276465976808, 29.99890960531435979 ) ) ;
#34750=ORIENTED_EDGE ( 'NONE', *, *, #26227, .F. ) ;
#34752=CARTESIAN_POINT ( 'NONE',  ( 10.72451020669898902, -18.67979575497178502, 97.91557627198103830 ) ) ;
#34753=CARTESIAN_POINT ( 'NONE',  ( 19.05341960407611168, 5.049401038298154454, 103.9572429386476671 ) ) ;
#34754=CARTESIAN_POINT ( 'NONE',  ( -0.05219959533937732626, 21.53943276465977519, 27.50109039468567929 ) ) ;
#34755=CARTESIAN_POINT ( 'NONE',  ( -8.224510206698948167, 14.34966873604960824, 35.41557627198102409 ) ) ;
#34756=CARTESIAN_POINT ( 'NONE',  ( 16.55341960407618274, -4.379528057220086978, 46.04275706135234714 ) ) ;
#34758=CARTESIAN_POINT ( 'NONE',  ( 5.049401038298161559, -19.05341960407611168, 47.70724293864770260 ) ) ;
#34759=CARTESIAN_POINT ( 'NONE',  ( -9.564922557961040184, 16.46253265017147172, 52.91775706135233293 ) ) ;
#34760=CARTESIAN_POINT ( 'NONE',  ( -16.46253265017160317, 9.564922557960807481, 80.83224293864769550 ) ) ;
#34763=CARTESIAN_POINT ( 'NONE',  ( 10.81492255796078972, 18.62759615963270932, 29.58224293864769905 ) ) ;
#34765=CARTESIAN_POINT ( 'NONE',  ( 8.224510206698742110, 14.34966873604972548, 22.08442372801901143 ) ) ;
#34766=CARTESIAN_POINT ( 'NONE',  ( 13.97604488694548053, -13.89961937509957401, 55.62609039468566863 ) ) ;
#34767=CARTESIAN_POINT ( 'NONE',  ( -10.81492255796078084, -18.62759615963271287, 107.0822429386476955 ) ) ;
#34768=CARTESIAN_POINT ( 'NONE',  ( 0.05219959533910956823, 16.53943276465976808, 29.99890960531435979 ) ) ;
#34769=CARTESIAN_POINT ( 'NONE',  ( -5.153800228976328057, -19.02544592524343514, 82.29057627198103830 ) ) ;
#34770=CARTESIAN_POINT ( 'NONE',  ( 5.823673210054125526, 21.52544592524343514, 54.79057627198104541 ) ) ;
#34771=CARTESIAN_POINT ( 'NONE',  ( 15.80617190586746368, 15.72974639402197994, 89.37390960531435269 ) ) ;
#34772=CARTESIAN_POINT ( 'NONE',  ( -14.34966873604972548, 8.224510206698743886, 28.33442372801902209 ) ) ;
#34773=CARTESIAN_POINT ( 'NONE',  ( 21.55341960407610458, 5.719274019375980345, 28.95724293864769905 ) ) ;
#34774=CARTESIAN_POINT ( 'NONE',  ( -0.05219959533937732626, 21.53943276465977519, 92.50109039468567573 ) ) ;
#34775=CARTESIAN_POINT ( 'NONE',  ( 19.02544592524343514, -5.153800228976328945, 73.54057627198103830 ) ) ;
#34777=CARTESIAN_POINT ( 'NONE',  ( 19.05341960407611168, 5.049401038298154454, 28.95724293864769550 ) ) ;
#34778=CARTESIAN_POINT ( 'NONE',  ( -9.564922557960796823, -16.46253265017161027, 87.08224293864769550 ) ) ;
#34779=CARTESIAN_POINT ( 'NONE',  ( -12.06949235617756955, 12.14591786802309770, 105.6239096053143669 ) ) ;
#34780=CARTESIAN_POINT ( 'NONE',  ( 9.474510206698729675, 16.51473224551082808, 107.0844237280190043 ) ) ;
#34782=CARTESIAN_POINT ( 'NONE',  ( 9.564922557960805705, 16.46253265017160317, 69.58224293864770971 ) ) ;
#34784=CARTESIAN_POINT ( 'NONE',  ( -5.823673210054431948, 21.52544592524334988, 97.70942372801904696 ) ) ;
#34785=CARTESIAN_POINT ( 'NONE',  ( 19.05341960407611168, 5.049401038298154454, 113.9572429386477097 ) ) ;
#34786=CARTESIAN_POINT ( 'NONE',  ( -0.05219959533934338120, 16.53943276465976808, 92.50109039468567573 ) ) ;
#34788=CARTESIAN_POINT ( 'NONE',  ( -9.564922557961040184, 16.46253265017147172, 62.91775706135233293 ) ) ;
#34789=CARTESIAN_POINT ( 'NONE',  ( -13.89961937509957401, -13.97604488694547875, 24.37609039468565442 ) ) ;
#34790=CARTESIAN_POINT ( 'NONE',  ( -16.88567814943164080, -6.947325034625593254, 46.29001122652586275 ) ) ;
#34791=CARTESIAN_POINT ( 'NONE',  ( 9.474510206698971260, -16.51473224551069308, 22.91557627198102765 ) ) ;
#34792=CARTESIAN_POINT ( 'NONE',  ( 14.29746914071037800, 8.314922557961029526, 111.6677570613523613 ) ) ;
#34794=CARTESIAN_POINT ( 'NONE',  ( -8.224510206698735004, -14.34966873604973081, 104.5844237280190185 ) ) ;
#34795=CARTESIAN_POINT ( 'NONE',  ( -15.49999999999999822, -5.500000000000000888, 22.00000000000000711 ) ) ;
#34796=CARTESIAN_POINT ( 'NONE',  ( 0.05219959533934541429, -16.53943276465976808, 75.00109039468568994 ) ) ;
#34797=CARTESIAN_POINT ( 'NONE',  ( -13.89961937509977652, 13.97604488694528158, 40.62390960531435979 ) ) ;
#34798=CARTESIAN_POINT ( 'NONE',  ( -18.62759615963255300, -10.81492255796106328, 99.16775706135234714 ) ) ;
#34799=CARTESIAN_POINT ( 'NONE',  ( 0.05219959533936267826, -19.03943276465977164, 100.0010903946856757 ) ) ;
#34800=CARTESIAN_POINT ( 'NONE',  ( -18.62759615963255300, -10.81492255796106328, 69.16775706135234714 ) ) ;
#34801=CARTESIAN_POINT ( 'NONE',  ( -5.153800228976607833, 19.02544592524334988, 47.70942372801900433 ) ) ;
#34802=CARTESIAN_POINT ( 'NONE',  ( -0.05219959533909027116, -19.03943276465977164, 82.49890960531436690 ) ) ;
#34803=CARTESIAN_POINT ( 'NONE',  ( -13.89961937509977652, 13.97604488694528158, 65.62390960531436690 ) ) ;
#34804=DIRECTION ( 'NONE',  ( -0.000000000000000000, -0.000000000000000000, 1.000000000000000000 ) ) ;
#34805=CARTESIAN_POINT ( 'NONE',  ( -5.823673210054116645, -21.52544592524344225, 52.29057627198102409 ) ) ;
#34806=CARTESIAN_POINT ( 'NONE',  ( -19.03943276465977164, 0.05219959533909376836, 41.24890960531435269 ) ) ;
#34807=CARTESIAN_POINT ( 'NONE',  ( -21.52544592524343514, 5.823673210054127303, 81.04057627198102409 ) ) ;
#34808=CARTESIAN_POINT ( 'NONE',  ( -0.05219959533934338120, 16.53943276465976808, 82.50109039468568994 ) ) ;
#34810=CARTESIAN_POINT ( 'NONE',  ( 0.05219959533910956823, 16.53943276465976808, 74.99890960531435269 ) ) ;
#34812=CARTESIAN_POINT ( 'NONE',  ( 8.224510206698742110, 14.34966873604972548, 37.08442372801901143 ) ) ;
#34813=CARTESIAN_POINT ( 'NONE',  ( 19.03943276465977164, -0.05219959533909143690, 23.74890960531435269 ) ) ;
#34814=CARTESIAN_POINT ( 'NONE',  ( -5.153800228976607833, 19.02544592524334988, 67.70942372801900433 ) ) ;
#34815=CARTESIAN_POINT ( 'NONE',  ( -8.224510206698948167, 14.34966873604960824, 75.41557627198102409 ) ) ;
#34816=CARTESIAN_POINT ( 'NONE',  ( -0.05219959533937732626, 21.53943276465977519, 47.50109039468568994 ) ) ;
#34817=CARTESIAN_POINT ( 'NONE',  ( -9.564922557960796823, -16.46253265017161027, 22.08224293864768839 ) ) ;
#34818=CARTESIAN_POINT ( 'NONE',  ( -21.55341960407610458, -5.719274019375992779, 86.45724293864770971 ) ) ;
#34820=CARTESIAN_POINT ( 'NONE',  ( 16.55341960407611168, 4.379528057220329451, 93.95724293864770971 ) ) ;
#34822=CARTESIAN_POINT ( 'NONE',  ( -16.51473224551069308, -9.474510206698971260, 41.66557627198103120 ) ) ;
#34824=CARTESIAN_POINT ( 'NONE',  ( -5.153800228976607833, 19.02544592524334988, 77.70942372801900433 ) ) ;
#34825=CARTESIAN_POINT ( 'NONE',  ( -0.05219959533937732626, 21.53943276465977519, 22.50109039468567573 ) ) ;
#34826=CARTESIAN_POINT ( 'NONE',  ( -9.474510206698964154, 16.51473224551069663, 75.41557627198103830 ) ) ;
#34827=CARTESIAN_POINT ( 'NONE',  ( 5.153800228976615827, -19.02544592524334988, 60.20942372801899012 ) ) ;
#34828=CARTESIAN_POINT ( 'NONE',  ( -19.03943276465977164, 0.05219959533909376836, 41.24890960531435269 ) ) ;
#34829=CARTESIAN_POINT ( 'NONE',  ( -16.55341960407611168, -4.379528057220339221, 56.45724293864768839 ) ) ;
#34830=CARTESIAN_POINT ( 'NONE',  ( -12.14591786802309592, -12.06949235617757132, 56.87390960531436690 ) ) ;
#34831=CARTESIAN_POINT ( 'NONE',  ( -5.049401038298153566, 19.05341960407611168, 80.20724293864769550 ) ) ;
#34832=CARTESIAN_POINT ( 'NONE',  ( 0.05219959533907565091, 21.53943276465977519, 104.9989096053143669 ) ) ;
#34833=CARTESIAN_POINT ( 'NONE',  ( 5.049401038298161559, -19.05341960407611168, 72.70724293864768129 ) ) ;
#34834=CARTESIAN_POINT ( 'NONE',  ( 5.823673210054125526, 21.52544592524343514, 74.79057627198105251 ) ) ;
#34835=CARTESIAN_POINT ( 'NONE',  ( 16.51473224551083163, -9.474510206698727899, 20.83442372801899722 ) ) ;
#34836=CARTESIAN_POINT ( 'NONE',  ( 9.474510206698971260, -16.51473224551069308, 37.91557627198102409 ) ) ;
#34837=CARTESIAN_POINT ( 'NONE',  ( 12.06949235617757843, -12.14591786802309237, 23.12390960531436335 ) ) ;
#34838=CARTESIAN_POINT ( 'NONE',  ( -12.06949235617756955, 12.14591786802309770, 95.62390960531436690 ) ) ;
#34839=CARTESIAN_POINT ( 'NONE',  ( 9.474510206698729675, 16.51473224551082808, 107.0844237280190043 ) ) ;
#34841=CARTESIAN_POINT ( 'NONE',  ( 15.80617190586769283, -15.72974639402175789, 30.62609039468567929 ) ) ;
#34842=CARTESIAN_POINT ( 'NONE',  ( 13.89961937509957401, 13.97604488694547697, 46.87609039468565442 ) ) ;
#34843=CARTESIAN_POINT ( 'NONE',  ( -4.379528057220328563, 16.55341960407611168, 25.20724293864769550 ) ) ;
#34844=CARTESIAN_POINT ( 'NONE',  ( 18.67979575497178502, 10.72451020669898547, 79.16557627198103830 ) ) ;
#34845=CARTESIAN_POINT ( 'NONE',  ( 13.97604488694527802, 13.89961937509977652, 104.3739096053143385 ) ) ;
#34846=CARTESIAN_POINT ( 'NONE',  ( 8.314922557960818139, 14.29746914071049879, 54.58224293864769550 ) ) ;
#34847=CARTESIAN_POINT ( 'NONE',  ( 16.46253265017160672, -9.564922557960803928, 33.33224293864770260 ) ) ;
#34848=CARTESIAN_POINT ( 'NONE',  ( 9.474510206698971260, -16.51473224551069308, 27.91557627198103120 ) ) ;
#34849=CARTESIAN_POINT ( 'NONE',  ( -10.81492255796105439, 18.62759615963255655, 107.9177570613523471 ) ) ;
#34850=CARTESIAN_POINT ( 'NONE',  ( -12.06949235617739369, -12.14591786802326823, 89.37609039468568994 ) ) ;
#34851=CARTESIAN_POINT ( 'NONE',  ( 5.823673210054444382, -21.52544592524334988, 45.20942372801901854 ) ) ;
#34852=CARTESIAN_POINT ( 'NONE',  ( -16.53943276465976808, -0.05219959533934237506, 43.75109039468568284 ) ) ;
#34853=CARTESIAN_POINT ( 'NONE',  ( 21.53943276465977519, -0.05219959533907433946, 23.74890960531435269 ) ) ;
#34854=CARTESIAN_POINT ( 'NONE',  ( 13.89961937509977652, -13.97604488694527269, 58.12390960531436690 ) ) ;
#34855=CARTESIAN_POINT ( 'NONE',  ( -0.05219959533909027116, -19.03943276465977164, 72.49890960531435269 ) ) ;
#34856=CARTESIAN_POINT ( 'NONE',  ( -16.55341960407617563, 4.379528057220093196, 58.54275706135235424 ) ) ;
#34857=CARTESIAN_POINT ( 'NONE',  ( -4.379528057220328563, 16.55341960407611168, 100.2072429386476955 ) ) ;
#34858=CARTESIAN_POINT ( 'NONE',  ( -8.224510206698948167, 14.34966873604960824, 25.41557627198103120 ) ) ;
#34860=CARTESIAN_POINT ( 'NONE',  ( 18.67979575497194134, -10.72451020669871369, 50.83442372801901143 ) ) ;
#34861=CARTESIAN_POINT ( 'NONE',  ( 5.153800228976335163, 19.02544592524342804, 89.79057627198102409 ) ) ;
#34862=CARTESIAN_POINT ( 'NONE',  ( 13.89961937509977652, -13.97604488694527269, 78.12390960531433848 ) ) ;
#34863=CARTESIAN_POINT ( 'NONE',  ( 16.46253265017160672, -9.564922557960803928, 103.3322429386476955 ) ) ;
#34864=CARTESIAN_POINT ( 'NONE',  ( 4.483927247898545687, 16.52544592524342804, 44.79057627198103120 ) ) ;
#34865=EDGE_CURVE ( 'NONE', #119129, #29984, #24199, .T. ) ;
#34866=CARTESIAN_POINT ( 'NONE',  ( -8.314922557961024197, 14.29746914071037800, 107.9177570613523471 ) ) ;
#34867=CARTESIAN_POINT ( 'NONE',  ( 14.29746914071049879, -8.314922557960816363, 38.33224293864768839 ) ) ;
#34869=CARTESIAN_POINT ( 'NONE',  ( -0.05219959533936034679, 19.03943276465977164, 32.50109039468566863 ) ) ;
#34870=CARTESIAN_POINT ( 'NONE',  ( 0.05219959533909260263, 19.03943276465977164, 74.99890960531435269 ) ) ;
#34871=CARTESIAN_POINT ( 'NONE',  ( -16.46253265017146816, -9.564922557961047289, 49.16775706135233293 ) ) ;
#34873=CARTESIAN_POINT ( 'NONE',  ( -17.49999999999999289, 5.500000000000034639, 55.79690382534172954 ) ) ;
#34874=CARTESIAN_POINT ( 'NONE',  ( 19.02544592524334988, 5.153800228976608722, 81.45942372801897591 ) ) ;
#34875=CARTESIAN_POINT ( 'NONE',  ( -14.34966873604972548, 8.224510206698743886, 73.33442372801901854 ) ) ;
#34876=CARTESIAN_POINT ( 'NONE',  ( 16.21995358207304605, 7.366697692864170754, 92.56448998487842061 ) ) ;
#34877=CARTESIAN_POINT ( 'NONE',  ( -13.89961937509977652, 13.97604488694528158, 100.6239096053143669 ) ) ;
#34878=CARTESIAN_POINT ( 'NONE',  ( -21.52544592524334988, -5.823673210054445271, 28.95942372801902209 ) ) ;
#34879=CARTESIAN_POINT ( 'NONE',  ( 19.02544592524334988, 5.153800228976608722, 96.45942372801897591 ) ) ;
#34880=CARTESIAN_POINT ( 'NONE',  ( 19.03943276465977164, -0.05219959533909143690, 113.7489096053143669 ) ) ;
#34881=CARTESIAN_POINT ( 'NONE',  ( 9.564922557960805705, 16.46253265017160317, 44.58224293864769550 ) ) ;
#34882=CARTESIAN_POINT ( 'NONE',  ( 13.89961937509977652, -13.97604488694527269, 88.12390960531438111 ) ) ;
#34883=CARTESIAN_POINT ( 'NONE',  ( -14.34966873604960291, -8.224510206698953496, 66.66557627198102409 ) ) ;
#34884=CARTESIAN_POINT ( 'NONE',  ( -16.51473224551069308, -9.474510206698971260, 51.66557627198102409 ) ) ;
#34885=CARTESIAN_POINT ( 'NONE',  ( -0.05219959533909027116, -19.03943276465977164, 67.49890960531436690 ) ) ;
#34886=CARTESIAN_POINT ( 'NONE',  ( 9.564922557961047289, -16.46253265017146816, 70.41775706135233293 ) ) ;
#34887=CARTESIAN_POINT ( 'NONE',  ( -19.03943276465977164, -0.05219959533935918106, 23.75109039468566152 ) ) ;
#34888=CARTESIAN_POINT ( 'NONE',  ( 5.153800228976335163, 19.02544592524342804, 64.79057627198100988 ) ) ;
#34889=CARTESIAN_POINT ( 'NONE',  ( 18.67979575497178502, 10.72451020669898547, 69.16557627198102409 ) ) ;
#34890=CARTESIAN_POINT ( 'NONE',  ( 4.379528057220339221, -16.55341960407611168, 72.70724293864769550 ) ) ;
#34891=CARTESIAN_POINT ( 'NONE',  ( -16.51473224551082808, 9.474510206698731452, 33.33442372801899722 ) ) ;
#34892=CARTESIAN_POINT ( 'NONE',  ( 9.564922557960805705, 16.46253265017160317, 114.5822429386476955 ) ) ;
#34893=CARTESIAN_POINT ( 'NONE',  ( -18.67979575497178146, -10.72451020669898902, 21.66557627198102409 ) ) ;
#34894=CARTESIAN_POINT ( 'NONE',  ( 19.03943276465977164, -0.05219959533909143690, 58.74890960531435979 ) ) ;
#34895=CARTESIAN_POINT ( 'NONE',  ( 19.03943276465977164, -0.05219959533909143690, 33.74890960531435979 ) ) ;
#34896=CARTESIAN_POINT ( 'NONE',  ( -4.483927247898539470, -16.52544592524342804, 107.2905762719810525 ) ) ;
#34897=CIRCLE ( 'NONE', #96227, 2.000000000000000000 ) ;
#34898=CARTESIAN_POINT ( 'NONE',  ( -10.72451020669898014, 18.67979575497178502, 110.4155762719810383 ) ) ;
#34900=CARTESIAN_POINT ( 'NONE',  ( 5.719274019375673035, 21.55341960407619339, 32.29275706135235424 ) ) ;
#34901=CARTESIAN_POINT ( 'NONE',  ( -16.53943276465976808, 0.05219959533911058130, 111.2489096053143669 ) ) ;
#34902=CARTESIAN_POINT ( 'NONE',  ( -21.53943276465977519, -0.05219959533937600094, 78.75109039468568994 ) ) ;
#34903=CARTESIAN_POINT ( 'NONE',  ( -5.823673210054116645, -21.52544592524344225, 87.29057627198103830 ) ) ;
#34904=CARTESIAN_POINT ( 'NONE',  ( 19.05341960407617918, -5.049401038297876454, 41.04275706135233293 ) ) ;
#34905=CARTESIAN_POINT ( 'NONE',  ( 18.10062525802553424, -5.500000000000021316, 76.01383468041922242 ) ) ;
#34906=CARTESIAN_POINT ( 'NONE',  ( -13.97604488694527625, -13.89961937509977830, 51.87390960531437401 ) ) ;
#34907=CARTESIAN_POINT ( 'NONE',  ( -16.55341960407617563, 4.379528057220093196, 43.54275706135235424 ) ) ;
#34908=CARTESIAN_POINT ( 'NONE',  ( 14.29746914071049879, -8.314922557960816363, 103.3322429386476955 ) ) ;
#34910=CARTESIAN_POINT ( 'NONE',  ( 19.03943276465977164, -0.05219959533909143690, 73.74890960531435269 ) ) ;
#34911=CARTESIAN_POINT ( 'NONE',  ( 14.29746914071049879, -8.314922557960816363, 88.33224293864769550 ) ) ;
#34912=CARTESIAN_POINT ( 'NONE',  ( 10.81492255796078972, 18.62759615963270932, 49.58224293864769550 ) ) ;
#34913=CARTESIAN_POINT ( 'NONE',  ( -14.29746914071049879, 8.314922557960819915, 60.83224293864769550 ) ) ;
#34914=CARTESIAN_POINT ( 'NONE',  ( -8.314922557961024197, 14.29746914071037800, 32.91775706135234714 ) ) ;
#34915=CARTESIAN_POINT ( 'NONE',  ( -10.72451020669870658, -18.67979575497194134, 84.58442372801903275 ) ) ;
#34916=CARTESIAN_POINT ( 'NONE',  ( -17.59860650958993844, 7.585241751806885979, 63.42337014262494677 ) ) ;
#34917=CARTESIAN_POINT ( 'NONE',  ( -14.29746914071037622, -8.314922557961029526, 94.16775706135237556 ) ) ;
#34918=CARTESIAN_POINT ( 'NONE',  ( -12.06949235617756955, 12.14591786802309770, 40.62390960531435269 ) ) ;
#34919=CARTESIAN_POINT ( 'NONE',  ( 0.05219959533909260263, 19.03943276465977164, 39.99890960531436690 ) ) ;
#34920=CARTESIAN_POINT ( 'NONE',  ( 18.67979575497194134, -10.72451020669871369, 100.8344237280190185 ) ) ;
#34921=CARTESIAN_POINT ( 'NONE',  ( -15.72974639402197994, 15.80617190586746368, 105.6239096053143669 ) ) ;
#34923=CARTESIAN_POINT ( 'NONE',  ( 10.81492255796106328, -18.62759615963255655, 60.41775706135235424 ) ) ;
#34924=CARTESIAN_POINT ( 'NONE',  ( 4.379528057220092307, 16.55341960407617563, 42.29275706135235424 ) ) ;
#34925=CARTESIAN_POINT ( 'NONE',  ( -16.55341960407611168, -4.379528057220339221, 66.45724293864768129 ) ) ;
#34926=CARTESIAN_POINT ( 'NONE',  ( -15.80617190586768217, 15.72974639402176855, 83.12609039468568994 ) ) ;
#34929=CARTESIAN_POINT ( 'NONE',  ( 14.29746914071037800, 8.314922557961029526, 106.6677570613523756 ) ) ;
#34930=CARTESIAN_POINT ( 'NONE',  ( 16.18388926212239909, 7.379444403734401803, 27.93953151366153165 ) ) ;
#34932=CARTESIAN_POINT ( 'NONE',  ( 12.14591786802309770, 12.06949235617756955, 29.37390960531435269 ) ) ;
#34933=CARTESIAN_POINT ( 'NONE',  ( 8.224510206698742110, 14.34966873604972548, 77.08442372801901854 ) ) ;
#34934=CARTESIAN_POINT ( 'NONE',  ( 19.03943276465977164, -0.05219959533909143690, 88.74890960531436690 ) ) ;
#34936=CARTESIAN_POINT ( 'NONE',  ( 9.474510206698971260, -16.51473224551069308, 102.9155762719810241 ) ) ;
#34937=CARTESIAN_POINT ( 'NONE',  ( 10.81492255796106328, -18.62759615963255655, 90.41775706135236135 ) ) ;
#34938=CARTESIAN_POINT ( 'NONE',  ( -16.53943276465976808, -0.05219959533934237506, 93.75109039468567573 ) ) ;
#34939=CARTESIAN_POINT ( 'NONE',  ( -8.224510206698948167, 14.34966873604960824, 60.41557627198102409 ) ) ;
#34940=CARTESIAN_POINT ( 'NONE',  ( -5.049401038298153566, 19.05341960407611168, 70.20724293864769550 ) ) ;
#34942=CARTESIAN_POINT ( 'NONE',  ( -12.14591786802326823, 12.06949235617739902, 23.12609039468567573 ) ) ;
#34943=CARTESIAN_POINT ( 'NONE',  ( -5.153800228976328057, -19.02544592524343514, 32.29057627198102409 ) ) ;
#34944=CARTESIAN_POINT ( 'NONE',  ( -13.97604488694527625, -13.89961937509977652, 91.87390960531432427 ) ) ;
#34945=CARTESIAN_POINT ( 'NONE',  ( -8.314922557961024197, 14.29746914071037800, 22.91775706135235069 ) ) ;
#34947=CARTESIAN_POINT ( 'NONE',  ( -0.05219959533936034679, 19.03943276465977164, 27.50109039468566507 ) ) ;
#34948=CARTESIAN_POINT ( 'NONE',  ( 14.29746914071037800, 8.314922557961029526, 96.66775706135234714 ) ) ;
#34949=CARTESIAN_POINT ( 'NONE',  ( 0.05219959533936267826, -19.03943276465977164, 100.0010903946856757 ) ) ;
#34950=CARTESIAN_POINT ( 'NONE',  ( -16.46253265017160317, 9.564922557960807481, 25.83224293864769194 ) ) ;
#34951=CARTESIAN_POINT ( 'NONE',  ( -8.224510206698735004, -14.34966873604973081, 64.58442372801900433 ) ) ;
#34952=CARTESIAN_POINT ( 'NONE',  ( 12.14591786802327356, -12.06949235617739191, 50.62609039468568994 ) ) ;
#34954=CARTESIAN_POINT ( 'NONE',  ( 5.049401038297881783, 19.05341960407617563, 67.29275706135234714 ) ) ;
#34955=CARTESIAN_POINT ( 'NONE',  ( -0.05219959533937732626, 21.53943276465977519, 112.5010903946857042 ) ) ;
#34956=CARTESIAN_POINT ( 'NONE',  ( 5.153800228976335163, 19.02544592524342804, 44.79057627198103830 ) ) ;
#34957=CARTESIAN_POINT ( 'NONE',  ( 13.97604488694527802, 13.89961937509977652, 79.37390960531435269 ) ) ;
#34958=CARTESIAN_POINT ( 'NONE',  ( -16.55341960407611168, -4.379528057220339221, 66.45724293864768129 ) ) ;
#34959=EDGE_CURVE ( 'NONE', #47253, #68796, #30535, .T. ) ;
#34960=CARTESIAN_POINT ( 'NONE',  ( -16.46253265017146816, -9.564922557961047289, 44.16775706135232582 ) ) ;
#34961=CARTESIAN_POINT ( 'NONE',  ( -21.52544592524343514, 5.823673210054127303, 56.04057627198102409 ) ) ;
#34962=CARTESIAN_POINT ( 'NONE',  ( 5.823673210054444382, -21.52544592524334988, 110.2094237280190185 ) ) ;
#34963=CARTESIAN_POINT ( 'NONE',  ( 5.049401038298161559, -19.05341960407611168, 92.70724293864769550 ) ) ;
#34964=CARTESIAN_POINT ( 'NONE',  ( 15.80617190586769283, -15.72974639402175789, 105.6260903946856899 ) ) ;
#34965=CARTESIAN_POINT ( 'NONE',  ( -0.05219959533907301413, -21.53943276465977519, 67.49890960531436690 ) ) ;
#34966=CARTESIAN_POINT ( 'NONE',  ( 19.03943276465977164, -0.05219959533909143690, 93.74890960531435269 ) ) ;
#34967=CARTESIAN_POINT ( 'NONE',  ( 0.05219959533936267826, -19.03943276465977164, 95.00109039468567573 ) ) ;
#34968=CARTESIAN_POINT ( 'NONE',  ( -16.51473224551069308, -9.474510206698971260, 106.6655762719810383 ) ) ;
#34969=CARTESIAN_POINT ( 'NONE',  ( 8.314922557961029526, -14.29746914071037800, 20.41775706135234714 ) ) ;
#34970=CARTESIAN_POINT ( 'NONE',  ( 9.564922557960805705, 16.46253265017160317, 24.58224293864769194 ) ) ;
#34971=CARTESIAN_POINT ( 'NONE',  ( 0.05219959533909260263, 19.03943276465977164, 89.99890960531436690 ) ) ;
#34972=CARTESIAN_POINT ( 'NONE',  ( 10.72451020669898902, -18.67979575497178502, 62.91557627198102409 ) ) ;
#34973=CARTESIAN_POINT ( 'NONE',  ( -4.379528057220086978, -16.55341960407618274, 44.79275706135234714 ) ) ;
#34974=CARTESIAN_POINT ( 'NONE',  ( 21.53943276465977519, 0.05219959533937863772, 51.25109039468568994 ) ) ;
#34975=CARTESIAN_POINT ( 'NONE',  ( 15.80617190586769283, -15.72974639402175789, 95.62609039468568994 ) ) ;
#34976=CARTESIAN_POINT ( 'NONE',  ( 16.55341960407618274, -4.379528057220086978, 101.0427570613523756 ) ) ;
#34977=CARTESIAN_POINT ( 'NONE',  ( 19.05341960407611168, 5.049401038298154454, 93.95724293864769550 ) ) ;
#34978=CARTESIAN_POINT ( 'NONE',  ( 0.05219959533910956823, 16.53943276465976808, 94.99890960531436690 ) ) ;
#34979=CARTESIAN_POINT ( 'NONE',  ( -0.05219959533934338120, 16.53943276465976808, 112.5010903946857042 ) ) ;
#34980=CARTESIAN_POINT ( 'NONE',  ( 13.97604488694548053, -13.89961937509957401, 70.62609039468567573 ) ) ;
#34981=CARTESIAN_POINT ( 'NONE',  ( 10.81492255796106328, -18.62759615963255655, 40.41775706135234714 ) ) ;
#34982=CARTESIAN_POINT ( 'NONE',  ( -16.52544592524342804, 4.483927247898546575, 86.04057627198102409 ) ) ;
#34983=CARTESIAN_POINT ( 'NONE',  ( -15.80617190586745835, -15.72974639402198527, 21.87390960531436690 ) ) ;
#34984=CARTESIAN_POINT ( 'NONE',  ( -16.55341960407611168, -4.379528057220339221, 21.45724293864769550 ) ) ;
#34985=CARTESIAN_POINT ( 'NONE',  ( 18.67979575497194134, -10.72451020669871369, 90.83442372801901854 ) ) ;
#34986=CARTESIAN_POINT ( 'NONE',  ( 12.06949235617739724, 12.14591786802326823, 51.87609039468568284 ) ) ;
#34987=CARTESIAN_POINT ( 'NONE',  ( 18.62759615963255655, 10.81492255796105972, 46.66775706135234714 ) ) ;
#34988=CARTESIAN_POINT ( 'NONE',  ( -5.823673210054431948, 21.52544592524334988, 32.70942372801900433 ) ) ;
#34989=CARTESIAN_POINT ( 'NONE',  ( -14.34966873604960291, -8.224510206698953496, 101.6655762719810383 ) ) ;
#34990=CARTESIAN_POINT ( 'NONE',  ( 16.51473224551069308, 9.474510206698969483, 24.16557627198102765 ) ) ;
#34991=CARTESIAN_POINT ( 'NONE',  ( -16.55341960407611168, -4.379528057220339221, 71.45724293864769550 ) ) ;
#34992=CARTESIAN_POINT ( 'NONE',  ( 0.05219959533909260263, 19.03943276465977164, 54.99890960531435979 ) ) ;
#34993=CARTESIAN_POINT ( 'NONE',  ( 12.14591786802327356, -12.06949235617739191, 110.6260903946857042 ) ) ;
#34994=CARTESIAN_POINT ( 'NONE',  ( -19.03943276465977164, 0.05219959533909376836, 36.24890960531436690 ) ) ;
#34995=CARTESIAN_POINT ( 'NONE',  ( 15.72974639402199770, -15.80617190586745480, 38.12390960531436690 ) ) ;
#34996=CARTESIAN_POINT ( 'NONE',  ( 14.34966873604960469, 8.224510206698951720, 84.16557627198103830 ) ) ;
#34997=CARTESIAN_POINT ( 'NONE',  ( -10.81492255796078084, -18.62759615963271287, 87.08224293864769550 ) ) ;
#34998=CARTESIAN_POINT ( 'NONE',  ( 19.03943276465977164, -0.05219959533909143690, 83.74890960531436690 ) ) ;
#34999=CARTESIAN_POINT ( 'NONE',  ( -5.049401038298153566, 19.05341960407611168, 55.20724293864769550 ) ) ;
#35000=CARTESIAN_POINT ( 'NONE',  ( 5.049401038297881783, 19.05341960407617563, 97.29275706135233293 ) ) ;
#35001=CARTESIAN_POINT ( 'NONE',  ( -0.05219959533907301413, -21.53943276465977519, 42.49890960531435979 ) ) ;
#35002=CARTESIAN_POINT ( 'NONE',  ( 18.67979575497194134, -10.72451020669871369, 70.83442372801901854 ) ) ;
#35003=CARTESIAN_POINT ( 'NONE',  ( 19.02544592524343514, -5.153800228976328945, 53.54057627198102409 ) ) ;
#35004=CARTESIAN_POINT ( 'NONE',  ( 13.97604488694527802, 13.89961937509977652, 89.37390960531436690 ) ) ;
#35006=CARTESIAN_POINT ( 'NONE',  ( 4.483927247898790824, -16.52544592524335698, 70.20942372801904696 ) ) ;
#35007=CARTESIAN_POINT ( 'NONE',  ( 18.67979575497194134, -10.72451020669871369, 45.83442372801901854 ) ) ;
#35008=CARTESIAN_POINT ( 'NONE',  ( 10.72451020669871369, 18.67979575497193778, 77.08442372801901854 ) ) ;
#35009=CARTESIAN_POINT ( 'NONE',  ( -19.03943276465977164, 0.05219959533909376836, 111.2489096053143669 ) ) ;
#35010=CARTESIAN_POINT ( 'NONE',  ( 18.67979575497178502, 10.72451020669898547, 104.1655762719810241 ) ) ;
#35011=CARTESIAN_POINT ( 'NONE',  ( 18.62759615963255655, 10.81492255796105972, 41.66775706135235424 ) ) ;
#35012=CARTESIAN_POINT ( 'NONE',  ( 12.14591786802327356, -12.06949235617739191, 70.62609039468567573 ) ) ;
#35013=CARTESIAN_POINT ( 'NONE',  ( 21.52544592524344225, -5.823673210054117533, 68.54057627198103830 ) ) ;
#35014=CARTESIAN_POINT ( 'NONE',  ( -19.05341960407617563, 5.049401038297882671, 28.54275706135232937 ) ) ;
#35015=CARTESIAN_POINT ( 'NONE',  ( -13.97604488694527625, -13.89961937509977652, 66.87390960531436690 ) ) ;
#35016=CARTESIAN_POINT ( 'NONE',  ( 16.55341960407618274, -4.379528057220086978, 96.04275706135236135 ) ) ;
#35017=CARTESIAN_POINT ( 'NONE',  ( 17.97161686093727795, -5.499999999999969802, 83.49637206859166838 ) ) ;
#35018=CARTESIAN_POINT ( 'NONE',  ( 9.474510206698971260, -16.51473224551069308, 102.9155762719810241 ) ) ;
#35020=CARTESIAN_POINT ( 'NONE',  ( -5.153800228976607833, 19.02544592524334988, 77.70942372801900433 ) ) ;
#35021=CARTESIAN_POINT ( 'NONE',  ( -10.81492255796078084, -18.62759615963271287, 52.08224293864768839 ) ) ;
#35022=CARTESIAN_POINT ( 'NONE',  ( 4.483927247898545687, 16.52544592524342804, 34.79057627198103120 ) ) ;
#35023=CARTESIAN_POINT ( 'NONE',  ( 9.564922557961047289, -16.46253265017146816, 105.4177570613523471 ) ) ;
#35024=CARTESIAN_POINT ( 'NONE',  ( -19.05341960407611168, -5.049401038298163336, 26.45724293864769550 ) ) ;
#35025=CARTESIAN_POINT ( 'NONE',  ( 14.34966873604972726, -8.224510206698740333, 20.83442372801901143 ) ) ;
#35026=CARTESIAN_POINT ( 'NONE',  ( 21.52544592524344225, -5.823673210054117533, 83.54057627198102409 ) ) ;
#35027=CARTESIAN_POINT ( 'NONE',  ( -19.03943276465977164, -0.05219959533935918106, 58.75109039468566863 ) ) ;
#35028=CARTESIAN_POINT ( 'NONE',  ( 4.379528057220092307, 16.55341960407617563, 77.29275706135234714 ) ) ;
#35029=CARTESIAN_POINT ( 'NONE',  ( 9.474510206698971260, -16.51473224551069308, 72.91557627198102409 ) ) ;
#35030=CARTESIAN_POINT ( 'NONE',  ( -16.52544592524342804, 4.483927247898546575, 81.04057627198102409 ) ) ;
#35031=CARTESIAN_POINT ( 'NONE',  ( -13.97604488694527625, -13.89961937509977652, 46.87390960531435979 ) ) ;
#35032=CARTESIAN_POINT ( 'NONE',  ( -12.06949235617756955, 12.14591786802309770, 50.62390960531435979 ) ) ;
#35033=DIRECTION ( 'NONE',  ( 0.000000000000000000, 0.000000000000000000, -1.000000000000000000 ) ) ;
#35035=CARTESIAN_POINT ( 'NONE',  ( 16.52544592524342804, -4.483927247898539470, 28.54057627198103120 ) ) ;
#35036=CARTESIAN_POINT ( 'NONE',  ( 16.46253265017160672, -9.564922557960803928, 83.33224293864768129 ) ) ;
#35038=CARTESIAN_POINT ( 'NONE',  ( 16.51473224551083163, -9.474510206698727899, 40.83442372801900433 ) ) ;
#35039=CARTESIAN_POINT ( 'NONE',  ( -16.52544592524335698, -4.483927247898792601, 43.95942372801902565 ) ) ;
#35040=CARTESIAN_POINT ( 'NONE',  ( 5.719274019375991003, -21.55341960407610458, 47.70724293864770260 ) ) ;
#35041=CARTESIAN_POINT ( 'NONE',  ( -13.89961937509957401, -13.97604488694547875, 29.37609039468565797 ) ) ;
#35042=CARTESIAN_POINT ( 'NONE',  ( -19.03943276465977164, 0.05219959533909376836, 81.24890960531436690 ) ) ;
#35043=CARTESIAN_POINT ( 'NONE',  ( 5.153800228976335163, 19.02544592524342804, 114.7905762719810241 ) ) ;
#35044=CARTESIAN_POINT ( 'NONE',  ( -13.89961937509977652, 13.97604488694528158, 115.6239096053143669 ) ) ;
#35045=CARTESIAN_POINT ( 'NONE',  ( -21.53943276465977519, -0.05219959533937600094, 43.75109039468568284 ) ) ;
#35046=CARTESIAN_POINT ( 'NONE',  ( 8.224510206698953496, -14.34966873604960469, 107.9155762719810241 ) ) ;
#35047=CARTESIAN_POINT ( 'NONE',  ( -15.80617190586745835, -15.72974639402198527, 81.87390960531435269 ) ) ;
#35048=CARTESIAN_POINT ( 'NONE',  ( 5.049401038298161559, -19.05341960407611168, 82.70724293864770971 ) ) ;
#35050=CARTESIAN_POINT ( 'NONE',  ( 21.52544592524334988, 5.823673210054432836, 31.45942372801901854 ) ) ;
#35052=CARTESIAN_POINT ( 'NONE',  ( 9.474510206698971260, -16.51473224551069308, 92.91557627198103830 ) ) ;
#35054=CARTESIAN_POINT ( 'NONE',  ( 13.97604488694527802, 13.89961937509977652, 29.37390960531435979 ) ) ;
#35055=CARTESIAN_POINT ( 'NONE',  ( 13.97604488694527802, 13.89961937509977652, 29.37390960531435979 ) ) ;
#35056=CARTESIAN_POINT ( 'NONE',  ( 16.46253265017146816, 9.564922557961045513, 101.6677570613523329 ) ) ;
#35058=CARTESIAN_POINT ( 'NONE',  ( -16.51473224551069308, -9.474510206698971260, 21.66557627198102765 ) ) ;
#35059=CARTESIAN_POINT ( 'NONE',  ( -10.72451020669870658, -18.67979575497194134, 79.58442372801903275 ) ) ;
#35060=CARTESIAN_POINT ( 'NONE',  ( 19.03943276465977164, -0.05219959533909143690, 63.74890960531435979 ) ) ;
#35061=CARTESIAN_POINT ( 'NONE',  ( -0.05219959533937732626, 21.53943276465977519, 32.50109039468568284 ) ) ;
#35062=CARTESIAN_POINT ( 'NONE',  ( 0.05219959533937995610, -21.53943276465977519, 20.00109039468568639 ) ) ;
#35064=CARTESIAN_POINT ( 'NONE',  ( 5.049401038298161559, -19.05341960407611168, 92.70724293864769550 ) ) ;
#35066=CARTESIAN_POINT ( 'NONE',  ( 8.224510206698742110, 14.34966873604972548, 22.08442372801901143 ) ) ;
#35067=CARTESIAN_POINT ( 'NONE',  ( 5.719274019375991003, -21.55341960407610458, 47.70724293864770260 ) ) ;
#35068=CARTESIAN_POINT ( 'NONE',  ( 21.55341960407619695, -5.719274019375665929, 76.04275706135237556 ) ) ;
#35069=CARTESIAN_POINT ( 'NONE',  ( 9.474510206698971260, -16.51473224551069308, 107.9155762719810383 ) ) ;
#35070=CARTESIAN_POINT ( 'NONE',  ( -19.03943276465977164, -0.05219959533935918106, 98.75109039468567573 ) ) ;
#35071=CARTESIAN_POINT ( 'NONE',  ( 13.89961937509977652, -13.97604488694527269, 58.12390960531436690 ) ) ;
#35072=CARTESIAN_POINT ( 'NONE',  ( -19.03943276465977164, 0.05219959533909376836, 91.24890960531436690 ) ) ;
#35073=CIRCLE ( 'NONE', #15605, 2.500000000000002220 ) ;
#35074=CARTESIAN_POINT ( 'NONE',  ( 12.06949235617757843, -12.14591786802309237, 88.12390960531436690 ) ) ;
#35075=CARTESIAN_POINT ( 'NONE',  ( 14.34966873604960469, 8.224510206698951720, 104.1655762719810241 ) ) ;
#35076=CARTESIAN_POINT ( 'NONE',  ( 16.51473224551069308, 9.474510206698969483, 114.1655762719810241 ) ) ;
#35077=CARTESIAN_POINT ( 'NONE',  ( 4.483927247898790824, -16.52544592524335698, 75.20942372801901854 ) ) ;
#35078=CARTESIAN_POINT ( 'NONE',  ( -4.483927247898539470, -16.52544592524342804, 52.29057627198102409 ) ) ;
#35079=CARTESIAN_POINT ( 'NONE',  ( 0.05219959533909260263, 19.03943276465977164, 39.99890960531436690 ) ) ;
#35080=CARTESIAN_POINT ( 'NONE',  ( 15.80617190586769283, -15.72974639402175789, 65.62609039468568994 ) ) ;
#35081=CARTESIAN_POINT ( 'NONE',  ( -16.46253265017146816, -9.564922557961047289, 89.16775706135234714 ) ) ;
#35082=CARTESIAN_POINT ( 'NONE',  ( -8.314922557960811034, -14.29746914071050412, 67.08224293864770971 ) ) ;
#35083=CARTESIAN_POINT ( 'NONE',  ( -21.53943276465977519, 0.05219959533907696930, 106.2489096053143811 ) ) ;
#35084=CARTESIAN_POINT ( 'NONE',  ( 21.52544592524344225, -5.823673210054117533, 43.54057627198103830 ) ) ;
#35085=CARTESIAN_POINT ( 'NONE',  ( -0.05219959533909027116, -19.03943276465977164, 112.4989096053143669 ) ) ;
#35087=CARTESIAN_POINT ( 'NONE',  ( -9.474510206698964154, 16.51473224551069663, 65.41557627198102409 ) ) ;
#35088=CARTESIAN_POINT ( 'NONE',  ( 8.314922557960818139, 14.29746914071049879, 39.58224293864769550 ) ) ;
#35089=CARTESIAN_POINT ( 'NONE',  ( -14.29746914071037622, -8.314922557961029526, 109.1677570613523613 ) ) ;
#35090=CARTESIAN_POINT ( 'NONE',  ( 0.05219959533934541429, -16.53943276465976808, 85.00109039468568994 ) ) ;
#35091=CARTESIAN_POINT ( 'NONE',  ( -19.05341960407617563, 5.049401038297882671, 33.54275706135231871 ) ) ;
#35093=CARTESIAN_POINT ( 'NONE',  ( 16.88567814943166567, 6.947325034625595030, 48.79001122652586275 ) ) ;
#35094=CARTESIAN_POINT ( 'NONE',  ( 5.153800228976335163, 19.02544592524342804, 94.79057627198103830 ) ) ;
#35095=CARTESIAN_POINT ( 'NONE',  ( 9.564922557960805705, 16.46253265017160317, 54.58224293864769550 ) ) ;
#35096=CARTESIAN_POINT ( 'NONE',  ( 8.314922557960818139, 14.29746914071049879, 59.58224293864770260 ) ) ;
#35097=CARTESIAN_POINT ( 'NONE',  ( 19.05341960407611168, 5.049401038298154454, 23.95724293864769194 ) ) ;
#35098=CARTESIAN_POINT ( 'NONE',  ( -21.53943276465977519, 0.05219959533907696930, 26.24890960531435624 ) ) ;
#35099=CARTESIAN_POINT ( 'NONE',  ( -18.67979575497178146, -10.72451020669898902, 56.66557627198103830 ) ) ;
#35100=CARTESIAN_POINT ( 'NONE',  ( -14.29746914071049879, 8.314922557960819915, 90.83224293864769550 ) ) ;
#35101=CARTESIAN_POINT ( 'NONE',  ( -4.379528057220086978, -16.55341960407618274, 44.79275706135234714 ) ) ;
#35102=EDGE_CURVE ( 'NONE', #6927, #183245, #18360, .T. ) ;
#35103=CARTESIAN_POINT ( 'NONE',  ( -12.14591786802309592, -12.06949235617757132, 81.87390960531435269 ) ) ;
#35105=CARTESIAN_POINT ( 'NONE',  ( 19.02544592524334988, 5.153800228976608722, 76.45942372801897591 ) ) ;
#35106=CARTESIAN_POINT ( 'NONE',  ( -13.89961937509977652, 13.97604488694528158, 115.6239096053143669 ) ) ;
#35108=LINE ( 'NONE', #65440, #141583 ) ;
#35109=CARTESIAN_POINT ( 'NONE',  ( 16.53943276465976808, 0.05219959533934440121, 26.25109039468567573 ) ) ;
#35110=CARTESIAN_POINT ( 'NONE',  ( -12.14591786802309592, -12.06949235617757132, 21.87390960531436690 ) ) ;
#35111=CARTESIAN_POINT ( 'NONE',  ( 16.46253265017146816, 9.564922557961045513, 76.66775706135234714 ) ) ;
#35112=CARTESIAN_POINT ( 'NONE',  ( -21.55341960407610458, -5.719274019375992779, 51.45724293864770260 ) ) ;
#35113=CARTESIAN_POINT ( 'NONE',  ( -21.52544592524334988, -5.823673210054445271, 63.95942372801901854 ) ) ;
#35115=CARTESIAN_POINT ( 'NONE',  ( 4.483927247898790824, -16.52544592524335698, 40.20942372801901854 ) ) ;
#35116=CARTESIAN_POINT ( 'NONE',  ( -16.46253265017160317, 9.564922557960807481, 25.83224293864769194 ) ) ;
#35117=CARTESIAN_POINT ( 'NONE',  ( -13.97604488694527625, -13.89961937509977652, 91.87390960531432427 ) ) ;
#35118=CARTESIAN_POINT ( 'NONE',  ( 9.564922557960805705, 16.46253265017160317, 24.58224293864769194 ) ) ;
#35119=CARTESIAN_POINT ( 'NONE',  ( 16.52544592524342804, -4.483927247898539470, 98.54057627198105251 ) ) ;
#35121=CARTESIAN_POINT ( 'NONE',  ( 9.564922557960805705, 16.46253265017160317, 104.5822429386476955 ) ) ;
#35123=CARTESIAN_POINT ( 'NONE',  ( 16.55341960407618274, -4.379528057220086978, 61.04275706135234714 ) ) ;
#35124=CARTESIAN_POINT ( 'NONE',  ( 5.153800228976615827, -19.02544592524334988, 105.2094237280190185 ) ) ;
#35125=CARTESIAN_POINT ( 'NONE',  ( -15.80617190586745835, -15.72974639402198527, 71.87390960531438111 ) ) ;
#35126=CARTESIAN_POINT ( 'NONE',  ( -9.564922557960796823, -16.46253265017161027, 37.08224293864768839 ) ) ;
#35127=CARTESIAN_POINT ( 'NONE',  ( -16.46253265017146816, -9.564922557961047289, 69.16775706135233293 ) ) ;
#35128=CARTESIAN_POINT ( 'NONE',  ( 10.72451020669898902, -18.67979575497178502, 112.9155762719810383 ) ) ;
#35129=CARTESIAN_POINT ( 'NONE',  ( -19.03943276465977164, 0.05219959533909376836, 71.24890960531435269 ) ) ;
#35130=CARTESIAN_POINT ( 'NONE',  ( -13.97604488694527625, -13.89961937509977652, 101.8739096053143811 ) ) ;
#35132=CARTESIAN_POINT ( 'NONE',  ( -0.05219959533934338120, 16.53943276465976808, 37.50109039468568284 ) ) ;
#35133=CARTESIAN_POINT ( 'NONE',  ( -21.55341960407610458, -5.719274019375992779, 106.4572429386477097 ) ) ;
#35134=CARTESIAN_POINT ( 'NONE',  ( -14.29746914071049879, 8.314922557960819915, 110.8322429386476955 ) ) ;
#35135=CARTESIAN_POINT ( 'NONE',  ( 5.153800228976335163, 19.02544592524342804, 94.79057627198103830 ) ) ;
#35136=CARTESIAN_POINT ( 'NONE',  ( -13.97604488694547697, 13.89961937509957934, 78.12609039468567573 ) ) ;
#35137=CARTESIAN_POINT ( 'NONE',  ( -5.719274019375978568, 21.55341960407610458, 80.20724293864769550 ) ) ;
#35138=CARTESIAN_POINT ( 'NONE',  ( -8.224510206698948167, 14.34966873604960824, 45.41557627198103830 ) ) ;
#35139=CARTESIAN_POINT ( 'NONE',  ( 19.05341960407617918, -5.049401038297876454, 26.04275706135233293 ) ) ;
#35140=CARTESIAN_POINT ( 'NONE',  ( 4.379528057220092307, 16.55341960407617563, 62.29275706135236845 ) ) ;
#35141=CARTESIAN_POINT ( 'NONE',  ( 16.51473224551069308, 9.474510206698969483, 94.16557627198103830 ) ) ;
#35142=CARTESIAN_POINT ( 'NONE',  ( 0.05219959533909260263, 19.03943276465977164, 49.99890960531435979 ) ) ;
#35143=CARTESIAN_POINT ( 'NONE',  ( 10.72451020669871369, 18.67979575497193778, 52.08442372801901854 ) ) ;
#35144=CARTESIAN_POINT ( 'NONE',  ( -15.72974639402176322, -15.80617190586768395, 64.37609039468568994 ) ) ;
#35145=CARTESIAN_POINT ( 'NONE',  ( 16.46253265017160672, -9.564922557960803928, 58.33224293864769550 ) ) ;
#35146=CARTESIAN_POINT ( 'NONE',  ( -21.55341960407619339, 5.719274019375674811, 33.54275706135234714 ) ) ;
#35147=CARTESIAN_POINT ( 'NONE',  ( 16.51473224551083163, -9.474510206698727899, 80.83442372801899012 ) ) ;
#35148=CARTESIAN_POINT ( 'NONE',  ( -13.89961937509977652, 13.97604488694528158, 45.62390960531433848 ) ) ;
#35149=CARTESIAN_POINT ( 'NONE',  ( -4.483927247898782831, 16.52544592524335698, 82.70942372801900433 ) ) ;
#35150=CARTESIAN_POINT ( 'NONE',  ( -9.474510206698964154, 16.51473224551069663, 70.41557627198102409 ) ) ;
#35151=CARTESIAN_POINT ( 'NONE',  ( 0.05219959533909260263, 19.03943276465977164, 114.9989096053143669 ) ) ;
#35152=CARTESIAN_POINT ( 'NONE',  ( -9.474510206698964154, 16.51473224551069663, 35.41557627198102409 ) ) ;
#35153=CARTESIAN_POINT ( 'NONE',  ( -18.67979575497178146, -10.72451020669898902, 86.66557627198102409 ) ) ;
#35154=CARTESIAN_POINT ( 'NONE',  ( -8.224510206698735004, -14.34966873604973081, 69.58442372801900433 ) ) ;
#35156=CARTESIAN_POINT ( 'NONE',  ( -5.153800228976607833, 19.02544592524334988, 27.70942372801899722 ) ) ;
#35158=CARTESIAN_POINT ( 'NONE',  ( -5.049401038298153566, 19.05341960407611168, 60.20724293864768129 ) ) ;
#35159=CARTESIAN_POINT ( 'NONE',  ( -14.29746914071049879, 8.314922557960819915, 50.83224293864770971 ) ) ;
#35160=CARTESIAN_POINT ( 'NONE',  ( 4.483927247898545687, 16.52544592524342804, 79.79057627198102409 ) ) ;
#35162=CARTESIAN_POINT ( 'NONE',  ( -9.564922557960796823, -16.46253265017161027, 107.0822429386476955 ) ) ;
#35163=CARTESIAN_POINT ( 'NONE',  ( -16.46253265017160317, 9.564922557960807481, 90.83224293864769550 ) ) ;
#35164=CARTESIAN_POINT ( 'NONE',  ( -10.81492255796105439, 18.62759615963255655, 52.91775706135235424 ) ) ;
#35165=CARTESIAN_POINT ( 'NONE',  ( -5.153800228976328057, -19.02544592524343514, 112.2905762719810099 ) ) ;
#35166=CARTESIAN_POINT ( 'NONE',  ( -15.72974639402176322, -15.80617190586768395, 99.37609039468568994 ) ) ;
#35167=CARTESIAN_POINT ( 'NONE',  ( 14.34966873604972726, -8.224510206698740333, 85.83442372801901854 ) ) ;
#35168=CARTESIAN_POINT ( 'NONE',  ( 21.53943276465977519, 0.05219959533937863772, 31.25109039468568639 ) ) ;
#35169=CARTESIAN_POINT ( 'NONE',  ( -5.153800228976328057, -19.02544592524343514, 107.2905762719810383 ) ) ;
#35170=CARTESIAN_POINT ( 'NONE',  ( 21.52544592524344225, -5.823673210054117533, 108.5405762719810241 ) ) ;
#35171=CARTESIAN_POINT ( 'NONE',  ( 14.29746914071049879, -8.314922557960816363, 63.33224293864770260 ) ) ;
#35172=CARTESIAN_POINT ( 'NONE',  ( -9.474510206698964154, 16.51473224551069663, 45.41557627198103120 ) ) ;
#35173=CARTESIAN_POINT ( 'NONE',  ( -16.52544592524342804, 4.483927247898546575, 76.04057627198102409 ) ) ;
#35174=CARTESIAN_POINT ( 'NONE',  ( -18.67979575497178146, -10.72451020669898902, 26.66557627198103475 ) ) ;
#35175=CARTESIAN_POINT ( 'NONE',  ( 9.564922557961047289, -16.46253265017146816, 25.41775706135234003 ) ) ;
#35176=CARTESIAN_POINT ( 'NONE',  ( 16.55341960407611168, 4.379528057220329451, 108.9572429386476955 ) ) ;
#35177=ORIENTED_EDGE ( 'NONE', *, *, #91919, .F. ) ;
#35178=CARTESIAN_POINT ( 'NONE',  ( -4.483927247898782831, 16.52544592524335698, 62.70942372801902565 ) ) ;
#35179=CARTESIAN_POINT ( 'NONE',  ( -13.97604488694527625, -13.89961937509977652, 61.87390960531435979 ) ) ;
#35181=CARTESIAN_POINT ( 'NONE',  ( -4.379528057220328563, 16.55341960407611168, 85.20724293864770971 ) ) ;
#35182=CARTESIAN_POINT ( 'NONE',  ( 0.05219959533907565091, 21.53943276465977519, 34.99890960531435979 ) ) ;
#35184=CARTESIAN_POINT ( 'NONE',  ( -12.06949235617739369, -12.14591786802326823, 109.3760903946857042 ) ) ;
#35185=CARTESIAN_POINT ( 'NONE',  ( -13.97604488694547697, 13.89961937509957934, 108.1260903946856331 ) ) ;
#35186=CARTESIAN_POINT ( 'NONE',  ( 18.62759615963255655, 10.81492255796105972, 76.66775706135234714 ) ) ;
#35187=CARTESIAN_POINT ( 'NONE',  ( 9.474510206698971260, -16.51473224551069308, 92.91557627198103830 ) ) ;
#35188=CARTESIAN_POINT ( 'NONE',  ( -10.72451020669898014, 18.67979575497178502, 105.4155762719810383 ) ) ;
#35189=CARTESIAN_POINT ( 'NONE',  ( 14.34966873604972726, -8.224510206698740333, 50.83442372801901143 ) ) ;
#35190=CARTESIAN_POINT ( 'NONE',  ( -13.89961937509977652, 13.97604488694528158, 30.62390960531435269 ) ) ;
#35191=CARTESIAN_POINT ( 'NONE',  ( 12.14591786802327356, -12.06949235617739191, 25.62609039468567929 ) ) ;
#35193=CARTESIAN_POINT ( 'NONE',  ( -9.474510206698720793, -16.51473224551083518, 99.58442372801900433 ) ) ;
#35194=CARTESIAN_POINT ( 'NONE',  ( -10.72451020669898014, 18.67979575497178502, 85.41557627198102409 ) ) ;
#35195=CARTESIAN_POINT ( 'NONE',  ( 5.049401038297881783, 19.05341960407617563, 52.29275706135234003 ) ) ;
#35197=CARTESIAN_POINT ( 'NONE',  ( 5.823673210054125526, 21.52544592524343514, 99.79057627198103830 ) ) ;
#35199=CARTESIAN_POINT ( 'NONE',  ( -19.03943276465977164, 0.05219959533909376836, 76.24890960531435269 ) ) ;
#35201=CARTESIAN_POINT ( 'NONE',  ( -8.224510206698735004, -14.34966873604973081, 34.58442372801900433 ) ) ;
#35203=CARTESIAN_POINT ( 'NONE',  ( -21.55341960407610458, -5.719274019375992779, 111.4572429386476813 ) ) ;
#35204=CARTESIAN_POINT ( 'NONE',  ( 16.52544592524342804, -4.483927247898539470, 68.54057627198103830 ) ) ;
#35205=CARTESIAN_POINT ( 'NONE',  ( 0.05219959533909260263, 19.03943276465977164, 69.99890960531435269 ) ) ;
#35206=CARTESIAN_POINT ( 'NONE',  ( 4.483927247898790824, -16.52544592524335698, 35.20942372801901854 ) ) ;
#35207=CARTESIAN_POINT ( 'NONE',  ( 16.51473224551083163, -9.474510206698727899, 45.83442372801900433 ) ) ;
#35208=CARTESIAN_POINT ( 'NONE',  ( -18.67979575497193778, 10.72451020669871902, 58.33442372801901143 ) ) ;
#35209=CARTESIAN_POINT ( 'NONE',  ( 9.474510206698729675, 16.51473224551082808, 107.0844237280190043 ) ) ;
#35210=CARTESIAN_POINT ( 'NONE',  ( 9.564922557960805705, 16.46253265017160317, 54.58224293864769550 ) ) ;
#35211=CARTESIAN_POINT ( 'NONE',  ( -5.153800228976607833, 19.02544592524334988, 87.70942372801897591 ) ) ;
#35212=CARTESIAN_POINT ( 'NONE',  ( -5.719274019375665041, -21.55341960407619695, 89.79275706135236135 ) ) ;
#35213=CARTESIAN_POINT ( 'NONE',  ( 13.97604488694548053, -13.89961937509957401, 60.62609039468564731 ) ) ;
#35214=CARTESIAN_POINT ( 'NONE',  ( -19.02544592524342804, 5.153800228976336051, 36.04057627198100988 ) ) ;
#35215=CARTESIAN_POINT ( 'NONE',  ( -18.62759615963270932, 10.81492255796079327, 55.83224293864770260 ) ) ;
#35216=CARTESIAN_POINT ( 'NONE',  ( 12.06949235617757843, -12.14591786802309237, 63.12390960531435979 ) ) ;
#35217=CARTESIAN_POINT ( 'NONE',  ( -17.97214573761833378, -5.499999999999956479, 101.4697004903865718 ) ) ;
#35218=CARTESIAN_POINT ( 'NONE',  ( 16.46253265017146816, 9.564922557961045513, 36.66775706135233293 ) ) ;
#35219=CARTESIAN_POINT ( 'NONE',  ( -16.55341960407617563, 4.379528057220093196, 103.5427570613523613 ) ) ;
#35220=CARTESIAN_POINT ( 'NONE',  ( 14.29746914071049879, -8.314922557960816363, 53.33224293864769550 ) ) ;
#35221=CARTESIAN_POINT ( 'NONE',  ( 21.52544592524334988, 5.823673210054432836, 86.45942372801901854 ) ) ;
#35223=CARTESIAN_POINT ( 'NONE',  ( -21.55341960407619339, 5.719274019375674811, 93.54275706135234714 ) ) ;
#35224=CARTESIAN_POINT ( 'NONE',  ( 18.67979575497178502, 10.72451020669898547, 89.16557627198102409 ) ) ;
#35225=CARTESIAN_POINT ( 'NONE',  ( -16.51473224551069308, -9.474510206698971260, 56.66557627198103120 ) ) ;
#35226=CARTESIAN_POINT ( 'NONE',  ( -5.719274019375665041, -21.55341960407619695, 74.79275706135234714 ) ) ;
#35227=CARTESIAN_POINT ( 'NONE',  ( -5.153800228976328057, -19.02544592524343514, 52.29057627198100988 ) ) ;
#35228=CARTESIAN_POINT ( 'NONE',  ( 19.03943276465977164, -0.05219959533909143690, 68.74890960531436690 ) ) ;
#35229=CARTESIAN_POINT ( 'NONE',  ( 16.55341960407611168, 4.379528057220329451, 108.9572429386476955 ) ) ;
#35230=CARTESIAN_POINT ( 'NONE',  ( 13.97604488694527802, 13.89961937509977652, 109.3739096053143669 ) ) ;
#35231=CARTESIAN_POINT ( 'NONE',  ( 16.53943276465976808, -0.05219959533910856209, 48.74890960531435979 ) ) ;
#35232=CARTESIAN_POINT ( 'NONE',  ( -19.03943276465977164, 0.05219959533909376836, 26.24890960531435624 ) ) ;
#35233=CARTESIAN_POINT ( 'NONE',  ( -12.06949235617756955, 12.14591786802309770, 75.62390960531439532 ) ) ;
#35234=CARTESIAN_POINT ( 'NONE',  ( -5.719274019375978568, 21.55341960407610458, 100.2072429386476955 ) ) ;
#35235=CARTESIAN_POINT ( 'NONE',  ( -10.72451020669870658, -18.67979575497194134, 34.58442372801900433 ) ) ;
#35237=CARTESIAN_POINT ( 'NONE',  ( 14.29746914071037800, 8.314922557961029526, 31.66775706135234358 ) ) ;
#35238=CARTESIAN_POINT ( 'NONE',  ( -15.72974639402197994, 15.80617190586746368, 85.62390960531436690 ) ) ;
#35239=CARTESIAN_POINT ( 'NONE',  ( 18.67979575497194134, -10.72451020669871369, 105.8344237280190328 ) ) ;
#35240=CARTESIAN_POINT ( 'NONE',  ( -9.564922557960796823, -16.46253265017161027, 87.08224293864769550 ) ) ;
#35241=CARTESIAN_POINT ( 'NONE',  ( -18.62759615963255300, -10.81492255796106328, 49.16775706135234003 ) ) ;
#35242=CARTESIAN_POINT ( 'NONE',  ( 18.67979575497178502, 10.72451020669898547, 24.16557627198103120 ) ) ;
#35243=CARTESIAN_POINT ( 'NONE',  ( -12.06949235617739369, -12.14591786802326823, 109.3760903946857042 ) ) ;
#35244=CARTESIAN_POINT ( 'NONE',  ( 10.72451020669871369, 18.67979575497193778, 52.08442372801901854 ) ) ;
#35245=CARTESIAN_POINT ( 'NONE',  ( -21.55341960407619339, 5.719274019375674811, 88.54275706135236135 ) ) ;
#35247=CARTESIAN_POINT ( 'NONE',  ( -21.55341960407619339, 5.719274019375674811, 113.5427570613523756 ) ) ;
#35248=CARTESIAN_POINT ( 'NONE',  ( -16.53943276465976808, -0.05219959533934237506, 83.75109039468568994 ) ) ;
#35249=CARTESIAN_POINT ( 'NONE',  ( 0.05219959533937995610, -21.53943276465977519, 45.00109039468568284 ) ) ;
#35250=CARTESIAN_POINT ( 'NONE',  ( -13.89961937509977652, 13.97604488694528158, 35.62390960531435269 ) ) ;
#35251=CARTESIAN_POINT ( 'NONE',  ( -5.823673210054431948, 21.52544592524334988, 97.70942372801904696 ) ) ;
#35252=CARTESIAN_POINT ( 'NONE',  ( 19.02544592524343514, -5.153800228976328945, 108.5405762719810383 ) ) ;
#35253=CARTESIAN_POINT ( 'NONE',  ( 10.72451020669898902, -18.67979575497178502, 97.91557627198103830 ) ) ;
#35255=CARTESIAN_POINT ( 'NONE',  ( -0.05219959533907301413, -21.53943276465977519, 67.49890960531436690 ) ) ;
#35256=CARTESIAN_POINT ( 'NONE',  ( 16.52544592524335698, 4.483927247898782831, 56.45942372801902565 ) ) ;
#35257=CARTESIAN_POINT ( 'NONE',  ( -8.314922557960811034, -14.29746914071050412, 67.08224293864770971 ) ) ;
#35259=CARTESIAN_POINT ( 'NONE',  ( 13.89961937509957401, 13.97604488694547697, 86.87609039468567573 ) ) ;
#35261=CARTESIAN_POINT ( 'NONE',  ( 12.06949235617739724, 12.14591786802326823, 26.87609039468567218 ) ) ;
#35262=CARTESIAN_POINT ( 'NONE',  ( -15.72974639402197994, 15.80617190586746368, 95.62390960531436690 ) ) ;
#35263=CARTESIAN_POINT ( 'NONE',  ( -10.72451020669898014, 18.67979575497178502, 75.41557627198102409 ) ) ;
#35264=CARTESIAN_POINT ( 'NONE',  ( 13.97604488694527802, 13.89961937509977652, 114.3739096053143669 ) ) ;
#35265=CARTESIAN_POINT ( 'NONE',  ( 14.34966873604972726, -8.224510206698740333, 50.83442372801901143 ) ) ;
#35266=CARTESIAN_POINT ( 'NONE',  ( 9.474510206698971260, -16.51473224551069308, 72.91557627198102409 ) ) ;
#35267=CARTESIAN_POINT ( 'NONE',  ( -21.53943276465977519, -0.05219959533937600094, 33.75109039468568284 ) ) ;
#35268=CARTESIAN_POINT ( 'NONE',  ( -19.05341960407617563, 5.049401038297882671, 98.54275706135233293 ) ) ;
#35269=CARTESIAN_POINT ( 'NONE',  ( 9.474510206698971260, -16.51473224551069308, 107.9155762719810383 ) ) ;
#35270=CARTESIAN_POINT ( 'NONE',  ( -13.97604488694527625, -13.89961937509977652, 86.87390960531436690 ) ) ;
#35271=CARTESIAN_POINT ( 'NONE',  ( 21.52544592524344225, -5.823673210054117533, 83.54057627198102409 ) ) ;
#35272=CARTESIAN_POINT ( 'NONE',  ( 9.564922557960805705, 16.46253265017160317, 64.58224293864769550 ) ) ;
#35274=CARTESIAN_POINT ( 'NONE',  ( 16.52544592524342804, -4.483927247898539470, 63.54057627198103830 ) ) ;
#35275=CARTESIAN_POINT ( 'NONE',  ( 0.05219959533907565091, 21.53943276465977519, 24.99890960531435624 ) ) ;
#35276=CARTESIAN_POINT ( 'NONE',  ( -17.72517630440429315, 5.500000000000143885, 60.92175719257210886 ) ) ;
#35277=CARTESIAN_POINT ( 'NONE',  ( -5.823673210054116645, -21.52544592524344225, 107.2905762719810525 ) ) ;
#35278=CARTESIAN_POINT ( 'NONE',  ( 9.564922557961047289, -16.46253265017146816, 60.41775706135233293 ) ) ;
#35279=CARTESIAN_POINT ( 'NONE',  ( 16.46253265017160672, -9.564922557960803928, 108.3322429386476955 ) ) ;
#35280=CARTESIAN_POINT ( 'NONE',  ( 18.56101223717332260, 5.499999999999942268, 68.94978406935678095 ) ) ;
#35281=CARTESIAN_POINT ( 'NONE',  ( -18.62759615963270932, 10.81492255796079327, 60.83224293864769550 ) ) ;
#35282=CARTESIAN_POINT ( 'NONE',  ( -13.89961937509977652, 13.97604488694528158, 85.62390960531433848 ) ) ;
#35283=CARTESIAN_POINT ( 'NONE',  ( -10.72451020669870658, -18.67979575497194134, 84.58442372801903275 ) ) ;
#35284=CARTESIAN_POINT ( 'NONE',  ( -0.05219959533909027116, -19.03943276465977164, 47.49890960531435979 ) ) ;
#35285=CARTESIAN_POINT ( 'NONE',  ( -8.224510206698948167, 14.34966873604960824, 85.41557627198102409 ) ) ;
#35286=CARTESIAN_POINT ( 'NONE',  ( 12.14591786802327356, -12.06949235617739191, 40.62609039468567573 ) ) ;
#35287=CARTESIAN_POINT ( 'NONE',  ( -21.52544592524334988, -5.823673210054445271, 68.95942372801901854 ) ) ;
#35289=CARTESIAN_POINT ( 'NONE',  ( 19.02544592524334988, 5.153800228976608722, 21.45942372801899012 ) ) ;
#35290=CARTESIAN_POINT ( 'NONE',  ( -16.51473224551082808, 9.474510206698731452, 83.33442372801899012 ) ) ;
#35292=CARTESIAN_POINT ( 'NONE',  ( -15.80617190586768217, 15.72974639402176855, 33.12609039468569705 ) ) ;
#35294=CARTESIAN_POINT ( 'NONE',  ( -19.53091890409952214, -5.500000000000037303, 45.06097431831420153 ) ) ;
#35295=CARTESIAN_POINT ( 'NONE',  ( 5.049401038297881783, 19.05341960407617563, 37.29275706135232582 ) ) ;
#35296=CARTESIAN_POINT ( 'NONE',  ( 16.51473224551069308, 9.474510206698969483, 59.16557627198102409 ) ) ;
#35297=CARTESIAN_POINT ( 'NONE',  ( 9.564922557961047289, -16.46253265017146816, 30.41775706135232937 ) ) ;
#35298=CARTESIAN_POINT ( 'NONE',  ( -12.14591786802326823, 12.06949235617739902, 98.12609039468570415 ) ) ;
#35299=CARTESIAN_POINT ( 'NONE',  ( -13.97604488694527625, -13.89961937509977652, 101.8739096053143811 ) ) ;
#35300=CARTESIAN_POINT ( 'NONE',  ( -10.81492255796105439, 18.62759615963255655, 82.91775706135234714 ) ) ;
#35303=CARTESIAN_POINT ( 'NONE',  ( -17.50000000000000711, -5.499999999999956479, 36.28230962303565121 ) ) ;
#35304=CARTESIAN_POINT ( 'NONE',  ( 10.81492255796106328, -18.62759615963255655, 80.41775706135234714 ) ) ;
#35305=CARTESIAN_POINT ( 'NONE',  ( 17.12812012977025233, -6.668231424566045007, 41.14051240676857191 ) ) ;
#35306=CARTESIAN_POINT ( 'NONE',  ( 16.51473224551069308, 9.474510206698969483, 99.16557627198102409 ) ) ;
#35309=CARTESIAN_POINT ( 'NONE',  ( 16.46253265017160672, -9.564922557960803928, 58.33224293864769550 ) ) ;
#35310=CARTESIAN_POINT ( 'NONE',  ( -21.53943276465977519, 0.05219959533907696930, 56.24890960531436690 ) ) ;
#35311=CARTESIAN_POINT ( 'NONE',  ( 14.29746914071049879, -8.314922557960816363, 28.33224293864769550 ) ) ;
#35312=CARTESIAN_POINT ( 'NONE',  ( 8.224510206698953496, -14.34966873604960469, 92.91557627198103830 ) ) ;
#35313=CARTESIAN_POINT ( 'NONE',  ( -19.03943276465977164, 0.05219959533909376836, 76.24890960531435269 ) ) ;
#35314=CARTESIAN_POINT ( 'NONE',  ( 5.719274019375673035, 21.55341960407619339, 112.2927570613523471 ) ) ;
#35315=CARTESIAN_POINT ( 'NONE',  ( 13.89961937509977652, -13.97604488694527269, 33.12390960531434558 ) ) ;
#35316=CARTESIAN_POINT ( 'NONE',  ( -8.314922557960811034, -14.29746914071050412, 97.08224293864770971 ) ) ;
#35317=CARTESIAN_POINT ( 'NONE',  ( 18.67979575497194134, -10.72451020669871369, 60.83442372801901854 ) ) ;
#35318=CARTESIAN_POINT ( 'NONE',  ( -15.80617190586745835, -15.72974639402198527, 81.87390960531435269 ) ) ;
#35319=CARTESIAN_POINT ( 'NONE',  ( 13.97604488694548053, -13.89961937509957401, 60.62609039468564731 ) ) ;
#35321=CARTESIAN_POINT ( 'NONE',  ( 16.51473224551069308, 9.474510206698969483, 109.1655762719810383 ) ) ;
#35322=CARTESIAN_POINT ( 'NONE',  ( 14.29746914071049879, -8.314922557960816363, 83.33224293864769550 ) ) ;
#35323=CARTESIAN_POINT ( 'NONE',  ( -0.05219959533936034679, 19.03943276465977164, 47.50109039468566863 ) ) ;
#35324=CARTESIAN_POINT ( 'NONE',  ( 9.564922557960805705, 16.46253265017160317, 64.58224293864769550 ) ) ;
#35326=CARTESIAN_POINT ( 'NONE',  ( -14.34966873604960291, -8.224510206698953496, 61.66557627198103120 ) ) ;
#35327=CARTESIAN_POINT ( 'NONE',  ( 0.05219959533936267826, -19.03943276465977164, 75.00109039468566152 ) ) ;
#35328=CARTESIAN_POINT ( 'NONE',  ( 17.26058549869090086, 6.457015423128633635, 33.87745837476071387 ) ) ;
#35329=CARTESIAN_POINT ( 'NONE',  ( -0.05219959533907301413, -21.53943276465977519, 42.49890960531435979 ) ) ;
#35331=CARTESIAN_POINT ( 'NONE',  ( -4.379528057220328563, 16.55341960407611168, 100.2072429386476955 ) ) ;
#35333=CARTESIAN_POINT ( 'NONE',  ( 5.153800228976335163, 19.02544592524342804, 54.79057627198103120 ) ) ;
#35334=CARTESIAN_POINT ( 'NONE',  ( 21.53943276465977519, -0.05219959533907433946, 58.74890960531436690 ) ) ;
#35335=CARTESIAN_POINT ( 'NONE',  ( 13.89961937509977652, -13.97604488694527269, 38.12390960531436690 ) ) ;
#35336=CARTESIAN_POINT ( 'NONE',  ( 8.224510206698742110, 14.34966873604972548, 82.08442372801901854 ) ) ;
#35337=CARTESIAN_POINT ( 'NONE',  ( 9.564922557960805705, 16.46253265017160317, 69.58224293864770971 ) ) ;
#35338=CARTESIAN_POINT ( 'NONE',  ( -13.97604488694547697, 13.89961937509957934, 48.12609039468566863 ) ) ;
#35340=CARTESIAN_POINT ( 'NONE',  ( -21.52544592524334988, -5.823673210054445271, 63.95942372801901854 ) ) ;
#35342=CARTESIAN_POINT ( 'NONE',  ( 5.823673210054125526, 21.52544592524343514, 44.79057627198103120 ) ) ;
#35343=CARTESIAN_POINT ( 'NONE',  ( -19.05341960407611168, -5.049401038298163336, 21.45724293864768839 ) ) ;
#35344=CARTESIAN_POINT ( 'NONE',  ( 14.29746914071037800, 8.314922557961029526, 91.66775706135234714 ) ) ;
#35345=CARTESIAN_POINT ( 'NONE',  ( 19.02544592524334988, 5.153800228976608722, 101.4594237280189759 ) ) ;
#35347=CARTESIAN_POINT ( 'NONE',  ( 17.97161686093722466, -5.500000000000139444, 43.49637206859164706 ) ) ;
#35348=CARTESIAN_POINT ( 'NONE',  ( 18.62759615963255655, 10.81492255796105972, 96.66775706135234714 ) ) ;
#35349=ORIENTED_EDGE ( 'NONE', *, *, #59756, .F. ) ;
#35350=CARTESIAN_POINT ( 'NONE',  ( 8.314922557960818139, 14.29746914071049879, 44.58224293864769550 ) ) ;
#35351=CARTESIAN_POINT ( 'NONE',  ( 16.53943276465976808, -0.05219959533910856209, 73.74890960531433848 ) ) ;
#35352=CARTESIAN_POINT ( 'NONE',  ( 15.80617190586746368, 15.72974639402197994, 99.37390960531436690 ) ) ;
#35353=CARTESIAN_POINT ( 'NONE',  ( -5.823673210054116645, -21.52544592524344225, 92.29057627198103830 ) ) ;
#35355=CARTESIAN_POINT ( 'NONE',  ( -21.52544592524343514, 5.823673210054127303, 36.04057627198102409 ) ) ;
#35356=CARTESIAN_POINT ( 'NONE',  ( 16.52544592524335698, 4.483927247898782831, 71.45942372801901854 ) ) ;
#35357=CARTESIAN_POINT ( 'NONE',  ( -16.52544592524342804, 4.483927247898546575, 76.04057627198102409 ) ) ;
#35358=CARTESIAN_POINT ( 'NONE',  ( -5.049401038298153566, 19.05341960407611168, 50.20724293864770260 ) ) ;
#35360=CARTESIAN_POINT ( 'NONE',  ( -16.55341960407617563, 4.379528057220093196, 98.54275706135234714 ) ) ;
#35361=CARTESIAN_POINT ( 'NONE',  ( -5.719274019375665041, -21.55341960407619695, 39.79275706135235424 ) ) ;
#35362=CARTESIAN_POINT ( 'NONE',  ( 19.03943276465977164, -0.05219959533909143690, 78.74890960531436690 ) ) ;
#35363=CARTESIAN_POINT ( 'NONE',  ( 21.55341960407619695, -5.719274019375665929, 56.04275706135235424 ) ) ;
#35364=CARTESIAN_POINT ( 'NONE',  ( -16.51473224551069308, -9.474510206698971260, 106.6655762719810383 ) ) ;
#35367=CARTESIAN_POINT ( 'NONE',  ( 15.80617190586769283, -15.72974639402175789, 55.62609039468568284 ) ) ;
#35368=CARTESIAN_POINT ( 'NONE',  ( -19.05341960407611168, -5.049401038298163336, 31.45724293864769550 ) ) ;
#35369=CARTESIAN_POINT ( 'NONE',  ( 5.049401038298161559, -19.05341960407611168, 22.70724293864769194 ) ) ;
#35370=CARTESIAN_POINT ( 'NONE',  ( 13.97604488694548053, -13.89961937509957401, 70.62609039468567573 ) ) ;
#35371=CARTESIAN_POINT ( 'NONE',  ( -21.53943276465977519, -0.05219959533937600094, 28.75109039468567929 ) ) ;
#35372=CARTESIAN_POINT ( 'NONE',  ( 19.02544592524334988, 5.153800228976608722, 61.45942372801900433 ) ) ;
#35373=CARTESIAN_POINT ( 'NONE',  ( -5.049401038298153566, 19.05341960407611168, 30.20724293864768839 ) ) ;
#35374=CARTESIAN_POINT ( 'NONE',  ( -12.14591786802326823, 12.06949235617739902, 88.12609039468570415 ) ) ;
#35375=CARTESIAN_POINT ( 'NONE',  ( -19.03943276465977164, -0.05219959533935918106, 58.75109039468566863 ) ) ;
#35376=CARTESIAN_POINT ( 'NONE',  ( 4.379528057220092307, 16.55341960407617563, 112.2927570613523471 ) ) ;
#35379=CARTESIAN_POINT ( 'NONE',  ( -19.03943276465977164, 0.05219959533909376836, 81.24890960531436690 ) ) ;
#35380=CARTESIAN_POINT ( 'NONE',  ( -18.62759615963255300, -10.81492255796106328, 89.16775706135236135 ) ) ;
#35381=CARTESIAN_POINT ( 'NONE',  ( -15.72974639402176322, -15.80617190586768395, 104.3760903946856899 ) ) ;
#35383=CARTESIAN_POINT ( 'NONE',  ( 15.80617190586769283, -15.72974639402175789, 80.62609039468567573 ) ) ;
#35384=CARTESIAN_POINT ( 'NONE',  ( -12.14591786802326823, 12.06949235617739902, 38.12609039468567573 ) ) ;
#35385=CARTESIAN_POINT ( 'NONE',  ( -16.46253265017160317, 9.564922557960807481, 80.83224293864769550 ) ) ;
#35386=CARTESIAN_POINT ( 'NONE',  ( -21.55341960407610458, -5.719274019375992779, 26.45724293864768839 ) ) ;
#35388=CARTESIAN_POINT ( 'NONE',  ( 9.474510206698971260, -16.51473224551069308, 82.91557627198103830 ) ) ;
#35389=CARTESIAN_POINT ( 'NONE',  ( -19.52851543214742591, -5.500000000000036415, 40.39357721762583253 ) ) ;
#35390=CARTESIAN_POINT ( 'NONE',  ( 5.049401038297881783, 19.05341960407617563, 77.29275706135231871 ) ) ;
#35391=CARTESIAN_POINT ( 'NONE',  ( -9.474510206698964154, 16.51473224551069663, 105.4155762719810383 ) ) ;
#35392=CARTESIAN_POINT ( 'NONE',  ( -5.719274019375665041, -21.55341960407619695, 99.79275706135234714 ) ) ;
#35393=CARTESIAN_POINT ( 'NONE',  ( 8.224510206698953496, -14.34966873604960469, 102.9155762719810383 ) ) ;
#35394=CARTESIAN_POINT ( 'NONE',  ( 18.67979575497178502, 10.72451020669898547, 49.16557627198102409 ) ) ;
#35395=CARTESIAN_POINT ( 'NONE',  ( 5.719274019375991003, -21.55341960407610458, 32.70724293864770260 ) ) ;
#35396=CARTESIAN_POINT ( 'NONE',  ( 12.14591786802309770, 12.06949235617756955, 99.37390960531436690 ) ) ;
#35398=CARTESIAN_POINT ( 'NONE',  ( 16.46253265017146816, 9.564922557961045513, 61.66775706135234003 ) ) ;
#35399=CARTESIAN_POINT ( 'NONE',  ( -16.55341960407611168, -4.379528057220339221, 26.45724293864768839 ) ) ;
#35400=CARTESIAN_POINT ( 'NONE',  ( 13.97604488694527802, 13.89961937509977652, 99.37390960531436690 ) ) ;
#35401=CARTESIAN_POINT ( 'NONE',  ( 18.67979575497194134, -10.72451020669871369, 80.83442372801901854 ) ) ;
#35402=CARTESIAN_POINT ( 'NONE',  ( 5.823673210054125526, 21.52544592524343514, 54.79057627198104541 ) ) ;
#35403=CARTESIAN_POINT ( 'NONE',  ( -21.52544592524334988, -5.823673210054445271, 43.95942372801902565 ) ) ;
#35404=CARTESIAN_POINT ( 'NONE',  ( -15.80617190586745835, -15.72974639402198527, 101.8739096053143811 ) ) ;
#35405=CARTESIAN_POINT ( 'NONE',  ( 5.823673210054444382, -21.52544592524334988, 40.20942372801901854 ) ) ;
#35406=CARTESIAN_POINT ( 'NONE',  ( -0.05219959533909027116, -19.03943276465977164, 27.49890960531435624 ) ) ;
#35407=CARTESIAN_POINT ( 'NONE',  ( -13.97604488694527625, -13.89961937509977652, 86.87390960531436690 ) ) ;
#35408=CARTESIAN_POINT ( 'NONE',  ( -4.379528057220328563, 16.55341960407611168, 100.2072429386476955 ) ) ;
#35409=CARTESIAN_POINT ( 'NONE',  ( 19.05341960407611168, 5.049401038298154454, 113.9572429386477097 ) ) ;
#35410=CARTESIAN_POINT ( 'NONE',  ( 12.14591786802309770, 12.06949235617756955, 49.37390960531436690 ) ) ;
#35411=CARTESIAN_POINT ( 'NONE',  ( -16.53943276465976808, -0.05219959533934237506, 113.7510903946856757 ) ) ;
#35412=CARTESIAN_POINT ( 'NONE',  ( -9.564922557960796823, -16.46253265017161027, 47.08224293864769550 ) ) ;
#35413=CARTESIAN_POINT ( 'NONE',  ( 12.14591786802309770, 12.06949235617756955, 114.3739096053143527 ) ) ;
#35414=CARTESIAN_POINT ( 'NONE',  ( -21.55341960407610458, -5.719274019375992779, 46.45724293864769550 ) ) ;
#35415=CARTESIAN_POINT ( 'NONE',  ( 16.51473224551083163, -9.474510206698727899, 30.83442372801900433 ) ) ;
#35416=CARTESIAN_POINT ( 'NONE',  ( -17.97214573761834799, -5.500000000000018652, 86.46970049038655759 ) ) ;
#35417=CARTESIAN_POINT ( 'NONE',  ( -4.483927247898539470, -16.52544592524342804, 42.29057627198103120 ) ) ;
#35418=CARTESIAN_POINT ( 'NONE',  ( -5.719274019375665041, -21.55341960407619695, 44.79275706135234714 ) ) ;
#35419=CARTESIAN_POINT ( 'NONE',  ( 19.03943276465977164, -0.05219959533909143690, 113.7489096053143669 ) ) ;
#35420=CARTESIAN_POINT ( 'NONE',  ( 8.224510206698742110, 14.34966873604972548, 57.08442372801901854 ) ) ;
#35421=CARTESIAN_POINT ( 'NONE',  ( -9.474510206698720793, -16.51473224551083518, 64.58442372801900433 ) ) ;
#35422=CARTESIAN_POINT ( 'NONE',  ( -8.224510206698948167, 14.34966873604960824, 25.41557627198103120 ) ) ;
#35423=CARTESIAN_POINT ( 'NONE',  ( -14.29746914071037622, -8.314922557961029526, 109.1677570613523613 ) ) ;
#35424=CARTESIAN_POINT ( 'NONE',  ( 0.05219959533909260263, 19.03943276465977164, 34.99890960531435979 ) ) ;
#35425=CARTESIAN_POINT ( 'NONE',  ( 5.153800228976335163, 19.02544592524342804, 64.79057627198100988 ) ) ;
#35426=CARTESIAN_POINT ( 'NONE',  ( -19.03943276465977164, 0.05219959533909376836, 21.24890960531436335 ) ) ;
#35427=CARTESIAN_POINT ( 'NONE',  ( -15.72974639402176322, -15.80617190586768395, 34.37609039468568284 ) ) ;
#35428=CARTESIAN_POINT ( 'NONE',  ( 16.46253265017160672, -9.564922557960803928, 43.33224293864769550 ) ) ;
#35430=CARTESIAN_POINT ( 'NONE',  ( -9.564922557960796823, -16.46253265017161027, 37.08224293864768839 ) ) ;
#35431=CARTESIAN_POINT ( 'NONE',  ( 13.89961937509977652, -13.97604488694527269, 113.1239096053143527 ) ) ;
#35433=CARTESIAN_POINT ( 'NONE',  ( 21.55341960407619695, -5.719274019375665929, 61.04275706135234714 ) ) ;
#35434=CARTESIAN_POINT ( 'NONE',  ( -8.224510206698948167, 14.34966873604960824, 100.4155762719810241 ) ) ;
#35435=CARTESIAN_POINT ( 'NONE',  ( -19.02544592524342804, 5.153800228976336051, 106.0405762719810241 ) ) ;
#35436=CARTESIAN_POINT ( 'NONE',  ( -16.55341960407617563, 4.379528057220093196, 78.54275706135236135 ) ) ;
#35437=CARTESIAN_POINT ( 'NONE',  ( 18.67979575497194134, -10.72451020669871369, 85.83442372801901854 ) ) ;
#35438=CARTESIAN_POINT ( 'NONE',  ( 12.14591786802327356, -12.06949235617739191, 55.62609039468568284 ) ) ;
#35439=CARTESIAN_POINT ( 'NONE',  ( -5.153800228976328057, -19.02544592524343514, 97.29057627198099567 ) ) ;
#35440=CARTESIAN_POINT ( 'NONE',  ( 14.34966873604972726, -8.224510206698740333, 35.83442372801901143 ) ) ;
#35441=CARTESIAN_POINT ( 'NONE',  ( -16.55341960407617563, 4.379528057220093196, 28.54275706135234358 ) ) ;
#35442=CARTESIAN_POINT ( 'NONE',  ( 8.224510206698742110, 14.34966873604972548, 87.08442372801901854 ) ) ;
#35443=CARTESIAN_POINT ( 'NONE',  ( 16.46253265017146816, 9.564922557961045513, 106.6677570613523471 ) ) ;
#35444=CARTESIAN_POINT ( 'NONE',  ( 18.67979575497178502, 10.72451020669898547, 99.16557627198100988 ) ) ;
#35445=CARTESIAN_POINT ( 'NONE',  ( 14.34966873604960469, 8.224510206698951720, 104.1655762719810241 ) ) ;
#35446=CARTESIAN_POINT ( 'NONE',  ( 19.03943276465977164, 0.05219959533936151252, 106.2510903946856615 ) ) ;
#35447=CARTESIAN_POINT ( 'NONE',  ( 16.52544592524335698, 4.483927247898782831, 71.45942372801901854 ) ) ;
#35449=CARTESIAN_POINT ( 'NONE',  ( 19.03943276465977164, 0.05219959533936151252, 71.25109039468566152 ) ) ;
#35450=EDGE_CURVE ( 'NONE', #194003, #23884, #22997, .T. ) ;
#35451=CARTESIAN_POINT ( 'NONE',  ( 14.34966873604960469, 8.224510206698951720, 44.16557627198103120 ) ) ;
#35452=CARTESIAN_POINT ( 'NONE',  ( -12.14591786802309592, -12.06949235617757132, 26.87390960531435979 ) ) ;
#35453=CARTESIAN_POINT ( 'NONE',  ( 12.06949235617757843, -12.14591786802309237, 88.12390960531436690 ) ) ;
#35454=CARTESIAN_POINT ( 'NONE',  ( -0.05219959533936034679, 19.03943276465977164, 27.50109039468566507 ) ) ;
#35455=CARTESIAN_POINT ( 'NONE',  ( -17.05116617787825106, 6.768360034955818172, 88.65675553259201536 ) ) ;
#35456=CARTESIAN_POINT ( 'NONE',  ( -18.67979575497193778, 10.72451020669871902, 43.33442372801901143 ) ) ;
#35457=CARTESIAN_POINT ( 'NONE',  ( 19.02544592524334988, 5.153800228976608722, 101.4594237280189759 ) ) ;
#35458=CARTESIAN_POINT ( 'NONE',  ( -19.03943276465977164, 0.05219959533909376836, 116.2489096053143669 ) ) ;
#35459=CARTESIAN_POINT ( 'NONE',  ( 9.474510206698971260, -16.51473224551069308, 92.91557627198103830 ) ) ;
#35460=CARTESIAN_POINT ( 'NONE',  ( -9.564922557960796823, -16.46253265017161027, 92.08224293864769550 ) ) ;
#35461=CARTESIAN_POINT ( 'NONE',  ( -18.67979575497178146, -10.72451020669898902, 61.66557627198103120 ) ) ;
#35462=CARTESIAN_POINT ( 'NONE',  ( 12.14591786802309770, 12.06949235617756955, 89.37390960531435269 ) ) ;
#35463=CARTESIAN_POINT ( 'NONE',  ( 19.02544592524343514, -5.153800228976328945, 73.54057627198103830 ) ) ;
#35464=CARTESIAN_POINT ( 'NONE',  ( -12.14591786802309592, -12.06949235617757132, 111.8739096053143669 ) ) ;
#35465=CARTESIAN_POINT ( 'NONE',  ( 5.823673210054444382, -21.52544592524334988, 45.20942372801901854 ) ) ;
#35468=CARTESIAN_POINT ( 'NONE',  ( 18.67979575497194134, -10.72451020669871369, 80.83442372801901854 ) ) ;
#35469=CARTESIAN_POINT ( 'NONE',  ( 19.02544592524343514, -5.153800228976328945, 58.54057627198102409 ) ) ;
#35470=CARTESIAN_POINT ( 'NONE',  ( 4.379528057220092307, 16.55341960407617563, 77.29275706135234714 ) ) ;
#35471=CARTESIAN_POINT ( 'NONE',  ( 5.719274019375673035, 21.55341960407619339, 32.29275706135235424 ) ) ;
#35472=CARTESIAN_POINT ( 'NONE',  ( -0.05219959533937732626, 21.53943276465977519, 22.50109039468567573 ) ) ;
#35473=CARTESIAN_POINT ( 'NONE',  ( -0.05219959533936034679, 19.03943276465977164, 47.50109039468566863 ) ) ;
#35474=CARTESIAN_POINT ( 'NONE',  ( -19.05341960407611168, -5.049401038298163336, 76.45724293864769550 ) ) ;
#35475=CARTESIAN_POINT ( 'NONE',  ( -9.564922557961040184, 16.46253265017147172, 27.91775706135232582 ) ) ;
#35476=CARTESIAN_POINT ( 'NONE',  ( 10.81492255796106328, -18.62759615963255655, 85.41775706135236135 ) ) ;
#35477=CARTESIAN_POINT ( 'NONE',  ( -21.53943276465977519, 0.05219959533907696930, 66.24890960531436690 ) ) ;
#35478=CARTESIAN_POINT ( 'NONE',  ( -12.14591786802309592, -12.06949235617757132, 51.87390960531437401 ) ) ;
#35479=CARTESIAN_POINT ( 'NONE',  ( 10.81492255796106328, -18.62759615963255655, 90.41775706135236135 ) ) ;
#35480=CARTESIAN_POINT ( 'NONE',  ( 5.049401038297881783, 19.05341960407617563, 32.29275706135233293 ) ) ;
#35481=CARTESIAN_POINT ( 'NONE',  ( 12.14591786802309770, 12.06949235617756955, 64.37390960531435269 ) ) ;
#35482=CARTESIAN_POINT ( 'NONE',  ( 9.564922557960805705, 16.46253265017160317, 24.58224293864769194 ) ) ;
#35483=CARTESIAN_POINT ( 'NONE',  ( 5.049401038297881783, 19.05341960407617563, 72.29275706135234714 ) ) ;
#35484=CARTESIAN_POINT ( 'NONE',  ( 16.53943276465976808, -0.05219959533910856209, 33.74890960531436690 ) ) ;
#35485=CARTESIAN_POINT ( 'NONE',  ( -15.72974639402176322, -15.80617190586768395, 84.37609039468570415 ) ) ;
#35486=CARTESIAN_POINT ( 'NONE',  ( 9.474510206698971260, -16.51473224551069308, 72.91557627198102409 ) ) ;
#35487=CARTESIAN_POINT ( 'NONE',  ( 5.049401038297881783, 19.05341960407617563, 47.29275706135231161 ) ) ;
#35488=CARTESIAN_POINT ( 'NONE',  ( 18.67979575497178502, 10.72451020669898547, 54.16557627198103120 ) ) ;
#35489=CARTESIAN_POINT ( 'NONE',  ( -10.72451020669870658, -18.67979575497194134, 49.58442372801901143 ) ) ;
#35490=CARTESIAN_POINT ( 'NONE',  ( 21.52544592524344225, -5.823673210054117533, 103.5405762719810383 ) ) ;
#35491=CARTESIAN_POINT ( 'NONE',  ( -0.05219959533936034679, 19.03943276465977164, 102.5010903946856757 ) ) ;
#35492=CARTESIAN_POINT ( 'NONE',  ( -8.224510206698735004, -14.34966873604973081, 64.58442372801900433 ) ) ;
#35494=CARTESIAN_POINT ( 'NONE',  ( -0.05219959533907301413, -21.53943276465977519, 102.4989096053143811 ) ) ;
#35495=CARTESIAN_POINT ( 'NONE',  ( 16.53943276465976808, -0.05219959533910856209, 103.7489096053143669 ) ) ;
#35497=CARTESIAN_POINT ( 'NONE',  ( 12.14591786802327356, -12.06949235617739191, 35.62609039468568994 ) ) ;
#35498=CARTESIAN_POINT ( 'NONE',  ( 0.05219959533907565091, 21.53943276465977519, 59.99890960531436690 ) ) ;
#35499=CARTESIAN_POINT ( 'NONE',  ( -0.05219959533934338120, 16.53943276465976808, 102.5010903946856899 ) ) ;
#35500=CARTESIAN_POINT ( 'NONE',  ( 19.02544592524343514, -5.153800228976328945, 33.54057627198102409 ) ) ;
#35501=CARTESIAN_POINT ( 'NONE',  ( -12.14591786802326823, 12.06949235617739902, 63.12609039468568994 ) ) ;
#35502=CARTESIAN_POINT ( 'NONE',  ( 5.153800228976615827, -19.02544592524334988, 60.20942372801899012 ) ) ;
#35503=CARTESIAN_POINT ( 'NONE',  ( -5.823673210054431948, 21.52544592524334988, 42.70942372801901854 ) ) ;
#35504=CARTESIAN_POINT ( 'NONE',  ( 21.55341960407610458, 5.719274019375980345, 53.95724293864770260 ) ) ;
#35505=CARTESIAN_POINT ( 'NONE',  ( -8.314922557961024197, 14.29746914071037800, 92.91775706135236135 ) ) ;
#35506=CARTESIAN_POINT ( 'NONE',  ( -18.67979575497193778, 10.72451020669871902, 63.33442372801900433 ) ) ;
#35507=CARTESIAN_POINT ( 'NONE',  ( -15.80617190586745835, -15.72974639402198527, 51.87390960531437401 ) ) ;
#35508=CARTESIAN_POINT ( 'NONE',  ( 18.62759615963271287, -10.81492255796078972, 28.33224293864769550 ) ) ;
#35510=CARTESIAN_POINT ( 'NONE',  ( 4.379528057220092307, 16.55341960407617563, 77.29275706135234714 ) ) ;
#35511=CARTESIAN_POINT ( 'NONE',  ( -18.67979575497178146, -10.72451020669898902, 26.66557627198103475 ) ) ;
#35513=CARTESIAN_POINT ( 'NONE',  ( -13.89961937509977652, 13.97604488694528158, 95.62390960531436690 ) ) ;
#35514=CARTESIAN_POINT ( 'NONE',  ( -16.53943276465976808, -0.05219959533934237506, 113.7510903946856757 ) ) ;
#35516=CARTESIAN_POINT ( 'NONE',  ( 12.14591786802309770, 12.06949235617756955, 104.3739096053143669 ) ) ;
#35517=CARTESIAN_POINT ( 'NONE',  ( -10.81492255796078084, -18.62759615963271287, 67.08224293864770971 ) ) ;
#35518=CARTESIAN_POINT ( 'NONE',  ( -12.14591786802326823, 12.06949235617739902, 88.12609039468570415 ) ) ;
#35519=CARTESIAN_POINT ( 'NONE',  ( -5.823673210054431948, 21.52544592524334988, 52.70942372801902565 ) ) ;
#35520=CARTESIAN_POINT ( 'NONE',  ( -19.02544592524334988, -5.153800228976617603, 103.9594237280190043 ) ) ;
#35521=CARTESIAN_POINT ( 'NONE',  ( -4.483927247898539470, -16.52544592524342804, 102.2905762719810383 ) ) ;
#35522=CARTESIAN_POINT ( 'NONE',  ( 16.51473224551069308, 9.474510206698969483, 49.16557627198102409 ) ) ;
#35523=CARTESIAN_POINT ( 'NONE',  ( 9.474510206698971260, -16.51473224551069308, 27.91557627198103120 ) ) ;
#35525=CARTESIAN_POINT ( 'NONE',  ( -13.97604488694527625, -13.89961937509977652, 86.87390960531436690 ) ) ;
#35526=CARTESIAN_POINT ( 'NONE',  ( 8.314922557961029526, -14.29746914071037800, 70.41775706135236135 ) ) ;
#35527=CARTESIAN_POINT ( 'NONE',  ( -21.55341960407619339, 5.719274019375674811, 108.5427570613523756 ) ) ;
#35528=CARTESIAN_POINT ( 'NONE',  ( -5.823673210054116645, -21.52544592524344225, 57.29057627198103120 ) ) ;
#35529=CARTESIAN_POINT ( 'NONE',  ( 16.53943276465976808, 0.05219959533934440121, 91.25109039468568994 ) ) ;
#35530=CARTESIAN_POINT ( 'NONE',  ( -13.89961937509957401, -13.97604488694547875, 79.37609039468567573 ) ) ;
#35531=CARTESIAN_POINT ( 'NONE',  ( 0.05219959533909260263, 19.03943276465977164, 29.99890960531435979 ) ) ;
#35532=CARTESIAN_POINT ( 'NONE',  ( 13.97604488694527802, 13.89961937509977652, 74.37390960531436690 ) ) ;
#35533=CARTESIAN_POINT ( 'NONE',  ( -13.97604488694527625, -13.89961937509977652, 36.87390960531436690 ) ) ;
#35534=CARTESIAN_POINT ( 'NONE',  ( 19.03943276465977164, 0.05219959533936151252, 66.25109039468567573 ) ) ;
#35535=B_SPLINE_CURVE_WITH_KNOTS ( 'NONE', 3,
 ( #96459, #111644, #15669, #2473, #93482, #94477, #47002, #186528, #142963, #170339, #169334, #184522, #65138, #80300, #173329, #156158, #30842, #158146, #19638, #155169, #1471, #109657, #33813, #48002, #110643, #187523, #126795, #92489, #81280, #95473, #16661, #63149 ),
 .UNSPECIFIED., .F., .F.,
 ( 4, 2, 2, 2, 2, 2, 2, 2, 2, 2, 2, 2, 2, 2, 2, 4 ),
 ( 2.625112965618923374E-17, 0.0003712461730036762612, 0.0007424923460073262847, 0.001113738519010976308, 0.001484984692014626332, 0.002227477038021933101, 0.002598723211025603507, 0.002969969384029273914, 0.003341215557032944320, 0.003712461730036614727, 0.004083707903040284699, 0.004454954076043955540, 0.004826200249047625512, 0.005197446422051296352, 0.005568692595054966325, 0.005939938768058637165 ),
 .UNSPECIFIED. ) ;
#35537=CARTESIAN_POINT ( 'NONE',  ( -5.049401038298153566, 19.05341960407611168, 95.20724293864770971 ) ) ;
#35538=CARTESIAN_POINT ( 'NONE',  ( -8.224510206698948167, 14.34966873604960824, 45.41557627198103830 ) ) ;
#35539=CARTESIAN_POINT ( 'NONE',  ( -18.62759615963270932, 10.81492255796079327, 55.83224293864770260 ) ) ;
#35541=CARTESIAN_POINT ( 'NONE',  ( -13.89961937509957401, -13.97604488694547875, 34.37609039468566863 ) ) ;
#35543=CARTESIAN_POINT ( 'NONE',  ( 5.049401038298161559, -19.05341960407611168, 47.70724293864770260 ) ) ;
#35544=CARTESIAN_POINT ( 'NONE',  ( 19.03943276465977164, -0.05219959533909143690, 73.74890960531435269 ) ) ;
#35545=CARTESIAN_POINT ( 'NONE',  ( 8.314922557961029526, -14.29746914071037800, 35.41775706135234003 ) ) ;
#35546=CARTESIAN_POINT ( 'NONE',  ( -18.56101223717332260, -5.500000000000007994, 101.4497840693567667 ) ) ;
#35548=CARTESIAN_POINT ( 'NONE',  ( -4.379528057220086978, -16.55341960407618274, 69.79275706135234714 ) ) ;
#35549=CARTESIAN_POINT ( 'NONE',  ( 0.05219959533907565091, 21.53943276465977519, 89.99890960531438111 ) ) ;
#35550=CARTESIAN_POINT ( 'NONE',  ( -16.52544592524335698, -4.483927247898792601, 43.95942372801902565 ) ) ;
#35551=CARTESIAN_POINT ( 'NONE',  ( -19.05341960407611168, -5.049401038298163336, 41.45724293864769550 ) ) ;
#35553=CARTESIAN_POINT ( 'NONE',  ( -21.55341960407619339, 5.719274019375674811, 58.54275706135235424 ) ) ;
#35554=CARTESIAN_POINT ( 'NONE',  ( -9.564922557961040184, 16.46253265017147172, 57.91775706135233293 ) ) ;
#35555=CARTESIAN_POINT ( 'NONE',  ( -21.52544592524334988, -5.823673210054445271, 88.95942372801901854 ) ) ;
#35556=CARTESIAN_POINT ( 'NONE',  ( 16.61371651742602040, 7.165104196376160139, 98.64584930007005426 ) ) ;
#35558=CARTESIAN_POINT ( 'NONE',  ( 18.67979575497178502, 10.72451020669898547, 49.16557627198102409 ) ) ;
#35560=CARTESIAN_POINT ( 'NONE',  ( -5.153800228976328057, -19.02544592524343514, 97.29057627198099567 ) ) ;
#35561=CARTESIAN_POINT ( 'NONE',  ( 8.314922557960818139, 14.29746914071049879, 104.5822429386477097 ) ) ;
#35562=CARTESIAN_POINT ( 'NONE',  ( 8.314922557961029526, -14.29746914071037800, 25.41775706135235779 ) ) ;
#35563=CARTESIAN_POINT ( 'NONE',  ( 12.06949235617757843, -12.14591786802309237, 23.12390960531436335 ) ) ;
#35565=CARTESIAN_POINT ( 'NONE',  ( -21.52544592524343514, 5.823673210054127303, 101.0405762719810383 ) ) ;
#35566=CARTESIAN_POINT ( 'NONE',  ( -16.55341960407611168, -4.379528057220339221, 41.45724293864769550 ) ) ;
#35568=CARTESIAN_POINT ( 'NONE',  ( -5.153800228976607833, 19.02544592524334988, 87.70942372801897591 ) ) ;
#35569=CARTESIAN_POINT ( 'NONE',  ( -9.474510206698720793, -16.51473224551083518, 19.58442372801899722 ) ) ;
#35570=CARTESIAN_POINT ( 'NONE',  ( -16.52544592524342804, 4.483927247898546575, 31.04057627198102409 ) ) ;
#35571=CARTESIAN_POINT ( 'NONE',  ( 5.823673210054125526, 21.52544592524343514, 89.79057627198103830 ) ) ;
#35572=CARTESIAN_POINT ( 'NONE',  ( -21.52544592524343514, 5.823673210054127303, 46.04057627198103830 ) ) ;
#35573=CARTESIAN_POINT ( 'NONE',  ( -19.03943276465977164, 0.05219959533909376836, 61.24890960531436690 ) ) ;
#35574=CARTESIAN_POINT ( 'NONE',  ( -4.483927247898539470, -16.52544592524342804, 32.29057627198102409 ) ) ;
#35575=CARTESIAN_POINT ( 'NONE',  ( -16.46253265017160317, 9.564922557960807481, 90.83224293864769550 ) ) ;
#35578=CARTESIAN_POINT ( 'NONE',  ( 19.52217212775660471, -5.499999999999922728, 62.43993709005261650 ) ) ;
#35579=CARTESIAN_POINT ( 'NONE',  ( -9.474510206698720793, -16.51473224551083518, 44.58442372801900433 ) ) ;
#35580=CARTESIAN_POINT ( 'NONE',  ( -21.53943276465977519, 0.05219959533907696930, 81.24890960531436690 ) ) ;
#35581=CARTESIAN_POINT ( 'NONE',  ( 12.06949235617757843, -12.14591786802309237, 98.12390960531436690 ) ) ;
#35582=CARTESIAN_POINT ( 'NONE',  ( 21.52544592524334988, 5.823673210054432836, 41.45942372801901143 ) ) ;
#35584=CARTESIAN_POINT ( 'NONE',  ( -4.379528057220086978, -16.55341960407618274, 104.7927570613523898 ) ) ;
#35585=CARTESIAN_POINT ( 'NONE',  ( 13.89961937509977652, -13.97604488694527269, 33.12390960531434558 ) ) ;
#35586=CARTESIAN_POINT ( 'NONE',  ( -5.153800228976328057, -19.02544592524343514, 92.29057627198099567 ) ) ;
#35587=CARTESIAN_POINT ( 'NONE',  ( 17.58332526062525147, 7.635886036038630920, 91.57665040441534643 ) ) ;
#35588=CARTESIAN_POINT ( 'NONE',  ( -19.02544592524342804, 5.153800228976336051, 31.04057627198102409 ) ) ;
#35589=CARTESIAN_POINT ( 'NONE',  ( -4.483927247898539470, -16.52544592524342804, 47.29057627198103120 ) ) ;
#35590=CARTESIAN_POINT ( 'NONE',  ( -10.81492255796105439, 18.62759615963255655, 77.91775706135231871 ) ) ;
#35591=FACE_OUTER_BOUND ( 'NONE', #126359, .T. ) ;
#35592=CARTESIAN_POINT ( 'NONE',  ( 14.29746914071037800, 8.314922557961029526, 66.66775706135234714 ) ) ;
#35593=CARTESIAN_POINT ( 'NONE',  ( -13.97604488694527625, -13.89961937509977652, 41.87390960531435979 ) ) ;
#35594=CARTESIAN_POINT ( 'NONE',  ( -19.05341960407611168, -5.049401038298163336, 46.45724293864768129 ) ) ;
#35596=CARTESIAN_POINT ( 'NONE',  ( -21.52544592524334988, -5.823673210054445271, 103.9594237280190185 ) ) ;
#35597=CARTESIAN_POINT ( 'NONE',  ( -8.314922557961024197, 14.29746914071037800, 62.91775706135236135 ) ) ;
#35598=CARTESIAN_POINT ( 'NONE',  ( -18.67979575497193778, 10.72451020669871902, 103.3344237280190043 ) ) ;
#35599=CARTESIAN_POINT ( 'NONE',  ( -15.80617190586745835, -15.72974639402198527, 36.87390960531435979 ) ) ;
#35600=CARTESIAN_POINT ( 'NONE',  ( 9.474510206698729675, 16.51473224551082808, 112.0844237280190043 ) ) ;
#35601=CARTESIAN_POINT ( 'NONE',  ( -10.81492255796105439, 18.62759615963255655, 72.91775706135234714 ) ) ;
#35602=CARTESIAN_POINT ( 'NONE',  ( 16.53943276465976808, 0.05219959533934440121, 41.25109039468568284 ) ) ;
#35603=CARTESIAN_POINT ( 'NONE',  ( 21.53943276465977519, -0.05219959533907433946, 98.74890960531438111 ) ) ;
#35604=CARTESIAN_POINT ( 'NONE',  ( -16.51473224551082808, 9.474510206698731452, 98.33442372801900433 ) ) ;
#35605=CARTESIAN_POINT ( 'NONE',  ( 5.049401038298161559, -19.05341960407611168, 67.70724293864769550 ) ) ;
#35606=CARTESIAN_POINT ( 'NONE',  ( -19.03943276465977164, -0.05219959533935918106, 113.7510903946856757 ) ) ;
#35608=CARTESIAN_POINT ( 'NONE',  ( 19.03943276465977164, 0.05219959533936151252, 106.2510903946856615 ) ) ;
#35609=CARTESIAN_POINT ( 'NONE',  ( 12.06949235617757843, -12.14591786802309237, 68.12390960531436690 ) ) ;
#35610=CARTESIAN_POINT ( 'NONE',  ( -16.52544592524335698, -4.483927247898792601, 73.95942372801901854 ) ) ;
#35611=CARTESIAN_POINT ( 'NONE',  ( 21.53943276465977519, 0.05219959533937863772, 21.25109039468567218 ) ) ;
#35612=CARTESIAN_POINT ( 'NONE',  ( 13.89961937509977652, -13.97604488694527269, 48.12390960531435979 ) ) ;
#35613=CARTESIAN_POINT ( 'NONE',  ( 0.05219959533909260263, 19.03943276465977164, 54.99890960531435979 ) ) ;
#35614=CARTESIAN_POINT ( 'NONE',  ( -14.29746914071037622, -8.314922557961029526, 69.16775706135234714 ) ) ;
#35618=CARTESIAN_POINT ( 'NONE',  ( -13.89961937509957401, -13.97604488694547875, 19.37609039468566507 ) ) ;
#35619=CARTESIAN_POINT ( 'NONE',  ( -0.05219959533909027116, -19.03943276465977164, 27.49890960531435624 ) ) ;
#35620=EDGE_LOOP ( 'NONE', ( #175029, #100166 ) ) ;
#35621=CARTESIAN_POINT ( 'NONE',  ( 4.483927247898790824, -16.52544592524335698, 20.20942372801900788 ) ) ;
#35622=CARTESIAN_POINT ( 'NONE',  ( -18.67979575497178146, -10.72451020669898902, 56.66557627198103830 ) ) ;
#35623=CARTESIAN_POINT ( 'NONE',  ( -9.474510206698720793, -16.51473224551083518, 44.58442372801900433 ) ) ;
#35624=CARTESIAN_POINT ( 'NONE',  ( -16.53943276465976808, -0.05219959533934237506, 28.75109039468567929 ) ) ;
#35625=CARTESIAN_POINT ( 'NONE',  ( 19.05341960407611168, 5.049401038298154454, 48.95724293864768129 ) ) ;
#35626=CARTESIAN_POINT ( 'NONE',  ( 5.049401038298161559, -19.05341960407611168, 47.70724293864770260 ) ) ;
#35627=CARTESIAN_POINT ( 'NONE',  ( -21.53943276465977519, 0.05219959533907696930, 91.24890960531436690 ) ) ;
#35628=CARTESIAN_POINT ( 'NONE',  ( 13.89961937509977652, -13.97604488694527269, 113.1239096053143527 ) ) ;
#35629=CARTESIAN_POINT ( 'NONE',  ( 9.564922557960805705, 16.46253265017160317, 44.58224293864769550 ) ) ;
#35631=CARTESIAN_POINT ( 'NONE',  ( 5.049401038297881783, 19.05341960407617563, 92.29275706135234714 ) ) ;
#35632=CARTESIAN_POINT ( 'NONE',  ( 4.379528057220339221, -16.55341960407611168, 62.70724293864769550 ) ) ;
#35633=CARTESIAN_POINT ( 'NONE',  ( -13.97604488694547697, 13.89961937509957934, 28.12609039468565797 ) ) ;
#35634=CARTESIAN_POINT ( 'NONE',  ( 21.53943276465977519, -0.05219959533907433946, 103.7489096053143669 ) ) ;
#35635=CARTESIAN_POINT ( 'NONE',  ( -21.53943276465977519, -0.05219959533937600094, 88.75109039468567573 ) ) ;
#35636=CARTESIAN_POINT ( 'NONE',  ( -13.97604488694527625, -13.89961937509977652, 31.87390960531435979 ) ) ;
#35637=CARTESIAN_POINT ( 'NONE',  ( -10.72451020669870658, -18.67979575497194134, 79.58442372801903275 ) ) ;
#35638=CARTESIAN_POINT ( 'NONE',  ( 16.55341960407611168, 4.379528057220329451, 28.95724293864769905 ) ) ;
#35639=CARTESIAN_POINT ( 'NONE',  ( 5.719274019375673035, 21.55341960407619339, 82.29275706135234714 ) ) ;
#35640=CARTESIAN_POINT ( 'NONE',  ( -19.05341960407611168, -5.049401038298163336, 66.45724293864769550 ) ) ;
#35641=CARTESIAN_POINT ( 'NONE',  ( 18.67979575497194134, -10.72451020669871369, 45.83442372801901854 ) ) ;
#35642=CARTESIAN_POINT ( 'NONE',  ( -0.05219959533909027116, -19.03943276465977164, 87.49890960531436690 ) ) ;
#35643=CARTESIAN_POINT ( 'NONE',  ( -12.06949235617756955, 12.14591786802309770, 95.62390960531436690 ) ) ;
#35644=CARTESIAN_POINT ( 'NONE',  ( -14.29746914071049879, 8.314922557960819915, 55.83224293864770260 ) ) ;
#35645=CARTESIAN_POINT ( 'NONE',  ( -15.72974639402197994, 15.80617190586746368, 65.62390960531436690 ) ) ;
#35646=CARTESIAN_POINT ( 'NONE',  ( 19.05341960407611168, 5.049401038298154454, 73.95724293864768129 ) ) ;
#35647=CARTESIAN_POINT ( 'NONE',  ( 18.62759615963271287, -10.81492255796078972, 88.33224293864769550 ) ) ;
#35648=CARTESIAN_POINT ( 'NONE',  ( -0.05219959533936034679, 19.03943276465977164, 62.50109039468566863 ) ) ;
#35649=CARTESIAN_POINT ( 'NONE',  ( 16.53943276465976808, -0.05219959533910856209, 78.74890960531436690 ) ) ;
#35650=CARTESIAN_POINT ( 'NONE',  ( -0.05219959533907301413, -21.53943276465977519, 47.49890960531435979 ) ) ;
#35651=EDGE_CURVE ( 'NONE', #84227, #56210, #32664, .T. ) ;
#35652=CARTESIAN_POINT ( 'NONE',  ( 16.55341960407618274, -4.379528057220086978, 101.0427570613523756 ) ) ;
#35654=CARTESIAN_POINT ( 'NONE',  ( -13.97604488694547697, 13.89961937509957934, 108.1260903946856331 ) ) ;
#35655=CARTESIAN_POINT ( 'NONE',  ( -16.53943276465976808, 0.05219959533911058130, 71.24890960531435269 ) ) ;
#35656=CARTESIAN_POINT ( 'NONE',  ( -17.50000000000014921, 3.292511757969705855, 35.06520270210535983 ) ) ;
#35657=CARTESIAN_POINT ( 'NONE',  ( -5.049401038298153566, 19.05341960407611168, 60.20724293864768129 ) ) ;
#35658=CARTESIAN_POINT ( 'NONE',  ( 0.05219959533910956823, 16.53943276465976808, 59.99890960531436690 ) ) ;
#35659=CARTESIAN_POINT ( 'NONE',  ( 5.049401038298161559, -19.05341960407611168, 102.7072429386476955 ) ) ;
#35660=CARTESIAN_POINT ( 'NONE',  ( 19.02544592524334988, 5.153800228976608722, 76.45942372801897591 ) ) ;
#35661=CARTESIAN_POINT ( 'NONE',  ( -13.89961937509977652, 13.97604488694528158, 65.62390960531436690 ) ) ;
#35662=CARTESIAN_POINT ( 'NONE',  ( 13.97604488694527802, 13.89961937509977652, 79.37390960531435269 ) ) ;
#35663=CARTESIAN_POINT ( 'NONE',  ( 0.05219959533909260263, 19.03943276465977164, 79.99890960531436690 ) ) ;
#35664=CARTESIAN_POINT ( 'NONE',  ( 18.62759615963271287, -10.81492255796078972, 68.33224293864769550 ) ) ;
#35665=CARTESIAN_POINT ( 'NONE',  ( -8.314922557961024197, 14.29746914071037800, 57.91775706135234714 ) ) ;
#35667=CARTESIAN_POINT ( 'NONE',  ( 5.049401038298161559, -19.05341960407611168, 47.70724293864770260 ) ) ;
#35668=CARTESIAN_POINT ( 'NONE',  ( 15.72974639402199770, -15.80617190586745480, 58.12390960531435979 ) ) ;
#35669=CARTESIAN_POINT ( 'NONE',  ( 5.049401038297881783, 19.05341960407617563, 92.29275706135234714 ) ) ;
#35670=CARTESIAN_POINT ( 'NONE',  ( 14.34966873604960469, 8.224510206698951720, 24.16557627198103120 ) ) ;
#35671=CARTESIAN_POINT ( 'NONE',  ( 10.72451020669871369, 18.67979575497193778, 42.08442372801901854 ) ) ;
#35672=CARTESIAN_POINT ( 'NONE',  ( -16.46253265017146816, -9.564922557961047289, 34.16775706135233293 ) ) ;
#35673=CARTESIAN_POINT ( 'NONE',  ( -4.379528057220086978, -16.55341960407618274, 54.79275706135235424 ) ) ;
#35674=CARTESIAN_POINT ( 'NONE',  ( -4.379528057220086978, -16.55341960407618274, 89.79275706135236135 ) ) ;
#35675=CARTESIAN_POINT ( 'NONE',  ( 19.49149378614656314, -5.499999999999759304, 41.93757513605356735 ) ) ;
#35676=CARTESIAN_POINT ( 'NONE',  ( -8.224510206698735004, -14.34966873604973081, 74.58442372801901854 ) ) ;
#35677=CARTESIAN_POINT ( 'NONE',  ( 15.72974639402199770, -15.80617190586745480, 23.12390960531436335 ) ) ;
#35678=CARTESIAN_POINT ( 'NONE',  ( 14.34966873604972726, -8.224510206698740333, 30.83442372801902209 ) ) ;
#35679=CARTESIAN_POINT ( 'NONE',  ( 13.97604488694527802, 13.89961937509977652, 44.37390960531435269 ) ) ;
#35680=CARTESIAN_POINT ( 'NONE',  ( 19.05341960407611168, 5.049401038298154454, 43.95724293864769550 ) ) ;
#35681=CARTESIAN_POINT ( 'NONE',  ( 9.474510206698971260, -16.51473224551069308, 57.91557627198103120 ) ) ;
#35682=CARTESIAN_POINT ( 'NONE',  ( -15.72974639402176322, -15.80617190586768395, 39.37609039468567573 ) ) ;
#35683=CARTESIAN_POINT ( 'NONE',  ( -8.314922557961024197, 14.29746914071037800, 42.91775706135235424 ) ) ;
#35684=CARTESIAN_POINT ( 'NONE',  ( 8.224510206698742110, 14.34966873604972548, 107.0844237280190043 ) ) ;
#35685=CARTESIAN_POINT ( 'NONE',  ( 16.51473224551069308, 9.474510206698969483, 34.16557627198102409 ) ) ;
#35686=CARTESIAN_POINT ( 'NONE',  ( -10.81492255796105439, 18.62759615963255655, 107.9177570613523471 ) ) ;
#35687=CARTESIAN_POINT ( 'NONE',  ( 16.55341960407618274, -4.379528057220086978, 21.04275706135234714 ) ) ;
#35689=CARTESIAN_POINT ( 'NONE',  ( -19.05341960407617563, 5.049401038297882671, 73.54275706135233293 ) ) ;
#35690=CARTESIAN_POINT ( 'NONE',  ( 8.224510206698953496, -14.34966873604960469, 67.91557627198102409 ) ) ;
#35691=CARTESIAN_POINT ( 'NONE',  ( 0.05219959533909260263, 19.03943276465977164, 44.99890960531435979 ) ) ;
#35692=CARTESIAN_POINT ( 'NONE',  ( 19.03943276465977164, 0.05219959533936151252, 76.25109039468566152 ) ) ;
#35694=CARTESIAN_POINT ( 'NONE',  ( 15.80617190586769283, -15.72974639402175789, 75.62609039468567573 ) ) ;
#35695=CARTESIAN_POINT ( 'NONE',  ( 0.05219959533934541429, -16.53943276465976808, 35.00109039468568284 ) ) ;
#35696=CARTESIAN_POINT ( 'NONE',  ( 16.52216118717208104, 7.221426719304524511, 38.57599021046993926 ) ) ;
#35697=CARTESIAN_POINT ( 'NONE',  ( -0.05219959533907301413, -21.53943276465977519, 32.49890960531435979 ) ) ;
#35698=CARTESIAN_POINT ( 'NONE',  ( -8.314922557961024197, 14.29746914071037800, 32.91775706135234714 ) ) ;
#35699=CARTESIAN_POINT ( 'NONE',  ( 13.89961937509978007, -13.97604488694527269, 28.12390960531435624 ) ) ;
#35700=CARTESIAN_POINT ( 'NONE',  ( -13.89961937509957401, -13.97604488694547875, 24.37609039468565442 ) ) ;
#35701=CARTESIAN_POINT ( 'NONE',  ( 18.10062525802554134, -5.500000000000023093, 66.01383468041920821 ) ) ;
#35702=CARTESIAN_POINT ( 'NONE',  ( 5.049401038298161559, -19.05341960407611168, 32.70724293864768129 ) ) ;
#35704=CARTESIAN_POINT ( 'NONE',  ( 9.564922557960805705, 16.46253265017160317, 64.58224293864769550 ) ) ;
#35705=CARTESIAN_POINT ( 'NONE',  ( -19.26498983726237313, 5.499999999999802824, 100.5531957742200575 ) ) ;
#35706=CARTESIAN_POINT ( 'NONE',  ( -10.81492255796105439, 18.62759615963255655, 112.9177570613523329 ) ) ;
#35707=CARTESIAN_POINT ( 'NONE',  ( -14.29746914071049879, 8.314922557960819915, 25.83224293864769194 ) ) ;
#35708=CARTESIAN_POINT ( 'NONE',  ( -19.03943276465977164, 0.05219959533909376836, 36.24890960531436690 ) ) ;
#35709=CARTESIAN_POINT ( 'NONE',  ( 13.89961937509977652, -13.97604488694527269, 93.12390960531436690 ) ) ;
#35710=CARTESIAN_POINT ( 'NONE',  ( -10.81492255796105439, 18.62759615963255655, 67.91775706135234714 ) ) ;
#35711=CARTESIAN_POINT ( 'NONE',  ( -9.474510206698964154, 16.51473224551069663, 55.41557627198103120 ) ) ;
#35712=CARTESIAN_POINT ( 'NONE',  ( 10.72451020669871369, 18.67979575497193778, 72.08442372801899012 ) ) ;
#35713=CARTESIAN_POINT ( 'NONE',  ( 16.51473224551083163, -9.474510206698727899, 90.83442372801900433 ) ) ;
#35714=CARTESIAN_POINT ( 'NONE',  ( -15.80617190586745835, -15.72974639402198527, 21.87390960531436690 ) ) ;
#35715=CARTESIAN_POINT ( 'NONE',  ( -16.46253265017160317, 9.564922557960807481, 35.83224293864768839 ) ) ;
#35716=CARTESIAN_POINT ( 'NONE',  ( 10.72451020669898902, -18.67979575497178502, 107.9155762719810241 ) ) ;
#35717=CARTESIAN_POINT ( 'NONE',  ( 19.03943276465977164, 0.05219959533936151252, 36.25109039468567573 ) ) ;
#35718=CARTESIAN_POINT ( 'NONE',  ( -14.29746914071049879, 8.314922557960819915, 110.8322429386476955 ) ) ;
#35719=CARTESIAN_POINT ( 'NONE',  ( 9.564922557960805705, 16.46253265017160317, 64.58224293864769550 ) ) ;
#35720=CARTESIAN_POINT ( 'NONE',  ( -13.89961937509957401, -13.97604488694547875, 109.3760903946856331 ) ) ;
#35721=CARTESIAN_POINT ( 'NONE',  ( -16.55341960407611168, -4.379528057220339221, 76.45724293864769550 ) ) ;
#35722=CARTESIAN_POINT ( 'NONE',  ( -21.53943276465977519, 0.05219959533907696930, 21.24890960531436690 ) ) ;
#35723=CARTESIAN_POINT ( 'NONE',  ( -5.049401038297874678, -19.05341960407617918, 84.79275706135233293 ) ) ;
#35724=CARTESIAN_POINT ( 'NONE',  ( -10.72451020669898014, 18.67979575497178502, 95.41557627198102409 ) ) ;
#35725=CARTESIAN_POINT ( 'NONE',  ( 18.62759615963255655, 10.81492255796105972, 41.66775706135235424 ) ) ;
#35726=CARTESIAN_POINT ( 'NONE',  ( 12.06949235617739724, 12.14591786802326823, 56.87609039468568994 ) ) ;
#35727=CARTESIAN_POINT ( 'NONE',  ( 0.05219959533934541429, -16.53943276465976808, 55.00109039468568284 ) ) ;
#35728=CARTESIAN_POINT ( 'NONE',  ( -21.55341960407619339, 5.719274019375674811, 53.54275706135234714 ) ) ;
#35729=CARTESIAN_POINT ( 'NONE',  ( 15.72974639402199770, -15.80617190586745480, 58.12390960531435979 ) ) ;
#35730=CARTESIAN_POINT ( 'NONE',  ( -19.05341960407611168, -5.049401038298163336, 51.45724293864770260 ) ) ;
#35732=CARTESIAN_POINT ( 'NONE',  ( -12.06949235617739369, -12.14591786802326823, 79.37609039468567573 ) ) ;
#35733=CARTESIAN_POINT ( 'NONE',  ( 15.72974639402199770, -15.80617190586745480, 98.12390960531436690 ) ) ;
#35734=CARTESIAN_POINT ( 'NONE',  ( 4.483927247898545687, 16.52544592524342804, 49.79057627198102409 ) ) ;
#35735=CARTESIAN_POINT ( 'NONE',  ( -14.34966873604972548, 8.224510206698743886, 63.33442372801900433 ) ) ;
#35736=CARTESIAN_POINT ( 'NONE',  ( 13.89961937509957401, 13.97604488694547697, 96.87609039468566152 ) ) ;
#35737=CARTESIAN_POINT ( 'NONE',  ( -10.81492255796078084, -18.62759615963271287, 97.08224293864770971 ) ) ;
#35738=CARTESIAN_POINT ( 'NONE',  ( 16.53943276465976808, -0.05219959533910856209, 43.74890960531435979 ) ) ;
#35740=CARTESIAN_POINT ( 'NONE',  ( 18.39443945427638738, -5.500000000000021316, 91.01745347608654413 ) ) ;
#35742=CARTESIAN_POINT ( 'NONE',  ( -5.823673210054116645, -21.52544592524344225, 72.29057627198102409 ) ) ;
#35743=CARTESIAN_POINT ( 'NONE',  ( 14.34966873604960469, 8.224510206698951720, 29.16557627198103120 ) ) ;
#35746=CARTESIAN_POINT ( 'NONE',  ( -5.719274019375978568, 21.55341960407610458, 95.20724293864769550 ) ) ;
#35747=CARTESIAN_POINT ( 'NONE',  ( -21.52544592524334988, -5.823673210054445271, 28.95942372801902209 ) ) ;
#35748=CARTESIAN_POINT ( 'NONE',  ( 4.379528057220339221, -16.55341960407611168, 32.70724293864770260 ) ) ;
#35749=CARTESIAN_POINT ( 'NONE',  ( -8.224510206698735004, -14.34966873604973081, 44.58442372801901854 ) ) ;
#35750=CARTESIAN_POINT ( 'NONE',  ( 0.05219959533909260263, 19.03943276465977164, 49.99890960531435979 ) ) ;
#35751=CARTESIAN_POINT ( 'NONE',  ( -13.97604488694527625, -13.89961937509977652, 76.87390960531433848 ) ) ;
#35752=ORIENTED_EDGE ( 'NONE', *, *, #140308, .T. ) ;
#35753=CARTESIAN_POINT ( 'NONE',  ( 18.67979575497178502, 10.72451020669898547, 39.16557627198102409 ) ) ;
#35755=CARTESIAN_POINT ( 'NONE',  ( 12.14591786802327356, -12.06949235617739191, 20.62609039468568639 ) ) ;
#35756=CARTESIAN_POINT ( 'NONE',  ( 13.89961937509957401, 13.97604488694547697, 51.87609039468566863 ) ) ;
#35757=CARTESIAN_POINT ( 'NONE',  ( -15.72974639402197994, 15.80617190586746368, 95.62390960531436690 ) ) ;
#35758=CARTESIAN_POINT ( 'NONE',  ( -4.483927247898539470, -16.52544592524342804, 37.29057627198102409 ) ) ;
#35759=CARTESIAN_POINT ( 'NONE',  ( 5.153800228976335163, 19.02544592524342804, 79.79057627198102409 ) ) ;
#35760=CARTESIAN_POINT ( 'NONE',  ( 21.52544592524344225, -5.823673210054117533, 48.54057627198103120 ) ) ;
#35761=CARTESIAN_POINT ( 'NONE',  ( -15.72974639402197994, 15.80617190586746368, 85.62390960531436690 ) ) ;
#35762=CARTESIAN_POINT ( 'NONE',  ( 8.314922557961029526, -14.29746914071037800, 25.41775706135235779 ) ) ;
#35763=CARTESIAN_POINT ( 'NONE',  ( -10.81492255796078084, -18.62759615963271287, 27.08224293864769550 ) ) ;
#35764=CARTESIAN_POINT ( 'NONE',  ( -10.72451020669870658, -18.67979575497194134, 79.58442372801903275 ) ) ;
#35765=CARTESIAN_POINT ( 'NONE',  ( -16.46253265017160317, 9.564922557960807481, 70.83224293864770971 ) ) ;
#35766=CARTESIAN_POINT ( 'NONE',  ( -5.049401038298153566, 19.05341960407611168, 30.20724293864768839 ) ) ;
#35767=CARTESIAN_POINT ( 'NONE',  ( -13.89961937509977652, 13.97604488694528158, 80.62390960531436690 ) ) ;
#35768=CARTESIAN_POINT ( 'NONE',  ( -4.483927247898539470, -16.52544592524342804, 87.29057627198103830 ) ) ;
#35770=CARTESIAN_POINT ( 'NONE',  ( -16.51473224551082808, 9.474510206698731452, 98.33442372801900433 ) ) ;
#35772=CARTESIAN_POINT ( 'NONE',  ( -16.46253265017160317, 9.564922557960807481, 75.83224293864769550 ) ) ;
#35773=CARTESIAN_POINT ( 'NONE',  ( 21.53943276465977519, 0.05219959533937863772, 81.25109039468568994 ) ) ;
#35774=CARTESIAN_POINT ( 'NONE',  ( -0.05219959533909027116, -19.03943276465977164, 112.4989096053143669 ) ) ;
#35775=CARTESIAN_POINT ( 'NONE',  ( 4.483927247898790824, -16.52544592524335698, 80.20942372801901854 ) ) ;
#35776=CARTESIAN_POINT ( 'NONE',  ( -16.81555441253551919, -7.025013491695478507, 74.36314554665749199 ) ) ;
#35777=CARTESIAN_POINT ( 'NONE',  ( 13.97604488694548053, -13.89961937509957401, 55.62609039468566863 ) ) ;
#35778=CARTESIAN_POINT ( 'NONE',  ( 21.52544592524334988, 5.823673210054432836, 111.4594237280190328 ) ) ;
#35782=CARTESIAN_POINT ( 'NONE',  ( -4.483927247898539470, -16.52544592524342804, 27.29057627198103120 ) ) ;
#35784=CARTESIAN_POINT ( 'NONE',  ( 0.05219959533934541429, -16.53943276465976808, 100.0010903946857042 ) ) ;
#35785=CARTESIAN_POINT ( 'NONE',  ( -19.35543954521081389, -5.499999999999486633, 84.58901960356449479 ) ) ;
#35786=CARTESIAN_POINT ( 'NONE',  ( 16.55341960407618274, -4.379528057220086978, 86.04275706135236135 ) ) ;
#35787=CARTESIAN_POINT ( 'NONE',  ( -19.05341960407611168, -5.049401038298163336, 21.45724293864768839 ) ) ;
#35788=CARTESIAN_POINT ( 'NONE',  ( -21.55341960407619339, 5.719274019375674811, 98.54275706135234714 ) ) ;
#35789=CARTESIAN_POINT ( 'NONE',  ( 16.46253265017146816, 9.564922557961045513, 101.6677570613523329 ) ) ;
#35790=CARTESIAN_POINT ( 'NONE',  ( -21.55341960407619339, 5.719274019375674811, 68.54275706135234714 ) ) ;
#35791=CARTESIAN_POINT ( 'NONE',  ( 5.049401038297881783, 19.05341960407617563, 42.29275706135234003 ) ) ;
#35792=CARTESIAN_POINT ( 'NONE',  ( 5.153800228976335163, 19.02544592524342804, 84.79057627198099567 ) ) ;
#35793=CARTESIAN_POINT ( 'NONE',  ( -5.049401038298153566, 19.05341960407611168, 70.20724293864769550 ) ) ;
#35794=DIRECTION ( 'NONE',  ( 1.000000000000000000, 0.000000000000000000, 0.000000000000000000 ) ) ;
#35795=CARTESIAN_POINT ( 'NONE',  ( 21.52544592524344225, -5.823673210054117533, 53.54057627198103120 ) ) ;
#35796=CARTESIAN_POINT ( 'NONE',  ( 0.05219959533909260263, 19.03943276465977164, 49.99890960531435979 ) ) ;
#35797=CARTESIAN_POINT ( 'NONE',  ( -12.06949235617739369, -12.14591786802326823, 79.37609039468567573 ) ) ;
#35800=CARTESIAN_POINT ( 'NONE',  ( -4.483927247898539470, -16.52544592524342804, 82.29057627198103830 ) ) ;
#35802=CARTESIAN_POINT ( 'NONE',  ( -4.483927247898782831, 16.52544592524335698, 37.70942372801900433 ) ) ;
#35803=CARTESIAN_POINT ( 'NONE',  ( 16.55341960407611168, 4.379528057220329451, 103.9572429386476813 ) ) ;
#35804=CARTESIAN_POINT ( 'NONE',  ( 19.02544592524334988, 5.153800228976608722, 71.45942372801900433 ) ) ;
#35805=CARTESIAN_POINT ( 'NONE',  ( 8.224510206698953496, -14.34966873604960469, 72.91557627198103830 ) ) ;
#35806=CARTESIAN_POINT ( 'NONE',  ( -18.67979575497193778, 10.72451020669871902, 38.33442372801900433 ) ) ;
#35807=CARTESIAN_POINT ( 'NONE',  ( -19.05341960407611168, -5.049401038298163336, 26.45724293864769550 ) ) ;
#35808=CARTESIAN_POINT ( 'NONE',  ( -21.53943276465977519, 0.05219959533907696930, 91.24890960531436690 ) ) ;
#35809=CARTESIAN_POINT ( 'NONE',  ( -19.05341960407611168, -5.049401038298163336, 106.4572429386476955 ) ) ;
#35810=CARTESIAN_POINT ( 'NONE',  ( -14.34966873604960291, -8.224510206698953496, 71.66557627198100988 ) ) ;
#35812=CARTESIAN_POINT ( 'NONE',  ( 19.03943276465977164, -0.05219959533909143690, 48.74890960531435979 ) ) ;
#35814=CARTESIAN_POINT ( 'NONE',  ( 19.05341960407617918, -5.049401038297876454, 81.04275706135231871 ) ) ;
#35815=CARTESIAN_POINT ( 'NONE',  ( -15.80617190586768217, 15.72974639402176855, 23.12609039468567573 ) ) ;
#35816=CARTESIAN_POINT ( 'NONE',  ( -13.89961937509977652, 13.97604488694528158, 70.62390960531432427 ) ) ;
#35817=CARTESIAN_POINT ( 'NONE',  ( -13.89961937509957401, -13.97604488694547875, 59.37609039468566863 ) ) ;
#35818=CARTESIAN_POINT ( 'NONE',  ( -9.564922557960796823, -16.46253265017161027, 47.08224293864769550 ) ) ;
#35819=ADVANCED_FACE ( 'NONE', ( #181204 ), #53848, .T. ) ;
#35820=CARTESIAN_POINT ( 'NONE',  ( -0.05219959533910754901, -16.53943276465976808, 62.49890960531436690 ) ) ;
#35821=CARTESIAN_POINT ( 'NONE',  ( 8.224510206698953496, -14.34966873604960469, 47.91557627198102409 ) ) ;
#35822=CARTESIAN_POINT ( 'NONE',  ( -13.89961937509977652, 13.97604488694528158, 80.62390960531436690 ) ) ;
#35823=CARTESIAN_POINT ( 'NONE',  ( -10.81492255796078084, -18.62759615963271287, 87.08224293864769550 ) ) ;
#35824=CARTESIAN_POINT ( 'NONE',  ( -9.564922557960796823, -16.46253265017161027, 77.08224293864769550 ) ) ;
#35825=CARTESIAN_POINT ( 'NONE',  ( 15.72974639402199770, -15.80617190586745480, 73.12390960531436690 ) ) ;
#35826=CARTESIAN_POINT ( 'NONE',  ( 21.53943276465977519, 0.05219959533937863772, 111.2510903946856899 ) ) ;
#35827=CARTESIAN_POINT ( 'NONE',  ( -19.03943276465977164, 0.05219959533909376836, 21.24890960531436335 ) ) ;
#35828=CARTESIAN_POINT ( 'NONE',  ( -12.14591786802326823, 12.06949235617739902, 113.1260903946856899 ) ) ;
#35829=CARTESIAN_POINT ( 'NONE',  ( -14.34966873604960291, -8.224510206698953496, 96.66557627198102409 ) ) ;
#35830=CARTESIAN_POINT ( 'NONE',  ( 16.51473224551083163, -9.474510206698727899, 100.8344237280190043 ) ) ;
#35831=VERTEX_POINT ( 'NONE', #115522 ) ;
#35832=CARTESIAN_POINT ( 'NONE',  ( 10.81492255796078972, 18.62759615963270932, 114.5822429386477097 ) ) ;
#35833=CARTESIAN_POINT ( 'NONE',  ( -9.564922557961040184, 16.46253265017147172, 47.91775706135233293 ) ) ;
#35834=CARTESIAN_POINT ( 'NONE',  ( 4.483927247898545687, 16.52544592524342804, 24.79057627198103120 ) ) ;
#35835=CARTESIAN_POINT ( 'NONE',  ( -5.049401038297874678, -19.05341960407617918, 44.79275706135232582 ) ) ;
#35836=CARTESIAN_POINT ( 'NONE',  ( 19.05341960407611168, 5.049401038298154454, 108.9572429386477097 ) ) ;
#35837=CARTESIAN_POINT ( 'NONE',  ( -16.55341960407611168, -4.379528057220339221, 56.45724293864768839 ) ) ;
#35839=CARTESIAN_POINT ( 'NONE',  ( 16.51473224551069308, 9.474510206698969483, 34.16557627198102409 ) ) ;
#35840=CARTESIAN_POINT ( 'NONE',  ( 5.823673210054444382, -21.52544592524334988, 105.2094237280190328 ) ) ;
#35841=CARTESIAN_POINT ( 'NONE',  ( 8.314922557961029526, -14.29746914071037800, 90.41775706135236135 ) ) ;
#35842=CARTESIAN_POINT ( 'NONE',  ( 15.72974639402176855, 15.80617190586768217, 46.87609039468568994 ) ) ;
#35843=CARTESIAN_POINT ( 'NONE',  ( -4.483927247898782831, 16.52544592524335698, 42.70942372801901854 ) ) ;
#35844=CARTESIAN_POINT ( 'NONE',  ( 21.52544592524344225, -5.823673210054117533, 23.54057627198102765 ) ) ;
#35845=CARTESIAN_POINT ( 'NONE',  ( -9.564922557960796823, -16.46253265017161027, 57.08224293864769550 ) ) ;
#35846=CARTESIAN_POINT ( 'NONE',  ( 5.153800228976335163, 19.02544592524342804, 59.79057627198100988 ) ) ;
#35847=CARTESIAN_POINT ( 'NONE',  ( -4.379528057220086978, -16.55341960407618274, 49.79275706135234714 ) ) ;
#35848=CARTESIAN_POINT ( 'NONE',  ( 12.14591786802309770, 12.06949235617756955, 99.37390960531436690 ) ) ;
#35849=CARTESIAN_POINT ( 'NONE',  ( -8.314922557961024197, 14.29746914071037800, 112.9177570613523329 ) ) ;
#35851=CARTESIAN_POINT ( 'NONE',  ( 21.52544592524334988, 5.823673210054432836, 56.45942372801902565 ) ) ;
#35852=CARTESIAN_POINT ( 'NONE',  ( 9.564922557960805705, 16.46253265017160317, 89.58224293864769550 ) ) ;
#35853=CARTESIAN_POINT ( 'NONE',  ( 0.05219959533909260263, 19.03943276465977164, 74.99890960531435269 ) ) ;
#35854=CARTESIAN_POINT ( 'NONE',  ( 16.51473224551069308, 9.474510206698969483, 99.16557627198102409 ) ) ;
#35855=CARTESIAN_POINT ( 'NONE',  ( -8.224510206698948167, 14.34966873604960824, 40.41557627198103120 ) ) ;
#35856=CARTESIAN_POINT ( 'NONE',  ( 4.379528057220092307, 16.55341960407617563, 107.2927570613523471 ) ) ;
#35857=CARTESIAN_POINT ( 'NONE',  ( -4.483927247898539470, -16.52544592524342804, 32.29057627198102409 ) ) ;
#35860=CARTESIAN_POINT ( 'NONE',  ( -0.05219959533936034679, 19.03943276465977164, 42.50109039468566152 ) ) ;
#35861=CARTESIAN_POINT ( 'NONE',  ( -19.05341960407611168, -5.049401038298163336, 61.45724293864769550 ) ) ;
#35862=CARTESIAN_POINT ( 'NONE',  ( 5.153800228976615827, -19.02544592524334988, 55.20942372801899722 ) ) ;
#35865=CARTESIAN_POINT ( 'NONE',  ( 5.153800228976615827, -19.02544592524334988, 90.20942372801900433 ) ) ;
#35866=CARTESIAN_POINT ( 'NONE',  ( -12.06949235617739369, -12.14591786802326823, 74.37609039468568994 ) ) ;
#35867=CARTESIAN_POINT ( 'NONE',  ( 17.50000000000000711, 5.499999999999976907, 93.78230962303565832 ) ) ;
#35868=CARTESIAN_POINT ( 'NONE',  ( 0.05219959533909260263, 19.03943276465977164, 99.99890960531436690 ) ) ;
#35869=CARTESIAN_POINT ( 'NONE',  ( 21.55341960407619695, -5.719274019375665929, 26.04275706135235779 ) ) ;
#35870=CARTESIAN_POINT ( 'NONE',  ( 9.474510206698729675, 16.51473224551082808, 92.08442372801900433 ) ) ;
#35871=CARTESIAN_POINT ( 'NONE',  ( 17.05116617787825106, 6.768360034955840376, 88.84324446740805570 ) ) ;
#35872=CARTESIAN_POINT ( 'NONE',  ( 0.05219959533909260263, 19.03943276465977164, 49.99890960531435979 ) ) ;
#35873=CARTESIAN_POINT ( 'NONE',  ( 16.46253265017160672, -9.564922557960803928, 88.33224293864769550 ) ) ;
#35874=CARTESIAN_POINT ( 'NONE',  ( 16.55341960407611168, 4.379528057220329451, 48.95724293864770971 ) ) ;
#35875=CARTESIAN_POINT ( 'NONE',  ( 16.46253265017160672, -9.564922557960803928, 48.33224293864769550 ) ) ;
#35876=CARTESIAN_POINT ( 'NONE',  ( 19.05341960407617918, -5.049401038297876454, 71.04275706135234714 ) ) ;
#35877=CARTESIAN_POINT ( 'NONE',  ( -19.02544592524334988, -5.153800228976617603, 23.95942372801900078 ) ) ;
#35878=CARTESIAN_POINT ( 'NONE',  ( -13.97604488694527625, -13.89961937509977652, 71.87390960531433848 ) ) ;
#35879=CARTESIAN_POINT ( 'NONE',  ( 18.62759615963271287, -10.81492255796078972, 58.33224293864768839 ) ) ;
#35880=CARTESIAN_POINT ( 'NONE',  ( 4.483927247898545687, 16.52544592524342804, 69.79057627198102409 ) ) ;
#35881=CARTESIAN_POINT ( 'NONE',  ( 19.03943276465977164, 0.05219959533936151252, 26.25109039468566507 ) ) ;
#35882=CARTESIAN_POINT ( 'NONE',  ( 5.049401038298161559, -19.05341960407611168, 112.7072429386476813 ) ) ;
#35883=CARTESIAN_POINT ( 'NONE',  ( -18.67979575497178146, -10.72451020669898902, 31.66557627198102054 ) ) ;
#35884=CARTESIAN_POINT ( 'NONE',  ( 19.03943276465977164, -0.05219959533909143690, 53.74890960531436690 ) ) ;
#35885=CARTESIAN_POINT ( 'NONE',  ( 16.46253265017160672, -9.564922557960803928, 33.33224293864770260 ) ) ;
#35886=CARTESIAN_POINT ( 'NONE',  ( 16.52544592524342804, -4.483927247898539470, 98.54057627198105251 ) ) ;
#35887=CARTESIAN_POINT ( 'NONE',  ( 21.55341960407610458, 5.719274019375980345, 103.9572429386476813 ) ) ;
#35889=CARTESIAN_POINT ( 'NONE',  ( -10.81492255796105439, 18.62759615963255655, 27.91775706135234358 ) ) ;
#35890=CARTESIAN_POINT ( 'NONE',  ( 16.46253265017160672, -9.564922557960803928, 98.33224293864769550 ) ) ;
#35891=CARTESIAN_POINT ( 'NONE',  ( 8.314922557960818139, 14.29746914071049879, 114.5822429386477097 ) ) ;
#35892=CARTESIAN_POINT ( 'NONE',  ( 21.52544592524334988, 5.823673210054432836, 76.45942372801901854 ) ) ;
#35893=CARTESIAN_POINT ( 'NONE',  ( 10.81492255796078972, 18.62759615963270932, 94.58224293864769550 ) ) ;
#35895=CARTESIAN_POINT ( 'NONE',  ( 17.50000000000000000, -5.500000000000000888, 108.2969038253417153 ) ) ;
#35898=CARTESIAN_POINT ( 'NONE',  ( -14.34966873604972548, 8.224510206698743886, 53.33442372801901854 ) ) ;
#35899=CARTESIAN_POINT ( 'NONE',  ( 4.483927247898545687, 16.52544592524342804, 104.7905762719810241 ) ) ;
#35901=CARTESIAN_POINT ( 'NONE',  ( 5.153800228976335163, 19.02544592524342804, 54.79057627198103120 ) ) ;
#35902=CARTESIAN_POINT ( 'NONE',  ( -16.52544592524342804, 4.483927247898546575, 96.04057627198102409 ) ) ;
#35903=CARTESIAN_POINT ( 'NONE',  ( 10.81492255796078972, 18.62759615963270932, 44.58224293864769550 ) ) ;
#35904=CARTESIAN_POINT ( 'NONE',  ( -12.06949235617756955, 12.14591786802309770, 70.62390960531436690 ) ) ;
#35905=CARTESIAN_POINT ( 'NONE',  ( -8.224510206698735004, -14.34966873604973081, 19.58442372801901143 ) ) ;
#35906=CARTESIAN_POINT ( 'NONE',  ( -18.62759615963255300, -10.81492255796106328, 89.16775706135236135 ) ) ;
#35907=CARTESIAN_POINT ( 'NONE',  ( 17.12812012977029141, -6.668231424565925991, 76.14051240676856480 ) ) ;
#35908=CARTESIAN_POINT ( 'NONE',  ( -12.06949235617739369, -12.14591786802326823, 104.3760903946856899 ) ) ;
#35909=CARTESIAN_POINT ( 'NONE',  ( 16.53943276465976808, -0.05219959533910856209, 38.74890960531435979 ) ) ;
#35910=CARTESIAN_POINT ( 'NONE',  ( -13.89961937509977652, 13.97604488694528158, 40.62390960531435979 ) ) ;
#35911=CARTESIAN_POINT ( 'NONE',  ( -16.46253265017160317, 9.564922557960807481, 90.83224293864769550 ) ) ;
#35912=CARTESIAN_POINT ( 'NONE',  ( -18.62759615963270932, 10.81492255796079327, 90.83224293864769550 ) ) ;
#35913=CARTESIAN_POINT ( 'NONE',  ( 4.379528057220092307, 16.55341960407617563, 37.29275706135235424 ) ) ;
#35914=CARTESIAN_POINT ( 'NONE',  ( 8.224510206698953496, -14.34966873604960469, 67.91557627198102409 ) ) ;
#35915=CARTESIAN_POINT ( 'NONE',  ( 10.72451020669871369, 18.67979575497193778, 92.08442372801901854 ) ) ;
#35916=CARTESIAN_POINT ( 'NONE',  ( 16.53943276465976808, 0.05219959533934440121, 101.2510903946856757 ) ) ;
#35917=CARTESIAN_POINT ( 'NONE',  ( 17.31747979337963272, -6.344076630960739926, 46.12055131934818064 ) ) ;
#35918=CARTESIAN_POINT ( 'NONE',  ( 17.50000000000000000, -7.500000000000000888, 120.0000000000000142 ) ) ;
#35919=CARTESIAN_POINT ( 'NONE',  ( 0.05219959533910956823, 16.53943276465976808, 29.99890960531435979 ) ) ;
#35920=CARTESIAN_POINT ( 'NONE',  ( -16.55341960407617563, 4.379528057220093196, 73.54275706135234714 ) ) ;
#35921=CARTESIAN_POINT ( 'NONE',  ( -13.97604488694527625, -13.89961937509977652, 81.87390960531436690 ) ) ;
#35922=CARTESIAN_POINT ( 'NONE',  ( -19.05341960407611168, -5.049401038298163336, 101.4572429386476955 ) ) ;
#35923=CARTESIAN_POINT ( 'NONE',  ( 15.80617190586769283, -15.72974639402175789, 85.62609039468568994 ) ) ;
#35924=CARTESIAN_POINT ( 'NONE',  ( -12.14591786802326823, 12.06949235617739902, 93.12609039468568994 ) ) ;
#35925=CARTESIAN_POINT ( 'NONE',  ( 16.55341960407611168, 4.379528057220329451, 58.95724293864770971 ) ) ;
#35926=CARTESIAN_POINT ( 'NONE',  ( -19.03943276465977164, 0.05219959533909376836, 71.24890960531435269 ) ) ;
#35927=ORIENTED_EDGE ( 'NONE', *, *, #94206, .T. ) ;
#35928=CARTESIAN_POINT ( 'NONE',  ( 16.46253265017146816, 9.564922557961045513, 106.6677570613523471 ) ) ;
#35929=CARTESIAN_POINT ( 'NONE',  ( -0.05219959533909027116, -19.03943276465977164, 32.49890960531435979 ) ) ;
#35930=CARTESIAN_POINT ( 'NONE',  ( 5.153800228976335163, 19.02544592524342804, 79.79057627198102409 ) ) ;
#35931=CARTESIAN_POINT ( 'NONE',  ( -19.03943276465977164, -0.05219959533935918106, 113.7510903946856757 ) ) ;
#35933=CARTESIAN_POINT ( 'NONE',  ( -16.46253265017146816, -9.564922557961047289, 19.16775706135233293 ) ) ;
#35934=CARTESIAN_POINT ( 'NONE',  ( 16.55341960407618274, -4.379528057220086978, 76.04275706135237556 ) ) ;
#35935=CARTESIAN_POINT ( 'NONE',  ( -13.97604488694547697, 13.89961937509957934, 113.1260903946856757 ) ) ;
#35936=CARTESIAN_POINT ( 'NONE',  ( 5.153800228976335163, 19.02544592524342804, 24.79057627198102765 ) ) ;
#35937=CARTESIAN_POINT ( 'NONE',  ( 16.55341960407618274, -4.379528057220086978, 61.04275706135234714 ) ) ;
#35938=CARTESIAN_POINT ( 'NONE',  ( -16.55341960407617563, 4.379528057220093196, 48.54275706135234714 ) ) ;
#35939=CARTESIAN_POINT ( 'NONE',  ( -9.564922557960796823, -16.46253265017161027, 27.08224293864769550 ) ) ;
#35940=CARTESIAN_POINT ( 'NONE',  ( 13.97604488694548053, -13.89961937509957401, 70.62609039468567573 ) ) ;
#35941=CARTESIAN_POINT ( 'NONE',  ( 18.62759615963255655, 10.81492255796105972, 111.6677570613523613 ) ) ;
#35942=CARTESIAN_POINT ( 'NONE',  ( -5.049401038298153566, 19.05341960407611168, 35.20724293864768839 ) ) ;
#35943=CARTESIAN_POINT ( 'NONE',  ( 13.97604488694527802, 13.89961937509977652, 74.37390960531436690 ) ) ;
#35944=CARTESIAN_POINT ( 'NONE',  ( -16.53943276465976808, 0.05219959533911058130, 66.24890960531436690 ) ) ;
#35945=CARTESIAN_POINT ( 'NONE',  ( 19.05341960407617918, -5.049401038297876454, 36.04275706135234003 ) ) ;
#35946=CARTESIAN_POINT ( 'NONE',  ( -18.67979575497178146, -10.72451020669898902, 36.66557627198103120 ) ) ;
#35947=CARTESIAN_POINT ( 'NONE',  ( -21.55341960407619339, 5.719274019375674811, 113.5427570613523756 ) ) ;
#35948=CARTESIAN_POINT ( 'NONE',  ( 16.46253265017160672, -9.564922557960803928, 93.33224293864769550 ) ) ;
#35949=CARTESIAN_POINT ( 'NONE',  ( -10.81492255796105439, 18.62759615963255655, 112.9177570613523329 ) ) ;
#35950=CARTESIAN_POINT ( 'NONE',  ( 15.72974639402199770, -15.80617190586745480, 63.12390960531435979 ) ) ;
#35951=CARTESIAN_POINT ( 'NONE',  ( -13.89961937509977652, 13.97604488694528158, 100.6239096053143669 ) ) ;
#35952=CARTESIAN_POINT ( 'NONE',  ( 9.474510206698729675, 16.51473224551082808, 72.08442372801900433 ) ) ;
#35953=CARTESIAN_POINT ( 'NONE',  ( 13.89961937509977652, -13.97604488694527269, 98.12390960531433848 ) ) ;
#35954=CARTESIAN_POINT ( 'NONE',  ( 13.97604488694548053, -13.89961937509957401, 95.62609039468563310 ) ) ;
#35955=CARTESIAN_POINT ( 'NONE',  ( 16.55341960407611168, 4.379528057220329451, 113.9572429386477239 ) ) ;
#35956=CARTESIAN_POINT ( 'NONE',  ( -19.03943276465977164, 0.05219959533909376836, 81.24890960531436690 ) ) ;
#35957=CARTESIAN_POINT ( 'NONE',  ( 0.05219959533907565091, 21.53943276465977519, 59.99890960531436690 ) ) ;
#35958=CARTESIAN_POINT ( 'NONE',  ( -4.379528057220086978, -16.55341960407618274, 29.79275706135234358 ) ) ;
#35959=CARTESIAN_POINT ( 'NONE',  ( -10.72451020669870658, -18.67979575497194134, 29.58442372801901854 ) ) ;
#35960=CARTESIAN_POINT ( 'NONE',  ( -21.52544592524334988, -5.823673210054445271, 98.95942372801903275 ) ) ;
#35961=CARTESIAN_POINT ( 'NONE',  ( 14.29746914071037800, 8.314922557961029526, 101.6677570613523613 ) ) ;
#35962=CARTESIAN_POINT ( 'NONE',  ( -19.02544592524342804, 5.153800228976336051, 91.04057627198100988 ) ) ;
#35963=CARTESIAN_POINT ( 'NONE',  ( -12.14591786802309592, -12.06949235617757132, 96.87390960531436690 ) ) ;
#35964=CARTESIAN_POINT ( 'NONE',  ( -4.483927247898539470, -16.52544592524342804, 27.29057627198103120 ) ) ;
#35965=CARTESIAN_POINT ( 'NONE',  ( -16.51473224551082808, 9.474510206698731452, 73.33442372801900433 ) ) ;
#35966=CARTESIAN_POINT ( 'NONE',  ( -21.52544592524334988, -5.823673210054445271, 38.95942372801901854 ) ) ;
#35967=CARTESIAN_POINT ( 'NONE',  ( 14.29746914071049879, -8.314922557960816363, 88.33224293864769550 ) ) ;
#35968=CARTESIAN_POINT ( 'NONE',  ( 9.564922557960805705, 16.46253265017160317, 114.5822429386476955 ) ) ;
#35969=CARTESIAN_POINT ( 'NONE',  ( 8.224510206698742110, 14.34966873604972548, 102.0844237280190185 ) ) ;
#35970=CARTESIAN_POINT ( 'NONE',  ( 10.72451020669871369, 18.67979575497193778, 82.08442372801901854 ) ) ;
#35971=CARTESIAN_POINT ( 'NONE',  ( -16.53943276465976808, -0.05219959533934237506, 43.75109039468568284 ) ) ;
#35972=CARTESIAN_POINT ( 'NONE',  ( 18.67979575497194134, -10.72451020669871369, 35.83442372801901143 ) ) ;
#35974=CARTESIAN_POINT ( 'NONE',  ( 5.823673210054125526, 21.52544592524343514, 114.7905762719810383 ) ) ;
#35975=CARTESIAN_POINT ( 'NONE',  ( 16.53943276465976808, -0.05219959533910856209, 88.74890960531436690 ) ) ;
#35976=CARTESIAN_POINT ( 'NONE',  ( 17.50000000000002132, -3.850315288878719322, 26.76629130603451046 ) ) ;
#35977=CARTESIAN_POINT ( 'NONE',  ( 4.379528057220339221, -16.55341960407611168, 72.70724293864769550 ) ) ;
#35978=CARTESIAN_POINT ( 'NONE',  ( 16.51473224551069308, 9.474510206698969483, 59.16557627198102409 ) ) ;
#35979=CARTESIAN_POINT ( 'NONE',  ( 0.05219959533934541429, -16.53943276465976808, 100.0010903946857042 ) ) ;
#35980=CARTESIAN_POINT ( 'NONE',  ( -9.564922557960796823, -16.46253265017161027, 37.08224293864768839 ) ) ;
#35981=CARTESIAN_POINT ( 'NONE',  ( -5.823673210054116645, -21.52544592524344225, 42.29057627198103120 ) ) ;
#35982=CARTESIAN_POINT ( 'NONE',  ( 16.53943276465976808, -0.05219959533910856209, 73.74890960531433848 ) ) ;
#35983=CARTESIAN_POINT ( 'NONE',  ( -10.72451020669898014, 18.67979575497178502, 85.41557627198102409 ) ) ;
#35984=CARTESIAN_POINT ( 'NONE',  ( 13.89961937509977652, -13.97604488694527269, 88.12390960531438111 ) ) ;
#35985=CARTESIAN_POINT ( 'NONE',  ( -5.153800228976328057, -19.02544592524343514, 32.29057627198102409 ) ) ;
#35986=CARTESIAN_POINT ( 'NONE',  ( -5.049401038297874678, -19.05341960407617918, 94.79275706135230450 ) ) ;
#35987=CARTESIAN_POINT ( 'NONE',  ( 0.05219959533907565091, 21.53943276465977519, 29.99890960531435979 ) ) ;
#35988=CARTESIAN_POINT ( 'NONE',  ( -15.80617190586768217, 15.72974639402176855, 68.12609039468567573 ) ) ;
#35989=CARTESIAN_POINT ( 'NONE',  ( -9.474510206698964154, 16.51473224551069663, 50.41557627198102409 ) ) ;
#35990=CARTESIAN_POINT ( 'NONE',  ( -13.89961937509977652, 13.97604488694528158, 90.62390960531432427 ) ) ;
#35991=ORIENTED_EDGE ( 'NONE', *, *, #88626, .F. ) ;
#35992=CARTESIAN_POINT ( 'NONE',  ( -14.34966873604972548, 8.224510206698743886, 58.33442372801901143 ) ) ;
#35993=CARTESIAN_POINT ( 'NONE',  ( -21.52544592524334988, -5.823673210054445271, 48.95942372801902565 ) ) ;
#35994=CARTESIAN_POINT ( 'NONE',  ( -18.67979575497193778, 10.72451020669871902, 78.33442372801901854 ) ) ;
#35995=CARTESIAN_POINT ( 'NONE',  ( 13.97604488694527802, 13.89961937509977652, 114.3739096053143669 ) ) ;
#35996=CARTESIAN_POINT ( 'NONE',  ( 0.05219959533907565091, 21.53943276465977519, 104.9989096053143669 ) ) ;
#35997=CARTESIAN_POINT ( 'NONE',  ( -21.53943276465977519, -0.05219959533937600094, 43.75109039468568284 ) ) ;
#35998=CARTESIAN_POINT ( 'NONE',  ( 16.55341960407618274, -4.379528057220086978, 71.04275706135234714 ) ) ;
#35999=CARTESIAN_POINT ( 'NONE',  ( 10.81492255796078972, 18.62759615963270932, 64.58224293864769550 ) ) ;
#36000=CARTESIAN_POINT ( 'NONE',  ( 19.03943276465977164, 0.05219959533936151252, 36.25109039468567573 ) ) ;
#36001=CARTESIAN_POINT ( 'NONE',  ( 0.05219959533909260263, 19.03943276465977164, 69.99890960531435269 ) ) ;
#36002=CARTESIAN_POINT ( 'NONE',  ( -16.52544592524335698, -4.483927247898792601, 108.9594237280190185 ) ) ;
#36003=CARTESIAN_POINT ( 'NONE',  ( -17.49999999999999645, -3.512728167236856436, 104.7719000481888685 ) ) ;
#36004=CARTESIAN_POINT ( 'NONE',  ( 16.46253265017160672, -9.564922557960803928, 108.3322429386476955 ) ) ;
#36006=CARTESIAN_POINT ( 'NONE',  ( 0.05219959533936267826, -19.03943276465977164, 85.00109039468567573 ) ) ;
#36007=CARTESIAN_POINT ( 'NONE',  ( -21.53943276465977519, 0.05219959533907696930, 61.24890960531435979 ) ) ;
#36008=CARTESIAN_POINT ( 'NONE',  ( -8.314922557960811034, -14.29746914071050412, 32.08224293864769550 ) ) ;
#36009=CARTESIAN_POINT ( 'NONE',  ( -16.46253265017146816, -9.564922557961047289, 99.16775706135233293 ) ) ;
#36011=CARTESIAN_POINT ( 'NONE',  ( 9.564922557961047289, -16.46253265017146816, 100.4177570613523329 ) ) ;
#36012=CARTESIAN_POINT ( 'NONE',  ( -18.67979575497178146, -10.72451020669898902, 91.66557627198103830 ) ) ;
#36013=CARTESIAN_POINT ( 'NONE',  ( -5.049401038297874678, -19.05341960407617918, 54.79275706135234003 ) ) ;
#36014=CARTESIAN_POINT ( 'NONE',  ( 16.81555441253554406, 7.025013491695466961, 106.8631455466574209 ) ) ;
#36015=CARTESIAN_POINT ( 'NONE',  ( -5.153800228976328057, -19.02544592524343514, 62.29057627198100988 ) ) ;
#36016=CARTESIAN_POINT ( 'NONE',  ( 4.483927247898545687, 16.52544592524342804, 59.79057627198103120 ) ) ;
#36017=CARTESIAN_POINT ( 'NONE',  ( -19.02544592524342804, 5.153800228976336051, 46.04057627198101699 ) ) ;
#36018=CARTESIAN_POINT ( 'NONE',  ( -4.483927247898539470, -16.52544592524342804, 47.29057627198103120 ) ) ;
#36021=CARTESIAN_POINT ( 'NONE',  ( -14.29746914071049879, 8.314922557960819915, 30.83224293864770260 ) ) ;
#36022=CARTESIAN_POINT ( 'NONE',  ( 19.02544592524343514, -5.153800228976328945, 63.54057627198103830 ) ) ;
#36024=CARTESIAN_POINT ( 'NONE',  ( 5.049401038297881783, 19.05341960407617563, 42.29275706135234003 ) ) ;
#36025=CARTESIAN_POINT ( 'NONE',  ( -12.14591786802326823, 12.06949235617739902, 43.12609039468568284 ) ) ;
#36026=CARTESIAN_POINT ( 'NONE',  ( -15.72974639402197994, 15.80617190586746368, 55.62390960531436690 ) ) ;
#36027=CARTESIAN_POINT ( 'NONE',  ( 15.72974639402176855, 15.80617190586768217, 106.8760903946856899 ) ) ;
#36028=CARTESIAN_POINT ( 'NONE',  ( 0.05219959533909260263, 19.03943276465977164, 74.99890960531435269 ) ) ;
#36030=CARTESIAN_POINT ( 'NONE',  ( 5.153800228976335163, 19.02544592524342804, 114.7905762719810241 ) ) ;
#36032=CARTESIAN_POINT ( 'NONE',  ( 5.719274019375673035, 21.55341960407619339, 37.29275706135235424 ) ) ;
#36033=CARTESIAN_POINT ( 'NONE',  ( -16.55341960407611168, -4.379528057220339221, 91.45724293864769550 ) ) ;
#36034=CARTESIAN_POINT ( 'NONE',  ( -10.72451020669898014, 18.67979575497178502, 90.41557627198103830 ) ) ;
#36035=CARTESIAN_POINT ( 'NONE',  ( 5.049401038298161559, -19.05341960407611168, 87.70724293864769550 ) ) ;
#36037=CARTESIAN_POINT ( 'NONE',  ( -13.97604488694527625, -13.89961937509977652, 91.87390960531432427 ) ) ;
#36038=CARTESIAN_POINT ( 'NONE',  ( -5.823673210054431948, 21.52544592524334988, 27.70942372801901854 ) ) ;
#36040=CARTESIAN_POINT ( 'NONE',  ( 16.51473224551069308, 9.474510206698969483, 89.16557627198103830 ) ) ;
#36041=CARTESIAN_POINT ( 'NONE',  ( -18.09918380851993902, -5.499999999999988454, 76.48618307335614475 ) ) ;
#36042=CARTESIAN_POINT ( 'NONE',  ( 8.224510206698953496, -14.34966873604960469, 112.9155762719810383 ) ) ;
#36043=CARTESIAN_POINT ( 'NONE',  ( -13.97604488694527625, -13.89961937509977652, 31.87390960531435979 ) ) ;
#36044=CARTESIAN_POINT ( 'NONE',  ( 16.46253265017146816, 9.564922557961045513, 111.6677570613523329 ) ) ;
#36046=CARTESIAN_POINT ( 'NONE',  ( 12.14591786802309770, 12.06949235617756955, 114.3739096053143527 ) ) ;
#36047=CARTESIAN_POINT ( 'NONE',  ( 21.55341960407619695, -5.719274019375665929, 71.04275706135234714 ) ) ;
#36048=CARTESIAN_POINT ( 'NONE',  ( -9.564922557960796823, -16.46253265017161027, 62.08224293864769550 ) ) ;
#36049=CARTESIAN_POINT ( 'NONE',  ( -15.72974639402176322, -15.80617190586768395, 39.37609039468567573 ) ) ;
#36050=CARTESIAN_POINT ( 'NONE',  ( 21.55341960407610458, 5.719274019375980345, 108.9572429386476955 ) ) ;
#36052=CARTESIAN_POINT ( 'NONE',  ( -19.03943276465977164, 0.05219959533909376836, 81.24890960531436690 ) ) ;
#36054=CARTESIAN_POINT ( 'NONE',  ( 0.05219959533934541429, -16.53943276465976808, 20.00109039468568639 ) ) ;
#36055=CARTESIAN_POINT ( 'NONE',  ( -21.52544592524343514, 5.823673210054127303, 46.04057627198103830 ) ) ;
#36056=CARTESIAN_POINT ( 'NONE',  ( -15.80617190586768217, 15.72974639402176855, 68.12609039468567573 ) ) ;
#36057=CARTESIAN_POINT ( 'NONE',  ( -16.51473224551069308, -9.474510206698971260, 111.6655762719810383 ) ) ;
#36058=CARTESIAN_POINT ( 'NONE',  ( 19.05341960407617918, -5.049401038297876454, 91.04275706135234714 ) ) ;
#36059=CARTESIAN_POINT ( 'NONE',  ( -5.153800228976328057, -19.02544592524343514, 62.29057627198100988 ) ) ;
#36060=CARTESIAN_POINT ( 'NONE',  ( -13.97604488694527625, -13.89961937509977652, 86.87390960531436690 ) ) ;
#36061=ADVANCED_FACE ( 'NONE', ( #70016 ), #40678, .F. ) ;
#36062=CARTESIAN_POINT ( 'NONE',  ( 14.34966873604960469, 8.224510206698951720, 89.16557627198102409 ) ) ;
#36063=CARTESIAN_POINT ( 'NONE',  ( -14.34966873604960291, -8.224510206698953496, 91.66557627198103830 ) ) ;
#36064=CARTESIAN_POINT ( 'NONE',  ( 16.46253265017160672, -9.564922557960803928, 113.3322429386476955 ) ) ;
#36065=CARTESIAN_POINT ( 'NONE',  ( 8.314922557960818139, 14.29746914071049879, 54.58224293864769550 ) ) ;
#36066=CARTESIAN_POINT ( 'NONE',  ( 19.02544592524343514, -5.153800228976328945, 43.54057627198103120 ) ) ;
#36067=CARTESIAN_POINT ( 'NONE',  ( 21.52544592524334988, 5.823673210054432836, 56.45942372801902565 ) ) ;
#36068=CARTESIAN_POINT ( 'NONE',  ( 5.049401038297881783, 19.05341960407617563, 97.29275706135233293 ) ) ;
#36069=CARTESIAN_POINT ( 'NONE',  ( 14.34966873604960469, 8.224510206698951720, 64.16557627198102409 ) ) ;
#36070=CARTESIAN_POINT ( 'NONE',  ( -5.823673210054116645, -21.52544592524344225, 112.2905762719810241 ) ) ;
#36071=CARTESIAN_POINT ( 'NONE',  ( -21.52544592524343514, 5.823673210054127303, 46.04057627198103830 ) ) ;
#36072=CARTESIAN_POINT ( 'NONE',  ( 16.51473224551069308, 9.474510206698969483, 114.1655762719810241 ) ) ;
#36074=CARTESIAN_POINT ( 'NONE',  ( -0.05219959533909027116, -19.03943276465977164, 62.49890960531435979 ) ) ;
#36075=CARTESIAN_POINT ( 'NONE',  ( -14.34966873604960291, -8.224510206698953496, 41.66557627198103120 ) ) ;
#36076=CARTESIAN_POINT ( 'NONE',  ( 4.483927247898790824, -16.52544592524335698, 100.2094237280190043 ) ) ;
#36077=CARTESIAN_POINT ( 'NONE',  ( 16.55341960407618274, -4.379528057220086978, 86.04275706135236135 ) ) ;
#36078=CARTESIAN_POINT ( 'NONE',  ( -19.05341960407617563, 5.049401038297882671, 43.54275706135232582 ) ) ;
#36080=CARTESIAN_POINT ( 'NONE',  ( 13.97604488694527802, 13.89961937509977652, 94.37390960531436690 ) ) ;
#36081=CARTESIAN_POINT ( 'NONE',  ( 13.97604488694527802, 13.89961937509977652, 49.37390960531434558 ) ) ;
#36082=CARTESIAN_POINT ( 'NONE',  ( 16.55341960407611168, 4.379528057220329451, 58.95724293864770971 ) ) ;
#36083=CARTESIAN_POINT ( 'NONE',  ( 16.18388926212238488, -7.379444403734519042, 102.0604684863385074 ) ) ;
#36084=CARTESIAN_POINT ( 'NONE',  ( -21.53943276465977519, 0.05219959533907696930, 21.24890960531436690 ) ) ;
#36085=CARTESIAN_POINT ( 'NONE',  ( -5.719274019375978568, 21.55341960407610458, 35.20724293864768839 ) ) ;
#36086=CARTESIAN_POINT ( 'NONE',  ( 8.224510206698953496, -14.34966873604960469, 87.91557627198103830 ) ) ;
#36087=CARTESIAN_POINT ( 'NONE',  ( 12.14591786802327356, -12.06949235617739191, 40.62609039468567573 ) ) ;
#36088=CARTESIAN_POINT ( 'NONE',  ( -16.55341960407611168, -4.379528057220339221, 81.45724293864769550 ) ) ;
#36089=CARTESIAN_POINT ( 'NONE',  ( -19.52217212775657273, 5.500000000000114575, 64.93993709005263781 ) ) ;
#36090=CARTESIAN_POINT ( 'NONE',  ( 19.03943276465977164, 0.05219959533936151252, 81.25109039468567573 ) ) ;
#36091=CARTESIAN_POINT ( 'NONE',  ( -0.05219959533909027116, -19.03943276465977164, 112.4989096053143669 ) ) ;
#36093=CARTESIAN_POINT ( 'NONE',  ( 13.89961937509978007, -13.97604488694527269, 43.12390960531435269 ) ) ;
#36094=CARTESIAN_POINT ( 'NONE',  ( -16.55341960407617563, 4.379528057220093196, 23.54275706135235424 ) ) ;
#36095=CARTESIAN_POINT ( 'NONE',  ( -4.379528057220086978, -16.55341960407618274, 104.7927570613523898 ) ) ;
#36096=CARTESIAN_POINT ( 'NONE',  ( 5.049401038297881783, 19.05341960407617563, 72.29275706135234714 ) ) ;
#36097=CARTESIAN_POINT ( 'NONE',  ( 21.52544592524344225, -5.823673210054117533, 48.54057627198103120 ) ) ;
#36098=CARTESIAN_POINT ( 'NONE',  ( -10.72451020669870658, -18.67979575497194134, 74.58442372801901854 ) ) ;
#36100=CARTESIAN_POINT ( 'NONE',  ( -16.55341960407617563, 4.379528057220093196, 28.54275706135234358 ) ) ;
#36101=CARTESIAN_POINT ( 'NONE',  ( -0.05219959533909027116, -19.03943276465977164, 22.49890960531436690 ) ) ;
#36102=CARTESIAN_POINT ( 'NONE',  ( 9.564922557960805705, 16.46253265017160317, 89.58224293864769550 ) ) ;
#36103=CARTESIAN_POINT ( 'NONE',  ( 0.05219959533909260263, 19.03943276465977164, 24.99890960531435269 ) ) ;
#36104=CARTESIAN_POINT ( 'NONE',  ( 8.224510206698953496, -14.34966873604960469, 92.91557627198103830 ) ) ;
#36106=CARTESIAN_POINT ( 'NONE',  ( -19.02544592524342804, 5.153800228976336051, 96.04057627198103830 ) ) ;
#36108=CARTESIAN_POINT ( 'NONE',  ( -0.05219959533936034679, 19.03943276465977164, 102.5010903946856757 ) ) ;
#36109=CARTESIAN_POINT ( 'NONE',  ( -5.823673210054116645, -21.52544592524344225, 72.29057627198102409 ) ) ;
#36110=CARTESIAN_POINT ( 'NONE',  ( 16.46253265017160672, -9.564922557960803928, 38.33224293864768839 ) ) ;
#36111=CARTESIAN_POINT ( 'NONE',  ( -13.89961937509957401, -13.97604488694547875, 64.37609039468567573 ) ) ;
#36112=CARTESIAN_POINT ( 'NONE',  ( -18.67979575497178146, -10.72451020669898902, 111.6655762719810525 ) ) ;
#36113=CARTESIAN_POINT ( 'NONE',  ( -9.474510206698964154, 16.51473224551069663, 75.41557627198103830 ) ) ;
#36114=CARTESIAN_POINT ( 'NONE',  ( 16.51473224551069308, 9.474510206698969483, 104.1655762719810241 ) ) ;
#36116=CARTESIAN_POINT ( 'NONE',  ( 12.06949235617739724, 12.14591786802326823, 31.87609039468567929 ) ) ;
#36117=CARTESIAN_POINT ( 'NONE',  ( -10.81492255796078084, -18.62759615963271287, 97.08224293864770971 ) ) ;
#36118=CARTESIAN_POINT ( 'NONE',  ( -16.52544592524342804, 4.483927247898546575, 106.0405762719810525 ) ) ;
#36119=CARTESIAN_POINT ( 'NONE',  ( 16.46253265017160672, -9.564922557960803928, 98.33224293864769550 ) ) ;
#36120=CARTESIAN_POINT ( 'NONE',  ( 19.02544592524334988, 5.153800228976608722, 56.45942372801898301 ) ) ;
#36121=CARTESIAN_POINT ( 'NONE',  ( -18.62759615963270932, 10.81492255796079327, 85.83224293864768129 ) ) ;
#36122=CARTESIAN_POINT ( 'NONE',  ( 8.224510206698953496, -14.34966873604960469, 42.91557627198103120 ) ) ;
#36123=CARTESIAN_POINT ( 'NONE',  ( 15.72974639402176855, 15.80617190586768217, 111.8760903946856615 ) ) ;
#36124=CARTESIAN_POINT ( 'NONE',  ( -12.06949235617739369, -12.14591786802326823, 59.37609039468568284 ) ) ;
#36125=CARTESIAN_POINT ( 'NONE',  ( 9.474510206698971260, -16.51473224551069308, 92.91557627198103830 ) ) ;
#36126=CARTESIAN_POINT ( 'NONE',  ( -5.049401038298153566, 19.05341960407611168, 50.20724293864770260 ) ) ;
#36127=CARTESIAN_POINT ( 'NONE',  ( 15.80617190586769283, -15.72974639402175789, 55.62609039468568284 ) ) ;
#36128=CARTESIAN_POINT ( 'NONE',  ( -10.81492255796105439, 18.62759615963255655, 67.91775706135234714 ) ) ;
#36129=CARTESIAN_POINT ( 'NONE',  ( -13.97604488694527625, -13.89961937509977652, 66.87390960531436690 ) ) ;
#36130=CARTESIAN_POINT ( 'NONE',  ( 5.719274019375673035, 21.55341960407619339, 32.29275706135235424 ) ) ;
#36132=CARTESIAN_POINT ( 'NONE',  ( -16.46253265017146816, -9.564922557961047289, 69.16775706135233293 ) ) ;
#36133=CARTESIAN_POINT ( 'NONE',  ( 0.05219959533909260263, 19.03943276465977164, 34.99890960531435979 ) ) ;
#36134=CARTESIAN_POINT ( 'NONE',  ( 4.379528057220092307, 16.55341960407617563, 82.29275706135234714 ) ) ;
#36135=CARTESIAN_POINT ( 'NONE',  ( 13.97604488694527802, 13.89961937509977652, 54.37390960531435979 ) ) ;
#36136=CARTESIAN_POINT ( 'NONE',  ( -16.51473224551069308, -9.474510206698971260, 26.66557627198103120 ) ) ;
#36137=CARTESIAN_POINT ( 'NONE',  ( -9.564922557960796823, -16.46253265017161027, 112.0822429386476955 ) ) ;
#36138=CARTESIAN_POINT ( 'NONE',  ( -5.049401038298153566, 19.05341960407611168, 40.20724293864768839 ) ) ;
#36139=CARTESIAN_POINT ( 'NONE',  ( 21.55341960407610458, 5.719274019375980345, 88.95724293864769550 ) ) ;
#36140=CARTESIAN_POINT ( 'NONE',  ( 4.483927247898790824, -16.52544592524335698, 75.20942372801901854 ) ) ;
#36142=CARTESIAN_POINT ( 'NONE',  ( -19.02544592524334988, -5.153800228976617603, 28.95942372801900433 ) ) ;
#36143=CARTESIAN_POINT ( 'NONE',  ( 5.153800228976335163, 19.02544592524342804, 54.79057627198103120 ) ) ;
#36144=CARTESIAN_POINT ( 'NONE',  ( -4.379528057220328563, 16.55341960407611168, 45.20724293864769550 ) ) ;
#36145=CARTESIAN_POINT ( 'NONE',  ( 8.314922557960818139, 14.29746914071049879, 84.58224293864769550 ) ) ;
#36146=CARTESIAN_POINT ( 'NONE',  ( 5.049401038298161559, -19.05341960407611168, 97.70724293864766707 ) ) ;
#36147=CARTESIAN_POINT ( 'NONE',  ( 13.89961937509977652, -13.97604488694527269, 83.12390960531436690 ) ) ;
#36148=CARTESIAN_POINT ( 'NONE',  ( -18.67979575497193778, 10.72451020669871902, 48.33442372801902565 ) ) ;
#36149=CARTESIAN_POINT ( 'NONE',  ( -0.05219959533909027116, -19.03943276465977164, 92.49890960531436690 ) ) ;
#36150=CARTESIAN_POINT ( 'NONE',  ( -21.53943276465977519, -0.05219959533937600094, 93.75109039468567573 ) ) ;
#36151=CARTESIAN_POINT ( 'NONE',  ( 16.55341960407618274, -4.379528057220086978, 86.04275706135236135 ) ) ;
#36152=CARTESIAN_POINT ( 'NONE',  ( -10.81492255796105439, 18.62759615963255655, 27.91775706135234358 ) ) ;
#36153=CARTESIAN_POINT ( 'NONE',  ( 10.81492255796078972, 18.62759615963270932, 109.5822429386476955 ) ) ;
#36154=CARTESIAN_POINT ( 'NONE',  ( -4.483927247898539470, -16.52544592524342804, 47.29057627198103120 ) ) ;
#36155=CARTESIAN_POINT ( 'NONE',  ( -16.46253265017160317, 9.564922557960807481, 35.83224293864768839 ) ) ;
#36156=CARTESIAN_POINT ( 'NONE',  ( 12.14591786802309770, 12.06949235617756955, 64.37390960531435269 ) ) ;
#36157=CARTESIAN_POINT ( 'NONE',  ( -18.62759615963270932, 10.81492255796079327, 30.83224293864770260 ) ) ;
#36158=CARTESIAN_POINT ( 'NONE',  ( 19.03943276465977164, 0.05219959533936151252, 36.25109039468567573 ) ) ;
#36159=CARTESIAN_POINT ( 'NONE',  ( 0.05219959533910956823, 16.53943276465976808, 94.99890960531436690 ) ) ;
#36161=CARTESIAN_POINT ( 'NONE',  ( 14.34966873604972726, -8.224510206698740333, 70.83442372801901854 ) ) ;
#36162=CARTESIAN_POINT ( 'NONE',  ( 16.51473224551069308, 9.474510206698969483, 74.16557627198103830 ) ) ;
#36164=CARTESIAN_POINT ( 'NONE',  ( -18.67979575497178146, -10.72451020669898902, 41.66557627198103120 ) ) ;
#36165=CARTESIAN_POINT ( 'NONE',  ( 8.224510206698742110, 14.34966873604972548, 97.08442372801904696 ) ) ;
#36166=CARTESIAN_POINT ( 'NONE',  ( 13.89961937509957401, 13.97604488694547697, 111.8760903946856757 ) ) ;
#36167=CARTESIAN_POINT ( 'NONE',  ( 15.80617190586769283, -15.72974639402175789, 85.62609039468568994 ) ) ;
#36168=CARTESIAN_POINT ( 'NONE',  ( -0.05219959533909027116, -19.03943276465977164, 77.49890960531435269 ) ) ;
#36169=CARTESIAN_POINT ( 'NONE',  ( -10.81492255796078084, -18.62759615963271287, 102.0822429386476955 ) ) ;
#36170=CARTESIAN_POINT ( 'NONE',  ( 12.14591786802327356, -12.06949235617739191, 55.62609039468568284 ) ) ;
#36171=CARTESIAN_POINT ( 'NONE',  ( 13.89961937509977652, -13.97604488694527269, 23.12390960531436335 ) ) ;
#36172=CARTESIAN_POINT ( 'NONE',  ( -8.314922557961024197, 14.29746914071037800, 22.91775706135235069 ) ) ;
#36173=CARTESIAN_POINT ( 'NONE',  ( -9.564922557961040184, 16.46253265017147172, 82.91775706135233293 ) ) ;
#36174=CARTESIAN_POINT ( 'NONE',  ( -18.62759615963270932, 10.81492255796079327, 80.83224293864769550 ) ) ;
#36175=CARTESIAN_POINT ( 'NONE',  ( 19.03943276465977164, 0.05219959533936151252, 56.25109039468566863 ) ) ;
#36177=CARTESIAN_POINT ( 'NONE',  ( 15.72974639402199770, -15.80617190586745480, 98.12390960531436690 ) ) ;
#36179=CARTESIAN_POINT ( 'NONE',  ( -0.05219959533909027116, -19.03943276465977164, 77.49890960531435269 ) ) ;
#36180=CARTESIAN_POINT ( 'NONE',  ( -8.314922557961024197, 14.29746914071037800, 27.91775706135234358 ) ) ;
#36182=CARTESIAN_POINT ( 'NONE',  ( 5.719274019375991003, -21.55341960407610458, 97.70724293864772392 ) ) ;
#36183=CARTESIAN_POINT ( 'NONE',  ( -16.52544592524342804, 4.483927247898546575, 66.04057627198103830 ) ) ;
#36184=CARTESIAN_POINT ( 'NONE',  ( 9.564922557960805705, 16.46253265017160317, 64.58224293864769550 ) ) ;
#36185=CARTESIAN_POINT ( 'NONE',  ( 10.72451020669871369, 18.67979575497193778, 87.08442372801901854 ) ) ;
#36186=CARTESIAN_POINT ( 'NONE',  ( -12.06949235617739369, -12.14591786802326823, 44.37609039468567573 ) ) ;
#36187=CARTESIAN_POINT ( 'NONE',  ( -19.03943276465977164, -0.05219959533935918106, 38.75109039468566152 ) ) ;
#36188=CARTESIAN_POINT ( 'NONE',  ( -21.53943276465977519, -0.05219959533937600094, 58.75109039468568994 ) ) ;
#36189=CARTESIAN_POINT ( 'NONE',  ( 21.55341960407610458, 5.719274019375980345, 53.95724293864770260 ) ) ;
#36190=CARTESIAN_POINT ( 'NONE',  ( 16.46253265017146816, 9.564922557961045513, 111.6677570613523329 ) ) ;
#36191=CARTESIAN_POINT ( 'NONE',  ( -19.05341960407611168, -5.049401038298163336, 51.45724293864770260 ) ) ;
#36192=CARTESIAN_POINT ( 'NONE',  ( -19.02544592524334988, -5.153800228976617603, 68.95942372801896170 ) ) ;
#36193=CARTESIAN_POINT ( 'NONE',  ( -10.81492255796105439, 18.62759615963255655, 87.91775706135234714 ) ) ;
#36194=CARTESIAN_POINT ( 'NONE',  ( 16.46253265017146816, 9.564922557961045513, 71.66775706135233293 ) ) ;
#36195=CARTESIAN_POINT ( 'NONE',  ( 9.474510206698971260, -16.51473224551069308, 32.91557627198102409 ) ) ;
#36196=CARTESIAN_POINT ( 'NONE',  ( 21.52544592524344225, -5.823673210054117533, 63.54057627198103830 ) ) ;
#36197=CARTESIAN_POINT ( 'NONE',  ( 12.06949235617757843, -12.14591786802309237, 68.12390960531436690 ) ) ;
#36199=CARTESIAN_POINT ( 'NONE',  ( -5.049401038297874678, -19.05341960407617918, 34.79275706135233293 ) ) ;
#36200=CARTESIAN_POINT ( 'NONE',  ( 14.34966873604972726, -8.224510206698740333, 85.83442372801901854 ) ) ;
#36201=CARTESIAN_POINT ( 'NONE',  ( -16.53943276465976808, 0.05219959533911058130, 56.24890960531436690 ) ) ;
#36202=CARTESIAN_POINT ( 'NONE',  ( 0.05219959533937995610, -21.53943276465977519, 85.00109039468568994 ) ) ;
#36203=CARTESIAN_POINT ( 'NONE',  ( -21.55341960407619339, 5.719274019375674811, 78.54275706135236135 ) ) ;
#36204=CARTESIAN_POINT ( 'NONE',  ( -0.05219959533907301413, -21.53943276465977519, 92.49890960531436690 ) ) ;
#36205=CARTESIAN_POINT ( 'NONE',  ( 9.474510206698971260, -16.51473224551069308, 47.91557627198102409 ) ) ;
#36206=CARTESIAN_POINT ( 'NONE',  ( -10.72451020669870658, -18.67979575497194134, 69.58442372801900433 ) ) ;
#36207=CARTESIAN_POINT ( 'NONE',  ( 19.02544592524343514, -5.153800228976328945, 38.54057627198103120 ) ) ;
#36209=CARTESIAN_POINT ( 'NONE',  ( -9.474510206698964154, 16.51473224551069663, 60.41557627198102409 ) ) ;
#36210=CARTESIAN_POINT ( 'NONE',  ( -12.14591786802309592, -12.06949235617757132, 106.8739096053143811 ) ) ;
#36211=CARTESIAN_POINT ( 'NONE',  ( -5.049401038298153566, 19.05341960407611168, 95.20724293864770971 ) ) ;
#36212=CARTESIAN_POINT ( 'NONE',  ( -8.224510206698948167, 14.34966873604960824, 50.41557627198103120 ) ) ;
#36213=CARTESIAN_POINT ( 'NONE',  ( 12.14591786802309770, 12.06949235617756955, 109.3739096053143811 ) ) ;
#36214=CARTESIAN_POINT ( 'NONE',  ( 10.81492255796078972, 18.62759615963270932, 84.58224293864769550 ) ) ;
#36215=CARTESIAN_POINT ( 'NONE',  ( -5.823673210054431948, 21.52544592524334988, 37.70942372801900433 ) ) ;
#36217=CARTESIAN_POINT ( 'NONE',  ( -12.06949235617739369, -12.14591786802326823, 39.37609039468567573 ) ) ;
#36218=CARTESIAN_POINT ( 'NONE',  ( 0.05219959533907565091, 21.53943276465977519, 89.99890960531438111 ) ) ;
#36220=CARTESIAN_POINT ( 'NONE',  ( 15.72974639402176855, 15.80617190586768217, 101.8760903946857042 ) ) ;
#36221=CARTESIAN_POINT ( 'NONE',  ( -19.05341960407611168, -5.049401038298163336, 96.45724293864769550 ) ) ;
#36222=CARTESIAN_POINT ( 'NONE',  ( -10.81492255796105439, 18.62759615963255655, 32.91775706135234714 ) ) ;
#36224=CARTESIAN_POINT ( 'NONE',  ( 10.72451020669898902, -18.67979575497178502, 32.91557627198102409 ) ) ;
#36225=CARTESIAN_POINT ( 'NONE',  ( -0.05219959533934338120, 16.53943276465976808, 102.5010903946856899 ) ) ;
#36226=CARTESIAN_POINT ( 'NONE',  ( -10.72451020669870658, -18.67979575497194134, 54.58442372801901143 ) ) ;
#36227=CARTESIAN_POINT ( 'NONE',  ( -18.67979575497193778, 10.72451020669871902, 88.33442372801901854 ) ) ;
#36228=CARTESIAN_POINT ( 'NONE',  ( 16.46253265017146816, 9.564922557961045513, 21.66775706135233648 ) ) ;
#36229=CARTESIAN_POINT ( 'NONE',  ( 0.05219959533934541429, -16.53943276465976808, 75.00109039468568994 ) ) ;
#36230=CARTESIAN_POINT ( 'NONE',  ( -18.67979575497193778, 10.72451020669871902, 38.33442372801900433 ) ) ;
#36231=CARTESIAN_POINT ( 'NONE',  ( -19.03943276465977164, 0.05219959533909376836, 31.24890960531435979 ) ) ;
#36232=CARTESIAN_POINT ( 'NONE',  ( 18.62759615963255655, 10.81492255796105972, 101.6677570613523613 ) ) ;
#36233=CARTESIAN_POINT ( 'NONE',  ( 16.51473224551069308, 9.474510206698969483, 104.1655762719810241 ) ) ;
#36234=CARTESIAN_POINT ( 'NONE',  ( 21.52544592524344225, -5.823673210054117533, 103.5405762719810383 ) ) ;
#36236=CARTESIAN_POINT ( 'NONE',  ( 18.62759615963271287, -10.81492255796078972, 73.33224293864769550 ) ) ;
#36237=CARTESIAN_POINT ( 'NONE',  ( -12.14591786802326823, 12.06949235617739902, 53.12609039468568284 ) ) ;
#36238=CARTESIAN_POINT ( 'NONE',  ( 12.14591786802309770, 12.06949235617756955, 49.37390960531436690 ) ) ;
#36240=CARTESIAN_POINT ( 'NONE',  ( -0.05219959533936034679, 19.03943276465977164, 92.50109039468566152 ) ) ;
#36242=CARTESIAN_POINT ( 'NONE',  ( 0.05219959533934541429, -16.53943276465976808, 25.00109039468567218 ) ) ;
#36243=CARTESIAN_POINT ( 'NONE',  ( 15.72974639402199770, -15.80617190586745480, 98.12390960531436690 ) ) ;
#36244=CARTESIAN_POINT ( 'NONE',  ( -15.72974639402197994, 15.80617190586746368, 70.62390960531436690 ) ) ;
#36245=CARTESIAN_POINT ( 'NONE',  ( -0.05219959533909027116, -19.03943276465977164, 107.4989096053143527 ) ) ;
#36246=CARTESIAN_POINT ( 'NONE',  ( 4.483927247898790824, -16.52544592524335698, 50.20942372801901854 ) ) ;
#36247=CARTESIAN_POINT ( 'NONE',  ( 5.153800228976335163, 19.02544592524342804, 64.79057627198100988 ) ) ;
#36248=CARTESIAN_POINT ( 'NONE',  ( -21.53943276465977519, -0.05219959533937600094, 23.75109039468567929 ) ) ;
#36249=CARTESIAN_POINT ( 'NONE',  ( 9.564922557961047289, -16.46253265017146816, 100.4177570613523329 ) ) ;
#36250=CARTESIAN_POINT ( 'NONE',  ( 16.46253265017160672, -9.564922557960803928, 113.3322429386476955 ) ) ;
#36251=CARTESIAN_POINT ( 'NONE',  ( -19.05341960407611168, -5.049401038298163336, 81.45724293864769550 ) ) ;
#36252=CARTESIAN_POINT ( 'NONE',  ( 10.72451020669898902, -18.67979575497178502, 92.91557627198103830 ) ) ;
#36253=CARTESIAN_POINT ( 'NONE',  ( -19.03943276465977164, 0.05219959533909376836, 61.24890960531436690 ) ) ;
#36254=DIRECTION ( 'NONE',  ( 1.000000000000000000, 0.000000000000000000, 0.000000000000000000 ) ) ;
#36255=CARTESIAN_POINT ( 'NONE',  ( -16.53943276465976808, 0.05219959533911058130, 71.24890960531435269 ) ) ;
#36256=CARTESIAN_POINT ( 'NONE',  ( 5.049401038298161559, -19.05341960407611168, 112.7072429386476813 ) ) ;
#36258=CARTESIAN_POINT ( 'NONE',  ( -21.55341960407610458, -5.719274019375992779, 96.45724293864770971 ) ) ;
#36259=CARTESIAN_POINT ( 'NONE',  ( 5.049401038297881783, 19.05341960407617563, 47.29275706135231161 ) ) ;
#36260=CARTESIAN_POINT ( 'NONE',  ( -9.564922557960796823, -16.46253265017161027, 112.0822429386476955 ) ) ;
#36262=CARTESIAN_POINT ( 'NONE',  ( -15.80617190586745835, -15.72974639402198527, 51.87390960531437401 ) ) ;
#36263=CARTESIAN_POINT ( 'NONE',  ( 5.049401038298161559, -19.05341960407611168, 82.70724293864770971 ) ) ;
#36264=CARTESIAN_POINT ( 'NONE',  ( 5.823673210054444382, -21.52544592524334988, 80.20942372801901854 ) ) ;
#36265=CARTESIAN_POINT ( 'NONE',  ( -16.51473224551069308, -9.474510206698971260, 36.66557627198102409 ) ) ;
#36266=CARTESIAN_POINT ( 'NONE',  ( 12.14591786802309770, 12.06949235617756955, 69.37390960531436690 ) ) ;
#36267=CARTESIAN_POINT ( 'NONE',  ( 8.224510206698742110, 14.34966873604972548, 22.08442372801901143 ) ) ;
#36268=CARTESIAN_POINT ( 'NONE',  ( 10.72451020669871369, 18.67979575497193778, 62.08442372801901143 ) ) ;
#36270=CARTESIAN_POINT ( 'NONE',  ( 16.46253265017146816, 9.564922557961045513, 26.66775706135234003 ) ) ;
#36271=CARTESIAN_POINT ( 'NONE',  ( 16.46253265017146816, 9.564922557961045513, 76.66775706135234714 ) ) ;
#36273=CARTESIAN_POINT ( 'NONE',  ( -21.53943276465977519, -0.05219959533937600094, 18.75109039468568639 ) ) ;
#36274=CARTESIAN_POINT ( 'NONE',  ( -18.22780087662126647, -5.499999999999827693, 43.98236817873107185 ) ) ;
#36275=CARTESIAN_POINT ( 'NONE',  ( -21.55341960407619339, 5.719274019375674811, 108.5427570613523756 ) ) ;
#36276=CARTESIAN_POINT ( 'NONE',  ( 16.51473224551069308, 9.474510206698969483, 54.16557627198103120 ) ) ;
#36277=CARTESIAN_POINT ( 'NONE',  ( 0.05219959533936267826, -19.03943276465977164, 35.00109039468566863 ) ) ;
#36278=CARTESIAN_POINT ( 'NONE',  ( -8.224510206698735004, -14.34966873604973081, 109.5844237280190328 ) ) ;
#36279=CARTESIAN_POINT ( 'NONE',  ( -19.05341960407611168, -5.049401038298163336, 101.4572429386476955 ) ) ;
#36280=CARTESIAN_POINT ( 'NONE',  ( -0.05219959533937732626, 21.53943276465977519, 67.50109039468568994 ) ) ;
#36283=CARTESIAN_POINT ( 'NONE',  ( 15.72974639402176855, 15.80617190586768217, 81.87609039468568994 ) ) ;
#36284=CARTESIAN_POINT ( 'NONE',  ( -5.719274019375665041, -21.55341960407619695, 104.7927570613523898 ) ) ;
#36286=CARTESIAN_POINT ( 'NONE',  ( 13.89961937509977652, -13.97604488694527269, 103.1239096053143527 ) ) ;
#36287=CARTESIAN_POINT ( 'NONE',  ( 5.153800228976615827, -19.02544592524334988, 25.20942372801900433 ) ) ;
#36288=CARTESIAN_POINT ( 'NONE',  ( 15.50000000000000178, 5.499999999999998224, 118.0000000000000142 ) ) ;
#36289=CARTESIAN_POINT ( 'NONE',  ( -5.153800228976328057, -19.02544592524343514, 42.29057627198101699 ) ) ;
#36290=CARTESIAN_POINT ( 'NONE',  ( -21.52544592524343514, 5.823673210054127303, 56.04057627198102409 ) ) ;
#36291=CARTESIAN_POINT ( 'NONE',  ( 8.314922557960818139, 14.29746914071049879, 24.58224293864768839 ) ) ;
#36292=CARTESIAN_POINT ( 'NONE',  ( -12.06949235617756955, 12.14591786802309770, 90.62390960531436690 ) ) ;
#36293=CARTESIAN_POINT ( 'NONE',  ( -9.564922557960796823, -16.46253265017161027, 82.08224293864768129 ) ) ;
#36294=CARTESIAN_POINT ( 'NONE',  ( -21.52544592524334988, -5.823673210054445271, 108.9594237280190185 ) ) ;
#36295=EDGE_CURVE ( 'NONE', #129907, #49283, #46983, .T. ) ;
#36296=CARTESIAN_POINT ( 'NONE',  ( -19.02544592524342804, 5.153800228976336051, 41.04057627198103120 ) ) ;
#36297=CARTESIAN_POINT ( 'NONE',  ( -12.06949235617756955, 12.14591786802309770, 105.6239096053143669 ) ) ;
#36298=CARTESIAN_POINT ( 'NONE',  ( -21.55341960407619339, 5.719274019375674811, 58.54275706135235424 ) ) ;
#36299=CARTESIAN_POINT ( 'NONE',  ( 21.52544592524344225, -5.823673210054117533, 93.54057627198103830 ) ) ;
#36300=CARTESIAN_POINT ( 'NONE',  ( -13.97604488694547697, 13.89961937509957934, 53.12609039468565442 ) ) ;
#36302=CARTESIAN_POINT ( 'NONE',  ( 5.153800228976335163, 19.02544592524342804, 109.7905762719810099 ) ) ;
#36303=CARTESIAN_POINT ( 'NONE',  ( 4.379528057220339221, -16.55341960407611168, 72.70724293864769550 ) ) ;
#36304=CARTESIAN_POINT ( 'NONE',  ( -16.51473224551082808, 9.474510206698731452, 43.33442372801900433 ) ) ;
#36305=CARTESIAN_POINT ( 'NONE',  ( 9.474510206698971260, -16.51473224551069308, 62.91557627198102409 ) ) ;
#36306=CARTESIAN_POINT ( 'NONE',  ( -14.34966873604960291, -8.224510206698953496, 51.66557627198102409 ) ) ;
#36307=CARTESIAN_POINT ( 'NONE',  ( 5.049401038297881783, 19.05341960407617563, 77.29275706135231871 ) ) ;
#36308=CARTESIAN_POINT ( 'NONE',  ( 17.71576930673726835, -5.499999999999973355, 101.0825735056735368 ) ) ;
#36309=CARTESIAN_POINT ( 'NONE',  ( 15.72974639402199770, -15.80617190586745480, 38.12390960531436690 ) ) ;
#36311=CARTESIAN_POINT ( 'NONE',  ( 4.483927247898545687, 16.52544592524342804, 94.79057627198105251 ) ) ;
#36313=CARTESIAN_POINT ( 'NONE',  ( -19.02544592524342804, 5.153800228976336051, 61.04057627198103120 ) ) ;
#36314=CARTESIAN_POINT ( 'NONE',  ( 5.719274019375991003, -21.55341960407610458, 62.70724293864769550 ) ) ;
#36315=CARTESIAN_POINT ( 'NONE',  ( 16.46253265017160672, -9.564922557960803928, 33.33224293864770260 ) ) ;
#36316=CARTESIAN_POINT ( 'NONE',  ( -16.52544592524335698, -4.483927247898792601, 73.95942372801901854 ) ) ;
#36317=CARTESIAN_POINT ( 'NONE',  ( 16.46253265017160672, -9.564922557960803928, 58.33224293864769550 ) ) ;
#36318=CARTESIAN_POINT ( 'NONE',  ( -19.03943276465977164, -0.05219959533935918106, 48.75109039468566863 ) ) ;
#36319=CARTESIAN_POINT ( 'NONE',  ( -10.72451020669870658, -18.67979575497194134, 74.58442372801901854 ) ) ;
#36320=CARTESIAN_POINT ( 'NONE',  ( 21.52544592524344225, -5.823673210054117533, 43.54057627198103830 ) ) ;
#36321=CARTESIAN_POINT ( 'NONE',  ( 5.049401038298161559, -19.05341960407611168, 27.70724293864769550 ) ) ;
#36322=CARTESIAN_POINT ( 'NONE',  ( -0.05219959533934338120, 16.53943276465976808, 87.50109039468568994 ) ) ;
#36323=CARTESIAN_POINT ( 'NONE',  ( 9.564922557961047289, -16.46253265017146816, 100.4177570613523329 ) ) ;
#36325=CARTESIAN_POINT ( 'NONE',  ( 19.39720447994795904, 5.499999999999970690, 77.16317477297180005 ) ) ;
#36326=CARTESIAN_POINT ( 'NONE',  ( -21.53943276465977519, 0.05219959533907696930, 61.24890960531435979 ) ) ;
#36327=CARTESIAN_POINT ( 'NONE',  ( 18.67979575497194134, -10.72451020669871369, 95.83442372801903275 ) ) ;
#36329=CARTESIAN_POINT ( 'NONE',  ( -12.06949235617756955, 12.14591786802309770, 50.62390960531435979 ) ) ;
#36330=CARTESIAN_POINT ( 'NONE',  ( -12.06949235617756955, 12.14591786802309770, 60.62390960531437401 ) ) ;
#36331=CARTESIAN_POINT ( 'NONE',  ( 5.823673210054125526, 21.52544592524343514, 79.79057627198102409 ) ) ;
#36332=CARTESIAN_POINT ( 'NONE',  ( -5.719274019375978568, 21.55341960407610458, 85.20724293864770971 ) ) ;
#36333=CARTESIAN_POINT ( 'NONE',  ( 17.50000000000000000, -5.499999999999992895, 76.21769037696435589 ) ) ;
#36334=CARTESIAN_POINT ( 'NONE',  ( -21.52544592524343514, 5.823673210054127303, 31.04057627198102409 ) ) ;
#36335=CARTESIAN_POINT ( 'NONE',  ( -12.14591786802326823, 12.06949235617739902, 68.12609039468567573 ) ) ;
#36336=CARTESIAN_POINT ( 'NONE',  ( 16.55341960407611168, 4.379528057220329451, 73.95724293864769550 ) ) ;
#36337=CARTESIAN_POINT ( 'NONE',  ( 16.46253265017160672, -9.564922557960803928, 48.33224293864769550 ) ) ;
#36339=VERTEX_POINT ( 'NONE', #12353 ) ;
#36340=CARTESIAN_POINT ( 'NONE',  ( 4.379528057220092307, 16.55341960407617563, 92.29275706135236135 ) ) ;
#36341=CARTESIAN_POINT ( 'NONE',  ( 18.67979575497194134, -10.72451020669871369, 25.83442372801901499 ) ) ;
#36342=CARTESIAN_POINT ( 'NONE',  ( 9.474510206698971260, -16.51473224551069308, 77.91557627198103830 ) ) ;
#36343=CARTESIAN_POINT ( 'NONE',  ( -15.80617190586768217, 15.72974639402176855, 48.12609039468568284 ) ) ;
#36344=CARTESIAN_POINT ( 'NONE',  ( -0.05219959533909027116, -19.03943276465977164, 107.4989096053143527 ) ) ;
#36347=CARTESIAN_POINT ( 'NONE',  ( 18.62759615963255655, 10.81492255796105972, 51.66775706135234714 ) ) ;
#36348=CARTESIAN_POINT ( 'NONE',  ( -5.153800228976328057, -19.02544592524343514, 42.29057627198101699 ) ) ;
#36349=CARTESIAN_POINT ( 'NONE',  ( -19.05341960407611168, -5.049401038298163336, 106.4572429386476955 ) ) ;
#36350=CARTESIAN_POINT ( 'NONE',  ( 9.564922557961047289, -16.46253265017146816, 55.41775706135234003 ) ) ;
#36351=CARTESIAN_POINT ( 'NONE',  ( 5.823673210054444382, -21.52544592524334988, 35.20942372801901854 ) ) ;
#36352=CARTESIAN_POINT ( 'NONE',  ( -19.02544592524334988, -5.153800228976617603, 58.95942372801900433 ) ) ;
#36353=CARTESIAN_POINT ( 'NONE',  ( -19.03943276465977164, 0.05219959533909376836, 21.24890960531436335 ) ) ;
#36354=CARTESIAN_POINT ( 'NONE',  ( -16.55341960407617563, 4.379528057220093196, 93.54275706135234714 ) ) ;
#36355=CARTESIAN_POINT ( 'NONE',  ( 13.89961937509957401, 13.97604488694547697, 66.87609039468567573 ) ) ;
#36356=CARTESIAN_POINT ( 'NONE',  ( 8.314922557961029526, -14.29746914071037800, 110.4177570613523756 ) ) ;
#36357=CARTESIAN_POINT ( 'NONE',  ( 18.22780087662122739, 5.500000000000000888, 86.48236817873107896 ) ) ;
#36358=CARTESIAN_POINT ( 'NONE',  ( 5.049401038298161559, -19.05341960407611168, 87.70724293864769550 ) ) ;
#36359=CARTESIAN_POINT ( 'NONE',  ( 18.62759615963255655, 10.81492255796105972, 86.66775706135234714 ) ) ;
#36360=CARTESIAN_POINT ( 'NONE',  ( 5.823673210054444382, -21.52544592524334988, 110.2094237280190185 ) ) ;
#36362=CARTESIAN_POINT ( 'NONE',  ( -19.03943276465977164, 0.05219959533909376836, 101.2489096053143669 ) ) ;
#36363=CARTESIAN_POINT ( 'NONE',  ( 10.81492255796106328, -18.62759615963255655, 70.41775706135236135 ) ) ;
#36364=CARTESIAN_POINT ( 'NONE',  ( -4.379528057220086978, -16.55341960407618274, 19.79275706135235069 ) ) ;
#36365=CARTESIAN_POINT ( 'NONE',  ( -19.02544592524342804, 5.153800228976336051, 86.04057627198103830 ) ) ;
#36366=CARTESIAN_POINT ( 'NONE',  ( -5.823673210054116645, -21.52544592524344225, 32.29057627198102409 ) ) ;
#36367=CARTESIAN_POINT ( 'NONE',  ( 13.97604488694527802, 13.89961937509977652, 99.37390960531436690 ) ) ;
#36368=LINE ( 'NONE', #33405, #111259 ) ;
#36369=CARTESIAN_POINT ( 'NONE',  ( -5.049401038298153566, 19.05341960407611168, 65.20724293864765286 ) ) ;
#36370=CARTESIAN_POINT ( 'NONE',  ( -16.53943276465976808, -0.05219959533934237506, 113.7510903946856757 ) ) ;
#36371=CARTESIAN_POINT ( 'NONE',  ( -19.49671883438228903, -5.499999999999981348, 39.89279849105682985 ) ) ;
#36372=CARTESIAN_POINT ( 'NONE',  ( -19.03943276465977164, -0.05219959533935918106, 73.75109039468566152 ) ) ;
#36373=CARTESIAN_POINT ( 'NONE',  ( 19.03943276465977164, -0.05219959533909143690, 93.74890960531435269 ) ) ;
#36374=CARTESIAN_POINT ( 'NONE',  ( -14.29746914071049879, 8.314922557960819915, 85.83224293864768129 ) ) ;
#36375=CARTESIAN_POINT ( 'NONE',  ( 15.72974639402199770, -15.80617190586745480, 43.12390960531435269 ) ) ;
#36376=CARTESIAN_POINT ( 'NONE',  ( 15.80617190586746368, 15.72974639402197994, 24.37390960531435979 ) ) ;
#36377=CARTESIAN_POINT ( 'NONE',  ( -8.314922557960811034, -14.29746914071050412, 107.0822429386476955 ) ) ;
#36378=CARTESIAN_POINT ( 'NONE',  ( -17.05116617787826883, 6.768360034955680504, 53.65675553259199404 ) ) ;
#36379=CARTESIAN_POINT ( 'NONE',  ( 5.153800228976615827, -19.02544592524334988, 50.20942372801897591 ) ) ;
#36380=CARTESIAN_POINT ( 'NONE',  ( -16.55341960407611168, -4.379528057220339221, 31.45724293864769550 ) ) ;
#36381=CARTESIAN_POINT ( 'NONE',  ( 13.89961937509977652, -13.97604488694527269, 108.1239096053143669 ) ) ;
#36382=CARTESIAN_POINT ( 'NONE',  ( -10.81492255796105439, 18.62759615963255655, 62.91775706135236135 ) ) ;
#36383=CARTESIAN_POINT ( 'NONE',  ( 5.823673210054125526, 21.52544592524343514, 59.79057627198103120 ) ) ;
#36384=CARTESIAN_POINT ( 'NONE',  ( 18.62759615963255655, 10.81492255796105972, 41.66775706135235424 ) ) ;
#36385=CARTESIAN_POINT ( 'NONE',  ( -5.823673210054116645, -21.52544592524344225, 102.2905762719810383 ) ) ;
#36386=CARTESIAN_POINT ( 'NONE',  ( 5.719274019375673035, 21.55341960407619339, 37.29275706135235424 ) ) ;
#36387=CARTESIAN_POINT ( 'NONE',  ( 12.06949235617757843, -12.14591786802309237, 103.1239096053143811 ) ) ;
#36388=CARTESIAN_POINT ( 'NONE',  ( 19.05341960407617918, -5.049401038297876454, 66.04275706135233293 ) ) ;
#36389=CARTESIAN_POINT ( 'NONE',  ( -19.05341960407611168, -5.049401038298163336, 41.45724293864769550 ) ) ;
#36390=CARTESIAN_POINT ( 'NONE',  ( 16.53943276465976808, -0.05219959533910856209, 103.7489096053143669 ) ) ;
#36391=CARTESIAN_POINT ( 'NONE',  ( -16.46253265017160317, 9.564922557960807481, 105.8322429386476955 ) ) ;
#36392=CARTESIAN_POINT ( 'NONE',  ( 14.34966873604960469, 8.224510206698951720, 39.16557627198102409 ) ) ;
#36393=CARTESIAN_POINT ( 'NONE',  ( -12.14591786802326823, 12.06949235617739902, 113.1260903946856899 ) ) ;
#36394=CARTESIAN_POINT ( 'NONE',  ( -0.05219959533909027116, -19.03943276465977164, 52.49890960531436690 ) ) ;
#36395=CARTESIAN_POINT ( 'NONE',  ( 19.05341960407611168, 5.049401038298154454, 23.95724293864769194 ) ) ;
#36396=CARTESIAN_POINT ( 'NONE',  ( -21.53943276465977519, -0.05219959533937600094, 113.7510903946856757 ) ) ;
#36397=CARTESIAN_POINT ( 'NONE',  ( 17.72560187377285601, 5.500000000000048850, 51.57814504131321343 ) ) ;
#36398=CARTESIAN_POINT ( 'NONE',  ( -16.55341960407611168, -4.379528057220339221, 41.45724293864769550 ) ) ;
#36399=CARTESIAN_POINT ( 'NONE',  ( -0.05219959533937732626, 21.53943276465977519, 42.50109039468567573 ) ) ;
#36401=CARTESIAN_POINT ( 'NONE',  ( 12.06949235617739724, 12.14591786802326823, 56.87609039468568994 ) ) ;
#36402=CARTESIAN_POINT ( 'NONE',  ( -14.29746914071049879, 8.314922557960819915, 25.83224293864769194 ) ) ;
#36403=CARTESIAN_POINT ( 'NONE',  ( 8.224510206698742110, 14.34966873604972548, 102.0844237280190185 ) ) ;
#36404=CARTESIAN_POINT ( 'NONE',  ( -12.06949235617739369, -12.14591786802326823, 29.37609039468568284 ) ) ;
#36405=CARTESIAN_POINT ( 'NONE',  ( 9.564922557960805705, 16.46253265017160317, 49.58224293864770260 ) ) ;
#36406=CARTESIAN_POINT ( 'NONE',  ( -0.05219959533909027116, -19.03943276465977164, 27.49890960531435624 ) ) ;
#36407=CARTESIAN_POINT ( 'NONE',  ( -5.823673210054431948, 21.52544592524334988, 22.70942372801901499 ) ) ;
#36408=CARTESIAN_POINT ( 'NONE',  ( -9.564922557960796823, -16.46253265017161027, 42.08224293864769550 ) ) ;
#36410=CARTESIAN_POINT ( 'NONE',  ( -19.03943276465977164, 0.05219959533909376836, 36.24890960531436690 ) ) ;
#36412=CARTESIAN_POINT ( 'NONE',  ( -15.72974639402197994, 15.80617190586746368, 25.62390960531435624 ) ) ;
#36414=CARTESIAN_POINT ( 'NONE',  ( -5.719274019375665041, -21.55341960407619695, 44.79275706135234714 ) ) ;
#36415=CARTESIAN_POINT ( 'NONE',  ( -16.52544592524342804, 4.483927247898546575, 106.0405762719810525 ) ) ;
#36416=CARTESIAN_POINT ( 'NONE',  ( -19.05341960407611168, -5.049401038298163336, 106.4572429386476955 ) ) ;
#36417=CARTESIAN_POINT ( 'NONE',  ( 14.29746914071037800, 8.314922557961029526, 81.66775706135236135 ) ) ;
#36418=CARTESIAN_POINT ( 'NONE',  ( 5.719274019375673035, 21.55341960407619339, 97.29275706135234714 ) ) ;
#36419=CARTESIAN_POINT ( 'NONE',  ( -4.379528057220086978, -16.55341960407618274, 59.79275706135234714 ) ) ;
#36420=CARTESIAN_POINT ( 'NONE',  ( 13.97604488694527802, 13.89961937509977652, 99.37390960531436690 ) ) ;
#36422=CARTESIAN_POINT ( 'NONE',  ( 8.314922557961029526, -14.29746914071037800, 45.41775706135234003 ) ) ;
#36423=CARTESIAN_POINT ( 'NONE',  ( -16.52544592524335698, -4.483927247898792601, 28.95942372801902209 ) ) ;
#36424=CARTESIAN_POINT ( 'NONE',  ( -4.483927247898782831, 16.52544592524335698, 87.70942372801901854 ) ) ;
#36425=CARTESIAN_POINT ( 'NONE',  ( -19.03943276465977164, -0.05219959533935918106, 103.7510903946856757 ) ) ;
#36426=CARTESIAN_POINT ( 'NONE',  ( 13.97604488694527802, 13.89961937509977652, 74.37390960531436690 ) ) ;
#36427=CARTESIAN_POINT ( 'NONE',  ( 15.72974639402199770, -15.80617190586745480, 93.12390960531436690 ) ) ;
#36428=CARTESIAN_POINT ( 'NONE',  ( 8.314922557960818139, 14.29746914071049879, 99.58224293864770971 ) ) ;
#36429=CARTESIAN_POINT ( 'NONE',  ( 13.89961937509957401, 13.97604488694547697, 101.8760903946856331 ) ) ;
#36430=CARTESIAN_POINT ( 'NONE',  ( 14.29746914071037800, 8.314922557961029526, 76.66775706135234714 ) ) ;
#36431=CARTESIAN_POINT ( 'NONE',  ( -16.79531203550683216, 7.028104445595353411, 43.74755011779542002 ) ) ;
#36432=CARTESIAN_POINT ( 'NONE',  ( -0.05219959533936034679, 19.03943276465977164, 72.50109039468566152 ) ) ;
#36433=CARTESIAN_POINT ( 'NONE',  ( 16.53943276465976808, -0.05219959533910856209, 43.74890960531435979 ) ) ;
#36434=CARTESIAN_POINT ( 'NONE',  ( -12.14591786802309592, -12.06949235617757132, 96.87390960531436690 ) ) ;
#36435=CARTESIAN_POINT ( 'NONE',  ( 13.97604488694548053, -13.89961937509957401, 40.62609039468564731 ) ) ;
#36436=CARTESIAN_POINT ( 'NONE',  ( -16.62475595723701005, 7.163666690055240593, 90.52713351810474762 ) ) ;
#36437=CARTESIAN_POINT ( 'NONE',  ( -10.81492255796105439, 18.62759615963255655, 42.91775706135235424 ) ) ;
#36438=CARTESIAN_POINT ( 'NONE',  ( 9.474510206698729675, 16.51473224551082808, 102.0844237280190043 ) ) ;
#36439=CARTESIAN_POINT ( 'NONE',  ( 19.05341960407611168, 5.049401038298154454, 113.9572429386477097 ) ) ;
#36440=CARTESIAN_POINT ( 'NONE',  ( 9.564922557960805705, 16.46253265017160317, 89.58224293864769550 ) ) ;
#36441=CARTESIAN_POINT ( 'NONE',  ( -18.67979575497193778, 10.72451020669871902, 108.3344237280190185 ) ) ;
#36442=CARTESIAN_POINT ( 'NONE',  ( -19.02544592524342804, 5.153800228976336051, 91.04057627198100988 ) ) ;
#36443=CARTESIAN_POINT ( 'NONE',  ( 10.81492255796078972, 18.62759615963270932, 39.58224293864769550 ) ) ;
#36444=CARTESIAN_POINT ( 'NONE',  ( 8.224510206698953496, -14.34966873604960469, 92.91557627198103830 ) ) ;
#36445=CARTESIAN_POINT ( 'NONE',  ( 13.89961937509977652, -13.97604488694527269, 58.12390960531436690 ) ) ;
#36446=CARTESIAN_POINT ( 'NONE',  ( 12.14591786802309770, 12.06949235617756955, 109.3739096053143811 ) ) ;
#36447=CARTESIAN_POINT ( 'NONE',  ( -18.62759615963255300, -10.81492255796106328, 24.16775706135235424 ) ) ;
#36448=CARTESIAN_POINT ( 'NONE',  ( 0.05219959533937995610, -21.53943276465977519, 75.00109039468568994 ) ) ;
#36449=CARTESIAN_POINT ( 'NONE',  ( 0.05219959533909260263, 19.03943276465977164, 39.99890960531436690 ) ) ;
#36450=CARTESIAN_POINT ( 'NONE',  ( -12.14591786802326823, 12.06949235617739902, 73.12609039468567573 ) ) ;
#36451=CARTESIAN_POINT ( 'NONE',  ( -18.67979575497178146, -10.72451020669898902, 111.6655762719810525 ) ) ;
#36452=CARTESIAN_POINT ( 'NONE',  ( -21.53943276465977519, -0.05219959533937600094, 23.75109039468567929 ) ) ;
#36453=CARTESIAN_POINT ( 'NONE',  ( -13.89961937509957401, -13.97604488694547875, 59.37609039468566863 ) ) ;
#36454=CARTESIAN_POINT ( 'NONE',  ( -16.46253265017160317, 9.564922557960807481, 70.83224293864770971 ) ) ;
#36455=CARTESIAN_POINT ( 'NONE',  ( -13.97604488694547697, 13.89961937509957934, 33.12609039468566863 ) ) ;
#36456=CARTESIAN_POINT ( 'NONE',  ( 21.55341960407619695, -5.719274019375665929, 66.04275706135236135 ) ) ;
#36457=ADVANCED_FACE ( 'NONE', ( #9352 ), #29280, .T. ) ;
#36458=CARTESIAN_POINT ( 'NONE',  ( -0.05219959533907301413, -21.53943276465977519, 67.49890960531436690 ) ) ;
#36459=CARTESIAN_POINT ( 'NONE',  ( 16.53943276465976808, -0.05219959533910856209, 48.74890960531435979 ) ) ;
#36460=CARTESIAN_POINT ( 'NONE',  ( -18.62759615963255300, -10.81492255796106328, 94.16775706135237556 ) ) ;
#36461=CARTESIAN_POINT ( 'NONE',  ( -5.153800228976607833, 19.02544592524334988, 22.70942372801899012 ) ) ;
#36462=CARTESIAN_POINT ( 'NONE',  ( -12.06949235617756955, 12.14591786802309770, 70.62390960531436690 ) ) ;
#36463=CARTESIAN_POINT ( 'NONE',  ( 13.97604488694527802, 13.89961937509977652, 24.37390960531435624 ) ) ;
#36464=CARTESIAN_POINT ( 'NONE',  ( -19.02544592524334988, -5.153800228976617603, 63.95942372801899012 ) ) ;
#36465=CARTESIAN_POINT ( 'NONE',  ( 0.05219959533910956823, 16.53943276465976808, 24.99890960531435624 ) ) ;
#36466=CARTESIAN_POINT ( 'NONE',  ( 21.55341960407619695, -5.719274019375665929, 81.04275706135236135 ) ) ;
#36467=CARTESIAN_POINT ( 'NONE',  ( -19.05341960407611168, -5.049401038298163336, 76.45724293864769550 ) ) ;
#36468=CARTESIAN_POINT ( 'NONE',  ( -9.474510206698720793, -16.51473224551083518, 49.58442372801899722 ) ) ;
#36469=CARTESIAN_POINT ( 'NONE',  ( -10.72451020669898014, 18.67979575497178502, 45.41557627198103830 ) ) ;
#36470=CARTESIAN_POINT ( 'NONE',  ( -10.81492255796105439, 18.62759615963255655, 42.91775706135235424 ) ) ;
#36471=CARTESIAN_POINT ( 'NONE',  ( 15.80617190586746368, 15.72974639402197994, 99.37390960531436690 ) ) ;
#36472=CARTESIAN_POINT ( 'NONE',  ( -9.474510206698720793, -16.51473224551083518, 99.58442372801900433 ) ) ;
#36473=CARTESIAN_POINT ( 'NONE',  ( 8.314922557961029526, -14.29746914071037800, 70.41775706135236135 ) ) ;
#36475=CARTESIAN_POINT ( 'NONE',  ( 21.52544592524344225, -5.823673210054117533, 113.5405762719810383 ) ) ;
#36476=CARTESIAN_POINT ( 'NONE',  ( 12.14591786802309770, 12.06949235617756955, 84.37390960531438111 ) ) ;
#36477=CARTESIAN_POINT ( 'NONE',  ( -17.31728774477272736, -6.344390552232389346, 99.18093348310682700 ) ) ;
#36478=CARTESIAN_POINT ( 'NONE',  ( -8.224510206698735004, -14.34966873604973081, 29.58442372801901854 ) ) ;
#36479=APPLICATION_CONTEXT ( 'automotive_design' ) ;
#36480=CARTESIAN_POINT ( 'NONE',  ( 18.62759615963271287, -10.81492255796078972, 58.33224293864768839 ) ) ;
#36481=CARTESIAN_POINT ( 'NONE',  ( -4.379528057220086978, -16.55341960407618274, 89.79275706135236135 ) ) ;
#36482=CARTESIAN_POINT ( 'NONE',  ( -16.51473224551069308, -9.474510206698971260, 26.66557627198103120 ) ) ;
#36483=CARTESIAN_POINT ( 'NONE',  ( 16.52544592524335698, 4.483927247898782831, 71.45942372801901854 ) ) ;
#36484=CARTESIAN_POINT ( 'NONE',  ( 10.72451020669871369, 18.67979575497193778, 42.08442372801901854 ) ) ;
#36485=CARTESIAN_POINT ( 'NONE',  ( 10.72451020669898902, -18.67979575497178502, 62.91557627198102409 ) ) ;
#36486=CARTESIAN_POINT ( 'NONE',  ( 8.314922557961029526, -14.29746914071037800, 90.41775706135236135 ) ) ;
#36487=CARTESIAN_POINT ( 'NONE',  ( 18.67979575497194134, -10.72451020669871369, 65.83442372801900433 ) ) ;
#36488=CARTESIAN_POINT ( 'NONE',  ( -5.823673210054116645, -21.52544592524344225, 52.29057627198102409 ) ) ;
#36489=CARTESIAN_POINT ( 'NONE',  ( 21.52544592524344225, -5.823673210054117533, 38.54057627198103120 ) ) ;
#36492=CARTESIAN_POINT ( 'NONE',  ( -4.483927247898782831, 16.52544592524335698, 62.70942372801902565 ) ) ;
#36493=CARTESIAN_POINT ( 'NONE',  ( -21.53943276465977519, 0.05219959533907696930, 26.24890960531435624 ) ) ;
#36495=CARTESIAN_POINT ( 'NONE',  ( -5.049401038298153566, 19.05341960407611168, 100.2072429386476955 ) ) ;
#36496=CARTESIAN_POINT ( 'NONE',  ( -4.379528057220328563, 16.55341960407611168, 25.20724293864769550 ) ) ;
#36497=CARTESIAN_POINT ( 'NONE',  ( -17.60691670004652210, -5.499999999999993783, 79.13333313366442212 ) ) ;
#36498=CARTESIAN_POINT ( 'NONE',  ( 16.52544592524342804, -4.483927247898539470, 113.5405762719810383 ) ) ;
#36499=CARTESIAN_POINT ( 'NONE',  ( 21.52544592524344225, -5.823673210054117533, 58.54057627198103120 ) ) ;
#36500=CARTESIAN_POINT ( 'NONE',  ( -0.05219959533909027116, -19.03943276465977164, 47.49890960531435979 ) ) ;
#36501=CARTESIAN_POINT ( 'NONE',  ( 12.06949235617739724, 12.14591786802326823, 91.87609039468568994 ) ) ;
#36502=CARTESIAN_POINT ( 'NONE',  ( 0.05219959533937995610, -21.53943276465977519, 30.00109039468568284 ) ) ;
#36503=CARTESIAN_POINT ( 'NONE',  ( 19.02544592524334988, 5.153800228976608722, 106.4594237280190185 ) ) ;
#36504=CARTESIAN_POINT ( 'NONE',  ( 16.53943276465976808, -0.05219959533910856209, 103.7489096053143669 ) ) ;
#36505=CARTESIAN_POINT ( 'NONE',  ( -16.46253265017160317, 9.564922557960807481, 50.83224293864770260 ) ) ;
#36506=CARTESIAN_POINT ( 'NONE',  ( -16.46253265017160317, 9.564922557960807481, 25.83224293864769194 ) ) ;
#36507=CARTESIAN_POINT ( 'NONE',  ( 17.60728821186571835, -5.499999999999883649, 63.36690927743005375 ) ) ;
#36508=CARTESIAN_POINT ( 'NONE',  ( 0.05219959533909260263, 19.03943276465977164, 94.99890960531436690 ) ) ;
#36509=CARTESIAN_POINT ( 'NONE',  ( 14.34966873604972726, -8.224510206698740333, 70.83442372801901854 ) ) ;
#36510=CARTESIAN_POINT ( 'NONE',  ( -5.823673210054431948, 21.52544592524334988, 112.7094237280190328 ) ) ;
#36511=CARTESIAN_POINT ( 'NONE',  ( -0.05219959533907301413, -21.53943276465977519, 52.49890960531435979 ) ) ;
#36512=CARTESIAN_POINT ( 'NONE',  ( -16.55341960407617563, 4.379528057220093196, 78.54275706135236135 ) ) ;
#36513=CARTESIAN_POINT ( 'NONE',  ( 0.05219959533936267826, -19.03943276465977164, 70.00109039468566152 ) ) ;
#36514=CARTESIAN_POINT ( 'NONE',  ( 5.049401038298161559, -19.05341960407611168, 32.70724293864768129 ) ) ;
#36515=CARTESIAN_POINT ( 'NONE',  ( 19.02544592524343514, -5.153800228976328945, 73.54057627198103830 ) ) ;
#36516=CARTESIAN_POINT ( 'NONE',  ( 19.03943276465977164, -0.05219959533909143690, 38.74890960531436690 ) ) ;
#36517=CARTESIAN_POINT ( 'NONE',  ( -13.89961937509957401, -13.97604488694547875, 79.37609039468567573 ) ) ;
#36518=CARTESIAN_POINT ( 'NONE',  ( -19.05341960407611168, -5.049401038298163336, 111.4572429386476671 ) ) ;
#36519=CARTESIAN_POINT ( 'NONE',  ( -9.564922557960796823, -16.46253265017161027, 92.08224293864769550 ) ) ;
#36520=CARTESIAN_POINT ( 'NONE',  ( -16.55341960407611168, -4.379528057220339221, 46.45724293864769550 ) ) ;
#36521=CARTESIAN_POINT ( 'NONE',  ( 15.72974639402199770, -15.80617190586745480, 53.12390960531436690 ) ) ;
#36522=CARTESIAN_POINT ( 'NONE',  ( -17.49999999999999645, 3.850315288878824571, 104.2662913060345176 ) ) ;
#36524=CARTESIAN_POINT ( 'NONE',  ( 5.153800228976615827, -19.02544592524334988, 25.20942372801900433 ) ) ;
#36525=CARTESIAN_POINT ( 'NONE',  ( -17.31728774477274513, -6.344390552232368030, 79.18093348310681279 ) ) ;
#36526=CARTESIAN_POINT ( 'NONE',  ( -16.46253265017160317, 9.564922557960807481, 55.83224293864769550 ) ) ;
#36527=CARTESIAN_POINT ( 'NONE',  ( 12.06949235617739724, 12.14591786802326823, 31.87609039468567929 ) ) ;
#36528=CARTESIAN_POINT ( 'NONE',  ( -19.53091890409951858, -5.499999999999989342, 100.0609743183141802 ) ) ;
#36530=CARTESIAN_POINT ( 'NONE',  ( 16.53943276465976808, 0.05219959533934440121, 76.25109039468568994 ) ) ;
#36531=CARTESIAN_POINT ( 'NONE',  ( -5.719274019375978568, 21.55341960407610458, 95.20724293864769550 ) ) ;
#36532=CARTESIAN_POINT ( 'NONE',  ( 9.564922557960805705, 16.46253265017160317, 39.58224293864768839 ) ) ;
#36533=CARTESIAN_POINT ( 'NONE',  ( 18.67979575497194134, -10.72451020669871369, 45.83442372801901854 ) ) ;
#36534=CARTESIAN_POINT ( 'NONE',  ( -0.05219959533936034679, 19.03943276465977164, 52.50109039468566863 ) ) ;
#36535=CARTESIAN_POINT ( 'NONE',  ( -0.05219959533909027116, -19.03943276465977164, 47.49890960531435979 ) ) ;
#36536=CARTESIAN_POINT ( 'NONE',  ( -5.823673210054431948, 21.52544592524334988, 92.70942372801901854 ) ) ;
#36537=CARTESIAN_POINT ( 'NONE',  ( 17.13100169013300444, 6.664070546373151771, 96.73210164300149927 ) ) ;
#36538=CARTESIAN_POINT ( 'NONE',  ( 12.06949235617757843, -12.14591786802309237, 43.12390960531435269 ) ) ;
#36540=CARTESIAN_POINT ( 'NONE',  ( -5.719274019375978568, 21.55341960407610458, 50.20724293864769550 ) ) ;
#36542=CARTESIAN_POINT ( 'NONE',  ( -19.05341960407611168, -5.049401038298163336, 101.4572429386476955 ) ) ;
#36543=CARTESIAN_POINT ( 'NONE',  ( 16.52544592524342804, -4.483927247898539470, 98.54057627198105251 ) ) ;
#36544=CARTESIAN_POINT ( 'NONE',  ( 16.53943276465976808, 0.05219959533934440121, 26.25109039468567573 ) ) ;
#36545=CARTESIAN_POINT ( 'NONE',  ( -4.379528057220086978, -16.55341960407618274, 104.7927570613523898 ) ) ;
#36548=CARTESIAN_POINT ( 'NONE',  ( 9.474510206698971260, -16.51473224551069308, 102.9155762719810241 ) ) ;
#36549=CARTESIAN_POINT ( 'NONE',  ( 15.80617190586746368, 15.72974639402197994, 104.3739096053143669 ) ) ;
#36551=CARTESIAN_POINT ( 'NONE',  ( 16.53943276465976808, -0.05219959533910856209, 23.74890960531435269 ) ) ;
#36552=CARTESIAN_POINT ( 'NONE',  ( -9.564922557960796823, -16.46253265017161027, 102.0822429386477097 ) ) ;
#36553=CARTESIAN_POINT ( 'NONE',  ( -19.02544592524334988, -5.153800228976617603, 98.95942372801900433 ) ) ;
#36554=CARTESIAN_POINT ( 'NONE',  ( -10.72451020669870658, -18.67979575497194134, 109.5844237280190328 ) ) ;
#36555=CARTESIAN_POINT ( 'NONE',  ( 10.72451020669898902, -18.67979575497178502, 92.91557627198103830 ) ) ;
#36556=CARTESIAN_POINT ( 'NONE',  ( 15.72974639402199770, -15.80617190586745480, 53.12390960531436690 ) ) ;
#36557=CARTESIAN_POINT ( 'NONE',  ( 19.02544592524343514, -5.153800228976328945, 58.54057627198102409 ) ) ;
#36558=CARTESIAN_POINT ( 'NONE',  ( -4.379528057220328563, 16.55341960407611168, 30.20724293864769550 ) ) ;
#36559=CARTESIAN_POINT ( 'NONE',  ( -19.05341960407611168, -5.049401038298163336, 81.45724293864769550 ) ) ;
#36561=CARTESIAN_POINT ( 'NONE',  ( 19.49149378614661288, -5.499999999999589662, 61.93757513605363130 ) ) ;
#36562=CARTESIAN_POINT ( 'NONE',  ( 5.153800228976615827, -19.02544592524334988, 40.20942372801898301 ) ) ;
#36563=CARTESIAN_POINT ( 'NONE',  ( 10.81492255796078972, 18.62759615963270932, 79.58224293864769550 ) ) ;
#36564=CARTESIAN_POINT ( 'NONE',  ( 14.34966873604960469, 8.224510206698951720, 84.16557627198103830 ) ) ;
#36565=CARTESIAN_POINT ( 'NONE',  ( -5.719274019375665041, -21.55341960407619695, 34.79275706135235424 ) ) ;
#36567=CARTESIAN_POINT ( 'NONE',  ( 16.53943276465976808, 0.05219959533934440121, 106.2510903946856757 ) ) ;
#36568=CARTESIAN_POINT ( 'NONE',  ( -13.97604488694527625, -13.89961937509977652, 21.87390960531435979 ) ) ;
#36569=CARTESIAN_POINT ( 'NONE',  ( 5.049401038298161559, -19.05341960407611168, 92.70724293864769550 ) ) ;
#36570=CARTESIAN_POINT ( 'NONE',  ( 9.474510206698971260, -16.51473224551069308, 22.91557627198102765 ) ) ;
#36571=CARTESIAN_POINT ( 'NONE',  ( -0.05219959533910754901, -16.53943276465976808, 47.49890960531435979 ) ) ;
#36573=CARTESIAN_POINT ( 'NONE',  ( 0.05219959533937995610, -21.53943276465977519, 65.00109039468568994 ) ) ;
#36575=CARTESIAN_POINT ( 'NONE',  ( 9.564922557960805705, 16.46253265017160317, 49.58224293864770260 ) ) ;
#36576=CARTESIAN_POINT ( 'NONE',  ( 16.46253265017160672, -9.564922557960803928, 58.33224293864769550 ) ) ;
#36577=ORIENTED_EDGE ( 'NONE', *, *, #150310, .T. ) ;
#36578=CARTESIAN_POINT ( 'NONE',  ( -13.89961937509957401, -13.97604488694547875, 19.37609039468566507 ) ) ;
#36579=CARTESIAN_POINT ( 'NONE',  ( 16.55341960407618274, -4.379528057220086978, 66.04275706135236135 ) ) ;
#36580=CARTESIAN_POINT ( 'NONE',  ( -15.72974639402176322, -15.80617190586768395, 89.37609039468568994 ) ) ;
#36581=CARTESIAN_POINT ( 'NONE',  ( -21.55341960407610458, -5.719274019375992779, 21.45724293864769550 ) ) ;
#36582=CARTESIAN_POINT ( 'NONE',  ( 5.049401038297881783, 19.05341960407617563, 92.29275706135234714 ) ) ;
#36583=CARTESIAN_POINT ( 'NONE',  ( 5.823673210054444382, -21.52544592524334988, 75.20942372801901854 ) ) ;
#36584=CARTESIAN_POINT ( 'NONE',  ( 8.314922557961029526, -14.29746914071037800, 30.41775706135234358 ) ) ;
#36585=CARTESIAN_POINT ( 'NONE',  ( 18.67979575497178502, 10.72451020669898547, 84.16557627198103830 ) ) ;
#36586=CARTESIAN_POINT ( 'NONE',  ( 0.05219959533936267826, -19.03943276465977164, 95.00109039468567573 ) ) ;
#36587=CARTESIAN_POINT ( 'NONE',  ( -19.02544592524342804, 5.153800228976336051, 61.04057627198103120 ) ) ;
#36588=CARTESIAN_POINT ( 'NONE',  ( -13.97604488694547697, 13.89961937509957934, 113.1260903946856757 ) ) ;
#36589=CARTESIAN_POINT ( 'NONE',  ( -16.46253265017146816, -9.564922557961047289, 99.16775706135233293 ) ) ;
#36590=CARTESIAN_POINT ( 'NONE',  ( -4.483927247898539470, -16.52544592524342804, 47.29057627198103120 ) ) ;
#36591=CARTESIAN_POINT ( 'NONE',  ( 19.05341960407617918, -5.049401038297876454, 81.04275706135231871 ) ) ;
#36592=CARTESIAN_POINT ( 'NONE',  ( 12.14591786802327356, -12.06949235617739191, 55.62609039468568284 ) ) ;
#36593=CARTESIAN_POINT ( 'NONE',  ( -21.53943276465977519, 0.05219959533907696930, 116.2489096053143669 ) ) ;
#36594=CARTESIAN_POINT ( 'NONE',  ( 5.049401038298161559, -19.05341960407611168, 37.70724293864768839 ) ) ;
#36595=CARTESIAN_POINT ( 'NONE',  ( 9.564922557960805705, 16.46253265017160317, 54.58224293864769550 ) ) ;
#36596=CARTESIAN_POINT ( 'NONE',  ( 12.14591786802327356, -12.06949235617739191, 60.62609039468567573 ) ) ;
#36599=CARTESIAN_POINT ( 'NONE',  ( -16.46253265017160317, 9.564922557960807481, 100.8322429386477097 ) ) ;
#36602=CARTESIAN_POINT ( 'NONE',  ( -16.46253265017146816, -9.564922557961047289, 109.1677570613523471 ) ) ;
#36603=CARTESIAN_POINT ( 'NONE',  ( 10.81492255796078972, 18.62759615963270932, 44.58224293864769550 ) ) ;
#36604=CARTESIAN_POINT ( 'NONE',  ( -19.03943276465977164, -0.05219959533935918106, 43.75109039468566863 ) ) ;
#36605=CARTESIAN_POINT ( 'NONE',  ( -4.483927247898782831, 16.52544592524335698, 27.70942372801901854 ) ) ;
#36606=CARTESIAN_POINT ( 'NONE',  ( -19.03943276465977164, 0.05219959533909376836, 31.24890960531435979 ) ) ;
#36607=CARTESIAN_POINT ( 'NONE',  ( 9.474510206698971260, -16.51473224551069308, 52.91557627198102409 ) ) ;
#36608=CARTESIAN_POINT ( 'NONE',  ( -18.62759615963270932, 10.81492255796079327, 90.83224293864769550 ) ) ;
#36609=CARTESIAN_POINT ( 'NONE',  ( 9.474510206698971260, -16.51473224551069308, 112.9155762719810383 ) ) ;
#36611=CARTESIAN_POINT ( 'NONE',  ( 9.564922557960805705, 16.46253265017160317, 54.58224293864769550 ) ) ;
#36613=CARTESIAN_POINT ( 'NONE',  ( -16.46253265017146816, -9.564922557961047289, 79.16775706135234714 ) ) ;
#36614=CARTESIAN_POINT ( 'NONE',  ( -16.53943276465976808, 0.05219959533911058130, 61.24890960531435979 ) ) ;
#36615=CARTESIAN_POINT ( 'NONE',  ( 18.62759615963255655, 10.81492255796105972, 101.6677570613523613 ) ) ;
#36616=CARTESIAN_POINT ( 'NONE',  ( -18.67979575497178146, -10.72451020669898902, 91.66557627198103830 ) ) ;
#36617=CARTESIAN_POINT ( 'NONE',  ( 5.719274019375673035, 21.55341960407619339, 82.29275706135234714 ) ) ;
#36618=CARTESIAN_POINT ( 'NONE',  ( -16.46253265017160317, 9.564922557960807481, 30.83224293864769550 ) ) ;
#36619=CARTESIAN_POINT ( 'NONE',  ( 10.72451020669871369, 18.67979575497193778, 72.08442372801899012 ) ) ;
#36620=CARTESIAN_POINT ( 'NONE',  ( -9.474510206698964154, 16.51473224551069663, 110.4155762719810383 ) ) ;
#36621=CARTESIAN_POINT ( 'NONE',  ( -16.55341960407611168, -4.379528057220339221, 26.45724293864768839 ) ) ;
#36622=CARTESIAN_POINT ( 'NONE',  ( -10.81492255796105439, 18.62759615963255655, 82.91775706135234714 ) ) ;
#36623=CARTESIAN_POINT ( 'NONE',  ( 9.564922557960805705, 16.46253265017160317, 69.58224293864770971 ) ) ;
#36624=CARTESIAN_POINT ( 'NONE',  ( -15.72974639402176322, -15.80617190586768395, 44.37609039468567573 ) ) ;
#36625=CARTESIAN_POINT ( 'NONE',  ( -19.02544592524342804, 5.153800228976336051, 76.04057627198102409 ) ) ;
#36626=CARTESIAN_POINT ( 'NONE',  ( 8.224510206698953496, -14.34966873604960469, 87.91557627198103830 ) ) ;
#36627=CARTESIAN_POINT ( 'NONE',  ( 0.05219959533910956823, 16.53943276465976808, 59.99890960531436690 ) ) ;
#36628=CARTESIAN_POINT ( 'NONE',  ( 15.80617190586746368, 15.72974639402197994, 69.37390960531436690 ) ) ;
#36629=CARTESIAN_POINT ( 'NONE',  ( 0.05219959533909260263, 19.03943276465977164, 59.99890960531436690 ) ) ;
#36630=CARTESIAN_POINT ( 'NONE',  ( 0.05219959533907565091, 21.53943276465977519, 74.99890960531435269 ) ) ;
#36631=CARTESIAN_POINT ( 'NONE',  ( 16.46253265017146816, 9.564922557961045513, 66.66775706135233293 ) ) ;
#36632=CARTESIAN_POINT ( 'NONE',  ( 9.564922557961047289, -16.46253265017146816, 30.41775706135232937 ) ) ;
#36633=CARTESIAN_POINT ( 'NONE',  ( -8.224510206698948167, 14.34966873604960824, 75.41557627198102409 ) ) ;
#36634=CARTESIAN_POINT ( 'NONE',  ( 0.05219959533907565091, 21.53943276465977519, 54.99890960531435269 ) ) ;
#36636=CARTESIAN_POINT ( 'NONE',  ( -16.52544592524335698, -4.483927247898792601, 93.95942372801903275 ) ) ;
#36638=CARTESIAN_POINT ( 'NONE',  ( -9.564922557961040184, 16.46253265017147172, 107.9177570613523471 ) ) ;
#36639=CARTESIAN_POINT ( 'NONE',  ( 14.34966873604960469, 8.224510206698951720, 69.16557627198102409 ) ) ;
#36641=CARTESIAN_POINT ( 'NONE',  ( 9.474510206698971260, -16.51473224551069308, 62.91557627198102409 ) ) ;
#36642=CARTESIAN_POINT ( 'NONE',  ( 8.224510206698953496, -14.34966873604960469, 57.91557627198103120 ) ) ;
#36643=CARTESIAN_POINT ( 'NONE',  ( -19.03943276465977164, 0.05219959533909376836, 101.2489096053143669 ) ) ;
#36644=CARTESIAN_POINT ( 'NONE',  ( 16.46253265017146816, 9.564922557961045513, 71.66775706135233293 ) ) ;
#36645=CARTESIAN_POINT ( 'NONE',  ( 9.474510206698971260, -16.51473224551069308, 62.91557627198102409 ) ) ;
#36646=CARTESIAN_POINT ( 'NONE',  ( 13.97604488694527802, 13.89961937509977652, 89.37390960531436690 ) ) ;
#36647=CARTESIAN_POINT ( 'NONE',  ( 19.05341960407611168, 5.049401038298154454, 68.95724293864769550 ) ) ;
#36649=CARTESIAN_POINT ( 'NONE',  ( 18.67979575497178502, 10.72451020669898547, 64.16557627198102409 ) ) ;
#36650=CARTESIAN_POINT ( 'NONE',  ( 16.53943276465976808, 0.05219959533934440121, 61.25109039468567573 ) ) ;
#36651=CARTESIAN_POINT ( 'NONE',  ( -19.05341960407617918, 5.049401038297883559, 103.5427570613523329 ) ) ;
#36652=CARTESIAN_POINT ( 'NONE',  ( -5.153800228976328057, -19.02544592524343514, 47.29057627198102409 ) ) ;
#36653=CARTESIAN_POINT ( 'NONE',  ( -10.72451020669898014, 18.67979575497178502, 55.41557627198102409 ) ) ;
#36654=CARTESIAN_POINT ( 'NONE',  ( -0.05219959533936034679, 19.03943276465977164, 77.50109039468566152 ) ) ;
#36655=CARTESIAN_POINT ( 'NONE',  ( -16.55341960407617563, 4.379528057220093196, 113.5427570613523756 ) ) ;
#36656=CARTESIAN_POINT ( 'NONE',  ( 15.72974639402176855, 15.80617190586768217, 31.87609039468567929 ) ) ;
#36657=CARTESIAN_POINT ( 'NONE',  ( 19.05341960407617918, -5.049401038297876454, 36.04275706135234003 ) ) ;
#36658=CARTESIAN_POINT ( 'NONE',  ( -14.34966873604972548, 8.224510206698743886, 63.33442372801900433 ) ) ;
#36659=CARTESIAN_POINT ( 'NONE',  ( 4.379528057220092307, 16.55341960407617563, 87.29275706135236135 ) ) ;
#36660=CARTESIAN_POINT ( 'NONE',  ( 4.483927247898790824, -16.52544592524335698, 75.20942372801901854 ) ) ;
#36661=CARTESIAN_POINT ( 'NONE',  ( -21.53943276465977519, 0.05219959533907696930, 21.24890960531436690 ) ) ;
#36662=CARTESIAN_POINT ( 'NONE',  ( -14.29746914071037622, -8.314922557961029526, 39.16775706135235424 ) ) ;
#36663=CARTESIAN_POINT ( 'NONE',  ( 19.05341960407611168, 5.049401038298154454, 48.95724293864768129 ) ) ;
#36664=CARTESIAN_POINT ( 'NONE',  ( -9.474510206698964154, 16.51473224551069663, 45.41557627198103120 ) ) ;
#36665=CARTESIAN_POINT ( 'NONE',  ( -19.02544592524342804, 5.153800228976336051, 56.04057627198100988 ) ) ;
#36666=CARTESIAN_POINT ( 'NONE',  ( 18.67979575497194134, -10.72451020669871369, 45.83442372801901854 ) ) ;
#36667=CARTESIAN_POINT ( 'NONE',  ( -12.06949235617739369, -12.14591786802326823, 54.37609039468568994 ) ) ;
#36668=CARTESIAN_POINT ( 'NONE',  ( 12.14591786802327356, -12.06949235617739191, 110.6260903946857042 ) ) ;
#36669=CARTESIAN_POINT ( 'NONE',  ( -13.89961937509977652, 13.97604488694528158, 25.62390960531434558 ) ) ;
#36670=CARTESIAN_POINT ( 'NONE',  ( 5.823673210054444382, -21.52544592524334988, 110.2094237280190185 ) ) ;
#36671=CARTESIAN_POINT ( 'NONE',  ( -19.03943276465977164, -0.05219959533935918106, 103.7510903946856757 ) ) ;
#36672=CARTESIAN_POINT ( 'NONE',  ( -9.564922557961040184, 16.46253265017147172, 62.91775706135233293 ) ) ;
#36673=CARTESIAN_POINT ( 'NONE',  ( 16.53943276465976808, -0.05219959533910856209, 68.74890960531435269 ) ) ;
#36674=CARTESIAN_POINT ( 'NONE',  ( -5.153800228976328057, -19.02544592524343514, 32.29057627198102409 ) ) ;
#36675=CARTESIAN_POINT ( 'NONE',  ( 13.89961937509957401, 13.97604488694547697, 76.87609039468566152 ) ) ;
#36676=CARTESIAN_POINT ( 'NONE',  ( 17.13100169013299734, -6.664070546373147330, 93.26789835699847231 ) ) ;
#36677=CARTESIAN_POINT ( 'NONE',  ( -0.05219959533937732626, 21.53943276465977519, 77.50109039468567573 ) ) ;
#36678=CARTESIAN_POINT ( 'NONE',  ( 4.483927247898790824, -16.52544592524335698, 40.20942372801901854 ) ) ;
#36679=CARTESIAN_POINT ( 'NONE',  ( -18.09805431107250229, 5.499999999999981348, 91.01606229291887473 ) ) ;
#36680=CARTESIAN_POINT ( 'NONE',  ( -18.62759615963270932, 10.81492255796079327, 35.83224293864768839 ) ) ;
#36681=CARTESIAN_POINT ( 'NONE',  ( -12.14591786802326823, 12.06949235617739902, 33.12609039468569705 ) ) ;
#36682=CARTESIAN_POINT ( 'NONE',  ( 0.05219959533909260263, 19.03943276465977164, 29.99890960531435979 ) ) ;
#36683=CARTESIAN_POINT ( 'NONE',  ( 10.81492255796106328, -18.62759615963255655, 110.4177570613523756 ) ) ;
#36685=CARTESIAN_POINT ( 'NONE',  ( -5.153800228976328057, -19.02544592524343514, 32.29057627198102409 ) ) ;
#36687=CARTESIAN_POINT ( 'NONE',  ( 9.474510206698971260, -16.51473224551069308, 62.91557627198102409 ) ) ;
#36688=CARTESIAN_POINT ( 'NONE',  ( 10.81492255796106328, -18.62759615963255655, 70.41775706135236135 ) ) ;
#36689=CARTESIAN_POINT ( 'NONE',  ( -19.02544592524334988, -5.153800228976617603, 18.95942372801899722 ) ) ;
#36690=CARTESIAN_POINT ( 'NONE',  ( -8.224510206698948167, 14.34966873604960824, 30.41557627198101699 ) ) ;
#36691=CARTESIAN_POINT ( 'NONE',  ( -19.02544592524342804, 5.153800228976336051, 26.04057627198103120 ) ) ;
#36692=CARTESIAN_POINT ( 'NONE',  ( 5.049401038298161559, -19.05341960407611168, 92.70724293864769550 ) ) ;
#36693=CARTESIAN_POINT ( 'NONE',  ( -18.67979575497193778, 10.72451020669871902, 63.33442372801900433 ) ) ;
#36694=CARTESIAN_POINT ( 'NONE',  ( -19.03943276465977164, 0.05219959533909376836, 31.24890960531435979 ) ) ;
#36695=CARTESIAN_POINT ( 'NONE',  ( -18.67979575497193778, 10.72451020669871902, 68.33442372801900433 ) ) ;
#36696=CARTESIAN_POINT ( 'NONE',  ( -5.153800228976607833, 19.02544592524334988, 92.70942372801901854 ) ) ;
#36697=CARTESIAN_POINT ( 'NONE',  ( -16.51473224551069308, -9.474510206698971260, 101.6655762719810241 ) ) ;
#36698=CARTESIAN_POINT ( 'NONE',  ( -19.03943276465977164, 0.05219959533909376836, 36.24890960531436690 ) ) ;
#36699=CARTESIAN_POINT ( 'NONE',  ( 21.55341960407610458, 5.719274019375980345, 113.9572429386477239 ) ) ;
#36700=CARTESIAN_POINT ( 'NONE',  ( 19.02544592524334988, 5.153800228976608722, 41.45942372801900433 ) ) ;
#36701=CARTESIAN_POINT ( 'NONE',  ( -16.51473224551069308, -9.474510206698971260, 21.66557627198102765 ) ) ;
#36702=CARTESIAN_POINT ( 'NONE',  ( -5.049401038298153566, 19.05341960407611168, 60.20724293864768129 ) ) ;
#36703=CARTESIAN_POINT ( 'NONE',  ( -9.564922557961040184, 16.46253265017147172, 102.9177570613523329 ) ) ;
#36704=CARTESIAN_POINT ( 'NONE',  ( 4.379528057220339221, -16.55341960407611168, 77.70724293864770971 ) ) ;
#36705=CARTESIAN_POINT ( 'NONE',  ( -21.52544592524343514, 5.823673210054127303, 26.04057627198103475 ) ) ;
#36706=CARTESIAN_POINT ( 'NONE',  ( -13.89961937509957401, -13.97604488694547875, 89.37609039468563310 ) ) ;
#36707=CARTESIAN_POINT ( 'NONE',  ( 18.67979575497178502, 10.72451020669898547, 89.16557627198102409 ) ) ;
#36708=CARTESIAN_POINT ( 'NONE',  ( 15.72974639402176855, 15.80617190586768217, 46.87609039468568994 ) ) ;
#36709=CARTESIAN_POINT ( 'NONE',  ( -16.53943276465976808, -0.05219959533934237506, 43.75109039468568284 ) ) ;
#36710=CARTESIAN_POINT ( 'NONE',  ( 14.34966873604972726, -8.224510206698740333, 40.83442372801901854 ) ) ;
#36711=CARTESIAN_POINT ( 'NONE',  ( 18.67979575497194134, -10.72451020669871369, 50.83442372801901143 ) ) ;
#36712=CARTESIAN_POINT ( 'NONE',  ( 18.62759615963271287, -10.81492255796078972, 58.33224293864768839 ) ) ;
#36713=CARTESIAN_POINT ( 'NONE',  ( 5.049401038298161559, -19.05341960407611168, 47.70724293864770260 ) ) ;
#36715=CARTESIAN_POINT ( 'NONE',  ( 16.53943276465976808, 0.05219959533934440121, 71.25109039468568994 ) ) ;
#36717=CARTESIAN_POINT ( 'NONE',  ( 10.72451020669898902, -18.67979575497178502, 107.9155762719810241 ) ) ;
#36718=CARTESIAN_POINT ( 'NONE',  ( -8.224510206698948167, 14.34966873604960824, 45.41557627198103830 ) ) ;
#36719=CARTESIAN_POINT ( 'NONE',  ( 4.379528057220092307, 16.55341960407617563, 67.29275706135234714 ) ) ;
#36720=CARTESIAN_POINT ( 'NONE',  ( 5.049401038297881783, 19.05341960407617563, 97.29275706135233293 ) ) ;
#36721=CARTESIAN_POINT ( 'NONE',  ( -10.72451020669898014, 18.67979575497178502, 95.41557627198102409 ) ) ;
#36722=CARTESIAN_POINT ( 'NONE',  ( -14.34966873604960291, -8.224510206698953496, 26.66557627198103475 ) ) ;
#36724=CARTESIAN_POINT ( 'NONE',  ( -12.14591786802326823, 12.06949235617739902, 73.12609039468567573 ) ) ;
#36726=CARTESIAN_POINT ( 'NONE',  ( 0.05219959533907565091, 21.53943276465977519, 79.99890960531435269 ) ) ;
#36727=CARTESIAN_POINT ( 'NONE',  ( 16.52544592524335698, 4.483927247898782831, 111.4594237280190328 ) ) ;
#36729=CARTESIAN_POINT ( 'NONE',  ( -17.49999999999998934, -5.624438216177603422, 54.18329655085358354 ) ) ;
#36730=CARTESIAN_POINT ( 'NONE',  ( 18.62759615963271287, -10.81492255796078972, 108.3322429386477097 ) ) ;
#36731=CARTESIAN_POINT ( 'NONE',  ( 21.52544592524344225, -5.823673210054117533, 108.5405762719810241 ) ) ;
#36732=CARTESIAN_POINT ( 'NONE',  ( -14.34966873604960291, -8.224510206698953496, 31.66557627198102054 ) ) ;
#36733=CARTESIAN_POINT ( 'NONE',  ( -8.314922557961024197, 14.29746914071037800, 42.91775706135235424 ) ) ;
#36734=CARTESIAN_POINT ( 'NONE',  ( 13.89961937509977652, -13.97604488694527269, 48.12390960531435979 ) ) ;
#36735=CARTESIAN_POINT ( 'NONE',  ( -5.049401038298153566, 19.05341960407611168, 65.20724293864765286 ) ) ;
#36737=CARTESIAN_POINT ( 'NONE',  ( -19.02544592524342804, 5.153800228976336051, 116.0405762719810383 ) ) ;
#36739=CARTESIAN_POINT ( 'NONE',  ( 13.97604488694548053, -13.89961937509957401, 110.6260903946856615 ) ) ;
#36740=CARTESIAN_POINT ( 'NONE',  ( -9.474510206698720793, -16.51473224551083518, 54.58442372801899722 ) ) ;
#36741=CARTESIAN_POINT ( 'NONE',  ( 5.823673210054125526, 21.52544592524343514, 84.79057627198102409 ) ) ;
#36742=CARTESIAN_POINT ( 'NONE',  ( -16.53943276465976808, 0.05219959533911058130, 26.24890960531435624 ) ) ;
#36743=CARTESIAN_POINT ( 'NONE',  ( 19.05341960407611168, 5.049401038298154454, 73.95724293864768129 ) ) ;
#36744=CARTESIAN_POINT ( 'NONE',  ( -5.719274019375978568, 21.55341960407610458, 40.20724293864769550 ) ) ;
#36745=CARTESIAN_POINT ( 'NONE',  ( -0.05219959533907301413, -21.53943276465977519, 77.49890960531433848 ) ) ;
#36746=CARTESIAN_POINT ( 'NONE',  ( 16.55341960407618274, -4.379528057220086978, 21.04275706135234714 ) ) ;
#36747=CARTESIAN_POINT ( 'NONE',  ( 15.72974639402199770, -15.80617190586745480, 23.12390960531436335 ) ) ;
#36748=CARTESIAN_POINT ( 'NONE',  ( 21.52544592524334988, 5.823673210054432836, 71.45942372801901854 ) ) ;
#36749=CARTESIAN_POINT ( 'NONE',  ( -13.89961937509977652, 13.97604488694528158, 75.62390960531438111 ) ) ;
#36750=CARTESIAN_POINT ( 'NONE',  ( -9.564922557960796823, -16.46253265017161027, 22.08224293864768839 ) ) ;
#36751=CARTESIAN_POINT ( 'NONE',  ( 16.51473224551069308, 9.474510206698969483, 64.16557627198102409 ) ) ;
#36752=CARTESIAN_POINT ( 'NONE',  ( 12.06949235617757843, -12.14591786802309237, 88.12390960531436690 ) ) ;
#36753=ORIENTED_EDGE ( 'NONE', *, *, #190985, .F. ) ;
#36754=CARTESIAN_POINT ( 'NONE',  ( -19.05341960407617563, 5.049401038297882671, 98.54275706135233293 ) ) ;
#36757=CARTESIAN_POINT ( 'NONE',  ( -5.153800228976328057, -19.02544592524343514, 67.29057627198102409 ) ) ;
#36758=CARTESIAN_POINT ( 'NONE',  ( 0.05219959533937995610, -21.53943276465977519, 80.00109039468568994 ) ) ;
#36759=CARTESIAN_POINT ( 'NONE',  ( -9.474510206698964154, 16.51473224551069663, 105.4155762719810383 ) ) ;
#36760=CARTESIAN_POINT ( 'NONE',  ( -12.06949235617739369, -12.14591786802326823, 84.37609039468570415 ) ) ;
#36761=CARTESIAN_POINT ( 'NONE',  ( -16.21995358207302118, -7.366697692864226710, 75.06448998487846325 ) ) ;
#36762=CARTESIAN_POINT ( 'NONE',  ( -16.51473224551082808, 9.474510206698731452, 63.33442372801900433 ) ) ;
#36763=CARTESIAN_POINT ( 'NONE',  ( 18.62759615963255655, 10.81492255796105972, 111.6677570613523613 ) ) ;
#36767=CARTESIAN_POINT ( 'NONE',  ( -8.314922557960811034, -14.29746914071050412, 22.08224293864769194 ) ) ;
#36769=CARTESIAN_POINT ( 'NONE',  ( 12.14591786802327356, -12.06949235617739191, 105.6260903946856899 ) ) ;
#36770=CARTESIAN_POINT ( 'NONE',  ( 16.79531203550646268, 7.028104445595625194, 68.75244988220443076 ) ) ;
#36771=CARTESIAN_POINT ( 'NONE',  ( -4.379528057220086978, -16.55341960407618274, 79.79275706135236135 ) ) ;
#36772=CARTESIAN_POINT ( 'NONE',  ( 15.80617190586769283, -15.72974639402175789, 80.62609039468567573 ) ) ;
#36773=CARTESIAN_POINT ( 'NONE',  ( -19.02544592524334988, -5.153800228976617603, 98.95942372801900433 ) ) ;
#36774=CARTESIAN_POINT ( 'NONE',  ( -5.823673210054431948, 21.52544592524334988, 67.70942372801901854 ) ) ;
#36775=CARTESIAN_POINT ( 'NONE',  ( -13.89961937509957401, -13.97604488694547875, 34.37609039468566863 ) ) ;
#36776=CARTESIAN_POINT ( 'NONE',  ( -19.02544592524342804, 5.153800228976336051, 76.04057627198102409 ) ) ;
#36777=CARTESIAN_POINT ( 'NONE',  ( 5.153800228976335163, 19.02544592524342804, 54.79057627198103120 ) ) ;
#36778=CARTESIAN_POINT ( 'NONE',  ( -5.719274019375978568, 21.55341960407610458, 95.20724293864769550 ) ) ;
#36781=CARTESIAN_POINT ( 'NONE',  ( 21.53943276465977519, -0.05219959533907433946, 53.74890960531437401 ) ) ;
#36782=CARTESIAN_POINT ( 'NONE',  ( -0.05219959533909027116, -19.03943276465977164, 52.49890960531436690 ) ) ;
#36783=CARTESIAN_POINT ( 'NONE',  ( -14.29746914071037622, -8.314922557961029526, 59.16775706135234714 ) ) ;
#36784=ORIENTED_EDGE ( 'NONE', *, *, #15442, .T. ) ;
#36785=CARTESIAN_POINT ( 'NONE',  ( -5.719274019375665041, -21.55341960407619695, 39.79275706135235424 ) ) ;
#36786=CARTESIAN_POINT ( 'NONE',  ( 8.314922557960818139, 14.29746914071049879, 64.58224293864769550 ) ) ;
#36788=CARTESIAN_POINT ( 'NONE',  ( 8.224510206698742110, 14.34966873604972548, 42.08442372801901854 ) ) ;
#36789=CARTESIAN_POINT ( 'NONE',  ( -12.14591786802309592, -12.06949235617757132, 106.8739096053143811 ) ) ;
#36790=CARTESIAN_POINT ( 'NONE',  ( -13.89961937509957401, -13.97604488694547875, 59.37609039468566863 ) ) ;
#36791=CARTESIAN_POINT ( 'NONE',  ( 0.05219959533910956823, 16.53943276465976808, 69.99890960531435269 ) ) ;
#36792=CARTESIAN_POINT ( 'NONE',  ( 10.72451020669871369, 18.67979575497193778, 37.08442372801901143 ) ) ;
#36794=CARTESIAN_POINT ( 'NONE',  ( 16.51473224551069308, 9.474510206698969483, 24.16557627198102765 ) ) ;
#36795=CARTESIAN_POINT ( 'NONE',  ( -18.62759615963270932, 10.81492255796079327, 95.83224293864770971 ) ) ;
#36796=CARTESIAN_POINT ( 'NONE',  ( 9.564922557960805705, 16.46253265017160317, 109.5822429386476955 ) ) ;
#36797=CARTESIAN_POINT ( 'NONE',  ( -12.06949235617756955, 12.14591786802309770, 80.62390960531438111 ) ) ;
#36800=CARTESIAN_POINT ( 'NONE',  ( -19.03943276465977164, -0.05219959533935918106, 78.75109039468567573 ) ) ;
#36801=CARTESIAN_POINT ( 'NONE',  ( -10.81492255796105439, 18.62759615963255655, 27.91775706135234358 ) ) ;
#36802=CARTESIAN_POINT ( 'NONE',  ( -5.153800228976328057, -19.02544592524343514, 67.29057627198102409 ) ) ;
#36803=CARTESIAN_POINT ( 'NONE',  ( 9.564922557961047289, -16.46253265017146816, 55.41775706135234003 ) ) ;
#36804=CARTESIAN_POINT ( 'NONE',  ( -13.97604488694527625, -13.89961937509977652, 31.87390960531435979 ) ) ;
#36805=CARTESIAN_POINT ( 'NONE',  ( 0.05219959533910956823, 16.53943276465976808, 59.99890960531436690 ) ) ;
#36806=CARTESIAN_POINT ( 'NONE',  ( -16.55341960407611168, -4.379528057220339221, 56.45724293864768839 ) ) ;
#36807=CARTESIAN_POINT ( 'NONE',  ( -16.51473224551069308, -9.474510206698971260, 56.66557627198103120 ) ) ;
#36808=CARTESIAN_POINT ( 'NONE',  ( 10.72451020669898902, -18.67979575497178502, 87.91557627198103830 ) ) ;
#36809=CARTESIAN_POINT ( 'NONE',  ( 13.89961937509977652, -13.97604488694527269, 63.12390960531435979 ) ) ;
#36810=CARTESIAN_POINT ( 'NONE',  ( 5.719274019375991003, -21.55341960407610458, 77.70724293864770971 ) ) ;
#36812=CARTESIAN_POINT ( 'NONE',  ( -10.72451020669870658, -18.67979575497194134, 99.58442372801900433 ) ) ;
#36813=CARTESIAN_POINT ( 'NONE',  ( -16.51473224551069308, -9.474510206698971260, 26.66557627198103120 ) ) ;
#36814=CARTESIAN_POINT ( 'NONE',  ( -16.53943276465976808, -0.05219959533934237506, 113.7510903946856757 ) ) ;
#36815=CARTESIAN_POINT ( 'NONE',  ( 0.05219959533910956823, 16.53943276465976808, 99.99890960531436690 ) ) ;
#36816=CARTESIAN_POINT ( 'NONE',  ( 19.05341960407617918, -5.049401038297876454, 96.04275706135231871 ) ) ;
#36818=CARTESIAN_POINT ( 'NONE',  ( -5.719274019375978568, 21.55341960407610458, 110.2072429386477239 ) ) ;
#36819=CARTESIAN_POINT ( 'NONE',  ( 5.049401038297881783, 19.05341960407617563, 57.29275706135231871 ) ) ;
#36820=CARTESIAN_POINT ( 'NONE',  ( 14.29746914071037800, 8.314922557961029526, 101.6677570613523613 ) ) ;
#36821=CARTESIAN_POINT ( 'NONE',  ( 19.02544592524334988, 5.153800228976608722, 41.45942372801900433 ) ) ;
#36822=CARTESIAN_POINT ( 'NONE',  ( -0.05219959533909027116, -19.03943276465977164, 107.4989096053143527 ) ) ;
#36823=CARTESIAN_POINT ( 'NONE',  ( 21.53943276465977519, -0.05219959533907433946, 58.74890960531436690 ) ) ;
#36824=CARTESIAN_POINT ( 'NONE',  ( -19.48894818550243357, 5.500000000000115463, 50.10307310435241845 ) ) ;
#36825=CARTESIAN_POINT ( 'NONE',  ( 9.564922557960805705, 16.46253265017160317, 39.58224293864768839 ) ) ;
#36826=CARTESIAN_POINT ( 'NONE',  ( 5.719274019375673035, 21.55341960407619339, 107.2927570613523471 ) ) ;
#36827=CARTESIAN_POINT ( 'NONE',  ( -14.34966873604972548, 8.224510206698743886, 78.33442372801901854 ) ) ;
#36828=CARTESIAN_POINT ( 'NONE',  ( 18.67979575497194134, -10.72451020669871369, 30.83442372801902209 ) ) ;
#36829=CARTESIAN_POINT ( 'NONE',  ( -12.14591786802326823, 12.06949235617739902, 48.12609039468568284 ) ) ;
#36830=CARTESIAN_POINT ( 'NONE',  ( 19.05341960407611168, 5.049401038298154454, 103.9572429386476671 ) ) ;
#36831=CARTESIAN_POINT ( 'NONE',  ( 19.02544592524343514, -5.153800228976328945, 48.54057627198103120 ) ) ;
#36832=CARTESIAN_POINT ( 'NONE',  ( 16.46253265017160672, -9.564922557960803928, 63.33224293864769550 ) ) ;
#36833=CARTESIAN_POINT ( 'NONE',  ( -16.52544592524335698, -4.483927247898792601, 48.95942372801902565 ) ) ;
#36834=CARTESIAN_POINT ( 'NONE',  ( 4.379528057220339221, -16.55341960407611168, 102.7072429386476955 ) ) ;
#36835=CARTESIAN_POINT ( 'NONE',  ( -12.14591786802326823, 12.06949235617739902, 108.1260903946856757 ) ) ;
#36837=CARTESIAN_POINT ( 'NONE',  ( -5.719274019375665041, -21.55341960407619695, 59.79275706135234714 ) ) ;
#36838=CARTESIAN_POINT ( 'NONE',  ( -0.05219959533909027116, -19.03943276465977164, 72.49890960531435269 ) ) ;
#36839=CARTESIAN_POINT ( 'NONE',  ( 16.51473224551069308, 9.474510206698969483, 64.16557627198102409 ) ) ;
#36840=CARTESIAN_POINT ( 'NONE',  ( -19.05341960407611168, -5.049401038298163336, 91.45724293864766707 ) ) ;
#36841=CARTESIAN_POINT ( 'NONE',  ( -0.05219959533910754901, -16.53943276465976808, 47.49890960531435979 ) ) ;
#36842=CARTESIAN_POINT ( 'NONE',  ( -8.314922557961024197, 14.29746914071037800, 112.9177570613523329 ) ) ;
#36844=CARTESIAN_POINT ( 'NONE',  ( 12.14591786802309770, 12.06949235617756955, 39.37390960531436690 ) ) ;
#36845=ORIENTED_EDGE ( 'NONE', *, *, #135302, .T. ) ;
#36847=CARTESIAN_POINT ( 'NONE',  ( -16.51473224551069308, -9.474510206698971260, 61.66557627198103120 ) ) ;
#36848=CARTESIAN_POINT ( 'NONE',  ( 9.474510206698729675, 16.51473224551082808, 37.08442372801899722 ) ) ;
#36851=CARTESIAN_POINT ( 'NONE',  ( 9.564922557961047289, -16.46253265017146816, 80.41775706135234714 ) ) ;
#36852=CARTESIAN_POINT ( 'NONE',  ( 12.06949235617739724, 12.14591786802326823, 66.87609039468568994 ) ) ;
#36854=CARTESIAN_POINT ( 'NONE',  ( 19.03943276465977164, -0.05219959533909143690, 93.74890960531435269 ) ) ;
#36855=CARTESIAN_POINT ( 'NONE',  ( 5.823673210054444382, -21.52544592524334988, 30.20942372801902565 ) ) ;
#36856=CARTESIAN_POINT ( 'NONE',  ( 16.46253265017146816, 9.564922557961045513, 71.66775706135233293 ) ) ;
#36857=CARTESIAN_POINT ( 'NONE',  ( 16.61371651742600619, 7.165104196376166357, 88.64584930007006847 ) ) ;
#36858=CARTESIAN_POINT ( 'NONE',  ( -16.51473224551069308, -9.474510206698971260, 46.66557627198102409 ) ) ;
#36859=CARTESIAN_POINT ( 'NONE',  ( 13.97604488694527802, 13.89961937509977652, 84.37390960531433848 ) ) ;
#36860=CARTESIAN_POINT ( 'NONE',  ( -8.224510206698948167, 14.34966873604960824, 50.41557627198103120 ) ) ;
#36861=CARTESIAN_POINT ( 'NONE',  ( 19.05341960407611168, 5.049401038298154454, 48.95724293864768129 ) ) ;
#36862=CARTESIAN_POINT ( 'NONE',  ( 5.049401038297881783, 19.05341960407617563, 47.29275706135231161 ) ) ;
#36864=CARTESIAN_POINT ( 'NONE',  ( -12.06949235617756955, 12.14591786802309770, 90.62390960531436690 ) ) ;
#36865=CARTESIAN_POINT ( 'NONE',  ( -13.89961937509957401, -13.97604488694547875, 29.37609039468565797 ) ) ;
#36866=CARTESIAN_POINT ( 'NONE',  ( -9.564922557960796823, -16.46253265017161027, 67.08224293864769550 ) ) ;
#36867=AXIS2_PLACEMENT_3D ( 'NONE', #95102, #156791, #30459 ) ;
#36868=CARTESIAN_POINT ( 'NONE',  ( -10.81492255796078084, -18.62759615963271287, 57.08224293864769550 ) ) ;
#36869=CARTESIAN_POINT ( 'NONE',  ( -16.53943276465976808, 0.05219959533911058130, 61.24890960531435979 ) ) ;
#36870=CARTESIAN_POINT ( 'NONE',  ( 5.049401038297881783, 19.05341960407617563, 27.29275706135232937 ) ) ;
#36871=CARTESIAN_POINT ( 'NONE',  ( 16.46253265017160672, -9.564922557960803928, 108.3322429386476955 ) ) ;
#36872=CARTESIAN_POINT ( 'NONE',  ( 15.80617190586746368, 15.72974639402197994, 29.37390960531435269 ) ) ;
#36873=CARTESIAN_POINT ( 'NONE',  ( 13.89961937509977652, -13.97604488694527269, 48.12390960531435979 ) ) ;
#36874=CARTESIAN_POINT ( 'NONE',  ( 5.049401038298161559, -19.05341960407611168, 42.70724293864767418 ) ) ;
#36875=CARTESIAN_POINT ( 'NONE',  ( 12.06949235617757843, -12.14591786802309237, 98.12390960531436690 ) ) ;
#36876=CARTESIAN_POINT ( 'NONE',  ( 21.55341960407610458, 5.719274019375980345, 108.9572429386476955 ) ) ;
#36877=CARTESIAN_POINT ( 'NONE',  ( -13.97604488694527625, -13.89961937509977652, 106.8739096053143669 ) ) ;
#36878=CARTESIAN_POINT ( 'NONE',  ( -0.05219959533937732626, 21.53943276465977519, 22.50109039468567573 ) ) ;
#36879=CARTESIAN_POINT ( 'NONE',  ( 9.474510206698971260, -16.51473224551069308, 107.9155762719810383 ) ) ;
#36880=CARTESIAN_POINT ( 'NONE',  ( 16.55341960407611168, 4.379528057220329451, 113.9572429386477239 ) ) ;
#36881=CARTESIAN_POINT ( 'NONE',  ( 5.823673210054444382, -21.52544592524334988, 85.20942372801901854 ) ) ;
#36882=CARTESIAN_POINT ( 'NONE',  ( -5.823673210054116645, -21.52544592524344225, 92.29057627198103830 ) ) ;
#36886=CARTESIAN_POINT ( 'NONE',  ( -12.06949235617739369, -12.14591786802326823, 49.37609039468569705 ) ) ;
#36887=CARTESIAN_POINT ( 'NONE',  ( -14.34966873604960291, -8.224510206698953496, 111.6655762719810525 ) ) ;
#36889=CARTESIAN_POINT ( 'NONE',  ( -17.50000000000002132, -4.049696124445859802, 110.8196032933405775 ) ) ;
#36890=CARTESIAN_POINT ( 'NONE',  ( 13.89961937509977652, -13.97604488694527269, 58.12390960531436690 ) ) ;
#36891=CARTESIAN_POINT ( 'NONE',  ( 0.05219959533910956823, 16.53943276465976808, 89.99890960531438111 ) ) ;
#36892=CARTESIAN_POINT ( 'NONE',  ( 5.719274019375991003, -21.55341960407610458, 47.70724293864770260 ) ) ;
#36893=CARTESIAN_POINT ( 'NONE',  ( 16.52544592524342804, -4.483927247898539470, 63.54057627198103830 ) ) ;
#36894=CARTESIAN_POINT ( 'NONE',  ( 12.06949235617739724, 12.14591786802326823, 26.87609039468567218 ) ) ;
#36895=CARTESIAN_POINT ( 'NONE',  ( 18.62759615963255655, 10.81492255796105972, 71.66775706135234714 ) ) ;
#36897=CARTESIAN_POINT ( 'NONE',  ( 17.26172910966779739, -6.454744622555850242, 78.30646908649222837 ) ) ;
#36898=CARTESIAN_POINT ( 'NONE',  ( 4.379528057220092307, 16.55341960407617563, 92.29275706135236135 ) ) ;
#36899=CARTESIAN_POINT ( 'NONE',  ( 12.14591786802309770, 12.06949235617756955, 44.37390960531435979 ) ) ;
#36900=CARTESIAN_POINT ( 'NONE',  ( 9.474510206698971260, -16.51473224551069308, 42.91557627198103120 ) ) ;
#36901=CARTESIAN_POINT ( 'NONE',  ( 9.474510206698971260, -16.51473224551069308, 92.91557627198103830 ) ) ;
#36902=CARTESIAN_POINT ( 'NONE',  ( 18.62759615963271287, -10.81492255796078972, 88.33224293864769550 ) ) ;
#36903=COLOUR_RGB ( '', 0.31764706, 0.68627451, 0.89019608) ;
#36904=CARTESIAN_POINT ( 'NONE',  ( -12.06949235617739369, -12.14591786802326823, 39.37609039468567573 ) ) ;
#36905=CARTESIAN_POINT ( 'NONE',  ( 14.34966873604960469, 8.224510206698951720, 64.16557627198102409 ) ) ;
#36906=CARTESIAN_POINT ( 'NONE',  ( -5.719274019375665041, -21.55341960407619695, 69.79275706135234714 ) ) ;
#36907=CARTESIAN_POINT ( 'NONE',  ( -14.29746914071037622, -8.314922557961029526, 104.1677570613523471 ) ) ;
#36909=DIRECTION ( 'NONE',  ( 1.000000000000000000, 0.000000000000000000, 0.000000000000000000 ) ) ;
#36910=CARTESIAN_POINT ( 'NONE',  ( 8.314922557960818139, 14.29746914071049879, 24.58224293864768839 ) ) ;
#36911=CARTESIAN_POINT ( 'NONE',  ( 8.314922557961029526, -14.29746914071037800, 75.41775706135233293 ) ) ;
#36912=CARTESIAN_POINT ( 'NONE',  ( 9.564922557960805705, 16.46253265017160317, 89.58224293864769550 ) ) ;
#36913=CARTESIAN_POINT ( 'NONE',  ( -19.02544592524342804, 5.153800228976336051, 101.0405762719810241 ) ) ;
#36914=CARTESIAN_POINT ( 'NONE',  ( 21.52544592524334988, 5.823673210054432836, 81.45942372801900433 ) ) ;
#36915=CARTESIAN_POINT ( 'NONE',  ( 8.314922557961029526, -14.29746914071037800, 85.41775706135236135 ) ) ;
#36916=CARTESIAN_POINT ( 'NONE',  ( -4.379528057220328563, 16.55341960407611168, 55.20724293864770260 ) ) ;
#36917=CARTESIAN_POINT ( 'NONE',  ( 5.153800228976335163, 19.02544592524342804, 74.79057627198103830 ) ) ;
#36919=CARTESIAN_POINT ( 'NONE',  ( -5.153800228976607833, 19.02544592524334988, 107.7094237280189759 ) ) ;
#36920=( BOUNDED_CURVE ( )  B_SPLINE_CURVE ( 2, ( #87042, #133544, #10215, #118390, #88031, #85026, #149719, #196250, #158139, #8203, #19631, #142955, #69878 ),
 .UNSPECIFIED., .F., .T. ) 
 B_SPLINE_CURVE_WITH_KNOTS ( ( 3, 2, 2, 2, 2, 2, 3 ),
 ( 0.3182199101112556661, 0.3201754385964912242, 0.3245614035087719396, 0.3289473684210526550, 0.3333333333333333148, 0.3377192982456140302, 0.3396291469087595050 ),
 .UNSPECIFIED. ) 
 CURVE ( )  GEOMETRIC_REPRESENTATION_ITEM ( )  RATIONAL_B_SPLINE_CURVE ( ( 0.9831626618144004848, 0.9848076720550091867, 1.000000000000000000, 0.9659258262890683122, 1.000000000000000000, 0.9659258262890683122, 1.000000000000000000, 0.9659258262890683122, 1.000000000000000000, 0.9659258262890683122, 1.000000000000000000, 0.9851625545550091179, 0.9832469066685282089 ) ) 
 REPRESENTATION_ITEM ( '' )  );
#36921=CARTESIAN_POINT ( 'NONE',  ( -8.314922557960811034, -14.29746914071050412, 112.0822429386477097 ) ) ;
#36922=CARTESIAN_POINT ( 'NONE',  ( -5.153800228976328057, -19.02544592524343514, 82.29057627198103830 ) ) ;
#36923=CARTESIAN_POINT ( 'NONE',  ( -12.06949235617739369, -12.14591786802326823, 24.37609039468567573 ) ) ;
#36925=CARTESIAN_POINT ( 'NONE',  ( 19.02544592524334988, 5.153800228976608722, 21.45942372801899012 ) ) ;
#36926=CARTESIAN_POINT ( 'NONE',  ( -16.52544592524335698, -4.483927247898792601, 83.95942372801900433 ) ) ;
#36927=CARTESIAN_POINT ( 'NONE',  ( -13.89961937509957401, -13.97604488694547875, 94.37609039468566152 ) ) ;
#36928=CARTESIAN_POINT ( 'NONE',  ( -16.53943276465976808, 0.05219959533911058130, 116.2489096053143669 ) ) ;
#36929=CARTESIAN_POINT ( 'NONE',  ( 14.29746914071037800, 8.314922557961029526, 66.66775706135234714 ) ) ;
#36930=CARTESIAN_POINT ( 'NONE',  ( -4.379528057220086978, -16.55341960407618274, 54.79275706135235424 ) ) ;
#36932=CARTESIAN_POINT ( 'NONE',  ( -19.03943276465977164, -0.05219959533935918106, 68.75109039468566152 ) ) ;
#36933=CARTESIAN_POINT ( 'NONE',  ( 18.62759615963255655, 10.81492255796105972, 96.66775706135234714 ) ) ;
#36934=CARTESIAN_POINT ( 'NONE',  ( -0.05219959533909027116, -19.03943276465977164, 37.49890960531436690 ) ) ;
#36935=CARTESIAN_POINT ( 'NONE',  ( 16.46253265017160672, -9.564922557960803928, 83.33224293864768129 ) ) ;
#36936=CARTESIAN_POINT ( 'NONE',  ( 12.06949235617757843, -12.14591786802309237, 78.12390960531436690 ) ) ;
#36938=CARTESIAN_POINT ( 'NONE',  ( 10.72451020669871369, 18.67979575497193778, 87.08442372801901854 ) ) ;
#36939=CARTESIAN_POINT ( 'NONE',  ( -9.564922557961040184, 16.46253265017147172, 37.91775706135233293 ) ) ;
#36940=CARTESIAN_POINT ( 'NONE',  ( 10.72451020669898902, -18.67979575497178502, 42.91557627198103120 ) ) ;
#36941=CARTESIAN_POINT ( 'NONE',  ( 15.80617190586769283, -15.72974639402175789, 110.6260903946857042 ) ) ;
#36942=CARTESIAN_POINT ( 'NONE',  ( 13.89961937509977652, -13.97604488694527269, 78.12390960531433848 ) ) ;
#36943=CARTESIAN_POINT ( 'NONE',  ( 15.80617190586769283, -15.72974639402175789, 110.6260903946857042 ) ) ;
#36944=CARTESIAN_POINT ( 'NONE',  ( -18.62759615963270932, 10.81492255796079327, 65.83224293864769550 ) ) ;
#36945=CARTESIAN_POINT ( 'NONE',  ( 9.564922557960805705, 16.46253265017160317, 99.58224293864770971 ) ) ;
#36946=CARTESIAN_POINT ( 'NONE',  ( 16.51473224551083163, -9.474510206698727899, 80.83442372801899012 ) ) ;
#36947=CARTESIAN_POINT ( 'NONE',  ( 5.049401038298161559, -19.05341960407611168, 107.7072429386476955 ) ) ;
#36948=CARTESIAN_POINT ( 'NONE',  ( -5.049401038297874678, -19.05341960407617918, 89.79275706135230450 ) ) ;
#36949=CARTESIAN_POINT ( 'NONE',  ( -0.05219959533934338120, 16.53943276465976808, 47.50109039468568994 ) ) ;
#36950=CARTESIAN_POINT ( 'NONE',  ( -16.52544592524342804, 4.483927247898546575, 116.0405762719810383 ) ) ;
#36951=CARTESIAN_POINT ( 'NONE',  ( 9.474510206698971260, -16.51473224551069308, 82.91557627198103830 ) ) ;
#36952=CARTESIAN_POINT ( 'NONE',  ( 5.719274019375991003, -21.55341960407610458, 57.70724293864770260 ) ) ;
#36953=CARTESIAN_POINT ( 'NONE',  ( -4.483927247898782831, 16.52544592524335698, 27.70942372801901854 ) ) ;
#36954=CARTESIAN_POINT ( 'NONE',  ( -18.67979575497193778, 10.72451020669871902, 28.33442372801902209 ) ) ;
#36955=CARTESIAN_POINT ( 'NONE',  ( 15.80617190586769283, -15.72974639402175789, 80.62609039468567573 ) ) ;
#36956=CARTESIAN_POINT ( 'NONE',  ( -16.52544592524335698, -4.483927247898792601, 88.95942372801901854 ) ) ;
#36957=CARTESIAN_POINT ( 'NONE',  ( 19.03943276465977164, -0.05219959533909143690, 88.74890960531436690 ) ) ;
#36958=CARTESIAN_POINT ( 'NONE',  ( 14.29746914071049879, -8.314922557960816363, 73.33224293864769550 ) ) ;
#36959=CARTESIAN_POINT ( 'NONE',  ( -4.483927247898782831, 16.52544592524335698, 112.7094237280190328 ) ) ;
#36960=CARTESIAN_POINT ( 'NONE',  ( 5.153800228976615827, -19.02544592524334988, 55.20942372801899722 ) ) ;
#36962=CARTESIAN_POINT ( 'NONE',  ( 5.823673210054444382, -21.52544592524334988, 45.20942372801901854 ) ) ;
#36963=CARTESIAN_POINT ( 'NONE',  ( -16.53943276465976808, 0.05219959533911058130, 96.24890960531435269 ) ) ;
#36964=CARTESIAN_POINT ( 'NONE',  ( -13.89961937509977652, 13.97604488694528158, 110.6239096053143243 ) ) ;
#36965=CARTESIAN_POINT ( 'NONE',  ( -16.52544592524335698, -4.483927247898792601, 98.95942372801903275 ) ) ;
#36966=CARTESIAN_POINT ( 'NONE',  ( 0.05219959533937995610, -21.53943276465977519, 90.00109039468567573 ) ) ;
#36967=CARTESIAN_POINT ( 'NONE',  ( 14.29746914071037800, 8.314922557961029526, 51.66775706135234714 ) ) ;
#36968=CARTESIAN_POINT ( 'NONE',  ( -0.05219959533937732626, 21.53943276465977519, 42.50109039468567573 ) ) ;
#36970=CARTESIAN_POINT ( 'NONE',  ( 5.823673210054444382, -21.52544592524334988, 20.20942372801900788 ) ) ;
#36971=CARTESIAN_POINT ( 'NONE',  ( 16.55341960407611168, 4.379528057220329451, 93.95724293864770971 ) ) ;
#36972=CARTESIAN_POINT ( 'NONE',  ( 17.50000000000001421, -3.209263204892543353, 27.26196825606273322 ) ) ;
#36973=CARTESIAN_POINT ( 'NONE',  ( 8.314922557960818139, 14.29746914071049879, 69.58224293864769550 ) ) ;
#36974=CARTESIAN_POINT ( 'NONE',  ( -12.06949235617739369, -12.14591786802326823, 99.37609039468568994 ) ) ;
#36975=CARTESIAN_POINT ( 'NONE',  ( 19.05341960407611168, 5.049401038298154454, 33.95724293864769550 ) ) ;
#36976=ADVANCED_FACE ( 'NONE', ( #144395 ), #145391, .F. ) ;
#36977=CARTESIAN_POINT ( 'NONE',  ( -21.55341960407610458, -5.719274019375992779, 46.45724293864769550 ) ) ;
#36978=CARTESIAN_POINT ( 'NONE',  ( 4.379528057220339221, -16.55341960407611168, 77.70724293864770971 ) ) ;
#36979=CARTESIAN_POINT ( 'NONE',  ( -5.719274019375978568, 21.55341960407610458, 75.20724293864769550 ) ) ;
#36980=CARTESIAN_POINT ( 'NONE',  ( -13.89961937509977652, 13.97604488694528158, 90.62390960531432427 ) ) ;
#36981=CARTESIAN_POINT ( 'NONE',  ( 5.049401038298161559, -19.05341960407611168, 32.70724293864768129 ) ) ;
#36982=CARTESIAN_POINT ( 'NONE',  ( -19.03943276465977164, -0.05219959533935918106, 93.75109039468566152 ) ) ;
#36983=CARTESIAN_POINT ( 'NONE',  ( -5.719274019375978568, 21.55341960407610458, 35.20724293864768839 ) ) ;
#36984=CARTESIAN_POINT ( 'NONE',  ( 10.72451020669871369, 18.67979575497193778, 57.08442372801901854 ) ) ;
#36985=CARTESIAN_POINT ( 'NONE',  ( 9.564922557960805705, 16.46253265017160317, 59.58224293864769550 ) ) ;
#36986=CARTESIAN_POINT ( 'NONE',  ( 19.02544592524343514, -5.153800228976328945, 83.54057627198100988 ) ) ;
#36988=CARTESIAN_POINT ( 'NONE',  ( -16.52544592524335698, -4.483927247898792601, 48.95942372801902565 ) ) ;
#36989=CARTESIAN_POINT ( 'NONE',  ( 0.05219959533937995610, -21.53943276465977519, 40.00109039468567573 ) ) ;
#36991=CARTESIAN_POINT ( 'NONE',  ( -10.81492255796105439, 18.62759615963255655, 77.91775706135231871 ) ) ;
#36992=CARTESIAN_POINT ( 'NONE',  ( 19.03943276465977164, -0.05219959533909143690, 113.7489096053143669 ) ) ;
#36993=CARTESIAN_POINT ( 'NONE',  ( 21.52544592524344225, -5.823673210054117533, 88.54057627198103830 ) ) ;
#36994=CARTESIAN_POINT ( 'NONE',  ( 10.81492255796106328, -18.62759615963255655, 30.41775706135234358 ) ) ;
#36995=CARTESIAN_POINT ( 'NONE',  ( -14.34966873604972548, 8.224510206698743886, 68.33442372801900433 ) ) ;
#36996=CARTESIAN_POINT ( 'NONE',  ( 5.719274019375991003, -21.55341960407610458, 62.70724293864769550 ) ) ;
#36997=CARTESIAN_POINT ( 'NONE',  ( -0.05219959533937732626, 21.53943276465977519, 112.5010903946857042 ) ) ;
#36998=CARTESIAN_POINT ( 'NONE',  ( -9.564922557960796823, -16.46253265017161027, 72.08224293864770971 ) ) ;
#36999=CARTESIAN_POINT ( 'NONE',  ( -14.29746914071037622, -8.314922557961029526, 99.16775706135234714 ) ) ;
#37000=CARTESIAN_POINT ( 'NONE',  ( -17.49999999999999645, -5.500000000000000888, 104.2030961746582847 ) ) ;
#37001=CARTESIAN_POINT ( 'NONE',  ( 19.05341960407611168, 5.049401038298154454, 83.95724293864766707 ) ) ;
#37002=CARTESIAN_POINT ( 'NONE',  ( 17.50000000000005329, 3.734851586428519887, 103.1808203866947480 ) ) ;
#37003=CARTESIAN_POINT ( 'NONE',  ( -19.05341960407617563, 5.049401038297882671, 78.54275706135233293 ) ) ;
#37004=CARTESIAN_POINT ( 'NONE',  ( 18.67979575497178502, 10.72451020669898547, 54.16557627198103120 ) ) ;
#37005=CARTESIAN_POINT ( 'NONE',  ( -16.55341960407611168, -4.379528057220339221, 21.45724293864769550 ) ) ;
#37006=CARTESIAN_POINT ( 'NONE',  ( 19.03943276465977164, 0.05219959533936151252, 101.2510903946856757 ) ) ;
#37007=CARTESIAN_POINT ( 'NONE',  ( 0.05219959533909260263, 19.03943276465977164, 39.99890960531436690 ) ) ;
#37008=CARTESIAN_POINT ( 'NONE',  ( -16.51473224551082808, 9.474510206698731452, 93.33442372801900433 ) ) ;
#37009=CARTESIAN_POINT ( 'NONE',  ( 15.80617190586746368, 15.72974639402197994, 89.37390960531435269 ) ) ;
#37010=CARTESIAN_POINT ( 'NONE',  ( -19.02544592524334988, -5.153800228976617603, 58.95942372801900433 ) ) ;
#37012=CARTESIAN_POINT ( 'NONE',  ( 0.05219959533909260263, 19.03943276465977164, 49.99890960531435979 ) ) ;
#37013=CARTESIAN_POINT ( 'NONE',  ( -12.14591786802309592, -12.06949235617757132, 56.87390960531436690 ) ) ;
#37014=AXIS2_PLACEMENT_3D ( 'NONE', #63551, #45402, #64547 ) ;
#37015=CARTESIAN_POINT ( 'NONE',  ( -19.05341960407611168, -5.049401038298163336, 46.45724293864768129 ) ) ;
#37016=CARTESIAN_POINT ( 'NONE',  ( -14.29746914071049879, 8.314922557960819915, 55.83224293864770260 ) ) ;
#37019=CARTESIAN_POINT ( 'NONE',  ( 16.53943276465976808, -0.05219959533910856209, 28.74890960531435624 ) ) ;
#37020=CARTESIAN_POINT ( 'NONE',  ( 19.02544592524343514, -5.153800228976328945, 68.54057627198103830 ) ) ;
#37022=CARTESIAN_POINT ( 'NONE',  ( -19.03943276465977164, -0.05219959533935918106, 38.75109039468566152 ) ) ;
#37023=CARTESIAN_POINT ( 'NONE',  ( -16.55341960407617563, 4.379528057220093196, 53.54275706135234714 ) ) ;
#37024=CARTESIAN_POINT ( 'NONE',  ( 15.72974639402199770, -15.80617190586745480, 53.12390960531436690 ) ) ;
#37025=CARTESIAN_POINT ( 'NONE',  ( 10.81492255796106328, -18.62759615963255655, 105.4177570613523613 ) ) ;
#37026=CARTESIAN_POINT ( 'NONE',  ( -16.51473224551069308, -9.474510206698971260, 76.66557627198103830 ) ) ;
#37028=CARTESIAN_POINT ( 'NONE',  ( 9.474510206698971260, -16.51473224551069308, 102.9155762719810241 ) ) ;
#37030=CARTESIAN_POINT ( 'NONE',  ( 15.72974639402176855, 15.80617190586768217, 26.87609039468567218 ) ) ;
#37031=CARTESIAN_POINT ( 'NONE',  ( -16.53943276465976808, 0.05219959533911058130, 91.24890960531436690 ) ) ;
#37033=CARTESIAN_POINT ( 'NONE',  ( 15.80617190586746368, 15.72974639402197994, 84.37390960531438111 ) ) ;
#37034=CARTESIAN_POINT ( 'NONE',  ( 13.97604488694527802, 13.89961937509977652, 84.37390960531433848 ) ) ;
#37035=CARTESIAN_POINT ( 'NONE',  ( -19.03943276465977164, 0.05219959533909376836, 91.24890960531436690 ) ) ;
#37036=CARTESIAN_POINT ( 'NONE',  ( -10.81492255796078084, -18.62759615963271287, 107.0822429386476955 ) ) ;
#37039=CARTESIAN_POINT ( 'NONE',  ( 5.153800228976335163, 19.02544592524342804, 79.79057627198102409 ) ) ;
#37041=CARTESIAN_POINT ( 'NONE',  ( 16.53943276465976808, -0.05219959533910856209, 108.7489096053143669 ) ) ;
#37042=CARTESIAN_POINT ( 'NONE',  ( -16.51473224551069308, -9.474510206698971260, 31.66557627198102054 ) ) ;
#37043=CARTESIAN_POINT ( 'NONE',  ( -16.46253265017146816, -9.564922557961047289, 99.16775706135233293 ) ) ;
#37045=CARTESIAN_POINT ( 'NONE',  ( -16.53943276465976808, 0.05219959533911058130, 106.2489096053143811 ) ) ;
#37046=CARTESIAN_POINT ( 'NONE',  ( -21.53943276465977519, -0.05219959533937600094, 73.75109039468567573 ) ) ;
#37047=CARTESIAN_POINT ( 'NONE',  ( -19.02544592524342804, 5.153800228976336051, 66.04057627198103830 ) ) ;
#37048=CARTESIAN_POINT ( 'NONE',  ( 15.80617190586769283, -15.72974639402175789, 35.62609039468568994 ) ) ;
#37049=CARTESIAN_POINT ( 'NONE',  ( -5.719274019375665041, -21.55341960407619695, 19.79275706135235069 ) ) ;
#37051=CARTESIAN_POINT ( 'NONE',  ( 9.564922557960805705, 16.46253265017160317, 84.58224293864769550 ) ) ;
#37053=CARTESIAN_POINT ( 'NONE',  ( 4.483927247898790824, -16.52544592524335698, 25.20942372801901854 ) ) ;
#37054=CARTESIAN_POINT ( 'NONE',  ( 15.80617190586746368, 15.72974639402197994, 29.37390960531435269 ) ) ;
#37055=CARTESIAN_POINT ( 'NONE',  ( 10.81492255796106328, -18.62759615963255655, 65.41775706135234714 ) ) ;
#37056=CARTESIAN_POINT ( 'NONE',  ( -19.02544592524342804, 5.153800228976336051, 111.0405762719810099 ) ) ;
#37057=CARTESIAN_POINT ( 'NONE',  ( 16.46253265017146816, 9.564922557961045513, 101.6677570613523329 ) ) ;
#37058=CARTESIAN_POINT ( 'NONE',  ( -5.153800228976328057, -19.02544592524343514, 47.29057627198102409 ) ) ;
#37059=CARTESIAN_POINT ( 'NONE',  ( 0.05219959533909260263, 19.03943276465977164, 79.99890960531436690 ) ) ;
#37060=CARTESIAN_POINT ( 'NONE',  ( 8.314922557960818139, 14.29746914071049879, 99.58224293864770971 ) ) ;
#37061=CARTESIAN_POINT ( 'NONE',  ( -16.51473224551069308, -9.474510206698971260, 96.66557627198102409 ) ) ;
#37062=CARTESIAN_POINT ( 'NONE',  ( -8.224510206698948167, 14.34966873604960824, 90.41557627198103830 ) ) ;
#37063=CARTESIAN_POINT ( 'NONE',  ( -19.05341960407611168, -5.049401038298163336, 111.4572429386476671 ) ) ;
#37064=CARTESIAN_POINT ( 'NONE',  ( -14.34966873604960291, -8.224510206698953496, 56.66557627198103830 ) ) ;
#37065=CARTESIAN_POINT ( 'NONE',  ( -19.02544592524342804, 5.153800228976336051, 41.04057627198103120 ) ) ;
#37066=CARTESIAN_POINT ( 'NONE',  ( -21.55341960407619339, 5.719274019375674811, 63.54275706135234003 ) ) ;
#37067=CARTESIAN_POINT ( 'NONE',  ( 9.564922557961047289, -16.46253265017146816, 95.41775706135233293 ) ) ;
#37068=CARTESIAN_POINT ( 'NONE',  ( 16.52544592524342804, -4.483927247898539470, 48.54057627198103120 ) ) ;
#37069=CARTESIAN_POINT ( 'NONE',  ( 18.62759615963271287, -10.81492255796078972, 108.3322429386477097 ) ) ;
#37070=CARTESIAN_POINT ( 'NONE',  ( -15.72974639402197994, 15.80617190586746368, 45.62390960531436690 ) ) ;
#37071=CARTESIAN_POINT ( 'NONE',  ( 18.22780087662122739, 5.500000000000000888, 71.48236817873106475 ) ) ;
#37073=CARTESIAN_POINT ( 'NONE',  ( -19.05341960407611168, -5.049401038298163336, 51.45724293864770260 ) ) ;
#37074=CARTESIAN_POINT ( 'NONE',  ( -4.483927247898539470, -16.52544592524342804, 22.29057627198102765 ) ) ;
#37075=AXIS2_PLACEMENT_3D ( 'NONE', #21616, #96448, #143954 ) ;
#37076=CARTESIAN_POINT ( 'NONE',  ( -14.29746914071037622, -8.314922557961029526, 99.16775706135234714 ) ) ;
#37077=CARTESIAN_POINT ( 'NONE',  ( -8.224510206698735004, -14.34966873604973081, 84.58442372801903275 ) ) ;
#37078=CARTESIAN_POINT ( 'NONE',  ( -9.474510206698720793, -16.51473224551083518, 39.58442372801899722 ) ) ;
#37080=CARTESIAN_POINT ( 'NONE',  ( -9.564922557960796823, -16.46253265017161027, 97.08224293864769550 ) ) ;
#37081=CARTESIAN_POINT ( 'NONE',  ( -5.153800228976328057, -19.02544592524343514, 57.29057627198103120 ) ) ;
#37082=CARTESIAN_POINT ( 'NONE',  ( -14.29746914071049879, 8.314922557960819915, 55.83224293864770260 ) ) ;
#37083=CARTESIAN_POINT ( 'NONE',  ( 17.72517630441460312, -5.499999999999972466, 48.42175719257602395 ) ) ;
#37084=CARTESIAN_POINT ( 'NONE',  ( 5.153800228976335163, 19.02544592524342804, 109.7905762719810099 ) ) ;
#37085=CARTESIAN_POINT ( 'NONE',  ( 5.719274019375991003, -21.55341960407610458, 37.70724293864769550 ) ) ;
#37086=CARTESIAN_POINT ( 'NONE',  ( -16.52544592524342804, 4.483927247898546575, 86.04057627198102409 ) ) ;
#37087=CARTESIAN_POINT ( 'NONE',  ( -16.55341960407617563, 4.379528057220093196, 43.54275706135235424 ) ) ;
#37088=CARTESIAN_POINT ( 'NONE',  ( 8.314922557960818139, 14.29746914071049879, 84.58224293864769550 ) ) ;
#37090=CARTESIAN_POINT ( 'NONE',  ( 5.049401038297881783, 19.05341960407617563, 72.29275706135234714 ) ) ;
#37091=CARTESIAN_POINT ( 'NONE',  ( -0.05219959533909027116, -19.03943276465977164, 97.49890960531436690 ) ) ;
#37092=CARTESIAN_POINT ( 'NONE',  ( -13.97604488694547697, 13.89961937509957934, 78.12609039468567573 ) ) ;
#37094=CARTESIAN_POINT ( 'NONE',  ( -16.55341960407617563, 4.379528057220093196, 28.54275706135234358 ) ) ;
#37095=CARTESIAN_POINT ( 'NONE',  ( 16.53943276465976808, 0.05219959533934440121, 111.2510903946856899 ) ) ;
#37096=CARTESIAN_POINT ( 'NONE',  ( -19.02544592524334988, -5.153800228976617603, 73.95942372801900433 ) ) ;
#37097=CARTESIAN_POINT ( 'NONE',  ( 10.72451020669898902, -18.67979575497178502, 37.91557627198102409 ) ) ;
#37098=CARTESIAN_POINT ( 'NONE',  ( -15.80617190586768217, 15.72974639402176855, 63.12609039468568994 ) ) ;
#37100=CARTESIAN_POINT ( 'NONE',  ( 16.53943276465976808, 0.05219959533934440121, 31.25109039468568639 ) ) ;
#37101=CARTESIAN_POINT ( 'NONE',  ( -19.05341960407611168, -5.049401038298163336, 26.45724293864769550 ) ) ;
#37102=CARTESIAN_POINT ( 'NONE',  ( -5.049401038298153566, 19.05341960407611168, 90.20724293864766707 ) ) ;
#37103=CARTESIAN_POINT ( 'NONE',  ( -9.474510206698964154, 16.51473224551069663, 25.41557627198103120 ) ) ;
#37104=CARTESIAN_POINT ( 'NONE',  ( 4.379528057220339221, -16.55341960407611168, 82.70724293864770971 ) ) ;
#37105=CARTESIAN_POINT ( 'NONE',  ( -13.97604488694527625, -13.89961937509977652, 86.87390960531436690 ) ) ;
#37107=CARTESIAN_POINT ( 'NONE',  ( -19.02544592524334988, -5.153800228976617603, 98.95942372801900433 ) ) ;
#37108=CARTESIAN_POINT ( 'NONE',  ( -21.53943276465977519, 0.05219959533907696930, 71.24890960531435269 ) ) ;
#37109=CARTESIAN_POINT ( 'NONE',  ( -19.05341960407611168, -5.049401038298163336, 41.45724293864769550 ) ) ;
#37110=CARTESIAN_POINT ( 'NONE',  ( 13.97604488694548053, -13.89961937509957401, 75.62609039468564731 ) ) ;
#37111=CARTESIAN_POINT ( 'NONE',  ( 5.823673210054444382, -21.52544592524334988, 20.20942372801900788 ) ) ;
#37112=CARTESIAN_POINT ( 'NONE',  ( -19.02544592524342804, 5.153800228976336051, 66.04057627198103830 ) ) ;
#37113=CARTESIAN_POINT ( 'NONE',  ( -19.05341960407611168, -5.049401038298163336, 111.4572429386476671 ) ) ;
#37114=ORIENTED_EDGE ( 'NONE', *, *, #125633, .F. ) ;
#37115=CARTESIAN_POINT ( 'NONE',  ( 8.314922557961029526, -14.29746914071037800, 40.41775706135234714 ) ) ;
#37116=CARTESIAN_POINT ( 'NONE',  ( 5.719274019375991003, -21.55341960407610458, 107.7072429386476955 ) ) ;
#37117=CARTESIAN_POINT ( 'NONE',  ( -4.483927247898539470, -16.52544592524342804, 112.2905762719810241 ) ) ;
#37118=CARTESIAN_POINT ( 'NONE',  ( -5.153800228976328057, -19.02544592524343514, 97.29057627198099567 ) ) ;
#37119=CARTESIAN_POINT ( 'NONE',  ( -19.02544592524334988, -5.153800228976617603, 63.95942372801899012 ) ) ;
#37120=CARTESIAN_POINT ( 'NONE',  ( 0.05219959533907565091, 21.53943276465977519, 84.99890960531436690 ) ) ;
#37121=CARTESIAN_POINT ( 'NONE',  ( 10.72451020669898902, -18.67979575497178502, 92.91557627198103830 ) ) ;
#37122=CARTESIAN_POINT ( 'NONE',  ( 16.53943276465976808, -0.05219959533910856209, 48.74890960531435979 ) ) ;
#37123=CARTESIAN_POINT ( 'NONE',  ( -16.51473224551082808, 9.474510206698731452, 23.33442372801900078 ) ) ;
#37124=CARTESIAN_POINT ( 'NONE',  ( -0.05219959533934338120, 16.53943276465976808, 62.50109039468568284 ) ) ;
#37125=CARTESIAN_POINT ( 'NONE',  ( 19.03943276465977164, -0.05219959533909143690, 93.74890960531435269 ) ) ;
#37126=CARTESIAN_POINT ( 'NONE',  ( -13.89961937509977652, 13.97604488694528158, 40.62390960531435979 ) ) ;
#37127=CARTESIAN_POINT ( 'NONE',  ( 15.72974639402176855, 15.80617190586768217, 51.87609039468568284 ) ) ;
#37128=CARTESIAN_POINT ( 'NONE',  ( -0.05219959533937732626, 21.53943276465977519, 72.50109039468568994 ) ) ;
#37129=CARTESIAN_POINT ( 'NONE',  ( -13.89961937509977652, 13.97604488694528158, 65.62390960531436690 ) ) ;
#37130=CARTESIAN_POINT ( 'NONE',  ( -5.719274019375665041, -21.55341960407619695, 39.79275706135235424 ) ) ;
#37131=CARTESIAN_POINT ( 'NONE',  ( -9.474510206698720793, -16.51473224551083518, 74.58442372801900433 ) ) ;
#37132=CARTESIAN_POINT ( 'NONE',  ( -19.02544592524334988, -5.153800228976617603, 78.95942372801900433 ) ) ;
#37133=CARTESIAN_POINT ( 'NONE',  ( 9.474510206698971260, -16.51473224551069308, 37.91557627198102409 ) ) ;
#37134=CARTESIAN_POINT ( 'NONE',  ( -14.34966873604972548, 8.224510206698743886, 88.33442372801901854 ) ) ;
#37135=CARTESIAN_POINT ( 'NONE',  ( -19.03943276465977164, 0.05219959533909376836, 46.24890960531435979 ) ) ;
#37137=CARTESIAN_POINT ( 'NONE',  ( -19.05341960407611168, -5.049401038298163336, 96.45724293864769550 ) ) ;
#37138=CARTESIAN_POINT ( 'NONE',  ( 16.51473224551069308, 9.474510206698969483, 39.16557627198103120 ) ) ;
#37140=CARTESIAN_POINT ( 'NONE',  ( 18.62759615963271287, -10.81492255796078972, 83.33224293864769550 ) ) ;
#37141=CARTESIAN_POINT ( 'NONE',  ( 12.14591786802327356, -12.06949235617739191, 65.62609039468568994 ) ) ;
#37142=CARTESIAN_POINT ( 'NONE',  ( 19.02544592524334988, 5.153800228976608722, 31.45942372801900433 ) ) ;
#37143=CARTESIAN_POINT ( 'NONE',  ( -13.97604488694527625, -13.89961937509977652, 51.87390960531436690 ) ) ;
#37144=CARTESIAN_POINT ( 'NONE',  ( -0.05219959533910754901, -16.53943276465976808, 47.49890960531435979 ) ) ;
#37145=CARTESIAN_POINT ( 'NONE',  ( -16.55341960407611168, -4.379528057220339221, 86.45724293864770971 ) ) ;
#37146=CARTESIAN_POINT ( 'NONE',  ( 9.564922557960805705, 16.46253265017160317, 74.58224293864769550 ) ) ;
#37147=CARTESIAN_POINT ( 'NONE',  ( 18.67979575497194134, -10.72451020669871369, 30.83442372801902209 ) ) ;
#37148=CARTESIAN_POINT ( 'NONE',  ( 19.05341960407611168, 5.049401038298154454, 98.95724293864766707 ) ) ;
#37149=CARTESIAN_POINT ( 'NONE',  ( 5.719274019375673035, 21.55341960407619339, 102.2927570613523613 ) ) ;
#37150=CARTESIAN_POINT ( 'NONE',  ( -14.34966873604972548, 8.224510206698743886, 83.33442372801903275 ) ) ;
#37151=CARTESIAN_POINT ( 'NONE',  ( 15.80617190586769283, -15.72974639402175789, 30.62609039468567929 ) ) ;
#37152=CARTESIAN_POINT ( 'NONE',  ( -5.719274019375978568, 21.55341960407610458, 95.20724293864769550 ) ) ;
#37153=CARTESIAN_POINT ( 'NONE',  ( 8.224510206698953496, -14.34966873604960469, 42.91557627198103120 ) ) ;
#37155=CARTESIAN_POINT ( 'NONE',  ( -5.049401038298153566, 19.05341960407611168, 35.20724293864768839 ) ) ;
#37156=CARTESIAN_POINT ( 'NONE',  ( 0.05219959533910956823, 16.53943276465976808, 64.99890960531435269 ) ) ;
#37157=CARTESIAN_POINT ( 'NONE',  ( -15.80617190586745835, -15.72974639402198527, 31.87390960531435979 ) ) ;
#37158=CARTESIAN_POINT ( 'NONE',  ( 16.46253265017146816, 9.564922557961045513, 31.66775706135232937 ) ) ;
#37159=CARTESIAN_POINT ( 'NONE',  ( 8.314922557960818139, 14.29746914071049879, 94.58224293864769550 ) ) ;
#37160=CARTESIAN_POINT ( 'NONE',  ( 19.03943276465977164, -0.05219959533909143690, 113.7489096053143669 ) ) ;
#37162=CARTESIAN_POINT ( 'NONE',  ( -16.53943276465976808, -0.05219959533934237506, 48.75109039468568284 ) ) ;
#37163=CARTESIAN_POINT ( 'NONE',  ( 0.05219959533909260263, 19.03943276465977164, 54.99890960531435979 ) ) ;
#37164=CARTESIAN_POINT ( 'NONE',  ( -16.66274659544009040, -6.346227724781252633, 20.60845629695331027 ) ) ;
#37165=CARTESIAN_POINT ( 'NONE',  ( -16.55341960407617563, 4.379528057220093196, 88.54275706135236135 ) ) ;
#37166=CARTESIAN_POINT ( 'NONE',  ( -13.89961937509957401, -13.97604488694547875, 109.3760903946856331 ) ) ;
#37167=CARTESIAN_POINT ( 'NONE',  ( 10.81492255796106328, -18.62759615963255655, 85.41775706135236135 ) ) ;
#37168=CARTESIAN_POINT ( 'NONE',  ( 5.049401038298161559, -19.05341960407611168, 77.70724293864765286 ) ) ;
#37169=CARTESIAN_POINT ( 'NONE',  ( 18.67979575497178502, 10.72451020669898547, 109.1655762719810383 ) ) ;
#37170=CARTESIAN_POINT ( 'NONE',  ( -0.05219959533934338120, 16.53943276465976808, 52.50109039468567573 ) ) ;
#37172=CARTESIAN_POINT ( 'NONE',  ( 16.52544592524342804, -4.483927247898539470, 113.5405762719810383 ) ) ;
#37173=CARTESIAN_POINT ( 'NONE',  ( 16.52544592524335698, 4.483927247898782831, 21.45942372801901499 ) ) ;
#37174=CARTESIAN_POINT ( 'NONE',  ( -16.46253265017146816, -9.564922557961047289, 79.16775706135234714 ) ) ;
#37175=CARTESIAN_POINT ( 'NONE',  ( -0.05219959533907301413, -21.53943276465977519, 82.49890960531436690 ) ) ;
#37176=CARTESIAN_POINT ( 'NONE',  ( -16.46253265017146816, -9.564922557961047289, 49.16775706135233293 ) ) ;
#37177=DIRECTION ( 'NONE',  ( 0.000000000000000000, 0.000000000000000000, -1.000000000000000000 ) ) ;
#37178=CARTESIAN_POINT ( 'NONE',  ( 15.80617190586746368, 15.72974639402197994, 109.3739096053143811 ) ) ;
#37179=CARTESIAN_POINT ( 'NONE',  ( 17.49999999999999645, 5.076555817581254182, 28.67951492049776974 ) ) ;
#37180=CARTESIAN_POINT ( 'NONE',  ( 19.03943276465977164, -0.05219959533909143690, 63.74890960531435979 ) ) ;
#37183=CARTESIAN_POINT ( 'NONE',  ( -8.224510206698735004, -14.34966873604973081, 19.58442372801901143 ) ) ;
#37185=CARTESIAN_POINT ( 'NONE',  ( -5.823673210054431948, 21.52544592524334988, 57.70942372801901143 ) ) ;
#37186=CARTESIAN_POINT ( 'NONE',  ( 10.72451020669898902, -18.67979575497178502, 102.9155762719810383 ) ) ;
#37187=CARTESIAN_POINT ( 'NONE',  ( 0.05219959533910956823, 16.53943276465976808, 69.99890960531435269 ) ) ;
#37188=CARTESIAN_POINT ( 'NONE',  ( 13.97604488694527802, 13.89961937509977652, 74.37390960531436690 ) ) ;
#37190=CARTESIAN_POINT ( 'NONE',  ( -10.72451020669870658, -18.67979575497194134, 79.58442372801903275 ) ) ;
#37191=CARTESIAN_POINT ( 'NONE',  ( -12.14591786802326823, 12.06949235617739902, 28.12609039468568284 ) ) ;
#37192=CARTESIAN_POINT ( 'NONE',  ( -16.51473224551082808, 9.474510206698731452, 23.33442372801900078 ) ) ;
#37193=CARTESIAN_POINT ( 'NONE',  ( 0.05219959533937995610, -21.53943276465977519, 55.00109039468568284 ) ) ;
#37194=CARTESIAN_POINT ( 'NONE',  ( 21.53943276465977519, -0.05219959533907433946, 108.7489096053143669 ) ) ;
#37195=CARTESIAN_POINT ( 'NONE',  ( -15.80617190586745835, -15.72974639402198527, 61.87390960531436690 ) ) ;
#37196=CARTESIAN_POINT ( 'NONE',  ( -13.97604488694547697, 13.89961937509957934, 108.1260903946856331 ) ) ;
#37198=CARTESIAN_POINT ( 'NONE',  ( 13.97604488694548053, -13.89961937509957401, 70.62609039468567573 ) ) ;
#37199=CARTESIAN_POINT ( 'NONE',  ( 18.62759615963255655, 10.81492255796105972, 81.66775706135236135 ) ) ;
#37200=CARTESIAN_POINT ( 'NONE',  ( 13.97604488694548053, -13.89961937509957401, 55.62609039468566863 ) ) ;
#37201=CARTESIAN_POINT ( 'NONE',  ( 16.46253265017160672, -9.564922557960803928, 38.33224293864768839 ) ) ;
#37202=CARTESIAN_POINT ( 'NONE',  ( 18.67979575497178502, 10.72451020669898547, 59.16557627198103120 ) ) ;
#37203=CARTESIAN_POINT ( 'NONE',  ( -8.224510206698948167, 14.34966873604960824, 55.41557627198102409 ) ) ;
#37204=CARTESIAN_POINT ( 'NONE',  ( -17.48847506799969054, -5.747544572773709781, 24.17302562156720924 ) ) ;
#37205=CARTESIAN_POINT ( 'NONE',  ( 16.51473224551083163, -9.474510206698727899, 25.83442372801900078 ) ) ;
#37206=CARTESIAN_POINT ( 'NONE',  ( 16.52544592524335698, 4.483927247898782831, 81.45942372801900433 ) ) ;
#37207=CARTESIAN_POINT ( 'NONE',  ( -12.06949235617756955, 12.14591786802309770, 50.62390960531435979 ) ) ;
#37208=CARTESIAN_POINT ( 'NONE',  ( -10.72451020669870658, -18.67979575497194134, 94.58442372801901854 ) ) ;
#37209=CARTESIAN_POINT ( 'NONE',  ( 21.52544592524334988, 5.823673210054432836, 81.45942372801900433 ) ) ;
#37210=CARTESIAN_POINT ( 'NONE',  ( 0.05219959533907565091, 21.53943276465977519, 79.99890960531435269 ) ) ;
#37211=CARTESIAN_POINT ( 'NONE',  ( -9.474510206698964154, 16.51473224551069663, 45.41557627198103120 ) ) ;
#37212=CARTESIAN_POINT ( 'NONE',  ( 5.719274019375673035, 21.55341960407619339, 57.29275706135234714 ) ) ;
#37213=CARTESIAN_POINT ( 'NONE',  ( 9.474510206698971260, -16.51473224551069308, 32.91557627198102409 ) ) ;
#37214=CARTESIAN_POINT ( 'NONE',  ( 16.51473224551069308, 9.474510206698969483, 54.16557627198103120 ) ) ;
#37215=CARTESIAN_POINT ( 'NONE',  ( 8.224510206698953496, -14.34966873604960469, 102.9155762719810383 ) ) ;
#37216=CARTESIAN_POINT ( 'NONE',  ( 16.46253265017160672, -9.564922557960803928, 103.3322429386476955 ) ) ;
#37217=CARTESIAN_POINT ( 'NONE',  ( 16.52544592524342804, -4.483927247898539470, 48.54057627198103120 ) ) ;
#37218=CARTESIAN_POINT ( 'NONE',  ( -19.03943276465977164, 0.05219959533909376836, 21.24890960531436335 ) ) ;
#37220=CARTESIAN_POINT ( 'NONE',  ( -5.823673210054116645, -21.52544592524344225, 87.29057627198103830 ) ) ;
#37221=CARTESIAN_POINT ( 'NONE',  ( 15.72974639402176855, 15.80617190586768217, 21.87609039468567573 ) ) ;
#37223=CARTESIAN_POINT ( 'NONE',  ( 0.05219959533934541429, -16.53943276465976808, 35.00109039468568284 ) ) ;
#37225=CARTESIAN_POINT ( 'NONE',  ( 18.62759615963271287, -10.81492255796078972, 68.33224293864769550 ) ) ;
#37226=CARTESIAN_POINT ( 'NONE',  ( -5.823673210054431948, 21.52544592524334988, 112.7094237280190328 ) ) ;
#37227=CARTESIAN_POINT ( 'NONE',  ( 9.474510206698971260, -16.51473224551069308, 92.91557627198103830 ) ) ;
#37228=CARTESIAN_POINT ( 'NONE',  ( -18.62759615963255300, -10.81492255796106328, 34.16775706135234714 ) ) ;
#37229=CARTESIAN_POINT ( 'NONE',  ( 10.72451020669898902, -18.67979575497178502, 27.91557627198103830 ) ) ;
#37230=CARTESIAN_POINT ( 'NONE',  ( 12.14591786802327356, -12.06949235617739191, 105.6260903946856899 ) ) ;
#37231=CARTESIAN_POINT ( 'NONE',  ( 10.81492255796106328, -18.62759615963255655, 45.41775706135234003 ) ) ;
#37232=CARTESIAN_POINT ( 'NONE',  ( -15.80617190586768217, 15.72974639402176855, 78.12609039468570415 ) ) ;
#37233=CARTESIAN_POINT ( 'NONE',  ( -15.80617190586768217, 15.72974639402176855, 113.1260903946856899 ) ) ;
#37234=CARTESIAN_POINT ( 'NONE',  ( -16.53943276465976808, -0.05219959533934237506, 68.75109039468568994 ) ) ;
#37235=CARTESIAN_POINT ( 'NONE',  ( -21.52544592524334988, -5.823673210054445271, 33.95942372801901143 ) ) ;
#37236=CARTESIAN_POINT ( 'NONE',  ( 16.51473224551069308, 9.474510206698969483, 34.16557627198102409 ) ) ;
#37237=CARTESIAN_POINT ( 'NONE',  ( 5.719274019375673035, 21.55341960407619339, 102.2927570613523613 ) ) ;
#37238=CARTESIAN_POINT ( 'NONE',  ( 9.564922557960805705, 16.46253265017160317, 104.5822429386476955 ) ) ;
#37239=CARTESIAN_POINT ( 'NONE',  ( -0.05219959533907301413, -21.53943276465977519, 102.4989096053143811 ) ) ;
#37241=CARTESIAN_POINT ( 'NONE',  ( 5.719274019375991003, -21.55341960407610458, 62.70724293864769550 ) ) ;
#37242=CARTESIAN_POINT ( 'NONE',  ( -12.06949235617739369, -12.14591786802326823, 54.37609039468568994 ) ) ;
#37243=CARTESIAN_POINT ( 'NONE',  ( -12.14591786802309592, -12.06949235617757132, 51.87390960531437401 ) ) ;
#37245=CARTESIAN_POINT ( 'NONE',  ( 16.51473224551083163, -9.474510206698727899, 80.83442372801899012 ) ) ;
#37247=CARTESIAN_POINT ( 'NONE',  ( -14.29746914071037622, -8.314922557961029526, 24.16775706135235424 ) ) ;
#37248=CARTESIAN_POINT ( 'NONE',  ( 0.05219959533907565091, 21.53943276465977519, 94.99890960531436690 ) ) ;
#37249=CARTESIAN_POINT ( 'NONE',  ( 12.06949235617757843, -12.14591786802309237, 68.12390960531436690 ) ) ;
#37250=CARTESIAN_POINT ( 'NONE',  ( 18.67979575497178502, 10.72451020669898547, 24.16557627198103120 ) ) ;
#37251=CARTESIAN_POINT ( 'NONE',  ( 12.14591786802327356, -12.06949235617739191, 45.62609039468567573 ) ) ;
#37252=CARTESIAN_POINT ( 'NONE',  ( 19.05341960407611168, 5.049401038298154454, 53.95724293864770260 ) ) ;
#37253=CARTESIAN_POINT ( 'NONE',  ( 21.53943276465977519, 0.05219959533937863772, 31.25109039468568639 ) ) ;
#37254=CARTESIAN_POINT ( 'NONE',  ( 16.51473224551083163, -9.474510206698727899, 100.8344237280190043 ) ) ;
#37255=CARTESIAN_POINT ( 'NONE',  ( -13.89961937509977652, 13.97604488694528158, 95.62390960531436690 ) ) ;
#37256=CARTESIAN_POINT ( 'NONE',  ( -19.03943276465977164, 0.05219959533909376836, 91.24890960531436690 ) ) ;
#37257=CARTESIAN_POINT ( 'NONE',  ( 21.55341960407610458, 5.719274019375980345, 88.95724293864769550 ) ) ;
#37258=CARTESIAN_POINT ( 'NONE',  ( 0.05219959533909260263, 19.03943276465977164, 59.99890960531436690 ) ) ;
#37259=CARTESIAN_POINT ( 'NONE',  ( -17.31728774477270960, -6.344390552232406222, 59.18093348310682700 ) ) ;
#37260=CARTESIAN_POINT ( 'NONE',  ( 0.05219959533910956823, 16.53943276465976808, 74.99890960531435269 ) ) ;
#37261=CARTESIAN_POINT ( 'NONE',  ( 0.05219959533909260263, 19.03943276465977164, 104.9989096053143669 ) ) ;
#37263=CARTESIAN_POINT ( 'NONE',  ( 9.564922557961047289, -16.46253265017146816, 85.41775706135233293 ) ) ;
#37264=CARTESIAN_POINT ( 'NONE',  ( -21.52544592524343514, 5.823673210054127303, 91.04057627198103830 ) ) ;
#37265=CARTESIAN_POINT ( 'NONE',  ( 9.474510206698729675, 16.51473224551082808, 52.08442372801900433 ) ) ;
#37266=CARTESIAN_POINT ( 'NONE',  ( 21.55341960407610458, 5.719274019375980345, 23.95724293864769550 ) ) ;
#37268=CARTESIAN_POINT ( 'NONE',  ( -5.719274019375978568, 21.55341960407610458, 50.20724293864769550 ) ) ;
#37269=CARTESIAN_POINT ( 'NONE',  ( 19.03943276465977164, -0.05219959533909143690, 88.74890960531436690 ) ) ;
#37270=CARTESIAN_POINT ( 'NONE',  ( -10.72451020669870658, -18.67979575497194134, 74.58442372801901854 ) ) ;
#37271=CARTESIAN_POINT ( 'NONE',  ( 9.564922557960805705, 16.46253265017160317, 44.58224293864769550 ) ) ;
#37273=CARTESIAN_POINT ( 'NONE',  ( -8.224510206698948167, 14.34966873604960824, 70.41557627198102409 ) ) ;
#37274=CARTESIAN_POINT ( 'NONE',  ( 12.14591786802327356, -12.06949235617739191, 20.62609039468568639 ) ) ;
#37275=CARTESIAN_POINT ( 'NONE',  ( 10.81492255796106328, -18.62759615963255655, 65.41775706135234714 ) ) ;
#37277=CARTESIAN_POINT ( 'NONE',  ( -19.03943276465977164, 0.05219959533909376836, 116.2489096053143669 ) ) ;
#37278=CARTESIAN_POINT ( 'NONE',  ( 19.05341960407617918, -5.049401038297876454, 86.04275706135233293 ) ) ;
#37280=CARTESIAN_POINT ( 'NONE',  ( 21.55341960407619695, -5.719274019375665929, 21.04275706135234714 ) ) ;
#37282=CARTESIAN_POINT ( 'NONE',  ( -0.05219959533936034679, 19.03943276465977164, 22.50109039468566152 ) ) ;
#37283=CARTESIAN_POINT ( 'NONE',  ( 19.05341960407611168, 5.049401038298154454, 58.95724293864768129 ) ) ;
#37284=CARTESIAN_POINT ( 'NONE',  ( -19.05341960407617563, 5.049401038297882671, 23.54275706135233648 ) ) ;
#37285=CARTESIAN_POINT ( 'NONE',  ( 8.314922557961029526, -14.29746914071037800, 105.4177570613523613 ) ) ;
#37286=CARTESIAN_POINT ( 'NONE',  ( -0.05219959533909027116, -19.03943276465977164, 97.49890960531436690 ) ) ;
#37287=CARTESIAN_POINT ( 'NONE',  ( 18.67979575497194134, -10.72451020669871369, 70.83442372801901854 ) ) ;
#37290=CARTESIAN_POINT ( 'NONE',  ( 15.72974639402176855, 15.80617190586768217, 71.87609039468568994 ) ) ;
#37291=CARTESIAN_POINT ( 'NONE',  ( -10.81492255796105439, 18.62759615963255655, 102.9177570613523756 ) ) ;
#37293=CARTESIAN_POINT ( 'NONE',  ( 13.89961937509977652, -13.97604488694527269, 93.12390960531436690 ) ) ;
#37294=CARTESIAN_POINT ( 'NONE',  ( -19.03943276465977164, -0.05219959533935918106, 18.75109039468567218 ) ) ;
#37296=CARTESIAN_POINT ( 'NONE',  ( -13.89961937509977652, 13.97604488694528158, 40.62390960531435979 ) ) ;
#37297=CARTESIAN_POINT ( 'NONE',  ( 21.53943276465977519, -0.05219959533907433946, 58.74890960531436690 ) ) ;
#37298=CARTESIAN_POINT ( 'NONE',  ( 16.52544592524335698, 4.483927247898782831, 101.4594237280190185 ) ) ;
#37299=CARTESIAN_POINT ( 'NONE',  ( 16.53943276465976808, -0.05219959533910856209, 93.74890960531436690 ) ) ;
#37300=CARTESIAN_POINT ( 'NONE',  ( -16.51473224551069308, -9.474510206698971260, 86.66557627198102409 ) ) ;
#37301=CARTESIAN_POINT ( 'NONE',  ( -15.80617190586768217, 15.72974639402176855, 98.12609039468570415 ) ) ;
#37302=CARTESIAN_POINT ( 'NONE',  ( 19.05341960407611168, 5.049401038298154454, 38.95724293864767418 ) ) ;
#37303=CARTESIAN_POINT ( 'NONE',  ( -12.14591786802309592, -12.06949235617757132, 106.8739096053143811 ) ) ;
#37304=CARTESIAN_POINT ( 'NONE',  ( -10.72451020669870658, -18.67979575497194134, 49.58442372801901143 ) ) ;
#37305=CARTESIAN_POINT ( 'NONE',  ( 10.81492255796078972, 18.62759615963270932, 89.58224293864768129 ) ) ;
#37306=CARTESIAN_POINT ( 'NONE',  ( 9.474510206698729675, 16.51473224551082808, 47.08442372801900433 ) ) ;
#37307=CARTESIAN_POINT ( 'NONE',  ( 9.474510206698971260, -16.51473224551069308, 47.91557627198102409 ) ) ;
#37308=CARTESIAN_POINT ( 'NONE',  ( 13.89961937509977652, -13.97604488694527269, 93.12390960531436690 ) ) ;
#37309=CARTESIAN_POINT ( 'NONE',  ( -16.53943276465976808, 0.05219959533911058130, 81.24890960531436690 ) ) ;
#37311=CARTESIAN_POINT ( 'NONE',  ( 13.97604488694548053, -13.89961937509957401, 45.62609039468566863 ) ) ;
#37312=CARTESIAN_POINT ( 'NONE',  ( 16.46253265017160672, -9.564922557960803928, 58.33224293864769550 ) ) ;
#37313=CARTESIAN_POINT ( 'NONE',  ( 12.14591786802309770, 12.06949235617756955, 44.37390960531435979 ) ) ;
#37314=CARTESIAN_POINT ( 'NONE',  ( -5.153800228976607833, 19.02544592524334988, 72.70942372801900433 ) ) ;
#37315=CARTESIAN_POINT ( 'NONE',  ( -18.22780087662124160, -5.499999999999927169, 88.98236817873107896 ) ) ;
#37316=CARTESIAN_POINT ( 'NONE',  ( 21.52544592524344225, -5.823673210054117533, 38.54057627198103120 ) ) ;
#37317=CARTESIAN_POINT ( 'NONE',  ( -0.05219959533910754901, -16.53943276465976808, 97.49890960531436690 ) ) ;
#37319=CARTESIAN_POINT ( 'NONE',  ( -16.51473224551069308, -9.474510206698971260, 56.66557627198103120 ) ) ;
#37320=CARTESIAN_POINT ( 'NONE',  ( -10.81492255796078084, -18.62759615963271287, 62.08224293864769550 ) ) ;
#37321=CARTESIAN_POINT ( 'NONE',  ( -9.564922557960796823, -16.46253265017161027, 27.08224293864769550 ) ) ;
#37322=CARTESIAN_POINT ( 'NONE',  ( 8.224510206698742110, 14.34966873604972548, 72.08442372801899012 ) ) ;
#37323=CARTESIAN_POINT ( 'NONE',  ( -16.46253265017160317, 9.564922557960807481, 60.83224293864769550 ) ) ;
#37324=CARTESIAN_POINT ( 'NONE',  ( 9.474510206698729675, 16.51473224551082808, 52.08442372801900433 ) ) ;
#37325=CARTESIAN_POINT ( 'NONE',  ( 21.53943276465977519, 0.05219959533937863772, 71.25109039468568994 ) ) ;
#37326=CARTESIAN_POINT ( 'NONE',  ( -18.67979575497178146, -10.72451020669898902, 51.66557627198102409 ) ) ;
#37327=CARTESIAN_POINT ( 'NONE',  ( 12.06949235617757843, -12.14591786802309237, 113.1239096053143953 ) ) ;
#37328=CARTESIAN_POINT ( 'NONE',  ( 8.314922557961029526, -14.29746914071037800, 90.41775706135236135 ) ) ;
#37329=CARTESIAN_POINT ( 'NONE',  ( 19.05341960407617918, -5.049401038297876454, 106.0427570613523471 ) ) ;
#37330=CARTESIAN_POINT ( 'NONE',  ( -13.97604488694527625, -13.89961937509977652, 21.87390960531435979 ) ) ;
#37332=CARTESIAN_POINT ( 'NONE',  ( -21.55341960407610458, -5.719274019375992779, 46.45724293864769550 ) ) ;
#37333=CARTESIAN_POINT ( 'NONE',  ( -21.52544592524334988, -5.823673210054445271, 88.95942372801901854 ) ) ;
#37335=CARTESIAN_POINT ( 'NONE',  ( 0.05219959533910956823, 16.53943276465976808, 44.99890960531435979 ) ) ;
#37336=CARTESIAN_POINT ( 'NONE',  ( 16.52544592524342804, -4.483927247898539470, 58.54057627198103120 ) ) ;
#37337=CARTESIAN_POINT ( 'NONE',  ( -21.53943276465977519, 0.05219959533907696930, 81.24890960531436690 ) ) ;
#37338=CARTESIAN_POINT ( 'NONE',  ( -5.719274019375978568, 21.55341960407610458, 90.20724293864770971 ) ) ;
#37340=CARTESIAN_POINT ( 'NONE',  ( -18.67979575497178146, -10.72451020669898902, 31.66557627198102054 ) ) ;
#37341=CARTESIAN_POINT ( 'NONE',  ( -16.53943276465976808, -0.05219959533934237506, 63.75109039468568284 ) ) ;
#37342=CARTESIAN_POINT ( 'NONE',  ( 12.14591786802309770, 12.06949235617756955, 74.37390960531436690 ) ) ;
#37343=CARTESIAN_POINT ( 'NONE',  ( 9.564922557960805705, 16.46253265017160317, 29.58224293864769550 ) ) ;
#37346=CARTESIAN_POINT ( 'NONE',  ( 16.55341960407618274, -4.379528057220086978, 81.04275706135236135 ) ) ;
#37347=CARTESIAN_POINT ( 'NONE',  ( -21.53943276465977519, 0.05219959533907696930, 111.2489096053143669 ) ) ;
#37348=CARTESIAN_POINT ( 'NONE',  ( -16.51473224551069308, -9.474510206698971260, 76.66557627198103830 ) ) ;
#37349=CARTESIAN_POINT ( 'NONE',  ( 5.719274019375673035, 21.55341960407619339, 52.29275706135236135 ) ) ;
#37350=CARTESIAN_POINT ( 'NONE',  ( -9.474510206698964154, 16.51473224551069663, 105.4155762719810383 ) ) ;
#37353=CARTESIAN_POINT ( 'NONE',  ( 18.67979575497194134, -10.72451020669871369, 40.83442372801901854 ) ) ;
#37354=CARTESIAN_POINT ( 'NONE',  ( 19.05341960407611168, 5.049401038298154454, 43.95724293864769550 ) ) ;
#37355=CARTESIAN_POINT ( 'NONE',  ( -9.564922557960796823, -16.46253265017161027, 97.08224293864769550 ) ) ;
#37356=CARTESIAN_POINT ( 'NONE',  ( -5.153800228976607833, 19.02544592524334988, 52.70942372801900433 ) ) ;
#37357=CARTESIAN_POINT ( 'NONE',  ( 0.05219959533937995610, -21.53943276465977519, 30.00109039468568284 ) ) ;
#37358=CARTESIAN_POINT ( 'NONE',  ( -9.564922557961040184, 16.46253265017147172, 47.91775706135233293 ) ) ;
#37359=CARTESIAN_POINT ( 'NONE',  ( -5.153800228976328057, -19.02544592524343514, 22.29057627198102765 ) ) ;
#37360=CARTESIAN_POINT ( 'NONE',  ( -8.314922557961024197, 14.29746914071037800, 92.91775706135236135 ) ) ;
#37361=CARTESIAN_POINT ( 'NONE',  ( 9.474510206698729675, 16.51473224551082808, 62.08442372801899722 ) ) ;
#37362=CARTESIAN_POINT ( 'NONE',  ( -16.52544592524335698, -4.483927247898792601, 108.9594237280190185 ) ) ;
#37364=CARTESIAN_POINT ( 'NONE',  ( 19.05341960407611168, 5.049401038298154454, 83.95724293864766707 ) ) ;
#37366=CARTESIAN_POINT ( 'NONE',  ( -21.55341960407619339, 5.719274019375674811, 93.54275706135234714 ) ) ;
#37367=CARTESIAN_POINT ( 'NONE',  ( 18.62759615963255655, 10.81492255796105972, 111.6677570613523613 ) ) ;
#37368=CARTESIAN_POINT ( 'NONE',  ( 17.60691670004650433, 5.500000000000063061, 66.63333313366440791 ) ) ;
#37369=CARTESIAN_POINT ( 'NONE',  ( -16.46253265017160317, 9.564922557960807481, 105.8322429386476955 ) ) ;
#37370=CARTESIAN_POINT ( 'NONE',  ( -18.62759615963255300, -10.81492255796106328, 69.16775706135234714 ) ) ;
#37371=CARTESIAN_POINT ( 'NONE',  ( -9.564922557961040184, 16.46253265017147172, 112.9177570613523329 ) ) ;
#37372=CARTESIAN_POINT ( 'NONE',  ( -16.51473224551069308, -9.474510206698971260, 81.66557627198103830 ) ) ;
#37373=CARTESIAN_POINT ( 'NONE',  ( -18.62759615963270932, 10.81492255796079327, 25.83224293864769194 ) ) ;
#37375=CARTESIAN_POINT ( 'NONE',  ( -16.51473224551069308, -9.474510206698971260, 96.66557627198102409 ) ) ;
#37376=CARTESIAN_POINT ( 'NONE',  ( -16.81555441253553695, -7.025013491695479395, 89.36314554665747778 ) ) ;
#37377=CARTESIAN_POINT ( 'NONE',  ( -19.03943276465977164, 0.05219959533909376836, 76.24890960531435269 ) ) ;
#37378=CARTESIAN_POINT ( 'NONE',  ( -19.02544592524342804, 5.153800228976336051, 66.04057627198103830 ) ) ;
#37379=CARTESIAN_POINT ( 'NONE',  ( 14.29746914071037800, 8.314922557961029526, 106.6677570613523756 ) ) ;
#37381=CARTESIAN_POINT ( 'NONE',  ( -13.97604488694547697, 13.89961937509957934, 73.12609039468568994 ) ) ;
#37382=CARTESIAN_POINT ( 'NONE',  ( 19.05341960407611168, 5.049401038298154454, 93.95724293864769550 ) ) ;
#37383=CARTESIAN_POINT ( 'NONE',  ( -12.06949235617756955, 12.14591786802309770, 80.62390960531438111 ) ) ;
#37384=CARTESIAN_POINT ( 'NONE',  ( 5.823673210054125526, 21.52544592524343514, 29.79057627198102409 ) ) ;
#37385=CARTESIAN_POINT ( 'NONE',  ( -19.03943276465977164, 0.05219959533909376836, 116.2489096053143669 ) ) ;
#37386=CARTESIAN_POINT ( 'NONE',  ( 16.52544592524342804, -4.483927247898539470, 108.5405762719810241 ) ) ;
#37387=CARTESIAN_POINT ( 'NONE',  ( -16.38665767535054485, 7.295008042176028162, 55.26400864214549102 ) ) ;
#37388=CARTESIAN_POINT ( 'NONE',  ( -5.049401038297874678, -19.05341960407617918, 39.79275706135232582 ) ) ;
#37389=CARTESIAN_POINT ( 'NONE',  ( 4.483927247898545687, 16.52544592524342804, 29.79057627198102409 ) ) ;
#37390=CARTESIAN_POINT ( 'NONE',  ( 19.02544592524343514, -5.153800228976328945, 98.54057627198100988 ) ) ;
#37391=CARTESIAN_POINT ( 'NONE',  ( 15.72974639402176855, 15.80617190586768217, 61.87609039468568284 ) ) ;
#37392=CARTESIAN_POINT ( 'NONE',  ( -21.52544592524343514, 5.823673210054127303, 61.04057627198103120 ) ) ;
#37393=CARTESIAN_POINT ( 'NONE',  ( -15.80617190586768217, 15.72974639402176855, 38.12609039468567573 ) ) ;
#37394=CARTESIAN_POINT ( 'NONE',  ( 15.80617190586746368, 15.72974639402197994, 84.37390960531438111 ) ) ;
#37395=CARTESIAN_POINT ( 'NONE',  ( 18.62759615963255655, 10.81492255796105972, 36.66775706135234714 ) ) ;
#37396=CARTESIAN_POINT ( 'NONE',  ( -16.53943276465976808, 0.05219959533911058130, 106.2489096053143811 ) ) ;
#37397=CARTESIAN_POINT ( 'NONE',  ( -16.51473224551082808, 9.474510206698731452, 73.33442372801900433 ) ) ;
#37398=CARTESIAN_POINT ( 'NONE',  ( 19.05341960407611168, 5.049401038298154454, 48.95724293864768129 ) ) ;
#37399=CARTESIAN_POINT ( 'NONE',  ( -4.483927247898539470, -16.52544592524342804, 87.29057627198103830 ) ) ;
#37400=CARTESIAN_POINT ( 'NONE',  ( 13.97604488694527802, 13.89961937509977652, 99.37390960531436690 ) ) ;
#37401=CARTESIAN_POINT ( 'NONE',  ( 16.51473224551069308, 9.474510206698969483, 109.1655762719810383 ) ) ;
#37402=CARTESIAN_POINT ( 'NONE',  ( 19.03943276465977164, -0.05219959533909143690, 38.74890960531436690 ) ) ;
#37404=CARTESIAN_POINT ( 'NONE',  ( -12.14591786802309592, -12.06949235617757132, 36.87390960531435979 ) ) ;
#37405=CARTESIAN_POINT ( 'NONE',  ( -8.314922557961024197, 14.29746914071037800, 102.9177570613523756 ) ) ;
#37406=CARTESIAN_POINT ( 'NONE',  ( 16.46253265017160672, -9.564922557960803928, 58.33224293864769550 ) ) ;
#37407=CARTESIAN_POINT ( 'NONE',  ( -8.314922557960811034, -14.29746914071050412, 112.0822429386477097 ) ) ;
#37408=CARTESIAN_POINT ( 'NONE',  ( 9.564922557961047289, -16.46253265017146816, 20.41775706135233293 ) ) ;
#37409=CARTESIAN_POINT ( 'NONE',  ( 16.46253265017160672, -9.564922557960803928, 108.3322429386476955 ) ) ;
#37410=CARTESIAN_POINT ( 'NONE',  ( 16.55341960407611168, 4.379528057220329451, 28.95724293864769905 ) ) ;
#37411=CARTESIAN_POINT ( 'NONE',  ( -21.52544592524334988, -5.823673210054445271, 48.95942372801902565 ) ) ;
#37412=CARTESIAN_POINT ( 'NONE',  ( -4.483927247898782831, 16.52544592524335698, 52.70942372801902565 ) ) ;
#37413=CARTESIAN_POINT ( 'NONE',  ( 16.55341960407611168, 4.379528057220329451, 33.95724293864769550 ) ) ;
#37414=CARTESIAN_POINT ( 'NONE',  ( 8.314922557961029526, -14.29746914071037800, 105.4177570613523613 ) ) ;
#37415=CARTESIAN_POINT ( 'NONE',  ( 16.52544592524335698, 4.483927247898782831, 21.45942372801901499 ) ) ;
#37416=CARTESIAN_POINT ( 'NONE',  ( 9.474510206698971260, -16.51473224551069308, 52.91557627198102409 ) ) ;
#37417=CARTESIAN_POINT ( 'NONE',  ( -14.34966873604960291, -8.224510206698953496, 111.6655762719810525 ) ) ;
#37418=CARTESIAN_POINT ( 'NONE',  ( 10.72451020669871369, 18.67979575497193778, 22.08442372801901143 ) ) ;
#37419=CARTESIAN_POINT ( 'NONE',  ( 19.05341960407611168, 5.049401038298154454, 48.95724293864768129 ) ) ;
#37420=CARTESIAN_POINT ( 'NONE',  ( -5.049401038298153566, 19.05341960407611168, 115.2072429386477097 ) ) ;
#37421=CARTESIAN_POINT ( 'NONE',  ( -16.51473224551069308, -9.474510206698971260, 26.66557627198103120 ) ) ;
#37422=CARTESIAN_POINT ( 'NONE',  ( -0.05219959533907301413, -21.53943276465977519, 27.49890960531435269 ) ) ;
#37424=CARTESIAN_POINT ( 'NONE',  ( 16.46253265017160672, -9.564922557960803928, 103.3322429386476955 ) ) ;
#37425=CARTESIAN_POINT ( 'NONE',  ( 21.55341960407619695, -5.719274019375665929, 41.04275706135236135 ) ) ;
#37426=CARTESIAN_POINT ( 'NONE',  ( 12.06949235617757843, -12.14591786802309237, 98.12390960531436690 ) ) ;
#37427=CARTESIAN_POINT ( 'NONE',  ( -21.53943276465977519, 0.05219959533907696930, 21.24890960531436690 ) ) ;
#37429=CARTESIAN_POINT ( 'NONE',  ( -8.224510206698735004, -14.34966873604973081, 79.58442372801903275 ) ) ;
#37430=CARTESIAN_POINT ( 'NONE',  ( -21.52544592524334988, -5.823673210054445271, 88.95942372801901854 ) ) ;
#37431=CARTESIAN_POINT ( 'NONE',  ( 12.06949235617739724, 12.14591786802326823, 56.87609039468568994 ) ) ;
#37432=CARTESIAN_POINT ( 'NONE',  ( -13.97604488694527625, -13.89961937509977652, 101.8739096053143811 ) ) ;
#37433=CARTESIAN_POINT ( 'NONE',  ( 16.55341960407618274, -4.379528057220086978, 46.04275706135234714 ) ) ;
#37434=CARTESIAN_POINT ( 'NONE',  ( 19.02544592524334988, 5.153800228976608722, 111.4594237280190043 ) ) ;
#37435=CARTESIAN_POINT ( 'NONE',  ( 4.379528057220092307, 16.55341960407617563, 82.29275706135234714 ) ) ;
#37436=CARTESIAN_POINT ( 'NONE',  ( -5.049401038297874678, -19.05341960407617918, 99.79275706135234714 ) ) ;
#37437=CARTESIAN_POINT ( 'NONE',  ( -13.89961937509977652, 13.97604488694528158, 70.62390960531432427 ) ) ;
#37438=CARTESIAN_POINT ( 'NONE',  ( 10.81492255796078972, 18.62759615963270932, 99.58224293864770971 ) ) ;
#37439=CARTESIAN_POINT ( 'NONE',  ( 14.29746914071049879, -8.314922557960816363, 88.33224293864769550 ) ) ;
#37440=CARTESIAN_POINT ( 'NONE',  ( 19.02544592524334988, 5.153800228976608722, 106.4594237280190185 ) ) ;
#37441=CARTESIAN_POINT ( 'NONE',  ( -4.483927247898782831, 16.52544592524335698, 67.70942372801901854 ) ) ;
#37443=CARTESIAN_POINT ( 'NONE',  ( 13.97604488694548053, -13.89961937509957401, 70.62609039468567573 ) ) ;
#37444=CARTESIAN_POINT ( 'NONE',  ( -14.29746914071049879, 8.314922557960819915, 35.83224293864768839 ) ) ;
#37445=CARTESIAN_POINT ( 'NONE',  ( -4.379528057220328563, 16.55341960407611168, 95.20724293864769550 ) ) ;
#37446=CARTESIAN_POINT ( 'NONE',  ( 0.05219959533936267826, -19.03943276465977164, 40.00109039468566152 ) ) ;
#37447=CARTESIAN_POINT ( 'NONE',  ( 15.72974639402176855, 15.80617190586768217, 26.87609039468567218 ) ) ;
#37448=CARTESIAN_POINT ( 'NONE',  ( 19.03943276465977164, 0.05219959533936151252, 96.25109039468567573 ) ) ;
#37449=CARTESIAN_POINT ( 'NONE',  ( 9.474510206698971260, -16.51473224551069308, 112.9155762719810383 ) ) ;
#37450=CARTESIAN_POINT ( 'NONE',  ( -9.564922557960796823, -16.46253265017161027, 87.08224293864769550 ) ) ;
#37451=CARTESIAN_POINT ( 'NONE',  ( -5.823673210054431948, 21.52544592524334988, 97.70942372801904696 ) ) ;
#37452=CARTESIAN_POINT ( 'NONE',  ( 9.474510206698971260, -16.51473224551069308, 72.91557627198102409 ) ) ;
#37453=CARTESIAN_POINT ( 'NONE',  ( 21.53943276465977519, -0.05219959533907433946, 38.74890960531435979 ) ) ;
#37454=CARTESIAN_POINT ( 'NONE',  ( -8.314922557960811034, -14.29746914071050412, 97.08224293864770971 ) ) ;
#37455=CARTESIAN_POINT ( 'NONE',  ( -19.03943276465977164, 0.05219959533909376836, 56.24890960531435979 ) ) ;
#37457=CARTESIAN_POINT ( 'NONE',  ( 4.483927247898545687, 16.52544592524342804, 109.7905762719810383 ) ) ;
#37458=CARTESIAN_POINT ( 'NONE',  ( -15.72974639402176322, -15.80617190586768395, 19.37609039468568639 ) ) ;
#37459=CARTESIAN_POINT ( 'NONE',  ( -5.823673210054431948, 21.52544592524334988, 67.70942372801901854 ) ) ;
#37460=CARTESIAN_POINT ( 'NONE',  ( -9.564922557960796823, -16.46253265017161027, 42.08224293864769550 ) ) ;
#37461=CARTESIAN_POINT ( 'NONE',  ( 12.14591786802327356, -12.06949235617739191, 75.62609039468567573 ) ) ;
#37463=CARTESIAN_POINT ( 'NONE',  ( 0.05219959533907565091, 21.53943276465977519, 109.9989096053143527 ) ) ;
#37465=CARTESIAN_POINT ( 'NONE',  ( -5.719274019375978568, 21.55341960407610458, 105.2072429386477097 ) ) ;
#37466=CARTESIAN_POINT ( 'NONE',  ( -9.564922557961040184, 16.46253265017147172, 47.91775706135233293 ) ) ;
#37467=CARTESIAN_POINT ( 'NONE',  ( -9.474510206698964154, 16.51473224551069663, 70.41557627198102409 ) ) ;
#37468=CARTESIAN_POINT ( 'NONE',  ( 9.474510206698729675, 16.51473224551082808, 37.08442372801899722 ) ) ;
#37469=CARTESIAN_POINT ( 'NONE',  ( 15.72974639402176855, 15.80617190586768217, 66.87609039468568994 ) ) ;
#37470=CARTESIAN_POINT ( 'NONE',  ( 21.55341960407610458, 5.719274019375980345, 73.95724293864769550 ) ) ;
#37471=CARTESIAN_POINT ( 'NONE',  ( -14.34966873604960291, -8.224510206698953496, 46.66557627198102409 ) ) ;
#37472=CARTESIAN_POINT ( 'NONE',  ( 21.53943276465977519, 0.05219959533937863772, 86.25109039468568994 ) ) ;
#37473=CARTESIAN_POINT ( 'NONE',  ( 19.03943276465977164, 0.05219959533936151252, 26.25109039468566507 ) ) ;
#37474=CARTESIAN_POINT ( 'NONE',  ( -16.55341960407611168, -4.379528057220339221, 66.45724293864768129 ) ) ;
#37475=CARTESIAN_POINT ( 'NONE',  ( 19.02544592524343514, -5.153800228976328945, 28.54057627198102409 ) ) ;
#37476=CARTESIAN_POINT ( 'NONE',  ( 9.474510206698729675, 16.51473224551082808, 52.08442372801900433 ) ) ;
#37477=CARTESIAN_POINT ( 'NONE',  ( -14.34966873604972548, 8.224510206698743886, 113.3344237280190328 ) ) ;
#37478=CARTESIAN_POINT ( 'NONE',  ( 21.55341960407619695, -5.719274019375665929, 86.04275706135236135 ) ) ;
#37479=CARTESIAN_POINT ( 'NONE',  ( 5.049401038297881783, 19.05341960407617563, 42.29275706135234003 ) ) ;
#37480=CARTESIAN_POINT ( 'NONE',  ( -10.81492255796078084, -18.62759615963271287, 57.08224293864769550 ) ) ;
#37481=CARTESIAN_POINT ( 'NONE',  ( -5.719274019375665041, -21.55341960407619695, 44.79275706135234714 ) ) ;
#37482=CARTESIAN_POINT ( 'NONE',  ( -10.72451020669898014, 18.67979575497178502, 100.4155762719810241 ) ) ;
#37483=CARTESIAN_POINT ( 'NONE',  ( 16.46253265017146816, 9.564922557961045513, 91.66775706135234714 ) ) ;
#37484=CARTESIAN_POINT ( 'NONE',  ( 16.52544592524335698, 4.483927247898782831, 61.45942372801901854 ) ) ;
#37486=CARTESIAN_POINT ( 'NONE',  ( 5.719274019375991003, -21.55341960407610458, 107.7072429386476955 ) ) ;
#37487=CARTESIAN_POINT ( 'NONE',  ( 14.34966873604960469, 8.224510206698951720, 94.16557627198103830 ) ) ;
#37488=CARTESIAN_POINT ( 'NONE',  ( -17.49999999999999645, -5.500000000000000888, 29.20309617465828467 ) ) ;
#37489=CARTESIAN_POINT ( 'NONE',  ( -14.29746914071037622, -8.314922557961029526, 24.16775706135235424 ) ) ;
#37490=CARTESIAN_POINT ( 'NONE',  ( 21.53943276465977519, -0.05219959533907433946, 53.74890960531437401 ) ) ;
#37491=CARTESIAN_POINT ( 'NONE',  ( 16.52544592524335698, 4.483927247898782831, 86.45942372801901854 ) ) ;
#37492=CARTESIAN_POINT ( 'NONE',  ( 17.50000000000000000, -5.499999999999992895, 36.21769037696435589 ) ) ;
#37493=CARTESIAN_POINT ( 'NONE',  ( -0.05219959533934338120, 16.53943276465976808, 67.50109039468568994 ) ) ;
#37494=CARTESIAN_POINT ( 'NONE',  ( -5.823673210054431948, 21.52544592524334988, 37.70942372801900433 ) ) ;
#37495=CARTESIAN_POINT ( 'NONE',  ( 0.05219959533907565091, 21.53943276465977519, 54.99890960531435269 ) ) ;
#37496=CARTESIAN_POINT ( 'NONE',  ( -16.55341960407617563, 4.379528057220093196, 88.54275706135236135 ) ) ;
#37497=CARTESIAN_POINT ( 'NONE',  ( 15.80617190586769283, -15.72974639402175789, 65.62609039468568994 ) ) ;
#37498=CARTESIAN_POINT ( 'NONE',  ( 18.62759615963271287, -10.81492255796078972, 53.33224293864769550 ) ) ;
#37499=CARTESIAN_POINT ( 'NONE',  ( 21.53943276465977519, -0.05219959533907433946, 33.74890960531436690 ) ) ;
#37501=CARTESIAN_POINT ( 'NONE',  ( -16.53943276465976808, -0.05219959533934237506, 68.75109039468568994 ) ) ;
#37502=CARTESIAN_POINT ( 'NONE',  ( 18.62759615963271287, -10.81492255796078972, 38.33224293864768839 ) ) ;
#37504=CARTESIAN_POINT ( 'NONE',  ( 19.02544592524343514, -5.153800228976328945, 103.5405762719809957 ) ) ;
#37505=CARTESIAN_POINT ( 'NONE',  ( 4.379528057220092307, 16.55341960407617563, 112.2927570613523471 ) ) ;
#37506=CARTESIAN_POINT ( 'NONE',  ( 17.72662750342724536, 5.500000000000079048, 73.90179492283743912 ) ) ;
#37507=CARTESIAN_POINT ( 'NONE',  ( 0.05219959533910956823, 16.53943276465976808, 109.9989096053143527 ) ) ;
#37508=CARTESIAN_POINT ( 'NONE',  ( 15.80617190586746368, 15.72974639402197994, 54.37390960531435979 ) ) ;
#37509=CARTESIAN_POINT ( 'NONE',  ( 16.46253265017160672, -9.564922557960803928, 48.33224293864769550 ) ) ;
#37510=CARTESIAN_POINT ( 'NONE',  ( 12.14591786802327356, -12.06949235617739191, 90.62609039468567573 ) ) ;
#37511=CARTESIAN_POINT ( 'NONE',  ( -18.67979575497193778, 10.72451020669871902, 28.33442372801902209 ) ) ;
#37512=CARTESIAN_POINT ( 'NONE',  ( -13.97604488694547697, 13.89961937509957934, 93.12609039468566152 ) ) ;
#37513=CARTESIAN_POINT ( 'NONE',  ( -12.14591786802309592, -12.06949235617757132, 96.87390960531436690 ) ) ;
#37514=CARTESIAN_POINT ( 'NONE',  ( 13.97604488694527802, 13.89961937509977652, 59.37390960531434558 ) ) ;
#37516=CARTESIAN_POINT ( 'NONE',  ( -9.474510206698964154, 16.51473224551069663, 25.41557627198103120 ) ) ;
#37518=CARTESIAN_POINT ( 'NONE',  ( 9.474510206698971260, -16.51473224551069308, 77.91557627198103830 ) ) ;
#37519=CARTESIAN_POINT ( 'NONE',  ( -4.379528057220086978, -16.55341960407618274, 64.79275706135234714 ) ) ;
#37520=CARTESIAN_POINT ( 'NONE',  ( -21.55341960407619339, 5.719274019375674811, 103.5427570613523613 ) ) ;
#37521=CARTESIAN_POINT ( 'NONE',  ( -5.719274019375978568, 21.55341960407610458, 50.20724293864769550 ) ) ;
#37522=CARTESIAN_POINT ( 'NONE',  ( 16.52544592524335698, 4.483927247898782831, 71.45942372801901854 ) ) ;
#37523=CARTESIAN_POINT ( 'NONE',  ( 9.564922557961047289, -16.46253265017146816, 65.41775706135233293 ) ) ;
#37525=CARTESIAN_POINT ( 'NONE',  ( -5.823673210054431948, 21.52544592524334988, 67.70942372801901854 ) ) ;
#37526=CARTESIAN_POINT ( 'NONE',  ( -0.05219959533909027116, -19.03943276465977164, 62.49890960531435979 ) ) ;
#37527=CARTESIAN_POINT ( 'NONE',  ( -19.02544592524342804, 5.153800228976336051, 36.04057627198100988 ) ) ;
#37528=CARTESIAN_POINT ( 'NONE',  ( 16.51473224551083163, -9.474510206698727899, 65.83442372801900433 ) ) ;
#37529=CARTESIAN_POINT ( 'NONE',  ( 19.02544592524343514, -5.153800228976328945, 108.5405762719810383 ) ) ;
#37530=CARTESIAN_POINT ( 'NONE',  ( -5.153800228976328057, -19.02544592524343514, 97.29057627198099567 ) ) ;
#37531=CARTESIAN_POINT ( 'NONE',  ( -8.314922557960811034, -14.29746914071050412, 57.08224293864769550 ) ) ;
#37532=CARTESIAN_POINT ( 'NONE',  ( 5.719274019375991003, -21.55341960407610458, 42.70724293864770260 ) ) ;
#37534=CARTESIAN_POINT ( 'NONE',  ( -19.02544592524334988, -5.153800228976617603, 23.95942372801900078 ) ) ;
#37535=CARTESIAN_POINT ( 'NONE',  ( 16.46253265017160672, -9.564922557960803928, 48.33224293864769550 ) ) ;
#37536=DIRECTION ( 'NONE',  ( -0.000000000000000000, -0.000000000000000000, 1.000000000000000000 ) ) ;
#37537=CARTESIAN_POINT ( 'NONE',  ( -17.48853670773244318, 5.747243402303103821, 108.6667129974999142 ) ) ;
#37538=CARTESIAN_POINT ( 'NONE',  ( 16.53943276465976808, 0.05219959533934440121, 81.25109039468568994 ) ) ;
#37539=CARTESIAN_POINT ( 'NONE',  ( -5.823673210054116645, -21.52544592524344225, 102.2905762719810383 ) ) ;
#37540=CARTESIAN_POINT ( 'NONE',  ( 14.34966873604960469, 8.224510206698951720, 49.16557627198102409 ) ) ;
#37541=CARTESIAN_POINT ( 'NONE',  ( 5.049401038298161559, -19.05341960407611168, 42.70724293864767418 ) ) ;
#37543=CARTESIAN_POINT ( 'NONE',  ( 10.72451020669871369, 18.67979575497193778, 47.08442372801901854 ) ) ;
#37544=CARTESIAN_POINT ( 'NONE',  ( -0.05219959533936034679, 19.03943276465977164, 42.50109039468566152 ) ) ;
#37545=CARTESIAN_POINT ( 'NONE',  ( -19.02544592524342804, 5.153800228976336051, 51.04057627198103120 ) ) ;
#37546=CARTESIAN_POINT ( 'NONE',  ( -18.62759615963255300, -10.81492255796106328, 94.16775706135237556 ) ) ;
#37549=CARTESIAN_POINT ( 'NONE',  ( -16.53943276465976808, 0.05219959533911058130, 46.24890960531435979 ) ) ;
#37550=CARTESIAN_POINT ( 'NONE',  ( 19.25918095147781983, 5.499999999999579892, 41.95284276293937609 ) ) ;
#37551=CARTESIAN_POINT ( 'NONE',  ( -18.67979575497178146, -10.72451020669898902, 36.66557627198103120 ) ) ;
#37554=CARTESIAN_POINT ( 'NONE',  ( 13.97604488694527802, 13.89961937509977652, 104.3739096053143385 ) ) ;
#37555=CARTESIAN_POINT ( 'NONE',  ( -0.05219959533910754901, -16.53943276465976808, 87.49890960531436690 ) ) ;
#37556=CARTESIAN_POINT ( 'NONE',  ( -8.314922557961024197, 14.29746914071037800, 22.91775706135235069 ) ) ;
#37557=CARTESIAN_POINT ( 'NONE',  ( 4.483927247898790824, -16.52544592524335698, 105.2094237280190328 ) ) ;
#37559=CARTESIAN_POINT ( 'NONE',  ( -9.474510206698964154, 16.51473224551069663, 95.41557627198102409 ) ) ;
#37560=CARTESIAN_POINT ( 'NONE',  ( -10.81492255796078084, -18.62759615963271287, 102.0822429386476955 ) ) ;
#37561=CARTESIAN_POINT ( 'NONE',  ( -0.05219959533910754901, -16.53943276465976808, 32.49890960531435979 ) ) ;
#37562=CARTESIAN_POINT ( 'NONE',  ( 5.153800228976335163, 19.02544592524342804, 94.79057627198103830 ) ) ;
#37563=CARTESIAN_POINT ( 'NONE',  ( -9.474510206698720793, -16.51473224551083518, 94.58442372801900433 ) ) ;
#37564=CARTESIAN_POINT ( 'NONE',  ( 15.80617190586769283, -15.72974639402175789, 110.6260903946857042 ) ) ;
#37565=CARTESIAN_POINT ( 'NONE',  ( 18.62759615963271287, -10.81492255796078972, 88.33224293864769550 ) ) ;
#37566=CARTESIAN_POINT ( 'NONE',  ( 0.05219959533907565091, 21.53943276465977519, 44.99890960531435979 ) ) ;
#37567=CARTESIAN_POINT ( 'NONE',  ( -0.05219959533909027116, -19.03943276465977164, 57.49890960531435979 ) ) ;
#37568=CARTESIAN_POINT ( 'NONE',  ( 4.483927247898545687, 16.52544592524342804, 34.79057627198103120 ) ) ;
#37569=CARTESIAN_POINT ( 'NONE',  ( -13.97604488694527625, -13.89961937509977652, 76.87390960531433848 ) ) ;
#37571=CARTESIAN_POINT ( 'NONE',  ( 16.51473224551069308, 9.474510206698969483, 79.16557627198103830 ) ) ;
#37572=CARTESIAN_POINT ( 'NONE',  ( 13.89961937509957401, 13.97604488694547697, 36.87609039468565442 ) ) ;
#37573=CARTESIAN_POINT ( 'NONE',  ( -14.29746914071049879, 8.314922557960819915, 90.83224293864769550 ) ) ;
#37574=CARTESIAN_POINT ( 'NONE',  ( 15.80617190586769283, -15.72974639402175789, 25.62609039468567929 ) ) ;
#37576=CARTESIAN_POINT ( 'NONE',  ( -16.52544592524335698, -4.483927247898792601, 103.9594237280190185 ) ) ;
#37577=CARTESIAN_POINT ( 'NONE',  ( -16.53943276465976808, 0.05219959533911058130, 116.2489096053143669 ) ) ;
#37578=CARTESIAN_POINT ( 'NONE',  ( 13.97604488694527802, 13.89961937509977652, 79.37390960531435269 ) ) ;
#37580=CARTESIAN_POINT ( 'NONE',  ( 13.97604488694527802, 13.89961937509977652, 24.37390960531435624 ) ) ;
#37581=CARTESIAN_POINT ( 'NONE',  ( 12.14591786802309770, 12.06949235617756955, 44.37390960531435979 ) ) ;
#37583=CARTESIAN_POINT ( 'NONE',  ( -5.719274019375665041, -21.55341960407619695, 54.79275706135235424 ) ) ;
#37585=CARTESIAN_POINT ( 'NONE',  ( -5.823673210054431948, 21.52544592524334988, 97.70942372801904696 ) ) ;
#37586=CARTESIAN_POINT ( 'NONE',  ( 19.02544592524343514, -5.153800228976328945, 38.54057627198103120 ) ) ;
#37587=CARTESIAN_POINT ( 'NONE',  ( 9.474510206698971260, -16.51473224551069308, 52.91557627198102409 ) ) ;
#37589=CARTESIAN_POINT ( 'NONE',  ( 15.72974639402176855, 15.80617190586768217, 91.87609039468568994 ) ) ;
#37590=CARTESIAN_POINT ( 'NONE',  ( 8.224510206698742110, 14.34966873604972548, 57.08442372801901854 ) ) ;
#37591=CARTESIAN_POINT ( 'NONE',  ( 10.81492255796106328, -18.62759615963255655, 90.41775706135236135 ) ) ;
#37592=CARTESIAN_POINT ( 'NONE',  ( -21.53943276465977519, 0.05219959533907696930, 26.24890960531435624 ) ) ;
#37593=CARTESIAN_POINT ( 'NONE',  ( 16.46253265017146816, 9.564922557961045513, 91.66775706135234714 ) ) ;
#37594=CARTESIAN_POINT ( 'NONE',  ( 10.81492255796106328, -18.62759615963255655, 75.41775706135233293 ) ) ;
#37595=CARTESIAN_POINT ( 'NONE',  ( -14.34966873604972548, 8.224510206698743886, 38.33442372801900433 ) ) ;
#37596=CARTESIAN_POINT ( 'NONE',  ( 21.53943276465977519, -0.05219959533907433946, 83.74890960531435269 ) ) ;
#37597=CARTESIAN_POINT ( 'NONE',  ( 16.51473224551083163, -9.474510206698727899, 85.83442372801900433 ) ) ;
#37598=CARTESIAN_POINT ( 'NONE',  ( -19.05341960407611168, -5.049401038298163336, 61.45724293864769550 ) ) ;
#37599=CARTESIAN_POINT ( 'NONE',  ( 9.474510206698729675, 16.51473224551082808, 102.0844237280190043 ) ) ;
#37600=CARTESIAN_POINT ( 'NONE',  ( -16.46253265017146816, -9.564922557961047289, 104.1677570613523329 ) ) ;
#37601=CARTESIAN_POINT ( 'NONE',  ( 4.379528057220339221, -16.55341960407611168, 52.70724293864769550 ) ) ;
#37602=CARTESIAN_POINT ( 'NONE',  ( -13.89961937509957401, -13.97604488694547875, 74.37609039468566152 ) ) ;
#37603=CARTESIAN_POINT ( 'NONE',  ( 12.06949235617739724, 12.14591786802326823, 61.87609039468568284 ) ) ;
#37604=CARTESIAN_POINT ( 'NONE',  ( -16.51473224551069308, -9.474510206698971260, 41.66557627198103120 ) ) ;
#37605=CARTESIAN_POINT ( 'NONE',  ( -5.153800228976328057, -19.02544592524343514, 52.29057627198100988 ) ) ;
#37606=CARTESIAN_POINT ( 'NONE',  ( -8.224510206698735004, -14.34966873604973081, 59.58442372801901854 ) ) ;
#37610=CARTESIAN_POINT ( 'NONE',  ( 16.51473224551069308, 9.474510206698969483, 99.16557627198102409 ) ) ;
#37613=CARTESIAN_POINT ( 'NONE',  ( -5.153800228976607833, 19.02544592524334988, 107.7094237280189759 ) ) ;
#37614=CARTESIAN_POINT ( 'NONE',  ( 18.67979575497178502, 10.72451020669898547, 39.16557627198102409 ) ) ;
#37615=CARTESIAN_POINT ( 'NONE',  ( 13.89961937509957401, 13.97604488694547697, 31.87609039468566863 ) ) ;
#37616=CARTESIAN_POINT ( 'NONE',  ( -12.06949235617739369, -12.14591786802326823, 29.37609039468568284 ) ) ;
#37617=CARTESIAN_POINT ( 'NONE',  ( 16.51473224551069308, 9.474510206698969483, 34.16557627198102409 ) ) ;
#37618=CARTESIAN_POINT ( 'NONE',  ( -16.46253265017160317, 9.564922557960807481, 45.83224293864769550 ) ) ;
#37619=CARTESIAN_POINT ( 'NONE',  ( -0.05219959533907301413, -21.53943276465977519, 87.49890960531436690 ) ) ;
#37620=CARTESIAN_POINT ( 'NONE',  ( 9.564922557960805705, 16.46253265017160317, 104.5822429386476955 ) ) ;
#37621=CARTESIAN_POINT ( 'NONE',  ( -19.03943276465977164, 0.05219959533909376836, 56.24890960531435979 ) ) ;
#37623=CARTESIAN_POINT ( 'NONE',  ( -13.97604488694547697, 13.89961937509957934, 83.12609039468564731 ) ) ;
#37624=CARTESIAN_POINT ( 'NONE',  ( -16.55341960407611168, -4.379528057220339221, 71.45724293864769550 ) ) ;
#37625=CARTESIAN_POINT ( 'NONE',  ( 5.719274019375991003, -21.55341960407610458, 47.70724293864770260 ) ) ;
#37626=CARTESIAN_POINT ( 'NONE',  ( 15.72974639402176855, 15.80617190586768217, 111.8760903946856615 ) ) ;
#37627=CARTESIAN_POINT ( 'NONE',  ( 21.52544592524344225, -5.823673210054117533, 98.54057627198105251 ) ) ;
#37628=CARTESIAN_POINT ( 'NONE',  ( -15.80617190586768217, 15.72974639402176855, 68.12609039468567573 ) ) ;
#37629=CARTESIAN_POINT ( 'NONE',  ( -5.823673210054431948, 21.52544592524334988, 72.70942372801901854 ) ) ;
#37630=CARTESIAN_POINT ( 'NONE',  ( -5.049401038298153566, 19.05341960407611168, 110.2072429386476671 ) ) ;
#37631=CARTESIAN_POINT ( 'NONE',  ( -8.314922557961024197, 14.29746914071037800, 107.9177570613523471 ) ) ;
#37632=CARTESIAN_POINT ( 'NONE',  ( -18.67979575497193778, 10.72451020669871902, 73.33442372801901854 ) ) ;
#37633=CARTESIAN_POINT ( 'NONE',  ( -9.474510206698964154, 16.51473224551069663, 60.41557627198102409 ) ) ;
#37634=CARTESIAN_POINT ( 'NONE',  ( 15.72974639402176855, 15.80617190586768217, 26.87609039468567218 ) ) ;
#37635=CARTESIAN_POINT ( 'NONE',  ( 13.89961937509977652, -13.97604488694527269, 88.12390960531438111 ) ) ;
#37636=CARTESIAN_POINT ( 'NONE',  ( -8.224510206698948167, 14.34966873604960824, 85.41557627198102409 ) ) ;
#37637=CARTESIAN_POINT ( 'NONE',  ( -4.483927247898539470, -16.52544592524342804, 52.29057627198102409 ) ) ;
#37638=CARTESIAN_POINT ( 'NONE',  ( 10.81492255796078972, 18.62759615963270932, 59.58224293864770260 ) ) ;
#37639=CARTESIAN_POINT ( 'NONE',  ( -9.564922557960796823, -16.46253265017161027, 67.08224293864769550 ) ) ;
#37640=CARTESIAN_POINT ( 'NONE',  ( -15.80617190586745835, -15.72974639402198527, 76.87390960531439532 ) ) ;
#37641=CARTESIAN_POINT ( 'NONE',  ( -19.03943276465977164, -0.05219959533935918106, 58.75109039468566863 ) ) ;
#37643=CARTESIAN_POINT ( 'NONE',  ( -9.474510206698720793, -16.51473224551083518, 24.58442372801900078 ) ) ;
#37644=CARTESIAN_POINT ( 'NONE',  ( -12.14591786802309592, -12.06949235617757132, 76.87390960531439532 ) ) ;
#37645=CARTESIAN_POINT ( 'NONE',  ( -15.72974639402197994, 15.80617190586746368, 50.62390960531435979 ) ) ;
#37646=ORIENTED_EDGE ( 'NONE', *, *, #85112, .T. ) ;
#37647=CARTESIAN_POINT ( 'NONE',  ( -17.49999999999998579, -5.500000000000015099, 41.28230962303565832 ) ) ;
#37648=CARTESIAN_POINT ( 'NONE',  ( -16.53943276465976808, -0.05219959533934237506, 93.75109039468567573 ) ) ;
#37650=CARTESIAN_POINT ( 'NONE',  ( -19.03943276465977164, -0.05219959533935918106, 93.75109039468566152 ) ) ;
#37651=CARTESIAN_POINT ( 'NONE',  ( 14.29746914071049879, -8.314922557960816363, 63.33224293864770260 ) ) ;
#37652=CARTESIAN_POINT ( 'NONE',  ( -18.56101223717332260, -5.499999999999947597, 61.44978406935677384 ) ) ;
#37653=CARTESIAN_POINT ( 'NONE',  ( -9.474510206698964154, 16.51473224551069663, 55.41557627198103120 ) ) ;
#37654=CARTESIAN_POINT ( 'NONE',  ( 12.06949235617757843, -12.14591786802309237, 53.12390960531436690 ) ) ;
#37655=CARTESIAN_POINT ( 'NONE',  ( -19.05341960407611168, -5.049401038298163336, 86.45724293864769550 ) ) ;
#37656=CARTESIAN_POINT ( 'NONE',  ( -5.049401038297874678, -19.05341960407617918, 79.79275706135233293 ) ) ;
#37657=CARTESIAN_POINT ( 'NONE',  ( -5.153800228976328057, -19.02544592524343514, 57.29057627198103120 ) ) ;
#37658=CARTESIAN_POINT ( 'NONE',  ( 16.51473224551069308, 9.474510206698969483, 84.16557627198102409 ) ) ;
#37659=CARTESIAN_POINT ( 'NONE',  ( 13.97604488694527802, 13.89961937509977652, 74.37390960531436690 ) ) ;
#37660=CARTESIAN_POINT ( 'NONE',  ( 21.55341960407610458, 5.719274019375980345, 63.95724293864770260 ) ) ;
#37661=CARTESIAN_POINT ( 'NONE',  ( 16.52544592524335698, 4.483927247898782831, 56.45942372801902565 ) ) ;
#37662=DIRECTION ( 'NONE',  ( 1.000000000000000000, 0.000000000000000000, 0.000000000000000000 ) ) ;
#37663=CARTESIAN_POINT ( 'NONE',  ( -9.474510206698964154, 16.51473224551069663, 45.41557627198103120 ) ) ;
#37664=CARTESIAN_POINT ( 'NONE',  ( 18.67979575497178502, 10.72451020669898547, 59.16557627198103120 ) ) ;
#37665=CARTESIAN_POINT ( 'NONE',  ( -16.51473224551082808, 9.474510206698731452, 83.33442372801899012 ) ) ;
#37666=CARTESIAN_POINT ( 'NONE',  ( -14.29746914071049879, 8.314922557960819915, 25.83224293864769194 ) ) ;
#37667=CARTESIAN_POINT ( 'NONE',  ( -9.564922557961040184, 16.46253265017147172, 42.91775706135234003 ) ) ;
#37668=CARTESIAN_POINT ( 'NONE',  ( 0.05219959533934541429, -16.53943276465976808, 60.00109039468568284 ) ) ;
#37669=CARTESIAN_POINT ( 'NONE',  ( -12.06949235617739369, -12.14591786802326823, 89.37609039468568994 ) ) ;
#37670=CARTESIAN_POINT ( 'NONE',  ( -17.60769864724391098, 5.499999999999988454, 73.65024842019163032 ) ) ;
#37671=CARTESIAN_POINT ( 'NONE',  ( -14.29746914071037622, -8.314922557961029526, 84.16775706135234714 ) ) ;
#37672=CARTESIAN_POINT ( 'NONE',  ( -18.62759615963270932, 10.81492255796079327, 30.83224293864770260 ) ) ;
#37673=CARTESIAN_POINT ( 'NONE',  ( 5.153800228976335163, 19.02544592524342804, 39.79057627198100988 ) ) ;
#37674=CARTESIAN_POINT ( 'NONE',  ( -9.474510206698964154, 16.51473224551069663, 50.41557627198102409 ) ) ;
#37675=CARTESIAN_POINT ( 'NONE',  ( -19.02544592524342804, 5.153800228976336051, 41.04057627198103120 ) ) ;
#37676=CARTESIAN_POINT ( 'NONE',  ( -21.53943276465977519, -0.05219959533937600094, 33.75109039468568284 ) ) ;
#37677=CARTESIAN_POINT ( 'NONE',  ( -14.29746914071037622, -8.314922557961029526, 49.16775706135234003 ) ) ;
#37678=CARTESIAN_POINT ( 'NONE',  ( -0.05219959533910754901, -16.53943276465976808, 22.49890960531436335 ) ) ;
#37679=CARTESIAN_POINT ( 'NONE',  ( -16.46253265017160317, 9.564922557960807481, 25.83224293864769194 ) ) ;
#37680=CARTESIAN_POINT ( 'NONE',  ( 5.153800228976615827, -19.02544592524334988, 20.20942372801899722 ) ) ;
#37681=CARTESIAN_POINT ( 'NONE',  ( -16.53943276465976808, -0.05219959533934237506, 18.75109039468568639 ) ) ;
#37682=CARTESIAN_POINT ( 'NONE',  ( -9.474510206698720793, -16.51473224551083518, 69.58442372801901854 ) ) ;
#37683=CARTESIAN_POINT ( 'NONE',  ( 0.05219959533910956823, 16.53943276465976808, 74.99890960531435269 ) ) ;
#37684=CARTESIAN_POINT ( 'NONE',  ( -19.02544592524342804, 5.153800228976336051, 36.04057627198100988 ) ) ;
#37685=CARTESIAN_POINT ( 'NONE',  ( 0.05219959533936267826, -19.03943276465977164, 75.00109039468566152 ) ) ;
#37686=CARTESIAN_POINT ( 'NONE',  ( 16.52216118717208815, -7.221426719304493425, 91.42400978953007495 ) ) ;
#37687=CARTESIAN_POINT ( 'NONE',  ( 10.72451020669871369, 18.67979575497193778, 72.08442372801899012 ) ) ;
#37688=CARTESIAN_POINT ( 'NONE',  ( -16.53943276465976808, -0.05219959533934237506, 43.75109039468568284 ) ) ;
#37690=CARTESIAN_POINT ( 'NONE',  ( -18.67979575497178146, -10.72451020669898902, 41.66557627198103120 ) ) ;
#37691=CARTESIAN_POINT ( 'NONE',  ( -12.06949235617739369, -12.14591786802326823, 24.37609039468567573 ) ) ;
#37693=CARTESIAN_POINT ( 'NONE',  ( 5.049401038297881783, 19.05341960407617563, 22.29275706135233648 ) ) ;
#37695=CARTESIAN_POINT ( 'NONE',  ( -19.02544592524342804, 5.153800228976336051, 41.04057627198103120 ) ) ;
#37697=CARTESIAN_POINT ( 'NONE',  ( -0.05219959533909027116, -19.03943276465977164, 52.49890960531436690 ) ) ;
#37699=CARTESIAN_POINT ( 'NONE',  ( 5.823673210054444382, -21.52544592524334988, 60.20942372801902565 ) ) ;
#37700=CARTESIAN_POINT ( 'NONE',  ( 16.46253265017146816, 9.564922557961045513, 21.66775706135233648 ) ) ;
#37701=CARTESIAN_POINT ( 'NONE',  ( -4.379528057220328563, 16.55341960407611168, 30.20724293864769550 ) ) ;
#37702=CARTESIAN_POINT ( 'NONE',  ( 5.153800228976335163, 19.02544592524342804, 29.79057627198102409 ) ) ;
#37704=CARTESIAN_POINT ( 'NONE',  ( 19.03943276465977164, -0.05219959533909143690, 98.74890960531436690 ) ) ;
#37705=CARTESIAN_POINT ( 'NONE',  ( 15.72974639402176855, 15.80617190586768217, 51.87609039468568284 ) ) ;
#37706=CARTESIAN_POINT ( 'NONE',  ( -19.03943276465977164, 0.05219959533909376836, 36.24890960531436690 ) ) ;
#37707=CARTESIAN_POINT ( 'NONE',  ( 5.719274019375673035, 21.55341960407619339, 72.29275706135236135 ) ) ;
#37708=CARTESIAN_POINT ( 'NONE',  ( -13.89961937509957401, -13.97604488694547875, 94.37609039468566152 ) ) ;
#37709=CARTESIAN_POINT ( 'NONE',  ( 0.05219959533909260263, 19.03943276465977164, 109.9989096053143669 ) ) ;
#37710=CARTESIAN_POINT ( 'NONE',  ( 0.05219959533909260263, 19.03943276465977164, 24.99890960531435269 ) ) ;
#37711=CARTESIAN_POINT ( 'NONE',  ( 0.05219959533907565091, 21.53943276465977519, 114.9989096053143669 ) ) ;
#37712=CARTESIAN_POINT ( 'NONE',  ( -19.05341960407617563, 5.049401038297882671, 38.54275706135233293 ) ) ;
#37713=CARTESIAN_POINT ( 'NONE',  ( 8.314922557960818139, 14.29746914071049879, 114.5822429386477097 ) ) ;
#37714=CARTESIAN_POINT ( 'NONE',  ( 19.05341960407611168, 5.049401038298154454, 68.95724293864769550 ) ) ;
#37715=CARTESIAN_POINT ( 'NONE',  ( -16.51473224551082808, 9.474510206698731452, 98.33442372801900433 ) ) ;
#37716=CARTESIAN_POINT ( 'NONE',  ( -14.34966873604960291, -8.224510206698953496, 66.66557627198102409 ) ) ;
#37717=CARTESIAN_POINT ( 'NONE',  ( -5.153800228976607833, 19.02544592524334988, 22.70942372801899012 ) ) ;
#37718=CARTESIAN_POINT ( 'NONE',  ( 0.05219959533909260263, 19.03943276465977164, 114.9989096053143669 ) ) ;
#37719=CARTESIAN_POINT ( 'NONE',  ( -19.02544592524334988, -5.153800228976617603, 93.95942372801900433 ) ) ;
#37720=CARTESIAN_POINT ( 'NONE',  ( 21.53943276465977519, -0.05219959533907433946, 88.74890960531436690 ) ) ;
#37721=CARTESIAN_POINT ( 'NONE',  ( -15.80617190586768217, 15.72974639402176855, 38.12609039468567573 ) ) ;
#37722=CARTESIAN_POINT ( 'NONE',  ( 4.483927247898790824, -16.52544592524335698, 40.20942372801901854 ) ) ;
#37723=CARTESIAN_POINT ( 'NONE',  ( 14.29746914071037800, 8.314922557961029526, 106.6677570613523756 ) ) ;
#37724=CARTESIAN_POINT ( 'NONE',  ( 16.53943276465976808, 0.05219959533934440121, 36.25109039468567573 ) ) ;
#37725=CARTESIAN_POINT ( 'NONE',  ( -18.62759615963255300, -10.81492255796106328, 44.16775706135234714 ) ) ;
#37726=CARTESIAN_POINT ( 'NONE',  ( -5.719274019375978568, 21.55341960407610458, 55.20724293864770260 ) ) ;
#37727=CARTESIAN_POINT ( 'NONE',  ( -0.05219959533909027116, -19.03943276465977164, 37.49890960531436690 ) ) ;
#37729=CARTESIAN_POINT ( 'NONE',  ( 16.55341960407618274, -4.379528057220086978, 76.04275706135237556 ) ) ;
#37730=CARTESIAN_POINT ( 'NONE',  ( 5.823673210054125526, 21.52544592524343514, 84.79057627198102409 ) ) ;
#37731=CARTESIAN_POINT ( 'NONE',  ( -14.34966873604960291, -8.224510206698953496, 36.66557627198103120 ) ) ;
#37732=CARTESIAN_POINT ( 'NONE',  ( 16.55341960407618274, -4.379528057220086978, 66.04275706135236135 ) ) ;
#37733=CARTESIAN_POINT ( 'NONE',  ( -9.474510206698720793, -16.51473224551083518, 94.58442372801900433 ) ) ;
#37734=CARTESIAN_POINT ( 'NONE',  ( 0.05219959533907565091, 21.53943276465977519, 104.9989096053143669 ) ) ;
#37735=CARTESIAN_POINT ( 'NONE',  ( -14.29746914071049879, 8.314922557960819915, 30.83224293864770260 ) ) ;
#37737=ORIENTED_EDGE ( 'NONE', *, *, #155971, .F. ) ;
#37738=CARTESIAN_POINT ( 'NONE',  ( 8.224510206698742110, 14.34966873604972548, 82.08442372801901854 ) ) ;
#37740=CARTESIAN_POINT ( 'NONE',  ( 15.80617190586746368, 15.72974639402197994, 79.37390960531436690 ) ) ;
#37742=CARTESIAN_POINT ( 'NONE',  ( 4.483927247898790824, -16.52544592524335698, 100.2094237280190043 ) ) ;
#37744=CARTESIAN_POINT ( 'NONE',  ( 19.39720447994795194, 5.499999999999968914, 87.16317477297175742 ) ) ;
#37745=CARTESIAN_POINT ( 'NONE',  ( -18.62759615963270932, 10.81492255796079327, 85.83224293864768129 ) ) ;
#37746=CARTESIAN_POINT ( 'NONE',  ( -10.72451020669898014, 18.67979575497178502, 105.4155762719810383 ) ) ;
#37747=CARTESIAN_POINT ( 'NONE',  ( 12.06949235617757843, -12.14591786802309237, 43.12390960531435269 ) ) ;
#37748=CARTESIAN_POINT ( 'NONE',  ( 16.52544592524335698, 4.483927247898782831, 31.45942372801901854 ) ) ;
#37749=CARTESIAN_POINT ( 'NONE',  ( -9.564922557960796823, -16.46253265017161027, 42.08224293864769550 ) ) ;
#37750=CARTESIAN_POINT ( 'NONE',  ( -16.46253265017160317, 9.564922557960807481, 60.83224293864769550 ) ) ;
#37751=ORIENTED_EDGE ( 'NONE', *, *, #111017, .T. ) ;
#37752=CARTESIAN_POINT ( 'NONE',  ( 0.05219959533909260263, 19.03943276465977164, 114.9989096053143669 ) ) ;
#37753=CARTESIAN_POINT ( 'NONE',  ( 17.97214573761831247, 5.500000000000080824, 78.96970049038658601 ) ) ;
#37754=CARTESIAN_POINT ( 'NONE',  ( 9.564922557961047289, -16.46253265017146816, 100.4177570613523329 ) ) ;
#37755=CARTESIAN_POINT ( 'NONE',  ( -19.05341960407617563, 5.049401038297882671, 53.54275706135231871 ) ) ;
#37756=CARTESIAN_POINT ( 'NONE',  ( -10.81492255796078084, -18.62759615963271287, 92.08224293864769550 ) ) ;
#37757=CARTESIAN_POINT ( 'NONE',  ( 12.06949235617739724, 12.14591786802326823, 111.8760903946856615 ) ) ;
#37758=CARTESIAN_POINT ( 'NONE',  ( 21.53943276465977519, -0.05219959533907433946, 43.74890960531435979 ) ) ;
#37759=CARTESIAN_POINT ( 'NONE',  ( 21.52544592524344225, -5.823673210054117533, 78.54057627198103830 ) ) ;
#37760=CARTESIAN_POINT ( 'NONE',  ( 0.05219959533936267826, -19.03943276465977164, 105.0010903946856615 ) ) ;
#37761=CARTESIAN_POINT ( 'NONE',  ( -16.46253265017160317, 9.564922557960807481, 100.8322429386477097 ) ) ;
#37762=CARTESIAN_POINT ( 'NONE',  ( -10.72451020669870658, -18.67979575497194134, 74.58442372801901854 ) ) ;
#37763=CARTESIAN_POINT ( 'NONE',  ( -19.03943276465977164, 0.05219959533909376836, 71.24890960531435269 ) ) ;
#37765=CARTESIAN_POINT ( 'NONE',  ( 9.474510206698971260, -16.51473224551069308, 67.91557627198102409 ) ) ;
#37766=CARTESIAN_POINT ( 'NONE',  ( 8.314922557960818139, 14.29746914071049879, 89.58224293864768129 ) ) ;
#37767=ORIENTED_EDGE ( 'NONE', *, *, #176141, .T. ) ;
#37768=CARTESIAN_POINT ( 'NONE',  ( 16.46253265017146816, 9.564922557961045513, 106.6677570613523471 ) ) ;
#37769=CARTESIAN_POINT ( 'NONE',  ( 17.26172910966779384, -6.454744622555844913, 83.30646908649222837 ) ) ;
#37770=CARTESIAN_POINT ( 'NONE',  ( 13.97604488694527802, 13.89961937509977652, 74.37390960531436690 ) ) ;
#37771=CARTESIAN_POINT ( 'NONE',  ( -10.72451020669870658, -18.67979575497194134, 84.58442372801903275 ) ) ;
#37772=CARTESIAN_POINT ( 'NONE',  ( -13.97604488694527625, -13.89961937509977652, 96.87390960531433848 ) ) ;
#37773=CARTESIAN_POINT ( 'NONE',  ( 12.14591786802327356, -12.06949235617739191, 75.62609039468567573 ) ) ;
#37774=CARTESIAN_POINT ( 'NONE',  ( -17.40805194822031154, -6.112264579159315758, 74.16628727489390371 ) ) ;
#37775=CARTESIAN_POINT ( 'NONE',  ( -0.05219959533936034679, 19.03943276465977164, 57.50109039468566863 ) ) ;
#37776=CARTESIAN_POINT ( 'NONE',  ( -10.72451020669870658, -18.67979575497194134, 109.5844237280190328 ) ) ;
#37780=CARTESIAN_POINT ( 'NONE',  ( 4.379528057220339221, -16.55341960407611168, 22.70724293864769194 ) ) ;
#37782=CARTESIAN_POINT ( 'NONE',  ( 14.34966873604972726, -8.224510206698740333, 95.83442372801903275 ) ) ;
#37784=CARTESIAN_POINT ( 'NONE',  ( -12.14591786802326823, 12.06949235617739902, 78.12609039468570415 ) ) ;
#37785=CARTESIAN_POINT ( 'NONE',  ( 10.81492255796106328, -18.62759615963255655, 80.41775706135234714 ) ) ;
#37786=CARTESIAN_POINT ( 'NONE',  ( 5.049401038297881783, 19.05341960407617563, 87.29275706135234714 ) ) ;
#37787=CARTESIAN_POINT ( 'NONE',  ( -16.46253265017146816, -9.564922557961047289, 39.16775706135234003 ) ) ;
#37788=CARTESIAN_POINT ( 'NONE',  ( 19.02544592524343514, -5.153800228976328945, 73.54057627198103830 ) ) ;
#37789=CARTESIAN_POINT ( 'NONE',  ( -0.05219959533909027116, -19.03943276465977164, 62.49890960531435979 ) ) ;
#37790=CARTESIAN_POINT ( 'NONE',  ( -19.48894818550241581, 5.500000000000114575, 40.10307310435242556 ) ) ;
#37791=CARTESIAN_POINT ( 'NONE',  ( 18.62759615963271287, -10.81492255796078972, 98.33224293864769550 ) ) ;
#37793=CARTESIAN_POINT ( 'NONE',  ( -10.72451020669898014, 18.67979575497178502, 45.41557627198103830 ) ) ;
#37794=CARTESIAN_POINT ( 'NONE',  ( -9.564922557960796823, -16.46253265017161027, 27.08224293864769550 ) ) ;
#37795=CARTESIAN_POINT ( 'NONE',  ( -8.224510206698735004, -14.34966873604973081, 69.58442372801900433 ) ) ;
#37797=EDGE_LOOP ( 'NONE', ( #196772, #74917, #34575, #186341 ) ) ;
#37798=CARTESIAN_POINT ( 'NONE',  ( 10.81492255796106328, -18.62759615963255655, 50.41775706135235424 ) ) ;
#37799=CARTESIAN_POINT ( 'NONE',  ( 16.52544592524342804, -4.483927247898539470, 68.54057627198103830 ) ) ;
#37801=CARTESIAN_POINT ( 'NONE',  ( 16.53943276465976808, 0.05219959533934440121, 36.25109039468567573 ) ) ;
#37802=CARTESIAN_POINT ( 'NONE',  ( -16.52544592524342804, 4.483927247898546575, 106.0405762719810525 ) ) ;
#37803=CARTESIAN_POINT ( 'NONE',  ( 0.05219959533936267826, -19.03943276465977164, 50.00109039468566863 ) ) ;
#37805=CARTESIAN_POINT ( 'NONE',  ( -4.483927247898539470, -16.52544592524342804, 57.29057627198103120 ) ) ;
#37806=CARTESIAN_POINT ( 'NONE',  ( 18.67979575497194134, -10.72451020669871369, 35.83442372801901143 ) ) ;
#37809=CARTESIAN_POINT ( 'NONE',  ( -15.80617190586745835, -15.72974639402198527, 96.87390960531436690 ) ) ;
#37810=CARTESIAN_POINT ( 'NONE',  ( -9.474510206698964154, 16.51473224551069663, 100.4155762719810241 ) ) ;
#37811=CARTESIAN_POINT ( 'NONE',  ( -16.55341960407611168, -4.379528057220339221, 76.45724293864769550 ) ) ;
#37812=CARTESIAN_POINT ( 'NONE',  ( 9.474510206698971260, -16.51473224551069308, 112.9155762719810383 ) ) ;
#37814=CARTESIAN_POINT ( 'NONE',  ( -9.474510206698720793, -16.51473224551083518, 84.58442372801900433 ) ) ;
#37815=CARTESIAN_POINT ( 'NONE',  ( -21.52544592524334988, -5.823673210054445271, 18.95942372801901143 ) ) ;
#37816=CARTESIAN_POINT ( 'NONE',  ( 0.05219959533909260263, 19.03943276465977164, 69.99890960531435269 ) ) ;
#37817=CARTESIAN_POINT ( 'NONE',  ( -0.05219959533936034679, 19.03943276465977164, 62.50109039468566863 ) ) ;
#37818=CARTESIAN_POINT ( 'NONE',  ( -0.05219959533909027116, -19.03943276465977164, 37.49890960531436690 ) ) ;
#37819=CARTESIAN_POINT ( 'NONE',  ( 10.81492255796106328, -18.62759615963255655, 65.41775706135234714 ) ) ;
#37822=CARTESIAN_POINT ( 'NONE',  ( -14.29746914071049879, 8.314922557960819915, 60.83224293864769550 ) ) ;
#37823=CARTESIAN_POINT ( 'NONE',  ( -13.89961937509977652, 13.97604488694528158, 65.62390960531436690 ) ) ;
#37824=CARTESIAN_POINT ( 'NONE',  ( 21.55341960407610458, 5.719274019375980345, 93.95724293864770971 ) ) ;
#37825=CARTESIAN_POINT ( 'NONE',  ( -0.05219959533909027116, -19.03943276465977164, 52.49890960531436690 ) ) ;
#37827=CARTESIAN_POINT ( 'NONE',  ( 15.72974639402199770, -15.80617190586745480, 78.12390960531436690 ) ) ;
#37828=CARTESIAN_POINT ( 'NONE',  ( 5.719274019375673035, 21.55341960407619339, 97.29275706135234714 ) ) ;
#37830=CARTESIAN_POINT ( 'NONE',  ( -16.53943276465976808, -0.05219959533934237506, 93.75109039468567573 ) ) ;
#37831=CARTESIAN_POINT ( 'NONE',  ( -4.483927247898539470, -16.52544592524342804, 102.2905762719810383 ) ) ;
#37832=CARTESIAN_POINT ( 'NONE',  ( 5.153800228976615827, -19.02544592524334988, 90.20942372801900433 ) ) ;
#37834=CARTESIAN_POINT ( 'NONE',  ( 15.80617190586769283, -15.72974639402175789, 20.62609039468568639 ) ) ;
#37835=CARTESIAN_POINT ( 'NONE',  ( -19.03943276465977164, -0.05219959533935918106, 53.75109039468566863 ) ) ;
#37836=CARTESIAN_POINT ( 'NONE',  ( -4.483927247898782831, 16.52544592524335698, 102.7094237280190185 ) ) ;
#37837=CARTESIAN_POINT ( 'NONE',  ( 19.02544592524334988, 5.153800228976608722, 36.45942372801900433 ) ) ;
#37838=CARTESIAN_POINT ( 'NONE',  ( 5.153800228976335163, 19.02544592524342804, 99.79057627198102409 ) ) ;
#37839=CARTESIAN_POINT ( 'NONE',  ( -21.55341960407610458, -5.719274019375992779, 61.45724293864770260 ) ) ;
#37841=CARTESIAN_POINT ( 'NONE',  ( 0.05219959533910956823, 16.53943276465976808, 114.9989096053143669 ) ) ;
#37842=CARTESIAN_POINT ( 'NONE',  ( -0.05219959533937732626, 21.53943276465977519, 112.5010903946857042 ) ) ;
#37843=CARTESIAN_POINT ( 'NONE',  ( -12.14591786802326823, 12.06949235617739902, 73.12609039468567573 ) ) ;
#37844=CARTESIAN_POINT ( 'NONE',  ( -15.80617190586768217, 15.72974639402176855, 33.12609039468569705 ) ) ;
#37845=CARTESIAN_POINT ( 'NONE',  ( 8.314922557961029526, -14.29746914071037800, 45.41775706135234003 ) ) ;
#37846=CARTESIAN_POINT ( 'NONE',  ( -9.474510206698964154, 16.51473224551069663, 105.4155762719810383 ) ) ;
#37847=CARTESIAN_POINT ( 'NONE',  ( 16.51473224551069308, 9.474510206698969483, 44.16557627198103120 ) ) ;
#37848=CARTESIAN_POINT ( 'NONE',  ( -19.03943276465977164, 0.05219959533909376836, 71.24890960531435269 ) ) ;
#37850=CARTESIAN_POINT ( 'NONE',  ( -16.52544592524335698, -4.483927247898792601, 43.95942372801902565 ) ) ;
#37851=CARTESIAN_POINT ( 'NONE',  ( -0.05219959533910754901, -16.53943276465976808, 92.49890960531436690 ) ) ;
#37852=CARTESIAN_POINT ( 'NONE',  ( 8.224510206698742110, 14.34966873604972548, 102.0844237280190185 ) ) ;
#37854=CARTESIAN_POINT ( 'NONE',  ( 21.55341960407619695, -5.719274019375665929, 61.04275706135234714 ) ) ;
#37855=CARTESIAN_POINT ( 'NONE',  ( 5.153800228976335163, 19.02544592524342804, 74.79057627198103830 ) ) ;
#37856=CARTESIAN_POINT ( 'NONE',  ( -16.46253265017160317, 9.564922557960807481, 65.83224293864769550 ) ) ;
#37857=CARTESIAN_POINT ( 'NONE',  ( 19.05341960407611168, 5.049401038298154454, 93.95724293864769550 ) ) ;
#37858=CARTESIAN_POINT ( 'NONE',  ( -14.29746914071049879, 8.314922557960819915, 50.83224293864770971 ) ) ;
#37859=CARTESIAN_POINT ( 'NONE',  ( -16.53943276465976808, -0.05219959533934237506, 98.75109039468568994 ) ) ;
#37860=CARTESIAN_POINT ( 'NONE',  ( 4.483927247898545687, 16.52544592524342804, 24.79057627198103120 ) ) ;
#37862=CARTESIAN_POINT ( 'NONE',  ( 13.97604488694548053, -13.89961937509957401, 45.62609039468566863 ) ) ;
#37864=CARTESIAN_POINT ( 'NONE',  ( 16.46253265017160672, -9.564922557960803928, 58.33224293864769550 ) ) ;
#37865=CARTESIAN_POINT ( 'NONE',  ( 16.51473224551083163, -9.474510206698727899, 40.83442372801900433 ) ) ;
#37868=CARTESIAN_POINT ( 'NONE',  ( 16.46253265017146816, 9.564922557961045513, 81.66775706135233293 ) ) ;
#37869=CARTESIAN_POINT ( 'NONE',  ( -0.05219959533934338120, 16.53943276465976808, 67.50109039468568994 ) ) ;
#37870=CARTESIAN_POINT ( 'NONE',  ( 16.20579543436678094, 7.371946100355098785, 93.06520834171877254 ) ) ;
#37871=( BOUNDED_CURVE ( )  B_SPLINE_CURVE ( 2, ( #101184, #41542, #87032, #69868, #146696, #40534, #162873, #86032, #117368, #165880, #11207, #102205, #103205 ),
 .UNSPECIFIED., .F., .T. ) 
 B_SPLINE_CURVE_WITH_KNOTS ( ( 3, 2, 2, 2, 2, 2, 3 ),
 ( 0.6076935943217820491, 0.6096491228070175517, 0.6140350877192982670, 0.6184210526315789824, 0.6228070175438596978, 0.6271929824561403022, 0.6291028311192857769 ),
 .UNSPECIFIED. ) 
 CURVE ( )  GEOMETRIC_REPRESENTATION_ITEM ( )  RATIONAL_B_SPLINE_CURVE ( ( 0.9831626618144007068, 0.9848076720550096308, 1.000000000000000000, 0.9659258262890683122, 1.000000000000000000, 0.9659258262890683122, 1.000000000000000000, 0.9659258262890683122, 1.000000000000000000, 0.9659258262890683122, 1.000000000000000000, 0.9851625545550091179, 0.9832469066685282089 ) ) 
 REPRESENTATION_ITEM ( '' )  );
#37872=CARTESIAN_POINT ( 'NONE',  ( 9.474510206698971260, -16.51473224551069308, 92.91557627198103830 ) ) ;
#37873=CARTESIAN_POINT ( 'NONE',  ( -0.05219959533937732626, 21.53943276465977519, 22.50109039468567573 ) ) ;
#37874=CARTESIAN_POINT ( 'NONE',  ( 19.05341960407617918, -5.049401038297876454, 76.04275706135230450 ) ) ;
#37875=CARTESIAN_POINT ( 'NONE',  ( 17.49999999999999645, 5.500000000000010658, 88.78230962303567253 ) ) ;
#37876=CARTESIAN_POINT ( 'NONE',  ( 0.05219959533909260263, 19.03943276465977164, 29.99890960531435979 ) ) ;
#37877=CARTESIAN_POINT ( 'NONE',  ( 13.97604488694527802, 13.89961937509977652, 89.37390960531436690 ) ) ;
#37878=CARTESIAN_POINT ( 'NONE',  ( 8.224510206698953496, -14.34966873604960469, 52.91557627198103830 ) ) ;
#37879=CARTESIAN_POINT ( 'NONE',  ( 9.474510206698971260, -16.51473224551069308, 42.91557627198103120 ) ) ;
#37880=CARTESIAN_POINT ( 'NONE',  ( 19.03943276465977164, 0.05219959533936151252, 46.25109039468566863 ) ) ;
#37882=CARTESIAN_POINT ( 'NONE',  ( -4.483927247898539470, -16.52544592524342804, 82.29057627198103830 ) ) ;
#37883=CARTESIAN_POINT ( 'NONE',  ( 9.474510206698729675, 16.51473224551082808, 32.08442372801900433 ) ) ;
#37884=CARTESIAN_POINT ( 'NONE',  ( -5.153800228976328057, -19.02544592524343514, 72.29057627198102409 ) ) ;
#37885=CARTESIAN_POINT ( 'NONE',  ( -21.55341960407610458, -5.719274019375992779, 61.45724293864770260 ) ) ;
#37886=CARTESIAN_POINT ( 'NONE',  ( 8.224510206698953496, -14.34966873604960469, 52.91557627198103830 ) ) ;
#37887=CARTESIAN_POINT ( 'NONE',  ( 13.97604488694548053, -13.89961937509957401, 25.62609039468566507 ) ) ;
#37888=CARTESIAN_POINT ( 'NONE',  ( -0.05219959533909027116, -19.03943276465977164, 102.4989096053143669 ) ) ;
#37889=CARTESIAN_POINT ( 'NONE',  ( 5.719274019375991003, -21.55341960407610458, 22.70724293864769194 ) ) ;
#37890=CARTESIAN_POINT ( 'NONE',  ( 5.049401038298161559, -19.05341960407611168, 47.70724293864770260 ) ) ;
#37891=CARTESIAN_POINT ( 'NONE',  ( 16.51473224551069308, 9.474510206698969483, 24.16557627198102765 ) ) ;
#37892=CARTESIAN_POINT ( 'NONE',  ( -4.379528057220328563, 16.55341960407611168, 95.20724293864769550 ) ) ;
#37893=CARTESIAN_POINT ( 'NONE',  ( 5.719274019375991003, -21.55341960407610458, 92.70724293864770971 ) ) ;
#37894=CARTESIAN_POINT ( 'NONE',  ( 9.474510206698971260, -16.51473224551069308, 107.9155762719810383 ) ) ;
#37895=CARTESIAN_POINT ( 'NONE',  ( -21.52544592524343514, 5.823673210054127303, 106.0405762719810525 ) ) ;
#37896=CARTESIAN_POINT ( 'NONE',  ( 0.05219959533909260263, 19.03943276465977164, 109.9989096053143669 ) ) ;
#37897=CARTESIAN_POINT ( 'NONE',  ( -13.89961937509977652, 13.97604488694528158, 25.62390960531434558 ) ) ;
#37898=CARTESIAN_POINT ( 'NONE',  ( 5.823673210054444382, -21.52544592524334988, 80.20942372801901854 ) ) ;
#37899=CARTESIAN_POINT ( 'NONE',  ( 21.55341960407610458, 5.719274019375980345, 88.95724293864769550 ) ) ;
#37900=LINE ( 'NONE', #113719, #124634 ) ;
#37902=CARTESIAN_POINT ( 'NONE',  ( 18.22780087662121673, 5.500000000000056843, 58.98459894673892023 ) ) ;
#37903=CARTESIAN_POINT ( 'NONE',  ( 12.14591786802327356, -12.06949235617739191, 40.62609039468567573 ) ) ;
#37904=CARTESIAN_POINT ( 'NONE',  ( -4.483927247898539470, -16.52544592524342804, 112.2905762719810241 ) ) ;
#37905=CARTESIAN_POINT ( 'NONE',  ( -17.50000000000000355, -3.209263204892571775, 110.2380317439372845 ) ) ;
#37906=CARTESIAN_POINT ( 'NONE',  ( -5.049401038298153566, 19.05341960407611168, 60.20724293864768129 ) ) ;
#37907=CARTESIAN_POINT ( 'NONE',  ( 14.29746914071049879, -8.314922557960816363, 93.33224293864769550 ) ) ;
#37908=CARTESIAN_POINT ( 'NONE',  ( -18.67979575497178146, -10.72451020669898902, 31.66557627198102054 ) ) ;
#37909=CARTESIAN_POINT ( 'NONE',  ( 8.224510206698953496, -14.34966873604960469, 62.91557627198102409 ) ) ;
#37910=CARTESIAN_POINT ( 'NONE',  ( 19.02544592524334988, 5.153800228976608722, 111.4594237280190043 ) ) ;
#37911=CARTESIAN_POINT ( 'NONE',  ( -21.53943276465977519, -0.05219959533937600094, 78.75109039468568994 ) ) ;
#37912=CARTESIAN_POINT ( 'NONE',  ( 14.34966873604972726, -8.224510206698740333, 100.8344237280190185 ) ) ;
#37913=CARTESIAN_POINT ( 'NONE',  ( -16.55341960407611168, -4.379528057220339221, 41.45724293864769550 ) ) ;
#37914=CARTESIAN_POINT ( 'NONE',  ( -19.05341960407611168, -5.049401038298163336, 41.45724293864769550 ) ) ;
#37915=CARTESIAN_POINT ( 'NONE',  ( 13.97604488694527802, 13.89961937509977652, 89.37390960531436690 ) ) ;
#37916=CARTESIAN_POINT ( 'NONE',  ( 21.53943276465977519, -0.05219959533907433946, 93.74890960531436690 ) ) ;
#37917=CARTESIAN_POINT ( 'NONE',  ( -4.379528057220086978, -16.55341960407618274, 29.79275706135234358 ) ) ;
#37918=CARTESIAN_POINT ( 'NONE',  ( -12.06949235617756955, 12.14591786802309770, 60.62390960531437401 ) ) ;
#37919=CARTESIAN_POINT ( 'NONE',  ( -18.67979575497193778, 10.72451020669871902, 68.33442372801900433 ) ) ;
#37920=CARTESIAN_POINT ( 'NONE',  ( -16.55341960407617563, 4.379528057220093196, 98.54275706135234714 ) ) ;
#37921=CARTESIAN_POINT ( 'NONE',  ( 16.79531203550682505, -7.028104445595340977, 46.24755011779544134 ) ) ;
#37923=CARTESIAN_POINT ( 'NONE',  ( 16.52544592524342804, -4.483927247898539470, 28.54057627198103120 ) ) ;
#37924=CARTESIAN_POINT ( 'NONE',  ( -4.379528057220086978, -16.55341960407618274, 79.79275706135236135 ) ) ;
#37925=CARTESIAN_POINT ( 'NONE',  ( 13.97604488694527802, 13.89961937509977652, 84.37390960531433848 ) ) ;
#37926=CARTESIAN_POINT ( 'NONE',  ( -19.05341960407611168, -5.049401038298163336, 81.45724293864769550 ) ) ;
#37927=CARTESIAN_POINT ( 'NONE',  ( 21.55341960407619695, -5.719274019375665929, 91.04275706135236135 ) ) ;
#37928=CARTESIAN_POINT ( 'NONE',  ( 12.14591786802327356, -12.06949235617739191, 90.62609039468567573 ) ) ;
#37929=CARTESIAN_POINT ( 'NONE',  ( 4.379528057220339221, -16.55341960407611168, 57.70724293864770260 ) ) ;
#37930=CARTESIAN_POINT ( 'NONE',  ( -19.05341960407611168, -5.049401038298163336, 66.45724293864769550 ) ) ;
#37932=CARTESIAN_POINT ( 'NONE',  ( -5.049401038297874678, -19.05341960407617918, 109.7927570613523187 ) ) ;
#37933=CARTESIAN_POINT ( 'NONE',  ( 16.55341960407611168, 4.379528057220329451, 103.9572429386476813 ) ) ;
#37934=CARTESIAN_POINT ( 'NONE',  ( 16.46253265017160672, -9.564922557960803928, 78.33224293864769550 ) ) ;
#37935=CARTESIAN_POINT ( 'NONE',  ( -14.34966873604972548, 8.224510206698743886, 23.33442372801901499 ) ) ;
#37937=CARTESIAN_POINT ( 'NONE',  ( 9.474510206698729675, 16.51473224551082808, 22.08442372801899722 ) ) ;
#37938=CARTESIAN_POINT ( 'NONE',  ( 12.06949235617739724, 12.14591786802326823, 81.87609039468568994 ) ) ;
#37939=CARTESIAN_POINT ( 'NONE',  ( -16.46253265017146816, -9.564922557961047289, 94.16775706135233293 ) ) ;
#37940=CARTESIAN_POINT ( 'NONE',  ( -9.564922557960796823, -16.46253265017161027, 22.08224293864768839 ) ) ;
#37942=CARTESIAN_POINT ( 'NONE',  ( 14.34966873604972726, -8.224510206698740333, 60.83442372801901854 ) ) ;
#37943=CARTESIAN_POINT ( 'NONE',  ( 0.05219959533934541429, -16.53943276465976808, 55.00109039468568284 ) ) ;
#37944=CARTESIAN_POINT ( 'NONE',  ( -19.03943276465977164, 0.05219959533909376836, 21.24890960531436335 ) ) ;
#37945=CARTESIAN_POINT ( 'NONE',  ( -5.049401038297874678, -19.05341960407617918, 59.79275706135231871 ) ) ;
#37946=CARTESIAN_POINT ( 'NONE',  ( 18.62759615963255655, 10.81492255796105972, 91.66775706135234714 ) ) ;
#37947=CARTESIAN_POINT ( 'NONE',  ( -13.97604488694527625, -13.89961937509977652, 36.87390960531436690 ) ) ;
#37948=CARTESIAN_POINT ( 'NONE',  ( -9.564922557960796823, -16.46253265017161027, 82.08224293864768129 ) ) ;
#37949=CARTESIAN_POINT ( 'NONE',  ( -4.483927247898539470, -16.52544592524342804, 77.29057627198102409 ) ) ;
#37952=CARTESIAN_POINT ( 'NONE',  ( 18.62759615963255655, 10.81492255796105972, 86.66775706135234714 ) ) ;
#37953=CARTESIAN_POINT ( 'NONE',  ( -19.03943276465977164, -0.05219959533935918106, 58.75109039468566863 ) ) ;
#37954=CARTESIAN_POINT ( 'NONE',  ( -16.46253265017146816, -9.564922557961047289, 39.16775706135234003 ) ) ;
#37955=CARTESIAN_POINT ( 'NONE',  ( 10.72451020669898902, -18.67979575497178502, 32.91557627198102409 ) ) ;
#37956=CARTESIAN_POINT ( 'NONE',  ( -0.05219959533937732626, 21.53943276465977519, 97.50109039468567573 ) ) ;
#37957=CARTESIAN_POINT ( 'NONE',  ( 19.05341960407611168, 5.049401038298154454, 83.95724293864766707 ) ) ;
#37958=CARTESIAN_POINT ( 'NONE',  ( -18.67979575497193778, 10.72451020669871902, 108.3344237280190185 ) ) ;
#37959=CARTESIAN_POINT ( 'NONE',  ( -21.52544592524343514, 5.823673210054127303, 51.04057627198103120 ) ) ;
#37960=CARTESIAN_POINT ( 'NONE',  ( -5.153800228976328057, -19.02544592524343514, 97.29057627198099567 ) ) ;
#37961=CARTESIAN_POINT ( 'NONE',  ( -16.46253265017146816, -9.564922557961047289, 74.16775706135234714 ) ) ;
#37962=CARTESIAN_POINT ( 'NONE',  ( -9.564922557960796823, -16.46253265017161027, 102.0822429386477097 ) ) ;
#37963=CARTESIAN_POINT ( 'NONE',  ( 16.51473224551083163, -9.474510206698727899, 100.8344237280190043 ) ) ;
#37964=CARTESIAN_POINT ( 'NONE',  ( -4.483927247898782831, 16.52544592524335698, 47.70942372801902565 ) ) ;
#37965=CARTESIAN_POINT ( 'NONE',  ( -4.379528057220328563, 16.55341960407611168, 105.2072429386477097 ) ) ;
#37966=CARTESIAN_POINT ( 'NONE',  ( 16.46253265017160672, -9.564922557960803928, 88.33224293864769550 ) ) ;
#37967=CARTESIAN_POINT ( 'NONE',  ( 15.80617190586746368, 15.72974639402197994, 64.37390960531435269 ) ) ;
#37968=CARTESIAN_POINT ( 'NONE',  ( -14.29746914071037622, -8.314922557961029526, 39.16775706135235424 ) ) ;
#37969=CARTESIAN_POINT ( 'NONE',  ( -5.719274019375665041, -21.55341960407619695, 39.79275706135235424 ) ) ;
#37970=CARTESIAN_POINT ( 'NONE',  ( 10.81492255796106328, -18.62759615963255655, 80.41775706135234714 ) ) ;
#37971=CARTESIAN_POINT ( 'NONE',  ( 4.379528057220092307, 16.55341960407617563, 77.29275706135234714 ) ) ;
#37972=CARTESIAN_POINT ( 'NONE',  ( -9.474510206698964154, 16.51473224551069663, 70.41557627198102409 ) ) ;
#37973=CARTESIAN_POINT ( 'NONE',  ( 12.06949235617757843, -12.14591786802309237, 83.12390960531436690 ) ) ;
#37974=CARTESIAN_POINT ( 'NONE',  ( -8.314922557960811034, -14.29746914071050412, 22.08224293864769194 ) ) ;
#37975=CARTESIAN_POINT ( 'NONE',  ( -13.89961937509957401, -13.97604488694547875, 54.37609039468565442 ) ) ;
#37977=CARTESIAN_POINT ( 'NONE',  ( 10.81492255796106328, -18.62759615963255655, 50.41775706135235424 ) ) ;
#37978=CARTESIAN_POINT ( 'NONE',  ( 16.52544592524342804, -4.483927247898539470, 83.54057627198102409 ) ) ;
#37979=CARTESIAN_POINT ( 'NONE',  ( -5.823673210054116645, -21.52544592524344225, 22.29057627198102765 ) ) ;
#37980=CARTESIAN_POINT ( 'NONE',  ( -16.53943276465976808, -0.05219959533934237506, 108.7510903946857042 ) ) ;
#37981=CARTESIAN_POINT ( 'NONE',  ( -0.05219959533937732626, 21.53943276465977519, 77.50109039468567573 ) ) ;
#37982=CARTESIAN_POINT ( 'NONE',  ( 12.14591786802327356, -12.06949235617739191, 40.62609039468567573 ) ) ;
#37983=CARTESIAN_POINT ( 'NONE',  ( -18.67979575497193778, 10.72451020669871902, 38.33442372801900433 ) ) ;
#37984=ADVANCED_FACE ( 'NONE', ( #13867 ), #96544, .T. ) ;
#37986=CARTESIAN_POINT ( 'NONE',  ( 5.719274019375673035, 21.55341960407619339, 22.29275706135235069 ) ) ;
#37987=CARTESIAN_POINT ( 'NONE',  ( -0.05219959533910754901, -16.53943276465976808, 97.49890960531436690 ) ) ;
#37988=CARTESIAN_POINT ( 'NONE',  ( -18.56101223717332260, -5.499999999999950262, 51.44978406935678095 ) ) ;
#37989=CARTESIAN_POINT ( 'NONE',  ( -16.55341960407611168, -4.379528057220339221, 56.45724293864768839 ) ) ;
#37990=CARTESIAN_POINT ( 'NONE',  ( 19.05341960407611168, 5.049401038298154454, 28.95724293864769550 ) ) ;
#37991=CARTESIAN_POINT ( 'NONE',  ( 21.53943276465977519, -0.05219959533907433946, 43.74890960531435979 ) ) ;
#37992=CARTESIAN_POINT ( 'NONE',  ( -4.483927247898539470, -16.52544592524342804, 77.29057627198102409 ) ) ;
#37994=CARTESIAN_POINT ( 'NONE',  ( 10.72451020669898902, -18.67979575497178502, 82.91557627198103830 ) ) ;
#37995=CARTESIAN_POINT ( 'NONE',  ( -19.05341960407611168, -5.049401038298163336, 81.45724293864769550 ) ) ;
#37996=CARTESIAN_POINT ( 'NONE',  ( 0.05219959533909260263, 19.03943276465977164, 39.99890960531436690 ) ) ;
#37997=CARTESIAN_POINT ( 'NONE',  ( -19.05341960407617563, 5.049401038297882671, 98.54275706135233293 ) ) ;
#37998=CARTESIAN_POINT ( 'NONE',  ( -5.823673210054116645, -21.52544592524344225, 27.29057627198103120 ) ) ;
#37999=CARTESIAN_POINT ( 'NONE',  ( -15.72974639402176322, -15.80617190586768395, 59.37609039468568284 ) ) ;
#38000=CARTESIAN_POINT ( 'NONE',  ( -21.53943276465977519, 0.05219959533907696930, 61.24890960531435979 ) ) ;
#38001=CARTESIAN_POINT ( 'NONE',  ( 5.049401038298161559, -19.05341960407611168, 37.70724293864768839 ) ) ;
#38002=CARTESIAN_POINT ( 'NONE',  ( -5.153800228976328057, -19.02544592524343514, 77.29057627198099567 ) ) ;
#38004=CARTESIAN_POINT ( 'NONE',  ( 8.224510206698742110, 14.34966873604972548, 47.08442372801901854 ) ) ;
#38005=CARTESIAN_POINT ( 'NONE',  ( -15.72974639402176322, -15.80617190586768395, 29.37609039468568284 ) ) ;
#38006=CARTESIAN_POINT ( 'NONE',  ( -10.72451020669870658, -18.67979575497194134, 69.58442372801900433 ) ) ;
#38007=CARTESIAN_POINT ( 'NONE',  ( -21.55341960407610458, -5.719274019375992779, 21.45724293864769550 ) ) ;
#38008=CARTESIAN_POINT ( 'NONE',  ( 21.53943276465977519, -0.05219959533907433946, 88.74890960531436690 ) ) ;
#38009=CARTESIAN_POINT ( 'NONE',  ( -15.72974639402176322, -15.80617190586768395, 29.37609039468568284 ) ) ;
#38010=CARTESIAN_POINT ( 'NONE',  ( -4.483927247898782831, 16.52544592524335698, 52.70942372801902565 ) ) ;
#38011=CARTESIAN_POINT ( 'NONE',  ( 5.719274019375991003, -21.55341960407610458, 67.70724293864769550 ) ) ;
#38012=CARTESIAN_POINT ( 'NONE',  ( 13.97604488694548053, -13.89961937509957401, 25.62609039468566507 ) ) ;
#38013=CARTESIAN_POINT ( 'NONE',  ( -5.049401038298153566, 19.05341960407611168, 50.20724293864770260 ) ) ;
#38014=CARTESIAN_POINT ( 'NONE',  ( -9.474510206698964154, 16.51473224551069663, 115.4155762719810241 ) ) ;
#38015=CARTESIAN_POINT ( 'NONE',  ( -19.02544592524342804, 5.153800228976336051, 96.04057627198103830 ) ) ;
#38017=CARTESIAN_POINT ( 'NONE',  ( -9.564922557961040184, 16.46253265017147172, 67.91775706135233293 ) ) ;
#38018=CARTESIAN_POINT ( 'NONE',  ( 18.67979575497178502, 10.72451020669898547, 39.16557627198102409 ) ) ;
#38019=CARTESIAN_POINT ( 'NONE',  ( 16.52544592524335698, 4.483927247898782831, 111.4594237280190328 ) ) ;
#38020=CARTESIAN_POINT ( 'NONE',  ( 13.89961937509957401, 13.97604488694547697, 101.8760903946856331 ) ) ;
#38021=CARTESIAN_POINT ( 'NONE',  ( 16.51473224551069308, 9.474510206698969483, 24.16557627198102765 ) ) ;
#38022=CARTESIAN_POINT ( 'NONE',  ( 5.153800228976615827, -19.02544592524334988, 25.20942372801900433 ) ) ;
#38023=CARTESIAN_POINT ( 'NONE',  ( 13.89961937509957401, 13.97604488694547697, 101.8760903946856331 ) ) ;
#38024=CARTESIAN_POINT ( 'NONE',  ( 15.72974639402199770, -15.80617190586745480, 88.12390960531436690 ) ) ;
#38025=CARTESIAN_POINT ( 'NONE',  ( 5.049401038297881783, 19.05341960407617563, 62.29275706135234003 ) ) ;
#38027=CARTESIAN_POINT ( 'NONE',  ( -19.05341960407611168, -5.049401038298163336, 56.45724293864768129 ) ) ;
#38028=CARTESIAN_POINT ( 'NONE',  ( -14.29746914071049879, 8.314922557960819915, 65.83224293864769550 ) ) ;
#38029=CARTESIAN_POINT ( 'NONE',  ( -16.51473224551069308, -9.474510206698971260, 41.66557627198103120 ) ) ;
#38030=CARTESIAN_POINT ( 'NONE',  ( 16.55341960407611168, 4.379528057220329451, 58.95724293864770971 ) ) ;
#38032=CARTESIAN_POINT ( 'NONE',  ( -0.05219959533910754901, -16.53943276465976808, 32.49890960531435979 ) ) ;
#38033=CARTESIAN_POINT ( 'NONE',  ( 0.05219959533909260263, 19.03943276465977164, 59.99890960531436690 ) ) ;
#38034=CARTESIAN_POINT ( 'NONE',  ( -9.564922557961040184, 16.46253265017147172, 22.91775706135233648 ) ) ;
#38035=CARTESIAN_POINT ( 'NONE',  ( -16.52544592524335698, -4.483927247898792601, 33.95942372801901143 ) ) ;
#38036=CARTESIAN_POINT ( 'NONE',  ( -10.81492255796078084, -18.62759615963271287, 47.08224293864770260 ) ) ;
#38037=CARTESIAN_POINT ( 'NONE',  ( 15.80617190586769283, -15.72974639402175789, 105.6260903946856899 ) ) ;
#38039=CARTESIAN_POINT ( 'NONE',  ( -5.049401038298153566, 19.05341960407611168, 65.20724293864765286 ) ) ;
#38041=CARTESIAN_POINT ( 'NONE',  ( 5.153800228976335163, 19.02544592524342804, 99.79057627198102409 ) ) ;
#38043=CARTESIAN_POINT ( 'NONE',  ( 5.823673210054444382, -21.52544592524334988, 25.20942372801901854 ) ) ;
#38044=CARTESIAN_POINT ( 'NONE',  ( 12.14591786802309770, 12.06949235617756955, 99.37390960531436690 ) ) ;
#38045=CARTESIAN_POINT ( 'NONE',  ( -10.72451020669898014, 18.67979575497178502, 85.41557627198102409 ) ) ;
#38046=CARTESIAN_POINT ( 'NONE',  ( -9.564922557960796823, -16.46253265017161027, 72.08224293864770971 ) ) ;
#38047=CARTESIAN_POINT ( 'NONE',  ( -13.89961937509977652, 13.97604488694528158, 90.62390960531432427 ) ) ;
#38048=CARTESIAN_POINT ( 'NONE',  ( -15.80617190586745835, -15.72974639402198527, 111.8739096053143669 ) ) ;
#38050=CARTESIAN_POINT ( 'NONE',  ( -5.153800228976328057, -19.02544592524343514, 67.29057627198102409 ) ) ;
#38052=CARTESIAN_POINT ( 'NONE',  ( 14.29746914071049879, -8.314922557960816363, 108.3322429386477097 ) ) ;
#38053=CARTESIAN_POINT ( 'NONE',  ( 5.153800228976335163, 19.02544592524342804, 24.79057627198102765 ) ) ;
#38054=CARTESIAN_POINT ( 'NONE',  ( -13.97604488694547697, 13.89961937509957934, 93.12609039468566152 ) ) ;
#38055=CARTESIAN_POINT ( 'NONE',  ( -9.564922557960796823, -16.46253265017161027, 22.08224293864768839 ) ) ;
#38056=CARTESIAN_POINT ( 'NONE',  ( 21.52544592524334988, 5.823673210054432836, 71.45942372801901854 ) ) ;
#38057=CARTESIAN_POINT ( 'NONE',  ( 16.51473224551069308, 9.474510206698969483, 64.16557627198102409 ) ) ;
#38058=CARTESIAN_POINT ( 'NONE',  ( 21.53943276465977519, 0.05219959533937863772, 31.25109039468568639 ) ) ;
#38059=CARTESIAN_POINT ( 'NONE',  ( 21.52544592524344225, -5.823673210054117533, 113.5405762719810383 ) ) ;
#38061=CARTESIAN_POINT ( 'NONE',  ( 0.05219959533909260263, 19.03943276465977164, 74.99890960531435269 ) ) ;
#38063=CARTESIAN_POINT ( 'NONE',  ( -16.52544592524335698, -4.483927247898792601, 23.95942372801901143 ) ) ;
#38064=CARTESIAN_POINT ( 'NONE',  ( -5.719274019375978568, 21.55341960407610458, 35.20724293864768839 ) ) ;
#38065=CARTESIAN_POINT ( 'NONE',  ( 21.55341960407619695, -5.719274019375665929, 66.04275706135236135 ) ) ;
#38066=CARTESIAN_POINT ( 'NONE',  ( 16.46253265017160672, -9.564922557960803928, 113.3322429386476955 ) ) ;
#38067=CARTESIAN_POINT ( 'NONE',  ( 19.02544592524334988, 5.153800228976608722, 96.45942372801897591 ) ) ;
#38068=CARTESIAN_POINT ( 'NONE',  ( -16.51473224551069308, -9.474510206698971260, 46.66557627198102409 ) ) ;
#38069=CARTESIAN_POINT ( 'NONE',  ( -16.46253265017160317, 9.564922557960807481, 70.83224293864770971 ) ) ;
#38070=CARTESIAN_POINT ( 'NONE',  ( -16.53943276465976808, 0.05219959533911058130, 91.24890960531436690 ) ) ;
#38071=CARTESIAN_POINT ( 'NONE',  ( 13.89961937509977652, -13.97604488694527269, 108.1239096053143669 ) ) ;
#38072=CARTESIAN_POINT ( 'NONE',  ( -16.55341960407611168, -4.379528057220339221, 96.45724293864770971 ) ) ;
#38073=CARTESIAN_POINT ( 'NONE',  ( -19.05341960407611168, -5.049401038298163336, 96.45724293864769550 ) ) ;
#38074=CARTESIAN_POINT ( 'NONE',  ( -16.55341960407611168, -4.379528057220339221, 56.45724293864768839 ) ) ;
#38075=CARTESIAN_POINT ( 'NONE',  ( 0.05219959533909260263, 19.03943276465977164, 44.99890960531435979 ) ) ;
#38076=CARTESIAN_POINT ( 'NONE',  ( 15.72974639402176855, 15.80617190586768217, 51.87609039468568284 ) ) ;
#38077=CARTESIAN_POINT ( 'NONE',  ( -16.51473224551082808, 9.474510206698731452, 98.33442372801900433 ) ) ;
#38078=CARTESIAN_POINT ( 'NONE',  ( 14.34966873604960469, 8.224510206698951720, 54.16557627198103120 ) ) ;
#38079=CARTESIAN_POINT ( 'NONE',  ( 15.72974639402199770, -15.80617190586745480, 93.12390960531436690 ) ) ;
#38080=CARTESIAN_POINT ( 'NONE',  ( -18.62759615963270932, 10.81492255796079327, 45.83224293864769550 ) ) ;
#38081=CARTESIAN_POINT ( 'NONE',  ( 19.35543954521080323, 5.499999999999572786, 72.08901960356452321 ) ) ;
#38082=CARTESIAN_POINT ( 'NONE',  ( 16.55341960407611168, 4.379528057220329451, 78.95724293864769550 ) ) ;
#38084=CARTESIAN_POINT ( 'NONE',  ( 0.05219959533909260263, 19.03943276465977164, 49.99890960531435979 ) ) ;
#38085=CARTESIAN_POINT ( 'NONE',  ( -4.379528057220086978, -16.55341960407618274, 109.7927570613523613 ) ) ;
#38087=CARTESIAN_POINT ( 'NONE',  ( 8.314922557961029526, -14.29746914071037800, 95.41775706135234714 ) ) ;
#38088=CARTESIAN_POINT ( 'NONE',  ( 4.483927247898790824, -16.52544592524335698, 85.20942372801901854 ) ) ;
#38089=CARTESIAN_POINT ( 'NONE',  ( 19.03943276465977164, 0.05219959533936151252, 41.25109039468566152 ) ) ;
#38090=CARTESIAN_POINT ( 'NONE',  ( -16.62475595723694965, 7.163666690055376485, 70.52713351810469078 ) ) ;
#38091=CARTESIAN_POINT ( 'NONE',  ( 5.153800228976335163, 19.02544592524342804, 109.7905762719810099 ) ) ;
#38092=CARTESIAN_POINT ( 'NONE',  ( -13.89961937509977652, 13.97604488694528158, 90.62390960531432427 ) ) ;
#38093=CARTESIAN_POINT ( 'NONE',  ( 5.049401038298161559, -19.05341960407611168, 32.70724293864768129 ) ) ;
#38094=CARTESIAN_POINT ( 'NONE',  ( 12.06949235617757843, -12.14591786802309237, 43.12390960531435269 ) ) ;
#38096=CARTESIAN_POINT ( 'NONE',  ( 19.02544592524343514, -5.153800228976328945, 108.5405762719810383 ) ) ;
#38097=CARTESIAN_POINT ( 'NONE',  ( 0.05219959533907565091, 21.53943276465977519, 34.99890960531435979 ) ) ;
#38098=CARTESIAN_POINT ( 'NONE',  ( -8.314922557960811034, -14.29746914071050412, 87.08224293864769550 ) ) ;
#38099=CARTESIAN_POINT ( 'NONE',  ( -14.34966873604972548, 8.224510206698743886, 43.33442372801901143 ) ) ;
#38100=CARTESIAN_POINT ( 'NONE',  ( 4.379528057220339221, -16.55341960407611168, 72.70724293864769550 ) ) ;
#38102=CARTESIAN_POINT ( 'NONE',  ( -0.05219959533936034679, 19.03943276465977164, 62.50109039468566863 ) ) ;
#38103=CARTESIAN_POINT ( 'NONE',  ( -16.51473224551069308, -9.474510206698971260, 96.66557627198102409 ) ) ;
#38104=CARTESIAN_POINT ( 'NONE',  ( -19.02544592524334988, -5.153800228976617603, 83.95942372801901854 ) ) ;
#38106=CARTESIAN_POINT ( 'NONE',  ( -16.52544592524335698, -4.483927247898792601, 33.95942372801901143 ) ) ;
#38107=CARTESIAN_POINT ( 'NONE',  ( -12.06949235617739369, -12.14591786802326823, 109.3760903946857042 ) ) ;
#38108=CARTESIAN_POINT ( 'NONE',  ( -13.97604488694547697, 13.89961937509957934, 78.12609039468567573 ) ) ;
#38109=CARTESIAN_POINT ( 'NONE',  ( -10.81492255796078084, -18.62759615963271287, 32.08224293864769550 ) ) ;
#38110=CARTESIAN_POINT ( 'NONE',  ( -15.80617190586768217, 15.72974639402176855, 68.12609039468567573 ) ) ;
#38112=CARTESIAN_POINT ( 'NONE',  ( 16.46253265017146816, 9.564922557961045513, 111.6677570613523329 ) ) ;
#38113=CARTESIAN_POINT ( 'NONE',  ( 19.03943276465977164, -0.05219959533909143690, 23.74890960531435269 ) ) ;
#38114=CARTESIAN_POINT ( 'NONE',  ( 0.05219959533909260263, 19.03943276465977164, 84.99890960531436690 ) ) ;
#38116=CARTESIAN_POINT ( 'NONE',  ( -19.02544592524342804, 5.153800228976336051, 26.04057627198103120 ) ) ;
#38117=CARTESIAN_POINT ( 'NONE',  ( -12.06949235617756955, 12.14591786802309770, 85.62390960531436690 ) ) ;
#38118=CARTESIAN_POINT ( 'NONE',  ( -5.153800228976328057, -19.02544592524343514, 77.29057627198099567 ) ) ;
#38120=CARTESIAN_POINT ( 'NONE',  ( -19.03943276465977164, 0.05219959533909376836, 86.24890960531436690 ) ) ;
#38122=CARTESIAN_POINT ( 'NONE',  ( 9.564922557961047289, -16.46253265017146816, 90.41775706135234714 ) ) ;
#38123=CARTESIAN_POINT ( 'NONE',  ( 21.55341960407610458, 5.719274019375980345, 73.95724293864769550 ) ) ;
#38124=CARTESIAN_POINT ( 'NONE',  ( -9.474510206698964154, 16.51473224551069663, 30.41557627198102054 ) ) ;
#38125=CARTESIAN_POINT ( 'NONE',  ( -16.51473224551082808, 9.474510206698731452, 68.33442372801900433 ) ) ;
#38126=CARTESIAN_POINT ( 'NONE',  ( -10.72451020669898014, 18.67979575497178502, 115.4155762719810241 ) ) ;
#38127=CARTESIAN_POINT ( 'NONE',  ( 9.474510206698971260, -16.51473224551069308, 67.91557627198102409 ) ) ;
#38128=CARTESIAN_POINT ( 'NONE',  ( -19.02544592524342804, 5.153800228976336051, 106.0405762719810241 ) ) ;
#38129=ORIENTED_EDGE ( 'NONE', *, *, #35651, .F. ) ;
#38131=CARTESIAN_POINT ( 'NONE',  ( -21.52544592524343514, 5.823673210054127303, 101.0405762719810383 ) ) ;
#38132=CARTESIAN_POINT ( 'NONE',  ( 0.05219959533910956823, 16.53943276465976808, 94.99890960531436690 ) ) ;
#38133=CARTESIAN_POINT ( 'NONE',  ( 13.97604488694527802, 13.89961937509977652, 84.37390960531433848 ) ) ;
#38134=CARTESIAN_POINT ( 'NONE',  ( -5.153800228976607833, 19.02544592524334988, 62.70942372801899722 ) ) ;
#38135=CARTESIAN_POINT ( 'NONE',  ( -21.53943276465977519, 0.05219959533907696930, 91.24890960531436690 ) ) ;
#38136=CARTESIAN_POINT ( 'NONE',  ( 18.62759615963271287, -10.81492255796078972, 68.33224293864769550 ) ) ;
#38137=CARTESIAN_POINT ( 'NONE',  ( -16.55341960407611168, -4.379528057220339221, 41.45724293864769550 ) ) ;
#38138=CARTESIAN_POINT ( 'NONE',  ( -9.564922557961040184, 16.46253265017147172, 27.91775706135232582 ) ) ;
#38139=CARTESIAN_POINT ( 'NONE',  ( 12.06949235617739724, 12.14591786802326823, 66.87609039468568994 ) ) ;
#38140=CARTESIAN_POINT ( 'NONE',  ( 5.153800228976335163, 19.02544592524342804, 94.79057627198103830 ) ) ;
#38141=CARTESIAN_POINT ( 'NONE',  ( 19.05341960407611168, 5.049401038298154454, 43.95724293864769550 ) ) ;
#38142=CARTESIAN_POINT ( 'NONE',  ( -0.05219959533937732626, 21.53943276465977519, 47.50109039468568994 ) ) ;
#38143=CARTESIAN_POINT ( 'NONE',  ( -18.67979575497193778, 10.72451020669871902, 53.33442372801901854 ) ) ;
#38144=CARTESIAN_POINT ( 'NONE',  ( -13.97604488694527625, -13.89961937509977652, 61.87390960531435979 ) ) ;
#38145=CARTESIAN_POINT ( 'NONE',  ( -21.53943276465977519, -0.05219959533937600094, 38.75109039468567573 ) ) ;
#38146=CARTESIAN_POINT ( 'NONE',  ( -19.02544592524334988, -5.153800228976617603, 78.95942372801900433 ) ) ;
#38147=CARTESIAN_POINT ( 'NONE',  ( 13.97604488694548053, -13.89961937509957401, 70.62609039468567573 ) ) ;
#38148=CARTESIAN_POINT ( 'NONE',  ( -13.89961937509977652, 13.97604488694528158, 40.62390960531435979 ) ) ;
#38149=CARTESIAN_POINT ( 'NONE',  ( -12.14591786802326823, 12.06949235617739902, 83.12609039468568994 ) ) ;
#38150=CARTESIAN_POINT ( 'NONE',  ( -19.03943276465977164, 0.05219959533909376836, 56.24890960531435979 ) ) ;
#38152=CARTESIAN_POINT ( 'NONE',  ( 13.89961937509977652, -13.97604488694527269, 103.1239096053143527 ) ) ;
#38153=CARTESIAN_POINT ( 'NONE',  ( -5.049401038298153566, 19.05341960407611168, 35.20724293864768839 ) ) ;
#38154=CARTESIAN_POINT ( 'NONE',  ( 5.823673210054125526, 21.52544592524343514, 79.79057627198102409 ) ) ;
#38155=CARTESIAN_POINT ( 'NONE',  ( 4.483927247898790824, -16.52544592524335698, 55.20942372801902565 ) ) ;
#38156=CARTESIAN_POINT ( 'NONE',  ( 19.02544592524334988, 5.153800228976608722, 21.45942372801899012 ) ) ;
#38157=CARTESIAN_POINT ( 'NONE',  ( -9.474510206698964154, 16.51473224551069663, 55.41557627198103120 ) ) ;
#38158=CARTESIAN_POINT ( 'NONE',  ( 4.379528057220339221, -16.55341960407611168, 47.70724293864770260 ) ) ;
#38159=CARTESIAN_POINT ( 'NONE',  ( 16.53943276465976808, -0.05219959533910856209, 83.74890960531435269 ) ) ;
#38160=CARTESIAN_POINT ( 'NONE',  ( 19.03943276465977164, -0.05219959533909143690, 73.74890960531435269 ) ) ;
#38161=CARTESIAN_POINT ( 'NONE',  ( 5.823673210054444382, -21.52544592524334988, 40.20942372801901854 ) ) ;
#38162=CARTESIAN_POINT ( 'NONE',  ( 19.02544592524343514, -5.153800228976328945, 98.54057627198100988 ) ) ;
#38163=CARTESIAN_POINT ( 'NONE',  ( 10.81492255796106328, -18.62759615963255655, 105.4177570613523613 ) ) ;
#38164=CARTESIAN_POINT ( 'NONE',  ( 4.483927247898790824, -16.52544592524335698, 70.20942372801904696 ) ) ;
#38165=CARTESIAN_POINT ( 'NONE',  ( -0.05219959533937732626, 21.53943276465977519, 27.50109039468567929 ) ) ;
#38166=CARTESIAN_POINT ( 'NONE',  ( 5.049401038298161559, -19.05341960407611168, 107.7072429386476955 ) ) ;
#38167=CARTESIAN_POINT ( 'NONE',  ( -21.55341960407610458, -5.719274019375992779, 91.45724293864769550 ) ) ;
#38168=CARTESIAN_POINT ( 'NONE',  ( -0.05219959533910754901, -16.53943276465976808, 47.49890960531435979 ) ) ;
#38169=CARTESIAN_POINT ( 'NONE',  ( 16.51473224551069308, 9.474510206698969483, 39.16557627198103120 ) ) ;
#38170=CARTESIAN_POINT ( 'NONE',  ( 14.34966873604960469, 8.224510206698951720, 74.16557627198102409 ) ) ;
#38171=CARTESIAN_POINT ( 'NONE',  ( 5.823673210054125526, 21.52544592524343514, 24.79057627198103120 ) ) ;
#38172=CARTESIAN_POINT ( 'NONE',  ( 9.474510206698729675, 16.51473224551082808, 32.08442372801900433 ) ) ;
#38173=CARTESIAN_POINT ( 'NONE',  ( -14.34966873604960291, -8.224510206698953496, 106.6655762719810383 ) ) ;
#38174=CARTESIAN_POINT ( 'NONE',  ( 13.89961937509977652, -13.97604488694527269, 113.1239096053143527 ) ) ;
#38176=CARTESIAN_POINT ( 'NONE',  ( -14.34966873604972548, 8.224510206698743886, 58.33442372801901143 ) ) ;
#38177=CARTESIAN_POINT ( 'NONE',  ( -13.89961937509977652, 13.97604488694528158, 50.62390960531435979 ) ) ;
#38179=CARTESIAN_POINT ( 'NONE',  ( -12.06949235617739369, -12.14591786802326823, 99.37609039468568994 ) ) ;
#38180=CARTESIAN_POINT ( 'NONE',  ( -9.474510206698720793, -16.51473224551083518, 94.58442372801900433 ) ) ;
#38181=CARTESIAN_POINT ( 'NONE',  ( -18.62759615963255300, -10.81492255796106328, 74.16775706135231871 ) ) ;
#38182=CARTESIAN_POINT ( 'NONE',  ( 13.89961937509977652, -13.97604488694527269, 68.12390960531436690 ) ) ;
#38183=CARTESIAN_POINT ( 'NONE',  ( -0.05219959533907301413, -21.53943276465977519, 87.49890960531436690 ) ) ;
#38184=CARTESIAN_POINT ( 'NONE',  ( 16.53943276465976808, 0.05219959533934440121, 46.25109039468567573 ) ) ;
#38185=CARTESIAN_POINT ( 'NONE',  ( -16.53943276465976808, 0.05219959533911058130, 106.2489096053143811 ) ) ;
#38186=CARTESIAN_POINT ( 'NONE',  ( 5.049401038297881783, 19.05341960407617563, 77.29275706135231871 ) ) ;
#38187=CARTESIAN_POINT ( 'NONE',  ( 5.823673210054125526, 21.52544592524343514, 79.79057627198102409 ) ) ;
#38188=CARTESIAN_POINT ( 'NONE',  ( -16.46253265017146816, -9.564922557961047289, 54.16775706135234003 ) ) ;
#38189=CARTESIAN_POINT ( 'NONE',  ( 19.03943276465977164, -0.05219959533909143690, 113.7489096053143669 ) ) ;
#38190=CARTESIAN_POINT ( 'NONE',  ( 18.67979575497178502, 10.72451020669898547, 84.16557627198103830 ) ) ;
#38191=CARTESIAN_POINT ( 'NONE',  ( 17.49999999999998934, 4.640572885337633124, 26.86211835451159757 ) ) ;
#38192=CARTESIAN_POINT ( 'NONE',  ( 16.51473224551069308, 9.474510206698969483, 69.16557627198102409 ) ) ;
#38194=CARTESIAN_POINT ( 'NONE',  ( 4.483927247898790824, -16.52544592524335698, 25.20942372801901854 ) ) ;
#38196=CARTESIAN_POINT ( 'NONE',  ( 5.153800228976335163, 19.02544592524342804, 44.79057627198103830 ) ) ;
#38197=CARTESIAN_POINT ( 'NONE',  ( 21.52544592524344225, -5.823673210054117533, 103.5405762719810383 ) ) ;
#38198=CARTESIAN_POINT ( 'NONE',  ( -16.52544592524342804, 4.483927247898546575, 56.04057627198102409 ) ) ;
#38199=CARTESIAN_POINT ( 'NONE',  ( -16.46253265017160317, 9.564922557960807481, 70.83224293864770971 ) ) ;
#38200=CARTESIAN_POINT ( 'NONE',  ( 10.81492255796106328, -18.62759615963255655, 80.41775706135234714 ) ) ;
#38201=CARTESIAN_POINT ( 'NONE',  ( 12.06949235617739724, 12.14591786802326823, 21.87609039468567573 ) ) ;
#38202=CARTESIAN_POINT ( 'NONE',  ( -19.02544592524334988, -5.153800228976617603, 33.95942372801897591 ) ) ;
#38203=CARTESIAN_POINT ( 'NONE',  ( -18.62759615963255300, -10.81492255796106328, 39.16775706135235424 ) ) ;
#38204=CARTESIAN_POINT ( 'NONE',  ( -0.05219959533907301413, -21.53943276465977519, 107.4989096053143669 ) ) ;
#38205=CARTESIAN_POINT ( 'NONE',  ( -18.62759615963270932, 10.81492255796079327, 55.83224293864770260 ) ) ;
#38206=CARTESIAN_POINT ( 'NONE',  ( 16.46253265017146816, 9.564922557961045513, 96.66775706135233293 ) ) ;
#38207=CARTESIAN_POINT ( 'NONE',  ( -16.51473224551082808, 9.474510206698731452, 63.33442372801900433 ) ) ;
#38208=CARTESIAN_POINT ( 'NONE',  ( -15.80617190586768217, 15.72974639402176855, 83.12609039468568994 ) ) ;
#38209=CARTESIAN_POINT ( 'NONE',  ( 19.03943276465977164, 0.05219959533936151252, 56.25109039468566863 ) ) ;
#38210=CARTESIAN_POINT ( 'NONE',  ( 19.05341960407611168, 5.049401038298154454, 28.95724293864769550 ) ) ;
#38211=CARTESIAN_POINT ( 'NONE',  ( 5.823673210054125526, 21.52544592524343514, 54.79057627198104541 ) ) ;
#38212=CARTESIAN_POINT ( 'NONE',  ( 12.14591786802309770, 12.06949235617756955, 44.37390960531435979 ) ) ;
#38214=CARTESIAN_POINT ( 'NONE',  ( 19.03943276465977164, 0.05219959533936151252, 26.25109039468566507 ) ) ;
#38215=CARTESIAN_POINT ( 'NONE',  ( -4.379528057220086978, -16.55341960407618274, 89.79275706135236135 ) ) ;
#38216=CARTESIAN_POINT ( 'NONE',  ( 0.05219959533910956823, 16.53943276465976808, 34.99890960531435979 ) ) ;
#38217=CARTESIAN_POINT ( 'NONE',  ( 18.62759615963255655, 10.81492255796105972, 81.66775706135236135 ) ) ;
#38218=CARTESIAN_POINT ( 'NONE',  ( 21.55341960407619695, -5.719274019375665929, 76.04275706135237556 ) ) ;
#38219=CARTESIAN_POINT ( 'NONE',  ( 10.72451020669898902, -18.67979575497178502, 87.91557627198103830 ) ) ;
#38220=EDGE_CURVE ( 'NONE', #49306, #101016, #167681, .T. ) ;
#38221=CARTESIAN_POINT ( 'NONE',  ( -9.564922557960796823, -16.46253265017161027, 42.08224293864769550 ) ) ;
#38222=CARTESIAN_POINT ( 'NONE',  ( 10.81492255796106328, -18.62759615963255655, 50.41775706135235424 ) ) ;
#38223=CARTESIAN_POINT ( 'NONE',  ( -19.05341960407611168, -5.049401038298163336, 41.45724293864769550 ) ) ;
#38224=CARTESIAN_POINT ( 'NONE',  ( -16.46253265017160317, 9.564922557960807481, 45.83224293864769550 ) ) ;
#38225=CARTESIAN_POINT ( 'NONE',  ( -16.53943276465976808, 0.05219959533911058130, 91.24890960531436690 ) ) ;
#38226=CARTESIAN_POINT ( 'NONE',  ( -5.049401038298153566, 19.05341960407611168, 105.2072429386476671 ) ) ;
#38227=CARTESIAN_POINT ( 'NONE',  ( 14.29746914071049879, -8.314922557960816363, 38.33224293864768839 ) ) ;
#38228=CARTESIAN_POINT ( 'NONE',  ( 14.29746914071049879, -8.314922557960816363, 113.3322429386476955 ) ) ;
#38229=CARTESIAN_POINT ( 'NONE',  ( -10.81492255796078084, -18.62759615963271287, 87.08224293864769550 ) ) ;
#38230=CARTESIAN_POINT ( 'NONE',  ( 21.52544592524334988, 5.823673210054432836, 26.45942372801901854 ) ) ;
#38232=CARTESIAN_POINT ( 'NONE',  ( 12.06949235617739724, 12.14591786802326823, 31.87609039468567929 ) ) ;
#38233=CARTESIAN_POINT ( 'NONE',  ( -18.67979575497178146, -10.72451020669898902, 76.66557627198103830 ) ) ;
#38234=CARTESIAN_POINT ( 'NONE',  ( 18.67979575497194134, -10.72451020669871369, 95.83442372801903275 ) ) ;
#38235=CARTESIAN_POINT ( 'NONE',  ( 19.05341960407611168, 5.049401038298154454, 93.95724293864769550 ) ) ;
#38236=CARTESIAN_POINT ( 'NONE',  ( -10.72451020669870658, -18.67979575497194134, 34.58442372801900433 ) ) ;
#38237=CARTESIAN_POINT ( 'NONE',  ( -21.52544592524343514, 5.823673210054127303, 31.04057627198102409 ) ) ;
#38238=CARTESIAN_POINT ( 'NONE',  ( -14.34966873604972548, 8.224510206698743886, 93.33442372801901854 ) ) ;
#38239=CARTESIAN_POINT ( 'NONE',  ( 15.80617190586769283, -15.72974639402175789, 65.62609039468568994 ) ) ;
#38240=CARTESIAN_POINT ( 'NONE',  ( 21.52544592524334988, 5.823673210054432836, 111.4594237280190328 ) ) ;
#38241=CARTESIAN_POINT ( 'NONE',  ( 4.379528057220092307, 16.55341960407617563, 72.29275706135236135 ) ) ;
#38242=CARTESIAN_POINT ( 'NONE',  ( -21.52544592524334988, -5.823673210054445271, 28.95942372801902209 ) ) ;
#38243=CARTESIAN_POINT ( 'NONE',  ( 13.97604488694527802, 13.89961937509977652, 29.37390960531435979 ) ) ;
#38244=CARTESIAN_POINT ( 'NONE',  ( -10.72451020669870658, -18.67979575497194134, 109.5844237280190328 ) ) ;
#38245=CARTESIAN_POINT ( 'NONE',  ( 5.049401038298161559, -19.05341960407611168, 112.7072429386476813 ) ) ;
#38246=CARTESIAN_POINT ( 'NONE',  ( -21.53943276465977519, 0.05219959533907696930, 106.2489096053143811 ) ) ;
#38248=CARTESIAN_POINT ( 'NONE',  ( 0.05219959533907565091, 21.53943276465977519, 59.99890960531436690 ) ) ;
#38249=CARTESIAN_POINT ( 'NONE',  ( 12.06949235617739724, 12.14591786802326823, 51.87609039468568284 ) ) ;
#38250=CARTESIAN_POINT ( 'NONE',  ( 12.06949235617757843, -12.14591786802309237, 53.12390960531436690 ) ) ;
#38252=CARTESIAN_POINT ( 'NONE',  ( 13.89961937509957401, 13.97604488694547697, 81.87609039468564731 ) ) ;
#38254=CARTESIAN_POINT ( 'NONE',  ( -16.31925111598457079, 7.325300261831521276, 105.1642453896725300 ) ) ;
#38255=CARTESIAN_POINT ( 'NONE',  ( 19.03943276465977164, 0.05219959533936151252, 106.2510903946856615 ) ) ;
#38256=CARTESIAN_POINT ( 'NONE',  ( 15.72974639402199770, -15.80617190586745480, 88.12390960531436690 ) ) ;
#38257=CARTESIAN_POINT ( 'NONE',  ( -8.224510206698948167, 14.34966873604960824, 70.41557627198102409 ) ) ;
#38258=CARTESIAN_POINT ( 'NONE',  ( 13.89961937509977652, -13.97604488694527269, 98.12390960531433848 ) ) ;
#38259=CARTESIAN_POINT ( 'NONE',  ( 4.379528057220092307, 16.55341960407617563, 47.29275706135234003 ) ) ;
#38260=CARTESIAN_POINT ( 'NONE',  ( 13.89961937509977652, -13.97604488694527269, 58.12390960531436690 ) ) ;
#38261=CARTESIAN_POINT ( 'NONE',  ( 10.72451020669871369, 18.67979575497193778, 32.08442372801901854 ) ) ;
#38262=CARTESIAN_POINT ( 'NONE',  ( 9.474510206698729675, 16.51473224551082808, 92.08442372801900433 ) ) ;
#38263=CARTESIAN_POINT ( 'NONE',  ( -19.03943276465977164, 0.05219959533909376836, 101.2489096053143669 ) ) ;
#38264=CARTESIAN_POINT ( 'NONE',  ( 9.564922557960805705, 16.46253265017160317, 84.58224293864769550 ) ) ;
#38265=CARTESIAN_POINT ( 'NONE',  ( -15.72974639402197994, 15.80617190586746368, 85.62390960531436690 ) ) ;
#38266=CARTESIAN_POINT ( 'NONE',  ( 5.049401038298161559, -19.05341960407611168, 47.70724293864770260 ) ) ;
#38267=CARTESIAN_POINT ( 'NONE',  ( -16.52216118717207394, -7.221426719304526287, 61.07599021046993215 ) ) ;
#38268=CARTESIAN_POINT ( 'NONE',  ( -4.379528057220328563, 16.55341960407611168, 65.20724293864768129 ) ) ;
#38269=CARTESIAN_POINT ( 'NONE',  ( 16.51473224551069308, 9.474510206698969483, 104.1655762719810241 ) ) ;
#38271=CARTESIAN_POINT ( 'NONE',  ( -19.03943276465977164, -0.05219959533935918106, 68.75109039468566152 ) ) ;
#38272=CARTESIAN_POINT ( 'NONE',  ( -21.53943276465977519, 0.05219959533907696930, 91.24890960531436690 ) ) ;
#38273=CARTESIAN_POINT ( 'NONE',  ( -13.89961937509957401, -13.97604488694547875, 54.37609039468565442 ) ) ;
#38274=CARTESIAN_POINT ( 'NONE',  ( 16.51473224551069308, 9.474510206698969483, 99.16557627198102409 ) ) ;
#38275=CARTESIAN_POINT ( 'NONE',  ( 19.19724070472096145, 5.499999999999974243, 68.56193348274381094 ) ) ;
#38276=CARTESIAN_POINT ( 'NONE',  ( 21.52544592524344225, -5.823673210054117533, 38.54057627198103120 ) ) ;
#38277=CARTESIAN_POINT ( 'NONE',  ( -19.02544592524342804, 5.153800228976336051, 91.04057627198100988 ) ) ;
#38278=CARTESIAN_POINT ( 'NONE',  ( 10.81492255796106328, -18.62759615963255655, 60.41775706135235424 ) ) ;
#38279=CARTESIAN_POINT ( 'NONE',  ( 16.51473224551069308, 9.474510206698969483, 39.16557627198103120 ) ) ;
#38280=CARTESIAN_POINT ( 'NONE',  ( 8.314922557960818139, 14.29746914071049879, 79.58224293864769550 ) ) ;
#38281=CARTESIAN_POINT ( 'NONE',  ( 4.483927247898790824, -16.52544592524335698, 25.20942372801901854 ) ) ;
#38282=CARTESIAN_POINT ( 'NONE',  ( 21.53943276465977519, 0.05219959533937863772, 56.25109039468568284 ) ) ;
#38283=VERTEX_POINT ( 'NONE', #154281 ) ;
#38284=CARTESIAN_POINT ( 'NONE',  ( 13.97604488694527802, 13.89961937509977652, 114.3739096053143669 ) ) ;
#38285=CARTESIAN_POINT ( 'NONE',  ( 9.474510206698729675, 16.51473224551082808, 67.08442372801900433 ) ) ;
#38287=CARTESIAN_POINT ( 'NONE',  ( -10.72451020669870658, -18.67979575497194134, 24.58442372801901499 ) ) ;
#38289=CARTESIAN_POINT ( 'NONE',  ( 5.153800228976615827, -19.02544592524334988, 25.20942372801900433 ) ) ;
#38290=CARTESIAN_POINT ( 'NONE',  ( -19.02544592524342804, 5.153800228976336051, 61.04057627198103120 ) ) ;
#38291=CARTESIAN_POINT ( 'NONE',  ( -5.823673210054431948, 21.52544592524334988, 112.7094237280190328 ) ) ;
#38292=CARTESIAN_POINT ( 'NONE',  ( -4.483927247898782831, 16.52544592524335698, 107.7094237280190328 ) ) ;
#38293=CARTESIAN_POINT ( 'NONE',  ( 19.03943276465977164, -0.05219959533909143690, 103.7489096053143669 ) ) ;
#38294=CARTESIAN_POINT ( 'NONE',  ( -18.62759615963255300, -10.81492255796106328, 79.16775706135234714 ) ) ;
#38298=CARTESIAN_POINT ( 'NONE',  ( -4.483927247898782831, 16.52544592524335698, 72.70942372801901854 ) ) ;
#38299=CARTESIAN_POINT ( 'NONE',  ( 21.52544592524334988, 5.823673210054432836, 66.45942372801903275 ) ) ;
#38300=CARTESIAN_POINT ( 'NONE',  ( -21.55341960407619339, 5.719274019375674811, 108.5427570613523756 ) ) ;
#38302=CARTESIAN_POINT ( 'NONE',  ( 9.474510206698971260, -16.51473224551069308, 87.91557627198102409 ) ) ;
#38303=CARTESIAN_POINT ( 'NONE',  ( 19.03943276465977164, -0.05219959533909143690, 113.7489096053143669 ) ) ;
#38306=CARTESIAN_POINT ( 'NONE',  ( -9.474510206698964154, 16.51473224551069663, 40.41557627198103120 ) ) ;
#38307=CARTESIAN_POINT ( 'NONE',  ( -10.72451020669898014, 18.67979575497178502, 40.41557627198103120 ) ) ;
#38308=CARTESIAN_POINT ( 'NONE',  ( 12.06949235617739724, 12.14591786802326823, 111.8760903946856615 ) ) ;
#38309=CARTESIAN_POINT ( 'NONE',  ( -16.55341960407611168, -4.379528057220339221, 96.45724293864770971 ) ) ;
#38310=CARTESIAN_POINT ( 'NONE',  ( 13.97604488694527802, 13.89961937509977652, 84.37390960531433848 ) ) ;
#38311=CARTESIAN_POINT ( 'NONE',  ( -0.05219959533937732626, 21.53943276465977519, 102.5010903946856899 ) ) ;
#38312=CARTESIAN_POINT ( 'NONE',  ( 19.02544592524343514, -5.153800228976328945, 33.54057627198102409 ) ) ;
#38313=CARTESIAN_POINT ( 'NONE',  ( 12.06949235617757843, -12.14591786802309237, 88.12390960531436690 ) ) ;
#38314=CARTESIAN_POINT ( 'NONE',  ( -18.62759615963255300, -10.81492255796106328, 54.16775706135235424 ) ) ;
#38315=CARTESIAN_POINT ( 'NONE',  ( 5.823673210054125526, 21.52544592524343514, 84.79057627198102409 ) ) ;
#38316=CARTESIAN_POINT ( 'NONE',  ( 9.474510206698729675, 16.51473224551082808, 57.08442372801900433 ) ) ;
#38317=CARTESIAN_POINT ( 'NONE',  ( -18.22780087662121673, -5.500000000000062172, 46.48459894673893444 ) ) ;
#38318=CARTESIAN_POINT ( 'NONE',  ( -16.46253265017160317, 9.564922557960807481, 90.83224293864769550 ) ) ;
#38319=CARTESIAN_POINT ( 'NONE',  ( 4.379528057220339221, -16.55341960407611168, 62.70724293864769550 ) ) ;
#38320=CARTESIAN_POINT ( 'NONE',  ( 0.05219959533936267826, -19.03943276465977164, 50.00109039468566863 ) ) ;
#38321=CARTESIAN_POINT ( 'NONE',  ( 0.05219959533910956823, 16.53943276465976808, 44.99890960531435979 ) ) ;
#38322=CARTESIAN_POINT ( 'NONE',  ( 9.474510206698729675, 16.51473224551082808, 77.08442372801900433 ) ) ;
#38323=CARTESIAN_POINT ( 'NONE',  ( -18.62759615963270932, 10.81492255796079327, 40.83224293864769550 ) ) ;
#38324=CARTESIAN_POINT ( 'NONE',  ( 12.06949235617757843, -12.14591786802309237, 103.1239096053143811 ) ) ;
#38326=CARTESIAN_POINT ( 'NONE',  ( -13.89961937509977652, 13.97604488694528158, 40.62390960531435979 ) ) ;
#38327=CARTESIAN_POINT ( 'NONE',  ( 21.55341960407610458, 5.719274019375980345, 43.95724293864769550 ) ) ;
#38328=CARTESIAN_POINT ( 'NONE',  ( 13.89961937509977652, -13.97604488694527269, 28.12390960531435624 ) ) ;
#38329=CARTESIAN_POINT ( 'NONE',  ( -16.55341960407617563, 4.379528057220093196, 78.54275706135236135 ) ) ;
#38330=CARTESIAN_POINT ( 'NONE',  ( -19.05341960407611168, -5.049401038298163336, 61.45724293864769550 ) ) ;
#38331=CARTESIAN_POINT ( 'NONE',  ( 19.05341960407617918, -5.049401038297876454, 41.04275706135233293 ) ) ;
#38332=CARTESIAN_POINT ( 'NONE',  ( -10.81492255796105439, 18.62759615963255655, 72.91775706135234714 ) ) ;
#38333=CARTESIAN_POINT ( 'NONE',  ( -18.67979575497178146, -10.72451020669898902, 46.66557627198102409 ) ) ;
#38334=CARTESIAN_POINT ( 'NONE',  ( -19.03943276465977164, 0.05219959533909376836, 26.24890960531435624 ) ) ;
#38335=CARTESIAN_POINT ( 'NONE',  ( -16.51473224551082808, 9.474510206698731452, 98.33442372801900433 ) ) ;
#38337=CARTESIAN_POINT ( 'NONE',  ( 17.50000000000001421, 3.385507783989948560, 37.35538298664832979 ) ) ;
#38338=CARTESIAN_POINT ( 'NONE',  ( -21.55341960407610458, -5.719274019375992779, 41.45724293864769550 ) ) ;
#38339=CARTESIAN_POINT ( 'NONE',  ( 9.474510206698971260, -16.51473224551069308, 27.91557627198103120 ) ) ;
#38340=CARTESIAN_POINT ( 'NONE',  ( 15.80617190586769283, -15.72974639402175789, 80.62609039468567573 ) ) ;
#38341=CARTESIAN_POINT ( 'NONE',  ( 14.29746914071049879, -8.314922557960816363, 43.33224293864769550 ) ) ;
#38342=CARTESIAN_POINT ( 'NONE',  ( -14.34966873604960291, -8.224510206698953496, 56.66557627198103830 ) ) ;
#38343=CARTESIAN_POINT ( 'NONE',  ( -18.67979575497178146, -10.72451020669898902, 81.66557627198103830 ) ) ;
#38344=CARTESIAN_POINT ( 'NONE',  ( 21.55341960407610458, 5.719274019375980345, 78.95724293864769550 ) ) ;
#38346=CARTESIAN_POINT ( 'NONE',  ( 10.81492255796078972, 18.62759615963270932, 29.58224293864769905 ) ) ;
#38348=CARTESIAN_POINT ( 'NONE',  ( 16.53943276465976808, 0.05219959533934440121, 51.25109039468568994 ) ) ;
#38349=CARTESIAN_POINT ( 'NONE',  ( -0.05219959533910754901, -16.53943276465976808, 82.49890960531436690 ) ) ;
#38350=CARTESIAN_POINT ( 'NONE',  ( -19.05341960407611168, -5.049401038298163336, 66.45724293864769550 ) ) ;
#38351=CARTESIAN_POINT ( 'NONE',  ( -9.564922557960796823, -16.46253265017161027, 37.08224293864768839 ) ) ;
#38352=CARTESIAN_POINT ( 'NONE',  ( 18.22780087662121673, 5.500000000000056843, 48.98459894673892734 ) ) ;
#38354=CARTESIAN_POINT ( 'NONE',  ( -4.483927247898782831, 16.52544592524335698, 77.70942372801900433 ) ) ;
#38355=CARTESIAN_POINT ( 'NONE',  ( -5.719274019375665041, -21.55341960407619695, 19.79275706135235069 ) ) ;
#38356=CARTESIAN_POINT ( 'NONE',  ( -19.05341960407611168, -5.049401038298163336, 86.45724293864769550 ) ) ;
#38357=CARTESIAN_POINT ( 'NONE',  ( 5.719274019375673035, 21.55341960407619339, 57.29275706135234714 ) ) ;
#38358=CARTESIAN_POINT ( 'NONE',  ( 19.03943276465977164, -0.05219959533909143690, 108.7489096053143527 ) ) ;
#38361=CARTESIAN_POINT ( 'NONE',  ( -15.72974639402176322, -15.80617190586768395, 39.37609039468567573 ) ) ;
#38362=CARTESIAN_POINT ( 'NONE',  ( 0.05219959533909260263, 19.03943276465977164, 24.99890960531435269 ) ) ;
#38363=CARTESIAN_POINT ( 'NONE',  ( -19.05341960407611168, -5.049401038298163336, 101.4572429386476955 ) ) ;
#38364=CARTESIAN_POINT ( 'NONE',  ( -19.05341960407617563, 5.049401038297882671, 58.54275706135234003 ) ) ;
#38365=CARTESIAN_POINT ( 'NONE',  ( 21.53943276465977519, -0.05219959533907433946, 108.7489096053143669 ) ) ;
#38366=CARTESIAN_POINT ( 'NONE',  ( 13.97604488694548053, -13.89961937509957401, 45.62609039468566863 ) ) ;
#38367=CARTESIAN_POINT ( 'NONE',  ( 5.153800228976335163, 19.02544592524342804, 24.79057627198102765 ) ) ;
#38368=CARTESIAN_POINT ( 'NONE',  ( -16.53943276465976808, -0.05219959533934237506, 93.75109039468567573 ) ) ;
#38369=CARTESIAN_POINT ( 'NONE',  ( 13.89961937509957401, 13.97604488694547697, 61.87609039468566863 ) ) ;
#38370=CARTESIAN_POINT ( 'NONE',  ( -16.52544592524335698, -4.483927247898792601, 98.95942372801903275 ) ) ;
#38373=CARTESIAN_POINT ( 'NONE',  ( -19.02544592524342804, 5.153800228976336051, 91.04057627198100988 ) ) ;
#38374=CARTESIAN_POINT ( 'NONE',  ( -10.72451020669870658, -18.67979575497194134, 89.58442372801901854 ) ) ;
#38375=CARTESIAN_POINT ( 'NONE',  ( -18.67979575497193778, 10.72451020669871902, 93.33442372801901854 ) ) ;
#38377=CARTESIAN_POINT ( 'NONE',  ( 13.97604488694527802, 13.89961937509977652, 104.3739096053143385 ) ) ;
#38378=CARTESIAN_POINT ( 'NONE',  ( 5.823673210054444382, -21.52544592524334988, 80.20942372801901854 ) ) ;
#38379=CARTESIAN_POINT ( 'NONE',  ( -5.049401038297874678, -19.05341960407617918, 109.7927570613523187 ) ) ;
#38380=CARTESIAN_POINT ( 'NONE',  ( -5.153800228976328057, -19.02544592524343514, 82.29057627198103830 ) ) ;
#38381=CARTESIAN_POINT ( 'NONE',  ( -5.719274019375978568, 21.55341960407610458, 35.20724293864768839 ) ) ;
#38382=CARTESIAN_POINT ( 'NONE',  ( 19.03943276465977164, -0.05219959533909143690, 98.74890960531436690 ) ) ;
#38384=CARTESIAN_POINT ( 'NONE',  ( 16.51473224551069308, 9.474510206698969483, 74.16557627198103830 ) ) ;
#38385=CARTESIAN_POINT ( 'NONE',  ( 13.97604488694527802, 13.89961937509977652, 64.37390960531436690 ) ) ;
#38386=CARTESIAN_POINT ( 'NONE',  ( -12.06949235617739369, -12.14591786802326823, 94.37609039468568994 ) ) ;
#38388=CARTESIAN_POINT ( 'NONE',  ( -19.02544592524334988, -5.153800228976617603, 58.95942372801900433 ) ) ;
#38389=CARTESIAN_POINT ( 'NONE',  ( -19.02544592524342804, 5.153800228976336051, 96.04057627198103830 ) ) ;
#38390=CARTESIAN_POINT ( 'NONE',  ( -16.55341960407611168, -4.379528057220339221, 86.45724293864770971 ) ) ;
#38391=CARTESIAN_POINT ( 'NONE',  ( -21.52544592524343514, 5.823673210054127303, 36.04057627198102409 ) ) ;
#38392=CARTESIAN_POINT ( 'NONE',  ( 13.89961937509977652, -13.97604488694527269, 113.1239096053143527 ) ) ;
#38393=CARTESIAN_POINT ( 'NONE',  ( -12.06949235617756955, 12.14591786802309770, 95.62390960531436690 ) ) ;
#38395=CARTESIAN_POINT ( 'NONE',  ( 13.89961937509957401, 13.97604488694547697, 46.87609039468565442 ) ) ;
#38396=CARTESIAN_POINT ( 'NONE',  ( -16.53943276465976808, 0.05219959533911058130, 21.24890960531436690 ) ) ;
#38397=CARTESIAN_POINT ( 'NONE',  ( 19.02544592524343514, -5.153800228976328945, 108.5405762719810383 ) ) ;
#38398=CARTESIAN_POINT ( 'NONE',  ( 5.719274019375673035, 21.55341960407619339, 67.29275706135234714 ) ) ;
#38399=CARTESIAN_POINT ( 'NONE',  ( -10.81492255796078084, -18.62759615963271287, 52.08224293864768839 ) ) ;
#38400=CARTESIAN_POINT ( 'NONE',  ( 10.72451020669871369, 18.67979575497193778, 37.08442372801901143 ) ) ;
#38401=CARTESIAN_POINT ( 'NONE',  ( 5.719274019375991003, -21.55341960407610458, 82.70724293864770971 ) ) ;
#38402=CARTESIAN_POINT ( 'NONE',  ( -5.823673210054431948, 21.52544592524334988, 42.70942372801901854 ) ) ;
#38403=CARTESIAN_POINT ( 'NONE',  ( 16.53943276465976808, -0.05219959533910856209, 113.7489096053143527 ) ) ;
#38404=CARTESIAN_POINT ( 'NONE',  ( 19.03943276465977164, 0.05219959533936151252, 71.25109039468566152 ) ) ;
#38405=CARTESIAN_POINT ( 'NONE',  ( 19.02544592524343514, -5.153800228976328945, 38.54057627198103120 ) ) ;
#38406=CARTESIAN_POINT ( 'NONE',  ( 16.52544592524342804, -4.483927247898539470, 88.54057627198103830 ) ) ;
#38407=CARTESIAN_POINT ( 'NONE',  ( -9.474510206698964154, 16.51473224551069663, 90.41557627198103830 ) ) ;
#38408=CARTESIAN_POINT ( 'NONE',  ( -5.049401038298153566, 19.05341960407611168, 90.20724293864766707 ) ) ;
#38409=CARTESIAN_POINT ( 'NONE',  ( 8.314922557960818139, 14.29746914071049879, 109.5822429386476955 ) ) ;
#38410=CARTESIAN_POINT ( 'NONE',  ( -8.224510206698948167, 14.34966873604960824, 35.41557627198102409 ) ) ;
#38411=CARTESIAN_POINT ( 'NONE',  ( 4.379528057220092307, 16.55341960407617563, 102.2927570613523613 ) ) ;
#38412=CARTESIAN_POINT ( 'NONE',  ( 19.03943276465977164, -0.05219959533909143690, 53.74890960531436690 ) ) ;
#38413=CARTESIAN_POINT ( 'NONE',  ( -5.153800228976328057, -19.02544592524343514, 22.29057627198102765 ) ) ;
#38414=CARTESIAN_POINT ( 'NONE',  ( 13.89961937509957401, 13.97604488694547697, 26.87609039468566507 ) ) ;
#38415=CARTESIAN_POINT ( 'NONE',  ( 16.51473224551069308, 9.474510206698969483, 114.1655762719810241 ) ) ;
#38416=CARTESIAN_POINT ( 'NONE',  ( -14.29746914071049879, 8.314922557960819915, 25.83224293864769194 ) ) ;
#38417=CARTESIAN_POINT ( 'NONE',  ( -18.62759615963255300, -10.81492255796106328, 49.16775706135234003 ) ) ;
#38418=CARTESIAN_POINT ( 'NONE',  ( 5.153800228976335163, 19.02544592524342804, 99.79057627198102409 ) ) ;
#38419=CARTESIAN_POINT ( 'NONE',  ( -16.55341960407617563, 4.379528057220093196, 43.54275706135235424 ) ) ;
#38421=CARTESIAN_POINT ( 'NONE',  ( 12.06949235617739724, 12.14591786802326823, 106.8760903946856899 ) ) ;
#38422=CARTESIAN_POINT ( 'NONE',  ( -14.29746914071037622, -8.314922557961029526, 94.16775706135237556 ) ) ;
#38423=CARTESIAN_POINT ( 'NONE',  ( -16.52544592524335698, -4.483927247898792601, 23.95942372801901143 ) ) ;
#38424=CARTESIAN_POINT ( 'NONE',  ( 16.51473224551069308, 9.474510206698969483, 44.16557627198103120 ) ) ;
#38425=CARTESIAN_POINT ( 'NONE',  ( -0.05219959533910754901, -16.53943276465976808, 102.4989096053143811 ) ) ;
#38426=CARTESIAN_POINT ( 'NONE',  ( -5.719274019375665041, -21.55341960407619695, 24.79275706135235779 ) ) ;
#38427=CARTESIAN_POINT ( 'NONE',  ( -0.05219959533909027116, -19.03943276465977164, 32.49890960531435979 ) ) ;
#38428=CARTESIAN_POINT ( 'NONE',  ( -5.049401038298153566, 19.05341960407611168, 105.2072429386476671 ) ) ;
#38429=CARTESIAN_POINT ( 'NONE',  ( -0.05219959533909027116, -19.03943276465977164, 37.49890960531436690 ) ) ;
#38430=CARTESIAN_POINT ( 'NONE',  ( 9.564922557960805705, 16.46253265017160317, 109.5822429386476955 ) ) ;
#38433=CARTESIAN_POINT ( 'NONE',  ( -13.97604488694527625, -13.89961937509977652, 96.87390960531433848 ) ) ;
#38434=CARTESIAN_POINT ( 'NONE',  ( 0.05219959533937995610, -21.53943276465977519, 40.00109039468567573 ) ) ;
#38435=CARTESIAN_POINT ( 'NONE',  ( -12.06949235617756955, 12.14591786802309770, 110.6239096053143669 ) ) ;
#38436=CARTESIAN_POINT ( 'NONE',  ( 16.51473224551069308, 9.474510206698969483, 114.1655762719810241 ) ) ;
#38437=CARTESIAN_POINT ( 'NONE',  ( -18.22780087662124160, -5.499999999999927169, 68.98236817873106475 ) ) ;
#38438=CARTESIAN_POINT ( 'NONE',  ( -12.14591786802326823, 12.06949235617739902, 68.12609039468567573 ) ) ;
#38439=CARTESIAN_POINT ( 'NONE',  ( -21.53943276465977519, -0.05219959533937600094, 93.75109039468567573 ) ) ;
#38440=CARTESIAN_POINT ( 'NONE',  ( 0.05219959533934541429, -16.53943276465976808, 35.00109039468568284 ) ) ;
#38441=CARTESIAN_POINT ( 'NONE',  ( -9.564922557960796823, -16.46253265017161027, 87.08224293864769550 ) ) ;
#38442=CARTESIAN_POINT ( 'NONE',  ( -9.474510206698720793, -16.51473224551083518, 109.5844237280190043 ) ) ;
#38443=CARTESIAN_POINT ( 'NONE',  ( -16.53943276465976808, -0.05219959533934237506, 88.75109039468567573 ) ) ;
#38444=B_SPLINE_CURVE_WITH_KNOTS ( 'NONE', 3,
 ( #91225, #77071, #44761, #78057, #47747, #108408 ),
 .UNSPECIFIED., .F., .F.,
 ( 4, 2, 4 ),
 ( 0.007228050697041513671, 0.007608510107494985755, 0.007988969517948456972 ),
 .UNSPECIFIED. ) ;
#38445=CARTESIAN_POINT ( 'NONE',  ( -13.89961937509957401, -13.97604488694547875, 99.37609039468567573 ) ) ;
#38446=CARTESIAN_POINT ( 'NONE',  ( -9.474510206698964154, 16.51473224551069663, 75.41557627198103830 ) ) ;
#38447=CARTESIAN_POINT ( 'NONE',  ( 15.72974639402199770, -15.80617190586745480, 98.12390960531436690 ) ) ;
#38448=CARTESIAN_POINT ( 'NONE',  ( 16.55341960407611168, 4.379528057220329451, 93.95724293864770971 ) ) ;
#38449=CARTESIAN_POINT ( 'NONE',  ( 19.03943276465977164, 0.05219959533936151252, 96.25109039468567573 ) ) ;
#38450=CARTESIAN_POINT ( 'NONE',  ( -4.483927247898782831, 16.52544592524335698, 57.70942372801901143 ) ) ;
#38451=CARTESIAN_POINT ( 'NONE',  ( -19.53037848336981241, 5.499999999999899636, 79.85532783611445495 ) ) ;
#38452=CARTESIAN_POINT ( 'NONE',  ( -5.049401038297874678, -19.05341960407617918, 69.79275706135233293 ) ) ;
#38453=CARTESIAN_POINT ( 'NONE',  ( -4.379528057220328563, 16.55341960407611168, 30.20724293864769550 ) ) ;
#38454=CARTESIAN_POINT ( 'NONE',  ( -14.29746914071049879, 8.314922557960819915, 95.83224293864770971 ) ) ;
#38455=CARTESIAN_POINT ( 'NONE',  ( -19.05341960407617563, 5.049401038297882671, 23.54275706135233648 ) ) ;
#38456=CARTESIAN_POINT ( 'NONE',  ( -17.48847506799948803, 5.747544572775297844, 40.82697437843290800 ) ) ;
#38457=CARTESIAN_POINT ( 'NONE',  ( 10.72451020669871369, 18.67979575497193778, 27.08442372801901854 ) ) ;
#38459=CARTESIAN_POINT ( 'NONE',  ( -13.97604488694527625, -13.89961937509977652, 71.87390960531433848 ) ) ;
#38460=CARTESIAN_POINT ( 'NONE',  ( 21.55341960407619695, -5.719274019375665929, 96.04275706135236135 ) ) ;
#38461=CARTESIAN_POINT ( 'NONE',  ( -9.474510206698964154, 16.51473224551069663, 70.41557627198102409 ) ) ;
#38462=CARTESIAN_POINT ( 'NONE',  ( 15.80617190586746368, 15.72974639402197994, 44.37390960531435979 ) ) ;
#38463=CARTESIAN_POINT ( 'NONE',  ( 8.314922557960818139, 14.29746914071049879, 84.58224293864769550 ) ) ;
#38464=CARTESIAN_POINT ( 'NONE',  ( 0.05219959533909260263, 19.03943276465977164, 59.99890960531436690 ) ) ;
#38465=CARTESIAN_POINT ( 'NONE',  ( 9.474510206698971260, -16.51473224551069308, 22.91557627198102765 ) ) ;
#38466=CARTESIAN_POINT ( 'NONE',  ( 21.55341960407619695, -5.719274019375665929, 31.04275706135234714 ) ) ;
#38467=CARTESIAN_POINT ( 'NONE',  ( -15.72974639402176322, -15.80617190586768395, 64.37609039468568994 ) ) ;
#38468=CARTESIAN_POINT ( 'NONE',  ( 5.049401038298161559, -19.05341960407611168, 42.70724293864767418 ) ) ;
#38469=CARTESIAN_POINT ( 'NONE',  ( -16.52544592524335698, -4.483927247898792601, 73.95942372801901854 ) ) ;
#38470=CARTESIAN_POINT ( 'NONE',  ( 21.53943276465977519, -0.05219959533907433946, 108.7489096053143669 ) ) ;
#38472=CARTESIAN_POINT ( 'NONE',  ( 15.80617190586746368, 15.72974639402197994, 109.3739096053143811 ) ) ;
#38473=CARTESIAN_POINT ( 'NONE',  ( 5.049401038297881783, 19.05341960407617563, 37.29275706135232582 ) ) ;
#38474=CARTESIAN_POINT ( 'NONE',  ( -5.049401038298153566, 19.05341960407611168, 70.20724293864769550 ) ) ;
#38475=CARTESIAN_POINT ( 'NONE',  ( -13.89961937509957401, -13.97604488694547875, 29.37609039468565797 ) ) ;
#38476=CARTESIAN_POINT ( 'NONE',  ( 21.52544592524334988, 5.823673210054432836, 71.45942372801901854 ) ) ;
#38477=CARTESIAN_POINT ( 'NONE',  ( -15.72974639402197994, 15.80617190586746368, 65.62390960531436690 ) ) ;
#38478=CARTESIAN_POINT ( 'NONE',  ( 14.34966873604960469, 8.224510206698951720, 34.16557627198102409 ) ) ;
#38479=CARTESIAN_POINT ( 'NONE',  ( 21.55341960407619695, -5.719274019375665929, 96.04275706135236135 ) ) ;
#38480=CARTESIAN_POINT ( 'NONE',  ( 19.03943276465977164, 0.05219959533936151252, 31.25109039468566863 ) ) ;
#38481=CARTESIAN_POINT ( 'NONE',  ( -12.14591786802309592, -12.06949235617757132, 61.87390960531436690 ) ) ;
#38482=CARTESIAN_POINT ( 'NONE',  ( 12.06949235617757843, -12.14591786802309237, 103.1239096053143811 ) ) ;
#38483=CARTESIAN_POINT ( 'NONE',  ( -19.05341960407617563, 5.049401038297882671, 63.54275706135234003 ) ) ;
#38484=CARTESIAN_POINT ( 'NONE',  ( -4.379528057220328563, 16.55341960407611168, 25.20724293864769550 ) ) ;
#38485=CARTESIAN_POINT ( 'NONE',  ( 18.67979575497194134, -10.72451020669871369, 70.83442372801901854 ) ) ;
#38486=CARTESIAN_POINT ( 'NONE',  ( -9.564922557960796823, -16.46253265017161027, 77.08224293864769550 ) ) ;
#38487=CARTESIAN_POINT ( 'NONE',  ( 16.46253265017146816, 9.564922557961045513, 46.66775706135233293 ) ) ;
#38488=CARTESIAN_POINT ( 'NONE',  ( -21.52544592524343514, 5.823673210054127303, 51.04057627198103120 ) ) ;
#38489=CARTESIAN_POINT ( 'NONE',  ( -10.81492255796105439, 18.62759615963255655, 47.91775706135234714 ) ) ;
#38490=CIRCLE ( 'NONE', #80468, 2.000000000000001776 ) ;
#38491=CARTESIAN_POINT ( 'NONE',  ( -5.719274019375978568, 21.55341960407610458, 100.2072429386476955 ) ) ;
#38492=CARTESIAN_POINT ( 'NONE',  ( -5.049401038297874678, -19.05341960407617918, 104.7927570613523471 ) ) ;
#38493=CARTESIAN_POINT ( 'NONE',  ( 14.34966873604972726, -8.224510206698740333, 65.83442372801900433 ) ) ;
#38495=CARTESIAN_POINT ( 'NONE',  ( -15.72974639402197994, 15.80617190586746368, 100.6239096053143811 ) ) ;
#38496=CARTESIAN_POINT ( 'NONE',  ( -12.06949235617756955, 12.14591786802309770, 95.62390960531436690 ) ) ;
#38497=CARTESIAN_POINT ( 'NONE',  ( -16.19135201231366494, -7.376712067591948419, 100.1868085405203317 ) ) ;
#38498=CARTESIAN_POINT ( 'NONE',  ( -14.29746914071037622, -8.314922557961029526, 19.16775706135234714 ) ) ;
#38499=CARTESIAN_POINT ( 'NONE',  ( 5.719274019375991003, -21.55341960407610458, 42.70724293864770260 ) ) ;
#38500=CARTESIAN_POINT ( 'NONE',  ( 0.05219959533934541429, -16.53943276465976808, 90.00109039468567573 ) ) ;
#38502=CARTESIAN_POINT ( 'NONE',  ( -16.55341960407617563, 4.379528057220093196, 63.54275706135234003 ) ) ;
#38503=CARTESIAN_POINT ( 'NONE',  ( -15.72974639402176322, -15.80617190586768395, 34.37609039468568284 ) ) ;
#38504=CARTESIAN_POINT ( 'NONE',  ( -5.719274019375978568, 21.55341960407610458, 40.20724293864769550 ) ) ;
#38505=CARTESIAN_POINT ( 'NONE',  ( -16.53943276465976808, -0.05219959533934237506, 88.75109039468567573 ) ) ;
#38506=CARTESIAN_POINT ( 'NONE',  ( -13.97604488694527625, -13.89961937509977652, 91.87390960531432427 ) ) ;
#38507=CARTESIAN_POINT ( 'NONE',  ( 0.05219959533937995610, -21.53943276465977519, 65.00109039468568994 ) ) ;
#38508=CARTESIAN_POINT ( 'NONE',  ( 15.72974639402199770, -15.80617190586745480, 38.12390960531436690 ) ) ;
#38509=CARTESIAN_POINT ( 'NONE',  ( -21.52544592524343514, 5.823673210054127303, 36.04057627198102409 ) ) ;
#38511=CARTESIAN_POINT ( 'NONE',  ( -19.02544592524334988, -5.153800228976617603, 58.95942372801900433 ) ) ;
#38512=CARTESIAN_POINT ( 'NONE',  ( -4.483927247898782831, 16.52544592524335698, 67.70942372801901854 ) ) ;
#38513=CARTESIAN_POINT ( 'NONE',  ( 5.823673210054125526, 21.52544592524343514, 29.79057627198102409 ) ) ;
#38515=CARTESIAN_POINT ( 'NONE',  ( 0.05219959533909260263, 19.03943276465977164, 89.99890960531436690 ) ) ;
#38516=CARTESIAN_POINT ( 'NONE',  ( -16.55341960407611168, -4.379528057220339221, 26.45724293864768839 ) ) ;
#38517=CARTESIAN_POINT ( 'NONE',  ( -18.09805431107249163, 5.499999999999980460, 86.01606229291887473 ) ) ;
#38518=CARTESIAN_POINT ( 'NONE',  ( -16.55341960407611168, -4.379528057220339221, 106.4572429386477097 ) ) ;
#38519=CARTESIAN_POINT ( 'NONE',  ( 10.72451020669898902, -18.67979575497178502, 52.91557627198103830 ) ) ;
#38520=CARTESIAN_POINT ( 'NONE',  ( -5.049401038298153566, 19.05341960407611168, 50.20724293864770260 ) ) ;
#38521=CARTESIAN_POINT ( 'NONE',  ( 14.34966873604972726, -8.224510206698740333, 80.83442372801901854 ) ) ;
#38522=CARTESIAN_POINT ( 'NONE',  ( 10.72451020669871369, 18.67979575497193778, 27.08442372801901854 ) ) ;
#38523=CARTESIAN_POINT ( 'NONE',  ( -9.474510206698720793, -16.51473224551083518, 84.58442372801900433 ) ) ;
#38524=CARTESIAN_POINT ( 'NONE',  ( -16.55341960407611168, -4.379528057220339221, 86.45724293864770971 ) ) ;
#38525=CARTESIAN_POINT ( 'NONE',  ( -0.05219959533909027116, -19.03943276465977164, 57.49890960531435979 ) ) ;
#38526=CARTESIAN_POINT ( 'NONE',  ( 9.474510206698971260, -16.51473224551069308, 32.91557627198102409 ) ) ;
#38527=CARTESIAN_POINT ( 'NONE',  ( 15.72974639402176855, 15.80617190586768217, 101.8760903946857042 ) ) ;
#38528=CARTESIAN_POINT ( 'NONE',  ( 9.474510206698971260, -16.51473224551069308, 82.91557627198103830 ) ) ;
#38529=CARTESIAN_POINT ( 'NONE',  ( 14.34966873604972726, -8.224510206698740333, 60.83442372801901854 ) ) ;
#38530=CARTESIAN_POINT ( 'NONE',  ( 15.72974639402176855, 15.80617190586768217, 86.87609039468568994 ) ) ;
#38531=CARTESIAN_POINT ( 'NONE',  ( -15.72974639402197994, 15.80617190586746368, 50.62390960531435979 ) ) ;
#38532=CARTESIAN_POINT ( 'NONE',  ( 16.52544592524335698, 4.483927247898782831, 76.45942372801901854 ) ) ;
#38533=CARTESIAN_POINT ( 'NONE',  ( 9.564922557961047289, -16.46253265017146816, 50.41775706135233293 ) ) ;
#38534=CARTESIAN_POINT ( 'NONE',  ( -13.89961937509957401, -13.97604488694547875, 64.37609039468567573 ) ) ;
#38536=CARTESIAN_POINT ( 'NONE',  ( -15.72974639402176322, -15.80617190586768395, 59.37609039468568284 ) ) ;
#38537=CARTESIAN_POINT ( 'NONE',  ( -5.153800228976328057, -19.02544592524343514, 62.29057627198100988 ) ) ;
#38538=CARTESIAN_POINT ( 'NONE',  ( 19.05341960407611168, 5.049401038298154454, 38.95724293864767418 ) ) ;
#38539=CARTESIAN_POINT ( 'NONE',  ( -5.049401038297874678, -19.05341960407617918, 64.79275706135233293 ) ) ;
#38540=CARTESIAN_POINT ( 'NONE',  ( 19.03943276465977164, -0.05219959533909143690, 113.7489096053143669 ) ) ;
#38541=CARTESIAN_POINT ( 'NONE',  ( -19.05341960407611168, -5.049401038298163336, 101.4572429386476955 ) ) ;
#38542=CARTESIAN_POINT ( 'NONE',  ( 16.52544592524342804, -4.483927247898539470, 48.54057627198103120 ) ) ;
#38543=CARTESIAN_POINT ( 'NONE',  ( -21.53943276465977519, 0.05219959533907696930, 46.24890960531435979 ) ) ;
#38545=CARTESIAN_POINT ( 'NONE',  ( 18.67979575497194134, -10.72451020669871369, 110.8344237280190043 ) ) ;
#38546=CARTESIAN_POINT ( 'NONE',  ( -17.12812012977029141, -6.668231424565922438, 81.35948759323146362 ) ) ;
#38547=CARTESIAN_POINT ( 'NONE',  ( 5.153800228976335163, 19.02544592524342804, 54.79057627198103120 ) ) ;
#38550=CARTESIAN_POINT ( 'NONE',  ( -16.55341960407617563, 4.379528057220093196, 78.54275706135236135 ) ) ;
#38551=CARTESIAN_POINT ( 'NONE',  ( -18.67979575497178146, -10.72451020669898902, 96.66557627198102409 ) ) ;
#38552=CARTESIAN_POINT ( 'NONE',  ( 4.483927247898545687, 16.52544592524342804, 49.79057627198102409 ) ) ;
#38553=CARTESIAN_POINT ( 'NONE',  ( 13.97604488694527802, 13.89961937509977652, 44.37390960531435269 ) ) ;
#38555=CARTESIAN_POINT ( 'NONE',  ( -15.80617190586768217, 15.72974639402176855, 38.12609039468567573 ) ) ;
#38556=CARTESIAN_POINT ( 'NONE',  ( 13.89961937509957401, 13.97604488694547697, 51.87609039468566863 ) ) ;
#38557=CARTESIAN_POINT ( 'NONE',  ( 9.564922557960805705, 16.46253265017160317, 34.58224293864770260 ) ) ;
#38558=CARTESIAN_POINT ( 'NONE',  ( 0.05219959533937995610, -21.53943276465977519, 90.00109039468567573 ) ) ;
#38561=CARTESIAN_POINT ( 'NONE',  ( 4.379528057220339221, -16.55341960407611168, 37.70724293864769550 ) ) ;
#38562=CARTESIAN_POINT ( 'NONE',  ( 17.50000000001358913, -5.500000000000039968, 73.29690382535059712 ) ) ;
#38563=CARTESIAN_POINT ( 'NONE',  ( -10.72451020669898014, 18.67979575497178502, 35.41557627198102409 ) ) ;
#38565=CARTESIAN_POINT ( 'NONE',  ( 5.153800228976335163, 19.02544592524342804, 94.79057627198103830 ) ) ;
#38566=CARTESIAN_POINT ( 'NONE',  ( 4.483927247898545687, 16.52544592524342804, 94.79057627198105251 ) ) ;
#38567=CARTESIAN_POINT ( 'NONE',  ( 16.55341960407618274, -4.379528057220086978, 26.04275706135235779 ) ) ;
#38568=CARTESIAN_POINT ( 'NONE',  ( 14.29746914071049879, -8.314922557960816363, 23.33224293864769194 ) ) ;
#38570=CARTESIAN_POINT ( 'NONE',  ( -16.51473224551069308, -9.474510206698971260, 96.66557627198102409 ) ) ;
#38571=CARTESIAN_POINT ( 'NONE',  ( -15.72974639402197994, 15.80617190586746368, 85.62390960531436690 ) ) ;
#38572=CARTESIAN_POINT ( 'NONE',  ( -0.05219959533910754901, -16.53943276465976808, 22.49890960531436335 ) ) ;
#38573=CARTESIAN_POINT ( 'NONE',  ( 16.46253265017160672, -9.564922557960803928, 103.3322429386476955 ) ) ;
#38574=CARTESIAN_POINT ( 'NONE',  ( 19.02544592524334988, 5.153800228976608722, 81.45942372801897591 ) ) ;
#38575=CARTESIAN_POINT ( 'NONE',  ( -15.80617190586768217, 15.72974639402176855, 108.1260903946856757 ) ) ;
#38576=CARTESIAN_POINT ( 'NONE',  ( -10.81492255796078084, -18.62759615963271287, 87.08224293864769550 ) ) ;
#38577=CARTESIAN_POINT ( 'NONE',  ( -21.53943276465977519, 0.05219959533907696930, 41.24890960531435269 ) ) ;
#38578=CARTESIAN_POINT ( 'NONE',  ( 5.153800228976335163, 19.02544592524342804, 64.79057627198100988 ) ) ;
#38579=CARTESIAN_POINT ( 'NONE',  ( -16.52544592524342804, 4.483927247898546575, 31.04057627198102409 ) ) ;
#38580=CARTESIAN_POINT ( 'NONE',  ( -9.474510206698964154, 16.51473224551069663, 75.41557627198103830 ) ) ;
#38583=CARTESIAN_POINT ( 'NONE',  ( -19.05341960407617563, 5.049401038297882671, 23.54275706135233648 ) ) ;
#38584=CARTESIAN_POINT ( 'NONE',  ( -8.224510206698948167, 14.34966873604960824, 85.41557627198102409 ) ) ;
#38585=CARTESIAN_POINT ( 'NONE',  ( 0.05219959533937995610, -21.53943276465977519, 20.00109039468568639 ) ) ;
#38587=CARTESIAN_POINT ( 'NONE',  ( -5.823673210054116645, -21.52544592524344225, 77.29057627198102409 ) ) ;
#38589=CARTESIAN_POINT ( 'NONE',  ( -14.34966873604972548, 8.224510206698743886, 93.33442372801901854 ) ) ;
#38590=CARTESIAN_POINT ( 'NONE',  ( 16.46253265017160672, -9.564922557960803928, 28.33224293864769550 ) ) ;
#38591=CARTESIAN_POINT ( 'NONE',  ( 13.97604488694527802, 13.89961937509977652, 74.37390960531436690 ) ) ;
#38593=CARTESIAN_POINT ( 'NONE',  ( -12.14591786802309592, -12.06949235617757132, 26.87390960531435979 ) ) ;
#38594=CARTESIAN_POINT ( 'NONE',  ( -0.05219959533937732626, 21.53943276465977519, 62.50109039468568284 ) ) ;
#38596=CARTESIAN_POINT ( 'NONE',  ( -21.52544592524334988, -5.823673210054445271, 98.95942372801903275 ) ) ;
#38597=CARTESIAN_POINT ( 'NONE',  ( -19.03943276465977164, 0.05219959533909376836, 46.24890960531435979 ) ) ;
#38598=CARTESIAN_POINT ( 'NONE',  ( -9.474510206698964154, 16.51473224551069663, 50.41557627198102409 ) ) ;
#38600=CARTESIAN_POINT ( 'NONE',  ( 21.55341960407619695, -5.719274019375665929, 91.04275706135236135 ) ) ;
#38601=CARTESIAN_POINT ( 'NONE',  ( 8.224510206698742110, 14.34966873604972548, 67.08442372801901854 ) ) ;
#38602=CARTESIAN_POINT ( 'NONE',  ( -5.719274019375665041, -21.55341960407619695, 89.79275706135236135 ) ) ;
#38603=CARTESIAN_POINT ( 'NONE',  ( 13.89961937509977652, -13.97604488694527269, 113.1239096053143527 ) ) ;
#38604=CARTESIAN_POINT ( 'NONE',  ( 5.049401038297881783, 19.05341960407617563, 87.29275706135234714 ) ) ;
#38605=CARTESIAN_POINT ( 'NONE',  ( -21.52544592524334988, -5.823673210054445271, 68.95942372801901854 ) ) ;
#38606=CARTESIAN_POINT ( 'NONE',  ( 0.05219959533934541429, -16.53943276465976808, 35.00109039468568284 ) ) ;
#38607=CARTESIAN_POINT ( 'NONE',  ( -15.80617190586745835, -15.72974639402198527, 86.87390960531438111 ) ) ;
#38608=CARTESIAN_POINT ( 'NONE',  ( -9.474510206698720793, -16.51473224551083518, 89.58442372801900433 ) ) ;
#38609=CARTESIAN_POINT ( 'NONE',  ( 19.02544592524343514, -5.153800228976328945, 58.54057627198102409 ) ) ;
#38610=CARTESIAN_POINT ( 'NONE',  ( -5.049401038297874678, -19.05341960407617918, 99.79275706135234714 ) ) ;
#38611=CARTESIAN_POINT ( 'NONE',  ( 19.02544592524334988, 5.153800228976608722, 101.4594237280189759 ) ) ;
#38612=CARTESIAN_POINT ( 'NONE',  ( 12.14591786802309770, 12.06949235617756955, 49.37390960531436690 ) ) ;
#38613=CARTESIAN_POINT ( 'NONE',  ( 5.153800228976615827, -19.02544592524334988, 80.20942372801901854 ) ) ;
#38614=CARTESIAN_POINT ( 'NONE',  ( -16.53943276465976808, -0.05219959533934237506, 63.75109039468568284 ) ) ;
#38615=CARTESIAN_POINT ( 'NONE',  ( 0.05219959533909260263, 19.03943276465977164, 39.99890960531436690 ) ) ;
#38616=CARTESIAN_POINT ( 'NONE',  ( 0.05219959533909260263, 19.03943276465977164, 59.99890960531436690 ) ) ;
#38618=CARTESIAN_POINT ( 'NONE',  ( -12.06949235617739369, -12.14591786802326823, 64.37609039468568994 ) ) ;
#38621=CARTESIAN_POINT ( 'NONE',  ( -9.564922557960796823, -16.46253265017161027, 107.0822429386476955 ) ) ;
#38622=CARTESIAN_POINT ( 'NONE',  ( 19.05341960407611168, 5.049401038298154454, 28.95724293864769550 ) ) ;
#38623=ORIENTED_EDGE ( 'NONE', *, *, #20347, .T. ) ;
#38624=CARTESIAN_POINT ( 'NONE',  ( 5.049401038297881783, 19.05341960407617563, 112.2927570613523471 ) ) ;
#38626=CARTESIAN_POINT ( 'NONE',  ( -5.823673210054116645, -21.52544592524344225, 32.29057627198102409 ) ) ;
#38627=CARTESIAN_POINT ( 'NONE',  ( -9.564922557961040184, 16.46253265017147172, 27.91775706135232582 ) ) ;
#38628=CARTESIAN_POINT ( 'NONE',  ( 12.06949235617739724, 12.14591786802326823, 21.87609039468567573 ) ) ;
#38629=CARTESIAN_POINT ( 'NONE',  ( 5.049401038298161559, -19.05341960407611168, 32.70724293864768129 ) ) ;
#38630=CARTESIAN_POINT ( 'NONE',  ( -0.05219959533909027116, -19.03943276465977164, 52.49890960531436690 ) ) ;
#38631=CARTESIAN_POINT ( 'NONE',  ( 21.52544592524344225, -5.823673210054117533, 78.54057627198103830 ) ) ;
#38632=CARTESIAN_POINT ( 'NONE',  ( 16.51473224551069308, 9.474510206698969483, 99.16557627198102409 ) ) ;
#38633=CARTESIAN_POINT ( 'NONE',  ( -16.51473224551069308, -9.474510206698971260, 36.66557627198102409 ) ) ;
#38635=CARTESIAN_POINT ( 'NONE',  ( 9.564922557961047289, -16.46253265017146816, 80.41775706135234714 ) ) ;
#38636=CARTESIAN_POINT ( 'NONE',  ( 14.29746914071049879, -8.314922557960816363, 73.33224293864769550 ) ) ;
#38637=CARTESIAN_POINT ( 'NONE',  ( 0.05219959533907565091, 21.53943276465977519, 44.99890960531435979 ) ) ;
#38638=CARTESIAN_POINT ( 'NONE',  ( -18.67979575497193778, 10.72451020669871902, 108.3344237280190185 ) ) ;
#38639=CARTESIAN_POINT ( 'NONE',  ( -5.719274019375978568, 21.55341960407610458, 95.20724293864769550 ) ) ;
#38640=CARTESIAN_POINT ( 'NONE',  ( -18.67979575497193778, 10.72451020669871902, 68.33442372801900433 ) ) ;
#38641=CARTESIAN_POINT ( 'NONE',  ( 10.81492255796106328, -18.62759615963255655, 75.41775706135233293 ) ) ;
#38642=CARTESIAN_POINT ( 'NONE',  ( 16.51473224551069308, 9.474510206698969483, 109.1655762719810383 ) ) ;
#38643=CARTESIAN_POINT ( 'NONE',  ( 14.34966873604972726, -8.224510206698740333, 110.8344237280190043 ) ) ;
#38644=CARTESIAN_POINT ( 'NONE',  ( -5.719274019375665041, -21.55341960407619695, 74.79275706135234714 ) ) ;
#38645=CARTESIAN_POINT ( 'NONE',  ( 5.153800228976335163, 19.02544592524342804, 69.79057627198103830 ) ) ;
#38646=CARTESIAN_POINT ( 'NONE',  ( -0.05219959533936034679, 19.03943276465977164, 32.50109039468566863 ) ) ;
#38647=CARTESIAN_POINT ( 'NONE',  ( 5.823673210054444382, -21.52544592524334988, 25.20942372801901854 ) ) ;
#38648=CARTESIAN_POINT ( 'NONE',  ( 5.049401038298161559, -19.05341960407611168, 62.70724293864769550 ) ) ;
#38649=CARTESIAN_POINT ( 'NONE',  ( -8.224510206698948167, 14.34966873604960824, 80.41557627198103830 ) ) ;
#38650=CARTESIAN_POINT ( 'NONE',  ( -4.483927247898539470, -16.52544592524342804, 42.29057627198103120 ) ) ;
#38651=CARTESIAN_POINT ( 'NONE',  ( -0.05219959533907301413, -21.53943276465977519, 62.49890960531436690 ) ) ;
#38652=CARTESIAN_POINT ( 'NONE',  ( -9.564922557960796823, -16.46253265017161027, 62.08224293864769550 ) ) ;
#38653=CARTESIAN_POINT ( 'NONE',  ( -21.55341960407610458, -5.719274019375992779, 71.45724293864769550 ) ) ;
#38654=CARTESIAN_POINT ( 'NONE',  ( -13.89961937509957401, -13.97604488694547875, 64.37609039468567573 ) ) ;
#38656=CARTESIAN_POINT ( 'NONE',  ( 8.314922557960818139, 14.29746914071049879, 69.58224293864769550 ) ) ;
#38657=CARTESIAN_POINT ( 'NONE',  ( -10.72451020669898014, 18.67979575497178502, 45.41557627198103830 ) ) ;
#38660=CARTESIAN_POINT ( 'NONE',  ( -4.379528057220086978, -16.55341960407618274, 89.79275706135236135 ) ) ;
#38663=CARTESIAN_POINT ( 'NONE',  ( -16.51473224551082808, 9.474510206698731452, 83.33442372801899012 ) ) ;
#38664=CARTESIAN_POINT ( 'NONE',  ( -12.14591786802309592, -12.06949235617757132, 71.87390960531438111 ) ) ;
#38665=CARTESIAN_POINT ( 'NONE',  ( -19.25176906914649777, -5.499999999999745093, 60.99927264242280245 ) ) ;
#38666=CARTESIAN_POINT ( 'NONE',  ( 13.97604488694527802, 13.89961937509977652, 49.37390960531434558 ) ) ;
#38667=CARTESIAN_POINT ( 'NONE',  ( -14.34966873604960291, -8.224510206698953496, 41.66557627198103120 ) ) ;
#38668=CARTESIAN_POINT ( 'NONE',  ( 13.97604488694527802, 13.89961937509977652, 89.37390960531436690 ) ) ;
#38669=CARTESIAN_POINT ( 'NONE',  ( 0.05219959533936267826, -19.03943276465977164, 80.00109039468567573 ) ) ;
#38670=CARTESIAN_POINT ( 'NONE',  ( 13.89961937509977652, -13.97604488694527269, 48.12390960531435979 ) ) ;
#38671=CARTESIAN_POINT ( 'NONE',  ( -18.67979575497193778, 10.72451020669871902, 63.33442372801900433 ) ) ;
#38672=CARTESIAN_POINT ( 'NONE',  ( -9.564922557960796823, -16.46253265017161027, 87.08224293864769550 ) ) ;
#38673=CARTESIAN_POINT ( 'NONE',  ( -13.97604488694527625, -13.89961937509977652, 21.87390960531435979 ) ) ;
#38674=CARTESIAN_POINT ( 'NONE',  ( -5.153800228976328057, -19.02544592524343514, 77.29057627198099567 ) ) ;
#38675=CARTESIAN_POINT ( 'NONE',  ( 10.72451020669898902, -18.67979575497178502, 47.91557627198102409 ) ) ;
#38676=CARTESIAN_POINT ( 'NONE',  ( 16.46253265017160672, -9.564922557960803928, 53.33224293864768839 ) ) ;
#38677=CARTESIAN_POINT ( 'NONE',  ( 21.53943276465977519, -0.05219959533907433946, 48.74890960531435979 ) ) ;
#38678=CARTESIAN_POINT ( 'NONE',  ( 9.564922557961047289, -16.46253265017146816, 85.41775706135233293 ) ) ;
#38679=CARTESIAN_POINT ( 'NONE',  ( -16.55341960407617563, 4.379528057220093196, 108.5427570613523756 ) ) ;
#38680=CARTESIAN_POINT ( 'NONE',  ( 16.46253265017146816, 9.564922557961045513, 31.66775706135232937 ) ) ;
#38681=CARTESIAN_POINT ( 'NONE',  ( 14.29746914071037800, 8.314922557961029526, 56.66775706135235424 ) ) ;
#38682=CARTESIAN_POINT ( 'NONE',  ( -16.53943276465976808, -0.05219959533934237506, 83.75109039468568994 ) ) ;
#38684=CARTESIAN_POINT ( 'NONE',  ( -14.34966873604972548, 8.224510206698743886, 78.33442372801901854 ) ) ;
#38685=CARTESIAN_POINT ( 'NONE',  ( -5.719274019375978568, 21.55341960407610458, 25.20724293864769550 ) ) ;
#38686=CARTESIAN_POINT ( 'NONE',  ( 5.153800228976335163, 19.02544592524342804, 34.79057627198102409 ) ) ;
#38687=CARTESIAN_POINT ( 'NONE',  ( 12.06949235617739724, 12.14591786802326823, 36.87609039468568994 ) ) ;
#38688=CARTESIAN_POINT ( 'NONE',  ( -5.153800228976328057, -19.02544592524343514, 52.29057627198100988 ) ) ;
#38689=CARTESIAN_POINT ( 'NONE',  ( -21.53943276465977519, -0.05219959533937600094, 43.75109039468568284 ) ) ;
#38690=CARTESIAN_POINT ( 'NONE',  ( 14.34966873604972726, -8.224510206698740333, 30.83442372801902209 ) ) ;
#38691=CARTESIAN_POINT ( 'NONE',  ( -0.05219959533934338120, 16.53943276465976808, 107.5010903946856899 ) ) ;
#38692=CARTESIAN_POINT ( 'NONE',  ( 13.97604488694527802, 13.89961937509977652, 34.37390960531436690 ) ) ;
#38693=CARTESIAN_POINT ( 'NONE',  ( 15.72974639402176855, 15.80617190586768217, 111.8760903946856615 ) ) ;
#38694=CARTESIAN_POINT ( 'NONE',  ( -16.46253265017146816, -9.564922557961047289, 109.1677570613523471 ) ) ;
#38695=CARTESIAN_POINT ( 'NONE',  ( 16.51473224551083163, -9.474510206698727899, 70.83442372801900433 ) ) ;
#38696=CARTESIAN_POINT ( 'NONE',  ( 12.14591786802309770, 12.06949235617756955, 74.37390960531436690 ) ) ;
#38697=CARTESIAN_POINT ( 'NONE',  ( -13.97604488694527625, -13.89961937509977652, 36.87390960531436690 ) ) ;
#38698=CARTESIAN_POINT ( 'NONE',  ( -5.049401038297874678, -19.05341960407617918, 79.79275706135233293 ) ) ;
#38699=CARTESIAN_POINT ( 'NONE',  ( 0.05219959533937995610, -21.53943276465977519, 65.00109039468568994 ) ) ;
#38700=CARTESIAN_POINT ( 'NONE',  ( -4.483927247898782831, 16.52544592524335698, 37.70942372801900433 ) ) ;
#38701=CARTESIAN_POINT ( 'NONE',  ( 18.39443945427639449, -5.500000000000022204, 56.01745347608652992 ) ) ;
#38702=CARTESIAN_POINT ( 'NONE',  ( 5.823673210054125526, 21.52544592524343514, 39.79057627198103830 ) ) ;
#38703=CARTESIAN_POINT ( 'NONE',  ( 16.53943276465976808, 0.05219959533934440121, 21.25109039468567218 ) ) ;
#38704=CARTESIAN_POINT ( 'NONE',  ( 16.46253265017160672, -9.564922557960803928, 113.3322429386476955 ) ) ;
#38706=CARTESIAN_POINT ( 'NONE',  ( -19.05341960407611168, -5.049401038298163336, 36.45724293864766707 ) ) ;
#38707=CARTESIAN_POINT ( 'NONE',  ( 15.80617190586769283, -15.72974639402175789, 105.6260903946856899 ) ) ;
#38708=CARTESIAN_POINT ( 'NONE',  ( 9.564922557960805705, 16.46253265017160317, 59.58224293864769550 ) ) ;
#38709=CARTESIAN_POINT ( 'NONE',  ( 15.80617190586769283, -15.72974639402175789, 65.62609039468568994 ) ) ;
#38710=CARTESIAN_POINT ( 'NONE',  ( -18.67979575497193778, 10.72451020669871902, 98.33442372801901854 ) ) ;
#38711=CARTESIAN_POINT ( 'NONE',  ( 14.29746914071049879, -8.314922557960816363, 28.33224293864769550 ) ) ;
#38712=CARTESIAN_POINT ( 'NONE',  ( -0.05219959533909027116, -19.03943276465977164, 32.49890960531435979 ) ) ;
#38713=CARTESIAN_POINT ( 'NONE',  ( -19.02544592524342804, 5.153800228976336051, 86.04057627198103830 ) ) ;
#38714=CARTESIAN_POINT ( 'NONE',  ( -0.05219959533937732626, 21.53943276465977519, 62.50109039468568284 ) ) ;
#38715=CARTESIAN_POINT ( 'NONE',  ( -9.564922557960796823, -16.46253265017161027, 42.08224293864769550 ) ) ;
#38716=CARTESIAN_POINT ( 'NONE',  ( -5.719274019375665041, -21.55341960407619695, 59.79275706135234714 ) ) ;
#38717=CARTESIAN_POINT ( 'NONE',  ( -19.05341960407617563, 5.049401038297882671, 88.54275706135230450 ) ) ;
#38718=CARTESIAN_POINT ( 'NONE',  ( 5.153800228976335163, 19.02544592524342804, 99.79057627198102409 ) ) ;
#38719=CARTESIAN_POINT ( 'NONE',  ( -4.379528057220328563, 16.55341960407611168, 115.2072429386476955 ) ) ;
#38720=CARTESIAN_POINT ( 'NONE',  ( 21.55341960407610458, 5.719274019375980345, 108.9572429386476955 ) ) ;
#38721=CARTESIAN_POINT ( 'NONE',  ( 5.049401038297881783, 19.05341960407617563, 32.29275706135233293 ) ) ;
#38722=CARTESIAN_POINT ( 'NONE',  ( 8.314922557960818139, 14.29746914071049879, 104.5822429386477097 ) ) ;
#38723=CARTESIAN_POINT ( 'NONE',  ( 19.03943276465977164, -0.05219959533909143690, 53.74890960531436690 ) ) ;
#38724=CARTESIAN_POINT ( 'NONE',  ( 19.02544592524334988, 5.153800228976608722, 91.45942372801900433 ) ) ;
#38725=CARTESIAN_POINT ( 'NONE',  ( 0.05219959533910956823, 16.53943276465976808, 59.99890960531436690 ) ) ;
#38726=CARTESIAN_POINT ( 'NONE',  ( -5.823673210054431948, 21.52544592524334988, 107.7094237280190328 ) ) ;
#38727=CARTESIAN_POINT ( 'NONE',  ( -15.72974639402197994, 15.80617190586746368, 25.62390960531435624 ) ) ;
#38728=CARTESIAN_POINT ( 'NONE',  ( 5.153800228976615827, -19.02544592524334988, 85.20942372801900433 ) ) ;
#38729=CARTESIAN_POINT ( 'NONE',  ( -21.55341960407610458, -5.719274019375992779, 96.45724293864770971 ) ) ;
#38730=CARTESIAN_POINT ( 'NONE',  ( 5.823673210054444382, -21.52544592524334988, 50.20942372801901854 ) ) ;
#38731=CARTESIAN_POINT ( 'NONE',  ( -12.14591786802326823, 12.06949235617739902, 48.12609039468568284 ) ) ;
#38732=CARTESIAN_POINT ( 'NONE',  ( 8.314922557961029526, -14.29746914071037800, 105.4177570613523613 ) ) ;
#38733=CARTESIAN_POINT ( 'NONE',  ( 0.05219959533934541429, -16.53943276465976808, 35.00109039468568284 ) ) ;
#38734=CARTESIAN_POINT ( 'NONE',  ( 15.80617190586769283, -15.72974639402175789, 50.62609039468568994 ) ) ;
#38735=CARTESIAN_POINT ( 'NONE',  ( 5.823673210054125526, 21.52544592524343514, 44.79057627198103120 ) ) ;
#38736=CARTESIAN_POINT ( 'NONE',  ( -5.049401038298153566, 19.05341960407611168, 30.20724293864768839 ) ) ;
#38738=CARTESIAN_POINT ( 'NONE',  ( 16.52544592524335698, 4.483927247898782831, 66.45942372801903275 ) ) ;
#38739=CARTESIAN_POINT ( 'NONE',  ( -0.05219959533907301413, -21.53943276465977519, 92.49890960531436690 ) ) ;
#38740=CARTESIAN_POINT ( 'NONE',  ( 12.06949235617757843, -12.14591786802309237, 43.12390960531435269 ) ) ;
#38741=CARTESIAN_POINT ( 'NONE',  ( 16.53943276465976808, 0.05219959533934440121, 61.25109039468567573 ) ) ;
#38742=CARTESIAN_POINT ( 'NONE',  ( 19.03943276465977164, 0.05219959533936151252, 96.25109039468567573 ) ) ;
#38743=CARTESIAN_POINT ( 'NONE',  ( -5.719274019375978568, 21.55341960407610458, 100.2072429386476955 ) ) ;
#38744=CARTESIAN_POINT ( 'NONE',  ( 4.379528057220339221, -16.55341960407611168, 37.70724293864769550 ) ) ;
#38745=VERTEX_POINT ( 'NONE', #5549 ) ;
#38746=CARTESIAN_POINT ( 'NONE',  ( -8.224510206698735004, -14.34966873604973081, 84.58442372801903275 ) ) ;
#38748=CARTESIAN_POINT ( 'NONE',  ( 5.823673210054125526, 21.52544592524343514, 79.79057627198102409 ) ) ;
#38750=CARTESIAN_POINT ( 'NONE',  ( 8.224510206698742110, 14.34966873604972548, 112.0844237280190185 ) ) ;
#38752=CARTESIAN_POINT ( 'NONE',  ( 0.000000000000000000, 5.499999999999998224, 120.0000000000000142 ) ) ;
#38753=CARTESIAN_POINT ( 'NONE',  ( 21.53943276465977519, -0.05219959533907433946, 88.74890960531436690 ) ) ;
#38754=CARTESIAN_POINT ( 'NONE',  ( 10.72451020669898902, -18.67979575497178502, 112.9155762719810383 ) ) ;
#38755=CARTESIAN_POINT ( 'NONE',  ( -14.34966873604960291, -8.224510206698953496, 36.66557627198103120 ) ) ;
#38756=CARTESIAN_POINT ( 'NONE',  ( 16.52544592524335698, 4.483927247898782831, 36.45942372801901143 ) ) ;
#38757=CARTESIAN_POINT ( 'NONE',  ( -16.51473224551069308, -9.474510206698971260, 36.66557627198102409 ) ) ;
#38758=CARTESIAN_POINT ( 'NONE',  ( 9.564922557960805705, 16.46253265017160317, 69.58224293864770971 ) ) ;
#38759=CARTESIAN_POINT ( 'NONE',  ( -10.81492255796078084, -18.62759615963271287, 22.08224293864769194 ) ) ;
#38760=CARTESIAN_POINT ( 'NONE',  ( 15.50000000000000178, -5.500000000000000888, 118.0000000000000142 ) ) ;
#38761=CARTESIAN_POINT ( 'NONE',  ( -9.564922557961040184, 16.46253265017147172, 107.9177570613523471 ) ) ;
#38762=CARTESIAN_POINT ( 'NONE',  ( 5.153800228976615827, -19.02544592524334988, 45.20942372801901143 ) ) ;
#38763=CARTESIAN_POINT ( 'NONE',  ( 21.52544592524344225, -5.823673210054117533, 93.54057627198103830 ) ) ;
#38764=EDGE_CURVE ( 'NONE', #179099, #64402, #174823, .T. ) ;
#38765=CARTESIAN_POINT ( 'NONE',  ( -12.14591786802309592, -12.06949235617757132, 21.87390960531436690 ) ) ;
#38766=CARTESIAN_POINT ( 'NONE',  ( -15.72974639402197994, 15.80617190586746368, 45.62390960531436690 ) ) ;
#38767=CARTESIAN_POINT ( 'NONE',  ( -5.719274019375978568, 21.55341960407610458, 85.20724293864770971 ) ) ;
#38768=CARTESIAN_POINT ( 'NONE',  ( 16.51473224551083163, -9.474510206698727899, 105.8344237280190043 ) ) ;
#38769=CARTESIAN_POINT ( 'NONE',  ( 16.46253265017160672, -9.564922557960803928, 103.3322429386476955 ) ) ;
#38770=CARTESIAN_POINT ( 'NONE',  ( -18.62759615963255300, -10.81492255796106328, 79.16775706135234714 ) ) ;
#38771=CARTESIAN_POINT ( 'NONE',  ( 19.05341960407611168, 5.049401038298154454, 73.95724293864768129 ) ) ;
#38773=CARTESIAN_POINT ( 'NONE',  ( -4.379528057220328563, 16.55341960407611168, 100.2072429386476955 ) ) ;
#38775=CARTESIAN_POINT ( 'NONE',  ( 0.05219959533909260263, 19.03943276465977164, 64.99890960531436690 ) ) ;
#38776=CARTESIAN_POINT ( 'NONE',  ( -12.14591786802309592, -12.06949235617757132, 96.87390960531436690 ) ) ;
#38778=CARTESIAN_POINT ( 'NONE',  ( 16.46253265017146816, 9.564922557961045513, 101.6677570613523329 ) ) ;
#38780=CARTESIAN_POINT ( 'NONE',  ( -19.02544592524342804, 5.153800228976336051, 66.04057627198103830 ) ) ;
#38781=CARTESIAN_POINT ( 'NONE',  ( -21.53943276465977519, -0.05219959533937600094, 88.75109039468567573 ) ) ;
#38782=CARTESIAN_POINT ( 'NONE',  ( -13.89961937509977652, 13.97604488694528158, 105.6239096053143527 ) ) ;
#38783=CARTESIAN_POINT ( 'NONE',  ( -16.52544592524335698, -4.483927247898792601, 83.95942372801900433 ) ) ;
#38784=CARTESIAN_POINT ( 'NONE',  ( -16.88567814943164791, -6.947325034625700724, 76.29001122652587696 ) ) ;
#38785=CARTESIAN_POINT ( 'NONE',  ( 5.153800228976615827, -19.02544592524334988, 55.20942372801899722 ) ) ;
#38786=CARTESIAN_POINT ( 'NONE',  ( 21.53943276465977519, 0.05219959533937863772, 106.2510903946856757 ) ) ;
#38789=CARTESIAN_POINT ( 'NONE',  ( -16.55341960407611168, -4.379528057220339221, 21.45724293864769550 ) ) ;
#38791=CARTESIAN_POINT ( 'NONE',  ( 16.55341960407618274, -4.379528057220086978, 96.04275706135236135 ) ) ;
#38793=CARTESIAN_POINT ( 'NONE',  ( -0.05219959533934338120, 16.53943276465976808, 72.50109039468568994 ) ) ;
#38794=CARTESIAN_POINT ( 'NONE',  ( -21.55341960407619339, 5.719274019375674811, 83.54275706135234714 ) ) ;
#38795=CARTESIAN_POINT ( 'NONE',  ( -19.03943276465977164, -0.05219959533935918106, 88.75109039468567573 ) ) ;
#38796=CARTESIAN_POINT ( 'NONE',  ( 5.153800228976615827, -19.02544592524334988, 40.20942372801898301 ) ) ;
#38797=CARTESIAN_POINT ( 'NONE',  ( 16.51473224551069308, 9.474510206698969483, 59.16557627198102409 ) ) ;
#38798=CARTESIAN_POINT ( 'NONE',  ( -13.89961937509977652, 13.97604488694528158, 60.62390960531436690 ) ) ;
#38800=CARTESIAN_POINT ( 'NONE',  ( -15.80617190586745835, -15.72974639402198527, 81.87390960531435269 ) ) ;
#38802=CARTESIAN_POINT ( 'NONE',  ( 5.719274019375991003, -21.55341960407610458, 42.70724293864770260 ) ) ;
#38803=CARTESIAN_POINT ( 'NONE',  ( 5.153800228976335163, 19.02544592524342804, 34.79057627198102409 ) ) ;
#38804=CARTESIAN_POINT ( 'NONE',  ( 16.53943276465976808, 0.05219959533934440121, 61.25109039468567573 ) ) ;
#38806=CARTESIAN_POINT ( 'NONE',  ( 15.72974639402176855, 15.80617190586768217, 41.87609039468568284 ) ) ;
#38807=CARTESIAN_POINT ( 'NONE',  ( -16.55341960407611168, -4.379528057220339221, 61.45724293864770260 ) ) ;
#38809=CARTESIAN_POINT ( 'NONE',  ( 16.52544592524335698, 4.483927247898782831, 31.45942372801901854 ) ) ;
#38810=CARTESIAN_POINT ( 'NONE',  ( -13.89961937509957401, -13.97604488694547875, 49.37609039468567573 ) ) ;
#38811=CARTESIAN_POINT ( 'NONE',  ( 12.06949235617757843, -12.14591786802309237, 63.12390960531435979 ) ) ;
#38812=CARTESIAN_POINT ( 'NONE',  ( 21.55341960407619695, -5.719274019375665929, 31.04275706135234714 ) ) ;
#38814=CARTESIAN_POINT ( 'NONE',  ( 21.53943276465977519, -0.05219959533907433946, 88.74890960531436690 ) ) ;
#38815=CARTESIAN_POINT ( 'NONE',  ( -13.97604488694527625, -13.89961937509977652, 106.8739096053143669 ) ) ;
#38816=CARTESIAN_POINT ( 'NONE',  ( -4.483927247898539470, -16.52544592524342804, 77.29057627198102409 ) ) ;
#38818=DIRECTION ( 'NONE',  ( 0.000000000000000000, 0.000000000000000000, -1.000000000000000000 ) ) ;
#38819=CARTESIAN_POINT ( 'NONE',  ( -19.03943276465977164, -0.05219959533935918106, 63.75109039468566863 ) ) ;
#38820=CARTESIAN_POINT ( 'NONE',  ( 15.80617190586746368, 15.72974639402197994, 114.3739096053143527 ) ) ;
#38821=CARTESIAN_POINT ( 'NONE',  ( 5.049401038298161559, -19.05341960407611168, 52.70724293864767418 ) ) ;
#38822=CARTESIAN_POINT ( 'NONE',  ( 16.46253265017146816, 9.564922557961045513, 41.66775706135234003 ) ) ;
#38823=CARTESIAN_POINT ( 'NONE',  ( -16.51473224551069308, -9.474510206698971260, 26.66557627198103120 ) ) ;
#38824=CARTESIAN_POINT ( 'NONE',  ( 5.823673210054444382, -21.52544592524334988, 65.20942372801901854 ) ) ;
#38825=CARTESIAN_POINT ( 'NONE',  ( -17.26058549869094705, -6.457015423128475540, 71.37745837476069255 ) ) ;
#38826=CARTESIAN_POINT ( 'NONE',  ( -16.52544592524342804, 4.483927247898546575, 51.04057627198103120 ) ) ;
#38827=CARTESIAN_POINT ( 'NONE',  ( -13.97604488694527625, -13.89961937509977652, 61.87390960531435979 ) ) ;
#38828=CARTESIAN_POINT ( 'NONE',  ( 5.719274019375991003, -21.55341960407610458, 92.70724293864770971 ) ) ;
#38829=CARTESIAN_POINT ( 'NONE',  ( -16.51473224551069308, -9.474510206698971260, 51.66557627198102409 ) ) ;
#38830=ORIENTED_EDGE ( 'NONE', *, *, #27973, .F. ) ;
#38831=CARTESIAN_POINT ( 'NONE',  ( -5.719274019375978568, 21.55341960407610458, 70.20724293864769550 ) ) ;
#38832=CARTESIAN_POINT ( 'NONE',  ( -21.55341960407619339, 5.719274019375674811, 93.54275706135234714 ) ) ;
#38833=CARTESIAN_POINT ( 'NONE',  ( -9.564922557960796823, -16.46253265017161027, 27.08224293864769550 ) ) ;
#38834=CARTESIAN_POINT ( 'NONE',  ( 8.224510206698742110, 14.34966873604972548, 92.08442372801901854 ) ) ;
#38835=CARTESIAN_POINT ( 'NONE',  ( 14.29746914071049879, -8.314922557960816363, 78.33224293864770971 ) ) ;
#38836=CARTESIAN_POINT ( 'NONE',  ( -0.05219959533936034679, 19.03943276465977164, 92.50109039468566152 ) ) ;
#38838=CARTESIAN_POINT ( 'NONE',  ( -0.05219959533907301413, -21.53943276465977519, 112.4989096053143669 ) ) ;
#38839=CARTESIAN_POINT ( 'NONE',  ( -9.564922557961040184, 16.46253265017147172, 42.91775706135234003 ) ) ;
#38840=CARTESIAN_POINT ( 'NONE',  ( 8.314922557961029526, -14.29746914071037800, 100.4177570613523471 ) ) ;
#38842=CARTESIAN_POINT ( 'NONE',  ( 19.03943276465977164, 0.05219959533936151252, 31.25109039468566863 ) ) ;
#38843=CARTESIAN_POINT ( 'NONE',  ( -13.97604488694527625, -13.89961937509977652, 86.87390960531436690 ) ) ;
#38844=CARTESIAN_POINT ( 'NONE',  ( -18.67979575497178146, -10.72451020669898902, 56.66557627198103830 ) ) ;
#38845=CARTESIAN_POINT ( 'NONE',  ( -18.22780087662114212, 5.499999999999995559, 48.51540105326107266 ) ) ;
#38846=CARTESIAN_POINT ( 'NONE',  ( -12.06949235617756955, 12.14591786802309770, 115.6239096053143669 ) ) ;
#38847=CARTESIAN_POINT ( 'NONE',  ( -18.62759615963255300, -10.81492255796106328, 104.1677570613523471 ) ) ;
#38848=CARTESIAN_POINT ( 'NONE',  ( 12.06949235617739724, 12.14591786802326823, 81.87609039468568994 ) ) ;
#38849=CARTESIAN_POINT ( 'NONE',  ( 15.72974639402176855, 15.80617190586768217, 26.87609039468567218 ) ) ;
#38850=CARTESIAN_POINT ( 'NONE',  ( -4.483927247898782831, 16.52544592524335698, 32.70942372801900433 ) ) ;
#38851=CARTESIAN_POINT ( 'NONE',  ( 9.474510206698971260, -16.51473224551069308, 107.9155762719810383 ) ) ;
#38852=CARTESIAN_POINT ( 'NONE',  ( 16.46253265017160672, -9.564922557960803928, 38.33224293864768839 ) ) ;
#38853=CARTESIAN_POINT ( 'NONE',  ( -16.46253265017160317, 9.564922557960807481, 65.83224293864769550 ) ) ;
#38854=CARTESIAN_POINT ( 'NONE',  ( 4.379528057220092307, 16.55341960407617563, 42.29275706135235424 ) ) ;
#38855=CARTESIAN_POINT ( 'NONE',  ( -8.314922557960811034, -14.29746914071050412, 97.08224293864770971 ) ) ;
#38856=CARTESIAN_POINT ( 'NONE',  ( -16.53943276465976808, -0.05219959533934237506, 98.75109039468568994 ) ) ;
#38857=CARTESIAN_POINT ( 'NONE',  ( -10.72451020669870658, -18.67979575497194134, 54.58442372801901143 ) ) ;
#38858=CARTESIAN_POINT ( 'NONE',  ( 9.474510206698971260, -16.51473224551069308, 77.91557627198103830 ) ) ;
#38859=CARTESIAN_POINT ( 'NONE',  ( 5.049401038298161559, -19.05341960407611168, 62.70724293864769550 ) ) ;
#38860=CARTESIAN_POINT ( 'NONE',  ( 13.89961937509977652, -13.97604488694527269, 98.12390960531433848 ) ) ;
#38862=CARTESIAN_POINT ( 'NONE',  ( -14.29746914071049879, 8.314922557960819915, 45.83224293864769550 ) ) ;
#38863=CARTESIAN_POINT ( 'NONE',  ( -12.14591786802326823, 12.06949235617739902, 93.12609039468568994 ) ) ;
#38865=CARTESIAN_POINT ( 'NONE',  ( 19.03943276465977164, 0.05219959533936151252, 46.25109039468566863 ) ) ;
#38867=CARTESIAN_POINT ( 'NONE',  ( 5.153800228976335163, 19.02544592524342804, 59.79057627198100988 ) ) ;
#38868=CARTESIAN_POINT ( 'NONE',  ( 19.02544592524334988, 5.153800228976608722, 36.45942372801900433 ) ) ;
#38870=CARTESIAN_POINT ( 'NONE',  ( -16.81555441253549787, -7.025013491695498047, 64.36314554665743515 ) ) ;
#38871=CARTESIAN_POINT ( 'NONE',  ( 16.53943276465976808, 0.05219959533934440121, 51.25109039468568994 ) ) ;
#38872=CARTESIAN_POINT ( 'NONE',  ( 13.89961937509957401, 13.97604488694547697, 76.87609039468566152 ) ) ;
#38873=CARTESIAN_POINT ( 'NONE',  ( -8.314922557961024197, 14.29746914071037800, 72.91775706135234714 ) ) ;
#38874=CARTESIAN_POINT ( 'NONE',  ( -16.46253265017160317, 9.564922557960807481, 95.83224293864769550 ) ) ;
#38875=CARTESIAN_POINT ( 'NONE',  ( -0.05219959533907301413, -21.53943276465977519, 107.4989096053143669 ) ) ;
#38876=CARTESIAN_POINT ( 'NONE',  ( -16.46253265017146816, -9.564922557961047289, 74.16775706135234714 ) ) ;
#38877=CARTESIAN_POINT ( 'NONE',  ( 9.564922557960805705, 16.46253265017160317, 99.58224293864770971 ) ) ;
#38878=CARTESIAN_POINT ( 'NONE',  ( -13.89961937509977652, 13.97604488694528158, 35.62390960531435269 ) ) ;
#38879=CARTESIAN_POINT ( 'NONE',  ( 16.51473224551069308, 9.474510206698969483, 94.16557627198103830 ) ) ;
#38880=CARTESIAN_POINT ( 'NONE',  ( 8.314922557960818139, 14.29746914071049879, 49.58224293864769550 ) ) ;
#38881=CARTESIAN_POINT ( 'NONE',  ( 19.02544592524343514, -5.153800228976328945, 33.54057627198102409 ) ) ;
#38882=CARTESIAN_POINT ( 'NONE',  ( -5.049401038297874678, -19.05341960407617918, 44.79275706135232582 ) ) ;
#38883=CARTESIAN_POINT ( 'NONE',  ( -16.52544592524342804, 4.483927247898546575, 86.04057627198102409 ) ) ;
#38884=CARTESIAN_POINT ( 'NONE',  ( 18.62759615963255655, 10.81492255796105972, 111.6677570613523613 ) ) ;
#38885=CARTESIAN_POINT ( 'NONE',  ( -16.51473224551069308, -9.474510206698971260, 51.66557627198102409 ) ) ;
#38886=CARTESIAN_POINT ( 'NONE',  ( -15.80617190586745835, -15.72974639402198527, 66.87390960531436690 ) ) ;
#38887=CARTESIAN_POINT ( 'NONE',  ( 14.29746914071049879, -8.314922557960816363, 48.33224293864770260 ) ) ;
#38888=CARTESIAN_POINT ( 'NONE',  ( 5.049401038297881783, 19.05341960407617563, 22.29275706135233648 ) ) ;
#38889=CARTESIAN_POINT ( 'NONE',  ( -19.02544592524342804, 5.153800228976336051, 111.0405762719810099 ) ) ;
#38890=CARTESIAN_POINT ( 'NONE',  ( -19.05341960407611168, -5.049401038298163336, 106.4572429386476955 ) ) ;
#38891=CARTESIAN_POINT ( 'NONE',  ( 19.02544592524343514, -5.153800228976328945, 43.54057627198103120 ) ) ;
#38892=CARTESIAN_POINT ( 'NONE',  ( 19.03943276465977164, -0.05219959533909143690, 23.74890960531435269 ) ) ;
#38893=CARTESIAN_POINT ( 'NONE',  ( 8.224510206698953496, -14.34966873604960469, 82.91557627198103830 ) ) ;
#38894=CARTESIAN_POINT ( 'NONE',  ( -10.81492255796078084, -18.62759615963271287, 92.08224293864769550 ) ) ;
#38895=CARTESIAN_POINT ( 'NONE',  ( -9.564922557960796823, -16.46253265017161027, 107.0822429386476955 ) ) ;
#38896=CARTESIAN_POINT ( 'NONE',  ( 5.823673210054125526, 21.52544592524343514, 114.7905762719810383 ) ) ;
#38897=CARTESIAN_POINT ( 'NONE',  ( -13.89961937509977652, 13.97604488694528158, 105.6239096053143527 ) ) ;
#38898=CARTESIAN_POINT ( 'NONE',  ( -0.05219959533910754901, -16.53943276465976808, 97.49890960531436690 ) ) ;
#38899=CARTESIAN_POINT ( 'NONE',  ( -21.53943276465977519, -0.05219959533937600094, 73.75109039468567573 ) ) ;
#38900=CARTESIAN_POINT ( 'NONE',  ( 21.53943276465977519, -0.05219959533907433946, 83.74890960531435269 ) ) ;
#38901=CARTESIAN_POINT ( 'NONE',  ( 17.48847506799970120, -5.747544572773742644, 108.3269743784328227 ) ) ;
#38904=CARTESIAN_POINT ( 'NONE',  ( -12.14591786802326823, 12.06949235617739902, 28.12609039468568284 ) ) ;
#38905=CARTESIAN_POINT ( 'NONE',  ( 12.14591786802309770, 12.06949235617756955, 109.3739096053143811 ) ) ;
#38906=CARTESIAN_POINT ( 'NONE',  ( -17.50000000000146372, -3.254303733634626106, 109.9760410692859267 ) ) ;
#38907=CARTESIAN_POINT ( 'NONE',  ( -13.89961937509977652, 13.97604488694528158, 65.62390960531436690 ) ) ;
#38908=CARTESIAN_POINT ( 'NONE',  ( 4.483927247898545687, 16.52544592524342804, 94.79057627198105251 ) ) ;
#38909=CARTESIAN_POINT ( 'NONE',  ( -10.81492255796078084, -18.62759615963271287, 37.08224293864768129 ) ) ;
#38910=CARTESIAN_POINT ( 'NONE',  ( 4.483927247898545687, 16.52544592524342804, 69.79057627198102409 ) ) ;
#38911=CARTESIAN_POINT ( 'NONE',  ( 13.89961937509957401, 13.97604488694547697, 111.8760903946856757 ) ) ;
#38912=CARTESIAN_POINT ( 'NONE',  ( 21.53943276465977519, 0.05219959533937863772, 76.25109039468568994 ) ) ;
#38913=CARTESIAN_POINT ( 'NONE',  ( 18.22780087662126647, 5.499999999999818812, 61.48236817873107185 ) ) ;
#38914=CARTESIAN_POINT ( 'NONE',  ( 19.03943276465977164, -0.05219959533909143690, 113.7489096053143669 ) ) ;
#38915=CARTESIAN_POINT ( 'NONE',  ( 4.483927247898790824, -16.52544592524335698, 95.20942372801903275 ) ) ;
#38916=CARTESIAN_POINT ( 'NONE',  ( 13.97604488694527802, 13.89961937509977652, 34.37390960531436690 ) ) ;
#38917=CARTESIAN_POINT ( 'NONE',  ( 13.89961937509977652, -13.97604488694527269, 83.12390960531436690 ) ) ;
#38918=CARTESIAN_POINT ( 'NONE',  ( -21.53943276465977519, 0.05219959533907696930, 101.2489096053143669 ) ) ;
#38919=CARTESIAN_POINT ( 'NONE',  ( -16.53943276465976808, -0.05219959533934237506, 23.75109039468567929 ) ) ;
#38920=CARTESIAN_POINT ( 'NONE',  ( -16.52544592524342804, 4.483927247898546575, 46.04057627198103830 ) ) ;
#38921=CARTESIAN_POINT ( 'NONE',  ( 21.55341960407619695, -5.719274019375665929, 76.04275706135237556 ) ) ;
#38922=CARTESIAN_POINT ( 'NONE',  ( 0.05219959533934541429, -16.53943276465976808, 95.00109039468568994 ) ) ;
#38923=CARTESIAN_POINT ( 'NONE',  ( 16.61371651742640054, -7.165104196375913226, 46.35415069992970416 ) ) ;
#38924=CARTESIAN_POINT ( 'NONE',  ( -17.44279575226823198, 5.990770900252464060, 80.83557567514318976 ) ) ;
#38925=CARTESIAN_POINT ( 'NONE',  ( 12.06949235617757843, -12.14591786802309237, 28.12390960531435979 ) ) ;
#38926=CARTESIAN_POINT ( 'NONE',  ( 16.55341960407618274, -4.379528057220086978, 56.04275706135235424 ) ) ;
#38927=CARTESIAN_POINT ( 'NONE',  ( 19.03943276465977164, -0.05219959533909143690, 73.74890960531435269 ) ) ;
#38928=CARTESIAN_POINT ( 'NONE',  ( 13.89961937509977652, -13.97604488694527269, 88.12390960531438111 ) ) ;
#38929=CARTESIAN_POINT ( 'NONE',  ( 18.62759615963255655, 10.81492255796105972, 91.66775706135234714 ) ) ;
#38930=CARTESIAN_POINT ( 'NONE',  ( 0.05219959533934541429, -16.53943276465976808, 95.00109039468568994 ) ) ;
#38931=CARTESIAN_POINT ( 'NONE',  ( 4.483927247898545687, 16.52544592524342804, 64.79057627198103830 ) ) ;
#38932=CARTESIAN_POINT ( 'NONE',  ( 19.02544592524343514, -5.153800228976328945, 73.54057627198103830 ) ) ;
#38934=CARTESIAN_POINT ( 'NONE',  ( 5.153800228976615827, -19.02544592524334988, 110.2094237280189901 ) ) ;
#38935=CARTESIAN_POINT ( 'NONE',  ( 12.14591786802309770, 12.06949235617756955, 114.3739096053143527 ) ) ;
#38936=CARTESIAN_POINT ( 'NONE',  ( 0.05219959533909260263, 19.03943276465977164, 84.99890960531436690 ) ) ;
#38937=CARTESIAN_POINT ( 'NONE',  ( -19.02544592524334988, -5.153800228976617603, 108.9594237280189759 ) ) ;
#38939=CARTESIAN_POINT ( 'NONE',  ( 21.52544592524334988, 5.823673210054432836, 106.4594237280190328 ) ) ;
#38940=CARTESIAN_POINT ( 'NONE',  ( -16.55341960407617563, 4.379528057220093196, 83.54275706135234714 ) ) ;
#38941=CARTESIAN_POINT ( 'NONE',  ( -19.03943276465977164, -0.05219959533935918106, 93.75109039468566152 ) ) ;
#38942=CARTESIAN_POINT ( 'NONE',  ( -12.14591786802309592, -12.06949235617757132, 111.8739096053143669 ) ) ;
#38943=CARTESIAN_POINT ( 'NONE',  ( 12.14591786802327356, -12.06949235617739191, 70.62609039468567573 ) ) ;
#38945=CARTESIAN_POINT ( 'NONE',  ( 9.564922557961047289, -16.46253265017146816, 55.41775706135234003 ) ) ;
#38946=CARTESIAN_POINT ( 'NONE',  ( 0.05219959533937995610, -21.53943276465977519, 100.0010903946857042 ) ) ;
#38947=CARTESIAN_POINT ( 'NONE',  ( 0.05219959533909260263, 19.03943276465977164, 39.99890960531436690 ) ) ;
#38948=CARTESIAN_POINT ( 'NONE',  ( 0.05219959533909260263, 19.03943276465977164, 74.99890960531435269 ) ) ;
#38949=CARTESIAN_POINT ( 'NONE',  ( -12.14591786802309592, -12.06949235617757132, 71.87390960531438111 ) ) ;
#38951=CARTESIAN_POINT ( 'NONE',  ( 15.80617190586769283, -15.72974639402175789, 85.62609039468568994 ) ) ;
#38952=CARTESIAN_POINT ( 'NONE',  ( -13.97604488694547697, 13.89961937509957934, 43.12609039468566152 ) ) ;
#38953=CARTESIAN_POINT ( 'NONE',  ( -16.51473224551082808, 9.474510206698731452, 38.33442372801899722 ) ) ;
#38954=CARTESIAN_POINT ( 'NONE',  ( -5.719274019375978568, 21.55341960407610458, 40.20724293864769550 ) ) ;
#38955=CARTESIAN_POINT ( 'NONE',  ( -15.80617190586768217, 15.72974639402176855, 93.12609039468568994 ) ) ;
#38956=CARTESIAN_POINT ( 'NONE',  ( -5.049401038298153566, 19.05341960407611168, 80.20724293864769550 ) ) ;
#38957=CARTESIAN_POINT ( 'NONE',  ( 10.81492255796106328, -18.62759615963255655, 95.41775706135234714 ) ) ;
#38958=CARTESIAN_POINT ( 'NONE',  ( -21.55341960407610458, -5.719274019375992779, 46.45724293864769550 ) ) ;
#38959=CARTESIAN_POINT ( 'NONE',  ( -5.049401038298153566, 19.05341960407611168, 80.20724293864769550 ) ) ;
#38960=CARTESIAN_POINT ( 'NONE',  ( 9.474510206698729675, 16.51473224551082808, 77.08442372801900433 ) ) ;
#38961=CARTESIAN_POINT ( 'NONE',  ( 19.05341960407611168, 5.049401038298154454, 98.95724293864766707 ) ) ;
#38963=CARTESIAN_POINT ( 'NONE',  ( -0.05219959533936034679, 19.03943276465977164, 92.50109039468566152 ) ) ;
#38964=CARTESIAN_POINT ( 'NONE',  ( 4.379528057220092307, 16.55341960407617563, 37.29275706135235424 ) ) ;
#38965=CARTESIAN_POINT ( 'NONE',  ( -14.34966873604960291, -8.224510206698953496, 101.6655762719810383 ) ) ;
#38966=CARTESIAN_POINT ( 'NONE',  ( -19.05341960407611168, -5.049401038298163336, 71.45724293864766707 ) ) ;
#38967=CARTESIAN_POINT ( 'NONE',  ( -15.80617190586745835, -15.72974639402198527, 66.87390960531436690 ) ) ;
#38968=CARTESIAN_POINT ( 'NONE',  ( 14.34966873604972726, -8.224510206698740333, 35.83442372801901143 ) ) ;
#38969=CARTESIAN_POINT ( 'NONE',  ( 5.719274019375673035, 21.55341960407619339, 37.29275706135235424 ) ) ;
#38970=CARTESIAN_POINT ( 'NONE',  ( -21.55341960407619339, 5.719274019375674811, 83.54275706135234714 ) ) ;
#38971=CARTESIAN_POINT ( 'NONE',  ( -8.224510206698735004, -14.34966873604973081, 89.58442372801901854 ) ) ;
#38972=CARTESIAN_POINT ( 'NONE',  ( 9.564922557960805705, 16.46253265017160317, 69.58224293864770971 ) ) ;
#38973=CARTESIAN_POINT ( 'NONE',  ( -12.14591786802309592, -12.06949235617757132, 71.87390960531438111 ) ) ;
#38974=CARTESIAN_POINT ( 'NONE',  ( -14.34966873604972548, 8.224510206698743886, 108.3344237280190185 ) ) ;
#38975=CARTESIAN_POINT ( 'NONE',  ( 9.564922557961047289, -16.46253265017146816, 50.41775706135233293 ) ) ;
#38976=CARTESIAN_POINT ( 'NONE',  ( 18.62759615963255655, 10.81492255796105972, 31.66775706135234358 ) ) ;
#38977=EDGE_CURVE ( 'NONE', #44164, #177566, #37900, .T. ) ;
#38978=CARTESIAN_POINT ( 'NONE',  ( -16.55341960407611168, -4.379528057220339221, 76.45724293864769550 ) ) ;
#38979=CARTESIAN_POINT ( 'NONE',  ( -9.564922557960796823, -16.46253265017161027, 97.08224293864769550 ) ) ;
#38980=CARTESIAN_POINT ( 'NONE',  ( -12.14591786802326823, 12.06949235617739902, 98.12609039468570415 ) ) ;
#38981=CARTESIAN_POINT ( 'NONE',  ( -10.72451020669870658, -18.67979575497194134, 74.58442372801901854 ) ) ;
#38982=CARTESIAN_POINT ( 'NONE',  ( -14.29746914071037622, -8.314922557961029526, 44.16775706135234714 ) ) ;
#38983=CARTESIAN_POINT ( 'NONE',  ( 10.72451020669871369, 18.67979575497193778, 37.08442372801901143 ) ) ;
#38984=CARTESIAN_POINT ( 'NONE',  ( 4.379528057220339221, -16.55341960407611168, 72.70724293864769550 ) ) ;
#38985=ORIENTED_EDGE ( 'NONE', *, *, #131013, .F. ) ;
#38986=CARTESIAN_POINT ( 'NONE',  ( -10.72451020669898014, 18.67979575497178502, 115.4155762719810241 ) ) ;
#38987=CARTESIAN_POINT ( 'NONE',  ( 17.50000000000001066, -5.076555817581232866, 26.32048507950225869 ) ) ;
#38988=CARTESIAN_POINT ( 'NONE',  ( -8.224510206698948167, 14.34966873604960824, 55.41557627198102409 ) ) ;
#38989=CARTESIAN_POINT ( 'NONE',  ( -13.89961937509977652, 13.97604488694528158, 30.62390960531435269 ) ) ;
#38990=CARTESIAN_POINT ( 'NONE',  ( 18.67979575497178502, 10.72451020669898547, 44.16557627198103120 ) ) ;
#38991=CARTESIAN_POINT ( 'NONE',  ( 14.29746914071049879, -8.314922557960816363, 78.33224293864770971 ) ) ;
#38992=CARTESIAN_POINT ( 'NONE',  ( -18.67979575497178146, -10.72451020669898902, 81.66557627198103830 ) ) ;
#38993=CARTESIAN_POINT ( 'NONE',  ( 9.474510206698971260, -16.51473224551069308, 92.91557627198103830 ) ) ;
#38994=CARTESIAN_POINT ( 'NONE',  ( 13.97604488694527802, 13.89961937509977652, 44.37390960531435269 ) ) ;
#38995=CARTESIAN_POINT ( 'NONE',  ( -19.02544592524334988, -5.153800228976617603, 78.95942372801900433 ) ) ;
#38996=CARTESIAN_POINT ( 'NONE',  ( 0.05219959533937995610, -21.53943276465977519, 60.00109039468568284 ) ) ;
#38997=CARTESIAN_POINT ( 'NONE',  ( 21.53943276465977519, -0.05219959533907433946, 63.74890960531435979 ) ) ;
#38998=CARTESIAN_POINT ( 'NONE',  ( 13.97604488694527802, 13.89961937509977652, 34.37390960531436690 ) ) ;
#38999=CARTESIAN_POINT ( 'NONE',  ( -5.049401038298153566, 19.05341960407611168, 75.20724293864769550 ) ) ;
#39000=ORIENTED_EDGE ( 'NONE', *, *, #167117, .T. ) ;
#39001=CARTESIAN_POINT ( 'NONE',  ( 4.379528057220092307, 16.55341960407617563, 52.29275706135236135 ) ) ;
#39002=CARTESIAN_POINT ( 'NONE',  ( -0.05219959533937732626, 21.53943276465977519, 37.50109039468568284 ) ) ;
#39004=CARTESIAN_POINT ( 'NONE',  ( -5.823673210054431948, 21.52544592524334988, 72.70942372801901854 ) ) ;
#39005=CARTESIAN_POINT ( 'NONE',  ( 9.474510206698971260, -16.51473224551069308, 97.91557627198102409 ) ) ;
#39006=CARTESIAN_POINT ( 'NONE',  ( -18.67979575497178146, -10.72451020669898902, 81.66557627198103830 ) ) ;
#39007=CARTESIAN_POINT ( 'NONE',  ( 18.67979575497194134, -10.72451020669871369, 30.83442372801902209 ) ) ;
#39008=CARTESIAN_POINT ( 'NONE',  ( 4.483927247898790824, -16.52544592524335698, 50.20942372801901854 ) ) ;
#39009=CARTESIAN_POINT ( 'NONE',  ( 10.81492255796078972, 18.62759615963270932, 54.58224293864769550 ) ) ;
#39010=CARTESIAN_POINT ( 'NONE',  ( -15.72974639402176322, -15.80617190586768395, 109.3760903946857042 ) ) ;
#39011=CARTESIAN_POINT ( 'NONE',  ( -13.97604488694527625, -13.89961937509977652, 56.87390960531434558 ) ) ;
#39012=CARTESIAN_POINT ( 'NONE',  ( -16.46253265017160317, 9.564922557960807481, 105.8322429386476955 ) ) ;
#39013=CARTESIAN_POINT ( 'NONE',  ( 16.51473224551069308, 9.474510206698969483, 94.16557627198103830 ) ) ;
#39015=CARTESIAN_POINT ( 'NONE',  ( 13.89961937509957401, 13.97604488694547697, 61.87609039468566863 ) ) ;
#39016=CARTESIAN_POINT ( 'NONE',  ( 21.53943276465977519, -0.05219959533907433946, 38.74890960531435979 ) ) ;
#39017=CARTESIAN_POINT ( 'NONE',  ( 4.379528057220339221, -16.55341960407611168, 27.70724293864769905 ) ) ;
#39018=CARTESIAN_POINT ( 'NONE',  ( 5.153800228976615827, -19.02544592524334988, 100.2094237280190043 ) ) ;
#39020=CARTESIAN_POINT ( 'NONE',  ( -5.823673210054431948, 21.52544592524334988, 112.7094237280190328 ) ) ;
#39021=CARTESIAN_POINT ( 'NONE',  ( -9.564922557961040184, 16.46253265017147172, 102.9177570613523329 ) ) ;
#39022=CARTESIAN_POINT ( 'NONE',  ( 19.05341960407617918, -5.049401038297876454, 61.04275706135232582 ) ) ;
#39024=CARTESIAN_POINT ( 'NONE',  ( 13.89961937509977652, -13.97604488694527269, 53.12390960531434558 ) ) ;
#39025=CARTESIAN_POINT ( 'NONE',  ( -14.34966873604960291, -8.224510206698953496, 61.66557627198103120 ) ) ;
#39026=CARTESIAN_POINT ( 'NONE',  ( 13.89961937509977652, -13.97604488694527269, 33.12390960531434558 ) ) ;
#39027=CARTESIAN_POINT ( 'NONE',  ( -4.379528057220328563, 16.55341960407611168, 35.20724293864768839 ) ) ;
#39029=CARTESIAN_POINT ( 'NONE',  ( -12.14591786802326823, 12.06949235617739902, 103.1260903946856757 ) ) ;
#39030=CARTESIAN_POINT ( 'NONE',  ( -19.05341960407611168, -5.049401038298163336, 66.45724293864769550 ) ) ;
#39031=CARTESIAN_POINT ( 'NONE',  ( 5.049401038297881783, 19.05341960407617563, 22.29275706135233648 ) ) ;
#39032=CARTESIAN_POINT ( 'NONE',  ( 14.34966873604972726, -8.224510206698740333, 30.83442372801902209 ) ) ;
#39033=CARTESIAN_POINT ( 'NONE',  ( -10.81492255796078084, -18.62759615963271287, 52.08224293864768839 ) ) ;
#39034=CARTESIAN_POINT ( 'NONE',  ( -10.81492255796105439, 18.62759615963255655, 107.9177570613523471 ) ) ;
#39035=CARTESIAN_POINT ( 'NONE',  ( -9.564922557960796823, -16.46253265017161027, 67.08224293864769550 ) ) ;
#39036=CARTESIAN_POINT ( 'NONE',  ( -9.564922557960796823, -16.46253265017161027, 102.0822429386477097 ) ) ;
#39037=CARTESIAN_POINT ( 'NONE',  ( -19.05341960407611168, -5.049401038298163336, 96.45724293864769550 ) ) ;
#39038=CARTESIAN_POINT ( 'NONE',  ( 18.62759615963255655, 10.81492255796105972, 21.66775706135235069 ) ) ;
#39039=CARTESIAN_POINT ( 'NONE',  ( -14.34966873604960291, -8.224510206698953496, 91.66557627198103830 ) ) ;
#39040=CARTESIAN_POINT ( 'NONE',  ( 10.72451020669898902, -18.67979575497178502, 82.91557627198103830 ) ) ;
#39041=CARTESIAN_POINT ( 'NONE',  ( -13.89961937509977652, 13.97604488694528158, 70.62390960531432427 ) ) ;
#39042=CARTESIAN_POINT ( 'NONE',  ( -0.05219959533909027116, -19.03943276465977164, 67.49890960531436690 ) ) ;
#39043=CARTESIAN_POINT ( 'NONE',  ( -10.72451020669898014, 18.67979575497178502, 115.4155762719810241 ) ) ;
#39045=CARTESIAN_POINT ( 'NONE',  ( -16.46253265017160317, 9.564922557960807481, 70.83224293864770971 ) ) ;
#39046=CARTESIAN_POINT ( 'NONE',  ( 19.26498983726236958, -5.499999999999790390, 98.05319577422005750 ) ) ;
#39047=CARTESIAN_POINT ( 'NONE',  ( 8.224510206698953496, -14.34966873604960469, 102.9155762719810383 ) ) ;
#39048=CARTESIAN_POINT ( 'NONE',  ( -16.51473224551069308, -9.474510206698971260, 21.66557627198102765 ) ) ;
#39049=CARTESIAN_POINT ( 'NONE',  ( 9.564922557961047289, -16.46253265017146816, 95.41775706135233293 ) ) ;
#39050=CARTESIAN_POINT ( 'NONE',  ( -16.53943276465976808, 0.05219959533911058130, 101.2489096053143669 ) ) ;
#39051=CARTESIAN_POINT ( 'NONE',  ( -21.55341960407619339, 5.719274019375674811, 68.54275706135234714 ) ) ;
#39052=CARTESIAN_POINT ( 'NONE',  ( -19.03943276465977164, 0.05219959533909376836, 61.24890960531436690 ) ) ;
#39053=CARTESIAN_POINT ( 'NONE',  ( -21.52544592524334988, -5.823673210054445271, 28.95942372801902209 ) ) ;
#39054=CARTESIAN_POINT ( 'NONE',  ( 5.823673210054125526, 21.52544592524343514, 109.7905762719810383 ) ) ;
#39056=CARTESIAN_POINT ( 'NONE',  ( -5.153800228976328057, -19.02544592524343514, 67.29057627198102409 ) ) ;
#39058=CARTESIAN_POINT ( 'NONE',  ( 4.379528057220092307, 16.55341960407617563, 22.29275706135235069 ) ) ;
#39059=CARTESIAN_POINT ( 'NONE',  ( -21.55341960407610458, -5.719274019375992779, 36.45724293864768839 ) ) ;
#39060=CARTESIAN_POINT ( 'NONE',  ( -18.67979575497193778, 10.72451020669871902, 63.33442372801900433 ) ) ;
#39061=CARTESIAN_POINT ( 'NONE',  ( -19.03943276465977164, 0.05219959533909376836, 116.2489096053143669 ) ) ;
#39062=( BOUNDED_SURFACE ( )  B_SPLINE_SURFACE ( 3, 2, ( 
 ( #156989, #32658, #2305, #143794, #159968, #96294, #98266, #4279, #157981, #63986, #3299, #142798, #81118, #50807, #128620, #35628, #36609, #94312, #173160, #155990, #65959, #21455, #186356, #189330, #127630, #125656, #6276, #124660, #158961, #188331, #48823, #80136, #18487, #20451, #47836, #79144, #144793, #141806, #17487, #112465, #64971, #187353, #190313, #49810, #110476, #174157, #172158, #95305, #5277, #51789, #113449, #175142, #83116, #179162, #99282, #23463, #37620, #162969, #101279, #161967, #116466, #176150, #8289, #9302, #69967, #70968, #132636, #177159, #117463, #178155, #130619, #131633, #85110, #146796, #191304, #160969, #22463, #194324, #193317, #39620, #52780, #54791, #38632, #100289, #114449, #24475, #86125, #129608, #84111, #145790, #147816, #67954, #55792, #7272, #68956, #192315, #53795, #115470, #39908, #127912, #22750, #84399, #145078, #98565, #114748, #189614, #82396, #85405, #6560, #113735, #174442, #192602, #36901, #146075, #131924, #21749, #129891, #176442, #178440, #68238, #112748, #24766, #35911, #191591, #97557, #23755, #159245, #20740, #144084, #37915, #54085, #147097, #115759, #8582, #193608, #99574, #161256, #101574, #55080, #116750, #53070, #160259, #5565, #7560, #175432, #100574, #67244, #69246, #163264, #51088, #162256, #128903, #130912, #70256, #86413, #83400, #177447, #190603, #52079, #38917, #4560, #66252, #102590, #27763, #151095, #87415, #88401, #57091, #150095, #166264, #9590, #135920, #183409, #71255, #89406, #12586, #11598, #41926, #58083, #132919, #25769, #28750, #73266, #118765, #117759, #196613, #120724, #42914, #44892, #152071, #134935, #105565, #106549, #164274, #136894, #168225, #165267, #149100, #40917, #74251, #119753, #29722, #197591, #10590, #26761, #179451, #43902, #181436, #13556, #72251, #133929, #194606, #195619, #182424, #180454, #104580, #148098, #167251, #90386, #59057, #121716, #103592, #75222, #56078, #198581, #60049, #351, #1342, #170214, #153046, #185384, #110518, #188374, #184397, #171210, #139853, #172199, #173201, #61035, #140856, #199566, #156030, #16537, #78184, #137885, #33684, #48863, #14547, #92363, #107530, #109528, #91354, #79186, #17527, #47875, #95347, #157031, #2345, #18529, #32700, #108535, #63023, #80176, #141848, #3339, #186398, #124701, #111516, #62021, #94351, #31707, #65013, #45877, #30715, #122707, #187395, #64026, #169207, #125696, #126670, #154049, #15544, #77202, #138871, #93356, #49851, #76206, #123685, #46874, #155042, #112505, #192358, #70009, #6317, #8333, #114492, #144833, #174199, #113491, #52823, #191345, #161011, #38676, #145831, #146840, #19513, #21498, #142840, #176194, #131678, #96335, #99328, #83159, #50848, #116509, #34677, #7313, #98310, #159001, #190355, #128660, #68998, #158022, #189371, #54835, #51832, #81158, #22505, #175186, #35667, #177203, #36652, #97315, #84152, #66002, #4319, #20494, #127671, #130664, #23506, #37663, #82142, #143838, #67996, #5317, #53841, #115515, #129649, #100332, #67001, #162010, #85154, #193359, #160010, #105323, #180210, #136649, #150852, #10345, #57844, #26516, #134690, #163012, #132679, #71011, #13321, #196375, #24519, #194367, #59807, #166020, #167011, #119516, #178197, #55834, #149845, #117507, #197352, #74010, #88160, #27520, #179204, #181198, #28512, #42675, #90147, #151831, #41680, #198331, #12346, #72001, #104336, #11349, #89161, #86170, #40672, #102342, #74986, #135680, #58816, #147860, #120484, #103344, #165023, #9346, #182175, #43661, #39662, #164031, #25529, #101323, #87173, #148854, #133675, #195366, #56845, #118521, #73020, #125465, #62779, #138632, #93117, #187162, #140621, #171967, #16300, #169973, #141620, #92119, #154802, #61782, #110285, #14303, #60795, #91121, #17291, #94115, #29488, #155794, #108294, #152810, #75970, #137643, #45640, #123451, #63792, #2111, #122467, #153807, #199330, #184159, #78945, #156802, #77950, #95113, #1103, #31465 ),
 ( #183170, #186157, #139617, #107292, #3109, #121477, #32462, #185143, #168963, #76961, #15301, #48633, #44653, #30469, #106306, #113, #167991, #47636, #46634, #124460, #33454, #109290, #170969, #18295, #79950, #34447, #21264, #38435, #4088, #66763, #173966, #174952, #143597, #126446, #158769, #83916, #161775, #157795, #144597, #113260, #145598, #146593, #96106, #52591, #97086, #82920, #192114, #81904, #190120, #36415, #100091, #128424, #172969, #84914, #19286, #51596, #80933, #7077, #142609, #65766, #127436, #98069, #114251, #68758, #175957, #130415, #53596, #159769, #6083, #23270, #115272, #176965, #5081, #20258, #189142, #67762, #35434, #160777, #50615, #129419, #64785, #188144, #22266, #112274, #191117, #49616, #111279, #37426, #99086, #54593, #24279, #40431, #102102, #72781, #162770, #87921, #11106, #147617, #148614, #117269, #10105, #26279, #69764, #196136, #43425, #131433, #149608, #134451, #71765, #163787, #118280, #193119, #85928, #88925, #133435, #178962, #177957, #56606, #180959, #103104, #105094, #12113, #195124, #165782, #166780, #9104, #197118, #28281, #25288, #70771, #101085, #57607, #179971, #89920, #119276, #132440, #86931, #39425, #104099, #41437, #73776, #194131, #55594, #116267, #164785, #42436, #27277, #150617, #8087, #135449, #58585, #120251, #181942, #124221, #138402, #59567, #182936, #121242, #75732, #153569, #93885, #32227, #152575, #183922, #44419, #29257, #109059, #186929, #123220, #125231, #31233, #61551, #90889, #30235, #169738, #108053, #77723, #155563, #62546, #63557, #136421, #200083, #106072, #92882, #48399, #13093, #16065, #184910, #167759, #33224, #151602, #185918, #15066, #137408, #107060, #45407, #47403, #74759, #14065, #91877, #139389, #168731, #154569, #78712, #76727, #46395, #871, #110056, #170736, #199088, #171736, #60556, #17057, #122231, #140388, #1876, #198101, #64554, #128194, #144361, #175709, #5848, #37187, #83681, #189892, #51367, #191871, #145359, #6841, #35204, #50387, #95877, #113028, #65535, #190879, #126218, #174720, #68520, #18063, #52355, #187914, #36183, #160540, #176725, #173735, #4845, #141387, #111046, #127195, #188907, #159525, #49383, #97837, #21022, #34214, #96857, #3856, #158541, #82677, #156565, #67524, #130174, #79718, #129181, #114011, #20031, #112047, #66531, #2875, #172733, #98845, #81673, #143356, #157560, #22029, #53354, #115032, #94884, #19053, #80700, #142377, #167290, #69528, #23031, #192883, #122746, #28787, #29763, #56359, #38198, #54361, #9868, #116033, #60088, #136933, #148373, #90426, #131193, #118041, #168266, #194885, #91397, #153086, #40183, #199608, #13595, #70531, #179732, #86689, #41202, #84676, #177722, #39190, #76246, #105603, #152112, #146355, #75262, #163546, #25046, #7842, #183449, #198622, #99854, #100848, #162530, #121756, #161538, #44933, #106590, #14590, #137924, #61074, #24034, #85688, #147375, #55356, #71527, #8864, #132200, #193891, #133194, #117026, #178721, #101862, #17568, #124743, #173241, #77241, #123727, #154089, #80215, #157072, #92403, #18568, #171251, #15583, #138909, #389, #108576, #186439, #126708, #65052, #185425, #16576, #62062, #46916, #141886, #19552, #156070, #158061, #64065, #94391, #170253, #63064, #2386, #140900, #110557, #188412, #95386, #96374, #169248, #32739, #31747, #125735, #81196, #45917, #48902, #79229, #93395, #66042, #184437, #3377, #47915, #155082, #139894, #78223, #49889, #4357, #187435, #109569, #172238, #30756, #33723, #1383, #111556, #34716, #142877, #107571, #101359, #67040, #129686, #36690, #37701, #6354, #189410, #21537, #146879, #24556, #20533, #7351, #193395, #38711, #115551, #68034, #177239, #160049, #145868, #54871, #144871, #52859, #99364, #163049, #191383, #35707, #147895, #97354, #114530, #159040, #8371, #82181, #143876, #5357, #161047, #100368, #70046, #162047, #131714, #116545, #22541, #84188, #86205, #178233, #39697, #176231, #83197, #128699 ),
 ( #69035, #130700, #174239, #9381, #85190, #50886, #190396, #51872, #192395, #127709, #23543, #53877, #112544, #113531, #175225, #98350, #75020, #12383, #88195, #42710, #136685, #90183, #121511, #166055, #119551, #91156, #41715, #104371, #11385, #59843, #164066, #10381, #40709, #167045, #43696, #179242, #105358, #57879, #102378, #25565, #87209, #195404, #73055, #13356, #151866, #72038, #103380, #148890, #133711, #28546, #106341, #27556, #44687, #150889, #181234, #56882, #149879, #89196, #74045, #197387, #198367, #182211, #183206, #55869, #135716, #118556, #58852, #120519, #168026, #29522, #134727, #152845, #71046, #165058, #132713, #194401, #117543, #180246, #26551, #196409, #49650, #32498, #63826, #122504, #78981, #139652, #1140, #60829, #156835, #172000, #76005, #15339, #30504, #94150, #14339, #2148, #140656, #171006, #95146, #79985, #125498, #18330, #155829, #31501, #186193, #141653, #33488, #64818, #109325, #62814, #34482, #185180, #47674, #154839, #3144, #107327, #153842, #184194, #110319, #187196, #45676, #48666, #124498, #169000, #92155, #76996, #138668, #16336, #126479, #188178, #148, #46670, #61817, #123487, #111314, #173003, #17326, #96140, #137679, #199365, #108330, #93153, #170010, #77985, #83952, #161808, #68794, #69799, #142643, #144633, #65801, #175992, #54626, #19320, #22301, #6116, #173999, #39457, #157829, #130452, #21299, #81938, #113295, #51631, #192150, #177990, #114290, #82956, #67799, #4121, #145632, #174986, #112309, #100126, #159803, #35470, #7112, #189175, #127469, #97119, #80967, #53631, #146629, #37461, #50648, #158802, #129454, #20291, #177000, #115307, #191153, #38469, #143630, #99123, #84947, #36450, #5114, #23303, #52627, #8121, #66796, #128459, #190155, #98107, #131467, #160813, #193153, #116301, #120286, #135484, #165817, #74792, #70805, #57644, #136454, #40465, #103138, #10140, #11142, #180007, #162804, #195160, #181978, #198135, #194164, #180995, #166815, #12149, #88961, #41474, #150651, #133469, #119310, #28316, #118314, #26315, #72816, #59604, #164820, #9139, #121278, #132475, #87956, #55628, #43461, #117301, #178997, #102137, #134485, #73814, #105129, #197154, #89955, #151635, #196172, #42472, #182971, #13130, #101118, #149644, #56641, #163822, #104134, #71800, #58619, #25323, #27314, #24313, #85962, #147651, #86965, #148651, #110092, #126252, #123254, #154604, #90923, #60591, #76763, #138436, #109094, #199124, #124258, #47437, #183955, #184945, #153606, #46430, #62580, #106108, #32263, #79752, #167793, #185953, #170773, #108089, #200117, #16099, #29293, #122266, #125267, #169773, #15102, #14099, #92918, #17093, #139423, #141422, #48435, #31267, #1913, #2909, #45442, #33259, #64587, #61586, #107095, #137444, #93920, #77757, #44455, #155598, #168765, #78746, #905, #152609, #75767, #30268, #91913, #140423, #186965, #171770, #63592, #94917, #156603, #18097, #145392, #23065, #159560, #161572, #67558, #97870, #65571, #66564, #5881, #144396, #114047, #191904, #98880, #99887, #172770, #174753, #95910, #129215, #84710, #49418, #52390, #36217, #3891, #69563, #187949, #160574, #51401, #112081, #143391, #81707, #22063, #7877, #190913, #113061, #21059, #34250, #175745, #4882, #142413, #130209, #189926, #127230, #37223, #19086, #157594, #188945, #111080, #83714, #176760, #6874, #80734, #50422, #82713, #173771, #68553, #53389, #115068, #38232, #35237, #146389, #96891, #158574, #20063, #128229, #133227, #89722, #103899, #163579, #10899, #179766, #87719, #116068, #85723, #24068, #166582, #149404, #180762, #39225, #195933, #56393, #118075, #177756, #73578, #88724, #192918, #132234, #147410, #72572, #131229, #119080, #57408, #134247, #11915, #196923, #42238, #135251, #165580, #148407, #102896, #58390, #150420, #181744, #26075, #41235, #151407, #101897, #164581, #71562, #120057, #8898, #70566, #100881, #27078, #43226, #162563, #25079, #104893, #28082, #12896, #193926, #55389 ),
 ( #117059, #54396, #178754, #40218, #86722, #9902, #194918, #140182, #139196, #78509, #15866, #91679, #46197, #1675, #93686, #125030, #169535, #123027, #94679, #45214, #107850, #14873, #63353, #167568, #13869, #44223, #170538, #47199, #182739, #108859, #61356, #105881, #29061, #90701, #198898, #76534, #16858, #155369, #75536, #106868, #152384, #137211, #32028, #109851, #31035, #48197, #154372, #184712, #60366, #153371, #92684, #77524, #671, #186726, #185709, #171536, #59371, #62341, #122038, #124011, #33024, #136227, #156358, #74560, #183728, #197902, #121043, #168542, #138210, #30040, #199892, #111841, #52156, #37997, #174519, #143159, #81472, #2675, #144159, #35000, #172530, #160338, #19831, #34016, #5644, #49188, #64352, #95673, #99652, #67321, #6640, #35986, #17860, #157360, #189694, #18854, #36982, #113813, #127991, #128982, #110846, #97633, #145157, #159322, #68318, #129969, #4639, #176521, #190680, #96655, #79516, #173530, #98644, #114827, #80500, #20818, #83479, #175508, #21827, #158342, #191669, #50184, #82474, #53148, #66330, #51166, #112827, #141186, #126021, #187717, #142173, #3657, #65335, #126995, #188702, #192681, #54164, #130989, #194688, #10670, #42007, #72334, #103672, #150180, #56158, #117839, #58166, #11681, #73346, #101655, #116827, #162332, #179532, #132001, #57172, #115837, #41002, #135019, #84474, #118850, #177526, #102669, #26844, #42997, #39984, #71335, #7639, #38995, #193689, #55157, #25850, #100651, #164354, #87493, #23833, #163347, #70334, #24843, #149182, #22828, #134009, #196695, #146152, #195700, #180533, #86492, #178518, #132997, #69323, #85483, #165350, #148177, #9670, #147172, #88485, #119833, #181518, #161336, #8661, #29804, #62106, #139938, #120804, #93438, #1428, #121798, #43984, #197671, #184479, #91440, #186484, #45958, #167334, #183491, #136000, #432, #153128, #108618, #182504, #59136, #166349, #105645, #138953, #75304, #106634, #104664, #123769, #185469, #169291, #78266, #74334, #61116, #63107, #28830, #168307, #13637, #14631, #46959, #90471, #199650, #155125, #27847, #170296, #152154, #137968, #31789, #89488, #44975, #76290, #151178, #136975, #198664, #60130, #30797, #122790, #107613, #92446, #154134, #15626, #77283, #16618, #124785, #12666, #38511, #86004, #171296, #68837, #130496, #188455, #141928, #158103, #32782, #125777, #131507, #49936, #157114, #17613, #96417, #23343, #145672, #147693, #54667, #173285, #8164, #9180, #64111, #39498, #70846, #65095, #187479, #140943, #192192, #34759, #132515, #53673, #110599, #126753, #79272, #146669, #22342, #116341, #48946, #2431, #109612, #172281, #84988, #18611, #111601, #47960, #69840, #193194, #115351, #24353, #33770, #7154, #94434, #95430, #83993, #80258, #177041, #100167, #156115, #3419, #178030, #161849, #101158, #162846, #59643, #105167, #182018, #72858, #43501, #26357, #12188, #121317, #11183, #119353, #104175, #167831, #196215, #102178, #14137, #163866, #57685, #25365, #13168, #87006, #148693, #10181, #27353, #166853, #74831, #28355, #136493, #183009, #88999, #150690, #90960, #44493, #106149, #134528, #149685, #195202, #73853, #164861, #87997, #181037, #58657, #71841, #135523, #197194, #133510, #42511, #103181, #165857, #120323, #55669, #89993, #29332, #117343, #151675, #198173, #152647, #75804, #194204, #179039, #56682, #40507, #118356, #180049, #41518, #77790, #78781, #124292, #156636, #48469, #154640, #63627, #18132, #30307, #171804, #79786, #169809, #153643, #107133, #47472, #16135, #2943, #109129, #76800, #31301, #168803, #140458, #139459, #110126, #91950, #15138, #199162, #138471, #1948, #123290, #92954, #137482, #186999, #125303, #155633, #141458, #200152, #170807, #60629, #61622, #939, #46466, #185989, #62614, #183993, #32300, #33292, #122303, #184982, #17129, #45477, #108126, #93955, #94952, #105805, #150342, #136153, #45137, #135175, #43148, #28004, #91604, #119983, #26004, #138131, #87646 ),
 ( #197828, #106794, #74487, #168468, #29966, #181669, #76454, #90628, #11838, #59294, #166506, #120963, #102825, #72496, #10826, #153293, #182662, #167492, #149332, #44146, #104817, #89644, #164511, #151332, #121960, #134170, #195858, #179690, #57330, #152310, #88646, #12821, #199812, #137135, #13796, #28988, #14794, #119006, #75461, #118001, #180689, #198822, #27001, #60287, #196849, #41162, #73503, #183653, #42165, #103825, #165505, #58315, #172447, #49108, #140103, #110766, #93604, #79435, #188622, #78428, #186646, #171457, #34920, #63269, #169458, #81395, #30959, #124950, #92606, #80420, #154296, #15786, #77446, #94600, #33935, #142093, #95593, #3578, #50103, #156279, #17780, #158265, #111763, #173452, #1594, #16779, #62264, #141106, #31949, #157277, #139117, #2594, #96576, #184638, #18773, #593, #64273, #126916, #143081, #48117, #32945, #107772, #123932, #155289, #109774, #125940, #185630, #187638, #65256, #47122, #19754, #170458, #61280, #122950, #46119, #108780, #173039, #49684, #93188, #111349, #126514, #157865, #2181, #155862, #127506, #78018, #140690, #47708, #96175, #184, #46705, #77031, #3179, #80019, #15375, #141688, #94183, #138703, #61852, #123521, #31535, #109358, #34517, #188212, #108368, #139687, #185214, #170045, #64852, #142678, #79015, #1173, #171040, #189210, #19355, #81004, #172034, #4157, #154873, #63861, #65836, #16370, #32531, #62848, #17360, #186228, #169035, #124532, #107362, #30541, #125532, #187229, #92193, #18366, #95184, #48700, #156870, #110352, #33522, #153877, #67834, #176029, #160849, #24349, #52664, #158839, #70843, #20327, #114326, #81976, #69836, #143670, #5151, #66833, #83989, #100163, #131503, #161845, #193190, #39494, #145668, #7149, #147689, #101154, #162841, #191188, #6154, #51667, #68833, #21335, #146665, #128497, #130492, #86000, #174035, #8160, #190192, #192188, #116337, #132511, #129490, #22338, #97156, #113331, #82993, #144669, #115347, #175024, #53669, #177037, #36487, #37497, #159842, #99159, #38507, #112345, #23339, #84983, #54663, #178026, #9176, #50688, #35506, #98143, #117339, #71836, #74828, #196209, #103176, #163861, #42507, #166849, #88995, #29327, #198169, #119349, #151670, #90956, #10176, #183005, #152643, #11178, #133505, #87001, #73848, #181033, #75800, #135519, #56677, #72853, #25360, #89989, #104171, #59639, #195197, #148688, #55665, #118350, #28351, #180044, #197190, #121313, #105163, #182014, #134523, #43497, #26352, #12184, #44489, #57681, #165853, #27349, #167827, #150686, #102173, #14133, #41513, #58654, #164856, #13164, #87992, #149680, #120320, #136489, #106145, #194200, #179035, #40501, #126282, #32296, #93952, #34281, #187979, #49448, #77786, #92950, #138467, #170804, #108122, #33289, #168799, #155630, #111111, #60625, #94949, #30303, #17126, #2940, #19116, #16131, #47469, #183989, #153639, #169805, #31298, #1944, #91946, #78778, #140454, #76796, #139455, #46462, #936, #63624, #199158, #154636, #125300, #156633, #171801, #186996, #62610, #124289, #109126, #122299, #15134, #18128, #185986, #48466, #107128, #110123, #79783, #141455, #172800, #64620, #95940, #157626, #137478, #200148, #45474, #61618, #123286, #184977, #173801, #160603, #5912, #162594, #22093, #143424, #97901, #112110, #176788, #67589, #84739, #96922, #35267, #142444, #158604, #115096, #51430, #82746, #80766, #99915, #38261, #145422, #54426, #50451, #37253, #116096, #20094, #144426, #189956, #190943, #159592, #3922, #174782, #161600, #177784, #98910, #65602, #68583, #6904, #83743, #23094, #146417, #130239, #127262, #7908, #69592, #66594, #131259, #192947, #39254, #175779, #129247, #100910, #113090, #114078, #21089, #188975, #81738, #4911, #128258, #36248, #53419, #52420, #191935, #10927, #132264, #55418, #193955, #148436, #26103, #166605, #104918, #25109, #56423, #117089, #101926, #181769, #59393, #195961, #197925, #103925, #134274, #163608, #102924, #42265 ),
 ( #40252, #105902, #24099, #135274, #87746, #9931, #179793, #118103, #58414, #44245, #180788, #149431, #72600, #8928, #150443, #41262, #178784, #28105, #57434, #86753, #11939, #71590, #70596, #133256, #85753, #73602, #12917, #165605, #147440, #194947, #119107, #164609, #43250, #120081, #27104, #196946, #88750, #89744, #151430, #74581, #136249, #121067, #182761, #126045, #140207, #199916, #47225, #15891, #124037, #152405, #122060, #60388, #2700, #185736, #16882, #75559, #32053, #92708, #154396, #13892, #109875, #125054, #29083, #168565, #183752, #31060, #91704, #123051, #61380, #1701, #187741, #108884, #77549, #139221, #137235, #93710, #184737, #45238, #171559, #169563, #106892, #155392, #198919, #30063, #153398, #49212, #78533, #156381, #170563, #167588, #14896, #696, #76557, #186751, #63377, #62368, #48221, #138233, #33049, #94704, #17886, #79540, #141210, #64377, #90722, #46222, #107875, #190708, #159350, #67348, #95698, #65360, #3682, #146180, #129008, #160364, #18879, #175535, #36012, #97661, #157386, #53178, #68344, #172555, #111867, #127021, #52181, #110870, #98670, #37009, #113839, #191695, #176548, #21854, #34041, #38024, #114854, #96681, #99680, #129995, #161364, #5672, #20846, #131017, #81498, #144186, #51193, #22855, #188728, #50213, #80525, #6666, #83505, #142199, #145182, #82504, #173557, #35026, #158369, #19858, #112854, #84502, #7665, #143185, #4665, #66357, #128018, #69349, #192707, #189720, #174545, #136751, #167109, #134793, #135782, #75084, #13420, #183271, #60895, #168089, #169068, #41779, #43762, #165124, #198435, #153911, #115863, #121576, #105426, #73124, #138735, #54190, #29586, #180311, #76069, #91217, #44751, #30574, #26616, #59908, #92225, #196474, #58919, #166123, #28610, #197453, #103445, #150956, #137745, #15406, #149946, #106407, #122571, #152908, #14405, #120587, #199429, #89264, #184261, #45743, #74112, #182281, #90248, #77063, #151931, #88259, #11452, #57945, #107395, #119616, #181299, #42777, #104439, #27625, #12450, #49718, #81034, #111383, #142710, #189242, #95217, #156903, #97186, #50720, #112378, #140724, #155896, #1207, #33555, #171073, #96207, #31569, #18399, #174070, #123554, #157896, #93220, #80050, #65868, #82009, #79050, #110386, #46740, #16404, #32563, #94217, #64883, #154905, #141719, #3209, #139719, #2214, #109393, #63895, #126544, #61884, #17394, #188243, #19385, #34548, #173071, #125566, #187263, #172068, #185249, #78050, #4189, #48732, #127540, #170078, #35539, #158872, #20361, #215, #108401, #62884, #124565, #186262, #47740, #132545, #40539, #160883, #83027, #36521, #23375, #68869, #25395, #85020, #6187, #22374, #175057, #39529, #130528, #147724, #159878, #98176, #5185, #21369, #178061, #114360, #145703, #161881, #143703, #131542, #69873, #100199, #24386, #9211, #8198, #66866, #70878, #86037, #129522, #194234, #162878, #55700, #38543, #192225, #163899, #176065, #177072, #84025, #117373, #144701, #67867, #113365, #101189, #116373, #51702, #179070, #53707, #191222, #52696, #37532, #99195, #7185, #102210, #128529, #115384, #146701, #193226, #54700, #190223, #122333, #58685, #60660, #166882, #197223, #164892, #165885, #105195, #43530, #13197, #90990, #198203, #199193, #71870, #73881, #195230, #28383, #184025, #148722, #151704, #135551, #103210, #168833, #87037, #59673, #150719, #11212, #42541, #181066, #121345, #107162, #90021, #12218, #120352, #133538, #74860, #104204, #41547, #29360, #89028, #26386, #136522, #118384, #56711, #88025, #10210, #183038, #75834, #44521, #180078, #149713, #182047, #72887, #106177, #167860, #152677, #14166, #134556, #137512, #45507, #196244, #57713, #119383, #27382, #189007, #2972, #62647, #110155, #78813, #187030, #15170, #185012, #123319, #65634, #48501, #79818, #138500, #94982, #155664, #17160, #76829, #172834, #188011, #91979, #31334, #46497, #34313, #111144, #92985, #124324, #200182, #108158, #49481, #127294 ),
 ( #140492, #61651, #171833, #50482, #153673, #156667, #1980, #169840, #112142, #30338, #141489, #93984, #154670, #186022, #47504, #64652, #16166, #33321, #63660, #125333, #77820, #18162, #109160, #139489, #95976, #32331, #971, #126314, #170839, #157660, #19149, #80799, #142477, #3955, #191967, #55453, #189988, #145455, #128290, #192981, #69626, #83775, #23127, #66626, #53453, #100945, #130272, #162629, #24136, #175813, #132299, #146450, #5944, #115129, #22125, #176821, #158635, #51462, #113124, #8964, #38293, #84772, #81770, #99947, #98943, #160634, #20126, #116129, #131292, #35299, #174814, #36279, #161633, #173834, #7943, #54459, #177818, #39288, #4942, #144459, #85788, #147474, #70633, #193991, #114110, #67620, #6937, #96955, #97934, #143457, #37286, #82778, #159627, #68616, #21122, #129281, #190976, #52453, #42299, #74618, #152441, #133291, #105938, #13927, #134309, #56459, #151465, #137273, #73636, #103960, #180820, #101962, #43283, #195995, #71625, #59430, #119140, #194981, #104952, #148473, #163643, #118138, #198955, #166638, #167623, #135307, #117124, #179827, #88783, #41297, #136284, #12953, #27136, #28140, #9965, #196979, #44280, #58446, #29119, #90758, #165638, #75594, #89780, #149465, #120114, #150476, #181805, #25145, #102958, #164642, #178818, #197960, #121103, #86787, #182797, #11971, #40288, #26138, #87780, #10960, #72634, #57468, #76592, #78570, #60422, #48257, #186787, #154432, #109911, #63414, #126079, #122095, #187775, #2733, #46258, #64410, #79575, #110903, #155427, #108919, #80558, #31096, #93746, #732, #49245, #153434, #199951, #30099, #156419, #33083, #168599, #94739, #47262, #91739, #14932, #138268, #184772, #62404, #172589, #141244, #61415, #92744, #123086, #107913, #17920, #95733, #32089, #34075, #140244, #170599, #169598, #139256, #1736, #16917, #171595, #157419, #18913, #142233, #45272, #125089, #15926, #183786, #106926, #77584, #124074, #185775, #19892, #85546, #3718, #114889, #67384, #128054, #159388, #97697, #7700, #22889, #54224, #98706, #52216, #23893, #174583, #37047, #144223, #192742, #96715, #143220, #173591, #99713, #176583, #111903, #38057, #190742, #35060, #158403, #81533, #189756, #5707, #146212, #84535, #4702, #36048, #66392, #51228, #161397, #39052, #175570, #177585, #83539, #113873, #112889, #82541, #21889, #160400, #130030, #69383, #131052, #115895, #188763, #145218, #20883, #6700, #100710, #65395, #68378, #191729, #129041, #127056, #50247, #162390, #53211, #71393, #102725, #41062, #181573, #167392, #103729, #72393, #10729, #132061, #73405, #164414, #101718, #89546, #149238, #163408, #135076, #178579, #193750, #24904, #28888, #196752, #136052, #165409, #147232, #86551, #118907, #148235, #166408, #43051, #57233, #58219, #40044, #26902, #74387, #88545, #197727, #59193, #134069, #105705, #119888, #179590, #150243, #195759, #11738, #55218, #9729, #133057, #182562, #104717, #27903, #116887, #151232, #180591, #42065, #194747, #12721, #120862, #8724, #56219, #117901, #44045, #70393, #25906, #87551, #184537, #78325, #93500, #156174, #90528, #17673, #32842, #76352, #171354, #91500, #122849, #198721, #168367, #48017, #125835, #62165, #64170, #170356, #492, #29863, #169350, #108678, #47019, #16676, #94492, #1487, #2489, #75361, #77346, #60188, #31848, #187538, #152210, #155186, #139012, #106694, #172339, #13694, #63165, #154195, #14690, #46017, #107673, #124844, #110659, #139998, #15685, #123829, #137031, #186544, #30859, #45036, #79331, #92506, #153187, #109673, #121858, #183550, #138029, #199712, #141001, #49004, #61177, #185527, #49994, #5461, #188517, #52961, #129786, #143980, #83297, #126810, #51973, #161149, #190500, #22646, #84293, #35807, #192496, #6454, #66144, #113632, #82289, #175327, #18668, #111659, #173346, #69138, #36794, #144973, #141987, #98459, #159139, #20636, #80314, #176336, #191483, #95488, #34817, #96472, #160153, #33828, #21644 ) ),
 .UNSPECIFIED., .T., .F., .F. ) 
 B_SPLINE_SURFACE_WITH_KNOTS ( ( 4, 3, 4 ),
 ( 3, 2, 2, 2, 2, 2, 2, 2, 2, 2, 2, 2, 2, 2, 2, 2, 2, 2, 2, 2, 2, 2, 2, 2, 2, 2, 2, 2, 2, 2, 2, 2, 2, 2, 2, 2, 2, 2, 2, 2, 2, 2, 2, 2, 2, 2, 2, 2, 2, 2, 2, 2, 2, 2, 2, 2, 2, 2, 2, 2, 2, 2, 2, 2, 2, 2, 2, 2, 2, 2, 2, 2, 2, 2, 2, 2, 2, 2, 2, 2, 2, 2, 2, 2, 2, 2, 2, 2, 2, 2, 2, 2, 2, 2, 2, 2, 2, 2, 2, 2, 2, 2, 2, 2, 2, 2, 2, 2, 2, 2, 2, 2, 2, 2, 2, 2, 2, 2, 2, 2, 2, 2, 2, 2, 2, 2, 2, 2, 2, 2, 2, 2, 2, 2, 2, 2, 2, 2, 2, 2, 2, 2, 2, 2, 2, 2, 2, 2, 2, 2, 2, 2, 2, 2, 2, 2, 2, 2, 2, 2, 2, 2, 2, 2, 2, 2, 2, 2, 2, 2, 2, 2, 2, 2, 2, 2, 2, 2, 2, 2, 2, 2, 2, 2, 2, 2, 2, 2, 2, 2, 2, 2, 2, 2, 2, 2, 2, 2, 2, 2, 2, 2, 2, 2, 2, 2, 2, 2, 2, 2, 2, 2, 2, 2, 2, 2, 2, 2, 2, 2, 2, 2, 2, 2, 2, 2, 2, 2, 3 ),
 ( 0.000000000000000000, 0.5000000000000000000, 1.000000000000000000 ),
 ( 0.000000000000000000, 0.004385964912280701511, 0.008771929824561403022, 0.01315789473684210453, 0.01754385964912280604, 0.02192982456140350755, 0.02631578947368420907, 0.03070175438596491058, 0.03508771929824561209, 0.03947368421052631360, 0.04385964912280701511, 0.04824561403508771662, 0.05263157894736841813, 0.05701754385964911964, 0.06140350877192982115, 0.06578947368421052266, 0.07017543859649122417, 0.07456140350877192569, 0.07894736842105262720, 0.08333333333333332871, 0.08771929824561403022, 0.09210526315789473173, 0.09649122807017543324, 0.1008771929824561348, 0.1052631578947368363, 0.1096491228070175378, 0.1140350877192982393, 0.1184210526315789408, 0.1228070175438596423, 0.1271929824561403577, 0.1315789473684210453, 0.1359649122807017607, 0.1403508771929824483, 0.1447368421052631637, 0.1491228070175438514, 0.1535087719298245668, 0.1578947368421052544, 0.1622807017543859698, 0.1666666666666666574, 0.1710526315789473728, 0.1754385964912280604, 0.1798245614035087758, 0.1842105263157894635, 0.1885964912280701788, 0.1929824561403508665, 0.1973684210526315819, 0.2017543859649122695, 0.2061403508771929849, 0.2105263157894736725, 0.2149122807017543879, 0.2192982456140350755, 0.2236842105263157909, 0.2280701754385964786, 0.2324561403508771940, 0.2368421052631578816, 0.2412280701754385970, 0.2456140350877192846, 0.2500000000000000000, 0.2543859649122807154, 0.2587719298245614308, 0.2631578947368420907, 0.2675438596491228060, 0.2719298245614035214, 0.2763157894736842368, 0.2807017543859648967, 0.2850877192982456121, 0.2894736842105263275, 0.2938596491228070429, 0.2982456140350877027, 0.3026315789473684181, 0.3070175438596491335, 0.3114035087719298489, 0.3157894736842105088, 0.3201754385964912242, 0.3245614035087719396, 0.3289473684210526550, 0.3333333333333333148, 0.3377192982456140302, 0.3421052631578947456, 0.3464912280701754610, 0.3508771929824561209, 0.3552631578947368363, 0.3596491228070175517, 0.3640350877192982670, 0.3684210526315789269, 0.3728070175438596423, 0.3771929824561403577, 0.3815789473684210731, 0.3859649122807017330, 0.3903508771929824483, 0.3947368421052631637, 0.3991228070175438791, 0.4035087719298245390, 0.4078947368421052544, 0.4122807017543859698, 0.4166666666666666852, 0.4210526315789473450, 0.4254385964912280604, 0.4298245614035087758, 0.4342105263157894912, 0.4385964912280701511, 0.4429824561403508665, 0.4473684210526315819, 0.4517543859649122973, 0.4561403508771929571, 0.4605263157894736725, 0.4649122807017543879, 0.4692982456140351033, 0.4736842105263157632, 0.4780701754385964786, 0.4824561403508771940, 0.4868421052631579093, 0.4912280701754385692, 0.4956140350877192846, 0.5000000000000000000, 0.5043859649122807154, 0.5087719298245614308, 0.5131578947368421462, 0.5175438596491228616, 0.5219298245614034659, 0.5263157894736841813, 0.5307017543859648967, 0.5350877192982456121, 0.5394736842105263275, 0.5438596491228070429, 0.5482456140350877583, 0.5526315789473684736, 0.5570175438596490780, 0.5614035087719297934, 0.5657894736842105088, 0.5701754385964912242, 0.5745614035087719396, 0.5789473684210526550, 0.5833333333333333703, 0.5877192982456140857, 0.5921052631578946901, 0.5964912280701754055, 0.6008771929824561209, 0.6052631578947368363, 0.6096491228070175517, 0.6140350877192982670, 0.6184210526315789824, 0.6228070175438596978, 0.6271929824561403022, 0.6315789473684210176, 0.6359649122807017330, 0.6403508771929824483, 0.6447368421052631637, 0.6491228070175438791, 0.6535087719298245945, 0.6578947368421053099, 0.6622807017543859143, 0.6666666666666666297, 0.6710526315789473450, 0.6754385964912280604, 0.6798245614035087758, 0.6842105263157894912, 0.6885964912280702066, 0.6929824561403509220, 0.6973684210526315264, 0.7017543859649122417, 0.7061403508771929571, 0.7105263157894736725, 0.7149122807017543879, 0.7192982456140351033, 0.7236842105263158187, 0.7280701754385965341, 0.7324561403508771384, 0.7368421052631578538, 0.7412280701754385692, 0.7456140350877192846, 0.7500000000000000000, 0.7543859649122807154, 0.7587719298245614308, 0.7631578947368421462, 0.7675438596491228616, 0.7719298245614034659, 0.7763157894736841813, 0.7807017543859648967, 0.7850877192982456121, 0.7894736842105263275, 0.7938596491228070429, 0.7982456140350877583, 0.8026315789473684736, 0.8070175438596490780, 0.8114035087719297934, 0.8157894736842105088, 0.8201754385964912242, 0.8245614035087719396, 0.8289473684210526550, 0.8333333333333333703, 0.8377192982456140857, 0.8421052631578946901, 0.8464912280701754055, 0.8508771929824561209, 0.8552631578947368363, 0.8596491228070175517, 0.8640350877192982670, 0.8684210526315789824, 0.8728070175438596978, 0.8771929824561403022, 0.8815789473684210176, 0.8859649122807017330, 0.8903508771929824483, 0.8947368421052631637, 0.8991228070175438791, 0.9035087719298245945, 0.9078947368421053099, 0.9122807017543859143, 0.9166666666666666297, 0.9210526315789473450, 0.9254385964912280604, 0.9298245614035087758, 0.9342105263157894912, 0.9385964912280702066, 0.9429824561403509220, 0.9473684210526315264, 0.9517543859649122417, 0.9561403508771929571, 0.9605263157894736725, 0.9649122807017543879, 0.9692982456140351033, 0.9736842105263158187, 0.9780701754385965341, 0.9824561403508771384, 0.9868421052631578538, 0.9912280701754385692, 0.9956140350877192846, 1.000000000000000000 ),
 .UNSPECIFIED. ) 
 GEOMETRIC_REPRESENTATION_ITEM ( )  RATIONAL_B_SPLINE_SURFACE ( (
 ( 1.000000000000000000, 0.9659258262890683122, 1.000000000000000000, 0.9659258262890683122, 1.000000000000000000, 0.9659258262890683122, 1.000000000000000000, 0.9659258262890683122, 1.000000000000000000, 0.9659258262890683122, 1.000000000000000000, 0.9659258262890683122, 1.000000000000000000, 0.9659258262890683122, 1.000000000000000000, 0.9659258262890683122, 1.000000000000000000, 0.9659258262890683122, 1.000000000000000000, 0.9659258262890683122, 1.000000000000000000, 0.9659258262890683122, 1.000000000000000000, 0.9659258262890683122, 1.000000000000000000, 0.9659258262890683122, 1.000000000000000000, 0.9659258262890683122, 1.000000000000000000, 0.9659258262890683122, 1.000000000000000000, 0.9659258262890683122, 1.000000000000000000, 0.9659258262890683122, 1.000000000000000000, 0.9659258262890683122, 1.000000000000000000, 0.9659258262890683122, 1.000000000000000000, 0.9659258262890683122, 1.000000000000000000, 0.9659258262890683122, 1.000000000000000000, 0.9659258262890683122, 1.000000000000000000, 0.9659258262890683122, 1.000000000000000000, 0.9659258262890683122, 1.000000000000000000, 0.9659258262890683122, 1.000000000000000000, 0.9659258262890683122, 1.000000000000000000, 0.9659258262890683122, 1.000000000000000000, 0.9659258262890683122, 1.000000000000000000, 0.9659258262890683122, 1.000000000000000000, 0.9659258262890683122, 1.000000000000000000, 0.9659258262890683122, 1.000000000000000000, 0.9659258262890683122, 1.000000000000000000, 0.9659258262890683122, 1.000000000000000000, 0.9659258262890683122, 1.000000000000000000, 0.9659258262890683122, 1.000000000000000000, 0.9659258262890683122, 1.000000000000000000, 0.9659258262890683122, 1.000000000000000000, 0.9659258262890683122, 1.000000000000000000, 0.9659258262890683122, 1.000000000000000000, 0.9659258262890683122, 1.000000000000000000, 0.9659258262890683122, 1.000000000000000000, 0.9659258262890683122, 1.000000000000000000, 0.9659258262890683122, 1.000000000000000000, 0.9659258262890683122, 1.000000000000000000, 0.9659258262890683122, 1.000000000000000000, 0.9659258262890683122, 1.000000000000000000, 0.9659258262890683122, 1.000000000000000000, 0.9659258262890683122, 1.000000000000000000, 0.9659258262890683122, 1.000000000000000000, 0.9659258262890683122, 1.000000000000000000, 0.9659258262890683122, 1.000000000000000000, 0.9659258262890683122, 1.000000000000000000, 0.9659258262890683122, 1.000000000000000000, 0.9659258262890683122, 1.000000000000000000, 0.9659258262890683122, 1.000000000000000000, 0.9659258262890683122, 1.000000000000000000, 0.9659258262890683122, 1.000000000000000000, 0.9659258262890683122, 1.000000000000000000, 0.9659258262890683122, 1.000000000000000000, 0.9659258262890683122, 1.000000000000000000, 0.9659258262890683122, 1.000000000000000000, 0.9659258262890683122, 1.000000000000000000, 0.9659258262890683122, 1.000000000000000000, 0.9659258262890683122, 1.000000000000000000, 0.9659258262890683122, 1.000000000000000000, 0.9659258262890683122, 1.000000000000000000, 0.9659258262890683122, 1.000000000000000000, 0.9659258262890683122, 1.000000000000000000, 0.9659258262890683122, 1.000000000000000000, 0.9659258262890683122, 1.000000000000000000, 0.9659258262890683122, 1.000000000000000000, 0.9659258262890683122, 1.000000000000000000, 0.9659258262890683122, 1.000000000000000000, 0.9659258262890683122, 1.000000000000000000, 0.9659258262890683122, 1.000000000000000000, 0.9659258262890683122, 1.000000000000000000, 0.9659258262890683122, 1.000000000000000000, 0.9659258262890683122, 1.000000000000000000, 0.9659258262890683122, 1.000000000000000000, 0.9659258262890683122, 1.000000000000000000, 0.9659258262890683122, 1.000000000000000000, 0.9659258262890683122, 1.000000000000000000, 0.9659258262890683122, 1.000000000000000000, 0.9659258262890683122, 1.000000000000000000, 0.9659258262890683122, 1.000000000000000000, 0.9659258262890683122, 1.000000000000000000, 0.9659258262890683122, 1.000000000000000000, 0.9659258262890683122, 1.000000000000000000, 0.9659258262890683122, 1.000000000000000000, 0.9659258262890683122, 1.000000000000000000, 0.9659258262890683122, 1.000000000000000000, 0.9659258262890683122, 1.000000000000000000, 0.9659258262890683122, 1.000000000000000000, 0.9659258262890683122, 1.000000000000000000, 0.9659258262890683122, 1.000000000000000000, 0.9659258262890683122, 1.000000000000000000, 0.9659258262890683122, 1.000000000000000000, 0.9659258262890683122, 1.000000000000000000, 0.9659258262890683122, 1.000000000000000000, 0.9659258262890683122, 1.000000000000000000, 0.9659258262890683122, 1.000000000000000000, 0.9659258262890683122, 1.000000000000000000, 0.9659258262890683122, 1.000000000000000000, 0.9659258262890683122, 1.000000000000000000, 0.9659258262890683122, 1.000000000000000000, 0.9659258262890683122, 1.000000000000000000, 0.9659258262890683122, 1.000000000000000000, 0.9659258262890683122, 1.000000000000000000, 0.9659258262890683122, 1.000000000000000000, 0.9659258262890683122, 1.000000000000000000, 0.9659258262890683122, 1.000000000000000000, 0.9659258262890683122, 1.000000000000000000, 0.9659258262890683122, 1.000000000000000000, 0.9659258262890683122, 1.000000000000000000, 0.9659258262890683122, 1.000000000000000000, 0.9659258262890683122, 1.000000000000000000, 0.9659258262890683122, 1.000000000000000000, 0.9659258262890683122, 1.000000000000000000, 0.9659258262890683122, 1.000000000000000000, 0.9659258262890683122, 1.000000000000000000, 0.9659258262890683122, 1.000000000000000000, 0.9659258262890683122, 1.000000000000000000, 0.9659258262890683122, 1.000000000000000000, 0.9659258262890683122, 1.000000000000000000, 0.9659258262890683122, 1.000000000000000000, 0.9659258262890683122, 1.000000000000000000, 0.9659258262890683122, 1.000000000000000000, 0.9659258262890683122, 1.000000000000000000, 0.9659258262890683122, 1.000000000000000000, 0.9659258262890683122, 1.000000000000000000, 0.9659258262890683122, 1.000000000000000000, 0.9659258262890683122, 1.000000000000000000, 0.9659258262890683122, 1.000000000000000000, 0.9659258262890683122, 1.000000000000000000, 0.9659258262890683122, 1.000000000000000000, 0.9659258262890683122, 1.000000000000000000, 0.9659258262890683122, 1.000000000000000000, 0.9659258262890683122, 1.000000000000000000, 0.9659258262890683122, 1.000000000000000000, 0.9659258262890683122, 1.000000000000000000, 0.9659258262890683122, 1.000000000000000000, 0.9659258262890683122, 1.000000000000000000, 0.9659258262890683122, 1.000000000000000000, 0.9659258262890683122, 1.000000000000000000, 0.9659258262890683122, 1.000000000000000000, 0.9659258262890683122, 1.000000000000000000, 0.9659258262890683122, 1.000000000000000000, 0.9659258262890683122, 1.000000000000000000, 0.9659258262890683122, 1.000000000000000000, 0.9659258262890683122, 1.000000000000000000, 0.9659258262890683122, 1.000000000000000000, 0.9659258262890683122, 1.000000000000000000, 0.9659258262890683122, 1.000000000000000000, 0.9659258262890683122, 1.000000000000000000, 0.9659258262890683122, 1.000000000000000000, 0.9659258262890683122, 1.000000000000000000, 0.9659258262890683122, 1.000000000000000000, 0.9659258262890683122, 1.000000000000000000, 0.9659258262890683122, 1.000000000000000000, 0.9659258262890683122, 1.000000000000000000, 0.9659258262890683122, 1.000000000000000000, 0.9659258262890683122, 1.000000000000000000, 0.9659258262890683122, 1.000000000000000000, 0.9659258262890683122, 1.000000000000000000, 0.9659258262890683122, 1.000000000000000000, 0.9659258262890683122, 1.000000000000000000, 0.9659258262890683122, 1.000000000000000000, 0.9659258262890683122, 1.000000000000000000, 0.9659258262890683122, 1.000000000000000000, 0.9659258262890683122, 1.000000000000000000, 0.9659258262890683122, 1.000000000000000000, 0.9659258262890683122, 1.000000000000000000, 0.9659258262890683122, 1.000000000000000000, 0.9659258262890683122, 1.000000000000000000, 0.9659258262890683122, 1.000000000000000000, 0.9659258262890683122, 1.000000000000000000, 0.9659258262890683122, 1.000000000000000000, 0.9659258262890683122, 1.000000000000000000, 0.9659258262890683122, 1.000000000000000000, 0.9659258262890683122, 1.000000000000000000, 0.9659258262890683122, 1.000000000000000000, 0.9659258262890683122, 1.000000000000000000, 0.9659258262890683122, 1.000000000000000000, 0.9659258262890683122, 1.000000000000000000, 0.9659258262890683122, 1.000000000000000000, 0.9659258262890683122, 1.000000000000000000, 0.9659258262890683122, 1.000000000000000000, 0.9659258262890683122, 1.000000000000000000, 0.9659258262890683122, 1.000000000000000000, 0.9659258262890683122, 1.000000000000000000, 0.9659258262890683122, 1.000000000000000000, 0.9659258262890683122, 1.000000000000000000, 0.9659258262890683122, 1.000000000000000000, 0.9659258262890683122, 1.000000000000000000, 0.9659258262890683122, 1.000000000000000000, 0.9659258262890683122, 1.000000000000000000, 0.9659258262890683122, 1.000000000000000000, 0.9659258262890683122, 1.000000000000000000, 0.9659258262890683122, 1.000000000000000000, 0.9659258262890683122, 1.000000000000000000, 0.9659258262890683122, 1.000000000000000000, 0.9659258262890683122, 1.000000000000000000, 0.9659258262890683122, 1.000000000000000000, 0.9659258262890683122, 1.000000000000000000, 0.9659258262890683122, 1.000000000000000000, 0.9659258262890683122, 1.000000000000000000, 0.9659258262890683122, 1.000000000000000000, 0.9659258262890683122, 1.000000000000000000, 0.9659258262890683122, 1.000000000000000000, 0.9659258262890683122, 1.000000000000000000, 0.9659258262890683122, 1.000000000000000000, 0.9659258262890683122, 1.000000000000000000, 0.9659258262890683122, 1.000000000000000000, 0.9659258262890683122, 1.000000000000000000, 0.9659258262890683122, 1.000000000000000000, 0.9659258262890683122, 1.000000000000000000, 0.9659258262890683122, 1.000000000000000000, 0.9659258262890683122, 1.000000000000000000, 0.9659258262890683122, 1.000000000000000000, 0.9659258262890683122, 1.000000000000000000, 0.9659258262890683122, 1.000000000000000000, 0.9659258262890683122, 1.000000000000000000, 0.9659258262890683122, 1.000000000000000000, 0.9659258262890683122, 1.000000000000000000, 0.9659258262890683122, 1.000000000000000000, 0.9659258262890683122, 1.000000000000000000, 0.9659258262890683122, 1.000000000000000000, 0.9659258262890683122, 1.000000000000000000),
 ( 0.3333333333333333703, 0.3219752754296894559, 0.3333333333333333703, 0.3219752754296894559, 0.3333333333333333703, 0.3219752754296894559, 0.3333333333333333703, 0.3219752754296894559, 0.3333333333333333703, 0.3219752754296894559, 0.3333333333333333703, 0.3219752754296894559, 0.3333333333333333703, 0.3219752754296894559, 0.3333333333333333703, 0.3219752754296894559, 0.3333333333333333703, 0.3219752754296894559, 0.3333333333333333703, 0.3219752754296894559, 0.3333333333333333703, 0.3219752754296894559, 0.3333333333333333703, 0.3219752754296894559, 0.3333333333333333703, 0.3219752754296894559, 0.3333333333333333703, 0.3219752754296894559, 0.3333333333333333703, 0.3219752754296894559, 0.3333333333333333703, 0.3219752754296894559, 0.3333333333333333703, 0.3219752754296894559, 0.3333333333333333703, 0.3219752754296894559, 0.3333333333333333703, 0.3219752754296894559, 0.3333333333333333703, 0.3219752754296894559, 0.3333333333333333703, 0.3219752754296894559, 0.3333333333333333703, 0.3219752754296894559, 0.3333333333333333703, 0.3219752754296894559, 0.3333333333333333703, 0.3219752754296894559, 0.3333333333333333703, 0.3219752754296894559, 0.3333333333333333703, 0.3219752754296894559, 0.3333333333333333703, 0.3219752754296894559, 0.3333333333333333703, 0.3219752754296894559, 0.3333333333333333703, 0.3219752754296894559, 0.3333333333333333703, 0.3219752754296894559, 0.3333333333333333703, 0.3219752754296894559, 0.3333333333333333703, 0.3219752754296894559, 0.3333333333333333703, 0.3219752754296894559, 0.3333333333333333703, 0.3219752754296894559, 0.3333333333333333703, 0.3219752754296894559, 0.3333333333333333703, 0.3219752754296894559, 0.3333333333333333703, 0.3219752754296894559, 0.3333333333333333703, 0.3219752754296894559, 0.3333333333333333703, 0.3219752754296894559, 0.3333333333333333703, 0.3219752754296894559, 0.3333333333333333703, 0.3219752754296894559, 0.3333333333333333703, 0.3219752754296894559, 0.3333333333333333703, 0.3219752754296894559, 0.3333333333333333703, 0.3219752754296894559, 0.3333333333333333703, 0.3219752754296894559, 0.3333333333333333703, 0.3219752754296894559, 0.3333333333333333703, 0.3219752754296894559, 0.3333333333333333703, 0.3219752754296894559, 0.3333333333333333703, 0.3219752754296894559, 0.3333333333333333703, 0.3219752754296894559, 0.3333333333333333703, 0.3219752754296894559, 0.3333333333333333703, 0.3219752754296894559, 0.3333333333333333703, 0.3219752754296894559, 0.3333333333333333703, 0.3219752754296894559, 0.3333333333333333703, 0.3219752754296894559, 0.3333333333333333703, 0.3219752754296894559, 0.3333333333333333703, 0.3219752754296894559, 0.3333333333333333703, 0.3219752754296894559, 0.3333333333333333703, 0.3219752754296894559, 0.3333333333333333703, 0.3219752754296894559, 0.3333333333333333703, 0.3219752754296894559, 0.3333333333333333703, 0.3219752754296894559, 0.3333333333333333703, 0.3219752754296894559, 0.3333333333333333703, 0.3219752754296894559, 0.3333333333333333703, 0.3219752754296894559, 0.3333333333333333703, 0.3219752754296894559, 0.3333333333333333703, 0.3219752754296894559, 0.3333333333333333703, 0.3219752754296894559, 0.3333333333333333703, 0.3219752754296894559, 0.3333333333333333703, 0.3219752754296894559, 0.3333333333333333703, 0.3219752754296894559, 0.3333333333333333703, 0.3219752754296894559, 0.3333333333333333703, 0.3219752754296894559, 0.3333333333333333703, 0.3219752754296894559, 0.3333333333333333703, 0.3219752754296894559, 0.3333333333333333703, 0.3219752754296894559, 0.3333333333333333703, 0.3219752754296894559, 0.3333333333333333703, 0.3219752754296894559, 0.3333333333333333703, 0.3219752754296894559, 0.3333333333333333703, 0.3219752754296894559, 0.3333333333333333703, 0.3219752754296894559, 0.3333333333333333703, 0.3219752754296894559, 0.3333333333333333703, 0.3219752754296894559, 0.3333333333333333703, 0.3219752754296894559, 0.3333333333333333703, 0.3219752754296894559, 0.3333333333333333703, 0.3219752754296894559, 0.3333333333333333703, 0.3219752754296894559, 0.3333333333333333703, 0.3219752754296894559, 0.3333333333333333703, 0.3219752754296894559, 0.3333333333333333703, 0.3219752754296894559, 0.3333333333333333703, 0.3219752754296894559, 0.3333333333333333703, 0.3219752754296894559, 0.3333333333333333703, 0.3219752754296894559, 0.3333333333333333703, 0.3219752754296894559, 0.3333333333333333703, 0.3219752754296894559, 0.3333333333333333703, 0.3219752754296894559, 0.3333333333333333703, 0.3219752754296894559, 0.3333333333333333703, 0.3219752754296894559, 0.3333333333333333703, 0.3219752754296894559, 0.3333333333333333703, 0.3219752754296894559, 0.3333333333333333703, 0.3219752754296894559, 0.3333333333333333703, 0.3219752754296894559, 0.3333333333333333703, 0.3219752754296894559, 0.3333333333333333703, 0.3219752754296894559, 0.3333333333333333703, 0.3219752754296894559, 0.3333333333333333703, 0.3219752754296894559, 0.3333333333333333703, 0.3219752754296894559, 0.3333333333333333703, 0.3219752754296894559, 0.3333333333333333703, 0.3219752754296894559, 0.3333333333333333703, 0.3219752754296894559, 0.3333333333333333703, 0.3219752754296894559, 0.3333333333333333703, 0.3219752754296894559, 0.3333333333333333703, 0.3219752754296894559, 0.3333333333333333703, 0.3219752754296894559, 0.3333333333333333703, 0.3219752754296894559, 0.3333333333333333703, 0.3219752754296894559, 0.3333333333333333703, 0.3219752754296894559, 0.3333333333333333703, 0.3219752754296894559, 0.3333333333333333703, 0.3219752754296894559, 0.3333333333333333703, 0.3219752754296894559, 0.3333333333333333703, 0.3219752754296894559, 0.3333333333333333703, 0.3219752754296894559, 0.3333333333333333703, 0.3219752754296894559, 0.3333333333333333703, 0.3219752754296894559, 0.3333333333333333703, 0.3219752754296894559, 0.3333333333333333703, 0.3219752754296894559, 0.3333333333333333703, 0.3219752754296894559, 0.3333333333333333703, 0.3219752754296894559, 0.3333333333333333703, 0.3219752754296894559, 0.3333333333333333703, 0.3219752754296894559, 0.3333333333333333703, 0.3219752754296894559, 0.3333333333333333703, 0.3219752754296894559, 0.3333333333333333703, 0.3219752754296894559, 0.3333333333333333703, 0.3219752754296894559, 0.3333333333333333703, 0.3219752754296894559, 0.3333333333333333703, 0.3219752754296894559, 0.3333333333333333703, 0.3219752754296894559, 0.3333333333333333703, 0.3219752754296894559, 0.3333333333333333703, 0.3219752754296894559, 0.3333333333333333703, 0.3219752754296894559, 0.3333333333333333703, 0.3219752754296894559, 0.3333333333333333703, 0.3219752754296894559, 0.3333333333333333703, 0.3219752754296894559, 0.3333333333333333703, 0.3219752754296894559, 0.3333333333333333703, 0.3219752754296894559, 0.3333333333333333703, 0.3219752754296894559, 0.3333333333333333703, 0.3219752754296894559, 0.3333333333333333703, 0.3219752754296894559, 0.3333333333333333703, 0.3219752754296894559, 0.3333333333333333703, 0.3219752754296894559, 0.3333333333333333703, 0.3219752754296894559, 0.3333333333333333703, 0.3219752754296894559, 0.3333333333333333703, 0.3219752754296894559, 0.3333333333333333703, 0.3219752754296894559, 0.3333333333333333703, 0.3219752754296894559, 0.3333333333333333703, 0.3219752754296894559, 0.3333333333333333703, 0.3219752754296894559, 0.3333333333333333703, 0.3219752754296894559, 0.3333333333333333703, 0.3219752754296894559, 0.3333333333333333703, 0.3219752754296894559, 0.3333333333333333703, 0.3219752754296894559, 0.3333333333333333703, 0.3219752754296894559, 0.3333333333333333703, 0.3219752754296894559, 0.3333333333333333703, 0.3219752754296894559, 0.3333333333333333703, 0.3219752754296894559, 0.3333333333333333703, 0.3219752754296894559, 0.3333333333333333703, 0.3219752754296894559, 0.3333333333333333703, 0.3219752754296894559, 0.3333333333333333703, 0.3219752754296894559, 0.3333333333333333703, 0.3219752754296894559, 0.3333333333333333703, 0.3219752754296894559, 0.3333333333333333703, 0.3219752754296894559, 0.3333333333333333703, 0.3219752754296894559, 0.3333333333333333703, 0.3219752754296894559, 0.3333333333333333703, 0.3219752754296894559, 0.3333333333333333703, 0.3219752754296894559, 0.3333333333333333703, 0.3219752754296894559, 0.3333333333333333703, 0.3219752754296894559, 0.3333333333333333703, 0.3219752754296894559, 0.3333333333333333703, 0.3219752754296894559, 0.3333333333333333703, 0.3219752754296894559, 0.3333333333333333703, 0.3219752754296894559, 0.3333333333333333703, 0.3219752754296894559, 0.3333333333333333703, 0.3219752754296894559, 0.3333333333333333703, 0.3219752754296894559, 0.3333333333333333703, 0.3219752754296894559, 0.3333333333333333703, 0.3219752754296894559, 0.3333333333333333703, 0.3219752754296894559, 0.3333333333333333703, 0.3219752754296894559, 0.3333333333333333703, 0.3219752754296894559, 0.3333333333333333703, 0.3219752754296894559, 0.3333333333333333703, 0.3219752754296894559, 0.3333333333333333703, 0.3219752754296894559, 0.3333333333333333703, 0.3219752754296894559, 0.3333333333333333703, 0.3219752754296894559, 0.3333333333333333703, 0.3219752754296894559, 0.3333333333333333703, 0.3219752754296894559, 0.3333333333333333703, 0.3219752754296894559, 0.3333333333333333703, 0.3219752754296894559, 0.3333333333333333703, 0.3219752754296894559, 0.3333333333333333703, 0.3219752754296894559, 0.3333333333333333703, 0.3219752754296894559, 0.3333333333333333703, 0.3219752754296894559, 0.3333333333333333703, 0.3219752754296894559, 0.3333333333333333703, 0.3219752754296894559, 0.3333333333333333703, 0.3219752754296894559, 0.3333333333333333703, 0.3219752754296894559, 0.3333333333333333703, 0.3219752754296894559, 0.3333333333333333703, 0.3219752754296894559, 0.3333333333333333703, 0.3219752754296894559, 0.3333333333333333703, 0.3219752754296894559, 0.3333333333333333703, 0.3219752754296894559, 0.3333333333333333703, 0.3219752754296894559, 0.3333333333333333703, 0.3219752754296894559, 0.3333333333333333703, 0.3219752754296894559, 0.3333333333333333703, 0.3219752754296894559, 0.3333333333333333703, 0.3219752754296894559, 0.3333333333333333703, 0.3219752754296894559, 0.3333333333333333703, 0.3219752754296894559, 0.3333333333333333703, 0.3219752754296894559, 0.3333333333333333703, 0.3219752754296894559, 0.3333333333333333703, 0.3219752754296894559, 0.3333333333333333703, 0.3219752754296894559, 0.3333333333333333703, 0.3219752754296894559, 0.3333333333333333703, 0.3219752754296894559, 0.3333333333333333703, 0.3219752754296894559, 0.3333333333333333703, 0.3219752754296894559, 0.3333333333333333703, 0.3219752754296894559, 0.3333333333333333703),
 ( 0.3333333333333333703, 0.3219752754296894559, 0.3333333333333333703, 0.3219752754296894559, 0.3333333333333333703, 0.3219752754296894559, 0.3333333333333333703, 0.3219752754296894559, 0.3333333333333333703, 0.3219752754296894559, 0.3333333333333333703, 0.3219752754296894559, 0.3333333333333333703, 0.3219752754296894559, 0.3333333333333333703, 0.3219752754296894559, 0.3333333333333333703, 0.3219752754296894559, 0.3333333333333333703, 0.3219752754296894559, 0.3333333333333333703, 0.3219752754296894559, 0.3333333333333333703, 0.3219752754296894559, 0.3333333333333333703, 0.3219752754296894559, 0.3333333333333333703, 0.3219752754296894559, 0.3333333333333333703, 0.3219752754296894559, 0.3333333333333333703, 0.3219752754296894559, 0.3333333333333333703, 0.3219752754296894559, 0.3333333333333333703, 0.3219752754296894559, 0.3333333333333333703, 0.3219752754296894559, 0.3333333333333333703, 0.3219752754296894559, 0.3333333333333333703, 0.3219752754296894559, 0.3333333333333333703, 0.3219752754296894559, 0.3333333333333333703, 0.3219752754296894559, 0.3333333333333333703, 0.3219752754296894559, 0.3333333333333333703, 0.3219752754296894559, 0.3333333333333333703, 0.3219752754296894559, 0.3333333333333333703, 0.3219752754296894559, 0.3333333333333333703, 0.3219752754296894559, 0.3333333333333333703, 0.3219752754296894559, 0.3333333333333333703, 0.3219752754296894559, 0.3333333333333333703, 0.3219752754296894559, 0.3333333333333333703, 0.3219752754296894559, 0.3333333333333333703, 0.3219752754296894559, 0.3333333333333333703, 0.3219752754296894559, 0.3333333333333333703, 0.3219752754296894559, 0.3333333333333333703, 0.3219752754296894559, 0.3333333333333333703, 0.3219752754296894559, 0.3333333333333333703, 0.3219752754296894559, 0.3333333333333333703, 0.3219752754296894559, 0.3333333333333333703, 0.3219752754296894559, 0.3333333333333333703, 0.3219752754296894559, 0.3333333333333333703, 0.3219752754296894559, 0.3333333333333333703, 0.3219752754296894559, 0.3333333333333333703, 0.3219752754296894559, 0.3333333333333333703, 0.3219752754296894559, 0.3333333333333333703, 0.3219752754296894559, 0.3333333333333333703, 0.3219752754296894559, 0.3333333333333333703, 0.3219752754296894559, 0.3333333333333333703, 0.3219752754296894559, 0.3333333333333333703, 0.3219752754296894559, 0.3333333333333333703, 0.3219752754296894559, 0.3333333333333333703, 0.3219752754296894559, 0.3333333333333333703, 0.3219752754296894559, 0.3333333333333333703, 0.3219752754296894559, 0.3333333333333333703, 0.3219752754296894559, 0.3333333333333333703, 0.3219752754296894559, 0.3333333333333333703, 0.3219752754296894559, 0.3333333333333333703, 0.3219752754296894559, 0.3333333333333333703, 0.3219752754296894559, 0.3333333333333333703, 0.3219752754296894559, 0.3333333333333333703, 0.3219752754296894559, 0.3333333333333333703, 0.3219752754296894559, 0.3333333333333333703, 0.3219752754296894559, 0.3333333333333333703, 0.3219752754296894559, 0.3333333333333333703, 0.3219752754296894559, 0.3333333333333333703, 0.3219752754296894559, 0.3333333333333333703, 0.3219752754296894559, 0.3333333333333333703, 0.3219752754296894559, 0.3333333333333333703, 0.3219752754296894559, 0.3333333333333333703, 0.3219752754296894559, 0.3333333333333333703, 0.3219752754296894559, 0.3333333333333333703, 0.3219752754296894559, 0.3333333333333333703, 0.3219752754296894559, 0.3333333333333333703, 0.3219752754296894559, 0.3333333333333333703, 0.3219752754296894559, 0.3333333333333333703, 0.3219752754296894559, 0.3333333333333333703, 0.3219752754296894559, 0.3333333333333333703, 0.3219752754296894559, 0.3333333333333333703, 0.3219752754296894559, 0.3333333333333333703, 0.3219752754296894559, 0.3333333333333333703, 0.3219752754296894559, 0.3333333333333333703, 0.3219752754296894559, 0.3333333333333333703, 0.3219752754296894559, 0.3333333333333333703, 0.3219752754296894559, 0.3333333333333333703, 0.3219752754296894559, 0.3333333333333333703, 0.3219752754296894559, 0.3333333333333333703, 0.3219752754296894559, 0.3333333333333333703, 0.3219752754296894559, 0.3333333333333333703, 0.3219752754296894559, 0.3333333333333333703, 0.3219752754296894559, 0.3333333333333333703, 0.3219752754296894559, 0.3333333333333333703, 0.3219752754296894559, 0.3333333333333333703, 0.3219752754296894559, 0.3333333333333333703, 0.3219752754296894559, 0.3333333333333333703, 0.3219752754296894559, 0.3333333333333333703, 0.3219752754296894559, 0.3333333333333333703, 0.3219752754296894559, 0.3333333333333333703, 0.3219752754296894559, 0.3333333333333333703, 0.3219752754296894559, 0.3333333333333333703, 0.3219752754296894559, 0.3333333333333333703, 0.3219752754296894559, 0.3333333333333333703, 0.3219752754296894559, 0.3333333333333333703, 0.3219752754296894559, 0.3333333333333333703, 0.3219752754296894559, 0.3333333333333333703, 0.3219752754296894559, 0.3333333333333333703, 0.3219752754296894559, 0.3333333333333333703, 0.3219752754296894559, 0.3333333333333333703, 0.3219752754296894559, 0.3333333333333333703, 0.3219752754296894559, 0.3333333333333333703, 0.3219752754296894559, 0.3333333333333333703, 0.3219752754296894559, 0.3333333333333333703, 0.3219752754296894559, 0.3333333333333333703, 0.3219752754296894559, 0.3333333333333333703, 0.3219752754296894559, 0.3333333333333333703, 0.3219752754296894559, 0.3333333333333333703, 0.3219752754296894559, 0.3333333333333333703, 0.3219752754296894559, 0.3333333333333333703, 0.3219752754296894559, 0.3333333333333333703, 0.3219752754296894559, 0.3333333333333333703, 0.3219752754296894559, 0.3333333333333333703, 0.3219752754296894559, 0.3333333333333333703, 0.3219752754296894559, 0.3333333333333333703, 0.3219752754296894559, 0.3333333333333333703, 0.3219752754296894559, 0.3333333333333333703, 0.3219752754296894559, 0.3333333333333333703, 0.3219752754296894559, 0.3333333333333333703, 0.3219752754296894559, 0.3333333333333333703, 0.3219752754296894559, 0.3333333333333333703, 0.3219752754296894559, 0.3333333333333333703, 0.3219752754296894559, 0.3333333333333333703, 0.3219752754296894559, 0.3333333333333333703, 0.3219752754296894559, 0.3333333333333333703, 0.3219752754296894559, 0.3333333333333333703, 0.3219752754296894559, 0.3333333333333333703, 0.3219752754296894559, 0.3333333333333333703, 0.3219752754296894559, 0.3333333333333333703, 0.3219752754296894559, 0.3333333333333333703, 0.3219752754296894559, 0.3333333333333333703, 0.3219752754296894559, 0.3333333333333333703, 0.3219752754296894559, 0.3333333333333333703, 0.3219752754296894559, 0.3333333333333333703, 0.3219752754296894559, 0.3333333333333333703, 0.3219752754296894559, 0.3333333333333333703, 0.3219752754296894559, 0.3333333333333333703, 0.3219752754296894559, 0.3333333333333333703, 0.3219752754296894559, 0.3333333333333333703, 0.3219752754296894559, 0.3333333333333333703, 0.3219752754296894559, 0.3333333333333333703, 0.3219752754296894559, 0.3333333333333333703, 0.3219752754296894559, 0.3333333333333333703, 0.3219752754296894559, 0.3333333333333333703, 0.3219752754296894559, 0.3333333333333333703, 0.3219752754296894559, 0.3333333333333333703, 0.3219752754296894559, 0.3333333333333333703, 0.3219752754296894559, 0.3333333333333333703, 0.3219752754296894559, 0.3333333333333333703, 0.3219752754296894559, 0.3333333333333333703, 0.3219752754296894559, 0.3333333333333333703, 0.3219752754296894559, 0.3333333333333333703, 0.3219752754296894559, 0.3333333333333333703, 0.3219752754296894559, 0.3333333333333333703, 0.3219752754296894559, 0.3333333333333333703, 0.3219752754296894559, 0.3333333333333333703, 0.3219752754296894559, 0.3333333333333333703, 0.3219752754296894559, 0.3333333333333333703, 0.3219752754296894559, 0.3333333333333333703, 0.3219752754296894559, 0.3333333333333333703, 0.3219752754296894559, 0.3333333333333333703, 0.3219752754296894559, 0.3333333333333333703, 0.3219752754296894559, 0.3333333333333333703, 0.3219752754296894559, 0.3333333333333333703, 0.3219752754296894559, 0.3333333333333333703, 0.3219752754296894559, 0.3333333333333333703, 0.3219752754296894559, 0.3333333333333333703, 0.3219752754296894559, 0.3333333333333333703, 0.3219752754296894559, 0.3333333333333333703, 0.3219752754296894559, 0.3333333333333333703, 0.3219752754296894559, 0.3333333333333333703, 0.3219752754296894559, 0.3333333333333333703, 0.3219752754296894559, 0.3333333333333333703, 0.3219752754296894559, 0.3333333333333333703, 0.3219752754296894559, 0.3333333333333333703, 0.3219752754296894559, 0.3333333333333333703, 0.3219752754296894559, 0.3333333333333333703, 0.3219752754296894559, 0.3333333333333333703, 0.3219752754296894559, 0.3333333333333333703, 0.3219752754296894559, 0.3333333333333333703, 0.3219752754296894559, 0.3333333333333333703, 0.3219752754296894559, 0.3333333333333333703, 0.3219752754296894559, 0.3333333333333333703, 0.3219752754296894559, 0.3333333333333333703, 0.3219752754296894559, 0.3333333333333333703, 0.3219752754296894559, 0.3333333333333333703, 0.3219752754296894559, 0.3333333333333333703, 0.3219752754296894559, 0.3333333333333333703, 0.3219752754296894559, 0.3333333333333333703, 0.3219752754296894559, 0.3333333333333333703, 0.3219752754296894559, 0.3333333333333333703, 0.3219752754296894559, 0.3333333333333333703, 0.3219752754296894559, 0.3333333333333333703, 0.3219752754296894559, 0.3333333333333333703, 0.3219752754296894559, 0.3333333333333333703, 0.3219752754296894559, 0.3333333333333333703, 0.3219752754296894559, 0.3333333333333333703, 0.3219752754296894559, 0.3333333333333333703, 0.3219752754296894559, 0.3333333333333333703, 0.3219752754296894559, 0.3333333333333333703, 0.3219752754296894559, 0.3333333333333333703, 0.3219752754296894559, 0.3333333333333333703, 0.3219752754296894559, 0.3333333333333333703, 0.3219752754296894559, 0.3333333333333333703, 0.3219752754296894559, 0.3333333333333333703, 0.3219752754296894559, 0.3333333333333333703, 0.3219752754296894559, 0.3333333333333333703, 0.3219752754296894559, 0.3333333333333333703, 0.3219752754296894559, 0.3333333333333333703, 0.3219752754296894559, 0.3333333333333333703, 0.3219752754296894559, 0.3333333333333333703, 0.3219752754296894559, 0.3333333333333333703, 0.3219752754296894559, 0.3333333333333333703, 0.3219752754296894559, 0.3333333333333333703, 0.3219752754296894559, 0.3333333333333333703, 0.3219752754296894559, 0.3333333333333333703, 0.3219752754296894559, 0.3333333333333333703, 0.3219752754296894559, 0.3333333333333333703, 0.3219752754296894559, 0.3333333333333333703, 0.3219752754296894559, 0.3333333333333333703, 0.3219752754296894559, 0.3333333333333333703),
 ( 1.000000000000000000, 0.9659258262890683122, 1.000000000000000000, 0.9659258262890683122, 1.000000000000000000, 0.9659258262890683122, 1.000000000000000000, 0.9659258262890683122, 1.000000000000000000, 0.9659258262890683122, 1.000000000000000000, 0.9659258262890683122, 1.000000000000000000, 0.9659258262890683122, 1.000000000000000000, 0.9659258262890683122, 1.000000000000000000, 0.9659258262890683122, 1.000000000000000000, 0.9659258262890683122, 1.000000000000000000, 0.9659258262890683122, 1.000000000000000000, 0.9659258262890683122, 1.000000000000000000, 0.9659258262890683122, 1.000000000000000000, 0.9659258262890683122, 1.000000000000000000, 0.9659258262890683122, 1.000000000000000000, 0.9659258262890683122, 1.000000000000000000, 0.9659258262890683122, 1.000000000000000000, 0.9659258262890683122, 1.000000000000000000, 0.9659258262890683122, 1.000000000000000000, 0.9659258262890683122, 1.000000000000000000, 0.9659258262890683122, 1.000000000000000000, 0.9659258262890683122, 1.000000000000000000, 0.9659258262890683122, 1.000000000000000000, 0.9659258262890683122, 1.000000000000000000, 0.9659258262890683122, 1.000000000000000000, 0.9659258262890683122, 1.000000000000000000, 0.9659258262890683122, 1.000000000000000000, 0.9659258262890683122, 1.000000000000000000, 0.9659258262890683122, 1.000000000000000000, 0.9659258262890683122, 1.000000000000000000, 0.9659258262890683122, 1.000000000000000000, 0.9659258262890683122, 1.000000000000000000, 0.9659258262890683122, 1.000000000000000000, 0.9659258262890683122, 1.000000000000000000, 0.9659258262890683122, 1.000000000000000000, 0.9659258262890683122, 1.000000000000000000, 0.9659258262890683122, 1.000000000000000000, 0.9659258262890683122, 1.000000000000000000, 0.9659258262890683122, 1.000000000000000000, 0.9659258262890683122, 1.000000000000000000, 0.9659258262890683122, 1.000000000000000000, 0.9659258262890683122, 1.000000000000000000, 0.9659258262890683122, 1.000000000000000000, 0.9659258262890683122, 1.000000000000000000, 0.9659258262890683122, 1.000000000000000000, 0.9659258262890683122, 1.000000000000000000, 0.9659258262890683122, 1.000000000000000000, 0.9659258262890683122, 1.000000000000000000, 0.9659258262890683122, 1.000000000000000000, 0.9659258262890683122, 1.000000000000000000, 0.9659258262890683122, 1.000000000000000000, 0.9659258262890683122, 1.000000000000000000, 0.9659258262890683122, 1.000000000000000000, 0.9659258262890683122, 1.000000000000000000, 0.9659258262890683122, 1.000000000000000000, 0.9659258262890683122, 1.000000000000000000, 0.9659258262890683122, 1.000000000000000000, 0.9659258262890683122, 1.000000000000000000, 0.9659258262890683122, 1.000000000000000000, 0.9659258262890683122, 1.000000000000000000, 0.9659258262890683122, 1.000000000000000000, 0.9659258262890683122, 1.000000000000000000, 0.9659258262890683122, 1.000000000000000000, 0.9659258262890683122, 1.000000000000000000, 0.9659258262890683122, 1.000000000000000000, 0.9659258262890683122, 1.000000000000000000, 0.9659258262890683122, 1.000000000000000000, 0.9659258262890683122, 1.000000000000000000, 0.9659258262890683122, 1.000000000000000000, 0.9659258262890683122, 1.000000000000000000, 0.9659258262890683122, 1.000000000000000000, 0.9659258262890683122, 1.000000000000000000, 0.9659258262890683122, 1.000000000000000000, 0.9659258262890683122, 1.000000000000000000, 0.9659258262890683122, 1.000000000000000000, 0.9659258262890683122, 1.000000000000000000, 0.9659258262890683122, 1.000000000000000000, 0.9659258262890683122, 1.000000000000000000, 0.9659258262890683122, 1.000000000000000000, 0.9659258262890683122, 1.000000000000000000, 0.9659258262890683122, 1.000000000000000000, 0.9659258262890683122, 1.000000000000000000, 0.9659258262890683122, 1.000000000000000000, 0.9659258262890683122, 1.000000000000000000, 0.9659258262890683122, 1.000000000000000000, 0.9659258262890683122, 1.000000000000000000, 0.9659258262890683122, 1.000000000000000000, 0.9659258262890683122, 1.000000000000000000, 0.9659258262890683122, 1.000000000000000000, 0.9659258262890683122, 1.000000000000000000, 0.9659258262890683122, 1.000000000000000000, 0.9659258262890683122, 1.000000000000000000, 0.9659258262890683122, 1.000000000000000000, 0.9659258262890683122, 1.000000000000000000, 0.9659258262890683122, 1.000000000000000000, 0.9659258262890683122, 1.000000000000000000, 0.9659258262890683122, 1.000000000000000000, 0.9659258262890683122, 1.000000000000000000, 0.9659258262890683122, 1.000000000000000000, 0.9659258262890683122, 1.000000000000000000, 0.9659258262890683122, 1.000000000000000000, 0.9659258262890683122, 1.000000000000000000, 0.9659258262890683122, 1.000000000000000000, 0.9659258262890683122, 1.000000000000000000, 0.9659258262890683122, 1.000000000000000000, 0.9659258262890683122, 1.000000000000000000, 0.9659258262890683122, 1.000000000000000000, 0.9659258262890683122, 1.000000000000000000, 0.9659258262890683122, 1.000000000000000000, 0.9659258262890683122, 1.000000000000000000, 0.9659258262890683122, 1.000000000000000000, 0.9659258262890683122, 1.000000000000000000, 0.9659258262890683122, 1.000000000000000000, 0.9659258262890683122, 1.000000000000000000, 0.9659258262890683122, 1.000000000000000000, 0.9659258262890683122, 1.000000000000000000, 0.9659258262890683122, 1.000000000000000000, 0.9659258262890683122, 1.000000000000000000, 0.9659258262890683122, 1.000000000000000000, 0.9659258262890683122, 1.000000000000000000, 0.9659258262890683122, 1.000000000000000000, 0.9659258262890683122, 1.000000000000000000, 0.9659258262890683122, 1.000000000000000000, 0.9659258262890683122, 1.000000000000000000, 0.9659258262890683122, 1.000000000000000000, 0.9659258262890683122, 1.000000000000000000, 0.9659258262890683122, 1.000000000000000000, 0.9659258262890683122, 1.000000000000000000, 0.9659258262890683122, 1.000000000000000000, 0.9659258262890683122, 1.000000000000000000, 0.9659258262890683122, 1.000000000000000000, 0.9659258262890683122, 1.000000000000000000, 0.9659258262890683122, 1.000000000000000000, 0.9659258262890683122, 1.000000000000000000, 0.9659258262890683122, 1.000000000000000000, 0.9659258262890683122, 1.000000000000000000, 0.9659258262890683122, 1.000000000000000000, 0.9659258262890683122, 1.000000000000000000, 0.9659258262890683122, 1.000000000000000000, 0.9659258262890683122, 1.000000000000000000, 0.9659258262890683122, 1.000000000000000000, 0.9659258262890683122, 1.000000000000000000, 0.9659258262890683122, 1.000000000000000000, 0.9659258262890683122, 1.000000000000000000, 0.9659258262890683122, 1.000000000000000000, 0.9659258262890683122, 1.000000000000000000, 0.9659258262890683122, 1.000000000000000000, 0.9659258262890683122, 1.000000000000000000, 0.9659258262890683122, 1.000000000000000000, 0.9659258262890683122, 1.000000000000000000, 0.9659258262890683122, 1.000000000000000000, 0.9659258262890683122, 1.000000000000000000, 0.9659258262890683122, 1.000000000000000000, 0.9659258262890683122, 1.000000000000000000, 0.9659258262890683122, 1.000000000000000000, 0.9659258262890683122, 1.000000000000000000, 0.9659258262890683122, 1.000000000000000000, 0.9659258262890683122, 1.000000000000000000, 0.9659258262890683122, 1.000000000000000000, 0.9659258262890683122, 1.000000000000000000, 0.9659258262890683122, 1.000000000000000000, 0.9659258262890683122, 1.000000000000000000, 0.9659258262890683122, 1.000000000000000000, 0.9659258262890683122, 1.000000000000000000, 0.9659258262890683122, 1.000000000000000000, 0.9659258262890683122, 1.000000000000000000, 0.9659258262890683122, 1.000000000000000000, 0.9659258262890683122, 1.000000000000000000, 0.9659258262890683122, 1.000000000000000000, 0.9659258262890683122, 1.000000000000000000, 0.9659258262890683122, 1.000000000000000000, 0.9659258262890683122, 1.000000000000000000, 0.9659258262890683122, 1.000000000000000000, 0.9659258262890683122, 1.000000000000000000, 0.9659258262890683122, 1.000000000000000000, 0.9659258262890683122, 1.000000000000000000, 0.9659258262890683122, 1.000000000000000000, 0.9659258262890683122, 1.000000000000000000, 0.9659258262890683122, 1.000000000000000000, 0.9659258262890683122, 1.000000000000000000, 0.9659258262890683122, 1.000000000000000000, 0.9659258262890683122, 1.000000000000000000, 0.9659258262890683122, 1.000000000000000000, 0.9659258262890683122, 1.000000000000000000, 0.9659258262890683122, 1.000000000000000000, 0.9659258262890683122, 1.000000000000000000, 0.9659258262890683122, 1.000000000000000000, 0.9659258262890683122, 1.000000000000000000, 0.9659258262890683122, 1.000000000000000000, 0.9659258262890683122, 1.000000000000000000, 0.9659258262890683122, 1.000000000000000000, 0.9659258262890683122, 1.000000000000000000, 0.9659258262890683122, 1.000000000000000000, 0.9659258262890683122, 1.000000000000000000, 0.9659258262890683122, 1.000000000000000000, 0.9659258262890683122, 1.000000000000000000, 0.9659258262890683122, 1.000000000000000000, 0.9659258262890683122, 1.000000000000000000, 0.9659258262890683122, 1.000000000000000000, 0.9659258262890683122, 1.000000000000000000, 0.9659258262890683122, 1.000000000000000000, 0.9659258262890683122, 1.000000000000000000, 0.9659258262890683122, 1.000000000000000000, 0.9659258262890683122, 1.000000000000000000, 0.9659258262890683122, 1.000000000000000000, 0.9659258262890683122, 1.000000000000000000, 0.9659258262890683122, 1.000000000000000000, 0.9659258262890683122, 1.000000000000000000, 0.9659258262890683122, 1.000000000000000000, 0.9659258262890683122, 1.000000000000000000, 0.9659258262890683122, 1.000000000000000000, 0.9659258262890683122, 1.000000000000000000, 0.9659258262890683122, 1.000000000000000000, 0.9659258262890683122, 1.000000000000000000, 0.9659258262890683122, 1.000000000000000000, 0.9659258262890683122, 1.000000000000000000, 0.9659258262890683122, 1.000000000000000000, 0.9659258262890683122, 1.000000000000000000, 0.9659258262890683122, 1.000000000000000000, 0.9659258262890683122, 1.000000000000000000, 0.9659258262890683122, 1.000000000000000000, 0.9659258262890683122, 1.000000000000000000, 0.9659258262890683122, 1.000000000000000000, 0.9659258262890683122, 1.000000000000000000, 0.9659258262890683122, 1.000000000000000000, 0.9659258262890683122, 1.000000000000000000, 0.9659258262890683122, 1.000000000000000000, 0.9659258262890683122, 1.000000000000000000),
 ( 0.3333333333333333703, 0.3219752754296894559, 0.3333333333333333703, 0.3219752754296894559, 0.3333333333333333703, 0.3219752754296894559, 0.3333333333333333703, 0.3219752754296894559, 0.3333333333333333703, 0.3219752754296894559, 0.3333333333333333703, 0.3219752754296894559, 0.3333333333333333703, 0.3219752754296894559, 0.3333333333333333703, 0.3219752754296894559, 0.3333333333333333703, 0.3219752754296894559, 0.3333333333333333703, 0.3219752754296894559, 0.3333333333333333703, 0.3219752754296894559, 0.3333333333333333703, 0.3219752754296894559, 0.3333333333333333703, 0.3219752754296894559, 0.3333333333333333703, 0.3219752754296894559, 0.3333333333333333703, 0.3219752754296894559, 0.3333333333333333703, 0.3219752754296894559, 0.3333333333333333703, 0.3219752754296894559, 0.3333333333333333703, 0.3219752754296894559, 0.3333333333333333703, 0.3219752754296894559, 0.3333333333333333703, 0.3219752754296894559, 0.3333333333333333703, 0.3219752754296894559, 0.3333333333333333703, 0.3219752754296894559, 0.3333333333333333703, 0.3219752754296894559, 0.3333333333333333703, 0.3219752754296894559, 0.3333333333333333703, 0.3219752754296894559, 0.3333333333333333703, 0.3219752754296894559, 0.3333333333333333703, 0.3219752754296894559, 0.3333333333333333703, 0.3219752754296894559, 0.3333333333333333703, 0.3219752754296894559, 0.3333333333333333703, 0.3219752754296894559, 0.3333333333333333703, 0.3219752754296894559, 0.3333333333333333703, 0.3219752754296894559, 0.3333333333333333703, 0.3219752754296894559, 0.3333333333333333703, 0.3219752754296894559, 0.3333333333333333703, 0.3219752754296894559, 0.3333333333333333703, 0.3219752754296894559, 0.3333333333333333703, 0.3219752754296894559, 0.3333333333333333703, 0.3219752754296894559, 0.3333333333333333703, 0.3219752754296894559, 0.3333333333333333703, 0.3219752754296894559, 0.3333333333333333703, 0.3219752754296894559, 0.3333333333333333703, 0.3219752754296894559, 0.3333333333333333703, 0.3219752754296894559, 0.3333333333333333703, 0.3219752754296894559, 0.3333333333333333703, 0.3219752754296894559, 0.3333333333333333703, 0.3219752754296894559, 0.3333333333333333703, 0.3219752754296894559, 0.3333333333333333703, 0.3219752754296894559, 0.3333333333333333703, 0.3219752754296894559, 0.3333333333333333703, 0.3219752754296894559, 0.3333333333333333703, 0.3219752754296894559, 0.3333333333333333703, 0.3219752754296894559, 0.3333333333333333703, 0.3219752754296894559, 0.3333333333333333703, 0.3219752754296894559, 0.3333333333333333703, 0.3219752754296894559, 0.3333333333333333703, 0.3219752754296894559, 0.3333333333333333703, 0.3219752754296894559, 0.3333333333333333703, 0.3219752754296894559, 0.3333333333333333703, 0.3219752754296894559, 0.3333333333333333703, 0.3219752754296894559, 0.3333333333333333703, 0.3219752754296894559, 0.3333333333333333703, 0.3219752754296894559, 0.3333333333333333703, 0.3219752754296894559, 0.3333333333333333703, 0.3219752754296894559, 0.3333333333333333703, 0.3219752754296894559, 0.3333333333333333703, 0.3219752754296894559, 0.3333333333333333703, 0.3219752754296894559, 0.3333333333333333703, 0.3219752754296894559, 0.3333333333333333703, 0.3219752754296894559, 0.3333333333333333703, 0.3219752754296894559, 0.3333333333333333703, 0.3219752754296894559, 0.3333333333333333703, 0.3219752754296894559, 0.3333333333333333703, 0.3219752754296894559, 0.3333333333333333703, 0.3219752754296894559, 0.3333333333333333703, 0.3219752754296894559, 0.3333333333333333703, 0.3219752754296894559, 0.3333333333333333703, 0.3219752754296894559, 0.3333333333333333703, 0.3219752754296894559, 0.3333333333333333703, 0.3219752754296894559, 0.3333333333333333703, 0.3219752754296894559, 0.3333333333333333703, 0.3219752754296894559, 0.3333333333333333703, 0.3219752754296894559, 0.3333333333333333703, 0.3219752754296894559, 0.3333333333333333703, 0.3219752754296894559, 0.3333333333333333703, 0.3219752754296894559, 0.3333333333333333703, 0.3219752754296894559, 0.3333333333333333703, 0.3219752754296894559, 0.3333333333333333703, 0.3219752754296894559, 0.3333333333333333703, 0.3219752754296894559, 0.3333333333333333703, 0.3219752754296894559, 0.3333333333333333703, 0.3219752754296894559, 0.3333333333333333703, 0.3219752754296894559, 0.3333333333333333703, 0.3219752754296894559, 0.3333333333333333703, 0.3219752754296894559, 0.3333333333333333703, 0.3219752754296894559, 0.3333333333333333703, 0.3219752754296894559, 0.3333333333333333703, 0.3219752754296894559, 0.3333333333333333703, 0.3219752754296894559, 0.3333333333333333703, 0.3219752754296894559, 0.3333333333333333703, 0.3219752754296894559, 0.3333333333333333703, 0.3219752754296894559, 0.3333333333333333703, 0.3219752754296894559, 0.3333333333333333703, 0.3219752754296894559, 0.3333333333333333703, 0.3219752754296894559, 0.3333333333333333703, 0.3219752754296894559, 0.3333333333333333703, 0.3219752754296894559, 0.3333333333333333703, 0.3219752754296894559, 0.3333333333333333703, 0.3219752754296894559, 0.3333333333333333703, 0.3219752754296894559, 0.3333333333333333703, 0.3219752754296894559, 0.3333333333333333703, 0.3219752754296894559, 0.3333333333333333703, 0.3219752754296894559, 0.3333333333333333703, 0.3219752754296894559, 0.3333333333333333703, 0.3219752754296894559, 0.3333333333333333703, 0.3219752754296894559, 0.3333333333333333703, 0.3219752754296894559, 0.3333333333333333703, 0.3219752754296894559, 0.3333333333333333703, 0.3219752754296894559, 0.3333333333333333703, 0.3219752754296894559, 0.3333333333333333703, 0.3219752754296894559, 0.3333333333333333703, 0.3219752754296894559, 0.3333333333333333703, 0.3219752754296894559, 0.3333333333333333703, 0.3219752754296894559, 0.3333333333333333703, 0.3219752754296894559, 0.3333333333333333703, 0.3219752754296894559, 0.3333333333333333703, 0.3219752754296894559, 0.3333333333333333703, 0.3219752754296894559, 0.3333333333333333703, 0.3219752754296894559, 0.3333333333333333703, 0.3219752754296894559, 0.3333333333333333703, 0.3219752754296894559, 0.3333333333333333703, 0.3219752754296894559, 0.3333333333333333703, 0.3219752754296894559, 0.3333333333333333703, 0.3219752754296894559, 0.3333333333333333703, 0.3219752754296894559, 0.3333333333333333703, 0.3219752754296894559, 0.3333333333333333703, 0.3219752754296894559, 0.3333333333333333703, 0.3219752754296894559, 0.3333333333333333703, 0.3219752754296894559, 0.3333333333333333703, 0.3219752754296894559, 0.3333333333333333703, 0.3219752754296894559, 0.3333333333333333703, 0.3219752754296894559, 0.3333333333333333703, 0.3219752754296894559, 0.3333333333333333703, 0.3219752754296894559, 0.3333333333333333703, 0.3219752754296894559, 0.3333333333333333703, 0.3219752754296894559, 0.3333333333333333703, 0.3219752754296894559, 0.3333333333333333703, 0.3219752754296894559, 0.3333333333333333703, 0.3219752754296894559, 0.3333333333333333703, 0.3219752754296894559, 0.3333333333333333703, 0.3219752754296894559, 0.3333333333333333703, 0.3219752754296894559, 0.3333333333333333703, 0.3219752754296894559, 0.3333333333333333703, 0.3219752754296894559, 0.3333333333333333703, 0.3219752754296894559, 0.3333333333333333703, 0.3219752754296894559, 0.3333333333333333703, 0.3219752754296894559, 0.3333333333333333703, 0.3219752754296894559, 0.3333333333333333703, 0.3219752754296894559, 0.3333333333333333703, 0.3219752754296894559, 0.3333333333333333703, 0.3219752754296894559, 0.3333333333333333703, 0.3219752754296894559, 0.3333333333333333703, 0.3219752754296894559, 0.3333333333333333703, 0.3219752754296894559, 0.3333333333333333703, 0.3219752754296894559, 0.3333333333333333703, 0.3219752754296894559, 0.3333333333333333703, 0.3219752754296894559, 0.3333333333333333703, 0.3219752754296894559, 0.3333333333333333703, 0.3219752754296894559, 0.3333333333333333703, 0.3219752754296894559, 0.3333333333333333703, 0.3219752754296894559, 0.3333333333333333703, 0.3219752754296894559, 0.3333333333333333703, 0.3219752754296894559, 0.3333333333333333703, 0.3219752754296894559, 0.3333333333333333703, 0.3219752754296894559, 0.3333333333333333703, 0.3219752754296894559, 0.3333333333333333703, 0.3219752754296894559, 0.3333333333333333703, 0.3219752754296894559, 0.3333333333333333703, 0.3219752754296894559, 0.3333333333333333703, 0.3219752754296894559, 0.3333333333333333703, 0.3219752754296894559, 0.3333333333333333703, 0.3219752754296894559, 0.3333333333333333703, 0.3219752754296894559, 0.3333333333333333703, 0.3219752754296894559, 0.3333333333333333703, 0.3219752754296894559, 0.3333333333333333703, 0.3219752754296894559, 0.3333333333333333703, 0.3219752754296894559, 0.3333333333333333703, 0.3219752754296894559, 0.3333333333333333703, 0.3219752754296894559, 0.3333333333333333703, 0.3219752754296894559, 0.3333333333333333703, 0.3219752754296894559, 0.3333333333333333703, 0.3219752754296894559, 0.3333333333333333703, 0.3219752754296894559, 0.3333333333333333703, 0.3219752754296894559, 0.3333333333333333703, 0.3219752754296894559, 0.3333333333333333703, 0.3219752754296894559, 0.3333333333333333703, 0.3219752754296894559, 0.3333333333333333703, 0.3219752754296894559, 0.3333333333333333703, 0.3219752754296894559, 0.3333333333333333703, 0.3219752754296894559, 0.3333333333333333703, 0.3219752754296894559, 0.3333333333333333703, 0.3219752754296894559, 0.3333333333333333703, 0.3219752754296894559, 0.3333333333333333703, 0.3219752754296894559, 0.3333333333333333703, 0.3219752754296894559, 0.3333333333333333703, 0.3219752754296894559, 0.3333333333333333703, 0.3219752754296894559, 0.3333333333333333703, 0.3219752754296894559, 0.3333333333333333703, 0.3219752754296894559, 0.3333333333333333703, 0.3219752754296894559, 0.3333333333333333703, 0.3219752754296894559, 0.3333333333333333703, 0.3219752754296894559, 0.3333333333333333703, 0.3219752754296894559, 0.3333333333333333703, 0.3219752754296894559, 0.3333333333333333703, 0.3219752754296894559, 0.3333333333333333703, 0.3219752754296894559, 0.3333333333333333703, 0.3219752754296894559, 0.3333333333333333703, 0.3219752754296894559, 0.3333333333333333703, 0.3219752754296894559, 0.3333333333333333703, 0.3219752754296894559, 0.3333333333333333703, 0.3219752754296894559, 0.3333333333333333703, 0.3219752754296894559, 0.3333333333333333703, 0.3219752754296894559, 0.3333333333333333703, 0.3219752754296894559, 0.3333333333333333703, 0.3219752754296894559, 0.3333333333333333703, 0.3219752754296894559, 0.3333333333333333703, 0.3219752754296894559, 0.3333333333333333703, 0.3219752754296894559, 0.3333333333333333703, 0.3219752754296894559, 0.3333333333333333703),
 ( 0.3333333333333333703, 0.3219752754296894559, 0.3333333333333333703, 0.3219752754296894559, 0.3333333333333333703, 0.3219752754296894559, 0.3333333333333333703, 0.3219752754296894559, 0.3333333333333333703, 0.3219752754296894559, 0.3333333333333333703, 0.3219752754296894559, 0.3333333333333333703, 0.3219752754296894559, 0.3333333333333333703, 0.3219752754296894559, 0.3333333333333333703, 0.3219752754296894559, 0.3333333333333333703, 0.3219752754296894559, 0.3333333333333333703, 0.3219752754296894559, 0.3333333333333333703, 0.3219752754296894559, 0.3333333333333333703, 0.3219752754296894559, 0.3333333333333333703, 0.3219752754296894559, 0.3333333333333333703, 0.3219752754296894559, 0.3333333333333333703, 0.3219752754296894559, 0.3333333333333333703, 0.3219752754296894559, 0.3333333333333333703, 0.3219752754296894559, 0.3333333333333333703, 0.3219752754296894559, 0.3333333333333333703, 0.3219752754296894559, 0.3333333333333333703, 0.3219752754296894559, 0.3333333333333333703, 0.3219752754296894559, 0.3333333333333333703, 0.3219752754296894559, 0.3333333333333333703, 0.3219752754296894559, 0.3333333333333333703, 0.3219752754296894559, 0.3333333333333333703, 0.3219752754296894559, 0.3333333333333333703, 0.3219752754296894559, 0.3333333333333333703, 0.3219752754296894559, 0.3333333333333333703, 0.3219752754296894559, 0.3333333333333333703, 0.3219752754296894559, 0.3333333333333333703, 0.3219752754296894559, 0.3333333333333333703, 0.3219752754296894559, 0.3333333333333333703, 0.3219752754296894559, 0.3333333333333333703, 0.3219752754296894559, 0.3333333333333333703, 0.3219752754296894559, 0.3333333333333333703, 0.3219752754296894559, 0.3333333333333333703, 0.3219752754296894559, 0.3333333333333333703, 0.3219752754296894559, 0.3333333333333333703, 0.3219752754296894559, 0.3333333333333333703, 0.3219752754296894559, 0.3333333333333333703, 0.3219752754296894559, 0.3333333333333333703, 0.3219752754296894559, 0.3333333333333333703, 0.3219752754296894559, 0.3333333333333333703, 0.3219752754296894559, 0.3333333333333333703, 0.3219752754296894559, 0.3333333333333333703, 0.3219752754296894559, 0.3333333333333333703, 0.3219752754296894559, 0.3333333333333333703, 0.3219752754296894559, 0.3333333333333333703, 0.3219752754296894559, 0.3333333333333333703, 0.3219752754296894559, 0.3333333333333333703, 0.3219752754296894559, 0.3333333333333333703, 0.3219752754296894559, 0.3333333333333333703, 0.3219752754296894559, 0.3333333333333333703, 0.3219752754296894559, 0.3333333333333333703, 0.3219752754296894559, 0.3333333333333333703, 0.3219752754296894559, 0.3333333333333333703, 0.3219752754296894559, 0.3333333333333333703, 0.3219752754296894559, 0.3333333333333333703, 0.3219752754296894559, 0.3333333333333333703, 0.3219752754296894559, 0.3333333333333333703, 0.3219752754296894559, 0.3333333333333333703, 0.3219752754296894559, 0.3333333333333333703, 0.3219752754296894559, 0.3333333333333333703, 0.3219752754296894559, 0.3333333333333333703, 0.3219752754296894559, 0.3333333333333333703, 0.3219752754296894559, 0.3333333333333333703, 0.3219752754296894559, 0.3333333333333333703, 0.3219752754296894559, 0.3333333333333333703, 0.3219752754296894559, 0.3333333333333333703, 0.3219752754296894559, 0.3333333333333333703, 0.3219752754296894559, 0.3333333333333333703, 0.3219752754296894559, 0.3333333333333333703, 0.3219752754296894559, 0.3333333333333333703, 0.3219752754296894559, 0.3333333333333333703, 0.3219752754296894559, 0.3333333333333333703, 0.3219752754296894559, 0.3333333333333333703, 0.3219752754296894559, 0.3333333333333333703, 0.3219752754296894559, 0.3333333333333333703, 0.3219752754296894559, 0.3333333333333333703, 0.3219752754296894559, 0.3333333333333333703, 0.3219752754296894559, 0.3333333333333333703, 0.3219752754296894559, 0.3333333333333333703, 0.3219752754296894559, 0.3333333333333333703, 0.3219752754296894559, 0.3333333333333333703, 0.3219752754296894559, 0.3333333333333333703, 0.3219752754296894559, 0.3333333333333333703, 0.3219752754296894559, 0.3333333333333333703, 0.3219752754296894559, 0.3333333333333333703, 0.3219752754296894559, 0.3333333333333333703, 0.3219752754296894559, 0.3333333333333333703, 0.3219752754296894559, 0.3333333333333333703, 0.3219752754296894559, 0.3333333333333333703, 0.3219752754296894559, 0.3333333333333333703, 0.3219752754296894559, 0.3333333333333333703, 0.3219752754296894559, 0.3333333333333333703, 0.3219752754296894559, 0.3333333333333333703, 0.3219752754296894559, 0.3333333333333333703, 0.3219752754296894559, 0.3333333333333333703, 0.3219752754296894559, 0.3333333333333333703, 0.3219752754296894559, 0.3333333333333333703, 0.3219752754296894559, 0.3333333333333333703, 0.3219752754296894559, 0.3333333333333333703, 0.3219752754296894559, 0.3333333333333333703, 0.3219752754296894559, 0.3333333333333333703, 0.3219752754296894559, 0.3333333333333333703, 0.3219752754296894559, 0.3333333333333333703, 0.3219752754296894559, 0.3333333333333333703, 0.3219752754296894559, 0.3333333333333333703, 0.3219752754296894559, 0.3333333333333333703, 0.3219752754296894559, 0.3333333333333333703, 0.3219752754296894559, 0.3333333333333333703, 0.3219752754296894559, 0.3333333333333333703, 0.3219752754296894559, 0.3333333333333333703, 0.3219752754296894559, 0.3333333333333333703, 0.3219752754296894559, 0.3333333333333333703, 0.3219752754296894559, 0.3333333333333333703, 0.3219752754296894559, 0.3333333333333333703, 0.3219752754296894559, 0.3333333333333333703, 0.3219752754296894559, 0.3333333333333333703, 0.3219752754296894559, 0.3333333333333333703, 0.3219752754296894559, 0.3333333333333333703, 0.3219752754296894559, 0.3333333333333333703, 0.3219752754296894559, 0.3333333333333333703, 0.3219752754296894559, 0.3333333333333333703, 0.3219752754296894559, 0.3333333333333333703, 0.3219752754296894559, 0.3333333333333333703, 0.3219752754296894559, 0.3333333333333333703, 0.3219752754296894559, 0.3333333333333333703, 0.3219752754296894559, 0.3333333333333333703, 0.3219752754296894559, 0.3333333333333333703, 0.3219752754296894559, 0.3333333333333333703, 0.3219752754296894559, 0.3333333333333333703, 0.3219752754296894559, 0.3333333333333333703, 0.3219752754296894559, 0.3333333333333333703, 0.3219752754296894559, 0.3333333333333333703, 0.3219752754296894559, 0.3333333333333333703, 0.3219752754296894559, 0.3333333333333333703, 0.3219752754296894559, 0.3333333333333333703, 0.3219752754296894559, 0.3333333333333333703, 0.3219752754296894559, 0.3333333333333333703, 0.3219752754296894559, 0.3333333333333333703, 0.3219752754296894559, 0.3333333333333333703, 0.3219752754296894559, 0.3333333333333333703, 0.3219752754296894559, 0.3333333333333333703, 0.3219752754296894559, 0.3333333333333333703, 0.3219752754296894559, 0.3333333333333333703, 0.3219752754296894559, 0.3333333333333333703, 0.3219752754296894559, 0.3333333333333333703, 0.3219752754296894559, 0.3333333333333333703, 0.3219752754296894559, 0.3333333333333333703, 0.3219752754296894559, 0.3333333333333333703, 0.3219752754296894559, 0.3333333333333333703, 0.3219752754296894559, 0.3333333333333333703, 0.3219752754296894559, 0.3333333333333333703, 0.3219752754296894559, 0.3333333333333333703, 0.3219752754296894559, 0.3333333333333333703, 0.3219752754296894559, 0.3333333333333333703, 0.3219752754296894559, 0.3333333333333333703, 0.3219752754296894559, 0.3333333333333333703, 0.3219752754296894559, 0.3333333333333333703, 0.3219752754296894559, 0.3333333333333333703, 0.3219752754296894559, 0.3333333333333333703, 0.3219752754296894559, 0.3333333333333333703, 0.3219752754296894559, 0.3333333333333333703, 0.3219752754296894559, 0.3333333333333333703, 0.3219752754296894559, 0.3333333333333333703, 0.3219752754296894559, 0.3333333333333333703, 0.3219752754296894559, 0.3333333333333333703, 0.3219752754296894559, 0.3333333333333333703, 0.3219752754296894559, 0.3333333333333333703, 0.3219752754296894559, 0.3333333333333333703, 0.3219752754296894559, 0.3333333333333333703, 0.3219752754296894559, 0.3333333333333333703, 0.3219752754296894559, 0.3333333333333333703, 0.3219752754296894559, 0.3333333333333333703, 0.3219752754296894559, 0.3333333333333333703, 0.3219752754296894559, 0.3333333333333333703, 0.3219752754296894559, 0.3333333333333333703, 0.3219752754296894559, 0.3333333333333333703, 0.3219752754296894559, 0.3333333333333333703, 0.3219752754296894559, 0.3333333333333333703, 0.3219752754296894559, 0.3333333333333333703, 0.3219752754296894559, 0.3333333333333333703, 0.3219752754296894559, 0.3333333333333333703, 0.3219752754296894559, 0.3333333333333333703, 0.3219752754296894559, 0.3333333333333333703, 0.3219752754296894559, 0.3333333333333333703, 0.3219752754296894559, 0.3333333333333333703, 0.3219752754296894559, 0.3333333333333333703, 0.3219752754296894559, 0.3333333333333333703, 0.3219752754296894559, 0.3333333333333333703, 0.3219752754296894559, 0.3333333333333333703, 0.3219752754296894559, 0.3333333333333333703, 0.3219752754296894559, 0.3333333333333333703, 0.3219752754296894559, 0.3333333333333333703, 0.3219752754296894559, 0.3333333333333333703, 0.3219752754296894559, 0.3333333333333333703, 0.3219752754296894559, 0.3333333333333333703, 0.3219752754296894559, 0.3333333333333333703, 0.3219752754296894559, 0.3333333333333333703, 0.3219752754296894559, 0.3333333333333333703, 0.3219752754296894559, 0.3333333333333333703, 0.3219752754296894559, 0.3333333333333333703, 0.3219752754296894559, 0.3333333333333333703, 0.3219752754296894559, 0.3333333333333333703, 0.3219752754296894559, 0.3333333333333333703, 0.3219752754296894559, 0.3333333333333333703, 0.3219752754296894559, 0.3333333333333333703, 0.3219752754296894559, 0.3333333333333333703, 0.3219752754296894559, 0.3333333333333333703, 0.3219752754296894559, 0.3333333333333333703, 0.3219752754296894559, 0.3333333333333333703, 0.3219752754296894559, 0.3333333333333333703, 0.3219752754296894559, 0.3333333333333333703, 0.3219752754296894559, 0.3333333333333333703, 0.3219752754296894559, 0.3333333333333333703, 0.3219752754296894559, 0.3333333333333333703, 0.3219752754296894559, 0.3333333333333333703, 0.3219752754296894559, 0.3333333333333333703, 0.3219752754296894559, 0.3333333333333333703, 0.3219752754296894559, 0.3333333333333333703, 0.3219752754296894559, 0.3333333333333333703, 0.3219752754296894559, 0.3333333333333333703, 0.3219752754296894559, 0.3333333333333333703, 0.3219752754296894559, 0.3333333333333333703, 0.3219752754296894559, 0.3333333333333333703, 0.3219752754296894559, 0.3333333333333333703, 0.3219752754296894559, 0.3333333333333333703),
 ( 1.000000000000000000, 0.9659258262890683122, 1.000000000000000000, 0.9659258262890683122, 1.000000000000000000, 0.9659258262890683122, 1.000000000000000000, 0.9659258262890683122, 1.000000000000000000, 0.9659258262890683122, 1.000000000000000000, 0.9659258262890683122, 1.000000000000000000, 0.9659258262890683122, 1.000000000000000000, 0.9659258262890683122, 1.000000000000000000, 0.9659258262890683122, 1.000000000000000000, 0.9659258262890683122, 1.000000000000000000, 0.9659258262890683122, 1.000000000000000000, 0.9659258262890683122, 1.000000000000000000, 0.9659258262890683122, 1.000000000000000000, 0.9659258262890683122, 1.000000000000000000, 0.9659258262890683122, 1.000000000000000000, 0.9659258262890683122, 1.000000000000000000, 0.9659258262890683122, 1.000000000000000000, 0.9659258262890683122, 1.000000000000000000, 0.9659258262890683122, 1.000000000000000000, 0.9659258262890683122, 1.000000000000000000, 0.9659258262890683122, 1.000000000000000000, 0.9659258262890683122, 1.000000000000000000, 0.9659258262890683122, 1.000000000000000000, 0.9659258262890683122, 1.000000000000000000, 0.9659258262890683122, 1.000000000000000000, 0.9659258262890683122, 1.000000000000000000, 0.9659258262890683122, 1.000000000000000000, 0.9659258262890683122, 1.000000000000000000, 0.9659258262890683122, 1.000000000000000000, 0.9659258262890683122, 1.000000000000000000, 0.9659258262890683122, 1.000000000000000000, 0.9659258262890683122, 1.000000000000000000, 0.9659258262890683122, 1.000000000000000000, 0.9659258262890683122, 1.000000000000000000, 0.9659258262890683122, 1.000000000000000000, 0.9659258262890683122, 1.000000000000000000, 0.9659258262890683122, 1.000000000000000000, 0.9659258262890683122, 1.000000000000000000, 0.9659258262890683122, 1.000000000000000000, 0.9659258262890683122, 1.000000000000000000, 0.9659258262890683122, 1.000000000000000000, 0.9659258262890683122, 1.000000000000000000, 0.9659258262890683122, 1.000000000000000000, 0.9659258262890683122, 1.000000000000000000, 0.9659258262890683122, 1.000000000000000000, 0.9659258262890683122, 1.000000000000000000, 0.9659258262890683122, 1.000000000000000000, 0.9659258262890683122, 1.000000000000000000, 0.9659258262890683122, 1.000000000000000000, 0.9659258262890683122, 1.000000000000000000, 0.9659258262890683122, 1.000000000000000000, 0.9659258262890683122, 1.000000000000000000, 0.9659258262890683122, 1.000000000000000000, 0.9659258262890683122, 1.000000000000000000, 0.9659258262890683122, 1.000000000000000000, 0.9659258262890683122, 1.000000000000000000, 0.9659258262890683122, 1.000000000000000000, 0.9659258262890683122, 1.000000000000000000, 0.9659258262890683122, 1.000000000000000000, 0.9659258262890683122, 1.000000000000000000, 0.9659258262890683122, 1.000000000000000000, 0.9659258262890683122, 1.000000000000000000, 0.9659258262890683122, 1.000000000000000000, 0.9659258262890683122, 1.000000000000000000, 0.9659258262890683122, 1.000000000000000000, 0.9659258262890683122, 1.000000000000000000, 0.9659258262890683122, 1.000000000000000000, 0.9659258262890683122, 1.000000000000000000, 0.9659258262890683122, 1.000000000000000000, 0.9659258262890683122, 1.000000000000000000, 0.9659258262890683122, 1.000000000000000000, 0.9659258262890683122, 1.000000000000000000, 0.9659258262890683122, 1.000000000000000000, 0.9659258262890683122, 1.000000000000000000, 0.9659258262890683122, 1.000000000000000000, 0.9659258262890683122, 1.000000000000000000, 0.9659258262890683122, 1.000000000000000000, 0.9659258262890683122, 1.000000000000000000, 0.9659258262890683122, 1.000000000000000000, 0.9659258262890683122, 1.000000000000000000, 0.9659258262890683122, 1.000000000000000000, 0.9659258262890683122, 1.000000000000000000, 0.9659258262890683122, 1.000000000000000000, 0.9659258262890683122, 1.000000000000000000, 0.9659258262890683122, 1.000000000000000000, 0.9659258262890683122, 1.000000000000000000, 0.9659258262890683122, 1.000000000000000000, 0.9659258262890683122, 1.000000000000000000, 0.9659258262890683122, 1.000000000000000000, 0.9659258262890683122, 1.000000000000000000, 0.9659258262890683122, 1.000000000000000000, 0.9659258262890683122, 1.000000000000000000, 0.9659258262890683122, 1.000000000000000000, 0.9659258262890683122, 1.000000000000000000, 0.9659258262890683122, 1.000000000000000000, 0.9659258262890683122, 1.000000000000000000, 0.9659258262890683122, 1.000000000000000000, 0.9659258262890683122, 1.000000000000000000, 0.9659258262890683122, 1.000000000000000000, 0.9659258262890683122, 1.000000000000000000, 0.9659258262890683122, 1.000000000000000000, 0.9659258262890683122, 1.000000000000000000, 0.9659258262890683122, 1.000000000000000000, 0.9659258262890683122, 1.000000000000000000, 0.9659258262890683122, 1.000000000000000000, 0.9659258262890683122, 1.000000000000000000, 0.9659258262890683122, 1.000000000000000000, 0.9659258262890683122, 1.000000000000000000, 0.9659258262890683122, 1.000000000000000000, 0.9659258262890683122, 1.000000000000000000, 0.9659258262890683122, 1.000000000000000000, 0.9659258262890683122, 1.000000000000000000, 0.9659258262890683122, 1.000000000000000000, 0.9659258262890683122, 1.000000000000000000, 0.9659258262890683122, 1.000000000000000000, 0.9659258262890683122, 1.000000000000000000, 0.9659258262890683122, 1.000000000000000000, 0.9659258262890683122, 1.000000000000000000, 0.9659258262890683122, 1.000000000000000000, 0.9659258262890683122, 1.000000000000000000, 0.9659258262890683122, 1.000000000000000000, 0.9659258262890683122, 1.000000000000000000, 0.9659258262890683122, 1.000000000000000000, 0.9659258262890683122, 1.000000000000000000, 0.9659258262890683122, 1.000000000000000000, 0.9659258262890683122, 1.000000000000000000, 0.9659258262890683122, 1.000000000000000000, 0.9659258262890683122, 1.000000000000000000, 0.9659258262890683122, 1.000000000000000000, 0.9659258262890683122, 1.000000000000000000, 0.9659258262890683122, 1.000000000000000000, 0.9659258262890683122, 1.000000000000000000, 0.9659258262890683122, 1.000000000000000000, 0.9659258262890683122, 1.000000000000000000, 0.9659258262890683122, 1.000000000000000000, 0.9659258262890683122, 1.000000000000000000, 0.9659258262890683122, 1.000000000000000000, 0.9659258262890683122, 1.000000000000000000, 0.9659258262890683122, 1.000000000000000000, 0.9659258262890683122, 1.000000000000000000, 0.9659258262890683122, 1.000000000000000000, 0.9659258262890683122, 1.000000000000000000, 0.9659258262890683122, 1.000000000000000000, 0.9659258262890683122, 1.000000000000000000, 0.9659258262890683122, 1.000000000000000000, 0.9659258262890683122, 1.000000000000000000, 0.9659258262890683122, 1.000000000000000000, 0.9659258262890683122, 1.000000000000000000, 0.9659258262890683122, 1.000000000000000000, 0.9659258262890683122, 1.000000000000000000, 0.9659258262890683122, 1.000000000000000000, 0.9659258262890683122, 1.000000000000000000, 0.9659258262890683122, 1.000000000000000000, 0.9659258262890683122, 1.000000000000000000, 0.9659258262890683122, 1.000000000000000000, 0.9659258262890683122, 1.000000000000000000, 0.9659258262890683122, 1.000000000000000000, 0.9659258262890683122, 1.000000000000000000, 0.9659258262890683122, 1.000000000000000000, 0.9659258262890683122, 1.000000000000000000, 0.9659258262890683122, 1.000000000000000000, 0.9659258262890683122, 1.000000000000000000, 0.9659258262890683122, 1.000000000000000000, 0.9659258262890683122, 1.000000000000000000, 0.9659258262890683122, 1.000000000000000000, 0.9659258262890683122, 1.000000000000000000, 0.9659258262890683122, 1.000000000000000000, 0.9659258262890683122, 1.000000000000000000, 0.9659258262890683122, 1.000000000000000000, 0.9659258262890683122, 1.000000000000000000, 0.9659258262890683122, 1.000000000000000000, 0.9659258262890683122, 1.000000000000000000, 0.9659258262890683122, 1.000000000000000000, 0.9659258262890683122, 1.000000000000000000, 0.9659258262890683122, 1.000000000000000000, 0.9659258262890683122, 1.000000000000000000, 0.9659258262890683122, 1.000000000000000000, 0.9659258262890683122, 1.000000000000000000, 0.9659258262890683122, 1.000000000000000000, 0.9659258262890683122, 1.000000000000000000, 0.9659258262890683122, 1.000000000000000000, 0.9659258262890683122, 1.000000000000000000, 0.9659258262890683122, 1.000000000000000000, 0.9659258262890683122, 1.000000000000000000, 0.9659258262890683122, 1.000000000000000000, 0.9659258262890683122, 1.000000000000000000, 0.9659258262890683122, 1.000000000000000000, 0.9659258262890683122, 1.000000000000000000, 0.9659258262890683122, 1.000000000000000000, 0.9659258262890683122, 1.000000000000000000, 0.9659258262890683122, 1.000000000000000000, 0.9659258262890683122, 1.000000000000000000, 0.9659258262890683122, 1.000000000000000000, 0.9659258262890683122, 1.000000000000000000, 0.9659258262890683122, 1.000000000000000000, 0.9659258262890683122, 1.000000000000000000, 0.9659258262890683122, 1.000000000000000000, 0.9659258262890683122, 1.000000000000000000, 0.9659258262890683122, 1.000000000000000000, 0.9659258262890683122, 1.000000000000000000, 0.9659258262890683122, 1.000000000000000000, 0.9659258262890683122, 1.000000000000000000, 0.9659258262890683122, 1.000000000000000000, 0.9659258262890683122, 1.000000000000000000, 0.9659258262890683122, 1.000000000000000000, 0.9659258262890683122, 1.000000000000000000, 0.9659258262890683122, 1.000000000000000000, 0.9659258262890683122, 1.000000000000000000, 0.9659258262890683122, 1.000000000000000000, 0.9659258262890683122, 1.000000000000000000, 0.9659258262890683122, 1.000000000000000000, 0.9659258262890683122, 1.000000000000000000, 0.9659258262890683122, 1.000000000000000000, 0.9659258262890683122, 1.000000000000000000, 0.9659258262890683122, 1.000000000000000000, 0.9659258262890683122, 1.000000000000000000, 0.9659258262890683122, 1.000000000000000000, 0.9659258262890683122, 1.000000000000000000, 0.9659258262890683122, 1.000000000000000000, 0.9659258262890683122, 1.000000000000000000, 0.9659258262890683122, 1.000000000000000000, 0.9659258262890683122, 1.000000000000000000, 0.9659258262890683122, 1.000000000000000000, 0.9659258262890683122, 1.000000000000000000, 0.9659258262890683122, 1.000000000000000000, 0.9659258262890683122, 1.000000000000000000, 0.9659258262890683122, 1.000000000000000000, 0.9659258262890683122, 1.000000000000000000) ) ) 
 REPRESENTATION_ITEM ( '' )  SURFACE ( )  );
#39063=CARTESIAN_POINT ( 'NONE',  ( 16.51473224551083163, -9.474510206698727899, 95.83442372801900433 ) ) ;
#39064=CARTESIAN_POINT ( 'NONE',  ( 16.51473224551069308, 9.474510206698969483, 44.16557627198103120 ) ) ;
#39065=CARTESIAN_POINT ( 'NONE',  ( -13.89961937509977652, 13.97604488694528158, 75.62390960531438111 ) ) ;
#39066=CARTESIAN_POINT ( 'NONE',  ( 16.55341960407611168, 4.379528057220329451, 98.95724293864770971 ) ) ;
#39067=CARTESIAN_POINT ( 'NONE',  ( 19.02544592524343514, -5.153800228976328945, 98.54057627198100988 ) ) ;
#39068=CARTESIAN_POINT ( 'NONE',  ( -4.379528057220328563, 16.55341960407611168, 90.20724293864770971 ) ) ;
#39069=CARTESIAN_POINT ( 'NONE',  ( 13.97604488694527802, 13.89961937509977652, 94.37390960531436690 ) ) ;
#39070=CARTESIAN_POINT ( 'NONE',  ( -12.14591786802309592, -12.06949235617757132, 41.87390960531435979 ) ) ;
#39071=CARTESIAN_POINT ( 'NONE',  ( -5.049401038298153566, 19.05341960407611168, 40.20724293864768839 ) ) ;
#39072=ORIENTED_EDGE ( 'NONE', *, *, #12002, .F. ) ;
#39073=CARTESIAN_POINT ( 'NONE',  ( 21.53943276465977519, 0.05219959533937863772, 51.25109039468568994 ) ) ;
#39074=CARTESIAN_POINT ( 'NONE',  ( 9.564922557961047289, -16.46253265017146816, 80.41775706135234714 ) ) ;
#39075=CARTESIAN_POINT ( 'NONE',  ( 14.29746914071049879, -8.314922557960816363, 48.33224293864770260 ) ) ;
#39076=CARTESIAN_POINT ( 'NONE',  ( -15.80617190586745835, -15.72974639402198527, 101.8739096053143811 ) ) ;
#39077=CARTESIAN_POINT ( 'NONE',  ( 15.72974639402199770, -15.80617190586745480, 53.12390960531436690 ) ) ;
#39078=CARTESIAN_POINT ( 'NONE',  ( 19.49190055781010500, 5.500000000000047962, 73.06116087098777712 ) ) ;
#39079=CARTESIAN_POINT ( 'NONE',  ( -4.483927247898539470, -16.52544592524342804, 82.29057627198103830 ) ) ;
#39080=CARTESIAN_POINT ( 'NONE',  ( -5.153800228976328057, -19.02544592524343514, 57.29057627198103120 ) ) ;
#39081=CARTESIAN_POINT ( 'NONE',  ( -0.05219959533910754901, -16.53943276465976808, 27.49890960531435269 ) ) ;
#39082=CARTESIAN_POINT ( 'NONE',  ( 4.379528057220092307, 16.55341960407617563, 107.2927570613523471 ) ) ;
#39083=CARTESIAN_POINT ( 'NONE',  ( -16.53943276465976808, -0.05219959533934237506, 68.75109039468568994 ) ) ;
#39084=CARTESIAN_POINT ( 'NONE',  ( 9.474510206698729675, 16.51473224551082808, 27.08442372801900433 ) ) ;
#39086=CARTESIAN_POINT ( 'NONE',  ( 13.97604488694527802, 13.89961937509977652, 109.3739096053143669 ) ) ;
#39087=CARTESIAN_POINT ( 'NONE',  ( -5.153800228976328057, -19.02544592524343514, 82.29057627198103830 ) ) ;
#39088=CARTESIAN_POINT ( 'NONE',  ( -19.02544592524342804, 5.153800228976336051, 41.04057627198103120 ) ) ;
#39089=CARTESIAN_POINT ( 'NONE',  ( 4.379528057220339221, -16.55341960407611168, 42.70724293864770260 ) ) ;
#39090=CARTESIAN_POINT ( 'NONE',  ( -9.564922557960796823, -16.46253265017161027, 112.0822429386476955 ) ) ;
#39091=CARTESIAN_POINT ( 'NONE',  ( -13.89961937509977652, 13.97604488694528158, 100.6239096053143669 ) ) ;
#39092=CARTESIAN_POINT ( 'NONE',  ( -21.55341960407610458, -5.719274019375992779, 41.45724293864769550 ) ) ;
#39093=CARTESIAN_POINT ( 'NONE',  ( -0.05219959533910754901, -16.53943276465976808, 82.49890960531436690 ) ) ;
#39094=CARTESIAN_POINT ( 'NONE',  ( -4.379528057220086978, -16.55341960407618274, 39.79275706135235424 ) ) ;
#39095=CARTESIAN_POINT ( 'NONE',  ( 0.05219959533910956823, 16.53943276465976808, 64.99890960531435269 ) ) ;
#39097=CARTESIAN_POINT ( 'NONE',  ( 19.02544592524334988, 5.153800228976608722, 66.45942372801899012 ) ) ;
#39098=CARTESIAN_POINT ( 'NONE',  ( -13.97604488694527625, -13.89961937509977652, 101.8739096053143811 ) ) ;
#39099=CARTESIAN_POINT ( 'NONE',  ( -19.05341960407617563, 5.049401038297882671, 73.54275706135233293 ) ) ;
#39101=CARTESIAN_POINT ( 'NONE',  ( -16.46253265017146816, -9.564922557961047289, 109.1677570613523471 ) ) ;
#39102=CARTESIAN_POINT ( 'NONE',  ( -0.05219959533934338120, 16.53943276465976808, 112.5010903946857042 ) ) ;
#39103=CARTESIAN_POINT ( 'NONE',  ( -9.564922557961040184, 16.46253265017147172, 67.91775706135233293 ) ) ;
#39104=CARTESIAN_POINT ( 'NONE',  ( 5.823673210054125526, 21.52544592524343514, 29.79057627198102409 ) ) ;
#39105=CARTESIAN_POINT ( 'NONE',  ( 5.823673210054444382, -21.52544592524334988, 70.20942372801904696 ) ) ;
#39107=CARTESIAN_POINT ( 'NONE',  ( -0.05219959533934338120, 16.53943276465976808, 27.50109039468567929 ) ) ;
#39108=CARTESIAN_POINT ( 'NONE',  ( 18.22780087662122384, -5.500000000000022204, 56.01540105326107977 ) ) ;
#39109=CARTESIAN_POINT ( 'NONE',  ( 0.05219959533909260263, 19.03943276465977164, 69.99890960531435269 ) ) ;
#39111=CARTESIAN_POINT ( 'NONE',  ( 12.14591786802309770, 12.06949235617756955, 89.37390960531435269 ) ) ;
#39112=CARTESIAN_POINT ( 'NONE',  ( -16.46253265017160317, 9.564922557960807481, 70.83224293864770971 ) ) ;
#39113=CARTESIAN_POINT ( 'NONE',  ( 16.46253265017160672, -9.564922557960803928, 88.33224293864769550 ) ) ;
#39114=CARTESIAN_POINT ( 'NONE',  ( 0.05219959533936267826, -19.03943276465977164, 95.00109039468567573 ) ) ;
#39115=CARTESIAN_POINT ( 'NONE',  ( 10.81492255796078972, 18.62759615963270932, 74.58224293864768129 ) ) ;
#39116=CARTESIAN_POINT ( 'NONE',  ( 0.05219959533909260263, 19.03943276465977164, 24.99890960531435269 ) ) ;
#39117=CARTESIAN_POINT ( 'NONE',  ( -16.51473224551082808, 9.474510206698731452, 58.33442372801900433 ) ) ;
#39118=CARTESIAN_POINT ( 'NONE',  ( 16.51473224551069308, 9.474510206698969483, 54.16557627198103120 ) ) ;
#39119=CARTESIAN_POINT ( 'NONE',  ( 19.02544592524343514, -5.153800228976328945, 88.54057627198102409 ) ) ;
#39122=CARTESIAN_POINT ( 'NONE',  ( -5.719274019375978568, 21.55341960407610458, 105.2072429386477097 ) ) ;
#39123=CARTESIAN_POINT ( 'NONE',  ( 4.379528057220339221, -16.55341960407611168, 87.70724293864769550 ) ) ;
#39124=CARTESIAN_POINT ( 'NONE',  ( 19.02544592524343514, -5.153800228976328945, 83.54057627198100988 ) ) ;
#39125=CARTESIAN_POINT ( 'NONE',  ( -5.049401038297874678, -19.05341960407617918, 59.79275706135231871 ) ) ;
#39126=CARTESIAN_POINT ( 'NONE',  ( -18.67979575497178146, -10.72451020669898902, 86.66557627198102409 ) ) ;
#39127=CARTESIAN_POINT ( 'NONE',  ( 15.72974639402199770, -15.80617190586745480, 73.12390960531436690 ) ) ;
#39128=CARTESIAN_POINT ( 'NONE',  ( -0.05219959533910754901, -16.53943276465976808, 32.49890960531435979 ) ) ;
#39129=CARTESIAN_POINT ( 'NONE',  ( -10.72451020669870658, -18.67979575497194134, 104.5844237280190185 ) ) ;
#39130=CARTESIAN_POINT ( 'NONE',  ( -8.314922557961024197, 14.29746914071037800, 62.91775706135236135 ) ) ;
#39131=CARTESIAN_POINT ( 'NONE',  ( -5.049401038298153566, 19.05341960407611168, 95.20724293864770971 ) ) ;
#39132=CARTESIAN_POINT ( 'NONE',  ( 13.97604488694527802, 13.89961937509977652, 29.37390960531435979 ) ) ;
#39133=CARTESIAN_POINT ( 'NONE',  ( 15.80617190586769283, -15.72974639402175789, 40.62609039468567573 ) ) ;
#39134=CARTESIAN_POINT ( 'NONE',  ( -10.72451020669870658, -18.67979575497194134, 49.58442372801901143 ) ) ;
#39135=CARTESIAN_POINT ( 'NONE',  ( -0.05219959533909027116, -19.03943276465977164, 57.49890960531435979 ) ) ;
#39136=CARTESIAN_POINT ( 'NONE',  ( 18.67979575497194134, -10.72451020669871369, 35.83442372801901143 ) ) ;
#39137=CARTESIAN_POINT ( 'NONE',  ( 9.564922557961047289, -16.46253265017146816, 75.41775706135234714 ) ) ;
#39138=CARTESIAN_POINT ( 'NONE',  ( 13.89961937509957401, 13.97604488694547697, 71.87609039468567573 ) ) ;
#39139=CARTESIAN_POINT ( 'NONE',  ( 19.03943276465977164, -0.05219959533909143690, 43.74890960531435979 ) ) ;
#39140=CARTESIAN_POINT ( 'NONE',  ( 16.52544592524335698, 4.483927247898782831, 71.45942372801901854 ) ) ;
#39141=CARTESIAN_POINT ( 'NONE',  ( 9.474510206698971260, -16.51473224551069308, 52.91557627198102409 ) ) ;
#39143=CARTESIAN_POINT ( 'NONE',  ( -16.51473224551069308, -9.474510206698971260, 101.6655762719810241 ) ) ;
#39144=CARTESIAN_POINT ( 'NONE',  ( -9.474510206698964154, 16.51473224551069663, 40.41557627198103120 ) ) ;
#39145=CARTESIAN_POINT ( 'NONE',  ( -10.81492255796078084, -18.62759615963271287, 77.08224293864769550 ) ) ;
#39146=CARTESIAN_POINT ( 'NONE',  ( 8.224510206698742110, 14.34966873604972548, 67.08442372801901854 ) ) ;
#39147=CARTESIAN_POINT ( 'NONE',  ( -5.823673210054431948, 21.52544592524334988, 112.7094237280190328 ) ) ;
#39148=CARTESIAN_POINT ( 'NONE',  ( -5.049401038298153566, 19.05341960407611168, 50.20724293864770260 ) ) ;
#39149=CARTESIAN_POINT ( 'NONE',  ( 0.05219959533910956823, 16.53943276465976808, 39.99890960531436690 ) ) ;
#39150=CARTESIAN_POINT ( 'NONE',  ( -14.34966873604960291, -8.224510206698953496, 86.66557627198102409 ) ) ;
#39151=CARTESIAN_POINT ( 'NONE',  ( 19.05341960407611168, 5.049401038298154454, 83.95724293864766707 ) ) ;
#39152=CARTESIAN_POINT ( 'NONE',  ( 0.05219959533937995610, -21.53943276465977519, 35.00109039468568284 ) ) ;
#39153=CARTESIAN_POINT ( 'NONE',  ( 13.89961937509977652, -13.97604488694527269, 88.12390960531438111 ) ) ;
#39154=CARTESIAN_POINT ( 'NONE',  ( 21.55341960407619695, -5.719274019375665929, 101.0427570613523756 ) ) ;
#39155=CARTESIAN_POINT ( 'NONE',  ( -14.34966873604972548, 8.224510206698743886, 68.33442372801900433 ) ) ;
#39156=CARTESIAN_POINT ( 'NONE',  ( -16.51473224551069308, -9.474510206698971260, 111.6655762719810383 ) ) ;
#39157=CARTESIAN_POINT ( 'NONE',  ( 15.72974639402199770, -15.80617190586745480, 88.12390960531436690 ) ) ;
#39158=CARTESIAN_POINT ( 'NONE',  ( 12.14591786802309770, 12.06949235617756955, 49.37390960531436690 ) ) ;
#39159=CARTESIAN_POINT ( 'NONE',  ( 16.46253265017160672, -9.564922557960803928, 38.33224293864768839 ) ) ;
#39160=CARTESIAN_POINT ( 'NONE',  ( 16.53943276465976808, -0.05219959533910856209, 63.74890960531435979 ) ) ;
#39161=CARTESIAN_POINT ( 'NONE',  ( -5.719274019375978568, 21.55341960407610458, 35.20724293864768839 ) ) ;
#39162=CARTESIAN_POINT ( 'NONE',  ( -21.52544592524343514, 5.823673210054127303, 26.04057627198103475 ) ) ;
#39163=CARTESIAN_POINT ( 'NONE',  ( -19.03943276465977164, -0.05219959533935918106, 33.75109039468566863 ) ) ;
#39164=CARTESIAN_POINT ( 'NONE',  ( 0.05219959533910956823, 16.53943276465976808, 104.9989096053143669 ) ) ;
#39165=CARTESIAN_POINT ( 'NONE',  ( 16.46253265017160672, -9.564922557960803928, 103.3322429386476955 ) ) ;
#39166=ORIENTED_EDGE ( 'NONE', *, *, #46412, .T. ) ;
#39167=CARTESIAN_POINT ( 'NONE',  ( 0.05219959533934541429, -16.53943276465976808, 55.00109039468568284 ) ) ;
#39168=CARTESIAN_POINT ( 'NONE',  ( -13.89961937509977652, 13.97604488694528158, 60.62390960531436690 ) ) ;
#39170=CARTESIAN_POINT ( 'NONE',  ( -9.564922557961040184, 16.46253265017147172, 57.91775706135233293 ) ) ;
#39171=CARTESIAN_POINT ( 'NONE',  ( -4.379528057220086978, -16.55341960407618274, 94.79275706135234714 ) ) ;
#39172=CARTESIAN_POINT ( 'NONE',  ( 5.049401038297881783, 19.05341960407617563, 92.29275706135234714 ) ) ;
#39173=CARTESIAN_POINT ( 'NONE',  ( -15.80617190586768217, 15.72974639402176855, 63.12609039468568994 ) ) ;
#39174=CARTESIAN_POINT ( 'NONE',  ( -19.05341960407611168, -5.049401038298163336, 71.45724293864766707 ) ) ;
#39175=CARTESIAN_POINT ( 'NONE',  ( 21.52544592524344225, -5.823673210054117533, 93.54057627198103830 ) ) ;
#39176=CARTESIAN_POINT ( 'NONE',  ( -12.06949235617756955, 12.14591786802309770, 110.6239096053143669 ) ) ;
#39177=B_SPLINE_CURVE_WITH_KNOTS ( 'NONE', 3,
 ( #126545, #127542, #96208, #157897, #19386, #81035, #129523, #190224, #191223, #142711, #97187, #5186, #189243, #84026, #82010, #66867, #128530, #36522, #21370, #114361, #68870, #195231 ),
 .UNSPECIFIED., .F., .F.,
 ( 4, 2, 2, 2, 2, 2, 2, 2, 2, 2, 4 ),
 ( 5.204170427930421283E-18, 0.001309639967555401930, 0.001964459951333100401, 0.002291869943221949528, 0.002455574939166360864, 0.002619279935110772201, 0.002782984931055183537, 0.002946689926999595741, 0.003274099918888392392, 0.003928919902666009115, 0.005238559870221241692 ),
 .UNSPECIFIED. ) ;
#39178=CARTESIAN_POINT ( 'NONE',  ( -19.05341960407617563, 5.049401038297882671, 83.54275706135233293 ) ) ;
#39179=CARTESIAN_POINT ( 'NONE',  ( -21.53943276465977519, 0.05219959533907696930, 71.24890960531435269 ) ) ;
#39180=CARTESIAN_POINT ( 'NONE',  ( -0.05219959533936034679, 19.03943276465977164, 47.50109039468566863 ) ) ;
#39181=CARTESIAN_POINT ( 'NONE',  ( 19.53091890409952569, 5.499999999999982236, 97.56097431831416600 ) ) ;
#39182=CARTESIAN_POINT ( 'NONE',  ( -5.823673210054116645, -21.52544592524344225, 87.29057627198103830 ) ) ;
#39183=CARTESIAN_POINT ( 'NONE',  ( 17.49999999999999645, 5.500000000000000888, 28.78230962303566542 ) ) ;
#39184=CARTESIAN_POINT ( 'NONE',  ( -13.97604488694527625, -13.89961937509977652, 61.87390960531435979 ) ) ;
#39185=DIRECTION ( 'NONE',  ( 0.000000000000000000, 0.000000000000000000, 1.000000000000000000 ) ) ;
#39186=CARTESIAN_POINT ( 'NONE',  ( 8.314922557961029526, -14.29746914071037800, 20.41775706135234714 ) ) ;
#39188=CARTESIAN_POINT ( 'NONE',  ( -0.05219959533909027116, -19.03943276465977164, 42.49890960531435269 ) ) ;
#39189=CARTESIAN_POINT ( 'NONE',  ( 18.67979575497178502, 10.72451020669898547, 109.1655762719810383 ) ) ;
#39190=CARTESIAN_POINT ( 'NONE',  ( -16.53943276465976808, 0.05219959533911058130, 51.24890960531436690 ) ) ;
#39191=B_SPLINE_CURVE_WITH_KNOTS ( 'NONE', 3,
 ( #77738, #91893, #46410, #47418, #170753, #93900, #169753, #166795, #153584, #122247, #43440, #107075, #139404, #155578, #58600, #89936, #120266, #183937, #181958, #45422 ),
 .UNSPECIFIED., .F., .F.,
 ( 4, 2, 2, 2, 2, 2, 2, 2, 2, 4 ),
 ( 0.000000000000000000, 0.0004987090165372690164, 0.0009974180330745380327, 0.001246772541343168800, 0.001496127049611799568, 0.001994836066149061320, 0.002493545082686322422, 0.002742899590954955575, 0.002992254099223587861, 0.003989672132298133916 ),
 .UNSPECIFIED. ) ;
#39192=CARTESIAN_POINT ( 'NONE',  ( -5.049401038298153566, 19.05341960407611168, 60.20724293864768129 ) ) ;
#39193=CARTESIAN_POINT ( 'NONE',  ( 15.80617190586769283, -15.72974639402175789, 80.62609039468567573 ) ) ;
#39194=CARTESIAN_POINT ( 'NONE',  ( -14.34966873604972548, 8.224510206698743886, 23.33442372801901499 ) ) ;
#39195=CARTESIAN_POINT ( 'NONE',  ( 19.03943276465977164, 0.05219959533936151252, 26.25109039468566507 ) ) ;
#39196=CARTESIAN_POINT ( 'NONE',  ( 12.14591786802309770, 12.06949235617756955, 24.37390960531435979 ) ) ;
#39197=CARTESIAN_POINT ( 'NONE',  ( -21.52544592524334988, -5.823673210054445271, 33.95942372801901143 ) ) ;
#39198=CARTESIAN_POINT ( 'NONE',  ( -5.719274019375978568, 21.55341960407610458, 115.2072429386476955 ) ) ;
#39199=CARTESIAN_POINT ( 'NONE',  ( 15.72974639402199770, -15.80617190586745480, 58.12390960531435979 ) ) ;
#39200=CARTESIAN_POINT ( 'NONE',  ( -9.474510206698720793, -16.51473224551083518, 94.58442372801900433 ) ) ;
#39201=CARTESIAN_POINT ( 'NONE',  ( -16.46253265017146816, -9.564922557961047289, 69.16775706135233293 ) ) ;
#39202=CARTESIAN_POINT ( 'NONE',  ( 18.67979575497194134, -10.72451020669871369, 75.83442372801900433 ) ) ;
#39203=CARTESIAN_POINT ( 'NONE',  ( 9.564922557961047289, -16.46253265017146816, 50.41775706135233293 ) ) ;
#39204=CARTESIAN_POINT ( 'NONE',  ( -4.379528057220328563, 16.55341960407611168, 115.2072429386476955 ) ) ;
#39205=CARTESIAN_POINT ( 'NONE',  ( -18.62759615963270932, 10.81492255796079327, 45.83224293864769550 ) ) ;
#39206=CARTESIAN_POINT ( 'NONE',  ( -4.379528057220328563, 16.55341960407611168, 50.20724293864769550 ) ) ;
#39207=CARTESIAN_POINT ( 'NONE',  ( -19.52837319214026479, 5.499999999999997335, 94.60471352585537375 ) ) ;
#39208=CARTESIAN_POINT ( 'NONE',  ( -15.72974639402176322, -15.80617190586768395, 109.3760903946857042 ) ) ;
#39209=CARTESIAN_POINT ( 'NONE',  ( 4.483927247898790824, -16.52544592524335698, 90.20942372801903275 ) ) ;
#39210=CARTESIAN_POINT ( 'NONE',  ( 12.06949235617757843, -12.14591786802309237, 43.12390960531435269 ) ) ;
#39211=CARTESIAN_POINT ( 'NONE',  ( 5.719274019375673035, 21.55341960407619339, 77.29275706135234714 ) ) ;
#39212=CARTESIAN_POINT ( 'NONE',  ( -15.72974639402176322, -15.80617190586768395, 74.37609039468568994 ) ) ;
#39213=CARTESIAN_POINT ( 'NONE',  ( -18.67979575497178146, -10.72451020669898902, 86.66557627198102409 ) ) ;
#39214=CARTESIAN_POINT ( 'NONE',  ( 13.89961937509977652, -13.97604488694527269, 33.12390960531434558 ) ) ;
#39215=CARTESIAN_POINT ( 'NONE',  ( 15.80617190586769283, -15.72974639402175789, 60.62609039468567573 ) ) ;
#39216=CARTESIAN_POINT ( 'NONE',  ( -0.05219959533909027116, -19.03943276465977164, 37.49890960531436690 ) ) ;
#39217=CARTESIAN_POINT ( 'NONE',  ( -19.02544592524342804, 5.153800228976336051, 51.04057627198103120 ) ) ;
#39218=CARTESIAN_POINT ( 'NONE',  ( -8.314922557960811034, -14.29746914071050412, 87.08224293864769550 ) ) ;
#39219=CARTESIAN_POINT ( 'NONE',  ( -0.05219959533909027116, -19.03943276465977164, 102.4989096053143669 ) ) ;
#39220=CARTESIAN_POINT ( 'NONE',  ( 16.53943276465976808, -0.05219959533910856209, 38.74890960531435979 ) ) ;
#39221=CARTESIAN_POINT ( 'NONE',  ( -16.53943276465976808, 0.05219959533911058130, 116.2489096053143669 ) ) ;
#39222=CARTESIAN_POINT ( 'NONE',  ( 5.719274019375991003, -21.55341960407610458, 77.70724293864770971 ) ) ;
#39223=CARTESIAN_POINT ( 'NONE',  ( -21.53943276465977519, -0.05219959533937600094, 18.75109039468568639 ) ) ;
#39225=CARTESIAN_POINT ( 'NONE',  ( -4.483927247898782831, 16.52544592524335698, 27.70942372801901854 ) ) ;
#39226=CARTESIAN_POINT ( 'NONE',  ( 15.80617190586746368, 15.72974639402197994, 69.37390960531436690 ) ) ;
#39227=CARTESIAN_POINT ( 'NONE',  ( 21.52544592524334988, 5.823673210054432836, 101.4594237280190185 ) ) ;
#39228=CARTESIAN_POINT ( 'NONE',  ( 0.05219959533909260263, 19.03943276465977164, 84.99890960531436690 ) ) ;
#39229=CARTESIAN_POINT ( 'NONE',  ( -21.55341960407619339, 5.719274019375674811, 33.54275706135234714 ) ) ;
#39230=CARTESIAN_POINT ( 'NONE',  ( 0.05219959533909260263, 19.03943276465977164, 109.9989096053143669 ) ) ;
#39231=CARTESIAN_POINT ( 'NONE',  ( -16.53943276465976808, -0.05219959533934237506, 93.75109039468567573 ) ) ;
#39232=CARTESIAN_POINT ( 'NONE',  ( 21.53943276465977519, 0.05219959533937863772, 76.25109039468568994 ) ) ;
#39233=CARTESIAN_POINT ( 'NONE',  ( 9.564922557961047289, -16.46253265017146816, 20.41775706135233293 ) ) ;
#39234=CARTESIAN_POINT ( 'NONE',  ( 16.52544592524335698, 4.483927247898782831, 81.45942372801900433 ) ) ;
#39235=CARTESIAN_POINT ( 'NONE',  ( -10.72451020669870658, -18.67979575497194134, 24.58442372801901499 ) ) ;
#39236=CARTESIAN_POINT ( 'NONE',  ( 16.46253265017160672, -9.564922557960803928, 38.33224293864768839 ) ) ;
#39237=CARTESIAN_POINT ( 'NONE',  ( -5.823673210054431948, 21.52544592524334988, 92.70942372801901854 ) ) ;
#39238=CARTESIAN_POINT ( 'NONE',  ( 19.02544592524343514, -5.153800228976328945, 88.54057627198102409 ) ) ;
#39239=CARTESIAN_POINT ( 'NONE',  ( -10.72451020669898014, 18.67979575497178502, 90.41557627198103830 ) ) ;
#39240=CARTESIAN_POINT ( 'NONE',  ( -13.89961937509957401, -13.97604488694547875, 54.37609039468565442 ) ) ;
#39242=CARTESIAN_POINT ( 'NONE',  ( 15.80617190586746368, 15.72974639402197994, 49.37390960531436690 ) ) ;
#39243=CARTESIAN_POINT ( 'NONE',  ( -9.564922557960796823, -16.46253265017161027, 92.08224293864769550 ) ) ;
#39244=CARTESIAN_POINT ( 'NONE',  ( 8.224510206698953496, -14.34966873604960469, 47.91557627198102409 ) ) ;
#39246=CARTESIAN_POINT ( 'NONE',  ( -19.05341960407617563, 5.049401038297882671, 73.54275706135233293 ) ) ;
#39247=CARTESIAN_POINT ( 'NONE',  ( -17.31728774477273447, 6.344390552232379576, 105.8190665168932014 ) ) ;
#39248=CARTESIAN_POINT ( 'NONE',  ( -16.46253265017146816, -9.564922557961047289, 104.1677570613523329 ) ) ;
#39249=CARTESIAN_POINT ( 'NONE',  ( 15.80617190586746368, 15.72974639402197994, 79.37390960531436690 ) ) ;
#39250=CARTESIAN_POINT ( 'NONE',  ( 0.05219959533910956823, 16.53943276465976808, 69.99890960531435269 ) ) ;
#39251=CARTESIAN_POINT ( 'NONE',  ( -19.02544592524342804, 5.153800228976336051, 96.04057627198103830 ) ) ;
#39252=CARTESIAN_POINT ( 'NONE',  ( 14.34966873604972726, -8.224510206698740333, 45.83442372801901854 ) ) ;
#39253=CARTESIAN_POINT ( 'NONE',  ( -16.46253265017160317, 9.564922557960807481, 60.83224293864769550 ) ) ;
#39254=CARTESIAN_POINT ( 'NONE',  ( 21.55341960407619695, -5.719274019375665929, 26.04275706135235779 ) ) ;
#39255=CARTESIAN_POINT ( 'NONE',  ( 9.474510206698729675, 16.51473224551082808, 97.08442372801900433 ) ) ;
#39256=CARTESIAN_POINT ( 'NONE',  ( -5.153800228976328057, -19.02544592524343514, 92.29057627198099567 ) ) ;
#39257=CARTESIAN_POINT ( 'NONE',  ( -19.02544592524342804, 5.153800228976336051, 76.04057627198102409 ) ) ;
#39258=CARTESIAN_POINT ( 'NONE',  ( -15.80617190586745835, -15.72974639402198527, 71.87390960531438111 ) ) ;
#39259=CARTESIAN_POINT ( 'NONE',  ( 5.153800228976335163, 19.02544592524342804, 44.79057627198103830 ) ) ;
#39261=CARTESIAN_POINT ( 'NONE',  ( -16.55341960407611168, -4.379528057220339221, 51.45724293864770260 ) ) ;
#39262=CARTESIAN_POINT ( 'NONE',  ( 0.05219959533909260263, 19.03943276465977164, 99.99890960531436690 ) ) ;
#39264=CARTESIAN_POINT ( 'NONE',  ( -9.564922557961040184, 16.46253265017147172, 67.91775706135233293 ) ) ;
#39265=CARTESIAN_POINT ( 'NONE',  ( 0.05219959533907565091, 21.53943276465977519, 94.99890960531436690 ) ) ;
#39266=CARTESIAN_POINT ( 'NONE',  ( 13.89961937509957401, 13.97604488694547697, 46.87609039468565442 ) ) ;
#39267=CARTESIAN_POINT ( 'NONE',  ( -19.02544592524342804, 5.153800228976336051, 96.04057627198103830 ) ) ;
#39268=CARTESIAN_POINT ( 'NONE',  ( 18.89770734986043621, 5.500000000000079936, 66.60214472496636517 ) ) ;
#39269=CARTESIAN_POINT ( 'NONE',  ( -18.67979575497178146, -10.72451020669898902, 41.66557627198103120 ) ) ;
#39270=CARTESIAN_POINT ( 'NONE',  ( 9.474510206698971260, -16.51473224551069308, 82.91557627198103830 ) ) ;
#39271=CARTESIAN_POINT ( 'NONE',  ( -21.52544592524334988, -5.823673210054445271, 68.95942372801901854 ) ) ;
#39272=CARTESIAN_POINT ( 'NONE',  ( -13.89961937509977652, 13.97604488694528158, 40.62390960531435979 ) ) ;
#39273=CARTESIAN_POINT ( 'NONE',  ( 4.483927247898545687, 16.52544592524342804, 79.79057627198102409 ) ) ;
#39274=ORIENTED_EDGE ( 'NONE', *, *, #56349, .T. ) ;
#39275=CARTESIAN_POINT ( 'NONE',  ( -12.14591786802326823, 12.06949235617739902, 28.12609039468568284 ) ) ;
#39276=CARTESIAN_POINT ( 'NONE',  ( -0.05219959533937732626, 21.53943276465977519, 47.50109039468568994 ) ) ;
#39279=CARTESIAN_POINT ( 'NONE',  ( 0.05219959533936267826, -19.03943276465977164, 60.00109039468566863 ) ) ;
#39281=CARTESIAN_POINT ( 'NONE',  ( 0.05219959533937995610, -21.53943276465977519, 20.00109039468568639 ) ) ;
#39282=CARTESIAN_POINT ( 'NONE',  ( 9.564922557960805705, 16.46253265017160317, 64.58224293864769550 ) ) ;
#39284=CARTESIAN_POINT ( 'NONE',  ( -18.67979575497193778, 10.72451020669871902, 113.3344237280190328 ) ) ;
#39285=CARTESIAN_POINT ( 'NONE',  ( -16.46253265017160317, 9.564922557960807481, 45.83224293864769550 ) ) ;
#39286=CARTESIAN_POINT ( 'NONE',  ( -16.51473224551082808, 9.474510206698731452, 23.33442372801900078 ) ) ;
#39287=CARTESIAN_POINT ( 'NONE',  ( 4.379528057220092307, 16.55341960407617563, 87.29275706135236135 ) ) ;
#39288=CARTESIAN_POINT ( 'NONE',  ( -5.049401038298153566, 19.05341960407611168, 100.2072429386476955 ) ) ;
#39289=CARTESIAN_POINT ( 'NONE',  ( 21.55341960407619695, -5.719274019375665929, 71.04275706135234714 ) ) ;
#39293=CARTESIAN_POINT ( 'NONE',  ( 16.52544592524335698, 4.483927247898782831, 71.45942372801901854 ) ) ;
#39294=CARTESIAN_POINT ( 'NONE',  ( 5.719274019375673035, 21.55341960407619339, 77.29275706135234714 ) ) ;
#39295=CARTESIAN_POINT ( 'NONE',  ( -10.81492255796105439, 18.62759615963255655, 97.91775706135236135 ) ) ;
#39297=CARTESIAN_POINT ( 'NONE',  ( 8.314922557961029526, -14.29746914071037800, 40.41775706135234714 ) ) ;
#39298=CARTESIAN_POINT ( 'NONE',  ( -0.05219959533909027116, -19.03943276465977164, 82.49890960531436690 ) ) ;
#39299=CARTESIAN_POINT ( 'NONE',  ( 0.05219959533909260263, 19.03943276465977164, 104.9989096053143669 ) ) ;
#39301=CARTESIAN_POINT ( 'NONE',  ( 13.89961937509977652, -13.97604488694527269, 43.12390960531434558 ) ) ;
#39302=CARTESIAN_POINT ( 'NONE',  ( -10.81492255796078084, -18.62759615963271287, 37.08224293864768129 ) ) ;
#39303=CARTESIAN_POINT ( 'NONE',  ( 16.52544592524335698, 4.483927247898782831, 111.4594237280190328 ) ) ;
#39304=CARTESIAN_POINT ( 'NONE',  ( 8.224510206698953496, -14.34966873604960469, 77.91557627198102409 ) ) ;
#39305=CARTESIAN_POINT ( 'NONE',  ( -0.05219959533909027116, -19.03943276465977164, 77.49890960531435269 ) ) ;
#39306=CARTESIAN_POINT ( 'NONE',  ( -10.72451020669870658, -18.67979575497194134, 109.5844237280190328 ) ) ;
#39307=CARTESIAN_POINT ( 'NONE',  ( -16.51473224551069308, -9.474510206698971260, 31.66557627198102054 ) ) ;
#39308=CARTESIAN_POINT ( 'NONE',  ( 8.314922557960818139, 14.29746914071049879, 84.58224293864769550 ) ) ;
#39309=CARTESIAN_POINT ( 'NONE',  ( -10.81492255796105439, 18.62759615963255655, 42.91775706135235424 ) ) ;
#39310=CARTESIAN_POINT ( 'NONE',  ( 21.55341960407610458, 5.719274019375980345, 88.95724293864769550 ) ) ;
#39311=CARTESIAN_POINT ( 'NONE',  ( -5.049401038297874678, -19.05341960407617918, 54.79275706135234003 ) ) ;
#39313=CARTESIAN_POINT ( 'NONE',  ( -16.46253265017160317, 9.564922557960807481, 100.8322429386477097 ) ) ;
#39314=CARTESIAN_POINT ( 'NONE',  ( 4.379528057220339221, -16.55341960407611168, 67.70724293864769550 ) ) ;
#39315=CARTESIAN_POINT ( 'NONE',  ( -0.05219959533910754901, -16.53943276465976808, 52.49890960531435979 ) ) ;
#39316=CARTESIAN_POINT ( 'NONE',  ( 16.55341960407611168, 4.379528057220329451, 28.95724293864769905 ) ) ;
#39317=CARTESIAN_POINT ( 'NONE',  ( 19.03943276465977164, 0.05219959533936151252, 76.25109039468566152 ) ) ;
#39320=CARTESIAN_POINT ( 'NONE',  ( -0.05219959533907301413, -21.53943276465977519, 27.49890960531435269 ) ) ;
#39321=CARTESIAN_POINT ( 'NONE',  ( 12.06949235617757843, -12.14591786802309237, 93.12390960531436690 ) ) ;
#39323=CARTESIAN_POINT ( 'NONE',  ( 19.05341960407611168, 5.049401038298154454, 43.95724293864769550 ) ) ;
#39324=CARTESIAN_POINT ( 'NONE',  ( 18.62759615963271287, -10.81492255796078972, 43.33224293864769550 ) ) ;
#39325=CARTESIAN_POINT ( 'NONE',  ( -13.89961937509977652, 13.97604488694528158, 30.62390960531435269 ) ) ;
#39326=CARTESIAN_POINT ( 'NONE',  ( -4.379528057220086978, -16.55341960407618274, 74.79275706135234714 ) ) ;
#39327=CARTESIAN_POINT ( 'NONE',  ( 19.02544592524343514, -5.153800228976328945, 58.54057627198102409 ) ) ;
#39328=CARTESIAN_POINT ( 'NONE',  ( 0.05219959533936267826, -19.03943276465977164, 45.00109039468566863 ) ) ;
#39329=CARTESIAN_POINT ( 'NONE',  ( -0.05219959533937732626, 21.53943276465977519, 72.50109039468568994 ) ) ;
#39330=CARTESIAN_POINT ( 'NONE',  ( -10.72451020669898014, 18.67979575497178502, 40.41557627198103120 ) ) ;
#39331=CARTESIAN_POINT ( 'NONE',  ( 16.52544592524342804, -4.483927247898539470, 108.5405762719810241 ) ) ;
#39332=CARTESIAN_POINT ( 'NONE',  ( -19.03943276465977164, -0.05219959533935918106, 88.75109039468567573 ) ) ;
#39335=CARTESIAN_POINT ( 'NONE',  ( 10.81492255796078972, 18.62759615963270932, 49.58224293864769550 ) ) ;
#39336=CARTESIAN_POINT ( 'NONE',  ( 9.474510206698971260, -16.51473224551069308, 22.91557627198102765 ) ) ;
#39337=CARTESIAN_POINT ( 'NONE',  ( -21.52544592524334988, -5.823673210054445271, 83.95942372801900433 ) ) ;
#39338=CARTESIAN_POINT ( 'NONE',  ( 0.05219959533910956823, 16.53943276465976808, 49.99890960531437401 ) ) ;
#39339=CARTESIAN_POINT ( 'NONE',  ( 12.14591786802327356, -12.06949235617739191, 65.62609039468568994 ) ) ;
#39340=CARTESIAN_POINT ( 'NONE',  ( -12.06949235617756955, 12.14591786802309770, 50.62390960531435979 ) ) ;
#39341=CARTESIAN_POINT ( 'NONE',  ( 5.823673210054125526, 21.52544592524343514, 84.79057627198102409 ) ) ;
#39342=CARTESIAN_POINT ( 'NONE',  ( 15.80617190586746368, 15.72974639402197994, 79.37390960531436690 ) ) ;
#39344=CARTESIAN_POINT ( 'NONE',  ( -18.67979575497178146, -10.72451020669898902, 21.66557627198102409 ) ) ;
#39345=CARTESIAN_POINT ( 'NONE',  ( 4.379528057220339221, -16.55341960407611168, 82.70724293864770971 ) ) ;
#39346=CARTESIAN_POINT ( 'NONE',  ( -16.51473224551069308, -9.474510206698971260, 61.66557627198103120 ) ) ;
#39347=CARTESIAN_POINT ( 'NONE',  ( 0.05219959533909260263, 19.03943276465977164, 34.99890960531435979 ) ) ;
#39350=CARTESIAN_POINT ( 'NONE',  ( -4.483927247898782831, 16.52544592524335698, 82.70942372801900433 ) ) ;
#39352=CARTESIAN_POINT ( 'NONE',  ( 18.62759615963255655, 10.81492255796105972, 26.66775706135235424 ) ) ;
#39353=CARTESIAN_POINT ( 'NONE',  ( 9.474510206698971260, -16.51473224551069308, 72.91557627198102409 ) ) ;
#39354=CARTESIAN_POINT ( 'NONE',  ( -15.80617190586768217, 15.72974639402176855, 53.12609039468568284 ) ) ;
#39355=CARTESIAN_POINT ( 'NONE',  ( 13.97604488694527802, 13.89961937509977652, 109.3739096053143669 ) ) ;
#39359=CARTESIAN_POINT ( 'NONE',  ( 21.52544592524334988, 5.823673210054432836, 46.45942372801901854 ) ) ;
#39360=CARTESIAN_POINT ( 'NONE',  ( 13.97604488694527802, 13.89961937509977652, 114.3739096053143669 ) ) ;
#39361=CARTESIAN_POINT ( 'NONE',  ( -13.97604488694527625, -13.89961937509977652, 101.8739096053143811 ) ) ;
#39362=CARTESIAN_POINT ( 'NONE',  ( -19.02544592524334988, -5.153800228976617603, 48.95942372801900433 ) ) ;
#39363=CARTESIAN_POINT ( 'NONE',  ( 10.72451020669898902, -18.67979575497178502, 107.9155762719810241 ) ) ;
#39364=CARTESIAN_POINT ( 'NONE',  ( -19.02544592524334988, -5.153800228976617603, 48.95942372801900433 ) ) ;
#39365=CARTESIAN_POINT ( 'NONE',  ( -13.97604488694547697, 13.89961937509957934, 48.12609039468566863 ) ) ;
#39366=CARTESIAN_POINT ( 'NONE',  ( 16.52544592524335698, 4.483927247898782831, 106.4594237280190328 ) ) ;
#39367=DIRECTION ( 'NONE',  ( 1.000000000000000000, -0.000000000000000000, -0.000000000000000000 ) ) ;
#39368=CARTESIAN_POINT ( 'NONE',  ( -16.46253265017160317, 9.564922557960807481, 65.83224293864769550 ) ) ;
#39369=CARTESIAN_POINT ( 'NONE',  ( 10.81492255796106328, -18.62759615963255655, 85.41775706135236135 ) ) ;
#39370=CARTESIAN_POINT ( 'NONE',  ( 5.823673210054444382, -21.52544592524334988, 100.2094237280190043 ) ) ;
#39372=CARTESIAN_POINT ( 'NONE',  ( -0.05219959533909027116, -19.03943276465977164, 97.49890960531436690 ) ) ;
#39373=CARTESIAN_POINT ( 'NONE',  ( 18.67979575497194134, -10.72451020669871369, 70.83442372801901854 ) ) ;
#39374=CARTESIAN_POINT ( 'NONE',  ( -4.379528057220086978, -16.55341960407618274, 24.79275706135235779 ) ) ;
#39375=CARTESIAN_POINT ( 'NONE',  ( -16.51473224551069308, -9.474510206698971260, 76.66557627198103830 ) ) ;
#39376=CARTESIAN_POINT ( 'NONE',  ( 10.81492255796078972, 18.62759615963270932, 24.58224293864768839 ) ) ;
#39377=CARTESIAN_POINT ( 'NONE',  ( 13.89961937509977652, -13.97604488694527269, 98.12390960531433848 ) ) ;
#39378=CARTESIAN_POINT ( 'NONE',  ( -13.97604488694547520, 13.89961937509957934, 88.12609039468564731 ) ) ;
#39379=CARTESIAN_POINT ( 'NONE',  ( 16.51473224551069308, 9.474510206698969483, 84.16557627198102409 ) ) ;
#39380=CARTESIAN_POINT ( 'NONE',  ( 16.51473224551069308, 9.474510206698969483, 64.16557627198102409 ) ) ;
#39381=CARTESIAN_POINT ( 'NONE',  ( -10.81492255796078084, -18.62759615963271287, 112.0822429386477097 ) ) ;
#39382=CARTESIAN_POINT ( 'NONE',  ( 8.314922557961029526, -14.29746914071037800, 95.41775706135234714 ) ) ;
#39384=CARTESIAN_POINT ( 'NONE',  ( -0.05219959533936034679, 19.03943276465977164, 62.50109039468566863 ) ) ;
#39385=CARTESIAN_POINT ( 'NONE',  ( 13.89961937509977652, -13.97604488694527269, 88.12390960531438111 ) ) ;
#39386=CARTESIAN_POINT ( 'NONE',  ( -12.06949235617756955, 12.14591786802309770, 90.62390960531436690 ) ) ;
#39387=CARTESIAN_POINT ( 'NONE',  ( -5.719274019375978568, 21.55341960407610458, 30.20724293864769550 ) ) ;
#39388=CARTESIAN_POINT ( 'NONE',  ( 18.62759615963271287, -10.81492255796078972, 28.33224293864769550 ) ) ;
#39389=CARTESIAN_POINT ( 'NONE',  ( 16.52544592524342804, -4.483927247898539470, 88.54057627198103830 ) ) ;
#39391=CARTESIAN_POINT ( 'NONE',  ( 19.02544592524334988, 5.153800228976608722, 46.45942372801899012 ) ) ;
#39392=CARTESIAN_POINT ( 'NONE',  ( -12.06949235617739369, -12.14591786802326823, 104.3760903946856899 ) ) ;
#39393=CARTESIAN_POINT ( 'NONE',  ( -19.02544592524342804, 5.153800228976336051, 86.04057627198103830 ) ) ;
#39394=CARTESIAN_POINT ( 'NONE',  ( -10.81492255796105439, 18.62759615963255655, 67.91775706135234714 ) ) ;
#39395=CARTESIAN_POINT ( 'NONE',  ( 15.72974639402199770, -15.80617190586745480, 58.12390960531435979 ) ) ;
#39396=CARTESIAN_POINT ( 'NONE',  ( -18.67979575497193778, 10.72451020669871902, 28.33442372801902209 ) ) ;
#39397=CARTESIAN_POINT ( 'NONE',  ( 15.80617190586746368, 15.72974639402197994, 89.37390960531435269 ) ) ;
#39398=CARTESIAN_POINT ( 'NONE',  ( -16.52544592524342804, 4.483927247898546575, 111.0405762719810525 ) ) ;
#39399=CARTESIAN_POINT ( 'NONE',  ( 9.474510206698729675, 16.51473224551082808, 72.08442372801900433 ) ) ;
#39400=CARTESIAN_POINT ( 'NONE',  ( 9.564922557960805705, 16.46253265017160317, 49.58224293864770260 ) ) ;
#39401=CARTESIAN_POINT ( 'NONE',  ( -13.97604488694527625, -13.89961937509977652, 96.87390960531433848 ) ) ;
#39402=CARTESIAN_POINT ( 'NONE',  ( -9.564922557960796823, -16.46253265017161027, 92.08224293864769550 ) ) ;
#39403=CARTESIAN_POINT ( 'NONE',  ( -0.05219959533909027116, -19.03943276465977164, 22.49890960531436690 ) ) ;
#39404=CARTESIAN_POINT ( 'NONE',  ( -16.52544592524342804, 4.483927247898546575, 46.04057627198103830 ) ) ;
#39405=CARTESIAN_POINT ( 'NONE',  ( 12.14591786802327356, -12.06949235617739191, 45.62609039468567573 ) ) ;
#39406=CARTESIAN_POINT ( 'NONE',  ( -15.80617190586768217, 15.72974639402176855, 103.1260903946856757 ) ) ;
#39407=CARTESIAN_POINT ( 'NONE',  ( 13.89961937509977652, -13.97604488694527269, 113.1239096053143527 ) ) ;
#39408=CARTESIAN_POINT ( 'NONE',  ( -4.483927247898539470, -16.52544592524342804, 27.29057627198103120 ) ) ;
#39409=CARTESIAN_POINT ( 'NONE',  ( -21.52544592524334988, -5.823673210054445271, 28.95942372801902209 ) ) ;
#39410=CARTESIAN_POINT ( 'NONE',  ( 19.02544592524343514, -5.153800228976328945, 98.54057627198100988 ) ) ;
#39411=CARTESIAN_POINT ( 'NONE',  ( 16.52544592524335698, 4.483927247898782831, 106.4594237280190328 ) ) ;
#39412=CARTESIAN_POINT ( 'NONE',  ( 14.34966873604972726, -8.224510206698740333, 95.83442372801903275 ) ) ;
#39413=CARTESIAN_POINT ( 'NONE',  ( 16.55341960407618274, -4.379528057220086978, 26.04275706135235779 ) ) ;
#39414=CARTESIAN_POINT ( 'NONE',  ( 13.89961937509977652, -13.97604488694527269, 53.12390960531434558 ) ) ;
#39415=B_SPLINE_CURVE_WITH_KNOTS ( 'NONE', 3,
 ( #158021, #128659, #112504, #51831, #19512, #126669 ),
 .UNSPECIFIED., .F., .F.,
 ( 4, 2, 4 ),
 ( 0.007228050697041587397, 0.007608510107495056879, 0.007988969517948526361 ),
 .UNSPECIFIED. ) ;
#39416=CARTESIAN_POINT ( 'NONE',  ( 8.314922557960818139, 14.29746914071049879, 104.5822429386477097 ) ) ;
#39417=CARTESIAN_POINT ( 'NONE',  ( 21.52544592524344225, -5.823673210054117533, 113.5405762719810383 ) ) ;
#39418=CARTESIAN_POINT ( 'NONE',  ( -5.153800228976328057, -19.02544592524343514, 32.29057627198102409 ) ) ;
#39419=CARTESIAN_POINT ( 'NONE',  ( 9.474510206698971260, -16.51473224551069308, 107.9155762719810383 ) ) ;
#39420=CARTESIAN_POINT ( 'NONE',  ( -5.049401038298153566, 19.05341960407611168, 30.20724293864768839 ) ) ;
#39421=CARTESIAN_POINT ( 'NONE',  ( -19.05341960407611168, -5.049401038298163336, 101.4572429386476955 ) ) ;
#39422=CARTESIAN_POINT ( 'NONE',  ( -17.40805194822032576, -6.112264579159275790, 34.16628727489390371 ) ) ;
#39423=CARTESIAN_POINT ( 'NONE',  ( 13.89961937509977652, -13.97604488694527269, 98.12390960531433848 ) ) ;
#39424=CARTESIAN_POINT ( 'NONE',  ( -10.81492255796105439, 18.62759615963255655, 47.91775706135234714 ) ) ;
#39425=CARTESIAN_POINT ( 'NONE',  ( 4.379528057220339221, -16.55341960407611168, 87.70724293864769550 ) ) ;
#39426=CARTESIAN_POINT ( 'NONE',  ( 16.51473224551069308, 9.474510206698969483, 99.16557627198102409 ) ) ;
#39428=CARTESIAN_POINT ( 'NONE',  ( -16.53943276465976808, -0.05219959533934237506, 68.75109039468568994 ) ) ;
#39429=CARTESIAN_POINT ( 'NONE',  ( -10.72451020669870658, -18.67979575497194134, 84.58442372801903275 ) ) ;
#39430=CARTESIAN_POINT ( 'NONE',  ( 12.06949235617739724, 12.14591786802326823, 41.87609039468568284 ) ) ;
#39431=CARTESIAN_POINT ( 'NONE',  ( -19.02544592524342804, 5.153800228976336051, 81.04057627198103830 ) ) ;
#39432=CARTESIAN_POINT ( 'NONE',  ( 5.049401038297881783, 19.05341960407617563, 112.2927570613523471 ) ) ;
#39433=CARTESIAN_POINT ( 'NONE',  ( -12.06949235617739369, -12.14591786802326823, 79.37609039468567573 ) ) ;
#39434=CARTESIAN_POINT ( 'NONE',  ( 16.46253265017146816, 9.564922557961045513, 91.66775706135234714 ) ) ;
#39435=CARTESIAN_POINT ( 'NONE',  ( -5.153800228976328057, -19.02544592524343514, 62.29057627198100988 ) ) ;
#39436=CARTESIAN_POINT ( 'NONE',  ( -18.67979575497178146, -10.72451020669898902, 101.6655762719810383 ) ) ;
#39437=CARTESIAN_POINT ( 'NONE',  ( 16.53943276465976808, -0.05219959533910856209, 88.74890960531436690 ) ) ;
#39438=CARTESIAN_POINT ( 'NONE',  ( 13.97604488694548053, -13.89961937509957401, 95.62609039468563310 ) ) ;
#39439=CARTESIAN_POINT ( 'NONE',  ( 16.53943276465976808, 0.05219959533934440121, 56.25109039468568284 ) ) ;
#39441=CARTESIAN_POINT ( 'NONE',  ( 5.153800228976615827, -19.02544592524334988, 55.20942372801899722 ) ) ;
#39442=CARTESIAN_POINT ( 'NONE',  ( 16.53943276465976808, -0.05219959533910856209, 38.74890960531435979 ) ) ;
#39443=CARTESIAN_POINT ( 'NONE',  ( 4.379528057220339221, -16.55341960407611168, 82.70724293864770971 ) ) ;
#39444=CARTESIAN_POINT ( 'NONE',  ( 21.55341960407619695, -5.719274019375665929, 111.0427570613523613 ) ) ;
#39446=CARTESIAN_POINT ( 'NONE',  ( 15.80617190586769283, -15.72974639402175789, 20.62609039468568639 ) ) ;
#39447=CARTESIAN_POINT ( 'NONE',  ( 19.03943276465977164, -0.05219959533909143690, 73.74890960531435269 ) ) ;
#39448=CARTESIAN_POINT ( 'NONE',  ( 10.72451020669871369, 18.67979575497193778, 92.08442372801901854 ) ) ;
#39449=CARTESIAN_POINT ( 'NONE',  ( -19.03943276465977164, 0.05219959533909376836, 76.24890960531435269 ) ) ;
#39450=CARTESIAN_POINT ( 'NONE',  ( 10.72451020669898902, -18.67979575497178502, 47.91557627198102409 ) ) ;
#39451=CARTESIAN_POINT ( 'NONE',  ( 8.224510206698953496, -14.34966873604960469, 77.91557627198102409 ) ) ;
#39452=CARTESIAN_POINT ( 'NONE',  ( 19.05341960407611168, 5.049401038298154454, 58.95724293864768129 ) ) ;
#39453=CARTESIAN_POINT ( 'NONE',  ( 14.34966873604960469, 8.224510206698951720, 109.1655762719810383 ) ) ;
#39454=CARTESIAN_POINT ( 'NONE',  ( -5.823673210054431948, 21.52544592524334988, 22.70942372801901499 ) ) ;
#39455=CARTESIAN_POINT ( 'NONE',  ( -10.81492255796105439, 18.62759615963255655, 67.91775706135234714 ) ) ;
#39456=CARTESIAN_POINT ( 'NONE',  ( -16.46253265017160317, 9.564922557960807481, 40.83224293864769550 ) ) ;
#39457=CARTESIAN_POINT ( 'NONE',  ( 16.55341960407618274, -4.379528057220086978, 81.04275706135236135 ) ) ;
#39458=CARTESIAN_POINT ( 'NONE',  ( -5.719274019375978568, 21.55341960407610458, 115.2072429386476955 ) ) ;
#39459=CARTESIAN_POINT ( 'NONE',  ( -18.62759615963270932, 10.81492255796079327, 115.8322429386477097 ) ) ;
#39460=CARTESIAN_POINT ( 'NONE',  ( -19.03943276465977164, -0.05219959533935918106, 33.75109039468566863 ) ) ;
#39461=CARTESIAN_POINT ( 'NONE',  ( -16.46253265017160317, 9.564922557960807481, 65.83224293864769550 ) ) ;
#39463=CARTESIAN_POINT ( 'NONE',  ( 21.55341960407619695, -5.719274019375665929, 71.04275706135234714 ) ) ;
#39464=CARTESIAN_POINT ( 'NONE',  ( 21.52544592524344225, -5.823673210054117533, 58.54057627198103120 ) ) ;
#39465=CARTESIAN_POINT ( 'NONE',  ( -8.314922557960811034, -14.29746914071050412, 32.08224293864769550 ) ) ;
#39466=CARTESIAN_POINT ( 'NONE',  ( 15.72974639402176855, 15.80617190586768217, 76.87609039468567573 ) ) ;
#39467=CARTESIAN_POINT ( 'NONE',  ( 21.55341960407619695, -5.719274019375665929, 106.0427570613523471 ) ) ;
#39468=CARTESIAN_POINT ( 'NONE',  ( 12.14591786802309770, 12.06949235617756955, 54.37390960531435979 ) ) ;
#39469=CARTESIAN_POINT ( 'NONE',  ( 0.05219959533910956823, 16.53943276465976808, 99.99890960531436690 ) ) ;
#39470=CARTESIAN_POINT ( 'NONE',  ( -5.153800228976607833, 19.02544592524334988, 57.70942372801899012 ) ) ;
#39471=CARTESIAN_POINT ( 'NONE',  ( 16.53943276465976808, -0.05219959533910856209, 28.74890960531435624 ) ) ;
#39472=CARTESIAN_POINT ( 'NONE',  ( -0.05219959533937732626, 21.53943276465977519, 67.50109039468568994 ) ) ;
#39473=CARTESIAN_POINT ( 'NONE',  ( 19.03943276465977164, -0.05219959533909143690, 68.74890960531436690 ) ) ;
#39474=CARTESIAN_POINT ( 'NONE',  ( 9.564922557961047289, -16.46253265017146816, 30.41775706135232937 ) ) ;
#39475=CARTESIAN_POINT ( 'NONE',  ( -5.823673210054116645, -21.52544592524344225, 42.29057627198103120 ) ) ;
#39476=CARTESIAN_POINT ( 'NONE',  ( -0.05219959533937732626, 21.53943276465977519, 42.50109039468567573 ) ) ;
#39477=CARTESIAN_POINT ( 'NONE',  ( -15.72974639402197994, 15.80617190586746368, 100.6239096053143811 ) ) ;
#39478=CARTESIAN_POINT ( 'NONE',  ( 19.05341960407617918, -5.049401038297876454, 96.04275706135231871 ) ) ;
#39479=CARTESIAN_POINT ( 'NONE',  ( 0.05219959533934541429, -16.53943276465976808, 55.00109039468568284 ) ) ;
#39481=CARTESIAN_POINT ( 'NONE',  ( -15.72974639402197994, 15.80617190586746368, 95.62390960531436690 ) ) ;
#39482=CARTESIAN_POINT ( 'NONE',  ( 4.379528057220339221, -16.55341960407611168, 92.70724293864770971 ) ) ;
#39483=CARTESIAN_POINT ( 'NONE',  ( -16.52216118717206683, -7.221426719304509412, 101.0759902104699108 ) ) ;
#39484=CARTESIAN_POINT ( 'NONE',  ( -5.153800228976607833, 19.02544592524334988, 112.7094237280190043 ) ) ;
#39486=CARTESIAN_POINT ( 'NONE',  ( -0.05219959533907301413, -21.53943276465977519, 42.49890960531435979 ) ) ;
#39487=CARTESIAN_POINT ( 'NONE',  ( -16.55341960407617563, 4.379528057220093196, 88.54275706135236135 ) ) ;
#39489=CARTESIAN_POINT ( 'NONE',  ( -4.379528057220086978, -16.55341960407618274, 49.79275706135234714 ) ) ;
#39490=CARTESIAN_POINT ( 'NONE',  ( 21.55341960407619695, -5.719274019375665929, 31.04275706135234714 ) ) ;
#39491=CARTESIAN_POINT ( 'NONE',  ( 21.53943276465977519, -0.05219959533907433946, 38.74890960531435979 ) ) ;
#39492=CARTESIAN_POINT ( 'NONE',  ( -4.379528057220086978, -16.55341960407618274, 79.79275706135236135 ) ) ;
#39493=CARTESIAN_POINT ( 'NONE',  ( -5.049401038298153566, 19.05341960407611168, 95.20724293864770971 ) ) ;
#39494=CARTESIAN_POINT ( 'NONE',  ( 5.719274019375673035, 21.55341960407619339, 72.29275706135236135 ) ) ;
#39495=CARTESIAN_POINT ( 'NONE',  ( 18.67979575497178502, 10.72451020669898547, 34.16557627198102409 ) ) ;
#39496=CARTESIAN_POINT ( 'NONE',  ( -18.67979575497178146, -10.72451020669898902, 21.66557627198102409 ) ) ;
#39498=CARTESIAN_POINT ( 'NONE',  ( -16.46253265017146816, -9.564922557961047289, 54.16775706135234003 ) ) ;
#39499=CARTESIAN_POINT ( 'NONE',  ( 12.14591786802327356, -12.06949235617739191, 70.62609039468567573 ) ) ;
#39500=CARTESIAN_POINT ( 'NONE',  ( 0.05219959533907565091, 21.53943276465977519, 34.99890960531435979 ) ) ;
#39502=CARTESIAN_POINT ( 'NONE',  ( 9.474510206698971260, -16.51473224551069308, 87.91557627198102409 ) ) ;
#39503=CARTESIAN_POINT ( 'NONE',  ( 8.314922557961029526, -14.29746914071037800, 110.4177570613523756 ) ) ;
#39505=CARTESIAN_POINT ( 'NONE',  ( 14.34966873604960469, 8.224510206698951720, 109.1655762719810383 ) ) ;
#39506=CARTESIAN_POINT ( 'NONE',  ( 5.823673210054125526, 21.52544592524343514, 49.79057627198102409 ) ) ;
#39507=CARTESIAN_POINT ( 'NONE',  ( 5.153800228976335163, 19.02544592524342804, 44.79057627198103830 ) ) ;
#39508=CARTESIAN_POINT ( 'NONE',  ( -8.314922557961024197, 14.29746914071037800, 72.91775706135234714 ) ) ;
#39509=CARTESIAN_POINT ( 'NONE',  ( -0.05219959533937732626, 21.53943276465977519, 32.50109039468568284 ) ) ;
#39510=CARTESIAN_POINT ( 'NONE',  ( -13.89961937509957401, -13.97604488694547875, 89.37609039468563310 ) ) ;
#39511=CARTESIAN_POINT ( 'NONE',  ( -14.34966873604960291, -8.224510206698953496, 86.66557627198102409 ) ) ;
#39512=CARTESIAN_POINT ( 'NONE',  ( -19.05341960407611168, -5.049401038298163336, 51.45724293864770260 ) ) ;
#39513=CARTESIAN_POINT ( 'NONE',  ( -19.05341960407611168, -5.049401038298163336, 26.45724293864769550 ) ) ;
#39514=CARTESIAN_POINT ( 'NONE',  ( -10.81492255796105439, 18.62759615963255655, 102.9177570613523756 ) ) ;
#39515=CARTESIAN_POINT ( 'NONE',  ( 19.05341960407611168, 5.049401038298154454, 83.95724293864766707 ) ) ;
#39516=CARTESIAN_POINT ( 'NONE',  ( -0.05219959533934338120, 16.53943276465976808, 62.50109039468568284 ) ) ;
#39517=CARTESIAN_POINT ( 'NONE',  ( 15.80617190586769283, -15.72974639402175789, 90.62609039468567573 ) ) ;
#39518=CARTESIAN_POINT ( 'NONE',  ( -10.81492255796078084, -18.62759615963271287, 52.08224293864768839 ) ) ;
#39519=CARTESIAN_POINT ( 'NONE',  ( -16.53943276465976808, -0.05219959533934237506, 73.75109039468567573 ) ) ;
#39520=CARTESIAN_POINT ( 'NONE',  ( 13.97604488694548053, -13.89961937509957401, 55.62609039468566863 ) ) ;
#39521=CARTESIAN_POINT ( 'NONE',  ( -19.03943276465977164, -0.05219959533935918106, 68.75109039468566152 ) ) ;
#39522=CARTESIAN_POINT ( 'NONE',  ( 5.719274019375673035, 21.55341960407619339, 67.29275706135234714 ) ) ;
#39523=CARTESIAN_POINT ( 'NONE',  ( -19.02544592524342804, 5.153800228976336051, 66.04057627198103830 ) ) ;
#39524=CARTESIAN_POINT ( 'NONE',  ( -5.153800228976328057, -19.02544592524343514, 22.29057627198102765 ) ) ;
#39525=CARTESIAN_POINT ( 'NONE',  ( -19.05341960407617563, 5.049401038297882671, 63.54275706135234003 ) ) ;
#39527=CARTESIAN_POINT ( 'NONE',  ( 19.05341960407611168, 5.049401038298154454, 98.95724293864766707 ) ) ;
#39528=CARTESIAN_POINT ( 'NONE',  ( -14.29746914071049879, 8.314922557960819915, 50.83224293864770971 ) ) ;
#39529=CARTESIAN_POINT ( 'NONE',  ( -21.55341960407610458, -5.719274019375992779, 51.45724293864770260 ) ) ;
#39531=CARTESIAN_POINT ( 'NONE',  ( 15.80617190586769283, -15.72974639402175789, 110.6260903946857042 ) ) ;
#39533=CARTESIAN_POINT ( 'NONE',  ( -16.51473224551069308, -9.474510206698971260, 46.66557627198102409 ) ) ;
#39534=CARTESIAN_POINT ( 'NONE',  ( 0.05219959533909260263, 19.03943276465977164, 29.99890960531435979 ) ) ;
#39537=CARTESIAN_POINT ( 'NONE',  ( -8.314922557961024197, 14.29746914071037800, 67.91775706135234714 ) ) ;
#39538=CARTESIAN_POINT ( 'NONE',  ( -15.72974639402197994, 15.80617190586746368, 80.62390960531438111 ) ) ;
#39539=CARTESIAN_POINT ( 'NONE',  ( -12.14591786802309592, -12.06949235617757132, 56.87390960531436690 ) ) ;
#39540=CARTESIAN_POINT ( 'NONE',  ( -9.474510206698964154, 16.51473224551069663, 45.41557627198103120 ) ) ;
#39542=CARTESIAN_POINT ( 'NONE',  ( -5.823673210054431948, 21.52544592524334988, 42.70942372801901854 ) ) ;
#39543=CARTESIAN_POINT ( 'NONE',  ( 19.02544592524334988, 5.153800228976608722, 46.45942372801899012 ) ) ;
#39544=CARTESIAN_POINT ( 'NONE',  ( -9.474510206698964154, 16.51473224551069663, 30.41557627198102054 ) ) ;
#39545=CARTESIAN_POINT ( 'NONE',  ( 15.72974639402176855, 15.80617190586768217, 76.87609039468567573 ) ) ;
#39546=CARTESIAN_POINT ( 'NONE',  ( 13.89961937509977652, -13.97604488694527269, 23.12390960531436335 ) ) ;
#39547=ORIENTED_EDGE ( 'NONE', *, *, #115114, .T. ) ;
#39548=CARTESIAN_POINT ( 'NONE',  ( -16.52544592524342804, 4.483927247898546575, 41.04057627198103120 ) ) ;
#39549=CARTESIAN_POINT ( 'NONE',  ( 17.49999999999999645, 3.209263204892637500, 112.7380317439374409 ) ) ;
#39550=CARTESIAN_POINT ( 'NONE',  ( 18.62759615963271287, -10.81492255796078972, 38.33224293864768839 ) ) ;
#39553=CARTESIAN_POINT ( 'NONE',  ( -19.02544592524342804, 5.153800228976336051, 96.04057627198103830 ) ) ;
#39554=CARTESIAN_POINT ( 'NONE',  ( -16.52544592524342804, 4.483927247898546575, 91.04057627198103830 ) ) ;
#39555=CARTESIAN_POINT ( 'NONE',  ( -16.55341960407617563, 4.379528057220093196, 28.54275706135234358 ) ) ;
#39556=ADVANCED_FACE ( 'NONE', ( #47609 ), #188116, .T. ) ;
#39557=CARTESIAN_POINT ( 'NONE',  ( -21.53943276465977519, 0.05219959533907696930, 66.24890960531436690 ) ) ;
#39559=CARTESIAN_POINT ( 'NONE',  ( 16.46253265017160672, -9.564922557960803928, 28.33224293864769550 ) ) ;
#39560=CARTESIAN_POINT ( 'NONE',  ( 5.153800228976335163, 19.02544592524342804, 84.79057627198099567 ) ) ;
#39561=CARTESIAN_POINT ( 'NONE',  ( 5.823673210054125526, 21.52544592524343514, 84.79057627198102409 ) ) ;
#39562=CARTESIAN_POINT ( 'NONE',  ( -4.483927247898539470, -16.52544592524342804, 22.29057627198102765 ) ) ;
#39563=CARTESIAN_POINT ( 'NONE',  ( 5.049401038298161559, -19.05341960407611168, 102.7072429386476955 ) ) ;
#39564=CARTESIAN_POINT ( 'NONE',  ( -13.89961937509957401, -13.97604488694547875, 79.37609039468567573 ) ) ;
#39565=CARTESIAN_POINT ( 'NONE',  ( 5.719274019375673035, 21.55341960407619339, 107.2927570613523471 ) ) ;
#39566=CARTESIAN_POINT ( 'NONE',  ( -5.719274019375978568, 21.55341960407610458, 80.20724293864769550 ) ) ;
#39567=CARTESIAN_POINT ( 'NONE',  ( -21.55341960407610458, -5.719274019375992779, 31.45724293864769550 ) ) ;
#39568=CARTESIAN_POINT ( 'NONE',  ( 19.02544592524343514, -5.153800228976328945, 63.54057627198103830 ) ) ;
#39569=CARTESIAN_POINT ( 'NONE',  ( -12.06949235617739369, -12.14591786802326823, 109.3760903946857042 ) ) ;
#39570=CARTESIAN_POINT ( 'NONE',  ( -16.46253265017160317, 9.564922557960807481, 80.83224293864769550 ) ) ;
#39572=CARTESIAN_POINT ( 'NONE',  ( 13.89961937509957401, 13.97604488694547697, 21.87609039468566152 ) ) ;
#39573=CARTESIAN_POINT ( 'NONE',  ( 8.224510206698953496, -14.34966873604960469, 87.91557627198103830 ) ) ;
#39574=CARTESIAN_POINT ( 'NONE',  ( 18.67979575497194134, -10.72451020669871369, 20.83442372801901143 ) ) ;
#39576=CARTESIAN_POINT ( 'NONE',  ( 15.80617190586746368, 15.72974639402197994, 74.37390960531436690 ) ) ;
#39577=CARTESIAN_POINT ( 'NONE',  ( -16.53943276465976808, -0.05219959533934237506, 88.75109039468567573 ) ) ;
#39578=CARTESIAN_POINT ( 'NONE',  ( 13.97604488694527802, 13.89961937509977652, 24.37390960531435624 ) ) ;
#39579=CARTESIAN_POINT ( 'NONE',  ( 19.02544592524343514, -5.153800228976328945, 78.54057627198099567 ) ) ;
#39580=CARTESIAN_POINT ( 'NONE',  ( -17.50000000000000355, -5.499999999999980460, 96.28230962303564411 ) ) ;
#39582=CARTESIAN_POINT ( 'NONE',  ( 4.483927247898545687, 16.52544592524342804, 24.79057627198103120 ) ) ;
#39583=CARTESIAN_POINT ( 'NONE',  ( -5.823673210054431948, 21.52544592524334988, 57.70942372801901143 ) ) ;
#39584=CARTESIAN_POINT ( 'NONE',  ( -13.97604488694527625, -13.89961937509977652, 111.8739096053143243 ) ) ;
#39585=CARTESIAN_POINT ( 'NONE',  ( -21.52544592524334988, -5.823673210054445271, 93.95942372801903275 ) ) ;
#39586=CARTESIAN_POINT ( 'NONE',  ( 19.03943276465977164, -0.05219959533909143690, 48.74890960531435979 ) ) ;
#39587=CARTESIAN_POINT ( 'NONE',  ( 19.02544592524343514, -5.153800228976328945, 53.54057627198102409 ) ) ;
#39589=CARTESIAN_POINT ( 'NONE',  ( 18.62759615963255655, 10.81492255796105972, 91.66775706135234714 ) ) ;
#39590=CARTESIAN_POINT ( 'NONE',  ( -14.29746914071037622, -8.314922557961029526, 59.16775706135234714 ) ) ;
#39591=CARTESIAN_POINT ( 'NONE',  ( -21.55341960407619339, 5.719274019375674811, 83.54275706135234714 ) ) ;
#39592=CARTESIAN_POINT ( 'NONE',  ( 21.53943276465977519, -0.05219959533907433946, 23.74890960531435269 ) ) ;
#39593=CARTESIAN_POINT ( 'NONE',  ( -16.46253265017146816, -9.564922557961047289, 94.16775706135233293 ) ) ;
#39594=CARTESIAN_POINT ( 'NONE',  ( 15.80617190586769283, -15.72974639402175789, 60.62609039468567573 ) ) ;
#39595=CARTESIAN_POINT ( 'NONE',  ( -0.05219959533934338120, 16.53943276465976808, 32.50109039468568284 ) ) ;
#39596=CARTESIAN_POINT ( 'NONE',  ( -10.81492255796078084, -18.62759615963271287, 87.08224293864769550 ) ) ;
#39597=CARTESIAN_POINT ( 'NONE',  ( 5.153800228976615827, -19.02544592524334988, 85.20942372801900433 ) ) ;
#39598=CARTESIAN_POINT ( 'NONE',  ( 9.564922557960805705, 16.46253265017160317, 69.58224293864770971 ) ) ;
#39599=CARTESIAN_POINT ( 'NONE',  ( 16.51473224551083163, -9.474510206698727899, 95.83442372801900433 ) ) ;
#39600=CARTESIAN_POINT ( 'NONE',  ( 13.89961937509957401, 13.97604488694547697, 96.87609039468566152 ) ) ;
#39601=CARTESIAN_POINT ( 'NONE',  ( 16.55341960407611168, 4.379528057220329451, 58.95724293864770971 ) ) ;
#39602=CARTESIAN_POINT ( 'NONE',  ( -16.51473224551082808, 9.474510206698731452, 83.33442372801899012 ) ) ;
#39603=CARTESIAN_POINT ( 'NONE',  ( -8.314922557961024197, 14.29746914071037800, 62.91775706135236135 ) ) ;
#39604=CARTESIAN_POINT ( 'NONE',  ( 5.049401038297881783, 19.05341960407617563, 37.29275706135232582 ) ) ;
#39605=CARTESIAN_POINT ( 'NONE',  ( -19.02544592524342804, 5.153800228976336051, 36.04057627198100988 ) ) ;
#39606=CARTESIAN_POINT ( 'NONE',  ( 16.51473224551069308, 9.474510206698969483, 49.16557627198102409 ) ) ;
#39607=CARTESIAN_POINT ( 'NONE',  ( 4.483927247898790824, -16.52544592524335698, 60.20942372801902565 ) ) ;
#39610=CARTESIAN_POINT ( 'NONE',  ( 19.03943276465977164, -0.05219959533909143690, 103.7489096053143669 ) ) ;
#39611=CARTESIAN_POINT ( 'NONE',  ( -5.049401038298153566, 19.05341960407611168, 25.20724293864768484 ) ) ;
#39613=CARTESIAN_POINT ( 'NONE',  ( 5.049401038297881783, 19.05341960407617563, 97.29275706135233293 ) ) ;
#39614=CARTESIAN_POINT ( 'NONE',  ( -15.80617190586745835, -15.72974639402198527, 36.87390960531435979 ) ) ;
#39615=CARTESIAN_POINT ( 'NONE',  ( -13.97604488694547697, 13.89961937509957934, 38.12609039468566152 ) ) ;
#39616=CARTESIAN_POINT ( 'NONE',  ( -0.05219959533934338120, 16.53943276465976808, 22.50109039468567573 ) ) ;
#39617=CARTESIAN_POINT ( 'NONE',  ( 9.564922557960805705, 16.46253265017160317, 34.58224293864770260 ) ) ;
#39618=CARTESIAN_POINT ( 'NONE',  ( -5.153800228976328057, -19.02544592524343514, 52.29057627198100988 ) ) ;
#39619=CARTESIAN_POINT ( 'NONE',  ( -10.81492255796078084, -18.62759615963271287, 67.08224293864770971 ) ) ;
#39620=CARTESIAN_POINT ( 'NONE',  ( 5.153800228976335163, 19.02544592524342804, 99.79057627198102409 ) ) ;
#39621=CARTESIAN_POINT ( 'NONE',  ( 16.51473224551069308, 9.474510206698969483, 39.16557627198103120 ) ) ;
#39623=CARTESIAN_POINT ( 'NONE',  ( 13.97604488694548053, -13.89961937509957401, 90.62609039468567573 ) ) ;
#39624=CARTESIAN_POINT ( 'NONE',  ( -8.224510206698948167, 14.34966873604960824, 55.41557627198102409 ) ) ;
#39625=CARTESIAN_POINT ( 'NONE',  ( 10.72451020669898902, -18.67979575497178502, 27.91557627198103830 ) ) ;
#39626=CARTESIAN_POINT ( 'NONE',  ( 18.62759615963255655, 10.81492255796105972, 106.6677570613523756 ) ) ;
#39627=CARTESIAN_POINT ( 'NONE',  ( 18.62759615963271287, -10.81492255796078972, 93.33224293864769550 ) ) ;
#39628=CARTESIAN_POINT ( 'NONE',  ( 15.72974639402176855, 15.80617190586768217, 71.87609039468568994 ) ) ;
#39629=CARTESIAN_POINT ( 'NONE',  ( -18.67979575497193778, 10.72451020669871902, 78.33442372801901854 ) ) ;
#39630=CARTESIAN_POINT ( 'NONE',  ( 9.564922557960805705, 16.46253265017160317, 114.5822429386476955 ) ) ;
#39631=CARTESIAN_POINT ( 'NONE',  ( 16.53943276465976808, 0.05219959533934440121, 101.2510903946856757 ) ) ;
#39632=CARTESIAN_POINT ( 'NONE',  ( -21.53943276465977519, -0.05219959533937600094, 63.75109039468568284 ) ) ;
#39633=CARTESIAN_POINT ( 'NONE',  ( -0.05219959533909027116, -19.03943276465977164, 62.49890960531435979 ) ) ;
#39634=CARTESIAN_POINT ( 'NONE',  ( -13.89961937509957401, -13.97604488694547875, 34.37609039468566863 ) ) ;
#39635=CARTESIAN_POINT ( 'NONE',  ( 15.80617190586769283, -15.72974639402175789, 25.62609039468567929 ) ) ;
#39636=CARTESIAN_POINT ( 'NONE',  ( 13.89961937509977652, -13.97604488694527269, 73.12390960531436690 ) ) ;
#39637=CARTESIAN_POINT ( 'NONE',  ( 8.314922557960818139, 14.29746914071049879, 84.58224293864769550 ) ) ;
#39638=CARTESIAN_POINT ( 'NONE',  ( 12.06949235617757843, -12.14591786802309237, 53.12390960531436690 ) ) ;
#39639=CARTESIAN_POINT ( 'NONE',  ( 15.80617190586746368, 15.72974639402197994, 54.37390960531435979 ) ) ;
#39640=CARTESIAN_POINT ( 'NONE',  ( 19.03943276465977164, -0.05219959533909143690, 63.74890960531435979 ) ) ;
#39641=CARTESIAN_POINT ( 'NONE',  ( 15.72974639402199770, -15.80617190586745480, 73.12390960531436690 ) ) ;
#39642=CARTESIAN_POINT ( 'NONE',  ( -13.97604488694547697, 13.89961937509957934, 48.12609039468566863 ) ) ;
#39643=CARTESIAN_POINT ( 'NONE',  ( 13.97604488694548053, -13.89961937509957401, 25.62609039468566507 ) ) ;
#39644=CARTESIAN_POINT ( 'NONE',  ( -12.06949235617756955, 12.14591786802309770, 60.62390960531437401 ) ) ;
#39645=CARTESIAN_POINT ( 'NONE',  ( 21.52544592524344225, -5.823673210054117533, 43.54057627198103830 ) ) ;
#39648=CARTESIAN_POINT ( 'NONE',  ( -16.52544592524335698, -4.483927247898792601, 78.95942372801901854 ) ) ;
#39650=CARTESIAN_POINT ( 'NONE',  ( -19.02544592524334988, -5.153800228976617603, 93.95942372801900433 ) ) ;
#39651=CARTESIAN_POINT ( 'NONE',  ( 8.314922557960818139, 14.29746914071049879, 49.58224293864769550 ) ) ;
#39653=CARTESIAN_POINT ( 'NONE',  ( -13.89961937509977652, 13.97604488694528158, 45.62390960531433848 ) ) ;
#39654=CARTESIAN_POINT ( 'NONE',  ( -4.483927247898539470, -16.52544592524342804, 37.29057627198102409 ) ) ;
#39655=CARTESIAN_POINT ( 'NONE',  ( -16.51473224551069308, -9.474510206698971260, 86.66557627198102409 ) ) ;
#39656=CARTESIAN_POINT ( 'NONE',  ( -0.05219959533909027116, -19.03943276465977164, 52.49890960531436690 ) ) ;
#39657=CARTESIAN_POINT ( 'NONE',  ( -15.72974639402176322, -15.80617190586768395, 59.37609039468568284 ) ) ;
#39658=CARTESIAN_POINT ( 'NONE',  ( 13.89961937509977652, -13.97604488694527269, 78.12390960531433848 ) ) ;
#39659=CARTESIAN_POINT ( 'NONE',  ( -16.51473224551069308, -9.474510206698971260, 31.66557627198102054 ) ) ;
#39660=CARTESIAN_POINT ( 'NONE',  ( -19.03943276465977164, 0.05219959533909376836, 71.24890960531435269 ) ) ;
#39661=CARTESIAN_POINT ( 'NONE',  ( -21.53943276465977519, 0.05219959533907696930, 46.24890960531435979 ) ) ;
#39662=CARTESIAN_POINT ( 'NONE',  ( -19.05341960407611168, -5.049401038298163336, 31.45724293864769550 ) ) ;
#39663=CARTESIAN_POINT ( 'NONE',  ( 18.62759615963271287, -10.81492255796078972, 58.33224293864768839 ) ) ;
#39664=CARTESIAN_POINT ( 'NONE',  ( -12.06949235617739369, -12.14591786802326823, 104.3760903946856899 ) ) ;
#39665=CARTESIAN_POINT ( 'NONE',  ( 9.564922557961047289, -16.46253265017146816, 20.41775706135233293 ) ) ;
#39666=CARTESIAN_POINT ( 'NONE',  ( -16.55341960407617563, 4.379528057220093196, 48.54275706135234714 ) ) ;
#39667=CARTESIAN_POINT ( 'NONE',  ( 12.14591786802327356, -12.06949235617739191, 80.62609039468567573 ) ) ;
#39668=CARTESIAN_POINT ( 'NONE',  ( -17.72696623605159516, 5.500000000000051514, 68.59811031808418136 ) ) ;
#39669=CARTESIAN_POINT ( 'NONE',  ( -4.483927247898782831, 16.52544592524335698, 67.70942372801901854 ) ) ;
#39670=CARTESIAN_POINT ( 'NONE',  ( 18.67979575497178502, 10.72451020669898547, 29.16557627198103120 ) ) ;
#39671=CARTESIAN_POINT ( 'NONE',  ( 9.474510206698971260, -16.51473224551069308, 27.91557627198103120 ) ) ;
#39672=CARTESIAN_POINT ( 'NONE',  ( -12.14591786802326823, 12.06949235617739902, 38.12609039468567573 ) ) ;
#39673=CARTESIAN_POINT ( 'NONE',  ( -19.05341960407611168, -5.049401038298163336, 51.45724293864770260 ) ) ;
#39674=CARTESIAN_POINT ( 'NONE',  ( 21.55341960407619695, -5.719274019375665929, 36.04275706135234714 ) ) ;
#39675=CARTESIAN_POINT ( 'NONE',  ( 4.379528057220092307, 16.55341960407617563, 42.29275706135235424 ) ) ;
#39676=CARTESIAN_POINT ( 'NONE',  ( -16.55341960407617563, 4.379528057220093196, 98.54275706135234714 ) ) ;
#39677=LINE ( 'NONE', #166035, #27890 ) ;
#39678=CARTESIAN_POINT ( 'NONE',  ( -5.823673210054431948, 21.52544592524334988, 97.70942372801904696 ) ) ;
#39679=CARTESIAN_POINT ( 'NONE',  ( -19.05341960407617563, 5.049401038297882671, 108.5427570613523187 ) ) ;
#39680=CARTESIAN_POINT ( 'NONE',  ( 0.05219959533936267826, -19.03943276465977164, 65.00109039468567573 ) ) ;
#39681=CARTESIAN_POINT ( 'NONE',  ( 4.483927247898545687, 16.52544592524342804, 74.79057627198105251 ) ) ;
#39682=CARTESIAN_POINT ( 'NONE',  ( -19.05341960407611168, -5.049401038298163336, 26.45724293864769550 ) ) ;
#39683=CARTESIAN_POINT ( 'NONE',  ( -19.02544592524334988, -5.153800228976617603, 58.95942372801900433 ) ) ;
#39685=CARTESIAN_POINT ( 'NONE',  ( -18.67979575497193778, 10.72451020669871902, 58.33442372801901143 ) ) ;
#39686=CARTESIAN_POINT ( 'NONE',  ( 16.52544592524335698, 4.483927247898782831, 26.45942372801901854 ) ) ;
#39688=CARTESIAN_POINT ( 'NONE',  ( -5.823673210054116645, -21.52544592524344225, 22.29057627198102765 ) ) ;
#39689=CARTESIAN_POINT ( 'NONE',  ( 16.46253265017146816, 9.564922557961045513, 106.6677570613523471 ) ) ;
#39690=CARTESIAN_POINT ( 'NONE',  ( -5.153800228976328057, -19.02544592524343514, 112.2905762719810099 ) ) ;
#39692=CARTESIAN_POINT ( 'NONE',  ( -5.153800228976328057, -19.02544592524343514, 22.29057627198102765 ) ) ;
#39693=CARTESIAN_POINT ( 'NONE',  ( -18.67979575497193778, 10.72451020669871902, 113.3344237280190328 ) ) ;
#39694=CARTESIAN_POINT ( 'NONE',  ( 0.05219959533909260263, 19.03943276465977164, 49.99890960531435979 ) ) ;
#39695=CARTESIAN_POINT ( 'NONE',  ( -18.62759615963255300, -10.81492255796106328, 69.16775706135234714 ) ) ;
#39696=CARTESIAN_POINT ( 'NONE',  ( 5.719274019375673035, 21.55341960407619339, 102.2927570613523613 ) ) ;
#39697=CARTESIAN_POINT ( 'NONE',  ( -12.14591786802309592, -12.06949235617757132, 21.87390960531436690 ) ) ;
#39698=CARTESIAN_POINT ( 'NONE',  ( -9.474510206698964154, 16.51473224551069663, 85.41557627198102409 ) ) ;
#39699=CARTESIAN_POINT ( 'NONE',  ( -18.67979575497193778, 10.72451020669871902, 58.33442372801901143 ) ) ;
#39700=CARTESIAN_POINT ( 'NONE',  ( 10.81492255796106328, -18.62759615963255655, 50.41775706135235424 ) ) ;
#39701=CARTESIAN_POINT ( 'NONE',  ( -5.153800228976607833, 19.02544592524334988, 77.70942372801900433 ) ) ;
#39702=CARTESIAN_POINT ( 'NONE',  ( 19.05341960407611168, 5.049401038298154454, 103.9572429386476671 ) ) ;
#39703=CARTESIAN_POINT ( 'NONE',  ( -9.564922557960796823, -16.46253265017161027, 22.08224293864768839 ) ) ;
#39704=CARTESIAN_POINT ( 'NONE',  ( -15.80617190586745835, -15.72974639402198527, 106.8739096053143811 ) ) ;
#39705=CARTESIAN_POINT ( 'NONE',  ( -9.474510206698720793, -16.51473224551083518, 39.58442372801899722 ) ) ;
#39706=CARTESIAN_POINT ( 'NONE',  ( -16.55341960407611168, -4.379528057220339221, 91.45724293864769550 ) ) ;
#39707=CARTESIAN_POINT ( 'NONE',  ( 19.02544592524343514, -5.153800228976328945, 43.54057627198103120 ) ) ;
#39708=CARTESIAN_POINT ( 'NONE',  ( -5.153800228976607833, 19.02544592524334988, 102.7094237280189759 ) ) ;
#39709=CARTESIAN_POINT ( 'NONE',  ( -16.53943276465976808, 0.05219959533911058130, 56.24890960531436690 ) ) ;
#39710=CARTESIAN_POINT ( 'NONE',  ( -21.53943276465977519, -0.05219959533937600094, 113.7510903946856757 ) ) ;
#39711=CARTESIAN_POINT ( 'NONE',  ( 0.05219959533909260263, 19.03943276465977164, 99.99890960531436690 ) ) ;
#39712=CARTESIAN_POINT ( 'NONE',  ( -0.05219959533936034679, 19.03943276465977164, 92.50109039468566152 ) ) ;
#39713=CARTESIAN_POINT ( 'NONE',  ( -10.81492255796078084, -18.62759615963271287, 92.08224293864769550 ) ) ;
#39714=CARTESIAN_POINT ( 'NONE',  ( -5.823673210054431948, 21.52544592524334988, 47.70942372801902565 ) ) ;
#39715=CARTESIAN_POINT ( 'NONE',  ( -14.29746914071037622, -8.314922557961029526, 49.16775706135234003 ) ) ;
#39716=CARTESIAN_POINT ( 'NONE',  ( 16.55341960407618274, -4.379528057220086978, 106.0427570613523471 ) ) ;
#39717=CARTESIAN_POINT ( 'NONE',  ( -14.34966873604972548, 8.224510206698743886, 43.33442372801901143 ) ) ;
#39718=CARTESIAN_POINT ( 'NONE',  ( -18.67979575497193778, 10.72451020669871902, 33.33442372801900433 ) ) ;
#39719=CARTESIAN_POINT ( 'NONE',  ( 15.72974639402199770, -15.80617190586745480, 48.12390960531436690 ) ) ;
#39720=CARTESIAN_POINT ( 'NONE',  ( 9.564922557960805705, 16.46253265017160317, 29.58224293864769550 ) ) ;
#39722=CARTESIAN_POINT ( 'NONE',  ( -4.379528057220086978, -16.55341960407618274, 59.79275706135234714 ) ) ;
#39725=CARTESIAN_POINT ( 'NONE',  ( 5.823673210054125526, 21.52544592524343514, 94.79057627198105251 ) ) ;
#39726=CARTESIAN_POINT ( 'NONE',  ( 4.379528057220339221, -16.55341960407611168, 32.70724293864770260 ) ) ;
#39727=CARTESIAN_POINT ( 'NONE',  ( -16.53943276465976808, -0.05219959533934237506, 68.75109039468568994 ) ) ;
#39728=CARTESIAN_POINT ( 'NONE',  ( -9.474510206698964154, 16.51473224551069663, 55.41557627198103120 ) ) ;
#39729=CARTESIAN_POINT ( 'NONE',  ( -16.51473224551082808, 9.474510206698731452, 88.33442372801900433 ) ) ;
#39730=CARTESIAN_POINT ( 'NONE',  ( 15.72974639402199770, -15.80617190586745480, 88.12390960531436690 ) ) ;
#39731=CARTESIAN_POINT ( 'NONE',  ( 14.34966873604960469, 8.224510206698951720, 29.16557627198103120 ) ) ;
#39734=CARTESIAN_POINT ( 'NONE',  ( 15.72974639402199770, -15.80617190586745480, 68.12390960531436690 ) ) ;
#39735=CARTESIAN_POINT ( 'NONE',  ( 14.34966873604972726, -8.224510206698740333, 105.8344237280190328 ) ) ;
#39736=ORIENTED_EDGE ( 'NONE', *, *, #17849, .F. ) ;
#39738=CARTESIAN_POINT ( 'NONE',  ( 5.823673210054125526, 21.52544592524343514, 94.79057627198105251 ) ) ;
#39739=CARTESIAN_POINT ( 'NONE',  ( 15.72974639402199770, -15.80617190586745480, 113.1239096053143953 ) ) ;
#39740=CARTESIAN_POINT ( 'NONE',  ( 14.29746914071049879, -8.314922557960816363, 23.33224293864769194 ) ) ;
#39741=CARTESIAN_POINT ( 'NONE',  ( -8.224510206698735004, -14.34966873604973081, 34.58442372801900433 ) ) ;
#39742=CARTESIAN_POINT ( 'NONE',  ( -16.51473224551069308, -9.474510206698971260, 31.66557627198102054 ) ) ;
#39743=CARTESIAN_POINT ( 'NONE',  ( -5.153800228976328057, -19.02544592524343514, 67.29057627198102409 ) ) ;
#39745=CARTESIAN_POINT ( 'NONE',  ( 5.153800228976335163, 19.02544592524342804, 114.7905762719810241 ) ) ;
#39746=FACE_OUTER_BOUND ( 'NONE', #94727, .T. ) ;
#39747=CARTESIAN_POINT ( 'NONE',  ( 13.89961937509957401, 13.97604488694547697, 111.8760903946856757 ) ) ;
#39748=CARTESIAN_POINT ( 'NONE',  ( 19.03943276465977164, 0.05219959533936151252, 36.25109039468567573 ) ) ;
#39749=CARTESIAN_POINT ( 'NONE',  ( 15.80617190586746368, 15.72974639402197994, 89.37390960531435269 ) ) ;
#39750=CARTESIAN_POINT ( 'NONE',  ( 12.06949235617757843, -12.14591786802309237, 23.12390960531436335 ) ) ;
#39752=CARTESIAN_POINT ( 'NONE',  ( 5.719274019375991003, -21.55341960407610458, 52.70724293864769550 ) ) ;
#39753=CARTESIAN_POINT ( 'NONE',  ( -21.52544592524343514, 5.823673210054127303, 86.04057627198102409 ) ) ;
#39754=CARTESIAN_POINT ( 'NONE',  ( -19.03943276465977164, -0.05219959533935918106, 108.7510903946856615 ) ) ;
#39755=CARTESIAN_POINT ( 'NONE',  ( -19.03943276465977164, 0.05219959533909376836, 101.2489096053143669 ) ) ;
#39756=CARTESIAN_POINT ( 'NONE',  ( 21.53943276465977519, 0.05219959533937863772, 76.25109039468568994 ) ) ;
#39757=CARTESIAN_POINT ( 'NONE',  ( -13.97604488694527625, -13.89961937509977652, 56.87390960531434558 ) ) ;
#39758=CARTESIAN_POINT ( 'NONE',  ( -16.55341960407611168, -4.379528057220339221, 106.4572429386477097 ) ) ;
#39760=CARTESIAN_POINT ( 'NONE',  ( 5.153800228976335163, 19.02544592524342804, 74.79057627198103830 ) ) ;
#39761=CARTESIAN_POINT ( 'NONE',  ( -0.05219959533910754901, -16.53943276465976808, 92.49890960531436690 ) ) ;
#39763=CARTESIAN_POINT ( 'NONE',  ( -13.97604488694547697, 13.89961937509957934, 93.12609039468566152 ) ) ;
#39765=CARTESIAN_POINT ( 'NONE',  ( 19.02544592524343514, -5.153800228976328945, 63.54057627198103830 ) ) ;
#39766=CARTESIAN_POINT ( 'NONE',  ( 10.72451020669871369, 18.67979575497193778, 87.08442372801901854 ) ) ;
#39767=CARTESIAN_POINT ( 'NONE',  ( 16.51473224551069308, 9.474510206698969483, 99.16557627198102409 ) ) ;
#39768=CARTESIAN_POINT ( 'NONE',  ( 16.52544592524335698, 4.483927247898782831, 76.45942372801901854 ) ) ;
#39769=CARTESIAN_POINT ( 'NONE',  ( -16.36317988757057051, -7.306389748694941844, 50.90210391636774290 ) ) ;
#39770=CARTESIAN_POINT ( 'NONE',  ( 19.03943276465977164, 0.05219959533936151252, 41.25109039468566152 ) ) ;
#39771=CARTESIAN_POINT ( 'NONE',  ( -18.67979575497193778, 10.72451020669871902, 93.33442372801901854 ) ) ;
#39774=CARTESIAN_POINT ( 'NONE',  ( 14.34966873604972726, -8.224510206698740333, 100.8344237280190185 ) ) ;
#39776=CARTESIAN_POINT ( 'NONE',  ( -8.314922557961024197, 14.29746914071037800, 87.91775706135234714 ) ) ;
#39777=CARTESIAN_POINT ( 'NONE',  ( 17.12812012977028076, 6.668231424565952636, 68.85948759323146362 ) ) ;
#39778=CARTESIAN_POINT ( 'NONE',  ( -14.34966873604972548, 8.224510206698743886, 73.33442372801901854 ) ) ;
#39780=CARTESIAN_POINT ( 'NONE',  ( 10.72451020669871369, 18.67979575497193778, 77.08442372801901854 ) ) ;
#39781=CARTESIAN_POINT ( 'NONE',  ( -5.153800228976607833, 19.02544592524334988, 92.70942372801901854 ) ) ;
#39782=CARTESIAN_POINT ( 'NONE',  ( 19.02544592524334988, 5.153800228976608722, 36.45942372801900433 ) ) ;
#39783=CARTESIAN_POINT ( 'NONE',  ( -13.89961937509977652, 13.97604488694528158, 65.62390960531436690 ) ) ;
#39784=CARTESIAN_POINT ( 'NONE',  ( -13.89961937509977652, 13.97604488694528158, 55.62390960531434558 ) ) ;
#39785=LINE ( 'NONE', #159126, #198290 ) ;
#39786=CARTESIAN_POINT ( 'NONE',  ( -5.719274019375978568, 21.55341960407610458, 75.20724293864769550 ) ) ;
#39787=CARTESIAN_POINT ( 'NONE',  ( 21.53943276465977519, -0.05219959533907433946, 33.74890960531436690 ) ) ;
#39788=CARTESIAN_POINT ( 'NONE',  ( -13.89961937509977652, 13.97604488694528158, 30.62390960531435269 ) ) ;
#39789=CARTESIAN_POINT ( 'NONE',  ( -8.314922557961024197, 14.29746914071037800, 62.91775706135236135 ) ) ;
#39792=CARTESIAN_POINT ( 'NONE',  ( 5.719274019375673035, 21.55341960407619339, 27.29275706135234358 ) ) ;
#39793=CARTESIAN_POINT ( 'NONE',  ( -12.06949235617756955, 12.14591786802309770, 70.62390960531436690 ) ) ;
#39795=CARTESIAN_POINT ( 'NONE',  ( 12.06949235617739724, 12.14591786802326823, 21.87609039468567573 ) ) ;
#39796=CARTESIAN_POINT ( 'NONE',  ( 13.97604488694548053, -13.89961937509957401, 50.62609039468566152 ) ) ;
#39797=CARTESIAN_POINT ( 'NONE',  ( -4.483927247898539470, -16.52544592524342804, 62.29057627198102409 ) ) ;
#39798=CARTESIAN_POINT ( 'NONE',  ( 15.80617190586769283, -15.72974639402175789, 35.62609039468568994 ) ) ;
#39799=CARTESIAN_POINT ( 'NONE',  ( -10.72451020669898014, 18.67979575497178502, 75.41557627198102409 ) ) ;
#39800=CARTESIAN_POINT ( 'NONE',  ( -9.474510206698964154, 16.51473224551069663, 105.4155762719810383 ) ) ;
#39801=CARTESIAN_POINT ( 'NONE',  ( -8.224510206698948167, 14.34966873604960824, 55.41557627198102409 ) ) ;
#39802=CARTESIAN_POINT ( 'NONE',  ( 16.51473224551069308, 9.474510206698969483, 114.1655762719810241 ) ) ;
#39804=CARTESIAN_POINT ( 'NONE',  ( -5.153800228976607833, 19.02544592524334988, 72.70942372801900433 ) ) ;
#39805=CARTESIAN_POINT ( 'NONE',  ( -21.55341960407610458, -5.719274019375992779, 106.4572429386477097 ) ) ;
#39806=CARTESIAN_POINT ( 'NONE',  ( -13.97604488694527625, -13.89961937509977652, 61.87390960531435979 ) ) ;
#39807=CARTESIAN_POINT ( 'NONE',  ( 13.89961937509957401, 13.97604488694547697, 46.87609039468565442 ) ) ;
#39808=CARTESIAN_POINT ( 'NONE',  ( -9.564922557960796823, -16.46253265017161027, 27.08224293864769550 ) ) ;
#39810=CARTESIAN_POINT ( 'NONE',  ( -0.05219959533937732626, 21.53943276465977519, 57.50109039468568994 ) ) ;
#39812=CARTESIAN_POINT ( 'NONE',  ( 12.06949235617757843, -12.14591786802309237, 43.12390960531435269 ) ) ;
#39813=CARTESIAN_POINT ( 'NONE',  ( -19.05341960407611168, -5.049401038298163336, 61.45724293864769550 ) ) ;
#39814=CARTESIAN_POINT ( 'NONE',  ( -15.80617190586745835, -15.72974639402198527, 86.87390960531438111 ) ) ;
#39815=CARTESIAN_POINT ( 'NONE',  ( -5.153800228976328057, -19.02544592524343514, 57.29057627198103120 ) ) ;
#39817=CARTESIAN_POINT ( 'NONE',  ( 0.05219959533907565091, 21.53943276465977519, 64.99890960531435269 ) ) ;
#39819=CARTESIAN_POINT ( 'NONE',  ( -15.72974639402176322, -15.80617190586768395, 99.37609039468568994 ) ) ;
#39821=CARTESIAN_POINT ( 'NONE',  ( -8.224510206698735004, -14.34966873604973081, 99.58442372801900433 ) ) ;
#39822=CARTESIAN_POINT ( 'NONE',  ( 8.224510206698953496, -14.34966873604960469, 87.91557627198103830 ) ) ;
#39823=CARTESIAN_POINT ( 'NONE',  ( -16.51473224551082808, 9.474510206698731452, 93.33442372801900433 ) ) ;
#39825=CARTESIAN_POINT ( 'NONE',  ( -16.46253265017146816, -9.564922557961047289, 34.16775706135233293 ) ) ;
#39826=CARTESIAN_POINT ( 'NONE',  ( 16.55341960407618274, -4.379528057220086978, 96.04275706135236135 ) ) ;
#39827=CARTESIAN_POINT ( 'NONE',  ( 16.46253265017146816, 9.564922557961045513, 36.66775706135233293 ) ) ;
#39828=CARTESIAN_POINT ( 'NONE',  ( -9.474510206698964154, 16.51473224551069663, 85.41557627198102409 ) ) ;
#39829=CARTESIAN_POINT ( 'NONE',  ( -10.72451020669898014, 18.67979575497178502, 60.41557627198102409 ) ) ;
#39830=CARTESIAN_POINT ( 'NONE',  ( -9.564922557960796823, -16.46253265017161027, 22.08224293864768839 ) ) ;
#39831=CARTESIAN_POINT ( 'NONE',  ( -19.02544592524342804, 5.153800228976336051, 26.04057627198103120 ) ) ;
#39832=CARTESIAN_POINT ( 'NONE',  ( 5.823673210054444382, -21.52544592524334988, 95.20942372801903275 ) ) ;
#39833=CARTESIAN_POINT ( 'NONE',  ( -16.53943276465976808, -0.05219959533934237506, 78.75109039468568994 ) ) ;
#39834=CARTESIAN_POINT ( 'NONE',  ( 21.53943276465977519, 0.05219959533937863772, 26.25109039468567573 ) ) ;
#39835=CARTESIAN_POINT ( 'NONE',  ( -14.34966873604972548, 8.224510206698743886, 33.33442372801900433 ) ) ;
#39836=CARTESIAN_POINT ( 'NONE',  ( 9.564922557960805705, 16.46253265017160317, 104.5822429386476955 ) ) ;
#39837=CARTESIAN_POINT ( 'NONE',  ( -13.97604488694527625, -13.89961937509977652, 41.87390960531435979 ) ) ;
#39838=CARTESIAN_POINT ( 'NONE',  ( 16.51473224551069308, 9.474510206698969483, 49.16557627198102409 ) ) ;
#39839=CARTESIAN_POINT ( 'NONE',  ( 8.224510206698742110, 14.34966873604972548, 42.08442372801901854 ) ) ;
#39840=CARTESIAN_POINT ( 'NONE',  ( 14.34966873604960469, 8.224510206698951720, 89.16557627198102409 ) ) ;
#39841=CARTESIAN_POINT ( 'NONE',  ( 12.14591786802327356, -12.06949235617739191, 100.6260903946857184 ) ) ;
#39842=CARTESIAN_POINT ( 'NONE',  ( -0.05219959533937732626, 21.53943276465977519, 42.50109039468567573 ) ) ;
#39843=CARTESIAN_POINT ( 'NONE',  ( 16.51473224551069308, 9.474510206698969483, 84.16557627198102409 ) ) ;
#39844=CARTESIAN_POINT ( 'NONE',  ( 9.474510206698971260, -16.51473224551069308, 62.91557627198102409 ) ) ;
#39845=CARTESIAN_POINT ( 'NONE',  ( 16.46253265017160672, -9.564922557960803928, 93.33224293864769550 ) ) ;
#39846=CARTESIAN_POINT ( 'NONE',  ( 4.379528057220339221, -16.55341960407611168, 37.70724293864769550 ) ) ;
#39847=CARTESIAN_POINT ( 'NONE',  ( -12.14591786802326823, 12.06949235617739902, 98.12609039468570415 ) ) ;
#39849=CARTESIAN_POINT ( 'NONE',  ( -5.049401038297874678, -19.05341960407617918, 49.79275706135231871 ) ) ;
#39850=CARTESIAN_POINT ( 'NONE',  ( -0.05219959533909027116, -19.03943276465977164, 112.4989096053143669 ) ) ;
#39851=CARTESIAN_POINT ( 'NONE',  ( 19.05341960407611168, 5.049401038298154454, 63.95724293864769550 ) ) ;
#39852=CARTESIAN_POINT ( 'NONE',  ( 13.97604488694548053, -13.89961937509957401, 35.62609039468567573 ) ) ;
#39854=CARTESIAN_POINT ( 'NONE',  ( 19.36337904590692460, -5.499999999999943157, 72.91494137495618588 ) ) ;
#39855=CARTESIAN_POINT ( 'NONE',  ( 12.14591786802327356, -12.06949235617739191, 45.62609039468567573 ) ) ;
#39856=CARTESIAN_POINT ( 'NONE',  ( 19.02544592524334988, 5.153800228976608722, 76.45942372801897591 ) ) ;
#39857=CARTESIAN_POINT ( 'NONE',  ( -16.55341960407617563, 4.379528057220093196, 53.54275706135234714 ) ) ;
#39858=CARTESIAN_POINT ( 'NONE',  ( 0.05219959533909260263, 19.03943276465977164, 114.9989096053143669 ) ) ;
#39859=CARTESIAN_POINT ( 'NONE',  ( -13.89961937509977652, 13.97604488694528158, 95.62390960531436690 ) ) ;
#39860=CARTESIAN_POINT ( 'NONE',  ( 5.719274019375991003, -21.55341960407610458, 112.7072429386476955 ) ) ;
#39861=CARTESIAN_POINT ( 'NONE',  ( -13.97604488694547697, 13.89961937509957934, 78.12609039468567573 ) ) ;
#39862=CARTESIAN_POINT ( 'NONE',  ( 19.05341960407611168, 5.049401038298154454, 98.95724293864766707 ) ) ;
#39863=CARTESIAN_POINT ( 'NONE',  ( -13.89961937509977652, 13.97604488694528158, 40.62390960531435979 ) ) ;
#39864=CARTESIAN_POINT ( 'NONE',  ( -13.89961937509977652, 13.97604488694528158, 75.62390960531438111 ) ) ;
#39865=CARTESIAN_POINT ( 'NONE',  ( 0.05219959533910956823, 16.53943276465976808, 44.99890960531435979 ) ) ;
#39866=CARTESIAN_POINT ( 'NONE',  ( -9.564922557960796823, -16.46253265017161027, 32.08224293864769550 ) ) ;
#39867=CARTESIAN_POINT ( 'NONE',  ( 16.51473224551083163, -9.474510206698727899, 55.83442372801899722 ) ) ;
#39868=CARTESIAN_POINT ( 'NONE',  ( -8.224510206698948167, 14.34966873604960824, 85.41557627198102409 ) ) ;
#39869=CARTESIAN_POINT ( 'NONE',  ( 18.67979575497194134, -10.72451020669871369, 105.8344237280190328 ) ) ;
#39870=CARTESIAN_POINT ( 'NONE',  ( 13.89961937509977652, -13.97604488694527269, 48.12390960531435979 ) ) ;
#39871=CARTESIAN_POINT ( 'NONE',  ( -21.55341960407610458, -5.719274019375992779, 51.45724293864770260 ) ) ;
#39872=CARTESIAN_POINT ( 'NONE',  ( 12.14591786802309770, 12.06949235617756955, 59.37390960531436690 ) ) ;
#39873=CARTESIAN_POINT ( 'NONE',  ( -5.823673210054431948, 21.52544592524334988, 107.7094237280190328 ) ) ;
#39874=CARTESIAN_POINT ( 'NONE',  ( -9.564922557960796823, -16.46253265017161027, 112.0822429386476955 ) ) ;
#39875=CARTESIAN_POINT ( 'NONE',  ( -5.049401038298153566, 19.05341960407611168, 105.2072429386476671 ) ) ;
#39876=CARTESIAN_POINT ( 'NONE',  ( -19.03943276465977164, 0.05219959533909376836, 41.24890960531435269 ) ) ;
#39877=CARTESIAN_POINT ( 'NONE',  ( 5.153800228976335163, 19.02544592524342804, 29.79057627198102409 ) ) ;
#39878=CARTESIAN_POINT ( 'NONE',  ( 14.29746914071049879, -8.314922557960816363, 83.33224293864769550 ) ) ;
#39879=CARTESIAN_POINT ( 'NONE',  ( -10.81492255796078084, -18.62759615963271287, 97.08224293864770971 ) ) ;
#39880=CARTESIAN_POINT ( 'NONE',  ( -5.153800228976328057, -19.02544592524343514, 107.2905762719810383 ) ) ;
#39881=CARTESIAN_POINT ( 'NONE',  ( 10.81492255796106328, -18.62759615963255655, 20.41775706135234714 ) ) ;
#39882=CARTESIAN_POINT ( 'NONE',  ( -16.51473224551069308, -9.474510206698971260, 101.6655762719810241 ) ) ;
#39883=CARTESIAN_POINT ( 'NONE',  ( 18.22780087662122384, -5.500000000000022204, 66.01540105326107266 ) ) ;
#39884=CARTESIAN_POINT ( 'NONE',  ( 12.14591786802309770, 12.06949235617756955, 109.3739096053143811 ) ) ;
#39885=CARTESIAN_POINT ( 'NONE',  ( -9.564922557960796823, -16.46253265017161027, 72.08224293864770971 ) ) ;
#39886=CARTESIAN_POINT ( 'NONE',  ( -10.81492255796078084, -18.62759615963271287, 77.08224293864769550 ) ) ;
#39889=CARTESIAN_POINT ( 'NONE',  ( 18.67979575497178502, 10.72451020669898547, 24.16557627198103120 ) ) ;
#39890=CARTESIAN_POINT ( 'NONE',  ( 19.46398650005389896, -5.499999999999940492, 67.68269651486370719 ) ) ;
#39891=CARTESIAN_POINT ( 'NONE',  ( 12.14591786802327356, -12.06949235617739191, 30.62609039468567929 ) ) ;
#39892=CARTESIAN_POINT ( 'NONE',  ( 4.379528057220339221, -16.55341960407611168, 97.70724293864772392 ) ) ;
#39893=CARTESIAN_POINT ( 'NONE',  ( 19.35633801406911658, -5.499999999999589662, 51.63373818172766505 ) ) ;
#39894=CARTESIAN_POINT ( 'NONE',  ( -0.05219959533909027116, -19.03943276465977164, 92.49890960531436690 ) ) ;
#39895=CARTESIAN_POINT ( 'NONE',  ( 13.97604488694527802, 13.89961937509977652, 64.37390960531436690 ) ) ;
#39896=CARTESIAN_POINT ( 'NONE',  ( -4.379528057220328563, 16.55341960407611168, 80.20724293864769550 ) ) ;
#39899=CARTESIAN_POINT ( 'NONE',  ( -21.55341960407610458, -5.719274019375992779, 36.45724293864768839 ) ) ;
#39901=CARTESIAN_POINT ( 'NONE',  ( -14.34966873604960291, -8.224510206698953496, 56.66557627198103830 ) ) ;
#39902=CARTESIAN_POINT ( 'NONE',  ( -14.29746914071037622, -8.314922557961029526, 19.16775706135234714 ) ) ;
#39903=CARTESIAN_POINT ( 'NONE',  ( 5.719274019375673035, 21.55341960407619339, 77.29275706135234714 ) ) ;
#39905=CARTESIAN_POINT ( 'NONE',  ( -10.81492255796078084, -18.62759615963271287, 22.08224293864769194 ) ) ;
#39906=CARTESIAN_POINT ( 'NONE',  ( -14.34966873604972548, 8.224510206698743886, 78.33442372801901854 ) ) ;
#39907=CARTESIAN_POINT ( 'NONE',  ( 19.02544592524343514, -5.153800228976328945, 28.54057627198102409 ) ) ;
#39908=CARTESIAN_POINT ( 'NONE',  ( -16.46253265017160317, 9.564922557960807481, 95.83224293864769550 ) ) ;
#39909=CARTESIAN_POINT ( 'NONE',  ( 0.05219959533907565091, 21.53943276465977519, 94.99890960531436690 ) ) ;
#39910=CARTESIAN_POINT ( 'NONE',  ( 12.06949235617739724, 12.14591786802326823, 31.87609039468567929 ) ) ;
#39911=CARTESIAN_POINT ( 'NONE',  ( 16.55341960407611168, 4.379528057220329451, 53.95724293864770260 ) ) ;
#39912=CARTESIAN_POINT ( 'NONE',  ( -0.05219959533937732626, 21.53943276465977519, 67.50109039468568994 ) ) ;
#39913=CARTESIAN_POINT ( 'NONE',  ( -16.53943276465976808, -0.05219959533934237506, 98.75109039468568994 ) ) ;
#39914=CARTESIAN_POINT ( 'NONE',  ( -21.55341960407610458, -5.719274019375992779, 21.45724293864769550 ) ) ;
#39915=CARTESIAN_POINT ( 'NONE',  ( -5.049401038298153566, 19.05341960407611168, 110.2072429386476813 ) ) ;
#39917=CARTESIAN_POINT ( 'NONE',  ( -16.55341960407617563, 4.379528057220093196, 108.5427570613523756 ) ) ;
#39918=CARTESIAN_POINT ( 'NONE',  ( -16.52544592524335698, -4.483927247898792601, 53.95942372801900433 ) ) ;
#39919=CARTESIAN_POINT ( 'NONE',  ( -13.97604488694527625, -13.89961937509977652, 66.87390960531436690 ) ) ;
#39920=CARTESIAN_POINT ( 'NONE',  ( -19.03943276465977164, 0.05219959533909376836, 81.24890960531436690 ) ) ;
#39921=CARTESIAN_POINT ( 'NONE',  ( -5.823673210054431948, 21.52544592524334988, 67.70942372801901854 ) ) ;
#39922=CARTESIAN_POINT ( 'NONE',  ( 8.224510206698742110, 14.34966873604972548, 77.08442372801901854 ) ) ;
#39923=CARTESIAN_POINT ( 'NONE',  ( 8.224510206698953496, -14.34966873604960469, 47.91557627198102409 ) ) ;
#39924=CARTESIAN_POINT ( 'NONE',  ( -19.03943276465977164, 0.05219959533909376836, 56.24890960531435979 ) ) ;
#39925=ORIENTED_EDGE ( 'NONE', *, *, #87651, .F. ) ;
#39926=CARTESIAN_POINT ( 'NONE',  ( 4.483927247898790824, -16.52544592524335698, 20.20942372801900788 ) ) ;
#39927=CARTESIAN_POINT ( 'NONE',  ( -8.224510206698948167, 14.34966873604960824, 105.4155762719810383 ) ) ;
#39928=CARTESIAN_POINT ( 'NONE',  ( 16.51473224551069308, 9.474510206698969483, 74.16557627198103830 ) ) ;
#39929=CARTESIAN_POINT ( 'NONE',  ( 16.46253265017146816, 9.564922557961045513, 96.66775706135233293 ) ) ;
#39931=CARTESIAN_POINT ( 'NONE',  ( -5.823673210054431948, 21.52544592524334988, 97.70942372801904696 ) ) ;
#39932=CARTESIAN_POINT ( 'NONE',  ( -8.224510206698735004, -14.34966873604973081, 74.58442372801901854 ) ) ;
#39933=CARTESIAN_POINT ( 'NONE',  ( 16.51473224551083163, -9.474510206698727899, 90.83442372801900433 ) ) ;
#39934=CARTESIAN_POINT ( 'NONE',  ( -10.81492255796078084, -18.62759615963271287, 57.08224293864769550 ) ) ;
#39935=CARTESIAN_POINT ( 'NONE',  ( -14.29746914071037622, -8.314922557961029526, 54.16775706135235424 ) ) ;
#39937=CARTESIAN_POINT ( 'NONE',  ( 9.474510206698729675, 16.51473224551082808, 57.08442372801900433 ) ) ;
#39938=CARTESIAN_POINT ( 'NONE',  ( 10.72451020669871369, 18.67979575497193778, 92.08442372801901854 ) ) ;
#39939=CARTESIAN_POINT ( 'NONE',  ( -19.05341960407611168, -5.049401038298163336, 31.45724293864769550 ) ) ;
#39940=CARTESIAN_POINT ( 'NONE',  ( -13.89961937509977652, 13.97604488694528158, 70.62390960531432427 ) ) ;
#39941=CARTESIAN_POINT ( 'NONE',  ( -8.224510206698948167, 14.34966873604960824, 55.41557627198102409 ) ) ;
#39942=CARTESIAN_POINT ( 'NONE',  ( 10.72451020669871369, 18.67979575497193778, 92.08442372801901854 ) ) ;
#39943=CARTESIAN_POINT ( 'NONE',  ( -0.05219959533936034679, 19.03943276465977164, 47.50109039468566863 ) ) ;
#39944=CARTESIAN_POINT ( 'NONE',  ( -19.03943276465977164, -0.05219959533935918106, 23.75109039468566152 ) ) ;
#39945=CARTESIAN_POINT ( 'NONE',  ( 0.05219959533909260263, 19.03943276465977164, 114.9989096053143669 ) ) ;
#39946=CARTESIAN_POINT ( 'NONE',  ( -5.719274019375665041, -21.55341960407619695, 99.79275706135234714 ) ) ;
#39947=CARTESIAN_POINT ( 'NONE',  ( -16.46253265017160317, 9.564922557960807481, 75.83224293864769550 ) ) ;
#39948=CARTESIAN_POINT ( 'NONE',  ( 0.05219959533937995610, -21.53943276465977519, 95.00109039468568994 ) ) ;
#39949=CARTESIAN_POINT ( 'NONE',  ( -21.52544592524343514, 5.823673210054127303, 46.04057627198103830 ) ) ;
#39950=CARTESIAN_POINT ( 'NONE',  ( 13.97604488694527802, 13.89961937509977652, 79.37390960531435269 ) ) ;
#39951=CARTESIAN_POINT ( 'NONE',  ( 13.97604488694548053, -13.89961937509957401, 70.62609039468567573 ) ) ;
#39952=CARTESIAN_POINT ( 'NONE',  ( -5.153800228976328057, -19.02544592524343514, 47.29057627198102409 ) ) ;
#39953=CARTESIAN_POINT ( 'NONE',  ( 16.46253265017160672, -9.564922557960803928, 88.33224293864769550 ) ) ;
#39954=CARTESIAN_POINT ( 'NONE',  ( 5.049401038297881783, 19.05341960407617563, 97.29275706135233293 ) ) ;
#39955=CARTESIAN_POINT ( 'NONE',  ( -12.14591786802326823, 12.06949235617739902, 38.12609039468567573 ) ) ;
#39956=CARTESIAN_POINT ( 'NONE',  ( -16.53943276465976808, 0.05219959533911058130, 106.2489096053143811 ) ) ;
#39957=CARTESIAN_POINT ( 'NONE',  ( 19.05341960407611168, 5.049401038298154454, 73.95724293864768129 ) ) ;
#39958=CARTESIAN_POINT ( 'NONE',  ( 21.55341960407610458, 5.719274019375980345, 48.95724293864770971 ) ) ;
#39959=CARTESIAN_POINT ( 'NONE',  ( 12.06949235617739724, 12.14591786802326823, 36.87609039468568994 ) ) ;
#39960=CARTESIAN_POINT ( 'NONE',  ( 18.67979575497194134, -10.72451020669871369, 30.83442372801902209 ) ) ;
#39961=CARTESIAN_POINT ( 'NONE',  ( -0.05219959533937732626, 21.53943276465977519, 82.50109039468568994 ) ) ;
#39962=CARTESIAN_POINT ( 'NONE',  ( -14.34966873604972548, 8.224510206698743886, 88.33442372801901854 ) ) ;
#39963=AXIS2_PLACEMENT_3D ( 'NONE', #83798, #126333, #189027 ) ;
#39964=CARTESIAN_POINT ( 'NONE',  ( -13.89961937509977652, 13.97604488694528158, 80.62390960531436690 ) ) ;
#39965=CARTESIAN_POINT ( 'NONE',  ( 14.34966873604972726, -8.224510206698740333, 105.8344237280190328 ) ) ;
#39966=CARTESIAN_POINT ( 'NONE',  ( 9.474510206698729675, 16.51473224551082808, 57.08442372801900433 ) ) ;
#39967=CARTESIAN_POINT ( 'NONE',  ( 15.80617190586769283, -15.72974639402175789, 35.62609039468568994 ) ) ;
#39968=CARTESIAN_POINT ( 'NONE',  ( 16.55341960407611168, 4.379528057220329451, 83.95724293864770971 ) ) ;
#39969=CARTESIAN_POINT ( 'NONE',  ( -5.153800228976328057, -19.02544592524343514, 102.2905762719810383 ) ) ;
#39970=CARTESIAN_POINT ( 'NONE',  ( -14.29746914071037622, -8.314922557961029526, 109.1677570613523613 ) ) ;
#39971=CARTESIAN_POINT ( 'NONE',  ( -21.52544592524334988, -5.823673210054445271, 68.95942372801901854 ) ) ;
#39972=CARTESIAN_POINT ( 'NONE',  ( -8.224510206698735004, -14.34966873604973081, 39.58442372801901143 ) ) ;
#39973=CARTESIAN_POINT ( 'NONE',  ( -21.52544592524334988, -5.823673210054445271, 33.95942372801901143 ) ) ;
#39974=CARTESIAN_POINT ( 'NONE',  ( -16.52544592524342804, 4.483927247898546575, 71.04057627198103830 ) ) ;
#39976=CARTESIAN_POINT ( 'NONE',  ( -15.72974639402197994, 15.80617190586746368, 110.6239096053143669 ) ) ;
#39977=CARTESIAN_POINT ( 'NONE',  ( -12.14591786802309592, -12.06949235617757132, 51.87390960531437401 ) ) ;
#39978=CARTESIAN_POINT ( 'NONE',  ( -13.89961937509977652, 13.97604488694528158, 25.62390960531434558 ) ) ;
#39979=CARTESIAN_POINT ( 'NONE',  ( -5.719274019375978568, 21.55341960407610458, 35.20724293864768839 ) ) ;
#39980=CARTESIAN_POINT ( 'NONE',  ( -12.06949235617756955, 12.14591786802309770, 60.62390960531437401 ) ) ;
#39981=CARTESIAN_POINT ( 'NONE',  ( -15.80617190586745835, -15.72974639402198527, 81.87390960531435269 ) ) ;
#39982=CARTESIAN_POINT ( 'NONE',  ( -19.03943276465977164, 0.05219959533909376836, 76.24890960531435269 ) ) ;
#39983=CARTESIAN_POINT ( 'NONE',  ( 9.474510206698971260, -16.51473224551069308, 37.91557627198102409 ) ) ;
#39984=CARTESIAN_POINT ( 'NONE',  ( -9.474510206698720793, -16.51473224551083518, 79.58442372801899012 ) ) ;
#39986=CARTESIAN_POINT ( 'NONE',  ( 18.67979575497194134, -10.72451020669871369, 60.83442372801901854 ) ) ;
#39987=CARTESIAN_POINT ( 'NONE',  ( 21.52544592524344225, -5.823673210054117533, 63.54057627198103830 ) ) ;
#39988=CARTESIAN_POINT ( 'NONE',  ( 0.05219959533909260263, 19.03943276465977164, 44.99890960531435979 ) ) ;
#39989=CARTESIAN_POINT ( 'NONE',  ( -0.05219959533909027116, -19.03943276465977164, 67.49890960531436690 ) ) ;
#39991=CARTESIAN_POINT ( 'NONE',  ( -14.34966873604972548, 8.224510206698743886, 48.33442372801902565 ) ) ;
#39992=CARTESIAN_POINT ( 'NONE',  ( 5.823673210054444382, -21.52544592524334988, 35.20942372801901854 ) ) ;
#39993=CARTESIAN_POINT ( 'NONE',  ( 15.72974639402176855, 15.80617190586768217, 56.87609039468568994 ) ) ;
#39994=CARTESIAN_POINT ( 'NONE',  ( 16.51473224551069308, 9.474510206698969483, 104.1655762719810241 ) ) ;
#39995=CARTESIAN_POINT ( 'NONE',  ( -15.72974639402197994, 15.80617190586746368, 80.62390960531438111 ) ) ;
#39996=CARTESIAN_POINT ( 'NONE',  ( 0.05219959533937995610, -21.53943276465977519, 25.00109039468567218 ) ) ;
#39997=CARTESIAN_POINT ( 'NONE',  ( -4.483927247898782831, 16.52544592524335698, 57.70942372801901143 ) ) ;
#39998=CARTESIAN_POINT ( 'NONE',  ( 15.80617190586746368, 15.72974639402197994, 44.37390960531435979 ) ) ;
#39999=CARTESIAN_POINT ( 'NONE',  ( 5.719274019375673035, 21.55341960407619339, 112.2927570613523471 ) ) ;
#40000=CARTESIAN_POINT ( 'NONE',  ( 19.03943276465977164, -0.05219959533909143690, 48.74890960531435979 ) ) ;
#40001=CARTESIAN_POINT ( 'NONE',  ( -9.564922557960796823, -16.46253265017161027, 107.0822429386476955 ) ) ;
#40002=CARTESIAN_POINT ( 'NONE',  ( -5.049401038298153566, 19.05341960407611168, 85.20724293864766707 ) ) ;
#40004=CARTESIAN_POINT ( 'NONE',  ( -19.05341960407617563, 5.049401038297882671, 68.54275706135230450 ) ) ;
#40005=CARTESIAN_POINT ( 'NONE',  ( 0.05219959533907565091, 21.53943276465977519, 49.99890960531437401 ) ) ;
#40006=CARTESIAN_POINT ( 'NONE',  ( -8.314922557960811034, -14.29746914071050412, 27.08224293864769550 ) ) ;
#40007=CARTESIAN_POINT ( 'NONE',  ( 19.05341960407617918, -5.049401038297876454, 86.04275706135233293 ) ) ;
#40009=CARTESIAN_POINT ( 'NONE',  ( 15.80617190586769283, -15.72974639402175789, 110.6260903946857042 ) ) ;
#40010=CARTESIAN_POINT ( 'NONE',  ( 16.46253265017146816, 9.564922557961045513, 101.6677570613523329 ) ) ;
#40011=CARTESIAN_POINT ( 'NONE',  ( -19.02544592524334988, -5.153800228976617603, 48.95942372801900433 ) ) ;
#40012=CARTESIAN_POINT ( 'NONE',  ( 16.21995358207305671, 7.366697692864192959, 107.5644899848784206 ) ) ;
#40013=CARTESIAN_POINT ( 'NONE',  ( 9.564922557960805705, 16.46253265017160317, 49.58224293864770260 ) ) ;
#40014=CARTESIAN_POINT ( 'NONE',  ( -12.06949235617756955, 12.14591786802309770, 55.62390960531436690 ) ) ;
#40015=CARTESIAN_POINT ( 'NONE',  ( -16.46253265017160317, 9.564922557960807481, 30.83224293864769550 ) ) ;
#40016=CARTESIAN_POINT ( 'NONE',  ( 16.55341960407611168, 4.379528057220329451, 33.95724293864769550 ) ) ;
#40018=CARTESIAN_POINT ( 'NONE',  ( 16.53943276465976808, 0.05219959533934440121, 111.2510903946856899 ) ) ;
#40019=CARTESIAN_POINT ( 'NONE',  ( 19.05341960407611168, 5.049401038298154454, 68.95724293864769550 ) ) ;
#40020=CARTESIAN_POINT ( 'NONE',  ( -19.03943276465977164, -0.05219959533935918106, 28.75109039468566507 ) ) ;
#40021=CARTESIAN_POINT ( 'NONE',  ( 8.224510206698742110, 14.34966873604972548, 32.08442372801901854 ) ) ;
#40022=CARTESIAN_POINT ( 'NONE',  ( -5.823673210054116645, -21.52544592524344225, 37.29057627198102409 ) ) ;
#40023=CARTESIAN_POINT ( 'NONE',  ( 10.72451020669871369, 18.67979575497193778, 102.0844237280190185 ) ) ;
#40024=CARTESIAN_POINT ( 'NONE',  ( -13.89961937509977652, 13.97604488694528158, 65.62390960531436690 ) ) ;
#40025=CARTESIAN_POINT ( 'NONE',  ( -13.97604488694527625, -13.89961937509977652, 111.8739096053143243 ) ) ;
#40026=CARTESIAN_POINT ( 'NONE',  ( 19.02544592524343514, -5.153800228976328945, 103.5405762719809957 ) ) ;
#40028=CARTESIAN_POINT ( 'NONE',  ( -5.823673210054431948, 21.52544592524334988, 22.70942372801901499 ) ) ;
#40029=CARTESIAN_POINT ( 'NONE',  ( 8.314922557960818139, 14.29746914071049879, 89.58224293864768129 ) ) ;
#40030=CARTESIAN_POINT ( 'NONE',  ( -5.719274019375978568, 21.55341960407610458, 80.20724293864769550 ) ) ;
#40031=CARTESIAN_POINT ( 'NONE',  ( 0.05219959533909260263, 19.03943276465977164, 64.99890960531436690 ) ) ;
#40032=CARTESIAN_POINT ( 'NONE',  ( -19.05341960407611168, -5.049401038298163336, 76.45724293864769550 ) ) ;
#40033=CARTESIAN_POINT ( 'NONE',  ( 5.719274019375991003, -21.55341960407610458, 112.7072429386476955 ) ) ;
#40034=ORIENTED_EDGE ( 'NONE', *, *, #178675, .F. ) ;
#40035=CARTESIAN_POINT ( 'NONE',  ( -9.564922557960796823, -16.46253265017161027, 77.08224293864769550 ) ) ;
#40038=CARTESIAN_POINT ( 'NONE',  ( 16.52544592524342804, -4.483927247898539470, 108.5405762719810241 ) ) ;
#40039=CARTESIAN_POINT ( 'NONE',  ( 13.89961937509977652, -13.97604488694527269, 23.12390960531436335 ) ) ;
#40040=CARTESIAN_POINT ( 'NONE',  ( 0.05219959533909260263, 19.03943276465977164, 69.99890960531435269 ) ) ;
#40041=CARTESIAN_POINT ( 'NONE',  ( 9.474510206698729675, 16.51473224551082808, 92.08442372801900433 ) ) ;
#40042=CARTESIAN_POINT ( 'NONE',  ( 12.14591786802309770, 12.06949235617756955, 104.3739096053143669 ) ) ;
#40043=CARTESIAN_POINT ( 'NONE',  ( 5.719274019375673035, 21.55341960407619339, 67.29275706135234714 ) ) ;
#40044=CARTESIAN_POINT ( 'NONE',  ( 13.97604488694527802, 13.89961937509977652, 49.37390960531434558 ) ) ;
#40045=CARTESIAN_POINT ( 'NONE',  ( 10.81492255796106328, -18.62759615963255655, 25.41775706135235779 ) ) ;
#40046=CARTESIAN_POINT ( 'NONE',  ( -15.80617190586745835, -15.72974639402198527, 106.8739096053143811 ) ) ;
#40048=CARTESIAN_POINT ( 'NONE',  ( 5.049401038298161559, -19.05341960407611168, 77.70724293864765286 ) ) ;
#40049=CARTESIAN_POINT ( 'NONE',  ( -0.05219959533936034679, 19.03943276465977164, 102.5010903946856757 ) ) ;
#40050=CARTESIAN_POINT ( 'NONE',  ( 10.81492255796078972, 18.62759615963270932, 34.58224293864770260 ) ) ;
#40051=CARTESIAN_POINT ( 'NONE',  ( 0.05219959533937995610, -21.53943276465977519, 65.00109039468568994 ) ) ;
#40052=CARTESIAN_POINT ( 'NONE',  ( -19.03943276465977164, 0.05219959533909376836, 101.2489096053143669 ) ) ;
#40053=CARTESIAN_POINT ( 'NONE',  ( -5.153800228976607833, 19.02544592524334988, 87.70942372801897591 ) ) ;
#40054=CARTESIAN_POINT ( 'NONE',  ( -5.049401038298153566, 19.05341960407611168, 45.20724293864769550 ) ) ;
#40055=CARTESIAN_POINT ( 'NONE',  ( 0.05219959533909260263, 19.03943276465977164, 74.99890960531435269 ) ) ;
#40056=CARTESIAN_POINT ( 'NONE',  ( 16.52544592524342804, -4.483927247898539470, 78.54057627198103830 ) ) ;
#40057=CARTESIAN_POINT ( 'NONE',  ( 19.05341960407611168, 5.049401038298154454, 108.9572429386477097 ) ) ;
#40058=CARTESIAN_POINT ( 'NONE',  ( 8.224510206698953496, -14.34966873604960469, 92.91557627198103830 ) ) ;
#40059=CARTESIAN_POINT ( 'NONE',  ( -13.89961937509977652, 13.97604488694528158, 95.62390960531436690 ) ) ;
#40060=CARTESIAN_POINT ( 'NONE',  ( -14.29746914071049879, 8.314922557960819915, 45.83224293864769550 ) ) ;
#40061=CARTESIAN_POINT ( 'NONE',  ( 13.97604488694527802, 13.89961937509977652, 34.37390960531436690 ) ) ;
#40062=ORIENTED_EDGE ( 'NONE', *, *, #173531, .T. ) ;
#40063=CARTESIAN_POINT ( 'NONE',  ( -21.53943276465977519, -0.05219959533937600094, 58.75109039468568994 ) ) ;
#40064=CARTESIAN_POINT ( 'NONE',  ( -19.02544592524334988, -5.153800228976617603, 73.95942372801900433 ) ) ;
#40065=CARTESIAN_POINT ( 'NONE',  ( 12.06949235617757843, -12.14591786802309237, 43.12390960531435269 ) ) ;
#40066=CARTESIAN_POINT ( 'NONE',  ( 21.52544592524344225, -5.823673210054117533, 93.54057627198103830 ) ) ;
#40067=CARTESIAN_POINT ( 'NONE',  ( 5.823673210054125526, 21.52544592524343514, 34.79057627198103120 ) ) ;
#40068=CARTESIAN_POINT ( 'NONE',  ( 4.483927247898545687, 16.52544592524342804, 84.79057627198102409 ) ) ;
#40069=CARTESIAN_POINT ( 'NONE',  ( 16.46253265017160672, -9.564922557960803928, 58.33224293864769550 ) ) ;
#40070=CARTESIAN_POINT ( 'NONE',  ( 16.53943276465976808, -0.05219959533910856209, 28.74890960531435624 ) ) ;
#40071=CARTESIAN_POINT ( 'NONE',  ( -12.06949235617739369, -12.14591786802326823, 104.3760903946856899 ) ) ;
#40072=CARTESIAN_POINT ( 'NONE',  ( -16.55341960407617563, 4.379528057220093196, 68.54275706135234714 ) ) ;
#40073=CARTESIAN_POINT ( 'NONE',  ( -5.049401038297874678, -19.05341960407617918, 29.79275706135232227 ) ) ;
#40074=CARTESIAN_POINT ( 'NONE',  ( 19.02544592524343514, -5.153800228976328945, 103.5405762719809957 ) ) ;
#40075=CARTESIAN_POINT ( 'NONE',  ( -19.05341960407611168, -5.049401038298163336, 76.45724293864769550 ) ) ;
#40076=CARTESIAN_POINT ( 'NONE',  ( 13.89961937509977652, -13.97604488694527269, 33.12390960531434558 ) ) ;
#40077=CARTESIAN_POINT ( 'NONE',  ( 8.314922557960818139, 14.29746914071049879, 44.58224293864769550 ) ) ;
#40078=CARTESIAN_POINT ( 'NONE',  ( -13.97604488694527625, -13.89961937509977652, 111.8739096053143243 ) ) ;
#40079=CARTESIAN_POINT ( 'NONE',  ( 0.05219959533909260263, 19.03943276465977164, 99.99890960531436690 ) ) ;
#40080=CARTESIAN_POINT ( 'NONE',  ( -18.67979575497178146, -10.72451020669898902, 36.66557627198103120 ) ) ;
#40081=CARTESIAN_POINT ( 'NONE',  ( -14.29746914071049879, 8.314922557960819915, 70.83224293864770971 ) ) ;
#40082=CARTESIAN_POINT ( 'NONE',  ( 14.34966873604972726, -8.224510206698740333, 20.83442372801901143 ) ) ;
#40083=CARTESIAN_POINT ( 'NONE',  ( -8.224510206698948167, 14.34966873604960824, 65.41557627198102409 ) ) ;
#40086=CARTESIAN_POINT ( 'NONE',  ( -19.03943276465977164, -0.05219959533935918106, 58.75109039468566863 ) ) ;
#40087=CARTESIAN_POINT ( 'NONE',  ( -16.46253265017160317, 9.564922557960807481, 100.8322429386477097 ) ) ;
#40088=CARTESIAN_POINT ( 'NONE',  ( 13.97604488694548053, -13.89961937509957401, 80.62609039468567573 ) ) ;
#40089=CARTESIAN_POINT ( 'NONE',  ( -9.474510206698720793, -16.51473224551083518, 39.58442372801899722 ) ) ;
#40090=CARTESIAN_POINT ( 'NONE',  ( 9.474510206698729675, 16.51473224551082808, 107.0844237280190043 ) ) ;
#40091=CARTESIAN_POINT ( 'NONE',  ( -16.55341960407617563, 4.379528057220093196, 93.54275706135234714 ) ) ;
#40092=CARTESIAN_POINT ( 'NONE',  ( 16.51473224551069308, 9.474510206698969483, 44.16557627198103120 ) ) ;
#40093=CARTESIAN_POINT ( 'NONE',  ( 15.80617190586746368, 15.72974639402197994, 34.37390960531435979 ) ) ;
#40094=CARTESIAN_POINT ( 'NONE',  ( -10.72451020669870658, -18.67979575497194134, 49.58442372801901143 ) ) ;
#40096=CARTESIAN_POINT ( 'NONE',  ( 16.52544592524335698, 4.483927247898782831, 21.45942372801901499 ) ) ;
#40098=CARTESIAN_POINT ( 'NONE',  ( 16.51473224551069308, 9.474510206698969483, 79.16557627198103830 ) ) ;
#40100=CARTESIAN_POINT ( 'NONE',  ( -16.55341960407611168, -4.379528057220339221, 86.45724293864770971 ) ) ;
#40101=CARTESIAN_POINT ( 'NONE',  ( -9.564922557960796823, -16.46253265017161027, 72.08224293864770971 ) ) ;
#40102=CARTESIAN_POINT ( 'NONE',  ( -19.05341960407611168, -5.049401038298163336, 81.45724293864769550 ) ) ;
#40104=CARTESIAN_POINT ( 'NONE',  ( -5.049401038297874678, -19.05341960407617918, 94.79275706135230450 ) ) ;
#40105=CARTESIAN_POINT ( 'NONE',  ( -18.67979575497178146, -10.72451020669898902, 61.66557627198103120 ) ) ;
#40106=CARTESIAN_POINT ( 'NONE',  ( 19.02544592524343514, -5.153800228976328945, 23.54057627198102054 ) ) ;
#40107=CARTESIAN_POINT ( 'NONE',  ( -5.049401038297874678, -19.05341960407617918, 59.79275706135231871 ) ) ;
#40108=CARTESIAN_POINT ( 'NONE',  ( 19.05341960407611168, 5.049401038298154454, 58.95724293864768129 ) ) ;
#40109=CARTESIAN_POINT ( 'NONE',  ( -16.51473224551069308, -9.474510206698971260, 91.66557627198103830 ) ) ;
#40110=ORIENTED_EDGE ( 'NONE', *, *, #19257, .T. ) ;
#40111=CARTESIAN_POINT ( 'NONE',  ( -5.719274019375978568, 21.55341960407610458, 95.20724293864769550 ) ) ;
#40112=CARTESIAN_POINT ( 'NONE',  ( -4.379528057220328563, 16.55341960407611168, 95.20724293864769550 ) ) ;
#40113=CARTESIAN_POINT ( 'NONE',  ( 19.05341960407617918, -5.049401038297876454, 61.04275706135232582 ) ) ;
#40114=CARTESIAN_POINT ( 'NONE',  ( -21.55341960407610458, -5.719274019375992779, 91.45724293864769550 ) ) ;
#40115=CARTESIAN_POINT ( 'NONE',  ( -21.52544592524343514, 5.823673210054127303, 71.04057627198103830 ) ) ;
#40116=CARTESIAN_POINT ( 'NONE',  ( 14.29746914071049879, -8.314922557960816363, 28.33224293864769550 ) ) ;
#40117=CARTESIAN_POINT ( 'NONE',  ( -10.81492255796105439, 18.62759615963255655, 107.9177570613523471 ) ) ;
#40118=CARTESIAN_POINT ( 'NONE',  ( 16.53943276465976808, 0.05219959533934440121, 51.25109039468568994 ) ) ;
#40119=CARTESIAN_POINT ( 'NONE',  ( 9.564922557960805705, 16.46253265017160317, 79.58224293864769550 ) ) ;
#40120=CARTESIAN_POINT ( 'NONE',  ( -9.564922557960796823, -16.46253265017161027, 37.08224293864768839 ) ) ;
#40122=CARTESIAN_POINT ( 'NONE',  ( -15.72974639402176322, -15.80617190586768395, 39.37609039468567573 ) ) ;
#40123=CARTESIAN_POINT ( 'NONE',  ( -15.72974639402176322, -15.80617190586768395, 54.37609039468568994 ) ) ;
#40124=CARTESIAN_POINT ( 'NONE',  ( 9.474510206698971260, -16.51473224551069308, 42.91557627198103120 ) ) ;
#40125=CARTESIAN_POINT ( 'NONE',  ( 15.72974639402176855, 15.80617190586768217, 26.87609039468567218 ) ) ;
#40126=CARTESIAN_POINT ( 'NONE',  ( -16.46253265017146816, -9.564922557961047289, 64.16775706135233293 ) ) ;
#40127=CARTESIAN_POINT ( 'NONE',  ( -16.46253265017146816, -9.564922557961047289, 69.16775706135233293 ) ) ;
#40128=CARTESIAN_POINT ( 'NONE',  ( -0.05219959533934338120, 16.53943276465976808, 32.50109039468568284 ) ) ;
#40129=CARTESIAN_POINT ( 'NONE',  ( -5.153800228976328057, -19.02544592524343514, 22.29057627198102765 ) ) ;
#40130=CARTESIAN_POINT ( 'NONE',  ( 16.53943276465976808, 0.05219959533934440121, 71.25109039468568994 ) ) ;
#40131=CARTESIAN_POINT ( 'NONE',  ( -5.153800228976328057, -19.02544592524343514, 42.29057627198101699 ) ) ;
#40133=CARTESIAN_POINT ( 'NONE',  ( -0.05219959533909027116, -19.03943276465977164, 92.49890960531436690 ) ) ;
#40134=CARTESIAN_POINT ( 'NONE',  ( 13.89961937509977652, -13.97604488694527269, 28.12390960531435624 ) ) ;
#40136=CARTESIAN_POINT ( 'NONE',  ( -18.67979575497178146, -10.72451020669898902, 76.66557627198103830 ) ) ;
#40137=CARTESIAN_POINT ( 'NONE',  ( -4.483927247898782831, 16.52544592524335698, 62.70942372801902565 ) ) ;
#40138=CARTESIAN_POINT ( 'NONE',  ( -18.67979575497193778, 10.72451020669871902, 113.3344237280190328 ) ) ;
#40139=CARTESIAN_POINT ( 'NONE',  ( 16.51473224551069308, 9.474510206698969483, 54.16557627198103120 ) ) ;
#40140=CARTESIAN_POINT ( 'NONE',  ( 14.34966873604960469, 8.224510206698951720, 29.16557627198103120 ) ) ;
#40141=CARTESIAN_POINT ( 'NONE',  ( -4.379528057220328563, 16.55341960407611168, 65.20724293864768129 ) ) ;
#40142=CARTESIAN_POINT ( 'NONE',  ( 19.05341960407611168, 5.049401038298154454, 73.95724293864768129 ) ) ;
#40143=CARTESIAN_POINT ( 'NONE',  ( 21.53943276465977519, 0.05219959533937863772, 41.25109039468568284 ) ) ;
#40144=CARTESIAN_POINT ( 'NONE',  ( 9.474510206698971260, -16.51473224551069308, 82.91557627198103830 ) ) ;
#40145=CARTESIAN_POINT ( 'NONE',  ( 15.80617190586769283, -15.72974639402175789, 80.62609039468567573 ) ) ;
#40146=CARTESIAN_POINT ( 'NONE',  ( 4.483927247898790824, -16.52544592524335698, 60.20942372801902565 ) ) ;
#40147=CARTESIAN_POINT ( 'NONE',  ( 5.153800228976335163, 19.02544592524342804, 114.7905762719810241 ) ) ;
#40148=CARTESIAN_POINT ( 'NONE',  ( 5.719274019375991003, -21.55341960407610458, 87.70724293864769550 ) ) ;
#40150=CARTESIAN_POINT ( 'NONE',  ( -8.224510206698948167, 14.34966873604960824, 50.41557627198103120 ) ) ;
#40151=CARTESIAN_POINT ( 'NONE',  ( 16.46253265017160672, -9.564922557960803928, 28.33224293864769550 ) ) ;
#40152=CARTESIAN_POINT ( 'NONE',  ( 8.314922557961029526, -14.29746914071037800, 55.41775706135234714 ) ) ;
#40153=CARTESIAN_POINT ( 'NONE',  ( -12.14591786802309592, -12.06949235617757132, 51.87390960531437401 ) ) ;
#40154=CARTESIAN_POINT ( 'NONE',  ( -15.80617190586745835, -15.72974639402198527, 21.87390960531436690 ) ) ;
#40155=CARTESIAN_POINT ( 'NONE',  ( -5.719274019375978568, 21.55341960407610458, 35.20724293864768839 ) ) ;
#40156=CARTESIAN_POINT ( 'NONE',  ( -10.72451020669870658, -18.67979575497194134, 109.5844237280190328 ) ) ;
#40157=CARTESIAN_POINT ( 'NONE',  ( 12.06949235617757843, -12.14591786802309237, 98.12390960531436690 ) ) ;
#40158=CARTESIAN_POINT ( 'NONE',  ( 19.05341960407611168, 5.049401038298154454, 93.95724293864769550 ) ) ;
#40160=CARTESIAN_POINT ( 'NONE',  ( -8.224510206698735004, -14.34966873604973081, 49.58442372801901143 ) ) ;
#40161=CARTESIAN_POINT ( 'NONE',  ( 5.153800228976335163, 19.02544592524342804, 54.79057627198103120 ) ) ;
#40162=CYLINDRICAL_SURFACE ( 'NONE', #143697, 2.500000000000002220 ) ;
#40163=CARTESIAN_POINT ( 'NONE',  ( -9.474510206698720793, -16.51473224551083518, 44.58442372801900433 ) ) ;
#40164=CARTESIAN_POINT ( 'NONE',  ( -16.55341960407617563, 4.379528057220093196, 98.54275706135234714 ) ) ;
#40165=CARTESIAN_POINT ( 'NONE',  ( -5.153800228976607833, 19.02544592524334988, 97.70942372801900433 ) ) ;
#40166=CARTESIAN_POINT ( 'NONE',  ( 18.67979575497194134, -10.72451020669871369, 60.83442372801901854 ) ) ;
#40167=CARTESIAN_POINT ( 'NONE',  ( 13.89961937509977652, -13.97604488694527269, 73.12390960531436690 ) ) ;
#40168=CARTESIAN_POINT ( 'NONE',  ( 21.53943276465977519, -0.05219959533907433946, 88.74890960531436690 ) ) ;
#40169=CARTESIAN_POINT ( 'NONE',  ( -14.29746914071049879, 8.314922557960819915, 105.8322429386476955 ) ) ;
#40170=CARTESIAN_POINT ( 'NONE',  ( 13.97604488694548053, -13.89961937509957401, 75.62609039468564731 ) ) ;
#40171=CARTESIAN_POINT ( 'NONE',  ( -15.72974639402197994, 15.80617190586746368, 80.62390960531438111 ) ) ;
#40172=CARTESIAN_POINT ( 'NONE',  ( 13.89961937509957401, 13.97604488694547697, 36.87609039468565442 ) ) ;
#40173=CARTESIAN_POINT ( 'NONE',  ( 19.25176906914649066, 5.499999999999787725, 98.49927264242275271 ) ) ;
#40174=CARTESIAN_POINT ( 'NONE',  ( -10.81492255796078084, -18.62759615963271287, 87.08224293864769550 ) ) ;
#40175=CARTESIAN_POINT ( 'NONE',  ( -19.53037848336980886, 5.499999999999903189, 54.85532783611443364 ) ) ;
#40176=CARTESIAN_POINT ( 'NONE',  ( -9.474510206698964154, 16.51473224551069663, 65.41557627198102409 ) ) ;
#40177=CARTESIAN_POINT ( 'NONE',  ( -17.60691670004652210, -5.499999999999992006, 89.13333313366439370 ) ) ;
#40178=CARTESIAN_POINT ( 'NONE',  ( 12.14591786802327356, -12.06949235617739191, 20.62609039468568639 ) ) ;
#40179=CARTESIAN_POINT ( 'NONE',  ( -18.22780087662119541, 5.500000000000102141, 66.01763182126894947 ) ) ;
#40180=CARTESIAN_POINT ( 'NONE',  ( 5.049401038298161559, -19.05341960407611168, 42.70724293864767418 ) ) ;
#40181=CARTESIAN_POINT ( 'NONE',  ( 16.46253265017160672, -9.564922557960803928, 108.3322429386476955 ) ) ;
#40182=CARTESIAN_POINT ( 'NONE',  ( 10.81492255796078972, 18.62759615963270932, 104.5822429386477097 ) ) ;
#40183=CARTESIAN_POINT ( 'NONE',  ( 12.06949235617757843, -12.14591786802309237, 53.12390960531436690 ) ) ;
#40184=CARTESIAN_POINT ( 'NONE',  ( 18.62759615963255655, 10.81492255796105972, 71.66775706135234714 ) ) ;
#40185=CARTESIAN_POINT ( 'NONE',  ( 14.34966873604972726, -8.224510206698740333, 20.83442372801901143 ) ) ;
#40186=CARTESIAN_POINT ( 'NONE',  ( 0.05219959533936267826, -19.03943276465977164, 35.00109039468566863 ) ) ;
#40187=CARTESIAN_POINT ( 'NONE',  ( -14.34966873604960291, -8.224510206698953496, 31.66557627198102054 ) ) ;
#40188=CARTESIAN_POINT ( 'NONE',  ( -21.55341960407610458, -5.719274019375992779, 111.4572429386476813 ) ) ;
#40189=CARTESIAN_POINT ( 'NONE',  ( -4.483927247898539470, -16.52544592524342804, 47.29057627198103120 ) ) ;
#40190=CARTESIAN_POINT ( 'NONE',  ( 9.474510206698729675, 16.51473224551082808, 92.08442372801900433 ) ) ;
#40191=CARTESIAN_POINT ( 'NONE',  ( 9.474510206698729675, 16.51473224551082808, 67.08442372801900433 ) ) ;
#40192=CARTESIAN_POINT ( 'NONE',  ( 10.81492255796106328, -18.62759615963255655, 65.41775706135234714 ) ) ;
#40193=B_SPLINE_CURVE_WITH_KNOTS ( 'NONE', 3,
 ( #571, #102058, #92587, #15766, #76434, #61259 ),
 .UNSPECIFIED., .F., .F.,
 ( 4, 2, 4 ),
 ( 0.003989672132298113100, 0.004372778065220548488, 0.004755883998142983876 ),
 .UNSPECIFIED. ) ;
#40194=CARTESIAN_POINT ( 'NONE',  ( -16.51473224551082808, 9.474510206698731452, 48.33442372801900433 ) ) ;
#40195=CARTESIAN_POINT ( 'NONE',  ( 0.05219959533909260263, 19.03943276465977164, 29.99890960531435979 ) ) ;
#40196=CARTESIAN_POINT ( 'NONE',  ( 10.72451020669898902, -18.67979575497178502, 47.91557627198102409 ) ) ;
#40197=CARTESIAN_POINT ( 'NONE',  ( 0.05219959533910956823, 16.53943276465976808, 44.99890960531435979 ) ) ;
#40198=CARTESIAN_POINT ( 'NONE',  ( -17.48853670773243607, -5.747243402303084281, 26.33328700250008936 ) ) ;
#40199=CARTESIAN_POINT ( 'NONE',  ( -10.81492255796105439, 18.62759615963255655, 112.9177570613523329 ) ) ;
#40200=CARTESIAN_POINT ( 'NONE',  ( -12.14591786802326823, 12.06949235617739902, 88.12609039468570415 ) ) ;
#40201=CARTESIAN_POINT ( 'NONE',  ( 16.53943276465976808, -0.05219959533910856209, 33.74890960531436690 ) ) ;
#40202=CARTESIAN_POINT ( 'NONE',  ( -10.81492255796105439, 18.62759615963255655, 77.91775706135231871 ) ) ;
#40203=CARTESIAN_POINT ( 'NONE',  ( 18.67979575497194134, -10.72451020669871369, 85.83442372801901854 ) ) ;
#40204=CARTESIAN_POINT ( 'NONE',  ( -21.55341960407610458, -5.719274019375992779, 86.45724293864770971 ) ) ;
#40206=CARTESIAN_POINT ( 'NONE',  ( -0.05219959533909027116, -19.03943276465977164, 42.49890960531435269 ) ) ;
#40207=CARTESIAN_POINT ( 'NONE',  ( 10.81492255796106328, -18.62759615963255655, 60.41775706135235424 ) ) ;
#40208=CARTESIAN_POINT ( 'NONE',  ( 16.51473224551069308, 9.474510206698969483, 34.16557627198102409 ) ) ;
#40209=CARTESIAN_POINT ( 'NONE',  ( 19.03943276465977164, -0.05219959533909143690, 53.74890960531436690 ) ) ;
#40210=CARTESIAN_POINT ( 'NONE',  ( -8.314922557960811034, -14.29746914071050412, 92.08224293864769550 ) ) ;
#40211=CARTESIAN_POINT ( 'NONE',  ( -5.153800228976328057, -19.02544592524343514, 102.2905762719810383 ) ) ;
#40212=CARTESIAN_POINT ( 'NONE',  ( 8.224510206698953496, -14.34966873604960469, 37.91557627198102409 ) ) ;
#40213=CARTESIAN_POINT ( 'NONE',  ( -19.05341960407611168, -5.049401038298163336, 21.45724293864768839 ) ) ;
#40214=CARTESIAN_POINT ( 'NONE',  ( 10.72451020669898902, -18.67979575497178502, 67.91557627198102409 ) ) ;
#40215=CARTESIAN_POINT ( 'NONE',  ( 10.72451020669871369, 18.67979575497193778, 22.08442372801901143 ) ) ;
#40217=CARTESIAN_POINT ( 'NONE',  ( -19.03943276465977164, 0.05219959533909376836, 76.24890960531435269 ) ) ;
#40218=CARTESIAN_POINT ( 'NONE',  ( -13.97604488694547697, 13.89961937509957934, 113.1260903946856757 ) ) ;
#40220=CARTESIAN_POINT ( 'NONE',  ( -10.81492255796078084, -18.62759615963271287, 67.08224293864770971 ) ) ;
#40222=CARTESIAN_POINT ( 'NONE',  ( 10.72451020669871369, 18.67979575497193778, 97.08442372801904696 ) ) ;
#40223=CARTESIAN_POINT ( 'NONE',  ( -9.474510206698964154, 16.51473224551069663, 75.41557627198103830 ) ) ;
#40224=CARTESIAN_POINT ( 'NONE',  ( -18.67979575497193778, 10.72451020669871902, 33.33442372801900433 ) ) ;
#40225=CARTESIAN_POINT ( 'NONE',  ( -13.89961937509977652, 13.97604488694528158, 110.6239096053143243 ) ) ;
#40226=CARTESIAN_POINT ( 'NONE',  ( -0.05219959533934338120, 16.53943276465976808, 92.50109039468567573 ) ) ;
#40227=CARTESIAN_POINT ( 'NONE',  ( -5.719274019375665041, -21.55341960407619695, 64.79275706135234714 ) ) ;
#40228=CARTESIAN_POINT ( 'NONE',  ( 0.05219959533937995610, -21.53943276465977519, 95.00109039468568994 ) ) ;
#40229=CARTESIAN_POINT ( 'NONE',  ( -12.06949235617739369, -12.14591786802326823, 79.37609039468567573 ) ) ;
#40230=CARTESIAN_POINT ( 'NONE',  ( 10.81492255796106328, -18.62759615963255655, 30.41775706135234358 ) ) ;
#40232=CARTESIAN_POINT ( 'NONE',  ( 19.02544592524343514, -5.153800228976328945, 23.54057627198102054 ) ) ;
#40233=CARTESIAN_POINT ( 'NONE',  ( -15.80617190586768217, 15.72974639402176855, 93.12609039468568994 ) ) ;
#40234=CARTESIAN_POINT ( 'NONE',  ( -9.564922557960796823, -16.46253265017161027, 97.08224293864769550 ) ) ;
#40235=CARTESIAN_POINT ( 'NONE',  ( 5.823673210054125526, 21.52544592524343514, 84.79057627198102409 ) ) ;
#40236=CARTESIAN_POINT ( 'NONE',  ( -13.97604488694547697, 13.89961937509957934, 58.12609039468566863 ) ) ;
#40238=CARTESIAN_POINT ( 'NONE',  ( 10.72451020669898902, -18.67979575497178502, 52.91557627198103830 ) ) ;
#40239=CARTESIAN_POINT ( 'NONE',  ( 9.564922557960805705, 16.46253265017160317, 94.58224293864769550 ) ) ;
#40240=CARTESIAN_POINT ( 'NONE',  ( 0.05219959533910956823, 16.53943276465976808, 49.99890960531437401 ) ) ;
#40242=CARTESIAN_POINT ( 'NONE',  ( -16.46253265017146816, -9.564922557961047289, 74.16775706135234714 ) ) ;
#40244=( BOUNDED_CURVE ( )  B_SPLINE_CURVE ( 2, ( #105971, #198986, #195014, #60454, #183816, #57501, #168630, #29152, #30130, #166671, #120146, #179859, #180854 ),
 .UNSPECIFIED., .F., .T. ) 
 B_SPLINE_CURVE_WITH_KNOTS ( ( 3, 2, 2, 2, 2, 2, 3 ),
 ( 0.3708971688807142786, 0.3728070175438596423, 0.3771929824561403577, 0.3815789473684210731, 0.3859649122807017330, 0.3903508771929824483, 0.3923064056782181175 ),
 .UNSPECIFIED. ) 
 CURVE ( )  GEOMETRIC_REPRESENTATION_ITEM ( )  RATIONAL_B_SPLINE_CURVE ( ( 0.9832469066685285419, 0.9851625545550100060, 1.000000000000000000, 0.9659258262890683122, 1.000000000000000000, 0.9659258262890683122, 1.000000000000000000, 0.9659258262890683122, 1.000000000000000000, 0.9659258262890683122, 1.000000000000000000, 0.9848076720550082985, 0.9831626618144002627 ) ) 
 REPRESENTATION_ITEM ( '' )  );
#40246=CARTESIAN_POINT ( 'NONE',  ( 19.03943276465977164, 0.05219959533936151252, 111.2510903946856757 ) ) ;
#40247=CARTESIAN_POINT ( 'NONE',  ( -15.80617190586745835, -15.72974639402198527, 81.87390960531435269 ) ) ;
#40248=CARTESIAN_POINT ( 'NONE',  ( 4.379528057220339221, -16.55341960407611168, 62.70724293864769550 ) ) ;
#40249=CARTESIAN_POINT ( 'NONE',  ( 13.97604488694527802, 13.89961937509977652, 99.37390960531436690 ) ) ;
#40250=CARTESIAN_POINT ( 'NONE',  ( 4.483927247898790824, -16.52544592524335698, 25.20942372801901854 ) ) ;
#40251=CARTESIAN_POINT ( 'NONE',  ( 5.153800228976335163, 19.02544592524342804, 54.79057627198103120 ) ) ;
#40252=CARTESIAN_POINT ( 'NONE',  ( -21.53943276465977519, 0.05219959533907696930, 116.2489096053143669 ) ) ;
#40253=CARTESIAN_POINT ( 'NONE',  ( -16.46253265017146816, -9.564922557961047289, 84.16775706135233293 ) ) ;
#40255=CARTESIAN_POINT ( 'NONE',  ( -19.03943276465977164, 0.05219959533909376836, 91.24890960531436690 ) ) ;
#40256=CARTESIAN_POINT ( 'NONE',  ( -19.02544592524342804, 5.153800228976336051, 71.04057627198099567 ) ) ;
#40257=CARTESIAN_POINT ( 'NONE',  ( -21.53943276465977519, 0.05219959533907696930, 71.24890960531435269 ) ) ;
#40258=CARTESIAN_POINT ( 'NONE',  ( -5.153800228976328057, -19.02544592524343514, 47.29057627198102409 ) ) ;
#40260=CARTESIAN_POINT ( 'NONE',  ( -16.52544592524342804, 4.483927247898546575, 51.04057627198103120 ) ) ;
#40261=CARTESIAN_POINT ( 'NONE',  ( 9.474510206698971260, -16.51473224551069308, 102.9155762719810241 ) ) ;
#40263=CARTESIAN_POINT ( 'NONE',  ( -9.474510206698720793, -16.51473224551083518, 64.58442372801900433 ) ) ;
#40264=CARTESIAN_POINT ( 'NONE',  ( 21.53943276465977519, -0.05219959533907433946, 88.74890960531436690 ) ) ;
#40265=CARTESIAN_POINT ( 'NONE',  ( -13.97604488694547697, 13.89961937509957934, 53.12609039468565442 ) ) ;
#40266=CARTESIAN_POINT ( 'NONE',  ( 19.03943276465977164, -0.05219959533909143690, 98.74890960531436690 ) ) ;
#40268=CARTESIAN_POINT ( 'NONE',  ( 0.05219959533907565091, 21.53943276465977519, 44.99890960531435979 ) ) ;
#40270=CARTESIAN_POINT ( 'NONE',  ( 19.05341960407611168, 5.049401038298154454, 68.95724293864769550 ) ) ;
#40271=CARTESIAN_POINT ( 'NONE',  ( -18.67979575497193778, 10.72451020669871902, 68.33442372801900433 ) ) ;
#40272=CARTESIAN_POINT ( 'NONE',  ( 16.51473224551069308, 9.474510206698969483, 44.16557627198103120 ) ) ;
#40273=CARTESIAN_POINT ( 'NONE',  ( 12.14591786802309770, 12.06949235617756955, 79.37390960531436690 ) ) ;
#40274=ORIENTED_EDGE ( 'NONE', *, *, #33819, .F. ) ;
#40275=CARTESIAN_POINT ( 'NONE',  ( -15.72974639402176322, -15.80617190586768395, 59.37609039468568284 ) ) ;
#40277=CARTESIAN_POINT ( 'NONE',  ( 9.564922557960805705, 16.46253265017160317, 109.5822429386476955 ) ) ;
#40278=CARTESIAN_POINT ( 'NONE',  ( 19.05341960407617918, -5.049401038297876454, 71.04275706135234714 ) ) ;
#40280=CARTESIAN_POINT ( 'NONE',  ( -5.719274019375978568, 21.55341960407610458, 115.2072429386476955 ) ) ;
#40281=CARTESIAN_POINT ( 'NONE',  ( 16.51473224551069308, 9.474510206698969483, 54.16557627198103120 ) ) ;
#40282=CARTESIAN_POINT ( 'NONE',  ( 16.52544592524335698, 4.483927247898782831, 36.45942372801901143 ) ) ;
#40284=CARTESIAN_POINT ( 'NONE',  ( -19.03943276465977164, -0.05219959533935918106, 23.75109039468566152 ) ) ;
#40285=CARTESIAN_POINT ( 'NONE',  ( -16.46253265017160317, 9.564922557960807481, 40.83224293864769550 ) ) ;
#40286=CARTESIAN_POINT ( 'NONE',  ( -13.89961937509957401, -13.97604488694547875, 19.37609039468566507 ) ) ;
#40287=CARTESIAN_POINT ( 'NONE',  ( -16.52544592524335698, -4.483927247898792601, 88.95942372801901854 ) ) ;
#40288=CARTESIAN_POINT ( 'NONE',  ( 19.03943276465977164, -0.05219959533909143690, 83.74890960531436690 ) ) ;
#40289=CARTESIAN_POINT ( 'NONE',  ( -10.81492255796105439, 18.62759615963255655, 67.91775706135234714 ) ) ;
#40291=CARTESIAN_POINT ( 'NONE',  ( -13.97604488694527625, -13.89961937509977652, 111.8739096053143243 ) ) ;
#40293=CARTESIAN_POINT ( 'NONE',  ( 8.314922557961029526, -14.29746914071037800, 55.41775706135234714 ) ) ;
#40294=CARTESIAN_POINT ( 'NONE',  ( 18.62759615963255655, 10.81492255796105972, 66.66775706135234714 ) ) ;
#40295=CARTESIAN_POINT ( 'NONE',  ( 15.72974639402176855, 15.80617190586768217, 96.87609039468568994 ) ) ;
#40297=CARTESIAN_POINT ( 'NONE',  ( -4.483927247898782831, 16.52544592524335698, 32.70942372801900433 ) ) ;
#40298=CARTESIAN_POINT ( 'NONE',  ( -13.97604488694527625, -13.89961937509977652, 81.87390960531436690 ) ) ;
#40301=CARTESIAN_POINT ( 'NONE',  ( 19.05341960407611168, 5.049401038298154454, 38.95724293864767418 ) ) ;
#40302=CARTESIAN_POINT ( 'NONE',  ( 18.67979575497178502, 10.72451020669898547, 49.16557627198102409 ) ) ;
#40303=CARTESIAN_POINT ( 'NONE',  ( -16.53943276465976808, -0.05219959533934237506, 103.7510903946857042 ) ) ;
#40304=CARTESIAN_POINT ( 'NONE',  ( 4.483927247898545687, 16.52544592524342804, 84.79057627198102409 ) ) ;
#40305=CARTESIAN_POINT ( 'NONE',  ( -13.89961937509977652, 13.97604488694528158, 70.62390960531432427 ) ) ;
#40306=CARTESIAN_POINT ( 'NONE',  ( -15.80617190586768217, 15.72974639402176855, 103.1260903946856757 ) ) ;
#40307=CARTESIAN_POINT ( 'NONE',  ( 8.314922557961029526, -14.29746914071037800, 25.41775706135235779 ) ) ;
#40308=CARTESIAN_POINT ( 'NONE',  ( 0.05219959533910956823, 16.53943276465976808, 94.99890960531436690 ) ) ;
#40309=CARTESIAN_POINT ( 'NONE',  ( 5.719274019375673035, 21.55341960407619339, 47.29275706135234003 ) ) ;
#40310=CARTESIAN_POINT ( 'NONE',  ( 18.62759615963271287, -10.81492255796078972, 78.33224293864770971 ) ) ;
#40311=CARTESIAN_POINT ( 'NONE',  ( 0.05219959533936267826, -19.03943276465977164, 55.00109039468566863 ) ) ;
#40312=CARTESIAN_POINT ( 'NONE',  ( -9.564922557960796823, -16.46253265017161027, 102.0822429386477097 ) ) ;
#40313=CARTESIAN_POINT ( 'NONE',  ( -16.52544592524342804, 4.483927247898546575, 61.04057627198103120 ) ) ;
#40314=CARTESIAN_POINT ( 'NONE',  ( -8.224510206698948167, 14.34966873604960824, 50.41557627198103120 ) ) ;
#40315=CARTESIAN_POINT ( 'NONE',  ( 16.53943276465976808, 0.05219959533934440121, 106.2510903946856757 ) ) ;
#40316=CARTESIAN_POINT ( 'NONE',  ( 13.97604488694548053, -13.89961937509957401, 70.62609039468567573 ) ) ;
#40317=CARTESIAN_POINT ( 'NONE',  ( -18.56197773271732032, 5.499999999999903189, 83.55066217314454491 ) ) ;
#40318=CARTESIAN_POINT ( 'NONE',  ( 10.81492255796078972, 18.62759615963270932, 24.58224293864768839 ) ) ;
#40319=CARTESIAN_POINT ( 'NONE',  ( 0.05219959533910956823, 16.53943276465976808, 84.99890960531436690 ) ) ;
#40321=CARTESIAN_POINT ( 'NONE',  ( -0.05219959533909027116, -19.03943276465977164, 42.49890960531435269 ) ) ;
#40322=CARTESIAN_POINT ( 'NONE',  ( 0.05219959533907565091, 21.53943276465977519, 54.99890960531435269 ) ) ;
#40323=CARTESIAN_POINT ( 'NONE',  ( 21.55341960407610458, 5.719274019375980345, 78.95724293864769550 ) ) ;
#40324=CARTESIAN_POINT ( 'NONE',  ( 19.05341960407611168, 5.049401038298154454, 23.95724293864769194 ) ) ;
#40325=CARTESIAN_POINT ( 'NONE',  ( -8.314922557961024197, 14.29746914071037800, 62.91775706135236135 ) ) ;
#40326=CARTESIAN_POINT ( 'NONE',  ( -9.474510206698964154, 16.51473224551069663, 55.41557627198103120 ) ) ;
#40327=CARTESIAN_POINT ( 'NONE',  ( 19.03943276465977164, 0.05219959533936151252, 46.25109039468566863 ) ) ;
#40328=CARTESIAN_POINT ( 'NONE',  ( -15.72974639402176322, -15.80617190586768395, 54.37609039468568994 ) ) ;
#40330=CARTESIAN_POINT ( 'NONE',  ( -14.34966873604960291, -8.224510206698953496, 111.6655762719810525 ) ) ;
#40332=CARTESIAN_POINT ( 'NONE',  ( 19.03943276465977164, 0.05219959533936151252, 86.25109039468567573 ) ) ;
#40334=CARTESIAN_POINT ( 'NONE',  ( -30.00000000000000000, 5.499999999999992895, 37.50000000000000000 ) ) ;
#40335=CARTESIAN_POINT ( 'NONE',  ( 0.05219959533907565091, 21.53943276465977519, 44.99890960531435979 ) ) ;
#40336=CARTESIAN_POINT ( 'NONE',  ( 16.62475595723694965, -7.163666690055214836, 68.02713351810464815 ) ) ;
#40337=CARTESIAN_POINT ( 'NONE',  ( 18.62759615963255655, 10.81492255796105972, 81.66775706135236135 ) ) ;
#40338=CARTESIAN_POINT ( 'NONE',  ( -4.483927247898539470, -16.52544592524342804, 27.29057627198103120 ) ) ;
#40339=CARTESIAN_POINT ( 'NONE',  ( 4.379528057220092307, 16.55341960407617563, 57.29275706135234714 ) ) ;
#40340=CARTESIAN_POINT ( 'NONE',  ( 4.379528057220339221, -16.55341960407611168, 62.70724293864769550 ) ) ;
#40341=CARTESIAN_POINT ( 'NONE',  ( -10.81492255796078084, -18.62759615963271287, 87.08224293864769550 ) ) ;
#40342=CARTESIAN_POINT ( 'NONE',  ( 5.823673210054125526, 21.52544592524343514, 69.79057627198102409 ) ) ;
#40344=CARTESIAN_POINT ( 'NONE',  ( 5.153800228976615827, -19.02544592524334988, 80.20942372801901854 ) ) ;
#40345=CARTESIAN_POINT ( 'NONE',  ( 18.62759615963271287, -10.81492255796078972, 23.33224293864769194 ) ) ;
#40346=CARTESIAN_POINT ( 'NONE',  ( -9.564922557960796823, -16.46253265017161027, 67.08224293864769550 ) ) ;
#40347=CARTESIAN_POINT ( 'NONE',  ( -19.02544592524342804, 5.153800228976336051, 31.04057627198102409 ) ) ;
#40348=CARTESIAN_POINT ( 'NONE',  ( -17.49999999999999645, -7.500000000000000888, 118.0000000000000142 ) ) ;
#40349=VERTEX_POINT ( 'NONE', #194475 ) ;
#40351=CARTESIAN_POINT ( 'NONE',  ( 4.379528057220092307, 16.55341960407617563, 82.29275706135234714 ) ) ;
#40352=CARTESIAN_POINT ( 'NONE',  ( -5.719274019375978568, 21.55341960407610458, 105.2072429386477097 ) ) ;
#40353=CARTESIAN_POINT ( 'NONE',  ( -13.97604488694527625, -13.89961937509977652, 71.87390960531433848 ) ) ;
#40354=CARTESIAN_POINT ( 'NONE',  ( 21.53943276465977519, 0.05219959533937863772, 41.25109039468568284 ) ) ;
#40355=CARTESIAN_POINT ( 'NONE',  ( -13.97604488694527625, -13.89961937509977652, 96.87390960531433848 ) ) ;
#40358=CARTESIAN_POINT ( 'NONE',  ( -5.823673210054431948, 21.52544592524334988, 47.70942372801902565 ) ) ;
#40359=CARTESIAN_POINT ( 'NONE',  ( -19.03943276465977164, 0.05219959533909376836, 21.24890960531436335 ) ) ;
#40360=CARTESIAN_POINT ( 'NONE',  ( 9.564922557960805705, 16.46253265017160317, 109.5822429386476955 ) ) ;
#40361=CARTESIAN_POINT ( 'NONE',  ( 9.564922557961047289, -16.46253265017146816, 60.41775706135233293 ) ) ;
#40362=CARTESIAN_POINT ( 'NONE',  ( -5.823673210054116645, -21.52544592524344225, 112.2905762719810241 ) ) ;
#40363=CARTESIAN_POINT ( 'NONE',  ( 16.51473224551083163, -9.474510206698727899, 50.83442372801899722 ) ) ;
#40364=CARTESIAN_POINT ( 'NONE',  ( 19.02544592524334988, 5.153800228976608722, 46.45942372801899012 ) ) ;
#40365=CARTESIAN_POINT ( 'NONE',  ( -16.55341960407617563, 4.379528057220093196, 103.5427570613523613 ) ) ;
#40368=VERTEX_POINT ( 'NONE', #160125 ) ;
#40369=CARTESIAN_POINT ( 'NONE',  ( -19.02544592524342804, 5.153800228976336051, 71.04057627198099567 ) ) ;
#40370=CARTESIAN_POINT ( 'NONE',  ( -5.719274019375665041, -21.55341960407619695, 79.79275706135236135 ) ) ;
#40371=CARTESIAN_POINT ( 'NONE',  ( 21.52544592524334988, 5.823673210054432836, 91.45942372801901854 ) ) ;
#40373=CARTESIAN_POINT ( 'NONE',  ( 9.564922557960805705, 16.46253265017160317, 84.58224293864769550 ) ) ;
#40374=CARTESIAN_POINT ( 'NONE',  ( 21.55341960407619695, -5.719274019375665929, 61.04275706135234714 ) ) ;
#40375=CARTESIAN_POINT ( 'NONE',  ( -19.03943276465977164, -0.05219959533935918106, 113.7510903946856757 ) ) ;
#40376=CARTESIAN_POINT ( 'NONE',  ( 16.51473224551069308, 9.474510206698969483, 69.16557627198102409 ) ) ;
#40377=CARTESIAN_POINT ( 'NONE',  ( 5.153800228976335163, 19.02544592524342804, 109.7905762719810099 ) ) ;
#40378=CARTESIAN_POINT ( 'NONE',  ( -0.05219959533909027116, -19.03943276465977164, 87.49890960531436690 ) ) ;
#40379=DIRECTION ( 'NONE',  ( 1.000000000000000000, -0.000000000000000000, 0.000000000000000000 ) ) ;
#40380=CARTESIAN_POINT ( 'NONE',  ( 19.03943276465977164, -0.05219959533909143690, 78.74890960531436690 ) ) ;
#40381=CARTESIAN_POINT ( 'NONE',  ( 0.05219959533909260263, 19.03943276465977164, 69.99890960531435269 ) ) ;
#40382=CARTESIAN_POINT ( 'NONE',  ( -18.67979575497178146, -10.72451020669898902, 106.6655762719810383 ) ) ;
#40383=CARTESIAN_POINT ( 'NONE',  ( 16.53943276465976808, 0.05219959533934440121, 101.2510903946856757 ) ) ;
#40386=CARTESIAN_POINT ( 'NONE',  ( -19.05341960407617563, 5.049401038297882671, 63.54275706135234003 ) ) ;
#40387=CARTESIAN_POINT ( 'NONE',  ( 13.89961937509977652, -13.97604488694527269, 98.12390960531433848 ) ) ;
#40388=CARTESIAN_POINT ( 'NONE',  ( 8.314922557960818139, 14.29746914071049879, 69.58224293864769550 ) ) ;
#40389=CARTESIAN_POINT ( 'NONE',  ( 8.314922557960818139, 14.29746914071049879, 104.5822429386477097 ) ) ;
#40391=CARTESIAN_POINT ( 'NONE',  ( -5.823673210054116645, -21.52544592524344225, 37.29057627198102409 ) ) ;
#40392=CARTESIAN_POINT ( 'NONE',  ( -5.049401038298153566, 19.05341960407611168, 115.2072429386477097 ) ) ;
#40393=CARTESIAN_POINT ( 'NONE',  ( -21.53943276465977519, 0.05219959533907696930, 21.24890960531436690 ) ) ;
#40394=CARTESIAN_POINT ( 'NONE',  ( 4.379528057220339221, -16.55341960407611168, 97.70724293864772392 ) ) ;
#40395=CARTESIAN_POINT ( 'NONE',  ( -16.31925111598457789, 7.325300261831452886, 55.16424538967250157 ) ) ;
#40396=CARTESIAN_POINT ( 'NONE',  ( -16.51473224551082808, 9.474510206698731452, 38.33442372801899722 ) ) ;
#40397=CARTESIAN_POINT ( 'NONE',  ( -4.379528057220086978, -16.55341960407618274, 104.7927570613523898 ) ) ;
#40398=CARTESIAN_POINT ( 'NONE',  ( -16.51473224551069308, -9.474510206698971260, 86.66557627198102409 ) ) ;
#40399=CARTESIAN_POINT ( 'NONE',  ( 10.72451020669871369, 18.67979575497193778, 57.08442372801901854 ) ) ;
#40400=CARTESIAN_POINT ( 'NONE',  ( -10.72451020669898014, 18.67979575497178502, 50.41557627198103120 ) ) ;
#40401=CARTESIAN_POINT ( 'NONE',  ( -5.823673210054431948, 21.52544592524334988, 32.70942372801900433 ) ) ;
#40402=CARTESIAN_POINT ( 'NONE',  ( 5.823673210054125526, 21.52544592524343514, 79.79057627198102409 ) ) ;
#40403=CARTESIAN_POINT ( 'NONE',  ( 4.379528057220339221, -16.55341960407611168, 102.7072429386476955 ) ) ;
#40404=CARTESIAN_POINT ( 'NONE',  ( -19.05341960407617563, 5.049401038297882671, 73.54275706135233293 ) ) ;
#40405=CARTESIAN_POINT ( 'NONE',  ( 9.564922557960805705, 16.46253265017160317, 39.58224293864768839 ) ) ;
#40406=CARTESIAN_POINT ( 'NONE',  ( -19.02544592524342804, 5.153800228976336051, 96.04057627198103830 ) ) ;
#40407=CARTESIAN_POINT ( 'NONE',  ( 16.51473224551069308, 9.474510206698969483, 89.16557627198103830 ) ) ;
#40408=CARTESIAN_POINT ( 'NONE',  ( -13.89961937509977652, 13.97604488694528158, 25.62390960531434558 ) ) ;
#40409=CARTESIAN_POINT ( 'NONE',  ( 12.14591786802309770, 12.06949235617756955, 39.37390960531436690 ) ) ;
#40410=CARTESIAN_POINT ( 'NONE',  ( -14.29746914071037622, -8.314922557961029526, 44.16775706135234714 ) ) ;
#40411=CARTESIAN_POINT ( 'NONE',  ( 21.53943276465977519, 0.05219959533937863772, 111.2510903946856899 ) ) ;
#40414=CARTESIAN_POINT ( 'NONE',  ( 16.55341960407611168, 4.379528057220329451, 23.95724293864769550 ) ) ;
#40415=CARTESIAN_POINT ( 'NONE',  ( -21.55341960407619339, 5.719274019375674811, 28.54275706135234358 ) ) ;
#40416=CARTESIAN_POINT ( 'NONE',  ( 9.564922557960805705, 16.46253265017160317, 99.58224293864770971 ) ) ;
#40417=CARTESIAN_POINT ( 'NONE',  ( 16.53943276465976808, 0.05219959533934440121, 101.2510903946856757 ) ) ;
#40418=CARTESIAN_POINT ( 'NONE',  ( -0.05219959533934338120, 16.53943276465976808, 92.50109039468567573 ) ) ;
#40419=CARTESIAN_POINT ( 'NONE',  ( -16.55341960407617563, 4.379528057220093196, 23.54275706135235424 ) ) ;
#40420=CARTESIAN_POINT ( 'NONE',  ( 13.89961937509977652, -13.97604488694527269, 48.12390960531435979 ) ) ;
#40421=CARTESIAN_POINT ( 'NONE',  ( 16.52544592524342804, -4.483927247898539470, 103.5405762719810383 ) ) ;
#40422=CARTESIAN_POINT ( 'NONE',  ( 21.55341960407619695, -5.719274019375665929, 26.04275706135235779 ) ) ;
#40423=CARTESIAN_POINT ( 'NONE',  ( 19.02544592524343514, -5.153800228976328945, 33.54057627198102409 ) ) ;
#40424=CARTESIAN_POINT ( 'NONE',  ( -0.05219959533909027116, -19.03943276465977164, 107.4989096053143527 ) ) ;
#40425=CARTESIAN_POINT ( 'NONE',  ( 21.52544592524334988, 5.823673210054432836, 31.45942372801901854 ) ) ;
#40427=CARTESIAN_POINT ( 'NONE',  ( 13.89961937509977652, -13.97604488694527269, 103.1239096053143527 ) ) ;
#40429=CARTESIAN_POINT ( 'NONE',  ( 19.05341960407611168, 5.049401038298154454, 98.95724293864766707 ) ) ;
#40430=CARTESIAN_POINT ( 'NONE',  ( -18.67979575497193778, 10.72451020669871902, 43.33442372801901143 ) ) ;
#40431=CARTESIAN_POINT ( 'NONE',  ( -4.483927247898539470, -16.52544592524342804, 97.29057627198105251 ) ) ;
#40432=CARTESIAN_POINT ( 'NONE',  ( -5.049401038298153566, 19.05341960407611168, 90.20724293864766707 ) ) ;
#40433=CARTESIAN_POINT ( 'NONE',  ( -8.224510206698735004, -14.34966873604973081, 64.58442372801900433 ) ) ;
#40434=CARTESIAN_POINT ( 'NONE',  ( 10.72451020669871369, 18.67979575497193778, 77.08442372801901854 ) ) ;
#40435=CARTESIAN_POINT ( 'NONE',  ( -0.05219959533934338120, 16.53943276465976808, 42.50109039468567573 ) ) ;
#40436=CARTESIAN_POINT ( 'NONE',  ( 13.97604488694527802, 13.89961937509977652, 79.37390960531435269 ) ) ;
#40437=CARTESIAN_POINT ( 'NONE',  ( -5.153800228976607833, 19.02544592524334988, 112.7094237280190043 ) ) ;
#40438=CARTESIAN_POINT ( 'NONE',  ( 4.483927247898790824, -16.52544592524335698, 70.20942372801904696 ) ) ;
#40439=CARTESIAN_POINT ( 'NONE',  ( 16.51473224551083163, -9.474510206698727899, 90.83442372801900433 ) ) ;
#40440=CARTESIAN_POINT ( 'NONE',  ( 16.51473224551069308, 9.474510206698969483, 64.16557627198102409 ) ) ;
#40441=CARTESIAN_POINT ( 'NONE',  ( 21.55341960407610458, 5.719274019375980345, 83.95724293864770971 ) ) ;
#40442=CARTESIAN_POINT ( 'NONE',  ( 16.53943276465976808, -0.05219959533910856209, 93.74890960531436690 ) ) ;
#40443=CARTESIAN_POINT ( 'NONE',  ( -0.05219959533936034679, 19.03943276465977164, 87.50109039468567573 ) ) ;
#40444=CARTESIAN_POINT ( 'NONE',  ( 14.34966873604972726, -8.224510206698740333, 60.83442372801901854 ) ) ;
#40445=CARTESIAN_POINT ( 'NONE',  ( -18.22780087662123805, 5.499999999999981348, 81.01763182126896368 ) ) ;
#40446=CARTESIAN_POINT ( 'NONE',  ( -19.02544592524334988, -5.153800228976617603, 53.95942372801898301 ) ) ;
#40447=CARTESIAN_POINT ( 'NONE',  ( 12.14591786802309770, 12.06949235617756955, 34.37390960531435979 ) ) ;
#40448=CARTESIAN_POINT ( 'NONE',  ( 12.14591786802309770, 12.06949235617756955, 79.37390960531436690 ) ) ;
#40449=CARTESIAN_POINT ( 'NONE',  ( 10.81492255796106328, -18.62759615963255655, 110.4177570613523756 ) ) ;
#40451=CARTESIAN_POINT ( 'NONE',  ( 5.823673210054444382, -21.52544592524334988, 25.20942372801901854 ) ) ;
#40452=CARTESIAN_POINT ( 'NONE',  ( -13.89961937509977652, 13.97604488694528158, 95.62390960531436690 ) ) ;
#40453=CARTESIAN_POINT ( 'NONE',  ( 9.474510206698971260, -16.51473224551069308, 77.91557627198103830 ) ) ;
#40454=CARTESIAN_POINT ( 'NONE',  ( 18.67979575497194134, -10.72451020669871369, 95.83442372801903275 ) ) ;
#40455=CARTESIAN_POINT ( 'NONE',  ( 19.02544592524343514, -5.153800228976328945, 78.54057627198099567 ) ) ;
#40456=CARTESIAN_POINT ( 'NONE',  ( -21.52544592524343514, 5.823673210054127303, 46.04057627198103830 ) ) ;
#40458=CARTESIAN_POINT ( 'NONE',  ( -4.379528057220328563, 16.55341960407611168, 75.20724293864769550 ) ) ;
#40459=CARTESIAN_POINT ( 'NONE',  ( -16.51473224551069308, -9.474510206698971260, 51.66557627198102409 ) ) ;
#40460=CARTESIAN_POINT ( 'NONE',  ( 12.06949235617757843, -12.14591786802309237, 103.1239096053143811 ) ) ;
#40461=CARTESIAN_POINT ( 'NONE',  ( -21.53943276465977519, -0.05219959533937600094, 18.75109039468568639 ) ) ;
#40463=CARTESIAN_POINT ( 'NONE',  ( 15.80617190586769283, -15.72974639402175789, 60.62609039468567573 ) ) ;
#40464=CARTESIAN_POINT ( 'NONE',  ( -5.153800228976328057, -19.02544592524343514, 47.29057627198102409 ) ) ;
#40465=CARTESIAN_POINT ( 'NONE',  ( -16.52544592524335698, -4.483927247898792601, 68.95942372801901854 ) ) ;
#40466=CARTESIAN_POINT ( 'NONE',  ( -15.72974639402197994, 15.80617190586746368, 110.6239096053143669 ) ) ;
#40467=CARTESIAN_POINT ( 'NONE',  ( -10.72451020669898014, 18.67979575497178502, 115.4155762719810241 ) ) ;
#40468=CARTESIAN_POINT ( 'NONE',  ( -19.02544592524334988, -5.153800228976617603, 43.95942372801899012 ) ) ;
#40469=CARTESIAN_POINT ( 'NONE',  ( 19.02544592524343514, -5.153800228976328945, 68.54057627198103830 ) ) ;
#40471=CARTESIAN_POINT ( 'NONE',  ( 5.823673210054444382, -21.52544592524334988, 75.20942372801901854 ) ) ;
#40472=CARTESIAN_POINT ( 'NONE',  ( 10.72451020669898902, -18.67979575497178502, 57.91557627198103120 ) ) ;
#40473=CARTESIAN_POINT ( 'NONE',  ( 0.05219959533910956823, 16.53943276465976808, 34.99890960531435979 ) ) ;
#40474=CARTESIAN_POINT ( 'NONE',  ( 5.719274019375673035, 21.55341960407619339, 72.29275706135236135 ) ) ;
#40475=CARTESIAN_POINT ( 'NONE',  ( 5.823673210054444382, -21.52544592524334988, 110.2094237280190185 ) ) ;
#40476=CARTESIAN_POINT ( 'NONE',  ( -16.53943276465976808, 0.05219959533911058130, 56.24890960531436690 ) ) ;
#40477=CARTESIAN_POINT ( 'NONE',  ( 16.53943276465976808, -0.05219959533910856209, 98.74890960531438111 ) ) ;
#40478=CARTESIAN_POINT ( 'NONE',  ( -9.474510206698720793, -16.51473224551083518, 49.58442372801899722 ) ) ;
#40479=CARTESIAN_POINT ( 'NONE',  ( 14.34966873604972726, -8.224510206698740333, 110.8344237280190043 ) ) ;
#40480=CARTESIAN_POINT ( 'NONE',  ( -0.05219959533937732626, 21.53943276465977519, 72.50109039468568994 ) ) ;
#40481=CARTESIAN_POINT ( 'NONE',  ( -19.05341960407611168, -5.049401038298163336, 61.45724293864769550 ) ) ;
#40482=CARTESIAN_POINT ( 'NONE',  ( -13.97604488694547697, 13.89961937509957934, 33.12609039468566863 ) ) ;
#40483=CARTESIAN_POINT ( 'NONE',  ( -0.05219959533907301413, -21.53943276465977519, 37.49890960531436690 ) ) ;
#40484=CARTESIAN_POINT ( 'NONE',  ( -0.05219959533937732626, 21.53943276465977519, 37.50109039468568284 ) ) ;
#40485=CARTESIAN_POINT ( 'NONE',  ( -5.823673210054116645, -21.52544592524344225, 92.29057627198103830 ) ) ;
#40486=CARTESIAN_POINT ( 'NONE',  ( 19.05341960407617918, -5.049401038297876454, 81.04275706135231871 ) ) ;
#40487=CARTESIAN_POINT ( 'NONE',  ( 4.379528057220092307, 16.55341960407617563, 47.29275706135234003 ) ) ;
#40489=CARTESIAN_POINT ( 'NONE',  ( -15.80617190586745835, -15.72974639402198527, 91.87390960531436690 ) ) ;
#40490=CARTESIAN_POINT ( 'NONE',  ( 14.29746914071049879, -8.314922557960816363, 83.33224293864769550 ) ) ;
#40492=CARTESIAN_POINT ( 'NONE',  ( -8.314922557961024197, 14.29746914071037800, 22.91775706135235069 ) ) ;
#40493=CARTESIAN_POINT ( 'NONE',  ( 15.72974639402199770, -15.80617190586745480, 48.12390960531436690 ) ) ;
#40494=CARTESIAN_POINT ( 'NONE',  ( -12.06949235617739369, -12.14591786802326823, 89.37609039468568994 ) ) ;
#40495=CARTESIAN_POINT ( 'NONE',  ( -0.05219959533909027116, -19.03943276465977164, 22.49890960531436690 ) ) ;
#40496=CARTESIAN_POINT ( 'NONE',  ( -4.379528057220086978, -16.55341960407618274, 59.79275706135234714 ) ) ;
#40497=CARTESIAN_POINT ( 'NONE',  ( 21.53943276465977519, 0.05219959533937863772, 21.25109039468567218 ) ) ;
#40498=CARTESIAN_POINT ( 'NONE',  ( 21.53943276465977519, -0.05219959533907433946, 48.74890960531435979 ) ) ;
#40499=CARTESIAN_POINT ( 'NONE',  ( 4.379528057220092307, 16.55341960407617563, 82.29275706135234714 ) ) ;
#40500=CARTESIAN_POINT ( 'NONE',  ( 9.564922557960805705, 16.46253265017160317, 99.58224293864770971 ) ) ;
#40501=CARTESIAN_POINT ( 'NONE',  ( -5.719274019375665041, -21.55341960407619695, 49.79275706135234714 ) ) ;
#40502=CARTESIAN_POINT ( 'NONE',  ( 19.02544592524343514, -5.153800228976328945, 23.54057627198102054 ) ) ;
#40504=CARTESIAN_POINT ( 'NONE',  ( 21.55341960407610458, 5.719274019375980345, 38.95724293864768839 ) ) ;
#40505=CARTESIAN_POINT ( 'NONE',  ( -18.67979575497178146, -10.72451020669898902, 26.66557627198103475 ) ) ;
#40507=CARTESIAN_POINT ( 'NONE',  ( -13.97604488694547697, 13.89961937509957934, 33.12609039468566863 ) ) ;
#40508=CARTESIAN_POINT ( 'NONE',  ( -8.224510206698735004, -14.34966873604973081, 64.58442372801900433 ) ) ;
#40509=CARTESIAN_POINT ( 'NONE',  ( -10.72451020669898014, 18.67979575497178502, 25.41557627198103120 ) ) ;
#40511=CARTESIAN_POINT ( 'NONE',  ( 9.564922557960805705, 16.46253265017160317, 79.58224293864769550 ) ) ;
#40512=CARTESIAN_POINT ( 'NONE',  ( 4.379528057220092307, 16.55341960407617563, 97.29275706135234714 ) ) ;
#40514=CARTESIAN_POINT ( 'NONE',  ( -16.52544592524342804, 4.483927247898546575, 91.04057627198103830 ) ) ;
#40515=CARTESIAN_POINT ( 'NONE',  ( 0.05219959533907565091, 21.53943276465977519, 44.99890960531435979 ) ) ;
#40516=CARTESIAN_POINT ( 'NONE',  ( 19.05341960407611168, 5.049401038298154454, 33.95724293864769550 ) ) ;
#40517=CARTESIAN_POINT ( 'NONE',  ( -16.53943276465976808, -0.05219959533934237506, 83.75109039468568994 ) ) ;
#40518=CARTESIAN_POINT ( 'NONE',  ( -21.55341960407619339, 5.719274019375674811, 38.54275706135234714 ) ) ;
#40519=CARTESIAN_POINT ( 'NONE',  ( 0.05219959533936267826, -19.03943276465977164, 85.00109039468567573 ) ) ;
#40520=CARTESIAN_POINT ( 'NONE',  ( 0.05219959533910956823, 16.53943276465976808, 94.99890960531436690 ) ) ;
#40521=CARTESIAN_POINT ( 'NONE',  ( -16.51473224551069308, -9.474510206698971260, 36.66557627198102409 ) ) ;
#40524=CARTESIAN_POINT ( 'NONE',  ( -21.52544592524334988, -5.823673210054445271, 103.9594237280190185 ) ) ;
#40525=CARTESIAN_POINT ( 'NONE',  ( -16.51473224551069308, -9.474510206698971260, 76.66557627198103830 ) ) ;
#40526=CARTESIAN_POINT ( 'NONE',  ( -4.483927247898782831, 16.52544592524335698, 57.70942372801901143 ) ) ;
#40527=CARTESIAN_POINT ( 'NONE',  ( 21.53943276465977519, 0.05219959533937863772, 91.25109039468568994 ) ) ;
#40528=CARTESIAN_POINT ( 'NONE',  ( -12.14591786802326823, 12.06949235617739902, 68.12609039468567573 ) ) ;
#40529=CARTESIAN_POINT ( 'NONE',  ( -13.97604488694547697, 13.89961937509957934, 53.12609039468565442 ) ) ;
#40530=CARTESIAN_POINT ( 'NONE',  ( 13.89961937509957401, 13.97604488694547697, 71.87609039468567573 ) ) ;
#40531=ORIENTED_EDGE ( 'NONE', *, *, #93872, .F. ) ;
#40532=CARTESIAN_POINT ( 'NONE',  ( -18.62759615963255300, -10.81492255796106328, 69.16775706135234714 ) ) ;
#40533=CARTESIAN_POINT ( 'NONE',  ( -0.05219959533909027116, -19.03943276465977164, 67.49890960531436690 ) ) ;
#40534=CARTESIAN_POINT ( 'NONE',  ( 5.049401038298163336, -19.05341960407611168, 57.70724293864769550 ) ) ;
#40535=CARTESIAN_POINT ( 'NONE',  ( -19.05341960407617563, 5.049401038297882671, 58.54275706135234003 ) ) ;
#40536=CARTESIAN_POINT ( 'NONE',  ( -5.153800228976328057, -19.02544592524343514, 112.2905762719810099 ) ) ;
#40537=CARTESIAN_POINT ( 'NONE',  ( 0.05219959533909260263, 19.03943276465977164, 84.99890960531436690 ) ) ;
#40538=CARTESIAN_POINT ( 'NONE',  ( 8.314922557960818139, 14.29746914071049879, 34.58224293864770260 ) ) ;
#40539=CARTESIAN_POINT ( 'NONE',  ( 21.53943276465977519, -0.05219959533907433946, 53.74890960531437401 ) ) ;
#40541=CARTESIAN_POINT ( 'NONE',  ( -17.50000000000000355, -5.499999999999980460, 96.28230962303564411 ) ) ;
#40542=CARTESIAN_POINT ( 'NONE',  ( 18.67979575497194134, -10.72451020669871369, 105.8344237280190328 ) ) ;
#40544=CARTESIAN_POINT ( 'NONE',  ( -0.05219959533909027116, -19.03943276465977164, 42.49890960531435269 ) ) ;
#40548=CARTESIAN_POINT ( 'NONE',  ( -5.719274019375665041, -21.55341960407619695, 64.79275706135234714 ) ) ;
#40550=CARTESIAN_POINT ( 'NONE',  ( 12.06949235617739724, 12.14591786802326823, 66.87609039468568994 ) ) ;
#40551=CARTESIAN_POINT ( 'NONE',  ( 5.823673210054125526, 21.52544592524343514, 84.79057627198102409 ) ) ;
#40552=CARTESIAN_POINT ( 'NONE',  ( -8.224510206698948167, 14.34966873604960824, 55.41557627198102409 ) ) ;
#40553=CARTESIAN_POINT ( 'NONE',  ( -16.51473224551069308, -9.474510206698971260, 26.66557627198103120 ) ) ;
#40555=CARTESIAN_POINT ( 'NONE',  ( 21.53943276465977519, 0.05219959533937863772, 46.25109039468567573 ) ) ;
#40556=CARTESIAN_POINT ( 'NONE',  ( -19.02544592524334988, -5.153800228976617603, 43.95942372801899012 ) ) ;
#40557=CARTESIAN_POINT ( 'NONE',  ( 16.51473224551069308, 9.474510206698969483, 34.16557627198102409 ) ) ;
#40558=CARTESIAN_POINT ( 'NONE',  ( 10.81492255796106328, -18.62759615963255655, 80.41775706135234714 ) ) ;
#40560=CARTESIAN_POINT ( 'NONE',  ( 8.224510206698953496, -14.34966873604960469, 32.91557627198102409 ) ) ;
#40562=CARTESIAN_POINT ( 'NONE',  ( -21.53943276465977519, 0.05219959533907696930, 41.24890960531435269 ) ) ;
#40564=CARTESIAN_POINT ( 'NONE',  ( -16.51473224551069308, -9.474510206698971260, 91.66557627198103830 ) ) ;
#40565=CARTESIAN_POINT ( 'NONE',  ( 8.224510206698953496, -14.34966873604960469, 87.91557627198103830 ) ) ;
#40566=CARTESIAN_POINT ( 'NONE',  ( 13.97604488694548053, -13.89961937509957401, 110.6260903946856615 ) ) ;
#40567=CARTESIAN_POINT ( 'NONE',  ( 5.823673210054125526, 21.52544592524343514, 69.79057627198102409 ) ) ;
#40569=CARTESIAN_POINT ( 'NONE',  ( 5.049401038298161559, -19.05341960407611168, 37.70724293864768839 ) ) ;
#40570=CARTESIAN_POINT ( 'NONE',  ( -19.05341960407611168, -5.049401038298163336, 91.45724293864766707 ) ) ;
#40571=CARTESIAN_POINT ( 'NONE',  ( -15.72974639402197994, 15.80617190586746368, 95.62390960531436690 ) ) ;
#40572=CARTESIAN_POINT ( 'NONE',  ( 4.483927247898790824, -16.52544592524335698, 110.2094237280190185 ) ) ;
#40573=CARTESIAN_POINT ( 'NONE',  ( -9.564922557960796823, -16.46253265017161027, 107.0822429386476955 ) ) ;
#40574=CARTESIAN_POINT ( 'NONE',  ( -5.153800228976607833, 19.02544592524334988, 82.70942372801897591 ) ) ;
#40575=CARTESIAN_POINT ( 'NONE',  ( 21.52544592524334988, 5.823673210054432836, 96.45942372801901854 ) ) ;
#40576=CARTESIAN_POINT ( 'NONE',  ( -21.52544592524343514, 5.823673210054127303, 76.04057627198102409 ) ) ;
#40577=CARTESIAN_POINT ( 'NONE',  ( 10.72451020669898902, -18.67979575497178502, 32.91557627198102409 ) ) ;
#40578=CARTESIAN_POINT ( 'NONE',  ( -9.474510206698964154, 16.51473224551069663, 45.41557627198103120 ) ) ;
#40579=CARTESIAN_POINT ( 'NONE',  ( 4.379528057220339221, -16.55341960407611168, 27.70724293864769905 ) ) ;
#40580=CARTESIAN_POINT ( 'NONE',  ( 13.89961937509977652, -13.97604488694527269, 78.12390960531433848 ) ) ;
#40581=ORIENTED_EDGE ( 'NONE', *, *, #99588, .F. ) ;
#40582=CARTESIAN_POINT ( 'NONE',  ( -17.49999999999999645, 5.499999999999997335, 110.7969038253417295 ) ) ;
#40583=CARTESIAN_POINT ( 'NONE',  ( -9.564922557961040184, 16.46253265017147172, 32.91775706135233293 ) ) ;
#40584=CARTESIAN_POINT ( 'NONE',  ( -12.06949235617756955, 12.14591786802309770, 90.62390960531436690 ) ) ;
#40585=CARTESIAN_POINT ( 'NONE',  ( 21.53943276465977519, 0.05219959533937863772, 26.25109039468567573 ) ) ;
#40587=CARTESIAN_POINT ( 'NONE',  ( 5.823673210054125526, 21.52544592524343514, 59.79057627198103120 ) ) ;
#40588=CARTESIAN_POINT ( 'NONE',  ( 14.34966873604972726, -8.224510206698740333, 95.83442372801903275 ) ) ;
#40589=CARTESIAN_POINT ( 'NONE',  ( -14.29746914071049879, 8.314922557960819915, 115.8322429386477097 ) ) ;
#40590=CARTESIAN_POINT ( 'NONE',  ( -5.153800228976328057, -19.02544592524343514, 77.29057627198099567 ) ) ;
#40591=CARTESIAN_POINT ( 'NONE',  ( 9.564922557960805705, 16.46253265017160317, 24.58224293864769194 ) ) ;
#40592=CARTESIAN_POINT ( 'NONE',  ( -16.55341960407611168, -4.379528057220339221, 31.45724293864769550 ) ) ;
#40593=CARTESIAN_POINT ( 'NONE',  ( 5.719274019375673035, 21.55341960407619339, 62.29275706135236845 ) ) ;
#40594=CARTESIAN_POINT ( 'NONE',  ( -0.05219959533909027116, -19.03943276465977164, 112.4989096053143669 ) ) ;
#40595=CARTESIAN_POINT ( 'NONE',  ( -18.62759615963255300, -10.81492255796106328, 99.16775706135234714 ) ) ;
#40596=CARTESIAN_POINT ( 'NONE',  ( 16.46253265017160672, -9.564922557960803928, 33.33224293864770260 ) ) ;
#40597=CARTESIAN_POINT ( 'NONE',  ( 19.02544592524343514, -5.153800228976328945, 33.54057627198102409 ) ) ;
#40599=CARTESIAN_POINT ( 'NONE',  ( 5.719274019375673035, 21.55341960407619339, 97.29275706135234714 ) ) ;
#40600=CARTESIAN_POINT ( 'NONE',  ( 12.06949235617739724, 12.14591786802326823, 46.87609039468568994 ) ) ;
#40601=CARTESIAN_POINT ( 'NONE',  ( 18.67979575497194134, -10.72451020669871369, 85.83442372801901854 ) ) ;
#40602=CARTESIAN_POINT ( 'NONE',  ( 9.564922557960805705, 16.46253265017160317, 114.5822429386476955 ) ) ;
#40603=CARTESIAN_POINT ( 'NONE',  ( 5.153800228976615827, -19.02544592524334988, 90.20942372801900433 ) ) ;
#40604=CARTESIAN_POINT ( 'NONE',  ( 5.719274019375673035, 21.55341960407619339, 57.29275706135234714 ) ) ;
#40605=CARTESIAN_POINT ( 'NONE',  ( 8.224510206698742110, 14.34966873604972548, 27.08442372801901854 ) ) ;
#40607=CARTESIAN_POINT ( 'NONE',  ( -5.049401038297874678, -19.05341960407617918, 84.79275706135233293 ) ) ;
#40608=CARTESIAN_POINT ( 'NONE',  ( 19.05341960407611168, 5.049401038298154454, 48.95724293864768129 ) ) ;
#40609=CARTESIAN_POINT ( 'NONE',  ( 9.474510206698729675, 16.51473224551082808, 97.08442372801900433 ) ) ;
#40610=CARTESIAN_POINT ( 'NONE',  ( 16.46253265017146816, 9.564922557961045513, 86.66775706135233293 ) ) ;
#40611=CARTESIAN_POINT ( 'NONE',  ( -4.483927247898539470, -16.52544592524342804, 57.29057627198103120 ) ) ;
#40612=CARTESIAN_POINT ( 'NONE',  ( -5.049401038297874678, -19.05341960407617918, 79.79275706135233293 ) ) ;
#40613=CARTESIAN_POINT ( 'NONE',  ( 8.314922557961029526, -14.29746914071037800, 65.41775706135234714 ) ) ;
#40614=CARTESIAN_POINT ( 'NONE',  ( -19.03943276465977164, -0.05219959533935918106, 28.75109039468566507 ) ) ;
#40615=CARTESIAN_POINT ( 'NONE',  ( 19.02544592524343514, -5.153800228976328945, 38.54057627198103120 ) ) ;
#40616=CARTESIAN_POINT ( 'NONE',  ( -19.03943276465977164, 0.05219959533909376836, 46.24890960531435979 ) ) ;
#40617=CARTESIAN_POINT ( 'NONE',  ( 0.05219959533934541429, -16.53943276465976808, 65.00109039468568994 ) ) ;
#40620=CARTESIAN_POINT ( 'NONE',  ( 16.51473224551069308, 9.474510206698969483, 109.1655762719810383 ) ) ;
#40623=CARTESIAN_POINT ( 'NONE',  ( -19.05341960407617563, 5.049401038297882671, 93.54275706135234714 ) ) ;
#40624=CARTESIAN_POINT ( 'NONE',  ( -15.80617190586745835, -15.72974639402198527, 41.87390960531435979 ) ) ;
#40625=CARTESIAN_POINT ( 'NONE',  ( -19.02544592524334988, -5.153800228976617603, 28.95942372801900433 ) ) ;
#40626=CARTESIAN_POINT ( 'NONE',  ( 5.153800228976615827, -19.02544592524334988, 105.2094237280190185 ) ) ;
#40627=CARTESIAN_POINT ( 'NONE',  ( -9.474510206698964154, 16.51473224551069663, 35.41557627198102409 ) ) ;
#40628=CARTESIAN_POINT ( 'NONE',  ( 16.46253265017160672, -9.564922557960803928, 43.33224293864769550 ) ) ;
#40629=CARTESIAN_POINT ( 'NONE',  ( -21.55341960407610458, -5.719274019375992779, 76.45724293864769550 ) ) ;
#40631=CARTESIAN_POINT ( 'NONE',  ( -16.51473224551069308, -9.474510206698971260, 31.66557627198102054 ) ) ;
#40633=CARTESIAN_POINT ( 'NONE',  ( -19.02544592524334988, -5.153800228976617603, 83.95942372801901854 ) ) ;
#40634=CARTESIAN_POINT ( 'NONE',  ( 8.314922557960818139, 14.29746914071049879, 59.58224293864770260 ) ) ;
#40635=CARTESIAN_POINT ( 'NONE',  ( -5.823673210054116645, -21.52544592524344225, 32.29057627198102409 ) ) ;
#40636=CARTESIAN_POINT ( 'NONE',  ( 10.72451020669871369, 18.67979575497193778, 107.0844237280190043 ) ) ;
#40637=CARTESIAN_POINT ( 'NONE',  ( 5.823673210054125526, 21.52544592524343514, 84.79057627198102409 ) ) ;
#40638=CARTESIAN_POINT ( 'NONE',  ( 15.80617190586769283, -15.72974639402175789, 70.62609039468567573 ) ) ;
#40639=CARTESIAN_POINT ( 'NONE',  ( 21.52544592524334988, 5.823673210054432836, 61.45942372801901854 ) ) ;
#40640=CARTESIAN_POINT ( 'NONE',  ( -5.049401038298153566, 19.05341960407611168, 105.2072429386476671 ) ) ;
#40641=CARTESIAN_POINT ( 'NONE',  ( 8.224510206698742110, 14.34966873604972548, 107.0844237280190043 ) ) ;
#40642=CARTESIAN_POINT ( 'NONE',  ( -5.823673210054431948, 21.52544592524334988, 57.70942372801901143 ) ) ;
#40643=CARTESIAN_POINT ( 'NONE',  ( -0.05219959533909027116, -19.03943276465977164, 57.49890960531435979 ) ) ;
#40644=CARTESIAN_POINT ( 'NONE',  ( -5.153800228976607833, 19.02544592524334988, 32.70942372801899722 ) ) ;
#40645=CARTESIAN_POINT ( 'NONE',  ( -18.67979575497193778, 10.72451020669871902, 28.33442372801902209 ) ) ;
#40646=CARTESIAN_POINT ( 'NONE',  ( -19.03943276465977164, 0.05219959533909376836, 66.24890960531436690 ) ) ;
#40647=CARTESIAN_POINT ( 'NONE',  ( -4.483927247898539470, -16.52544592524342804, 77.29057627198102409 ) ) ;
#40648=CARTESIAN_POINT ( 'NONE',  ( -0.05219959533910754901, -16.53943276465976808, 47.49890960531435979 ) ) ;
#40649=CARTESIAN_POINT ( 'NONE',  ( 21.52544592524344225, -5.823673210054117533, 63.54057627198103830 ) ) ;
#40650=CARTESIAN_POINT ( 'NONE',  ( 16.46253265017160672, -9.564922557960803928, 53.33224293864768839 ) ) ;
#40651=CARTESIAN_POINT ( 'NONE',  ( -10.81492255796078084, -18.62759615963271287, 72.08224293864769550 ) ) ;
#40652=CARTESIAN_POINT ( 'NONE',  ( -16.46253265017146816, -9.564922557961047289, 49.16775706135233293 ) ) ;
#40654=CARTESIAN_POINT ( 'NONE',  ( -16.53943276465976808, 0.05219959533911058130, 61.24890960531435979 ) ) ;
#40655=CARTESIAN_POINT ( 'NONE',  ( 21.53943276465977519, -0.05219959533907433946, 43.74890960531435979 ) ) ;
#40656=ORIENTED_EDGE ( 'NONE', *, *, #71324, .T. ) ;
#40657=CARTESIAN_POINT ( 'NONE',  ( 16.29526858892874941, 7.335722546920130149, 103.2967059780020662 ) ) ;
#40658=CARTESIAN_POINT ( 'NONE',  ( -8.314922557961024197, 14.29746914071037800, 82.91775706135234714 ) ) ;
#40660=CARTESIAN_POINT ( 'NONE',  ( 13.89961937509957401, 13.97604488694547697, 91.87609039468567573 ) ) ;
#40661=CARTESIAN_POINT ( 'NONE',  ( -4.483927247898539470, -16.52544592524342804, 52.29057627198102409 ) ) ;
#40662=CARTESIAN_POINT ( 'NONE',  ( -18.39639308325436673, -5.500000000000039080, 61.48252246182197212 ) ) ;
#40663=CARTESIAN_POINT ( 'NONE',  ( 19.05341960407611168, 5.049401038298154454, 43.95724293864769550 ) ) ;
#40664=CARTESIAN_POINT ( 'NONE',  ( -16.52544592524342804, 4.483927247898546575, 36.04057627198102409 ) ) ;
#40665=CARTESIAN_POINT ( 'NONE',  ( 13.97604488694527802, 13.89961937509977652, 94.37390960531436690 ) ) ;
#40666=CARTESIAN_POINT ( 'NONE',  ( -16.51473224551069308, -9.474510206698971260, 56.66557627198103120 ) ) ;
#40667=CARTESIAN_POINT ( 'NONE',  ( -21.52544592524334988, -5.823673210054445271, 53.95942372801900433 ) ) ;
#40668=CARTESIAN_POINT ( 'NONE',  ( 19.03943276465977164, -0.05219959533909143690, 68.74890960531436690 ) ) ;
#40669=CARTESIAN_POINT ( 'NONE',  ( -9.564922557960796823, -16.46253265017161027, 27.08224293864769550 ) ) ;
#40670=CARTESIAN_POINT ( 'NONE',  ( -0.05219959533909027116, -19.03943276465977164, 72.49890960531435269 ) ) ;
#40671=CARTESIAN_POINT ( 'NONE',  ( 21.52544592524344225, -5.823673210054117533, 48.54057627198103120 ) ) ;
#40672=CARTESIAN_POINT ( 'NONE',  ( 19.05341960407611168, 5.049401038298154454, 33.95724293864769550 ) ) ;
#40673=CARTESIAN_POINT ( 'NONE',  ( 5.823673210054125526, 21.52544592524343514, 34.79057627198103120 ) ) ;
#40674=CARTESIAN_POINT ( 'NONE',  ( -14.34966873604972548, 8.224510206698743886, 108.3344237280190185 ) ) ;
#40675=CARTESIAN_POINT ( 'NONE',  ( -16.46253265017146816, -9.564922557961047289, 24.16775706135233648 ) ) ;
#40676=CARTESIAN_POINT ( 'NONE',  ( -12.14591786802326823, 12.06949235617739902, 43.12609039468568284 ) ) ;
#40677=CARTESIAN_POINT ( 'NONE',  ( 8.224510206698742110, 14.34966873604972548, 87.08442372801901854 ) ) ;
#40678=CYLINDRICAL_SURFACE ( 'NONE', #4812, 2.500000000000002220 ) ;
#40679=CARTESIAN_POINT ( 'NONE',  ( 16.53943276465976808, 0.05219959533934440121, 61.25109039468567573 ) ) ;
#40680=CARTESIAN_POINT ( 'NONE',  ( -13.97604488694527625, -13.89961937509977652, 106.8739096053143669 ) ) ;
#40681=CARTESIAN_POINT ( 'NONE',  ( 9.474510206698971260, -16.51473224551069308, 37.91557627198102409 ) ) ;
#40682=CARTESIAN_POINT ( 'NONE',  ( 14.34966873604972726, -8.224510206698740333, 40.83442372801901854 ) ) ;
#40683=CARTESIAN_POINT ( 'NONE',  ( -0.05219959533909027116, -19.03943276465977164, 42.49890960531435269 ) ) ;
#40684=CARTESIAN_POINT ( 'NONE',  ( -10.81492255796105439, 18.62759615963255655, 32.91775706135234714 ) ) ;
#40685=CARTESIAN_POINT ( 'NONE',  ( -12.06949235617739369, -12.14591786802326823, 29.37609039468568284 ) ) ;
#40686=CARTESIAN_POINT ( 'NONE',  ( -16.53943276465976808, -0.05219959533934237506, 98.75109039468568994 ) ) ;
#40688=CARTESIAN_POINT ( 'NONE',  ( -5.719274019375665041, -21.55341960407619695, 94.79275706135234714 ) ) ;
#40689=CARTESIAN_POINT ( 'NONE',  ( 19.05341960407617918, -5.049401038297876454, 96.04275706135231871 ) ) ;
#40690=CARTESIAN_POINT ( 'NONE',  ( -9.564922557961040184, 16.46253265017147172, 57.91775706135233293 ) ) ;
#40691=CARTESIAN_POINT ( 'NONE',  ( 16.52544592524342804, -4.483927247898539470, 58.54057627198103120 ) ) ;
#40692=CARTESIAN_POINT ( 'NONE',  ( 16.55341960407611168, 4.379528057220329451, 113.9572429386477239 ) ) ;
#40693=CARTESIAN_POINT ( 'NONE',  ( 16.51473224551083163, -9.474510206698727899, 60.83442372801900433 ) ) ;
#40694=CARTESIAN_POINT ( 'NONE',  ( 16.31925111598458145, 7.325300261831480420, 77.33575461032749843 ) ) ;
#40695=CARTESIAN_POINT ( 'NONE',  ( -21.53943276465977519, -0.05219959533937600094, 63.75109039468568284 ) ) ;
#40696=CARTESIAN_POINT ( 'NONE',  ( 16.53943276465976808, 0.05219959533934440121, 21.25109039468567218 ) ) ;
#40698=CARTESIAN_POINT ( 'NONE',  ( 21.53943276465977519, -0.05219959533907433946, 23.74890960531435269 ) ) ;
#40699=CARTESIAN_POINT ( 'NONE',  ( 9.474510206698729675, 16.51473224551082808, 107.0844237280190043 ) ) ;
#40700=CARTESIAN_POINT ( 'NONE',  ( 5.049401038298161559, -19.05341960407611168, 112.7072429386476813 ) ) ;
#40702=CARTESIAN_POINT ( 'NONE',  ( 19.03943276465977164, -0.05219959533909143690, 23.74890960531435269 ) ) ;
#40703=CARTESIAN_POINT ( 'NONE',  ( -0.05219959533937732626, 21.53943276465977519, 102.5010903946856899 ) ) ;
#40704=CARTESIAN_POINT ( 'NONE',  ( 0.05219959533909260263, 19.03943276465977164, 59.99890960531436690 ) ) ;
#40706=CARTESIAN_POINT ( 'NONE',  ( 18.62759615963255655, 10.81492255796105972, 71.66775706135234714 ) ) ;
#40707=ADVANCED_FACE ( 'NONE', ( #129760 ), #61712, .T. ) ;
#40708=CARTESIAN_POINT ( 'NONE',  ( -18.62759615963255300, -10.81492255796106328, 104.1677570613523471 ) ) ;
#40709=CARTESIAN_POINT ( 'NONE',  ( 8.224510206698742110, 14.34966873604972548, 107.0844237280190043 ) ) ;
#40710=CARTESIAN_POINT ( 'NONE',  ( 9.474510206698971260, -16.51473224551069308, 72.91557627198102409 ) ) ;
#40711=CARTESIAN_POINT ( 'NONE',  ( 18.62759615963255655, 10.81492255796105972, 51.66775706135234714 ) ) ;
#40712=CARTESIAN_POINT ( 'NONE',  ( 21.55341960407619695, -5.719274019375665929, 51.04275706135234714 ) ) ;
#40713=CARTESIAN_POINT ( 'NONE',  ( -16.46253265017146816, -9.564922557961047289, 84.16775706135233293 ) ) ;
#40714=CARTESIAN_POINT ( 'NONE',  ( 9.474510206698971260, -16.51473224551069308, 102.9155762719810241 ) ) ;
#40715=CARTESIAN_POINT ( 'NONE',  ( 19.03943276465977164, -0.05219959533909143690, 23.74890960531435269 ) ) ;
#40716=CARTESIAN_POINT ( 'NONE',  ( 18.62759615963271287, -10.81492255796078972, 103.3322429386476955 ) ) ;
#40717=CARTESIAN_POINT ( 'NONE',  ( 5.153800228976615827, -19.02544592524334988, 20.20942372801899722 ) ) ;
#40718=CARTESIAN_POINT ( 'NONE',  ( 16.55341960407611168, 4.379528057220329451, 103.9572429386476813 ) ) ;
#40719=CARTESIAN_POINT ( 'NONE',  ( -13.89961937509977652, 13.97604488694528158, 50.62390960531435979 ) ) ;
#40720=CARTESIAN_POINT ( 'NONE',  ( -19.05341960407617563, 5.049401038297882671, 93.54275706135234714 ) ) ;
#40721=CARTESIAN_POINT ( 'NONE',  ( -4.483927247898539470, -16.52544592524342804, 67.29057627198103830 ) ) ;
#40722=CARTESIAN_POINT ( 'NONE',  ( 10.81492255796106328, -18.62759615963255655, 105.4177570613523613 ) ) ;
#40723=CARTESIAN_POINT ( 'NONE',  ( -5.049401038298153566, 19.05341960407611168, 105.2072429386476671 ) ) ;
#40724=CARTESIAN_POINT ( 'NONE',  ( 19.05341960407617918, -5.049401038297876454, 76.04275706135230450 ) ) ;
#40725=CARTESIAN_POINT ( 'NONE',  ( -5.823673210054116645, -21.52544592524344225, 82.29057627198103830 ) ) ;
#40726=CARTESIAN_POINT ( 'NONE',  ( -21.55341960407619339, 5.719274019375674811, 33.54275706135234714 ) ) ;
#40727=CARTESIAN_POINT ( 'NONE',  ( -4.483927247898782831, 16.52544592524335698, 37.70942372801900433 ) ) ;
#40728=CARTESIAN_POINT ( 'NONE',  ( 16.55341960407618274, -4.379528057220086978, 96.04275706135236135 ) ) ;
#40729=CARTESIAN_POINT ( 'NONE',  ( -0.05219959533934338120, 16.53943276465976808, 37.50109039468568284 ) ) ;
#40730=CARTESIAN_POINT ( 'NONE',  ( 21.53943276465977519, 0.05219959533937863772, 41.25109039468568284 ) ) ;
#40731=CARTESIAN_POINT ( 'NONE',  ( -21.52544592524343514, 5.823673210054127303, 41.04057627198103120 ) ) ;
#40732=CARTESIAN_POINT ( 'NONE',  ( -16.46253265017160317, 9.564922557960807481, 35.83224293864768839 ) ) ;
#40734=CARTESIAN_POINT ( 'NONE',  ( -0.05219959533934338120, 16.53943276465976808, 62.50109039468568284 ) ) ;
#40735=CARTESIAN_POINT ( 'NONE',  ( 15.80617190586746368, 15.72974639402197994, 84.37390960531438111 ) ) ;
#40736=CARTESIAN_POINT ( 'NONE',  ( 8.314922557960818139, 14.29746914071049879, 39.58224293864769550 ) ) ;
#40737=CARTESIAN_POINT ( 'NONE',  ( -16.53943276465976808, -0.05219959533934237506, 53.75109039468568994 ) ) ;
#40738=CARTESIAN_POINT ( 'NONE',  ( 5.049401038298161559, -19.05341960407611168, 57.70724293864769550 ) ) ;
#40739=CARTESIAN_POINT ( 'NONE',  ( 14.34966873604972726, -8.224510206698740333, 90.83442372801901854 ) ) ;
#40740=CARTESIAN_POINT ( 'NONE',  ( -13.97604488694547697, 13.89961937509957934, 83.12609039468564731 ) ) ;
#40741=CARTESIAN_POINT ( 'NONE',  ( -5.719274019375978568, 21.55341960407610458, 80.20724293864769550 ) ) ;
#40742=CARTESIAN_POINT ( 'NONE',  ( 16.55341960407611168, 4.379528057220329451, 28.95724293864769905 ) ) ;
#40745=EDGE_CURVE ( 'NONE', #21338, #141920, #151982, .T. ) ;
#40746=CARTESIAN_POINT ( 'NONE',  ( 10.72451020669898902, -18.67979575497178502, 57.91557627198103120 ) ) ;
#40747=CARTESIAN_POINT ( 'NONE',  ( -0.05219959533934338120, 16.53943276465976808, 102.5010903946856899 ) ) ;
#40749=CARTESIAN_POINT ( 'NONE',  ( 17.50000000000005684, -3.926509638704657856, 102.9170501086137790 ) ) ;
#40750=CARTESIAN_POINT ( 'NONE',  ( 18.62759615963271287, -10.81492255796078972, 88.33224293864769550 ) ) ;
#40751=CIRCLE ( 'NONE', #179615, 2.500000000000002220 ) ;
#40752=CARTESIAN_POINT ( 'NONE',  ( -16.53943276465976808, 0.05219959533911058130, 21.24890960531436690 ) ) ;
#40753=CARTESIAN_POINT ( 'NONE',  ( 0.05219959533934541429, -16.53943276465976808, 40.00109039468567573 ) ) ;
#40754=CARTESIAN_POINT ( 'NONE',  ( -9.474510206698964154, 16.51473224551069663, 30.41557627198102054 ) ) ;
#40755=CARTESIAN_POINT ( 'NONE',  ( 13.89961937509977652, -13.97604488694527269, 63.12390960531435979 ) ) ;
#40757=CARTESIAN_POINT ( 'NONE',  ( -18.62759615963270932, 10.81492255796079327, 25.83224293864769194 ) ) ;
#40759=CARTESIAN_POINT ( 'NONE',  ( 14.34966873604972726, -8.224510206698740333, 100.8344237280190185 ) ) ;
#40760=CARTESIAN_POINT ( 'NONE',  ( 19.05341960407617918, -5.049401038297876454, 101.0427570613523045 ) ) ;
#40761=CARTESIAN_POINT ( 'NONE',  ( 19.02544592524334988, 5.153800228976608722, 36.45942372801900433 ) ) ;
#40762=CARTESIAN_POINT ( 'NONE',  ( 15.80617190586746368, 15.72974639402197994, 84.37390960531438111 ) ) ;
#40763=CARTESIAN_POINT ( 'NONE',  ( 16.55341960407618274, -4.379528057220086978, 111.0427570613523613 ) ) ;
#40764=CARTESIAN_POINT ( 'NONE',  ( 5.823673210054125526, 21.52544592524343514, 29.79057627198102409 ) ) ;
#40765=CARTESIAN_POINT ( 'NONE',  ( 13.89961937509957401, 13.97604488694547697, 111.8760903946856757 ) ) ;
#40766=CARTESIAN_POINT ( 'NONE',  ( 9.564922557960805705, 16.46253265017160317, 109.5822429386476955 ) ) ;
#40767=CARTESIAN_POINT ( 'NONE',  ( -5.823673210054431948, 21.52544592524334988, 62.70942372801902565 ) ) ;
#40768=CARTESIAN_POINT ( 'NONE',  ( 16.46253265017160672, -9.564922557960803928, 58.33224293864769550 ) ) ;
#40769=CARTESIAN_POINT ( 'NONE',  ( -12.06949235617756955, 12.14591786802309770, 95.62390960531436690 ) ) ;
#40771=CARTESIAN_POINT ( 'NONE',  ( -16.51473224551069308, -9.474510206698971260, 71.66557627198102409 ) ) ;
#40772=CARTESIAN_POINT ( 'NONE',  ( 4.379528057220339221, -16.55341960407611168, 72.70724293864769550 ) ) ;
#40773=ORIENTED_EDGE ( 'NONE', *, *, #96707, .F. ) ;
#40774=CARTESIAN_POINT ( 'NONE',  ( 16.46253265017146816, 9.564922557961045513, 86.66775706135233293 ) ) ;
#40776=CARTESIAN_POINT ( 'NONE',  ( -19.03943276465977164, 0.05219959533909376836, 66.24890960531436690 ) ) ;
#40778=CARTESIAN_POINT ( 'NONE',  ( -9.564922557960796823, -16.46253265017161027, 72.08224293864770971 ) ) ;
#40779=CARTESIAN_POINT ( 'NONE',  ( -19.02544592524342804, 5.153800228976336051, 101.0405762719810241 ) ) ;
#40780=CARTESIAN_POINT ( 'NONE',  ( 8.314922557961029526, -14.29746914071037800, 60.41775706135235424 ) ) ;
#40782=CARTESIAN_POINT ( 'NONE',  ( -19.03943276465977164, -0.05219959533935918106, 43.75109039468566863 ) ) ;
#40783=CARTESIAN_POINT ( 'NONE',  ( 10.72451020669871369, 18.67979575497193778, 97.08442372801904696 ) ) ;
#40785=CARTESIAN_POINT ( 'NONE',  ( 5.049401038298161559, -19.05341960407611168, 112.7072429386476813 ) ) ;
#40786=CARTESIAN_POINT ( 'NONE',  ( -8.224510206698735004, -14.34966873604973081, 99.58442372801900433 ) ) ;
#40788=CARTESIAN_POINT ( 'NONE',  ( 16.52544592524335698, 4.483927247898782831, 86.45942372801901854 ) ) ;
#40790=CARTESIAN_POINT ( 'NONE',  ( -8.224510206698735004, -14.34966873604973081, 69.58442372801900433 ) ) ;
#40791=VERTEX_POINT ( 'NONE', #7662 ) ;
#40792=CARTESIAN_POINT ( 'NONE',  ( -10.72451020669870658, -18.67979575497194134, 79.58442372801903275 ) ) ;
#40793=CARTESIAN_POINT ( 'NONE',  ( 5.153800228976615827, -19.02544592524334988, 85.20942372801900433 ) ) ;
#40794=CARTESIAN_POINT ( 'NONE',  ( -0.05219959533936034679, 19.03943276465977164, 32.50109039468566863 ) ) ;
#40795=CARTESIAN_POINT ( 'NONE',  ( -16.51473224551069308, -9.474510206698971260, 71.66557627198102409 ) ) ;
#40796=CARTESIAN_POINT ( 'NONE',  ( 5.049401038298161559, -19.05341960407611168, 57.70724293864769550 ) ) ;
#40797=CARTESIAN_POINT ( 'NONE',  ( 16.45676962205255833, -7.258233047195244758, 22.85181134416914617 ) ) ;
#40798=CARTESIAN_POINT ( 'NONE',  ( 0.05219959533907565091, 21.53943276465977519, 79.99890960531435269 ) ) ;
#40799=CARTESIAN_POINT ( 'NONE',  ( 15.72974639402199770, -15.80617190586745480, 38.12390960531436690 ) ) ;
#40800=CARTESIAN_POINT ( 'NONE',  ( 0.05219959533909260263, 19.03943276465977164, 39.99890960531436690 ) ) ;
#40801=CARTESIAN_POINT ( 'NONE',  ( 8.314922557961029526, -14.29746914071037800, 65.41775706135234714 ) ) ;
#40803=CARTESIAN_POINT ( 'NONE',  ( 21.52544592524334988, 5.823673210054432836, 36.45942372801901143 ) ) ;
#40804=CARTESIAN_POINT ( 'NONE',  ( -16.53943276465976808, 0.05219959533911058130, 61.24890960531435979 ) ) ;
#40806=CARTESIAN_POINT ( 'NONE',  ( 0.05219959533934541429, -16.53943276465976808, 20.00109039468568639 ) ) ;
#40807=CARTESIAN_POINT ( 'NONE',  ( 16.51473224551083163, -9.474510206698727899, 50.83442372801899722 ) ) ;
#40808=CARTESIAN_POINT ( 'NONE',  ( 16.53943276465976808, -0.05219959533910856209, 53.74890960531437401 ) ) ;
#40809=CARTESIAN_POINT ( 'NONE',  ( 5.719274019375673035, 21.55341960407619339, 22.29275706135235069 ) ) ;
#40810=CARTESIAN_POINT ( 'NONE',  ( 0.05219959533909260263, 19.03943276465977164, 99.99890960531436690 ) ) ;
#40811=CARTESIAN_POINT ( 'NONE',  ( -5.719274019375978568, 21.55341960407610458, 80.20724293864769550 ) ) ;
#40812=CARTESIAN_POINT ( 'NONE',  ( -19.03943276465977164, 0.05219959533909376836, 86.24890960531436690 ) ) ;
#40813=CARTESIAN_POINT ( 'NONE',  ( 12.14591786802309770, 12.06949235617756955, 59.37390960531436690 ) ) ;
#40816=CARTESIAN_POINT ( 'NONE',  ( 19.02544592524334988, 5.153800228976608722, 71.45942372801900433 ) ) ;
#40817=CARTESIAN_POINT ( 'NONE',  ( -15.72974639402197994, 15.80617190586746368, 105.6239096053143669 ) ) ;
#40818=CARTESIAN_POINT ( 'NONE',  ( -5.153800228976328057, -19.02544592524343514, 62.29057627198100988 ) ) ;
#40819=CARTESIAN_POINT ( 'NONE',  ( -9.474510206698720793, -16.51473224551083518, 49.58442372801899722 ) ) ;
#40820=CARTESIAN_POINT ( 'NONE',  ( -16.51473224551069308, -9.474510206698971260, 31.66557627198102054 ) ) ;
#40821=CARTESIAN_POINT ( 'NONE',  ( 15.72974639402176855, 15.80617190586768217, 61.87609039468568284 ) ) ;
#40823=CARTESIAN_POINT ( 'NONE',  ( -14.29746914071049879, 8.314922557960819915, 45.83224293864769550 ) ) ;
#40824=CARTESIAN_POINT ( 'NONE',  ( 19.05341960407611168, 5.049401038298154454, 58.95724293864768129 ) ) ;
#40825=CARTESIAN_POINT ( 'NONE',  ( -15.72974639402197994, 15.80617190586746368, 70.62390960531436690 ) ) ;
#40826=CARTESIAN_POINT ( 'NONE',  ( -9.474510206698964154, 16.51473224551069663, 55.41557627198103120 ) ) ;
#40828=CARTESIAN_POINT ( 'NONE',  ( -10.72451020669898014, 18.67979575497178502, 65.41557627198102409 ) ) ;
#40829=CARTESIAN_POINT ( 'NONE',  ( -5.719274019375665041, -21.55341960407619695, 94.79275706135234714 ) ) ;
#40830=CARTESIAN_POINT ( 'NONE',  ( 18.22780087662121673, 5.500000000000056843, 73.98459894673894155 ) ) ;
#40831=CARTESIAN_POINT ( 'NONE',  ( 16.55341960407618274, -4.379528057220086978, 101.0427570613523756 ) ) ;
#40832=CARTESIAN_POINT ( 'NONE',  ( 0.05219959533910956823, 16.53943276465976808, 84.99890960531436690 ) ) ;
#40833=CARTESIAN_POINT ( 'NONE',  ( -13.97604488694547697, 13.89961937509957934, 88.12609039468563310 ) ) ;
#40835=CARTESIAN_POINT ( 'NONE',  ( -13.89961937509957401, -13.97604488694547875, 44.37609039468566863 ) ) ;
#40836=CARTESIAN_POINT ( 'NONE',  ( 12.06949235617739724, 12.14591786802326823, 106.8760903946856899 ) ) ;
#40837=CARTESIAN_POINT ( 'NONE',  ( 5.049401038297881783, 19.05341960407617563, 27.29275706135232937 ) ) ;
#40838=CARTESIAN_POINT ( 'NONE',  ( -19.05341960407611168, -5.049401038298163336, 86.45724293864769550 ) ) ;
#40839=CARTESIAN_POINT ( 'NONE',  ( -21.53943276465977519, 0.05219959533907696930, 56.24890960531436690 ) ) ;
#40840=CARTESIAN_POINT ( 'NONE',  ( -18.39635199886965822, 5.500000000000101252, 51.01967076359998998 ) ) ;
#40841=CARTESIAN_POINT ( 'NONE',  ( 12.06949235617757843, -12.14591786802309237, 113.1239096053143953 ) ) ;
#40842=CARTESIAN_POINT ( 'NONE',  ( -10.72451020669870658, -18.67979575497194134, 89.58442372801901854 ) ) ;
#40843=CARTESIAN_POINT ( 'NONE',  ( 16.52544592524335698, 4.483927247898782831, 81.45942372801900433 ) ) ;
#40844=CARTESIAN_POINT ( 'NONE',  ( -15.72974639402176322, -15.80617190586768395, 24.37609039468567573 ) ) ;
#40845=CARTESIAN_POINT ( 'NONE',  ( -4.379528057220086978, -16.55341960407618274, 24.79275706135235779 ) ) ;
#40846=CARTESIAN_POINT ( 'NONE',  ( -19.05341960407611168, -5.049401038298163336, 111.4572429386476671 ) ) ;
#40847=CARTESIAN_POINT ( 'NONE',  ( 9.564922557960805705, 16.46253265017160317, 44.58224293864769550 ) ) ;
#40848=CARTESIAN_POINT ( 'NONE',  ( 9.564922557960805705, 16.46253265017160317, 49.58224293864770260 ) ) ;
#40850=CARTESIAN_POINT ( 'NONE',  ( -14.34966873604972548, 8.224510206698743886, 33.33442372801900433 ) ) ;
#40851=CARTESIAN_POINT ( 'NONE',  ( 16.53943276465976808, -0.05219959533910856209, 93.74890960531436690 ) ) ;
#40852=CARTESIAN_POINT ( 'NONE',  ( -16.55341960407617563, 4.379528057220093196, 98.54275706135234714 ) ) ;
#40853=CARTESIAN_POINT ( 'NONE',  ( 5.719274019375673035, 21.55341960407619339, 37.29275706135235424 ) ) ;
#40854=CARTESIAN_POINT ( 'NONE',  ( 5.153800228976335163, 19.02544592524342804, 79.79057627198102409 ) ) ;
#40855=CARTESIAN_POINT ( 'NONE',  ( -19.02544592524342804, 5.153800228976336051, 66.04057627198103830 ) ) ;
#40856=CARTESIAN_POINT ( 'NONE',  ( -19.03943276465977164, 0.05219959533909376836, 86.24890960531436690 ) ) ;
#40857=CARTESIAN_POINT ( 'NONE',  ( -0.05219959533910754901, -16.53943276465976808, 27.49890960531435269 ) ) ;
#40858=CARTESIAN_POINT ( 'NONE',  ( 14.29746914071037800, 8.314922557961029526, 101.6677570613523613 ) ) ;
#40859=ORIENTED_EDGE ( 'NONE', *, *, #46300, .T. ) ;
#40860=CARTESIAN_POINT ( 'NONE',  ( -16.51473224551082808, 9.474510206698731452, 48.33442372801900433 ) ) ;
#40861=CARTESIAN_POINT ( 'NONE',  ( 19.02544592524343514, -5.153800228976328945, 113.5405762719810241 ) ) ;
#40862=CARTESIAN_POINT ( 'NONE',  ( 0.05219959533909260263, 19.03943276465977164, 44.99890960531435979 ) ) ;
#40863=CARTESIAN_POINT ( 'NONE',  ( -13.89961937509957401, -13.97604488694547875, 34.37609039468566863 ) ) ;
#40865=CARTESIAN_POINT ( 'NONE',  ( -0.05219959533934338120, 16.53943276465976808, 47.50109039468568994 ) ) ;
#40866=CARTESIAN_POINT ( 'NONE',  ( 9.474510206698729675, 16.51473224551082808, 72.08442372801900433 ) ) ;
#40867=CARTESIAN_POINT ( 'NONE',  ( 4.379528057220092307, 16.55341960407617563, 52.29275706135236135 ) ) ;
#40869=CARTESIAN_POINT ( 'NONE',  ( -9.564922557960796823, -16.46253265017161027, 92.08224293864769550 ) ) ;
#40870=CARTESIAN_POINT ( 'NONE',  ( -10.72451020669898014, 18.67979575497178502, 115.4155762719810241 ) ) ;
#40871=CARTESIAN_POINT ( 'NONE',  ( -13.89961937509957401, -13.97604488694547875, 79.37609039468567573 ) ) ;
#40872=CARTESIAN_POINT ( 'NONE',  ( 13.89961937509977652, -13.97604488694527269, 108.1239096053143669 ) ) ;
#40873=CARTESIAN_POINT ( 'NONE',  ( 9.474510206698971260, -16.51473224551069308, 32.91557627198102409 ) ) ;
#40875=CARTESIAN_POINT ( 'NONE',  ( -19.03943276465977164, 0.05219959533909376836, 76.24890960531435269 ) ) ;
#40876=CARTESIAN_POINT ( 'NONE',  ( 0.05219959533910956823, 16.53943276465976808, 29.99890960531435979 ) ) ;
#40877=CARTESIAN_POINT ( 'NONE',  ( -19.02544592524342804, 5.153800228976336051, 31.04057627198102409 ) ) ;
#40878=CARTESIAN_POINT ( 'NONE',  ( -0.05219959533936034679, 19.03943276465977164, 52.50109039468566863 ) ) ;
#40879=CARTESIAN_POINT ( 'NONE',  ( 16.55341960407611168, 4.379528057220329451, 83.95724293864770971 ) ) ;
#40880=CARTESIAN_POINT ( 'NONE',  ( -15.80617190586768217, 15.72974639402176855, 108.1260903946856757 ) ) ;
#40881=CARTESIAN_POINT ( 'NONE',  ( 9.564922557960805705, 16.46253265017160317, 49.58224293864770260 ) ) ;
#40882=CARTESIAN_POINT ( 'NONE',  ( -5.719274019375978568, 21.55341960407610458, 50.20724293864769550 ) ) ;
#40883=CARTESIAN_POINT ( 'NONE',  ( -16.55341960407611168, -4.379528057220339221, 56.45724293864768839 ) ) ;
#40884=CARTESIAN_POINT ( 'NONE',  ( 10.81492255796106328, -18.62759615963255655, 105.4177570613523613 ) ) ;
#40885=CARTESIAN_POINT ( 'NONE',  ( -9.474510206698964154, 16.51473224551069663, 95.41557627198102409 ) ) ;
#40886=CARTESIAN_POINT ( 'NONE',  ( 9.474510206698971260, -16.51473224551069308, 112.9155762719810383 ) ) ;
#40887=CARTESIAN_POINT ( 'NONE',  ( 16.51473224551069308, 9.474510206698969483, 44.16557627198103120 ) ) ;
#40888=CARTESIAN_POINT ( 'NONE',  ( -16.51473224551069308, -9.474510206698971260, 26.66557627198103120 ) ) ;
#40889=CARTESIAN_POINT ( 'NONE',  ( 4.379528057220339221, -16.55341960407611168, 92.70724293864770971 ) ) ;
#40890=CARTESIAN_POINT ( 'NONE',  ( -15.72974639402197994, 15.80617190586746368, 90.62390960531436690 ) ) ;
#40891=CARTESIAN_POINT ( 'NONE',  ( 13.97604488694527802, 13.89961937509977652, 99.37390960531436690 ) ) ;
#40892=CARTESIAN_POINT ( 'NONE',  ( 15.80617190586769283, -15.72974639402175789, 20.62609039468568639 ) ) ;
#40893=CARTESIAN_POINT ( 'NONE',  ( -0.05219959533909027116, -19.03943276465977164, 92.49890960531436690 ) ) ;
#40895=CARTESIAN_POINT ( 'NONE',  ( -14.34966873604960291, -8.224510206698953496, 96.66557627198102409 ) ) ;
#40896=VECTOR ( 'NONE', #77106, 1000.000000000000000 ) ;
#40897=CARTESIAN_POINT ( 'NONE',  ( -16.51473224551069308, -9.474510206698971260, 76.66557627198103830 ) ) ;
#40898=CARTESIAN_POINT ( 'NONE',  ( 21.53943276465977519, -0.05219959533907433946, 78.74890960531436690 ) ) ;
#40901=CARTESIAN_POINT ( 'NONE',  ( -5.823673210054116645, -21.52544592524344225, 32.29057627198102409 ) ) ;
#40902=CARTESIAN_POINT ( 'NONE',  ( 18.56197773271731677, -5.499999999999892530, 66.05066217314451649 ) ) ;
#40903=CARTESIAN_POINT ( 'NONE',  ( 14.29746914071037800, 8.314922557961029526, 31.66775706135234358 ) ) ;
#40904=CARTESIAN_POINT ( 'NONE',  ( -12.06949235617756955, 12.14591786802309770, 100.6239096053143811 ) ) ;
#40906=CARTESIAN_POINT ( 'NONE',  ( -9.474510206698964154, 16.51473224551069663, 90.41557627198103830 ) ) ;
#40907=CARTESIAN_POINT ( 'NONE',  ( -5.049401038298153566, 19.05341960407611168, 50.20724293864770260 ) ) ;
#40908=CARTESIAN_POINT ( 'NONE',  ( 8.314922557960818139, 14.29746914071049879, 74.58224293864768129 ) ) ;
#40909=CARTESIAN_POINT ( 'NONE',  ( 18.67979575497178502, 10.72451020669898547, 29.16557627198103120 ) ) ;
#40910=CARTESIAN_POINT ( 'NONE',  ( 0.05219959533910956823, 16.53943276465976808, 49.99890960531437401 ) ) ;
#40911=CARTESIAN_POINT ( 'NONE',  ( -19.05341960407617563, 5.049401038297882671, 103.5427570613523329 ) ) ;
#40912=CARTESIAN_POINT ( 'NONE',  ( -21.55341960407619339, 5.719274019375674811, 68.54275706135234714 ) ) ;
#40914=CARTESIAN_POINT ( 'NONE',  ( -5.823673210054116645, -21.52544592524344225, 22.29057627198102765 ) ) ;
#40915=CARTESIAN_POINT ( 'NONE',  ( -16.53943276465976808, -0.05219959533934237506, 83.75109039468568994 ) ) ;
#40916=CARTESIAN_POINT ( 'NONE',  ( 9.474510206698971260, -16.51473224551069308, 22.91557627198102765 ) ) ;
#40917=CARTESIAN_POINT ( 'NONE',  ( 0.05219959533909260263, 19.03943276465977164, 74.99890960531435269 ) ) ;
#40918=CARTESIAN_POINT ( 'NONE',  ( 15.72974639402199770, -15.80617190586745480, 78.12390960531436690 ) ) ;
#40919=CARTESIAN_POINT ( 'NONE',  ( 14.29746914071037800, 8.314922557961029526, 31.66775706135234358 ) ) ;
#40920=CARTESIAN_POINT ( 'NONE',  ( 4.379528057220339221, -16.55341960407611168, 47.70724293864770260 ) ) ;
#40921=CARTESIAN_POINT ( 'NONE',  ( 15.80617190586769283, -15.72974639402175789, 75.62609039468567573 ) ) ;
#40922=CARTESIAN_POINT ( 'NONE',  ( 16.52544592524335698, 4.483927247898782831, 86.45942372801901854 ) ) ;
#40923=CARTESIAN_POINT ( 'NONE',  ( -0.05219959533907301413, -21.53943276465977519, 27.49890960531435269 ) ) ;
#40924=CARTESIAN_POINT ( 'NONE',  ( 19.03943276465977164, -0.05219959533909143690, 113.7489096053143669 ) ) ;
#40925=CARTESIAN_POINT ( 'NONE',  ( -16.18388926212238133, 7.379444403734528812, 79.56046848633847901 ) ) ;
#40926=CARTESIAN_POINT ( 'NONE',  ( 12.06949235617739724, 12.14591786802326823, 106.8760903946856899 ) ) ;
#40927=CARTESIAN_POINT ( 'NONE',  ( 8.224510206698742110, 14.34966873604972548, 57.08442372801901854 ) ) ;
#40928=CARTESIAN_POINT ( 'NONE',  ( -9.564922557960796823, -16.46253265017161027, 72.08224293864770971 ) ) ;
#40930=CARTESIAN_POINT ( 'NONE',  ( -0.05219959533909027116, -19.03943276465977164, 92.49890960531436690 ) ) ;
#40931=CARTESIAN_POINT ( 'NONE',  ( -0.05219959533937732626, 21.53943276465977519, 77.50109039468567573 ) ) ;
#40932=CARTESIAN_POINT ( 'NONE',  ( 8.314922557961029526, -14.29746914071037800, 75.41775706135233293 ) ) ;
#40933=CARTESIAN_POINT ( 'NONE',  ( 8.224510206698953496, -14.34966873604960469, 52.91557627198103830 ) ) ;
#40934=CARTESIAN_POINT ( 'NONE',  ( 13.97604488694527802, 13.89961937509977652, 49.37390960531434558 ) ) ;
#40935=CARTESIAN_POINT ( 'NONE',  ( 13.89961937509977652, -13.97604488694527269, 43.12390960531434558 ) ) ;
#40937=CARTESIAN_POINT ( 'NONE',  ( 13.89961937509957401, 13.97604488694547697, 96.87609039468566152 ) ) ;
#40938=CARTESIAN_POINT ( 'NONE',  ( -16.55341960407611168, -4.379528057220339221, 111.4572429386476813 ) ) ;
#40939=CARTESIAN_POINT ( 'NONE',  ( -13.97604488694527625, -13.89961937509977652, 61.87390960531435979 ) ) ;
#40940=CARTESIAN_POINT ( 'NONE',  ( -16.51473224551082808, 9.474510206698731452, 103.3344237280190043 ) ) ;
#40942=CARTESIAN_POINT ( 'NONE',  ( -10.81492255796105439, 18.62759615963255655, 107.9177570613523471 ) ) ;
#40943=CARTESIAN_POINT ( 'NONE',  ( -4.483927247898782831, 16.52544592524335698, 62.70942372801902565 ) ) ;
#40944=CARTESIAN_POINT ( 'NONE',  ( -19.05341960407617563, 5.049401038297882671, 88.54275706135230450 ) ) ;
#40945=CARTESIAN_POINT ( 'NONE',  ( -21.55341960407610458, -5.719274019375992779, 56.45724293864768839 ) ) ;
#40946=CARTESIAN_POINT ( 'NONE',  ( -4.379528057220086978, -16.55341960407618274, 49.79275706135234714 ) ) ;
#40948=CARTESIAN_POINT ( 'NONE',  ( 9.564922557961047289, -16.46253265017146816, 60.41775706135233293 ) ) ;
#40949=CARTESIAN_POINT ( 'NONE',  ( 18.62759615963255655, 10.81492255796105972, 101.6677570613523613 ) ) ;
#40950=CARTESIAN_POINT ( 'NONE',  ( -12.14591786802309592, -12.06949235617757132, 111.8739096053143669 ) ) ;
#40951=CARTESIAN_POINT ( 'NONE',  ( -5.049401038298153566, 19.05341960407611168, 65.20724293864765286 ) ) ;
#40952=CARTESIAN_POINT ( 'NONE',  ( 4.483927247898545687, 16.52544592524342804, 54.79057627198104541 ) ) ;
#40953=CARTESIAN_POINT ( 'NONE',  ( 15.72974639402176855, 15.80617190586768217, 86.87609039468568994 ) ) ;
#40955=CARTESIAN_POINT ( 'NONE',  ( 0.05219959533936267826, -19.03943276465977164, 45.00109039468566863 ) ) ;
#40956=CARTESIAN_POINT ( 'NONE',  ( -16.46253265017146816, -9.564922557961047289, 24.16775706135233648 ) ) ;
#40957=CARTESIAN_POINT ( 'NONE',  ( 21.53943276465977519, -0.05219959533907433946, 23.74890960531435269 ) ) ;
#40958=CARTESIAN_POINT ( 'NONE',  ( 5.719274019375673035, 21.55341960407619339, 97.29275706135234714 ) ) ;
#40959=CARTESIAN_POINT ( 'NONE',  ( -0.05219959533909027116, -19.03943276465977164, 72.49890960531435269 ) ) ;
#40960=CARTESIAN_POINT ( 'NONE',  ( -21.52544592524334988, -5.823673210054445271, 88.95942372801901854 ) ) ;
#40961=CARTESIAN_POINT ( 'NONE',  ( -10.81492255796078084, -18.62759615963271287, 52.08224293864768839 ) ) ;
#40962=CARTESIAN_POINT ( 'NONE',  ( -16.46253265017160317, 9.564922557960807481, 85.83224293864769550 ) ) ;
#40963=CARTESIAN_POINT ( 'NONE',  ( -9.474510206698720793, -16.51473224551083518, 59.58442372801900433 ) ) ;
#40964=CARTESIAN_POINT ( 'NONE',  ( -13.97604488694527625, -13.89961937509977652, 46.87390960531435979 ) ) ;
#40965=CARTESIAN_POINT ( 'NONE',  ( -19.02544592524342804, 5.153800228976336051, 96.04057627198103830 ) ) ;
#40966=CARTESIAN_POINT ( 'NONE',  ( -16.51473224551082808, 9.474510206698731452, 88.33442372801900433 ) ) ;
#40968=CARTESIAN_POINT ( 'NONE',  ( 12.06949235617739724, 12.14591786802326823, 46.87609039468568994 ) ) ;
#40969=CARTESIAN_POINT ( 'NONE',  ( -12.14591786802309592, -12.06949235617757132, 101.8739096053143811 ) ) ;
#40970=CARTESIAN_POINT ( 'NONE',  ( 5.153800228976335163, 19.02544592524342804, 69.79057627198103830 ) ) ;
#40972=CARTESIAN_POINT ( 'NONE',  ( -15.72974639402197994, 15.80617190586746368, 50.62390960531435979 ) ) ;
#40973=B_SPLINE_CURVE_WITH_KNOTS ( 'NONE', 3,
 ( #125798, #62128, #107635, #18631, #122810, #48966, #172302, #61138, #169312, #3439, #65115, #126773, #188478, #15647, #46980, #453, #111622, #77306, #138975, #123792, #142939, #81258 ),
 .UNSPECIFIED., .F., .F.,
 ( 4, 2, 2, 2, 2, 2, 2, 2, 2, 2, 4 ),
 ( 2.194270917860438266E-17, 0.001309639967555297629, 0.001964459951332936036, 0.002291869943221755239, 0.002455574939166158335, 0.002619279935110561432, 0.002782984931054964528, 0.002946689926999367624, 0.003274099918888187261, 0.003928919902665813958, 0.005238559870221069087 ),
 .UNSPECIFIED. ) ;
#40974=CARTESIAN_POINT ( 'NONE',  ( 12.14591786802327356, -12.06949235617739191, 20.62609039468568639 ) ) ;
#40975=CARTESIAN_POINT ( 'NONE',  ( -15.72974639402176322, -15.80617190586768395, 19.37609039468568639 ) ) ;
#40976=CARTESIAN_POINT ( 'NONE',  ( -5.823673210054431948, 21.52544592524334988, 82.70942372801900433 ) ) ;
#40977=CARTESIAN_POINT ( 'NONE',  ( 8.224510206698742110, 14.34966873604972548, 82.08442372801901854 ) ) ;
#40978=CARTESIAN_POINT ( 'NONE',  ( 5.049401038298161559, -19.05341960407611168, 77.70724293864765286 ) ) ;
#40979=CARTESIAN_POINT ( 'NONE',  ( 14.34966873604972726, -8.224510206698740333, 95.83442372801903275 ) ) ;
#40980=CARTESIAN_POINT ( 'NONE',  ( 16.51473224551083163, -9.474510206698727899, 60.83442372801900433 ) ) ;
#40981=CARTESIAN_POINT ( 'NONE',  ( -21.55341960407619339, 5.719274019375674811, 33.54275706135234714 ) ) ;
#40982=CARTESIAN_POINT ( 'NONE',  ( -8.224510206698948167, 14.34966873604960824, 75.41557627198102409 ) ) ;
#40983=CARTESIAN_POINT ( 'NONE',  ( 13.89961937509977652, -13.97604488694527269, 93.12390960531436690 ) ) ;
#40984=CARTESIAN_POINT ( 'NONE',  ( -16.52544592524335698, -4.483927247898792601, 88.95942372801901854 ) ) ;
#40985=B_SPLINE_CURVE_WITH_KNOTS ( 'NONE', 3,
 ( #54945, #196483, #11462, #118629, #57953, #150964, #116617, #72113, #74119, #180320, #73133, #178306, #147966, #133787, #101433, #134803, #104448, #165133, #39769, #181307, #166131, #151939, #27633, #102450, #120595, #89274, #148964, #41788, #90256, #163124, #9453, #86275 ),
 .UNSPECIFIED., .F., .F.,
 ( 4, 2, 2, 2, 2, 2, 2, 2, 2, 2, 2, 2, 2, 2, 2, 4 ),
 ( 2.969368287472575283E-17, 0.0003712461730037006557, 0.0007424923460073716043, 0.001113738519011042661, 0.001484984692014713501, 0.002227477038022055399, 0.002598723211025726239, 0.002969969384029397079, 0.003341215557033067919, 0.003712461730036738759, 0.004083707903040409599, 0.004454954076044081307, 0.004826200249047752147, 0.005197446422051422987, 0.005568692595055093827, 0.005939938768058764668 ),
 .UNSPECIFIED. ) ;
#40986=CARTESIAN_POINT ( 'NONE',  ( -10.81492255796105439, 18.62759615963255655, 67.91775706135234714 ) ) ;
#40987=CARTESIAN_POINT ( 'NONE',  ( 14.34966873604972726, -8.224510206698740333, 30.83442372801902209 ) ) ;
#40988=CARTESIAN_POINT ( 'NONE',  ( -18.62759615963255300, -10.81492255796106328, 34.16775706135234714 ) ) ;
#40989=CARTESIAN_POINT ( 'NONE',  ( -14.34966873604960291, -8.224510206698953496, 66.66557627198102409 ) ) ;
#40991=CARTESIAN_POINT ( 'NONE',  ( 21.52544592524344225, -5.823673210054117533, 98.54057627198105251 ) ) ;
#40992=CARTESIAN_POINT ( 'NONE',  ( -8.224510206698948167, 14.34966873604960824, 50.41557627198103120 ) ) ;
#40994=CARTESIAN_POINT ( 'NONE',  ( 9.474510206698971260, -16.51473224551069308, 22.91557627198102765 ) ) ;
#40995=CARTESIAN_POINT ( 'NONE',  ( 21.55341960407610458, 5.719274019375980345, 23.95724293864769550 ) ) ;
#40996=CARTESIAN_POINT ( 'NONE',  ( -21.52544592524334988, -5.823673210054445271, 43.95942372801902565 ) ) ;
#40997=CARTESIAN_POINT ( 'NONE',  ( 4.483927247898545687, 16.52544592524342804, 59.79057627198103120 ) ) ;
#40999=CARTESIAN_POINT ( 'NONE',  ( 21.52544592524344225, -5.823673210054117533, 68.54057627198103830 ) ) ;
#41000=CARTESIAN_POINT ( 'NONE',  ( 13.97604488694527802, 13.89961937509977652, 69.37390960531436690 ) ) ;
#41001=CARTESIAN_POINT ( 'NONE',  ( -19.05341960407611168, -5.049401038298163336, 21.45724293864768839 ) ) ;
#41002=CARTESIAN_POINT ( 'NONE',  ( 19.03943276465977164, 0.05219959533936151252, 81.25109039468567573 ) ) ;
#41003=CARTESIAN_POINT ( 'NONE',  ( -21.52544592524343514, 5.823673210054127303, 61.04057627198103120 ) ) ;
#41004=CARTESIAN_POINT ( 'NONE',  ( -13.89961937509977652, 13.97604488694528158, 40.62390960531435979 ) ) ;
#41005=CARTESIAN_POINT ( 'NONE',  ( -16.51473224551069308, -9.474510206698971260, 71.66557627198102409 ) ) ;
#41007=CARTESIAN_POINT ( 'NONE',  ( -16.55341960407617563, 4.379528057220093196, 48.54275706135234714 ) ) ;
#41008=CARTESIAN_POINT ( 'NONE',  ( 15.72974639402176855, 15.80617190586768217, 26.87609039468567218 ) ) ;
#41009=CARTESIAN_POINT ( 'NONE',  ( 15.80617190586769283, -15.72974639402175789, 55.62609039468568284 ) ) ;
#41010=CARTESIAN_POINT ( 'NONE',  ( -0.05219959533909027116, -19.03943276465977164, 107.4989096053143527 ) ) ;
#41011=CARTESIAN_POINT ( 'NONE',  ( -21.52544592524343514, 5.823673210054127303, 86.04057627198102409 ) ) ;
#41012=CARTESIAN_POINT ( 'NONE',  ( 21.53943276465977519, 0.05219959533937863772, 21.25109039468567218 ) ) ;
#41013=CARTESIAN_POINT ( 'NONE',  ( 14.34966873604972726, -8.224510206698740333, 55.83442372801901854 ) ) ;
#41015=CARTESIAN_POINT ( 'NONE',  ( -18.67979575497178146, -10.72451020669898902, 46.66557627198102409 ) ) ;
#41016=CARTESIAN_POINT ( 'NONE',  ( -19.02544592524334988, -5.153800228976617603, 23.95942372801900078 ) ) ;
#41017=CARTESIAN_POINT ( 'NONE',  ( -9.474510206698964154, 16.51473224551069663, 55.41557627198103120 ) ) ;
#41018=CARTESIAN_POINT ( 'NONE',  ( 19.03943276465977164, -0.05219959533909143690, 113.7489096053143669 ) ) ;
#41019=CARTESIAN_POINT ( 'NONE',  ( -19.02544592524342804, 5.153800228976336051, 91.04057627198100988 ) ) ;
#41020=CARTESIAN_POINT ( 'NONE',  ( 17.49999999999999645, -5.624438216177558125, 88.31670344914645909 ) ) ;
#41021=CARTESIAN_POINT ( 'NONE',  ( 16.51473224551083163, -9.474510206698727899, 65.83442372801900433 ) ) ;
#41022=CARTESIAN_POINT ( 'NONE',  ( 21.53943276465977519, -0.05219959533907433946, 48.74890960531435979 ) ) ;
#41023=CARTESIAN_POINT ( 'NONE',  ( 16.52544592524335698, 4.483927247898782831, 101.4594237280190185 ) ) ;
#41024=CARTESIAN_POINT ( 'NONE',  ( 5.153800228976615827, -19.02544592524334988, 80.20942372801901854 ) ) ;
#41025=DIRECTION ( 'NONE',  ( 0.000000000000000000, 1.000000000000000000, 0.000000000000000000 ) ) ;
#41026=CARTESIAN_POINT ( 'NONE',  ( 9.474510206698729675, 16.51473224551082808, 22.08442372801899722 ) ) ;
#41027=CARTESIAN_POINT ( 'NONE',  ( -13.89961937509957401, -13.97604488694547875, 79.37609039468567573 ) ) ;
#41028=CARTESIAN_POINT ( 'NONE',  ( -19.02544592524334988, -5.153800228976617603, 43.95942372801899012 ) ) ;
#41029=CARTESIAN_POINT ( 'NONE',  ( 17.60691670004650788, 5.500000000000063949, 71.63333313366440791 ) ) ;
#41030=CARTESIAN_POINT ( 'NONE',  ( -16.46253265017160317, 9.564922557960807481, 50.83224293864770260 ) ) ;
#41031=CARTESIAN_POINT ( 'NONE',  ( -16.52544592524342804, 4.483927247898546575, 51.04057627198103120 ) ) ;
#41032=CARTESIAN_POINT ( 'NONE',  ( -9.474510206698964154, 16.51473224551069663, 35.41557627198102409 ) ) ;
#41033=CARTESIAN_POINT ( 'NONE',  ( -16.53943276465976808, 0.05219959533911058130, 41.24890960531435269 ) ) ;
#41035=CARTESIAN_POINT ( 'NONE',  ( -16.55341960407617563, 4.379528057220093196, 108.5427570613523756 ) ) ;
#41036=CARTESIAN_POINT ( 'NONE',  ( 5.049401038298161559, -19.05341960407611168, 52.70724293864767418 ) ) ;
#41037=CARTESIAN_POINT ( 'NONE',  ( 13.97604488694548053, -13.89961937509957401, 25.62609039468566507 ) ) ;
#41038=CARTESIAN_POINT ( 'NONE',  ( -16.52544592524335698, -4.483927247898792601, 38.95942372801901854 ) ) ;
#41039=CARTESIAN_POINT ( 'NONE',  ( 21.53943276465977519, -0.05219959533907433946, 43.74890960531435979 ) ) ;
#41040=CARTESIAN_POINT ( 'NONE',  ( -18.62759615963255300, -10.81492255796106328, 89.16775706135236135 ) ) ;
#41042=CARTESIAN_POINT ( 'NONE',  ( 16.51473224551069308, 9.474510206698969483, 59.16557627198102409 ) ) ;
#41043=CARTESIAN_POINT ( 'NONE',  ( -5.153800228976328057, -19.02544592524343514, 107.2905762719810383 ) ) ;
#41044=CARTESIAN_POINT ( 'NONE',  ( -0.05219959533909027116, -19.03943276465977164, 97.49890960531436690 ) ) ;
#41046=CARTESIAN_POINT ( 'NONE',  ( -5.719274019375665041, -21.55341960407619695, 24.79275706135235779 ) ) ;
#41048=CARTESIAN_POINT ( 'NONE',  ( -8.314922557960811034, -14.29746914071050412, 82.08224293864768129 ) ) ;
#41049=CARTESIAN_POINT ( 'NONE',  ( -15.80617190586745835, -15.72974639402198527, 76.87390960531439532 ) ) ;
#41050=CARTESIAN_POINT ( 'NONE',  ( 13.89961937509977652, -13.97604488694527269, 68.12390960531436690 ) ) ;
#41051=CARTESIAN_POINT ( 'NONE',  ( -0.05219959533909027116, -19.03943276465977164, 77.49890960531435269 ) ) ;
#41052=CARTESIAN_POINT ( 'NONE',  ( 18.62759615963271287, -10.81492255796078972, 113.3322429386476955 ) ) ;
#41054=CARTESIAN_POINT ( 'NONE',  ( -5.049401038298153566, 19.05341960407611168, 80.20724293864769550 ) ) ;
#41056=CARTESIAN_POINT ( 'NONE',  ( 4.379528057220339221, -16.55341960407611168, 107.7072429386476955 ) ) ;
#41058=CARTESIAN_POINT ( 'NONE',  ( 19.05341960407611168, 5.049401038298154454, 68.95724293864769550 ) ) ;
#41059=CARTESIAN_POINT ( 'NONE',  ( -0.05219959533936034679, 19.03943276465977164, 87.50109039468567573 ) ) ;
#41060=CARTESIAN_POINT ( 'NONE',  ( -0.05219959533910754901, -16.53943276465976808, 97.49890960531436690 ) ) ;
#41061=CARTESIAN_POINT ( 'NONE',  ( -18.62759615963255300, -10.81492255796106328, 54.16775706135235424 ) ) ;
#41062=CARTESIAN_POINT ( 'NONE',  ( -9.474510206698964154, 16.51473224551069663, 55.41557627198103120 ) ) ;
#41063=CARTESIAN_POINT ( 'NONE',  ( 15.80617190586769283, -15.72974639402175789, 25.62609039468567929 ) ) ;
#41064=CARTESIAN_POINT ( 'NONE',  ( 4.483927247898545687, 16.52544592524342804, 99.79057627198103830 ) ) ;
#41066=CARTESIAN_POINT ( 'NONE',  ( -9.564922557960796823, -16.46253265017161027, 72.08224293864770971 ) ) ;
#41068=CARTESIAN_POINT ( 'NONE',  ( -16.53943276465976808, -0.05219959533934237506, 18.75109039468568639 ) ) ;
#41069=CARTESIAN_POINT ( 'NONE',  ( 10.72451020669898902, -18.67979575497178502, 32.91557627198102409 ) ) ;
#41070=CARTESIAN_POINT ( 'NONE',  ( 21.53943276465977519, 0.05219959533937863772, 51.25109039468568994 ) ) ;
#41071=CARTESIAN_POINT ( 'NONE',  ( 5.049401038298161559, -19.05341960407611168, 92.70724293864769550 ) ) ;
#41072=CARTESIAN_POINT ( 'NONE',  ( 9.474510206698729675, 16.51473224551082808, 77.08442372801900433 ) ) ;
#41073=CARTESIAN_POINT ( 'NONE',  ( -5.153800228976328057, -19.02544592524343514, 77.29057627198099567 ) ) ;
#41074=CARTESIAN_POINT ( 'NONE',  ( -16.55341960407611168, -4.379528057220339221, 76.45724293864769550 ) ) ;
#41075=CARTESIAN_POINT ( 'NONE',  ( 16.46253265017160672, -9.564922557960803928, 108.3322429386476955 ) ) ;
#41076=CARTESIAN_POINT ( 'NONE',  ( -0.05219959533910754901, -16.53943276465976808, 77.49890960531433848 ) ) ;
#41077=CARTESIAN_POINT ( 'NONE',  ( 19.05341960407611168, 5.049401038298154454, 98.95724293864766707 ) ) ;
#41078=CARTESIAN_POINT ( 'NONE',  ( -5.049401038298153566, 19.05341960407611168, 50.20724293864770260 ) ) ;
#41079=CARTESIAN_POINT ( 'NONE',  ( 16.55341960407611168, 4.379528057220329451, 48.95724293864770971 ) ) ;
#41081=CARTESIAN_POINT ( 'NONE',  ( 13.89961937509977652, -13.97604488694527269, 33.12390960531434558 ) ) ;
#41083=CARTESIAN_POINT ( 'NONE',  ( -0.05219959533937732626, 21.53943276465977519, 42.50109039468567573 ) ) ;
#41084=CARTESIAN_POINT ( 'NONE',  ( 5.049401038297881783, 19.05341960407617563, 82.29275706135229029 ) ) ;
#41085=CARTESIAN_POINT ( 'NONE',  ( -16.52544592524342804, 4.483927247898546575, 51.04057627198103120 ) ) ;
#41086=CARTESIAN_POINT ( 'NONE',  ( 10.81492255796078972, 18.62759615963270932, 94.58224293864769550 ) ) ;
#41087=CARTESIAN_POINT ( 'NONE',  ( -18.62759615963270932, 10.81492255796079327, 35.83224293864768839 ) ) ;
#41088=CARTESIAN_POINT ( 'NONE',  ( 8.224510206698953496, -14.34966873604960469, 87.91557627198103830 ) ) ;
#41089=CARTESIAN_POINT ( 'NONE',  ( -19.05341960407611168, -5.049401038298163336, 41.45724293864769550 ) ) ;
#41090=CARTESIAN_POINT ( 'NONE',  ( 8.314922557960818139, 14.29746914071049879, 29.58224293864769905 ) ) ;
#41091=CARTESIAN_POINT ( 'NONE',  ( -12.14591786802326823, 12.06949235617739902, 88.12609039468570415 ) ) ;
#41092=CARTESIAN_POINT ( 'NONE',  ( -8.224510206698735004, -14.34966873604973081, 74.58442372801901854 ) ) ;
#41093=CARTESIAN_POINT ( 'NONE',  ( 16.51473224551083163, -9.474510206698727899, 20.83442372801899722 ) ) ;
#41094=CARTESIAN_POINT ( 'NONE',  ( -19.03943276465977164, 0.05219959533909376836, 86.24890960531436690 ) ) ;
#41095=CARTESIAN_POINT ( 'NONE',  ( -13.97604488694527625, -13.89961937509977652, 81.87390960531436690 ) ) ;
#41096=CARTESIAN_POINT ( 'NONE',  ( 16.53943276465976808, 0.05219959533934440121, 91.25109039468568994 ) ) ;
#41097=CARTESIAN_POINT ( 'NONE',  ( 19.02544592524343514, -5.153800228976328945, 43.54057627198103120 ) ) ;
#41098=CARTESIAN_POINT ( 'NONE',  ( 12.06949235617757843, -12.14591786802309237, 53.12390960531436690 ) ) ;
#41099=CARTESIAN_POINT ( 'NONE',  ( 13.97604488694527802, 13.89961937509977652, 99.37390960531436690 ) ) ;
#41100=CARTESIAN_POINT ( 'NONE',  ( -18.62759615963270932, 10.81492255796079327, 30.83224293864770260 ) ) ;
#41101=CARTESIAN_POINT ( 'NONE',  ( -0.05219959533910754901, -16.53943276465976808, 77.49890960531433848 ) ) ;
#41102=ORIENTED_EDGE ( 'NONE', *, *, #162015, .F. ) ;
#41103=CARTESIAN_POINT ( 'NONE',  ( -14.29746914071049879, 8.314922557960819915, 70.83224293864770971 ) ) ;
#41105=CARTESIAN_POINT ( 'NONE',  ( 9.564922557961047289, -16.46253265017146816, 65.41775706135233293 ) ) ;
#41106=CARTESIAN_POINT ( 'NONE',  ( 16.46253265017160672, -9.564922557960803928, 103.3322429386476955 ) ) ;
#41107=CARTESIAN_POINT ( 'NONE',  ( -13.97604488694547697, 13.89961937509957934, 83.12609039468564731 ) ) ;
#41109=CARTESIAN_POINT ( 'NONE',  ( 13.97604488694548053, -13.89961937509957401, 105.6260903946856757 ) ) ;
#41110=CARTESIAN_POINT ( 'NONE',  ( -8.314922557961024197, 14.29746914071037800, 97.91775706135236135 ) ) ;
#41111=CARTESIAN_POINT ( 'NONE',  ( -9.564922557960796823, -16.46253265017161027, 42.08224293864769550 ) ) ;
#41112=CARTESIAN_POINT ( 'NONE',  ( 21.55341960407610458, 5.719274019375980345, 28.95724293864769905 ) ) ;
#41113=CARTESIAN_POINT ( 'NONE',  ( -15.72974639402176322, -15.80617190586768395, 54.37609039468568994 ) ) ;
#41114=CARTESIAN_POINT ( 'NONE',  ( -16.53943276465976808, -0.05219959533934237506, 23.75109039468567929 ) ) ;
#41116=CARTESIAN_POINT ( 'NONE',  ( 13.89961937509977652, -13.97604488694527269, 73.12390960531436690 ) ) ;
#41117=EDGE_CURVE ( 'NONE', #142306, #50018, #159348, .T. ) ;
#41118=CARTESIAN_POINT ( 'NONE',  ( 19.02544592524343514, -5.153800228976328945, 113.5405762719810241 ) ) ;
#41119=CARTESIAN_POINT ( 'NONE',  ( -16.53943276465976808, 0.05219959533911058130, 71.24890960531435269 ) ) ;
#41120=CARTESIAN_POINT ( 'NONE',  ( -16.46253265017160317, 9.564922557960807481, 80.83224293864769550 ) ) ;
#41121=CARTESIAN_POINT ( 'NONE',  ( 9.564922557960805705, 16.46253265017160317, 84.58224293864769550 ) ) ;
#41123=CARTESIAN_POINT ( 'NONE',  ( 16.46253265017146816, 9.564922557961045513, 86.66775706135233293 ) ) ;
#41124=CARTESIAN_POINT ( 'NONE',  ( 18.67979575497178502, 10.72451020669898547, 59.16557627198103120 ) ) ;
#41125=CARTESIAN_POINT ( 'NONE',  ( 16.46253265017160672, -9.564922557960803928, 33.33224293864770260 ) ) ;
#41126=CARTESIAN_POINT ( 'NONE',  ( -13.89961937509957401, -13.97604488694547875, 54.37609039468565442 ) ) ;
#41127=CARTESIAN_POINT ( 'NONE',  ( -9.564922557960796823, -16.46253265017161027, 62.08224293864769550 ) ) ;
#41128=CARTESIAN_POINT ( 'NONE',  ( -19.05341960407611168, -5.049401038298163336, 91.45724293864766707 ) ) ;
#41129=ORIENTED_EDGE ( 'NONE', *, *, #93805, .F. ) ;
#41130=CARTESIAN_POINT ( 'NONE',  ( -10.72451020669898014, 18.67979575497178502, 90.41557627198103830 ) ) ;
#41131=CARTESIAN_POINT ( 'NONE',  ( 16.52544592524342804, -4.483927247898539470, 93.54057627198103830 ) ) ;
#41132=CARTESIAN_POINT ( 'NONE',  ( 5.049401038297881783, 19.05341960407617563, 47.29275706135231161 ) ) ;
#41133=CARTESIAN_POINT ( 'NONE',  ( -15.72974639402197994, 15.80617190586746368, 90.62390960531436690 ) ) ;
#41134=CARTESIAN_POINT ( 'NONE',  ( -0.05219959533907301413, -21.53943276465977519, 77.49890960531433848 ) ) ;
#41135=CARTESIAN_POINT ( 'NONE',  ( 8.224510206698953496, -14.34966873604960469, 32.91557627198102409 ) ) ;
#41136=CARTESIAN_POINT ( 'NONE',  ( -5.823673210054431948, 21.52544592524334988, 107.7094237280190328 ) ) ;
#41137=CARTESIAN_POINT ( 'NONE',  ( -0.05219959533934338120, 16.53943276465976808, 47.50109039468568994 ) ) ;
#41138=CARTESIAN_POINT ( 'NONE',  ( 16.51473224551069308, 9.474510206698969483, 84.16557627198102409 ) ) ;
#41139=CARTESIAN_POINT ( 'NONE',  ( 9.474510206698971260, -16.51473224551069308, 32.91557627198102409 ) ) ;
#41141=CARTESIAN_POINT ( 'NONE',  ( 0.05219959533937995610, -21.53943276465977519, 40.00109039468567573 ) ) ;
#41142=CARTESIAN_POINT ( 'NONE',  ( -5.823673210054431948, 21.52544592524334988, 52.70942372801902565 ) ) ;
#41143=CARTESIAN_POINT ( 'NONE',  ( 19.05341960407611168, 5.049401038298154454, 53.95724293864770260 ) ) ;
#41144=CARTESIAN_POINT ( 'NONE',  ( 10.81492255796078972, 18.62759615963270932, 114.5822429386477097 ) ) ;
#41145=CARTESIAN_POINT ( 'NONE',  ( -9.564922557961040184, 16.46253265017147172, 62.91775706135233293 ) ) ;
#41146=EDGE_CURVE ( 'NONE', #68158, #133003, #194626, .T. ) ;
#41147=CARTESIAN_POINT ( 'NONE',  ( -13.89961937509977652, 13.97604488694528158, 35.62390960531435269 ) ) ;
#41148=CARTESIAN_POINT ( 'NONE',  ( 12.14591786802327356, -12.06949235617739191, 25.62609039468567929 ) ) ;
#41149=CARTESIAN_POINT ( 'NONE',  ( -19.03943276465977164, 0.05219959533909376836, 31.24890960531435979 ) ) ;
#41150=CARTESIAN_POINT ( 'NONE',  ( -0.05219959533934338120, 16.53943276465976808, 72.50109039468568994 ) ) ;
#41151=CARTESIAN_POINT ( 'NONE',  ( -5.153800228976328057, -19.02544592524343514, 37.29057627198102409 ) ) ;
#41153=CARTESIAN_POINT ( 'NONE',  ( 0.05219959533909260263, 19.03943276465977164, 89.99890960531436690 ) ) ;
#41154=CARTESIAN_POINT ( 'NONE',  ( -16.51473224551069308, -9.474510206698971260, 26.66557627198103120 ) ) ;
#41155=CARTESIAN_POINT ( 'NONE',  ( -10.81492255796078084, -18.62759615963271287, 72.08224293864769550 ) ) ;
#41156=CARTESIAN_POINT ( 'NONE',  ( 8.224510206698742110, 14.34966873604972548, 57.08442372801901854 ) ) ;
#41157=CARTESIAN_POINT ( 'NONE',  ( -0.05219959533937732626, 21.53943276465977519, 107.5010903946856899 ) ) ;
#41158=CARTESIAN_POINT ( 'NONE',  ( -19.02544592524342804, 5.153800228976336051, 36.04057627198100988 ) ) ;
#41159=CARTESIAN_POINT ( 'NONE',  ( 16.52544592524342804, -4.483927247898539470, 33.54057627198102409 ) ) ;
#41160=CARTESIAN_POINT ( 'NONE',  ( -12.14591786802309592, -12.06949235617757132, 61.87390960531436690 ) ) ;
#41161=CARTESIAN_POINT ( 'NONE',  ( -16.51473224551069308, -9.474510206698971260, 66.66557627198102409 ) ) ;
#41162=CARTESIAN_POINT ( 'NONE',  ( -15.72974639402176322, -15.80617190586768395, 104.3760903946856899 ) ) ;
#41163=CARTESIAN_POINT ( 'NONE',  ( 21.55341960407619695, -5.719274019375665929, 36.04275706135234714 ) ) ;
#41164=CARTESIAN_POINT ( 'NONE',  ( 19.02544592524343514, -5.153800228976328945, 73.54057627198103830 ) ) ;
#41165=CARTESIAN_POINT ( 'NONE',  ( 15.72974639402176855, 15.80617190586768217, 91.87609039468568994 ) ) ;
#41166=CARTESIAN_POINT ( 'NONE',  ( 4.379528057220092307, 16.55341960407617563, 62.29275706135236845 ) ) ;
#41167=CARTESIAN_POINT ( 'NONE',  ( 16.46253265017160672, -9.564922557960803928, 108.3322429386476955 ) ) ;
#41168=CARTESIAN_POINT ( 'NONE',  ( 16.53943276465976808, -0.05219959533910856209, 38.74890960531435979 ) ) ;
#41169=CARTESIAN_POINT ( 'NONE',  ( -5.153800228976328057, -19.02544592524343514, 22.29057627198102765 ) ) ;
#41170=CARTESIAN_POINT ( 'NONE',  ( 0.05219959533934541429, -16.53943276465976808, 55.00109039468568284 ) ) ;
#41171=CARTESIAN_POINT ( 'NONE',  ( -0.05219959533910754901, -16.53943276465976808, 57.49890960531435979 ) ) ;
#41172=CARTESIAN_POINT ( 'NONE',  ( 19.05341960407611168, 5.049401038298154454, 108.9572429386477097 ) ) ;
#41173=CARTESIAN_POINT ( 'NONE',  ( 10.81492255796078972, 18.62759615963270932, 29.58224293864769905 ) ) ;
#41174=CARTESIAN_POINT ( 'NONE',  ( -5.153800228976607833, 19.02544592524334988, 22.70942372801899012 ) ) ;
#41175=CARTESIAN_POINT ( 'NONE',  ( 14.29746914071049879, -8.314922557960816363, 88.33224293864769550 ) ) ;
#41176=CARTESIAN_POINT ( 'NONE',  ( 19.02544592524343514, -5.153800228976328945, 93.54057627198102409 ) ) ;
#41178=CARTESIAN_POINT ( 'NONE',  ( -16.53943276465976808, -0.05219959533934237506, 53.75109039468568994 ) ) ;
#41179=CARTESIAN_POINT ( 'NONE',  ( 0.05219959533909260263, 19.03943276465977164, 49.99890960531435979 ) ) ;
#41180=CARTESIAN_POINT ( 'NONE',  ( 17.60689202196056158, 5.500000000000022204, 101.6333492360910782 ) ) ;
#41181=CARTESIAN_POINT ( 'NONE',  ( 9.474510206698729675, 16.51473224551082808, 42.08442372801900433 ) ) ;
#41182=CARTESIAN_POINT ( 'NONE',  ( -9.474510206698964154, 16.51473224551069663, 45.41557627198103120 ) ) ;
#41183=CARTESIAN_POINT ( 'NONE',  ( 14.29746914071037800, 8.314922557961029526, 81.66775706135236135 ) ) ;
#41184=CARTESIAN_POINT ( 'NONE',  ( -13.89961937509957401, -13.97604488694547875, 94.37609039468566152 ) ) ;
#41185=CARTESIAN_POINT ( 'NONE',  ( -21.55341960407619339, 5.719274019375674811, 68.54275706135234714 ) ) ;
#41186=CARTESIAN_POINT ( 'NONE',  ( -19.05341960407611168, -5.049401038298163336, 66.45724293864769550 ) ) ;
#41187=CARTESIAN_POINT ( 'NONE',  ( -0.05219959533907301413, -21.53943276465977519, 97.49890960531436690 ) ) ;
#41188=CARTESIAN_POINT ( 'NONE',  ( 0.05219959533910956823, 16.53943276465976808, 99.99890960531436690 ) ) ;
#41190=CARTESIAN_POINT ( 'NONE',  ( 9.474510206698729675, 16.51473224551082808, 72.08442372801900433 ) ) ;
#41191=CARTESIAN_POINT ( 'NONE',  ( 0.05219959533907565091, 21.53943276465977519, 69.99890960531435269 ) ) ;
#41192=CARTESIAN_POINT ( 'NONE',  ( -9.564922557961040184, 16.46253265017147172, 47.91775706135233293 ) ) ;
#41193=CARTESIAN_POINT ( 'NONE',  ( 13.89961937509977652, -13.97604488694527269, 113.1239096053143527 ) ) ;
#41194=CARTESIAN_POINT ( 'NONE',  ( -5.719274019375978568, 21.55341960407610458, 95.20724293864769550 ) ) ;
#41196=CARTESIAN_POINT ( 'NONE',  ( 14.34966873604972726, -8.224510206698740333, 25.83442372801901499 ) ) ;
#41198=CARTESIAN_POINT ( 'NONE',  ( -0.05219959533934338120, 16.53943276465976808, 27.50109039468567929 ) ) ;
#41199=CARTESIAN_POINT ( 'NONE',  ( 16.51473224551069308, 9.474510206698969483, 49.16557627198102409 ) ) ;
#41200=CARTESIAN_POINT ( 'NONE',  ( -5.049401038298153566, 19.05341960407611168, 105.2072429386476671 ) ) ;
#41201=CARTESIAN_POINT ( 'NONE',  ( 21.53943276465977519, -0.05219959533907433946, 93.74890960531436690 ) ) ;
#41202=CARTESIAN_POINT ( 'NONE',  ( -12.14591786802309592, -12.06949235617757132, 51.87390960531437401 ) ) ;
#41203=CARTESIAN_POINT ( 'NONE',  ( -5.823673210054431948, 21.52544592524334988, 72.70942372801901854 ) ) ;
#41204=CARTESIAN_POINT ( 'NONE',  ( -8.224510206698735004, -14.34966873604973081, 29.58442372801901854 ) ) ;
#41205=CARTESIAN_POINT ( 'NONE',  ( -0.05219959533936034679, 19.03943276465977164, 22.50109039468566152 ) ) ;
#41206=CARTESIAN_POINT ( 'NONE',  ( 4.379528057220339221, -16.55341960407611168, 32.70724293864770260 ) ) ;
#41207=CARTESIAN_POINT ( 'NONE',  ( -21.53943276465977519, -0.05219959533937600094, 18.75109039468568639 ) ) ;
#41208=CARTESIAN_POINT ( 'NONE',  ( -12.06949235617756955, 12.14591786802309770, 45.62390960531436690 ) ) ;
#41209=CARTESIAN_POINT ( 'NONE',  ( 5.049401038297881783, 19.05341960407617563, 97.29275706135233293 ) ) ;
#41210=CARTESIAN_POINT ( 'NONE',  ( 16.51473224551083163, -9.474510206698727899, 60.83442372801900433 ) ) ;
#41211=CARTESIAN_POINT ( 'NONE',  ( 10.81492255796106328, -18.62759615963255655, 70.41775706135236135 ) ) ;
#41212=CARTESIAN_POINT ( 'NONE',  ( -19.05341960407617563, 5.049401038297882671, 48.54275706135233293 ) ) ;
#41213=CARTESIAN_POINT ( 'NONE',  ( 9.474510206698971260, -16.51473224551069308, 27.91557627198103120 ) ) ;
#41214=CARTESIAN_POINT ( 'NONE',  ( 18.62759615963271287, -10.81492255796078972, 38.33224293864768839 ) ) ;
#41215=CARTESIAN_POINT ( 'NONE',  ( -14.34966873604960291, -8.224510206698953496, 51.66557627198102409 ) ) ;
#41216=CARTESIAN_POINT ( 'NONE',  ( -16.88567814943161238, -6.947325034625785101, 26.29001122652587696 ) ) ;
#41217=CARTESIAN_POINT ( 'NONE',  ( 13.89961937509957401, 13.97604488694547697, 21.87609039468566152 ) ) ;
#41218=CARTESIAN_POINT ( 'NONE',  ( 8.314922557961029526, -14.29746914071037800, 65.41775706135234714 ) ) ;
#41219=CARTESIAN_POINT ( 'NONE',  ( -4.379528057220328563, 16.55341960407611168, 35.20724293864768839 ) ) ;
#41220=CARTESIAN_POINT ( 'NONE',  ( -15.72974639402176322, -15.80617190586768395, 74.37609039468568994 ) ) ;
#41221=CARTESIAN_POINT ( 'NONE',  ( 5.719274019375673035, 21.55341960407619339, 67.29275706135234714 ) ) ;
#41222=CARTESIAN_POINT ( 'NONE',  ( 5.823673210054125526, 21.52544592524343514, 84.79057627198102409 ) ) ;
#41223=CARTESIAN_POINT ( 'NONE',  ( -19.05341960407611168, -5.049401038298163336, 41.45724293864769550 ) ) ;
#41224=CARTESIAN_POINT ( 'NONE',  ( -18.67979575497193778, 10.72451020669871902, 38.33442372801900433 ) ) ;
#41225=CARTESIAN_POINT ( 'NONE',  ( -4.379528057220328563, 16.55341960407611168, 115.2072429386476955 ) ) ;
#41226=CARTESIAN_POINT ( 'NONE',  ( -13.89961937509977652, 13.97604488694528158, 55.62390960531434558 ) ) ;
#41227=CARTESIAN_POINT ( 'NONE',  ( -16.52544592524342804, 4.483927247898546575, 91.04057627198103830 ) ) ;
#41228=CARTESIAN_POINT ( 'NONE',  ( 13.89961937509977652, -13.97604488694527269, 83.12390960531436690 ) ) ;
#41229=CARTESIAN_POINT ( 'NONE',  ( 4.379528057220339221, -16.55341960407611168, 42.70724293864770260 ) ) ;
#41230=CARTESIAN_POINT ( 'NONE',  ( 4.379528057220339221, -16.55341960407611168, 97.70724293864772392 ) ) ;
#41231=CARTESIAN_POINT ( 'NONE',  ( -18.62759615963270932, 10.81492255796079327, 65.83224293864769550 ) ) ;
#41232=CARTESIAN_POINT ( 'NONE',  ( 15.80617190586746368, 15.72974639402197994, 114.3739096053143527 ) ) ;
#41233=CARTESIAN_POINT ( 'NONE',  ( -19.02544592524342804, 5.153800228976336051, 111.0405762719810099 ) ) ;
#41234=CARTESIAN_POINT ( 'NONE',  ( -19.02544592524342804, 5.153800228976336051, 61.04057627198103120 ) ) ;
#41235=CARTESIAN_POINT ( 'NONE',  ( 4.379528057220092307, 16.55341960407617563, 22.29275706135235069 ) ) ;
#41236=CARTESIAN_POINT ( 'NONE',  ( -21.55341960407610458, -5.719274019375992779, 76.45724293864769550 ) ) ;
#41237=CARTESIAN_POINT ( 'NONE',  ( 0.05219959533937995610, -21.53943276465977519, 90.00109039468567573 ) ) ;
#41238=CARTESIAN_POINT ( 'NONE',  ( -0.05219959533909027116, -19.03943276465977164, 82.49890960531436690 ) ) ;
#41239=CARTESIAN_POINT ( 'NONE',  ( -5.823673210054431948, 21.52544592524334988, 22.70942372801901499 ) ) ;
#41240=CARTESIAN_POINT ( 'NONE',  ( 18.62759615963271287, -10.81492255796078972, 23.33224293864769194 ) ) ;
#41241=CARTESIAN_POINT ( 'NONE',  ( -4.483927247898782831, 16.52544592524335698, 87.70942372801901854 ) ) ;
#41242=CARTESIAN_POINT ( 'NONE',  ( 21.53943276465977519, 0.05219959533937863772, 71.25109039468568994 ) ) ;
#41243=CARTESIAN_POINT ( 'NONE',  ( -18.67979575497193778, 10.72451020669871902, 98.33442372801901854 ) ) ;
#41244=CARTESIAN_POINT ( 'NONE',  ( -0.05219959533934338120, 16.53943276465976808, 57.50109039468568994 ) ) ;
#41245=CARTESIAN_POINT ( 'NONE',  ( -18.67979575497193778, 10.72451020669871902, 33.33442372801900433 ) ) ;
#41246=CARTESIAN_POINT ( 'NONE',  ( 19.05341960407611168, 5.049401038298154454, 23.95724293864769194 ) ) ;
#41247=CARTESIAN_POINT ( 'NONE',  ( 15.80617190586769283, -15.72974639402175789, 90.62609039468567573 ) ) ;
#41248=CARTESIAN_POINT ( 'NONE',  ( 13.97604488694527802, 13.89961937509977652, 94.37390960531436690 ) ) ;
#41249=CARTESIAN_POINT ( 'NONE',  ( -21.55341960407610458, -5.719274019375992779, 96.45724293864770971 ) ) ;
#41250=CARTESIAN_POINT ( 'NONE',  ( 19.03943276465977164, 0.05219959533936151252, 56.25109039468566863 ) ) ;
#41251=CARTESIAN_POINT ( 'NONE',  ( -18.67979575497178146, -10.72451020669898902, 51.66557627198102409 ) ) ;
#41252=CARTESIAN_POINT ( 'NONE',  ( -19.03943276465977164, 0.05219959533909376836, 101.2489096053143669 ) ) ;
#41253=CARTESIAN_POINT ( 'NONE',  ( -14.29746914071049879, 8.314922557960819915, 40.83224293864769550 ) ) ;
#41255=CARTESIAN_POINT ( 'NONE',  ( 19.03943276465977164, 0.05219959533936151252, 71.25109039468566152 ) ) ;
#41256=CARTESIAN_POINT ( 'NONE',  ( -18.89770734986048595, -5.500000000000010658, 79.10214472496643623 ) ) ;
#41257=CARTESIAN_POINT ( 'NONE',  ( -19.05341960407617563, 5.049401038297882671, 108.5427570613523187 ) ) ;
#41258=CARTESIAN_POINT ( 'NONE',  ( -18.67979575497178146, -10.72451020669898902, 81.66557627198103830 ) ) ;
#41259=CARTESIAN_POINT ( 'NONE',  ( 4.379528057220339221, -16.55341960407611168, 67.70724293864769550 ) ) ;
#41260=CARTESIAN_POINT ( 'NONE',  ( 14.34966873604972726, -8.224510206698740333, 30.83442372801902209 ) ) ;
#41261=CARTESIAN_POINT ( 'NONE',  ( 0.05219959533909260263, 19.03943276465977164, 44.99890960531435979 ) ) ;
#41262=CARTESIAN_POINT ( 'NONE',  ( 15.72974639402199770, -15.80617190586745480, 113.1239096053143953 ) ) ;
#41263=CARTESIAN_POINT ( 'NONE',  ( -13.97604488694547697, 13.89961937509957934, 78.12609039468567573 ) ) ;
#41264=CARTESIAN_POINT ( 'NONE',  ( 0.05219959533909260263, 19.03943276465977164, 89.99890960531436690 ) ) ;
#41265=CARTESIAN_POINT ( 'NONE',  ( 13.89961937509977652, -13.97604488694527269, 68.12390960531436690 ) ) ;
#41266=CARTESIAN_POINT ( 'NONE',  ( -10.81492255796078084, -18.62759615963271287, 82.08224293864768129 ) ) ;
#41267=CARTESIAN_POINT ( 'NONE',  ( -19.03943276465977164, 0.05219959533909376836, 41.24890960531435269 ) ) ;
#41269=CARTESIAN_POINT ( 'NONE',  ( 16.53943276465976808, -0.05219959533910856209, 48.74890960531435979 ) ) ;
#41270=CARTESIAN_POINT ( 'NONE',  ( -5.153800228976328057, -19.02544592524343514, 87.29057627198103830 ) ) ;
#41272=CARTESIAN_POINT ( 'NONE',  ( 13.89961937509957401, 13.97604488694547697, 71.87609039468567573 ) ) ;
#41273=CARTESIAN_POINT ( 'NONE',  ( 21.53943276465977519, -0.05219959533907433946, 78.74890960531436690 ) ) ;
#41274=CARTESIAN_POINT ( 'NONE',  ( 13.89961937509957401, 13.97604488694547697, 36.87609039468565442 ) ) ;
#41275=CARTESIAN_POINT ( 'NONE',  ( -16.46253265017160317, 9.564922557960807481, 105.8322429386476955 ) ) ;
#41276=CARTESIAN_POINT ( 'NONE',  ( -17.50000000000014211, 3.292511757969745378, 115.0652027021053669 ) ) ;
#41277=CARTESIAN_POINT ( 'NONE',  ( -0.05219959533907301413, -21.53943276465977519, 37.49890960531436690 ) ) ;
#41279=CARTESIAN_POINT ( 'NONE',  ( -16.51473224551069308, -9.474510206698971260, 66.66557627198102409 ) ) ;
#41280=CARTESIAN_POINT ( 'NONE',  ( 15.80617190586769283, -15.72974639402175789, 70.62609039468567573 ) ) ;
#41281=CARTESIAN_POINT ( 'NONE',  ( -16.46253265017160317, 9.564922557960807481, 30.83224293864769550 ) ) ;
#41282=CARTESIAN_POINT ( 'NONE',  ( -21.55341960407619339, 5.719274019375674811, 23.54275706135235424 ) ) ;
#41283=EDGE_LOOP ( 'NONE', ( #53747, #179327, #163086, #55728 ) ) ;
#41284=CARTESIAN_POINT ( 'NONE',  ( -21.53943276465977519, -0.05219959533937600094, 48.75109039468568284 ) ) ;
#41285=ORIENTED_EDGE ( 'NONE', *, *, #8998, .F. ) ;
#41287=CARTESIAN_POINT ( 'NONE',  ( -5.153800228976607833, 19.02544592524334988, 72.70942372801900433 ) ) ;
#41290=CARTESIAN_POINT ( 'NONE',  ( -18.67979575497178146, -10.72451020669898902, 106.6655762719810383 ) ) ;
#41291=CARTESIAN_POINT ( 'NONE',  ( -9.474510206698964154, 16.51473224551069663, 65.41557627198102409 ) ) ;
#41292=CARTESIAN_POINT ( 'NONE',  ( -4.483927247898782831, 16.52544592524335698, 32.70942372801900433 ) ) ;
#41294=CARTESIAN_POINT ( 'NONE',  ( -18.62759615963255300, -10.81492255796106328, 104.1677570613523471 ) ) ;
#41295=CARTESIAN_POINT ( 'NONE',  ( -16.51473224551069308, -9.474510206698971260, 36.66557627198102409 ) ) ;
#41296=CARTESIAN_POINT ( 'NONE',  ( 18.62759615963255655, 10.81492255796105972, 111.6677570613523613 ) ) ;
#41297=CARTESIAN_POINT ( 'NONE',  ( 13.97604488694527802, 13.89961937509977652, 89.37390960531436690 ) ) ;
#41298=CARTESIAN_POINT ( 'NONE',  ( 15.80617190586769283, -15.72974639402175789, 65.62609039468568994 ) ) ;
#41302=CARTESIAN_POINT ( 'NONE',  ( -16.52544592524335698, -4.483927247898792601, 53.95942372801900433 ) ) ;
#41303=CARTESIAN_POINT ( 'NONE',  ( 18.67979575497194134, -10.72451020669871369, 75.83442372801900433 ) ) ;
#41304=CARTESIAN_POINT ( 'NONE',  ( 0.05219959533937995610, -21.53943276465977519, 90.00109039468567573 ) ) ;
#41306=CARTESIAN_POINT ( 'NONE',  ( -16.52544592524335698, -4.483927247898792601, 33.95942372801901143 ) ) ;
#41307=CARTESIAN_POINT ( 'NONE',  ( -19.02544592524342804, 5.153800228976336051, 86.04057627198103830 ) ) ;
#41308=CARTESIAN_POINT ( 'NONE',  ( -19.05341960407611168, -5.049401038298163336, 111.4572429386476671 ) ) ;
#41309=ORIENTED_EDGE ( 'NONE', *, *, #191998, .T. ) ;
#41311=CARTESIAN_POINT ( 'NONE',  ( 17.26058549869088665, 6.457015423128626530, 43.87745837476069255 ) ) ;
#41312=CARTESIAN_POINT ( 'NONE',  ( 16.51473224551069308, 9.474510206698969483, 29.16557627198103475 ) ) ;
#41313=CARTESIAN_POINT ( 'NONE',  ( -0.05219959533907301413, -21.53943276465977519, 47.49890960531435979 ) ) ;
#41314=CARTESIAN_POINT ( 'NONE',  ( -12.14591786802326823, 12.06949235617739902, 108.1260903946856757 ) ) ;
#41315=CARTESIAN_POINT ( 'NONE',  ( 4.483927247898545687, 16.52544592524342804, 89.79057627198103830 ) ) ;
#41316=CARTESIAN_POINT ( 'NONE',  ( 19.05341960407611168, 5.049401038298154454, 63.95724293864769550 ) ) ;
#41317=CARTESIAN_POINT ( 'NONE',  ( 21.52544592524334988, 5.823673210054432836, 91.45942372801901854 ) ) ;
#41318=CARTESIAN_POINT ( 'NONE',  ( -16.55341960407617563, 4.379528057220093196, 23.54275706135235424 ) ) ;
#41319=CARTESIAN_POINT ( 'NONE',  ( -16.53943276465976808, 0.05219959533911058130, 91.24890960531436690 ) ) ;
#41320=CARTESIAN_POINT ( 'NONE',  ( -18.67979575497193778, 10.72451020669871902, 48.33442372801902565 ) ) ;
#41321=CARTESIAN_POINT ( 'NONE',  ( -15.80617190586745835, -15.72974639402198527, 76.87390960531439532 ) ) ;
#41322=CARTESIAN_POINT ( 'NONE',  ( -19.05341960407617563, 5.049401038297882671, 43.54275706135232582 ) ) ;
#41324=CARTESIAN_POINT ( 'NONE',  ( -13.89961937509977652, 13.97604488694528158, 95.62390960531436690 ) ) ;
#41325=CARTESIAN_POINT ( 'NONE',  ( -4.483927247898539470, -16.52544592524342804, 62.29057627198102409 ) ) ;
#41326=CARTESIAN_POINT ( 'NONE',  ( -4.483927247898539470, -16.52544592524342804, 37.29057627198102409 ) ) ;
#41327=CARTESIAN_POINT ( 'NONE',  ( -8.314922557961024197, 14.29746914071037800, 112.9177570613523329 ) ) ;
#41328=CARTESIAN_POINT ( 'NONE',  ( -5.153800228976607833, 19.02544592524334988, 62.70942372801899722 ) ) ;
#41330=CARTESIAN_POINT ( 'NONE',  ( 13.89961937509977652, -13.97604488694527269, 113.1239096053143527 ) ) ;
#41331=CARTESIAN_POINT ( 'NONE',  ( 16.52544592524342804, -4.483927247898539470, 93.54057627198103830 ) ) ;
#41333=CARTESIAN_POINT ( 'NONE',  ( -19.05341960407611168, -5.049401038298163336, 51.45724293864770260 ) ) ;
#41334=CARTESIAN_POINT ( 'NONE',  ( -0.05219959533907301413, -21.53943276465977519, 47.49890960531435979 ) ) ;
#41335=CARTESIAN_POINT ( 'NONE',  ( -18.67979575497178146, -10.72451020669898902, 81.66557627198103830 ) ) ;
#41336=CARTESIAN_POINT ( 'NONE',  ( 9.474510206698971260, -16.51473224551069308, 22.91557627198102765 ) ) ;
#41337=CARTESIAN_POINT ( 'NONE',  ( 12.06949235617739724, 12.14591786802326823, 66.87609039468568994 ) ) ;
#41338=CARTESIAN_POINT ( 'NONE',  ( -9.564922557960796823, -16.46253265017161027, 42.08224293864769550 ) ) ;
#41339=CARTESIAN_POINT ( 'NONE',  ( 10.81492255796106328, -18.62759615963255655, 55.41775706135234714 ) ) ;
#41340=CARTESIAN_POINT ( 'NONE',  ( -0.05219959533910754901, -16.53943276465976808, 102.4989096053143811 ) ) ;
#41341=CARTESIAN_POINT ( 'NONE',  ( 0.05219959533936267826, -19.03943276465977164, 85.00109039468567573 ) ) ;
#41343=CARTESIAN_POINT ( 'NONE',  ( 17.49999999999999645, 4.119547552400690371, 37.01912384492517560 ) ) ;
#41344=CARTESIAN_POINT ( 'NONE',  ( 21.55341960407610458, 5.719274019375980345, 43.95724293864769550 ) ) ;
#41345=CARTESIAN_POINT ( 'NONE',  ( 17.31728774477273447, -6.344390552232384017, 68.31906651689318721 ) ) ;
#41346=CARTESIAN_POINT ( 'NONE',  ( 10.72451020669871369, 18.67979575497193778, 82.08442372801901854 ) ) ;
#41347=CARTESIAN_POINT ( 'NONE',  ( -8.314922557960811034, -14.29746914071050412, 32.08224293864769550 ) ) ;
#41348=CARTESIAN_POINT ( 'NONE',  ( 16.52544592524335698, 4.483927247898782831, 51.45942372801901854 ) ) ;
#41349=CARTESIAN_POINT ( 'NONE',  ( -4.379528057220328563, 16.55341960407611168, 40.20724293864769550 ) ) ;
#41350=CARTESIAN_POINT ( 'NONE',  ( 5.823673210054125526, 21.52544592524343514, 64.79057627198103830 ) ) ;
#41351=CARTESIAN_POINT ( 'NONE',  ( 10.81492255796078972, 18.62759615963270932, 69.58224293864769550 ) ) ;
#41353=CARTESIAN_POINT ( 'NONE',  ( 0.05219959533936267826, -19.03943276465977164, 80.00109039468567573 ) ) ;
#41354=CARTESIAN_POINT ( 'NONE',  ( 16.46253265017160672, -9.564922557960803928, 108.3322429386476955 ) ) ;
#41355=CARTESIAN_POINT ( 'NONE',  ( -0.05219959533909027116, -19.03943276465977164, 42.49890960531435269 ) ) ;
#41356=CARTESIAN_POINT ( 'NONE',  ( -4.483927247898539470, -16.52544592524342804, 112.2905762719810241 ) ) ;
#41358=ORIENTED_EDGE ( 'NONE', *, *, #102901, .T. ) ;
#41359=CARTESIAN_POINT ( 'NONE',  ( -0.05219959533934338120, 16.53943276465976808, 87.50109039468568994 ) ) ;
#41360=CARTESIAN_POINT ( 'NONE',  ( 5.719274019375991003, -21.55341960407610458, 102.7072429386476955 ) ) ;
#41361=CARTESIAN_POINT ( 'NONE',  ( -13.89961937509977652, 13.97604488694528158, 70.62390960531432427 ) ) ;
#41362=CARTESIAN_POINT ( 'NONE',  ( 15.80617190586769283, -15.72974639402175789, 35.62609039468568994 ) ) ;
#41363=CARTESIAN_POINT ( 'NONE',  ( -5.049401038298153566, 19.05341960407611168, 95.20724293864770971 ) ) ;
#41365=ORIENTED_EDGE ( 'NONE', *, *, #67877, .F. ) ;
#41366=CARTESIAN_POINT ( 'NONE',  ( 15.72974639402176855, 15.80617190586768217, 31.87609039468567929 ) ) ;
#41367=CARTESIAN_POINT ( 'NONE',  ( -16.46253265017160317, 9.564922557960807481, 30.83224293864769550 ) ) ;
#41368=CARTESIAN_POINT ( 'NONE',  ( -19.05341960407617563, 5.049401038297882671, 88.54275706135230450 ) ) ;
#41369=CARTESIAN_POINT ( 'NONE',  ( 9.474510206698729675, 16.51473224551082808, 42.08442372801900433 ) ) ;
#41370=CARTESIAN_POINT ( 'NONE',  ( 10.72451020669898902, -18.67979575497178502, 112.9155762719810383 ) ) ;
#41371=CARTESIAN_POINT ( 'NONE',  ( 16.51473224551083163, -9.474510206698727899, 45.83442372801900433 ) ) ;
#41372=CARTESIAN_POINT ( 'NONE',  ( 19.02544592524334988, 5.153800228976608722, 51.45942372801900433 ) ) ;
#41373=CARTESIAN_POINT ( 'NONE',  ( -4.379528057220086978, -16.55341960407618274, 94.79275706135234714 ) ) ;
#41376=CARTESIAN_POINT ( 'NONE',  ( -16.51473224551069308, -9.474510206698971260, 71.66557627198102409 ) ) ;
#41377=CARTESIAN_POINT ( 'NONE',  ( -18.62759615963255300, -10.81492255796106328, 84.16775706135234714 ) ) ;
#41378=CARTESIAN_POINT ( 'NONE',  ( -5.719274019375665041, -21.55341960407619695, 99.79275706135234714 ) ) ;
#41380=CARTESIAN_POINT ( 'NONE',  ( 16.51473224551069308, 9.474510206698969483, 89.16557627198103830 ) ) ;
#41381=CARTESIAN_POINT ( 'NONE',  ( -18.62759615963255300, -10.81492255796106328, 59.16775706135234714 ) ) ;
#41382=CARTESIAN_POINT ( 'NONE',  ( 9.474510206698729675, 16.51473224551082808, 97.08442372801900433 ) ) ;
#41384=CARTESIAN_POINT ( 'NONE',  ( -19.03943276465977164, 0.05219959533909376836, 71.24890960531435269 ) ) ;
#41385=CARTESIAN_POINT ( 'NONE',  ( 9.564922557960805705, 16.46253265017160317, 114.5822429386476955 ) ) ;
#41386=CARTESIAN_POINT ( 'NONE',  ( -19.03943276465977164, 0.05219959533909376836, 81.24890960531436690 ) ) ;
#41387=CARTESIAN_POINT ( 'NONE',  ( -17.31728774477274513, -6.344390552232373359, 89.18093348310689805 ) ) ;
#41388=CARTESIAN_POINT ( 'NONE',  ( 16.51473224551069308, 9.474510206698969483, 69.16557627198102409 ) ) ;
#41389=CARTESIAN_POINT ( 'NONE',  ( 5.153800228976335163, 19.02544592524342804, 49.79057627198100988 ) ) ;
#41390=CARTESIAN_POINT ( 'NONE',  ( 5.823673210054444382, -21.52544592524334988, 20.20942372801900788 ) ) ;
#41391=CARTESIAN_POINT ( 'NONE',  ( 4.379528057220092307, 16.55341960407617563, 97.29275706135234714 ) ) ;
#41394=CARTESIAN_POINT ( 'NONE',  ( -16.46253265017146816, -9.564922557961047289, 59.16775706135233293 ) ) ;
#41395=CARTESIAN_POINT ( 'NONE',  ( -16.46253265017160317, 9.564922557960807481, 85.83224293864769550 ) ) ;
#41396=CARTESIAN_POINT ( 'NONE',  ( -16.55341960407611168, -4.379528057220339221, 76.45724293864769550 ) ) ;
#41397=CARTESIAN_POINT ( 'NONE',  ( -0.05219959533910754901, -16.53943276465976808, 112.4989096053143669 ) ) ;
#41398=CARTESIAN_POINT ( 'NONE',  ( -21.53943276465977519, 0.05219959533907696930, 26.24890960531435624 ) ) ;
#41399=CARTESIAN_POINT ( 'NONE',  ( -19.05341960407611168, -5.049401038298163336, 106.4572429386476955 ) ) ;
#41400=CARTESIAN_POINT ( 'NONE',  ( 16.53943276465976808, -0.05219959533910856209, 88.74890960531436690 ) ) ;
#41401=CARTESIAN_POINT ( 'NONE',  ( 9.474510206698971260, -16.51473224551069308, 112.9155762719810383 ) ) ;
#41402=CARTESIAN_POINT ( 'NONE',  ( -19.05341960407617563, 5.049401038297882671, 33.54275706135231871 ) ) ;
#41403=CARTESIAN_POINT ( 'NONE',  ( 14.34966873604972726, -8.224510206698740333, 100.8344237280190185 ) ) ;
#41404=CARTESIAN_POINT ( 'NONE',  ( -0.05219959533909027116, -19.03943276465977164, 82.49890960531436690 ) ) ;
#41405=CARTESIAN_POINT ( 'NONE',  ( -0.05219959533937732626, 21.53943276465977519, 47.50109039468568994 ) ) ;
#41406=CARTESIAN_POINT ( 'NONE',  ( -10.72451020669898014, 18.67979575497178502, 40.41557627198103120 ) ) ;
#41407=CARTESIAN_POINT ( 'NONE',  ( -21.55341960407619339, 5.719274019375674811, 38.54275706135234714 ) ) ;
#41408=CARTESIAN_POINT ( 'NONE',  ( 21.53943276465977519, -0.05219959533907433946, 83.74890960531435269 ) ) ;
#41409=CARTESIAN_POINT ( 'NONE',  ( -4.483927247898539470, -16.52544592524342804, 92.29057627198103830 ) ) ;
#41410=CARTESIAN_POINT ( 'NONE',  ( 19.03943276465977164, 0.05219959533936151252, 56.25109039468566863 ) ) ;
#41411=CARTESIAN_POINT ( 'NONE',  ( -13.89961937509977652, 13.97604488694528158, 35.62390960531435269 ) ) ;
#41412=CARTESIAN_POINT ( 'NONE',  ( -19.05341960407611168, -5.049401038298163336, 101.4572429386476955 ) ) ;
#41413=CARTESIAN_POINT ( 'NONE',  ( -19.02544592524342804, 5.153800228976336051, 101.0405762719810241 ) ) ;
#41414=CARTESIAN_POINT ( 'NONE',  ( -16.53943276465976808, 0.05219959533911058130, 111.2489096053143669 ) ) ;
#41415=CARTESIAN_POINT ( 'NONE',  ( -12.14591786802309592, -12.06949235617757132, 26.87390960531435979 ) ) ;
#41416=CARTESIAN_POINT ( 'NONE',  ( 14.34966873604972726, -8.224510206698740333, 40.83442372801901854 ) ) ;
#41417=CARTESIAN_POINT ( 'NONE',  ( 18.67979575497194134, -10.72451020669871369, 100.8344237280190185 ) ) ;
#41418=CARTESIAN_POINT ( 'NONE',  ( -19.02544592524342804, 5.153800228976336051, 111.0405762719810099 ) ) ;
#41419=CARTESIAN_POINT ( 'NONE',  ( 4.483927247898790824, -16.52544592524335698, 110.2094237280190185 ) ) ;
#41420=CARTESIAN_POINT ( 'NONE',  ( 5.823673210054444382, -21.52544592524334988, 30.20942372801902565 ) ) ;
#41421=CARTESIAN_POINT ( 'NONE',  ( 16.51473224551069308, 9.474510206698969483, 49.16557627198102409 ) ) ;
#41422=CARTESIAN_POINT ( 'NONE',  ( -8.224510206698735004, -14.34966873604973081, 44.58442372801901854 ) ) ;
#41423=CARTESIAN_POINT ( 'NONE',  ( -16.55341960407617563, 4.379528057220093196, 108.5427570613523756 ) ) ;
#41424=CARTESIAN_POINT ( 'NONE',  ( -4.483927247898782831, 16.52544592524335698, 97.70942372801904696 ) ) ;
#41425=CARTESIAN_POINT ( 'NONE',  ( -19.02544592524334988, -5.153800228976617603, 108.9594237280189759 ) ) ;
#41426=CARTESIAN_POINT ( 'NONE',  ( 9.564922557960805705, 16.46253265017160317, 29.58224293864769550 ) ) ;
#41427=CARTESIAN_POINT ( 'NONE',  ( 4.483927247898545687, 16.52544592524342804, 109.7905762719810383 ) ) ;
#41428=CARTESIAN_POINT ( 'NONE',  ( -21.52544592524343514, 5.823673210054127303, 101.0405762719810383 ) ) ;
#41429=CARTESIAN_POINT ( 'NONE',  ( -13.89961937509977652, 13.97604488694528158, 30.62390960531435269 ) ) ;
#41430=CARTESIAN_POINT ( 'NONE',  ( -19.05341960407611168, -5.049401038298163336, 106.4572429386476955 ) ) ;
#41431=CARTESIAN_POINT ( 'NONE',  ( 21.52544592524334988, 5.823673210054432836, 36.45942372801901143 ) ) ;
#41433=CARTESIAN_POINT ( 'NONE',  ( -16.46253265017160317, 9.564922557960807481, 110.8322429386476955 ) ) ;
#41435=CARTESIAN_POINT ( 'NONE',  ( 5.153800228976335163, 19.02544592524342804, 104.7905762719809957 ) ) ;
#41436=CARTESIAN_POINT ( 'NONE',  ( 10.81492255796106328, -18.62759615963255655, 30.41775706135234358 ) ) ;
#41437=CARTESIAN_POINT ( 'NONE',  ( -4.483927247898539470, -16.52544592524342804, 87.29057627198103830 ) ) ;
#41438=CARTESIAN_POINT ( 'NONE',  ( 16.46253265017160672, -9.564922557960803928, 93.33224293864769550 ) ) ;
#41439=CARTESIAN_POINT ( 'NONE',  ( 5.153800228976617603, -19.02544592524335343, 70.20942372801900433 ) ) ;
#41440=CARTESIAN_POINT ( 'NONE',  ( 16.55341960407618274, -4.379528057220086978, 61.04275706135234714 ) ) ;
#41442=CARTESIAN_POINT ( 'NONE',  ( 5.719274019375673035, 21.55341960407619339, 82.29275706135234714 ) ) ;
#41443=CIRCLE ( 'NONE', #106078, 2.000000000000001776 ) ;
#41444=CARTESIAN_POINT ( 'NONE',  ( -4.379528057220086978, -16.55341960407618274, 39.79275706135235424 ) ) ;
#41445=CARTESIAN_POINT ( 'NONE',  ( -19.03943276465977164, 0.05219959533909376836, 76.24890960531435269 ) ) ;
#41446=CARTESIAN_POINT ( 'NONE',  ( -16.51473224551082808, 9.474510206698731452, 103.3344237280190043 ) ) ;
#41447=CARTESIAN_POINT ( 'NONE',  ( 0.05219959533934541429, -16.53943276465976808, 75.00109039468568994 ) ) ;
#41448=CARTESIAN_POINT ( 'NONE',  ( -15.72974639402176322, -15.80617190586768395, 109.3760903946857042 ) ) ;
#41449=CARTESIAN_POINT ( 'NONE',  ( 19.05341960407617918, -5.049401038297876454, 91.04275706135234714 ) ) ;
#41450=CARTESIAN_POINT ( 'NONE',  ( 13.89961937509977652, -13.97604488694527269, 68.12390960531436690 ) ) ;
#41451=CARTESIAN_POINT ( 'NONE',  ( 21.55341960407610458, 5.719274019375980345, 78.95724293864769550 ) ) ;
#41452=CARTESIAN_POINT ( 'NONE',  ( 14.29746914071049879, -8.314922557960816363, 93.33224293864769550 ) ) ;
#41453=CARTESIAN_POINT ( 'NONE',  ( -13.97604488694547697, 13.89961937509957934, 93.12609039468566152 ) ) ;
#41454=CARTESIAN_POINT ( 'NONE',  ( -4.379528057220086978, -16.55341960407618274, 59.79275706135234714 ) ) ;
#41456=CARTESIAN_POINT ( 'NONE',  ( -5.049401038297874678, -19.05341960407617918, 54.79275706135234003 ) ) ;
#41457=CARTESIAN_POINT ( 'NONE',  ( 4.379528057220339221, -16.55341960407611168, 37.70724293864769550 ) ) ;
#41458=CARTESIAN_POINT ( 'NONE',  ( -4.483927247898539470, -16.52544592524342804, 82.29057627198103830 ) ) ;
#41459=CARTESIAN_POINT ( 'NONE',  ( 0.05219959533936267826, -19.03943276465977164, 20.00109039468567218 ) ) ;
#41460=CARTESIAN_POINT ( 'NONE',  ( -17.58332526062528345, -7.635886036038592728, 44.07665040441535353 ) ) ;
#41461=CARTESIAN_POINT ( 'NONE',  ( -18.62759615963255300, -10.81492255796106328, 19.16775706135234714 ) ) ;
#41462=CARTESIAN_POINT ( 'NONE',  ( 13.89961937509977652, -13.97604488694527269, 98.12390960531433848 ) ) ;
#41463=CARTESIAN_POINT ( 'NONE',  ( 16.51473224551069308, 9.474510206698969483, 79.16557627198103830 ) ) ;
#41464=CARTESIAN_POINT ( 'NONE',  ( 5.719274019375673035, 21.55341960407619339, 92.29275706135236135 ) ) ;
#41465=CARTESIAN_POINT ( 'NONE',  ( 9.474510206698971260, -16.51473224551069308, 77.91557627198103830 ) ) ;
#41466=CARTESIAN_POINT ( 'NONE',  ( -0.05219959533907301413, -21.53943276465977519, 32.49890960531435979 ) ) ;
#41467=CARTESIAN_POINT ( 'NONE',  ( 8.314922557960818139, 14.29746914071049879, 79.58224293864769550 ) ) ;
#41469=CARTESIAN_POINT ( 'NONE',  ( 9.564922557960805705, 16.46253265017160317, 44.58224293864769550 ) ) ;
#41470=CARTESIAN_POINT ( 'NONE',  ( 16.53943276465976808, -0.05219959533910856209, 103.7489096053143669 ) ) ;
#41471=CARTESIAN_POINT ( 'NONE',  ( -0.05219959533907301413, -21.53943276465977519, 107.4989096053143669 ) ) ;
#41472=CARTESIAN_POINT ( 'NONE',  ( -18.67979575497193778, 10.72451020669871902, 58.33442372801901143 ) ) ;
#41473=CARTESIAN_POINT ( 'NONE',  ( 19.02544592524343514, -5.153800228976328945, 28.54057627198102409 ) ) ;
#41474=CARTESIAN_POINT ( 'NONE',  ( 16.55341960407618274, -4.379528057220086978, 66.04275706135236135 ) ) ;
#41475=CARTESIAN_POINT ( 'NONE',  ( 15.80617190586746368, 15.72974639402197994, 99.37390960531436690 ) ) ;
#41476=CARTESIAN_POINT ( 'NONE',  ( 21.55341960407610458, 5.719274019375980345, 113.9572429386477239 ) ) ;
#41477=CARTESIAN_POINT ( 'NONE',  ( 5.049401038297881783, 19.05341960407617563, 42.29275706135234003 ) ) ;
#41478=CARTESIAN_POINT ( 'NONE',  ( 19.05341960407611168, 5.049401038298154454, 53.95724293864770260 ) ) ;
#41479=CARTESIAN_POINT ( 'NONE',  ( 16.51473224551069308, 9.474510206698969483, 114.1655762719810241 ) ) ;
#41480=CARTESIAN_POINT ( 'NONE',  ( -5.719274019375665041, -21.55341960407619695, 59.79275706135234714 ) ) ;
#41481=CARTESIAN_POINT ( 'NONE',  ( -10.72451020669898014, 18.67979575497178502, 60.41557627198102409 ) ) ;
#41482=CARTESIAN_POINT ( 'NONE',  ( -4.483927247898539470, -16.52544592524342804, 42.29057627198103120 ) ) ;
#41483=CARTESIAN_POINT ( 'NONE',  ( 18.62759615963255655, 10.81492255796105972, 71.66775706135234714 ) ) ;
#41484=CARTESIAN_POINT ( 'NONE',  ( -5.719274019375665041, -21.55341960407619695, 104.7927570613523898 ) ) ;
#41485=CARTESIAN_POINT ( 'NONE',  ( 8.224510206698953496, -14.34966873604960469, 52.91557627198103830 ) ) ;
#41486=CARTESIAN_POINT ( 'NONE',  ( -8.314922557960811034, -14.29746914071050412, 107.0822429386476955 ) ) ;
#41487=CARTESIAN_POINT ( 'NONE',  ( 13.89961937509957401, 13.97604488694547697, 41.87609039468566152 ) ) ;
#41488=CARTESIAN_POINT ( 'NONE',  ( 16.55341960407618274, -4.379528057220086978, 101.0427570613523756 ) ) ;
#41489=CARTESIAN_POINT ( 'NONE',  ( 21.53943276465977519, 0.05219959533937863772, 71.25109039468568994 ) ) ;
#41490=ADVANCED_FACE ( 'NONE', ( #148200 ), #89511, .F. ) ;
#41491=CARTESIAN_POINT ( 'NONE',  ( -9.474510206698964154, 16.51473224551069663, 55.41557627198103120 ) ) ;
#41492=CARTESIAN_POINT ( 'NONE',  ( 16.46253265017146816, 9.564922557961045513, 31.66775706135232937 ) ) ;
#41493=CARTESIAN_POINT ( 'NONE',  ( -5.719274019375978568, 21.55341960407610458, 40.20724293864769550 ) ) ;
#41495=CARTESIAN_POINT ( 'NONE',  ( -18.67979575497193778, 10.72451020669871902, 28.33442372801902209 ) ) ;
#41496=CARTESIAN_POINT ( 'NONE',  ( -15.72974639402197994, 15.80617190586746368, 85.62390960531436690 ) ) ;
#41497=CARTESIAN_POINT ( 'NONE',  ( -5.153800228976607833, 19.02544592524334988, 87.70942372801897591 ) ) ;
#41498=CARTESIAN_POINT ( 'NONE',  ( -12.06949235617739369, -12.14591786802326823, 54.37609039468568994 ) ) ;
#41500=CARTESIAN_POINT ( 'NONE',  ( -5.823673210054116645, -21.52544592524344225, 92.29057627198103830 ) ) ;
#41501=CARTESIAN_POINT ( 'NONE',  ( -12.06949235617756955, 12.14591786802309770, 80.62390960531438111 ) ) ;
#41502=CARTESIAN_POINT ( 'NONE',  ( -17.50000000000000000, -5.622605283950869115, 101.3120731059611046 ) ) ;
#41503=CARTESIAN_POINT ( 'NONE',  ( -14.34966873604972548, 8.224510206698743886, 28.33442372801902209 ) ) ;
#41504=CARTESIAN_POINT ( 'NONE',  ( 5.823673210054125526, 21.52544592524343514, 49.79057627198102409 ) ) ;
#41505=CARTESIAN_POINT ( 'NONE',  ( -16.52544592524335698, -4.483927247898792601, 73.95942372801901854 ) ) ;
#41506=CARTESIAN_POINT ( 'NONE',  ( 0.05219959533909260263, 19.03943276465977164, 24.99890960531435269 ) ) ;
#41507=EDGE_CURVE ( 'NONE', #96464, #7679, #11985, .T. ) ;
#41508=CARTESIAN_POINT ( 'NONE',  ( -16.55341960407617563, 4.379528057220093196, 58.54275706135235424 ) ) ;
#41509=CARTESIAN_POINT ( 'NONE',  ( 15.80617190586769283, -15.72974639402175789, 25.62609039468567929 ) ) ;
#41510=CARTESIAN_POINT ( 'NONE',  ( -18.67979575497178146, -10.72451020669898902, 51.66557627198102409 ) ) ;
#41511=CARTESIAN_POINT ( 'NONE',  ( 14.34966873604972726, -8.224510206698740333, 70.83442372801901854 ) ) ;
#41512=CARTESIAN_POINT ( 'NONE',  ( 19.05341960407611168, 5.049401038298154454, 98.95724293864766707 ) ) ;
#41513=CARTESIAN_POINT ( 'NONE',  ( 10.72451020669871369, 18.67979575497193778, 52.08442372801901854 ) ) ;
#41514=CARTESIAN_POINT ( 'NONE',  ( 5.049401038298161559, -19.05341960407611168, 32.70724293864768129 ) ) ;
#41515=CARTESIAN_POINT ( 'NONE',  ( -18.62759615963270932, 10.81492255796079327, 40.83224293864769550 ) ) ;
#41516=CARTESIAN_POINT ( 'NONE',  ( -10.81492255796078084, -18.62759615963271287, 22.08224293864769194 ) ) ;
#41518=CARTESIAN_POINT ( 'NONE',  ( -0.05219959533936034679, 19.03943276465977164, 32.50109039468566863 ) ) ;
#41519=CARTESIAN_POINT ( 'NONE',  ( -4.483927247898782831, 16.52544592524335698, 52.70942372801902565 ) ) ;
#41520=CARTESIAN_POINT ( 'NONE',  ( 16.51473224551069308, 9.474510206698969483, 109.1655762719810383 ) ) ;
#41522=CARTESIAN_POINT ( 'NONE',  ( 19.02544592524343514, -5.153800228976328945, 83.54057627198100988 ) ) ;
#41523=CARTESIAN_POINT ( 'NONE',  ( 8.224510206698742110, 14.34966873604972548, 102.0844237280190185 ) ) ;
#41525=CARTESIAN_POINT ( 'NONE',  ( 8.314922557960818139, 14.29746914071049879, 89.58224293864768129 ) ) ;
#41526=CARTESIAN_POINT ( 'NONE',  ( 21.53943276465977519, -0.05219959533907433946, 53.74890960531437401 ) ) ;
#41527=CARTESIAN_POINT ( 'NONE',  ( 9.474510206698971260, -16.51473224551069308, 37.91557627198102409 ) ) ;
#41528=CARTESIAN_POINT ( 'NONE',  ( -16.52544592524335698, -4.483927247898792601, 73.95942372801901854 ) ) ;
#41529=CARTESIAN_POINT ( 'NONE',  ( -5.719274019375665041, -21.55341960407619695, 24.79275706135235779 ) ) ;
#41530=CARTESIAN_POINT ( 'NONE',  ( -5.049401038297874678, -19.05341960407617918, 89.79275706135230450 ) ) ;
#41531=CARTESIAN_POINT ( 'NONE',  ( -19.02544592524342804, 5.153800228976336051, 36.04057627198100988 ) ) ;
#41533=CARTESIAN_POINT ( 'NONE',  ( -21.53943276465977519, -0.05219959533937600094, 103.7510903946857042 ) ) ;
#41534=CARTESIAN_POINT ( 'NONE',  ( -9.474510206698964154, 16.51473224551069663, 80.41557627198103830 ) ) ;
#41535=CARTESIAN_POINT ( 'NONE',  ( 12.06949235617739724, 12.14591786802326823, 61.87609039468568284 ) ) ;
#41536=CARTESIAN_POINT ( 'NONE',  ( -5.719274019375665041, -21.55341960407619695, 89.79275706135236135 ) ) ;
#41537=CARTESIAN_POINT ( 'NONE',  ( -19.05341960407617563, 5.049401038297882671, 48.54275706135233293 ) ) ;
#41539=CARTESIAN_POINT ( 'NONE',  ( 0.05219959533936267826, -19.03943276465977164, 60.00109039468566863 ) ) ;
#41540=ORIENTED_EDGE ( 'NONE', *, *, #98398, .F. ) ;
#41541=CARTESIAN_POINT ( 'NONE',  ( 10.81492255796106328, -18.62759615963255655, 55.41775706135234714 ) ) ;
#41542=CARTESIAN_POINT ( 'NONE',  ( 17.58332526062526568, -7.635886036038552760, 58.42334959558466778 ) ) ;
#41543=CARTESIAN_POINT ( 'NONE',  ( 19.02544592524334988, 5.153800228976608722, 51.45942372801900433 ) ) ;
#41544=CARTESIAN_POINT ( 'NONE',  ( -0.05219959533909027116, -19.03943276465977164, 97.49890960531436690 ) ) ;
#41545=CARTESIAN_POINT ( 'NONE',  ( 19.05341960407611168, 5.049401038298154454, 78.95724293864769550 ) ) ;
#41546=CARTESIAN_POINT ( 'NONE',  ( -14.34966873604960291, -8.224510206698953496, 36.66557627198103120 ) ) ;
#41547=CARTESIAN_POINT ( 'NONE',  ( 10.72451020669898902, -18.67979575497178502, 32.91557627198102409 ) ) ;
#41550=CARTESIAN_POINT ( 'NONE',  ( 21.52544592524334988, 5.823673210054432836, 111.4594237280190328 ) ) ;
#41552=CARTESIAN_POINT ( 'NONE',  ( 19.02544592524343514, -5.153800228976328945, 33.54057627198102409 ) ) ;
#41553=CARTESIAN_POINT ( 'NONE',  ( -13.97604488694527625, -13.89961937509977652, 21.87390960531435979 ) ) ;
#41556=CARTESIAN_POINT ( 'NONE',  ( 16.52544592524335698, 4.483927247898782831, 66.45942372801903275 ) ) ;
#41557=CARTESIAN_POINT ( 'NONE',  ( -18.62759615963270932, 10.81492255796079327, 80.83224293864769550 ) ) ;
#41558=CARTESIAN_POINT ( 'NONE',  ( -4.379528057220328563, 16.55341960407611168, 55.20724293864770260 ) ) ;
#41559=CARTESIAN_POINT ( 'NONE',  ( 5.049401038298161559, -19.05341960407611168, 22.70724293864769194 ) ) ;
#41560=CARTESIAN_POINT ( 'NONE',  ( -19.05341960407611168, -5.049401038298163336, 106.4572429386476955 ) ) ;
#41561=CARTESIAN_POINT ( 'NONE',  ( 10.72451020669871369, 18.67979575497193778, 27.08442372801901854 ) ) ;
#41562=CARTESIAN_POINT ( 'NONE',  ( 16.51473224551083163, -9.474510206698727899, 30.83442372801900433 ) ) ;
#41563=CARTESIAN_POINT ( 'NONE',  ( 9.474510206698971260, -16.51473224551069308, 32.91557627198102409 ) ) ;
#41564=CARTESIAN_POINT ( 'NONE',  ( 21.53943276465977519, 0.05219959533937863772, 86.25109039468568994 ) ) ;
#41565=CARTESIAN_POINT ( 'NONE',  ( 16.79531203550645202, -7.028104445595737992, 31.24755011779557989 ) ) ;
#41566=CARTESIAN_POINT ( 'NONE',  ( -12.06949235617756955, 12.14591786802309770, 30.62390960531436335 ) ) ;
#41568=CARTESIAN_POINT ( 'NONE',  ( -15.80617190586745835, -15.72974639402198527, 36.87390960531435979 ) ) ;
#41569=CARTESIAN_POINT ( 'NONE',  ( 4.379528057220339221, -16.55341960407611168, 97.70724293864772392 ) ) ;
#41571=CARTESIAN_POINT ( 'NONE',  ( -19.03943276465977164, 0.05219959533909376836, 86.24890960531436690 ) ) ;
#41572=CARTESIAN_POINT ( 'NONE',  ( -16.55341960407611168, -4.379528057220339221, 91.45724293864769550 ) ) ;
#41573=CARTESIAN_POINT ( 'NONE',  ( -0.05219959533936034679, 19.03943276465977164, 107.5010903946856615 ) ) ;
#41574=CARTESIAN_POINT ( 'NONE',  ( 18.67979575497178502, 10.72451020669898547, 59.16557627198103120 ) ) ;
#41575=ORIENTED_EDGE ( 'NONE', *, *, #80930, .F. ) ;
#41576=CARTESIAN_POINT ( 'NONE',  ( 19.05341960407611168, 5.049401038298154454, 33.95724293864769550 ) ) ;
#41577=CARTESIAN_POINT ( 'NONE',  ( 9.564922557960805705, 16.46253265017160317, 89.58224293864769550 ) ) ;
#41578=CARTESIAN_POINT ( 'NONE',  ( -18.67979575497178146, -10.72451020669898902, 91.66557627198103830 ) ) ;
#41579=CARTESIAN_POINT ( 'NONE',  ( 16.53943276465976808, 0.05219959533934440121, 106.2510903946856757 ) ) ;
#41580=CARTESIAN_POINT ( 'NONE',  ( -16.51473224551069308, -9.474510206698971260, 91.66557627198103830 ) ) ;
#41581=CARTESIAN_POINT ( 'NONE',  ( -0.05219959533936034679, 19.03943276465977164, 82.50109039468567573 ) ) ;
#41582=CARTESIAN_POINT ( 'NONE',  ( 10.81492255796106328, -18.62759615963255655, 90.41775706135236135 ) ) ;
#41583=CARTESIAN_POINT ( 'NONE',  ( -21.52544592524343514, 5.823673210054127303, 81.04057627198102409 ) ) ;
#41584=CARTESIAN_POINT ( 'NONE',  ( -18.67979575497178146, -10.72451020669898902, 36.66557627198103120 ) ) ;
#41585=CARTESIAN_POINT ( 'NONE',  ( -13.97604488694527625, -13.89961937509977652, 56.87390960531434558 ) ) ;
#41586=CARTESIAN_POINT ( 'NONE',  ( -4.379528057220086978, -16.55341960407618274, 109.7927570613523613 ) ) ;
#41587=CARTESIAN_POINT ( 'NONE',  ( 13.89961937509977652, -13.97604488694527269, 68.12390960531436690 ) ) ;
#41590=CARTESIAN_POINT ( 'NONE',  ( 9.564922557961047289, -16.46253265017146816, 25.41775706135234003 ) ) ;
#41591=CARTESIAN_POINT ( 'NONE',  ( 16.55341960407611168, 4.379528057220329451, 73.95724293864769550 ) ) ;
#41592=CARTESIAN_POINT ( 'NONE',  ( -18.62759615963255300, -10.81492255796106328, 19.16775706135234714 ) ) ;
#41594=CARTESIAN_POINT ( 'NONE',  ( -18.62759615963270932, 10.81492255796079327, 65.83224293864769550 ) ) ;
#41595=CARTESIAN_POINT ( 'NONE',  ( -14.34966873604972548, 8.224510206698743886, 98.33442372801901854 ) ) ;
#41596=CARTESIAN_POINT ( 'NONE',  ( 4.483927247898545687, 16.52544592524342804, 104.7905762719810241 ) ) ;
#41597=CARTESIAN_POINT ( 'NONE',  ( 19.02544592524343514, -5.153800228976328945, 68.54057627198103830 ) ) ;
#41599=CARTESIAN_POINT ( 'NONE',  ( -8.224510206698948167, 14.34966873604960824, 25.41557627198103120 ) ) ;
#41600=CARTESIAN_POINT ( 'NONE',  ( 21.53943276465977519, 0.05219959533937863772, 46.25109039468567573 ) ) ;
#41601=CARTESIAN_POINT ( 'NONE',  ( -16.51473224551069308, -9.474510206698971260, 111.6655762719810383 ) ) ;
#41602=CARTESIAN_POINT ( 'NONE',  ( 21.55341960407619695, -5.719274019375665929, 76.04275706135237556 ) ) ;
#41603=CARTESIAN_POINT ( 'NONE',  ( 13.97604488694527802, 13.89961937509977652, 34.37390960531436690 ) ) ;
#41604=CARTESIAN_POINT ( 'NONE',  ( -13.97604488694527625, -13.89961937509977652, 31.87390960531435979 ) ) ;
#41606=CARTESIAN_POINT ( 'NONE',  ( -10.81492255796105439, 18.62759615963255655, 92.91775706135236135 ) ) ;
#41607=CARTESIAN_POINT ( 'NONE',  ( -14.29746914071037622, -8.314922557961029526, 49.16775706135234003 ) ) ;
#41608=CARTESIAN_POINT ( 'NONE',  ( 21.55341960407619695, -5.719274019375665929, 76.04275706135237556 ) ) ;
#41609=CARTESIAN_POINT ( 'NONE',  ( 16.46253265017160672, -9.564922557960803928, 98.33224293864769550 ) ) ;
#41610=CARTESIAN_POINT ( 'NONE',  ( -16.51473224551082808, 9.474510206698731452, 83.33442372801899012 ) ) ;
#41611=CARTESIAN_POINT ( 'NONE',  ( 21.53943276465977519, 0.05219959533937863772, 61.25109039468567573 ) ) ;
#41612=CARTESIAN_POINT ( 'NONE',  ( 5.049401038297881783, 19.05341960407617563, 112.2927570613523471 ) ) ;
#41613=CARTESIAN_POINT ( 'NONE',  ( 16.51473224551083163, -9.474510206698727899, 80.83442372801899012 ) ) ;
#41614=CARTESIAN_POINT ( 'NONE',  ( 0.05219959533909260263, 19.03943276465977164, 54.99890960531435979 ) ) ;
#41615=CARTESIAN_POINT ( 'NONE',  ( 19.05341960407617918, -5.049401038297876454, 91.04275706135234714 ) ) ;
#41616=CARTESIAN_POINT ( 'NONE',  ( -8.314922557960811034, -14.29746914071050412, 27.08224293864769550 ) ) ;
#41617=CARTESIAN_POINT ( 'NONE',  ( 9.474510206698729675, 16.51473224551082808, 92.08442372801900433 ) ) ;
#41618=CARTESIAN_POINT ( 'NONE',  ( 16.52544592524342804, -4.483927247898539470, 43.54057627198103830 ) ) ;
#41620=CARTESIAN_POINT ( 'NONE',  ( -19.03943276465977164, -0.05219959533935918106, 63.75109039468566863 ) ) ;
#41621=CARTESIAN_POINT ( 'NONE',  ( -4.483927247898782831, 16.52544592524335698, 47.70942372801902565 ) ) ;
#41622=CARTESIAN_POINT ( 'NONE',  ( 5.153800228976615827, -19.02544592524334988, 30.20942372801900433 ) ) ;
#41623=CARTESIAN_POINT ( 'NONE',  ( -0.05219959533909027116, -19.03943276465977164, 27.49890960531435624 ) ) ;
#41624=CARTESIAN_POINT ( 'NONE',  ( -5.153800228976328057, -19.02544592524343514, 47.29057627198102409 ) ) ;
#41625=CARTESIAN_POINT ( 'NONE',  ( -4.379528057220086978, -16.55341960407618274, 44.79275706135234714 ) ) ;
#41628=CARTESIAN_POINT ( 'NONE',  ( -0.05219959533909027116, -19.03943276465977164, 87.49890960531436690 ) ) ;
#41629=CARTESIAN_POINT ( 'NONE',  ( 9.564922557961047289, -16.46253265017146816, 85.41775706135233293 ) ) ;
#41631=CARTESIAN_POINT ( 'NONE',  ( -9.564922557961040184, 16.46253265017147172, 102.9177570613523329 ) ) ;
#41632=CARTESIAN_POINT ( 'NONE',  ( -15.80617190586745835, -15.72974639402198527, 31.87390960531435979 ) ) ;
#41633=CARTESIAN_POINT ( 'NONE',  ( 9.474510206698729675, 16.51473224551082808, 27.08442372801900433 ) ) ;
#41634=CARTESIAN_POINT ( 'NONE',  ( 19.03943276465977164, 0.05219959533936151252, 111.2510903946856757 ) ) ;
#41635=CARTESIAN_POINT ( 'NONE',  ( -12.06949235617756955, 12.14591786802309770, 105.6239096053143669 ) ) ;
#41636=CARTESIAN_POINT ( 'NONE',  ( -9.564922557960796823, -16.46253265017161027, 37.08224293864768839 ) ) ;
#41637=CARTESIAN_POINT ( 'NONE',  ( 21.53943276465977519, -0.05219959533907433946, 68.74890960531435269 ) ) ;
#41638=CARTESIAN_POINT ( 'NONE',  ( 5.153800228976335163, 19.02544592524342804, 39.79057627198100988 ) ) ;
#41640=CARTESIAN_POINT ( 'NONE',  ( 0.05219959533936267826, -19.03943276465977164, 65.00109039468567573 ) ) ;
#41641=CARTESIAN_POINT ( 'NONE',  ( 14.34966873604960469, 8.224510206698951720, 59.16557627198103120 ) ) ;
#41642=CARTESIAN_POINT ( 'NONE',  ( 21.52544592524344225, -5.823673210054117533, 33.54057627198102409 ) ) ;
#41643=CARTESIAN_POINT ( 'NONE',  ( 21.52544592524334988, 5.823673210054432836, 96.45942372801901854 ) ) ;
#41644=CARTESIAN_POINT ( 'NONE',  ( 10.72451020669898902, -18.67979575497178502, 77.91557627198102409 ) ) ;
#41645=CARTESIAN_POINT ( 'NONE',  ( 21.52544592524334988, 5.823673210054432836, 76.45942372801901854 ) ) ;
#41646=CARTESIAN_POINT ( 'NONE',  ( -21.53943276465977519, -0.05219959533937600094, 58.75109039468568994 ) ) ;
#41648=CARTESIAN_POINT ( 'NONE',  ( -16.51473224551069308, -9.474510206698971260, 101.6655762719810241 ) ) ;
#41649=CARTESIAN_POINT ( 'NONE',  ( -12.14591786802326823, 12.06949235617739902, 93.12609039468568994 ) ) ;
#41650=CARTESIAN_POINT ( 'NONE',  ( -15.80617190586768217, 15.72974639402176855, 68.12609039468567573 ) ) ;
#41651=CARTESIAN_POINT ( 'NONE',  ( -13.97604488694527625, -13.89961937509977652, 51.87390960531436690 ) ) ;
#41652=CARTESIAN_POINT ( 'NONE',  ( 18.67979575497194134, -10.72451020669871369, 30.83442372801902209 ) ) ;
#41653=CARTESIAN_POINT ( 'NONE',  ( 19.03943276465977164, -0.05219959533909143690, 73.74890960531435269 ) ) ;
#41654=CARTESIAN_POINT ( 'NONE',  ( -16.53943276465976808, 0.05219959533911058130, 76.24890960531435269 ) ) ;
#41655=CARTESIAN_POINT ( 'NONE',  ( 14.34966873604960469, 8.224510206698951720, 44.16557627198103120 ) ) ;
#41656=CARTESIAN_POINT ( 'NONE',  ( 21.53943276465977519, -0.05219959533907433946, 63.74890960531435979 ) ) ;
#41657=ADVANCED_FACE ( 'NONE', ( #64138 ), #47985, .F. ) ;
#41658=CARTESIAN_POINT ( 'NONE',  ( -0.05219959533909027116, -19.03943276465977164, 42.49890960531435269 ) ) ;
#41659=CARTESIAN_POINT ( 'NONE',  ( 15.72974639402199770, -15.80617190586745480, 58.12390960531435979 ) ) ;
#41660=CARTESIAN_POINT ( 'NONE',  ( 0.05219959533936267826, -19.03943276465977164, 50.00109039468566863 ) ) ;
#41661=CARTESIAN_POINT ( 'NONE',  ( -5.049401038297874678, -19.05341960407618274, 24.79275706135234358 ) ) ;
#41662=CARTESIAN_POINT ( 'NONE',  ( 14.29746914071049879, -8.314922557960816363, 58.33224293864768839 ) ) ;
#41663=CARTESIAN_POINT ( 'NONE',  ( 0.05219959533907565091, 21.53943276465977519, 34.99890960531435979 ) ) ;
#41665=CARTESIAN_POINT ( 'NONE',  ( 17.05116617787824396, 6.768360034955816396, 103.8432444674080273 ) ) ;
#41666=CARTESIAN_POINT ( 'NONE',  ( -16.55341960407617563, 4.379528057220093196, 83.54275706135234714 ) ) ;
#41667=CARTESIAN_POINT ( 'NONE',  ( -16.46253265017146816, -9.564922557961047289, 84.16775706135233293 ) ) ;
#41668=CARTESIAN_POINT ( 'NONE',  ( -16.53943276465976808, 0.05219959533911058130, 56.24890960531436690 ) ) ;
#41670=CARTESIAN_POINT ( 'NONE',  ( 19.02544592524343514, -5.153800228976328945, 53.54057627198102409 ) ) ;
#41671=CARTESIAN_POINT ( 'NONE',  ( 0.05219959533910956823, 16.53943276465976808, 39.99890960531436690 ) ) ;
#41672=CARTESIAN_POINT ( 'NONE',  ( 5.153800228976335163, 19.02544592524342804, 94.79057627198103830 ) ) ;
#41673=CARTESIAN_POINT ( 'NONE',  ( 9.474510206698971260, -16.51473224551069308, 47.91557627198102409 ) ) ;
#41674=CARTESIAN_POINT ( 'NONE',  ( -21.55341960407619339, 5.719274019375674811, 63.54275706135234003 ) ) ;
#41675=CARTESIAN_POINT ( 'NONE',  ( -16.46253265017160317, 9.564922557960807481, 75.83224293864769550 ) ) ;
#41676=CARTESIAN_POINT ( 'NONE',  ( 13.89961937509977652, -13.97604488694527269, 28.12390960531435624 ) ) ;
#41677=CARTESIAN_POINT ( 'NONE',  ( 19.03943276465977164, -0.05219959533909143690, 63.74890960531435979 ) ) ;
#41678=CARTESIAN_POINT ( 'NONE',  ( 15.72974639402199770, -15.80617190586745480, 53.12390960531436690 ) ) ;
#41680=CARTESIAN_POINT ( 'NONE',  ( -13.89961937509977652, 13.97604488694528158, 35.62390960531435269 ) ) ;
#41681=CARTESIAN_POINT ( 'NONE',  ( 21.53943276465977519, -0.05219959533907433946, 38.74890960531435979 ) ) ;
#41682=CARTESIAN_POINT ( 'NONE',  ( -12.14591786802326823, 12.06949235617739902, 108.1260903946856757 ) ) ;
#41683=CARTESIAN_POINT ( 'NONE',  ( -21.55341960407619339, 5.719274019375674811, 113.5427570613523756 ) ) ;
#41684=CARTESIAN_POINT ( 'NONE',  ( -16.53943276465976808, -0.05219959533934237506, 48.75109039468568284 ) ) ;
#41685=CARTESIAN_POINT ( 'NONE',  ( 4.483927247898790824, -16.52544592524335698, 80.20942372801901854 ) ) ;
#41687=CARTESIAN_POINT ( 'NONE',  ( -14.34966873604972548, 8.224510206698743886, 68.33442372801900433 ) ) ;
#41688=CARTESIAN_POINT ( 'NONE',  ( -16.53943276465976808, -0.05219959533934237506, 58.75109039468568994 ) ) ;
#41689=CARTESIAN_POINT ( 'NONE',  ( -0.05219959533909027116, -19.03943276465977164, 102.4989096053143669 ) ) ;
#41690=CARTESIAN_POINT ( 'NONE',  ( 9.564922557960805705, 16.46253265017160317, 29.58224293864769550 ) ) ;
#41691=CARTESIAN_POINT ( 'NONE',  ( 12.06949235617739724, 12.14591786802326823, 41.87609039468568284 ) ) ;
#41692=CARTESIAN_POINT ( 'NONE',  ( -13.89961937509977652, 13.97604488694528158, 50.62390960531435979 ) ) ;
#41693=CARTESIAN_POINT ( 'NONE',  ( -21.53943276465977519, -0.05219959533937600094, 28.75109039468567929 ) ) ;
#41694=CARTESIAN_POINT ( 'NONE',  ( -16.55341960407617563, 4.379528057220093196, 33.54275706135234714 ) ) ;
#41695=CARTESIAN_POINT ( 'NONE',  ( -14.29746914071037622, -8.314922557961029526, 99.16775706135234714 ) ) ;
#41697=CARTESIAN_POINT ( 'NONE',  ( 21.53943276465977519, 0.05219959533937863772, 101.2510903946856757 ) ) ;
#41698=CARTESIAN_POINT ( 'NONE',  ( -5.153800228976607833, 19.02544592524334988, 102.7094237280189759 ) ) ;
#41699=CARTESIAN_POINT ( 'NONE',  ( 14.29746914071049879, -8.314922557960816363, 63.33224293864770260 ) ) ;
#41700=CARTESIAN_POINT ( 'NONE',  ( 16.51473224551069308, 9.474510206698969483, 29.16557627198103475 ) ) ;
#41701=CARTESIAN_POINT ( 'NONE',  ( 19.05341960407617918, -5.049401038297876454, 66.04275706135233293 ) ) ;
#41702=CARTESIAN_POINT ( 'NONE',  ( 16.21995358207276894, -7.366697692864364377, 57.43551001512073384 ) ) ;
#41703=CARTESIAN_POINT ( 'NONE',  ( 5.719274019375673035, 21.55341960407619339, 67.29275706135234714 ) ) ;
#41704=CARTESIAN_POINT ( 'NONE',  ( -12.14591786802326823, 12.06949235617739902, 23.12609039468567573 ) ) ;
#41705=CARTESIAN_POINT ( 'NONE',  ( -17.60769864724391098, 5.499999999999987566, 63.65024842019166584 ) ) ;
#41706=CARTESIAN_POINT ( 'NONE',  ( 5.153800228976335163, 19.02544592524342804, 114.7905762719810241 ) ) ;
#41707=CARTESIAN_POINT ( 'NONE',  ( -9.474510206698720793, -16.51473224551083518, 109.5844237280190043 ) ) ;
#41708=CARTESIAN_POINT ( 'NONE',  ( -9.474510206698964154, 16.51473224551069663, 115.4155762719810241 ) ) ;
#41710=CARTESIAN_POINT ( 'NONE',  ( -13.97604488694527625, -13.89961937509977652, 21.87390960531435979 ) ) ;
#41711=CARTESIAN_POINT ( 'NONE',  ( 18.62759615963255655, 10.81492255796105972, 101.6677570613523613 ) ) ;
#41712=CARTESIAN_POINT ( 'NONE',  ( -13.97604488694527625, -13.89961937509977652, 36.87390960531436690 ) ) ;
#41713=CARTESIAN_POINT ( 'NONE',  ( -5.719274019375665041, -21.55341960407619695, 49.79275706135234714 ) ) ;
#41714=CARTESIAN_POINT ( 'NONE',  ( -15.72974639402176322, -15.80617190586768395, 99.37609039468568994 ) ) ;
#41715=CARTESIAN_POINT ( 'NONE',  ( -14.34966873604972548, 8.224510206698743886, 108.3344237280190185 ) ) ;
#41716=CARTESIAN_POINT ( 'NONE',  ( 9.564922557960805705, 16.46253265017160317, 79.58224293864769550 ) ) ;
#41717=B_SPLINE_CURVE_WITH_KNOTS ( 'NONE', 3,
 ( #195606, #13545, #44882, #165255, #121706, #26749, #120711, #57079, #118753, #88388, #183399, #168215, #166250, #41914, #27750, #61025, #89393, #29712, #12572, #74238, #91344, #14535, #90375, #135907, #197578, #59045, #137875, #105554, #136882, #198568, #167240, #156019 ),
 .UNSPECIFIED., .F., .F.,
 ( 4, 2, 2, 2, 2, 2, 2, 2, 2, 2, 2, 2, 2, 2, 2, 4 ),
 ( 1.684111863762029156E-17, 0.0003712461730037040710, 0.0007424923460073912284, 0.001113738519011078657, 0.001484984692014765760, 0.002227477038022137798, 0.002598723211025810373, 0.002969969384029482080, 0.003341215557033154655, 0.003712461730036826363, 0.004083707903040498070, 0.004454954076044169778, 0.004826200249047842353, 0.005197446422051514060, 0.005568692595055185768, 0.005939938768058857475 ),
 .UNSPECIFIED. ) ;
#41718=CARTESIAN_POINT ( 'NONE',  ( -10.81492255796105439, 18.62759615963255655, 62.91775706135236135 ) ) ;
#41719=CARTESIAN_POINT ( 'NONE',  ( -21.55341960407619339, 5.719274019375674811, 48.54275706135234714 ) ) ;
#41720=CARTESIAN_POINT ( 'NONE',  ( -13.97604488694547697, 13.89961937509957934, 83.12609039468564731 ) ) ;
#41721=CARTESIAN_POINT ( 'NONE',  ( -13.97604488694527625, -13.89961937509977652, 91.87390960531432427 ) ) ;
#41722=CARTESIAN_POINT ( 'NONE',  ( 12.14591786802309770, 12.06949235617756955, 114.3739096053143527 ) ) ;
#41723=CARTESIAN_POINT ( 'NONE',  ( -21.52544592524343514, 5.823673210054127303, 96.04057627198102409 ) ) ;
#41724=CARTESIAN_POINT ( 'NONE',  ( -9.474510206698720793, -16.51473224551083518, 24.58442372801900078 ) ) ;
#41725=CARTESIAN_POINT ( 'NONE',  ( -4.483927247898539470, -16.52544592524342804, 92.29057627198103830 ) ) ;
#41726=CARTESIAN_POINT ( 'NONE',  ( -5.153800228976328057, -19.02544592524343514, 52.29057627198100988 ) ) ;
#41727=CARTESIAN_POINT ( 'NONE',  ( 19.05341960407617918, -5.049401038297876454, 81.04275706135231871 ) ) ;
#41728=CARTESIAN_POINT ( 'NONE',  ( -16.53943276465976808, 0.05219959533911058130, 51.24890960531436690 ) ) ;
#41729=CARTESIAN_POINT ( 'NONE',  ( 10.72451020669871369, 18.67979575497193778, 107.0844237280190043 ) ) ;
#41730=CARTESIAN_POINT ( 'NONE',  ( -13.97604488694527625, -13.89961937509977652, 106.8739096053143669 ) ) ;
#41731=CARTESIAN_POINT ( 'NONE',  ( 16.51473224551083163, -9.474510206698727899, 80.83442372801899012 ) ) ;
#41732=CARTESIAN_POINT ( 'NONE',  ( 10.72451020669898902, -18.67979575497178502, 82.91557627198103830 ) ) ;
#41733=CARTESIAN_POINT ( 'NONE',  ( -10.72451020669870658, -18.67979575497194134, 34.58442372801900433 ) ) ;
#41734=CARTESIAN_POINT ( 'NONE',  ( -8.314922557961024197, 14.29746914071037800, 27.91775706135234358 ) ) ;
#41735=CARTESIAN_POINT ( 'NONE',  ( -8.314922557961024197, 14.29746914071037800, 92.91775706135236135 ) ) ;
#41736=CARTESIAN_POINT ( 'NONE',  ( 17.49999999999999289, 5.624438216177601646, 61.68329655085356222 ) ) ;
#41737=CARTESIAN_POINT ( 'NONE',  ( 15.72974639402176855, 15.80617190586768217, 36.87609039468568994 ) ) ;
#41738=CARTESIAN_POINT ( 'NONE',  ( -5.823673210054116645, -21.52544592524344225, 37.29057627198102409 ) ) ;
#41739=CARTESIAN_POINT ( 'NONE',  ( -8.224510206698948167, 14.34966873604960824, 110.4155762719810383 ) ) ;
#41741=CARTESIAN_POINT ( 'NONE',  ( -14.34966873604972548, 8.224510206698743886, 63.33442372801900433 ) ) ;
#41742=CARTESIAN_POINT ( 'NONE',  ( -12.06949235617756955, 12.14591786802309770, 90.62390960531436690 ) ) ;
#41743=CARTESIAN_POINT ( 'NONE',  ( -18.62759615963270932, 10.81492255796079327, 85.83224293864768129 ) ) ;
#41744=CARTESIAN_POINT ( 'NONE',  ( 12.06949235617757843, -12.14591786802309237, 23.12390960531436335 ) ) ;
#41745=CARTESIAN_POINT ( 'NONE',  ( -12.14591786802326823, 12.06949235617739902, 48.12609039468568284 ) ) ;
#41746=CARTESIAN_POINT ( 'NONE',  ( -0.05219959533909027116, -19.03943276465977164, 52.49890960531436690 ) ) ;
#41747=CARTESIAN_POINT ( 'NONE',  ( -8.314922557961024197, 14.29746914071037800, 87.91775706135234714 ) ) ;
#41748=CARTESIAN_POINT ( 'NONE',  ( 5.153800228976615827, -19.02544592524334988, 85.20942372801900433 ) ) ;
#41749=CARTESIAN_POINT ( 'NONE',  ( -18.62759615963270932, 10.81492255796079327, 85.83224293864768129 ) ) ;
#41750=CARTESIAN_POINT ( 'NONE',  ( 16.52544592524335698, 4.483927247898782831, 106.4594237280190328 ) ) ;
#41752=CARTESIAN_POINT ( 'NONE',  ( -21.53943276465977519, 0.05219959533907696930, 66.24890960531436690 ) ) ;
#41753=CARTESIAN_POINT ( 'NONE',  ( 16.55341960407618274, -4.379528057220086978, 96.04275706135236135 ) ) ;
#41754=ORIENTED_EDGE ( 'NONE', *, *, #41507, .T. ) ;
#41755=CARTESIAN_POINT ( 'NONE',  ( 5.823673210054125526, 21.52544592524343514, 24.79057627198103120 ) ) ;
#41757=CARTESIAN_POINT ( 'NONE',  ( 10.72451020669898902, -18.67979575497178502, 92.91557627198103830 ) ) ;
#41758=CARTESIAN_POINT ( 'NONE',  ( -4.483927247898782831, 16.52544592524335698, 112.7094237280190328 ) ) ;
#41759=CARTESIAN_POINT ( 'NONE',  ( 8.314922557961029526, -14.29746914071037800, 40.41775706135234714 ) ) ;
#41760=CARTESIAN_POINT ( 'NONE',  ( 19.05341960407611168, 5.049401038298154454, 38.95724293864767418 ) ) ;
#41761=CARTESIAN_POINT ( 'NONE',  ( 12.14591786802327356, -12.06949235617739191, 35.62609039468568994 ) ) ;
#41762=CARTESIAN_POINT ( 'NONE',  ( 13.97604488694527802, 13.89961937509977652, 54.37390960531435979 ) ) ;
#41764=CARTESIAN_POINT ( 'NONE',  ( 16.51473224551069308, 9.474510206698969483, 109.1655762719810383 ) ) ;
#41765=CARTESIAN_POINT ( 'NONE',  ( -19.03943276465977164, 0.05219959533909376836, 116.2489096053143669 ) ) ;
#41766=CARTESIAN_POINT ( 'NONE',  ( 4.483927247898790824, -16.52544592524335698, 105.2094237280190328 ) ) ;
#41767=CARTESIAN_POINT ( 'NONE',  ( 16.51473224551083163, -9.474510206698727899, 95.83442372801900433 ) ) ;
#41768=CARTESIAN_POINT ( 'NONE',  ( 5.049401038297881783, 19.05341960407617563, 37.29275706135232582 ) ) ;
#41769=CARTESIAN_POINT ( 'NONE',  ( 21.55341960407610458, 5.719274019375980345, 73.95724293864769550 ) ) ;
#41770=CARTESIAN_POINT ( 'NONE',  ( -4.379528057220086978, -16.55341960407618274, 104.7927570613523898 ) ) ;
#41771=CARTESIAN_POINT ( 'NONE',  ( 10.81492255796078972, 18.62759615963270932, 34.58224293864770260 ) ) ;
#41772=CARTESIAN_POINT ( 'NONE',  ( 13.89961937509957401, 13.97604488694547697, 101.8760903946856331 ) ) ;
#41773=CARTESIAN_POINT ( 'NONE',  ( 5.153800228976335163, 19.02544592524342804, 109.7905762719810099 ) ) ;
#41774=CARTESIAN_POINT ( 'NONE',  ( -18.67979575497193778, 10.72451020669871902, 58.33442372801901143 ) ) ;
#41775=CARTESIAN_POINT ( 'NONE',  ( 13.89961937509977652, -13.97604488694527269, 58.12390960531436690 ) ) ;
#41776=CARTESIAN_POINT ( 'NONE',  ( 0.05219959533910956823, 16.53943276465976808, 94.99890960531436690 ) ) ;
#41778=CARTESIAN_POINT ( 'NONE',  ( -12.14591786802309592, -12.06949235617757132, 81.87390960531435269 ) ) ;
#41779=CARTESIAN_POINT ( 'NONE',  ( 21.52544592524344225, -5.823673210054117533, 78.54057627198103830 ) ) ;
#41781=CARTESIAN_POINT ( 'NONE',  ( 9.564922557961047289, -16.46253265017146816, 85.41775706135233293 ) ) ;
#41782=CARTESIAN_POINT ( 'NONE',  ( 18.89770734986048595, 5.499999999999949374, 91.60214472496640781 ) ) ;
#41783=CARTESIAN_POINT ( 'NONE',  ( -16.51473224551069308, -9.474510206698971260, 66.66557627198102409 ) ) ;
#41784=CARTESIAN_POINT ( 'NONE',  ( 17.50000000001358913, -5.500000000000039968, 73.29690382535059712 ) ) ;
#41785=CARTESIAN_POINT ( 'NONE',  ( -13.89961937509977652, 13.97604488694528158, 80.62390960531436690 ) ) ;
#41786=CARTESIAN_POINT ( 'NONE',  ( -5.153800228976328057, -19.02544592524343514, 87.29057627198103830 ) ) ;
#41787=CARTESIAN_POINT ( 'NONE',  ( 16.52544592524335698, 4.483927247898782831, 66.45942372801903275 ) ) ;
#41788=CARTESIAN_POINT ( 'NONE',  ( -17.40861289039001747, -6.110651285853280434, 51.37232470827432707 ) ) ;
#41789=CARTESIAN_POINT ( 'NONE',  ( -13.89961937509957401, -13.97604488694547875, 49.37609039468567573 ) ) ;
#41791=CARTESIAN_POINT ( 'NONE',  ( -19.02544592524342804, 5.153800228976336051, 106.0405762719810241 ) ) ;
#41792=CARTESIAN_POINT ( 'NONE',  ( -8.224510206698735004, -14.34966873604973081, 104.5844237280190185 ) ) ;
#41794=CARTESIAN_POINT ( 'NONE',  ( 4.483927247898790824, -16.52544592524335698, 95.20942372801903275 ) ) ;
#41795=CYLINDRICAL_SURFACE ( 'NONE', #77586, 2.000000000000001776 ) ;
#41796=CARTESIAN_POINT ( 'NONE',  ( -4.379528057220086978, -16.55341960407618274, 69.79275706135234714 ) ) ;
#41798=CARTESIAN_POINT ( 'NONE',  ( -5.823673210054431948, 21.52544592524334988, 67.70942372801901854 ) ) ;
#41799=CARTESIAN_POINT ( 'NONE',  ( 13.97604488694548053, -13.89961937509957401, 90.62609039468567573 ) ) ;
#41800=CARTESIAN_POINT ( 'NONE',  ( -9.474510206698720793, -16.51473224551083518, 24.58442372801900078 ) ) ;
#41801=CARTESIAN_POINT ( 'NONE',  ( -5.049401038298153566, 19.05341960407611168, 60.20724293864768129 ) ) ;
#41802=CARTESIAN_POINT ( 'NONE',  ( 19.02544592524343514, -5.153800228976328945, 43.54057627198103120 ) ) ;
#41804=CARTESIAN_POINT ( 'NONE',  ( 5.719274019375991003, -21.55341960407610458, 82.70724293864770971 ) ) ;
#41805=CARTESIAN_POINT ( 'NONE',  ( -5.719274019375978568, 21.55341960407610458, 30.20724293864769550 ) ) ;
#41806=CARTESIAN_POINT ( 'NONE',  ( -9.564922557960796823, -16.46253265017161027, 37.08224293864768839 ) ) ;
#41807=CARTESIAN_POINT ( 'NONE',  ( -4.483927247898782831, 16.52544592524335698, 52.70942372801902565 ) ) ;
#41809=CARTESIAN_POINT ( 'NONE',  ( -15.80617190586768217, 15.72974639402176855, 33.12609039468569705 ) ) ;
#41810=CARTESIAN_POINT ( 'NONE',  ( 14.29746914071049879, -8.314922557960816363, 53.33224293864769550 ) ) ;
#41812=CARTESIAN_POINT ( 'NONE',  ( 12.14591786802327356, -12.06949235617739191, 25.62609039468567929 ) ) ;
#41813=CARTESIAN_POINT ( 'NONE',  ( -19.05341960407617563, 5.049401038297882671, 33.54275706135231871 ) ) ;
#41814=CARTESIAN_POINT ( 'NONE',  ( 0.05219959533910956823, 16.53943276465976808, 54.99890960531435269 ) ) ;
#41815=CARTESIAN_POINT ( 'NONE',  ( -18.67979575497178146, -10.72451020669898902, 111.6655762719810525 ) ) ;
#41817=CARTESIAN_POINT ( 'NONE',  ( 21.52544592524344225, -5.823673210054117533, 78.54057627198103830 ) ) ;
#41818=CARTESIAN_POINT ( 'NONE',  ( -16.51473224551069308, -9.474510206698971260, 86.66557627198102409 ) ) ;
#41819=CARTESIAN_POINT ( 'NONE',  ( -8.314922557960811034, -14.29746914071050412, 57.08224293864769550 ) ) ;
#41820=CARTESIAN_POINT ( 'NONE',  ( -19.03943276465977164, 0.05219959533909376836, 106.2489096053143669 ) ) ;
#41823=CARTESIAN_POINT ( 'NONE',  ( -9.564922557961040184, 16.46253265017147172, 62.91775706135233293 ) ) ;
#41824=CARTESIAN_POINT ( 'NONE',  ( 18.62759615963271287, -10.81492255796078972, 108.3322429386477097 ) ) ;
#41825=CARTESIAN_POINT ( 'NONE',  ( 13.89961937509977652, -13.97604488694527269, 53.12390960531434558 ) ) ;
#41826=CARTESIAN_POINT ( 'NONE',  ( 5.049401038297881783, 19.05341960407617563, 47.29275706135231161 ) ) ;
#41827=CARTESIAN_POINT ( 'NONE',  ( -19.05341960407611168, -5.049401038298163336, 21.45724293864768839 ) ) ;
#41828=CARTESIAN_POINT ( 'NONE',  ( -15.72974639402176322, -15.80617190586768395, 59.37609039468568284 ) ) ;
#41829=CARTESIAN_POINT ( 'NONE',  ( -17.48853670773247515, -5.747243402303015003, 71.33328700250007159 ) ) ;
#41830=CARTESIAN_POINT ( 'NONE',  ( -8.314922557960811034, -14.29746914071050412, 37.08224293864768129 ) ) ;
#41831=CARTESIAN_POINT ( 'NONE',  ( 5.153800228976335163, 19.02544592524342804, 54.79057627198103120 ) ) ;
#41832=CARTESIAN_POINT ( 'NONE',  ( -18.62759615963270932, 10.81492255796079327, 75.83224293864769550 ) ) ;
#41834=CARTESIAN_POINT ( 'NONE',  ( -5.049401038298153566, 19.05341960407611168, 40.20724293864768839 ) ) ;
#41836=CARTESIAN_POINT ( 'NONE',  ( -5.823673210054116645, -21.52544592524344225, 72.29057627198102409 ) ) ;
#41838=CARTESIAN_POINT ( 'NONE',  ( -10.81492255796105439, 18.62759615963255655, 82.91775706135234714 ) ) ;
#41840=CARTESIAN_POINT ( 'NONE',  ( 8.224510206698742110, 14.34966873604972548, 97.08442372801904696 ) ) ;
#41841=CARTESIAN_POINT ( 'NONE',  ( 8.224510206698953496, -14.34966873604960469, 82.91557627198103830 ) ) ;
#41843=CARTESIAN_POINT ( 'NONE',  ( -9.564922557960796823, -16.46253265017161027, 72.08224293864770971 ) ) ;
#41845=CARTESIAN_POINT ( 'NONE',  ( 13.97604488694548053, -13.89961937509957401, 45.62609039468566863 ) ) ;
#41846=CARTESIAN_POINT ( 'NONE',  ( -4.483927247898782831, 16.52544592524335698, 82.70942372801900433 ) ) ;
#41847=CARTESIAN_POINT ( 'NONE',  ( 5.049401038297881783, 19.05341960407617563, 22.29275706135233648 ) ) ;
#41848=CARTESIAN_POINT ( 'NONE',  ( 13.89961937509977652, -13.97604488694527269, 88.12390960531438111 ) ) ;
#41849=CARTESIAN_POINT ( 'NONE',  ( -21.52544592524343514, 5.823673210054127303, 51.04057627198103120 ) ) ;
#41851=CARTESIAN_POINT ( 'NONE',  ( -16.46253265017160317, 9.564922557960807481, 25.83224293864769194 ) ) ;
#41852=CARTESIAN_POINT ( 'NONE',  ( 5.719274019375673035, 21.55341960407619339, 102.2927570613523613 ) ) ;
#41853=CARTESIAN_POINT ( 'NONE',  ( -4.379528057220086978, -16.55341960407618274, 59.79275706135234714 ) ) ;
#41854=CARTESIAN_POINT ( 'NONE',  ( 21.53943276465977519, 0.05219959533937863772, 21.25109039468567218 ) ) ;
#41855=CARTESIAN_POINT ( 'NONE',  ( 4.379528057220092307, 16.55341960407617563, 27.29275706135234358 ) ) ;
#41856=CARTESIAN_POINT ( 'NONE',  ( 0.05219959533909260263, 19.03943276465977164, 89.99890960531436690 ) ) ;
#41857=CARTESIAN_POINT ( 'NONE',  ( 13.89961937509977652, -13.97604488694527269, 38.12390960531436690 ) ) ;
#41858=CARTESIAN_POINT ( 'NONE',  ( 13.97604488694527802, 13.89961937509977652, 54.37390960531435979 ) ) ;
#41860=CARTESIAN_POINT ( 'NONE',  ( -12.06949235617739369, -12.14591786802326823, 29.37609039468568284 ) ) ;
#41861=CARTESIAN_POINT ( 'NONE',  ( 16.55341960407611168, 4.379528057220329451, 88.95724293864769550 ) ) ;
#41862=CARTESIAN_POINT ( 'NONE',  ( -4.379528057220086978, -16.55341960407618274, 99.79275706135234714 ) ) ;
#41863=CARTESIAN_POINT ( 'NONE',  ( -21.53943276465977519, -0.05219959533937600094, 48.75109039468568284 ) ) ;
#41864=CARTESIAN_POINT ( 'NONE',  ( -19.03943276465977164, 0.05219959533909376836, 61.24890960531436690 ) ) ;
#41865=CARTESIAN_POINT ( 'NONE',  ( -16.51473224551069308, -9.474510206698971260, 51.66557627198102409 ) ) ;
#41866=CARTESIAN_POINT ( 'NONE',  ( 9.474510206698971260, -16.51473224551069308, 82.91557627198103830 ) ) ;
#41867=CARTESIAN_POINT ( 'NONE',  ( -8.224510206698948167, 14.34966873604960824, 35.41557627198102409 ) ) ;
#41868=CARTESIAN_POINT ( 'NONE',  ( 8.314922557961029526, -14.29746914071037800, 105.4177570613523613 ) ) ;
#41870=CARTESIAN_POINT ( 'NONE',  ( -16.51473224551082808, 9.474510206698731452, 28.33442372801900433 ) ) ;
#41871=CARTESIAN_POINT ( 'NONE',  ( 19.02544592524343514, -5.153800228976328945, 108.5405762719810383 ) ) ;
#41872=CARTESIAN_POINT ( 'NONE',  ( 9.564922557960805705, 16.46253265017160317, 54.58224293864769550 ) ) ;
#41873=CARTESIAN_POINT ( 'NONE',  ( -19.05341960407617563, 5.049401038297882671, 28.54275706135232937 ) ) ;
#41875=CARTESIAN_POINT ( 'NONE',  ( -16.55341960407617563, 4.379528057220093196, 48.54275706135234714 ) ) ;
#41876=CARTESIAN_POINT ( 'NONE',  ( -19.05341960407617563, 5.049401038297882671, 68.54275706135230450 ) ) ;
#41877=CARTESIAN_POINT ( 'NONE',  ( 0.05219959533934541429, -16.53943276465976808, 50.00109039468568994 ) ) ;
#41879=CARTESIAN_POINT ( 'NONE',  ( 13.89961937509977652, -13.97604488694527269, 73.12390960531436690 ) ) ;
#41880=CARTESIAN_POINT ( 'NONE',  ( -18.62759615963270932, 10.81492255796079327, 110.8322429386476955 ) ) ;
#41881=CARTESIAN_POINT ( 'NONE',  ( 19.05341960407617918, -5.049401038297876454, 66.04275706135233293 ) ) ;
#41882=CARTESIAN_POINT ( 'NONE',  ( 19.02544592524343514, -5.153800228976328945, 108.5405762719810383 ) ) ;
#41883=CARTESIAN_POINT ( 'NONE',  ( -19.02544592524342804, 5.153800228976336051, 36.04057627198100988 ) ) ;
#41884=CARTESIAN_POINT ( 'NONE',  ( 19.03943276465977164, -0.05219959533909143690, 73.74890960531435269 ) ) ;
#41885=CARTESIAN_POINT ( 'NONE',  ( -14.34966873604960291, -8.224510206698953496, 36.66557627198103120 ) ) ;
#41886=CARTESIAN_POINT ( 'NONE',  ( -13.89961937509977652, 13.97604488694528158, 40.62390960531435979 ) ) ;
#41887=CARTESIAN_POINT ( 'NONE',  ( -13.89961937509957401, -13.97604488694547875, 44.37609039468566863 ) ) ;
#41888=CARTESIAN_POINT ( 'NONE',  ( -8.314922557960811034, -14.29746914071050412, 77.08224293864769550 ) ) ;
#41889=CARTESIAN_POINT ( 'NONE',  ( 5.719274019375673035, 21.55341960407619339, 112.2927570613523471 ) ) ;
#41890=CARTESIAN_POINT ( 'NONE',  ( 19.03943276465977164, -0.05219959533909143690, 58.74890960531435979 ) ) ;
#41892=CARTESIAN_POINT ( 'NONE',  ( 15.72974639402199770, -15.80617190586745480, 48.12390960531436690 ) ) ;
#41893=CARTESIAN_POINT ( 'NONE',  ( -8.224510206698948167, 14.34966873604960824, 50.41557627198103120 ) ) ;
#41894=CARTESIAN_POINT ( 'NONE',  ( -10.72451020669870658, -18.67979575497194134, 99.58442372801900433 ) ) ;
#41895=CARTESIAN_POINT ( 'NONE',  ( -13.89961937509977652, 13.97604488694528158, 95.62390960531436690 ) ) ;
#41896=CARTESIAN_POINT ( 'NONE',  ( 9.564922557960805705, 16.46253265017160317, 104.5822429386476955 ) ) ;
#41897=CARTESIAN_POINT ( 'NONE',  ( -9.474510206698964154, 16.51473224551069663, 45.41557627198103120 ) ) ;
#41898=CARTESIAN_POINT ( 'NONE',  ( 19.02544592524343514, -5.153800228976328945, 28.54057627198102409 ) ) ;
#41899=CARTESIAN_POINT ( 'NONE',  ( 16.52544592524342804, -4.483927247898539470, 93.54057627198103830 ) ) ;
#41900=CARTESIAN_POINT ( 'NONE',  ( 18.62759615963271287, -10.81492255796078972, 98.33224293864769550 ) ) ;
#41901=CARTESIAN_POINT ( 'NONE',  ( -9.564922557960796823, -16.46253265017161027, 82.08224293864768129 ) ) ;
#41902=CARTESIAN_POINT ( 'NONE',  ( 21.55341960407610458, 5.719274019375980345, 98.95724293864770971 ) ) ;
#41903=CARTESIAN_POINT ( 'NONE',  ( -16.46253265017160317, 9.564922557960807481, 95.83224293864769550 ) ) ;
#41905=CARTESIAN_POINT ( 'NONE',  ( -12.06949235617756955, 12.14591786802309770, 105.6239096053143669 ) ) ;
#41906=CARTESIAN_POINT ( 'NONE',  ( 13.89961937509977652, -13.97604488694527269, 68.12390960531436690 ) ) ;
#41907=CARTESIAN_POINT ( 'NONE',  ( 0.05219959533907565091, 21.53943276465977519, 84.99890960531436690 ) ) ;
#41910=CARTESIAN_POINT ( 'NONE',  ( 21.53943276465977519, -0.05219959533907433946, 28.74890960531435624 ) ) ;
#41912=CARTESIAN_POINT ( 'NONE',  ( 16.52544592524335698, 4.483927247898782831, 36.45942372801901143 ) ) ;
#41913=CARTESIAN_POINT ( 'NONE',  ( -4.379528057220328563, 16.55341960407611168, 95.20724293864769550 ) ) ;
#41914=CARTESIAN_POINT ( 'NONE',  ( -16.21995358207304250, -7.366697692864176084, 95.06448998487844904 ) ) ;
#41915=CARTESIAN_POINT ( 'NONE',  ( 5.049401038298161559, -19.05341960407611168, 92.70724293864769550 ) ) ;
#41916=CARTESIAN_POINT ( 'NONE',  ( 19.02544592524343514, -5.153800228976328945, 48.54057627198103120 ) ) ;
#41917=CARTESIAN_POINT ( 'NONE',  ( -14.29746914071049879, 8.314922557960819915, 80.83224293864769550 ) ) ;
#41918=CARTESIAN_POINT ( 'NONE',  ( -10.81492255796078084, -18.62759615963271287, 32.08224293864769550 ) ) ;
#41919=CARTESIAN_POINT ( 'NONE',  ( 16.52544592524342804, -4.483927247898539470, 48.54057627198103120 ) ) ;
#41920=CARTESIAN_POINT ( 'NONE',  ( -5.153800228976607833, 19.02544592524334988, 102.7094237280189759 ) ) ;
#41921=CARTESIAN_POINT ( 'NONE',  ( 0.05219959533937995610, -21.53943276465977519, 65.00109039468568994 ) ) ;
#41923=CARTESIAN_POINT ( 'NONE',  ( 5.153800228976335163, 19.02544592524342804, 94.79057627198103830 ) ) ;
#41924=CARTESIAN_POINT ( 'NONE',  ( 8.314922557961029526, -14.29746914071037800, 85.41775706135236135 ) ) ;
#41925=CARTESIAN_POINT ( 'NONE',  ( -19.03943276465977164, 0.05219959533909376836, 26.24890960531435624 ) ) ;
#41926=CARTESIAN_POINT ( 'NONE',  ( 13.97604488694527802, 13.89961937509977652, 79.37390960531435269 ) ) ;
#41927=CARTESIAN_POINT ( 'NONE',  ( -10.72451020669898014, 18.67979575497178502, 75.41557627198102409 ) ) ;
#41928=CARTESIAN_POINT ( 'NONE',  ( 14.29746914071037800, 8.314922557961029526, 21.66775706135235069 ) ) ;
#41929=CARTESIAN_POINT ( 'NONE',  ( -16.52544592524342804, 4.483927247898546575, 51.04057627198103120 ) ) ;
#41930=CARTESIAN_POINT ( 'NONE',  ( -5.823673210054431948, 21.52544592524334988, 62.70942372801902565 ) ) ;
#41931=CARTESIAN_POINT ( 'NONE',  ( 4.379528057220092307, 16.55341960407617563, 82.29275706135234714 ) ) ;
#41932=CARTESIAN_POINT ( 'NONE',  ( 18.62759615963271287, -10.81492255796078972, 23.33224293864769194 ) ) ;
#41933=CARTESIAN_POINT ( 'NONE',  ( 16.88567814943164791, 6.947325034625595030, 28.79001122652586631 ) ) ;
#41935=CARTESIAN_POINT ( 'NONE',  ( -12.06949235617739369, -12.14591786802326823, 109.3760903946857042 ) ) ;
#41936=CARTESIAN_POINT ( 'NONE',  ( 16.55341960407618274, -4.379528057220086978, 66.04275706135236135 ) ) ;
#41937=CARTESIAN_POINT ( 'NONE',  ( 0.05219959533909260263, 19.03943276465977164, 74.99890960531435269 ) ) ;
#41938=CARTESIAN_POINT ( 'NONE',  ( 9.474510206698971260, -16.51473224551069308, 92.91557627198103830 ) ) ;
#41939=CARTESIAN_POINT ( 'NONE',  ( 10.81492255796106328, -18.62759615963255655, 75.41775706135233293 ) ) ;
#41940=CARTESIAN_POINT ( 'NONE',  ( 14.34966873604972726, -8.224510206698740333, 75.83442372801900433 ) ) ;
#41941=CARTESIAN_POINT ( 'NONE',  ( -8.224510206698948167, 14.34966873604960824, 45.41557627198103830 ) ) ;
#41942=CARTESIAN_POINT ( 'NONE',  ( 13.97604488694527802, 13.89961937509977652, 59.37390960531434558 ) ) ;
#41943=CARTESIAN_POINT ( 'NONE',  ( -5.049401038298153566, 19.05341960407611168, 50.20724293864770260 ) ) ;
#41944=CARTESIAN_POINT ( 'NONE',  ( 16.52544592524335698, 4.483927247898782831, 36.45942372801901143 ) ) ;
#41945=ORIENTED_EDGE ( 'NONE', *, *, #58944, .T. ) ;
#41946=CARTESIAN_POINT ( 'NONE',  ( 19.03943276465977164, 0.05219959533936151252, 96.25109039468567573 ) ) ;
#41947=CARTESIAN_POINT ( 'NONE',  ( -4.483927247898539470, -16.52544592524342804, 97.29057627198105251 ) ) ;
#41948=CARTESIAN_POINT ( 'NONE',  ( 16.46253265017160672, -9.564922557960803928, 63.33224293864769550 ) ) ;
#41949=CARTESIAN_POINT ( 'NONE',  ( -13.89961937509957401, -13.97604488694547875, 104.3760903946856757 ) ) ;
#41951=CARTESIAN_POINT ( 'NONE',  ( 0.05219959533937995610, -21.53943276465977519, 110.0010903946856757 ) ) ;
#41952=CARTESIAN_POINT ( 'NONE',  ( -12.14591786802326823, 12.06949235617739902, 73.12609039468567573 ) ) ;
#41954=CARTESIAN_POINT ( 'NONE',  ( 5.719274019375991003, -21.55341960407610458, 62.70724293864769550 ) ) ;
#41955=CARTESIAN_POINT ( 'NONE',  ( 8.224510206698742110, 14.34966873604972548, 57.08442372801901854 ) ) ;
#41957=CARTESIAN_POINT ( 'NONE',  ( 5.049401038297881783, 19.05341960407617563, 62.29275706135234003 ) ) ;
#41958=CARTESIAN_POINT ( 'NONE',  ( 16.51473224551069308, 9.474510206698969483, 94.16557627198103830 ) ) ;
#41959=CARTESIAN_POINT ( 'NONE',  ( 0.05219959533910956823, 16.53943276465976808, 109.9989096053143527 ) ) ;
#41960=CARTESIAN_POINT ( 'NONE',  ( 16.46253265017160672, -9.564922557960803928, 63.33224293864769550 ) ) ;
#41961=CARTESIAN_POINT ( 'NONE',  ( 14.29746914071049879, -8.314922557960816363, 53.33224293864769550 ) ) ;
#41962=CARTESIAN_POINT ( 'NONE',  ( 18.62759615963255655, 10.81492255796105972, 81.66775706135236135 ) ) ;
#41963=CARTESIAN_POINT ( 'NONE',  ( -13.89961937509957401, -13.97604488694547875, 44.37609039468566863 ) ) ;
#41964=CARTESIAN_POINT ( 'NONE',  ( -5.049401038297874678, -19.05341960407617918, 34.79275706135233293 ) ) ;
#41965=CARTESIAN_POINT ( 'NONE',  ( -18.67979575497178146, -10.72451020669898902, 26.66557627198103475 ) ) ;
#41966=CARTESIAN_POINT ( 'NONE',  ( -5.719274019375665041, -21.55341960407619695, 94.79275706135234714 ) ) ;
#41967=CARTESIAN_POINT ( 'NONE',  ( -19.05341960407611168, -5.049401038298163336, 66.45724293864769550 ) ) ;
#41968=CARTESIAN_POINT ( 'NONE',  ( -15.80617190586768217, 15.72974639402176855, 98.12609039468570415 ) ) ;
#41969=CARTESIAN_POINT ( 'NONE',  ( -18.62759615963270932, 10.81492255796079327, 50.83224293864770971 ) ) ;
#41970=CARTESIAN_POINT ( 'NONE',  ( -19.03943276465977164, 0.05219959533909376836, 86.24890960531436690 ) ) ;
#41971=CARTESIAN_POINT ( 'NONE',  ( -9.564922557961040184, 16.46253265017147172, 57.91775706135233293 ) ) ;
#41972=CARTESIAN_POINT ( 'NONE',  ( 16.51473224551069308, 9.474510206698969483, 39.16557627198103120 ) ) ;
#41973=CARTESIAN_POINT ( 'NONE',  ( -5.153800228976328057, -19.02544592524343514, 92.29057627198099567 ) ) ;
#41974=CARTESIAN_POINT ( 'NONE',  ( -13.97604488694547697, 13.89961937509957934, 88.12609039468563310 ) ) ;
#41975=CARTESIAN_POINT ( 'NONE',  ( -16.52544592524335698, -4.483927247898792601, 33.95942372801901143 ) ) ;
#41976=CARTESIAN_POINT ( 'NONE',  ( 16.55341960407611168, 4.379528057220329451, 98.95724293864770971 ) ) ;
#41977=CARTESIAN_POINT ( 'NONE',  ( -19.05341960407611168, -5.049401038298163336, 66.45724293864769550 ) ) ;
#41978=CARTESIAN_POINT ( 'NONE',  ( 0.05219959533907565091, 21.53943276465977519, 49.99890960531437401 ) ) ;
#41980=CARTESIAN_POINT ( 'NONE',  ( -5.049401038297874678, -19.05341960407617918, 109.7927570613523187 ) ) ;
#41981=CARTESIAN_POINT ( 'NONE',  ( 21.55341960407610458, 5.719274019375980345, 113.9572429386477239 ) ) ;
#41982=CARTESIAN_POINT ( 'NONE',  ( 21.52544592524334988, 5.823673210054432836, 66.45942372801903275 ) ) ;
#41983=CARTESIAN_POINT ( 'NONE',  ( 16.53943276465976808, 0.05219959533934440121, 71.25109039468568994 ) ) ;
#41984=CARTESIAN_POINT ( 'NONE',  ( -19.02544592524342804, 5.153800228976336051, 71.04057627198099567 ) ) ;
#41985=CARTESIAN_POINT ( 'NONE',  ( -4.379528057220086978, -16.55341960407618274, 99.79275706135234714 ) ) ;
#41986=CARTESIAN_POINT ( 'NONE',  ( -9.564922557961040184, 16.46253265017147172, 42.91775706135234003 ) ) ;
#41987=CARTESIAN_POINT ( 'NONE',  ( 5.823673210054444382, -21.52544592524334988, 30.20942372801902565 ) ) ;
#41988=CARTESIAN_POINT ( 'NONE',  ( 12.06949235617757843, -12.14591786802309237, 73.12390960531436690 ) ) ;
#41989=CARTESIAN_POINT ( 'NONE',  ( -13.89961937509977652, 13.97604488694528158, 100.6239096053143669 ) ) ;
#41990=CARTESIAN_POINT ( 'NONE',  ( -0.05219959533934338120, 16.53943276465976808, 87.50109039468568994 ) ) ;
#41991=CARTESIAN_POINT ( 'NONE',  ( 5.719274019375673035, 21.55341960407619339, 67.29275706135234714 ) ) ;
#41992=CARTESIAN_POINT ( 'NONE',  ( -12.14591786802326823, 12.06949235617739902, 28.12609039468568284 ) ) ;
#41993=CARTESIAN_POINT ( 'NONE',  ( 15.80617190586769283, -15.72974639402175789, 25.62609039468567929 ) ) ;
#41994=CARTESIAN_POINT ( 'NONE',  ( 8.314922557960818139, 14.29746914071049879, 69.58224293864769550 ) ) ;
#41996=CARTESIAN_POINT ( 'NONE',  ( 10.81492255796078972, 18.62759615963270932, 94.58224293864769550 ) ) ;
#41997=CARTESIAN_POINT ( 'NONE',  ( -16.53943276465976808, 0.05219959533911058130, 56.24890960531436690 ) ) ;
#41999=CARTESIAN_POINT ( 'NONE',  ( -5.049401038298153566, 19.05341960407611168, 25.20724293864768484 ) ) ;
#42000=CARTESIAN_POINT ( 'NONE',  ( -10.72451020669898014, 18.67979575497178502, 30.41557627198101699 ) ) ;
#42001=CARTESIAN_POINT ( 'NONE',  ( -18.62759615963255300, -10.81492255796106328, 39.16775706135235424 ) ) ;
#42002=CARTESIAN_POINT ( 'NONE',  ( 16.52544592524342804, -4.483927247898539470, 63.54057627198103830 ) ) ;
#42003=AXIS2_PLACEMENT_3D ( 'NONE', #143837, #37662, #191344 ) ;
#42004=CARTESIAN_POINT ( 'NONE',  ( -10.72451020669898014, 18.67979575497178502, 70.41557627198102409 ) ) ;
#42005=CARTESIAN_POINT ( 'NONE',  ( 9.474510206698971260, -16.51473224551069308, 77.91557627198103830 ) ) ;
#42006=CARTESIAN_POINT ( 'NONE',  ( -19.02544592524342804, 5.153800228976336051, 31.04057627198102409 ) ) ;
#42007=CARTESIAN_POINT ( 'NONE',  ( -9.474510206698720793, -16.51473224551083518, 84.58442372801900433 ) ) ;
#42008=CARTESIAN_POINT ( 'NONE',  ( 18.62759615963271287, -10.81492255796078972, 53.33224293864769550 ) ) ;
#42009=CARTESIAN_POINT ( 'NONE',  ( 5.153800228976335163, 19.02544592524342804, 34.79057627198102409 ) ) ;
#42010=CARTESIAN_POINT ( 'NONE',  ( 13.89961937509977652, -13.97604488694527269, 73.12390960531436690 ) ) ;
#42012=CARTESIAN_POINT ( 'NONE',  ( 8.224510206698742110, 14.34966873604972548, 32.08442372801901854 ) ) ;
#42013=CARTESIAN_POINT ( 'NONE',  ( -18.62759615963255300, -10.81492255796106328, 29.16775706135234003 ) ) ;
#42014=CARTESIAN_POINT ( 'NONE',  ( 21.52544592524334988, 5.823673210054432836, 56.45942372801902565 ) ) ;
#42015=CARTESIAN_POINT ( 'NONE',  ( 9.564922557960805705, 16.46253265017160317, 109.5822429386476955 ) ) ;
#42016=CARTESIAN_POINT ( 'NONE',  ( -18.67979575497178146, -10.72451020669898902, 66.66557627198102409 ) ) ;
#42017=CARTESIAN_POINT ( 'NONE',  ( 5.823673210054125526, 21.52544592524343514, 104.7905762719810241 ) ) ;
#42018=CARTESIAN_POINT ( 'NONE',  ( 12.14591786802327356, -12.06949235617739191, 45.62609039468567573 ) ) ;
#42019=CARTESIAN_POINT ( 'NONE',  ( -5.719274019375978568, 21.55341960407610458, 55.20724293864770260 ) ) ;
#42020=CARTESIAN_POINT ( 'NONE',  ( 5.823673210054444382, -21.52544592524334988, 100.2094237280190043 ) ) ;
#42021=CARTESIAN_POINT ( 'NONE',  ( -13.89961937509977652, 13.97604488694528158, 60.62390960531436690 ) ) ;
#42022=CARTESIAN_POINT ( 'NONE',  ( 13.97604488694527802, 13.89961937509977652, 104.3739096053143385 ) ) ;
#42023=CARTESIAN_POINT ( 'NONE',  ( -5.153800228976328057, -19.02544592524343514, 82.29057627198103830 ) ) ;
#42024=CARTESIAN_POINT ( 'NONE',  ( 16.19135201231354415, -7.376712067591904010, 87.31319145947881566 ) ) ;
#42026=CARTESIAN_POINT ( 'NONE',  ( 0.05219959533936267826, -19.03943276465977164, 65.00109039468567573 ) ) ;
#42027=CARTESIAN_POINT ( 'NONE',  ( 16.46253265017146816, 9.564922557961045513, 21.66775706135233648 ) ) ;
#42028=CARTESIAN_POINT ( 'NONE',  ( -18.62759615963270932, 10.81492255796079327, 40.83224293864769550 ) ) ;
#42029=CARTESIAN_POINT ( 'NONE',  ( -14.29746914071037622, -8.314922557961029526, 99.16775706135234714 ) ) ;
#42030=CARTESIAN_POINT ( 'NONE',  ( 0.05219959533936267826, -19.03943276465977164, 85.00109039468567573 ) ) ;
#42032=CARTESIAN_POINT ( 'NONE',  ( -19.05341960407617563, 5.049401038297882671, 23.54275706135233648 ) ) ;
#42033=CARTESIAN_POINT ( 'NONE',  ( 9.474510206698729675, 16.51473224551082808, 82.08442372801899012 ) ) ;
#42034=CARTESIAN_POINT ( 'NONE',  ( -9.564922557961040184, 16.46253265017147172, 42.91775706135234003 ) ) ;
#42035=CARTESIAN_POINT ( 'NONE',  ( 17.44270441346516876, 5.991230190323038940, 108.8633507926423363 ) ) ;
#42036=CARTESIAN_POINT ( 'NONE',  ( -0.05219959533909027116, -19.03943276465977164, 37.49890960531436690 ) ) ;
#42037=CARTESIAN_POINT ( 'NONE',  ( -4.483927247898539470, -16.52544592524342804, 47.29057627198103120 ) ) ;
#42038=CARTESIAN_POINT ( 'NONE',  ( 19.02544592524343514, -5.153800228976328945, 33.54057627198102409 ) ) ;
#42039=CARTESIAN_POINT ( 'NONE',  ( -16.55341960407611168, -4.379528057220339221, 41.45724293864769550 ) ) ;
#42041=CARTESIAN_POINT ( 'NONE',  ( 14.29746914071037800, 8.314922557961029526, 106.6677570613523756 ) ) ;
#42042=CARTESIAN_POINT ( 'NONE',  ( -13.89961937509977652, 13.97604488694528158, 55.62390960531434558 ) ) ;
#42043=CARTESIAN_POINT ( 'NONE',  ( 16.51473224551083163, -9.474510206698727899, 30.83442372801900433 ) ) ;
#42044=CARTESIAN_POINT ( 'NONE',  ( -16.53943276465976808, -0.05219959533934237506, 38.75109039468567573 ) ) ;
#42045=CARTESIAN_POINT ( 'NONE',  ( 15.72974639402199770, -15.80617190586745480, 43.12390960531435269 ) ) ;
#42046=CARTESIAN_POINT ( 'NONE',  ( -10.72451020669870658, -18.67979575497194134, 89.58442372801901854 ) ) ;
#42048=CARTESIAN_POINT ( 'NONE',  ( 19.02544592524343514, -5.153800228976328945, 103.5405762719809957 ) ) ;
#42049=CARTESIAN_POINT ( 'NONE',  ( 9.474510206698971260, -16.51473224551069308, 87.91557627198102409 ) ) ;
#42051=CARTESIAN_POINT ( 'NONE',  ( 21.52544592524344225, -5.823673210054117533, 103.5405762719810383 ) ) ;
#42052=CARTESIAN_POINT ( 'NONE',  ( -4.379528057220328563, 16.55341960407611168, 80.20724293864769550 ) ) ;
#42053=CARTESIAN_POINT ( 'NONE',  ( -21.52544592524343514, 5.823673210054127303, 81.04057627198102409 ) ) ;
#42054=CARTESIAN_POINT ( 'NONE',  ( 19.02544592524343514, -5.153800228976328945, 73.54057627198103830 ) ) ;
#42055=CARTESIAN_POINT ( 'NONE',  ( 5.049401038298161559, -19.05341960407611168, 72.70724293864768129 ) ) ;
#42056=CARTESIAN_POINT ( 'NONE',  ( 15.80617190586746368, 15.72974639402197994, 94.37390960531436690 ) ) ;
#42058=CARTESIAN_POINT ( 'NONE',  ( 0.05219959533909260263, 19.03943276465977164, 54.99890960531435979 ) ) ;
#42059=CARTESIAN_POINT ( 'NONE',  ( -16.55341960407611168, -4.379528057220339221, 96.45724293864770971 ) ) ;
#42061=CARTESIAN_POINT ( 'NONE',  ( -5.049401038298153566, 19.05341960407611168, 65.20724293864765286 ) ) ;
#42062=CARTESIAN_POINT ( 'NONE',  ( -16.51473224551082808, 9.474510206698731452, 78.33442372801900433 ) ) ;
#42063=CARTESIAN_POINT ( 'NONE',  ( -0.05219959533910754901, -16.53943276465976808, 92.49890960531436690 ) ) ;
#42064=CARTESIAN_POINT ( 'NONE',  ( 10.72451020669871369, 18.67979575497193778, 57.08442372801901854 ) ) ;
#42065=CARTESIAN_POINT ( 'NONE',  ( 5.153800228976335163, 19.02544592524342804, 44.79057627198103830 ) ) ;
#42066=CARTESIAN_POINT ( 'NONE',  ( 10.72451020669871369, 18.67979575497193778, 22.08442372801901143 ) ) ;
#42067=CARTESIAN_POINT ( 'NONE',  ( 12.06949235617757843, -12.14591786802309237, 103.1239096053143811 ) ) ;
#42069=CARTESIAN_POINT ( 'NONE',  ( 19.05341960407611168, 5.049401038298154454, 68.95724293864769550 ) ) ;
#42070=CARTESIAN_POINT ( 'NONE',  ( 17.31728774477275579, 6.344390552232371583, 111.6809334831068270 ) ) ;
#42071=CARTESIAN_POINT ( 'NONE',  ( 16.46253265017146816, 9.564922557961045513, 111.6677570613523329 ) ) ;
#42072=CARTESIAN_POINT ( 'NONE',  ( -0.05219959533909027116, -19.03943276465977164, 107.4989096053143527 ) ) ;
#42073=CARTESIAN_POINT ( 'NONE',  ( 21.52544592524334988, 5.823673210054432836, 46.45942372801901854 ) ) ;
#42074=CARTESIAN_POINT ( 'NONE',  ( -0.05219959533909027116, -19.03943276465977164, 92.49890960531436690 ) ) ;
#42075=CARTESIAN_POINT ( 'NONE',  ( -13.97604488694547697, 13.89961937509957934, 83.12609039468564731 ) ) ;
#42076=CARTESIAN_POINT ( 'NONE',  ( -5.049401038298153566, 19.05341960407611168, 65.20724293864765286 ) ) ;
#42077=CARTESIAN_POINT ( 'NONE',  ( -14.34966873604960291, -8.224510206698953496, 81.66557627198103830 ) ) ;
#42078=CARTESIAN_POINT ( 'NONE',  ( -19.03943276465977164, 0.05219959533909376836, 101.2489096053143669 ) ) ;
#42079=CARTESIAN_POINT ( 'NONE',  ( -12.14591786802309592, -12.06949235617757132, 76.87390960531439532 ) ) ;
#42080=CARTESIAN_POINT ( 'NONE',  ( 5.153800228976335163, 19.02544592524342804, 104.7905762719809957 ) ) ;
#42081=CARTESIAN_POINT ( 'NONE',  ( -19.05341960407617563, 5.049401038297882671, 48.54275706135233293 ) ) ;
#42082=CARTESIAN_POINT ( 'NONE',  ( 9.564922557960805705, 16.46253265017160317, 44.58224293864769550 ) ) ;
#42083=CARTESIAN_POINT ( 'NONE',  ( -0.05219959533910754901, -16.53943276465976808, 42.49890960531435979 ) ) ;
#42084=CARTESIAN_POINT ( 'NONE',  ( 9.564922557960805705, 16.46253265017160317, 24.58224293864769194 ) ) ;
#42085=ORIENTED_EDGE ( 'NONE', *, *, #164773, .F. ) ;
#42086=CARTESIAN_POINT ( 'NONE',  ( 18.62759615963255655, 10.81492255796105972, 46.66775706135234714 ) ) ;
#42087=CARTESIAN_POINT ( 'NONE',  ( -0.05219959533936034679, 19.03943276465977164, 82.50109039468567573 ) ) ;
#42088=CARTESIAN_POINT ( 'NONE',  ( 14.34966873604960469, 8.224510206698951720, 34.16557627198102409 ) ) ;
#42089=CARTESIAN_POINT ( 'NONE',  ( 18.67979575497178502, 10.72451020669898547, 94.16557627198103830 ) ) ;
#42090=CARTESIAN_POINT ( 'NONE',  ( -5.719274019375978568, 21.55341960407610458, 40.20724293864769550 ) ) ;
#42091=CARTESIAN_POINT ( 'NONE',  ( 14.34966873604960469, 8.224510206698951720, 79.16557627198103830 ) ) ;
#42092=CARTESIAN_POINT ( 'NONE',  ( -13.97604488694527625, -13.89961937509977652, 36.87390960531436690 ) ) ;
#42093=CARTESIAN_POINT ( 'NONE',  ( -16.53943276465976808, -0.05219959533934237506, 108.7510903946857042 ) ) ;
#42094=CARTESIAN_POINT ( 'NONE',  ( -12.06949235617739369, -12.14591786802326823, 69.37609039468567573 ) ) ;
#42095=CARTESIAN_POINT ( 'NONE',  ( -13.89961937509957401, -13.97604488694547875, 24.37609039468565442 ) ) ;
#42096=CARTESIAN_POINT ( 'NONE',  ( 9.474510206698971260, -16.51473224551069308, 92.91557627198103830 ) ) ;
#42097=CARTESIAN_POINT ( 'NONE',  ( 13.89961937509977652, -13.97604488694527269, 73.12390960531436690 ) ) ;
#42098=CARTESIAN_POINT ( 'NONE',  ( -16.53943276465976808, -0.05219959533934237506, 78.75109039468568994 ) ) ;
#42099=CARTESIAN_POINT ( 'NONE',  ( -0.05219959533909027116, -19.03943276465977164, 32.49890960531435979 ) ) ;
#42101=CARTESIAN_POINT ( 'NONE',  ( 8.224510206698953496, -14.34966873604960469, 52.91557627198103830 ) ) ;
#42102=CARTESIAN_POINT ( 'NONE',  ( -16.46253265017160317, 9.564922557960807481, 115.8322429386477097 ) ) ;
#42103=CARTESIAN_POINT ( 'NONE',  ( -19.02544592524342804, 5.153800228976336051, 86.04057627198103830 ) ) ;
#42104=CARTESIAN_POINT ( 'NONE',  ( 5.719274019375991003, -21.55341960407610458, 27.70724293864769905 ) ) ;
#42105=CARTESIAN_POINT ( 'NONE',  ( 16.52544592524342804, -4.483927247898539470, 78.54057627198103830 ) ) ;
#42106=B_SPLINE_CURVE_WITH_KNOTS ( 'NONE', 3,
 ( #138987, #123804, #185502, #156149, #46993, #108652, #170330, #32817, #17647, #140976, #2464, #64146, #125810, #191461, #68113, #21618, #129765, #117627, #145951, #178314, #9463, #36770, #194479, #52939, #39777, #98434, #160130, #163132, #24635, #114613, #176312, #55951 ),
 .UNSPECIFIED., .F., .F.,
 ( 4, 2, 2, 2, 2, 2, 2, 2, 2, 2, 2, 2, 2, 2, 2, 4 ),
 ( 2.625112965618923374E-17, 0.0003712461730037037999, 0.0007424923460073813621, 0.001113738519011058924, 0.001484984692014736487, 0.002227477038022089659, 0.002598723211025752260, 0.002969969384029414426, 0.003341215557033077026, 0.003712461730036739193, 0.004083707903040401793, 0.004454954076044063092, 0.004826200249047726126, 0.005197446422051388293, 0.005568692595055050459, 0.005939938768058712626 ),
 .UNSPECIFIED. ) ;
#42108=CARTESIAN_POINT ( 'NONE',  ( -8.224510206698948167, 14.34966873604960824, 60.41557627198102409 ) ) ;
#42109=CARTESIAN_POINT ( 'NONE',  ( -8.224510206698735004, -14.34966873604973081, 49.58442372801901143 ) ) ;
#42110=CARTESIAN_POINT ( 'NONE',  ( 17.97182807773871360, -5.500000000000039080, 86.03038844047287625 ) ) ;
#42111=CARTESIAN_POINT ( 'NONE',  ( -9.474510206698720793, -16.51473224551083518, 69.58442372801901854 ) ) ;
#42112=CARTESIAN_POINT ( 'NONE',  ( -16.51473224551069308, -9.474510206698971260, 86.66557627198102409 ) ) ;
#42113=CARTESIAN_POINT ( 'NONE',  ( -13.89961937509957401, -13.97604488694547875, 64.37609039468567573 ) ) ;
#42115=CARTESIAN_POINT ( 'NONE',  ( -4.483927247898782831, 16.52544592524335698, 22.70942372801901499 ) ) ;
#42116=CARTESIAN_POINT ( 'NONE',  ( -12.06949235617739369, -12.14591786802326823, 99.37609039468568994 ) ) ;
#42117=CARTESIAN_POINT ( 'NONE',  ( -0.05219959533909027116, -19.03943276465977164, 42.49890960531435269 ) ) ;
#42118=CARTESIAN_POINT ( 'NONE',  ( -15.72974639402197994, 15.80617190586746368, 25.62390960531435624 ) ) ;
#42119=CARTESIAN_POINT ( 'NONE',  ( -21.55341960407619339, 5.719274019375674811, 48.54275706135234714 ) ) ;
#42120=CARTESIAN_POINT ( 'NONE',  ( -14.29746914071037622, -8.314922557961029526, 24.16775706135235424 ) ) ;
#42122=CARTESIAN_POINT ( 'NONE',  ( 13.97604488694527802, 13.89961937509977652, 74.37390960531436690 ) ) ;
#42123=CARTESIAN_POINT ( 'NONE',  ( -9.474510206698964154, 16.51473224551069663, 115.4155762719810241 ) ) ;
#42124=CARTESIAN_POINT ( 'NONE',  ( 12.06949235617757843, -12.14591786802309237, 68.12390960531436690 ) ) ;
#42125=CARTESIAN_POINT ( 'NONE',  ( 13.89961937509977652, -13.97604488694527269, 83.12390960531436690 ) ) ;
#42126=CARTESIAN_POINT ( 'NONE',  ( -19.02544592524342804, 5.153800228976336051, 71.04057627198099567 ) ) ;
#42127=EDGE_CURVE ( 'NONE', #199942, #99274, #157141, .T. ) ;
#42128=CARTESIAN_POINT ( 'NONE',  ( 16.51473224551083163, -9.474510206698727899, 95.83442372801900433 ) ) ;
#42129=CARTESIAN_POINT ( 'NONE',  ( 15.72974639402199770, -15.80617190586745480, 68.12390960531436690 ) ) ;
#42130=CARTESIAN_POINT ( 'NONE',  ( 19.05341960407611168, 5.049401038298154454, 28.95724293864769550 ) ) ;
#42131=CARTESIAN_POINT ( 'NONE',  ( -9.474510206698720793, -16.51473224551083518, 59.58442372801900433 ) ) ;
#42132=CARTESIAN_POINT ( 'NONE',  ( 5.049401038298161559, -19.05341960407611168, 57.70724293864769550 ) ) ;
#42133=CARTESIAN_POINT ( 'NONE',  ( 16.51473224551069308, 9.474510206698969483, 89.16557627198103830 ) ) ;
#42135=CARTESIAN_POINT ( 'NONE',  ( 18.67979575497178502, 10.72451020669898547, 84.16557627198103830 ) ) ;
#42136=CARTESIAN_POINT ( 'NONE',  ( -8.314922557960811034, -14.29746914071050412, 92.08224293864769550 ) ) ;
#42137=CARTESIAN_POINT ( 'NONE',  ( -9.474510206698720793, -16.51473224551083518, 44.58442372801900433 ) ) ;
#42138=CARTESIAN_POINT ( 'NONE',  ( 0.05219959533907565091, 21.53943276465977519, 69.99890960531435269 ) ) ;
#42139=CARTESIAN_POINT ( 'NONE',  ( 15.80617190586746368, 15.72974639402197994, 74.37390960531436690 ) ) ;
#42140=CARTESIAN_POINT ( 'NONE',  ( -14.34966873604960291, -8.224510206698953496, 31.66557627198102054 ) ) ;
#42141=CARTESIAN_POINT ( 'NONE',  ( -5.719274019375665041, -21.55341960407619695, 109.7927570613523613 ) ) ;
#42142=CARTESIAN_POINT ( 'NONE',  ( 16.46253265017160672, -9.564922557960803928, 73.33224293864769550 ) ) ;
#42143=CARTESIAN_POINT ( 'NONE',  ( 13.89961937509977652, -13.97604488694527269, 38.12390960531436690 ) ) ;
#42145=CARTESIAN_POINT ( 'NONE',  ( 0.05219959533937995610, -21.53943276465977519, 35.00109039468568284 ) ) ;
#42146=CARTESIAN_POINT ( 'NONE',  ( 10.81492255796106328, -18.62759615963255655, 50.41775706135235424 ) ) ;
#42147=CARTESIAN_POINT ( 'NONE',  ( -9.474510206698964154, 16.51473224551069663, 50.41557627198102409 ) ) ;
#42148=CARTESIAN_POINT ( 'NONE',  ( 18.67979575497178502, 10.72451020669898547, 114.1655762719810383 ) ) ;
#42149=CARTESIAN_POINT ( 'NONE',  ( -16.46253265017146816, -9.564922557961047289, 59.16775706135233293 ) ) ;
#42150=CARTESIAN_POINT ( 'NONE',  ( 19.02544592524343514, -5.153800228976328945, 33.54057627198102409 ) ) ;
#42151=CARTESIAN_POINT ( 'NONE',  ( -8.314922557961024197, 14.29746914071037800, 32.91775706135234714 ) ) ;
#42152=CARTESIAN_POINT ( 'NONE',  ( -16.51473224551069308, -9.474510206698971260, 21.66557627198102765 ) ) ;
#42153=CARTESIAN_POINT ( 'NONE',  ( 8.314922557961029526, -14.29746914071037800, 75.41775706135233293 ) ) ;
#42154=CARTESIAN_POINT ( 'NONE',  ( -16.51473224551069308, -9.474510206698971260, 41.66557627198103120 ) ) ;
#42156=CARTESIAN_POINT ( 'NONE',  ( -5.153800228976328057, -19.02544592524343514, 87.29057627198103830 ) ) ;
#42157=CARTESIAN_POINT ( 'NONE',  ( -13.97604488694527625, -13.89961937509977652, 26.87390960531434558 ) ) ;
#42158=CARTESIAN_POINT ( 'NONE',  ( 18.62759615963271287, -10.81492255796078972, 73.33224293864769550 ) ) ;
#42159=CARTESIAN_POINT ( 'NONE',  ( 16.55341960407618274, -4.379528057220086978, 51.04275706135234714 ) ) ;
#42160=CARTESIAN_POINT ( 'NONE',  ( -5.153800228976607833, 19.02544592524334988, 22.70942372801899012 ) ) ;
#42161=CARTESIAN_POINT ( 'NONE',  ( 5.153800228976335163, 19.02544592524342804, 39.79057627198100988 ) ) ;
#42162=CARTESIAN_POINT ( 'NONE',  ( -16.55341960407611168, -4.379528057220339221, 36.45724293864768839 ) ) ;
#42163=CARTESIAN_POINT ( 'NONE',  ( -16.52544592524342804, 4.483927247898546575, 66.04057627198103830 ) ) ;
#42164=CARTESIAN_POINT ( 'NONE',  ( -19.05341960407611168, -5.049401038298163336, 61.45724293864769550 ) ) ;
#42165=CARTESIAN_POINT ( 'NONE',  ( -21.53943276465977519, -0.05219959533937600094, 103.7510903946857042 ) ) ;
#42166=CARTESIAN_POINT ( 'NONE',  ( 5.823673210054444382, -21.52544592524334988, 30.20942372801902565 ) ) ;
#42167=CARTESIAN_POINT ( 'NONE',  ( -16.46253265017160317, 9.564922557960807481, 75.83224293864769550 ) ) ;
#42168=CARTESIAN_POINT ( 'NONE',  ( -5.719274019375665041, -21.55341960407619695, 84.79275706135234714 ) ) ;
#42169=CARTESIAN_POINT ( 'NONE',  ( 16.53943276465976808, 0.05219959533934440121, 71.25109039468568994 ) ) ;
#42170=CARTESIAN_POINT ( 'NONE',  ( -12.06949235617739369, -12.14591786802326823, 34.37609039468568284 ) ) ;
#42171=CARTESIAN_POINT ( 'NONE',  ( 14.34966873604960469, 8.224510206698951720, 94.16557627198103830 ) ) ;
#42172=CARTESIAN_POINT ( 'NONE',  ( -13.97604488694527625, -13.89961937509977652, 111.8739096053143243 ) ) ;
#42173=CARTESIAN_POINT ( 'NONE',  ( -4.483927247898539470, -16.52544592524342804, 27.29057627198103120 ) ) ;
#42174=CARTESIAN_POINT ( 'NONE',  ( 16.46253265017160672, -9.564922557960803928, 23.33224293864769194 ) ) ;
#42175=CARTESIAN_POINT ( 'NONE',  ( -14.34966873604972548, 8.224510206698743886, 48.33442372801902565 ) ) ;
#42176=CARTESIAN_POINT ( 'NONE',  ( -16.52544592524342804, 4.483927247898546575, 61.04057627198103120 ) ) ;
#42177=CARTESIAN_POINT ( 'NONE',  ( 4.483927247898790824, -16.52544592524335698, 105.2094237280190328 ) ) ;
#42178=CARTESIAN_POINT ( 'NONE',  ( 13.97604488694527802, 13.89961937509977652, 114.3739096053143669 ) ) ;
#42179=CARTESIAN_POINT ( 'NONE',  ( -0.05219959533907301413, -21.53943276465977519, 27.49890960531435269 ) ) ;
#42180=CARTESIAN_POINT ( 'NONE',  ( 15.80617190586769283, -15.72974639402175789, 110.6260903946857042 ) ) ;
#42181=CARTESIAN_POINT ( 'NONE',  ( -16.55341960407611168, -4.379528057220339221, 86.45724293864770971 ) ) ;
#42182=CARTESIAN_POINT ( 'NONE',  ( 19.05341960407611168, 5.049401038298154454, 88.95724293864769550 ) ) ;
#42183=ORIENTED_EDGE ( 'NONE', *, *, #157696, .T. ) ;
#42184=CARTESIAN_POINT ( 'NONE',  ( -0.05219959533934338120, 16.53943276465976808, 37.50109039468568284 ) ) ;
#42185=CARTESIAN_POINT ( 'NONE',  ( -16.46253265017160317, 9.564922557960807481, 40.83224293864769550 ) ) ;
#42186=CARTESIAN_POINT ( 'NONE',  ( -8.224510206698735004, -14.34966873604973081, 39.58442372801901143 ) ) ;
#42188=CARTESIAN_POINT ( 'NONE',  ( 5.153800228976615827, -19.02544592524334988, 45.20942372801901143 ) ) ;
#42189=CARTESIAN_POINT ( 'NONE',  ( 16.51473224551069308, 9.474510206698969483, 49.16557627198102409 ) ) ;
#42190=CARTESIAN_POINT ( 'NONE',  ( -16.52544592524335698, -4.483927247898792601, 73.95942372801901854 ) ) ;
#42191=CARTESIAN_POINT ( 'NONE',  ( 0.05219959533936267826, -19.03943276465977164, 100.0010903946856757 ) ) ;
#42192=CARTESIAN_POINT ( 'NONE',  ( -19.03943276465977164, 0.05219959533909376836, 61.24890960531436690 ) ) ;
#42193=CARTESIAN_POINT ( 'NONE',  ( 0.05219959533910956823, 16.53943276465976808, 104.9989096053143669 ) ) ;
#42194=CARTESIAN_POINT ( 'NONE',  ( -5.049401038297874678, -19.05341960407617918, 69.79275706135233293 ) ) ;
#42195=CARTESIAN_POINT ( 'NONE',  ( -5.823673210054116645, -21.52544592524344225, 57.29057627198103120 ) ) ;
#42196=CARTESIAN_POINT ( 'NONE',  ( 13.89961937509957401, 13.97604488694547697, 46.87609039468565442 ) ) ;
#42197=CARTESIAN_POINT ( 'NONE',  ( 19.20446147854524810, 5.499999999999942268, 96.88999695167673565 ) ) ;
#42198=CARTESIAN_POINT ( 'NONE',  ( -18.62759615963270932, 10.81492255796079327, 95.83224293864770971 ) ) ;
#42199=CARTESIAN_POINT ( 'NONE',  ( -17.12812012977029497, 6.668231424565929544, 83.64051240676855059 ) ) ;
#42201=CARTESIAN_POINT ( 'NONE',  ( 16.51473224551083163, -9.474510206698727899, 105.8344237280190043 ) ) ;
#42202=CARTESIAN_POINT ( 'NONE',  ( -18.39635199886966177, 5.500000000000101252, 61.01967076359998998 ) ) ;
#42203=CARTESIAN_POINT ( 'NONE',  ( 16.55341960407618274, -4.379528057220086978, 31.04275706135234714 ) ) ;
#42204=CARTESIAN_POINT ( 'NONE',  ( -9.564922557960796823, -16.46253265017161027, 47.08224293864769550 ) ) ;
#42205=CARTESIAN_POINT ( 'NONE',  ( -13.89961937509977652, 13.97604488694528158, 110.6239096053143243 ) ) ;
#42206=CARTESIAN_POINT ( 'NONE',  ( 21.55341960407610458, 5.719274019375980345, 88.95724293864769550 ) ) ;
#42207=CARTESIAN_POINT ( 'NONE',  ( 10.72451020669871369, 18.67979575497193778, 67.08442372801901854 ) ) ;
#42208=CARTESIAN_POINT ( 'NONE',  ( -9.564922557961040184, 16.46253265017147172, 112.9177570613523329 ) ) ;
#42209=CARTESIAN_POINT ( 'NONE',  ( 13.97604488694548053, -13.89961937509957401, 20.62609039468567573 ) ) ;
#42210=CARTESIAN_POINT ( 'NONE',  ( -8.224510206698948167, 14.34966873604960824, 35.41557627198102409 ) ) ;
#42211=CARTESIAN_POINT ( 'NONE',  ( -0.05219959533907301413, -21.53943276465977519, 102.4989096053143811 ) ) ;
#42212=CARTESIAN_POINT ( 'NONE',  ( -8.314922557960811034, -14.29746914071050412, 47.08224293864770260 ) ) ;
#42213=CARTESIAN_POINT ( 'NONE',  ( -19.05341960407617563, 5.049401038297882671, 88.54275706135230450 ) ) ;
#42214=CARTESIAN_POINT ( 'NONE',  ( -0.05219959533936034679, 19.03943276465977164, 52.50109039468566863 ) ) ;
#42215=CARTESIAN_POINT ( 'NONE',  ( -21.55341960407619339, 5.719274019375674811, 68.54275706135234714 ) ) ;
#42216=CARTESIAN_POINT ( 'NONE',  ( 19.03943276465977164, 0.05219959533936151252, 41.25109039468566152 ) ) ;
#42217=CARTESIAN_POINT ( 'NONE',  ( -9.564922557960796823, -16.46253265017161027, 27.08224293864769550 ) ) ;
#42218=CARTESIAN_POINT ( 'NONE',  ( -10.81492255796078084, -18.62759615963271287, 42.08224293864769550 ) ) ;
#42219=CARTESIAN_POINT ( 'NONE',  ( -4.379528057220328563, 16.55341960407611168, 40.20724293864769550 ) ) ;
#42220=CARTESIAN_POINT ( 'NONE',  ( -0.05219959533937732626, 21.53943276465977519, 107.5010903946856899 ) ) ;
#42221=CARTESIAN_POINT ( 'NONE',  ( -14.34966873604972548, 8.224510206698743886, 73.33442372801901854 ) ) ;
#42222=CARTESIAN_POINT ( 'NONE',  ( -8.224510206698948167, 14.34966873604960824, 35.41557627198102409 ) ) ;
#42223=CARTESIAN_POINT ( 'NONE',  ( 5.823673210054444382, -21.52544592524334988, 70.20942372801904696 ) ) ;
#42224=CARTESIAN_POINT ( 'NONE',  ( -10.81492255796105439, 18.62759615963255655, 72.91775706135234714 ) ) ;
#42225=CARTESIAN_POINT ( 'NONE',  ( -18.67979575497178146, -10.72451020669898902, 71.66557627198100988 ) ) ;
#42226=CARTESIAN_POINT ( 'NONE',  ( 9.564922557960805705, 16.46253265017160317, 44.58224293864769550 ) ) ;
#42227=CARTESIAN_POINT ( 'NONE',  ( -5.823673210054431948, 21.52544592524334988, 37.70942372801900433 ) ) ;
#42228=CARTESIAN_POINT ( 'NONE',  ( 14.29746914071049879, -8.314922557960816363, 113.3322429386476955 ) ) ;
#42229=CARTESIAN_POINT ( 'NONE',  ( 19.05341960407611168, 5.049401038298154454, 33.95724293864769550 ) ) ;
#42230=CARTESIAN_POINT ( 'NONE',  ( 4.379528057220339221, -16.55341960407611168, 97.70724293864772392 ) ) ;
#42231=CARTESIAN_POINT ( 'NONE',  ( 16.46253265017160672, -9.564922557960803928, 88.33224293864769550 ) ) ;
#42232=CARTESIAN_POINT ( 'NONE',  ( 12.06949235617757843, -12.14591786802309237, 43.12390960531435269 ) ) ;
#42233=CARTESIAN_POINT ( 'NONE',  ( 12.06949235617757843, -12.14591786802309237, 98.12390960531436690 ) ) ;
#42234=CARTESIAN_POINT ( 'NONE',  ( 5.823673210054125526, 21.52544592524343514, 64.79057627198103830 ) ) ;
#42235=CARTESIAN_POINT ( 'NONE',  ( -21.53943276465977519, 0.05219959533907696930, 101.2489096053143669 ) ) ;
#42237=CARTESIAN_POINT ( 'NONE',  ( -13.97604488694527625, -13.89961937509977652, 61.87390960531435979 ) ) ;
#42238=CARTESIAN_POINT ( 'NONE',  ( -14.29746914071037622, -8.314922557961029526, 24.16775706135235424 ) ) ;
#42239=CARTESIAN_POINT ( 'NONE',  ( 5.719274019375991003, -21.55341960407610458, 57.70724293864770260 ) ) ;
#42240=CARTESIAN_POINT ( 'NONE',  ( 15.80617190586769283, -15.72974639402175789, 95.62609039468568994 ) ) ;
#42241=CARTESIAN_POINT ( 'NONE',  ( 19.03943276465977164, -0.05219959533909143690, 73.74890960531435269 ) ) ;
#42242=CARTESIAN_POINT ( 'NONE',  ( 18.67979575497178502, 10.72451020669898547, 114.1655762719810383 ) ) ;
#42243=CARTESIAN_POINT ( 'NONE',  ( 9.474510206698971260, -16.51473224551069308, 107.9155762719810383 ) ) ;
#42244=CARTESIAN_POINT ( 'NONE',  ( -12.14591786802326823, 12.06949235617739902, 93.12609039468568994 ) ) ;
#42245=CARTESIAN_POINT ( 'NONE',  ( 18.62759615963255655, 10.81492255796105972, 71.66775706135234714 ) ) ;
#42246=CARTESIAN_POINT ( 'NONE',  ( 15.80617190586769283, -15.72974639402175789, 95.62609039468568994 ) ) ;
#42247=CARTESIAN_POINT ( 'NONE',  ( 8.314922557961029526, -14.29746914071037800, 55.41775706135234714 ) ) ;
#42248=CARTESIAN_POINT ( 'NONE',  ( 18.67979575497194134, -10.72451020669871369, 20.83442372801901143 ) ) ;
#42249=CARTESIAN_POINT ( 'NONE',  ( -19.03943276465977164, 0.05219959533909376836, 21.24890960531436335 ) ) ;
#42250=CARTESIAN_POINT ( 'NONE',  ( 10.81492255796106328, -18.62759615963255655, 85.41775706135236135 ) ) ;
#42251=CARTESIAN_POINT ( 'NONE',  ( 15.80617190586746368, 15.72974639402197994, 89.37390960531435269 ) ) ;
#42252=CARTESIAN_POINT ( 'NONE',  ( -16.46253265017146816, -9.564922557961047289, 49.16775706135233293 ) ) ;
#42253=CARTESIAN_POINT ( 'NONE',  ( 5.719274019375991003, -21.55341960407610458, 57.70724293864770260 ) ) ;
#42254=CARTESIAN_POINT ( 'NONE',  ( -5.049401038298153566, 19.05341960407611168, 100.2072429386476955 ) ) ;
#42255=CARTESIAN_POINT ( 'NONE',  ( -12.06949235617756955, 12.14591786802309770, 40.62390960531435269 ) ) ;
#42258=CARTESIAN_POINT ( 'NONE',  ( -19.53091890409952924, -5.499999999999945821, 80.06097431831415179 ) ) ;
#42260=CARTESIAN_POINT ( 'NONE',  ( 5.049401038297881783, 19.05341960407617563, 102.2927570613523045 ) ) ;
#42261=CARTESIAN_POINT ( 'NONE',  ( -21.53943276465977519, 0.05219959533907696930, 91.24890960531436690 ) ) ;
#42262=CARTESIAN_POINT ( 'NONE',  ( -0.05219959533910754901, -16.53943276465976808, 52.49890960531435979 ) ) ;
#42263=CARTESIAN_POINT ( 'NONE',  ( -16.55341960407617563, 4.379528057220093196, 28.54275706135234358 ) ) ;
#42264=CARTESIAN_POINT ( 'NONE',  ( -19.05341960407611168, -5.049401038298163336, 46.45724293864768129 ) ) ;
#42265=CARTESIAN_POINT ( 'NONE',  ( -21.53943276465977519, -0.05219959533937600094, 18.75109039468568639 ) ) ;
#42266=CARTESIAN_POINT ( 'NONE',  ( -19.05341960407617563, 5.049401038297882671, 83.54275706135233293 ) ) ;
#42267=CARTESIAN_POINT ( 'NONE',  ( 9.564922557960805705, 16.46253265017160317, 84.58224293864769550 ) ) ;
#42268=CARTESIAN_POINT ( 'NONE',  ( -12.14591786802326823, 12.06949235617739902, 28.12609039468568284 ) ) ;
#42269=( BOUNDED_CURVE ( )  B_SPLINE_CURVE ( 2, ( #121208, #182899, #44383, #106038, #11066, #87882, #29222, #90855, #196101, #72744, #71727, #119241, #14028 ),
 .UNSPECIFIED., .F., .F. ) 
 B_SPLINE_CURVE_WITH_KNOTS ( ( 3, 2, 2, 2, 2, 2, 3 ),
 ( 0.3445356995849399029, 0.3464912280701754610, 0.3508771929824561209, 0.3552631578947368363, 0.3596491228070175517, 0.3640350877192982670, 0.3659449363824437418 ),
 .UNSPECIFIED. ) 
 CURVE ( )  GEOMETRIC_REPRESENTATION_ITEM ( )  RATIONAL_B_SPLINE_CURVE ( ( 0.9831626618144004848, 0.9848076720550091867, 1.000000000000000000, 0.9659258262890683122, 1.000000000000000000, 0.9659258262890683122, 1.000000000000000000, 0.9659258262890683122, 1.000000000000000000, 0.9659258262890683122, 1.000000000000000000, 0.9851625545550088958, 0.9832469066685279868 ) ) 
 REPRESENTATION_ITEM ( '' )  );
#42270=CARTESIAN_POINT ( 'NONE',  ( 5.153800228976335163, 19.02544592524342804, 74.79057627198103830 ) ) ;
#42271=CARTESIAN_POINT ( 'NONE',  ( 15.72974639402199770, -15.80617190586745480, 78.12390960531436690 ) ) ;
#42272=CARTESIAN_POINT ( 'NONE',  ( -16.46253265017160317, 9.564922557960807481, 30.83224293864769550 ) ) ;
#42274=CARTESIAN_POINT ( 'NONE',  ( -16.55341960407611168, -4.379528057220339221, 56.45724293864768839 ) ) ;
#42275=CARTESIAN_POINT ( 'NONE',  ( -19.05341960407611168, -5.049401038298163336, 96.45724293864769550 ) ) ;
#42277=CARTESIAN_POINT ( 'NONE',  ( -5.049401038297874678, -19.05341960407617918, 64.79275706135233293 ) ) ;
#42278=CARTESIAN_POINT ( 'NONE',  ( -21.52544592524343514, 5.823673210054127303, 71.04057627198103830 ) ) ;
#42279=CARTESIAN_POINT ( 'NONE',  ( 9.474510206698729675, 16.51473224551082808, 42.08442372801900433 ) ) ;
#42280=CARTESIAN_POINT ( 'NONE',  ( -16.51473224551069308, -9.474510206698971260, 101.6655762719810241 ) ) ;
#42281=DIRECTION ( 'NONE',  ( 0.000000000000000000, 0.04175967627138096189, 0.9991276842514722478 ) ) ;
#42282=CARTESIAN_POINT ( 'NONE',  ( -21.53943276465977519, 0.05219959533907696930, 46.24890960531435979 ) ) ;
#42283=CARTESIAN_POINT ( 'NONE',  ( -19.03943276465977164, 0.05219959533909376836, 76.24890960531435269 ) ) ;
#42284=CARTESIAN_POINT ( 'NONE',  ( 21.55341960407619695, -5.719274019375665929, 61.04275706135234714 ) ) ;
#42285=CARTESIAN_POINT ( 'NONE',  ( 9.474510206698971260, -16.51473224551069308, 27.91557627198103120 ) ) ;
#42286=CARTESIAN_POINT ( 'NONE',  ( -15.80617190586768217, 15.72974639402176855, 23.12609039468567573 ) ) ;
#42288=CARTESIAN_POINT ( 'NONE',  ( -21.52544592524334988, -5.823673210054445271, 48.95942372801902565 ) ) ;
#42290=CARTESIAN_POINT ( 'NONE',  ( 19.02544592524343514, -5.153800228976328945, 98.54057627198100988 ) ) ;
#42292=CARTESIAN_POINT ( 'NONE',  ( -5.823673210054116645, -21.52544592524344225, 102.2905762719810383 ) ) ;
#42293=CARTESIAN_POINT ( 'NONE',  ( -16.46253265017160317, 9.564922557960807481, 55.83224293864769550 ) ) ;
#42294=CARTESIAN_POINT ( 'NONE',  ( 12.06949235617739724, 12.14591786802326823, 36.87609039468568994 ) ) ;
#42296=CARTESIAN_POINT ( 'NONE',  ( -5.719274019375665041, -21.55341960407619695, 104.7927570613523898 ) ) ;
#42297=CARTESIAN_POINT ( 'NONE',  ( 16.46253265017160672, -9.564922557960803928, 43.33224293864769550 ) ) ;
#42298=CARTESIAN_POINT ( 'NONE',  ( -10.81492255796105439, 18.62759615963255655, 102.9177570613523756 ) ) ;
#42299=CARTESIAN_POINT ( 'NONE',  ( -16.46253265017160317, 9.564922557960807481, 95.83224293864769550 ) ) ;
#42300=CARTESIAN_POINT ( 'NONE',  ( -10.72451020669870658, -18.67979575497194134, 59.58442372801901854 ) ) ;
#42302=CARTESIAN_POINT ( 'NONE',  ( -19.05341960407611168, -5.049401038298163336, 111.4572429386476671 ) ) ;
#42303=CARTESIAN_POINT ( 'NONE',  ( -17.50000000000000711, 4.640572885337600262, 30.63788164548843085 ) ) ;
#42304=CARTESIAN_POINT ( 'NONE',  ( 16.52544592524335698, 4.483927247898782831, 46.45942372801901854 ) ) ;
#42305=CARTESIAN_POINT ( 'NONE',  ( 10.72451020669871369, 18.67979575497193778, 62.08442372801901143 ) ) ;
#42306=CARTESIAN_POINT ( 'NONE',  ( 18.62759615963255655, 10.81492255796105972, 86.66775706135234714 ) ) ;
#42308=CARTESIAN_POINT ( 'NONE',  ( -16.52544592524335698, -4.483927247898792601, 23.95942372801901143 ) ) ;
#42309=CARTESIAN_POINT ( 'NONE',  ( -5.153800228976328057, -19.02544592524343514, 67.29057627198102409 ) ) ;
#42310=CARTESIAN_POINT ( 'NONE',  ( 9.564922557960805705, 16.46253265017160317, 114.5822429386476955 ) ) ;
#42311=DIRECTION ( 'NONE',  ( -1.000000000000000000, -0.000000000000000000, -0.000000000000000000 ) ) ;
#42312=CARTESIAN_POINT ( 'NONE',  ( -13.97604488694527625, -13.89961937509977652, 26.87390960531434558 ) ) ;
#42313=CARTESIAN_POINT ( 'NONE',  ( -21.52544592524343514, 5.823673210054127303, 41.04057627198103120 ) ) ;
#42314=CARTESIAN_POINT ( 'NONE',  ( -14.34966873604972548, 8.224510206698743886, 93.33442372801901854 ) ) ;
#42315=CARTESIAN_POINT ( 'NONE',  ( -14.29746914071049879, 8.314922557960819915, 80.83224293864769550 ) ) ;
#42316=CARTESIAN_POINT ( 'NONE',  ( 16.46253265017160672, -9.564922557960803928, 63.33224293864769550 ) ) ;
#42317=CARTESIAN_POINT ( 'NONE',  ( -21.55341960407619339, 5.719274019375674811, 88.54275706135236135 ) ) ;
#42319=CARTESIAN_POINT ( 'NONE',  ( 16.55341960407618274, -4.379528057220086978, 26.04275706135235779 ) ) ;
#42320=CARTESIAN_POINT ( 'NONE',  ( -16.52544592524342804, 4.483927247898546575, 91.04057627198103830 ) ) ;
#42321=CARTESIAN_POINT ( 'NONE',  ( 10.81492255796106328, -18.62759615963255655, 45.41775706135234003 ) ) ;
#42322=CARTESIAN_POINT ( 'NONE',  ( -10.72451020669898014, 18.67979575497178502, 75.41557627198102409 ) ) ;
#42323=CARTESIAN_POINT ( 'NONE',  ( -5.049401038297874678, -19.05341960407617918, 34.79275706135233293 ) ) ;
#42325=CARTESIAN_POINT ( 'NONE',  ( 19.05341960407611168, 5.049401038298154454, 88.95724293864769550 ) ) ;
#42326=CARTESIAN_POINT ( 'NONE',  ( 16.55341960407611168, 4.379528057220329451, 58.95724293864770971 ) ) ;
#42327=CARTESIAN_POINT ( 'NONE',  ( -12.06949235617756955, 12.14591786802309770, 30.62390960531436335 ) ) ;
#42328=CARTESIAN_POINT ( 'NONE',  ( 16.55341960407618274, -4.379528057220086978, 111.0427570613523613 ) ) ;
#42329=CARTESIAN_POINT ( 'NONE',  ( -0.05219959533936034679, 19.03943276465977164, 67.50109039468566152 ) ) ;
#42330=CARTESIAN_POINT ( 'NONE',  ( 17.13100169013298668, 6.664070546373165982, 46.73210164300152059 ) ) ;
#42331=CARTESIAN_POINT ( 'NONE',  ( 13.97604488694527802, 13.89961937509977652, 114.3739096053143669 ) ) ;
#42333=CARTESIAN_POINT ( 'NONE',  ( 8.314922557960818139, 14.29746914071049879, 94.58224293864769550 ) ) ;
#42334=CARTESIAN_POINT ( 'NONE',  ( -17.60769864724390388, 5.499999999999984013, 58.65024842019164453 ) ) ;
#42335=CARTESIAN_POINT ( 'NONE',  ( -16.46253265017160317, 9.564922557960807481, 45.83224293864769550 ) ) ;
#42336=CARTESIAN_POINT ( 'NONE',  ( 0.05219959533907565091, 21.53943276465977519, 49.99890960531437401 ) ) ;
#42337=CARTESIAN_POINT ( 'NONE',  ( -15.72974639402197994, 15.80617190586746368, 65.62390960531436690 ) ) ;
#42338=CARTESIAN_POINT ( 'NONE',  ( -12.06949235617756955, 12.14591786802309770, 115.6239096053143669 ) ) ;
#42339=CARTESIAN_POINT ( 'NONE',  ( -16.53943276465976808, -0.05219959533934237506, 58.75109039468568994 ) ) ;
#42340=CARTESIAN_POINT ( 'NONE',  ( -19.02544592524342804, 5.153800228976336051, 46.04057627198101699 ) ) ;
#42341=CARTESIAN_POINT ( 'NONE',  ( -18.67979575497193778, 10.72451020669871902, 58.33442372801901143 ) ) ;
#42342=CARTESIAN_POINT ( 'NONE',  ( 16.55341960407611168, 4.379528057220329451, 108.9572429386476955 ) ) ;
#42343=CARTESIAN_POINT ( 'NONE',  ( -5.049401038297874678, -19.05341960407617918, 94.79275706135230450 ) ) ;
#42346=CARTESIAN_POINT ( 'NONE',  ( 10.72451020669898902, -18.67979575497178502, 27.91557627198103830 ) ) ;
#42347=CARTESIAN_POINT ( 'NONE',  ( 19.03943276465977164, -0.05219959533909143690, 23.74890960531435269 ) ) ;
#42348=CARTESIAN_POINT ( 'NONE',  ( -15.80617190586768217, 15.72974639402176855, 68.12609039468567573 ) ) ;
#42349=CARTESIAN_POINT ( 'NONE',  ( -8.314922557961024197, 14.29746914071037800, 62.91775706135236135 ) ) ;
#42350=CARTESIAN_POINT ( 'NONE',  ( 16.53943276465976808, -0.05219959533910856209, 48.74890960531435979 ) ) ;
#42351=CARTESIAN_POINT ( 'NONE',  ( 18.62759615963271287, -10.81492255796078972, 63.33224293864770260 ) ) ;
#42352=CARTESIAN_POINT ( 'NONE',  ( -18.67979575497178146, -10.72451020669898902, 61.66557627198103120 ) ) ;
#42354=CARTESIAN_POINT ( 'NONE',  ( -16.51473224551082808, 9.474510206698731452, 88.33442372801900433 ) ) ;
#42355=CARTESIAN_POINT ( 'NONE',  ( -13.89961937509977652, 13.97604488694528158, 110.6239096053143243 ) ) ;
#42356=CARTESIAN_POINT ( 'NONE',  ( 5.153800228976335163, 19.02544592524342804, 54.79057627198103120 ) ) ;
#42357=CARTESIAN_POINT ( 'NONE',  ( -16.52544592524342804, 4.483927247898546575, 111.0405762719810525 ) ) ;
#42358=CARTESIAN_POINT ( 'NONE',  ( -13.89961937509977652, 13.97604488694528158, 110.6239096053143243 ) ) ;
#42360=CARTESIAN_POINT ( 'NONE',  ( -8.314922557961024197, 14.29746914071037800, 67.91775706135234714 ) ) ;
#42361=CARTESIAN_POINT ( 'NONE',  ( 10.81492255796078972, 18.62759615963270932, 104.5822429386477097 ) ) ;
#42362=CARTESIAN_POINT ( 'NONE',  ( 16.51473224551069308, 9.474510206698969483, 64.16557627198102409 ) ) ;
#42363=CARTESIAN_POINT ( 'NONE',  ( -10.72451020669870658, -18.67979575497194134, 34.58442372801900433 ) ) ;
#42364=CARTESIAN_POINT ( 'NONE',  ( -19.05341960407611168, -5.049401038298163336, 101.4572429386476955 ) ) ;
#42367=CARTESIAN_POINT ( 'NONE',  ( 18.62759615963255655, 10.81492255796105972, 36.66775706135234714 ) ) ;
#42368=CARTESIAN_POINT ( 'NONE',  ( 19.03943276465977164, -0.05219959533909143690, 28.74890960531435624 ) ) ;
#42369=CARTESIAN_POINT ( 'NONE',  ( -9.564922557961040184, 16.46253265017147172, 87.91775706135233293 ) ) ;
#42370=CARTESIAN_POINT ( 'NONE',  ( 19.05341960407617918, -5.049401038297876454, 46.04275706135233293 ) ) ;
#42371=CARTESIAN_POINT ( 'NONE',  ( -0.05219959533907301413, -21.53943276465977519, 112.4989096053143669 ) ) ;
#42372=CARTESIAN_POINT ( 'NONE',  ( 13.97604488694548053, -13.89961937509957401, 35.62609039468567573 ) ) ;
#42373=CARTESIAN_POINT ( 'NONE',  ( -13.97604488694547697, 13.89961937509957934, 53.12609039468565442 ) ) ;
#42374=CARTESIAN_POINT ( 'NONE',  ( -4.483927247898782831, 16.52544592524335698, 87.70942372801901854 ) ) ;
#42376=CARTESIAN_POINT ( 'NONE',  ( 13.97604488694527802, 13.89961937509977652, 69.37390960531436690 ) ) ;
#42377=CARTESIAN_POINT ( 'NONE',  ( 18.62759615963255655, 10.81492255796105972, 81.66775706135236135 ) ) ;
#42378=CARTESIAN_POINT ( 'NONE',  ( 15.80617190586769283, -15.72974639402175789, 95.62609039468568994 ) ) ;
#42380=CARTESIAN_POINT ( 'NONE',  ( -5.153800228976328057, -19.02544592524343514, 92.29057627198099567 ) ) ;
#42381=CARTESIAN_POINT ( 'NONE',  ( 5.719274019375673035, 21.55341960407619339, 67.29275706135234714 ) ) ;
#42382=CARTESIAN_POINT ( 'NONE',  ( 19.05341960407617918, -5.049401038297876454, 96.04275706135231871 ) ) ;
#42383=CARTESIAN_POINT ( 'NONE',  ( -5.049401038298153566, 19.05341960407611168, 60.20724293864768129 ) ) ;
#42384=CARTESIAN_POINT ( 'NONE',  ( -0.05219959533909027116, -19.03943276465977164, 112.4989096053143669 ) ) ;
#42385=CARTESIAN_POINT ( 'NONE',  ( -19.03943276465977164, 0.05219959533909376836, 76.24890960531435269 ) ) ;
#42386=CARTESIAN_POINT ( 'NONE',  ( 17.50000000000003553, -5.001413817666677808, 23.20927153282391942 ) ) ;
#42387=CARTESIAN_POINT ( 'NONE',  ( -16.46253265017160317, 9.564922557960807481, 65.83224293864769550 ) ) ;
#42388=CARTESIAN_POINT ( 'NONE',  ( -16.51473224551069308, -9.474510206698971260, 46.66557627198102409 ) ) ;
#42389=CARTESIAN_POINT ( 'NONE',  ( 21.52544592524334988, 5.823673210054432836, 21.45942372801901499 ) ) ;
#42390=CARTESIAN_POINT ( 'NONE',  ( -4.483927247898782831, 16.52544592524335698, 87.70942372801901854 ) ) ;
#42393=CARTESIAN_POINT ( 'NONE',  ( -9.564922557961040184, 16.46253265017147172, 57.91775706135233293 ) ) ;
#42394=CARTESIAN_POINT ( 'NONE',  ( -9.474510206698964154, 16.51473224551069663, 85.41557627198102409 ) ) ;
#42395=CARTESIAN_POINT ( 'NONE',  ( 4.379528057220339221, -16.55341960407611168, 67.70724293864769550 ) ) ;
#42396=CARTESIAN_POINT ( 'NONE',  ( 12.06949235617757843, -12.14591786802309237, 103.1239096053143811 ) ) ;
#42397=CARTESIAN_POINT ( 'NONE',  ( 16.51473224551069308, 9.474510206698969483, 109.1655762719810383 ) ) ;
#42398=CARTESIAN_POINT ( 'NONE',  ( 16.51473224551069308, 9.474510206698969483, 99.16557627198102409 ) ) ;
#42399=CARTESIAN_POINT ( 'NONE',  ( -4.483927247898539470, -16.52544592524342804, 87.29057627198103830 ) ) ;
#42400=CARTESIAN_POINT ( 'NONE',  ( -19.03943276465977164, 0.05219959533909376836, 116.2489096053143669 ) ) ;
#42401=CARTESIAN_POINT ( 'NONE',  ( -19.03943276465977164, -0.05219959533935918106, 28.75109039468566507 ) ) ;
#42402=CARTESIAN_POINT ( 'NONE',  ( -16.55341960407617563, 4.379528057220093196, 108.5427570613523756 ) ) ;
#42403=CARTESIAN_POINT ( 'NONE',  ( -5.049401038298153566, 19.05341960407611168, 95.20724293864770971 ) ) ;
#42404=CARTESIAN_POINT ( 'NONE',  ( 0.05219959533937995610, -21.53943276465977519, 55.00109039468568284 ) ) ;
#42405=CARTESIAN_POINT ( 'NONE',  ( 21.53943276465977519, -0.05219959533907433946, 43.74890960531435979 ) ) ;
#42406=CARTESIAN_POINT ( 'NONE',  ( 21.52544592524334988, 5.823673210054432836, 21.45942372801901499 ) ) ;
#42407=CARTESIAN_POINT ( 'NONE',  ( -5.719274019375978568, 21.55341960407610458, 70.20724293864769550 ) ) ;
#42408=CARTESIAN_POINT ( 'NONE',  ( 14.34966873604960469, 8.224510206698951720, 89.16557627198102409 ) ) ;
#42409=CARTESIAN_POINT ( 'NONE',  ( -9.564922557961040184, 16.46253265017147172, 62.91775706135233293 ) ) ;
#42410=CARTESIAN_POINT ( 'NONE',  ( -13.97604488694527625, -13.89961937509977652, 26.87390960531434558 ) ) ;
#42411=CARTESIAN_POINT ( 'NONE',  ( 5.049401038298161559, -19.05341960407611168, 87.70724293864769550 ) ) ;
#42412=CARTESIAN_POINT ( 'NONE',  ( -5.049401038298153566, 19.05341960407611168, 95.20724293864770971 ) ) ;
#42413=CARTESIAN_POINT ( 'NONE',  ( 14.29746914071049879, -8.314922557960816363, 113.3322429386476955 ) ) ;
#42415=CARTESIAN_POINT ( 'NONE',  ( -16.53943276465976808, -0.05219959533934237506, 113.7510903946856757 ) ) ;
#42416=CARTESIAN_POINT ( 'NONE',  ( 12.06949235617739724, 12.14591786802326823, 41.87609039468568284 ) ) ;
#42417=CARTESIAN_POINT ( 'NONE',  ( -21.55341960407619339, 5.719274019375674811, 103.5427570613523613 ) ) ;
#42418=CARTESIAN_POINT ( 'NONE',  ( -5.153800228976328057, -19.02544592524343514, 102.2905762719810383 ) ) ;
#42419=CARTESIAN_POINT ( 'NONE',  ( -5.823673210054431948, 21.52544592524334988, 27.70942372801901854 ) ) ;
#42420=CARTESIAN_POINT ( 'NONE',  ( 0.05219959533909260263, 19.03943276465977164, 49.99890960531435979 ) ) ;
#42421=CARTESIAN_POINT ( 'NONE',  ( -12.06949235617739369, -12.14591786802326823, 49.37609039468569705 ) ) ;
#42422=CARTESIAN_POINT ( 'NONE',  ( 8.314922557961029526, -14.29746914071037800, 95.41775706135234714 ) ) ;
#42423=CARTESIAN_POINT ( 'NONE',  ( -5.049401038297874678, -19.05341960407617918, 109.7927570613523187 ) ) ;
#42425=CARTESIAN_POINT ( 'NONE',  ( 16.46253265017160672, -9.564922557960803928, 28.33224293864769550 ) ) ;
#42426=CARTESIAN_POINT ( 'NONE',  ( 8.224510206698953496, -14.34966873604960469, 92.91557627198103830 ) ) ;
#42427=CARTESIAN_POINT ( 'NONE',  ( 15.72974639402199770, -15.80617190586745480, 98.12390960531436690 ) ) ;
#42428=CARTESIAN_POINT ( 'NONE',  ( 16.46253265017146816, 9.564922557961045513, 86.66775706135233293 ) ) ;
#42429=CARTESIAN_POINT ( 'NONE',  ( 13.97604488694527802, 13.89961937509977652, 34.37390960531436690 ) ) ;
#42430=CARTESIAN_POINT ( 'NONE',  ( -16.46253265017160317, 9.564922557960807481, 100.8322429386477097 ) ) ;
#42431=CARTESIAN_POINT ( 'NONE',  ( -21.53943276465977519, -0.05219959533937600094, 38.75109039468567573 ) ) ;
#42432=CARTESIAN_POINT ( 'NONE',  ( -5.049401038298153566, 19.05341960407611168, 100.2072429386476955 ) ) ;
#42434=CARTESIAN_POINT ( 'NONE',  ( -9.474510206698964154, 16.51473224551069663, 85.41557627198102409 ) ) ;
#42435=CARTESIAN_POINT ( 'NONE',  ( 21.53943276465977519, 0.05219959533937863772, 26.25109039468567573 ) ) ;
#42436=CARTESIAN_POINT ( 'NONE',  ( -16.52544592524342804, 4.483927247898546575, 86.04057627198102409 ) ) ;
#42437=CARTESIAN_POINT ( 'NONE',  ( -16.51473224551069308, -9.474510206698971260, 91.66557627198103830 ) ) ;
#42438=CARTESIAN_POINT ( 'NONE',  ( -5.049401038297874678, -19.05341960407617918, 19.79275706135233293 ) ) ;
#42439=CARTESIAN_POINT ( 'NONE',  ( -0.05219959533934338120, 16.53943276465976808, 57.50109039468568994 ) ) ;
#42440=CARTESIAN_POINT ( 'NONE',  ( -18.62759615963255300, -10.81492255796106328, 84.16775706135234714 ) ) ;
#42441=CARTESIAN_POINT ( 'NONE',  ( 4.379528057220092307, 16.55341960407617563, 42.29275706135235424 ) ) ;
#42442=CARTESIAN_POINT ( 'NONE',  ( -19.05341960407611168, -5.049401038298163336, 86.45724293864769550 ) ) ;
#42443=CARTESIAN_POINT ( 'NONE',  ( -9.474510206698720793, -16.51473224551083518, 99.58442372801900433 ) ) ;
#42444=CARTESIAN_POINT ( 'NONE',  ( -16.55341960407617563, 4.379528057220093196, 68.54275706135234714 ) ) ;
#42445=CARTESIAN_POINT ( 'NONE',  ( -15.80617190586768217, 15.72974639402176855, 113.1260903946856899 ) ) ;
#42446=CARTESIAN_POINT ( 'NONE',  ( -9.474510206698720793, -16.51473224551083518, 79.58442372801899012 ) ) ;
#42447=CARTESIAN_POINT ( 'NONE',  ( 5.153800228976335163, 19.02544592524342804, 59.79057627198100988 ) ) ;
#42448=CARTESIAN_POINT ( 'NONE',  ( 15.80617190586746368, 15.72974639402197994, 79.37390960531436690 ) ) ;
#42449=CARTESIAN_POINT ( 'NONE',  ( 12.14591786802309770, 12.06949235617756955, 74.37390960531436690 ) ) ;
#42450=CARTESIAN_POINT ( 'NONE',  ( -0.05219959533936034679, 19.03943276465977164, 97.50109039468567573 ) ) ;
#42452=CARTESIAN_POINT ( 'NONE',  ( -5.153800228976607833, 19.02544592524334988, 52.70942372801900433 ) ) ;
#42453=CARTESIAN_POINT ( 'NONE',  ( -0.05219959533934338120, 16.53943276465976808, 107.5010903946856899 ) ) ;
#42454=CARTESIAN_POINT ( 'NONE',  ( -8.314922557960811034, -14.29746914071050412, 82.08224293864768129 ) ) ;
#42455=CARTESIAN_POINT ( 'NONE',  ( 5.823673210054444382, -21.52544592524334988, 110.2094237280190185 ) ) ;
#42456=CARTESIAN_POINT ( 'NONE',  ( 0.05219959533936267826, -19.03943276465977164, 45.00109039468566863 ) ) ;
#42457=CARTESIAN_POINT ( 'NONE',  ( 18.62759615963271287, -10.81492255796078972, 108.3322429386477097 ) ) ;
#42458=CARTESIAN_POINT ( 'NONE',  ( -9.474510206698964154, 16.51473224551069663, 105.4155762719810383 ) ) ;
#42459=CARTESIAN_POINT ( 'NONE',  ( -5.153800228976328057, -19.02544592524343514, 82.29057627198103830 ) ) ;
#42460=CARTESIAN_POINT ( 'NONE',  ( -10.72451020669870658, -18.67979575497194134, 84.58442372801903275 ) ) ;
#42461=CARTESIAN_POINT ( 'NONE',  ( -9.474510206698964154, 16.51473224551069663, 60.41557627198102409 ) ) ;
#42463=CARTESIAN_POINT ( 'NONE',  ( 19.03943276465977164, -0.05219959533909143690, 43.74890960531435979 ) ) ;
#42464=CARTESIAN_POINT ( 'NONE',  ( -15.80617190586745835, -15.72974639402198527, 26.87390960531435979 ) ) ;
#42465=CARTESIAN_POINT ( 'NONE',  ( -16.52544592524342804, 4.483927247898546575, 81.04057627198102409 ) ) ;
#42466=CARTESIAN_POINT ( 'NONE',  ( -13.89961937509977652, 13.97604488694528158, 45.62390960531433848 ) ) ;
#42467=CARTESIAN_POINT ( 'NONE',  ( 14.29746914071049879, -8.314922557960816363, 93.33224293864769550 ) ) ;
#42468=EDGE_CURVE ( 'NONE', #163715, #60746, #86801, .T. ) ;
#42469=CARTESIAN_POINT ( 'NONE',  ( -18.62759615963270932, 10.81492255796079327, 105.8322429386476955 ) ) ;
#42470=CARTESIAN_POINT ( 'NONE',  ( -10.72451020669870658, -18.67979575497194134, 54.58442372801901143 ) ) ;
#42471=CARTESIAN_POINT ( 'NONE',  ( 16.51473224551069308, 9.474510206698969483, 29.16557627198103475 ) ) ;
#42472=CARTESIAN_POINT ( 'NONE',  ( 12.14591786802327356, -12.06949235617739191, 60.62609039468567573 ) ) ;
#42473=CARTESIAN_POINT ( 'NONE',  ( -18.62759615963270932, 10.81492255796079327, 105.8322429386476955 ) ) ;
#42474=CARTESIAN_POINT ( 'NONE',  ( 5.823673210054125526, 21.52544592524343514, 94.79057627198105251 ) ) ;
#42475=CARTESIAN_POINT ( 'NONE',  ( 19.03943276465977164, 0.05219959533936151252, 41.25109039468566152 ) ) ;
#42476=CARTESIAN_POINT ( 'NONE',  ( 9.564922557960805705, 16.46253265017160317, 49.58224293864770260 ) ) ;
#42478=CARTESIAN_POINT ( 'NONE',  ( 21.53943276465977519, 0.05219959533937863772, 51.25109039468568994 ) ) ;
#42479=CARTESIAN_POINT ( 'NONE',  ( 15.72974639402199770, -15.80617190586745480, 58.12390960531435979 ) ) ;
#42480=CARTESIAN_POINT ( 'NONE',  ( 16.55341960407611168, 4.379528057220329451, 43.95724293864769550 ) ) ;
#42481=CARTESIAN_POINT ( 'NONE',  ( 15.72974639402176855, 15.80617190586768217, 81.87609039468568994 ) ) ;
#42482=CARTESIAN_POINT ( 'NONE',  ( -5.823673210054431948, 21.52544592524334988, 107.7094237280190328 ) ) ;
#42483=CARTESIAN_POINT ( 'NONE',  ( 8.224510206698953496, -14.34966873604960469, 102.9155762719810383 ) ) ;
#42484=CARTESIAN_POINT ( 'NONE',  ( -0.05219959533936034679, 19.03943276465977164, 42.50109039468566152 ) ) ;
#42485=CARTESIAN_POINT ( 'NONE',  ( -8.314922557961024197, 14.29746914071037800, 107.9177570613523471 ) ) ;
#42486=CARTESIAN_POINT ( 'NONE',  ( 21.55341960407619695, -5.719274019375665929, 71.04275706135234714 ) ) ;
#42487=CARTESIAN_POINT ( 'NONE',  ( 5.153800228976335163, 19.02544592524342804, 54.79057627198103120 ) ) ;
#42488=CARTESIAN_POINT ( 'NONE',  ( -5.049401038297874678, -19.05341960407617918, 29.79275706135232227 ) ) ;
#42489=CARTESIAN_POINT ( 'NONE',  ( -21.52544592524343514, 5.823673210054127303, 36.04057627198102409 ) ) ;
#42490=CARTESIAN_POINT ( 'NONE',  ( -18.67979575497193778, 10.72451020669871902, 33.33442372801900433 ) ) ;
#42491=CARTESIAN_POINT ( 'NONE',  ( -10.81492255796078084, -18.62759615963271287, 92.08224293864769550 ) ) ;
#42492=CARTESIAN_POINT ( 'NONE',  ( -13.97604488694547697, 13.89961937509957934, 83.12609039468564731 ) ) ;
#42493=CARTESIAN_POINT ( 'NONE',  ( 4.379528057220092307, 16.55341960407617563, 57.29275706135234714 ) ) ;
#42494=CARTESIAN_POINT ( 'NONE',  ( 17.72662750342724891, 5.500000000000081712, 63.90179492283743201 ) ) ;
#42495=CARTESIAN_POINT ( 'NONE',  ( -21.55341960407610458, -5.719274019375992779, 91.45724293864769550 ) ) ;
#42496=CARTESIAN_POINT ( 'NONE',  ( 4.483927247898790824, -16.52544592524335698, 75.20942372801901854 ) ) ;
#42497=CARTESIAN_POINT ( 'NONE',  ( 12.06949235617757843, -12.14591786802309237, 83.12390960531436690 ) ) ;
#42499=CARTESIAN_POINT ( 'NONE',  ( 16.51473224551083163, -9.474510206698727899, 110.8344237280190043 ) ) ;
#42500=CARTESIAN_POINT ( 'NONE',  ( -0.05219959533907301413, -21.53943276465977519, 32.49890960531435979 ) ) ;
#42502=CARTESIAN_POINT ( 'NONE',  ( -0.05219959533934338120, 16.53943276465976808, 57.50109039468568994 ) ) ;
#42503=CARTESIAN_POINT ( 'NONE',  ( -21.52544592524334988, -5.823673210054445271, 23.95942372801901143 ) ) ;
#42504=CARTESIAN_POINT ( 'NONE',  ( -18.67979575497178146, -10.72451020669898902, 41.66557627198103120 ) ) ;
#42505=CARTESIAN_POINT ( 'NONE',  ( 4.379528057220092307, 16.55341960407617563, 77.29275706135234714 ) ) ;
#42506=CARTESIAN_POINT ( 'NONE',  ( -19.03943276465977164, 0.05219959533909376836, 81.24890960531436690 ) ) ;
#42507=CARTESIAN_POINT ( 'NONE',  ( 18.62759615963255655, 10.81492255796105972, 61.66775706135235424 ) ) ;
#42508=CARTESIAN_POINT ( 'NONE',  ( 5.049401038298161559, -19.05341960407611168, 22.70724293864769194 ) ) ;
#42509=CARTESIAN_POINT ( 'NONE',  ( 18.62759615963271287, -10.81492255796078972, 38.33224293864768839 ) ) ;
#42511=CARTESIAN_POINT ( 'NONE',  ( 19.03943276465977164, 0.05219959533936151252, 36.25109039468567573 ) ) ;
#42512=CARTESIAN_POINT ( 'NONE',  ( -0.05219959533934338120, 16.53943276465976808, 57.50109039468568994 ) ) ;
#42513=CARTESIAN_POINT ( 'NONE',  ( 16.51473224551069308, 9.474510206698969483, 114.1655762719810241 ) ) ;
#42516=CARTESIAN_POINT ( 'NONE',  ( -5.153800228976328057, -19.02544592524343514, 87.29057627198103830 ) ) ;
#42517=CARTESIAN_POINT ( 'NONE',  ( -12.06949235617739369, -12.14591786802326823, 99.37609039468568994 ) ) ;
#42518=CARTESIAN_POINT ( 'NONE',  ( -19.03943276465977164, 0.05219959533909376836, 116.2489096053143669 ) ) ;
#42519=CARTESIAN_POINT ( 'NONE',  ( 12.06949235617757843, -12.14591786802309237, 98.12390960531436690 ) ) ;
#42520=CARTESIAN_POINT ( 'NONE',  ( 0.05219959533907565091, 21.53943276465977519, 39.99890960531436690 ) ) ;
#42521=CARTESIAN_POINT ( 'NONE',  ( -13.89961937509977652, 13.97604488694528158, 25.62390960531434558 ) ) ;
#42522=CARTESIAN_POINT ( 'NONE',  ( 14.34966873604972726, -8.224510206698740333, 75.83442372801900433 ) ) ;
#42523=CARTESIAN_POINT ( 'NONE',  ( 5.719274019375991003, -21.55341960407610458, 112.7072429386476955 ) ) ;
#42524=CARTESIAN_POINT ( 'NONE',  ( 19.02544592524334988, 5.153800228976608722, 71.45942372801900433 ) ) ;
#42525=CARTESIAN_POINT ( 'NONE',  ( 5.153800228976335163, 19.02544592524342804, 34.79057627198102409 ) ) ;
#42527=CARTESIAN_POINT ( 'NONE',  ( 5.823673210054444382, -21.52544592524334988, 100.2094237280190043 ) ) ;
#42528=CARTESIAN_POINT ( 'NONE',  ( -19.03943276465977164, 0.05219959533909376836, 61.24890960531436690 ) ) ;
#42530=CARTESIAN_POINT ( 'NONE',  ( -16.55341960407617563, 4.379528057220093196, 53.54275706135234714 ) ) ;
#42531=CARTESIAN_POINT ( 'NONE',  ( 5.719274019375673035, 21.55341960407619339, 87.29275706135236135 ) ) ;
#42532=CARTESIAN_POINT ( 'NONE',  ( 13.97604488694548053, -13.89961937509957401, 40.62609039468564731 ) ) ;
#42533=CARTESIAN_POINT ( 'NONE',  ( -13.97604488694547697, 13.89961937509957934, 53.12609039468565442 ) ) ;
#42535=CARTESIAN_POINT ( 'NONE',  ( -5.823673210054431948, 21.52544592524334988, 47.70942372801902565 ) ) ;
#42537=CARTESIAN_POINT ( 'NONE',  ( -19.03943276465977164, -0.05219959533935918106, 48.75109039468566863 ) ) ;
#42538=CARTESIAN_POINT ( 'NONE',  ( 16.51473224551069308, 9.474510206698969483, 94.16557627198103830 ) ) ;
#42539=CARTESIAN_POINT ( 'NONE',  ( -16.51473224551069308, -9.474510206698971260, 86.66557627198102409 ) ) ;
#42540=CARTESIAN_POINT ( 'NONE',  ( -14.34966873604960291, -8.224510206698953496, 41.66557627198103120 ) ) ;
#42541=CARTESIAN_POINT ( 'NONE',  ( 0.05219959533907565091, 21.53943276465977519, 34.99890960531435979 ) ) ;
#42544=CARTESIAN_POINT ( 'NONE',  ( 10.72451020669871369, 18.67979575497193778, 107.0844237280190043 ) ) ;
#42546=CARTESIAN_POINT ( 'NONE',  ( -9.474510206698964154, 16.51473224551069663, 35.41557627198102409 ) ) ;
#42547=CARTESIAN_POINT ( 'NONE',  ( 19.05341960407611168, 5.049401038298154454, 23.95724293864769194 ) ) ;
#42550=CARTESIAN_POINT ( 'NONE',  ( -16.55341960407617563, 4.379528057220093196, 58.54275706135235424 ) ) ;
#42551=CARTESIAN_POINT ( 'NONE',  ( -10.72451020669898014, 18.67979575497178502, 80.41557627198103830 ) ) ;
#42552=CARTESIAN_POINT ( 'NONE',  ( 14.34966873604960469, 8.224510206698951720, 39.16557627198102409 ) ) ;
#42553=CARTESIAN_POINT ( 'NONE',  ( 13.97604488694527802, 13.89961937509977652, 34.37390960531436690 ) ) ;
#42554=CARTESIAN_POINT ( 'NONE',  ( -9.474510206698964154, 16.51473224551069663, 110.4155762719810383 ) ) ;
#42555=CARTESIAN_POINT ( 'NONE',  ( 18.62759615963255655, 10.81492255796105972, 26.66775706135235424 ) ) ;
#42556=CARTESIAN_POINT ( 'NONE',  ( 13.89961937509957401, 13.97604488694547697, 31.87609039468566863 ) ) ;
#42557=CARTESIAN_POINT ( 'NONE',  ( 5.049401038298161559, -19.05341960407611168, 32.70724293864768129 ) ) ;
#42558=CARTESIAN_POINT ( 'NONE',  ( -10.72451020669870658, -18.67979575497194134, 79.58442372801903275 ) ) ;
#42560=CARTESIAN_POINT ( 'NONE',  ( 8.314922557960818139, 14.29746914071049879, 24.58224293864768839 ) ) ;
#42561=CARTESIAN_POINT ( 'NONE',  ( 17.50000000000000000, 3.305555262949673612, 112.8748284784341251 ) ) ;
#42562=CARTESIAN_POINT ( 'NONE',  ( 10.72451020669898902, -18.67979575497178502, 32.91557627198102409 ) ) ;
#42563=CARTESIAN_POINT ( 'NONE',  ( 14.34966873604960469, 8.224510206698951720, 109.1655762719810383 ) ) ;
#42565=CARTESIAN_POINT ( 'NONE',  ( 19.05341960407611168, 5.049401038298154454, 83.95724293864766707 ) ) ;
#42566=CARTESIAN_POINT ( 'NONE',  ( -16.52544592524342804, 4.483927247898546575, 76.04057627198102409 ) ) ;
#42567=CARTESIAN_POINT ( 'NONE',  ( -19.02544592524334988, -5.153800228976617603, 108.9594237280189759 ) ) ;
#42568=CARTESIAN_POINT ( 'NONE',  ( -10.81492255796078084, -18.62759615963271287, 57.08224293864769550 ) ) ;
#42570=CARTESIAN_POINT ( 'NONE',  ( 9.564922557960805705, 16.46253265017160317, 34.58224293864770260 ) ) ;
#42571=CARTESIAN_POINT ( 'NONE',  ( 0.05219959533909260263, 19.03943276465977164, 84.99890960531436690 ) ) ;
#42572=CARTESIAN_POINT ( 'NONE',  ( 0.05219959533907565091, 21.53943276465977519, 94.99890960531436690 ) ) ;
#42573=CARTESIAN_POINT ( 'NONE',  ( 16.55341960407618274, -4.379528057220086978, 111.0427570613523613 ) ) ;
#42574=CARTESIAN_POINT ( 'NONE',  ( -19.03943276465977164, 0.05219959533909376836, 86.24890960531436690 ) ) ;
#42575=CARTESIAN_POINT ( 'NONE',  ( -13.97604488694547697, 13.89961937509957934, 78.12609039468567573 ) ) ;
#42576=CARTESIAN_POINT ( 'NONE',  ( -5.823673210054431948, 21.52544592524334988, 92.70942372801901854 ) ) ;
#42577=CARTESIAN_POINT ( 'NONE',  ( 5.719274019375991003, -21.55341960407610458, 77.70724293864770971 ) ) ;
#42578=CARTESIAN_POINT ( 'NONE',  ( -5.719274019375978568, 21.55341960407610458, 35.20724293864768839 ) ) ;
#42579=CARTESIAN_POINT ( 'NONE',  ( -9.474510206698964154, 16.51473224551069663, 50.41557627198102409 ) ) ;
#42580=CARTESIAN_POINT ( 'NONE',  ( -12.14591786802309592, -12.06949235617757132, 21.87390960531436690 ) ) ;
#42581=CARTESIAN_POINT ( 'NONE',  ( 19.03943276465977164, -0.05219959533909143690, 58.74890960531435979 ) ) ;
#42583=CARTESIAN_POINT ( 'NONE',  ( -5.049401038297874678, -19.05341960407617918, 24.79275706135233648 ) ) ;
#42584=CARTESIAN_POINT ( 'NONE',  ( 12.06949235617757843, -12.14591786802309237, 73.12390960531436690 ) ) ;
#42585=CARTESIAN_POINT ( 'NONE',  ( -0.05219959533907301413, -21.53943276465977519, 107.4989096053143669 ) ) ;
#42586=CARTESIAN_POINT ( 'NONE',  ( -5.823673210054116645, -21.52544592524344225, 112.2905762719810241 ) ) ;
#42588=CARTESIAN_POINT ( 'NONE',  ( 10.72451020669898902, -18.67979575497178502, 52.91557627198103830 ) ) ;
#42589=CARTESIAN_POINT ( 'NONE',  ( 14.34966873604972726, -8.224510206698740333, 90.83442372801901854 ) ) ;
#42590=CARTESIAN_POINT ( 'NONE',  ( -12.06949235617756955, 12.14591786802309770, 100.6239096053143811 ) ) ;
#42591=CARTESIAN_POINT ( 'NONE',  ( -5.153800228976328057, -19.02544592524343514, 57.29057627198103120 ) ) ;
#42592=CARTESIAN_POINT ( 'NONE',  ( -14.29746914071049879, 8.314922557960819915, 25.83224293864769194 ) ) ;
#42593=ORIENTED_EDGE ( 'NONE', *, *, #47203, .T. ) ;
#42594=CARTESIAN_POINT ( 'NONE',  ( -15.80617190586768217, 15.72974639402176855, 48.12609039468568284 ) ) ;
#42595=CARTESIAN_POINT ( 'NONE',  ( 19.05341960407611168, 5.049401038298154454, 108.9572429386477097 ) ) ;
#42596=CARTESIAN_POINT ( 'NONE',  ( 18.62759615963255655, 10.81492255796105972, 76.66775706135234714 ) ) ;
#42597=CARTESIAN_POINT ( 'NONE',  ( -19.05341960407611168, -5.049401038298163336, 36.45724293864766707 ) ) ;
#42598=CARTESIAN_POINT ( 'NONE',  ( 13.97604488694527802, 13.89961937509977652, 44.37390960531435269 ) ) ;
#42599=ORIENTED_EDGE ( 'NONE', *, *, #7273, .T. ) ;
#42600=CARTESIAN_POINT ( 'NONE',  ( 18.62759615963255655, 10.81492255796105972, 86.66775706135234714 ) ) ;
#42601=CARTESIAN_POINT ( 'NONE',  ( -16.52544592524335698, -4.483927247898792601, 48.95942372801902565 ) ) ;
#42602=CARTESIAN_POINT ( 'NONE',  ( -18.67979575497193778, 10.72451020669871902, 73.33442372801901854 ) ) ;
#42603=CARTESIAN_POINT ( 'NONE',  ( 9.474510206698971260, -16.51473224551069308, 102.9155762719810241 ) ) ;
#42604=CARTESIAN_POINT ( 'NONE',  ( 0.05219959533936267826, -19.03943276465977164, 80.00109039468567573 ) ) ;
#42605=CARTESIAN_POINT ( 'NONE',  ( -21.55341960407619339, 5.719274019375674811, 58.54275706135235424 ) ) ;
#42606=CARTESIAN_POINT ( 'NONE',  ( 14.34966873604972726, -8.224510206698740333, 20.83442372801901143 ) ) ;
#42607=CARTESIAN_POINT ( 'NONE',  ( -13.97604488694547697, 13.89961937509957934, 78.12609039468567573 ) ) ;
#42608=CARTESIAN_POINT ( 'NONE',  ( -5.153800228976328057, -19.02544592524343514, 52.29057627198100988 ) ) ;
#42609=CARTESIAN_POINT ( 'NONE',  ( 19.03943276465977164, 0.05219959533936151252, 86.25109039468567573 ) ) ;
#42610=CARTESIAN_POINT ( 'NONE',  ( -12.14591786802309592, -12.06949235617757132, 21.87390960531436690 ) ) ;
#42611=CARTESIAN_POINT ( 'NONE',  ( -13.89961937509957401, -13.97604488694547875, 84.37609039468567573 ) ) ;
#42612=CARTESIAN_POINT ( 'NONE',  ( 12.14591786802309770, 12.06949235617756955, 34.37390960531435979 ) ) ;
#42613=CARTESIAN_POINT ( 'NONE',  ( -19.05341960407617563, 5.049401038297882671, 68.54275706135230450 ) ) ;
#42614=CARTESIAN_POINT ( 'NONE',  ( 14.29746914071037800, 8.314922557961029526, 46.66775706135234714 ) ) ;
#42615=CARTESIAN_POINT ( 'NONE',  ( 5.153800228976615827, -19.02544592524334988, 20.20942372801899722 ) ) ;
#42616=CARTESIAN_POINT ( 'NONE',  ( 13.97604488694527802, 13.89961937509977652, 39.37390960531435269 ) ) ;
#42617=CARTESIAN_POINT ( 'NONE',  ( 8.314922557961029526, -14.29746914071037800, 40.41775706135234714 ) ) ;
#42620=CIRCLE ( 'NONE', #181481, 2.000000000000001776 ) ;
#42621=CARTESIAN_POINT ( 'NONE',  ( -19.03943276465977164, 0.05219959533909376836, 96.24890960531436690 ) ) ;
#42623=LINE ( 'NONE', #198281, #197634 ) ;
#42624=CARTESIAN_POINT ( 'NONE',  ( 16.46253265017146816, 9.564922557961045513, 101.6677570613523329 ) ) ;
#42625=CARTESIAN_POINT ( 'NONE',  ( 19.05341960407611168, 5.049401038298154454, 113.9572429386477097 ) ) ;
#42626=CARTESIAN_POINT ( 'NONE',  ( -19.05341960407617563, 5.049401038297882671, 23.54275706135233648 ) ) ;
#42627=CARTESIAN_POINT ( 'NONE',  ( 16.53943276465976808, 0.05219959533934440121, 21.25109039468567218 ) ) ;
#42628=CARTESIAN_POINT ( 'NONE',  ( 13.89961937509977652, -13.97604488694527269, 23.12390960531436335 ) ) ;
#42629=CARTESIAN_POINT ( 'NONE',  ( 9.474510206698971260, -16.51473224551069308, 37.91557627198102409 ) ) ;
#42630=CARTESIAN_POINT ( 'NONE',  ( 21.55341960407610458, 5.719274019375980345, 68.95724293864769550 ) ) ;
#42632=CARTESIAN_POINT ( 'NONE',  ( -19.03943276465977164, 0.05219959533909376836, 41.24890960531435269 ) ) ;
#42633=CARTESIAN_POINT ( 'NONE',  ( -5.153800228976607833, 19.02544592524335343, 47.70942372801900433 ) ) ;
#42634=CARTESIAN_POINT ( 'NONE',  ( -5.049401038297874678, -19.05341960407617918, 64.79275706135233293 ) ) ;
#42635=CARTESIAN_POINT ( 'NONE',  ( 12.14591786802309770, 12.06949235617756955, 49.37390960531436690 ) ) ;
#42636=CARTESIAN_POINT ( 'NONE',  ( -21.55341960407610458, -5.719274019375992779, 31.45724293864769550 ) ) ;
#42637=CARTESIAN_POINT ( 'NONE',  ( -10.72451020669870658, -18.67979575497194134, 94.58442372801901854 ) ) ;
#42638=EDGE_CURVE ( 'NONE', #111352, #198671, #40985, .T. ) ;
#42639=CARTESIAN_POINT ( 'NONE',  ( -18.62759615963270932, 10.81492255796079327, 80.83224293864769550 ) ) ;
#42640=CARTESIAN_POINT ( 'NONE',  ( -18.67979575497193778, 10.72451020669871902, 53.33442372801901854 ) ) ;
#42641=CARTESIAN_POINT ( 'NONE',  ( -15.72974639402176322, -15.80617190586768395, 64.37609039468568994 ) ) ;
#42642=CARTESIAN_POINT ( 'NONE',  ( -13.97604488694527625, -13.89961937509977652, 101.8739096053143811 ) ) ;
#42643=CARTESIAN_POINT ( 'NONE',  ( -8.314922557961024197, 14.29746914071037800, 87.91775706135234714 ) ) ;
#42644=CARTESIAN_POINT ( 'NONE',  ( 21.52544592524334988, 5.823673210054432836, 61.45942372801901854 ) ) ;
#42645=CARTESIAN_POINT ( 'NONE',  ( 9.474510206698971260, -16.51473224551069308, 57.91557627198103120 ) ) ;
#42646=CARTESIAN_POINT ( 'NONE',  ( 19.05341960407611168, 5.049401038298154454, 23.95724293864769194 ) ) ;
#42647=CARTESIAN_POINT ( 'NONE',  ( 9.564922557960805705, 16.46253265017160317, 54.58224293864769550 ) ) ;
#42648=CARTESIAN_POINT ( 'NONE',  ( 16.55341960407611168, 4.379528057220329451, 68.95724293864769550 ) ) ;
#42649=CARTESIAN_POINT ( 'NONE',  ( -16.53943276465976808, 0.05219959533911058130, 36.24890960531435979 ) ) ;
#42650=CARTESIAN_POINT ( 'NONE',  ( -10.81492255796078084, -18.62759615963271287, 47.08224293864770260 ) ) ;
#42651=CARTESIAN_POINT ( 'NONE',  ( -19.02544592524342804, 5.153800228976336051, 51.04057627198103120 ) ) ;
#42652=CARTESIAN_POINT ( 'NONE',  ( 15.80617190586746368, 15.72974639402197994, 59.37390960531436690 ) ) ;
#42653=CARTESIAN_POINT ( 'NONE',  ( 9.564922557961047289, -16.46253265017146816, 50.41775706135233293 ) ) ;
#42655=CARTESIAN_POINT ( 'NONE',  ( -14.34966873604960291, -8.224510206698953496, 61.66557627198103120 ) ) ;
#42656=CARTESIAN_POINT ( 'NONE',  ( 18.67979575497178502, 10.72451020669898547, 39.16557627198102409 ) ) ;
#42658=ORIENTED_EDGE ( 'NONE', *, *, #190013, .F. ) ;
#42659=CARTESIAN_POINT ( 'NONE',  ( 16.18388926212237422, 7.379444403734533253, 102.9395315136615210 ) ) ;
#42660=CARTESIAN_POINT ( 'NONE',  ( 4.379528057220092307, 16.55341960407617563, 82.29275706135234714 ) ) ;
#42661=CARTESIAN_POINT ( 'NONE',  ( -5.049401038297874678, -19.05341960407617918, 69.79275706135233293 ) ) ;
#42662=CARTESIAN_POINT ( 'NONE',  ( 4.483927247898545687, 16.52544592524342804, 49.79057627198102409 ) ) ;
#42664=CARTESIAN_POINT ( 'NONE',  ( -9.564922557960796823, -16.46253265017161027, 52.08224293864768839 ) ) ;
#42665=CARTESIAN_POINT ( 'NONE',  ( -16.55341960407611168, -4.379528057220339221, 41.45724293864769550 ) ) ;
#42666=CARTESIAN_POINT ( 'NONE',  ( -9.474510206698964154, 16.51473224551069663, 50.41557627198102409 ) ) ;
#42668=CARTESIAN_POINT ( 'NONE',  ( 5.153800228976335163, 19.02544592524342804, 69.79057627198103830 ) ) ;
#42669=CARTESIAN_POINT ( 'NONE',  ( -16.51473224551069308, -9.474510206698971260, 36.66557627198102409 ) ) ;
#42670=CARTESIAN_POINT ( 'NONE',  ( 0.05219959533937995610, -21.53943276465977519, 45.00109039468568284 ) ) ;
#42671=CARTESIAN_POINT ( 'NONE',  ( 5.049401038298161559, -19.05341960407611168, 77.70724293864765286 ) ) ;
#42672=CARTESIAN_POINT ( 'NONE',  ( 13.97604488694527802, 13.89961937509977652, 29.37390960531435979 ) ) ;
#42673=CARTESIAN_POINT ( 'NONE',  ( 16.46253265017160672, -9.564922557960803928, 58.33224293864769550 ) ) ;
#42674=CARTESIAN_POINT ( 'NONE',  ( 10.81492255796078972, 18.62759615963270932, 44.58224293864769550 ) ) ;
#42675=CARTESIAN_POINT ( 'NONE',  ( -19.03943276465977164, 0.05219959533909376836, 36.24890960531436690 ) ) ;
#42676=CARTESIAN_POINT ( 'NONE',  ( -10.72451020669898014, 18.67979575497178502, 40.41557627198103120 ) ) ;
#42677=CARTESIAN_POINT ( 'NONE',  ( -14.34966873604972548, 8.224510206698743886, 98.33442372801901854 ) ) ;
#42678=CARTESIAN_POINT ( 'NONE',  ( -16.46253265017146816, -9.564922557961047289, 29.16775706135232937 ) ) ;
#42679=CARTESIAN_POINT ( 'NONE',  ( 12.14591786802327356, -12.06949235617739191, 50.62609039468568994 ) ) ;
#42680=CARTESIAN_POINT ( 'NONE',  ( 16.52544592524335698, 4.483927247898782831, 81.45942372801900433 ) ) ;
#42681=CARTESIAN_POINT ( 'NONE',  ( -18.22780087662122028, 5.500000000000031086, 68.51540105326107266 ) ) ;
#42682=CARTESIAN_POINT ( 'NONE',  ( -14.29746914071037622, -8.314922557961029526, 69.16775706135234714 ) ) ;
#42683=CARTESIAN_POINT ( 'NONE',  ( 12.06949235617739724, 12.14591786802326823, 46.87609039468568994 ) ) ;
#42684=CARTESIAN_POINT ( 'NONE',  ( -19.05341960407611168, -5.049401038298163336, 111.4572429386476671 ) ) ;
#42685=CARTESIAN_POINT ( 'NONE',  ( 16.52544592524335698, 4.483927247898782831, 36.45942372801901143 ) ) ;
#42686=CARTESIAN_POINT ( 'NONE',  ( -5.049401038298153566, 19.05341960407611168, 30.20724293864768839 ) ) ;
#42687=CARTESIAN_POINT ( 'NONE',  ( -10.81492255796105439, 18.62759615963255655, 22.91775706135235069 ) ) ;
#42688=CARTESIAN_POINT ( 'NONE',  ( 8.314922557961029526, -14.29746914071037800, 30.41775706135234358 ) ) ;
#42689=CARTESIAN_POINT ( 'NONE',  ( -14.34966873604972548, 8.224510206698743886, 98.33442372801901854 ) ) ;
#42690=CARTESIAN_POINT ( 'NONE',  ( -18.09918380851993902, -5.499999999999988454, 71.48618307335610211 ) ) ;
#42691=CARTESIAN_POINT ( 'NONE',  ( 21.55341960407619695, -5.719274019375665929, 106.0427570613523471 ) ) ;
#42692=CARTESIAN_POINT ( 'NONE',  ( -19.03943276465977164, -0.05219959533935918106, 98.75109039468567573 ) ) ;
#42693=CARTESIAN_POINT ( 'NONE',  ( -16.55341960407611168, -4.379528057220339221, 61.45724293864770260 ) ) ;
#42694=CARTESIAN_POINT ( 'NONE',  ( -19.03943276465977164, 0.05219959533909376836, 26.24890960531435624 ) ) ;
#42695=CARTESIAN_POINT ( 'NONE',  ( -19.05341960407617563, 5.049401038297882671, 58.54275706135234003 ) ) ;
#42696=CARTESIAN_POINT ( 'NONE',  ( 16.29526858892876007, 7.335722546920145248, 78.29670597800209464 ) ) ;
#42697=CARTESIAN_POINT ( 'NONE',  ( -15.72974639402176322, -15.80617190586768395, 59.37609039468568284 ) ) ;
#42698=CARTESIAN_POINT ( 'NONE',  ( -16.53943276465976808, -0.05219959533934237506, 28.75109039468567929 ) ) ;
#42700=CARTESIAN_POINT ( 'NONE',  ( 19.02544592524343514, -5.153800228976328945, 113.5405762719810241 ) ) ;
#42701=CARTESIAN_POINT ( 'NONE',  ( 15.72974639402199770, -15.80617190586745480, 78.12390960531436690 ) ) ;
#42702=CARTESIAN_POINT ( 'NONE',  ( -16.51473224551082808, 9.474510206698731452, 113.3344237280190043 ) ) ;
#42703=CARTESIAN_POINT ( 'NONE',  ( 16.46253265017160672, -9.564922557960803928, 108.3322429386476955 ) ) ;
#42705=CARTESIAN_POINT ( 'NONE',  ( 0.05219959533910956823, 16.53943276465976808, 114.9989096053143669 ) ) ;
#42706=CARTESIAN_POINT ( 'NONE',  ( -10.72451020669870658, -18.67979575497194134, 109.5844237280190328 ) ) ;
#42707=CARTESIAN_POINT ( 'NONE',  ( 19.02544592524343514, -5.153800228976328945, 48.54057627198103120 ) ) ;
#42708=CARTESIAN_POINT ( 'NONE',  ( 10.81492255796106328, -18.62759615963255655, 55.41775706135234714 ) ) ;
#42709=CARTESIAN_POINT ( 'NONE',  ( -18.62759615963255300, -10.81492255796106328, 99.16775706135234714 ) ) ;
#42710=CARTESIAN_POINT ( 'NONE',  ( -4.379528057220086978, -16.55341960407618274, 109.7927570613523613 ) ) ;
#42711=CARTESIAN_POINT ( 'NONE',  ( -0.05219959533909027116, -19.03943276465977164, 77.49890960531435269 ) ) ;
#42712=CARTESIAN_POINT ( 'NONE',  ( -10.81492255796105439, 18.62759615963255655, 42.91775706135235424 ) ) ;
#42713=CARTESIAN_POINT ( 'NONE',  ( 5.823673210054444382, -21.52544592524334988, 55.20942372801902565 ) ) ;
#42714=CARTESIAN_POINT ( 'NONE',  ( 9.474510206698729675, 16.51473224551082808, 82.08442372801899012 ) ) ;
#42715=CARTESIAN_POINT ( 'NONE',  ( -9.564922557960796823, -16.46253265017161027, 87.08224293864769550 ) ) ;
#42716=CARTESIAN_POINT ( 'NONE',  ( 8.314922557960818139, 14.29746914071049879, 109.5822429386476955 ) ) ;
#42717=CARTESIAN_POINT ( 'NONE',  ( 15.72974639402199770, -15.80617190586745480, 93.12390960531436690 ) ) ;
#42718=CARTESIAN_POINT ( 'NONE',  ( -8.314922557960811034, -14.29746914071050412, 72.08224293864769550 ) ) ;
#42719=CARTESIAN_POINT ( 'NONE',  ( 18.62759615963255655, 10.81492255796105972, 111.6677570613523613 ) ) ;
#42720=CARTESIAN_POINT ( 'NONE',  ( 16.52544592524342804, -4.483927247898539470, 98.54057627198105251 ) ) ;
#42721=CARTESIAN_POINT ( 'NONE',  ( 0.05219959533909260263, 19.03943276465977164, 44.99890960531435979 ) ) ;
#42722=CARTESIAN_POINT ( 'NONE',  ( -5.049401038297874678, -19.05341960407617918, 79.79275706135233293 ) ) ;
#42723=CARTESIAN_POINT ( 'NONE',  ( 4.379528057220339221, -16.55341960407611168, 47.70724293864770260 ) ) ;
#42724=CARTESIAN_POINT ( 'NONE',  ( -0.05219959533937732626, 21.53943276465977519, 112.5010903946857042 ) ) ;
#42725=CARTESIAN_POINT ( 'NONE',  ( 13.97604488694527802, 13.89961937509977652, 104.3739096053143385 ) ) ;
#42726=CARTESIAN_POINT ( 'NONE',  ( 9.564922557961047289, -16.46253265017146816, 80.41775706135234714 ) ) ;
#42727=CARTESIAN_POINT ( 'NONE',  ( -10.72451020669898014, 18.67979575497178502, 75.41557627198102409 ) ) ;
#42728=CARTESIAN_POINT ( 'NONE',  ( 10.72451020669871369, 18.67979575497193778, 27.08442372801901854 ) ) ;
#42729=CARTESIAN_POINT ( 'NONE',  ( -16.53943276465976808, -0.05219959533934237506, 33.75109039468568284 ) ) ;
#42730=CARTESIAN_POINT ( 'NONE',  ( 14.29746914071037800, 8.314922557961029526, 96.66775706135234714 ) ) ;
#42731=CARTESIAN_POINT ( 'NONE',  ( 17.40805194822031154, 6.112264579159360167, 61.66628727489387529 ) ) ;
#42732=CARTESIAN_POINT ( 'NONE',  ( -21.52544592524334988, -5.823673210054445271, 33.95942372801901143 ) ) ;
#42733=CARTESIAN_POINT ( 'NONE',  ( -10.81492255796078084, -18.62759615963271287, 47.08224293864770260 ) ) ;
#42734=CARTESIAN_POINT ( 'NONE',  ( -8.224510206698948167, 14.34966873604960824, 115.4155762719810241 ) ) ;
#42736=CARTESIAN_POINT ( 'NONE',  ( -4.483927247898782831, 16.52544592524335698, 67.70942372801901854 ) ) ;
#42737=CARTESIAN_POINT ( 'NONE',  ( 4.379528057220339221, -16.55341960407611168, 97.70724293864772392 ) ) ;
#42738=CARTESIAN_POINT ( 'NONE',  ( -18.67979575497178146, -10.72451020669898902, 76.66557627198103830 ) ) ;
#42739=CARTESIAN_POINT ( 'NONE',  ( 8.314922557960818139, 14.29746914071049879, 29.58224293864769905 ) ) ;
#42740=CARTESIAN_POINT ( 'NONE',  ( 8.224510206698742110, 14.34966873604972548, 52.08442372801901854 ) ) ;
#42741=CARTESIAN_POINT ( 'NONE',  ( 9.564922557960805705, 16.46253265017160317, 44.58224293864769550 ) ) ;
#42742=CARTESIAN_POINT ( 'NONE',  ( 16.53943276465976808, 0.05219959533934440121, 96.25109039468568994 ) ) ;
#42743=CARTESIAN_POINT ( 'NONE',  ( 13.89961937509957401, 13.97604488694547697, 91.87609039468567573 ) ) ;
#42744=CARTESIAN_POINT ( 'NONE',  ( -0.05219959533907301413, -21.53943276465977519, 87.49890960531436690 ) ) ;
#42745=CARTESIAN_POINT ( 'NONE',  ( 0.05219959533934541429, -16.53943276465976808, 105.0010903946856757 ) ) ;
#42746=ORIENTED_EDGE ( 'NONE', *, *, #48034, .T. ) ;
#42747=CARTESIAN_POINT ( 'NONE',  ( 19.03943276465977164, -0.05219959533909143690, 113.7489096053143669 ) ) ;
#42748=CARTESIAN_POINT ( 'NONE',  ( -18.62759615963270932, 10.81492255796079327, 55.83224293864770260 ) ) ;
#42749=CARTESIAN_POINT ( 'NONE',  ( -8.314922557961024197, 14.29746914071037800, 97.91775706135236135 ) ) ;
#42751=CARTESIAN_POINT ( 'NONE',  ( 10.81492255796078972, 18.62759615963270932, 24.58224293864768839 ) ) ;
#42752=CARTESIAN_POINT ( 'NONE',  ( -18.87075004821565472, 5.500000000000079048, 73.67408112101047379 ) ) ;
#42753=CARTESIAN_POINT ( 'NONE',  ( -18.62759615963270932, 10.81492255796079327, 80.83224293864769550 ) ) ;
#42754=CARTESIAN_POINT ( 'NONE',  ( -4.379528057220328563, 16.55341960407611168, 30.20724293864769550 ) ) ;
#42755=CARTESIAN_POINT ( 'NONE',  ( -4.379528057220086978, -16.55341960407618274, 19.79275706135235069 ) ) ;
#42756=CARTESIAN_POINT ( 'NONE',  ( 13.89961937509977652, -13.97604488694527269, 38.12390960531436690 ) ) ;
#42757=CARTESIAN_POINT ( 'NONE',  ( 14.34966873604972726, -8.224510206698740333, 30.83442372801902209 ) ) ;
#42758=CARTESIAN_POINT ( 'NONE',  ( 0.05219959533909260263, 19.03943276465977164, 54.99890960531435979 ) ) ;
#42760=CARTESIAN_POINT ( 'NONE',  ( -16.51473224551069308, -9.474510206698971260, 106.6655762719810383 ) ) ;
#42761=CARTESIAN_POINT ( 'NONE',  ( -19.05341960407611168, -5.049401038298163336, 106.4572429386476955 ) ) ;
#42763=CARTESIAN_POINT ( 'NONE',  ( -14.34966873604972548, 8.224510206698743886, 83.33442372801903275 ) ) ;
#42764=CARTESIAN_POINT ( 'NONE',  ( 19.03943276465977164, 0.05219959533936151252, 96.25109039468567573 ) ) ;
#42765=CARTESIAN_POINT ( 'NONE',  ( -5.153800228976607833, 19.02544592524334988, 42.70942372801901143 ) ) ;
#42766=CARTESIAN_POINT ( 'NONE',  ( -21.52544592524343514, 5.823673210054127303, 71.04057627198103830 ) ) ;
#42767=CARTESIAN_POINT ( 'NONE',  ( -4.483927247898782831, 16.52544592524335698, 97.70942372801904696 ) ) ;
#42768=CARTESIAN_POINT ( 'NONE',  ( -0.05219959533907301413, -21.53943276465977519, 27.49890960531435269 ) ) ;
#42769=CARTESIAN_POINT ( 'NONE',  ( 9.474510206698729675, 16.51473224551082808, 87.08442372801900433 ) ) ;
#42770=CARTESIAN_POINT ( 'NONE',  ( -5.049401038298153566, 19.05341960407611168, 50.20724293864770260 ) ) ;
#42771=CARTESIAN_POINT ( 'NONE',  ( 0.05219959533909260263, 19.03943276465977164, 94.99890960531436690 ) ) ;
#42772=CARTESIAN_POINT ( 'NONE',  ( -0.05219959533937732626, 21.53943276465977519, 57.50109039468568994 ) ) ;
#42773=CARTESIAN_POINT ( 'NONE',  ( 19.02544592524343514, -5.153800228976328945, 58.54057627198102409 ) ) ;
#42774=CARTESIAN_POINT ( 'NONE',  ( 14.29746914071049879, -8.314922557960816363, 103.3322429386476955 ) ) ;
#42775=CARTESIAN_POINT ( 'NONE',  ( -17.40805194822031865, -6.112264579159316646, 84.16628727489391792 ) ) ;
#42776=CARTESIAN_POINT ( 'NONE',  ( 8.224510206698953496, -14.34966873604960469, 82.91557627198103830 ) ) ;
#42777=CARTESIAN_POINT ( 'NONE',  ( 15.72974639402199770, -15.80617190586745480, 68.12390960531436690 ) ) ;
#42778=CARTESIAN_POINT ( 'NONE',  ( -16.51473224551082808, 9.474510206698731452, 88.33442372801900433 ) ) ;
#42780=CARTESIAN_POINT ( 'NONE',  ( 19.05341960407611168, 5.049401038298154454, 58.95724293864768129 ) ) ;
#42782=CARTESIAN_POINT ( 'NONE',  ( -19.03943276465977164, 0.05219959533909376836, 81.24890960531436690 ) ) ;
#42783=CARTESIAN_POINT ( 'NONE',  ( -13.97604488694527625, -13.89961937509977652, 81.87390960531436690 ) ) ;
#42784=CARTESIAN_POINT ( 'NONE',  ( -16.52544592524335698, -4.483927247898792601, 63.95942372801901854 ) ) ;
#42786=CARTESIAN_POINT ( 'NONE',  ( 0.05219959533936267826, -19.03943276465977164, 45.00109039468566863 ) ) ;
#42788=CARTESIAN_POINT ( 'NONE',  ( 19.03943276465977164, -0.05219959533909143690, 113.7489096053143669 ) ) ;
#42789=CARTESIAN_POINT ( 'NONE',  ( -4.379528057220086978, -16.55341960407618274, 104.7927570613523898 ) ) ;
#42792=CARTESIAN_POINT ( 'NONE',  ( -12.14591786802326823, 12.06949235617739902, 78.12609039468570415 ) ) ;
#42793=CARTESIAN_POINT ( 'NONE',  ( -16.88567814943165857, 6.947325034625572826, 28.70998877347415501 ) ) ;
#42794=CARTESIAN_POINT ( 'NONE',  ( 16.55341960407618274, -4.379528057220086978, 56.04275706135235424 ) ) ;
#42795=CARTESIAN_POINT ( 'NONE',  ( -5.049401038298153566, 19.05341960407611168, 75.20724293864769550 ) ) ;
#42796=CARTESIAN_POINT ( 'NONE',  ( -18.67979575497193778, 10.72451020669871902, 63.33442372801900433 ) ) ;
#42797=CARTESIAN_POINT ( 'NONE',  ( -5.049401038297874678, -19.05341960407617918, 74.79275706135231871 ) ) ;
#42798=CARTESIAN_POINT ( 'NONE',  ( 5.153800228976615827, -19.02544592524334988, 30.20942372801900433 ) ) ;
#42799=CARTESIAN_POINT ( 'NONE',  ( -13.89961937509977652, 13.97604488694528158, 70.62390960531432427 ) ) ;
#42800=CARTESIAN_POINT ( 'NONE',  ( 19.03943276465977164, -0.05219959533909143690, 38.74890960531436690 ) ) ;
#42801=CARTESIAN_POINT ( 'NONE',  ( 17.29445255458983510, -6.392944142058904156, 23.31418393918777454 ) ) ;
#42802=CARTESIAN_POINT ( 'NONE',  ( 21.53943276465977519, -0.05219959533907433946, 83.74890960531435269 ) ) ;
#42803=CARTESIAN_POINT ( 'NONE',  ( -10.72451020669898014, 18.67979575497178502, 30.41557627198101699 ) ) ;
#42804=CARTESIAN_POINT ( 'NONE',  ( -19.02544592524342804, 5.153800228976336051, 26.04057627198103120 ) ) ;
#42805=CARTESIAN_POINT ( 'NONE',  ( 0.05219959533934541429, -16.53943276465976808, 55.00109039468568284 ) ) ;
#42807=CARTESIAN_POINT ( 'NONE',  ( -5.719274019375665041, -21.55341960407619695, 34.79275706135235424 ) ) ;
#42808=CARTESIAN_POINT ( 'NONE',  ( 12.14591786802309770, 12.06949235617756955, 49.37390960531436690 ) ) ;
#42810=CARTESIAN_POINT ( 'NONE',  ( -16.53943276465976808, -0.05219959533934237506, 23.75109039468567929 ) ) ;
#42811=CARTESIAN_POINT ( 'NONE',  ( -9.474510206698720793, -16.51473224551083518, 34.58442372801899722 ) ) ;
#42812=CARTESIAN_POINT ( 'NONE',  ( 8.224510206698953496, -14.34966873604960469, 47.91557627198102409 ) ) ;
#42813=CARTESIAN_POINT ( 'NONE',  ( 10.72451020669898902, -18.67979575497178502, 112.9155762719810383 ) ) ;
#42815=CARTESIAN_POINT ( 'NONE',  ( -21.55341960407610458, -5.719274019375992779, 81.45724293864769550 ) ) ;
#42816=CARTESIAN_POINT ( 'NONE',  ( 5.153800228976335163, 19.02544592524342804, 94.79057627198103830 ) ) ;
#42817=CARTESIAN_POINT ( 'NONE',  ( -12.14591786802309592, -12.06949235617757132, 66.87390960531436690 ) ) ;
#42818=CARTESIAN_POINT ( 'NONE',  ( 5.049401038298161559, -19.05341960407611168, 97.70724293864766707 ) ) ;
#42820=CARTESIAN_POINT ( 'NONE',  ( -5.153800228976607833, 19.02544592524334988, 67.70942372801900433 ) ) ;
#42821=CARTESIAN_POINT ( 'NONE',  ( 5.719274019375991003, -21.55341960407610458, 107.7072429386476955 ) ) ;
#42822=CARTESIAN_POINT ( 'NONE',  ( 19.02544592524343514, -5.153800228976328945, 58.54057627198102409 ) ) ;
#42823=CARTESIAN_POINT ( 'NONE',  ( -5.153800228976328057, -19.02544592524343514, 22.29057627198102765 ) ) ;
#42824=CARTESIAN_POINT ( 'NONE',  ( 21.52544592524334988, 5.823673210054432836, 46.45942372801901854 ) ) ;
#42826=CARTESIAN_POINT ( 'NONE',  ( -14.29746914071049879, 8.314922557960819915, 35.83224293864768839 ) ) ;
#42827=CARTESIAN_POINT ( 'NONE',  ( 5.049401038298161559, -19.05341960407611168, 47.70724293864770260 ) ) ;
#42828=CARTESIAN_POINT ( 'NONE',  ( -9.564922557960796823, -16.46253265017161027, 102.0822429386477097 ) ) ;
#42829=CARTESIAN_POINT ( 'NONE',  ( 18.62759615963271287, -10.81492255796078972, 78.33224293864770971 ) ) ;
#42831=CARTESIAN_POINT ( 'NONE',  ( -0.05219959533909027116, -19.03943276465977164, 42.49890960531435269 ) ) ;
#42833=CARTESIAN_POINT ( 'NONE',  ( 5.823673210054125526, 21.52544592524343514, 64.79057627198103830 ) ) ;
#42834=CARTESIAN_POINT ( 'NONE',  ( -21.53943276465977519, -0.05219959533937600094, 88.75109039468567573 ) ) ;
#42836=CARTESIAN_POINT ( 'NONE',  ( 16.55341960407618274, -4.379528057220086978, 86.04275706135236135 ) ) ;
#42837=CARTESIAN_POINT ( 'NONE',  ( 14.29746914071049879, -8.314922557960816363, 83.33224293864769550 ) ) ;
#42838=CARTESIAN_POINT ( 'NONE',  ( -9.474510206698964154, 16.51473224551069663, 70.41557627198102409 ) ) ;
#42840=CARTESIAN_POINT ( 'NONE',  ( 16.46253265017146816, 9.564922557961045513, 36.66775706135233293 ) ) ;
#42841=CARTESIAN_POINT ( 'NONE',  ( 8.314922557961029526, -14.29746914071037800, 90.41775706135236135 ) ) ;
#42842=CARTESIAN_POINT ( 'NONE',  ( -15.72974639402176322, -15.80617190586768395, 109.3760903946857042 ) ) ;
#42843=CARTESIAN_POINT ( 'NONE',  ( -13.97604488694527625, -13.89961937509977652, 91.87390960531432427 ) ) ;
#42844=CARTESIAN_POINT ( 'NONE',  ( -15.72974639402197994, 15.80617190586746368, 50.62390960531435979 ) ) ;
#42845=CARTESIAN_POINT ( 'NONE',  ( -5.823673210054431948, 21.52544592524334988, 92.70942372801901854 ) ) ;
#42846=CARTESIAN_POINT ( 'NONE',  ( -8.314922557961024197, 14.29746914071037800, 57.91775706135234714 ) ) ;
#42847=CARTESIAN_POINT ( 'NONE',  ( 18.67979575497194134, -10.72451020669871369, 20.83442372801901143 ) ) ;
#42848=CARTESIAN_POINT ( 'NONE',  ( 8.314922557961029526, -14.29746914071037800, 25.41775706135235779 ) ) ;
#42849=CARTESIAN_POINT ( 'NONE',  ( -13.97604488694527625, -13.89961937509977652, 86.87390960531436690 ) ) ;
#42850=CARTESIAN_POINT ( 'NONE',  ( -8.314922557961024197, 14.29746914071037800, 27.91775706135234358 ) ) ;
#42851=CARTESIAN_POINT ( 'NONE',  ( -9.474510206698964154, 16.51473224551069663, 50.41557627198102409 ) ) ;
#42852=CARTESIAN_POINT ( 'NONE',  ( -8.224510206698735004, -14.34966873604973081, 34.58442372801900433 ) ) ;
#42853=CARTESIAN_POINT ( 'NONE',  ( -8.224510206698948167, 14.34966873604960824, 80.41557627198103830 ) ) ;
#42854=CARTESIAN_POINT ( 'NONE',  ( -12.14591786802326823, 12.06949235617739902, 88.12609039468570415 ) ) ;
#42855=CARTESIAN_POINT ( 'NONE',  ( -18.67979575497193778, 10.72451020669871902, 43.33442372801901143 ) ) ;
#42856=CARTESIAN_POINT ( 'NONE',  ( 9.564922557960805705, 16.46253265017160317, 64.58224293864769550 ) ) ;
#42857=CARTESIAN_POINT ( 'NONE',  ( 19.02544592524343514, -5.153800228976328945, 83.54057627198100988 ) ) ;
#42858=CARTESIAN_POINT ( 'NONE',  ( 0.05219959533910956823, 16.53943276465976808, 29.99890960531435979 ) ) ;
#42859=CARTESIAN_POINT ( 'NONE',  ( 8.314922557961029526, -14.29746914071037800, 85.41775706135236135 ) ) ;
#42861=CARTESIAN_POINT ( 'NONE',  ( 0.05219959533936267826, -19.03943276465977164, 25.00109039468566152 ) ) ;
#42862=CARTESIAN_POINT ( 'NONE',  ( 9.564922557960805705, 16.46253265017160317, 94.58224293864769550 ) ) ;
#42864=CARTESIAN_POINT ( 'NONE',  ( 9.474510206698971260, -16.51473224551069308, 42.91557627198103120 ) ) ;
#42865=CARTESIAN_POINT ( 'NONE',  ( 0.05219959533909260263, 19.03943276465977164, 114.9989096053143669 ) ) ;
#42866=CARTESIAN_POINT ( 'NONE',  ( 8.224510206698742110, 14.34966873604972548, 42.08442372801901854 ) ) ;
#42867=CARTESIAN_POINT ( 'NONE',  ( 19.05341960407617918, -5.049401038297876454, 71.04275706135234714 ) ) ;
#42868=CARTESIAN_POINT ( 'NONE',  ( 14.29746914071037800, 8.314922557961029526, 56.66775706135235424 ) ) ;
#42870=CARTESIAN_POINT ( 'NONE',  ( 19.05341960407611168, 5.049401038298154454, 83.95724293864766707 ) ) ;
#42871=CARTESIAN_POINT ( 'NONE',  ( 5.823673210054125526, 21.52544592524343514, 109.7905762719810383 ) ) ;
#42872=CARTESIAN_POINT ( 'NONE',  ( 16.46253265017146816, 9.564922557961045513, 66.66775706135233293 ) ) ;
#42873=CARTESIAN_POINT ( 'NONE',  ( -16.46253265017160317, 9.564922557960807481, 110.8322429386476955 ) ) ;
#42875=CARTESIAN_POINT ( 'NONE',  ( -5.153800228976328057, -19.02544592524343514, 72.29057627198102409 ) ) ;
#42876=CARTESIAN_POINT ( 'NONE',  ( -12.06949235617756955, 12.14591786802309770, 35.62390960531437401 ) ) ;
#42877=FACE_OUTER_BOUND ( 'NONE', #77092, .T. ) ;
#42878=CARTESIAN_POINT ( 'NONE',  ( 9.474510206698729675, 16.51473224551082808, 32.08442372801900433 ) ) ;
#42879=CARTESIAN_POINT ( 'NONE',  ( -4.379528057220328563, 16.55341960407611168, 80.20724293864769550 ) ) ;
#42880=CARTESIAN_POINT ( 'NONE',  ( 15.80617190586769283, -15.72974639402175789, 110.6260903946857042 ) ) ;
#42881=CARTESIAN_POINT ( 'NONE',  ( -19.02544592524342804, 5.153800228976336051, 51.04057627198103120 ) ) ;
#42882=CARTESIAN_POINT ( 'NONE',  ( 4.483927247898545687, 16.52544592524342804, 39.79057627198103830 ) ) ;
#42883=CARTESIAN_POINT ( 'NONE',  ( 21.53943276465977519, 0.05219959533937863772, 101.2510903946856757 ) ) ;
#42884=CARTESIAN_POINT ( 'NONE',  ( 16.51473224551069308, 9.474510206698969483, 94.16557627198103830 ) ) ;
#42885=CARTESIAN_POINT ( 'NONE',  ( -9.564922557960796823, -16.46253265017161027, 107.0822429386476955 ) ) ;
#42886=CARTESIAN_POINT ( 'NONE',  ( -5.153800228976328057, -19.02544592524343514, 37.29057627198102409 ) ) ;
#42887=CARTESIAN_POINT ( 'NONE',  ( -8.314922557960811034, -14.29746914071050412, 102.0822429386476955 ) ) ;
#42888=CARTESIAN_POINT ( 'NONE',  ( -12.06949235617756955, 12.14591786802309770, 70.62390960531436690 ) ) ;
#42889=CARTESIAN_POINT ( 'NONE',  ( -10.81492255796078084, -18.62759615963271287, 87.08224293864769550 ) ) ;
#42890=CARTESIAN_POINT ( 'NONE',  ( -19.02544592524342804, 5.153800228976336051, 86.04057627198103830 ) ) ;
#42891=CARTESIAN_POINT ( 'NONE',  ( -21.52544592524343514, 5.823673210054127303, 101.0405762719810383 ) ) ;
#42892=CARTESIAN_POINT ( 'NONE',  ( -9.564922557960796823, -16.46253265017161027, 87.08224293864769550 ) ) ;
#42894=CARTESIAN_POINT ( 'NONE',  ( -16.52544592524342804, 4.483927247898546575, 106.0405762719810525 ) ) ;
#42895=CARTESIAN_POINT ( 'NONE',  ( -5.153800228976328057, -19.02544592524343514, 72.29057627198102409 ) ) ;
#42896=CARTESIAN_POINT ( 'NONE',  ( -15.72974639402197994, 15.80617190586746368, 80.62390960531438111 ) ) ;
#42898=CARTESIAN_POINT ( 'NONE',  ( -0.05219959533907301413, -21.53943276465977519, 32.49890960531435979 ) ) ;
#42900=CARTESIAN_POINT ( 'NONE',  ( 4.379528057220092307, 16.55341960407617563, 27.29275706135234358 ) ) ;
#42901=CARTESIAN_POINT ( 'NONE',  ( -8.224510206698948167, 14.34966873604960824, 90.41557627198103830 ) ) ;
#42902=CARTESIAN_POINT ( 'NONE',  ( -17.72662750342724891, -5.500000000000086153, 46.40179492283740359 ) ) ;
#42903=CARTESIAN_POINT ( 'NONE',  ( 0.05219959533909260263, 19.03943276465977164, 89.99890960531436690 ) ) ;
#42904=CARTESIAN_POINT ( 'NONE',  ( 19.03943276465977164, -0.05219959533909143690, 48.74890960531435979 ) ) ;
#42905=CARTESIAN_POINT ( 'NONE',  ( -16.52544592524342804, 4.483927247898546575, 86.04057627198102409 ) ) ;
#42906=CARTESIAN_POINT ( 'NONE',  ( 0.05219959533907565091, 21.53943276465977519, 24.99890960531435624 ) ) ;
#42907=CARTESIAN_POINT ( 'NONE',  ( -16.53943276465976808, 0.05219959533911058130, 51.24890960531436690 ) ) ;
#42908=CARTESIAN_POINT ( 'NONE',  ( -5.049401038297874678, -19.05341960407617918, 104.7927570613523471 ) ) ;
#42909=CARTESIAN_POINT ( 'NONE',  ( 21.53943276465977519, 0.05219959533937863772, 66.25109039468567573 ) ) ;
#42911=CARTESIAN_POINT ( 'NONE',  ( 19.02544592524343514, -5.153800228976328945, 98.54057627198100988 ) ) ;
#42912=CARTESIAN_POINT ( 'NONE',  ( -8.314922557961024197, 14.29746914071037800, 87.91775706135234714 ) ) ;
#42913=CARTESIAN_POINT ( 'NONE',  ( -19.03943276465977164, 0.05219959533909376836, 31.24890960531435979 ) ) ;
#42914=CARTESIAN_POINT ( 'NONE',  ( -5.153800228976328057, -19.02544592524343514, 77.29057627198099567 ) ) ;
#42915=CARTESIAN_POINT ( 'NONE',  ( -21.53943276465977519, 0.05219959533907696930, 81.24890960531436690 ) ) ;
#42916=CARTESIAN_POINT ( 'NONE',  ( -12.06949235617739369, -12.14591786802326823, 19.37609039468568639 ) ) ;
#42918=CARTESIAN_POINT ( 'NONE',  ( 4.483927247898545687, 16.52544592524342804, 49.79057627198102409 ) ) ;
#42919=CARTESIAN_POINT ( 'NONE',  ( 10.81492255796106328, -18.62759615963255655, 55.41775706135234714 ) ) ;
#42920=CARTESIAN_POINT ( 'NONE',  ( 8.314922557961029526, -14.29746914071037800, 80.41775706135234714 ) ) ;
#42921=CARTESIAN_POINT ( 'NONE',  ( -5.823673210054116645, -21.52544592524344225, 22.29057627198102765 ) ) ;
#42922=CARTESIAN_POINT ( 'NONE',  ( -9.474510206698964154, 16.51473224551069663, 115.4155762719810241 ) ) ;
#42924=CARTESIAN_POINT ( 'NONE',  ( -4.483927247898782831, 16.52544592524335698, 112.7094237280190328 ) ) ;
#42925=CARTESIAN_POINT ( 'NONE',  ( -12.14591786802326823, 12.06949235617739902, 58.12609039468568994 ) ) ;
#42926=CARTESIAN_POINT ( 'NONE',  ( -13.97604488694527625, -13.89961937509977652, 71.87390960531433848 ) ) ;
#42927=CARTESIAN_POINT ( 'NONE',  ( -5.049401038298153566, 19.05341960407611168, 75.20724293864769550 ) ) ;
#42928=CARTESIAN_POINT ( 'NONE',  ( 21.53943276465977519, 0.05219959533937863772, 76.25109039468568994 ) ) ;
#42929=CARTESIAN_POINT ( 'NONE',  ( -12.14591786802326823, 12.06949235617739902, 78.12609039468570415 ) ) ;
#42930=CARTESIAN_POINT ( 'NONE',  ( 14.29746914071049879, -8.314922557960816363, 53.33224293864769550 ) ) ;
#42931=CARTESIAN_POINT ( 'NONE',  ( -5.049401038298153566, 19.05341960407611168, 55.20724293864769550 ) ) ;
#42932=CARTESIAN_POINT ( 'NONE',  ( -5.153800228976328057, -19.02544592524343514, 47.29057627198102409 ) ) ;
#42933=CARTESIAN_POINT ( 'NONE',  ( 12.06949235617739724, 12.14591786802326823, 36.87609039468568994 ) ) ;
#42934=ORIENTED_EDGE ( 'NONE', *, *, #70410, .F. ) ;
#42935=CARTESIAN_POINT ( 'NONE',  ( 0.05219959533936267826, -19.03943276465977164, 100.0010903946856757 ) ) ;
#42936=CARTESIAN_POINT ( 'NONE',  ( -8.314922557960811034, -14.29746914071050412, 92.08224293864769550 ) ) ;
#42937=CARTESIAN_POINT ( 'NONE',  ( -19.03943276465977164, 0.05219959533909376836, 66.24890960531436690 ) ) ;
#42938=CARTESIAN_POINT ( 'NONE',  ( -5.049401038297874678, -19.05341960407617918, 99.79275706135234714 ) ) ;
#42940=CARTESIAN_POINT ( 'NONE',  ( 15.80617190586769283, -15.72974639402175789, 100.6260903946857184 ) ) ;
#42941=CARTESIAN_POINT ( 'NONE',  ( -12.06949235617739369, -12.14591786802326823, 64.37609039468568994 ) ) ;
#42942=DIRECTION ( 'NONE',  ( -0.000000000000000000, 1.000000000000000000, 0.000000000000000000 ) ) ;
#42943=CARTESIAN_POINT ( 'NONE',  ( 0.05219959533907565091, 21.53943276465977519, 64.99890960531435269 ) ) ;
#42944=CARTESIAN_POINT ( 'NONE',  ( -8.314922557961024197, 14.29746914071037800, 52.91775706135235424 ) ) ;
#42946=CARTESIAN_POINT ( 'NONE',  ( -9.474510206698720793, -16.51473224551083518, 44.58442372801900433 ) ) ;
#42947=CARTESIAN_POINT ( 'NONE',  ( 19.03943276465977164, -0.05219959533909143690, 83.74890960531436690 ) ) ;
#42948=CARTESIAN_POINT ( 'NONE',  ( -16.51473224551069308, -9.474510206698971260, 21.66557627198102765 ) ) ;
#42949=CARTESIAN_POINT ( 'NONE',  ( -16.46253265017160317, 9.564922557960807481, 70.83224293864770971 ) ) ;
#42950=CARTESIAN_POINT ( 'NONE',  ( 15.80617190586769283, -15.72974639402175789, 70.62609039468567573 ) ) ;
#42951=CARTESIAN_POINT ( 'NONE',  ( 13.97604488694548053, -13.89961937509957401, 40.62609039468564731 ) ) ;
#42952=CARTESIAN_POINT ( 'NONE',  ( 9.474510206698729675, 16.51473224551082808, 27.08442372801900433 ) ) ;
#42953=CARTESIAN_POINT ( 'NONE',  ( -0.05219959533909027116, -19.03943276465977164, 57.49890960531435979 ) ) ;
#42954=CARTESIAN_POINT ( 'NONE',  ( 9.564922557960805705, 16.46253265017160317, 114.5822429386476955 ) ) ;
#42955=CARTESIAN_POINT ( 'NONE',  ( 5.823673210054444382, -21.52544592524334988, 80.20942372801901854 ) ) ;
#42956=CARTESIAN_POINT ( 'NONE',  ( 5.153800228976335163, 19.02544592524342804, 64.79057627198100988 ) ) ;
#42958=CARTESIAN_POINT ( 'NONE',  ( -10.72451020669870658, -18.67979575497194134, 99.58442372801900433 ) ) ;
#42959=CARTESIAN_POINT ( 'NONE',  ( 15.72974639402199770, -15.80617190586745480, 38.12390960531436690 ) ) ;
#42960=CARTESIAN_POINT ( 'NONE',  ( 13.97604488694527802, 13.89961937509977652, 84.37390960531433848 ) ) ;
#42961=CARTESIAN_POINT ( 'NONE',  ( 5.719274019375673035, 21.55341960407619339, 42.29275706135235424 ) ) ;
#42962=CARTESIAN_POINT ( 'NONE',  ( 19.05341960407617918, -5.049401038297876454, 61.04275706135232582 ) ) ;
#42963=CARTESIAN_POINT ( 'NONE',  ( 0.05219959533909260263, 19.03943276465977164, 39.99890960531436690 ) ) ;
#42964=CARTESIAN_POINT ( 'NONE',  ( 5.049401038298161559, -19.05341960407611168, 92.70724293864769550 ) ) ;
#42965=CARTESIAN_POINT ( 'NONE',  ( 16.53943276465976808, 0.05219959533934440121, 26.25109039468567573 ) ) ;
#42966=CARTESIAN_POINT ( 'NONE',  ( -4.379528057220328563, 16.55341960407611168, 85.20724293864770971 ) ) ;
#42967=CARTESIAN_POINT ( 'NONE',  ( -5.049401038298153566, 19.05341960407611168, 65.20724293864765286 ) ) ;
#42968=CARTESIAN_POINT ( 'NONE',  ( 15.80617190586746368, 15.72974639402197994, 54.37390960531435979 ) ) ;
#42969=CARTESIAN_POINT ( 'NONE',  ( 16.55341960407618274, -4.379528057220086978, 21.04275706135234714 ) ) ;
#42970=CARTESIAN_POINT ( 'NONE',  ( 21.53943276465977519, -0.05219959533907433946, 113.7489096053143527 ) ) ;
#42971=CARTESIAN_POINT ( 'NONE',  ( 18.62759615963255655, 10.81492255796105972, 66.66775706135234714 ) ) ;
#42972=CARTESIAN_POINT ( 'NONE',  ( 0.05219959533934541429, -16.53943276465976808, 75.00109039468568994 ) ) ;
#42973=CARTESIAN_POINT ( 'NONE',  ( -14.29746914071037622, -8.314922557961029526, 64.16775706135234714 ) ) ;
#42974=CARTESIAN_POINT ( 'NONE',  ( -5.049401038298153566, 19.05341960407611168, 65.20724293864765286 ) ) ;
#42975=CARTESIAN_POINT ( 'NONE',  ( 12.06949235617739724, 12.14591786802326823, 96.87609039468568994 ) ) ;
#42976=CARTESIAN_POINT ( 'NONE',  ( -19.03943276465977164, -0.05219959533935918106, 48.75109039468566863 ) ) ;
#42977=CARTESIAN_POINT ( 'NONE',  ( -0.05219959533907301413, -21.53943276465977519, 112.4989096053143669 ) ) ;
#42978=CARTESIAN_POINT ( 'NONE',  ( -12.14591786802309592, -12.06949235617757132, 71.87390960531438111 ) ) ;
#42979=CARTESIAN_POINT ( 'NONE',  ( 5.153800228976335163, 19.02544592524342804, 94.79057627198103830 ) ) ;
#42980=CARTESIAN_POINT ( 'NONE',  ( 0.05219959533934541429, -16.53943276465976808, 95.00109039468568994 ) ) ;
#42981=CARTESIAN_POINT ( 'NONE',  ( -15.80617190586768217, 15.72974639402176855, 58.12609039468568994 ) ) ;
#42982=CARTESIAN_POINT ( 'NONE',  ( -8.314922557961024197, 14.29746914071037800, 32.91775706135234714 ) ) ;
#42983=CARTESIAN_POINT ( 'NONE',  ( 10.72451020669871369, 18.67979575497193778, 22.08442372801901143 ) ) ;
#42984=CARTESIAN_POINT ( 'NONE',  ( -8.314922557960811034, -14.29746914071050412, 52.08224293864768839 ) ) ;
#42986=CARTESIAN_POINT ( 'NONE',  ( 15.80617190586746368, 15.72974639402197994, 99.37390960531436690 ) ) ;
#42988=CARTESIAN_POINT ( 'NONE',  ( 16.55341960407611168, 4.379528057220329451, 33.95724293864769550 ) ) ;
#42991=CARTESIAN_POINT ( 'NONE',  ( -10.72451020669898014, 18.67979575497178502, 35.41557627198102409 ) ) ;
#42992=CARTESIAN_POINT ( 'NONE',  ( 18.67979575497194134, -10.72451020669871369, 30.83442372801902209 ) ) ;
#42993=CARTESIAN_POINT ( 'NONE',  ( -16.52544592524342804, 4.483927247898546575, 71.04057627198103830 ) ) ;
#42994=CARTESIAN_POINT ( 'NONE',  ( 15.72974639402199770, -15.80617190586745480, 73.12390960531436690 ) ) ;
#42995=CARTESIAN_POINT ( 'NONE',  ( -16.51473224551069308, -9.474510206698971260, 76.66557627198103830 ) ) ;
#42996=CARTESIAN_POINT ( 'NONE',  ( -13.89961937509977652, 13.97604488694528158, 25.62390960531434558 ) ) ;
#42997=CARTESIAN_POINT ( 'NONE',  ( -5.049401038297874678, -19.05341960407617918, 79.79275706135233293 ) ) ;
#42998=CARTESIAN_POINT ( 'NONE',  ( -15.80617190586745835, -15.72974639402198527, 51.87390960531437401 ) ) ;
#42999=CARTESIAN_POINT ( 'NONE',  ( -19.03943276465977164, 0.05219959533909376836, 61.24890960531436690 ) ) ;
#43000=ORIENTED_EDGE ( 'NONE', *, *, #85306, .F. ) ;
#43001=CARTESIAN_POINT ( 'NONE',  ( 8.314922557961029526, -14.29746914071037800, 40.41775706135234714 ) ) ;
#43002=CARTESIAN_POINT ( 'NONE',  ( -10.72451020669898014, 18.67979575497178502, 110.4155762719810383 ) ) ;
#43003=CARTESIAN_POINT ( 'NONE',  ( 14.29746914071049879, -8.314922557960816363, 43.33224293864769550 ) ) ;
#43004=CARTESIAN_POINT ( 'NONE',  ( -19.02544592524342804, 5.153800228976336051, 101.0405762719810241 ) ) ;
#43005=CARTESIAN_POINT ( 'NONE',  ( 21.52544592524344225, -5.823673210054117533, 78.54057627198103830 ) ) ;
#43006=CARTESIAN_POINT ( 'NONE',  ( 0.05219959533907565091, 21.53943276465977519, 104.9989096053143669 ) ) ;
#43007=CARTESIAN_POINT ( 'NONE',  ( -16.55341960407617563, 4.379528057220093196, 38.54275706135234714 ) ) ;
#43008=CARTESIAN_POINT ( 'NONE',  ( -21.53943276465977519, 0.05219959533907696930, 46.24890960531435979 ) ) ;
#43009=CARTESIAN_POINT ( 'NONE',  ( 10.72451020669871369, 18.67979575497193778, 97.08442372801904696 ) ) ;
#43010=CARTESIAN_POINT ( 'NONE',  ( -9.564922557960796823, -16.46253265017161027, 42.08224293864769550 ) ) ;
#43011=CARTESIAN_POINT ( 'NONE',  ( 16.46253265017160672, -9.564922557960803928, 103.3322429386476955 ) ) ;
#43012=CARTESIAN_POINT ( 'NONE',  ( 5.049401038298161559, -19.05341960407611168, 82.70724293864770971 ) ) ;
#43013=CARTESIAN_POINT ( 'NONE',  ( 17.40805194821984259, -6.112264579160781253, 88.33371272510609629 ) ) ;
#43014=CARTESIAN_POINT ( 'NONE',  ( -5.049401038297874678, -19.05341960407617918, 54.79275706135234003 ) ) ;
#43015=CARTESIAN_POINT ( 'NONE',  ( 10.72451020669871369, 18.67979575497193778, 112.0844237280190185 ) ) ;
#43016=CARTESIAN_POINT ( 'NONE',  ( 21.52544592524344225, -5.823673210054117533, 28.54057627198103120 ) ) ;
#43017=CARTESIAN_POINT ( 'NONE',  ( -14.34966873604972548, 8.224510206698743886, 98.33442372801901854 ) ) ;
#43018=CARTESIAN_POINT ( 'NONE',  ( 9.564922557961047289, -16.46253265017146816, 80.41775706135234714 ) ) ;
#43020=CARTESIAN_POINT ( 'NONE',  ( -19.02544592524334988, -5.153800228976617603, 88.95942372801897591 ) ) ;
#43021=CARTESIAN_POINT ( 'NONE',  ( -9.474510206698720793, -16.51473224551083518, 44.58442372801900433 ) ) ;
#43022=CARTESIAN_POINT ( 'NONE',  ( -16.31925111598457079, -7.325300261831483084, 44.83575461032751264 ) ) ;
#43023=CARTESIAN_POINT ( 'NONE',  ( 19.03943276465977164, -0.05219959533909143690, 43.74890960531435979 ) ) ;
#43024=CARTESIAN_POINT ( 'NONE',  ( -8.224510206698948167, 14.34966873604960824, 55.41557627198102409 ) ) ;
#43026=CARTESIAN_POINT ( 'NONE',  ( 16.51473224551069308, 9.474510206698969483, 29.16557627198103475 ) ) ;
#43027=CARTESIAN_POINT ( 'NONE',  ( -16.52544592524342804, 4.483927247898546575, 36.04057627198102409 ) ) ;
#43029=CARTESIAN_POINT ( 'NONE',  ( -12.06949235617739369, -12.14591786802326823, 109.3760903946857042 ) ) ;
#43030=CARTESIAN_POINT ( 'NONE',  ( 16.51473224551069308, 9.474510206698969483, 54.16557627198103120 ) ) ;
#43031=CARTESIAN_POINT ( 'NONE',  ( 0.05219959533937995610, -21.53943276465977519, 105.0010903946856757 ) ) ;
#43032=CARTESIAN_POINT ( 'NONE',  ( 4.379528057220092307, 16.55341960407617563, 22.29275706135235069 ) ) ;
#43033=CARTESIAN_POINT ( 'NONE',  ( 10.81492255796078972, 18.62759615963270932, 39.58224293864769550 ) ) ;
#43034=CARTESIAN_POINT ( 'NONE',  ( 21.55341960407619695, -5.719274019375665929, 86.04275706135236135 ) ) ;
#43035=CARTESIAN_POINT ( 'NONE',  ( -13.89961937509977652, 13.97604488694528158, 100.6239096053143669 ) ) ;
#43036=CARTESIAN_POINT ( 'NONE',  ( 5.153800228976335163, 19.02544592524342804, 79.79057627198102409 ) ) ;
#43038=CARTESIAN_POINT ( 'NONE',  ( -21.53943276465977519, 0.05219959533907696930, 106.2489096053143811 ) ) ;
#43039=CARTESIAN_POINT ( 'NONE',  ( 12.14591786802309770, 12.06949235617756955, 84.37390960531438111 ) ) ;
#43040=CARTESIAN_POINT ( 'NONE',  ( -5.823673210054116645, -21.52544592524344225, 72.29057627198102409 ) ) ;
#43041=CARTESIAN_POINT ( 'NONE',  ( 19.05341960407611168, 5.049401038298154454, 78.95724293864769550 ) ) ;
#43042=CARTESIAN_POINT ( 'NONE',  ( 10.72451020669898902, -18.67979575497178502, 97.91557627198103830 ) ) ;
#43043=ORIENTED_EDGE ( 'NONE', *, *, #74692, .T. ) ;
#43044=CARTESIAN_POINT ( 'NONE',  ( -19.05341960407611168, -5.049401038298163336, 66.45724293864769550 ) ) ;
#43045=CARTESIAN_POINT ( 'NONE',  ( -14.34966873604960291, -8.224510206698953496, 91.66557627198103830 ) ) ;
#43047=CARTESIAN_POINT ( 'NONE',  ( 19.02544592524343514, -5.153800228976328945, 63.54057627198103830 ) ) ;
#43048=CARTESIAN_POINT ( 'NONE',  ( -16.46253265017146816, -9.564922557961047289, 74.16775706135234714 ) ) ;
#43049=CARTESIAN_POINT ( 'NONE',  ( -16.55341960407611168, -4.379528057220339221, 96.45724293864770971 ) ) ;
#43050=CARTESIAN_POINT ( 'NONE',  ( 21.53943276465977519, 0.05219959533937863772, 56.25109039468568284 ) ) ;
#43051=CARTESIAN_POINT ( 'NONE',  ( 0.05219959533909260263, 19.03943276465977164, 49.99890960531435979 ) ) ;
#43052=CARTESIAN_POINT ( 'NONE',  ( 5.719274019375673035, 21.55341960407619339, 22.29275706135235069 ) ) ;
#43053=CARTESIAN_POINT ( 'NONE',  ( -14.34966873604960291, -8.224510206698953496, 106.6655762719810383 ) ) ;
#43055=CARTESIAN_POINT ( 'NONE',  ( -16.46253265017160317, 9.564922557960807481, 60.83224293864769550 ) ) ;
#43056=CARTESIAN_POINT ( 'NONE',  ( 17.50000000000000355, 5.624438216177583882, 111.6832965508535551 ) ) ;
#43057=CARTESIAN_POINT ( 'NONE',  ( -19.03943276465977164, -0.05219959533935918106, 103.7510903946856757 ) ) ;
#43058=CARTESIAN_POINT ( 'NONE',  ( -16.46253265017160317, 9.564922557960807481, 115.8322429386477097 ) ) ;
#43059=CARTESIAN_POINT ( 'NONE',  ( 21.55341960407619695, -5.719274019375665929, 56.04275706135235424 ) ) ;
#43060=CARTESIAN_POINT ( 'NONE',  ( 0.05219959533909260263, 19.03943276465977164, 94.99890960531436690 ) ) ;
#43061=CARTESIAN_POINT ( 'NONE',  ( -16.51473224551082808, 9.474510206698731452, 83.33442372801899012 ) ) ;
#43062=CARTESIAN_POINT ( 'NONE',  ( 13.89961937509977652, -13.97604488694527269, 58.12390960531436690 ) ) ;
#43063=CARTESIAN_POINT ( 'NONE',  ( -16.55341960407611168, -4.379528057220339221, 81.45724293864769550 ) ) ;
#43064=CARTESIAN_POINT ( 'NONE',  ( -13.89961937509977652, 13.97604488694528158, 85.62390960531433848 ) ) ;
#43065=CARTESIAN_POINT ( 'NONE',  ( 12.06949235617757843, -12.14591786802309237, 83.12390960531436690 ) ) ;
#43066=CARTESIAN_POINT ( 'NONE',  ( 9.564922557960805705, 16.46253265017160317, 84.58224293864769550 ) ) ;
#43067=CARTESIAN_POINT ( 'NONE',  ( -0.05219959533936034679, 19.03943276465977164, 37.50109039468567573 ) ) ;
#43068=CARTESIAN_POINT ( 'NONE',  ( -9.474510206698964154, 16.51473224551069663, 45.41557627198103120 ) ) ;
#43069=CARTESIAN_POINT ( 'NONE',  ( -16.52544592524342804, 4.483927247898546575, 46.04057627198103830 ) ) ;
#43070=CARTESIAN_POINT ( 'NONE',  ( -0.05219959533909027116, -19.03943276465977164, 22.49890960531436690 ) ) ;
#43072=CARTESIAN_POINT ( 'NONE',  ( 5.823673210054444382, -21.52544592524334988, 40.20942372801901854 ) ) ;
#43073=CARTESIAN_POINT ( 'NONE',  ( 0.05219959533936267826, -19.03943276465977164, 80.00109039468567573 ) ) ;
#43074=CARTESIAN_POINT ( 'NONE',  ( 14.34966873604960469, 8.224510206698951720, 29.16557627198103120 ) ) ;
#43075=CARTESIAN_POINT ( 'NONE',  ( -10.81492255796078084, -18.62759615963271287, 92.08224293864769550 ) ) ;
#43076=CARTESIAN_POINT ( 'NONE',  ( -10.81492255796078084, -18.62759615963271287, 37.08224293864768129 ) ) ;
#43077=CARTESIAN_POINT ( 'NONE',  ( -16.52544592524342804, 4.483927247898546575, 66.04057627198103830 ) ) ;
#43078=CARTESIAN_POINT ( 'NONE',  ( 13.89961937509977652, -13.97604488694527269, 43.12390960531434558 ) ) ;
#43079=CARTESIAN_POINT ( 'NONE',  ( -14.29746914071037622, -8.314922557961029526, 104.1677570613523471 ) ) ;
#43080=CARTESIAN_POINT ( 'NONE',  ( 8.224510206698742110, 14.34966873604972548, 77.08442372801901854 ) ) ;
#43081=CARTESIAN_POINT ( 'NONE',  ( -5.719274019375978568, 21.55341960407610458, 35.20724293864768839 ) ) ;
#43082=CARTESIAN_POINT ( 'NONE',  ( 16.46253265017146816, 9.564922557961045513, 21.66775706135233648 ) ) ;
#43083=CARTESIAN_POINT ( 'NONE',  ( 16.51473224551069308, 9.474510206698969483, 94.16557627198103830 ) ) ;
#43084=CARTESIAN_POINT ( 'NONE',  ( -19.03943276465977164, 0.05219959533909376836, 71.24890960531435269 ) ) ;
#43085=CARTESIAN_POINT ( 'NONE',  ( -16.55341960407617563, 4.379528057220093196, 78.54275706135236135 ) ) ;
#43086=CARTESIAN_POINT ( 'NONE',  ( 9.474510206698971260, -16.51473224551069308, 22.91557627198102765 ) ) ;
#43087=CARTESIAN_POINT ( 'NONE',  ( -8.224510206698948167, 14.34966873604960824, 30.41557627198101699 ) ) ;
#43088=CARTESIAN_POINT ( 'NONE',  ( -5.153800228976328057, -19.02544592524343514, 107.2905762719810383 ) ) ;
#43089=CARTESIAN_POINT ( 'NONE',  ( 16.51473224551069308, 9.474510206698969483, 89.16557627198103830 ) ) ;
#43090=CARTESIAN_POINT ( 'NONE',  ( 15.80617190586746368, 15.72974639402197994, 24.37390960531435979 ) ) ;
#43091=CARTESIAN_POINT ( 'NONE',  ( -14.34966873604960291, -8.224510206698953496, 76.66557627198103830 ) ) ;
#43093=CARTESIAN_POINT ( 'NONE',  ( 4.483927247898545687, 16.52544592524342804, 64.79057627198103830 ) ) ;
#43094=CARTESIAN_POINT ( 'NONE',  ( -12.06949235617739369, -12.14591786802326823, 59.37609039468568284 ) ) ;
#43095=CARTESIAN_POINT ( 'NONE',  ( -18.22780087662121673, -5.500000000000063061, 56.48459894673892734 ) ) ;
#43096=CARTESIAN_POINT ( 'NONE',  ( -19.02544592524334988, -5.153800228976617603, 53.95942372801898301 ) ) ;
#43097=CARTESIAN_POINT ( 'NONE',  ( -19.05341960407611168, -5.049401038298163336, 91.45724293864766707 ) ) ;
#43098=CARTESIAN_POINT ( 'NONE',  ( -5.049401038297874678, -19.05341960407617918, 59.79275706135231871 ) ) ;
#43099=B_SPLINE_CURVE_WITH_KNOTS ( 'NONE', 3,
 ( #63653, #5937, #158628, #141483, #49474, #50475 ),
 .UNSPECIFIED., .F., .F.,
 ( 4, 2, 4 ),
 ( 0.007228050697041690613, 0.007608510107495180044, 0.007988969517948670343 ),
 .UNSPECIFIED. ) ;
#43101=CARTESIAN_POINT ( 'NONE',  ( 16.51473224551083163, -9.474510206698727899, 110.8344237280190043 ) ) ;
#43102=CARTESIAN_POINT ( 'NONE',  ( -4.483927247898782831, 16.52544592524335698, 92.70942372801901854 ) ) ;
#43103=CARTESIAN_POINT ( 'NONE',  ( -16.46253265017160317, 9.564922557960807481, 35.83224293864768839 ) ) ;
#43104=CARTESIAN_POINT ( 'NONE',  ( 10.72451020669898902, -18.67979575497178502, 27.91557627198103830 ) ) ;
#43105=CARTESIAN_POINT ( 'NONE',  ( 10.72451020669871369, 18.67979575497193778, 57.08442372801901854 ) ) ;
#43106=CARTESIAN_POINT ( 'NONE',  ( -5.049401038297874678, -19.05341960407617918, 99.79275706135234714 ) ) ;
#43107=CARTESIAN_POINT ( 'NONE',  ( -9.474510206698720793, -16.51473224551083518, 54.58442372801899722 ) ) ;
#43108=CARTESIAN_POINT ( 'NONE',  ( 5.049401038298161559, -19.05341960407611168, 77.70724293864765286 ) ) ;
#43110=CARTESIAN_POINT ( 'NONE',  ( -12.14591786802309592, -12.06949235617757132, 71.87390960531438111 ) ) ;
#43111=CARTESIAN_POINT ( 'NONE',  ( 5.049401038298161559, -19.05341960407611168, 67.70724293864769550 ) ) ;
#43112=CARTESIAN_POINT ( 'NONE',  ( 9.474510206698971260, -16.51473224551069308, 72.91557627198102409 ) ) ;
#43113=CARTESIAN_POINT ( 'NONE',  ( -13.89961937509957401, -13.97604488694547875, 84.37609039468567573 ) ) ;
#43114=CARTESIAN_POINT ( 'NONE',  ( -15.80617190586745835, -15.72974639402198527, 66.87390960531436690 ) ) ;
#43115=CARTESIAN_POINT ( 'NONE',  ( -13.97604488694527625, -13.89961937509977652, 21.87390960531435979 ) ) ;
#43116=CARTESIAN_POINT ( 'NONE',  ( -16.46253265017146816, -9.564922557961047289, 59.16775706135233293 ) ) ;
#43117=CARTESIAN_POINT ( 'NONE',  ( 13.89961937509977652, -13.97604488694527269, 58.12390960531436690 ) ) ;
#43118=CARTESIAN_POINT ( 'NONE',  ( 5.049401038298161559, -19.05341960407611168, 92.70724293864769550 ) ) ;
#43119=CARTESIAN_POINT ( 'NONE',  ( -15.80617190586745835, -15.72974639402198527, 86.87390960531438111 ) ) ;
#43120=CARTESIAN_POINT ( 'NONE',  ( 12.14591786802309770, 12.06949235617756955, 74.37390960531436690 ) ) ;
#43121=CARTESIAN_POINT ( 'NONE',  ( -13.97604488694547697, 13.89961937509957934, 48.12609039468566863 ) ) ;
#43122=CARTESIAN_POINT ( 'NONE',  ( 10.72451020669898902, -18.67979575497178502, 82.91557627198103830 ) ) ;
#43123=CARTESIAN_POINT ( 'NONE',  ( -21.52544592524343514, 5.823673210054127303, 66.04057627198103830 ) ) ;
#43124=CARTESIAN_POINT ( 'NONE',  ( 4.379528057220339221, -16.55341960407611168, 37.70724293864769550 ) ) ;
#43125=CARTESIAN_POINT ( 'NONE',  ( -15.72974639402176322, -15.80617190586768395, 99.37609039468568994 ) ) ;
#43126=CARTESIAN_POINT ( 'NONE',  ( -13.97604488694527625, -13.89961937509977652, 76.87390960531433848 ) ) ;
#43127=CARTESIAN_POINT ( 'NONE',  ( 16.46253265017160672, -9.564922557960803928, 38.33224293864768839 ) ) ;
#43128=CARTESIAN_POINT ( 'NONE',  ( -5.823673210054431948, 21.52544592524334988, 37.70942372801900433 ) ) ;
#43129=CARTESIAN_POINT ( 'NONE',  ( 18.67979575497194134, -10.72451020669871369, 40.83442372801901854 ) ) ;
#43130=CARTESIAN_POINT ( 'NONE',  ( -19.05341960407611168, -5.049401038298163336, 46.45724293864768129 ) ) ;
#43131=CARTESIAN_POINT ( 'NONE',  ( -0.05219959533937732626, 21.53943276465977519, 27.50109039468567929 ) ) ;
#43132=CARTESIAN_POINT ( 'NONE',  ( -19.03943276465977164, -0.05219959533935918106, 63.75109039468566863 ) ) ;
#43133=CARTESIAN_POINT ( 'NONE',  ( -19.02544592524342804, 5.153800228976336051, 36.04057627198100988 ) ) ;
#43134=CARTESIAN_POINT ( 'NONE',  ( 8.224510206698742110, 14.34966873604972548, 27.08442372801901854 ) ) ;
#43135=CARTESIAN_POINT ( 'NONE',  ( -19.05341960407611168, -5.049401038298163336, 21.45724293864768839 ) ) ;
#43136=CARTESIAN_POINT ( 'NONE',  ( -14.34966873604972548, 8.224510206698743886, 73.33442372801901854 ) ) ;
#43137=CARTESIAN_POINT ( 'NONE',  ( 16.46253265017160672, -9.564922557960803928, 38.33224293864768839 ) ) ;
#43139=CARTESIAN_POINT ( 'NONE',  ( -9.564922557960796823, -16.46253265017161027, 92.08224293864769550 ) ) ;
#43140=CARTESIAN_POINT ( 'NONE',  ( -16.51473224551069308, -9.474510206698971260, 21.66557627198102765 ) ) ;
#43141=CARTESIAN_POINT ( 'NONE',  ( -10.72451020669898014, 18.67979575497178502, 65.41557627198102409 ) ) ;
#43142=CARTESIAN_POINT ( 'NONE',  ( -16.55341960407617563, 4.379528057220093196, 48.54275706135234714 ) ) ;
#43143=CARTESIAN_POINT ( 'NONE',  ( -21.53943276465977519, -0.05219959533937600094, 103.7510903946857042 ) ) ;
#43144=CARTESIAN_POINT ( 'NONE',  ( 9.564922557960805705, 16.46253265017160317, 34.58224293864770260 ) ) ;
#43145=CARTESIAN_POINT ( 'NONE',  ( 16.55341960407611168, 4.379528057220329451, 33.95724293864769550 ) ) ;
#43146=CARTESIAN_POINT ( 'NONE',  ( -4.483927247898539470, -16.52544592524342804, 67.29057627198103830 ) ) ;
#43147=CARTESIAN_POINT ( 'NONE',  ( 19.05341960407611168, 5.049401038298154454, 58.95724293864768129 ) ) ;
#43148=CARTESIAN_POINT ( 'NONE',  ( 0.05219959533936267826, -19.03943276465977164, 20.00109039468567218 ) ) ;
#43149=CARTESIAN_POINT ( 'NONE',  ( -10.72451020669870658, -18.67979575497194134, 24.58442372801901499 ) ) ;
#43150=CARTESIAN_POINT ( 'NONE',  ( -19.03943276465977164, 0.05219959533909376836, 81.24890960531436690 ) ) ;
#43152=CARTESIAN_POINT ( 'NONE',  ( -15.80617190586768217, 15.72974639402176855, 88.12609039468570415 ) ) ;
#43153=CARTESIAN_POINT ( 'NONE',  ( 4.379528057220092307, 16.55341960407617563, 57.29275706135234714 ) ) ;
#43154=CARTESIAN_POINT ( 'NONE',  ( 4.379528057220092307, 16.55341960407617563, 32.29275706135235424 ) ) ;
#43156=CARTESIAN_POINT ( 'NONE',  ( 14.29746914071049879, -8.314922557960816363, 88.33224293864769550 ) ) ;
#43157=CARTESIAN_POINT ( 'NONE',  ( -15.80617190586768217, 15.72974639402176855, 98.12609039468570415 ) ) ;
#43158=CARTESIAN_POINT ( 'NONE',  ( -4.379528057220328563, 16.55341960407611168, 35.20724293864768839 ) ) ;
#43159=CARTESIAN_POINT ( 'NONE',  ( -9.474510206698964154, 16.51473224551069663, 25.41557627198103120 ) ) ;
#43160=CARTESIAN_POINT ( 'NONE',  ( -12.14591786802326823, 12.06949235617739902, 58.12609039468568994 ) ) ;
#43161=CARTESIAN_POINT ( 'NONE',  ( 4.483927247898545687, 16.52544592524342804, 59.79057627198103120 ) ) ;
#43162=CARTESIAN_POINT ( 'NONE',  ( -16.55341960407617563, 4.379528057220093196, 103.5427570613523613 ) ) ;
#43163=CARTESIAN_POINT ( 'NONE',  ( 13.97604488694527802, 13.89961937509977652, 109.3739096053143669 ) ) ;
#43164=CARTESIAN_POINT ( 'NONE',  ( 5.823673210054125526, 21.52544592524343514, 34.79057627198103120 ) ) ;
#43165=CARTESIAN_POINT ( 'NONE',  ( 10.72451020669871369, 18.67979575497193778, 112.0844237280190185 ) ) ;
#43166=CARTESIAN_POINT ( 'NONE',  ( -4.379528057220328563, 16.55341960407611168, 80.20724293864769550 ) ) ;
#43167=CARTESIAN_POINT ( 'NONE',  ( -5.049401038298153566, 19.05341960407611168, 95.20724293864770971 ) ) ;
#43168=ORIENTED_EDGE ( 'NONE', *, *, #157696, .F. ) ;
#43169=CARTESIAN_POINT ( 'NONE',  ( 16.52544592524335698, 4.483927247898782831, 46.45942372801901854 ) ) ;
#43170=CARTESIAN_POINT ( 'NONE',  ( -13.89961937509977652, 13.97604488694528158, 35.62390960531435269 ) ) ;
#43171=CARTESIAN_POINT ( 'NONE',  ( -4.483927247898782831, 16.52544592524335698, 47.70942372801902565 ) ) ;
#43172=CARTESIAN_POINT ( 'NONE',  ( -13.89961937509957401, -13.97604488694547875, 49.37609039468567573 ) ) ;
#43173=CARTESIAN_POINT ( 'NONE',  ( 0.05219959533909260263, 19.03943276465977164, 44.99890960531435979 ) ) ;
#43174=CARTESIAN_POINT ( 'NONE',  ( -8.224510206698735004, -14.34966873604973081, 84.58442372801903275 ) ) ;
#43175=CARTESIAN_POINT ( 'NONE',  ( 9.474510206698729675, 16.51473224551082808, 77.08442372801900433 ) ) ;
#43176=CARTESIAN_POINT ( 'NONE',  ( 9.564922557961047289, -16.46253265017146816, 35.41775706135233293 ) ) ;
#43177=CARTESIAN_POINT ( 'NONE',  ( -16.46253265017160317, 9.564922557960807481, 60.83224293864769550 ) ) ;
#43178=CARTESIAN_POINT ( 'NONE',  ( -0.05219959533910754901, -16.53943276465976808, 92.49890960531436690 ) ) ;
#43179=CARTESIAN_POINT ( 'NONE',  ( 16.51473224551083163, -9.474510206698727899, 65.83442372801900433 ) ) ;
#43180=CARTESIAN_POINT ( 'NONE',  ( 21.53943276465977519, -0.05219959533907433946, 68.74890960531435269 ) ) ;
#43181=CARTESIAN_POINT ( 'NONE',  ( -13.89961937509957401, -13.97604488694547875, 44.37609039468566863 ) ) ;
#43182=CARTESIAN_POINT ( 'NONE',  ( 16.51473224551069308, 9.474510206698969483, 99.16557627198102409 ) ) ;
#43183=CARTESIAN_POINT ( 'NONE',  ( 18.62759615963271287, -10.81492255796078972, 73.33224293864769550 ) ) ;
#43184=CARTESIAN_POINT ( 'NONE',  ( -16.38665767535055195, 7.295008042176048590, 85.26400864214548392 ) ) ;
#43185=CARTESIAN_POINT ( 'NONE',  ( 9.564922557961047289, -16.46253265017146816, 105.4177570613523471 ) ) ;
#43186=CARTESIAN_POINT ( 'NONE',  ( 18.22780087662123805, 5.499999999999960032, 96.48236817873105053 ) ) ;
#43187=CARTESIAN_POINT ( 'NONE',  ( 16.52544592524335698, 4.483927247898782831, 31.45942372801901854 ) ) ;
#43188=CARTESIAN_POINT ( 'NONE',  ( 5.049401038298161559, -19.05341960407611168, 37.70724293864768839 ) ) ;
#43189=CARTESIAN_POINT ( 'NONE',  ( 19.05341960407611168, 5.049401038298154454, 113.9572429386477097 ) ) ;
#43190=CARTESIAN_POINT ( 'NONE',  ( -10.72451020669898014, 18.67979575497178502, 85.41557627198102409 ) ) ;
#43191=CARTESIAN_POINT ( 'NONE',  ( 10.81492255796106328, -18.62759615963255655, 55.41775706135234714 ) ) ;
#43193=CARTESIAN_POINT ( 'NONE',  ( 5.049401038297881783, 19.05341960407617563, 102.2927570613523045 ) ) ;
#43194=CARTESIAN_POINT ( 'NONE',  ( 19.03943276465977164, 0.05219959533936151252, 21.25109039468565797 ) ) ;
#43195=CARTESIAN_POINT ( 'NONE',  ( 8.224510206698742110, 14.34966873604972548, 107.0844237280190043 ) ) ;
#43196=EDGE_CURVE ( 'NONE', #85848, #1176, #104262, .T. ) ;
#43197=CARTESIAN_POINT ( 'NONE',  ( -21.52544592524343514, 5.823673210054127303, 101.0405762719810383 ) ) ;
#43198=CARTESIAN_POINT ( 'NONE',  ( -8.224510206698948167, 14.34966873604960824, 45.41557627198103830 ) ) ;
#43199=CARTESIAN_POINT ( 'NONE',  ( 5.049401038297881783, 19.05341960407617563, 77.29275706135231871 ) ) ;
#43200=CARTESIAN_POINT ( 'NONE',  ( -9.564922557961040184, 16.46253265017147172, 52.91775706135233293 ) ) ;
#43201=CARTESIAN_POINT ( 'NONE',  ( 18.62759615963255655, 10.81492255796105972, 71.66775706135234714 ) ) ;
#43202=CARTESIAN_POINT ( 'NONE',  ( 16.46253265017146816, 9.564922557961045513, 36.66775706135233293 ) ) ;
#43203=CARTESIAN_POINT ( 'NONE',  ( 4.483927247898545687, 16.52544592524342804, 104.7905762719810241 ) ) ;
#43204=CARTESIAN_POINT ( 'NONE',  ( -15.72974639402197994, 15.80617190586746368, 50.62390960531435979 ) ) ;
#43205=CARTESIAN_POINT ( 'NONE',  ( -4.379528057220328563, 16.55341960407611168, 30.20724293864769550 ) ) ;
#43206=CARTESIAN_POINT ( 'NONE',  ( 19.03943276465977164, 0.05219959533936151252, 21.25109039468565797 ) ) ;
#43207=CARTESIAN_POINT ( 'NONE',  ( -12.06949235617739369, -12.14591786802326823, 74.37609039468568994 ) ) ;
#43208=CARTESIAN_POINT ( 'NONE',  ( 4.483927247898545687, 16.52544592524342804, 24.79057627198103120 ) ) ;
#43209=CARTESIAN_POINT ( 'NONE',  ( -18.67979575497193778, 10.72451020669871902, 63.33442372801900433 ) ) ;
#43210=CARTESIAN_POINT ( 'NONE',  ( 15.80617190586769283, -15.72974639402175789, 65.62609039468568994 ) ) ;
#43211=CARTESIAN_POINT ( 'NONE',  ( -15.72974639402197994, 15.80617190586746368, 70.62390960531436690 ) ) ;
#43212=VERTEX_POINT ( 'NONE', #110393 ) ;
#43213=CARTESIAN_POINT ( 'NONE',  ( -16.51473224551069308, -9.474510206698971260, 26.66557627198103120 ) ) ;
#43214=CARTESIAN_POINT ( 'NONE',  ( 10.72451020669871369, 18.67979575497193778, 47.08442372801901854 ) ) ;
#43215=CARTESIAN_POINT ( 'NONE',  ( -16.46253265017160317, 9.564922557960807481, 25.83224293864769194 ) ) ;
#43216=CARTESIAN_POINT ( 'NONE',  ( -0.05219959533909027116, -19.03943276465977164, 42.49890960531435269 ) ) ;
#43217=CARTESIAN_POINT ( 'NONE',  ( -12.14591786802309592, -12.06949235617757132, 76.87390960531439532 ) ) ;
#43218=CARTESIAN_POINT ( 'NONE',  ( 9.564922557960805705, 16.46253265017160317, 84.58224293864769550 ) ) ;
#43219=CARTESIAN_POINT ( 'NONE',  ( 0.05219959533910956823, 16.53943276465976808, 24.99890960531435624 ) ) ;
#43220=CARTESIAN_POINT ( 'NONE',  ( -8.314922557960811034, -14.29746914071050412, 102.0822429386476955 ) ) ;
#43221=CARTESIAN_POINT ( 'NONE',  ( 21.55341960407610458, 5.719274019375980345, 68.95724293864769550 ) ) ;
#43222=CARTESIAN_POINT ( 'NONE',  ( 10.72451020669898902, -18.67979575497178502, 102.9155762719810383 ) ) ;
#43223=CARTESIAN_POINT ( 'NONE',  ( -0.05219959533909027116, -19.03943276465977164, 112.4989096053143669 ) ) ;
#43224=EDGE_CURVE ( 'NONE', #104654, #86900, #38444, .T. ) ;
#43225=CARTESIAN_POINT ( 'NONE',  ( 13.97604488694527802, 13.89961937509977652, 69.37390960531436690 ) ) ;
#43226=CARTESIAN_POINT ( 'NONE',  ( 4.483927247898790824, -16.52544592524335698, 20.20942372801900788 ) ) ;
#43227=CARTESIAN_POINT ( 'NONE',  ( 18.62759615963271287, -10.81492255796078972, 53.33224293864769550 ) ) ;
#43228=CARTESIAN_POINT ( 'NONE',  ( -10.72451020669870658, -18.67979575497194134, 79.58442372801903275 ) ) ;
#43229=CARTESIAN_POINT ( 'NONE',  ( 5.153800228976335163, 19.02544592524342804, 84.79057627198099567 ) ) ;
#43231=CARTESIAN_POINT ( 'NONE',  ( -18.67979575497178146, -10.72451020669898902, 21.66557627198102409 ) ) ;
#43232=CARTESIAN_POINT ( 'NONE',  ( -14.34966873604972548, 8.224510206698743886, 78.33442372801901854 ) ) ;
#43233=CARTESIAN_POINT ( 'NONE',  ( 5.719274019375673035, 21.55341960407619339, 52.29275706135236135 ) ) ;
#43234=CARTESIAN_POINT ( 'NONE',  ( -18.62759615963255300, -10.81492255796106328, 99.16775706135234714 ) ) ;
#43235=CARTESIAN_POINT ( 'NONE',  ( 16.55341960407618274, -4.379528057220086978, 66.04275706135236135 ) ) ;
#43236=CARTESIAN_POINT ( 'NONE',  ( 21.53943276465977519, -0.05219959533907433946, 108.7489096053143669 ) ) ;
#43237=CARTESIAN_POINT ( 'NONE',  ( -19.03943276465977164, 0.05219959533909376836, 116.2489096053143669 ) ) ;
#43238=CARTESIAN_POINT ( 'NONE',  ( 5.719274019375991003, -21.55341960407610458, 87.70724293864769550 ) ) ;
#43239=CARTESIAN_POINT ( 'NONE',  ( -5.153800228976607833, 19.02544592524334988, 52.70942372801900433 ) ) ;
#43240=CARTESIAN_POINT ( 'NONE',  ( 10.72451020669898902, -18.67979575497178502, 42.91557627198103120 ) ) ;
#43241=CARTESIAN_POINT ( 'NONE',  ( 0.05219959533909260263, 19.03943276465977164, 94.99890960531436690 ) ) ;
#43242=CARTESIAN_POINT ( 'NONE',  ( 16.53943276465976808, -0.05219959533910856209, 38.74890960531435979 ) ) ;
#43243=CARTESIAN_POINT ( 'NONE',  ( -16.62475595723697452, 7.163666690055237041, 65.52713351810467657 ) ) ;
#43245=CARTESIAN_POINT ( 'NONE',  ( -13.89961937509957401, -13.97604488694547875, 99.37609039468567573 ) ) ;
#43246=CARTESIAN_POINT ( 'NONE',  ( -5.823673210054116645, -21.52544592524344225, 77.29057627198102409 ) ) ;
#43247=CARTESIAN_POINT ( 'NONE',  ( -14.34966873604960291, -8.224510206698953496, 51.66557627198102409 ) ) ;
#43248=CARTESIAN_POINT ( 'NONE',  ( 16.53943276465976808, 0.05219959533934440121, 36.25109039468567573 ) ) ;
#43249=CARTESIAN_POINT ( 'NONE',  ( 5.049401038298161559, -19.05341960407611168, 42.70724293864767418 ) ) ;
#43250=CARTESIAN_POINT ( 'NONE',  ( 10.81492255796078972, 18.62759615963270932, 109.5822429386476955 ) ) ;
#43251=CARTESIAN_POINT ( 'NONE',  ( -5.049401038297874678, -19.05341960407617918, 79.79275706135233293 ) ) ;
#43252=CARTESIAN_POINT ( 'NONE',  ( 5.049401038298161559, -19.05341960407611168, 77.70724293864765286 ) ) ;
#43253=CARTESIAN_POINT ( 'NONE',  ( -5.153800228976328057, -19.02544592524343514, 77.29057627198099567 ) ) ;
#43254=CARTESIAN_POINT ( 'NONE',  ( -15.72974639402197994, 15.80617190586746368, 75.62390960531439532 ) ) ;
#43255=CARTESIAN_POINT ( 'NONE',  ( 5.049401038298161559, -19.05341960407611168, 37.70724293864768839 ) ) ;
#43257=CARTESIAN_POINT ( 'NONE',  ( 0.05219959533910956823, 16.53943276465976808, 59.99890960531436690 ) ) ;
#43258=CARTESIAN_POINT ( 'NONE',  ( 0.05219959533909260263, 19.03943276465977164, 94.99890960531436690 ) ) ;
#43260=CARTESIAN_POINT ( 'NONE',  ( -19.03943276465977164, -0.05219959533935918106, 58.75109039468566863 ) ) ;
#43261=CARTESIAN_POINT ( 'NONE',  ( -15.72974639402197994, 15.80617190586746368, 80.62390960531438111 ) ) ;
#43262=CARTESIAN_POINT ( 'NONE',  ( -9.564922557961040184, 16.46253265017147172, 32.91775706135233293 ) ) ;
#43263=CARTESIAN_POINT ( 'NONE',  ( -9.564922557960796823, -16.46253265017161027, 87.08224293864769550 ) ) ;
#43265=CARTESIAN_POINT ( 'NONE',  ( 5.823673210054125526, 21.52544592524343514, 24.79057627198103120 ) ) ;
#43266=CARTESIAN_POINT ( 'NONE',  ( -19.05341960407611168, -5.049401038298163336, 76.45724293864769550 ) ) ;
#43267=CARTESIAN_POINT ( 'NONE',  ( 15.72974639402176855, 15.80617190586768217, 46.87609039468568994 ) ) ;
#43268=CARTESIAN_POINT ( 'NONE',  ( -19.05341960407611168, -5.049401038298163336, 31.45724293864769550 ) ) ;
#43269=CARTESIAN_POINT ( 'NONE',  ( 21.55341960407610458, 5.719274019375980345, 108.9572429386476955 ) ) ;
#43270=CARTESIAN_POINT ( 'NONE',  ( -16.51473224551069308, -9.474510206698971260, 96.66557627198102409 ) ) ;
#43272=CARTESIAN_POINT ( 'NONE',  ( 0.05219959533937995610, -21.53943276465977519, 35.00109039468568284 ) ) ;
#43274=CARTESIAN_POINT ( 'NONE',  ( -19.05341960407611168, -5.049401038298163336, 106.4572429386476955 ) ) ;
#43275=CARTESIAN_POINT ( 'NONE',  ( 0.05219959533909260263, 19.03943276465977164, 89.99890960531436690 ) ) ;
#43276=CARTESIAN_POINT ( 'NONE',  ( -10.81492255796078084, -18.62759615963271287, 107.0822429386476955 ) ) ;
#43277=CARTESIAN_POINT ( 'NONE',  ( -19.03943276465977164, 0.05219959533909376836, 61.24890960531436690 ) ) ;
#43278=CARTESIAN_POINT ( 'NONE',  ( 16.55341960407618274, -4.379528057220086978, 26.04275706135235779 ) ) ;
#43280=CARTESIAN_POINT ( 'NONE',  ( 18.67979575497194134, -10.72451020669871369, 100.8344237280190185 ) ) ;
#43281=CARTESIAN_POINT ( 'NONE',  ( 19.03943276465977164, -0.05219959533909143690, 38.74890960531436690 ) ) ;
#43282=CARTESIAN_POINT ( 'NONE',  ( 10.81492255796106328, -18.62759615963255655, 95.41775706135234714 ) ) ;
#43283=CARTESIAN_POINT ( 'NONE',  ( 9.474510206698971260, -16.51473224551069308, 92.91557627198103830 ) ) ;
#43284=CARTESIAN_POINT ( 'NONE',  ( 18.67979575497194134, -10.72451020669871369, 60.83442372801901854 ) ) ;
#43286=CARTESIAN_POINT ( 'NONE',  ( -16.51473224551069308, -9.474510206698971260, 101.6655762719810241 ) ) ;
#43287=DIRECTION ( 'NONE',  ( -1.000000000000000000, -0.000000000000000000, -0.000000000000000000 ) ) ;
#43288=CARTESIAN_POINT ( 'NONE',  ( -4.379528057220086978, -16.55341960407618274, 49.79275706135234714 ) ) ;
#43289=CARTESIAN_POINT ( 'NONE',  ( 4.379528057220092307, 16.55341960407617563, 67.29275706135234714 ) ) ;
#43290=CARTESIAN_POINT ( 'NONE',  ( -10.81492255796105439, 18.62759615963255655, 52.91775706135235424 ) ) ;
#43291=CARTESIAN_POINT ( 'NONE',  ( 10.72451020669871369, 18.67979575497193778, 87.08442372801901854 ) ) ;
#43294=CARTESIAN_POINT ( 'NONE',  ( -16.53943276465976808, -0.05219959533934237506, 33.75109039468568284 ) ) ;
#43295=CARTESIAN_POINT ( 'NONE',  ( -16.51473224551069308, -9.474510206698971260, 76.66557627198103830 ) ) ;
#43296=CARTESIAN_POINT ( 'NONE',  ( -19.05341960407611168, -5.049401038298163336, 91.45724293864766707 ) ) ;
#43298=CARTESIAN_POINT ( 'NONE',  ( -9.564922557960796823, -16.46253265017161027, 27.08224293864769550 ) ) ;
#43299=CARTESIAN_POINT ( 'NONE',  ( 18.67979575497178502, 10.72451020669898547, 34.16557627198102409 ) ) ;
#43300=CARTESIAN_POINT ( 'NONE',  ( -12.14591786802326823, 12.06949235617739902, 88.12609039468570415 ) ) ;
#43301=CARTESIAN_POINT ( 'NONE',  ( 16.52544592524342804, -4.483927247898539470, 88.54057627198103830 ) ) ;
#43302=CARTESIAN_POINT ( 'NONE',  ( 13.89961937509977652, -13.97604488694527269, 68.12390960531436690 ) ) ;
#43303=CARTESIAN_POINT ( 'NONE',  ( 21.55341960407619695, -5.719274019375665929, 96.04275706135236135 ) ) ;
#43305=CARTESIAN_POINT ( 'NONE',  ( -8.224510206698735004, -14.34966873604973081, 29.58442372801901854 ) ) ;
#43306=CARTESIAN_POINT ( 'NONE',  ( -8.224510206698948167, 14.34966873604960824, 80.41557627198103830 ) ) ;
#43307=CARTESIAN_POINT ( 'NONE',  ( 18.62759615963255655, 10.81492255796105972, 36.66775706135234714 ) ) ;
#43308=CARTESIAN_POINT ( 'NONE',  ( 10.72451020669898902, -18.67979575497178502, 67.91557627198102409 ) ) ;
#43309=CARTESIAN_POINT ( 'NONE',  ( 9.474510206698729675, 16.51473224551082808, 42.08442372801900433 ) ) ;
#43311=CARTESIAN_POINT ( 'NONE',  ( -19.05341960407611168, -5.049401038298163336, 76.45724293864769550 ) ) ;
#43312=CARTESIAN_POINT ( 'NONE',  ( -8.314922557960811034, -14.29746914071050412, 47.08224293864770260 ) ) ;
#43314=CARTESIAN_POINT ( 'NONE',  ( 12.14591786802309770, 12.06949235617756955, 29.37390960531435269 ) ) ;
#43315=CARTESIAN_POINT ( 'NONE',  ( 12.06949235617739724, 12.14591786802326823, 106.8760903946856899 ) ) ;
#43316=CARTESIAN_POINT ( 'NONE',  ( -16.51473224551082808, 9.474510206698731452, 68.33442372801900433 ) ) ;
#43317=CARTESIAN_POINT ( 'NONE',  ( 17.49999999999999645, 5.624438216177601646, 46.68329655085357643 ) ) ;
#43318=CARTESIAN_POINT ( 'NONE',  ( 10.72451020669898902, -18.67979575497178502, 22.91557627198102765 ) ) ;
#43319=CARTESIAN_POINT ( 'NONE',  ( 4.483927247898545687, 16.52544592524342804, 84.79057627198102409 ) ) ;
#43320=CARTESIAN_POINT ( 'NONE',  ( 18.22780087662122384, 5.500000000000018652, 93.98459894673892734 ) ) ;
#43321=CARTESIAN_POINT ( 'NONE',  ( 5.049401038298161559, -19.05341960407611168, 27.70724293864769550 ) ) ;
#43322=CARTESIAN_POINT ( 'NONE',  ( 18.62759615963271287, -10.81492255796078972, 38.33224293864768839 ) ) ;
#43323=CARTESIAN_POINT ( 'NONE',  ( -10.81492255796078084, -18.62759615963271287, 72.08224293864769550 ) ) ;
#43324=CARTESIAN_POINT ( 'NONE',  ( -8.224510206698948167, 14.34966873604960824, 115.4155762719810241 ) ) ;
#43325=CARTESIAN_POINT ( 'NONE',  ( -16.52544592524335698, -4.483927247898792601, 68.95942372801901854 ) ) ;
#43326=CARTESIAN_POINT ( 'NONE',  ( -9.564922557960796823, -16.46253265017161027, 52.08224293864768839 ) ) ;
#43327=CARTESIAN_POINT ( 'NONE',  ( 18.67979575497194134, -10.72451020669871369, 50.83442372801901143 ) ) ;
#43328=CARTESIAN_POINT ( 'NONE',  ( -0.05219959533910754901, -16.53943276465976808, 107.4989096053143669 ) ) ;
#43329=CARTESIAN_POINT ( 'NONE',  ( -16.46253265017146816, -9.564922557961047289, 89.16775706135234714 ) ) ;
#43332=CARTESIAN_POINT ( 'NONE',  ( -18.62759615963270932, 10.81492255796079327, 35.83224293864768839 ) ) ;
#43334=CARTESIAN_POINT ( 'NONE',  ( -15.72974639402176322, -15.80617190586768395, 64.37609039468568994 ) ) ;
#43335=CARTESIAN_POINT ( 'NONE',  ( -12.06949235617739369, -12.14591786802326823, 54.37609039468568994 ) ) ;
#43336=CARTESIAN_POINT ( 'NONE',  ( -16.53943276465976808, 0.05219959533911058130, 41.24890960531435269 ) ) ;
#43337=CARTESIAN_POINT ( 'NONE',  ( 15.80617190586746368, 15.72974639402197994, 64.37390960531435269 ) ) ;
#43338=CARTESIAN_POINT ( 'NONE',  ( -21.53943276465977519, 0.05219959533907696930, 66.24890960531436690 ) ) ;
#43340=CARTESIAN_POINT ( 'NONE',  ( 16.51473224551083163, -9.474510206698727899, 80.83442372801899012 ) ) ;
#43341=CARTESIAN_POINT ( 'NONE',  ( -19.05341960407611168, -5.049401038298163336, 111.4572429386476671 ) ) ;
#43342=CARTESIAN_POINT ( 'NONE',  ( 16.46253265017160672, -9.564922557960803928, 48.33224293864769550 ) ) ;
#43343=CARTESIAN_POINT ( 'NONE',  ( 12.14591786802309770, 12.06949235617756955, 109.3739096053143811 ) ) ;
#43346=CARTESIAN_POINT ( 'NONE',  ( 12.14591786802327356, -12.06949235617739191, 65.62609039468568994 ) ) ;
#43347=CARTESIAN_POINT ( 'NONE',  ( -21.53943276465977519, 0.05219959533907696930, 101.2489096053143669 ) ) ;
#43348=CARTESIAN_POINT ( 'NONE',  ( -19.03943276465977164, 0.05219959533909376836, 56.24890960531435979 ) ) ;
#43349=CARTESIAN_POINT ( 'NONE',  ( 5.719274019375673035, 21.55341960407619339, 47.29275706135234003 ) ) ;
#43350=CARTESIAN_POINT ( 'NONE',  ( 9.564922557960805705, 16.46253265017160317, 94.58224293864769550 ) ) ;
#43352=ORIENTED_EDGE ( 'NONE', *, *, #109475, .F. ) ;
#43353=CARTESIAN_POINT ( 'NONE',  ( -10.72451020669870658, -18.67979575497194134, 34.58442372801900433 ) ) ;
#43354=CARTESIAN_POINT ( 'NONE',  ( -13.97604488694527625, -13.89961937509977652, 101.8739096053143811 ) ) ;
#43355=CARTESIAN_POINT ( 'NONE',  ( 9.474510206698729675, 16.51473224551082808, 92.08442372801900433 ) ) ;
#43356=CARTESIAN_POINT ( 'NONE',  ( -9.564922557961040184, 16.46253265017147172, 42.91775706135234003 ) ) ;
#43357=CARTESIAN_POINT ( 'NONE',  ( 10.81492255796078972, 18.62759615963270932, 104.5822429386477097 ) ) ;
#43358=CARTESIAN_POINT ( 'NONE',  ( -13.89961937509957401, -13.97604488694547875, 34.37609039468566863 ) ) ;
#43359=CARTESIAN_POINT ( 'NONE',  ( 19.05341960407617918, -5.049401038297876454, 51.04275706135231871 ) ) ;
#43360=CARTESIAN_POINT ( 'NONE',  ( -4.483927247898782831, 16.52544592524335698, 97.70942372801904696 ) ) ;
#43362=CARTESIAN_POINT ( 'NONE',  ( 13.97604488694527802, 13.89961937509977652, 74.37390960531436690 ) ) ;
#43363=CARTESIAN_POINT ( 'NONE',  ( -15.72974639402176322, -15.80617190586768395, 79.37609039468567573 ) ) ;
#43364=CARTESIAN_POINT ( 'NONE',  ( -10.72451020669870658, -18.67979575497194134, 79.58442372801903275 ) ) ;
#43366=CARTESIAN_POINT ( 'NONE',  ( -16.51473224551069308, -9.474510206698971260, 86.66557627198102409 ) ) ;
#43367=CARTESIAN_POINT ( 'NONE',  ( 18.62759615963255655, 10.81492255796105972, 56.66775706135235424 ) ) ;
#43368=CARTESIAN_POINT ( 'NONE',  ( 16.51473224551083163, -9.474510206698727899, 100.8344237280190043 ) ) ;
#43369=CARTESIAN_POINT ( 'NONE',  ( -0.05219959533909027116, -19.03943276465977164, 72.49890960531435269 ) ) ;
#43370=CARTESIAN_POINT ( 'NONE',  ( 19.05341960407611168, 5.049401038298154454, 108.9572429386477097 ) ) ;
#43371=CARTESIAN_POINT ( 'NONE',  ( 9.564922557960805705, 16.46253265017160317, 79.58224293864769550 ) ) ;
#43372=CARTESIAN_POINT ( 'NONE',  ( 17.49999999999997158, -3.354790192122885539, 22.07749092806899682 ) ) ;
#43373=CARTESIAN_POINT ( 'NONE',  ( 5.153800228976335163, 19.02544592524342804, 69.79057627198103830 ) ) ;
#43374=CARTESIAN_POINT ( 'NONE',  ( -0.05219959533909027116, -19.03943276465977164, 52.49890960531436690 ) ) ;
#43375=CARTESIAN_POINT ( 'NONE',  ( -21.55341960407610458, -5.719274019375992779, 111.4572429386476813 ) ) ;
#43376=CARTESIAN_POINT ( 'NONE',  ( 14.29746914071037800, 8.314922557961029526, 81.66775706135236135 ) ) ;
#43378=CARTESIAN_POINT ( 'NONE',  ( 19.03943276465977164, 0.05219959533936151252, 46.25109039468566863 ) ) ;
#43379=CARTESIAN_POINT ( 'NONE',  ( 19.03943276465977164, -0.05219959533909143690, 78.74890960531436690 ) ) ;
#43380=CARTESIAN_POINT ( 'NONE',  ( 12.06949235617757843, -12.14591786802309237, 78.12390960531436690 ) ) ;
#43381=CARTESIAN_POINT ( 'NONE',  ( -16.53943276465976808, 0.05219959533911058130, 106.2489096053143811 ) ) ;
#43382=CARTESIAN_POINT ( 'NONE',  ( -10.81492255796078084, -18.62759615963271287, 22.08224293864769194 ) ) ;
#43384=CARTESIAN_POINT ( 'NONE',  ( 19.02544592524343514, -5.153800228976328945, 103.5405762719809957 ) ) ;
#43385=CARTESIAN_POINT ( 'NONE',  ( 16.55341960407611168, 4.379528057220329451, 83.95724293864770971 ) ) ;
#43387=CARTESIAN_POINT ( 'NONE',  ( -5.153800228976607833, 19.02544592524334988, 27.70942372801899722 ) ) ;
#43388=CARTESIAN_POINT ( 'NONE',  ( -4.483927247898782831, 16.52544592524335698, 87.70942372801901854 ) ) ;
#43389=CARTESIAN_POINT ( 'NONE',  ( 16.51473224551069308, 9.474510206698969483, 89.16557627198103830 ) ) ;
#43391=CARTESIAN_POINT ( 'NONE',  ( -5.823673210054431948, 21.52544592524334988, 52.70942372801902565 ) ) ;
#43392=CARTESIAN_POINT ( 'NONE',  ( -18.62759615963270932, 10.81492255796079327, 40.83224293864769550 ) ) ;
#43393=CARTESIAN_POINT ( 'NONE',  ( 5.823673210054125526, 21.52544592524343514, 114.7905762719810383 ) ) ;
#43394=CARTESIAN_POINT ( 'NONE',  ( 21.52544592524344225, -5.823673210054117533, 68.54057627198103830 ) ) ;
#43395=CARTESIAN_POINT ( 'NONE',  ( 4.379528057220339221, -16.55341960407611168, 97.70724293864772392 ) ) ;
#43396=CARTESIAN_POINT ( 'NONE',  ( -19.02544592524334988, -5.153800228976617603, 53.95942372801898301 ) ) ;
#43398=CARTESIAN_POINT ( 'NONE',  ( -9.564922557960796823, -16.46253265017161027, 37.08224293864768839 ) ) ;
#43399=CARTESIAN_POINT ( 'NONE',  ( -5.153800228976328057, -19.02544592524343514, 82.29057627198103830 ) ) ;
#43400=CARTESIAN_POINT ( 'NONE',  ( 5.153800228976335163, 19.02544592524342804, 84.79057627198099567 ) ) ;
#43401=CARTESIAN_POINT ( 'NONE',  ( 12.06949235617757843, -12.14591786802309237, 103.1239096053143811 ) ) ;
#43403=CARTESIAN_POINT ( 'NONE',  ( 8.224510206698953496, -14.34966873604960469, 22.91557627198102765 ) ) ;
#43404=CARTESIAN_POINT ( 'NONE',  ( 16.55341960407618274, -4.379528057220086978, 36.04275706135234714 ) ) ;
#43405=CARTESIAN_POINT ( 'NONE',  ( 15.80617190586769283, -15.72974639402175789, 100.6260903946857184 ) ) ;
#43406=CARTESIAN_POINT ( 'NONE',  ( 0.05219959533909260263, 19.03943276465977164, 94.99890960531436690 ) ) ;
#43407=CARTESIAN_POINT ( 'NONE',  ( 18.67979575497194134, -10.72451020669871369, 35.83442372801901143 ) ) ;
#43408=CARTESIAN_POINT ( 'NONE',  ( 19.02544592524343514, -5.153800228976328945, 48.54057627198103120 ) ) ;
#43409=CARTESIAN_POINT ( 'NONE',  ( 14.29746914071037800, 8.314922557961029526, 41.66775706135235424 ) ) ;
#43411=CARTESIAN_POINT ( 'NONE',  ( 16.51473224551083163, -9.474510206698727899, 110.8344237280190043 ) ) ;
#43412=CARTESIAN_POINT ( 'NONE',  ( 19.03943276465977164, -0.05219959533909143690, 38.74890960531436690 ) ) ;
#43413=CARTESIAN_POINT ( 'NONE',  ( 4.483927247898545687, 16.52544592524342804, 99.79057627198103830 ) ) ;
#43414=CARTESIAN_POINT ( 'NONE',  ( -21.55341960407610458, -5.719274019375992779, 106.4572429386477097 ) ) ;
#43415=CARTESIAN_POINT ( 'NONE',  ( -19.02544592524334988, -5.153800228976617603, 83.95942372801901854 ) ) ;
#43417=CARTESIAN_POINT ( 'NONE',  ( 13.89961937509977652, -13.97604488694527269, 88.12390960531438111 ) ) ;
#43418=CARTESIAN_POINT ( 'NONE',  ( 15.80617190586769283, -15.72974639402175789, 30.62609039468567929 ) ) ;
#43419=CARTESIAN_POINT ( 'NONE',  ( -5.049401038298153566, 19.05341960407611168, 25.20724293864768484 ) ) ;
#43420=CARTESIAN_POINT ( 'NONE',  ( 5.153800228976335163, 19.02544592524342804, 89.79057627198102409 ) ) ;
#43422=CARTESIAN_POINT ( 'NONE',  ( 16.79531203550644847, -7.028104445595642957, 111.2475501177955977 ) ) ;
#43423=CARTESIAN_POINT ( 'NONE',  ( 9.474510206698971260, -16.51473224551069308, 82.91557627198103830 ) ) ;
#43424=CARTESIAN_POINT ( 'NONE',  ( 18.62759615963255655, 10.81492255796105972, 36.66775706135234714 ) ) ;
#43425=CARTESIAN_POINT ( 'NONE',  ( 8.314922557960818139, 14.29746914071049879, 94.58224293864769550 ) ) ;
#43426=CARTESIAN_POINT ( 'NONE',  ( -9.474510206698964154, 16.51473224551069663, 100.4155762719810241 ) ) ;
#43427=CARTESIAN_POINT ( 'NONE',  ( 13.89961937509957401, 13.97604488694547697, 21.87609039468566152 ) ) ;
#43428=CARTESIAN_POINT ( 'NONE',  ( -12.14591786802326823, 12.06949235617739902, 53.12609039468568284 ) ) ;
#43429=CARTESIAN_POINT ( 'NONE',  ( 21.53943276465977519, 0.05219959533937863772, 76.25109039468568994 ) ) ;
#43430=CARTESIAN_POINT ( 'NONE',  ( 4.483927247898790824, -16.52544592524335698, 30.20942372801902565 ) ) ;
#43431=CARTESIAN_POINT ( 'NONE',  ( -5.153800228976328057, -19.02544592524343514, 67.29057627198102409 ) ) ;
#43432=CARTESIAN_POINT ( 'NONE',  ( 19.02544592524334988, 5.153800228976608722, 96.45942372801897591 ) ) ;
#43433=CARTESIAN_POINT ( 'NONE',  ( -14.29746914071037622, -8.314922557961029526, 74.16775706135231871 ) ) ;
#43434=CARTESIAN_POINT ( 'NONE',  ( 15.80617190586769283, -15.72974639402175789, 110.6260903946857042 ) ) ;
#43435=CARTESIAN_POINT ( 'NONE',  ( 13.97604488694548053, -13.89961937509957401, 80.62609039468567573 ) ) ;
#43436=CARTESIAN_POINT ( 'NONE',  ( -9.564922557960796823, -16.46253265017161027, 62.08224293864769550 ) ) ;
#43437=CARTESIAN_POINT ( 'NONE',  ( -15.80617190586745835, -15.72974639402198527, 81.87390960531435269 ) ) ;
#43438=CARTESIAN_POINT ( 'NONE',  ( 8.224510206698953496, -14.34966873604960469, 77.91557627198102409 ) ) ;
#43439=CARTESIAN_POINT ( 'NONE',  ( 13.97604488694548053, -13.89961937509957401, 75.62609039468564731 ) ) ;
#43440=CARTESIAN_POINT ( 'NONE',  ( -19.52851543214745078, -5.499999999999944045, 70.39357721762578990 ) ) ;
#43441=CARTESIAN_POINT ( 'NONE',  ( 16.51473224551083163, -9.474510206698727899, 50.83442372801899722 ) ) ;
#43442=CARTESIAN_POINT ( 'NONE',  ( 16.55341960407618274, -4.379528057220086978, 106.0427570613523471 ) ) ;
#43443=CARTESIAN_POINT ( 'NONE',  ( -14.29746914071049879, 8.314922557960819915, 80.83224293864769550 ) ) ;
#43444=CARTESIAN_POINT ( 'NONE',  ( -0.05219959533937732626, 21.53943276465977519, 102.5010903946856899 ) ) ;
#43446=CARTESIAN_POINT ( 'NONE',  ( 21.53943276465977519, -0.05219959533907433946, 113.7489096053143527 ) ) ;
#43447=( BOUNDED_SURFACE ( )  B_SPLINE_SURFACE ( 3, 2, ( 
 ( #145350, #194875, #23021, #55346, #56348, #146346, #10859, #68511, #72528, #131184, #26033, #118031, #38189, #179722, #161529, #41193, #87678, #134204, #195892, #57367, #7833, #6832, #130165, #191862, #53344, #176716, #12856, #153328, #122986, #88681, #168504, #30002, #13829, #75495, #104850, #181701, #152344, #150377, #44181, #137168, #138169, #92642, #15822, #45174, #77483, #14830, #76492, #27036, #30993, #199850, #136186, #151365, #167526, #74521, #198857, #60323, #61316, #73537, #197861, #105839, #58348, #121998, #183688, #106829, #629, #123970, #166540, #184673, #90662, #91640, #62300, #46156, #11873, #107811, #185667, #135210, #169493, #154332, #47158, #196882, #29022, #28038, #43182, #139152, #120016, #165539, #89679, #59328, #120997, #182696, #173490, #158304, #189653, #94638, #141145, #66291, #78466, #79477, #128941, #51127, #187677, #112787, #33974, #188663, #2635, #49147, #95631, #65295, #156318, #16816, #35948, #31986, #125979, #34963, #17819, #18814, #174481, #126954, #19792, #97594, #159282, #143119, #93643, #64311, #140141, #96615, #80458, #4599, #110805, #50142, #172487, #81433, #127950, #155328, #111801, #20779, #157318, #142132, #48155, #124989, #3616, #1633, #82434, #144122, #5603, #67282, #190642, #108817, #170496, #63310, #186685, #109813, #171496, #32985, #22790, #37957, #54124, #161295, #162295, #85445, #86454, #160298, #84437, #130951, #145116, #147135, #8623, #70295, #87455, #10631, #191630, #24805, #177487, #38956, #149141, #193648, #113774, #178480, #72292, #175470, #131963, #116789, #133970, #36942, #115797, #53110, #68280, #23795, #98604, #148139, #9630, #21788, #71297, #55120, #39947, #101618, #132960, #99615, #146115, #194648, #83439, #7599, #52118, #56118, #192641, #117801, #100612, #163307, #69285, #179494, #40959, #102631, #164316, #6601, #25809, #129931, #114788, #176481, #181478, #105607, #61078, #152116, #106594, #137928, #76250, #29767, #180495, #104620, #26804, #60092, #167294, #88445, #92407, #75266, #196656, #182464, #89446, #58125, #184441, #41967, #122750, #166309, #199612, #120763, #11641, #198626, #134979, #42956, #45921, #107575, #169253, #28791, #73308, #119794, #57133, #27806, #150140, #168270, #151136, #136937, #12627, #90430, #13599, #121760, #91401, #74292, #183453, #135961, #44937, #30760, #154093, #103634, #153090, #43945, #118809, #197631, #14594, #15587, #165311, #59097, #77245, #195662, #20537, #80219, #138913, #393, #95390, #65056, #32743, #16580, #141890, #3381, #35711, #126713, #48907, #62066, #47919, #2390, #186443, #159044, #127713, #185430, #108580, #19556, #155086, #123731, #81200, #187439, #94395, #109573, #142881, #125739, #50890, #46920, #156074, #63068, #17572, #170257, #1387, #124747, #97358, #96378, #4362, #18572, #78227, #66046, #31751, #189414, #157076, #140904, #171256, #93400, #188416, #112548, #139898, #79233, #110561, #49894, #111560, #64069, #172242, #173245, #33728, #34720, #158065, #174243, #5361, #114535, #42463, #165808, #73804, #131718, #160054, #43452, #84192, #104126, #38715, #175229, #27305, #105120, #85194, #99368, #88952, #58611, #21541, #70050, #120278, #176235, #83201, #100372, #116549, #144875, #8375, #178237, #150643, #145872, #6358, #113535, #143880, #115556, #192399, #54875, #12140, #69039, #37706, #68038, #135476, #128703, #197145, #191387, #181970, #7355, #98355, #146883, #129690, #52863, #166807, #82187, #67044, #53881, #161051, #22545, #190400, #51876, #130704, #162051, #177243, #193400, #36694, #23547, #31258, #92909, #76753, #138428, #167785, #44446, #15094, #13121, #107086, #200109, #897, #155590, #78738, #108080, #140414, #77749, #16091, #89947, #93912, #62571, #199115, #14091, #30260, #137435, #61577, #123246, #124249, #136446, #60582, #168757, #121269, #184937, #46422, #169764, #63584, #186956, #29284, #185944, #153596, #154595, #125258, #139415, #151627, #47429, #48427, #74784, #109085 ),
 ( #110083, #170765, #182963, #122258, #91904, #32254, #198127, #183947, #17085, #1904, #28307, #59595, #106100, #90915, #152601, #75758, #45433, #64579, #52383, #191897, #174746, #188936, #175738, #145385, #49409, #159553, #6867, #3883, #172761, #189919, #5874, #111072, #97863, #67551, #129208, #35229, #95902, #2901, #33251, #4874, #81699, #144389, #156594, #80726, #126244, #36210, #143382, #187940, #68546, #51394, #34241, #158566, #65562, #157586, #160567, #18088, #98871, #142405, #114040, #96883, #19078, #21050, #127222, #50413, #37215, #22056, #83707, #66557, #112073, #173762, #94909, #190906, #20055, #113054, #128222, #82705, #130202, #79744, #53382, #171762, #141413, #25071, #54388, #131220, #101889, #99880, #193918, #86714, #87710, #42230, #165571, #194910, #27070, #164573, #102888, #176752, #180754, #149396, #85716, #100874, #117051, #24061, #148399, #9893, #10891, #23058, #147402, #55381, #7870, #71554, #133219, #56385, #150411, #73570, #116061, #72564, #40210, #163571, #11906, #118067, #38225, #41227, #135243, #161565, #179757, #26067, #196915, #84703, #178746, #177749, #192911, #134239, #146382, #195924, #57400, #69556, #119072, #103891, #88716, #115059, #39218, #162556, #8890, #70558, #132225, #29054, #78501, #139188, #137204, #663, #183721, #138202, #152377, #198890, #45207, #14864, #105873, #166573, #185701, #181736, #75529, #123019, #44214, #168535, #124003, #76525, #169526, #62333, #47190, #92676, #108850, #106861, #74552, #61348, #197894, #167560, #170530, #32020, #93678, #30033, #136219, #59363, #120049, #154364, #60358, #199884, #90694, #46189, #15858, #43217, #184704, #107842, #91671, #153362, #121032, #182730, #31026, #104885, #122031, #77516, #155361, #16850, #140174, #58382, #28073, #89714, #151399, #12889, #13862, #35977, #172521, #187707, #3648, #110837, #111831, #34991, #97624, #109843, #34006, #80490, #94671, #96645, #158333, #19822, #36973, #160329, #141176, #174510, #126986, #188693, #98634, #143149, #63345, #127981, #21819, #125022, #81463, #66320, #83471, #186718, #65326, #2666, #17851, #173520, #48188, #159314, #20809, #171528, #82465, #4630, #189684, #51157, #144151, #49179, #95663, #5636, #33016, #157350, #1667, #67313, #142164, #128973, #50174, #112817, #18845, #190672, #52148, #113805, #175500, #156350, #79507, #64343, #126012, #9660, #130982, #55150, #10661, #101647, #56149, #87484, #25840, #179523, #129961, #54156, #176511, #71327, #116820, #37989, #41997, #24834, #146145, #131994, #38988, #7632, #134000, #191661, #72324, #115829, #163339, #192673, #132989, #102660, #68310, #148169, #194680, #193680, #178511, #84467, #161328, #39977, #53140, #23826, #86484, #117830, #195691, #57162, #40992, #118841, #164345, #149172, #6632, #180524, #103663, #177518, #100644, #147165, #162325, #165341, #26834, #145148, #114819, #85476, #8653, #99645, #22821, #69316, #70327, #123760, #46949, #27837, #61108, #13629, #75296, #185459, #29796, #150171, #14623, #108609, #11671, #44968, #153119, #170286, #73337, #90462, #89478, #104653, #60123, #135010, #184471, #122781, #58156, #45950, #121790, #76280, #137959, #169283, #74324, #120795, #107605, #119824, #59128, #88474, #30789, #167326, #92437, #136967, #168300, #182495, #28822, #198656, #106626, #135991, #196687, #15617, #181509, #105637, #199642, #197662, #183484, #154123, #91432, #77274, #138943, #423, #62097, #42988, #43975, #166339, #151169, #12657, #152146, #128736, #111590, #32773, #18601, #125768, #94425, #20569, #78256, #159075, #140934, #112580, #157105, #47951, #34749, #171286, #79262, #174274, #35743, #82221, #141919, #109602, #156106, #93429, #66077, #33761, #173276, #17603, #97389, #1418, #143911, #188446, #95421, #2421, #155115, #158095, #5393, #190432, #187468, #80249, #49926, #96408, #64101, #113567, #19587, #124776, #48937, #3410, #65085, #16609, #110590, #189445, #67076, #51908, #81230, #172272, #31780 ),
 ( #126744, #142911, #4393, #127743, #50922, #139929, #63097, #186474, #38750, #99402, #6391, #36727, #8411, #85231, #147932, #55908, #7391, #68070, #9418, #145906, #54911, #129724, #146921, #70084, #131753, #71083, #53916, #116583, #115590, #178272, #25602, #133751, #160087, #193435, #23583, #98389, #191421, #132750, #39735, #21574, #22580, #194437, #117582, #56920, #101397, #175261, #83233, #163090, #24594, #69075, #52897, #86242, #179282, #72077, #40747, #102416, #144908, #84228, #100407, #130741, #195445, #164103, #114572, #176270, #87246, #37742, #161085, #148929, #10419, #192433, #177279, #162088, #105398, #30545, #187, #12422, #42749, #74085, #118595, #181272, #104412, #77035, #76044, #184233, #134765, #41753, #199404, #167084, #135755, #166095, #60867, #28586, #92197, #180285, #88233, #152883, #183246, #122543, #43737, #90222, #153881, #59884, #103418, #44727, #15378, #165097, #75059, #106383, #26590, #149918, #120558, #57918, #196448, #151906, #11424, #14378, #91193, #73094, #137720, #13395, #168064, #29562, #45714, #27597, #150929, #107367, #119589, #89235, #138706, #169039, #197426, #58892, #136725, #198407, #182252, #121550, #187233, #18370, #109362, #170049, #189213, #185219, #79019, #126517, #47712, #172038, #127509, #80022, #173043, #4161, #142682, #96180, #46710, #171044, #93192, #188216, #33525, #154877, #158843, #141691, #62854, #48703, #155867, #124536, #50692, #108373, #112350, #32534, #65839, #110356, #78022, #64855, #1177, #94187, #174041, #35510, #97159, #95187, #139691, #186233, #123525, #157869, #63866, #3182, #17364, #49689, #19358, #31540, #111354, #34520, #156873, #81007, #140694, #2184, #20331, #16375, #125537, #81980, #143673, #61856, #55670, #84989, #117344, #54668, #193195, #66837, #70847, #39499, #176033, #191192, #7155, #116342, #178031, #128500, #132516, #101159, #37501, #52668, #68838, #114330, #115352, #38512, #162847, #113335, #99163, #83994, #98146, #100168, #161850, #23344, #175027, #24354, #69841, #147694, #130497, #192193, #40508, #146670, #190195, #131508, #102179, #51673, #8165, #86005, #87007, #36492, #53674, #144672, #21339, #177042, #159846, #9181, #194205, #82997, #179040, #163867, #25366, #5154, #6157, #160853, #22343, #67837, #129494, #145673, #168804, #29333, #27354, #90961, #73854, #28356, #42512, #89000, #135524, #105168, #196216, #56683, #75805, #71842, #165858, #13169, #134529, #58658, #14138, #166854, #59644, #152648, #137483, #183010, #133511, #57686, #180050, #74832, #120324, #41519, #45478, #89994, #149686, #197195, #104176, #11184, #199163, #195203, #60630, #119354, #122304, #182019, #164862, #151676, #87998, #181038, #183995, #107134, #30308, #43502, #26358, #72859, #10182, #44494, #150691, #136494, #12189, #198174, #106150, #118357, #121318, #167832, #148694, #103182, #184983, #123291, #124293, #15139, #139460, #47473, #63628, #33293, #97652, #93956, #159342, #140459, #78782, #91951, #20838, #125304, #154641, #31302, #62615, #92955, #109130, #170808, #187000, #138472, #16136, #940, #61623, #32301, #155635, #17130, #200153, #48470, #1949, #171805, #185990, #110127, #82495, #144178, #76801, #5664, #153644, #46467, #108127, #169811, #77791, #57335, #74492, #11843, #88651, #44150, #134175, #168472, #45141, #42170, #106798, #105809, #137139, #121964, #153297, #58320, #104822, #29970, #103830, #43154, #95341, #14798, #151337, #76458, #197833, #152314, #166511, #12826, #59299, #28992, #119988, #180694, #199816, #195863, #89649, #198826, #181674, #182666, #138135, #90632, #183657, #61284, #125691, #91609, #119011, #28009, #165510, #60291, #167496, #27007, #172194, #13800, #73508, #120967, #136158, #135180, #187390, #150347, #48858, #75466, #110513, #33679, #196854, #157026, #72501, #94950, #62611, #108123, #139456, #142445, #168800, #93953, #32297, #45475, #138468, #156634, #155631, #107129, #31299, #2941, #141456, #65603, #125301, #183990, #30304 ),
 ( #186997, #937, #187980, #157627, #61619, #171802, #19117, #16132, #184978, #1945, #18129, #123287, #110124, #79784, #64621, #47470, #169806, #15135, #91947, #17127, #78779, #126283, #49449, #77787, #76797, #111112, #154637, #63625, #200149, #140455, #48467, #33290, #172801, #124290, #34282, #185987, #92951, #109127, #3923, #153640, #95941, #80767, #46463, #170805, #99916, #175780, #188976, #174783, #146418, #84740, #8929, #68584, #127263, #50452, #83744, #53420, #21090, #4912, #130240, #191936, #24100, #115097, #37254, #112111, #36249, #190944, #97902, #147441, #116097, #173802, #96923, #7909, #143425, #35268, #69593, #98911, #82747, #159593, #131260, #114079, #39255, #158605, #160604, #22094, #20095, #144427, #189957, #51431, #85754, #192948, #54427, #6905, #66595, #177785, #81739, #100911, #145423, #129248, #113091, #128259, #176789, #162595, #5913, #67590, #38262, #161601, #23095, #52421, #152406, #88751, #163609, #102925, #72601, #134275, #193956, #164610, #28106, #151431, #59394, #120082, #148437, #29084, #195962, #89745, #27105, #118104, #12918, #57435, #182762, #70597, #119108, #180789, #178785, #87747, #133257, #194948, #90723, #74582, #136250, #150444, #86754, #197926, #40253, #121068, #11940, #42266, #56424, #132265, #196947, #44246, #167589, #26104, #103926, #73603, #135275, #149432, #55419, #58415, #25110, #10928, #165606, #181770, #117090, #43251, #105903, #101927, #9932, #104919, #71591, #179794, #166606, #41263, #170564, #106893, #94705, #34042, #16883, #31061, #17887, #187742, #91705, #1702, #49213, #46223, #14897, #32054, #48222, #153399, #140208, #109876, #171560, #77550, #138234, #45239, #75560, #47226, #124038, #186752, #156382, #107876, #168566, #33050, #184738, #93711, #30064, #185737, #108885, #155393, #79541, #92709, #125055, #154397, #199917, #169564, #172556, #198920, #78534, #62369, #137236, #76558, #141211, #63378, #60389, #61381, #2701, #64378, #95699, #126046, #13893, #122061, #110871, #183753, #15892, #123052, #139222, #697, #54191, #145183, #67349, #80526, #66358, #20847, #4666, #177553, #146181, #3683, #127022, #38025, #173558, #142200, #99681, #5673, #51194, #39022, #144187, #129009, #65361, #174546, #19859, #81499, #115864, #114855, #22856, #37010, #35027, #84503, #188729, #7666, #113840, #159351, #143186, #18880, #83506, #69350, #157387, #112855, #190709, #175536, #98671, #189721, #50214, #160365, #111868, #36013, #82505, #52182, #96682, #97662, #176549, #161365, #131018, #6667, #158370, #128019, #21855, #192708, #68345, #129996, #191696, #53179, #103698, #117868, #104688, #74357, #178545, #88514, #136023, #133025, #101684, #118876, #135046, #40011, #26871, #196722, #58190, #164382, #24870, #132027, #162359, #134035, #10698, #73374, #181542, #194715, #193716, #119858, #71361, #180560, #55185, #72361, #195728, #57201, #43021, #179558, #11707, #41028, #86519, #56184, #59163, #85511, #42034, #149207, #23860, #116854, #166376, #165377, #147199, #148203, #27872, #89513, #182531, #150210, #100677, #8690, #151203, #12691, #102694, #163373, #197697, #120831, #70360, #9696, #25875, #87519, #153157, #107642, #91469, #64140, #32811, #90498, #13664, #124813, #60157, #167360, #186513, #92474, #137996, #14658, #47987, #30826, #156143, #137002, #138981, #459, #62134, #75331, #78293, #108646, #109640, #169319, #154162, #79301, #185496, #105674, #170324, #140970, #28858, #123798, #31816, #125804, #152180, #45987, #183520, #121826, #15654, #198690, #139967, #16646, #45003, #1456, #77313, #93467, #155154, #171323, #29832, #76318, #63134, #106663, #199680, #44013, #94462, #122817, #17641, #46987, #2458, #61145, #184507, #168336, #143949, #34789, #95458, #114607, #110628, #4428, #51943, #173314, #97425, #52932, #5429, #98426, #129758, #68106, #21611, #172309, #96444, #18639, #113603, #159111, #80285, #84263, #67113, #188486, #174309, #81265, #49965, #176304, #33798 ),
 ( #65122, #48973, #83269, #189480, #128771, #158131, #175297, #144943, #157143, #190470, #36763, #35778, #20605, #126780, #3446, #82257, #141957, #66115, #160123, #6425, #37776, #99440, #191455, #161120, #22617, #145944, #111629, #7425, #69109, #19623, #142946, #50958, #127780, #187506, #112617, #167861, #38786, #163126, #9456, #24629, #15171, #148966, #23620, #86277, #132786, #194473, #53950, #147968, #90991, #14167, #122334, #183039, #8446, #91980, #55945, #152678, #87281, #85267, #75835, #153674, #133789, #71120, #137513, #107163, #70119, #121346, #168834, #117621, #131790, #10455, #29361, #193470, #59674, #199194, #60661, #179319, #54947, #162123, #192467, #164140, #40783, #106178, #184026, #102452, #146958, #45508, #101435, #72116, #116619, #25637, #195481, #44522, #30339, #130775, #115626, #177315, #178308, #100443, #39771, #61652, #187031, #125334, #138501, #31335, #49482, #48502, #200183, #124325, #95977, #34314, #158636, #18163, #76830, #123320, #33322, #2973, #170840, #154671, #79819, #141490, #173835, #64653, #110156, #185013, #186023, #140493, #47505, #96956, #65635, #46498, #108159, #157661, #92986, #169841, #19150, #171834, #32332, #109161, #80800, #63661, #189008, #16167, #94983, #156668, #77821, #93985, #139490, #972, #35300, #142478, #3956, #126315, #62648, #127295, #155665, #50483, #188012, #78814, #17161, #1981, #111145, #112143, #172835, #114111, #68617, #176822, #38294, #54460, #190977, #5945, #22126, #129282, #130273, #53454, #116130, #128291, #52454, #98944, #113125, #115130, #99948, #161634, #189989, #177819, #84773, #162630, #145456, #6938, #55454, #23128, #81771, #146451, #117125, #143458, #7944, #69627, #101963, #82779, #4943, #131293, #147475, #178819, #175814, #191968, #192982, #39289, #37287, #20127, #100946, #174815, #160635, #83776, #24137, #66627, #85789, #8965, #70634, #132300, #193992, #97935, #40289, #51463, #36280, #159628, #21123, #144460, #67621, #166639, #180821, #167624, #137274, #41298, #151466, #198956, #195996, #164643, #181806, #197961, #102959, #89781, #59431, #121104, #27137, #87781, #194982, #25146, #196980, #73637, #136285, #44281, #57469, #56460, #182798, #134310, #43284, #118139, #135308, #58447, #120115, #105939, #42300, #74619, #103961, #149466, #119141, #122096, #148474, #104953, #11972, #86788, #179828, #29120, #28141, #9966, #10961, #90759, #152442, #45273, #12954, #163644, #71626, #13928, #75595, #165639, #26139, #60423, #183787, #133292, #72635, #88784, #150477, #15927, #170600, #154433, #127057, #63415, #17921, #49246, #187776, #141245, #91740, #77585, #138269, #171596, #16918, #199952, #3719, #186788, #107914, #93747, #733, #169599, #95734, #153435, #34076, #139257, #110904, #32090, #123087, #109912, #46259, #62405, #14933, #172590, #33084, #106927, #184773, #31097, #168600, #2734, #108920, #125090, #124075, #94740, #64411, #30100, #156420, #79576, #155428, #78571, #92745, #185776, #140245, #76593, #47263, #1737, #126080, #157420, #18914, #48258, #80559, #142234, #65396, #61416, #188764, #84536, #20884, #36049, #52217, #159389, #160401, #83540, #146213, #158404, #82542, #129042, #143221, #145219, #6701, #68379, #19893, #7701, #114890, #192743, #175571, #37048, #85547, #191730, #111904, #176584, #147233, #173592, #81534, #144224, #113874, #70394, #98707, #189757, #66393, #21890, #35061, #69384, #22890, #4703, #131053, #130031, #38058, #99714, #54225, #97698, #5708, #115896, #128055, #67385, #132062, #177586, #190743, #39053, #53212, #161398, #100711, #162391, #23894, #8725, #50248, #51229, #96716, #112890, #174584, #58220, #179591, #103730, #59194, #41063, #40045, #136053, #119889, #193751, #71394, #133058, #55219, #27904, #195760, #11739, #102726, #181574, #151233, #116888, #196753, #43052, #42066, #165410, #194748, #9730, #180592, #178580, #72394, #26903, #166409, #120863, #44046, #73406, #105706, #104718, #89547, #101719, #182563 ),
 ( #167393, #75362, #88546, #150244, #163409, #10730, #56220, #117902, #152211, #12722, #28889, #135077, #164415, #90529, #74388, #197728, #134070, #57234, #25907, #24905, #13695, #86552, #148236, #87552, #149239, #118908, #155187, #169351, #18669, #16677, #29864, #30860, #139013, #493, #60189, #92507, #94493, #17674, #125836, #186545, #14691, #95489, #62166, #156175, #93501, #91501, #79332, #157175, #139999, #154196, #141002, #110660, #76353, #124845, #172340, #15686, #138030, #78326, #171355, #199713, #63166, #32843, #2490, #123830, #61178, #168368, #198722, #170357, #47020, #109674, #64171, #77347, #153188, #187539, #107674, #1488, #122850, #108679, #31849, #48018, #49005, #185528, #137032, #121859, #33829, #183551, #45037, #184538, #106695, #46018, #141988, #127808, #99470, #37809, #162151, #21645, #80315, #3476, #36795, #6455, #174338, #158161, #83298, #144974, #177343, #68136, #190501, #65153, #189512, #143981, #50986, #100472, #69139, #126811, #49995, #161150, #96473, #188518, #22647, #128802, #35808, #112646, #84294, #67144, #192497, #111660, #51974, #113633, #173347, #97454, #142978, #4456, #38814, #145973, #7455, #160154, #19653, #130806, #175328, #191484, #159140, #20637, #66145, #34818, #129787, #53981, #81294, #82290, #98460, #52962, #114639, #5462, #176337, #115654, #116647, #55974, #25666, #87311, #146987, #117651, #181336, #104478, #12487, #73163, #101464, #182322, #148995, #42815, #180349, #178337, #166162, #43801, #26656, #40811, #27663, #197490, #163155, #11492, #58957, #179348, #24658, #41817, #57982, #86307, #149986, #119654, #89303, #10484, #147996, #54977, #85295, #56984, #133820, #196512, #150995, #102481, #39799, #74148, #194501, #103485, #9485, #195511, #118658, #165163, #135820, #164168, #134833, #72144, #71149, #120625, #105464, #88298, #132815, #23647, #8474, #70149, #131819, #193499, #29621, #28649, #93256, #94253, #63929, #60934, #15444, #123591, #185285, #199467, #48767, #46777, #59947, #122608, #169104, #30611, #90285, #184298, #124601, #47776, #155933, #16438, #44791, #125598, #92264, #186296, #108436, #121614, #109429, #187295, #170112, #45780, #171109, #140758, #106444, #154941, #2246, #107432, #168125, #31606, #1242, #91253, #78087, #62921, #32600, #153948, #152944, #198475, #151969, #252, #77102, #139755, #17428, #138771, #183309, #79085, #137782, #167150, #14443, #61921, #13457, #75121, #136789, #76106, #21403, #189277, #34583, #65902, #68904, #95251, #20397, #158906, #172102, #64916, #83061, #82045, #33588, #157928, #129554, #67901, #192261, #51736, #110421, #156936, #66901, #36556, #4224, #188278, #113398, #175088, #7219, #98210, #143741, #18433, #19418, #174103, #81066, #130563, #99229, #80083, #141752, #191254, #126577, #3242, #52729, #5220, #127576, #142744, #114394, #97220, #22409, #49751, #128564, #190259, #111420, #50753, #173106, #96240, #112411, #35572, #159914, #144735, #6222, #176096, #37566, #160916, #84060, #145738, #26423, #24422, #133578, #85057, #163935, #87073, #148758, #88063, #132582, #164930, #194270, #178097, #9247, #12255, #38577, #25432, #102247, #115417, #8234, #149750, #10247, #177106, #101225, #72926, #11252, #135587, #195268, #53743, #100233, #71906, #180116, #147761, #131578, #56752, #118423, #150757, #41584, #103248, #161915, #162914, #117411, #86071, #73917, #42578, #23409, #146738, #134595, #69912, #193262, #196281, #57750, #70914, #55737, #119420, #40577, #165924, #54736, #181104, #104241, #116408, #179108, #39567, #27420, #89066, #154711, #62683, #76867, #13233, #124364, #168870, #108198, #75873, #14205, #59711, #58721, #123358, #186060, #94020, #91028, #45545, #153712, #15208, #29398, #78850, #138537, #90058, #152714, #199232, #60697, #120390, #137549, #16204, #77859, #47543, #46539, #74896, #155701, #122373, #139526, #15, #151740, #1009, #17196, #61689, #184062, #109197, #170876, #136559, #185051, #32367, #107200 ),
 ( #197259, #169880, #30375, #182084, #43567, #198240, #31373, #105232, #92019, #121384, #93023, #166920, #183076, #28421, #44559, #106214, #167898, #64691, #171870, #2018, #176616, #50522, #115928, #23924, #172872, #33359, #177618, #111182, #22922, #95018, #114923, #38091, #99746, #39086, #19189, #54257, #80838, #126352, #96014, #101752, #125372, #161430, #189047, #63697, #156706, #100742, #84568, #187068, #188049, #162423, #85579, #24937, #146246, #140528, #48538, #7732, #69418, #34353, #18200, #131084, #192773, #40074, #147265, #8755, #110192, #49519, #3993, #157699, #163440, #132092, #79858, #141526, #70426, #3014, #142515, #193781, #55250, #65673, #127335, #116918, #178611, #198757, #168402, #73436, #135107, #194777, #103761, #149269, #10761, #45070, #44080, #152244, #166441, #102758, #13729, #58251, #197760, #165440, #26935, #72425, #148267, #12755, #75395, #183585, #180624, #196783, #43083, #104750, #118939, #86583, #27936, #179622, #42096, #88577, #150275, #9759, #11771, #105739, #167426, #137067, #136086, #164445, #106728, #151265, #119919, #117933, #71423, #89579, #87582, #181605, #74420, #134103, #60222, #133087, #121892, #195793, #28922, #59227, #25939, #120896, #57265, #182596, #56251, #90562, #41094, #29897, #107707, #169386, #91535, #64207, #31883, #48054, #77380, #17712, #187574, #153222, #32880, #94530, #78361, #140035, #30894, #46052, #16711, #14727, #108713, #1524, #2527, #157213, #80354, #109710, #142026, #79369, #141040, #76387, #95527, #125874, #528, #15720, #93537, #139048, #63202, #124882, #49042, #138064, #62200, #170392, #122883, #186581, #171393, #156212, #199745, #110697, #172377, #33867, #155222, #18707, #65191, #3515, #61211, #126850, #188556, #184571, #92541, #123864, #50034, #111698, #154230, #185562, #47056, #145012, #34855, #69179, #146011, #143015, #7494, #6493, #37848, #22685, #54019, #159178, #5498, #130845, #4493, #144017, #193540, #115693, #52011, #177381, #98498, #53001, #67181, #113670, #160191, #129825, #20673, #81332, #100510, #96510, #190537, #99508, #82327, #83335, #38853, #191524, #84332, #162189, #23687, #192536, #158200, #128838, #66183, #85335, #127845, #175364, #36832, #189551, #68173, #114679, #176375, #51023, #147027, #161189, #8511, #21681, #70189, #131857, #55014, #19690, #173385, #112684, #174376, #35846, #97492, #180388, #136830, #118696, #56011, #132852, #88335, #178374, #12522, #89339, #86346, #151031, #150026, #181373, #166197, #197526, #102522, #149034, #74186, #148033, #87348, #198513, #58995, #195549, #120661, #41858, #196549, #10522, #75158, #103525, #182359, #116684, #119689, #133859, #43837, #90321, #194540, #104516, #152007, #72185, #117689, #134871, #135856, #179386, #42851, #105501, #167187, #165200, #40848, #9522, #39838, #11531, #26695, #28686, #13493, #57023, #71188, #101504, #73201, #58019, #164205, #27698, #163193, #24697, #25703, #92303, #139791, #153986, #199505, #169144, #63965, #183346, #61959, #290, #121651, #91291, #1279, #123626, #44828, #122645, #186331, #124637, #125635, #31643, #59984, #106483, #154977, #62956, #77140, #184335, #47814, #109463, #168162, #171146, #93292, #152982, #15483, #46812, #138809, #29659, #14481, #60971, #45817, #76143, #30649, #107468, #137821, #108471, #32635, #185321, #170149, #16473, #78122, #94289, #155967, #17464, #79121, #140794, #2282, #121314, #60626, #43498, #57682, #44490, #14134, #118351, #28352, #75801, #72854, #41514, #58655, #74829, #180045, #166850, #136490, #198170, #104172, #164857, #71837, #102174, #73849, #150687, #13165, #183006, #134524, #133506, #59640, #11179, #120321, #195198, #12185, #135520, #197191, #106146, #119350, #151671, #181034, #26353, #196210, #199159, #25361, #182015, #88996, #163862, #56678, #167828, #105164, #87002, #87993, #29328, #90957, #122300, #89990, #40502, #148689, #152644, #137479, #42508, #103177, #10177, #149681, #165854, #27350, #103971, #102969 ) ),
 .UNSPECIFIED., .T., .F., .F. ) 
 B_SPLINE_SURFACE_WITH_KNOTS ( ( 4, 3, 4 ),
 ( 3, 2, 2, 2, 2, 2, 2, 2, 2, 2, 2, 2, 2, 2, 2, 2, 2, 2, 2, 2, 2, 2, 2, 2, 2, 2, 2, 2, 2, 2, 2, 2, 2, 2, 2, 2, 2, 2, 2, 2, 2, 2, 2, 2, 2, 2, 2, 2, 2, 2, 2, 2, 2, 2, 2, 2, 2, 2, 2, 2, 2, 2, 2, 2, 2, 2, 2, 2, 2, 2, 2, 2, 2, 2, 2, 2, 2, 2, 2, 2, 2, 2, 2, 2, 2, 2, 2, 2, 2, 2, 2, 2, 2, 2, 2, 2, 2, 2, 2, 2, 2, 2, 2, 2, 2, 2, 2, 2, 2, 2, 2, 2, 2, 2, 2, 2, 2, 2, 2, 2, 2, 2, 2, 2, 2, 2, 2, 2, 2, 2, 2, 2, 2, 2, 2, 2, 2, 2, 2, 2, 2, 2, 2, 2, 2, 2, 2, 2, 2, 2, 2, 2, 2, 2, 2, 2, 2, 2, 2, 2, 2, 2, 2, 2, 2, 2, 2, 2, 2, 2, 2, 2, 2, 2, 2, 2, 2, 2, 2, 2, 2, 2, 2, 2, 2, 2, 2, 2, 2, 2, 2, 2, 2, 2, 2, 2, 2, 2, 2, 2, 2, 2, 2, 2, 2, 2, 2, 2, 2, 2, 2, 2, 2, 2, 2, 2, 2, 2, 2, 2, 2, 2, 2, 2, 2, 2, 2, 2, 3 ),
 ( 0.000000000000000000, 0.5000000000000000000, 1.000000000000000000 ),
 ( 0.000000000000000000, 0.004385964912280701511, 0.008771929824561403022, 0.01315789473684210453, 0.01754385964912280604, 0.02192982456140350755, 0.02631578947368420907, 0.03070175438596491058, 0.03508771929824561209, 0.03947368421052631360, 0.04385964912280701511, 0.04824561403508771662, 0.05263157894736841813, 0.05701754385964911964, 0.06140350877192982115, 0.06578947368421052266, 0.07017543859649122417, 0.07456140350877192569, 0.07894736842105262720, 0.08333333333333332871, 0.08771929824561403022, 0.09210526315789473173, 0.09649122807017543324, 0.1008771929824561348, 0.1052631578947368363, 0.1096491228070175378, 0.1140350877192982393, 0.1184210526315789408, 0.1228070175438596423, 0.1271929824561403577, 0.1315789473684210453, 0.1359649122807017607, 0.1403508771929824483, 0.1447368421052631637, 0.1491228070175438514, 0.1535087719298245668, 0.1578947368421052544, 0.1622807017543859698, 0.1666666666666666574, 0.1710526315789473728, 0.1754385964912280604, 0.1798245614035087758, 0.1842105263157894635, 0.1885964912280701788, 0.1929824561403508665, 0.1973684210526315819, 0.2017543859649122695, 0.2061403508771929849, 0.2105263157894736725, 0.2149122807017543879, 0.2192982456140350755, 0.2236842105263157909, 0.2280701754385964786, 0.2324561403508771940, 0.2368421052631578816, 0.2412280701754385970, 0.2456140350877192846, 0.2500000000000000000, 0.2543859649122807154, 0.2587719298245614308, 0.2631578947368420907, 0.2675438596491228060, 0.2719298245614035214, 0.2763157894736842368, 0.2807017543859648967, 0.2850877192982456121, 0.2894736842105263275, 0.2938596491228070429, 0.2982456140350877027, 0.3026315789473684181, 0.3070175438596491335, 0.3114035087719298489, 0.3157894736842105088, 0.3201754385964912242, 0.3245614035087719396, 0.3289473684210526550, 0.3333333333333333148, 0.3377192982456140302, 0.3421052631578947456, 0.3464912280701754610, 0.3508771929824561209, 0.3552631578947368363, 0.3596491228070175517, 0.3640350877192982670, 0.3684210526315789269, 0.3728070175438596423, 0.3771929824561403577, 0.3815789473684210731, 0.3859649122807017330, 0.3903508771929824483, 0.3947368421052631637, 0.3991228070175438791, 0.4035087719298245390, 0.4078947368421052544, 0.4122807017543859698, 0.4166666666666666852, 0.4210526315789473450, 0.4254385964912280604, 0.4298245614035087758, 0.4342105263157894912, 0.4385964912280701511, 0.4429824561403508665, 0.4473684210526315819, 0.4517543859649122973, 0.4561403508771929571, 0.4605263157894736725, 0.4649122807017543879, 0.4692982456140351033, 0.4736842105263157632, 0.4780701754385964786, 0.4824561403508771940, 0.4868421052631579093, 0.4912280701754385692, 0.4956140350877192846, 0.5000000000000000000, 0.5043859649122807154, 0.5087719298245614308, 0.5131578947368421462, 0.5175438596491228616, 0.5219298245614034659, 0.5263157894736841813, 0.5307017543859648967, 0.5350877192982456121, 0.5394736842105263275, 0.5438596491228070429, 0.5482456140350877583, 0.5526315789473684736, 0.5570175438596490780, 0.5614035087719297934, 0.5657894736842105088, 0.5701754385964912242, 0.5745614035087719396, 0.5789473684210526550, 0.5833333333333333703, 0.5877192982456140857, 0.5921052631578946901, 0.5964912280701754055, 0.6008771929824561209, 0.6052631578947368363, 0.6096491228070175517, 0.6140350877192982670, 0.6184210526315789824, 0.6228070175438596978, 0.6271929824561403022, 0.6315789473684210176, 0.6359649122807017330, 0.6403508771929824483, 0.6447368421052631637, 0.6491228070175438791, 0.6535087719298245945, 0.6578947368421053099, 0.6622807017543859143, 0.6666666666666666297, 0.6710526315789473450, 0.6754385964912280604, 0.6798245614035087758, 0.6842105263157894912, 0.6885964912280702066, 0.6929824561403509220, 0.6973684210526315264, 0.7017543859649122417, 0.7061403508771929571, 0.7105263157894736725, 0.7149122807017543879, 0.7192982456140351033, 0.7236842105263158187, 0.7280701754385965341, 0.7324561403508771384, 0.7368421052631578538, 0.7412280701754385692, 0.7456140350877192846, 0.7500000000000000000, 0.7543859649122807154, 0.7587719298245614308, 0.7631578947368421462, 0.7675438596491228616, 0.7719298245614034659, 0.7763157894736841813, 0.7807017543859648967, 0.7850877192982456121, 0.7894736842105263275, 0.7938596491228070429, 0.7982456140350877583, 0.8026315789473684736, 0.8070175438596490780, 0.8114035087719297934, 0.8157894736842105088, 0.8201754385964912242, 0.8245614035087719396, 0.8289473684210526550, 0.8333333333333333703, 0.8377192982456140857, 0.8421052631578946901, 0.8464912280701754055, 0.8508771929824561209, 0.8552631578947368363, 0.8596491228070175517, 0.8640350877192982670, 0.8684210526315789824, 0.8728070175438596978, 0.8771929824561403022, 0.8815789473684210176, 0.8859649122807017330, 0.8903508771929824483, 0.8947368421052631637, 0.8991228070175438791, 0.9035087719298245945, 0.9078947368421053099, 0.9122807017543859143, 0.9166666666666666297, 0.9210526315789473450, 0.9254385964912280604, 0.9298245614035087758, 0.9342105263157894912, 0.9385964912280702066, 0.9429824561403509220, 0.9473684210526315264, 0.9517543859649122417, 0.9561403508771929571, 0.9605263157894736725, 0.9649122807017543879, 0.9692982456140351033, 0.9736842105263158187, 0.9780701754385965341, 0.9824561403508771384, 0.9868421052631578538, 0.9912280701754385692, 0.9956140350877192846, 1.000000000000000000 ),
 .UNSPECIFIED. ) 
 GEOMETRIC_REPRESENTATION_ITEM ( )  RATIONAL_B_SPLINE_SURFACE ( (
 ( 1.000000000000000000, 0.9659258262890683122, 1.000000000000000000, 0.9659258262890683122, 1.000000000000000000, 0.9659258262890683122, 1.000000000000000000, 0.9659258262890683122, 1.000000000000000000, 0.9659258262890683122, 1.000000000000000000, 0.9659258262890683122, 1.000000000000000000, 0.9659258262890683122, 1.000000000000000000, 0.9659258262890683122, 1.000000000000000000, 0.9659258262890683122, 1.000000000000000000, 0.9659258262890683122, 1.000000000000000000, 0.9659258262890683122, 1.000000000000000000, 0.9659258262890683122, 1.000000000000000000, 0.9659258262890683122, 1.000000000000000000, 0.9659258262890683122, 1.000000000000000000, 0.9659258262890683122, 1.000000000000000000, 0.9659258262890683122, 1.000000000000000000, 0.9659258262890683122, 1.000000000000000000, 0.9659258262890683122, 1.000000000000000000, 0.9659258262890683122, 1.000000000000000000, 0.9659258262890683122, 1.000000000000000000, 0.9659258262890683122, 1.000000000000000000, 0.9659258262890683122, 1.000000000000000000, 0.9659258262890683122, 1.000000000000000000, 0.9659258262890683122, 1.000000000000000000, 0.9659258262890683122, 1.000000000000000000, 0.9659258262890683122, 1.000000000000000000, 0.9659258262890683122, 1.000000000000000000, 0.9659258262890683122, 1.000000000000000000, 0.9659258262890683122, 1.000000000000000000, 0.9659258262890683122, 1.000000000000000000, 0.9659258262890683122, 1.000000000000000000, 0.9659258262890683122, 1.000000000000000000, 0.9659258262890683122, 1.000000000000000000, 0.9659258262890683122, 1.000000000000000000, 0.9659258262890683122, 1.000000000000000000, 0.9659258262890683122, 1.000000000000000000, 0.9659258262890683122, 1.000000000000000000, 0.9659258262890683122, 1.000000000000000000, 0.9659258262890683122, 1.000000000000000000, 0.9659258262890683122, 1.000000000000000000, 0.9659258262890683122, 1.000000000000000000, 0.9659258262890683122, 1.000000000000000000, 0.9659258262890683122, 1.000000000000000000, 0.9659258262890683122, 1.000000000000000000, 0.9659258262890683122, 1.000000000000000000, 0.9659258262890683122, 1.000000000000000000, 0.9659258262890683122, 1.000000000000000000, 0.9659258262890683122, 1.000000000000000000, 0.9659258262890683122, 1.000000000000000000, 0.9659258262890683122, 1.000000000000000000, 0.9659258262890683122, 1.000000000000000000, 0.9659258262890683122, 1.000000000000000000, 0.9659258262890683122, 1.000000000000000000, 0.9659258262890683122, 1.000000000000000000, 0.9659258262890683122, 1.000000000000000000, 0.9659258262890683122, 1.000000000000000000, 0.9659258262890683122, 1.000000000000000000, 0.9659258262890683122, 1.000000000000000000, 0.9659258262890683122, 1.000000000000000000, 0.9659258262890683122, 1.000000000000000000, 0.9659258262890683122, 1.000000000000000000, 0.9659258262890683122, 1.000000000000000000, 0.9659258262890683122, 1.000000000000000000, 0.9659258262890683122, 1.000000000000000000, 0.9659258262890683122, 1.000000000000000000, 0.9659258262890683122, 1.000000000000000000, 0.9659258262890683122, 1.000000000000000000, 0.9659258262890683122, 1.000000000000000000, 0.9659258262890683122, 1.000000000000000000, 0.9659258262890683122, 1.000000000000000000, 0.9659258262890683122, 1.000000000000000000, 0.9659258262890683122, 1.000000000000000000, 0.9659258262890683122, 1.000000000000000000, 0.9659258262890683122, 1.000000000000000000, 0.9659258262890683122, 1.000000000000000000, 0.9659258262890683122, 1.000000000000000000, 0.9659258262890683122, 1.000000000000000000, 0.9659258262890683122, 1.000000000000000000, 0.9659258262890683122, 1.000000000000000000, 0.9659258262890683122, 1.000000000000000000, 0.9659258262890683122, 1.000000000000000000, 0.9659258262890683122, 1.000000000000000000, 0.9659258262890683122, 1.000000000000000000, 0.9659258262890683122, 1.000000000000000000, 0.9659258262890683122, 1.000000000000000000, 0.9659258262890683122, 1.000000000000000000, 0.9659258262890683122, 1.000000000000000000, 0.9659258262890683122, 1.000000000000000000, 0.9659258262890683122, 1.000000000000000000, 0.9659258262890683122, 1.000000000000000000, 0.9659258262890683122, 1.000000000000000000, 0.9659258262890683122, 1.000000000000000000, 0.9659258262890683122, 1.000000000000000000, 0.9659258262890683122, 1.000000000000000000, 0.9659258262890683122, 1.000000000000000000, 0.9659258262890683122, 1.000000000000000000, 0.9659258262890683122, 1.000000000000000000, 0.9659258262890683122, 1.000000000000000000, 0.9659258262890683122, 1.000000000000000000, 0.9659258262890683122, 1.000000000000000000, 0.9659258262890683122, 1.000000000000000000, 0.9659258262890683122, 1.000000000000000000, 0.9659258262890683122, 1.000000000000000000, 0.9659258262890683122, 1.000000000000000000, 0.9659258262890683122, 1.000000000000000000, 0.9659258262890683122, 1.000000000000000000, 0.9659258262890683122, 1.000000000000000000, 0.9659258262890683122, 1.000000000000000000, 0.9659258262890683122, 1.000000000000000000, 0.9659258262890683122, 1.000000000000000000, 0.9659258262890683122, 1.000000000000000000, 0.9659258262890683122, 1.000000000000000000, 0.9659258262890683122, 1.000000000000000000, 0.9659258262890683122, 1.000000000000000000, 0.9659258262890683122, 1.000000000000000000, 0.9659258262890683122, 1.000000000000000000, 0.9659258262890683122, 1.000000000000000000, 0.9659258262890683122, 1.000000000000000000, 0.9659258262890683122, 1.000000000000000000, 0.9659258262890683122, 1.000000000000000000, 0.9659258262890683122, 1.000000000000000000, 0.9659258262890683122, 1.000000000000000000, 0.9659258262890683122, 1.000000000000000000, 0.9659258262890683122, 1.000000000000000000, 0.9659258262890683122, 1.000000000000000000, 0.9659258262890683122, 1.000000000000000000, 0.9659258262890683122, 1.000000000000000000, 0.9659258262890683122, 1.000000000000000000, 0.9659258262890683122, 1.000000000000000000, 0.9659258262890683122, 1.000000000000000000, 0.9659258262890683122, 1.000000000000000000, 0.9659258262890683122, 1.000000000000000000, 0.9659258262890683122, 1.000000000000000000, 0.9659258262890683122, 1.000000000000000000, 0.9659258262890683122, 1.000000000000000000, 0.9659258262890683122, 1.000000000000000000, 0.9659258262890683122, 1.000000000000000000, 0.9659258262890683122, 1.000000000000000000, 0.9659258262890683122, 1.000000000000000000, 0.9659258262890683122, 1.000000000000000000, 0.9659258262890683122, 1.000000000000000000, 0.9659258262890683122, 1.000000000000000000, 0.9659258262890683122, 1.000000000000000000, 0.9659258262890683122, 1.000000000000000000, 0.9659258262890683122, 1.000000000000000000, 0.9659258262890683122, 1.000000000000000000, 0.9659258262890683122, 1.000000000000000000, 0.9659258262890683122, 1.000000000000000000, 0.9659258262890683122, 1.000000000000000000, 0.9659258262890683122, 1.000000000000000000, 0.9659258262890683122, 1.000000000000000000, 0.9659258262890683122, 1.000000000000000000, 0.9659258262890683122, 1.000000000000000000, 0.9659258262890683122, 1.000000000000000000, 0.9659258262890683122, 1.000000000000000000, 0.9659258262890683122, 1.000000000000000000, 0.9659258262890683122, 1.000000000000000000, 0.9659258262890683122, 1.000000000000000000, 0.9659258262890683122, 1.000000000000000000, 0.9659258262890683122, 1.000000000000000000, 0.9659258262890683122, 1.000000000000000000, 0.9659258262890683122, 1.000000000000000000, 0.9659258262890683122, 1.000000000000000000, 0.9659258262890683122, 1.000000000000000000, 0.9659258262890683122, 1.000000000000000000, 0.9659258262890683122, 1.000000000000000000, 0.9659258262890683122, 1.000000000000000000, 0.9659258262890683122, 1.000000000000000000, 0.9659258262890683122, 1.000000000000000000, 0.9659258262890683122, 1.000000000000000000, 0.9659258262890683122, 1.000000000000000000, 0.9659258262890683122, 1.000000000000000000, 0.9659258262890683122, 1.000000000000000000, 0.9659258262890683122, 1.000000000000000000, 0.9659258262890683122, 1.000000000000000000, 0.9659258262890683122, 1.000000000000000000, 0.9659258262890683122, 1.000000000000000000, 0.9659258262890683122, 1.000000000000000000, 0.9659258262890683122, 1.000000000000000000, 0.9659258262890683122, 1.000000000000000000, 0.9659258262890683122, 1.000000000000000000, 0.9659258262890683122, 1.000000000000000000, 0.9659258262890683122, 1.000000000000000000, 0.9659258262890683122, 1.000000000000000000, 0.9659258262890683122, 1.000000000000000000, 0.9659258262890683122, 1.000000000000000000, 0.9659258262890683122, 1.000000000000000000, 0.9659258262890683122, 1.000000000000000000, 0.9659258262890683122, 1.000000000000000000, 0.9659258262890683122, 1.000000000000000000, 0.9659258262890683122, 1.000000000000000000, 0.9659258262890683122, 1.000000000000000000, 0.9659258262890683122, 1.000000000000000000, 0.9659258262890683122, 1.000000000000000000, 0.9659258262890683122, 1.000000000000000000, 0.9659258262890683122, 1.000000000000000000, 0.9659258262890683122, 1.000000000000000000, 0.9659258262890683122, 1.000000000000000000, 0.9659258262890683122, 1.000000000000000000, 0.9659258262890683122, 1.000000000000000000, 0.9659258262890683122, 1.000000000000000000, 0.9659258262890683122, 1.000000000000000000, 0.9659258262890683122, 1.000000000000000000, 0.9659258262890683122, 1.000000000000000000, 0.9659258262890683122, 1.000000000000000000, 0.9659258262890683122, 1.000000000000000000, 0.9659258262890683122, 1.000000000000000000, 0.9659258262890683122, 1.000000000000000000, 0.9659258262890683122, 1.000000000000000000, 0.9659258262890683122, 1.000000000000000000, 0.9659258262890683122, 1.000000000000000000, 0.9659258262890683122, 1.000000000000000000, 0.9659258262890683122, 1.000000000000000000, 0.9659258262890683122, 1.000000000000000000, 0.9659258262890683122, 1.000000000000000000, 0.9659258262890683122, 1.000000000000000000, 0.9659258262890683122, 1.000000000000000000, 0.9659258262890683122, 1.000000000000000000, 0.9659258262890683122, 1.000000000000000000, 0.9659258262890683122, 1.000000000000000000, 0.9659258262890683122, 1.000000000000000000, 0.9659258262890683122, 1.000000000000000000, 0.9659258262890683122, 1.000000000000000000, 0.9659258262890683122, 1.000000000000000000, 0.9659258262890683122, 1.000000000000000000, 0.9659258262890683122, 1.000000000000000000, 0.9659258262890683122, 1.000000000000000000, 0.9659258262890683122, 1.000000000000000000),
 ( 0.3333333333333333703, 0.3219752754296894559, 0.3333333333333333703, 0.3219752754296894559, 0.3333333333333333703, 0.3219752754296894559, 0.3333333333333333703, 0.3219752754296894559, 0.3333333333333333703, 0.3219752754296894559, 0.3333333333333333703, 0.3219752754296894559, 0.3333333333333333703, 0.3219752754296894559, 0.3333333333333333703, 0.3219752754296894559, 0.3333333333333333703, 0.3219752754296894559, 0.3333333333333333703, 0.3219752754296894559, 0.3333333333333333703, 0.3219752754296894559, 0.3333333333333333703, 0.3219752754296894559, 0.3333333333333333703, 0.3219752754296894559, 0.3333333333333333703, 0.3219752754296894559, 0.3333333333333333703, 0.3219752754296894559, 0.3333333333333333703, 0.3219752754296894559, 0.3333333333333333703, 0.3219752754296894559, 0.3333333333333333703, 0.3219752754296894559, 0.3333333333333333703, 0.3219752754296894559, 0.3333333333333333703, 0.3219752754296894559, 0.3333333333333333703, 0.3219752754296894559, 0.3333333333333333703, 0.3219752754296894559, 0.3333333333333333703, 0.3219752754296894559, 0.3333333333333333703, 0.3219752754296894559, 0.3333333333333333703, 0.3219752754296894559, 0.3333333333333333703, 0.3219752754296894559, 0.3333333333333333703, 0.3219752754296894559, 0.3333333333333333703, 0.3219752754296894559, 0.3333333333333333703, 0.3219752754296894559, 0.3333333333333333703, 0.3219752754296894559, 0.3333333333333333703, 0.3219752754296894559, 0.3333333333333333703, 0.3219752754296894559, 0.3333333333333333703, 0.3219752754296894559, 0.3333333333333333703, 0.3219752754296894559, 0.3333333333333333703, 0.3219752754296894559, 0.3333333333333333703, 0.3219752754296894559, 0.3333333333333333703, 0.3219752754296894559, 0.3333333333333333703, 0.3219752754296894559, 0.3333333333333333703, 0.3219752754296894559, 0.3333333333333333703, 0.3219752754296894559, 0.3333333333333333703, 0.3219752754296894559, 0.3333333333333333703, 0.3219752754296894559, 0.3333333333333333703, 0.3219752754296894559, 0.3333333333333333703, 0.3219752754296894559, 0.3333333333333333703, 0.3219752754296894559, 0.3333333333333333703, 0.3219752754296894559, 0.3333333333333333703, 0.3219752754296894559, 0.3333333333333333703, 0.3219752754296894559, 0.3333333333333333703, 0.3219752754296894559, 0.3333333333333333703, 0.3219752754296894559, 0.3333333333333333703, 0.3219752754296894559, 0.3333333333333333703, 0.3219752754296894559, 0.3333333333333333703, 0.3219752754296894559, 0.3333333333333333703, 0.3219752754296894559, 0.3333333333333333703, 0.3219752754296894559, 0.3333333333333333703, 0.3219752754296894559, 0.3333333333333333703, 0.3219752754296894559, 0.3333333333333333703, 0.3219752754296894559, 0.3333333333333333703, 0.3219752754296894559, 0.3333333333333333703, 0.3219752754296894559, 0.3333333333333333703, 0.3219752754296894559, 0.3333333333333333703, 0.3219752754296894559, 0.3333333333333333703, 0.3219752754296894559, 0.3333333333333333703, 0.3219752754296894559, 0.3333333333333333703, 0.3219752754296894559, 0.3333333333333333703, 0.3219752754296894559, 0.3333333333333333703, 0.3219752754296894559, 0.3333333333333333703, 0.3219752754296894559, 0.3333333333333333703, 0.3219752754296894559, 0.3333333333333333703, 0.3219752754296894559, 0.3333333333333333703, 0.3219752754296894559, 0.3333333333333333703, 0.3219752754296894559, 0.3333333333333333703, 0.3219752754296894559, 0.3333333333333333703, 0.3219752754296894559, 0.3333333333333333703, 0.3219752754296894559, 0.3333333333333333703, 0.3219752754296894559, 0.3333333333333333703, 0.3219752754296894559, 0.3333333333333333703, 0.3219752754296894559, 0.3333333333333333703, 0.3219752754296894559, 0.3333333333333333703, 0.3219752754296894559, 0.3333333333333333703, 0.3219752754296894559, 0.3333333333333333703, 0.3219752754296894559, 0.3333333333333333703, 0.3219752754296894559, 0.3333333333333333703, 0.3219752754296894559, 0.3333333333333333703, 0.3219752754296894559, 0.3333333333333333703, 0.3219752754296894559, 0.3333333333333333703, 0.3219752754296894559, 0.3333333333333333703, 0.3219752754296894559, 0.3333333333333333703, 0.3219752754296894559, 0.3333333333333333703, 0.3219752754296894559, 0.3333333333333333703, 0.3219752754296894559, 0.3333333333333333703, 0.3219752754296894559, 0.3333333333333333703, 0.3219752754296894559, 0.3333333333333333703, 0.3219752754296894559, 0.3333333333333333703, 0.3219752754296894559, 0.3333333333333333703, 0.3219752754296894559, 0.3333333333333333703, 0.3219752754296894559, 0.3333333333333333703, 0.3219752754296894559, 0.3333333333333333703, 0.3219752754296894559, 0.3333333333333333703, 0.3219752754296894559, 0.3333333333333333703, 0.3219752754296894559, 0.3333333333333333703, 0.3219752754296894559, 0.3333333333333333703, 0.3219752754296894559, 0.3333333333333333703, 0.3219752754296894559, 0.3333333333333333703, 0.3219752754296894559, 0.3333333333333333703, 0.3219752754296894559, 0.3333333333333333703, 0.3219752754296894559, 0.3333333333333333703, 0.3219752754296894559, 0.3333333333333333703, 0.3219752754296894559, 0.3333333333333333703, 0.3219752754296894559, 0.3333333333333333703, 0.3219752754296894559, 0.3333333333333333703, 0.3219752754296894559, 0.3333333333333333703, 0.3219752754296894559, 0.3333333333333333703, 0.3219752754296894559, 0.3333333333333333703, 0.3219752754296894559, 0.3333333333333333703, 0.3219752754296894559, 0.3333333333333333703, 0.3219752754296894559, 0.3333333333333333703, 0.3219752754296894559, 0.3333333333333333703, 0.3219752754296894559, 0.3333333333333333703, 0.3219752754296894559, 0.3333333333333333703, 0.3219752754296894559, 0.3333333333333333703, 0.3219752754296894559, 0.3333333333333333703, 0.3219752754296894559, 0.3333333333333333703, 0.3219752754296894559, 0.3333333333333333703, 0.3219752754296894559, 0.3333333333333333703, 0.3219752754296894559, 0.3333333333333333703, 0.3219752754296894559, 0.3333333333333333703, 0.3219752754296894559, 0.3333333333333333703, 0.3219752754296894559, 0.3333333333333333703, 0.3219752754296894559, 0.3333333333333333703, 0.3219752754296894559, 0.3333333333333333703, 0.3219752754296894559, 0.3333333333333333703, 0.3219752754296894559, 0.3333333333333333703, 0.3219752754296894559, 0.3333333333333333703, 0.3219752754296894559, 0.3333333333333333703, 0.3219752754296894559, 0.3333333333333333703, 0.3219752754296894559, 0.3333333333333333703, 0.3219752754296894559, 0.3333333333333333703, 0.3219752754296894559, 0.3333333333333333703, 0.3219752754296894559, 0.3333333333333333703, 0.3219752754296894559, 0.3333333333333333703, 0.3219752754296894559, 0.3333333333333333703, 0.3219752754296894559, 0.3333333333333333703, 0.3219752754296894559, 0.3333333333333333703, 0.3219752754296894559, 0.3333333333333333703, 0.3219752754296894559, 0.3333333333333333703, 0.3219752754296894559, 0.3333333333333333703, 0.3219752754296894559, 0.3333333333333333703, 0.3219752754296894559, 0.3333333333333333703, 0.3219752754296894559, 0.3333333333333333703, 0.3219752754296894559, 0.3333333333333333703, 0.3219752754296894559, 0.3333333333333333703, 0.3219752754296894559, 0.3333333333333333703, 0.3219752754296894559, 0.3333333333333333703, 0.3219752754296894559, 0.3333333333333333703, 0.3219752754296894559, 0.3333333333333333703, 0.3219752754296894559, 0.3333333333333333703, 0.3219752754296894559, 0.3333333333333333703, 0.3219752754296894559, 0.3333333333333333703, 0.3219752754296894559, 0.3333333333333333703, 0.3219752754296894559, 0.3333333333333333703, 0.3219752754296894559, 0.3333333333333333703, 0.3219752754296894559, 0.3333333333333333703, 0.3219752754296894559, 0.3333333333333333703, 0.3219752754296894559, 0.3333333333333333703, 0.3219752754296894559, 0.3333333333333333703, 0.3219752754296894559, 0.3333333333333333703, 0.3219752754296894559, 0.3333333333333333703, 0.3219752754296894559, 0.3333333333333333703, 0.3219752754296894559, 0.3333333333333333703, 0.3219752754296894559, 0.3333333333333333703, 0.3219752754296894559, 0.3333333333333333703, 0.3219752754296894559, 0.3333333333333333703, 0.3219752754296894559, 0.3333333333333333703, 0.3219752754296894559, 0.3333333333333333703, 0.3219752754296894559, 0.3333333333333333703, 0.3219752754296894559, 0.3333333333333333703, 0.3219752754296894559, 0.3333333333333333703, 0.3219752754296894559, 0.3333333333333333703, 0.3219752754296894559, 0.3333333333333333703, 0.3219752754296894559, 0.3333333333333333703, 0.3219752754296894559, 0.3333333333333333703, 0.3219752754296894559, 0.3333333333333333703, 0.3219752754296894559, 0.3333333333333333703, 0.3219752754296894559, 0.3333333333333333703, 0.3219752754296894559, 0.3333333333333333703, 0.3219752754296894559, 0.3333333333333333703, 0.3219752754296894559, 0.3333333333333333703, 0.3219752754296894559, 0.3333333333333333703, 0.3219752754296894559, 0.3333333333333333703, 0.3219752754296894559, 0.3333333333333333703, 0.3219752754296894559, 0.3333333333333333703, 0.3219752754296894559, 0.3333333333333333703, 0.3219752754296894559, 0.3333333333333333703, 0.3219752754296894559, 0.3333333333333333703, 0.3219752754296894559, 0.3333333333333333703, 0.3219752754296894559, 0.3333333333333333703, 0.3219752754296894559, 0.3333333333333333703, 0.3219752754296894559, 0.3333333333333333703, 0.3219752754296894559, 0.3333333333333333703, 0.3219752754296894559, 0.3333333333333333703, 0.3219752754296894559, 0.3333333333333333703, 0.3219752754296894559, 0.3333333333333333703, 0.3219752754296894559, 0.3333333333333333703, 0.3219752754296894559, 0.3333333333333333703, 0.3219752754296894559, 0.3333333333333333703, 0.3219752754296894559, 0.3333333333333333703, 0.3219752754296894559, 0.3333333333333333703, 0.3219752754296894559, 0.3333333333333333703, 0.3219752754296894559, 0.3333333333333333703, 0.3219752754296894559, 0.3333333333333333703, 0.3219752754296894559, 0.3333333333333333703, 0.3219752754296894559, 0.3333333333333333703, 0.3219752754296894559, 0.3333333333333333703, 0.3219752754296894559, 0.3333333333333333703, 0.3219752754296894559, 0.3333333333333333703, 0.3219752754296894559, 0.3333333333333333703, 0.3219752754296894559, 0.3333333333333333703, 0.3219752754296894559, 0.3333333333333333703, 0.3219752754296894559, 0.3333333333333333703, 0.3219752754296894559, 0.3333333333333333703, 0.3219752754296894559, 0.3333333333333333703, 0.3219752754296894559, 0.3333333333333333703, 0.3219752754296894559, 0.3333333333333333703, 0.3219752754296894559, 0.3333333333333333703, 0.3219752754296894559, 0.3333333333333333703, 0.3219752754296894559, 0.3333333333333333703, 0.3219752754296894559, 0.3333333333333333703),
 ( 0.3333333333333333703, 0.3219752754296894559, 0.3333333333333333703, 0.3219752754296894559, 0.3333333333333333703, 0.3219752754296894559, 0.3333333333333333703, 0.3219752754296894559, 0.3333333333333333703, 0.3219752754296894559, 0.3333333333333333703, 0.3219752754296894559, 0.3333333333333333703, 0.3219752754296894559, 0.3333333333333333703, 0.3219752754296894559, 0.3333333333333333703, 0.3219752754296894559, 0.3333333333333333703, 0.3219752754296894559, 0.3333333333333333703, 0.3219752754296894559, 0.3333333333333333703, 0.3219752754296894559, 0.3333333333333333703, 0.3219752754296894559, 0.3333333333333333703, 0.3219752754296894559, 0.3333333333333333703, 0.3219752754296894559, 0.3333333333333333703, 0.3219752754296894559, 0.3333333333333333703, 0.3219752754296894559, 0.3333333333333333703, 0.3219752754296894559, 0.3333333333333333703, 0.3219752754296894559, 0.3333333333333333703, 0.3219752754296894559, 0.3333333333333333703, 0.3219752754296894559, 0.3333333333333333703, 0.3219752754296894559, 0.3333333333333333703, 0.3219752754296894559, 0.3333333333333333703, 0.3219752754296894559, 0.3333333333333333703, 0.3219752754296894559, 0.3333333333333333703, 0.3219752754296894559, 0.3333333333333333703, 0.3219752754296894559, 0.3333333333333333703, 0.3219752754296894559, 0.3333333333333333703, 0.3219752754296894559, 0.3333333333333333703, 0.3219752754296894559, 0.3333333333333333703, 0.3219752754296894559, 0.3333333333333333703, 0.3219752754296894559, 0.3333333333333333703, 0.3219752754296894559, 0.3333333333333333703, 0.3219752754296894559, 0.3333333333333333703, 0.3219752754296894559, 0.3333333333333333703, 0.3219752754296894559, 0.3333333333333333703, 0.3219752754296894559, 0.3333333333333333703, 0.3219752754296894559, 0.3333333333333333703, 0.3219752754296894559, 0.3333333333333333703, 0.3219752754296894559, 0.3333333333333333703, 0.3219752754296894559, 0.3333333333333333703, 0.3219752754296894559, 0.3333333333333333703, 0.3219752754296894559, 0.3333333333333333703, 0.3219752754296894559, 0.3333333333333333703, 0.3219752754296894559, 0.3333333333333333703, 0.3219752754296894559, 0.3333333333333333703, 0.3219752754296894559, 0.3333333333333333703, 0.3219752754296894559, 0.3333333333333333703, 0.3219752754296894559, 0.3333333333333333703, 0.3219752754296894559, 0.3333333333333333703, 0.3219752754296894559, 0.3333333333333333703, 0.3219752754296894559, 0.3333333333333333703, 0.3219752754296894559, 0.3333333333333333703, 0.3219752754296894559, 0.3333333333333333703, 0.3219752754296894559, 0.3333333333333333703, 0.3219752754296894559, 0.3333333333333333703, 0.3219752754296894559, 0.3333333333333333703, 0.3219752754296894559, 0.3333333333333333703, 0.3219752754296894559, 0.3333333333333333703, 0.3219752754296894559, 0.3333333333333333703, 0.3219752754296894559, 0.3333333333333333703, 0.3219752754296894559, 0.3333333333333333703, 0.3219752754296894559, 0.3333333333333333703, 0.3219752754296894559, 0.3333333333333333703, 0.3219752754296894559, 0.3333333333333333703, 0.3219752754296894559, 0.3333333333333333703, 0.3219752754296894559, 0.3333333333333333703, 0.3219752754296894559, 0.3333333333333333703, 0.3219752754296894559, 0.3333333333333333703, 0.3219752754296894559, 0.3333333333333333703, 0.3219752754296894559, 0.3333333333333333703, 0.3219752754296894559, 0.3333333333333333703, 0.3219752754296894559, 0.3333333333333333703, 0.3219752754296894559, 0.3333333333333333703, 0.3219752754296894559, 0.3333333333333333703, 0.3219752754296894559, 0.3333333333333333703, 0.3219752754296894559, 0.3333333333333333703, 0.3219752754296894559, 0.3333333333333333703, 0.3219752754296894559, 0.3333333333333333703, 0.3219752754296894559, 0.3333333333333333703, 0.3219752754296894559, 0.3333333333333333703, 0.3219752754296894559, 0.3333333333333333703, 0.3219752754296894559, 0.3333333333333333703, 0.3219752754296894559, 0.3333333333333333703, 0.3219752754296894559, 0.3333333333333333703, 0.3219752754296894559, 0.3333333333333333703, 0.3219752754296894559, 0.3333333333333333703, 0.3219752754296894559, 0.3333333333333333703, 0.3219752754296894559, 0.3333333333333333703, 0.3219752754296894559, 0.3333333333333333703, 0.3219752754296894559, 0.3333333333333333703, 0.3219752754296894559, 0.3333333333333333703, 0.3219752754296894559, 0.3333333333333333703, 0.3219752754296894559, 0.3333333333333333703, 0.3219752754296894559, 0.3333333333333333703, 0.3219752754296894559, 0.3333333333333333703, 0.3219752754296894559, 0.3333333333333333703, 0.3219752754296894559, 0.3333333333333333703, 0.3219752754296894559, 0.3333333333333333703, 0.3219752754296894559, 0.3333333333333333703, 0.3219752754296894559, 0.3333333333333333703, 0.3219752754296894559, 0.3333333333333333703, 0.3219752754296894559, 0.3333333333333333703, 0.3219752754296894559, 0.3333333333333333703, 0.3219752754296894559, 0.3333333333333333703, 0.3219752754296894559, 0.3333333333333333703, 0.3219752754296894559, 0.3333333333333333703, 0.3219752754296894559, 0.3333333333333333703, 0.3219752754296894559, 0.3333333333333333703, 0.3219752754296894559, 0.3333333333333333703, 0.3219752754296894559, 0.3333333333333333703, 0.3219752754296894559, 0.3333333333333333703, 0.3219752754296894559, 0.3333333333333333703, 0.3219752754296894559, 0.3333333333333333703, 0.3219752754296894559, 0.3333333333333333703, 0.3219752754296894559, 0.3333333333333333703, 0.3219752754296894559, 0.3333333333333333703, 0.3219752754296894559, 0.3333333333333333703, 0.3219752754296894559, 0.3333333333333333703, 0.3219752754296894559, 0.3333333333333333703, 0.3219752754296894559, 0.3333333333333333703, 0.3219752754296894559, 0.3333333333333333703, 0.3219752754296894559, 0.3333333333333333703, 0.3219752754296894559, 0.3333333333333333703, 0.3219752754296894559, 0.3333333333333333703, 0.3219752754296894559, 0.3333333333333333703, 0.3219752754296894559, 0.3333333333333333703, 0.3219752754296894559, 0.3333333333333333703, 0.3219752754296894559, 0.3333333333333333703, 0.3219752754296894559, 0.3333333333333333703, 0.3219752754296894559, 0.3333333333333333703, 0.3219752754296894559, 0.3333333333333333703, 0.3219752754296894559, 0.3333333333333333703, 0.3219752754296894559, 0.3333333333333333703, 0.3219752754296894559, 0.3333333333333333703, 0.3219752754296894559, 0.3333333333333333703, 0.3219752754296894559, 0.3333333333333333703, 0.3219752754296894559, 0.3333333333333333703, 0.3219752754296894559, 0.3333333333333333703, 0.3219752754296894559, 0.3333333333333333703, 0.3219752754296894559, 0.3333333333333333703, 0.3219752754296894559, 0.3333333333333333703, 0.3219752754296894559, 0.3333333333333333703, 0.3219752754296894559, 0.3333333333333333703, 0.3219752754296894559, 0.3333333333333333703, 0.3219752754296894559, 0.3333333333333333703, 0.3219752754296894559, 0.3333333333333333703, 0.3219752754296894559, 0.3333333333333333703, 0.3219752754296894559, 0.3333333333333333703, 0.3219752754296894559, 0.3333333333333333703, 0.3219752754296894559, 0.3333333333333333703, 0.3219752754296894559, 0.3333333333333333703, 0.3219752754296894559, 0.3333333333333333703, 0.3219752754296894559, 0.3333333333333333703, 0.3219752754296894559, 0.3333333333333333703, 0.3219752754296894559, 0.3333333333333333703, 0.3219752754296894559, 0.3333333333333333703, 0.3219752754296894559, 0.3333333333333333703, 0.3219752754296894559, 0.3333333333333333703, 0.3219752754296894559, 0.3333333333333333703, 0.3219752754296894559, 0.3333333333333333703, 0.3219752754296894559, 0.3333333333333333703, 0.3219752754296894559, 0.3333333333333333703, 0.3219752754296894559, 0.3333333333333333703, 0.3219752754296894559, 0.3333333333333333703, 0.3219752754296894559, 0.3333333333333333703, 0.3219752754296894559, 0.3333333333333333703, 0.3219752754296894559, 0.3333333333333333703, 0.3219752754296894559, 0.3333333333333333703, 0.3219752754296894559, 0.3333333333333333703, 0.3219752754296894559, 0.3333333333333333703, 0.3219752754296894559, 0.3333333333333333703, 0.3219752754296894559, 0.3333333333333333703, 0.3219752754296894559, 0.3333333333333333703, 0.3219752754296894559, 0.3333333333333333703, 0.3219752754296894559, 0.3333333333333333703, 0.3219752754296894559, 0.3333333333333333703, 0.3219752754296894559, 0.3333333333333333703, 0.3219752754296894559, 0.3333333333333333703, 0.3219752754296894559, 0.3333333333333333703, 0.3219752754296894559, 0.3333333333333333703, 0.3219752754296894559, 0.3333333333333333703, 0.3219752754296894559, 0.3333333333333333703, 0.3219752754296894559, 0.3333333333333333703, 0.3219752754296894559, 0.3333333333333333703, 0.3219752754296894559, 0.3333333333333333703, 0.3219752754296894559, 0.3333333333333333703, 0.3219752754296894559, 0.3333333333333333703, 0.3219752754296894559, 0.3333333333333333703, 0.3219752754296894559, 0.3333333333333333703, 0.3219752754296894559, 0.3333333333333333703, 0.3219752754296894559, 0.3333333333333333703, 0.3219752754296894559, 0.3333333333333333703, 0.3219752754296894559, 0.3333333333333333703, 0.3219752754296894559, 0.3333333333333333703, 0.3219752754296894559, 0.3333333333333333703, 0.3219752754296894559, 0.3333333333333333703, 0.3219752754296894559, 0.3333333333333333703, 0.3219752754296894559, 0.3333333333333333703, 0.3219752754296894559, 0.3333333333333333703, 0.3219752754296894559, 0.3333333333333333703, 0.3219752754296894559, 0.3333333333333333703, 0.3219752754296894559, 0.3333333333333333703, 0.3219752754296894559, 0.3333333333333333703, 0.3219752754296894559, 0.3333333333333333703, 0.3219752754296894559, 0.3333333333333333703, 0.3219752754296894559, 0.3333333333333333703, 0.3219752754296894559, 0.3333333333333333703, 0.3219752754296894559, 0.3333333333333333703, 0.3219752754296894559, 0.3333333333333333703, 0.3219752754296894559, 0.3333333333333333703, 0.3219752754296894559, 0.3333333333333333703, 0.3219752754296894559, 0.3333333333333333703, 0.3219752754296894559, 0.3333333333333333703, 0.3219752754296894559, 0.3333333333333333703, 0.3219752754296894559, 0.3333333333333333703, 0.3219752754296894559, 0.3333333333333333703, 0.3219752754296894559, 0.3333333333333333703, 0.3219752754296894559, 0.3333333333333333703, 0.3219752754296894559, 0.3333333333333333703, 0.3219752754296894559, 0.3333333333333333703, 0.3219752754296894559, 0.3333333333333333703, 0.3219752754296894559, 0.3333333333333333703, 0.3219752754296894559, 0.3333333333333333703, 0.3219752754296894559, 0.3333333333333333703, 0.3219752754296894559, 0.3333333333333333703, 0.3219752754296894559, 0.3333333333333333703, 0.3219752754296894559, 0.3333333333333333703),
 ( 1.000000000000000000, 0.9659258262890683122, 1.000000000000000000, 0.9659258262890683122, 1.000000000000000000, 0.9659258262890683122, 1.000000000000000000, 0.9659258262890683122, 1.000000000000000000, 0.9659258262890683122, 1.000000000000000000, 0.9659258262890683122, 1.000000000000000000, 0.9659258262890683122, 1.000000000000000000, 0.9659258262890683122, 1.000000000000000000, 0.9659258262890683122, 1.000000000000000000, 0.9659258262890683122, 1.000000000000000000, 0.9659258262890683122, 1.000000000000000000, 0.9659258262890683122, 1.000000000000000000, 0.9659258262890683122, 1.000000000000000000, 0.9659258262890683122, 1.000000000000000000, 0.9659258262890683122, 1.000000000000000000, 0.9659258262890683122, 1.000000000000000000, 0.9659258262890683122, 1.000000000000000000, 0.9659258262890683122, 1.000000000000000000, 0.9659258262890683122, 1.000000000000000000, 0.9659258262890683122, 1.000000000000000000, 0.9659258262890683122, 1.000000000000000000, 0.9659258262890683122, 1.000000000000000000, 0.9659258262890683122, 1.000000000000000000, 0.9659258262890683122, 1.000000000000000000, 0.9659258262890683122, 1.000000000000000000, 0.9659258262890683122, 1.000000000000000000, 0.9659258262890683122, 1.000000000000000000, 0.9659258262890683122, 1.000000000000000000, 0.9659258262890683122, 1.000000000000000000, 0.9659258262890683122, 1.000000000000000000, 0.9659258262890683122, 1.000000000000000000, 0.9659258262890683122, 1.000000000000000000, 0.9659258262890683122, 1.000000000000000000, 0.9659258262890683122, 1.000000000000000000, 0.9659258262890683122, 1.000000000000000000, 0.9659258262890683122, 1.000000000000000000, 0.9659258262890683122, 1.000000000000000000, 0.9659258262890683122, 1.000000000000000000, 0.9659258262890683122, 1.000000000000000000, 0.9659258262890683122, 1.000000000000000000, 0.9659258262890683122, 1.000000000000000000, 0.9659258262890683122, 1.000000000000000000, 0.9659258262890683122, 1.000000000000000000, 0.9659258262890683122, 1.000000000000000000, 0.9659258262890683122, 1.000000000000000000, 0.9659258262890683122, 1.000000000000000000, 0.9659258262890683122, 1.000000000000000000, 0.9659258262890683122, 1.000000000000000000, 0.9659258262890683122, 1.000000000000000000, 0.9659258262890683122, 1.000000000000000000, 0.9659258262890683122, 1.000000000000000000, 0.9659258262890683122, 1.000000000000000000, 0.9659258262890683122, 1.000000000000000000, 0.9659258262890683122, 1.000000000000000000, 0.9659258262890683122, 1.000000000000000000, 0.9659258262890683122, 1.000000000000000000, 0.9659258262890683122, 1.000000000000000000, 0.9659258262890683122, 1.000000000000000000, 0.9659258262890683122, 1.000000000000000000, 0.9659258262890683122, 1.000000000000000000, 0.9659258262890683122, 1.000000000000000000, 0.9659258262890683122, 1.000000000000000000, 0.9659258262890683122, 1.000000000000000000, 0.9659258262890683122, 1.000000000000000000, 0.9659258262890683122, 1.000000000000000000, 0.9659258262890683122, 1.000000000000000000, 0.9659258262890683122, 1.000000000000000000, 0.9659258262890683122, 1.000000000000000000, 0.9659258262890683122, 1.000000000000000000, 0.9659258262890683122, 1.000000000000000000, 0.9659258262890683122, 1.000000000000000000, 0.9659258262890683122, 1.000000000000000000, 0.9659258262890683122, 1.000000000000000000, 0.9659258262890683122, 1.000000000000000000, 0.9659258262890683122, 1.000000000000000000, 0.9659258262890683122, 1.000000000000000000, 0.9659258262890683122, 1.000000000000000000, 0.9659258262890683122, 1.000000000000000000, 0.9659258262890683122, 1.000000000000000000, 0.9659258262890683122, 1.000000000000000000, 0.9659258262890683122, 1.000000000000000000, 0.9659258262890683122, 1.000000000000000000, 0.9659258262890683122, 1.000000000000000000, 0.9659258262890683122, 1.000000000000000000, 0.9659258262890683122, 1.000000000000000000, 0.9659258262890683122, 1.000000000000000000, 0.9659258262890683122, 1.000000000000000000, 0.9659258262890683122, 1.000000000000000000, 0.9659258262890683122, 1.000000000000000000, 0.9659258262890683122, 1.000000000000000000, 0.9659258262890683122, 1.000000000000000000, 0.9659258262890683122, 1.000000000000000000, 0.9659258262890683122, 1.000000000000000000, 0.9659258262890683122, 1.000000000000000000, 0.9659258262890683122, 1.000000000000000000, 0.9659258262890683122, 1.000000000000000000, 0.9659258262890683122, 1.000000000000000000, 0.9659258262890683122, 1.000000000000000000, 0.9659258262890683122, 1.000000000000000000, 0.9659258262890683122, 1.000000000000000000, 0.9659258262890683122, 1.000000000000000000, 0.9659258262890683122, 1.000000000000000000, 0.9659258262890683122, 1.000000000000000000, 0.9659258262890683122, 1.000000000000000000, 0.9659258262890683122, 1.000000000000000000, 0.9659258262890683122, 1.000000000000000000, 0.9659258262890683122, 1.000000000000000000, 0.9659258262890683122, 1.000000000000000000, 0.9659258262890683122, 1.000000000000000000, 0.9659258262890683122, 1.000000000000000000, 0.9659258262890683122, 1.000000000000000000, 0.9659258262890683122, 1.000000000000000000, 0.9659258262890683122, 1.000000000000000000, 0.9659258262890683122, 1.000000000000000000, 0.9659258262890683122, 1.000000000000000000, 0.9659258262890683122, 1.000000000000000000, 0.9659258262890683122, 1.000000000000000000, 0.9659258262890683122, 1.000000000000000000, 0.9659258262890683122, 1.000000000000000000, 0.9659258262890683122, 1.000000000000000000, 0.9659258262890683122, 1.000000000000000000, 0.9659258262890683122, 1.000000000000000000, 0.9659258262890683122, 1.000000000000000000, 0.9659258262890683122, 1.000000000000000000, 0.9659258262890683122, 1.000000000000000000, 0.9659258262890683122, 1.000000000000000000, 0.9659258262890683122, 1.000000000000000000, 0.9659258262890683122, 1.000000000000000000, 0.9659258262890683122, 1.000000000000000000, 0.9659258262890683122, 1.000000000000000000, 0.9659258262890683122, 1.000000000000000000, 0.9659258262890683122, 1.000000000000000000, 0.9659258262890683122, 1.000000000000000000, 0.9659258262890683122, 1.000000000000000000, 0.9659258262890683122, 1.000000000000000000, 0.9659258262890683122, 1.000000000000000000, 0.9659258262890683122, 1.000000000000000000, 0.9659258262890683122, 1.000000000000000000, 0.9659258262890683122, 1.000000000000000000, 0.9659258262890683122, 1.000000000000000000, 0.9659258262890683122, 1.000000000000000000, 0.9659258262890683122, 1.000000000000000000, 0.9659258262890683122, 1.000000000000000000, 0.9659258262890683122, 1.000000000000000000, 0.9659258262890683122, 1.000000000000000000, 0.9659258262890683122, 1.000000000000000000, 0.9659258262890683122, 1.000000000000000000, 0.9659258262890683122, 1.000000000000000000, 0.9659258262890683122, 1.000000000000000000, 0.9659258262890683122, 1.000000000000000000, 0.9659258262890683122, 1.000000000000000000, 0.9659258262890683122, 1.000000000000000000, 0.9659258262890683122, 1.000000000000000000, 0.9659258262890683122, 1.000000000000000000, 0.9659258262890683122, 1.000000000000000000, 0.9659258262890683122, 1.000000000000000000, 0.9659258262890683122, 1.000000000000000000, 0.9659258262890683122, 1.000000000000000000, 0.9659258262890683122, 1.000000000000000000, 0.9659258262890683122, 1.000000000000000000, 0.9659258262890683122, 1.000000000000000000, 0.9659258262890683122, 1.000000000000000000, 0.9659258262890683122, 1.000000000000000000, 0.9659258262890683122, 1.000000000000000000, 0.9659258262890683122, 1.000000000000000000, 0.9659258262890683122, 1.000000000000000000, 0.9659258262890683122, 1.000000000000000000, 0.9659258262890683122, 1.000000000000000000, 0.9659258262890683122, 1.000000000000000000, 0.9659258262890683122, 1.000000000000000000, 0.9659258262890683122, 1.000000000000000000, 0.9659258262890683122, 1.000000000000000000, 0.9659258262890683122, 1.000000000000000000, 0.9659258262890683122, 1.000000000000000000, 0.9659258262890683122, 1.000000000000000000, 0.9659258262890683122, 1.000000000000000000, 0.9659258262890683122, 1.000000000000000000, 0.9659258262890683122, 1.000000000000000000, 0.9659258262890683122, 1.000000000000000000, 0.9659258262890683122, 1.000000000000000000, 0.9659258262890683122, 1.000000000000000000, 0.9659258262890683122, 1.000000000000000000, 0.9659258262890683122, 1.000000000000000000, 0.9659258262890683122, 1.000000000000000000, 0.9659258262890683122, 1.000000000000000000, 0.9659258262890683122, 1.000000000000000000, 0.9659258262890683122, 1.000000000000000000, 0.9659258262890683122, 1.000000000000000000, 0.9659258262890683122, 1.000000000000000000, 0.9659258262890683122, 1.000000000000000000, 0.9659258262890683122, 1.000000000000000000, 0.9659258262890683122, 1.000000000000000000, 0.9659258262890683122, 1.000000000000000000, 0.9659258262890683122, 1.000000000000000000, 0.9659258262890683122, 1.000000000000000000, 0.9659258262890683122, 1.000000000000000000, 0.9659258262890683122, 1.000000000000000000, 0.9659258262890683122, 1.000000000000000000, 0.9659258262890683122, 1.000000000000000000, 0.9659258262890683122, 1.000000000000000000, 0.9659258262890683122, 1.000000000000000000, 0.9659258262890683122, 1.000000000000000000, 0.9659258262890683122, 1.000000000000000000, 0.9659258262890683122, 1.000000000000000000, 0.9659258262890683122, 1.000000000000000000, 0.9659258262890683122, 1.000000000000000000, 0.9659258262890683122, 1.000000000000000000, 0.9659258262890683122, 1.000000000000000000, 0.9659258262890683122, 1.000000000000000000, 0.9659258262890683122, 1.000000000000000000, 0.9659258262890683122, 1.000000000000000000, 0.9659258262890683122, 1.000000000000000000, 0.9659258262890683122, 1.000000000000000000, 0.9659258262890683122, 1.000000000000000000, 0.9659258262890683122, 1.000000000000000000, 0.9659258262890683122, 1.000000000000000000, 0.9659258262890683122, 1.000000000000000000, 0.9659258262890683122, 1.000000000000000000, 0.9659258262890683122, 1.000000000000000000, 0.9659258262890683122, 1.000000000000000000, 0.9659258262890683122, 1.000000000000000000, 0.9659258262890683122, 1.000000000000000000, 0.9659258262890683122, 1.000000000000000000, 0.9659258262890683122, 1.000000000000000000, 0.9659258262890683122, 1.000000000000000000, 0.9659258262890683122, 1.000000000000000000, 0.9659258262890683122, 1.000000000000000000, 0.9659258262890683122, 1.000000000000000000),
 ( 0.3333333333333333703, 0.3219752754296894559, 0.3333333333333333703, 0.3219752754296894559, 0.3333333333333333703, 0.3219752754296894559, 0.3333333333333333703, 0.3219752754296894559, 0.3333333333333333703, 0.3219752754296894559, 0.3333333333333333703, 0.3219752754296894559, 0.3333333333333333703, 0.3219752754296894559, 0.3333333333333333703, 0.3219752754296894559, 0.3333333333333333703, 0.3219752754296894559, 0.3333333333333333703, 0.3219752754296894559, 0.3333333333333333703, 0.3219752754296894559, 0.3333333333333333703, 0.3219752754296894559, 0.3333333333333333703, 0.3219752754296894559, 0.3333333333333333703, 0.3219752754296894559, 0.3333333333333333703, 0.3219752754296894559, 0.3333333333333333703, 0.3219752754296894559, 0.3333333333333333703, 0.3219752754296894559, 0.3333333333333333703, 0.3219752754296894559, 0.3333333333333333703, 0.3219752754296894559, 0.3333333333333333703, 0.3219752754296894559, 0.3333333333333333703, 0.3219752754296894559, 0.3333333333333333703, 0.3219752754296894559, 0.3333333333333333703, 0.3219752754296894559, 0.3333333333333333703, 0.3219752754296894559, 0.3333333333333333703, 0.3219752754296894559, 0.3333333333333333703, 0.3219752754296894559, 0.3333333333333333703, 0.3219752754296894559, 0.3333333333333333703, 0.3219752754296894559, 0.3333333333333333703, 0.3219752754296894559, 0.3333333333333333703, 0.3219752754296894559, 0.3333333333333333703, 0.3219752754296894559, 0.3333333333333333703, 0.3219752754296894559, 0.3333333333333333703, 0.3219752754296894559, 0.3333333333333333703, 0.3219752754296894559, 0.3333333333333333703, 0.3219752754296894559, 0.3333333333333333703, 0.3219752754296894559, 0.3333333333333333703, 0.3219752754296894559, 0.3333333333333333703, 0.3219752754296894559, 0.3333333333333333703, 0.3219752754296894559, 0.3333333333333333703, 0.3219752754296894559, 0.3333333333333333703, 0.3219752754296894559, 0.3333333333333333703, 0.3219752754296894559, 0.3333333333333333703, 0.3219752754296894559, 0.3333333333333333703, 0.3219752754296894559, 0.3333333333333333703, 0.3219752754296894559, 0.3333333333333333703, 0.3219752754296894559, 0.3333333333333333703, 0.3219752754296894559, 0.3333333333333333703, 0.3219752754296894559, 0.3333333333333333703, 0.3219752754296894559, 0.3333333333333333703, 0.3219752754296894559, 0.3333333333333333703, 0.3219752754296894559, 0.3333333333333333703, 0.3219752754296894559, 0.3333333333333333703, 0.3219752754296894559, 0.3333333333333333703, 0.3219752754296894559, 0.3333333333333333703, 0.3219752754296894559, 0.3333333333333333703, 0.3219752754296894559, 0.3333333333333333703, 0.3219752754296894559, 0.3333333333333333703, 0.3219752754296894559, 0.3333333333333333703, 0.3219752754296894559, 0.3333333333333333703, 0.3219752754296894559, 0.3333333333333333703, 0.3219752754296894559, 0.3333333333333333703, 0.3219752754296894559, 0.3333333333333333703, 0.3219752754296894559, 0.3333333333333333703, 0.3219752754296894559, 0.3333333333333333703, 0.3219752754296894559, 0.3333333333333333703, 0.3219752754296894559, 0.3333333333333333703, 0.3219752754296894559, 0.3333333333333333703, 0.3219752754296894559, 0.3333333333333333703, 0.3219752754296894559, 0.3333333333333333703, 0.3219752754296894559, 0.3333333333333333703, 0.3219752754296894559, 0.3333333333333333703, 0.3219752754296894559, 0.3333333333333333703, 0.3219752754296894559, 0.3333333333333333703, 0.3219752754296894559, 0.3333333333333333703, 0.3219752754296894559, 0.3333333333333333703, 0.3219752754296894559, 0.3333333333333333703, 0.3219752754296894559, 0.3333333333333333703, 0.3219752754296894559, 0.3333333333333333703, 0.3219752754296894559, 0.3333333333333333703, 0.3219752754296894559, 0.3333333333333333703, 0.3219752754296894559, 0.3333333333333333703, 0.3219752754296894559, 0.3333333333333333703, 0.3219752754296894559, 0.3333333333333333703, 0.3219752754296894559, 0.3333333333333333703, 0.3219752754296894559, 0.3333333333333333703, 0.3219752754296894559, 0.3333333333333333703, 0.3219752754296894559, 0.3333333333333333703, 0.3219752754296894559, 0.3333333333333333703, 0.3219752754296894559, 0.3333333333333333703, 0.3219752754296894559, 0.3333333333333333703, 0.3219752754296894559, 0.3333333333333333703, 0.3219752754296894559, 0.3333333333333333703, 0.3219752754296894559, 0.3333333333333333703, 0.3219752754296894559, 0.3333333333333333703, 0.3219752754296894559, 0.3333333333333333703, 0.3219752754296894559, 0.3333333333333333703, 0.3219752754296894559, 0.3333333333333333703, 0.3219752754296894559, 0.3333333333333333703, 0.3219752754296894559, 0.3333333333333333703, 0.3219752754296894559, 0.3333333333333333703, 0.3219752754296894559, 0.3333333333333333703, 0.3219752754296894559, 0.3333333333333333703, 0.3219752754296894559, 0.3333333333333333703, 0.3219752754296894559, 0.3333333333333333703, 0.3219752754296894559, 0.3333333333333333703, 0.3219752754296894559, 0.3333333333333333703, 0.3219752754296894559, 0.3333333333333333703, 0.3219752754296894559, 0.3333333333333333703, 0.3219752754296894559, 0.3333333333333333703, 0.3219752754296894559, 0.3333333333333333703, 0.3219752754296894559, 0.3333333333333333703, 0.3219752754296894559, 0.3333333333333333703, 0.3219752754296894559, 0.3333333333333333703, 0.3219752754296894559, 0.3333333333333333703, 0.3219752754296894559, 0.3333333333333333703, 0.3219752754296894559, 0.3333333333333333703, 0.3219752754296894559, 0.3333333333333333703, 0.3219752754296894559, 0.3333333333333333703, 0.3219752754296894559, 0.3333333333333333703, 0.3219752754296894559, 0.3333333333333333703, 0.3219752754296894559, 0.3333333333333333703, 0.3219752754296894559, 0.3333333333333333703, 0.3219752754296894559, 0.3333333333333333703, 0.3219752754296894559, 0.3333333333333333703, 0.3219752754296894559, 0.3333333333333333703, 0.3219752754296894559, 0.3333333333333333703, 0.3219752754296894559, 0.3333333333333333703, 0.3219752754296894559, 0.3333333333333333703, 0.3219752754296894559, 0.3333333333333333703, 0.3219752754296894559, 0.3333333333333333703, 0.3219752754296894559, 0.3333333333333333703, 0.3219752754296894559, 0.3333333333333333703, 0.3219752754296894559, 0.3333333333333333703, 0.3219752754296894559, 0.3333333333333333703, 0.3219752754296894559, 0.3333333333333333703, 0.3219752754296894559, 0.3333333333333333703, 0.3219752754296894559, 0.3333333333333333703, 0.3219752754296894559, 0.3333333333333333703, 0.3219752754296894559, 0.3333333333333333703, 0.3219752754296894559, 0.3333333333333333703, 0.3219752754296894559, 0.3333333333333333703, 0.3219752754296894559, 0.3333333333333333703, 0.3219752754296894559, 0.3333333333333333703, 0.3219752754296894559, 0.3333333333333333703, 0.3219752754296894559, 0.3333333333333333703, 0.3219752754296894559, 0.3333333333333333703, 0.3219752754296894559, 0.3333333333333333703, 0.3219752754296894559, 0.3333333333333333703, 0.3219752754296894559, 0.3333333333333333703, 0.3219752754296894559, 0.3333333333333333703, 0.3219752754296894559, 0.3333333333333333703, 0.3219752754296894559, 0.3333333333333333703, 0.3219752754296894559, 0.3333333333333333703, 0.3219752754296894559, 0.3333333333333333703, 0.3219752754296894559, 0.3333333333333333703, 0.3219752754296894559, 0.3333333333333333703, 0.3219752754296894559, 0.3333333333333333703, 0.3219752754296894559, 0.3333333333333333703, 0.3219752754296894559, 0.3333333333333333703, 0.3219752754296894559, 0.3333333333333333703, 0.3219752754296894559, 0.3333333333333333703, 0.3219752754296894559, 0.3333333333333333703, 0.3219752754296894559, 0.3333333333333333703, 0.3219752754296894559, 0.3333333333333333703, 0.3219752754296894559, 0.3333333333333333703, 0.3219752754296894559, 0.3333333333333333703, 0.3219752754296894559, 0.3333333333333333703, 0.3219752754296894559, 0.3333333333333333703, 0.3219752754296894559, 0.3333333333333333703, 0.3219752754296894559, 0.3333333333333333703, 0.3219752754296894559, 0.3333333333333333703, 0.3219752754296894559, 0.3333333333333333703, 0.3219752754296894559, 0.3333333333333333703, 0.3219752754296894559, 0.3333333333333333703, 0.3219752754296894559, 0.3333333333333333703, 0.3219752754296894559, 0.3333333333333333703, 0.3219752754296894559, 0.3333333333333333703, 0.3219752754296894559, 0.3333333333333333703, 0.3219752754296894559, 0.3333333333333333703, 0.3219752754296894559, 0.3333333333333333703, 0.3219752754296894559, 0.3333333333333333703, 0.3219752754296894559, 0.3333333333333333703, 0.3219752754296894559, 0.3333333333333333703, 0.3219752754296894559, 0.3333333333333333703, 0.3219752754296894559, 0.3333333333333333703, 0.3219752754296894559, 0.3333333333333333703, 0.3219752754296894559, 0.3333333333333333703, 0.3219752754296894559, 0.3333333333333333703, 0.3219752754296894559, 0.3333333333333333703, 0.3219752754296894559, 0.3333333333333333703, 0.3219752754296894559, 0.3333333333333333703, 0.3219752754296894559, 0.3333333333333333703, 0.3219752754296894559, 0.3333333333333333703, 0.3219752754296894559, 0.3333333333333333703, 0.3219752754296894559, 0.3333333333333333703, 0.3219752754296894559, 0.3333333333333333703, 0.3219752754296894559, 0.3333333333333333703, 0.3219752754296894559, 0.3333333333333333703, 0.3219752754296894559, 0.3333333333333333703, 0.3219752754296894559, 0.3333333333333333703, 0.3219752754296894559, 0.3333333333333333703, 0.3219752754296894559, 0.3333333333333333703, 0.3219752754296894559, 0.3333333333333333703, 0.3219752754296894559, 0.3333333333333333703, 0.3219752754296894559, 0.3333333333333333703, 0.3219752754296894559, 0.3333333333333333703, 0.3219752754296894559, 0.3333333333333333703, 0.3219752754296894559, 0.3333333333333333703, 0.3219752754296894559, 0.3333333333333333703, 0.3219752754296894559, 0.3333333333333333703, 0.3219752754296894559, 0.3333333333333333703, 0.3219752754296894559, 0.3333333333333333703, 0.3219752754296894559, 0.3333333333333333703, 0.3219752754296894559, 0.3333333333333333703, 0.3219752754296894559, 0.3333333333333333703, 0.3219752754296894559, 0.3333333333333333703, 0.3219752754296894559, 0.3333333333333333703, 0.3219752754296894559, 0.3333333333333333703, 0.3219752754296894559, 0.3333333333333333703, 0.3219752754296894559, 0.3333333333333333703, 0.3219752754296894559, 0.3333333333333333703, 0.3219752754296894559, 0.3333333333333333703, 0.3219752754296894559, 0.3333333333333333703, 0.3219752754296894559, 0.3333333333333333703, 0.3219752754296894559, 0.3333333333333333703, 0.3219752754296894559, 0.3333333333333333703, 0.3219752754296894559, 0.3333333333333333703, 0.3219752754296894559, 0.3333333333333333703),
 ( 0.3333333333333333703, 0.3219752754296894559, 0.3333333333333333703, 0.3219752754296894559, 0.3333333333333333703, 0.3219752754296894559, 0.3333333333333333703, 0.3219752754296894559, 0.3333333333333333703, 0.3219752754296894559, 0.3333333333333333703, 0.3219752754296894559, 0.3333333333333333703, 0.3219752754296894559, 0.3333333333333333703, 0.3219752754296894559, 0.3333333333333333703, 0.3219752754296894559, 0.3333333333333333703, 0.3219752754296894559, 0.3333333333333333703, 0.3219752754296894559, 0.3333333333333333703, 0.3219752754296894559, 0.3333333333333333703, 0.3219752754296894559, 0.3333333333333333703, 0.3219752754296894559, 0.3333333333333333703, 0.3219752754296894559, 0.3333333333333333703, 0.3219752754296894559, 0.3333333333333333703, 0.3219752754296894559, 0.3333333333333333703, 0.3219752754296894559, 0.3333333333333333703, 0.3219752754296894559, 0.3333333333333333703, 0.3219752754296894559, 0.3333333333333333703, 0.3219752754296894559, 0.3333333333333333703, 0.3219752754296894559, 0.3333333333333333703, 0.3219752754296894559, 0.3333333333333333703, 0.3219752754296894559, 0.3333333333333333703, 0.3219752754296894559, 0.3333333333333333703, 0.3219752754296894559, 0.3333333333333333703, 0.3219752754296894559, 0.3333333333333333703, 0.3219752754296894559, 0.3333333333333333703, 0.3219752754296894559, 0.3333333333333333703, 0.3219752754296894559, 0.3333333333333333703, 0.3219752754296894559, 0.3333333333333333703, 0.3219752754296894559, 0.3333333333333333703, 0.3219752754296894559, 0.3333333333333333703, 0.3219752754296894559, 0.3333333333333333703, 0.3219752754296894559, 0.3333333333333333703, 0.3219752754296894559, 0.3333333333333333703, 0.3219752754296894559, 0.3333333333333333703, 0.3219752754296894559, 0.3333333333333333703, 0.3219752754296894559, 0.3333333333333333703, 0.3219752754296894559, 0.3333333333333333703, 0.3219752754296894559, 0.3333333333333333703, 0.3219752754296894559, 0.3333333333333333703, 0.3219752754296894559, 0.3333333333333333703, 0.3219752754296894559, 0.3333333333333333703, 0.3219752754296894559, 0.3333333333333333703, 0.3219752754296894559, 0.3333333333333333703, 0.3219752754296894559, 0.3333333333333333703, 0.3219752754296894559, 0.3333333333333333703, 0.3219752754296894559, 0.3333333333333333703, 0.3219752754296894559, 0.3333333333333333703, 0.3219752754296894559, 0.3333333333333333703, 0.3219752754296894559, 0.3333333333333333703, 0.3219752754296894559, 0.3333333333333333703, 0.3219752754296894559, 0.3333333333333333703, 0.3219752754296894559, 0.3333333333333333703, 0.3219752754296894559, 0.3333333333333333703, 0.3219752754296894559, 0.3333333333333333703, 0.3219752754296894559, 0.3333333333333333703, 0.3219752754296894559, 0.3333333333333333703, 0.3219752754296894559, 0.3333333333333333703, 0.3219752754296894559, 0.3333333333333333703, 0.3219752754296894559, 0.3333333333333333703, 0.3219752754296894559, 0.3333333333333333703, 0.3219752754296894559, 0.3333333333333333703, 0.3219752754296894559, 0.3333333333333333703, 0.3219752754296894559, 0.3333333333333333703, 0.3219752754296894559, 0.3333333333333333703, 0.3219752754296894559, 0.3333333333333333703, 0.3219752754296894559, 0.3333333333333333703, 0.3219752754296894559, 0.3333333333333333703, 0.3219752754296894559, 0.3333333333333333703, 0.3219752754296894559, 0.3333333333333333703, 0.3219752754296894559, 0.3333333333333333703, 0.3219752754296894559, 0.3333333333333333703, 0.3219752754296894559, 0.3333333333333333703, 0.3219752754296894559, 0.3333333333333333703, 0.3219752754296894559, 0.3333333333333333703, 0.3219752754296894559, 0.3333333333333333703, 0.3219752754296894559, 0.3333333333333333703, 0.3219752754296894559, 0.3333333333333333703, 0.3219752754296894559, 0.3333333333333333703, 0.3219752754296894559, 0.3333333333333333703, 0.3219752754296894559, 0.3333333333333333703, 0.3219752754296894559, 0.3333333333333333703, 0.3219752754296894559, 0.3333333333333333703, 0.3219752754296894559, 0.3333333333333333703, 0.3219752754296894559, 0.3333333333333333703, 0.3219752754296894559, 0.3333333333333333703, 0.3219752754296894559, 0.3333333333333333703, 0.3219752754296894559, 0.3333333333333333703, 0.3219752754296894559, 0.3333333333333333703, 0.3219752754296894559, 0.3333333333333333703, 0.3219752754296894559, 0.3333333333333333703, 0.3219752754296894559, 0.3333333333333333703, 0.3219752754296894559, 0.3333333333333333703, 0.3219752754296894559, 0.3333333333333333703, 0.3219752754296894559, 0.3333333333333333703, 0.3219752754296894559, 0.3333333333333333703, 0.3219752754296894559, 0.3333333333333333703, 0.3219752754296894559, 0.3333333333333333703, 0.3219752754296894559, 0.3333333333333333703, 0.3219752754296894559, 0.3333333333333333703, 0.3219752754296894559, 0.3333333333333333703, 0.3219752754296894559, 0.3333333333333333703, 0.3219752754296894559, 0.3333333333333333703, 0.3219752754296894559, 0.3333333333333333703, 0.3219752754296894559, 0.3333333333333333703, 0.3219752754296894559, 0.3333333333333333703, 0.3219752754296894559, 0.3333333333333333703, 0.3219752754296894559, 0.3333333333333333703, 0.3219752754296894559, 0.3333333333333333703, 0.3219752754296894559, 0.3333333333333333703, 0.3219752754296894559, 0.3333333333333333703, 0.3219752754296894559, 0.3333333333333333703, 0.3219752754296894559, 0.3333333333333333703, 0.3219752754296894559, 0.3333333333333333703, 0.3219752754296894559, 0.3333333333333333703, 0.3219752754296894559, 0.3333333333333333703, 0.3219752754296894559, 0.3333333333333333703, 0.3219752754296894559, 0.3333333333333333703, 0.3219752754296894559, 0.3333333333333333703, 0.3219752754296894559, 0.3333333333333333703, 0.3219752754296894559, 0.3333333333333333703, 0.3219752754296894559, 0.3333333333333333703, 0.3219752754296894559, 0.3333333333333333703, 0.3219752754296894559, 0.3333333333333333703, 0.3219752754296894559, 0.3333333333333333703, 0.3219752754296894559, 0.3333333333333333703, 0.3219752754296894559, 0.3333333333333333703, 0.3219752754296894559, 0.3333333333333333703, 0.3219752754296894559, 0.3333333333333333703, 0.3219752754296894559, 0.3333333333333333703, 0.3219752754296894559, 0.3333333333333333703, 0.3219752754296894559, 0.3333333333333333703, 0.3219752754296894559, 0.3333333333333333703, 0.3219752754296894559, 0.3333333333333333703, 0.3219752754296894559, 0.3333333333333333703, 0.3219752754296894559, 0.3333333333333333703, 0.3219752754296894559, 0.3333333333333333703, 0.3219752754296894559, 0.3333333333333333703, 0.3219752754296894559, 0.3333333333333333703, 0.3219752754296894559, 0.3333333333333333703, 0.3219752754296894559, 0.3333333333333333703, 0.3219752754296894559, 0.3333333333333333703, 0.3219752754296894559, 0.3333333333333333703, 0.3219752754296894559, 0.3333333333333333703, 0.3219752754296894559, 0.3333333333333333703, 0.3219752754296894559, 0.3333333333333333703, 0.3219752754296894559, 0.3333333333333333703, 0.3219752754296894559, 0.3333333333333333703, 0.3219752754296894559, 0.3333333333333333703, 0.3219752754296894559, 0.3333333333333333703, 0.3219752754296894559, 0.3333333333333333703, 0.3219752754296894559, 0.3333333333333333703, 0.3219752754296894559, 0.3333333333333333703, 0.3219752754296894559, 0.3333333333333333703, 0.3219752754296894559, 0.3333333333333333703, 0.3219752754296894559, 0.3333333333333333703, 0.3219752754296894559, 0.3333333333333333703, 0.3219752754296894559, 0.3333333333333333703, 0.3219752754296894559, 0.3333333333333333703, 0.3219752754296894559, 0.3333333333333333703, 0.3219752754296894559, 0.3333333333333333703, 0.3219752754296894559, 0.3333333333333333703, 0.3219752754296894559, 0.3333333333333333703, 0.3219752754296894559, 0.3333333333333333703, 0.3219752754296894559, 0.3333333333333333703, 0.3219752754296894559, 0.3333333333333333703, 0.3219752754296894559, 0.3333333333333333703, 0.3219752754296894559, 0.3333333333333333703, 0.3219752754296894559, 0.3333333333333333703, 0.3219752754296894559, 0.3333333333333333703, 0.3219752754296894559, 0.3333333333333333703, 0.3219752754296894559, 0.3333333333333333703, 0.3219752754296894559, 0.3333333333333333703, 0.3219752754296894559, 0.3333333333333333703, 0.3219752754296894559, 0.3333333333333333703, 0.3219752754296894559, 0.3333333333333333703, 0.3219752754296894559, 0.3333333333333333703, 0.3219752754296894559, 0.3333333333333333703, 0.3219752754296894559, 0.3333333333333333703, 0.3219752754296894559, 0.3333333333333333703, 0.3219752754296894559, 0.3333333333333333703, 0.3219752754296894559, 0.3333333333333333703, 0.3219752754296894559, 0.3333333333333333703, 0.3219752754296894559, 0.3333333333333333703, 0.3219752754296894559, 0.3333333333333333703, 0.3219752754296894559, 0.3333333333333333703, 0.3219752754296894559, 0.3333333333333333703, 0.3219752754296894559, 0.3333333333333333703, 0.3219752754296894559, 0.3333333333333333703, 0.3219752754296894559, 0.3333333333333333703, 0.3219752754296894559, 0.3333333333333333703, 0.3219752754296894559, 0.3333333333333333703, 0.3219752754296894559, 0.3333333333333333703, 0.3219752754296894559, 0.3333333333333333703, 0.3219752754296894559, 0.3333333333333333703, 0.3219752754296894559, 0.3333333333333333703, 0.3219752754296894559, 0.3333333333333333703, 0.3219752754296894559, 0.3333333333333333703, 0.3219752754296894559, 0.3333333333333333703, 0.3219752754296894559, 0.3333333333333333703, 0.3219752754296894559, 0.3333333333333333703, 0.3219752754296894559, 0.3333333333333333703, 0.3219752754296894559, 0.3333333333333333703, 0.3219752754296894559, 0.3333333333333333703, 0.3219752754296894559, 0.3333333333333333703, 0.3219752754296894559, 0.3333333333333333703, 0.3219752754296894559, 0.3333333333333333703, 0.3219752754296894559, 0.3333333333333333703, 0.3219752754296894559, 0.3333333333333333703, 0.3219752754296894559, 0.3333333333333333703, 0.3219752754296894559, 0.3333333333333333703, 0.3219752754296894559, 0.3333333333333333703, 0.3219752754296894559, 0.3333333333333333703, 0.3219752754296894559, 0.3333333333333333703, 0.3219752754296894559, 0.3333333333333333703, 0.3219752754296894559, 0.3333333333333333703, 0.3219752754296894559, 0.3333333333333333703, 0.3219752754296894559, 0.3333333333333333703, 0.3219752754296894559, 0.3333333333333333703, 0.3219752754296894559, 0.3333333333333333703, 0.3219752754296894559, 0.3333333333333333703, 0.3219752754296894559, 0.3333333333333333703, 0.3219752754296894559, 0.3333333333333333703, 0.3219752754296894559, 0.3333333333333333703, 0.3219752754296894559, 0.3333333333333333703, 0.3219752754296894559, 0.3333333333333333703),
 ( 1.000000000000000000, 0.9659258262890683122, 1.000000000000000000, 0.9659258262890683122, 1.000000000000000000, 0.9659258262890683122, 1.000000000000000000, 0.9659258262890683122, 1.000000000000000000, 0.9659258262890683122, 1.000000000000000000, 0.9659258262890683122, 1.000000000000000000, 0.9659258262890683122, 1.000000000000000000, 0.9659258262890683122, 1.000000000000000000, 0.9659258262890683122, 1.000000000000000000, 0.9659258262890683122, 1.000000000000000000, 0.9659258262890683122, 1.000000000000000000, 0.9659258262890683122, 1.000000000000000000, 0.9659258262890683122, 1.000000000000000000, 0.9659258262890683122, 1.000000000000000000, 0.9659258262890683122, 1.000000000000000000, 0.9659258262890683122, 1.000000000000000000, 0.9659258262890683122, 1.000000000000000000, 0.9659258262890683122, 1.000000000000000000, 0.9659258262890683122, 1.000000000000000000, 0.9659258262890683122, 1.000000000000000000, 0.9659258262890683122, 1.000000000000000000, 0.9659258262890683122, 1.000000000000000000, 0.9659258262890683122, 1.000000000000000000, 0.9659258262890683122, 1.000000000000000000, 0.9659258262890683122, 1.000000000000000000, 0.9659258262890683122, 1.000000000000000000, 0.9659258262890683122, 1.000000000000000000, 0.9659258262890683122, 1.000000000000000000, 0.9659258262890683122, 1.000000000000000000, 0.9659258262890683122, 1.000000000000000000, 0.9659258262890683122, 1.000000000000000000, 0.9659258262890683122, 1.000000000000000000, 0.9659258262890683122, 1.000000000000000000, 0.9659258262890683122, 1.000000000000000000, 0.9659258262890683122, 1.000000000000000000, 0.9659258262890683122, 1.000000000000000000, 0.9659258262890683122, 1.000000000000000000, 0.9659258262890683122, 1.000000000000000000, 0.9659258262890683122, 1.000000000000000000, 0.9659258262890683122, 1.000000000000000000, 0.9659258262890683122, 1.000000000000000000, 0.9659258262890683122, 1.000000000000000000, 0.9659258262890683122, 1.000000000000000000, 0.9659258262890683122, 1.000000000000000000, 0.9659258262890683122, 1.000000000000000000, 0.9659258262890683122, 1.000000000000000000, 0.9659258262890683122, 1.000000000000000000, 0.9659258262890683122, 1.000000000000000000, 0.9659258262890683122, 1.000000000000000000, 0.9659258262890683122, 1.000000000000000000, 0.9659258262890683122, 1.000000000000000000, 0.9659258262890683122, 1.000000000000000000, 0.9659258262890683122, 1.000000000000000000, 0.9659258262890683122, 1.000000000000000000, 0.9659258262890683122, 1.000000000000000000, 0.9659258262890683122, 1.000000000000000000, 0.9659258262890683122, 1.000000000000000000, 0.9659258262890683122, 1.000000000000000000, 0.9659258262890683122, 1.000000000000000000, 0.9659258262890683122, 1.000000000000000000, 0.9659258262890683122, 1.000000000000000000, 0.9659258262890683122, 1.000000000000000000, 0.9659258262890683122, 1.000000000000000000, 0.9659258262890683122, 1.000000000000000000, 0.9659258262890683122, 1.000000000000000000, 0.9659258262890683122, 1.000000000000000000, 0.9659258262890683122, 1.000000000000000000, 0.9659258262890683122, 1.000000000000000000, 0.9659258262890683122, 1.000000000000000000, 0.9659258262890683122, 1.000000000000000000, 0.9659258262890683122, 1.000000000000000000, 0.9659258262890683122, 1.000000000000000000, 0.9659258262890683122, 1.000000000000000000, 0.9659258262890683122, 1.000000000000000000, 0.9659258262890683122, 1.000000000000000000, 0.9659258262890683122, 1.000000000000000000, 0.9659258262890683122, 1.000000000000000000, 0.9659258262890683122, 1.000000000000000000, 0.9659258262890683122, 1.000000000000000000, 0.9659258262890683122, 1.000000000000000000, 0.9659258262890683122, 1.000000000000000000, 0.9659258262890683122, 1.000000000000000000, 0.9659258262890683122, 1.000000000000000000, 0.9659258262890683122, 1.000000000000000000, 0.9659258262890683122, 1.000000000000000000, 0.9659258262890683122, 1.000000000000000000, 0.9659258262890683122, 1.000000000000000000, 0.9659258262890683122, 1.000000000000000000, 0.9659258262890683122, 1.000000000000000000, 0.9659258262890683122, 1.000000000000000000, 0.9659258262890683122, 1.000000000000000000, 0.9659258262890683122, 1.000000000000000000, 0.9659258262890683122, 1.000000000000000000, 0.9659258262890683122, 1.000000000000000000, 0.9659258262890683122, 1.000000000000000000, 0.9659258262890683122, 1.000000000000000000, 0.9659258262890683122, 1.000000000000000000, 0.9659258262890683122, 1.000000000000000000, 0.9659258262890683122, 1.000000000000000000, 0.9659258262890683122, 1.000000000000000000, 0.9659258262890683122, 1.000000000000000000, 0.9659258262890683122, 1.000000000000000000, 0.9659258262890683122, 1.000000000000000000, 0.9659258262890683122, 1.000000000000000000, 0.9659258262890683122, 1.000000000000000000, 0.9659258262890683122, 1.000000000000000000, 0.9659258262890683122, 1.000000000000000000, 0.9659258262890683122, 1.000000000000000000, 0.9659258262890683122, 1.000000000000000000, 0.9659258262890683122, 1.000000000000000000, 0.9659258262890683122, 1.000000000000000000, 0.9659258262890683122, 1.000000000000000000, 0.9659258262890683122, 1.000000000000000000, 0.9659258262890683122, 1.000000000000000000, 0.9659258262890683122, 1.000000000000000000, 0.9659258262890683122, 1.000000000000000000, 0.9659258262890683122, 1.000000000000000000, 0.9659258262890683122, 1.000000000000000000, 0.9659258262890683122, 1.000000000000000000, 0.9659258262890683122, 1.000000000000000000, 0.9659258262890683122, 1.000000000000000000, 0.9659258262890683122, 1.000000000000000000, 0.9659258262890683122, 1.000000000000000000, 0.9659258262890683122, 1.000000000000000000, 0.9659258262890683122, 1.000000000000000000, 0.9659258262890683122, 1.000000000000000000, 0.9659258262890683122, 1.000000000000000000, 0.9659258262890683122, 1.000000000000000000, 0.9659258262890683122, 1.000000000000000000, 0.9659258262890683122, 1.000000000000000000, 0.9659258262890683122, 1.000000000000000000, 0.9659258262890683122, 1.000000000000000000, 0.9659258262890683122, 1.000000000000000000, 0.9659258262890683122, 1.000000000000000000, 0.9659258262890683122, 1.000000000000000000, 0.9659258262890683122, 1.000000000000000000, 0.9659258262890683122, 1.000000000000000000, 0.9659258262890683122, 1.000000000000000000, 0.9659258262890683122, 1.000000000000000000, 0.9659258262890683122, 1.000000000000000000, 0.9659258262890683122, 1.000000000000000000, 0.9659258262890683122, 1.000000000000000000, 0.9659258262890683122, 1.000000000000000000, 0.9659258262890683122, 1.000000000000000000, 0.9659258262890683122, 1.000000000000000000, 0.9659258262890683122, 1.000000000000000000, 0.9659258262890683122, 1.000000000000000000, 0.9659258262890683122, 1.000000000000000000, 0.9659258262890683122, 1.000000000000000000, 0.9659258262890683122, 1.000000000000000000, 0.9659258262890683122, 1.000000000000000000, 0.9659258262890683122, 1.000000000000000000, 0.9659258262890683122, 1.000000000000000000, 0.9659258262890683122, 1.000000000000000000, 0.9659258262890683122, 1.000000000000000000, 0.9659258262890683122, 1.000000000000000000, 0.9659258262890683122, 1.000000000000000000, 0.9659258262890683122, 1.000000000000000000, 0.9659258262890683122, 1.000000000000000000, 0.9659258262890683122, 1.000000000000000000, 0.9659258262890683122, 1.000000000000000000, 0.9659258262890683122, 1.000000000000000000, 0.9659258262890683122, 1.000000000000000000, 0.9659258262890683122, 1.000000000000000000, 0.9659258262890683122, 1.000000000000000000, 0.9659258262890683122, 1.000000000000000000, 0.9659258262890683122, 1.000000000000000000, 0.9659258262890683122, 1.000000000000000000, 0.9659258262890683122, 1.000000000000000000, 0.9659258262890683122, 1.000000000000000000, 0.9659258262890683122, 1.000000000000000000, 0.9659258262890683122, 1.000000000000000000, 0.9659258262890683122, 1.000000000000000000, 0.9659258262890683122, 1.000000000000000000, 0.9659258262890683122, 1.000000000000000000, 0.9659258262890683122, 1.000000000000000000, 0.9659258262890683122, 1.000000000000000000, 0.9659258262890683122, 1.000000000000000000, 0.9659258262890683122, 1.000000000000000000, 0.9659258262890683122, 1.000000000000000000, 0.9659258262890683122, 1.000000000000000000, 0.9659258262890683122, 1.000000000000000000, 0.9659258262890683122, 1.000000000000000000, 0.9659258262890683122, 1.000000000000000000, 0.9659258262890683122, 1.000000000000000000, 0.9659258262890683122, 1.000000000000000000, 0.9659258262890683122, 1.000000000000000000, 0.9659258262890683122, 1.000000000000000000, 0.9659258262890683122, 1.000000000000000000, 0.9659258262890683122, 1.000000000000000000, 0.9659258262890683122, 1.000000000000000000, 0.9659258262890683122, 1.000000000000000000, 0.9659258262890683122, 1.000000000000000000, 0.9659258262890683122, 1.000000000000000000, 0.9659258262890683122, 1.000000000000000000, 0.9659258262890683122, 1.000000000000000000, 0.9659258262890683122, 1.000000000000000000, 0.9659258262890683122, 1.000000000000000000, 0.9659258262890683122, 1.000000000000000000, 0.9659258262890683122, 1.000000000000000000, 0.9659258262890683122, 1.000000000000000000, 0.9659258262890683122, 1.000000000000000000, 0.9659258262890683122, 1.000000000000000000, 0.9659258262890683122, 1.000000000000000000, 0.9659258262890683122, 1.000000000000000000, 0.9659258262890683122, 1.000000000000000000, 0.9659258262890683122, 1.000000000000000000, 0.9659258262890683122, 1.000000000000000000, 0.9659258262890683122, 1.000000000000000000, 0.9659258262890683122, 1.000000000000000000, 0.9659258262890683122, 1.000000000000000000, 0.9659258262890683122, 1.000000000000000000, 0.9659258262890683122, 1.000000000000000000, 0.9659258262890683122, 1.000000000000000000, 0.9659258262890683122, 1.000000000000000000, 0.9659258262890683122, 1.000000000000000000, 0.9659258262890683122, 1.000000000000000000, 0.9659258262890683122, 1.000000000000000000, 0.9659258262890683122, 1.000000000000000000, 0.9659258262890683122, 1.000000000000000000, 0.9659258262890683122, 1.000000000000000000, 0.9659258262890683122, 1.000000000000000000, 0.9659258262890683122, 1.000000000000000000, 0.9659258262890683122, 1.000000000000000000, 0.9659258262890683122, 1.000000000000000000, 0.9659258262890683122, 1.000000000000000000, 0.9659258262890683122, 1.000000000000000000, 0.9659258262890683122, 1.000000000000000000) ) ) 
 REPRESENTATION_ITEM ( '' )  SURFACE ( )  );
#43448=CARTESIAN_POINT ( 'NONE',  ( 9.474510206698971260, -16.51473224551069308, 102.9155762719810241 ) ) ;
#43449=CARTESIAN_POINT ( 'NONE',  ( 5.049401038298161559, -19.05341960407611168, 67.70724293864769550 ) ) ;
#43450=CARTESIAN_POINT ( 'NONE',  ( 15.72974639402176855, 15.80617190586768217, 81.87609039468568994 ) ) ;
#43451=CARTESIAN_POINT ( 'NONE',  ( -13.97604488694527625, -13.89961937509977652, 56.87390960531434558 ) ) ;
#43452=CARTESIAN_POINT ( 'NONE',  ( 5.049401038298161559, -19.05341960407611168, 42.70724293864767418 ) ) ;
#43453=CARTESIAN_POINT ( 'NONE',  ( 10.81492255796078972, 18.62759615963270932, 24.58224293864768839 ) ) ;
#43454=CARTESIAN_POINT ( 'NONE',  ( -8.224510206698948167, 14.34966873604960824, 65.41557627198102409 ) ) ;
#43455=CARTESIAN_POINT ( 'NONE',  ( -9.474510206698964154, 16.51473224551069663, 40.41557627198103120 ) ) ;
#43456=CARTESIAN_POINT ( 'NONE',  ( 4.379528057220339221, -16.55341960407611168, 97.70724293864772392 ) ) ;
#43457=CARTESIAN_POINT ( 'NONE',  ( 0.05219959533907565091, 21.53943276465977519, 109.9989096053143527 ) ) ;
#43458=CARTESIAN_POINT ( 'NONE',  ( -21.53943276465977519, -0.05219959533937600094, 43.75109039468568284 ) ) ;
#43459=CARTESIAN_POINT ( 'NONE',  ( 5.153800228976335163, 19.02544592524342804, 34.79057627198102409 ) ) ;
#43461=CARTESIAN_POINT ( 'NONE',  ( -8.314922557961024197, 14.29746914071037800, 62.91775706135236135 ) ) ;
#43462=CARTESIAN_POINT ( 'NONE',  ( -10.72451020669898014, 18.67979575497178502, 100.4155762719810241 ) ) ;
#43463=CARTESIAN_POINT ( 'NONE',  ( -18.67979575497178146, -10.72451020669898902, 96.66557627198102409 ) ) ;
#43464=CARTESIAN_POINT ( 'NONE',  ( 9.474510206698729675, 16.51473224551082808, 32.08442372801900433 ) ) ;
#43465=CARTESIAN_POINT ( 'NONE',  ( 19.02544592524343514, -5.153800228976328945, 48.54057627198103120 ) ) ;
#43467=CARTESIAN_POINT ( 'NONE',  ( -10.72451020669870658, -18.67979575497194134, 54.58442372801901143 ) ) ;
#43468=CARTESIAN_POINT ( 'NONE',  ( -5.823673210054116645, -21.52544592524344225, 62.29057627198102409 ) ) ;
#43469=CARTESIAN_POINT ( 'NONE',  ( 12.14591786802309770, 12.06949235617756955, 29.37390960531435269 ) ) ;
#43470=CARTESIAN_POINT ( 'NONE',  ( 15.80617190586769283, -15.72974639402175789, 75.62609039468567573 ) ) ;
#43471=CARTESIAN_POINT ( 'NONE',  ( 18.62759615963255655, 10.81492255796105972, 106.6677570613523756 ) ) ;
#43472=CARTESIAN_POINT ( 'NONE',  ( -9.474510206698720793, -16.51473224551083518, 44.58442372801900433 ) ) ;
#43473=CARTESIAN_POINT ( 'NONE',  ( 8.224510206698742110, 14.34966873604972548, 97.08442372801904696 ) ) ;
#43474=CARTESIAN_POINT ( 'NONE',  ( 18.67979575497194134, -10.72451020669871369, 55.83442372801901854 ) ) ;
#43475=CARTESIAN_POINT ( 'NONE',  ( 5.049401038298161559, -19.05341960407611168, 62.70724293864769550 ) ) ;
#43476=CARTESIAN_POINT ( 'NONE',  ( -13.89961937509957401, -13.97604488694547875, 39.37609039468566152 ) ) ;
#43477=CARTESIAN_POINT ( 'NONE',  ( 15.80617190586746368, 15.72974639402197994, 44.37390960531435979 ) ) ;
#43479=CARTESIAN_POINT ( 'NONE',  ( -15.80617190586768217, 15.72974639402176855, 33.12609039468569705 ) ) ;
#43480=CARTESIAN_POINT ( 'NONE',  ( 0.05219959533907565091, 21.53943276465977519, 89.99890960531438111 ) ) ;
#43481=CARTESIAN_POINT ( 'NONE',  ( 19.02544592524334988, 5.153800228976608722, 91.45942372801900433 ) ) ;
#43482=CARTESIAN_POINT ( 'NONE',  ( 14.29746914071037800, 8.314922557961029526, 51.66775706135234714 ) ) ;
#43484=CARTESIAN_POINT ( 'NONE',  ( 18.67979575497178502, 10.72451020669898547, 89.16557627198102409 ) ) ;
#43485=CARTESIAN_POINT ( 'NONE',  ( 14.34966873604972726, -8.224510206698740333, 80.83442372801901854 ) ) ;
#43486=CARTESIAN_POINT ( 'NONE',  ( 14.29746914071049879, -8.314922557960816363, 73.33224293864769550 ) ) ;
#43488=CARTESIAN_POINT ( 'NONE',  ( -5.153800228976607833, 19.02544592524334988, 102.7094237280189759 ) ) ;
#43489=CARTESIAN_POINT ( 'NONE',  ( -21.55341960407610458, -5.719274019375992779, 36.45724293864768839 ) ) ;
#43491=CARTESIAN_POINT ( 'NONE',  ( -0.05219959533934338120, 16.53943276465976808, 52.50109039468567573 ) ) ;
#43492=CARTESIAN_POINT ( 'NONE',  ( -18.62759615963270932, 10.81492255796079327, 110.8322429386476955 ) ) ;
#43494=CARTESIAN_POINT ( 'NONE',  ( 5.719274019375991003, -21.55341960407610458, 37.70724293864769550 ) ) ;
#43495=CARTESIAN_POINT ( 'NONE',  ( -8.314922557961024197, 14.29746914071037800, 67.91775706135234714 ) ) ;
#43496=CARTESIAN_POINT ( 'NONE',  ( 19.02544592524343514, -5.153800228976328945, 88.54057627198102409 ) ) ;
#43497=CARTESIAN_POINT ( 'NONE',  ( -15.72974639402176322, -15.80617190586768395, 54.37609039468568994 ) ) ;
#43498=CARTESIAN_POINT ( 'NONE',  ( 13.97604488694527802, 13.89961937509977652, 34.37390960531436690 ) ) ;
#43499=CARTESIAN_POINT ( 'NONE',  ( -15.72974639402197994, 15.80617190586746368, 25.62390960531435624 ) ) ;
#43501=CARTESIAN_POINT ( 'NONE',  ( -5.049401038297874678, -19.05341960407617918, 44.79275706135232582 ) ) ;
#43502=CARTESIAN_POINT ( 'NONE',  ( -16.55341960407617563, 4.379528057220093196, 48.54275706135234714 ) ) ;
#43503=CARTESIAN_POINT ( 'NONE',  ( 19.02544592524343514, -5.153800228976328945, 113.5405762719810241 ) ) ;
#43504=CARTESIAN_POINT ( 'NONE',  ( 16.46253265017160672, -9.564922557960803928, 73.33224293864769550 ) ) ;
#43505=CARTESIAN_POINT ( 'NONE',  ( 16.55341960407618274, -4.379528057220086978, 106.0427570613523471 ) ) ;
#43507=CARTESIAN_POINT ( 'NONE',  ( 0.05219959533910956823, 16.53943276465976808, 94.99890960531436690 ) ) ;
#43508=CARTESIAN_POINT ( 'NONE',  ( 15.80617190586746368, 15.72974639402197994, 34.37390960531435979 ) ) ;
#43509=CARTESIAN_POINT ( 'NONE',  ( -19.03943276465977164, 0.05219959533909376836, 26.24890960531435624 ) ) ;
#43510=CARTESIAN_POINT ( 'NONE',  ( -4.379528057220086978, -16.55341960407618274, 69.79275706135234714 ) ) ;
#43511=CARTESIAN_POINT ( 'NONE',  ( -21.52544592524343514, 5.823673210054127303, 116.0405762719810383 ) ) ;
#43512=CARTESIAN_POINT ( 'NONE',  ( -13.89961937509957401, -13.97604488694547875, 74.37609039468566152 ) ) ;
#43513=CARTESIAN_POINT ( 'NONE',  ( -19.05341960407611168, -5.049401038298163336, 41.45724293864769550 ) ) ;
#43514=CARTESIAN_POINT ( 'NONE',  ( -21.55341960407610458, -5.719274019375992779, 71.45724293864769550 ) ) ;
#43516=CARTESIAN_POINT ( 'NONE',  ( 15.80617190586769283, -15.72974639402175789, 85.62609039468568994 ) ) ;
#43517=CARTESIAN_POINT ( 'NONE',  ( 5.049401038298161559, -19.05341960407611168, 67.70724293864769550 ) ) ;
#43518=CARTESIAN_POINT ( 'NONE',  ( 4.483927247898790824, -16.52544592524335698, 50.20942372801901854 ) ) ;
#43519=CARTESIAN_POINT ( 'NONE',  ( 21.53943276465977519, 0.05219959533937863772, 76.25109039468568994 ) ) ;
#43520=CARTESIAN_POINT ( 'NONE',  ( -13.97604488694547697, 13.89961937509957934, 43.12609039468566152 ) ) ;
#43522=CARTESIAN_POINT ( 'NONE',  ( 19.03943276465977164, 0.05219959533936151252, 56.25109039468566863 ) ) ;
#43524=CARTESIAN_POINT ( 'NONE',  ( 18.67979575497194134, -10.72451020669871369, 55.83442372801901854 ) ) ;
#43525=CARTESIAN_POINT ( 'NONE',  ( 13.97604488694527802, 13.89961937509977652, 24.37390960531435624 ) ) ;
#43526=CARTESIAN_POINT ( 'NONE',  ( -0.05219959533936034679, 19.03943276465977164, 52.50109039468566863 ) ) ;
#43527=CARTESIAN_POINT ( 'NONE',  ( -16.51473224551069308, -9.474510206698971260, 96.66557627198102409 ) ) ;
#43528=CARTESIAN_POINT ( 'NONE',  ( 13.89961937509977652, -13.97604488694527269, 78.12390960531433848 ) ) ;
#43529=CARTESIAN_POINT ( 'NONE',  ( 16.52544592524342804, -4.483927247898539470, 43.54057627198103830 ) ) ;
#43530=CARTESIAN_POINT ( 'NONE',  ( 21.55341960407610458, 5.719274019375980345, 38.95724293864768839 ) ) ;
#43533=CARTESIAN_POINT ( 'NONE',  ( -21.55341960407619339, 5.719274019375674811, 98.54275706135234714 ) ) ;
#43535=CARTESIAN_POINT ( 'NONE',  ( 16.46253265017160672, -9.564922557960803928, 38.33224293864768839 ) ) ;
#43536=CARTESIAN_POINT ( 'NONE',  ( -0.05219959533909027116, -19.03943276465977164, 107.4989096053143527 ) ) ;
#43538=CARTESIAN_POINT ( 'NONE',  ( 12.14591786802327356, -12.06949235617739191, 55.62609039468568284 ) ) ;
#43539=CARTESIAN_POINT ( 'NONE',  ( 5.719274019375991003, -21.55341960407610458, 87.70724293864769550 ) ) ;
#43540=CARTESIAN_POINT ( 'NONE',  ( 8.314922557960818139, 14.29746914071049879, 34.58224293864770260 ) ) ;
#43541=CARTESIAN_POINT ( 'NONE',  ( -0.05219959533909027116, -19.03943276465977164, 27.49890960531435624 ) ) ;
#43542=CARTESIAN_POINT ( 'NONE',  ( 9.564922557960805705, 16.46253265017160317, 104.5822429386476955 ) ) ;
#43543=CARTESIAN_POINT ( 'NONE',  ( 21.55341960407619695, -5.719274019375665929, 31.04275706135234714 ) ) ;
#43544=CARTESIAN_POINT ( 'NONE',  ( -19.02544592524334988, -5.153800228976617603, 28.95942372801900433 ) ) ;
#43545=CARTESIAN_POINT ( 'NONE',  ( -19.03943276465977164, 0.05219959533909376836, 26.24890960531435624 ) ) ;
#43546=CARTESIAN_POINT ( 'NONE',  ( 21.52544592524334988, 5.823673210054432836, 76.45942372801901854 ) ) ;
#43547=CARTESIAN_POINT ( 'NONE',  ( 17.50000000000002132, 5.499999999999984013, 98.78230962303568674 ) ) ;
#43548=CARTESIAN_POINT ( 'NONE',  ( 16.55341960407611168, 4.379528057220329451, 33.95724293864769550 ) ) ;
#43550=CARTESIAN_POINT ( 'NONE',  ( -18.67979575497178146, -10.72451020669898902, 21.66557627198102409 ) ) ;
#43551=CARTESIAN_POINT ( 'NONE',  ( 14.29746914071049879, -8.314922557960816363, 88.33224293864769550 ) ) ;
#43553=CARTESIAN_POINT ( 'NONE',  ( 16.51473224551069308, 9.474510206698969483, 79.16557627198103830 ) ) ;
#43554=CARTESIAN_POINT ( 'NONE',  ( -8.224510206698948167, 14.34966873604960824, 70.41557627198102409 ) ) ;
#43555=CARTESIAN_POINT ( 'NONE',  ( 13.97604488694548053, -13.89961937509957401, 105.6260903946856757 ) ) ;
#43556=CARTESIAN_POINT ( 'NONE',  ( -15.72974639402197994, 15.80617190586746368, 65.62390960531436690 ) ) ;
#43558=CARTESIAN_POINT ( 'NONE',  ( -16.46253265017160317, 9.564922557960807481, 30.83224293864769550 ) ) ;
#43560=CARTESIAN_POINT ( 'NONE',  ( 13.89961937509977652, -13.97604488694527269, 83.12390960531436690 ) ) ;
#43561=CARTESIAN_POINT ( 'NONE',  ( 10.72451020669898902, -18.67979575497178502, 72.91557627198103830 ) ) ;
#43562=CARTESIAN_POINT ( 'NONE',  ( -8.314922557961024197, 14.29746914071037800, 107.9177570613523471 ) ) ;
#43563=CARTESIAN_POINT ( 'NONE',  ( 5.049401038298161559, -19.05341960407611168, 87.70724293864769550 ) ) ;
#43564=CARTESIAN_POINT ( 'NONE',  ( 19.02544592524334988, 5.153800228976608722, 61.45942372801900433 ) ) ;
#43565=CARTESIAN_POINT ( 'NONE',  ( -18.67979575497193778, 10.72451020669871902, 98.33442372801901854 ) ) ;
#43566=CARTESIAN_POINT ( 'NONE',  ( -10.81492255796078084, -18.62759615963271287, 82.08224293864768129 ) ) ;
#43567=CARTESIAN_POINT ( 'NONE',  ( -9.474510206698964154, 16.51473224551069663, 115.4155762719810241 ) ) ;
#43568=CARTESIAN_POINT ( 'NONE',  ( -19.02544592524342804, 5.153800228976336051, 46.04057627198101699 ) ) ;
#43569=CARTESIAN_POINT ( 'NONE',  ( 16.52544592524335698, 4.483927247898782831, 111.4594237280190328 ) ) ;
#43570=CARTESIAN_POINT ( 'NONE',  ( 9.474510206698971260, -16.51473224551069308, 57.91557627198103120 ) ) ;
#43572=CARTESIAN_POINT ( 'NONE',  ( -10.72451020669870658, -18.67979575497194134, 104.5844237280190185 ) ) ;
#43574=CARTESIAN_POINT ( 'NONE',  ( 14.34966873604960469, 8.224510206698951720, 74.16557627198102409 ) ) ;
#43575=CARTESIAN_POINT ( 'NONE',  ( -10.72451020669898014, 18.67979575497178502, 110.4155762719810383 ) ) ;
#43576=CARTESIAN_POINT ( 'NONE',  ( -21.52544592524343514, 5.823673210054127303, 101.0405762719810383 ) ) ;
#43578=CARTESIAN_POINT ( 'NONE',  ( -10.72451020669898014, 18.67979575497178502, 60.41557627198102409 ) ) ;
#43579=CARTESIAN_POINT ( 'NONE',  ( 12.06949235617739724, 12.14591786802326823, 86.87609039468568994 ) ) ;
#43580=CARTESIAN_POINT ( 'NONE',  ( -8.224510206698948167, 14.34966873604960824, 110.4155762719810383 ) ) ;
#43581=CARTESIAN_POINT ( 'NONE',  ( 16.46253265017160672, -9.564922557960803928, 53.33224293864768839 ) ) ;
#43582=CARTESIAN_POINT ( 'NONE',  ( -8.314922557961024197, 14.29746914071037800, 102.9177570613523756 ) ) ;
#43583=CARTESIAN_POINT ( 'NONE',  ( 10.81492255796106328, -18.62759615963255655, 50.41775706135235424 ) ) ;
#43584=CARTESIAN_POINT ( 'NONE',  ( -9.474510206698964154, 16.51473224551069663, 115.4155762719810241 ) ) ;
#43585=CARTESIAN_POINT ( 'NONE',  ( 10.81492255796106328, -18.62759615963255655, 85.41775706135236135 ) ) ;
#43586=CARTESIAN_POINT ( 'NONE',  ( -19.03943276465977164, 0.05219959533909376836, 36.24890960531436690 ) ) ;
#43587=CARTESIAN_POINT ( 'NONE',  ( 5.153800228976335163, 19.02544592524342804, 44.79057627198103830 ) ) ;
#43588=ORIENTED_EDGE ( 'NONE', *, *, #51079, .T. ) ;
#43589=CARTESIAN_POINT ( 'NONE',  ( 21.53943276465977519, 0.05219959533937863772, 71.25109039468568994 ) ) ;
#43590=CARTESIAN_POINT ( 'NONE',  ( 19.02544592524343514, -5.153800228976328945, 103.5405762719809957 ) ) ;
#43591=CARTESIAN_POINT ( 'NONE',  ( 9.564922557961047289, -16.46253265017146816, 75.41775706135234714 ) ) ;
#43592=CARTESIAN_POINT ( 'NONE',  ( 21.52544592524334988, 5.823673210054432836, 51.45942372801901854 ) ) ;
#43593=CARTESIAN_POINT ( 'NONE',  ( -16.52544592524335698, -4.483927247898792601, 23.95942372801901143 ) ) ;
#43594=CARTESIAN_POINT ( 'NONE',  ( 19.03943276465977164, 0.05219959533936151252, 71.25109039468566152 ) ) ;
#43595=CARTESIAN_POINT ( 'NONE',  ( 5.049401038298161559, -19.05341960407611168, 47.70724293864770260 ) ) ;
#43596=CARTESIAN_POINT ( 'NONE',  ( 16.46253265017146816, 9.564922557961045513, 86.66775706135233293 ) ) ;
#43597=EDGE_CURVE ( 'NONE', #155866, #52144, #192804, .T. ) ;
#43598=CARTESIAN_POINT ( 'NONE',  ( -8.224510206698948167, 14.34966873604960824, 30.41557627198101699 ) ) ;
#43599=CARTESIAN_POINT ( 'NONE',  ( -19.05341960407617563, 5.049401038297882671, 93.54275706135234714 ) ) ;
#43600=CARTESIAN_POINT ( 'NONE',  ( -4.483927247898539470, -16.52544592524342804, 37.29057627198102409 ) ) ;
#43601=CARTESIAN_POINT ( 'NONE',  ( 19.05341960407617918, -5.049401038297876454, 66.04275706135233293 ) ) ;
#43602=CARTESIAN_POINT ( 'NONE',  ( 0.05219959533934541429, -16.53943276465976808, 45.00109039468568284 ) ) ;
#43603=CARTESIAN_POINT ( 'NONE',  ( 5.049401038297881783, 19.05341960407617563, 22.29275706135233648 ) ) ;
#43604=CARTESIAN_POINT ( 'NONE',  ( -16.46253265017160317, 9.564922557960807481, 40.83224293864769550 ) ) ;
#43606=CARTESIAN_POINT ( 'NONE',  ( 14.34966873604972726, -8.224510206698740333, 45.83442372801901854 ) ) ;
#43609=CARTESIAN_POINT ( 'NONE',  ( 5.049401038298161559, -19.05341960407611168, 92.70724293864769550 ) ) ;
#43610=CARTESIAN_POINT ( 'NONE',  ( 18.22780087662122384, -5.500000000000022204, 86.01540105326108687 ) ) ;
#43612=CARTESIAN_POINT ( 'NONE',  ( 9.474510206698729675, 16.51473224551082808, 87.08442372801900433 ) ) ;
#43613=CARTESIAN_POINT ( 'NONE',  ( 9.564922557960805705, 16.46253265017160317, 114.5822429386476955 ) ) ;
#43614=CARTESIAN_POINT ( 'NONE',  ( 16.46253265017146816, 9.564922557961045513, 21.66775706135233648 ) ) ;
#43615=CARTESIAN_POINT ( 'NONE',  ( -19.05341960407617563, 5.049401038297882671, 98.54275706135233293 ) ) ;
#43616=CARTESIAN_POINT ( 'NONE',  ( 12.06949235617757843, -12.14591786802309237, 113.1239096053143953 ) ) ;
#43617=CARTESIAN_POINT ( 'NONE',  ( -19.05341960407611168, -5.049401038298163336, 41.45724293864769550 ) ) ;
#43618=CARTESIAN_POINT ( 'NONE',  ( 21.55341960407610458, 5.719274019375980345, 53.95724293864770260 ) ) ;
#43619=CARTESIAN_POINT ( 'NONE',  ( -0.05219959533909027116, -19.03943276465977164, 22.49890960531436690 ) ) ;
#43621=CARTESIAN_POINT ( 'NONE',  ( -0.05219959533936034679, 19.03943276465977164, 67.50109039468566152 ) ) ;
#43622=CARTESIAN_POINT ( 'NONE',  ( -16.55341960407611168, -4.379528057220339221, 51.45724293864770260 ) ) ;
#43623=CARTESIAN_POINT ( 'NONE',  ( -15.72974639402197994, 15.80617190586746368, 35.62390960531437401 ) ) ;
#43625=CARTESIAN_POINT ( 'NONE',  ( -5.719274019375665041, -21.55341960407619695, 94.79275706135234714 ) ) ;
#43626=CARTESIAN_POINT ( 'NONE',  ( 0.05219959533907565091, 21.53943276465977519, 79.99890960531435269 ) ) ;
#43627=CARTESIAN_POINT ( 'NONE',  ( 5.719274019375673035, 21.55341960407619339, 62.29275706135236845 ) ) ;
#43628=CARTESIAN_POINT ( 'NONE',  ( -21.52544592524334988, -5.823673210054445271, 63.95942372801901854 ) ) ;
#43629=CARTESIAN_POINT ( 'NONE',  ( 16.51473224551069308, 9.474510206698969483, 94.16557627198103830 ) ) ;
#43630=CARTESIAN_POINT ( 'NONE',  ( -12.14591786802326823, 12.06949235617739902, 98.12609039468570415 ) ) ;
#43631=CARTESIAN_POINT ( 'NONE',  ( -15.72974639402176322, -15.80617190586768395, 69.37609039468567573 ) ) ;
#43632=CARTESIAN_POINT ( 'NONE',  ( -14.29746914071049879, 8.314922557960819915, 115.8322429386477097 ) ) ;
#43634=CARTESIAN_POINT ( 'NONE',  ( -4.483927247898539470, -16.52544592524342804, 62.29057627198102409 ) ) ;
#43635=CARTESIAN_POINT ( 'NONE',  ( 4.379528057220339221, -16.55341960407611168, 32.70724293864770260 ) ) ;
#43636=CARTESIAN_POINT ( 'NONE',  ( 21.55341960407610458, 5.719274019375980345, 38.95724293864768839 ) ) ;
#43637=CARTESIAN_POINT ( 'NONE',  ( 0.05219959533909260263, 19.03943276465977164, 44.99890960531435979 ) ) ;
#43638=CARTESIAN_POINT ( 'NONE',  ( -21.53943276465977519, 0.05219959533907696930, 61.24890960531435979 ) ) ;
#43639=CARTESIAN_POINT ( 'NONE',  ( -5.049401038297874678, -19.05341960407617918, 54.79275706135234003 ) ) ;
#43640=CARTESIAN_POINT ( 'NONE',  ( -16.21995358207306026, -7.366697692864122793, 40.06448998487842772 ) ) ;
#43641=CARTESIAN_POINT ( 'NONE',  ( 12.14591786802309770, 12.06949235617756955, 44.37390960531435979 ) ) ;
#43642=CARTESIAN_POINT ( 'NONE',  ( -5.719274019375978568, 21.55341960407610458, 30.20724293864769550 ) ) ;
#43643=ORIENTED_EDGE ( 'NONE', *, *, #60477, .F. ) ;
#43646=CARTESIAN_POINT ( 'NONE',  ( -12.06949235617739369, -12.14591786802326823, 74.37609039468568994 ) ) ;
#43647=CARTESIAN_POINT ( 'NONE',  ( -19.02544592524334988, -5.153800228976617603, 78.95942372801900433 ) ) ;
#43649=CARTESIAN_POINT ( 'NONE',  ( 8.314922557960818139, 14.29746914071049879, 44.58224293864769550 ) ) ;
#43650=CARTESIAN_POINT ( 'NONE',  ( 17.05587630539789146, -6.762274262135623992, 53.24180309037312497 ) ) ;
#43651=CARTESIAN_POINT ( 'NONE',  ( 16.53943276465976808, -0.05219959533910856209, 23.74890960531435269 ) ) ;
#43652=CARTESIAN_POINT ( 'NONE',  ( -13.97604488694527625, -13.89961937509977652, 46.87390960531435979 ) ) ;
#43653=CARTESIAN_POINT ( 'NONE',  ( -0.05219959533909027116, -19.03943276465977164, 72.49890960531435269 ) ) ;
#43654=AXIS2_PLACEMENT_3D ( 'NONE', #27724, #151056, #174160 ) ;
#43655=CARTESIAN_POINT ( 'NONE',  ( 19.02544592524343514, -5.153800228976328945, 43.54057627198103120 ) ) ;
#43656=CARTESIAN_POINT ( 'NONE',  ( -15.72974639402176322, -15.80617190586768395, 49.37609039468569705 ) ) ;
#43657=CARTESIAN_POINT ( 'NONE',  ( -19.05341960407611168, -5.049401038298163336, 66.45724293864769550 ) ) ;
#43659=CARTESIAN_POINT ( 'NONE',  ( 9.564922557960805705, 16.46253265017160317, 64.58224293864769550 ) ) ;
#43660=CARTESIAN_POINT ( 'NONE',  ( 10.72451020669898902, -18.67979575497178502, 42.91557627198103120 ) ) ;
#43661=CARTESIAN_POINT ( 'NONE',  ( -16.51473224551069308, -9.474510206698971260, 31.66557627198102054 ) ) ;
#43662=CARTESIAN_POINT ( 'NONE',  ( -18.67979575497178146, -10.72451020669898902, 41.66557627198103120 ) ) ;
#43663=CARTESIAN_POINT ( 'NONE',  ( -4.483927247898782831, 16.52544592524335698, 92.70942372801901854 ) ) ;
#43664=CARTESIAN_POINT ( 'NONE',  ( -9.564922557961040184, 16.46253265017147172, 27.91775706135232582 ) ) ;
#43665=CARTESIAN_POINT ( 'NONE',  ( -14.34966873604972548, 8.224510206698743886, 73.33442372801901854 ) ) ;
#43666=CARTESIAN_POINT ( 'NONE',  ( 0.05219959533909260263, 19.03943276465977164, 114.9989096053143669 ) ) ;
#43667=CARTESIAN_POINT ( 'NONE',  ( -4.483927247898782831, 16.52544592524335698, 47.70942372801902565 ) ) ;
#43668=CARTESIAN_POINT ( 'NONE',  ( 4.483927247898790824, -16.52544592524335698, 35.20942372801901854 ) ) ;
#43669=CARTESIAN_POINT ( 'NONE',  ( 13.97604488694527802, 13.89961937509977652, 109.3739096053143669 ) ) ;
#43670=CARTESIAN_POINT ( 'NONE',  ( 8.314922557961029526, -14.29746914071037800, 30.41775706135234358 ) ) ;
#43671=CARTESIAN_POINT ( 'NONE',  ( 9.564922557960805705, 16.46253265017160317, 39.58224293864768839 ) ) ;
#43672=CARTESIAN_POINT ( 'NONE',  ( -10.72451020669870658, -18.67979575497194134, 29.58442372801901854 ) ) ;
#43673=CARTESIAN_POINT ( 'NONE',  ( 9.474510206698729675, 16.51473224551082808, 112.0844237280190043 ) ) ;
#43674=CARTESIAN_POINT ( 'NONE',  ( 8.314922557961029526, -14.29746914071037800, 105.4177570613523613 ) ) ;
#43676=CARTESIAN_POINT ( 'NONE',  ( 0.05219959533937995610, -21.53943276465977519, 105.0010903946856757 ) ) ;
#43677=CARTESIAN_POINT ( 'NONE',  ( -0.05219959533936034679, 19.03943276465977164, 92.50109039468566152 ) ) ;
#43678=CARTESIAN_POINT ( 'NONE',  ( 16.55341960407611168, 4.379528057220329451, 53.95724293864770260 ) ) ;
#43679=CARTESIAN_POINT ( 'NONE',  ( -14.29746914071049879, 8.314922557960819915, 115.8322429386477097 ) ) ;
#43680=CARTESIAN_POINT ( 'NONE',  ( -19.05341960407617563, 5.049401038297882671, 63.54275706135234003 ) ) ;
#43682=CARTESIAN_POINT ( 'NONE',  ( 10.72451020669871369, 18.67979575497193778, 47.08442372801901854 ) ) ;
#43683=CARTESIAN_POINT ( 'NONE',  ( -16.55341960407617563, 4.379528057220093196, 23.54275706135235424 ) ) ;
#43685=CARTESIAN_POINT ( 'NONE',  ( -9.564922557960796823, -16.46253265017161027, 112.0822429386476955 ) ) ;
#43686=CARTESIAN_POINT ( 'NONE',  ( 21.55341960407610458, 5.719274019375980345, 73.95724293864769550 ) ) ;
#43687=CARTESIAN_POINT ( 'NONE',  ( -19.03943276465977164, -0.05219959533935918106, 108.7510903946856615 ) ) ;
#43688=CARTESIAN_POINT ( 'NONE',  ( -16.51473224551069308, -9.474510206698971260, 96.66557627198102409 ) ) ;
#43690=CARTESIAN_POINT ( 'NONE',  ( -16.46253265017160317, 9.564922557960807481, 30.83224293864769550 ) ) ;
#43691=CARTESIAN_POINT ( 'NONE',  ( -0.05219959533937732626, 21.53943276465977519, 97.50109039468567573 ) ) ;
#43692=CARTESIAN_POINT ( 'NONE',  ( 16.51473224551069308, 9.474510206698969483, 44.16557627198103120 ) ) ;
#43694=CARTESIAN_POINT ( 'NONE',  ( 15.80617190586769283, -15.72974639402175789, 45.62609039468567573 ) ) ;
#43695=CARTESIAN_POINT ( 'NONE',  ( 15.72974639402176855, 15.80617190586768217, 91.87609039468568994 ) ) ;
#43696=CARTESIAN_POINT ( 'NONE',  ( 14.29746914071037800, 8.314922557961029526, 106.6677570613523756 ) ) ;
#43697=CARTESIAN_POINT ( 'NONE',  ( -5.153800228976328057, -19.02544592524343514, 77.29057627198099567 ) ) ;
#43698=CARTESIAN_POINT ( 'NONE',  ( -15.72974639402176322, -15.80617190586768395, 49.37609039468569705 ) ) ;
#43699=CARTESIAN_POINT ( 'NONE',  ( 15.80617190586769283, -15.72974639402175789, 35.62609039468568994 ) ) ;
#43700=CARTESIAN_POINT ( 'NONE',  ( 13.89961937509957401, 13.97604488694547697, 76.87609039468566152 ) ) ;
#43701=CARTESIAN_POINT ( 'NONE',  ( -19.05341960407611168, -5.049401038298163336, 86.45724293864769550 ) ) ;
#43702=CARTESIAN_POINT ( 'NONE',  ( -0.05219959533910754901, -16.53943276465976808, 102.4989096053143811 ) ) ;
#43703=CARTESIAN_POINT ( 'NONE',  ( 18.67979575497178502, 10.72451020669898547, 94.16557627198103830 ) ) ;
#43704=CARTESIAN_POINT ( 'NONE',  ( -8.314922557960811034, -14.29746914071050412, 77.08224293864769550 ) ) ;
#43705=CARTESIAN_POINT ( 'NONE',  ( 21.55341960407619695, -5.719274019375665929, 111.0427570613523613 ) ) ;
#43706=CARTESIAN_POINT ( 'NONE',  ( 16.53943276465976808, -0.05219959533910856209, 98.74890960531438111 ) ) ;
#43707=CARTESIAN_POINT ( 'NONE',  ( 13.89961937509977652, -13.97604488694527269, 33.12390960531434558 ) ) ;
#43708=CARTESIAN_POINT ( 'NONE',  ( 5.049401038297881783, 19.05341960407617563, 82.29275706135229029 ) ) ;
#43709=CIRCLE ( 'NONE', #156707, 2.000000000000001776 ) ;
#43710=CARTESIAN_POINT ( 'NONE',  ( 4.379528057220339221, -16.55341960407611168, 42.70724293864770260 ) ) ;
#43711=CARTESIAN_POINT ( 'NONE',  ( -21.52544592524334988, -5.823673210054445271, 93.95942372801903275 ) ) ;
#43712=CARTESIAN_POINT ( 'NONE',  ( 9.474510206698971260, -16.51473224551069308, 107.9155762719810383 ) ) ;
#43713=CARTESIAN_POINT ( 'NONE',  ( 0.05219959533936267826, -19.03943276465977164, 70.00109039468566152 ) ) ;
#43714=CARTESIAN_POINT ( 'NONE',  ( 21.55341960407610458, 5.719274019375980345, 83.95724293864770971 ) ) ;
#43715=CARTESIAN_POINT ( 'NONE',  ( 0.05219959533937995610, -21.53943276465977519, 30.00109039468568284 ) ) ;
#43716=CARTESIAN_POINT ( 'NONE',  ( -16.52544592524335698, -4.483927247898792601, 23.95942372801901143 ) ) ;
#43717=CARTESIAN_POINT ( 'NONE',  ( -8.224510206698735004, -14.34966873604973081, 89.58442372801901854 ) ) ;
#43718=CARTESIAN_POINT ( 'NONE',  ( -13.89961937509977652, 13.97604488694528158, 30.62390960531435269 ) ) ;
#43719=CARTESIAN_POINT ( 'NONE',  ( -21.55341960407619339, 5.719274019375674811, 38.54275706135234714 ) ) ;
#43720=CARTESIAN_POINT ( 'NONE',  ( 13.97604488694527802, 13.89961937509977652, 24.37390960531435624 ) ) ;
#43722=CARTESIAN_POINT ( 'NONE',  ( -12.14591786802326823, 12.06949235617739902, 53.12609039468568284 ) ) ;
#43723=CARTESIAN_POINT ( 'NONE',  ( -14.29746914071049879, 8.314922557960819915, 80.83224293864769550 ) ) ;
#43724=CARTESIAN_POINT ( 'NONE',  ( 18.67979575497178502, 10.72451020669898547, 74.16557627198102409 ) ) ;
#43725=CARTESIAN_POINT ( 'NONE',  ( -14.34966873604960291, -8.224510206698953496, 31.66557627198102054 ) ) ;
#43726=CARTESIAN_POINT ( 'NONE',  ( -8.314922557961024197, 14.29746914071037800, 52.91775706135235424 ) ) ;
#43727=CARTESIAN_POINT ( 'NONE',  ( 9.474510206698971260, -16.51473224551069308, 42.91557627198103120 ) ) ;
#43728=CARTESIAN_POINT ( 'NONE',  ( 14.29746914071037800, 8.314922557961029526, 91.66775706135234714 ) ) ;
#43729=CARTESIAN_POINT ( 'NONE',  ( -13.89961937509957401, -13.97604488694547875, 89.37609039468563310 ) ) ;
#43730=CARTESIAN_POINT ( 'NONE',  ( 21.52544592524344225, -5.823673210054117533, 88.54057627198103830 ) ) ;
#43731=CARTESIAN_POINT ( 'NONE',  ( 16.53943276465976808, 0.05219959533934440121, 111.2510903946856899 ) ) ;
#43734=CARTESIAN_POINT ( 'NONE',  ( -0.05219959533907301413, -21.53943276465977519, 57.49890960531435979 ) ) ;
#43735=ORIENTED_EDGE ( 'NONE', *, *, #44529, .F. ) ;
#43736=ORIENTED_EDGE ( 'NONE', *, *, #53248, .F. ) ;
#43737=CARTESIAN_POINT ( 'NONE',  ( -14.34966873604972548, 8.224510206698743886, 93.33442372801901854 ) ) ;
#43739=CARTESIAN_POINT ( 'NONE',  ( -5.823673210054116645, -21.52544592524344225, 22.29057627198102765 ) ) ;
#43741=CARTESIAN_POINT ( 'NONE',  ( -0.05219959533907301413, -21.53943276465977519, 72.49890960531435269 ) ) ;
#43742=CARTESIAN_POINT ( 'NONE',  ( -8.314922557961024197, 14.29746914071037800, 112.9177570613523329 ) ) ;
#43743=CARTESIAN_POINT ( 'NONE',  ( -12.06949235617739369, -12.14591786802326823, 24.37609039468567573 ) ) ;
#43744=CARTESIAN_POINT ( 'NONE',  ( -12.06949235617756955, 12.14591786802309770, 115.6239096053143669 ) ) ;
#43745=CARTESIAN_POINT ( 'NONE',  ( 8.224510206698742110, 14.34966873604972548, 32.08442372801901854 ) ) ;
#43746=CARTESIAN_POINT ( 'NONE',  ( 19.02544592524343514, -5.153800228976328945, 58.54057627198102409 ) ) ;
#43748=CARTESIAN_POINT ( 'NONE',  ( 19.03943276465977164, -0.05219959533909143690, 103.7489096053143669 ) ) ;
#43749=CARTESIAN_POINT ( 'NONE',  ( -16.55341960407617563, 4.379528057220093196, 93.54275706135234714 ) ) ;
#43750=CARTESIAN_POINT ( 'NONE',  ( 0.05219959533936267826, -19.03943276465977164, 95.00109039468567573 ) ) ;
#43751=CARTESIAN_POINT ( 'NONE',  ( -16.46253265017146816, -9.564922557961047289, 24.16775706135233648 ) ) ;
#43752=CARTESIAN_POINT ( 'NONE',  ( 21.53943276465977519, -0.05219959533907433946, 73.74890960531433848 ) ) ;
#43753=CARTESIAN_POINT ( 'NONE',  ( 0.05219959533934541429, -16.53943276465976808, 95.00109039468568994 ) ) ;
#43754=CARTESIAN_POINT ( 'NONE',  ( -9.564922557961040184, 16.46253265017147172, 92.91775706135233293 ) ) ;
#43755=CARTESIAN_POINT ( 'NONE',  ( 16.51473224551069308, 9.474510206698969483, 44.16557627198103120 ) ) ;
#43756=CARTESIAN_POINT ( 'NONE',  ( -5.049401038298153566, 19.05341960407611168, 85.20724293864766707 ) ) ;
#43757=CARTESIAN_POINT ( 'NONE',  ( 10.72451020669871369, 18.67979575497193778, 62.08442372801901143 ) ) ;
#43758=CARTESIAN_POINT ( 'NONE',  ( -9.474510206698964154, 16.51473224551069663, 65.41557627198102409 ) ) ;
#43759=CARTESIAN_POINT ( 'NONE',  ( -14.29746914071049879, 8.314922557960819915, 80.83224293864769550 ) ) ;
#43760=CARTESIAN_POINT ( 'NONE',  ( -16.20579543436679160, -7.371946100355097897, 85.56520834171882939 ) ) ;
#43761=CARTESIAN_POINT ( 'NONE',  ( 8.314922557960818139, 14.29746914071049879, 79.58224293864769550 ) ) ;
#43762=CARTESIAN_POINT ( 'NONE',  ( 18.62759615963271287, -10.81492255796078972, 78.33224293864770971 ) ) ;
#43763=CARTESIAN_POINT ( 'NONE',  ( -5.049401038297874678, -19.05341960407617918, 89.79275706135230450 ) ) ;
#43765=CARTESIAN_POINT ( 'NONE',  ( -16.51473224551082808, 9.474510206698731452, 43.33442372801900433 ) ) ;
#43767=CARTESIAN_POINT ( 'NONE',  ( 13.97604488694527802, 13.89961937509977652, 79.37390960531435269 ) ) ;
#43768=CARTESIAN_POINT ( 'NONE',  ( -9.474510206698964154, 16.51473224551069663, 80.41557627198103830 ) ) ;
#43769=CARTESIAN_POINT ( 'NONE',  ( -12.14591786802326823, 12.06949235617739902, 63.12609039468568994 ) ) ;
#43771=CARTESIAN_POINT ( 'NONE',  ( -19.02544592524334988, -5.153800228976617603, 48.95942372801900433 ) ) ;
#43772=CARTESIAN_POINT ( 'NONE',  ( -17.49999999999999645, 5.499999999999992895, 98.71769037696435589 ) ) ;
#43773=CARTESIAN_POINT ( 'NONE',  ( -16.51473224551069308, -9.474510206698971260, 106.6655762719810383 ) ) ;
#43774=CARTESIAN_POINT ( 'NONE',  ( 12.06949235617739724, 12.14591786802326823, 96.87609039468568994 ) ) ;
#43776=CARTESIAN_POINT ( 'NONE',  ( 4.483927247898790824, -16.52544592524335698, 75.20942372801901854 ) ) ;
#43777=CARTESIAN_POINT ( 'NONE',  ( -16.81555441253551564, 7.025013491695477619, 30.63685445334257551 ) ) ;
#43778=CARTESIAN_POINT ( 'NONE',  ( -16.52544592524335698, -4.483927247898792601, 48.95942372801902565 ) ) ;
#43779=CARTESIAN_POINT ( 'NONE',  ( 16.51473224551069308, 9.474510206698969483, 74.16557627198103830 ) ) ;
#43780=CARTESIAN_POINT ( 'NONE',  ( 21.53943276465977519, 0.05219959533937863772, 71.25109039468568994 ) ) ;
#43781=CARTESIAN_POINT ( 'NONE',  ( -9.474510206698720793, -16.51473224551083518, 69.58442372801901854 ) ) ;
#43782=CARTESIAN_POINT ( 'NONE',  ( 19.05341960407617918, -5.049401038297876454, 21.04275706135232582 ) ) ;
#43784=CARTESIAN_POINT ( 'NONE',  ( 5.049401038298161559, -19.05341960407611168, 57.70724293864769550 ) ) ;
#43785=CARTESIAN_POINT ( 'NONE',  ( 0.05219959533909260263, 19.03943276465977164, 49.99890960531435979 ) ) ;
#43787=CARTESIAN_POINT ( 'NONE',  ( -5.823673210054116645, -21.52544592524344225, 67.29057627198103830 ) ) ;
#43788=CARTESIAN_POINT ( 'NONE',  ( -15.72974639402197994, 15.80617190586746368, 35.62390960531437401 ) ) ;
#43789=CARTESIAN_POINT ( 'NONE',  ( 19.03943276465977164, -0.05219959533909143690, 23.74890960531435269 ) ) ;
#43790=CARTESIAN_POINT ( 'NONE',  ( -12.06949235617739369, -12.14591786802326823, 49.37609039468569705 ) ) ;
#43792=EDGE_CURVE ( 'NONE', #60746, #8743, #141726, .T. ) ;
#43793=CARTESIAN_POINT ( 'NONE',  ( -15.72974639402176322, -15.80617190586768395, 34.37609039468568284 ) ) ;
#43794=CARTESIAN_POINT ( 'NONE',  ( -0.05219959533910754901, -16.53943276465976808, 47.49890960531435979 ) ) ;
#43796=CARTESIAN_POINT ( 'NONE',  ( -0.05219959533936034679, 19.03943276465977164, 102.5010903946856757 ) ) ;
#43797=CARTESIAN_POINT ( 'NONE',  ( 16.46253265017146816, 9.564922557961045513, 36.66775706135233293 ) ) ;
#43798=CARTESIAN_POINT ( 'NONE',  ( 8.224510206698953496, -14.34966873604960469, 42.91557627198103120 ) ) ;
#43799=CARTESIAN_POINT ( 'NONE',  ( -21.52544592524343514, 5.823673210054127303, 116.0405762719810383 ) ) ;
#43801=CARTESIAN_POINT ( 'NONE',  ( -15.72974639402197994, 15.80617190586746368, 80.62390960531438111 ) ) ;
#43802=CARTESIAN_POINT ( 'NONE',  ( 13.97604488694527802, 13.89961937509977652, 89.37390960531436690 ) ) ;
#43803=CARTESIAN_POINT ( 'NONE',  ( 16.52544592524342804, -4.483927247898539470, 58.54057627198103120 ) ) ;
#43804=CARTESIAN_POINT ( 'NONE',  ( -9.564922557960796823, -16.46253265017161027, 102.0822429386477097 ) ) ;
#43806=CARTESIAN_POINT ( 'NONE',  ( 0.05219959533936267826, -19.03943276465977164, 50.00109039468566863 ) ) ;
#43807=CARTESIAN_POINT ( 'NONE',  ( -10.81492255796078084, -18.62759615963271287, 112.0822429386477097 ) ) ;
#43808=CARTESIAN_POINT ( 'NONE',  ( 5.049401038298161559, -19.05341960407611168, 42.70724293864767418 ) ) ;
#43809=CARTESIAN_POINT ( 'NONE',  ( -9.564922557960796823, -16.46253265017161027, 22.08224293864768839 ) ) ;
#43810=CARTESIAN_POINT ( 'NONE',  ( -5.823673210054431948, 21.52544592524334988, 52.70942372801902565 ) ) ;
#43812=CARTESIAN_POINT ( 'NONE',  ( 14.34966873604960469, 8.224510206698951720, 44.16557627198103120 ) ) ;
#43813=CARTESIAN_POINT ( 'NONE',  ( 13.97604488694527802, 13.89961937509977652, 49.37390960531434558 ) ) ;
#43814=CARTESIAN_POINT ( 'NONE',  ( -13.89961937509977652, 13.97604488694528158, 95.62390960531436690 ) ) ;
#43815=CARTESIAN_POINT ( 'NONE',  ( -5.719274019375978568, 21.55341960407610458, 75.20724293864769550 ) ) ;
#43817=CARTESIAN_POINT ( 'NONE',  ( -19.05341960407611168, -5.049401038298163336, 51.45724293864770260 ) ) ;
#43818=CARTESIAN_POINT ( 'NONE',  ( -18.67979575497178146, -10.72451020669898902, 56.66557627198103830 ) ) ;
#43819=CARTESIAN_POINT ( 'NONE',  ( -15.72974639402176322, -15.80617190586768395, 84.37609039468570415 ) ) ;
#43820=DIRECTION ( 'NONE',  ( 1.000000000000000000, 0.000000000000000000, 0.000000000000000000 ) ) ;
#43821=CARTESIAN_POINT ( 'NONE',  ( -4.483927247898782831, 16.52544592524335698, 77.70942372801900433 ) ) ;
#43822=CARTESIAN_POINT ( 'NONE',  ( -0.05219959533910754901, -16.53943276465976808, 72.49890960531435269 ) ) ;
#43823=CARTESIAN_POINT ( 'NONE',  ( -16.46253265017160317, 9.564922557960807481, 70.83224293864770971 ) ) ;
#43825=CARTESIAN_POINT ( 'NONE',  ( -5.153800228976607833, 19.02544592524334988, 22.70942372801899012 ) ) ;
#43826=CARTESIAN_POINT ( 'NONE',  ( 16.52544592524335698, 4.483927247898782831, 91.45942372801901854 ) ) ;
#43827=CARTESIAN_POINT ( 'NONE',  ( -16.46253265017146816, -9.564922557961047289, 19.16775706135233293 ) ) ;
#43828=CARTESIAN_POINT ( 'NONE',  ( 19.05341960407611168, 5.049401038298154454, 73.95724293864768129 ) ) ;
#43829=CARTESIAN_POINT ( 'NONE',  ( 5.719274019375991003, -21.55341960407610458, 52.70724293864769550 ) ) ;
#43830=CARTESIAN_POINT ( 'NONE',  ( 14.29746914071037800, 8.314922557961029526, 31.66775706135234358 ) ) ;
#43831=CARTESIAN_POINT ( 'NONE',  ( -10.81492255796105439, 18.62759615963255655, 97.91775706135236135 ) ) ;
#43832=CARTESIAN_POINT ( 'NONE',  ( -16.52544592524335698, -4.483927247898792601, 58.95942372801902565 ) ) ;
#43833=CARTESIAN_POINT ( 'NONE',  ( 0.05219959533907565091, 21.53943276465977519, 109.9989096053143527 ) ) ;
#43834=CARTESIAN_POINT ( 'NONE',  ( 5.153800228976615827, -19.02544592524334988, 110.2094237280189901 ) ) ;
#43835=CARTESIAN_POINT ( 'NONE',  ( 19.05341960407611168, 5.049401038298154454, 93.95724293864769550 ) ) ;
#43836=CARTESIAN_POINT ( 'NONE',  ( 14.29746914071037800, 8.314922557961029526, 31.66775706135234358 ) ) ;
#43837=CARTESIAN_POINT ( 'NONE',  ( -0.05219959533909027116, -19.03943276465977164, 52.49890960531436690 ) ) ;
#43838=CARTESIAN_POINT ( 'NONE',  ( -12.06949235617739369, -12.14591786802326823, 34.37609039468568284 ) ) ;
#43839=CARTESIAN_POINT ( 'NONE',  ( 12.06949235617757843, -12.14591786802309237, 73.12390960531436690 ) ) ;
#43840=CARTESIAN_POINT ( 'NONE',  ( 16.55341960407618274, -4.379528057220086978, 86.04275706135236135 ) ) ;
#43841=CARTESIAN_POINT ( 'NONE',  ( -10.81492255796105439, 18.62759615963255655, 42.91775706135235424 ) ) ;
#43842=CARTESIAN_POINT ( 'NONE',  ( 13.89961937509977652, -13.97604488694527269, 63.12390960531435979 ) ) ;
#43843=CARTESIAN_POINT ( 'NONE',  ( -19.03943276465977164, 0.05219959533909376836, 81.24890960531436690 ) ) ;
#43844=CARTESIAN_POINT ( 'NONE',  ( 12.06949235617739724, 12.14591786802326823, 86.87609039468568994 ) ) ;
#43846=ORIENTED_EDGE ( 'NONE', *, *, #88147, .F. ) ;
#43847=ORIENTED_EDGE ( 'NONE', *, *, #191998, .F. ) ;
#43848=CARTESIAN_POINT ( 'NONE',  ( 0.05219959533936267826, -19.03943276465977164, 35.00109039468566863 ) ) ;
#43849=CARTESIAN_POINT ( 'NONE',  ( 16.46253265017160672, -9.564922557960803928, 93.33224293864769550 ) ) ;
#43850=CARTESIAN_POINT ( 'NONE',  ( 5.049401038298161559, -19.05341960407611168, 47.70724293864770260 ) ) ;
#43851=CARTESIAN_POINT ( 'NONE',  ( 16.46253265017160672, -9.564922557960803928, 108.3322429386476955 ) ) ;
#43852=CARTESIAN_POINT ( 'NONE',  ( -0.05219959533934338120, 16.53943276465976808, 37.50109039468568284 ) ) ;
#43853=B_SPLINE_CURVE_WITH_KNOTS ( 'NONE', 3,
 ( #29922, #108741, #153250, #75421, #186606, #15746, #198781, #109734, #137095, #91562, #141066, #77405, #76413, #140062, #60247, #199770, #121918, #14752, #47080, #184597, #46078, #185590 ),
 .UNSPECIFIED., .F., .F.,
 ( 4, 2, 2, 2, 2, 2, 2, 2, 2, 2, 4 ),
 ( 2.602085213965211027E-18, 0.001309639967555396075, 0.001964459951333086523, 0.002291869943221923507, 0.002455574939166342216, 0.002619279935110760058, 0.002782984931055178333, 0.002946689926999596608, 0.003274099918888406270, 0.003928919902666004778, 0.005238559870221203528 ),
 .UNSPECIFIED. ) ;
#43854=CARTESIAN_POINT ( 'NONE',  ( -19.02544592524334988, -5.153800228976617603, 58.95942372801900433 ) ) ;
#43855=CARTESIAN_POINT ( 'NONE',  ( -4.379528057220086978, -16.55341960407618274, 59.79275706135234714 ) ) ;
#43856=CARTESIAN_POINT ( 'NONE',  ( 16.46253265017160672, -9.564922557960803928, 108.3322429386476955 ) ) ;
#43857=CARTESIAN_POINT ( 'NONE',  ( -19.05341960407611168, -5.049401038298163336, 76.45724293864769550 ) ) ;
#43858=CARTESIAN_POINT ( 'NONE',  ( -15.72974639402197994, 15.80617190586746368, 100.6239096053143811 ) ) ;
#43859=CARTESIAN_POINT ( 'NONE',  ( -16.51473224551082808, 9.474510206698731452, 63.33442372801900433 ) ) ;
#43860=CARTESIAN_POINT ( 'NONE',  ( -19.02544592524342804, 5.153800228976336051, 96.04057627198103830 ) ) ;
#43861=DIRECTION ( 'NONE',  ( 1.000000000000000000, -0.000000000000000000, -0.000000000000000000 ) ) ;
#43862=CARTESIAN_POINT ( 'NONE',  ( 13.89961937509977652, -13.97604488694527269, 78.12390960531433848 ) ) ;
#43863=CARTESIAN_POINT ( 'NONE',  ( -12.06949235617756955, 12.14591786802309770, 30.62390960531436335 ) ) ;
#43864=CARTESIAN_POINT ( 'NONE',  ( -19.05341960407611168, -5.049401038298163336, 26.45724293864769550 ) ) ;
#43865=CARTESIAN_POINT ( 'NONE',  ( 19.02544592524334988, 5.153800228976608722, 41.45942372801900433 ) ) ;
#43866=CARTESIAN_POINT ( 'NONE',  ( 0.05219959533910956823, 16.53943276465976808, 74.99890960531435269 ) ) ;
#43867=CARTESIAN_POINT ( 'NONE',  ( 10.81492255796106328, -18.62759615963255655, 100.4177570613523471 ) ) ;
#43868=CARTESIAN_POINT ( 'NONE',  ( -0.05219959533909027116, -19.03943276465977164, 42.49890960531435269 ) ) ;
#43869=CARTESIAN_POINT ( 'NONE',  ( 8.314922557960818139, 14.29746914071049879, 34.58224293864770260 ) ) ;
#43870=CARTESIAN_POINT ( 'NONE',  ( 0.05219959533937995610, -21.53943276465977519, 110.0010903946856757 ) ) ;
#43871=CARTESIAN_POINT ( 'NONE',  ( 13.97604488694527802, 13.89961937509977652, 94.37390960531436690 ) ) ;
#43872=CARTESIAN_POINT ( 'NONE',  ( -5.153800228976328057, -19.02544592524343514, 92.29057627198099567 ) ) ;
#43873=CARTESIAN_POINT ( 'NONE',  ( -19.02544592524342804, 5.153800228976336051, 31.04057627198102409 ) ) ;
#43874=CARTESIAN_POINT ( 'NONE',  ( 12.06949235617757843, -12.14591786802309237, 113.1239096053143953 ) ) ;
#43875=CARTESIAN_POINT ( 'NONE',  ( 4.483927247898545687, 16.52544592524342804, 79.79057627198102409 ) ) ;
#43876=CARTESIAN_POINT ( 'NONE',  ( -21.55341960407610458, -5.719274019375992779, 81.45724293864769550 ) ) ;
#43877=CARTESIAN_POINT ( 'NONE',  ( 19.05341960407611168, 5.049401038298154454, 88.95724293864769550 ) ) ;
#43878=CARTESIAN_POINT ( 'NONE',  ( -5.823673210054116645, -21.52544592524344225, 92.29057627198103830 ) ) ;
#43879=CARTESIAN_POINT ( 'NONE',  ( 5.153800228976335163, 19.02544592524342804, 84.79057627198099567 ) ) ;
#43881=CARTESIAN_POINT ( 'NONE',  ( -18.22780087662126647, -5.499999999999827693, 63.98236817873107185 ) ) ;
#43882=CARTESIAN_POINT ( 'NONE',  ( 14.34966873604960469, 8.224510206698951720, 89.16557627198102409 ) ) ;
#43883=CARTESIAN_POINT ( 'NONE',  ( 16.51473224551069308, 9.474510206698969483, 69.16557627198102409 ) ) ;
#43884=CARTESIAN_POINT ( 'NONE',  ( 18.62759615963271287, -10.81492255796078972, 68.33224293864769550 ) ) ;
#43886=CARTESIAN_POINT ( 'NONE',  ( -10.72451020669898014, 18.67979575497178502, 35.41557627198102409 ) ) ;
#43888=CARTESIAN_POINT ( 'NONE',  ( -12.14591786802326823, 12.06949235617739902, 23.12609039468567573 ) ) ;
#43890=CARTESIAN_POINT ( 'NONE',  ( 0.05219959533910956823, 16.53943276465976808, 94.99890960531436690 ) ) ;
#43892=CARTESIAN_POINT ( 'NONE',  ( 5.153800228976335163, 19.02544592524342804, 84.79057627198099567 ) ) ;
#43893=CARTESIAN_POINT ( 'NONE',  ( -9.474510206698964154, 16.51473224551069663, 50.41557627198102409 ) ) ;
#43894=CARTESIAN_POINT ( 'NONE',  ( -14.34966873604960291, -8.224510206698953496, 81.66557627198103830 ) ) ;
#43895=CARTESIAN_POINT ( 'NONE',  ( 5.153800228976335163, 19.02544592524342804, 109.7905762719810099 ) ) ;
#43896=CARTESIAN_POINT ( 'NONE',  ( 0.05219959533936267826, -19.03943276465977164, 105.0010903946856615 ) ) ;
#43897=CARTESIAN_POINT ( 'NONE',  ( -21.52544592524334988, -5.823673210054445271, 58.95942372801902565 ) ) ;
#43898=CARTESIAN_POINT ( 'NONE',  ( 19.02544592524343514, -5.153800228976328945, 93.54057627198102409 ) ) ;
#43899=CARTESIAN_POINT ( 'NONE',  ( -21.53943276465977519, 0.05219959533907696930, 81.24890960531436690 ) ) ;
#43900=CARTESIAN_POINT ( 'NONE',  ( 16.55341960407618274, -4.379528057220086978, 66.04275706135236135 ) ) ;
#43901=CARTESIAN_POINT ( 'NONE',  ( 0.05219959533909260263, 19.03943276465977164, 24.99890960531435269 ) ) ;
#43902=CARTESIAN_POINT ( 'NONE',  ( 16.46253265017160672, -9.564922557960803928, 73.33224293864769550 ) ) ;
#43903=CARTESIAN_POINT ( 'NONE',  ( -21.52544592524343514, 5.823673210054127303, 81.04057627198102409 ) ) ;
#43904=CARTESIAN_POINT ( 'NONE',  ( 19.02544592524334988, 5.153800228976608722, 111.4594237280190043 ) ) ;
#43905=CARTESIAN_POINT ( 'NONE',  ( -14.29746914071049879, 8.314922557960819915, 40.83224293864769550 ) ) ;
#43906=CARTESIAN_POINT ( 'NONE',  ( -18.62759615963255300, -10.81492255796106328, 54.16775706135235424 ) ) ;
#43908=CARTESIAN_POINT ( 'NONE',  ( 4.483927247898790824, -16.52544592524335698, 90.20942372801903275 ) ) ;
#43909=CARTESIAN_POINT ( 'NONE',  ( -19.03943276465977164, 0.05219959533909376836, 116.2489096053143669 ) ) ;
#43911=CARTESIAN_POINT ( 'NONE',  ( -16.36317988757059183, 7.306389748694926745, 79.09789608363225000 ) ) ;
#43912=CARTESIAN_POINT ( 'NONE',  ( 14.29746914071037800, 8.314922557961029526, 101.6677570613523613 ) ) ;
#43913=CARTESIAN_POINT ( 'NONE',  ( -0.05219959533934338120, 16.53943276465976808, 47.50109039468568994 ) ) ;
#43914=CARTESIAN_POINT ( 'NONE',  ( 19.05341960407611168, 5.049401038298154454, 63.95724293864769550 ) ) ;
#43915=CARTESIAN_POINT ( 'NONE',  ( 16.51473224551069308, 9.474510206698969483, 69.16557627198102409 ) ) ;
#43916=CARTESIAN_POINT ( 'NONE',  ( 12.06949235617739724, 12.14591786802326823, 71.87609039468568994 ) ) ;
#43917=CARTESIAN_POINT ( 'NONE',  ( 0.05219959533910956823, 16.53943276465976808, 49.99890960531437401 ) ) ;
#43918=CARTESIAN_POINT ( 'NONE',  ( -5.153800228976328057, -19.02544592524343514, 52.29057627198100988 ) ) ;
#43919=CARTESIAN_POINT ( 'NONE',  ( -0.05219959533909027116, -19.03943276465977164, 52.49890960531436690 ) ) ;
#43920=CARTESIAN_POINT ( 'NONE',  ( 16.55341960407618274, -4.379528057220086978, 46.04275706135234714 ) ) ;
#43921=CARTESIAN_POINT ( 'NONE',  ( -5.049401038297874678, -19.05341960407617918, 99.79275706135234714 ) ) ;
#43922=CARTESIAN_POINT ( 'NONE',  ( -16.53943276465976808, 0.05219959533911058130, 101.2489096053143669 ) ) ;
#43923=CARTESIAN_POINT ( 'NONE',  ( 5.153800228976335163, 19.02544592524342804, 59.79057627198100988 ) ) ;
#43924=CARTESIAN_POINT ( 'NONE',  ( 19.05341960407617918, -5.049401038297876454, 101.0427570613523045 ) ) ;
#43926=CARTESIAN_POINT ( 'NONE',  ( 18.62759615963255655, 10.81492255796105972, 96.66775706135234714 ) ) ;
#43927=CARTESIAN_POINT ( 'NONE',  ( 0.05219959533934541429, -16.53943276465976808, 65.00109039468568994 ) ) ;
#43929=CARTESIAN_POINT ( 'NONE',  ( 18.67979575497178502, 10.72451020669898547, 64.16557627198102409 ) ) ;
#43930=CARTESIAN_POINT ( 'NONE',  ( -16.52544592524335698, -4.483927247898792601, 48.95942372801902565 ) ) ;
#43931=DIRECTION ( 'NONE',  ( 0.000000000000000000, 0.000000000000000000, 1.000000000000000000 ) ) ;
#43932=CARTESIAN_POINT ( 'NONE',  ( -0.05219959533936034679, 19.03943276465977164, 42.50109039468566152 ) ) ;
#43934=CARTESIAN_POINT ( 'NONE',  ( 13.97604488694527802, 13.89961937509977652, 89.37390960531436690 ) ) ;
#43935=CARTESIAN_POINT ( 'NONE',  ( -19.03943276465977164, 0.05219959533909376836, 26.24890960531435624 ) ) ;
#43936=CARTESIAN_POINT ( 'NONE',  ( -19.05341960407611168, -5.049401038298163336, 71.45724293864766707 ) ) ;
#43937=DIRECTION ( 'NONE',  ( 0.000000000000000000, 0.000000000000000000, -1.000000000000000000 ) ) ;
#43938=CARTESIAN_POINT ( 'NONE',  ( -10.72451020669870658, -18.67979575497194134, 74.58442372801901854 ) ) ;
#43939=CARTESIAN_POINT ( 'NONE',  ( 9.474510206698971260, -16.51473224551069308, 92.91557627198103830 ) ) ;
#43940=CARTESIAN_POINT ( 'NONE',  ( 13.89961937509957401, 13.97604488694547697, 31.87609039468566863 ) ) ;
#43941=CARTESIAN_POINT ( 'NONE',  ( 5.153800228976615827, -19.02544592524334988, 30.20942372801900433 ) ) ;
#43942=CARTESIAN_POINT ( 'NONE',  ( -19.03943276465977164, 0.05219959533909376836, 61.24890960531436690 ) ) ;
#43943=CARTESIAN_POINT ( 'NONE',  ( 21.55341960407610458, 5.719274019375980345, 28.95724293864769905 ) ) ;
#43944=CARTESIAN_POINT ( 'NONE',  ( 21.53943276465977519, 0.05219959533937863772, 81.25109039468568994 ) ) ;
#43945=CARTESIAN_POINT ( 'NONE',  ( 13.97604488694527802, 13.89961937509977652, 59.37390960531434558 ) ) ;
#43946=CARTESIAN_POINT ( 'NONE',  ( -18.62759615963255300, -10.81492255796106328, 84.16775706135234714 ) ) ;
#43947=CARTESIAN_POINT ( 'NONE',  ( 21.55341960407610458, 5.719274019375980345, 33.95724293864769550 ) ) ;
#43948=CARTESIAN_POINT ( 'NONE',  ( -19.05341960407611168, -5.049401038298163336, 76.45724293864769550 ) ) ;
#43949=CARTESIAN_POINT ( 'NONE',  ( -10.72451020669870658, -18.67979575497194134, 39.58442372801901143 ) ) ;
#43950=CARTESIAN_POINT ( 'NONE',  ( 16.51473224551083163, -9.474510206698727899, 65.83442372801900433 ) ) ;
#43951=CARTESIAN_POINT ( 'NONE',  ( -0.05219959533909027116, -19.03943276465977164, 42.49890960531435269 ) ) ;
#43952=CARTESIAN_POINT ( 'NONE',  ( 13.97604488694527802, 13.89961937509977652, 89.37390960531436690 ) ) ;
#43953=CARTESIAN_POINT ( 'NONE',  ( 14.34966873604972726, -8.224510206698740333, 25.83442372801901499 ) ) ;
#43954=CARTESIAN_POINT ( 'NONE',  ( 12.06949235617757843, -12.14591786802309237, 83.12390960531436690 ) ) ;
#43955=CARTESIAN_POINT ( 'NONE',  ( 0.05219959533909260263, 19.03943276465977164, 54.99890960531435979 ) ) ;
#43956=CARTESIAN_POINT ( 'NONE',  ( -10.72451020669898014, 18.67979575497178502, 55.41557627198102409 ) ) ;
#43957=CARTESIAN_POINT ( 'NONE',  ( 0.05219959533934541429, -16.53943276465976808, 20.00109039468568639 ) ) ;
#43958=CARTESIAN_POINT ( 'NONE',  ( 18.67979575497194134, -10.72451020669871369, 20.83442372801901143 ) ) ;
#43959=CARTESIAN_POINT ( 'NONE',  ( -0.05219959533937732626, 21.53943276465977519, 67.50109039468568994 ) ) ;
#43960=CARTESIAN_POINT ( 'NONE',  ( -12.06949235617739369, -12.14591786802326823, 69.37609039468567573 ) ) ;
#43961=CARTESIAN_POINT ( 'NONE',  ( 14.34966873604972726, -8.224510206698740333, 70.83442372801901854 ) ) ;
#43962=CARTESIAN_POINT ( 'NONE',  ( -9.474510206698964154, 16.51473224551069663, 65.41557627198102409 ) ) ;
#43963=CARTESIAN_POINT ( 'NONE',  ( 8.314922557961029526, -14.29746914071037800, 95.41775706135234714 ) ) ;
#43964=CARTESIAN_POINT ( 'NONE',  ( -19.05341960407617563, 5.049401038297882671, 48.54275706135233293 ) ) ;
#43965=CARTESIAN_POINT ( 'NONE',  ( 10.81492255796078972, 18.62759615963270932, 109.5822429386476955 ) ) ;
#43966=CARTESIAN_POINT ( 'NONE',  ( 4.483927247898545687, 16.52544592524342804, 59.79057627198103120 ) ) ;
#43967=CARTESIAN_POINT ( 'NONE',  ( -16.46253265017160317, 9.564922557960807481, 85.83224293864769550 ) ) ;
#43968=CARTESIAN_POINT ( 'NONE',  ( -16.55341960407617563, 4.379528057220093196, 88.54275706135236135 ) ) ;
#43969=CARTESIAN_POINT ( 'NONE',  ( 5.719274019375673035, 21.55341960407619339, 52.29275706135236135 ) ) ;
#43970=CARTESIAN_POINT ( 'NONE',  ( 4.483927247898790824, -16.52544592524335698, 35.20942372801901854 ) ) ;
#43971=CARTESIAN_POINT ( 'NONE',  ( 21.53943276465977519, 0.05219959533937863772, 26.25109039468567573 ) ) ;
#43972=CARTESIAN_POINT ( 'NONE',  ( 14.34966873604960469, 8.224510206698951720, 64.16557627198102409 ) ) ;
#43974=CARTESIAN_POINT ( 'NONE',  ( -21.53943276465977519, 0.05219959533907696930, 96.24890960531435269 ) ) ;
#43975=CARTESIAN_POINT ( 'NONE',  ( 16.53943276465976808, -0.05219959533910856209, 33.74890960531436690 ) ) ;
#43978=CARTESIAN_POINT ( 'NONE',  ( -15.80617190586745835, -15.72974639402198527, 26.87390960531435979 ) ) ;
#43979=CARTESIAN_POINT ( 'NONE',  ( 18.67979575497194134, -10.72451020669871369, 40.83442372801901854 ) ) ;
#43980=CARTESIAN_POINT ( 'NONE',  ( 4.379528057220339221, -16.55341960407611168, 67.70724293864769550 ) ) ;
#43982=CARTESIAN_POINT ( 'NONE',  ( -16.46253265017160317, 9.564922557960807481, 80.83224293864769550 ) ) ;
#43983=CARTESIAN_POINT ( 'NONE',  ( -13.97604488694527625, -13.89961937509977652, 26.87390960531434558 ) ) ;
#43984=CARTESIAN_POINT ( 'NONE',  ( 16.51473224551083163, -9.474510206698727899, 70.83442372801900433 ) ) ;
#43985=CARTESIAN_POINT ( 'NONE',  ( 5.823673210054125526, 21.52544592524343514, 44.79057627198103120 ) ) ;
#43987=CARTESIAN_POINT ( 'NONE',  ( -16.46253265017160317, 9.564922557960807481, 60.83224293864769550 ) ) ;
#43988=CARTESIAN_POINT ( 'NONE',  ( 16.55341960407618274, -4.379528057220086978, 31.04275706135234714 ) ) ;
#43989=CARTESIAN_POINT ( 'NONE',  ( -5.719274019375978568, 21.55341960407610458, 115.2072429386476955 ) ) ;
#43990=CARTESIAN_POINT ( 'NONE',  ( 8.314922557960818139, 14.29746914071049879, 49.58224293864769550 ) ) ;
#43992=CARTESIAN_POINT ( 'NONE',  ( -19.02544592524342804, 5.153800228976336051, 86.04057627198103830 ) ) ;
#43993=CARTESIAN_POINT ( 'NONE',  ( 21.52544592524344225, -5.823673210054117533, 68.54057627198103830 ) ) ;
#43994=CARTESIAN_POINT ( 'NONE',  ( -21.55341960407610458, -5.719274019375992779, 106.4572429386477097 ) ) ;
#43995=CARTESIAN_POINT ( 'NONE',  ( 8.224510206698742110, 14.34966873604972548, 32.08442372801901854 ) ) ;
#43997=CARTESIAN_POINT ( 'NONE',  ( 5.719274019375991003, -21.55341960407610458, 42.70724293864770260 ) ) ;
#43998=CARTESIAN_POINT ( 'NONE',  ( -0.05219959533937732626, 21.53943276465977519, 102.5010903946856899 ) ) ;
#43999=CARTESIAN_POINT ( 'NONE',  ( 5.153800228976335163, 19.02544592524342804, 99.79057627198102409 ) ) ;
#44001=CARTESIAN_POINT ( 'NONE',  ( 19.05341960407611168, 5.049401038298154454, 38.95724293864767418 ) ) ;
#44002=CARTESIAN_POINT ( 'NONE',  ( 19.02544592524343514, -5.153800228976328945, 93.54057627198102409 ) ) ;
#44003=CARTESIAN_POINT ( 'NONE',  ( 0.05219959533909260263, 19.03943276465977164, 74.99890960531435269 ) ) ;
#44005=CARTESIAN_POINT ( 'NONE',  ( 13.89961937509957401, 13.97604488694547697, 56.87609039468564731 ) ) ;
#44006=CARTESIAN_POINT ( 'NONE',  ( -10.72451020669870658, -18.67979575497194134, 109.5844237280190328 ) ) ;
#44007=CARTESIAN_POINT ( 'NONE',  ( -5.719274019375978568, 21.55341960407610458, 35.20724293864768839 ) ) ;
#44008=CARTESIAN_POINT ( 'NONE',  ( -14.34966873604972548, 8.224510206698743886, 108.3344237280190185 ) ) ;
#44009=EDGE_CURVE ( 'NONE', #194071, #21815, #45609, .T. ) ;
#44010=CARTESIAN_POINT ( 'NONE',  ( -9.474510206698720793, -16.51473224551083518, 84.58442372801900433 ) ) ;
#44011=CARTESIAN_POINT ( 'NONE',  ( -16.18388926212240975, 7.379444403734375157, 59.56046848633847191 ) ) ;
#44012=CARTESIAN_POINT ( 'NONE',  ( 13.89961937509957401, 13.97604488694547697, 81.87609039468564731 ) ) ;
#44013=CARTESIAN_POINT ( 'NONE',  ( 19.02544592524334988, 5.153800228976608722, 26.45942372801899722 ) ) ;
#44015=CARTESIAN_POINT ( 'NONE',  ( -9.564922557960796823, -16.46253265017161027, 37.08224293864768839 ) ) ;
#44016=CARTESIAN_POINT ( 'NONE',  ( 8.314922557960818139, 14.29746914071049879, 49.58224293864769550 ) ) ;
#44017=CARTESIAN_POINT ( 'NONE',  ( -17.48853670773245028, -5.747243402303093163, 111.3332870025001000 ) ) ;
#44018=CARTESIAN_POINT ( 'NONE',  ( -16.53943276465976808, 0.05219959533911058130, 26.24890960531435624 ) ) ;
#44020=CARTESIAN_POINT ( 'NONE',  ( -12.06949235617739369, -12.14591786802326823, 89.37609039468568994 ) ) ;
#44021=CARTESIAN_POINT ( 'NONE',  ( -19.02544592524342804, 5.153800228976336051, 46.04057627198101699 ) ) ;
#44022=CARTESIAN_POINT ( 'NONE',  ( -21.55341960407619339, 5.719274019375674811, 113.5427570613523756 ) ) ;
#44023=CARTESIAN_POINT ( 'NONE',  ( 9.474510206698729675, 16.51473224551082808, 112.0844237280190043 ) ) ;
#44024=CARTESIAN_POINT ( 'NONE',  ( -21.55341960407619339, 5.719274019375674811, 93.54275706135234714 ) ) ;
#44026=CARTESIAN_POINT ( 'NONE',  ( -19.03943276465977164, 0.05219959533909376836, 96.24890960531436690 ) ) ;
#44027=CARTESIAN_POINT ( 'NONE',  ( -16.46253265017160317, 9.564922557960807481, 80.83224293864769550 ) ) ;
#44029=CARTESIAN_POINT ( 'NONE',  ( 21.52544592524344225, -5.823673210054117533, 108.5405762719810241 ) ) ;
#44031=CARTESIAN_POINT ( 'NONE',  ( -14.29746914071049879, 8.314922557960819915, 80.83224293864769550 ) ) ;
#44032=CARTESIAN_POINT ( 'NONE',  ( 15.72974639402199770, -15.80617190586745480, 73.12390960531436690 ) ) ;
#44033=CARTESIAN_POINT ( 'NONE',  ( -5.049401038298153566, 19.05341960407611168, 60.20724293864768129 ) ) ;
#44034=CARTESIAN_POINT ( 'NONE',  ( -0.05219959533907301413, -21.53943276465977519, 102.4989096053143811 ) ) ;
#44035=CARTESIAN_POINT ( 'NONE',  ( 8.314922557961029526, -14.29746914071037800, 90.41775706135236135 ) ) ;
#44037=CARTESIAN_POINT ( 'NONE',  ( -19.02544592524342804, 5.153800228976336051, 66.04057627198103830 ) ) ;
#44039=CARTESIAN_POINT ( 'NONE',  ( -16.53943276465976808, 0.05219959533911058130, 91.24890960531436690 ) ) ;
#44041=CARTESIAN_POINT ( 'NONE',  ( -5.153800228976328057, -19.02544592524343514, 62.29057627198100988 ) ) ;
#44042=CARTESIAN_POINT ( 'NONE',  ( -16.51473224551082808, 9.474510206698731452, 73.33442372801900433 ) ) ;
#44043=CARTESIAN_POINT ( 'NONE',  ( -14.34966873604960291, -8.224510206698953496, 81.66557627198103830 ) ) ;
#44044=CARTESIAN_POINT ( 'NONE',  ( 18.67979575497194134, -10.72451020669871369, 55.83442372801901854 ) ) ;
#44045=CARTESIAN_POINT ( 'NONE',  ( 16.46253265017160672, -9.564922557960803928, 43.33224293864769550 ) ) ;
#44046=CARTESIAN_POINT ( 'NONE',  ( 0.05219959533937995610, -21.53943276465977519, 20.00109039468568639 ) ) ;
#44047=CARTESIAN_POINT ( 'NONE',  ( -4.483927247898539470, -16.52544592524342804, 107.2905762719810525 ) ) ;
#44049=CARTESIAN_POINT ( 'NONE',  ( -19.05341960407611168, -5.049401038298163336, 56.45724293864768129 ) ) ;
#44051=CARTESIAN_POINT ( 'NONE',  ( 0.05219959533936267826, -19.03943276465977164, 95.00109039468567573 ) ) ;
#44052=CARTESIAN_POINT ( 'NONE',  ( 5.153800228976335163, 19.02544592524342804, 109.7905762719810099 ) ) ;
#44053=CARTESIAN_POINT ( 'NONE',  ( -15.80617190586768217, 15.72974639402176855, 53.12609039468568284 ) ) ;
#44054=CARTESIAN_POINT ( 'NONE',  ( 19.03943276465977164, -0.05219959533909143690, 88.74890960531436690 ) ) ;
#44055=CARTESIAN_POINT ( 'NONE',  ( -9.474510206698720793, -16.51473224551083518, 79.58442372801899012 ) ) ;
#44056=CARTESIAN_POINT ( 'NONE',  ( 16.51473224551069308, 9.474510206698969483, 54.16557627198103120 ) ) ;
#44057=CARTESIAN_POINT ( 'NONE',  ( -16.52544592524342804, 4.483927247898546575, 71.04057627198103830 ) ) ;
#44058=CARTESIAN_POINT ( 'NONE',  ( -12.06949235617756955, 12.14591786802309770, 75.62390960531439532 ) ) ;
#44059=CARTESIAN_POINT ( 'NONE',  ( -16.51473224551069308, -9.474510206698971260, 86.66557627198102409 ) ) ;
#44060=CARTESIAN_POINT ( 'NONE',  ( 12.14591786802309770, 12.06949235617756955, 79.37390960531436690 ) ) ;
#44061=CARTESIAN_POINT ( 'NONE',  ( -13.89961937509977652, 13.97604488694528158, 90.62390960531432427 ) ) ;
#44062=CARTESIAN_POINT ( 'NONE',  ( -9.564922557961040184, 16.46253265017147172, 37.91775706135233293 ) ) ;
#44063=CARTESIAN_POINT ( 'NONE',  ( -13.97604488694527625, -13.89961937509977652, 51.87390960531436690 ) ) ;
#44064=CARTESIAN_POINT ( 'NONE',  ( -14.29746914071049879, 8.314922557960819915, 25.83224293864769194 ) ) ;
#44065=CARTESIAN_POINT ( 'NONE',  ( -9.564922557960796823, -16.46253265017161027, 27.08224293864769550 ) ) ;
#44067=CARTESIAN_POINT ( 'NONE',  ( -5.823673210054431948, 21.52544592524334988, 47.70942372801902565 ) ) ;
#44068=CARTESIAN_POINT ( 'NONE',  ( 13.97604488694548053, -13.89961937509957401, 70.62609039468567573 ) ) ;
#44069=CARTESIAN_POINT ( 'NONE',  ( -12.14591786802309592, -12.06949235617757132, 41.87390960531435979 ) ) ;
#44070=CARTESIAN_POINT ( 'NONE',  ( 18.62759615963271287, -10.81492255796078972, 83.33224293864769550 ) ) ;
#44071=CARTESIAN_POINT ( 'NONE',  ( 0.05219959533909260263, 19.03943276465977164, 114.9989096053143669 ) ) ;
#44073=CARTESIAN_POINT ( 'NONE',  ( -4.379528057220328563, 16.55341960407611168, 70.20724293864769550 ) ) ;
#44074=CARTESIAN_POINT ( 'NONE',  ( -19.02544592524342804, 5.153800228976336051, 46.04057627198101699 ) ) ;
#44075=CARTESIAN_POINT ( 'NONE',  ( 16.46253265017146816, 9.564922557961045513, 36.66775706135233293 ) ) ;
#44076=CARTESIAN_POINT ( 'NONE',  ( 8.224510206698742110, 14.34966873604972548, 107.0844237280190043 ) ) ;
#44077=CARTESIAN_POINT ( 'NONE',  ( -12.14591786802326823, 12.06949235617739902, 63.12609039468568994 ) ) ;
#44078=CARTESIAN_POINT ( 'NONE',  ( 15.72974639402199770, -15.80617190586745480, 43.12390960531435269 ) ) ;
#44079=CARTESIAN_POINT ( 'NONE',  ( -19.02544592524334988, -5.153800228976617603, 18.95942372801899722 ) ) ;
#44080=CARTESIAN_POINT ( 'NONE',  ( -0.05219959533909027116, -19.03943276465977164, 97.49890960531436690 ) ) ;
#44082=CARTESIAN_POINT ( 'NONE',  ( -0.05219959533934338120, 16.53943276465976808, 72.50109039468568994 ) ) ;
#44083=CARTESIAN_POINT ( 'NONE',  ( 8.314922557960818139, 14.29746914071049879, 114.5822429386477097 ) ) ;
#44084=CARTESIAN_POINT ( 'NONE',  ( -12.06949235617756955, 12.14591786802309770, 30.62390960531436335 ) ) ;
#44085=CARTESIAN_POINT ( 'NONE',  ( 19.05341960407611168, 5.049401038298154454, 98.95724293864766707 ) ) ;
#44086=CARTESIAN_POINT ( 'NONE',  ( -13.97604488694527625, -13.89961937509977652, 86.87390960531436690 ) ) ;
#44087=CARTESIAN_POINT ( 'NONE',  ( -21.55341960407610458, -5.719274019375992779, 31.45724293864769550 ) ) ;
#44088=CARTESIAN_POINT ( 'NONE',  ( -12.14591786802309592, -12.06949235617757132, 71.87390960531438111 ) ) ;
#44089=B_SPLINE_CURVE_WITH_KNOTS ( 'NONE', 3,
 ( #64606, #187966, #110110, #112097, #138454, #63610 ),
 .UNSPECIFIED., .F., .F.,
 ( 4, 2, 4 ),
 ( 0.007228050697041590866, 0.007608510107495068155, 0.007988969517948545443 ),
 .UNSPECIFIED. ) ;
#44090=CARTESIAN_POINT ( 'NONE',  ( -8.224510206698948167, 14.34966873604960824, 50.41557627198103120 ) ) ;
#44091=CARTESIAN_POINT ( 'NONE',  ( 14.29746914071037800, 8.314922557961029526, 56.66775706135235424 ) ) ;
#44092=CARTESIAN_POINT ( 'NONE',  ( -17.60779699588839264, -5.500000000000014211, 56.34981316670103979 ) ) ;
#44093=CARTESIAN_POINT ( 'NONE',  ( 13.97604488694548053, -13.89961937509957401, 55.62609039468566863 ) ) ;
#44094=CARTESIAN_POINT ( 'NONE',  ( -5.153800228976328057, -19.02544592524343514, 92.29057627198099567 ) ) ;
#44095=CARTESIAN_POINT ( 'NONE',  ( -9.564922557961040184, 16.46253265017147172, 67.91775706135233293 ) ) ;
#44097=CARTESIAN_POINT ( 'NONE',  ( -19.05341960407617563, 5.049401038297882671, 53.54275706135231871 ) ) ;
#44098=CARTESIAN_POINT ( 'NONE',  ( -16.46253265017146816, -9.564922557961047289, 99.16775706135233293 ) ) ;
#44099=CARTESIAN_POINT ( 'NONE',  ( -8.224510206698735004, -14.34966873604973081, 94.58442372801901854 ) ) ;
#44101=CARTESIAN_POINT ( 'NONE',  ( -16.51473224551069308, -9.474510206698971260, 41.66557627198103120 ) ) ;
#44102=CARTESIAN_POINT ( 'NONE',  ( -19.02544592524342804, 5.153800228976336051, 111.0405762719810099 ) ) ;
#44103=CARTESIAN_POINT ( 'NONE',  ( -21.52544592524334988, -5.823673210054445271, 53.95942372801900433 ) ) ;
#44104=CARTESIAN_POINT ( 'NONE',  ( 9.474510206698729675, 16.51473224551082808, 97.08442372801900433 ) ) ;
#44106=CARTESIAN_POINT ( 'NONE',  ( -13.89961937509977652, 13.97604488694528158, 60.62390960531436690 ) ) ;
#44108=CARTESIAN_POINT ( 'NONE',  ( 12.14591786802309770, 12.06949235617756955, 74.37390960531436690 ) ) ;
#44109=CARTESIAN_POINT ( 'NONE',  ( 19.03943276465977164, -0.05219959533909143690, 68.74890960531436690 ) ) ;
#44110=CARTESIAN_POINT ( 'NONE',  ( -19.02544592524342804, 5.153800228976336051, 81.04057627198103830 ) ) ;
#44111=CARTESIAN_POINT ( 'NONE',  ( -5.153800228976607833, 19.02544592524334988, 82.70942372801897591 ) ) ;
#44112=CARTESIAN_POINT ( 'NONE',  ( -21.52544592524343514, 5.823673210054127303, 66.04057627198103830 ) ) ;
#44113=CARTESIAN_POINT ( 'NONE',  ( 16.55341960407611168, 4.379528057220329451, 113.9572429386477239 ) ) ;
#44114=CARTESIAN_POINT ( 'NONE',  ( 19.05341960407617918, -5.049401038297876454, 41.04275706135233293 ) ) ;
#44115=CARTESIAN_POINT ( 'NONE',  ( -16.46253265017160317, 9.564922557960807481, 80.83224293864769550 ) ) ;
#44116=CARTESIAN_POINT ( 'NONE',  ( 15.72974639402199770, -15.80617190586745480, 88.12390960531436690 ) ) ;
#44117=CARTESIAN_POINT ( 'NONE',  ( -12.14591786802309592, -12.06949235617757132, 76.87390960531439532 ) ) ;
#44118=CARTESIAN_POINT ( 'NONE',  ( -5.049401038297874678, -19.05341960407617918, 44.79275706135232582 ) ) ;
#44119=CARTESIAN_POINT ( 'NONE',  ( -5.823673210054116645, -21.52544592524344225, 77.29057627198102409 ) ) ;
#44120=CARTESIAN_POINT ( 'NONE',  ( 18.67979575497178502, 10.72451020669898547, 64.16557627198102409 ) ) ;
#44121=CARTESIAN_POINT ( 'NONE',  ( -18.62759615963270932, 10.81492255796079327, 40.83224293864769550 ) ) ;
#44122=CARTESIAN_POINT ( 'NONE',  ( -21.53943276465977519, -0.05219959533937600094, 93.75109039468567573 ) ) ;
#44123=CARTESIAN_POINT ( 'NONE',  ( 13.97604488694527802, 13.89961937509977652, 84.37390960531433848 ) ) ;
#44124=CARTESIAN_POINT ( 'NONE',  ( -19.03943276465977164, 0.05219959533909376836, 21.24890960531436335 ) ) ;
#44125=CARTESIAN_POINT ( 'NONE',  ( 0.05219959533937995610, -21.53943276465977519, 30.00109039468568284 ) ) ;
#44127=CARTESIAN_POINT ( 'NONE',  ( 10.72451020669871369, 18.67979575497193778, 42.08442372801901854 ) ) ;
#44128=CARTESIAN_POINT ( 'NONE',  ( 16.46253265017160672, -9.564922557960803928, 53.33224293864768839 ) ) ;
#44129=CARTESIAN_POINT ( 'NONE',  ( -15.72974639402176322, -15.80617190586768395, 24.37609039468567573 ) ) ;
#44130=CARTESIAN_POINT ( 'NONE',  ( 16.46253265017146816, 9.564922557961045513, 61.66775706135234003 ) ) ;
#44131=CARTESIAN_POINT ( 'NONE',  ( -16.46253265017160317, 9.564922557960807481, 35.83224293864768839 ) ) ;
#44132=CARTESIAN_POINT ( 'NONE',  ( -4.379528057220086978, -16.55341960407618274, 24.79275706135235779 ) ) ;
#44133=CARTESIAN_POINT ( 'NONE',  ( 0.05219959533909260263, 19.03943276465977164, 29.99890960531435979 ) ) ;
#44134=CARTESIAN_POINT ( 'NONE',  ( 4.379528057220092307, 16.55341960407617563, 57.29275706135234714 ) ) ;
#44135=CARTESIAN_POINT ( 'NONE',  ( 9.474510206698971260, -16.51473224551069308, 37.91557627198102409 ) ) ;
#44137=CARTESIAN_POINT ( 'NONE',  ( -19.03943276465977164, 0.05219959533909376836, 91.24890960531436690 ) ) ;
#44138=CARTESIAN_POINT ( 'NONE',  ( -9.564922557960796823, -16.46253265017161027, 22.08224293864768839 ) ) ;
#44139=CARTESIAN_POINT ( 'NONE',  ( -15.80617190586745835, -15.72974639402198527, 56.87390960531436690 ) ) ;
#44140=CARTESIAN_POINT ( 'NONE',  ( -8.224510206698735004, -14.34966873604973081, 49.58442372801901143 ) ) ;
#44141=CARTESIAN_POINT ( 'NONE',  ( 0.05219959533937995610, -21.53943276465977519, 100.0010903946857042 ) ) ;
#44142=CARTESIAN_POINT ( 'NONE',  ( -0.05219959533909027116, -19.03943276465977164, 37.49890960531436690 ) ) ;
#44143=CARTESIAN_POINT ( 'NONE',  ( 8.314922557960818139, 14.29746914071049879, 29.58224293864769905 ) ) ;
#44144=CARTESIAN_POINT ( 'NONE',  ( -4.483927247898539470, -16.52544592524342804, 62.29057627198102409 ) ) ;
#44145=CARTESIAN_POINT ( 'NONE',  ( 9.474510206698971260, -16.51473224551069308, 67.91557627198102409 ) ) ;
#44146=CARTESIAN_POINT ( 'NONE',  ( -5.719274019375665041, -21.55341960407619695, 109.7927570613523613 ) ) ;
#44147=CARTESIAN_POINT ( 'NONE',  ( -10.72451020669870658, -18.67979575497194134, 29.58442372801901854 ) ) ;
#44148=CARTESIAN_POINT ( 'NONE',  ( -15.80617190586768217, 15.72974639402176855, 83.12609039468568994 ) ) ;
#44149=CARTESIAN_POINT ( 'NONE',  ( 14.34966873604972726, -8.224510206698740333, 50.83442372801901143 ) ) ;
#44150=CARTESIAN_POINT ( 'NONE',  ( 4.483927247898790824, -16.52544592524335698, 35.20942372801901854 ) ) ;
#44151=CARTESIAN_POINT ( 'NONE',  ( 8.224510206698953496, -14.34966873604960469, 92.91557627198103830 ) ) ;
#44152=CARTESIAN_POINT ( 'NONE',  ( -10.81492255796105439, 18.62759615963255655, 97.91775706135236135 ) ) ;
#44153=CARTESIAN_POINT ( 'NONE',  ( 12.06949235617757843, -12.14591786802309237, 38.12390960531436690 ) ) ;
#44154=CARTESIAN_POINT ( 'NONE',  ( 13.89961937509977652, -13.97604488694527269, 23.12390960531436335 ) ) ;
#44155=CARTESIAN_POINT ( 'NONE',  ( -8.224510206698735004, -14.34966873604973081, 39.58442372801901143 ) ) ;
#44156=CARTESIAN_POINT ( 'NONE',  ( 12.14591786802309770, 12.06949235617756955, 59.37390960531436690 ) ) ;
#44157=CARTESIAN_POINT ( 'NONE',  ( 8.314922557961029526, -14.29746914071037800, 105.4177570613523613 ) ) ;
#44158=CARTESIAN_POINT ( 'NONE',  ( -19.03943276465977164, 0.05219959533909376836, 101.2489096053143669 ) ) ;
#44159=CARTESIAN_POINT ( 'NONE',  ( -5.153800228976328057, -19.02544592524343514, 107.2905762719810383 ) ) ;
#44160=CARTESIAN_POINT ( 'NONE',  ( -21.55341960407619339, 5.719274019375674811, 108.5427570613523756 ) ) ;
#44162=CARTESIAN_POINT ( 'NONE',  ( 8.314922557960818139, 14.29746914071049879, 89.58224293864768129 ) ) ;
#44163=CARTESIAN_POINT ( 'NONE',  ( -19.05341960407611168, -5.049401038298163336, 96.45724293864769550 ) ) ;
#44164=VERTEX_POINT ( 'NONE', #192878 ) ;
#44165=CARTESIAN_POINT ( 'NONE',  ( -12.14591786802326823, 12.06949235617739902, 38.12609039468567573 ) ) ;
#44166=CARTESIAN_POINT ( 'NONE',  ( -0.05219959533909027116, -19.03943276465977164, 42.49890960531435269 ) ) ;
#44167=CARTESIAN_POINT ( 'NONE',  ( 19.03943276465977164, -0.05219959533909143690, 103.7489096053143669 ) ) ;
#44168=CARTESIAN_POINT ( 'NONE',  ( -0.05219959533934338120, 16.53943276465976808, 42.50109039468567573 ) ) ;
#44170=CARTESIAN_POINT ( 'NONE',  ( 19.05341960407617918, -5.049401038297876454, 46.04275706135233293 ) ) ;
#44171=CARTESIAN_POINT ( 'NONE',  ( -16.51473224551069308, -9.474510206698971260, 41.66557627198103120 ) ) ;
#44172=CARTESIAN_POINT ( 'NONE',  ( -4.483927247898782831, 16.52544592524335698, 77.70942372801900433 ) ) ;
#44173=CARTESIAN_POINT ( 'NONE',  ( -16.46253265017146816, -9.564922557961047289, 89.16775706135234714 ) ) ;
#44174=CARTESIAN_POINT ( 'NONE',  ( 5.049401038297881783, 19.05341960407617563, 27.29275706135232937 ) ) ;
#44175=CARTESIAN_POINT ( 'NONE',  ( 0.05219959533909260263, 19.03943276465977164, 64.99890960531436690 ) ) ;
#44176=CARTESIAN_POINT ( 'NONE',  ( -12.06949235617756955, 12.14591786802309770, 100.6239096053143811 ) ) ;
#44178=CARTESIAN_POINT ( 'NONE',  ( 9.474510206698729675, 16.51473224551082808, 67.08442372801900433 ) ) ;
#44179=CARTESIAN_POINT ( 'NONE',  ( 5.823673210054125526, 21.52544592524343514, 59.79057627198103120 ) ) ;
#44180=CARTESIAN_POINT ( 'NONE',  ( 16.46253265017146816, 9.564922557961045513, 31.66775706135232937 ) ) ;
#44181=CARTESIAN_POINT ( 'NONE',  ( 16.46253265017160672, -9.564922557960803928, 108.3322429386476955 ) ) ;
#44182=CARTESIAN_POINT ( 'NONE',  ( 5.719274019375991003, -21.55341960407610458, 72.70724293864769550 ) ) ;
#44183=CARTESIAN_POINT ( 'NONE',  ( -17.48853670773246805, 5.747243402303039872, 83.66671299749991420 ) ) ;
#44184=CARTESIAN_POINT ( 'NONE',  ( -9.564922557961040184, 16.46253265017147172, 107.9177570613523471 ) ) ;
#44186=CARTESIAN_POINT ( 'NONE',  ( -16.52544592524335698, -4.483927247898792601, 28.95942372801902209 ) ) ;
#44187=CARTESIAN_POINT ( 'NONE',  ( 13.89961937509977652, -13.97604488694527269, 33.12390960531434558 ) ) ;
#44188=CARTESIAN_POINT ( 'NONE',  ( 19.02544592524343514, -5.153800228976328945, 113.5405762719810241 ) ) ;
#44189=CARTESIAN_POINT ( 'NONE',  ( 15.80617190586746368, 15.72974639402197994, 94.37390960531436690 ) ) ;
#44190=CARTESIAN_POINT ( 'NONE',  ( 21.52544592524334988, 5.823673210054432836, 61.45942372801901854 ) ) ;
#44191=CARTESIAN_POINT ( 'NONE',  ( -19.02544592524334988, -5.153800228976617603, 103.9594237280190043 ) ) ;
#44192=CARTESIAN_POINT ( 'NONE',  ( 15.80617190586769283, -15.72974639402175789, 105.6260903946856899 ) ) ;
#44193=CARTESIAN_POINT ( 'NONE',  ( -16.55341960407617563, 4.379528057220093196, 113.5427570613523756 ) ) ;
#44194=CARTESIAN_POINT ( 'NONE',  ( 21.52544592524344225, -5.823673210054117533, 103.5405762719810383 ) ) ;
#44195=CARTESIAN_POINT ( 'NONE',  ( 4.483927247898545687, 16.52544592524342804, 54.79057627198104541 ) ) ;
#44196=CARTESIAN_POINT ( 'NONE',  ( -19.03943276465977164, -0.05219959533935918106, 83.75109039468567573 ) ) ;
#44197=CARTESIAN_POINT ( 'NONE',  ( -19.03943276465977164, -0.05219959533935918106, 58.75109039468566863 ) ) ;
#44198=CARTESIAN_POINT ( 'NONE',  ( 5.719274019375673035, 21.55341960407619339, 62.29275706135236845 ) ) ;
#44199=CARTESIAN_POINT ( 'NONE',  ( -19.05341960407617563, 5.049401038297882671, 38.54275706135233293 ) ) ;
#44200=CARTESIAN_POINT ( 'NONE',  ( 4.483927247898545687, 16.52544592524342804, 99.79057627198103830 ) ) ;
#44201=CARTESIAN_POINT ( 'NONE',  ( -15.72974639402197994, 15.80617190586746368, 35.62390960531437401 ) ) ;
#44202=CARTESIAN_POINT ( 'NONE',  ( 16.55341960407611168, 4.379528057220329451, 33.95724293864769550 ) ) ;
#44203=CARTESIAN_POINT ( 'NONE',  ( -21.52544592524334988, -5.823673210054445271, 93.95942372801903275 ) ) ;
#44204=CARTESIAN_POINT ( 'NONE',  ( -8.314922557961024197, 14.29746914071037800, 72.91775706135234714 ) ) ;
#44205=CARTESIAN_POINT ( 'NONE',  ( -12.06949235617756955, 12.14591786802309770, 30.62390960531436335 ) ) ;
#44206=CARTESIAN_POINT ( 'NONE',  ( 0.05219959533937995610, -21.53943276465977519, 60.00109039468568284 ) ) ;
#44207=CARTESIAN_POINT ( 'NONE',  ( -15.80617190586768217, 15.72974639402176855, 73.12609039468567573 ) ) ;
#44208=CARTESIAN_POINT ( 'NONE',  ( -0.05219959533907301413, -21.53943276465977519, 67.49890960531436690 ) ) ;
#44210=CARTESIAN_POINT ( 'NONE',  ( 9.564922557960805705, 16.46253265017160317, 24.58224293864769194 ) ) ;
#44211=CARTESIAN_POINT ( 'NONE',  ( 5.823673210054444382, -21.52544592524334988, 45.20942372801901854 ) ) ;
#44212=CARTESIAN_POINT ( 'NONE',  ( -13.97604488694527625, -13.89961937509977652, 21.87390960531435979 ) ) ;
#44213=CARTESIAN_POINT ( 'NONE',  ( -16.51473224551069308, -9.474510206698971260, 36.66557627198102409 ) ) ;
#44214=CARTESIAN_POINT ( 'NONE',  ( -0.05219959533910754901, -16.53943276465976808, 82.49890960531436690 ) ) ;
#44215=CARTESIAN_POINT ( 'NONE',  ( -13.97604488694527625, -13.89961937509977652, 91.87390960531432427 ) ) ;
#44216=CARTESIAN_POINT ( 'NONE',  ( -16.55341960407611168, -4.379528057220339221, 26.45724293864768839 ) ) ;
#44217=CARTESIAN_POINT ( 'NONE',  ( -16.52544592524342804, 4.483927247898546575, 96.04057627198102409 ) ) ;
#44218=CARTESIAN_POINT ( 'NONE',  ( -21.53943276465977519, 0.05219959533907696930, 66.24890960531436690 ) ) ;
#44220=CARTESIAN_POINT ( 'NONE',  ( -10.72451020669898014, 18.67979575497178502, 105.4155762719810383 ) ) ;
#44221=CARTESIAN_POINT ( 'NONE',  ( -19.03943276465977164, 0.05219959533909376836, 111.2489096053143669 ) ) ;
#44222=CARTESIAN_POINT ( 'NONE',  ( -5.153800228976328057, -19.02544592524343514, 62.29057627198100988 ) ) ;
#44223=CARTESIAN_POINT ( 'NONE',  ( -19.05341960407617563, 5.049401038297882671, 108.5427570613523187 ) ) ;
#44224=CARTESIAN_POINT ( 'NONE',  ( -5.823673210054116645, -21.52544592524344225, 62.29057627198102409 ) ) ;
#44225=CARTESIAN_POINT ( 'NONE',  ( -0.05219959533937732626, 21.53943276465977519, 82.50109039468568994 ) ) ;
#44226=B_SPLINE_CURVE_WITH_KNOTS ( 'NONE', 3,
 ( #192591, #131913, #146064, #194594, #7548, #193597, #39893, #101561, #52067, #24754, #148086, #179439, #164262, #175420, #28738, #11586, #184386, #103580, #106538, #119741 ),
 .UNSPECIFIED., .F., .F.,
 ( 4, 2, 2, 2, 2, 2, 2, 2, 2, 4 ),
 ( 0.004000878361811995541, 0.004499404418916006301, 0.004997930476020017061, 0.005496456533124027821, 0.005994982590228037714, 0.006244245618780033119, 0.006493508647332028524, 0.006992034704436018468, 0.007490560761540008411, 0.007989086818643999222 ),
 .UNSPECIFIED. ) ;
#44227=CARTESIAN_POINT ( 'NONE',  ( -13.89961937509977652, 13.97604488694528158, 70.62390960531432427 ) ) ;
#44228=CARTESIAN_POINT ( 'NONE',  ( 16.51473224551069308, 9.474510206698969483, 104.1655762719810241 ) ) ;
#44229=CARTESIAN_POINT ( 'NONE',  ( -8.224510206698735004, -14.34966873604973081, 79.58442372801903275 ) ) ;
#44230=CARTESIAN_POINT ( 'NONE',  ( 21.52544592524334988, 5.823673210054432836, 61.45942372801901854 ) ) ;
#44231=CARTESIAN_POINT ( 'NONE',  ( -18.67979575497193778, 10.72451020669871902, 103.3344237280190043 ) ) ;
#44232=CARTESIAN_POINT ( 'NONE',  ( -15.72974639402197994, 15.80617190586746368, 115.6239096053143669 ) ) ;
#44233=CARTESIAN_POINT ( 'NONE',  ( 5.823673210054125526, 21.52544592524343514, 79.79057627198102409 ) ) ;
#44234=CARTESIAN_POINT ( 'NONE',  ( -9.564922557961040184, 16.46253265017147172, 42.91775706135234003 ) ) ;
#44235=CARTESIAN_POINT ( 'NONE',  ( 5.823673210054125526, 21.52544592524343514, 39.79057627198103830 ) ) ;
#44236=CARTESIAN_POINT ( 'NONE',  ( -16.46253265017160317, 9.564922557960807481, 80.83224293864769550 ) ) ;
#44237=CARTESIAN_POINT ( 'NONE',  ( 14.34966873604960469, 8.224510206698951720, 39.16557627198102409 ) ) ;
#44238=CARTESIAN_POINT ( 'NONE',  ( -16.36317988757060249, 7.306389748694932962, 64.09789608363229263 ) ) ;
#44240=CARTESIAN_POINT ( 'NONE',  ( -16.51473224551082808, 9.474510206698731452, 93.33442372801900433 ) ) ;
#44241=CARTESIAN_POINT ( 'NONE',  ( -21.52544592524343514, 5.823673210054127303, 71.04057627198103830 ) ) ;
#44242=CARTESIAN_POINT ( 'NONE',  ( 4.483927247898545687, 16.52544592524342804, 54.79057627198104541 ) ) ;
#44243=CARTESIAN_POINT ( 'NONE',  ( 16.55341960407618274, -4.379528057220086978, 26.04275706135235779 ) ) ;
#44244=CARTESIAN_POINT ( 'NONE',  ( -9.564922557960796823, -16.46253265017161027, 47.08224293864769550 ) ) ;
#44245=CARTESIAN_POINT ( 'NONE',  ( 15.80617190586746368, 15.72974639402197994, 114.3739096053143527 ) ) ;
#44246=CARTESIAN_POINT ( 'NONE',  ( -5.153800228976607833, 19.02544592524334988, 82.70942372801897591 ) ) ;
#44247=CARTESIAN_POINT ( 'NONE',  ( -19.02544592524342804, 5.153800228976336051, 86.04057627198103830 ) ) ;
#44248=CARTESIAN_POINT ( 'NONE',  ( -16.53943276465976808, 0.05219959533911058130, 86.24890960531436690 ) ) ;
#44249=CARTESIAN_POINT ( 'NONE',  ( -0.05219959533909027116, -19.03943276465977164, 67.49890960531436690 ) ) ;
#44250=CARTESIAN_POINT ( 'NONE',  ( -4.483927247898539470, -16.52544592524342804, 72.29057627198102409 ) ) ;
#44251=CARTESIAN_POINT ( 'NONE',  ( -19.03943276465977164, 0.05219959533909376836, 26.24890960531435624 ) ) ;
#44253=CARTESIAN_POINT ( 'NONE',  ( -4.483927247898539470, -16.52544592524342804, 37.29057627198102409 ) ) ;
#44254=CARTESIAN_POINT ( 'NONE',  ( -19.02544592524342804, 5.153800228976336051, 96.04057627198103830 ) ) ;
#44256=CARTESIAN_POINT ( 'NONE',  ( 19.03943276465977164, 0.05219959533936151252, 51.25109039468567573 ) ) ;
#44257=CARTESIAN_POINT ( 'NONE',  ( 16.52544592524335698, 4.483927247898782831, 66.45942372801903275 ) ) ;
#44258=CARTESIAN_POINT ( 'NONE',  ( 18.62759615963271287, -10.81492255796078972, 78.33224293864770971 ) ) ;
#44259=CARTESIAN_POINT ( 'NONE',  ( 9.474510206698729675, 16.51473224551082808, 37.08442372801899722 ) ) ;
#44260=CARTESIAN_POINT ( 'NONE',  ( 13.97604488694527802, 13.89961937509977652, 89.37390960531436690 ) ) ;
#44261=CARTESIAN_POINT ( 'NONE',  ( -17.50000000000014566, 3.417042746626947736, 115.1738039623247403 ) ) ;
#44262=CARTESIAN_POINT ( 'NONE',  ( 0.05219959533907565091, 21.53943276465977519, 34.99890960531435979 ) ) ;
#44263=CARTESIAN_POINT ( 'NONE',  ( 5.153800228976335163, 19.02544592524342804, 74.79057627198103830 ) ) ;
#44264=CARTESIAN_POINT ( 'NONE',  ( 21.53943276465977519, 0.05219959533937863772, 51.25109039468568994 ) ) ;
#44265=CARTESIAN_POINT ( 'NONE',  ( 0.05219959533910956823, 16.53943276465976808, 114.9989096053143669 ) ) ;
#44266=CARTESIAN_POINT ( 'NONE',  ( -18.67979575497193778, 10.72451020669871902, 23.33442372801901499 ) ) ;
#44267=CARTESIAN_POINT ( 'NONE',  ( 16.51473224551069308, 9.474510206698969483, 99.16557627198102409 ) ) ;
#44269=CARTESIAN_POINT ( 'NONE',  ( -18.67979575497193778, 10.72451020669871902, 38.33442372801900433 ) ) ;
#44271=CARTESIAN_POINT ( 'NONE',  ( 19.05341960407611168, 5.049401038298154454, 93.95724293864769550 ) ) ;
#44273=CARTESIAN_POINT ( 'NONE',  ( 18.62759615963271287, -10.81492255796078972, 108.3322429386477097 ) ) ;
#44274=CARTESIAN_POINT ( 'NONE',  ( 5.049401038298161559, -19.05341960407611168, 47.70724293864770260 ) ) ;
#44275=CARTESIAN_POINT ( 'NONE',  ( -4.379528057220086978, -16.55341960407618274, 24.79275706135235779 ) ) ;
#44277=CARTESIAN_POINT ( 'NONE',  ( -15.72974639402176322, -15.80617190586768395, 99.37609039468568994 ) ) ;
#44278=CARTESIAN_POINT ( 'NONE',  ( 19.02544592524343514, -5.153800228976328945, 28.54057627198102409 ) ) ;
#44279=CARTESIAN_POINT ( 'NONE',  ( -21.53943276465977519, -0.05219959533937600094, 103.7510903946857042 ) ) ;
#44280=CARTESIAN_POINT ( 'NONE',  ( 9.474510206698971260, -16.51473224551069308, 87.91557627198102409 ) ) ;
#44281=CARTESIAN_POINT ( 'NONE',  ( 15.72974639402176855, 15.80617190586768217, 61.87609039468568284 ) ) ;
#44283=CARTESIAN_POINT ( 'NONE',  ( 13.89961937509977652, -13.97604488694527269, 98.12390960531433848 ) ) ;
#44285=CARTESIAN_POINT ( 'NONE',  ( 12.06949235617739724, 12.14591786802326823, 56.87609039468568994 ) ) ;
#44286=CARTESIAN_POINT ( 'NONE',  ( 4.483927247898790824, -16.52544592524335698, 65.20942372801901854 ) ) ;
#44287=CARTESIAN_POINT ( 'NONE',  ( 5.823673210054444382, -21.52544592524334988, 55.20942372801902565 ) ) ;
#44288=CARTESIAN_POINT ( 'NONE',  ( 18.62759615963255655, 10.81492255796105972, 91.66775706135234714 ) ) ;
#44290=CARTESIAN_POINT ( 'NONE',  ( -0.05219959533934338120, 16.53943276465976808, 32.50109039468568284 ) ) ;
#44291=CARTESIAN_POINT ( 'NONE',  ( 19.02544592524343514, -5.153800228976328945, 68.54057627198103830 ) ) ;
#44292=CARTESIAN_POINT ( 'NONE',  ( 9.564922557960805705, 16.46253265017160317, 94.58224293864769550 ) ) ;
#44293=CARTESIAN_POINT ( 'NONE',  ( -16.46253265017160317, 9.564922557960807481, 110.8322429386476955 ) ) ;
#44294=CARTESIAN_POINT ( 'NONE',  ( -0.05219959533909027116, -19.03943276465977164, 27.49890960531435624 ) ) ;
#44295=CARTESIAN_POINT ( 'NONE',  ( 5.823673210054125526, 21.52544592524343514, 34.79057627198103120 ) ) ;
#44296=CARTESIAN_POINT ( 'NONE',  ( 16.53943276465976808, 0.05219959533934440121, 86.25109039468568994 ) ) ;
#44297=CARTESIAN_POINT ( 'NONE',  ( -16.52544592524342804, 4.483927247898546575, 66.04057627198103830 ) ) ;
#44298=CARTESIAN_POINT ( 'NONE',  ( 5.153800228976335163, 19.02544592524342804, 69.79057627198103830 ) ) ;
#44299=CARTESIAN_POINT ( 'NONE',  ( -5.823673210054431948, 21.52544592524334988, 92.70942372801901854 ) ) ;
#44301=CARTESIAN_POINT ( 'NONE',  ( 16.55341960407618274, -4.379528057220086978, 21.04275706135234714 ) ) ;
#44302=CARTESIAN_POINT ( 'NONE',  ( 14.34966873604960469, 8.224510206698951720, 69.16557627198102409 ) ) ;
#44303=CARTESIAN_POINT ( 'NONE',  ( -15.80617190586768217, 15.72974639402176855, 33.12609039468569705 ) ) ;
#44304=CARTESIAN_POINT ( 'NONE',  ( -18.67979575497178146, -10.72451020669898902, 71.66557627198100988 ) ) ;
#44305=CARTESIAN_POINT ( 'NONE',  ( -0.05219959533936034679, 19.03943276465977164, 32.50109039468566863 ) ) ;
#44307=CARTESIAN_POINT ( 'NONE',  ( 19.02544592524343514, -5.153800228976328945, 88.54057627198102409 ) ) ;
#44308=CARTESIAN_POINT ( 'NONE',  ( -16.52544592524342804, 4.483927247898546575, 56.04057627198102409 ) ) ;
#44309=CARTESIAN_POINT ( 'NONE',  ( -12.14591786802309592, -12.06949235617757132, 31.87390960531435979 ) ) ;
#44310=CARTESIAN_POINT ( 'NONE',  ( 12.06949235617739724, 12.14591786802326823, 111.8760903946856615 ) ) ;
#44311=CARTESIAN_POINT ( 'NONE',  ( 0.05219959533936267826, -19.03943276465977164, 60.00109039468566863 ) ) ;
#44313=CARTESIAN_POINT ( 'NONE',  ( 5.153800228976335163, 19.02544592524342804, 99.79057627198102409 ) ) ;
#44314=CARTESIAN_POINT ( 'NONE',  ( -16.55341960407611168, -4.379528057220339221, 76.45724293864769550 ) ) ;
#44316=CARTESIAN_POINT ( 'NONE',  ( -19.03943276465977164, 0.05219959533909376836, 26.24890960531435624 ) ) ;
#44317=CARTESIAN_POINT ( 'NONE',  ( 21.52544592524344225, -5.823673210054117533, 38.54057627198103120 ) ) ;
#44318=CARTESIAN_POINT ( 'NONE',  ( -10.72451020669898014, 18.67979575497178502, 65.41557627198102409 ) ) ;
#44319=CARTESIAN_POINT ( 'NONE',  ( -0.05219959533909027116, -19.03943276465977164, 22.49890960531436690 ) ) ;
#44320=CARTESIAN_POINT ( 'NONE',  ( 12.06949235617739724, 12.14591786802326823, 71.87609039468568994 ) ) ;
#44321=CARTESIAN_POINT ( 'NONE',  ( 16.46253265017160672, -9.564922557960803928, 48.33224293864769550 ) ) ;
#44322=CARTESIAN_POINT ( 'NONE',  ( 5.823673210054444382, -21.52544592524334988, 55.20942372801902565 ) ) ;
#44324=CARTESIAN_POINT ( 'NONE',  ( -16.52544592524342804, 4.483927247898546575, 91.04057627198103830 ) ) ;
#44327=CARTESIAN_POINT ( 'NONE',  ( -18.62759615963270932, 10.81492255796079327, 40.83224293864769550 ) ) ;
#44329=CARTESIAN_POINT ( 'NONE',  ( -5.823673210054431948, 21.52544592524334988, 72.70942372801901854 ) ) ;
#44331=CARTESIAN_POINT ( 'NONE',  ( 8.224510206698742110, 14.34966873604972548, 57.08442372801901854 ) ) ;
#44332=CARTESIAN_POINT ( 'NONE',  ( -4.379528057220328563, 16.55341960407611168, 45.20724293864769550 ) ) ;
#44333=CARTESIAN_POINT ( 'NONE',  ( 15.72974639402199770, -15.80617190586745480, 73.12390960531436690 ) ) ;
#44334=CARTESIAN_POINT ( 'NONE',  ( -21.55341960407610458, -5.719274019375992779, 56.45724293864768839 ) ) ;
#44336=CARTESIAN_POINT ( 'NONE',  ( -16.51473224551082808, 9.474510206698731452, 78.33442372801900433 ) ) ;
#44337=CARTESIAN_POINT ( 'NONE',  ( -13.89961937509977652, 13.97604488694528158, 95.62390960531436690 ) ) ;
#44338=CARTESIAN_POINT ( 'NONE',  ( 5.153800228976335163, 19.02544592524342804, 44.79057627198103830 ) ) ;
#44339=CARTESIAN_POINT ( 'NONE',  ( 16.46253265017160672, -9.564922557960803928, 23.33224293864769194 ) ) ;
#44340=CARTESIAN_POINT ( 'NONE',  ( 13.97604488694527802, 13.89961937509977652, 109.3739096053143669 ) ) ;
#44342=CARTESIAN_POINT ( 'NONE',  ( -8.314922557961024197, 14.29746914071037800, 62.91775706135236135 ) ) ;
#44343=CARTESIAN_POINT ( 'NONE',  ( -5.719274019375978568, 21.55341960407610458, 100.2072429386476955 ) ) ;
#44344=CARTESIAN_POINT ( 'NONE',  ( -13.89961937509977652, 13.97604488694528158, 50.62390960531435979 ) ) ;
#44345=CARTESIAN_POINT ( 'NONE',  ( -18.62759615963255300, -10.81492255796106328, 44.16775706135234714 ) ) ;
#44346=CARTESIAN_POINT ( 'NONE',  ( -13.97604488694527625, -13.89961937509977652, 91.87390960531432427 ) ) ;
#44349=CARTESIAN_POINT ( 'NONE',  ( 10.72451020669871369, 18.67979575497193778, 37.08442372801901143 ) ) ;
#44350=CARTESIAN_POINT ( 'NONE',  ( -16.46253265017160317, 9.564922557960807481, 100.8322429386477097 ) ) ;
#44351=CARTESIAN_POINT ( 'NONE',  ( -19.02544592524334988, -5.153800228976617603, 93.95942372801900433 ) ) ;
#44352=CARTESIAN_POINT ( 'NONE',  ( -19.03943276465977164, -0.05219959533935918106, 38.75109039468566152 ) ) ;
#44353=CARTESIAN_POINT ( 'NONE',  ( 21.52544592524344225, -5.823673210054117533, 93.54057627198103830 ) ) ;
#44354=CARTESIAN_POINT ( 'NONE',  ( -9.474510206698720793, -16.51473224551083518, 34.58442372801899722 ) ) ;
#44355=CARTESIAN_POINT ( 'NONE',  ( -0.05219959533936034679, 19.03943276465977164, 42.50109039468566152 ) ) ;
#44356=CARTESIAN_POINT ( 'NONE',  ( -14.29746914071037622, -8.314922557961029526, 94.16775706135237556 ) ) ;
#44358=CARTESIAN_POINT ( 'NONE',  ( 16.51473224551069308, 9.474510206698969483, 59.16557627198102409 ) ) ;
#44360=CARTESIAN_POINT ( 'NONE',  ( 0.05219959533937995610, -21.53943276465977519, 70.00109039468568994 ) ) ;
#44362=CARTESIAN_POINT ( 'NONE',  ( 10.81492255796106328, -18.62759615963255655, 85.41775706135236135 ) ) ;
#44364=CARTESIAN_POINT ( 'NONE',  ( 16.46253265017160672, -9.564922557960803928, 88.33224293864769550 ) ) ;
#44365=CARTESIAN_POINT ( 'NONE',  ( 10.72451020669871369, 18.67979575497193778, 57.08442372801901854 ) ) ;
#44366=CARTESIAN_POINT ( 'NONE',  ( -16.46253265017146816, -9.564922557961047289, 104.1677570613523329 ) ) ;
#44367=CARTESIAN_POINT ( 'NONE',  ( -19.05341960407611168, -5.049401038298163336, 61.45724293864769550 ) ) ;
#44368=CARTESIAN_POINT ( 'NONE',  ( -13.89961937509977652, 13.97604488694528158, 110.6239096053143243 ) ) ;
#44369=CARTESIAN_POINT ( 'NONE',  ( 19.03943276465977164, -0.05219959533909143690, 78.74890960531436690 ) ) ;
#44371=CARTESIAN_POINT ( 'NONE',  ( -9.564922557960796823, -16.46253265017161027, 67.08224293864769550 ) ) ;
#44372=CARTESIAN_POINT ( 'NONE',  ( 19.05341960407611168, 5.049401038298154454, 48.95724293864768129 ) ) ;
#44373=CARTESIAN_POINT ( 'NONE',  ( 15.80617190586746368, 15.72974639402197994, 94.37390960531436690 ) ) ;
#44374=CARTESIAN_POINT ( 'NONE',  ( 4.379528057220092307, 16.55341960407617563, 92.29275706135236135 ) ) ;
#44376=CARTESIAN_POINT ( 'NONE',  ( 13.97604488694548053, -13.89961937509957401, 50.62609039468566152 ) ) ;
#44377=CARTESIAN_POINT ( 'NONE',  ( -9.474510206698964154, 16.51473224551069663, 80.41557627198103830 ) ) ;
#44378=CARTESIAN_POINT ( 'NONE',  ( -12.14591786802309592, -12.06949235617757132, 71.87390960531438111 ) ) ;
#44379=CARTESIAN_POINT ( 'NONE',  ( 12.14591786802309770, 12.06949235617756955, 109.3739096053143811 ) ) ;
#44380=CARTESIAN_POINT ( 'NONE',  ( -16.51473224551069308, -9.474510206698971260, 111.6655762719810383 ) ) ;
#44381=( BOUNDED_CURVE ( )  B_SPLINE_CURVE ( 2, ( #156949, #31621, #32614, #169121, #80097, #15461, #138787, #46791, #108450, #178112, #22422, #35587, #162928 ),
 .UNSPECIFIED., .F., .T. ) 
 B_SPLINE_CURVE_WITH_KNOTS ( ( 3, 2, 2, 2, 2, 2, 3 ),
 ( 0.2130024320386090242, 0.2149122807017543879, 0.2192982456140350755, 0.2236842105263157909, 0.2280701754385964786, 0.2324561403508771940, 0.2344116688361128631 ),
 .UNSPECIFIED. ) 
 CURVE ( )  GEOMETRIC_REPRESENTATION_ITEM ( )  RATIONAL_B_SPLINE_CURVE ( ( 0.9832469066685285419, 0.9851625545550100060, 1.000000000000000000, 0.9659258262890683122, 1.000000000000000000, 0.9659258262890683122, 1.000000000000000000, 0.9659258262890683122, 1.000000000000000000, 0.9659258262890683122, 1.000000000000000000, 0.9848076720550082985, 0.9831626618144004848 ) ) 
 REPRESENTATION_ITEM ( '' )  );
#44382=CARTESIAN_POINT ( 'NONE',  ( -13.89961937509977652, 13.97604488694528158, 100.6239096053143669 ) ) ;
#44383=CARTESIAN_POINT ( 'NONE',  ( 16.46253265017160672, -9.564922557960803928, 83.33224293864768129 ) ) ;
#44384=CARTESIAN_POINT ( 'NONE',  ( -16.51473224551082808, 9.474510206698731452, 33.33442372801899722 ) ) ;
#44385=CARTESIAN_POINT ( 'NONE',  ( 0.05219959533934541429, -16.53943276465976808, 90.00109039468567573 ) ) ;
#44386=CARTESIAN_POINT ( 'NONE',  ( -9.564922557960796823, -16.46253265017161027, 72.08224293864770971 ) ) ;
#44387=CARTESIAN_POINT ( 'NONE',  ( -5.719274019375665041, -21.55341960407619695, 49.79275706135234714 ) ) ;
#44388=CARTESIAN_POINT ( 'NONE',  ( 21.53943276465977519, -0.05219959533907433946, 38.74890960531435979 ) ) ;
#44389=CARTESIAN_POINT ( 'NONE',  ( -15.72974639402176322, -15.80617190586768395, 19.37609039468568639 ) ) ;
#44390=CARTESIAN_POINT ( 'NONE',  ( 21.55341960407610458, 5.719274019375980345, 68.95724293864769550 ) ) ;
#44391=CARTESIAN_POINT ( 'NONE',  ( 4.483927247898545687, 16.52544592524342804, 94.79057627198105251 ) ) ;
#44392=CARTESIAN_POINT ( 'NONE',  ( 19.03943276465977164, 0.05219959533936151252, 51.25109039468567573 ) ) ;
#44394=CARTESIAN_POINT ( 'NONE',  ( -19.02544592524342804, 5.153800228976336051, 36.04057627198100988 ) ) ;
#44395=CARTESIAN_POINT ( 'NONE',  ( 5.153800228976335163, 19.02544592524342804, 79.79057627198102409 ) ) ;
#44396=CARTESIAN_POINT ( 'NONE',  ( -5.153800228976328057, -19.02544592524343514, 82.29057627198103830 ) ) ;
#44398=CARTESIAN_POINT ( 'NONE',  ( -14.34966873604960291, -8.224510206698953496, 106.6655762719810383 ) ) ;
#44399=ORIENTED_EDGE ( 'NONE', *, *, #15491, .F. ) ;
#44400=CARTESIAN_POINT ( 'NONE',  ( 4.379528057220339221, -16.55341960407611168, 22.70724293864769194 ) ) ;
#44401=CARTESIAN_POINT ( 'NONE',  ( -12.14591786802326823, 12.06949235617739902, 33.12609039468569705 ) ) ;
#44402=CARTESIAN_POINT ( 'NONE',  ( -18.67979575497193778, 10.72451020669871902, 93.33442372801901854 ) ) ;
#44403=CARTESIAN_POINT ( 'NONE',  ( 19.02544592524343514, -5.153800228976328945, 103.5405762719809957 ) ) ;
#44404=CARTESIAN_POINT ( 'NONE',  ( 10.72451020669898902, -18.67979575497178502, 112.9155762719810383 ) ) ;
#44405=CARTESIAN_POINT ( 'NONE',  ( 16.46253265017160672, -9.564922557960803928, 43.33224293864769550 ) ) ;
#44406=CARTESIAN_POINT ( 'NONE',  ( -14.29746914071037622, -8.314922557961029526, 49.16775706135234003 ) ) ;
#44407=CARTESIAN_POINT ( 'NONE',  ( 16.46253265017146816, 9.564922557961045513, 111.6677570613523329 ) ) ;
#44408=CARTESIAN_POINT ( 'NONE',  ( 16.51473224551069308, 9.474510206698969483, 39.16557627198103120 ) ) ;
#44409=CARTESIAN_POINT ( 'NONE',  ( -0.05219959533910754901, -16.53943276465976808, 92.49890960531436690 ) ) ;
#44410=CARTESIAN_POINT ( 'NONE',  ( -10.81492255796078084, -18.62759615963271287, 107.0822429386476955 ) ) ;
#44411=CARTESIAN_POINT ( 'NONE',  ( -19.03943276465977164, -0.05219959533935918106, 68.75109039468566152 ) ) ;
#44412=CARTESIAN_POINT ( 'NONE',  ( -0.05219959533909027116, -19.03943276465977164, 22.49890960531436690 ) ) ;
#44413=CARTESIAN_POINT ( 'NONE',  ( -10.72451020669870658, -18.67979575497194134, 19.58442372801901143 ) ) ;
#44415=CARTESIAN_POINT ( 'NONE',  ( 13.97604488694527802, 13.89961937509977652, 94.37390960531436690 ) ) ;
#44416=LINE ( 'NONE', #14061, #55114 ) ;
#44417=CARTESIAN_POINT ( 'NONE',  ( -5.153800228976328057, -19.02544592524343514, 87.29057627198103830 ) ) ;
#44418=CARTESIAN_POINT ( 'NONE',  ( 5.823673210054444382, -21.52544592524334988, 30.20942372801902565 ) ) ;
#44419=CARTESIAN_POINT ( 'NONE',  ( -8.314922557960811034, -14.29746914071050412, 82.08224293864768129 ) ) ;
#44420=CARTESIAN_POINT ( 'NONE',  ( -0.05219959533909027116, -19.03943276465977164, 77.49890960531435269 ) ) ;
#44421=CARTESIAN_POINT ( 'NONE',  ( 13.89961937509957401, 13.97604488694547697, 26.87609039468566507 ) ) ;
#44422=CARTESIAN_POINT ( 'NONE',  ( -14.29746914071037622, -8.314922557961029526, 49.16775706135234003 ) ) ;
#44423=CARTESIAN_POINT ( 'NONE',  ( 19.03943276465977164, 0.05219959533936151252, 56.25109039468566863 ) ) ;
#44424=CARTESIAN_POINT ( 'NONE',  ( 18.67979575497194134, -10.72451020669871369, 60.83442372801901854 ) ) ;
#44425=CARTESIAN_POINT ( 'NONE',  ( -12.06949235617739369, -12.14591786802326823, 29.37609039468568284 ) ) ;
#44426=CARTESIAN_POINT ( 'NONE',  ( -19.03943276465977164, 0.05219959533909376836, 71.24890960531435269 ) ) ;
#44427=CARTESIAN_POINT ( 'NONE',  ( 19.03943276465977164, 0.05219959533936151252, 96.25109039468567573 ) ) ;
#44428=CARTESIAN_POINT ( 'NONE',  ( 4.483927247898790824, -16.52544592524335698, 65.20942372801901854 ) ) ;
#44429=CARTESIAN_POINT ( 'NONE',  ( -21.52544592524334988, -5.823673210054445271, 103.9594237280190185 ) ) ;
#44430=CARTESIAN_POINT ( 'NONE',  ( -0.05219959533936034679, 19.03943276465977164, 82.50109039468567573 ) ) ;
#44431=CARTESIAN_POINT ( 'NONE',  ( -9.474510206698964154, 16.51473224551069663, 50.41557627198102409 ) ) ;
#44432=CARTESIAN_POINT ( 'NONE',  ( 10.81492255796078972, 18.62759615963270932, 84.58224293864769550 ) ) ;
#44433=CARTESIAN_POINT ( 'NONE',  ( -12.06949235617756955, 12.14591786802309770, 80.62390960531438111 ) ) ;
#44434=CARTESIAN_POINT ( 'NONE',  ( 9.474510206698729675, 16.51473224551082808, 82.08442372801899012 ) ) ;
#44435=CARTESIAN_POINT ( 'NONE',  ( 17.50000000000004263, -5.622605283950769639, 61.18792689403890961 ) ) ;
#44436=CARTESIAN_POINT ( 'NONE',  ( 19.02544592524334988, 5.153800228976608722, 46.45942372801899012 ) ) ;
#44437=CARTESIAN_POINT ( 'NONE',  ( -0.05219959533910754901, -16.53943276465976808, 22.49890960531436335 ) ) ;
#44438=CARTESIAN_POINT ( 'NONE',  ( 0.05219959533910956823, 16.53943276465976808, 69.99890960531435269 ) ) ;
#44439=CARTESIAN_POINT ( 'NONE',  ( 5.719274019375673035, 21.55341960407619339, 97.29275706135234714 ) ) ;
#44441=CARTESIAN_POINT ( 'NONE',  ( 21.52544592524344225, -5.823673210054117533, 103.5405762719810383 ) ) ;
#44442=CARTESIAN_POINT ( 'NONE',  ( -19.05341960407611168, -5.049401038298163336, 71.45724293864766707 ) ) ;
#44443=CARTESIAN_POINT ( 'NONE',  ( -21.52544592524334988, -5.823673210054445271, 78.95942372801901854 ) ) ;
#44444=CARTESIAN_POINT ( 'NONE',  ( 13.89961937509977652, -13.97604488694527269, 68.12390960531436690 ) ) ;
#44446=CARTESIAN_POINT ( 'NONE',  ( 5.153800228976335163, 19.02544592524342804, 29.79057627198102409 ) ) ;
#44447=CARTESIAN_POINT ( 'NONE',  ( 10.81492255796078972, 18.62759615963270932, 34.58224293864770260 ) ) ;
#44448=CARTESIAN_POINT ( 'NONE',  ( -4.483927247898539470, -16.52544592524342804, 62.29057627198102409 ) ) ;
#44449=CARTESIAN_POINT ( 'NONE',  ( -19.05341960407611168, -5.049401038298163336, 46.45724293864768129 ) ) ;
#44450=CARTESIAN_POINT ( 'NONE',  ( 14.34966873604960469, 8.224510206698951720, 99.16557627198100988 ) ) ;
#44452=CARTESIAN_POINT ( 'NONE',  ( -21.55341960407610458, -5.719274019375992779, 111.4572429386476813 ) ) ;
#44453=CARTESIAN_POINT ( 'NONE',  ( -21.52544592524334988, -5.823673210054445271, 53.95942372801900433 ) ) ;
#44454=CARTESIAN_POINT ( 'NONE',  ( -13.97604488694527625, -13.89961937509977652, 36.87390960531436690 ) ) ;
#44455=CARTESIAN_POINT ( 'NONE',  ( 8.224510206698742110, 14.34966873604972548, 47.08442372801901854 ) ) ;
#44456=CARTESIAN_POINT ( 'NONE',  ( 5.719274019375991003, -21.55341960407610458, 102.7072429386476955 ) ) ;
#44457=CARTESIAN_POINT ( 'NONE',  ( -18.67979575497178146, -10.72451020669898902, 91.66557627198103830 ) ) ;
#44458=CARTESIAN_POINT ( 'NONE',  ( -19.03943276465977164, -0.05219959533935918106, 23.75109039468566152 ) ) ;
#44459=CARTESIAN_POINT ( 'NONE',  ( -19.02544592524342804, 5.153800228976336051, 56.04057627198100988 ) ) ;
#44460=CARTESIAN_POINT ( 'NONE',  ( -5.153800228976328057, -19.02544592524343514, 112.2905762719810099 ) ) ;
#44461=CARTESIAN_POINT ( 'NONE',  ( -21.55341960407619339, 5.719274019375674811, 58.54275706135235424 ) ) ;
#44462=CARTESIAN_POINT ( 'NONE',  ( 18.67979575497178502, 10.72451020669898547, 44.16557627198103120 ) ) ;
#44463=CARTESIAN_POINT ( 'NONE',  ( -4.483927247898782831, 16.52544592524335698, 112.7094237280190328 ) ) ;
#44464=CARTESIAN_POINT ( 'NONE',  ( -18.67979575497193778, 10.72451020669871902, 63.33442372801900433 ) ) ;
#44465=CARTESIAN_POINT ( 'NONE',  ( 21.53943276465977519, 0.05219959533937863772, 101.2510903946856757 ) ) ;
#44466=CARTESIAN_POINT ( 'NONE',  ( -19.03943276465977164, -0.05219959533935918106, 38.75109039468566152 ) ) ;
#44467=CARTESIAN_POINT ( 'NONE',  ( -16.52544592524335698, -4.483927247898792601, 103.9594237280190185 ) ) ;
#44468=CARTESIAN_POINT ( 'NONE',  ( -18.62759615963255300, -10.81492255796106328, 49.16775706135234003 ) ) ;
#44469=CARTESIAN_POINT ( 'NONE',  ( 16.46253265017160672, -9.564922557960803928, 58.33224293864769550 ) ) ;
#44470=CARTESIAN_POINT ( 'NONE',  ( -13.89961937509957401, -13.97604488694547875, 19.37609039468566507 ) ) ;
#44471=CARTESIAN_POINT ( 'NONE',  ( -19.02544592524342804, 5.153800228976336051, 116.0405762719810383 ) ) ;
#44472=CARTESIAN_POINT ( 'NONE',  ( 10.72451020669871369, 18.67979575497193778, 32.08442372801901854 ) ) ;
#44473=CARTESIAN_POINT ( 'NONE',  ( -21.53943276465977519, 0.05219959533907696930, 86.24890960531436690 ) ) ;
#44474=CARTESIAN_POINT ( 'NONE',  ( 12.14591786802327356, -12.06949235617739191, 40.62609039468567573 ) ) ;
#44475=CARTESIAN_POINT ( 'NONE',  ( 17.50000000000000000, 5.499999999999997335, 31.70309617465830243 ) ) ;
#44476=CARTESIAN_POINT ( 'NONE',  ( -10.72451020669898014, 18.67979575497178502, 75.41557627198102409 ) ) ;
#44477=CARTESIAN_POINT ( 'NONE',  ( 8.224510206698742110, 14.34966873604972548, 62.08442372801901143 ) ) ;
#44478=CARTESIAN_POINT ( 'NONE',  ( -12.14591786802309592, -12.06949235617757132, 71.87390960531438111 ) ) ;
#44480=CARTESIAN_POINT ( 'NONE',  ( -5.153800228976607833, 19.02544592524334988, 97.70942372801900433 ) ) ;
#44481=CARTESIAN_POINT ( 'NONE',  ( -21.52544592524343514, 5.823673210054127303, 36.04057627198102409 ) ) ;
#44484=CARTESIAN_POINT ( 'NONE',  ( 16.52544592524335698, 4.483927247898782831, 36.45942372801901143 ) ) ;
#44485=CARTESIAN_POINT ( 'NONE',  ( -18.67979575497178146, -10.72451020669898902, 106.6655762719810383 ) ) ;
#44486=CARTESIAN_POINT ( 'NONE',  ( 18.62759615963271287, -10.81492255796078972, 33.33224293864769550 ) ) ;
#44487=CARTESIAN_POINT ( 'NONE',  ( -16.53943276465976808, -0.05219959533934237506, 73.75109039468567573 ) ) ;
#44488=CARTESIAN_POINT ( 'NONE',  ( -16.51473224551069308, -9.474510206698971260, 81.66557627198103830 ) ) ;
#44489=CARTESIAN_POINT ( 'NONE',  ( -21.53943276465977519, -0.05219959533937600094, 53.75109039468568994 ) ) ;
#44490=CARTESIAN_POINT ( 'NONE',  ( 19.05341960407611168, 5.049401038298154454, 33.95724293864769550 ) ) ;
#44491=CARTESIAN_POINT ( 'NONE',  ( -13.89961937509977652, 13.97604488694528158, 115.6239096053143669 ) ) ;
#44493=CARTESIAN_POINT ( 'NONE',  ( -16.46253265017146816, -9.564922557961047289, 39.16775706135234003 ) ) ;
#44494=CARTESIAN_POINT ( 'NONE',  ( -4.483927247898782831, 16.52544592524335698, 47.70942372801902565 ) ) ;
#44495=CARTESIAN_POINT ( 'NONE',  ( 5.153800228976335163, 19.02544592524342804, 114.7905762719810241 ) ) ;
#44496=CARTESIAN_POINT ( 'NONE',  ( -13.89961937509977652, 13.97604488694528158, 70.62390960531432427 ) ) ;
#44497=CARTESIAN_POINT ( 'NONE',  ( 8.224510206698742110, 14.34966873604972548, 97.08442372801904696 ) ) ;
#44499=CARTESIAN_POINT ( 'NONE',  ( 4.379528057220339221, -16.55341960407611168, 97.70724293864772392 ) ) ;
#44500=CARTESIAN_POINT ( 'NONE',  ( 5.823673210054125526, 21.52544592524343514, 34.79057627198103120 ) ) ;
#44501=CARTESIAN_POINT ( 'NONE',  ( -9.564922557960796823, -16.46253265017161027, 37.08224293864768839 ) ) ;
#44502=CARTESIAN_POINT ( 'NONE',  ( 16.55341960407618274, -4.379528057220086978, 61.04275706135234714 ) ) ;
#44503=CARTESIAN_POINT ( 'NONE',  ( -21.53943276465977519, 0.05219959533907696930, 116.2489096053143669 ) ) ;
#44504=CARTESIAN_POINT ( 'NONE',  ( 5.049401038297881783, 19.05341960407617563, 72.29275706135234714 ) ) ;
#44505=CARTESIAN_POINT ( 'NONE',  ( 16.46253265017160672, -9.564922557960803928, 38.33224293864768839 ) ) ;
#44506=CARTESIAN_POINT ( 'NONE',  ( 0.05219959533907565091, 21.53943276465977519, 64.99890960531435269 ) ) ;
#44507=CARTESIAN_POINT ( 'NONE',  ( -9.474510206698964154, 16.51473224551069663, 115.4155762719810241 ) ) ;
#44508=CARTESIAN_POINT ( 'NONE',  ( 21.52544592524334988, 5.823673210054432836, 91.45942372801901854 ) ) ;
#44509=CARTESIAN_POINT ( 'NONE',  ( 13.97604488694527802, 13.89961937509977652, 64.37390960531436690 ) ) ;
#44510=CARTESIAN_POINT ( 'NONE',  ( 12.14591786802327356, -12.06949235617739191, 55.62609039468568284 ) ) ;
#44511=CARTESIAN_POINT ( 'NONE',  ( 13.89961937509977652, -13.97604488694527269, 63.12390960531435979 ) ) ;
#44512=CARTESIAN_POINT ( 'NONE',  ( -10.72451020669870658, -18.67979575497194134, 84.58442372801903275 ) ) ;
#44513=CARTESIAN_POINT ( 'NONE',  ( 16.46253265017146816, 9.564922557961045513, 41.66775706135234003 ) ) ;
#44514=CARTESIAN_POINT ( 'NONE',  ( -9.474510206698720793, -16.51473224551083518, 54.58442372801899722 ) ) ;
#44515=CARTESIAN_POINT ( 'NONE',  ( 0.05219959533937995610, -21.53943276465977519, 55.00109039468568284 ) ) ;
#44517=CARTESIAN_POINT ( 'NONE',  ( -9.474510206698720793, -16.51473224551083518, 44.58442372801900433 ) ) ;
#44518=CARTESIAN_POINT ( 'NONE',  ( -9.474510206698964154, 16.51473224551069663, 95.41557627198102409 ) ) ;
#44519=CARTESIAN_POINT ( 'NONE',  ( 13.89961937509977652, -13.97604488694527269, 83.12390960531436690 ) ) ;
#44520=CARTESIAN_POINT ( 'NONE',  ( -0.05219959533910754901, -16.53943276465976808, 32.49890960531435979 ) ) ;
#44521=CARTESIAN_POINT ( 'NONE',  ( -15.72974639402197994, 15.80617190586746368, 30.62390960531436335 ) ) ;
#44522=CARTESIAN_POINT ( 'NONE',  ( -5.719274019375665041, -21.55341960407619695, 94.79275706135234714 ) ) ;
#44525=CARTESIAN_POINT ( 'NONE',  ( 10.72451020669871369, 18.67979575497193778, 92.08442372801901854 ) ) ;
#44527=CARTESIAN_POINT ( 'NONE',  ( 9.564922557960805705, 16.46253265017160317, 34.58224293864770260 ) ) ;
#44529=EDGE_CURVE ( 'NONE', #142736, #3830, #81669, .T. ) ;
#44531=CARTESIAN_POINT ( 'NONE',  ( 0.05219959533934541429, -16.53943276465976808, 45.00109039468568284 ) ) ;
#44532=CARTESIAN_POINT ( 'NONE',  ( -18.62759615963270932, 10.81492255796079327, 65.83224293864769550 ) ) ;
#44533=CARTESIAN_POINT ( 'NONE',  ( 8.314922557960818139, 14.29746914071049879, 44.58224293864769550 ) ) ;
#44534=CARTESIAN_POINT ( 'NONE',  ( 16.55341960407611168, 4.379528057220329451, 108.9572429386476955 ) ) ;
#44535=CARTESIAN_POINT ( 'NONE',  ( 16.46253265017160672, -9.564922557960803928, 113.3322429386476955 ) ) ;
#44536=CARTESIAN_POINT ( 'NONE',  ( 0.05219959533937995610, -21.53943276465977519, 25.00109039468567218 ) ) ;
#44537=CARTESIAN_POINT ( 'NONE',  ( 13.89961937509957401, 13.97604488694547697, 41.87609039468566152 ) ) ;
#44538=CARTESIAN_POINT ( 'NONE',  ( -14.29746914071049879, 8.314922557960819915, 115.8322429386477097 ) ) ;
#44539=CARTESIAN_POINT ( 'NONE',  ( 15.72974639402176855, 15.80617190586768217, 61.87609039468568284 ) ) ;
#44540=CARTESIAN_POINT ( 'NONE',  ( 17.40861289039004944, -6.110651285853252901, 31.12767529172569780 ) ) ;
#44541=CARTESIAN_POINT ( 'NONE',  ( -8.314922557960811034, -14.29746914071050412, 27.08224293864769550 ) ) ;
#44542=CARTESIAN_POINT ( 'NONE',  ( -0.05219959533936034679, 19.03943276465977164, 67.50109039468566152 ) ) ;
#44543=CARTESIAN_POINT ( 'NONE',  ( 21.52544592524344225, -5.823673210054117533, 23.54057627198102765 ) ) ;
#44544=CARTESIAN_POINT ( 'NONE',  ( -8.224510206698948167, 14.34966873604960824, 85.41557627198102409 ) ) ;
#44546=CARTESIAN_POINT ( 'NONE',  ( -5.153800228976328057, -19.02544592524343514, 72.29057627198102409 ) ) ;
#44547=CARTESIAN_POINT ( 'NONE',  ( 0.05219959533910956823, 16.53943276465976808, 69.99890960531435269 ) ) ;
#44548=CARTESIAN_POINT ( 'NONE',  ( -0.05219959533936034679, 19.03943276465977164, 102.5010903946856757 ) ) ;
#44549=CARTESIAN_POINT ( 'NONE',  ( -5.719274019375978568, 21.55341960407610458, 45.20724293864769550 ) ) ;
#44550=ORIENTED_EDGE ( 'NONE', *, *, #192276, .T. ) ;
#44551=CARTESIAN_POINT ( 'NONE',  ( 12.06949235617757843, -12.14591786802309237, 113.1239096053143953 ) ) ;
#44552=CARTESIAN_POINT ( 'NONE',  ( -13.97604488694527625, -13.89961937509977652, 66.87390960531436690 ) ) ;
#44553=CARTESIAN_POINT ( 'NONE',  ( 10.81492255796078972, 18.62759615963270932, 79.58224293864769550 ) ) ;
#44554=CARTESIAN_POINT ( 'NONE',  ( 16.52544592524335698, 4.483927247898782831, 111.4594237280190328 ) ) ;
#44555=CARTESIAN_POINT ( 'NONE',  ( -19.03943276465977164, 0.05219959533909376836, 91.24890960531436690 ) ) ;
#44556=CARTESIAN_POINT ( 'NONE',  ( -19.03943276465977164, -0.05219959533935918106, 73.75109039468566152 ) ) ;
#44557=CARTESIAN_POINT ( 'NONE',  ( -21.52544592524334988, -5.823673210054445271, 93.95942372801903275 ) ) ;
#44558=CARTESIAN_POINT ( 'NONE',  ( 21.53943276465977519, -0.05219959533907433946, 68.74890960531435269 ) ) ;
#44559=CARTESIAN_POINT ( 'NONE',  ( 16.46253265017160672, -9.564922557960803928, 113.3322429386476955 ) ) ;
#44560=CARTESIAN_POINT ( 'NONE',  ( 13.89961937509977652, -13.97604488694527269, 53.12390960531434558 ) ) ;
#44561=CARTESIAN_POINT ( 'NONE',  ( 12.06949235617739724, 12.14591786802326823, 101.8760903946857042 ) ) ;
#44562=CARTESIAN_POINT ( 'NONE',  ( -16.51473224551069308, -9.474510206698971260, 66.66557627198102409 ) ) ;
#44563=CARTESIAN_POINT ( 'NONE',  ( -8.314922557961024197, 14.29746914071037800, 22.91775706135235069 ) ) ;
#44565=CARTESIAN_POINT ( 'NONE',  ( 18.62759615963255655, 10.81492255796105972, 111.6677570613523613 ) ) ;
#44566=CARTESIAN_POINT ( 'NONE',  ( 14.29746914071049879, -8.314922557960816363, 78.33224293864770971 ) ) ;
#44567=CARTESIAN_POINT ( 'NONE',  ( -15.72974639402197994, 15.80617190586746368, 105.6239096053143669 ) ) ;
#44568=CARTESIAN_POINT ( 'NONE',  ( 21.55341960407610458, 5.719274019375980345, 98.95724293864770971 ) ) ;
#44570=CARTESIAN_POINT ( 'NONE',  ( 0.05219959533907565091, 21.53943276465977519, 64.99890960531435269 ) ) ;
#44571=CARTESIAN_POINT ( 'NONE',  ( -0.05219959533934338120, 16.53943276465976808, 77.50109039468567573 ) ) ;
#44572=CARTESIAN_POINT ( 'NONE',  ( 12.06949235617757843, -12.14591786802309237, 103.1239096053143811 ) ) ;
#44573=CARTESIAN_POINT ( 'NONE',  ( -13.97604488694527625, -13.89961937509977652, 61.87390960531435979 ) ) ;
#44574=CARTESIAN_POINT ( 'NONE',  ( -16.55341960407611168, -4.379528057220339221, 21.45724293864769550 ) ) ;
#44575=CARTESIAN_POINT ( 'NONE',  ( -5.823673210054431948, 21.52544592524334988, 47.70942372801902565 ) ) ;
#44576=CARTESIAN_POINT ( 'NONE',  ( -19.05341960407611168, -5.049401038298163336, 101.4572429386476955 ) ) ;
#44577=CARTESIAN_POINT ( 'NONE',  ( 10.81492255796106328, -18.62759615963255655, 80.41775706135234714 ) ) ;
#44578=CARTESIAN_POINT ( 'NONE',  ( 19.02544592524343514, -5.153800228976328945, 33.54057627198102409 ) ) ;
#44579=CARTESIAN_POINT ( 'NONE',  ( -16.51473224551069308, -9.474510206698971260, 41.66557627198103120 ) ) ;
#44580=VERTEX_POINT ( 'NONE', #145354 ) ;
#44581=CARTESIAN_POINT ( 'NONE',  ( -15.80617190586768217, 15.72974639402176855, 78.12609039468570415 ) ) ;
#44582=CARTESIAN_POINT ( 'NONE',  ( -5.153800228976328057, -19.02544592524343514, 102.2905762719810383 ) ) ;
#44583=CARTESIAN_POINT ( 'NONE',  ( 5.153800228976615827, -19.02544592524334988, 80.20942372801901854 ) ) ;
#44584=CARTESIAN_POINT ( 'NONE',  ( -15.80617190586768217, 15.72974639402176855, 38.12609039468567573 ) ) ;
#44585=CARTESIAN_POINT ( 'NONE',  ( -8.314922557961024197, 14.29746914071037800, 22.91775706135235069 ) ) ;
#44586=CARTESIAN_POINT ( 'NONE',  ( -5.153800228976607833, 19.02544592524334988, 72.70942372801900433 ) ) ;
#44587=CARTESIAN_POINT ( 'NONE',  ( -19.02544592524342804, 5.153800228976336051, 51.04057627198103120 ) ) ;
#44588=CARTESIAN_POINT ( 'NONE',  ( -13.89961937509957401, -13.97604488694547875, 84.37609039468567573 ) ) ;
#44590=CARTESIAN_POINT ( 'NONE',  ( 12.14591786802309770, 12.06949235617756955, 24.37390960531435979 ) ) ;
#44591=CARTESIAN_POINT ( 'NONE',  ( 19.05341960407617918, -5.049401038297876454, 91.04275706135234714 ) ) ;
#44592=CARTESIAN_POINT ( 'NONE',  ( 0.05219959533910956823, 16.53943276465976808, 34.99890960531435979 ) ) ;
#44593=CARTESIAN_POINT ( 'NONE',  ( -0.05219959533936034679, 19.03943276465977164, 67.50109039468566152 ) ) ;
#44594=CARTESIAN_POINT ( 'NONE',  ( -4.483927247898782831, 16.52544592524335698, 42.70942372801901854 ) ) ;
#44595=CARTESIAN_POINT ( 'NONE',  ( 9.564922557961047289, -16.46253265017146816, 30.41775706135232937 ) ) ;
#44597=CARTESIAN_POINT ( 'NONE',  ( 16.46253265017160672, -9.564922557960803928, 28.33224293864769550 ) ) ;
#44598=CARTESIAN_POINT ( 'NONE',  ( 18.56197773271727769, -5.500000000000078160, 71.05066217314453070 ) ) ;
#44599=CARTESIAN_POINT ( 'NONE',  ( 12.06949235617739724, 12.14591786802326823, 51.87609039468568284 ) ) ;
#44602=CARTESIAN_POINT ( 'NONE',  ( -13.89961937509977652, 13.97604488694528158, 90.62390960531432427 ) ) ;
#44604=ORIENTED_EDGE ( 'NONE', *, *, #130089, .F. ) ;
#44605=CARTESIAN_POINT ( 'NONE',  ( -19.02544592524334988, -5.153800228976617603, 78.95942372801900433 ) ) ;
#44606=CARTESIAN_POINT ( 'NONE',  ( -5.719274019375978568, 21.55341960407610458, 30.20724293864769550 ) ) ;
#44607=CARTESIAN_POINT ( 'NONE',  ( -19.03943276465977164, -0.05219959533935918106, 23.75109039468566152 ) ) ;
#44608=CARTESIAN_POINT ( 'NONE',  ( 19.03943276465977164, 0.05219959533936151252, 96.25109039468567573 ) ) ;
#44609=CARTESIAN_POINT ( 'NONE',  ( 14.34966873604960469, 8.224510206698951720, 109.1655762719810383 ) ) ;
#44610=CARTESIAN_POINT ( 'NONE',  ( -13.89961937509977652, 13.97604488694528158, 40.62390960531435979 ) ) ;
#44611=CARTESIAN_POINT ( 'NONE',  ( 18.67979575497178502, 10.72451020669898547, 59.16557627198103120 ) ) ;
#44612=CARTESIAN_POINT ( 'NONE',  ( -0.05219959533910754901, -16.53943276465976808, 112.4989096053143669 ) ) ;
#44614=CARTESIAN_POINT ( 'NONE',  ( 16.46253265017146816, 9.564922557961045513, 66.66775706135233293 ) ) ;
#44615=CARTESIAN_POINT ( 'NONE',  ( -4.379528057220328563, 16.55341960407611168, 35.20724293864768839 ) ) ;
#44616=VECTOR ( 'NONE', #52347, 1000.000000000000000 ) ;
#44617=CARTESIAN_POINT ( 'NONE',  ( 13.97604488694527802, 13.89961937509977652, 109.3739096053143669 ) ) ;
#44618=CARTESIAN_POINT ( 'NONE',  ( 10.81492255796106328, -18.62759615963255655, 90.41775706135236135 ) ) ;
#44619=CARTESIAN_POINT ( 'NONE',  ( -21.55341960407610458, -5.719274019375992779, 86.45724293864770971 ) ) ;
#44620=CARTESIAN_POINT ( 'NONE',  ( -5.719274019375665041, -21.55341960407619695, 54.79275706135235424 ) ) ;
#44621=CARTESIAN_POINT ( 'NONE',  ( 18.62759615963255655, 10.81492255796105972, 61.66775706135235424 ) ) ;
#44622=CARTESIAN_POINT ( 'NONE',  ( 9.564922557960805705, 16.46253265017160317, 94.58224293864769550 ) ) ;
#44623=CARTESIAN_POINT ( 'NONE',  ( -0.05219959533934338120, 16.53943276465976808, 92.50109039468567573 ) ) ;
#44624=CARTESIAN_POINT ( 'NONE',  ( -5.823673210054431948, 21.52544592524334988, 47.70942372801902565 ) ) ;
#44625=( BOUNDED_CURVE ( )  B_SPLINE_CURVE ( 2, ( #11310, #196335, #57803, #119474, #181157, #42633, #104296, #27479, #12306, #58775, #120443, #50578, #126407 ),
 .UNSPECIFIED., .F., .T. ) 
 B_SPLINE_CURVE_WITH_KNOTS ( ( 3, 2, 2, 2, 2, 2, 3 ),
 ( 0.6866866425649248429, 0.6885964912280702066, 0.6929824561403509220, 0.6973684210526315264, 0.7017543859649122417, 0.7061403508771929571, 0.7080958793624286818 ),
 .UNSPECIFIED. ) 
 CURVE ( )  GEOMETRIC_REPRESENTATION_ITEM ( )  RATIONAL_B_SPLINE_CURVE ( ( 0.9832469066685285419, 0.9851625545550100060, 1.000000000000000000, 0.9659258262890683122, 1.000000000000000000, 0.9659258262890683122, 1.000000000000000000, 0.9659258262890683122, 1.000000000000000000, 0.9659258262890683122, 1.000000000000000000, 0.9848076720550078544, 0.9831626618144001517 ) ) 
 REPRESENTATION_ITEM ( '' )  );
#44626=CARTESIAN_POINT ( 'NONE',  ( 12.06949235617757843, -12.14591786802309237, 113.1239096053143953 ) ) ;
#44627=CARTESIAN_POINT ( 'NONE',  ( -8.314922557960811034, -14.29746914071050412, 72.08224293864769550 ) ) ;
#44628=CARTESIAN_POINT ( 'NONE',  ( 16.52544592524342804, -4.483927247898539470, 38.54057627198103120 ) ) ;
#44629=CARTESIAN_POINT ( 'NONE',  ( -0.05219959533907301413, -21.53943276465977519, 42.49890960531435979 ) ) ;
#44630=CARTESIAN_POINT ( 'NONE',  ( -19.05341960407611168, -5.049401038298163336, 66.45724293864769550 ) ) ;
#44631=CARTESIAN_POINT ( 'NONE',  ( -16.51473224551069308, -9.474510206698971260, 46.66557627198102409 ) ) ;
#44632=CARTESIAN_POINT ( 'NONE',  ( -5.719274019375978568, 21.55341960407610458, 60.20724293864768839 ) ) ;
#44633=CARTESIAN_POINT ( 'NONE',  ( -19.05341960407617563, 5.049401038297882671, 43.54275706135232582 ) ) ;
#44635=CARTESIAN_POINT ( 'NONE',  ( 14.34966873604960469, 8.224510206698951720, 49.16557627198102409 ) ) ;
#44636=CARTESIAN_POINT ( 'NONE',  ( 5.823673210054125526, 21.52544592524343514, 24.79057627198103120 ) ) ;
#44638=VERTEX_POINT ( 'NONE', #99849 ) ;
#44640=CARTESIAN_POINT ( 'NONE',  ( -14.29746914071037622, -8.314922557961029526, 69.16775706135234714 ) ) ;
#44641=CARTESIAN_POINT ( 'NONE',  ( -13.89961937509957401, -13.97604488694547875, 79.37609039468567573 ) ) ;
#44642=CARTESIAN_POINT ( 'NONE',  ( -16.52544592524342804, 4.483927247898546575, 41.04057627198103120 ) ) ;
#44643=CARTESIAN_POINT ( 'NONE',  ( -19.53091890409952214, -5.500000000000036415, 60.06097431831418731 ) ) ;
#44644=CARTESIAN_POINT ( 'NONE',  ( 16.52544592524342804, -4.483927247898539470, 33.54057627198102409 ) ) ;
#44645=CARTESIAN_POINT ( 'NONE',  ( -5.049401038298153566, 19.05341960407611168, 55.20724293864769550 ) ) ;
#44646=CARTESIAN_POINT ( 'NONE',  ( 9.474510206698971260, -16.51473224551069308, 77.91557627198103830 ) ) ;
#44647=CARTESIAN_POINT ( 'NONE',  ( 5.049401038298161559, -19.05341960407611168, 42.70724293864767418 ) ) ;
#44648=CARTESIAN_POINT ( 'NONE',  ( 15.80617190586769283, -15.72974639402175789, 50.62609039468568994 ) ) ;
#44649=CARTESIAN_POINT ( 'NONE',  ( -5.153800228976328057, -19.02544592524343514, 62.29057627198100988 ) ) ;
#44651=CARTESIAN_POINT ( 'NONE',  ( 0.05219959533909260263, 19.03943276465977164, 64.99890960531436690 ) ) ;
#44652=CARTESIAN_POINT ( 'NONE',  ( -21.55341960407610458, -5.719274019375992779, 31.45724293864769550 ) ) ;
#44653=CARTESIAN_POINT ( 'NONE',  ( 16.53943276465976808, -0.05219959533910856209, 113.7489096053143527 ) ) ;
#44654=CARTESIAN_POINT ( 'NONE',  ( 18.62759615963271287, -10.81492255796078972, 43.33224293864769550 ) ) ;
#44655=CARTESIAN_POINT ( 'NONE',  ( 16.55341960407618274, -4.379528057220086978, 86.04275706135236135 ) ) ;
#44656=CARTESIAN_POINT ( 'NONE',  ( -21.55341960407619339, 5.719274019375674811, 103.5427570613523613 ) ) ;
#44657=CARTESIAN_POINT ( 'NONE',  ( -16.53943276465976808, -0.05219959533934237506, 68.75109039468568994 ) ) ;
#44658=CARTESIAN_POINT ( 'NONE',  ( 19.03943276465977164, -0.05219959533909143690, 108.7489096053143527 ) ) ;
#44659=CARTESIAN_POINT ( 'NONE',  ( -12.06949235617739369, -12.14591786802326823, 54.37609039468568994 ) ) ;
#44660=CARTESIAN_POINT ( 'NONE',  ( -14.29746914071037622, -8.314922557961029526, 34.16775706135234714 ) ) ;
#44661=CARTESIAN_POINT ( 'NONE',  ( -19.02544592524342804, 5.153800228976336051, 111.0405762719810099 ) ) ;
#44662=CARTESIAN_POINT ( 'NONE',  ( -4.379528057220086978, -16.55341960407618274, 29.79275706135234358 ) ) ;
#44663=CARTESIAN_POINT ( 'NONE',  ( -13.89961937509977652, 13.97604488694528158, 35.62390960531435269 ) ) ;
#44664=CARTESIAN_POINT ( 'NONE',  ( -21.55341960407619339, 5.719274019375674811, 28.54275706135234358 ) ) ;
#44665=CARTESIAN_POINT ( 'NONE',  ( -8.224510206698735004, -14.34966873604973081, 24.58442372801901499 ) ) ;
#44666=CARTESIAN_POINT ( 'NONE',  ( 0.05219959533934541429, -16.53943276465976808, 80.00109039468568994 ) ) ;
#44668=CARTESIAN_POINT ( 'NONE',  ( -18.67979575497193778, 10.72451020669871902, 93.33442372801901854 ) ) ;
#44669=CARTESIAN_POINT ( 'NONE',  ( -9.474510206698720793, -16.51473224551083518, 99.58442372801900433 ) ) ;
#44670=CARTESIAN_POINT ( 'NONE',  ( -4.483927247898539470, -16.52544592524342804, 57.29057627198103120 ) ) ;
#44671=CARTESIAN_POINT ( 'NONE',  ( 0.05219959533910956823, 16.53943276465976808, 109.9989096053143527 ) ) ;
#44672=CARTESIAN_POINT ( 'NONE',  ( -19.05341960407617563, 5.049401038297882671, 53.54275706135231871 ) ) ;
#44673=CARTESIAN_POINT ( 'NONE',  ( 17.40861289039009918, -6.110651285853051284, 56.12767529172571557 ) ) ;
#44674=CARTESIAN_POINT ( 'NONE',  ( -0.05219959533937732626, 21.53943276465977519, 52.50109039468567573 ) ) ;
#44675=CARTESIAN_POINT ( 'NONE',  ( -19.03943276465977164, -0.05219959533935918106, 103.7510903946856757 ) ) ;
#44677=CARTESIAN_POINT ( 'NONE',  ( 9.564922557960805705, 16.46253265017160317, 109.5822429386476955 ) ) ;
#44678=CARTESIAN_POINT ( 'NONE',  ( 18.67979575497178502, 10.72451020669898547, 79.16557627198103830 ) ) ;
#44679=CARTESIAN_POINT ( 'NONE',  ( -13.89961937509957401, -13.97604488694547875, 99.37609039468567573 ) ) ;
#44680=CARTESIAN_POINT ( 'NONE',  ( 5.049401038298161559, -19.05341960407611168, 107.7072429386476955 ) ) ;
#44682=CARTESIAN_POINT ( 'NONE',  ( -8.224510206698948167, 14.34966873604960824, 110.4155762719810383 ) ) ;
#44683=CARTESIAN_POINT ( 'NONE',  ( 18.67979575497194134, -10.72451020669871369, 95.83442372801903275 ) ) ;
#44684=CARTESIAN_POINT ( 'NONE',  ( -19.03943276465977164, 0.05219959533909376836, 41.24890960531435269 ) ) ;
#44685=CARTESIAN_POINT ( 'NONE',  ( 21.55341960407619695, -5.719274019375665929, 56.04275706135235424 ) ) ;
#44686=CARTESIAN_POINT ( 'NONE',  ( -15.80617190586768217, 15.72974639402176855, 88.12609039468570415 ) ) ;
#44687=CARTESIAN_POINT ( 'NONE',  ( -8.314922557961024197, 14.29746914071037800, 102.9177570613523756 ) ) ;
#44688=CARTESIAN_POINT ( 'NONE',  ( -19.02544592524342804, 5.153800228976336051, 71.04057627198099567 ) ) ;
#44689=CARTESIAN_POINT ( 'NONE',  ( 21.52544592524334988, 5.823673210054432836, 41.45942372801901143 ) ) ;
#44690=CARTESIAN_POINT ( 'NONE',  ( -5.823673210054431948, 21.52544592524334988, 37.70942372801900433 ) ) ;
#44691=CARTESIAN_POINT ( 'NONE',  ( 19.02544592524334988, 5.153800228976608722, 66.45942372801899012 ) ) ;
#44692=CARTESIAN_POINT ( 'NONE',  ( 19.03943276465977164, -0.05219959533909143690, 93.74890960531435269 ) ) ;
#44693=CARTESIAN_POINT ( 'NONE',  ( 0.05219959533910956823, 16.53943276465976808, 109.9989096053143527 ) ) ;
#44694=CARTESIAN_POINT ( 'NONE',  ( -18.62759615963270932, 10.81492255796079327, 100.8322429386477097 ) ) ;
#44695=CARTESIAN_POINT ( 'NONE',  ( 16.53943276465976808, -0.05219959533910856209, 68.74890960531435269 ) ) ;
#44696=CARTESIAN_POINT ( 'NONE',  ( 9.474510206698729675, 16.51473224551082808, 22.08442372801899722 ) ) ;
#44697=CARTESIAN_POINT ( 'NONE',  ( 8.224510206698953496, -14.34966873604960469, 82.91557627198103830 ) ) ;
#44698=CARTESIAN_POINT ( 'NONE',  ( -5.049401038298153566, 19.05341960407611168, 30.20724293864768839 ) ) ;
#44699=CARTESIAN_POINT ( 'NONE',  ( -19.02544592524334988, -5.153800228976617603, 88.95942372801897591 ) ) ;
#44700=CARTESIAN_POINT ( 'NONE',  ( -8.314922557960811034, -14.29746914071050412, 52.08224293864768839 ) ) ;
#44701=CARTESIAN_POINT ( 'NONE',  ( -15.80617190586768217, 15.72974639402176855, 98.12609039468570415 ) ) ;
#44702=CARTESIAN_POINT ( 'NONE',  ( -13.97604488694527625, -13.89961937509977652, 91.87390960531432427 ) ) ;
#44703=CARTESIAN_POINT ( 'NONE',  ( 9.474510206698729675, 16.51473224551082808, 62.08442372801899722 ) ) ;
#44704=CARTESIAN_POINT ( 'NONE',  ( -21.53943276465977519, 0.05219959533907696930, 76.24890960531435269 ) ) ;
#44705=CARTESIAN_POINT ( 'NONE',  ( -21.53943276465977519, -0.05219959533937600094, 33.75109039468568284 ) ) ;
#44706=CARTESIAN_POINT ( 'NONE',  ( 12.06949235617739724, 12.14591786802326823, 31.87609039468567929 ) ) ;
#44707=CARTESIAN_POINT ( 'NONE',  ( -8.224510206698735004, -14.34966873604973081, 99.58442372801900433 ) ) ;
#44708=CARTESIAN_POINT ( 'NONE',  ( -19.02544592524342804, 5.153800228976336051, 31.04057627198102409 ) ) ;
#44709=CARTESIAN_POINT ( 'NONE',  ( -21.53943276465977519, -0.05219959533937600094, 18.75109039468568639 ) ) ;
#44710=CARTESIAN_POINT ( 'NONE',  ( -5.049401038298153566, 19.05341960407611168, 25.20724293864768484 ) ) ;
#44712=CARTESIAN_POINT ( 'NONE',  ( -16.52544592524335698, -4.483927247898792601, 43.95942372801902565 ) ) ;
#44713=CARTESIAN_POINT ( 'NONE',  ( -0.05219959533910754901, -16.53943276465976808, 77.49890960531433848 ) ) ;
#44714=CARTESIAN_POINT ( 'NONE',  ( -18.62759615963270932, 10.81492255796079327, 75.83224293864769550 ) ) ;
#44715=CARTESIAN_POINT ( 'NONE',  ( -12.14591786802309592, -12.06949235617757132, 26.87390960531435979 ) ) ;
#44716=CARTESIAN_POINT ( 'NONE',  ( -14.34966873604972548, 8.224510206698743886, 48.33442372801902565 ) ) ;
#44717=CARTESIAN_POINT ( 'NONE',  ( 16.46253265017160672, -9.564922557960803928, 43.33224293864769550 ) ) ;
#44718=CARTESIAN_POINT ( 'NONE',  ( -16.52544592524335698, -4.483927247898792601, 83.95942372801900433 ) ) ;
#44719=CARTESIAN_POINT ( 'NONE',  ( -16.46253265017146816, -9.564922557961047289, 69.16775706135233293 ) ) ;
#44720=CARTESIAN_POINT ( 'NONE',  ( 10.72451020669898902, -18.67979575497178502, 67.91557627198102409 ) ) ;
#44721=CARTESIAN_POINT ( 'NONE',  ( -16.53943276465976808, -0.05219959533934237506, 108.7510903946857042 ) ) ;
#44724=CARTESIAN_POINT ( 'NONE',  ( 18.62759615963271287, -10.81492255796078972, 43.33224293864769550 ) ) ;
#44726=ORIENTED_EDGE ( 'NONE', *, *, #45727, .F. ) ;
#44727=CARTESIAN_POINT ( 'NONE',  ( 4.379528057220092307, 16.55341960407617563, 92.29275706135236135 ) ) ;
#44729=CARTESIAN_POINT ( 'NONE',  ( 19.05341960407611168, 5.049401038298154454, 113.9572429386477097 ) ) ;
#44730=CARTESIAN_POINT ( 'NONE',  ( 17.50000000000001066, -3.242565516153302241, 102.5000000000090807 ) ) ;
#44731=CARTESIAN_POINT ( 'NONE',  ( 21.53943276465977519, -0.05219959533907433946, 68.74890960531435269 ) ) ;
#44732=CARTESIAN_POINT ( 'NONE',  ( -8.224510206698735004, -14.34966873604973081, 104.5844237280190185 ) ) ;
#44733=CARTESIAN_POINT ( 'NONE',  ( -0.05219959533934338120, 16.53943276465976808, 27.50109039468567929 ) ) ;
#44734=CARTESIAN_POINT ( 'NONE',  ( 16.51473224551069308, 9.474510206698969483, 24.16557627198102765 ) ) ;
#44735=CARTESIAN_POINT ( 'NONE',  ( -4.379528057220086978, -16.55341960407618274, 24.79275706135235779 ) ) ;
#44736=CARTESIAN_POINT ( 'NONE',  ( -5.049401038298153566, 19.05341960407611168, 60.20724293864768129 ) ) ;
#44738=CARTESIAN_POINT ( 'NONE',  ( -19.03943276465977164, 0.05219959533909376836, 101.2489096053143669 ) ) ;
#44739=CARTESIAN_POINT ( 'NONE',  ( 16.53943276465976808, 0.05219959533934440121, 91.25109039468568994 ) ) ;
#44740=CARTESIAN_POINT ( 'NONE',  ( 19.05341960407617918, -5.049401038297876454, 86.04275706135233293 ) ) ;
#44741=CARTESIAN_POINT ( 'NONE',  ( -19.03943276465977164, -0.05219959533935918106, 28.75109039468566507 ) ) ;
#44742=CARTESIAN_POINT ( 'NONE',  ( 18.62759615963271287, -10.81492255796078972, 78.33224293864770971 ) ) ;
#44743=CARTESIAN_POINT ( 'NONE',  ( -8.224510206698735004, -14.34966873604973081, 104.5844237280190185 ) ) ;
#44744=CARTESIAN_POINT ( 'NONE',  ( -5.049401038297874678, -19.05341960407617918, 94.79275706135230450 ) ) ;
#44745=CARTESIAN_POINT ( 'NONE',  ( -9.474510206698964154, 16.51473224551069663, 45.41557627198103120 ) ) ;
#44746=CARTESIAN_POINT ( 'NONE',  ( -19.02544592524342804, 5.153800228976336051, 91.04057627198100988 ) ) ;
#44747=CARTESIAN_POINT ( 'NONE',  ( 15.80617190586769283, -15.72974639402175789, 55.62609039468568284 ) ) ;
#44748=CARTESIAN_POINT ( 'NONE',  ( -16.46253265017160317, 9.564922557960807481, 45.83224293864769550 ) ) ;
#44749=CARTESIAN_POINT ( 'NONE',  ( -16.31925111598453881, -7.325300261831592330, 84.83575461032749843 ) ) ;
#44750=CARTESIAN_POINT ( 'NONE',  ( 4.483927247898545687, 16.52544592524342804, 79.79057627198102409 ) ) ;
#44751=CARTESIAN_POINT ( 'NONE',  ( -10.72451020669898014, 18.67979575497178502, 75.41557627198102409 ) ) ;
#44754=CARTESIAN_POINT ( 'NONE',  ( -5.153800228976607833, 19.02544592524334988, 37.70942372801899722 ) ) ;
#44757=CARTESIAN_POINT ( 'NONE',  ( -13.89961937509977652, 13.97604488694528158, 75.62390960531438111 ) ) ;
#44758=CARTESIAN_POINT ( 'NONE',  ( 5.153800228976335163, 19.02544592524342804, 89.79057627198102409 ) ) ;
#44760=CARTESIAN_POINT ( 'NONE',  ( -12.14591786802326823, 12.06949235617739902, 68.12609039468567573 ) ) ;
#44761=CARTESIAN_POINT ( 'NONE',  ( -17.72662750342725957, -5.500000000000095923, 66.40179492283743912 ) ) ;
#44762=CARTESIAN_POINT ( 'NONE',  ( 19.05341960407617918, -5.049401038297876454, 31.04275706135232227 ) ) ;
#44763=CARTESIAN_POINT ( 'NONE',  ( -16.31925111598457079, 7.325300261831543480, 110.1642453896725442 ) ) ;
#44764=CARTESIAN_POINT ( 'NONE',  ( 19.05341960407611168, 5.049401038298154454, 113.9572429386477097 ) ) ;
#44765=CARTESIAN_POINT ( 'NONE',  ( -0.05219959533934338120, 16.53943276465976808, 87.50109039468568994 ) ) ;
#44767=CARTESIAN_POINT ( 'NONE',  ( -14.34966873604972548, 8.224510206698743886, 73.33442372801901854 ) ) ;
#44768=CARTESIAN_POINT ( 'NONE',  ( -16.29526858892872809, 7.335722546920264264, 29.20329402199793378 ) ) ;
#44769=CARTESIAN_POINT ( 'NONE',  ( 8.314922557961029526, -14.29746914071037800, 60.41775706135235424 ) ) ;
#44771=CARTESIAN_POINT ( 'NONE',  ( -18.62759615963255300, -10.81492255796106328, 69.16775706135234714 ) ) ;
#44772=CARTESIAN_POINT ( 'NONE',  ( -19.02544592524334988, -5.153800228976617603, 78.95942372801900433 ) ) ;
#44773=CARTESIAN_POINT ( 'NONE',  ( -9.474510206698720793, -16.51473224551083518, 29.58442372801900433 ) ) ;
#44774=CARTESIAN_POINT ( 'NONE',  ( -16.46253265017160317, 9.564922557960807481, 45.83224293864769550 ) ) ;
#44775=CARTESIAN_POINT ( 'NONE',  ( 0.05219959533909260263, 19.03943276465977164, 44.99890960531435979 ) ) ;
#44776=CARTESIAN_POINT ( 'NONE',  ( 16.54732454198001790, -7.207534646770589859, 22.94022044411182293 ) ) ;
#44777=CARTESIAN_POINT ( 'NONE',  ( 21.52544592524344225, -5.823673210054117533, 73.54057627198102409 ) ) ;
#44778=CARTESIAN_POINT ( 'NONE',  ( -18.62759615963270932, 10.81492255796079327, 25.83224293864769194 ) ) ;
#44779=CARTESIAN_POINT ( 'NONE',  ( -19.03943276465977164, 0.05219959533909376836, 21.24890960531436335 ) ) ;
#44780=CARTESIAN_POINT ( 'NONE',  ( 8.314922557961029526, -14.29746914071037800, 45.41775706135234003 ) ) ;
#44783=CARTESIAN_POINT ( 'NONE',  ( -15.72974639402197994, 15.80617190586746368, 115.6239096053143669 ) ) ;
#44784=CARTESIAN_POINT ( 'NONE',  ( -8.224510206698948167, 14.34966873604960824, 50.41557627198103120 ) ) ;
#44786=CARTESIAN_POINT ( 'NONE',  ( -5.153800228976607833, 19.02544592524334988, 107.7094237280189759 ) ) ;
#44787=CARTESIAN_POINT ( 'NONE',  ( -16.46253265017146816, -9.564922557961047289, 34.16775706135233293 ) ) ;
#44788=CARTESIAN_POINT ( 'NONE',  ( 8.314922557960818139, 14.29746914071049879, 39.58224293864769550 ) ) ;
#44789=CARTESIAN_POINT ( 'NONE',  ( -10.72451020669870658, -18.67979575497194134, 24.58442372801901499 ) ) ;
#44790=CARTESIAN_POINT ( 'NONE',  ( 17.50000000000000000, 5.499999999999997335, 120.0000000000000142 ) ) ;
#44791=CARTESIAN_POINT ( 'NONE',  ( -21.53943276465977519, 0.05219959533907696930, 66.24890960531436690 ) ) ;
#44792=CARTESIAN_POINT ( 'NONE',  ( 13.89961937509977652, -13.97604488694527269, 93.12390960531436690 ) ) ;
#44793=CARTESIAN_POINT ( 'NONE',  ( 16.52544592524342804, -4.483927247898539470, 43.54057627198103830 ) ) ;
#44794=CARTESIAN_POINT ( 'NONE',  ( -13.97604488694527625, -13.89961937509977652, 101.8739096053143811 ) ) ;
#44796=CARTESIAN_POINT ( 'NONE',  ( -19.02544592524334988, -5.153800228976617603, 53.95942372801898301 ) ) ;
#44797=CARTESIAN_POINT ( 'NONE',  ( -21.55341960407610458, -5.719274019375992779, 96.45724293864770971 ) ) ;
#44798=CARTESIAN_POINT ( 'NONE',  ( 13.89961937509977652, -13.97604488694527269, 43.12390960531434558 ) ) ;
#44799=CARTESIAN_POINT ( 'NONE',  ( 14.34966873604960469, 8.224510206698951720, 109.1655762719810383 ) ) ;
#44800=CARTESIAN_POINT ( 'NONE',  ( -15.72974639402176322, -15.80617190586768395, 44.37609039468567573 ) ) ;
#44802=CARTESIAN_POINT ( 'NONE',  ( 4.379528057220339221, -16.55341960407611168, 22.70724293864769194 ) ) ;
#44803=CARTESIAN_POINT ( 'NONE',  ( 19.02544592524343514, -5.153800228976328945, 48.54057627198103120 ) ) ;
#44804=CARTESIAN_POINT ( 'NONE',  ( -0.05219959533909027116, -19.03943276465977164, 102.4989096053143669 ) ) ;
#44805=CARTESIAN_POINT ( 'NONE',  ( 15.80617190586746368, 15.72974639402197994, 69.37390960531436690 ) ) ;
#44807=CARTESIAN_POINT ( 'NONE',  ( 5.153800228976335163, 19.02544592524342804, 44.79057627198103830 ) ) ;
#44808=CARTESIAN_POINT ( 'NONE',  ( 0.05219959533907565091, 21.53943276465977519, 49.99890960531437401 ) ) ;
#44809=CARTESIAN_POINT ( 'NONE',  ( -21.55341960407619339, 5.719274019375674811, 88.54275706135236135 ) ) ;
#44811=CARTESIAN_POINT ( 'NONE',  ( -14.34966873604972548, 8.224510206698743886, 83.33442372801903275 ) ) ;
#44812=CARTESIAN_POINT ( 'NONE',  ( 14.29746914071049879, -8.314922557960816363, 63.33224293864770260 ) ) ;
#44813=CARTESIAN_POINT ( 'NONE',  ( -8.224510206698735004, -14.34966873604973081, 89.58442372801901854 ) ) ;
#44814=CARTESIAN_POINT ( 'NONE',  ( 13.89961937509977652, -13.97604488694527269, 73.12390960531436690 ) ) ;
#44816=CARTESIAN_POINT ( 'NONE',  ( 13.97604488694548053, -13.89961937509957401, 20.62609039468567573 ) ) ;
#44817=CARTESIAN_POINT ( 'NONE',  ( -4.379528057220086978, -16.55341960407618274, 84.79275706135234714 ) ) ;
#44818=CARTESIAN_POINT ( 'NONE',  ( -18.62759615963255300, -10.81492255796106328, 109.1677570613523613 ) ) ;
#44819=CARTESIAN_POINT ( 'NONE',  ( 5.153800228976335163, 19.02544592524342804, 79.79057627198102409 ) ) ;
#44820=CARTESIAN_POINT ( 'NONE',  ( -0.05219959533907301413, -21.53943276465977519, 42.49890960531435979 ) ) ;
#44821=CARTESIAN_POINT ( 'NONE',  ( -0.05219959533934338120, 16.53943276465976808, 22.50109039468567573 ) ) ;
#44822=CARTESIAN_POINT ( 'NONE',  ( -21.55341960407619339, 5.719274019375674811, 88.54275706135236135 ) ) ;
#44823=CARTESIAN_POINT ( 'NONE',  ( -16.52544592524335698, -4.483927247898792601, 68.95942372801901854 ) ) ;
#44824=CARTESIAN_POINT ( 'NONE',  ( 18.67979575497178502, 10.72451020669898547, 109.1655762719810383 ) ) ;
#44825=CARTESIAN_POINT ( 'NONE',  ( -13.97604488694547697, 13.89961937509957934, 108.1260903946856331 ) ) ;
#44826=CARTESIAN_POINT ( 'NONE',  ( 9.474510206698971260, -16.51473224551069308, 97.91557627198102409 ) ) ;
#44827=CARTESIAN_POINT ( 'NONE',  ( -12.14591786802326823, 12.06949235617739902, 28.12609039468568284 ) ) ;
#44828=CARTESIAN_POINT ( 'NONE',  ( 16.46253265017160672, -9.564922557960803928, 43.33224293864769550 ) ) ;
#44829=CARTESIAN_POINT ( 'NONE',  ( 14.29746914071037800, 8.314922557961029526, 36.66775706135234714 ) ) ;
#44830=CARTESIAN_POINT ( 'NONE',  ( -16.55341960407611168, -4.379528057220339221, 76.45724293864769550 ) ) ;
#44831=CARTESIAN_POINT ( 'NONE',  ( -16.55341960407617563, 4.379528057220093196, 83.54275706135234714 ) ) ;
#44833=CARTESIAN_POINT ( 'NONE',  ( -5.823673210054431948, 21.52544592524334988, 32.70942372801900433 ) ) ;
#44834=CARTESIAN_POINT ( 'NONE',  ( -9.564922557960796823, -16.46253265017161027, 62.08224293864769550 ) ) ;
#44835=CARTESIAN_POINT ( 'NONE',  ( -19.02544592524342804, 5.153800228976336051, 86.04057627198103830 ) ) ;
#44836=CARTESIAN_POINT ( 'NONE',  ( -0.05219959533934338120, 16.53943276465976808, 82.50109039468568994 ) ) ;
#44840=CARTESIAN_POINT ( 'NONE',  ( -9.474510206698720793, -16.51473224551083518, 29.58442372801900433 ) ) ;
#44841=CARTESIAN_POINT ( 'NONE',  ( 19.02544592524343514, -5.153800228976328945, 93.54057627198102409 ) ) ;
#44842=CARTESIAN_POINT ( 'NONE',  ( -19.02544592524342804, 5.153800228976336051, 51.04057627198103120 ) ) ;
#44843=CARTESIAN_POINT ( 'NONE',  ( 5.153800228976335163, 19.02544592524342804, 114.7905762719810241 ) ) ;
#44844=ORIENTED_EDGE ( 'NONE', *, *, #20020, .F. ) ;
#44845=CARTESIAN_POINT ( 'NONE',  ( 14.34966873604972726, -8.224510206698740333, 30.83442372801902209 ) ) ;
#44846=CARTESIAN_POINT ( 'NONE',  ( 0.05219959533936267826, -19.03943276465977164, 55.00109039468566863 ) ) ;
#44847=CARTESIAN_POINT ( 'NONE',  ( 4.483927247898790824, -16.52544592524335698, 40.20942372801901854 ) ) ;
#44848=CARTESIAN_POINT ( 'NONE',  ( -0.05219959533909027116, -19.03943276465977164, 107.4989096053143527 ) ) ;
#44849=CARTESIAN_POINT ( 'NONE',  ( -19.02544592524342804, 5.153800228976336051, 71.04057627198099567 ) ) ;
#44850=CARTESIAN_POINT ( 'NONE',  ( 10.81492255796078972, 18.62759615963270932, 94.58224293864769550 ) ) ;
#44851=CARTESIAN_POINT ( 'NONE',  ( -5.049401038297874678, -19.05341960407617918, 59.79275706135231871 ) ) ;
#44852=CARTESIAN_POINT ( 'NONE',  ( -19.02544592524342804, 5.153800228976336051, 86.04057627198103830 ) ) ;
#44853=CARTESIAN_POINT ( 'NONE',  ( -19.05341960407611168, -5.049401038298163336, 21.45724293864768839 ) ) ;
#44854=CARTESIAN_POINT ( 'NONE',  ( -13.97604488694527625, -13.89961937509977652, 61.87390960531435979 ) ) ;
#44855=CARTESIAN_POINT ( 'NONE',  ( -16.55341960407617563, 4.379528057220093196, 108.5427570613523756 ) ) ;
#44856=CARTESIAN_POINT ( 'NONE',  ( 9.564922557960805705, 16.46253265017160317, 69.58224293864770971 ) ) ;
#44857=CARTESIAN_POINT ( 'NONE',  ( 13.89961937509957401, 13.97604488694547697, 36.87609039468565442 ) ) ;
#44858=B_SPLINE_CURVE_WITH_KNOTS ( 'NONE', 3,
 ( #76463, #64280, #121969, #60295, #183661, #123939, #109781, #79443, #16786, #95600, #62271, #108787, #94607, #168476, #46126, #137143, #45146, #93611, #107780, #198831, #78436, #169465, #106802, #47129, #157285, #75470, #29974, #1601, #91613, #14802, #185637, #138140 ),
 .UNSPECIFIED., .F., .F.,
 ( 4, 2, 2, 2, 2, 2, 2, 2, 2, 2, 2, 2, 2, 2, 2, 4 ),
 ( 8.673617379884034509E-19, 0.0003712461730036735507, 0.0007424923460073462340, 0.001113738519011018809, 0.001484984692014691601, 0.002227477038022048893, 0.002598723211025715830, 0.002969969384029382767, 0.003341215557033050138, 0.003712461730036717509, 0.004083707903040385313, 0.004454954076044052684, 0.004826200249047720055, 0.005197446422051387425, 0.005568692595055054796, 0.005939938768058721300 ),
 .UNSPECIFIED. ) ;
#44859=CARTESIAN_POINT ( 'NONE',  ( -4.483927247898539470, -16.52544592524342804, 72.29057627198102409 ) ) ;
#44860=CARTESIAN_POINT ( 'NONE',  ( -21.52544592524334988, -5.823673210054445271, 93.95942372801903275 ) ) ;
#44861=CARTESIAN_POINT ( 'NONE',  ( 9.474510206698971260, -16.51473224551069308, 32.91557627198102409 ) ) ;
#44862=CARTESIAN_POINT ( 'NONE',  ( 8.314922557961029526, -14.29746914071037800, 55.41775706135234714 ) ) ;
#44863=CARTESIAN_POINT ( 'NONE',  ( -4.379528057220328563, 16.55341960407611168, 40.20724293864769550 ) ) ;
#44864=CARTESIAN_POINT ( 'NONE',  ( 21.55341960407619695, -5.719274019375665929, 91.04275706135236135 ) ) ;
#44865=CARTESIAN_POINT ( 'NONE',  ( 16.46253265017160672, -9.564922557960803928, 88.33224293864769550 ) ) ;
#44866=CARTESIAN_POINT ( 'NONE',  ( -19.05341960407611168, -5.049401038298163336, 96.45724293864769550 ) ) ;
#44867=CARTESIAN_POINT ( 'NONE',  ( 12.06949235617757843, -12.14591786802309237, 103.1239096053143811 ) ) ;
#44868=CARTESIAN_POINT ( 'NONE',  ( -8.224510206698948167, 14.34966873604960824, 80.41557627198103830 ) ) ;
#44869=CARTESIAN_POINT ( 'NONE',  ( -18.62759615963270932, 10.81492255796079327, 85.83224293864768129 ) ) ;
#44870=CARTESIAN_POINT ( 'NONE',  ( 19.05341960407611168, 5.049401038298154454, 93.95724293864769550 ) ) ;
#44871=CARTESIAN_POINT ( 'NONE',  ( 15.80617190586746368, 15.72974639402197994, 104.3739096053143669 ) ) ;
#44872=CARTESIAN_POINT ( 'NONE',  ( -19.02544592524342804, 5.153800228976336051, 96.04057627198103830 ) ) ;
#44873=CARTESIAN_POINT ( 'NONE',  ( -18.22780087662123094, -5.499999999999984901, 91.48459894673894155 ) ) ;
#44874=CARTESIAN_POINT ( 'NONE',  ( 16.53943276465976808, -0.05219959533910856209, 93.74890960531436690 ) ) ;
#44875=CARTESIAN_POINT ( 'NONE',  ( 16.46253265017160672, -9.564922557960803928, 63.33224293864769550 ) ) ;
#44876=CARTESIAN_POINT ( 'NONE',  ( 10.81492255796078972, 18.62759615963270932, 64.58224293864769550 ) ) ;
#44877=CARTESIAN_POINT ( 'NONE',  ( 17.12812012977024878, -6.668231424566041454, 26.14051240676857191 ) ) ;
#44878=CARTESIAN_POINT ( 'NONE',  ( -8.314922557961024197, 14.29746914071037800, 112.9177570613523329 ) ) ;
#44879=CARTESIAN_POINT ( 'NONE',  ( 17.50000000000000000, -5.500000000000000888, 120.0000000000000142 ) ) ;
#44880=CARTESIAN_POINT ( 'NONE',  ( -12.06949235617739369, -12.14591786802326823, 19.37609039468568639 ) ) ;
#44881=CARTESIAN_POINT ( 'NONE',  ( 14.34966873604960469, 8.224510206698951720, 84.16557627198103830 ) ) ;
#44882=CARTESIAN_POINT ( 'NONE',  ( -17.48847506799967633, -5.747544572773783500, 94.17302562156720569 ) ) ;
#44883=CARTESIAN_POINT ( 'NONE',  ( 19.05341960407611168, 5.049401038298154454, 78.95724293864769550 ) ) ;
#44884=CARTESIAN_POINT ( 'NONE',  ( -9.474510206698964154, 16.51473224551069663, 40.41557627198103120 ) ) ;
#44885=CARTESIAN_POINT ( 'NONE',  ( -12.06949235617756955, 12.14591786802309770, 60.62390960531437401 ) ) ;
#44886=CARTESIAN_POINT ( 'NONE',  ( 9.564922557960805705, 16.46253265017160317, 109.5822429386476955 ) ) ;
#44887=CARTESIAN_POINT ( 'NONE',  ( 5.049401038297881783, 19.05341960407617563, 102.2927570613523045 ) ) ;
#44888=CARTESIAN_POINT ( 'NONE',  ( -5.049401038298153566, 19.05341960407611168, 95.20724293864770971 ) ) ;
#44889=CARTESIAN_POINT ( 'NONE',  ( 10.72451020669898902, -18.67979575497178502, 72.91557627198103830 ) ) ;
#44890=CARTESIAN_POINT ( 'NONE',  ( 0.05219959533934541429, -16.53943276465976808, 70.00109039468568994 ) ) ;
#44891=CARTESIAN_POINT ( 'NONE',  ( -5.153800228976607833, 19.02544592524335343, 107.7094237280189901 ) ) ;
#44892=CARTESIAN_POINT ( 'NONE',  ( -9.564922557960796823, -16.46253265017161027, 77.08224293864769550 ) ) ;
#44893=CARTESIAN_POINT ( 'NONE',  ( -21.55341960407610458, -5.719274019375992779, 86.45724293864770971 ) ) ;
#44894=CARTESIAN_POINT ( 'NONE',  ( -9.474510206698720793, -16.51473224551083518, 109.5844237280190043 ) ) ;
#44895=CARTESIAN_POINT ( 'NONE',  ( -14.29746914071049879, 8.314922557960819915, 35.83224293864768839 ) ) ;
#44896=CARTESIAN_POINT ( 'NONE',  ( -21.55341960407619339, 5.719274019375674811, 53.54275706135234714 ) ) ;
#44898=CARTESIAN_POINT ( 'NONE',  ( -16.55341960407617563, 4.379528057220093196, 83.54275706135234714 ) ) ;
#44899=CARTESIAN_POINT ( 'NONE',  ( -5.153800228976328057, -19.02544592524343514, 107.2905762719810383 ) ) ;
#44901=CARTESIAN_POINT ( 'NONE',  ( -16.52216118717209170, 7.221426719304500530, 78.92400978953006074 ) ) ;
#44902=CARTESIAN_POINT ( 'NONE',  ( 14.34966873604972726, -8.224510206698740333, 100.8344237280190185 ) ) ;
#44903=CARTESIAN_POINT ( 'NONE',  ( 16.55341960407618274, -4.379528057220086978, 41.04275706135236135 ) ) ;
#44904=CARTESIAN_POINT ( 'NONE',  ( -5.049401038298153566, 19.05341960407611168, 60.20724293864768129 ) ) ;
#44905=CARTESIAN_POINT ( 'NONE',  ( -9.474510206698964154, 16.51473224551069663, 75.41557627198103830 ) ) ;
#44906=CARTESIAN_POINT ( 'NONE',  ( -21.55341960407619339, 5.719274019375674811, 63.54275706135234003 ) ) ;
#44907=CARTESIAN_POINT ( 'NONE',  ( -8.314922557961024197, 14.29746914071037800, 57.91775706135234714 ) ) ;
#44908=CARTESIAN_POINT ( 'NONE',  ( 8.224510206698953496, -14.34966873604960469, 37.91557627198102409 ) ) ;
#44909=CARTESIAN_POINT ( 'NONE',  ( 19.02544592524343514, -5.153800228976328945, 43.54057627198103120 ) ) ;
#44910=CARTESIAN_POINT ( 'NONE',  ( 13.97604488694527802, 13.89961937509977652, 44.37390960531435269 ) ) ;
#44911=CARTESIAN_POINT ( 'NONE',  ( 12.06949235617739724, 12.14591786802326823, 41.87609039468568284 ) ) ;
#44913=CARTESIAN_POINT ( 'NONE',  ( 16.51473224551083163, -9.474510206698727899, 90.83442372801900433 ) ) ;
#44914=CARTESIAN_POINT ( 'NONE',  ( -8.314922557960811034, -14.29746914071050412, 102.0822429386476955 ) ) ;
#44915=CARTESIAN_POINT ( 'NONE',  ( -13.89961937509977652, 13.97604488694528158, 55.62390960531434558 ) ) ;
#44916=CARTESIAN_POINT ( 'NONE',  ( 9.564922557961047289, -16.46253265017146816, 85.41775706135233293 ) ) ;
#44918=CARTESIAN_POINT ( 'NONE',  ( -15.80617190586768217, 15.72974639402176855, 88.12609039468570415 ) ) ;
#44919=CARTESIAN_POINT ( 'NONE',  ( -16.53943276465976808, -0.05219959533934237506, 73.75109039468567573 ) ) ;
#44921=CARTESIAN_POINT ( 'NONE',  ( -10.72451020669898014, 18.67979575497178502, 55.41557627198102409 ) ) ;
#44922=CARTESIAN_POINT ( 'NONE',  ( 4.483927247898790824, -16.52544592524335698, 35.20942372801901854 ) ) ;
#44923=CARTESIAN_POINT ( 'NONE',  ( -19.52837319214027545, 5.499999999999899636, 69.60471352585538796 ) ) ;
#44924=CARTESIAN_POINT ( 'NONE',  ( -9.564922557961040184, 16.46253265017147172, 42.91775706135234003 ) ) ;
#44925=CARTESIAN_POINT ( 'NONE',  ( 5.153800228976335163, 19.02544592524342804, 94.79057627198103830 ) ) ;
#44926=CARTESIAN_POINT ( 'NONE',  ( -13.97604488694527625, -13.89961937509977652, 21.87390960531435979 ) ) ;
#44927=CARTESIAN_POINT ( 'NONE',  ( 9.474510206698971260, -16.51473224551069308, 57.91557627198103120 ) ) ;
#44929=CARTESIAN_POINT ( 'NONE',  ( 18.62759615963255655, 10.81492255796105972, 71.66775706135234714 ) ) ;
#44931=CARTESIAN_POINT ( 'NONE',  ( -16.51473224551082808, 9.474510206698731452, 28.33442372801900433 ) ) ;
#44932=CARTESIAN_POINT ( 'NONE',  ( 15.80617190586769283, -15.72974639402175789, 110.6260903946857042 ) ) ;
#44933=CARTESIAN_POINT ( 'NONE',  ( 8.224510206698953496, -14.34966873604960469, 47.91557627198102409 ) ) ;
#44934=CARTESIAN_POINT ( 'NONE',  ( -16.46253265017160317, 9.564922557960807481, 50.83224293864770260 ) ) ;
#44935=CARTESIAN_POINT ( 'NONE',  ( 16.46253265017160672, -9.564922557960803928, 103.3322429386476955 ) ) ;
#44936=CARTESIAN_POINT ( 'NONE',  ( 15.72974639402176855, 15.80617190586768217, 76.87609039468567573 ) ) ;
#44937=CARTESIAN_POINT ( 'NONE',  ( -9.474510206698964154, 16.51473224551069663, 60.41557627198102409 ) ) ;
#44938=EDGE_CURVE ( 'NONE', #10027, #114473, #130169, .T. ) ;
#44939=CARTESIAN_POINT ( 'NONE',  ( -21.52544592524334988, -5.823673210054445271, 73.95942372801901854 ) ) ;
#44940=CARTESIAN_POINT ( 'NONE',  ( -18.62759615963270932, 10.81492255796079327, 40.83224293864769550 ) ) ;
#44941=B_SPLINE_CURVE_WITH_KNOTS ( 'NONE', 3,
 ( #168687, #30188, #42386, #91830, #104049, #165729, #153523, #15020, #76681, #184864, #88873, #28232, #58538, #89872, #12065, #43372, #13044, #74711 ),
 .UNSPECIFIED., .F., .F.,
 ( 4, 2, 2, 2, 2, 2, 2, 2, 4 ),
 ( 8.542522420166516410E-18, 0.0007580895335617857762, 0.001516179067123562879, 0.001895223833904452785, 0.002274268600685342909, 0.002463790984075790898, 0.002653313367466239320, 0.002842835750856687743, 0.003032358134247136166 ),
 .UNSPECIFIED. ) ;
#44942=CARTESIAN_POINT ( 'NONE',  ( 5.823673210054444382, -21.52544592524334988, 40.20942372801901854 ) ) ;
#44943=CARTESIAN_POINT ( 'NONE',  ( -16.51473224551082808, 9.474510206698731452, 63.33442372801900433 ) ) ;
#44944=CARTESIAN_POINT ( 'NONE',  ( 13.97604488694527802, 13.89961937509977652, 34.37390960531436690 ) ) ;
#44945=CARTESIAN_POINT ( 'NONE',  ( -19.05341960407611168, -5.049401038298163336, 76.45724293864769550 ) ) ;
#44946=CARTESIAN_POINT ( 'NONE',  ( -12.14591786802326823, 12.06949235617739902, 33.12609039468569705 ) ) ;
#44947=CARTESIAN_POINT ( 'NONE',  ( -16.55341960407611168, -4.379528057220339221, 91.45724293864769550 ) ) ;
#44948=CARTESIAN_POINT ( 'NONE',  ( 5.049401038298161559, -19.05341960407611168, 57.70724293864769550 ) ) ;
#44949=CARTESIAN_POINT ( 'NONE',  ( -21.52544592524343514, 5.823673210054127303, 36.04057627198102409 ) ) ;
#44950=CARTESIAN_POINT ( 'NONE',  ( 16.51473224551083163, -9.474510206698727899, 110.8344237280190043 ) ) ;
#44951=CARTESIAN_POINT ( 'NONE',  ( -21.52544592524334988, -5.823673210054445271, 18.95942372801901143 ) ) ;
#44952=CARTESIAN_POINT ( 'NONE',  ( -18.67979575497193778, 10.72451020669871902, 68.33442372801900433 ) ) ;
#44953=CARTESIAN_POINT ( 'NONE',  ( 16.55341960407618274, -4.379528057220086978, 66.04275706135236135 ) ) ;
#44954=CARTESIAN_POINT ( 'NONE',  ( 0.05219959533934541429, -16.53943276465976808, 70.00109039468568994 ) ) ;
#44955=CARTESIAN_POINT ( 'NONE',  ( 5.153800228976335163, 19.02544592524342804, 59.79057627198100988 ) ) ;
#44956=CARTESIAN_POINT ( 'NONE',  ( 0.05219959533934541429, -16.53943276465976808, 85.00109039468568994 ) ) ;
#44957=CARTESIAN_POINT ( 'NONE',  ( 19.02544592524334988, 5.153800228976608722, 36.45942372801900433 ) ) ;
#44958=CARTESIAN_POINT ( 'NONE',  ( -18.62759615963255300, -10.81492255796106328, 24.16775706135235424 ) ) ;
#44959=CARTESIAN_POINT ( 'NONE',  ( 16.55341960407611168, 4.379528057220329451, 58.95724293864770971 ) ) ;
#44960=CARTESIAN_POINT ( 'NONE',  ( -16.46253265017160317, 9.564922557960807481, 80.83224293864769550 ) ) ;
#44961=CARTESIAN_POINT ( 'NONE',  ( 12.06949235617739724, 12.14591786802326823, 86.87609039468568994 ) ) ;
#44962=CARTESIAN_POINT ( 'NONE',  ( 10.72451020669871369, 18.67979575497193778, 62.08442372801901143 ) ) ;
#44963=CARTESIAN_POINT ( 'NONE',  ( 12.06949235617739724, 12.14591786802326823, 31.87609039468567929 ) ) ;
#44964=CARTESIAN_POINT ( 'NONE',  ( -15.72974639402176322, -15.80617190586768395, 19.37609039468568639 ) ) ;
#44965=CARTESIAN_POINT ( 'NONE',  ( 12.06949235617757843, -12.14591786802309237, 58.12390960531435979 ) ) ;
#44966=ORIENTED_EDGE ( 'NONE', *, *, #136135, .T. ) ;
#44967=CARTESIAN_POINT ( 'NONE',  ( -21.55341960407610458, -5.719274019375992779, 101.4572429386476955 ) ) ;
#44968=CARTESIAN_POINT ( 'NONE',  ( 16.52544592524342804, -4.483927247898539470, 43.54057627198103830 ) ) ;
#44971=CARTESIAN_POINT ( 'NONE',  ( 5.049401038298161559, -19.05341960407611168, 112.7072429386476813 ) ) ;
#44972=CARTESIAN_POINT ( 'NONE',  ( -15.72974639402176322, -15.80617190586768395, 34.37609039468568284 ) ) ;
#44973=CARTESIAN_POINT ( 'NONE',  ( -4.483927247898539470, -16.52544592524342804, 52.29057627198102409 ) ) ;
#44974=CARTESIAN_POINT ( 'NONE',  ( -13.97604488694527625, -13.89961937509977652, 66.87390960531436690 ) ) ;
#44975=CARTESIAN_POINT ( 'NONE',  ( 5.049401038297881783, 19.05341960407617563, 62.29275706135234003 ) ) ;
#44976=CARTESIAN_POINT ( 'NONE',  ( -13.97604488694527625, -13.89961937509977652, 91.87390960531432427 ) ) ;
#44977=CARTESIAN_POINT ( 'NONE',  ( -21.55341960407610458, -5.719274019375992779, 51.45724293864770260 ) ) ;
#44979=CARTESIAN_POINT ( 'NONE',  ( -0.05219959533909027116, -19.03943276465977164, 62.49890960531435979 ) ) ;
#44980=CARTESIAN_POINT ( 'NONE',  ( -16.55341960407617563, 4.379528057220093196, 43.54275706135235424 ) ) ;
#44981=CARTESIAN_POINT ( 'NONE',  ( 16.51473224551083163, -9.474510206698727899, 65.83442372801900433 ) ) ;
#44982=CARTESIAN_POINT ( 'NONE',  ( 21.53943276465977519, -0.05219959533907433946, 108.7489096053143669 ) ) ;
#44983=CARTESIAN_POINT ( 'NONE',  ( 16.52544592524342804, -4.483927247898539470, 48.54057627198103120 ) ) ;
#44985=CARTESIAN_POINT ( 'NONE',  ( -9.564922557960796823, -16.46253265017161027, 97.08224293864769550 ) ) ;
#44986=CARTESIAN_POINT ( 'NONE',  ( 15.72974639402199770, -15.80617190586745480, 78.12390960531436690 ) ) ;
#44987=CARTESIAN_POINT ( 'NONE',  ( 21.53943276465977519, -0.05219959533907433946, 108.7489096053143669 ) ) ;
#44988=CARTESIAN_POINT ( 'NONE',  ( -4.483927247898782831, 16.52544592524335698, 37.70942372801900433 ) ) ;
#44989=CARTESIAN_POINT ( 'NONE',  ( 18.67979575497178502, 10.72451020669898547, 34.16557627198102409 ) ) ;
#44990=CARTESIAN_POINT ( 'NONE',  ( 0.05219959533937995610, -21.53943276465977519, 105.0010903946856757 ) ) ;
#44991=CARTESIAN_POINT ( 'NONE',  ( 9.564922557960805705, 16.46253265017160317, 99.58224293864770971 ) ) ;
#44993=CARTESIAN_POINT ( 'NONE',  ( 19.03943276465977164, -0.05219959533909143690, 43.74890960531435979 ) ) ;
#44994=CARTESIAN_POINT ( 'NONE',  ( -0.05219959533909027116, -19.03943276465977164, 97.49890960531436690 ) ) ;
#44995=CARTESIAN_POINT ( 'NONE',  ( -9.564922557960796823, -16.46253265017161027, 77.08224293864769550 ) ) ;
#44996=CARTESIAN_POINT ( 'NONE',  ( 17.26172910966714369, -6.454744622557084810, 88.30646908649210047 ) ) ;
#44997=CARTESIAN_POINT ( 'NONE',  ( -9.564922557961040184, 16.46253265017147172, 57.91775706135233293 ) ) ;
#44998=CARTESIAN_POINT ( 'NONE',  ( -5.719274019375665041, -21.55341960407619695, 109.7927570613523613 ) ) ;
#44999=CARTESIAN_POINT ( 'NONE',  ( 5.719274019375991003, -21.55341960407610458, 32.70724293864770260 ) ) ;
#45000=CARTESIAN_POINT ( 'NONE',  ( 8.314922557961029526, -14.29746914071037800, 110.4177570613523756 ) ) ;
#45001=CARTESIAN_POINT ( 'NONE',  ( 16.51473224551069308, 9.474510206698969483, 39.16557627198103120 ) ) ;
#45002=CARTESIAN_POINT ( 'NONE',  ( 16.51473224551083163, -9.474510206698727899, 80.83442372801899012 ) ) ;
#45003=CARTESIAN_POINT ( 'NONE',  ( -19.03943276465977164, -0.05219959533935918106, 28.75109039468566507 ) ) ;
#45004=CARTESIAN_POINT ( 'NONE',  ( -17.31728774477270250, -6.344390552232404445, 44.18093348310681989 ) ) ;
#45005=CARTESIAN_POINT ( 'NONE',  ( -19.03943276465977164, 0.05219959533909376836, 36.24890960531436690 ) ) ;
#45006=CARTESIAN_POINT ( 'NONE',  ( 14.34966873604960469, 8.224510206698951720, 39.16557627198102409 ) ) ;
#45007=CARTESIAN_POINT ( 'NONE',  ( -16.29526858892874586, -7.335722546920139031, 110.7967059780020662 ) ) ;
#45008=CARTESIAN_POINT ( 'NONE',  ( 14.34966873604960469, 8.224510206698951720, 24.16557627198103120 ) ) ;
#45010=CARTESIAN_POINT ( 'NONE',  ( -12.14591786802326823, 12.06949235617739902, 88.12609039468570415 ) ) ;
#45011=CARTESIAN_POINT ( 'NONE',  ( -9.474510206698964154, 16.51473224551069663, 50.41557627198102409 ) ) ;
#45013=CARTESIAN_POINT ( 'NONE',  ( -5.823673210054431948, 21.52544592524334988, 102.7094237280190185 ) ) ;
#45014=CARTESIAN_POINT ( 'NONE',  ( -19.02544592524334988, -5.153800228976617603, 108.9594237280189759 ) ) ;
#45015=CARTESIAN_POINT ( 'NONE',  ( -5.823673210054431948, 21.52544592524334988, 87.70942372801901854 ) ) ;
#45016=CARTESIAN_POINT ( 'NONE',  ( 16.51473224551083163, -9.474510206698727899, 70.83442372801900433 ) ) ;
#45017=CARTESIAN_POINT ( 'NONE',  ( -13.97604488694527625, -13.89961937509977652, 86.87390960531436690 ) ) ;
#45018=CARTESIAN_POINT ( 'NONE',  ( -0.05219959533909027116, -19.03943276465977164, 87.49890960531436690 ) ) ;
#45020=CARTESIAN_POINT ( 'NONE',  ( -21.55341960407610458, -5.719274019375992779, 111.4572429386476813 ) ) ;
#45022=CARTESIAN_POINT ( 'NONE',  ( 8.314922557960818139, 14.29746914071049879, 84.58224293864769550 ) ) ;
#45023=CARTESIAN_POINT ( 'NONE',  ( -5.823673210054116645, -21.52544592524344225, 57.29057627198103120 ) ) ;
#45024=CARTESIAN_POINT ( 'NONE',  ( -9.474510206698964154, 16.51473224551069663, 55.41557627198103120 ) ) ;
#45025=CARTESIAN_POINT ( 'NONE',  ( 15.80617190586746368, 15.72974639402197994, 99.37390960531436690 ) ) ;
#45026=CARTESIAN_POINT ( 'NONE',  ( -8.224510206698735004, -14.34966873604973081, 84.58442372801903275 ) ) ;
#45027=EDGE_CURVE ( 'NONE', #199255, #15707, #117637, .T. ) ;
#45029=CARTESIAN_POINT ( 'NONE',  ( -0.05219959533909027116, -19.03943276465977164, 62.49890960531435979 ) ) ;
#45030=CARTESIAN_POINT ( 'NONE',  ( 8.314922557960818139, 14.29746914071049879, 94.58224293864769550 ) ) ;
#45032=CARTESIAN_POINT ( 'NONE',  ( -9.564922557960796823, -16.46253265017161027, 52.08224293864768839 ) ) ;
#45033=CARTESIAN_POINT ( 'NONE',  ( 9.564922557961047289, -16.46253265017146816, 85.41775706135233293 ) ) ;
#45034=CARTESIAN_POINT ( 'NONE',  ( 4.483927247898545687, 16.52544592524342804, 84.79057627198102409 ) ) ;
#45035=CARTESIAN_POINT ( 'NONE',  ( 15.80617190586769283, -15.72974639402175789, 55.62609039468568284 ) ) ;
#45036=CARTESIAN_POINT ( 'NONE',  ( -13.97604488694527625, -13.89961937509977652, 31.87390960531435979 ) ) ;
#45037=CARTESIAN_POINT ( 'NONE',  ( 18.62759615963271287, -10.81492255796078972, 98.33224293864769550 ) ) ;
#45038=CARTESIAN_POINT ( 'NONE',  ( 14.29746914071049879, -8.314922557960816363, 103.3322429386476955 ) ) ;
#45040=CARTESIAN_POINT ( 'NONE',  ( -19.03943276465977164, 0.05219959533909376836, 56.24890960531435979 ) ) ;
#45042=CARTESIAN_POINT ( 'NONE',  ( -9.474510206698720793, -16.51473224551083518, 99.58442372801900433 ) ) ;
#45043=CARTESIAN_POINT ( 'NONE',  ( -19.05341960407611168, -5.049401038298163336, 111.4572429386476671 ) ) ;
#45044=CARTESIAN_POINT ( 'NONE',  ( 15.80617190586769283, -15.72974639402175789, 55.62609039468568284 ) ) ;
#45045=CARTESIAN_POINT ( 'NONE',  ( -9.474510206698964154, 16.51473224551069663, 80.41557627198103830 ) ) ;
#45046=CARTESIAN_POINT ( 'NONE',  ( 9.474510206698729675, 16.51473224551082808, 67.08442372801900433 ) ) ;
#45047=CARTESIAN_POINT ( 'NONE',  ( -5.049401038298153566, 19.05341960407611168, 60.20724293864768129 ) ) ;
#45048=CARTESIAN_POINT ( 'NONE',  ( -4.379528057220328563, 16.55341960407611168, 80.20724293864769550 ) ) ;
#45049=CARTESIAN_POINT ( 'NONE',  ( 16.52544592524342804, -4.483927247898539470, 68.54057627198103830 ) ) ;
#45050=CARTESIAN_POINT ( 'NONE',  ( -13.89961937509977652, 13.97604488694528158, 90.62390960531432427 ) ) ;
#45051=CARTESIAN_POINT ( 'NONE',  ( 16.55341960407611168, 4.379528057220329451, 83.95724293864770971 ) ) ;
#45052=CARTESIAN_POINT ( 'NONE',  ( -13.97604488694527625, -13.89961937509977652, 81.87390960531436690 ) ) ;
#45053=CARTESIAN_POINT ( 'NONE',  ( 19.05341960407617918, -5.049401038297876454, 26.04275706135233293 ) ) ;
#45054=CARTESIAN_POINT ( 'NONE',  ( 13.97604488694527802, 13.89961937509977652, 54.37390960531435979 ) ) ;
#45055=CARTESIAN_POINT ( 'NONE',  ( 12.06949235617757843, -12.14591786802309237, 33.12390960531435979 ) ) ;
#45056=CARTESIAN_POINT ( 'NONE',  ( -0.05219959533910754901, -16.53943276465976808, 112.4989096053143669 ) ) ;
#45057=ORIENTED_EDGE ( 'NONE', *, *, #10333, .F. ) ;
#45058=CARTESIAN_POINT ( 'NONE',  ( -10.72451020669870658, -18.67979575497194134, 39.58442372801901143 ) ) ;
#45059=CARTESIAN_POINT ( 'NONE',  ( 9.474510206698729675, 16.51473224551082808, 67.08442372801900433 ) ) ;
#45060=CARTESIAN_POINT ( 'NONE',  ( -4.379528057220328563, 16.55341960407611168, 40.20724293864769550 ) ) ;
#45061=CARTESIAN_POINT ( 'NONE',  ( 10.81492255796078972, 18.62759615963270932, 84.58224293864769550 ) ) ;
#45062=CARTESIAN_POINT ( 'NONE',  ( 5.049401038298161559, -19.05341960407611168, 112.7072429386476813 ) ) ;
#45063=CARTESIAN_POINT ( 'NONE',  ( -8.224510206698948167, 14.34966873604960824, 65.41557627198102409 ) ) ;
#45064=CARTESIAN_POINT ( 'NONE',  ( 19.05341960407611168, 5.049401038298154454, 38.95724293864767418 ) ) ;
#45065=CARTESIAN_POINT ( 'NONE',  ( 13.89961937509957401, 13.97604488694547697, 31.87609039468566863 ) ) ;
#45066=CARTESIAN_POINT ( 'NONE',  ( -14.34966873604972548, 8.224510206698743886, 98.33442372801901854 ) ) ;
#45067=CARTESIAN_POINT ( 'NONE',  ( 4.483927247898790824, -16.52544592524335698, 60.20942372801902565 ) ) ;
#45068=CARTESIAN_POINT ( 'NONE',  ( -21.52544592524343514, 5.823673210054127303, 31.04057627198102409 ) ) ;
#45069=CARTESIAN_POINT ( 'NONE',  ( 18.62759615963255655, 10.81492255796105972, 101.6677570613523613 ) ) ;
#45070=CARTESIAN_POINT ( 'NONE',  ( 5.049401038298161559, -19.05341960407611168, 97.70724293864766707 ) ) ;
#45071=CARTESIAN_POINT ( 'NONE',  ( 8.224510206698742110, 14.34966873604972548, 77.08442372801901854 ) ) ;
#45072=CARTESIAN_POINT ( 'NONE',  ( 16.55341960407611168, 4.379528057220329451, 113.9572429386477239 ) ) ;
#45073=CARTESIAN_POINT ( 'NONE',  ( 16.55341960407611168, 4.379528057220329451, 28.95724293864769905 ) ) ;
#45074=CARTESIAN_POINT ( 'NONE',  ( 16.51473224551069308, 9.474510206698969483, 109.1655762719810383 ) ) ;
#45075=CARTESIAN_POINT ( 'NONE',  ( -19.05341960407611168, -5.049401038298163336, 86.45724293864769550 ) ) ;
#45076=CARTESIAN_POINT ( 'NONE',  ( -0.05219959533907301413, -21.53943276465977519, 27.49890960531435269 ) ) ;
#45077=CARTESIAN_POINT ( 'NONE',  ( -4.379528057220328563, 16.55341960407611168, 55.20724293864770260 ) ) ;
#45078=CARTESIAN_POINT ( 'NONE',  ( -14.34966873604960291, -8.224510206698953496, 36.66557627198103120 ) ) ;
#45079=VERTEX_POINT ( 'NONE', #174716 ) ;
#45080=CARTESIAN_POINT ( 'NONE',  ( -8.224510206698948167, 14.34966873604960824, 55.41557627198102409 ) ) ;
#45081=CARTESIAN_POINT ( 'NONE',  ( 14.34966873604972726, -8.224510206698740333, 55.83442372801901854 ) ) ;
#45083=CARTESIAN_POINT ( 'NONE',  ( -16.51473224551082808, 9.474510206698731452, 48.33442372801900433 ) ) ;
#45084=CARTESIAN_POINT ( 'NONE',  ( -19.02544592524342804, 5.153800228976336051, 91.04057627198100988 ) ) ;
#45085=CARTESIAN_POINT ( 'NONE',  ( 16.51473224551083163, -9.474510206698727899, 65.83442372801900433 ) ) ;
#45087=CARTESIAN_POINT ( 'NONE',  ( 0.05219959533936267826, -19.03943276465977164, 55.00109039468566863 ) ) ;
#45088=CARTESIAN_POINT ( 'NONE',  ( -13.97604488694547697, 13.89961937509957934, 93.12609039468566152 ) ) ;
#45089=CARTESIAN_POINT ( 'NONE',  ( -0.05219959533934338120, 16.53943276465976808, 77.50109039468567573 ) ) ;
#45091=CARTESIAN_POINT ( 'NONE',  ( -19.05341960407611168, -5.049401038298163336, 26.45724293864769550 ) ) ;
#45092=CARTESIAN_POINT ( 'NONE',  ( -5.049401038298153566, 19.05341960407611168, 115.2072429386477097 ) ) ;
#45093=CARTESIAN_POINT ( 'NONE',  ( 21.55341960407619695, -5.719274019375665929, 46.04275706135234714 ) ) ;
#45094=CARTESIAN_POINT ( 'NONE',  ( 16.46253265017146816, 9.564922557961045513, 101.6677570613523329 ) ) ;
#45096=CARTESIAN_POINT ( 'NONE',  ( 19.05341960407611168, 5.049401038298154454, 58.95724293864768129 ) ) ;
#45097=CARTESIAN_POINT ( 'NONE',  ( 19.05341960407611168, 5.049401038298154454, 98.95724293864766707 ) ) ;
#45098=CARTESIAN_POINT ( 'NONE',  ( 0.05219959533910956823, 16.53943276465976808, 69.99890960531435269 ) ) ;
#45099=CARTESIAN_POINT ( 'NONE',  ( 16.51473224551069308, 9.474510206698969483, 59.16557627198102409 ) ) ;
#45100=CARTESIAN_POINT ( 'NONE',  ( -13.97604488694527625, -13.89961937509977652, 76.87390960531433848 ) ) ;
#45101=CARTESIAN_POINT ( 'NONE',  ( 19.02544592524334988, 5.153800228976608722, 81.45942372801897591 ) ) ;
#45102=CARTESIAN_POINT ( 'NONE',  ( -0.05219959533907301413, -21.53943276465977519, 52.49890960531435979 ) ) ;
#45103=CARTESIAN_POINT ( 'NONE',  ( -4.379528057220328563, 16.55341960407611168, 110.2072429386477239 ) ) ;
#45104=CARTESIAN_POINT ( 'NONE',  ( 19.03943276465977164, 0.05219959533936151252, 41.25109039468566152 ) ) ;
#45105=CARTESIAN_POINT ( 'NONE',  ( 5.049401038298161559, -19.05341960407611168, 77.70724293864765286 ) ) ;
#45106=CARTESIAN_POINT ( 'NONE',  ( 21.55341960407610458, 5.719274019375980345, 78.95724293864769550 ) ) ;
#45107=CARTESIAN_POINT ( 'NONE',  ( 14.34966873604960469, 8.224510206698951720, 84.16557627198103830 ) ) ;
#45108=CARTESIAN_POINT ( 'NONE',  ( -19.03943276465977164, -0.05219959533935918106, 53.75109039468566863 ) ) ;
#45109=CARTESIAN_POINT ( 'NONE',  ( 15.72974639402199770, -15.80617190586745480, 73.12390960531436690 ) ) ;
#45110=CARTESIAN_POINT ( 'NONE',  ( -18.67979575497178146, -10.72451020669898902, 66.66557627198102409 ) ) ;
#45111=CARTESIAN_POINT ( 'NONE',  ( -10.72451020669898014, 18.67979575497178502, 35.41557627198102409 ) ) ;
#45112=CARTESIAN_POINT ( 'NONE',  ( -5.719274019375665041, -21.55341960407619695, 94.79275706135234714 ) ) ;
#45113=CARTESIAN_POINT ( 'NONE',  ( 19.05341960407611168, 5.049401038298154454, 63.95724293864769550 ) ) ;
#45114=CARTESIAN_POINT ( 'NONE',  ( -8.314922557960811034, -14.29746914071050412, 112.0822429386477097 ) ) ;
#45115=CARTESIAN_POINT ( 'NONE',  ( 0.05219959533937995610, -21.53943276465977519, 20.00109039468568639 ) ) ;
#45116=CARTESIAN_POINT ( 'NONE',  ( -10.72451020669870658, -18.67979575497194134, 39.58442372801901143 ) ) ;
#45117=CARTESIAN_POINT ( 'NONE',  ( 13.89961937509977652, -13.97604488694527269, 28.12390960531435624 ) ) ;
#45118=CARTESIAN_POINT ( 'NONE',  ( -5.719274019375978568, 21.55341960407610458, 105.2072429386477097 ) ) ;
#45119=CARTESIAN_POINT ( 'NONE',  ( -5.049401038297874678, -19.05341960407617918, 44.79275706135232582 ) ) ;
#45120=CARTESIAN_POINT ( 'NONE',  ( -16.46253265017160317, 9.564922557960807481, 40.83224293864769550 ) ) ;
#45121=CARTESIAN_POINT ( 'NONE',  ( -5.153800228976328057, -19.02544592524343514, 22.29057627198102765 ) ) ;
#45123=CARTESIAN_POINT ( 'NONE',  ( -12.14591786802326823, 12.06949235617739902, 58.12609039468568994 ) ) ;
#45124=CARTESIAN_POINT ( 'NONE',  ( -9.564922557960796823, -16.46253265017161027, 27.08224293864769550 ) ) ;
#45126=CARTESIAN_POINT ( 'NONE',  ( -19.05341960407611168, -5.049401038298163336, 81.45724293864769550 ) ) ;
#45127=CARTESIAN_POINT ( 'NONE',  ( -0.05219959533910754901, -16.53943276465976808, 102.4989096053143811 ) ) ;
#45128=CARTESIAN_POINT ( 'NONE',  ( -15.72974639402197994, 15.80617190586746368, 55.62390960531436690 ) ) ;
#45129=CARTESIAN_POINT ( 'NONE',  ( -16.52544592524335698, -4.483927247898792601, 43.95942372801902565 ) ) ;
#45130=CARTESIAN_POINT ( 'NONE',  ( -10.81492255796105439, 18.62759615963255655, 97.91775706135236135 ) ) ;
#45132=CARTESIAN_POINT ( 'NONE',  ( -9.474510206698964154, 16.51473224551069663, 40.41557627198103120 ) ) ;
#45133=CARTESIAN_POINT ( 'NONE',  ( -14.29746914071037622, -8.314922557961029526, 109.1677570613523613 ) ) ;
#45134=CARTESIAN_POINT ( 'NONE',  ( -12.06949235617756955, 12.14591786802309770, 55.62390960531436690 ) ) ;
#45135=CIRCLE ( 'NONE', #138630, 2.500000000000002220 ) ;
#45136=CARTESIAN_POINT ( 'NONE',  ( -9.474510206698964154, 16.51473224551069663, 70.41557627198102409 ) ) ;
#45137=CARTESIAN_POINT ( 'NONE',  ( 9.564922557961047289, -16.46253265017146816, 20.41775706135233293 ) ) ;
#45138=CARTESIAN_POINT ( 'NONE',  ( 21.53943276465977519, 0.05219959533937863772, 26.25109039468567573 ) ) ;
#45139=CARTESIAN_POINT ( 'NONE',  ( 10.81492255796106328, -18.62759615963255655, 75.41775706135233293 ) ) ;
#45140=CARTESIAN_POINT ( 'NONE',  ( 16.55341960407618274, -4.379528057220086978, 51.04275706135234714 ) ) ;
#45141=CARTESIAN_POINT ( 'NONE',  ( -8.224510206698735004, -14.34966873604973081, 34.58442372801900433 ) ) ;
#45142=CARTESIAN_POINT ( 'NONE',  ( -8.314922557960811034, -14.29746914071050412, 77.08224293864769550 ) ) ;
#45143=CARTESIAN_POINT ( 'NONE',  ( 18.67979575497194134, -10.72451020669871369, 105.8344237280190328 ) ) ;
#45145=CARTESIAN_POINT ( 'NONE',  ( -4.379528057220328563, 16.55341960407611168, 30.20724293864769550 ) ) ;
#45146=CARTESIAN_POINT ( 'NONE',  ( -16.20579543436677383, 7.371946100355101450, 114.4347916582812985 ) ) ;
#45147=CARTESIAN_POINT ( 'NONE',  ( 16.55341960407618274, -4.379528057220086978, 36.04275706135234714 ) ) ;
#45148=CARTESIAN_POINT ( 'NONE',  ( -8.314922557960811034, -14.29746914071050412, 47.08224293864770260 ) ) ;
#45149=CARTESIAN_POINT ( 'NONE',  ( -12.14591786802326823, 12.06949235617739902, 83.12609039468568994 ) ) ;
#45150=CARTESIAN_POINT ( 'NONE',  ( -5.049401038298153566, 19.05341960407611168, 100.2072429386476955 ) ) ;
#45151=CARTESIAN_POINT ( 'NONE',  ( -19.03943276465977164, 0.05219959533909376836, 111.2489096053143669 ) ) ;
#45152=CARTESIAN_POINT ( 'NONE',  ( 5.719274019375673035, 21.55341960407619339, 102.2927570613523613 ) ) ;
#45153=CARTESIAN_POINT ( 'NONE',  ( -8.314922557961024197, 14.29746914071037800, 102.9177570613523756 ) ) ;
#45154=CARTESIAN_POINT ( 'NONE',  ( -12.14591786802309592, -12.06949235617757132, 91.87390960531436690 ) ) ;
#45155=CARTESIAN_POINT ( 'NONE',  ( -0.05219959533909027116, -19.03943276465977164, 87.49890960531436690 ) ) ;
#45157=CARTESIAN_POINT ( 'NONE',  ( 14.29746914071037800, 8.314922557961029526, 36.66775706135234714 ) ) ;
#45158=CARTESIAN_POINT ( 'NONE',  ( 19.02544592524343514, -5.153800228976328945, 38.54057627198103120 ) ) ;
#45159=CARTESIAN_POINT ( 'NONE',  ( -19.03943276465977164, 0.05219959533909376836, 111.2489096053143669 ) ) ;
#45160=CARTESIAN_POINT ( 'NONE',  ( 14.34966873604972726, -8.224510206698740333, 45.83442372801901854 ) ) ;
#45162=CARTESIAN_POINT ( 'NONE',  ( -13.97604488694547697, 13.89961937509957934, 38.12609039468566152 ) ) ;
#45163=CARTESIAN_POINT ( 'NONE',  ( -14.34966873604972548, 8.224510206698743886, 103.3344237280190043 ) ) ;
#45164=CARTESIAN_POINT ( 'NONE',  ( -19.03943276465977164, 0.05219959533909376836, 31.24890960531435979 ) ) ;
#45165=CARTESIAN_POINT ( 'NONE',  ( 16.53943276465976808, 0.05219959533934440121, 76.25109039468568994 ) ) ;
#45166=CARTESIAN_POINT ( 'NONE',  ( 16.51473224551083163, -9.474510206698727899, 85.83442372801900433 ) ) ;
#45167=CARTESIAN_POINT ( 'NONE',  ( -5.153800228976607833, 19.02544592524334988, 22.70942372801899012 ) ) ;
#45168=CARTESIAN_POINT ( 'NONE',  ( -5.049401038298153566, 19.05341960407611168, 65.20724293864765286 ) ) ;
#45169=CARTESIAN_POINT ( 'NONE',  ( 8.314922557960818139, 14.29746914071049879, 94.58224293864769550 ) ) ;
#45171=CARTESIAN_POINT ( 'NONE',  ( -5.153800228976607833, 19.02544592524334988, 62.70942372801899722 ) ) ;
#45172=CARTESIAN_POINT ( 'NONE',  ( -18.67979575497178146, -10.72451020669898902, 66.66557627198102409 ) ) ;
#45173=CARTESIAN_POINT ( 'NONE',  ( 13.97604488694548053, -13.89961937509957401, 25.62609039468566507 ) ) ;
#45174=CARTESIAN_POINT ( 'NONE',  ( -5.153800228976328057, -19.02544592524343514, 107.2905762719810383 ) ) ;
#45176=CARTESIAN_POINT ( 'NONE',  ( -0.05219959533907301413, -21.53943276465977519, 82.49890960531436690 ) ) ;
#45177=CARTESIAN_POINT ( 'NONE',  ( -19.02544592524342804, 5.153800228976336051, 116.0405762719810383 ) ) ;
#45178=CARTESIAN_POINT ( 'NONE',  ( 13.97604488694548053, -13.89961937509957401, 105.6260903946856757 ) ) ;
#45180=CARTESIAN_POINT ( 'NONE',  ( -4.483927247898782831, 16.52544592524335698, 27.70942372801901854 ) ) ;
#45181=CARTESIAN_POINT ( 'NONE',  ( -0.05219959533909027116, -19.03943276465977164, 27.49890960531435624 ) ) ;
#45182=CARTESIAN_POINT ( 'NONE',  ( 5.049401038298161559, -19.05341960407611168, 92.70724293864769550 ) ) ;
#45183=CARTESIAN_POINT ( 'NONE',  ( 0.05219959533907565091, 21.53943276465977519, 94.99890960531436690 ) ) ;
#45184=CARTESIAN_POINT ( 'NONE',  ( 4.483927247898790824, -16.52544592524335698, 60.20942372801902565 ) ) ;
#45185=CARTESIAN_POINT ( 'NONE',  ( -21.53943276465977519, -0.05219959533937600094, 58.75109039468568994 ) ) ;
#45186=CARTESIAN_POINT ( 'NONE',  ( 19.05341960407617918, -5.049401038297876454, 101.0427570613523045 ) ) ;
#45187=CARTESIAN_POINT ( 'NONE',  ( 21.52544592524334988, 5.823673210054432836, 111.4594237280190328 ) ) ;
#45188=CARTESIAN_POINT ( 'NONE',  ( -12.06949235617739369, -12.14591786802326823, 109.3760903946857042 ) ) ;
#45189=CARTESIAN_POINT ( 'NONE',  ( 0.05219959533907565091, 21.53943276465977519, 94.99890960531436690 ) ) ;
#45190=CARTESIAN_POINT ( 'NONE',  ( 14.29746914071049879, -8.314922557960816363, 33.33224293864769550 ) ) ;
#45191=CARTESIAN_POINT ( 'NONE',  ( -0.05219959533936034679, 19.03943276465977164, 87.50109039468567573 ) ) ;
#45192=CARTESIAN_POINT ( 'NONE',  ( -10.72451020669870658, -18.67979575497194134, 59.58442372801901854 ) ) ;
#45193=CARTESIAN_POINT ( 'NONE',  ( 19.05341960407617918, -5.049401038297876454, 36.04275706135234003 ) ) ;
#45194=CARTESIAN_POINT ( 'NONE',  ( 12.06949235617757843, -12.14591786802309237, 108.1239096053143811 ) ) ;
#45195=CARTESIAN_POINT ( 'NONE',  ( -10.81492255796078084, -18.62759615963271287, 32.08224293864769550 ) ) ;
#45196=CARTESIAN_POINT ( 'NONE',  ( -16.53943276465976808, 0.05219959533911058130, 36.24890960531435979 ) ) ;
#45197=CARTESIAN_POINT ( 'NONE',  ( 5.719274019375673035, 21.55341960407619339, 92.29275706135236135 ) ) ;
#45198=CARTESIAN_POINT ( 'NONE',  ( -16.55341960407617563, 4.379528057220093196, 73.54275706135234714 ) ) ;
#45199=CARTESIAN_POINT ( 'NONE',  ( 8.224510206698953496, -14.34966873604960469, 27.91557627198103830 ) ) ;
#45200=CARTESIAN_POINT ( 'NONE',  ( -18.67979575497193778, 10.72451020669871902, 68.33442372801900433 ) ) ;
#45201=CARTESIAN_POINT ( 'NONE',  ( -0.05219959533937732626, 21.53943276465977519, 57.50109039468568994 ) ) ;
#45203=CARTESIAN_POINT ( 'NONE',  ( 13.89961937509978007, -13.97604488694527269, 63.12390960531435979 ) ) ;
#45204=CARTESIAN_POINT ( 'NONE',  ( 15.80617190586769283, -15.72974639402175789, 40.62609039468567573 ) ) ;
#45205=CARTESIAN_POINT ( 'NONE',  ( 19.05341960407611168, 5.049401038298154454, 28.95724293864769550 ) ) ;
#45206=CARTESIAN_POINT ( 'NONE',  ( -19.02544592524342804, 5.153800228976336051, 41.04057627198103120 ) ) ;
#45207=CARTESIAN_POINT ( 'NONE',  ( 14.34966873604960469, 8.224510206698951720, 84.16557627198103830 ) ) ;
#45208=CARTESIAN_POINT ( 'NONE',  ( -9.474510206698964154, 16.51473224551069663, 90.41557627198103830 ) ) ;
#45209=CARTESIAN_POINT ( 'NONE',  ( -4.483927247898539470, -16.52544592524342804, 27.29057627198103120 ) ) ;
#45210=CARTESIAN_POINT ( 'NONE',  ( -5.719274019375978568, 21.55341960407610458, 60.20724293864768839 ) ) ;
#45211=CARTESIAN_POINT ( 'NONE',  ( -21.52544592524343514, 5.823673210054127303, 106.0405762719810525 ) ) ;
#45212=CARTESIAN_POINT ( 'NONE',  ( 0.05219959533909260263, 19.03943276465977164, 99.99890960531436690 ) ) ;
#45213=CARTESIAN_POINT ( 'NONE',  ( -9.474510206698964154, 16.51473224551069663, 65.41557627198102409 ) ) ;
#45214=CARTESIAN_POINT ( 'NONE',  ( -5.049401038297874678, -19.05341960407617918, 109.7927570613523187 ) ) ;
#45215=CARTESIAN_POINT ( 'NONE',  ( 21.53943276465977519, -0.05219959533907433946, 53.74890960531437401 ) ) ;
#45216=CARTESIAN_POINT ( 'NONE',  ( -5.823673210054431948, 21.52544592524334988, 82.70942372801900433 ) ) ;
#45217=CARTESIAN_POINT ( 'NONE',  ( -5.049401038298153566, 19.05341960407611168, 65.20724293864765286 ) ) ;
#45218=CARTESIAN_POINT ( 'NONE',  ( -5.153800228976328057, -19.02544592524343514, 92.29057627198099567 ) ) ;
#45219=CARTESIAN_POINT ( 'NONE',  ( 12.14591786802327356, -12.06949235617739191, 70.62609039468567573 ) ) ;
#45220=CARTESIAN_POINT ( 'NONE',  ( -18.62759615963255300, -10.81492255796106328, 64.16775706135234714 ) ) ;
#45221=CARTESIAN_POINT ( 'NONE',  ( -10.81492255796105439, 18.62759615963255655, 82.91775706135234714 ) ) ;
#45222=CARTESIAN_POINT ( 'NONE',  ( 5.823673210054125526, 21.52544592524343514, 114.7905762719810383 ) ) ;
#45223=CARTESIAN_POINT ( 'NONE',  ( -14.29746914071037622, -8.314922557961029526, 84.16775706135234714 ) ) ;
#45224=B_SPLINE_CURVE_WITH_KNOTS ( 'NONE', 3,
 ( #146197, #163390, #129026, #22873, #6685, #176567 ),
 .UNSPECIFIED., .F., .F.,
 ( 4, 2, 4 ),
 ( 0.003989672132298099222, 0.004372778065220536345, 0.004755883998142972600 ),
 .UNSPECIFIED. ) ;
#45225=CARTESIAN_POINT ( 'NONE',  ( -18.67979575497178146, -10.72451020669898902, 76.66557627198103830 ) ) ;
#45226=CARTESIAN_POINT ( 'NONE',  ( -9.564922557961040184, 16.46253265017147172, 52.91775706135233293 ) ) ;
#45227=CARTESIAN_POINT ( 'NONE',  ( 15.80617190586746368, 15.72974639402197994, 44.37390960531435979 ) ) ;
#45228=CARTESIAN_POINT ( 'NONE',  ( 13.89961937509977652, -13.97604488694527269, 88.12390960531438111 ) ) ;
#45229=CARTESIAN_POINT ( 'NONE',  ( 4.379528057220339221, -16.55341960407611168, 27.70724293864769905 ) ) ;
#45231=CARTESIAN_POINT ( 'NONE',  ( 15.72974639402199770, -15.80617190586745480, 23.12390960531436335 ) ) ;
#45233=CARTESIAN_POINT ( 'NONE',  ( -9.474510206698720793, -16.51473224551083518, 89.58442372801900433 ) ) ;
#45234=CARTESIAN_POINT ( 'NONE',  ( 5.823673210054125526, 21.52544592524343514, 74.79057627198105251 ) ) ;
#45235=CARTESIAN_POINT ( 'NONE',  ( 14.29746914071049879, -8.314922557960816363, 53.33224293864769550 ) ) ;
#45236=CARTESIAN_POINT ( 'NONE',  ( -19.03943276465977164, -0.05219959533935918106, 113.7510903946856757 ) ) ;
#45237=CARTESIAN_POINT ( 'NONE',  ( -5.049401038298153566, 19.05341960407611168, 40.20724293864768839 ) ) ;
#45238=CARTESIAN_POINT ( 'NONE',  ( -5.719274019375978568, 21.55341960407610458, 100.2072429386476955 ) ) ;
#45239=CARTESIAN_POINT ( 'NONE',  ( -19.05341960407617563, 5.049401038297882671, 73.54275706135233293 ) ) ;
#45240=CARTESIAN_POINT ( 'NONE',  ( 0.05219959533909260263, 19.03943276465977164, 84.99890960531436690 ) ) ;
#45241=CARTESIAN_POINT ( 'NONE',  ( 16.55341960407611168, 4.379528057220329451, 83.95724293864770971 ) ) ;
#45242=CARTESIAN_POINT ( 'NONE',  ( -5.153800228976328057, -19.02544592524343514, 57.29057627198103120 ) ) ;
#45243=CARTESIAN_POINT ( 'NONE',  ( -8.314922557960811034, -14.29746914071050412, 62.08224293864769550 ) ) ;
#45244=CARTESIAN_POINT ( 'NONE',  ( 13.89961937509977652, -13.97604488694527269, 28.12390960531435624 ) ) ;
#45245=CARTESIAN_POINT ( 'NONE',  ( -17.01956338556749415, -5.458179474447081070, 20.69910624262117338 ) ) ;
#45246=CARTESIAN_POINT ( 'NONE',  ( -14.34966873604960291, -8.224510206698953496, 41.66557627198103120 ) ) ;
#45247=CARTESIAN_POINT ( 'NONE',  ( 13.97604488694527802, 13.89961937509977652, 89.37390960531436690 ) ) ;
#45249=CARTESIAN_POINT ( 'NONE',  ( -5.153800228976607833, 19.02544592524334988, 52.70942372801900433 ) ) ;
#45250=CARTESIAN_POINT ( 'NONE',  ( -16.52544592524335698, -4.483927247898792601, 53.95942372801900433 ) ) ;
#45251=CARTESIAN_POINT ( 'NONE',  ( -21.55341960407610458, -5.719274019375992779, 76.45724293864769550 ) ) ;
#45252=CARTESIAN_POINT ( 'NONE',  ( 5.049401038297881783, 19.05341960407617563, 32.29275706135233293 ) ) ;
#45253=CARTESIAN_POINT ( 'NONE',  ( 0.05219959533909260263, 19.03943276465977164, 89.99890960531436690 ) ) ;
#45255=CARTESIAN_POINT ( 'NONE',  ( -15.80617190586745835, -15.72974639402198527, 26.87390960531435979 ) ) ;
#45256=CARTESIAN_POINT ( 'NONE',  ( 16.46253265017160672, -9.564922557960803928, 58.33224293864769550 ) ) ;
#45257=CARTESIAN_POINT ( 'NONE',  ( -21.53943276465977519, -0.05219959533937600094, 48.75109039468568284 ) ) ;
#45258=CARTESIAN_POINT ( 'NONE',  ( 16.46253265017160672, -9.564922557960803928, 23.33224293864769194 ) ) ;
#45259=CARTESIAN_POINT ( 'NONE',  ( 10.81492255796106328, -18.62759615963255655, 20.41775706135234714 ) ) ;
#45260=CARTESIAN_POINT ( 'NONE',  ( 9.564922557960805705, 16.46253265017160317, 89.58224293864769550 ) ) ;
#45262=CARTESIAN_POINT ( 'NONE',  ( 15.72974639402176855, 15.80617190586768217, 36.87609039468568994 ) ) ;
#45264=CARTESIAN_POINT ( 'NONE',  ( -19.05341960407611168, -5.049401038298163336, 96.45724293864769550 ) ) ;
#45265=CARTESIAN_POINT ( 'NONE',  ( -5.049401038298153566, 19.05341960407611168, 90.20724293864768129 ) ) ;
#45266=CARTESIAN_POINT ( 'NONE',  ( 10.81492255796078972, 18.62759615963270932, 104.5822429386477097 ) ) ;
#45267=CARTESIAN_POINT ( 'NONE',  ( 5.153800228976335163, 19.02544592524342804, 49.79057627198100988 ) ) ;
#45268=CARTESIAN_POINT ( 'NONE',  ( 8.314922557961029526, -14.29746914071037800, 25.41775706135235779 ) ) ;
#45270=CARTESIAN_POINT ( 'NONE',  ( -13.89961937509977652, 13.97604488694528158, 25.62390960531434558 ) ) ;
#45271=CARTESIAN_POINT ( 'NONE',  ( -15.80617190586768217, 15.72974639402176855, 103.1260903946856757 ) ) ;
#45272=CARTESIAN_POINT ( 'NONE',  ( -16.46253265017160317, 9.564922557960807481, 70.83224293864770971 ) ) ;
#45273=CARTESIAN_POINT ( 'NONE',  ( 21.55341960407619695, -5.719274019375665929, 56.04275706135235424 ) ) ;
#45276=CARTESIAN_POINT ( 'NONE',  ( 0.05219959533909260263, 19.03943276465977164, 94.99890960531436690 ) ) ;
#45278=CARTESIAN_POINT ( 'NONE',  ( -14.29746914071037622, -8.314922557961029526, 39.16775706135235424 ) ) ;
#45279=CARTESIAN_POINT ( 'NONE',  ( 14.34966873604972726, -8.224510206698740333, 65.83442372801900433 ) ) ;
#45280=CARTESIAN_POINT ( 'NONE',  ( -0.05219959533937732626, 21.53943276465977519, 62.50109039468568284 ) ) ;
#45281=CARTESIAN_POINT ( 'NONE',  ( 5.719274019375673035, 21.55341960407619339, 87.29275706135236135 ) ) ;
#45283=CARTESIAN_POINT ( 'NONE',  ( -16.53943276465976808, -0.05219959533934237506, 18.75109039468568639 ) ) ;
#45284=CARTESIAN_POINT ( 'NONE',  ( -19.05341960407611168, -5.049401038298163336, 76.45724293864769550 ) ) ;
#45285=CARTESIAN_POINT ( 'NONE',  ( 16.51473224551069308, 9.474510206698969483, 99.16557627198102409 ) ) ;
#45286=CARTESIAN_POINT ( 'NONE',  ( 16.53943276465976808, -0.05219959533910856209, 113.7489096053143527 ) ) ;
#45287=CARTESIAN_POINT ( 'NONE',  ( 10.72451020669898902, -18.67979575497178502, 32.91557627198102409 ) ) ;
#45289=CARTESIAN_POINT ( 'NONE',  ( -16.55341960407617563, 4.379528057220093196, 93.54275706135234714 ) ) ;
#45290=CARTESIAN_POINT ( 'NONE',  ( 14.29746914071049879, -8.314922557960816363, 73.33224293864769550 ) ) ;
#45291=CARTESIAN_POINT ( 'NONE',  ( 16.46253265017160672, -9.564922557960803928, 58.33224293864769550 ) ) ;
#45292=CARTESIAN_POINT ( 'NONE',  ( -21.52544592524334988, -5.823673210054445271, 88.95942372801901854 ) ) ;
#45294=CARTESIAN_POINT ( 'NONE',  ( -16.51473224551082808, 9.474510206698731452, 103.3344237280190043 ) ) ;
#45295=CARTESIAN_POINT ( 'NONE',  ( -8.224510206698948167, 14.34966873604960824, 75.41557627198102409 ) ) ;
#45296=CARTESIAN_POINT ( 'NONE',  ( -18.62759615963255300, -10.81492255796106328, 34.16775706135234714 ) ) ;
#45297=CARTESIAN_POINT ( 'NONE',  ( 18.62759615963271287, -10.81492255796078972, 63.33224293864770260 ) ) ;
#45298=CARTESIAN_POINT ( 'NONE',  ( 13.89961937509957401, 13.97604488694547697, 36.87609039468565442 ) ) ;
#45300=CARTESIAN_POINT ( 'NONE',  ( 19.03943276465977164, -0.05219959533909143690, 83.74890960531436690 ) ) ;
#45301=CARTESIAN_POINT ( 'NONE',  ( -8.314922557960811034, -14.29746914071050412, 52.08224293864768839 ) ) ;
#45303=CARTESIAN_POINT ( 'NONE',  ( 8.314922557960818139, 14.29746914071049879, 34.58224293864770260 ) ) ;
#45304=CARTESIAN_POINT ( 'NONE',  ( 14.29746914071037800, 8.314922557961029526, 96.66775706135234714 ) ) ;
#45305=CARTESIAN_POINT ( 'NONE',  ( -13.97604488694547697, 13.89961937509957934, 48.12609039468566863 ) ) ;
#45307=CARTESIAN_POINT ( 'NONE',  ( 19.05341960407611168, 5.049401038298154454, 103.9572429386476671 ) ) ;
#45308=CARTESIAN_POINT ( 'NONE',  ( 16.53943276465976808, -0.05219959533910856209, 78.74890960531436690 ) ) ;
#45309=CARTESIAN_POINT ( 'NONE',  ( -16.51473224551082808, 9.474510206698731452, 38.33442372801899722 ) ) ;
#45310=CARTESIAN_POINT ( 'NONE',  ( 16.51473224551069308, 9.474510206698969483, 29.16557627198103475 ) ) ;
#45311=CARTESIAN_POINT ( 'NONE',  ( 21.55341960407610458, 5.719274019375980345, 38.95724293864768839 ) ) ;
#45312=CARTESIAN_POINT ( 'NONE',  ( 10.81492255796078972, 18.62759615963270932, 69.58224293864769550 ) ) ;
#45313=CARTESIAN_POINT ( 'NONE',  ( -8.314922557960811034, -14.29746914071050412, 112.0822429386477097 ) ) ;
#45314=CARTESIAN_POINT ( 'NONE',  ( -16.55341960407617563, 4.379528057220093196, 58.54275706135235424 ) ) ;
#45315=CARTESIAN_POINT ( 'NONE',  ( 18.67979575497194134, -10.72451020669871369, 40.83442372801901854 ) ) ;
#45316=B_SPLINE_CURVE_WITH_KNOTS ( 'NONE', 3,
 ( #13592, #75259, #65050, #93392, #33721, #171247, #5355, #143874, #79226, #3375, #32736, #20531, #96371, #186436, #126706, #156067, #112542, #63059, #47912, #109566 ),
 .UNSPECIFIED., .F., .F.,
 ( 4, 2, 2, 2, 2, 2, 2, 2, 2, 4 ),
 ( 0.000000000000000000, 0.0004987090165372804005, 0.0009974180330745608010, 0.001246772541343200893, 0.001496127049611841201, 0.001994836066149102520, 0.002493545082686363622, 0.002742899590954984632, 0.002992254099223606075, 0.003989672132298083609 ),
 .UNSPECIFIED. ) ;
#45317=CARTESIAN_POINT ( 'NONE',  ( -14.29746914071049879, 8.314922557960819915, 85.83224293864768129 ) ) ;
#45319=CARTESIAN_POINT ( 'NONE',  ( -17.49999999999999645, 5.499999999999997335, 25.79690382534172244 ) ) ;
#45320=CARTESIAN_POINT ( 'NONE',  ( 21.55341960407610458, 5.719274019375980345, 33.95724293864769550 ) ) ;
#45323=CARTESIAN_POINT ( 'NONE',  ( -12.14591786802326823, 12.06949235617739902, 48.12609039468568284 ) ) ;
#45324=CARTESIAN_POINT ( 'NONE',  ( -8.224510206698948167, 14.34966873604960824, 40.41557627198103120 ) ) ;
#45325=CARTESIAN_POINT ( 'NONE',  ( -15.80617190586745835, -15.72974639402198527, 66.87390960531436690 ) ) ;
#45326=CARTESIAN_POINT ( 'NONE',  ( 19.03943276465977164, 0.05219959533936151252, 81.25109039468567573 ) ) ;
#45327=CARTESIAN_POINT ( 'NONE',  ( -15.72974639402197994, 15.80617190586746368, 55.62390960531436690 ) ) ;
#45329=CARTESIAN_POINT ( 'NONE',  ( 19.03943276465977164, -0.05219959533909143690, 43.74890960531435979 ) ) ;
#45330=CARTESIAN_POINT ( 'NONE',  ( 19.03943276465977164, -0.05219959533909143690, 98.74890960531436690 ) ) ;
#45331=CARTESIAN_POINT ( 'NONE',  ( 13.97604488694527802, 13.89961937509977652, 49.37390960531434558 ) ) ;
#45332=CARTESIAN_POINT ( 'NONE',  ( 16.52544592524342804, -4.483927247898539470, 108.5405762719810241 ) ) ;
#45333=CARTESIAN_POINT ( 'NONE',  ( 19.03943276465977164, -0.05219959533909143690, 113.7489096053143669 ) ) ;
#45335=CARTESIAN_POINT ( 'NONE',  ( 14.29746914071037800, 8.314922557961029526, 66.66775706135234714 ) ) ;
#45336=CARTESIAN_POINT ( 'NONE',  ( 18.67979575497178502, 10.72451020669898547, 89.16557627198102409 ) ) ;
#45337=CARTESIAN_POINT ( 'NONE',  ( 19.03943276465977164, -0.05219959533909143690, 58.74890960531435979 ) ) ;
#45338=CARTESIAN_POINT ( 'NONE',  ( 0.05219959533937995610, -21.53943276465977519, 25.00109039468567218 ) ) ;
#45339=CARTESIAN_POINT ( 'NONE',  ( 5.153800228976335163, 19.02544592524342804, 89.79057627198102409 ) ) ;
#45342=CARTESIAN_POINT ( 'NONE',  ( -10.72451020669870658, -18.67979575497194134, 19.58442372801901143 ) ) ;
#45343=CARTESIAN_POINT ( 'NONE',  ( -9.474510206698964154, 16.51473224551069663, 30.41557627198102054 ) ) ;
#45344=CARTESIAN_POINT ( 'NONE',  ( -19.03943276465977164, 0.05219959533909376836, 101.2489096053143669 ) ) ;
#45345=CARTESIAN_POINT ( 'NONE',  ( -9.564922557961040184, 16.46253265017147172, 82.91775706135233293 ) ) ;
#45346=CARTESIAN_POINT ( 'NONE',  ( -19.05341960407617563, 5.049401038297882671, 43.54275706135232582 ) ) ;
#45347=CARTESIAN_POINT ( 'NONE',  ( 18.67979575497178502, 10.72451020669898547, 104.1655762719810241 ) ) ;
#45348=CARTESIAN_POINT ( 'NONE',  ( 9.564922557961047289, -16.46253265017146816, 35.41775706135233293 ) ) ;
#45349=CARTESIAN_POINT ( 'NONE',  ( 16.46253265017146816, 9.564922557961045513, 31.66775706135232937 ) ) ;
#45350=CARTESIAN_POINT ( 'NONE',  ( 16.53943276465976808, 0.05219959533934440121, 96.25109039468568994 ) ) ;
#45351=CARTESIAN_POINT ( 'NONE',  ( -13.89961937509977652, 13.97604488694528158, 110.6239096053143243 ) ) ;
#45352=CARTESIAN_POINT ( 'NONE',  ( 16.51473224551069308, 9.474510206698969483, 54.16557627198103120 ) ) ;
#45353=CARTESIAN_POINT ( 'NONE',  ( 15.72974639402176855, 15.80617190586768217, 61.87609039468568284 ) ) ;
#45354=CARTESIAN_POINT ( 'NONE',  ( 0.05219959533937995610, -21.53943276465977519, 75.00109039468568994 ) ) ;
#45355=CARTESIAN_POINT ( 'NONE',  ( -9.474510206698964154, 16.51473224551069663, 115.4155762719810241 ) ) ;
#45356=CARTESIAN_POINT ( 'NONE',  ( 19.05341960407611168, 5.049401038298154454, 78.95724293864769550 ) ) ;
#45357=CARTESIAN_POINT ( 'NONE',  ( 10.72451020669871369, 18.67979575497193778, 47.08442372801901854 ) ) ;
#45358=CARTESIAN_POINT ( 'NONE',  ( 5.049401038297881783, 19.05341960407617563, 102.2927570613523045 ) ) ;
#45359=CARTESIAN_POINT ( 'NONE',  ( -19.05341960407611168, -5.049401038298163336, 51.45724293864770260 ) ) ;
#45360=CARTESIAN_POINT ( 'NONE',  ( 19.05341960407611168, 5.049401038298154454, 103.9572429386476671 ) ) ;
#45361=CARTESIAN_POINT ( 'NONE',  ( -16.46253265017160317, 9.564922557960807481, 80.83224293864769550 ) ) ;
#45363=CARTESIAN_POINT ( 'NONE',  ( 5.153800228976335163, 19.02544592524342804, 59.79057627198100988 ) ) ;
#45364=CARTESIAN_POINT ( 'NONE',  ( -18.62759615963270932, 10.81492255796079327, 95.83224293864770971 ) ) ;
#45365=CARTESIAN_POINT ( 'NONE',  ( -14.29746914071037622, -8.314922557961029526, 84.16775706135234714 ) ) ;
#45367=CARTESIAN_POINT ( 'NONE',  ( 5.153800228976615827, -19.02544592524334988, 50.20942372801897591 ) ) ;
#45368=CARTESIAN_POINT ( 'NONE',  ( -16.51473224551069308, -9.474510206698971260, 81.66557627198103830 ) ) ;
#45369=CARTESIAN_POINT ( 'NONE',  ( -12.14591786802309592, -12.06949235617757132, 51.87390960531437401 ) ) ;
#45370=CARTESIAN_POINT ( 'NONE',  ( 8.314922557960818139, 14.29746914071049879, 94.58224293864769550 ) ) ;
#45371=CARTESIAN_POINT ( 'NONE',  ( -0.05219959533907301413, -21.53943276465977519, 22.49890960531436335 ) ) ;
#45372=CARTESIAN_POINT ( 'NONE',  ( -19.05341960407611168, -5.049401038298163336, 111.4572429386476671 ) ) ;
#45373=CARTESIAN_POINT ( 'NONE',  ( 5.153800228976335163, 19.02544592524342804, 114.7905762719810241 ) ) ;
#45374=CARTESIAN_POINT ( 'NONE',  ( 19.02544592524334988, 5.153800228976608722, 36.45942372801900433 ) ) ;
#45375=CARTESIAN_POINT ( 'NONE',  ( 14.29746914071037800, 8.314922557961029526, 91.66775706135234714 ) ) ;
#45376=CARTESIAN_POINT ( 'NONE',  ( -9.474510206698964154, 16.51473224551069663, 75.41557627198103830 ) ) ;
#45377=CARTESIAN_POINT ( 'NONE',  ( -5.719274019375665041, -21.55341960407619695, 34.79275706135235424 ) ) ;
#45378=CARTESIAN_POINT ( 'NONE',  ( -10.81492255796078084, -18.62759615963271287, 32.08224293864769550 ) ) ;
#45379=CARTESIAN_POINT ( 'NONE',  ( 18.67979575497178502, 10.72451020669898547, 114.1655762719810383 ) ) ;
#45380=CARTESIAN_POINT ( 'NONE',  ( 10.81492255796078972, 18.62759615963270932, 69.58224293864769550 ) ) ;
#45381=CARTESIAN_POINT ( 'NONE',  ( -8.224510206698948167, 14.34966873604960824, 95.41557627198102409 ) ) ;
#45382=CARTESIAN_POINT ( 'NONE',  ( 13.97604488694548053, -13.89961937509957401, 50.62609039468566152 ) ) ;
#45383=CARTESIAN_POINT ( 'NONE',  ( -9.564922557960796823, -16.46253265017161027, 32.08224293864769550 ) ) ;
#45384=CARTESIAN_POINT ( 'NONE',  ( -5.049401038298153566, 19.05341960407611168, 90.20724293864766707 ) ) ;
#45385=CARTESIAN_POINT ( 'NONE',  ( -9.564922557960796823, -16.46253265017161027, 82.08224293864768129 ) ) ;
#45387=CARTESIAN_POINT ( 'NONE',  ( -4.379528057220328563, 16.55341960407611168, 105.2072429386477097 ) ) ;
#45389=CARTESIAN_POINT ( 'NONE',  ( -14.29746914071049879, 8.314922557960819915, 30.83224293864770260 ) ) ;
#45390=CARTESIAN_POINT ( 'NONE',  ( 16.55341960407618274, -4.379528057220086978, 21.04275706135234714 ) ) ;
#45391=CARTESIAN_POINT ( 'NONE',  ( -5.719274019375665041, -21.55341960407619695, 99.79275706135234714 ) ) ;
#45392=CARTESIAN_POINT ( 'NONE',  ( 16.46253265017160672, -9.564922557960803928, 98.33224293864769550 ) ) ;
#45393=CARTESIAN_POINT ( 'NONE',  ( -18.67979575497178146, -10.72451020669898902, 111.6655762719810525 ) ) ;
#45394=CARTESIAN_POINT ( 'NONE',  ( -9.474510206698964154, 16.51473224551069663, 45.41557627198103120 ) ) ;
#45395=CARTESIAN_POINT ( 'NONE',  ( -8.314922557961024197, 14.29746914071037800, 42.91775706135235424 ) ) ;
#45396=CARTESIAN_POINT ( 'NONE',  ( -16.53943276465976808, -0.05219959533934237506, 18.75109039468568639 ) ) ;
#45397=CARTESIAN_POINT ( 'NONE',  ( -4.379528057220328563, 16.55341960407611168, 100.2072429386476955 ) ) ;
#45398=CARTESIAN_POINT ( 'NONE',  ( 0.05219959533907565091, 21.53943276465977519, 104.9989096053143669 ) ) ;
#45399=CARTESIAN_POINT ( 'NONE',  ( 13.89961937509957401, 13.97604488694547697, 66.87609039468567573 ) ) ;
#45401=CARTESIAN_POINT ( 'NONE',  ( -15.72974639402197994, 15.80617190586746368, 115.6239096053143669 ) ) ;
#45402=DIRECTION ( 'NONE',  ( 0.000000000000000000, 0.000000000000000000, -1.000000000000000000 ) ) ;
#45403=CARTESIAN_POINT ( 'NONE',  ( -5.153800228976328057, -19.02544592524343514, 92.29057627198099567 ) ) ;
#45404=CARTESIAN_POINT ( 'NONE',  ( 17.48847506799970120, -5.747544572773743532, 113.3269743784328227 ) ) ;
#45405=CARTESIAN_POINT ( 'NONE',  ( 19.05341960407611168, 5.049401038298154454, 78.95724293864769550 ) ) ;
#45406=CARTESIAN_POINT ( 'NONE',  ( 21.53943276465977519, 0.05219959533937863772, 31.25109039468568639 ) ) ;
#45407=CARTESIAN_POINT ( 'NONE',  ( -12.06949235617756955, 12.14591786802309770, 75.62390960531439532 ) ) ;
#45408=CARTESIAN_POINT ( 'NONE',  ( 19.05341960407611168, 5.049401038298154454, 88.95724293864769550 ) ) ;
#45409=CARTESIAN_POINT ( 'NONE',  ( 4.483927247898790824, -16.52544592524335698, 50.20942372801901854 ) ) ;
#45410=CARTESIAN_POINT ( 'NONE',  ( 16.46253265017146816, 9.564922557961045513, 56.66775706135233293 ) ) ;
#45411=CARTESIAN_POINT ( 'NONE',  ( 15.80617190586769283, -15.72974639402175789, 65.62609039468568994 ) ) ;
#45412=CARTESIAN_POINT ( 'NONE',  ( -0.05219959533934338120, 16.53943276465976808, 27.50109039468567929 ) ) ;
#45413=CARTESIAN_POINT ( 'NONE',  ( 13.97604488694527802, 13.89961937509977652, 74.37390960531436690 ) ) ;
#45414=CARTESIAN_POINT ( 'NONE',  ( 5.049401038297881783, 19.05341960407617563, 97.29275706135233293 ) ) ;
#45415=CARTESIAN_POINT ( 'NONE',  ( 14.34966873604972726, -8.224510206698740333, 60.83442372801901854 ) ) ;
#45416=CARTESIAN_POINT ( 'NONE',  ( -10.81492255796105439, 18.62759615963255655, 102.9177570613523756 ) ) ;
#45417=CARTESIAN_POINT ( 'NONE',  ( -19.03943276465977164, -0.05219959533935918106, 83.75109039468567573 ) ) ;
#45418=CARTESIAN_POINT ( 'NONE',  ( 19.02544592524343514, -5.153800228976328945, 48.54057627198103120 ) ) ;
#45419=CARTESIAN_POINT ( 'NONE',  ( -15.72974639402197994, 15.80617190586746368, 70.62390960531436690 ) ) ;
#45420=CARTESIAN_POINT ( 'NONE',  ( 12.06949235617757843, -12.14591786802309237, 78.12390960531436690 ) ) ;
#45421=CARTESIAN_POINT ( 'NONE',  ( 16.46253265017146816, 9.564922557961045513, 81.66775706135233293 ) ) ;
#45422=CARTESIAN_POINT ( 'NONE',  ( -18.22780087662124160, -5.499999999999927169, 68.98236817873106475 ) ) ;
#45423=CARTESIAN_POINT ( 'NONE',  ( 5.049401038297881783, 19.05341960407617563, 37.29275706135232582 ) ) ;
#45424=CARTESIAN_POINT ( 'NONE',  ( -4.483927247898782831, 16.52544592524335698, 112.7094237280190328 ) ) ;
#45425=CARTESIAN_POINT ( 'NONE',  ( -12.06949235617756955, 12.14591786802309770, 65.62390960531436690 ) ) ;
#45426=CARTESIAN_POINT ( 'NONE',  ( -21.55341960407619339, 5.719274019375674811, 108.5427570613523756 ) ) ;
#45428=CARTESIAN_POINT ( 'NONE',  ( 10.81492255796078972, 18.62759615963270932, 114.5822429386477097 ) ) ;
#45429=CARTESIAN_POINT ( 'NONE',  ( 19.02544592524343514, -5.153800228976328945, 63.54057627198103830 ) ) ;
#45430=CARTESIAN_POINT ( 'NONE',  ( -10.81492255796105439, 18.62759615963255655, 87.91775706135234714 ) ) ;
#45431=CARTESIAN_POINT ( 'NONE',  ( 19.05341960407611168, 5.049401038298154454, 68.95724293864769550 ) ) ;
#45433=CARTESIAN_POINT ( 'NONE',  ( 8.224510206698953496, -14.34966873604960469, 112.9155762719810383 ) ) ;
#45434=CARTESIAN_POINT ( 'NONE',  ( -15.72974639402197994, 15.80617190586746368, 35.62390960531437401 ) ) ;
#45435=CARTESIAN_POINT ( 'NONE',  ( -16.52544592524342804, 4.483927247898546575, 66.04057627198103830 ) ) ;
#45436=CARTESIAN_POINT ( 'NONE',  ( -19.03943276465977164, 0.05219959533909376836, 46.24890960531435979 ) ) ;
#45437=CARTESIAN_POINT ( 'NONE',  ( -12.06949235617756955, 12.14591786802309770, 85.62390960531436690 ) ) ;
#45438=CARTESIAN_POINT ( 'NONE',  ( 18.62759615963271287, -10.81492255796078972, 113.3322429386476955 ) ) ;
#45440=CARTESIAN_POINT ( 'NONE',  ( 15.72974639402176855, 15.80617190586768217, 51.87609039468568284 ) ) ;
#45441=CARTESIAN_POINT ( 'NONE',  ( -5.153800228976328057, -19.02544592524343514, 37.29057627198102409 ) ) ;
#45442=CARTESIAN_POINT ( 'NONE',  ( -16.53943276465976808, -0.05219959533934237506, 48.75109039468568284 ) ) ;
#45443=CARTESIAN_POINT ( 'NONE',  ( -5.823673210054116645, -21.52544592524344225, 92.29057627198103830 ) ) ;
#45444=CARTESIAN_POINT ( 'NONE',  ( 5.049401038297881783, 19.05341960407617563, 27.29275706135232937 ) ) ;
#45445=CARTESIAN_POINT ( 'NONE',  ( -13.97604488694527625, -13.89961937509977652, 56.87390960531434558 ) ) ;
#45446=CARTESIAN_POINT ( 'NONE',  ( -5.153800228976328057, -19.02544592524343514, 107.2905762719810383 ) ) ;
#45447=CARTESIAN_POINT ( 'NONE',  ( 0.05219959533937995610, -21.53943276465977519, 55.00109039468568284 ) ) ;
#45448=CARTESIAN_POINT ( 'NONE',  ( 15.72974639402199770, -15.80617190586745480, 48.12390960531436690 ) ) ;
#45449=CARTESIAN_POINT ( 'NONE',  ( 16.55341960407611168, 4.379528057220329451, 28.95724293864769905 ) ) ;
#45450=CARTESIAN_POINT ( 'NONE',  ( -0.05219959533937732626, 21.53943276465977519, 62.50109039468568284 ) ) ;
#45451=CARTESIAN_POINT ( 'NONE',  ( -15.72974639402176322, -15.80617190586768395, 99.37609039468568994 ) ) ;
#45452=CARTESIAN_POINT ( 'NONE',  ( -19.02544592524334988, -5.153800228976617603, 33.95942372801897591 ) ) ;
#45453=CARTESIAN_POINT ( 'NONE',  ( -16.55341960407617563, 4.379528057220093196, 98.54275706135234714 ) ) ;
#45454=CARTESIAN_POINT ( 'NONE',  ( -15.72974639402176322, -15.80617190586768395, 59.37609039468568284 ) ) ;
#45455=CARTESIAN_POINT ( 'NONE',  ( 5.049401038298161559, -19.05341960407611168, 52.70724293864767418 ) ) ;
#45456=CARTESIAN_POINT ( 'NONE',  ( -15.80617190586768217, 15.72974639402176855, 113.1260903946856899 ) ) ;
#45457=CARTESIAN_POINT ( 'NONE',  ( 5.153800228976335163, 19.02544592524342804, 114.7905762719810241 ) ) ;
#45458=CARTESIAN_POINT ( 'NONE',  ( -15.72974639402197994, 15.80617190586746368, 110.6239096053143669 ) ) ;
#45459=CARTESIAN_POINT ( 'NONE',  ( -21.53943276465977519, 0.05219959533907696930, 71.24890960531435269 ) ) ;
#45460=CARTESIAN_POINT ( 'NONE',  ( -4.379528057220086978, -16.55341960407618274, 44.79275706135234714 ) ) ;
#45462=CARTESIAN_POINT ( 'NONE',  ( -18.67979575497178146, -10.72451020669898902, 81.66557627198103830 ) ) ;
#45463=CARTESIAN_POINT ( 'NONE',  ( 12.14591786802327356, -12.06949235617739191, 60.62609039468567573 ) ) ;
#45464=CARTESIAN_POINT ( 'NONE',  ( -16.55341960407611168, -4.379528057220339221, 81.45724293864769550 ) ) ;
#45466=CARTESIAN_POINT ( 'NONE',  ( -13.97604488694547697, 13.89961937509957934, 108.1260903946856331 ) ) ;
#45467=CARTESIAN_POINT ( 'NONE',  ( -5.719274019375978568, 21.55341960407610458, 30.20724293864769550 ) ) ;
#45469=CARTESIAN_POINT ( 'NONE',  ( -16.55341960407617563, 4.379528057220093196, 43.54275706135235424 ) ) ;
#45470=CARTESIAN_POINT ( 'NONE',  ( 15.80617190586746368, 15.72974639402197994, 114.3739096053143527 ) ) ;
#45471=CARTESIAN_POINT ( 'NONE',  ( -21.52544592524343514, 5.823673210054127303, 36.04057627198102409 ) ) ;
#45472=CARTESIAN_POINT ( 'NONE',  ( 14.29746914071037800, 8.314922557961029526, 71.66775706135234714 ) ) ;
#45473=CARTESIAN_POINT ( 'NONE',  ( 9.564922557960805705, 16.46253265017160317, 79.58224293864769550 ) ) ;
#45474=CARTESIAN_POINT ( 'NONE',  ( 10.72451020669871369, 18.67979575497193778, 37.08442372801901143 ) ) ;
#45475=CARTESIAN_POINT ( 'NONE',  ( 16.55341960407618274, -4.379528057220086978, 21.04275706135234714 ) ) ;
#45476=CARTESIAN_POINT ( 'NONE',  ( -10.81492255796078084, -18.62759615963271287, 32.08224293864769550 ) ) ;
#45477=CARTESIAN_POINT ( 'NONE',  ( 13.89961937509957401, 13.97604488694547697, 21.87609039468566152 ) ) ;
#45478=CARTESIAN_POINT ( 'NONE',  ( -0.05219959533934338120, 16.53943276465976808, 52.50109039468567573 ) ) ;
#45479=CARTESIAN_POINT ( 'NONE',  ( -19.03943276465977164, 0.05219959533909376836, 101.2489096053143669 ) ) ;
#45480=CARTESIAN_POINT ( 'NONE',  ( 10.72451020669898902, -18.67979575497178502, 107.9155762719810241 ) ) ;
#45481=CARTESIAN_POINT ( 'NONE',  ( -9.564922557960796823, -16.46253265017161027, 72.08224293864770971 ) ) ;
#45484=CARTESIAN_POINT ( 'NONE',  ( -16.52544592524342804, 4.483927247898546575, 86.04057627198102409 ) ) ;
#45485=CARTESIAN_POINT ( 'NONE',  ( -21.52544592524343514, 5.823673210054127303, 36.04057627198102409 ) ) ;
#45486=CARTESIAN_POINT ( 'NONE',  ( -17.44279575226823908, 5.990770900252464948, 35.83557567514318976 ) ) ;
#45487=CARTESIAN_POINT ( 'NONE',  ( 4.483927247898790824, -16.52544592524335698, 60.20942372801902565 ) ) ;
#45488=CARTESIAN_POINT ( 'NONE',  ( -21.53943276465977519, -0.05219959533937600094, 18.75109039468568639 ) ) ;
#45489=CARTESIAN_POINT ( 'NONE',  ( 19.05341960407617918, -5.049401038297876454, 81.04275706135231871 ) ) ;
#45491=CARTESIAN_POINT ( 'NONE',  ( 5.719274019375991003, -21.55341960407610458, 62.70724293864769550 ) ) ;
#45492=CARTESIAN_POINT ( 'NONE',  ( -13.89961937509977652, 13.97604488694528158, 100.6239096053143669 ) ) ;
#45493=CARTESIAN_POINT ( 'NONE',  ( -21.53943276465977519, -0.05219959533937600094, 93.75109039468567573 ) ) ;
#45494=CARTESIAN_POINT ( 'NONE',  ( 9.564922557960805705, 16.46253265017160317, 64.58224293864769550 ) ) ;
#45495=CARTESIAN_POINT ( 'NONE',  ( -8.224510206698735004, -14.34966873604973081, 49.58442372801901143 ) ) ;
#45496=CARTESIAN_POINT ( 'NONE',  ( 0.05219959533909260263, 19.03943276465977164, 59.99890960531436690 ) ) ;
#45497=CARTESIAN_POINT ( 'NONE',  ( 21.55341960407619695, -5.719274019375665929, 81.04275706135236135 ) ) ;
#45498=ORIENTED_EDGE ( 'NONE', *, *, #174403, .T. ) ;
#45499=CARTESIAN_POINT ( 'NONE',  ( -16.46253265017146816, -9.564922557961047289, 39.16775706135234003 ) ) ;
#45500=CARTESIAN_POINT ( 'NONE',  ( -13.89961937509957401, -13.97604488694547875, 54.37609039468565442 ) ) ;
#45501=CARTESIAN_POINT ( 'NONE',  ( 15.72974639402176855, 15.80617190586768217, 46.87609039468568994 ) ) ;
#45502=CARTESIAN_POINT ( 'NONE',  ( 18.22780087662121673, 5.500000000000056843, 53.98459894673893444 ) ) ;
#45503=CARTESIAN_POINT ( 'NONE',  ( 13.89961937509957401, 13.97604488694547697, 51.87609039468566863 ) ) ;
#45504=CARTESIAN_POINT ( 'NONE',  ( 16.46253265017160672, -9.564922557960803928, 98.33224293864769550 ) ) ;
#45505=CARTESIAN_POINT ( 'NONE',  ( -0.05219959533909027116, -19.03943276465977164, 72.49890960531435269 ) ) ;
#45506=CARTESIAN_POINT ( 'NONE',  ( -14.34966873604960291, -8.224510206698953496, 26.66557627198103475 ) ) ;
#45507=CARTESIAN_POINT ( 'NONE',  ( 18.62759615963271287, -10.81492255796078972, 28.33224293864769550 ) ) ;
#45508=CARTESIAN_POINT ( 'NONE',  ( 21.55341960407619695, -5.719274019375665929, 96.04275706135236135 ) ) ;
#45511=CARTESIAN_POINT ( 'NONE',  ( -18.67979575497193778, 10.72451020669871902, 103.3344237280190043 ) ) ;
#45513=CARTESIAN_POINT ( 'NONE',  ( 9.474510206698971260, -16.51473224551069308, 22.91557627198102765 ) ) ;
#45514=CARTESIAN_POINT ( 'NONE',  ( 9.474510206698971260, -16.51473224551069308, 112.9155762719810383 ) ) ;
#45516=CARTESIAN_POINT ( 'NONE',  ( 0.05219959533934541429, -16.53943276465976808, 50.00109039468568994 ) ) ;
#45517=CARTESIAN_POINT ( 'NONE',  ( 15.72974639402199770, -15.80617190586745480, 73.12390960531436690 ) ) ;
#45519=CARTESIAN_POINT ( 'NONE',  ( 8.314922557960818139, 14.29746914071049879, 39.58224293864769550 ) ) ;
#45520=CARTESIAN_POINT ( 'NONE',  ( -16.52544592524342804, 4.483927247898546575, 106.0405762719810525 ) ) ;
#45521=CARTESIAN_POINT ( 'NONE',  ( -19.03943276465977164, 0.05219959533909376836, 96.24890960531436690 ) ) ;
#45522=CARTESIAN_POINT ( 'NONE',  ( 5.153800228976615827, -19.02544592524334988, 35.20942372801899722 ) ) ;
#45523=CARTESIAN_POINT ( 'NONE',  ( -9.564922557960796823, -16.46253265017161027, 22.08224293864768839 ) ) ;
#45524=CARTESIAN_POINT ( 'NONE',  ( -5.823673210054431948, 21.52544592524334988, 62.70942372801902565 ) ) ;
#45525=CARTESIAN_POINT ( 'NONE',  ( 18.22780087662123805, -5.499999999999976019, 98.51763182126896368 ) ) ;
#45526=CARTESIAN_POINT ( 'NONE',  ( 12.06949235617739724, 12.14591786802326823, 111.8760903946856615 ) ) ;
#45528=CARTESIAN_POINT ( 'NONE',  ( -10.81492255796078084, -18.62759615963271287, 27.08224293864769550 ) ) ;
#45529=CARTESIAN_POINT ( 'NONE',  ( 0.05219959533910956823, 16.53943276465976808, 94.99890960531436690 ) ) ;
#45530=CARTESIAN_POINT ( 'NONE',  ( -5.153800228976607833, 19.02544592524334988, 57.70942372801899012 ) ) ;
#45531=CARTESIAN_POINT ( 'NONE',  ( 0.05219959533909260263, 19.03943276465977164, 79.99890960531436690 ) ) ;
#45532=CARTESIAN_POINT ( 'NONE',  ( 12.06949235617757843, -12.14591786802309237, 78.12390960531436690 ) ) ;
#45533=CARTESIAN_POINT ( 'NONE',  ( 5.153800228976615827, -19.02544592524334988, 90.20942372801900433 ) ) ;
#45534=CARTESIAN_POINT ( 'NONE',  ( 18.67979575497178502, 10.72451020669898547, 44.16557627198103120 ) ) ;
#45535=ORIENTED_EDGE ( 'NONE', *, *, #73081, .T. ) ;
#45536=CARTESIAN_POINT ( 'NONE',  ( -5.049401038298153566, 19.05341960407611168, 25.20724293864768484 ) ) ;
#45537=CARTESIAN_POINT ( 'NONE',  ( -16.46253265017146816, -9.564922557961047289, 99.16775706135233293 ) ) ;
#45538=CARTESIAN_POINT ( 'NONE',  ( -9.564922557960796823, -16.46253265017161027, 67.08224293864769550 ) ) ;
#45539=CARTESIAN_POINT ( 'NONE',  ( -21.52544592524343514, 5.823673210054127303, 81.04057627198102409 ) ) ;
#45540=CARTESIAN_POINT ( 'NONE',  ( 8.314922557961029526, -14.29746914071037800, 85.41775706135236135 ) ) ;
#45541=CARTESIAN_POINT ( 'NONE',  ( 13.89961937509977652, -13.97604488694527269, 83.12390960531436690 ) ) ;
#45542=CARTESIAN_POINT ( 'NONE',  ( -19.05341960407617563, 5.049401038297882671, 68.54275706135230450 ) ) ;
#45543=CARTESIAN_POINT ( 'NONE',  ( -15.72974639402176322, -15.80617190586768395, 84.37609039468570415 ) ) ;
#45544=CARTESIAN_POINT ( 'NONE',  ( 5.823673210054125526, 21.52544592524343514, 59.79057627198103120 ) ) ;
#45545=CARTESIAN_POINT ( 'NONE',  ( 5.719274019375991003, -21.55341960407610458, 27.70724293864769905 ) ) ;
#45546=CARTESIAN_POINT ( 'NONE',  ( 5.153800228976335163, 19.02544592524342804, 39.79057627198100988 ) ) ;
#45547=CARTESIAN_POINT ( 'NONE',  ( 16.52544592524335698, 4.483927247898782831, 106.4594237280190328 ) ) ;
#45548=CARTESIAN_POINT ( 'NONE',  ( 5.153800228976335163, 19.02544592524342804, 44.79057627198103830 ) ) ;
#45549=CARTESIAN_POINT ( 'NONE',  ( -16.51473224551082808, 9.474510206698731452, 113.3344237280190043 ) ) ;
#45551=CARTESIAN_POINT ( 'NONE',  ( -15.72974639402176322, -15.80617190586768395, 109.3760903946857042 ) ) ;
#45552=CARTESIAN_POINT ( 'NONE',  ( 14.34966873604960469, 8.224510206698951720, 79.16557627198103830 ) ) ;
#45554=CARTESIAN_POINT ( 'NONE',  ( 0.05219959533907565091, 21.53943276465977519, 104.9989096053143669 ) ) ;
#45555=CARTESIAN_POINT ( 'NONE',  ( 0.05219959533907565091, 21.53943276465977519, 104.9989096053143669 ) ) ;
#45557=CARTESIAN_POINT ( 'NONE',  ( -5.823673210054116645, -21.52544592524344225, 47.29057627198103120 ) ) ;
#45558=CARTESIAN_POINT ( 'NONE',  ( -16.53943276465976808, -0.05219959533934237506, 78.75109039468568994 ) ) ;
#45559=CARTESIAN_POINT ( 'NONE',  ( -0.05219959533910754901, -16.53943276465976808, 107.4989096053143669 ) ) ;
#45560=CARTESIAN_POINT ( 'NONE',  ( 5.153800228976335163, 19.02544592524342804, 54.79057627198103120 ) ) ;
#45561=CARTESIAN_POINT ( 'NONE',  ( -18.56453257813361191, 5.500000000000043521, 50.99000423690686290 ) ) ;
#45562=CARTESIAN_POINT ( 'NONE',  ( -8.314922557960811034, -14.29746914071050412, 22.08224293864769194 ) ) ;
#45564=CARTESIAN_POINT ( 'NONE',  ( -18.67979575497193778, 10.72451020669871902, 53.33442372801901854 ) ) ;
#45565=CARTESIAN_POINT ( 'NONE',  ( -16.51473224551069308, -9.474510206698971260, 91.66557627198103830 ) ) ;
#45566=CARTESIAN_POINT ( 'NONE',  ( 15.72974639402176855, 15.80617190586768217, 86.87609039468568994 ) ) ;
#45567=CARTESIAN_POINT ( 'NONE',  ( -13.97604488694527625, -13.89961937509977652, 21.87390960531435979 ) ) ;
#45568=CARTESIAN_POINT ( 'NONE',  ( 9.474510206698971260, -16.51473224551069308, 22.91557627198102765 ) ) ;
#45569=VERTEX_POINT ( 'NONE', #14586 ) ;
#45570=CARTESIAN_POINT ( 'NONE',  ( 10.72451020669871369, 18.67979575497193778, 72.08442372801899012 ) ) ;
#45571=CARTESIAN_POINT ( 'NONE',  ( -19.02544592524342804, 5.153800228976336051, 51.04057627198103120 ) ) ;
#45572=CARTESIAN_POINT ( 'NONE',  ( 0.05219959533909260263, 19.03943276465977164, 99.99890960531436690 ) ) ;
#45573=CARTESIAN_POINT ( 'NONE',  ( 13.97604488694548053, -13.89961937509957401, 80.62609039468567573 ) ) ;
#45574=CARTESIAN_POINT ( 'NONE',  ( -18.67979575497193778, 10.72451020669871902, 38.33442372801900433 ) ) ;
#45575=CARTESIAN_POINT ( 'NONE',  ( -19.03943276465977164, -0.05219959533935918106, 103.7510903946856757 ) ) ;
#45576=CARTESIAN_POINT ( 'NONE',  ( 13.89961937509957401, 13.97604488694547697, 71.87609039468567573 ) ) ;
#45577=CARTESIAN_POINT ( 'NONE',  ( 19.05341960407611168, 5.049401038298154454, 43.95724293864769550 ) ) ;
#45578=CARTESIAN_POINT ( 'NONE',  ( -16.46253265017146816, -9.564922557961047289, 89.16775706135234714 ) ) ;
#45579=CARTESIAN_POINT ( 'NONE',  ( 4.379528057220092307, 16.55341960407617563, 107.2927570613523471 ) ) ;
#45580=CARTESIAN_POINT ( 'NONE',  ( 0.05219959533936267826, -19.03943276465977164, 75.00109039468566152 ) ) ;
#45581=CARTESIAN_POINT ( 'NONE',  ( -4.483927247898539470, -16.52544592524342804, 42.29057627198103120 ) ) ;
#45582=CARTESIAN_POINT ( 'NONE',  ( -5.153800228976607833, 19.02544592524334988, 67.70942372801900433 ) ) ;
#45583=CARTESIAN_POINT ( 'NONE',  ( 21.53943276465977519, 0.05219959533937863772, 101.2510903946856757 ) ) ;
#45584=CARTESIAN_POINT ( 'NONE',  ( -16.46253265017146816, -9.564922557961047289, 24.16775706135233648 ) ) ;
#45585=CARTESIAN_POINT ( 'NONE',  ( 19.02544592524343514, -5.153800228976328945, 33.54057627198102409 ) ) ;
#45587=CARTESIAN_POINT ( 'NONE',  ( -8.314922557961024197, 14.29746914071037800, 42.91775706135235424 ) ) ;
#45590=CARTESIAN_POINT ( 'NONE',  ( 13.97604488694527802, 13.89961937509977652, 94.37390960531436690 ) ) ;
#45593=CARTESIAN_POINT ( 'NONE',  ( -19.02544592524334988, -5.153800228976617603, 83.95942372801901854 ) ) ;
#45594=B_SPLINE_CURVE_WITH_KNOTS ( 'NONE', 3,
 ( #122054, #61373, #136243, #28099, #151424, #10921, #199909, #195955, #26097, #181763, #197918, #42258, #183746, #59387, #179787, #121061, #73596, #41256, #168559, #58408 ),
 .UNSPECIFIED., .F., .F.,
 ( 4, 2, 2, 2, 2, 2, 2, 2, 2, 4 ),
 ( 3.469446951953614189E-18, 0.0004987090165372655469, 0.0009974180330745276244, 0.001246772541343162512, 0.001496127049611797183, 0.001994836066149062188, 0.002493545082686327626, 0.002742899590954957743, 0.002992254099223588728, 0.003989672132298103559 ),
 .UNSPECIFIED. ) ;
#45595=CARTESIAN_POINT ( 'NONE',  ( -15.80617190586745835, -15.72974639402198527, 26.87390960531435979 ) ) ;
#45596=CARTESIAN_POINT ( 'NONE',  ( 19.05341960407617918, -5.049401038297876454, 21.04275706135232582 ) ) ;
#45597=CARTESIAN_POINT ( 'NONE',  ( 16.46253265017146816, 9.564922557961045513, 101.6677570613523329 ) ) ;
#45598=CARTESIAN_POINT ( 'NONE',  ( 4.483927247898545687, 16.52544592524342804, 114.7905762719810383 ) ) ;
#45599=CARTESIAN_POINT ( 'NONE',  ( -9.564922557960796823, -16.46253265017161027, 27.08224293864769550 ) ) ;
#45600=CARTESIAN_POINT ( 'NONE',  ( 15.80617190586746368, 15.72974639402197994, 64.37390960531435269 ) ) ;
#45601=CARTESIAN_POINT ( 'NONE',  ( 18.67979575497178502, 10.72451020669898547, 54.16557627198103120 ) ) ;
#45602=CARTESIAN_POINT ( 'NONE',  ( -16.46253265017160317, 9.564922557960807481, 25.83224293864769194 ) ) ;
#45604=CARTESIAN_POINT ( 'NONE',  ( -9.564922557961040184, 16.46253265017147172, 72.91775706135233293 ) ) ;
#45605=CARTESIAN_POINT ( 'NONE',  ( 16.52544592524342804, -4.483927247898539470, 38.54057627198103120 ) ) ;
#45606=CARTESIAN_POINT ( 'NONE',  ( 10.81492255796078972, 18.62759615963270932, 24.58224293864768839 ) ) ;
#45607=CARTESIAN_POINT ( 'NONE',  ( -0.05219959533937732626, 21.53943276465977519, 87.50109039468568994 ) ) ;
#45608=CARTESIAN_POINT ( 'NONE',  ( -21.52544592524343514, 5.823673210054127303, 76.04057627198102409 ) ) ;
#45609=B_SPLINE_CURVE_WITH_KNOTS ( 'NONE', 3,
 ( #133546, #132552, #102216, #118391, #88032, #85027 ),
 .UNSPECIFIED., .F., .F.,
 ( 4, 2, 4 ),
 ( 3.469446951953613804E-18, 0.0003837532665635201958, 0.0007675065331270369221 ),
 .UNSPECIFIED. ) ;
#45610=CARTESIAN_POINT ( 'NONE',  ( -18.62759615963255300, -10.81492255796106328, 64.16775706135234714 ) ) ;
#45611=CARTESIAN_POINT ( 'NONE',  ( 0.05219959533937995610, -21.53943276465977519, 50.00109039468568994 ) ) ;
#45612=CARTESIAN_POINT ( 'NONE',  ( -13.97604488694527625, -13.89961937509977652, 96.87390960531433848 ) ) ;
#45613=CARTESIAN_POINT ( 'NONE',  ( 14.29746914071037800, 8.314922557961029526, 91.66775706135234714 ) ) ;
#45614=CARTESIAN_POINT ( 'NONE',  ( 13.89961937509977652, -13.97604488694527269, 23.12390960531436335 ) ) ;
#45616=CARTESIAN_POINT ( 'NONE',  ( 8.224510206698953496, -14.34966873604960469, 67.91557627198102409 ) ) ;
#45617=CARTESIAN_POINT ( 'NONE',  ( 4.483927247898545687, 16.52544592524342804, 34.79057627198103120 ) ) ;
#45618=CARTESIAN_POINT ( 'NONE',  ( 9.474510206698971260, -16.51473224551069308, 62.91557627198102409 ) ) ;
#45619=CARTESIAN_POINT ( 'NONE',  ( 0.05219959533909260263, 19.03943276465977164, 29.99890960531435979 ) ) ;
#45620=CARTESIAN_POINT ( 'NONE',  ( -21.55341960407610458, -5.719274019375992779, 61.45724293864770260 ) ) ;
#45621=CARTESIAN_POINT ( 'NONE',  ( 19.03943276465977164, 0.05219959533936151252, 36.25109039468567573 ) ) ;
#45623=CARTESIAN_POINT ( 'NONE',  ( -14.29746914071049879, 8.314922557960819915, 45.83224293864769550 ) ) ;
#45624=CARTESIAN_POINT ( 'NONE',  ( -10.72451020669898014, 18.67979575497178502, 25.41557627198103120 ) ) ;
#45625=ORIENTED_EDGE ( 'NONE', *, *, #156075, .F. ) ;
#45627=CARTESIAN_POINT ( 'NONE',  ( -8.224510206698735004, -14.34966873604973081, 74.58442372801901854 ) ) ;
#45628=CARTESIAN_POINT ( 'NONE',  ( 9.474510206698729675, 16.51473224551082808, 72.08442372801900433 ) ) ;
#45629=CARTESIAN_POINT ( 'NONE',  ( -4.379528057220328563, 16.55341960407611168, 40.20724293864769550 ) ) ;
#45630=CARTESIAN_POINT ( 'NONE',  ( 16.38665767535058038, -7.295008042175997076, 52.76400864214550523 ) ) ;
#45631=CARTESIAN_POINT ( 'NONE',  ( 16.53943276465976808, -0.05219959533910856209, 33.74890960531436690 ) ) ;
#45632=CARTESIAN_POINT ( 'NONE',  ( -16.46253265017160317, 9.564922557960807481, 50.83224293864770260 ) ) ;
#45633=CARTESIAN_POINT ( 'NONE',  ( 13.89961937509977652, -13.97604488694527269, 78.12390960531433848 ) ) ;
#45634=CARTESIAN_POINT ( 'NONE',  ( 9.474510206698971260, -16.51473224551069308, 42.91557627198103120 ) ) ;
#45635=CARTESIAN_POINT ( 'NONE',  ( -15.80617190586768217, 15.72974639402176855, 43.12609039468568284 ) ) ;
#45636=CARTESIAN_POINT ( 'NONE',  ( -5.049401038298153566, 19.05341960407611168, 55.20724293864769550 ) ) ;
#45638=CARTESIAN_POINT ( 'NONE',  ( -16.51473224551069308, -9.474510206698971260, 56.66557627198103120 ) ) ;
#45639=CARTESIAN_POINT ( 'NONE',  ( 10.72451020669898902, -18.67979575497178502, 32.91557627198102409 ) ) ;
#45640=CARTESIAN_POINT ( 'NONE',  ( 19.05341960407611168, 5.049401038298154454, 23.95724293864769194 ) ) ;
#45641=CARTESIAN_POINT ( 'NONE',  ( -18.62759615963270932, 10.81492255796079327, 25.83224293864769194 ) ) ;
#45642=CARTESIAN_POINT ( 'NONE',  ( -8.314922557961024197, 14.29746914071037800, 87.91775706135234714 ) ) ;
#45644=CARTESIAN_POINT ( 'NONE',  ( 5.823673210054444382, -21.52544592524334988, 105.2094237280190328 ) ) ;
#45645=CARTESIAN_POINT ( 'NONE',  ( 8.314922557961029526, -14.29746914071037800, 70.41775706135236135 ) ) ;
#45646=CARTESIAN_POINT ( 'NONE',  ( -16.51473224551069308, -9.474510206698971260, 106.6655762719810383 ) ) ;
#45647=CARTESIAN_POINT ( 'NONE',  ( 14.34966873604972726, -8.224510206698740333, 50.83442372801901143 ) ) ;
#45648=CARTESIAN_POINT ( 'NONE',  ( -14.34966873604972548, 8.224510206698743886, 38.33442372801900433 ) ) ;
#45649=CARTESIAN_POINT ( 'NONE',  ( 14.29746914071037800, 8.314922557961029526, 101.6677570613523613 ) ) ;
#45650=CARTESIAN_POINT ( 'NONE',  ( -12.06949235617739369, -12.14591786802326823, 29.37609039468568284 ) ) ;
#45651=CARTESIAN_POINT ( 'NONE',  ( -16.51473224551069308, -9.474510206698971260, 36.66557627198102409 ) ) ;
#45652=CARTESIAN_POINT ( 'NONE',  ( 15.80617190586746368, 15.72974639402197994, 104.3739096053143669 ) ) ;
#45653=CARTESIAN_POINT ( 'NONE',  ( -12.06949235617739369, -12.14591786802326823, 19.37609039468568639 ) ) ;
#45654=CARTESIAN_POINT ( 'NONE',  ( 12.06949235617739724, 12.14591786802326823, 91.87609039468568994 ) ) ;
#45655=CARTESIAN_POINT ( 'NONE',  ( -17.13100169013226193, 6.664070546374124326, 45.76789835699824494 ) ) ;
#45656=CARTESIAN_POINT ( 'NONE',  ( -18.67979575497193778, 10.72451020669871902, 88.33442372801901854 ) ) ;
#45657=CARTESIAN_POINT ( 'NONE',  ( -16.46253265017146816, -9.564922557961047289, 84.16775706135233293 ) ) ;
#45658=CARTESIAN_POINT ( 'NONE',  ( 8.224510206698953496, -14.34966873604960469, 57.91557627198103120 ) ) ;
#45659=CARTESIAN_POINT ( 'NONE',  ( 12.06949235617757843, -12.14591786802309237, 43.12390960531435269 ) ) ;
#45660=CARTESIAN_POINT ( 'NONE',  ( -16.55341960407611168, -4.379528057220339221, 101.4572429386476955 ) ) ;
#45661=CARTESIAN_POINT ( 'NONE',  ( 16.46253265017146816, 9.564922557961045513, 41.66775706135234003 ) ) ;
#45663=CARTESIAN_POINT ( 'NONE',  ( 0.05219959533937995610, -21.53943276465977519, 50.00109039468568994 ) ) ;
#45664=CARTESIAN_POINT ( 'NONE',  ( -9.564922557961040184, 16.46253265017147172, 102.9177570613523329 ) ) ;
#45665=CARTESIAN_POINT ( 'NONE',  ( 17.48847506799968343, 5.747544572773809257, 81.67302562156720569 ) ) ;
#45666=CARTESIAN_POINT ( 'NONE',  ( -13.89961937509977652, 13.97604488694528158, 110.6239096053143243 ) ) ;
#45667=CARTESIAN_POINT ( 'NONE',  ( -5.719274019375978568, 21.55341960407610458, 70.20724293864769550 ) ) ;
#45668=CARTESIAN_POINT ( 'NONE',  ( -19.03943276465977164, -0.05219959533935918106, 98.75109039468567573 ) ) ;
#45669=CARTESIAN_POINT ( 'NONE',  ( -9.564922557960796823, -16.46253265017161027, 107.0822429386476955 ) ) ;
#45670=CARTESIAN_POINT ( 'NONE',  ( -5.049401038297874678, -19.05341960407618274, 49.79275706135232582 ) ) ;
#45671=CARTESIAN_POINT ( 'NONE',  ( -14.29746914071049879, 8.314922557960819915, 105.8322429386476955 ) ) ;
#45672=CARTESIAN_POINT ( 'NONE',  ( 15.80617190586769283, -15.72974639402175789, 100.6260903946857184 ) ) ;
#45673=CARTESIAN_POINT ( 'NONE',  ( 9.474510206698971260, -16.51473224551069308, 37.91557627198102409 ) ) ;
#45674=CARTESIAN_POINT ( 'NONE',  ( -15.80617190586768217, 15.72974639402176855, 48.12609039468568284 ) ) ;
#45675=CARTESIAN_POINT ( 'NONE',  ( -10.81492255796105439, 18.62759615963255655, 87.91775706135234714 ) ) ;
#45676=CARTESIAN_POINT ( 'NONE',  ( -16.53943276465976808, -0.05219959533934237506, 88.75109039468567573 ) ) ;
#45677=CARTESIAN_POINT ( 'NONE',  ( 5.719274019375673035, 21.55341960407619339, 47.29275706135234003 ) ) ;
#45678=CARTESIAN_POINT ( 'NONE',  ( 21.52544592524334988, 5.823673210054432836, 46.45942372801901854 ) ) ;
#45679=CARTESIAN_POINT ( 'NONE',  ( -16.51473224551082808, 9.474510206698731452, 63.33442372801900433 ) ) ;
#45680=CARTESIAN_POINT ( 'NONE',  ( -16.46253265017160317, 9.564922557960807481, 95.83224293864769550 ) ) ;
#45681=CARTESIAN_POINT ( 'NONE',  ( -16.55341960407611168, -4.379528057220339221, 101.4572429386476955 ) ) ;
#45682=CARTESIAN_POINT ( 'NONE',  ( 21.52544592524344225, -5.823673210054117533, 88.54057627198103830 ) ) ;
#45683=CARTESIAN_POINT ( 'NONE',  ( 16.52544592524342804, -4.483927247898539470, 63.54057627198103830 ) ) ;
#45684=CARTESIAN_POINT ( 'NONE',  ( 10.81492255796106328, -18.62759615963255655, 105.4177570613523613 ) ) ;
#45685=CARTESIAN_POINT ( 'NONE',  ( -8.314922557960811034, -14.29746914071050412, 87.08224293864769550 ) ) ;
#45686=CARTESIAN_POINT ( 'NONE',  ( 16.51473224551069308, 9.474510206698969483, 34.16557627198102409 ) ) ;
#45687=CARTESIAN_POINT ( 'NONE',  ( 5.153800228976615827, -19.02544592524334988, 80.20942372801901854 ) ) ;
#45688=CARTESIAN_POINT ( 'NONE',  ( 12.06949235617757843, -12.14591786802309237, 48.12390960531436690 ) ) ;
#45689=CARTESIAN_POINT ( 'NONE',  ( 0.05219959533937995610, -21.53943276465977519, 90.00109039468567573 ) ) ;
#45690=CARTESIAN_POINT ( 'NONE',  ( -0.05219959533909027116, -19.03943276465977164, 92.49890960531436690 ) ) ;
#45691=CARTESIAN_POINT ( 'NONE',  ( 9.474510206698729675, 16.51473224551082808, 57.08442372801900433 ) ) ;
#45692=CARTESIAN_POINT ( 'NONE',  ( -15.72974639402197994, 15.80617190586746368, 70.62390960531436690 ) ) ;
#45693=CARTESIAN_POINT ( 'NONE',  ( 18.67979575497194134, -10.72451020669871369, 20.83442372801901143 ) ) ;
#45694=CARTESIAN_POINT ( 'NONE',  ( 16.53943276465976808, 0.05219959533934440121, 26.25109039468567573 ) ) ;
#45695=CARTESIAN_POINT ( 'NONE',  ( -16.52544592524335698, -4.483927247898792601, 83.95942372801900433 ) ) ;
#45696=CARTESIAN_POINT ( 'NONE',  ( 5.153800228976335163, 19.02544592524342804, 24.79057627198102765 ) ) ;
#45697=CARTESIAN_POINT ( 'NONE',  ( 10.72451020669871369, 18.67979575497193778, 27.08442372801901854 ) ) ;
#45698=CARTESIAN_POINT ( 'NONE',  ( -14.29746914071049879, 8.314922557960819915, 115.8322429386477097 ) ) ;
#45700=CARTESIAN_POINT ( 'NONE',  ( -8.314922557961024197, 14.29746914071037800, 52.91775706135235424 ) ) ;
#45701=CARTESIAN_POINT ( 'NONE',  ( 14.29746914071049879, -8.314922557960816363, 78.33224293864770971 ) ) ;
#45702=CARTESIAN_POINT ( 'NONE',  ( -15.80617190586745835, -15.72974639402198527, 81.87390960531435269 ) ) ;
#45703=CARTESIAN_POINT ( 'NONE',  ( -16.52544592524342804, 4.483927247898546575, 31.04057627198102409 ) ) ;
#45704=CARTESIAN_POINT ( 'NONE',  ( -16.52544592524335698, -4.483927247898792601, 33.95942372801901143 ) ) ;
#45705=CARTESIAN_POINT ( 'NONE',  ( -19.05341960407611168, -5.049401038298163336, 46.45724293864768129 ) ) ;
#45706=CARTESIAN_POINT ( 'NONE',  ( 4.483927247898790824, -16.52544592524335698, 75.20942372801901854 ) ) ;
#45707=CARTESIAN_POINT ( 'NONE',  ( 5.153800228976615827, -19.02544592524334988, 80.20942372801901854 ) ) ;
#45708=CARTESIAN_POINT ( 'NONE',  ( -18.67979575497178146, -10.72451020669898902, 71.66557627198100988 ) ) ;
#45709=CARTESIAN_POINT ( 'NONE',  ( -8.314922557961024197, 14.29746914071037800, 107.9177570613523471 ) ) ;
#45712=CARTESIAN_POINT ( 'NONE',  ( -5.719274019375978568, 21.55341960407610458, 45.20724293864769550 ) ) ;
#45714=CARTESIAN_POINT ( 'NONE',  ( -14.34966873604972548, 8.224510206698743886, 88.33442372801901854 ) ) ;
#45715=CARTESIAN_POINT ( 'NONE',  ( 15.80617190586746368, 15.72974639402197994, 49.37390960531436690 ) ) ;
#45717=CARTESIAN_POINT ( 'NONE',  ( -19.05341960407611168, -5.049401038298163336, 111.4572429386476671 ) ) ;
#45719=CARTESIAN_POINT ( 'NONE',  ( 5.153800228976335163, 19.02544592524342804, 24.79057627198102765 ) ) ;
#45720=CARTESIAN_POINT ( 'NONE',  ( 21.53943276465977519, -0.05219959533907433946, 73.74890960531433848 ) ) ;
#45721=CARTESIAN_POINT ( 'NONE',  ( -16.53943276465976808, -0.05219959533934237506, 103.7510903946857042 ) ) ;
#45722=CARTESIAN_POINT ( 'NONE',  ( 10.72451020669871369, 18.67979575497193778, 62.08442372801901143 ) ) ;
#45723=CARTESIAN_POINT ( 'NONE',  ( -16.55341960407617563, 4.379528057220093196, 23.54275706135235424 ) ) ;
#45724=CARTESIAN_POINT ( 'NONE',  ( -16.46253265017160317, 9.564922557960807481, 25.83224293864769194 ) ) ;
#45725=CARTESIAN_POINT ( 'NONE',  ( -16.52544592524335698, -4.483927247898792601, 33.95942372801901143 ) ) ;
#45726=CARTESIAN_POINT ( 'NONE',  ( -19.05341960407611168, -5.049401038298163336, 46.45724293864768129 ) ) ;
#45727=EDGE_CURVE ( 'NONE', #15160, #151905, #133188, .T. ) ;
#45729=CARTESIAN_POINT ( 'NONE',  ( -19.05341960407611168, -5.049401038298163336, 111.4572429386476671 ) ) ;
#45730=CARTESIAN_POINT ( 'NONE',  ( -14.34966873604972548, 8.224510206698743886, 88.33442372801901854 ) ) ;
#45731=CARTESIAN_POINT ( 'NONE',  ( 13.97604488694548053, -13.89961937509957401, 95.62609039468563310 ) ) ;
#45732=CARTESIAN_POINT ( 'NONE',  ( -15.80617190586768217, 15.72974639402176855, 113.1260903946856899 ) ) ;
#45733=CARTESIAN_POINT ( 'NONE',  ( -21.52544592524343514, 5.823673210054127303, 81.04057627198102409 ) ) ;
#45734=CARTESIAN_POINT ( 'NONE',  ( 8.314922557961029526, -14.29746914071037800, 100.4177570613523471 ) ) ;
#45735=CARTESIAN_POINT ( 'NONE',  ( -9.474510206698720793, -16.51473224551083518, 99.58442372801900433 ) ) ;
#45736=CARTESIAN_POINT ( 'NONE',  ( -13.97604488694527625, -13.89961937509977652, 51.87390960531436690 ) ) ;
#45737=CARTESIAN_POINT ( 'NONE',  ( -9.474510206698964154, 16.51473224551069663, 90.41557627198103830 ) ) ;
#45738=CARTESIAN_POINT ( 'NONE',  ( 5.823673210054444382, -21.52544592524334988, 50.20942372801901854 ) ) ;
#45739=CARTESIAN_POINT ( 'NONE',  ( 9.564922557960805705, 16.46253265017160317, 49.58224293864770260 ) ) ;
#45741=CARTESIAN_POINT ( 'NONE',  ( 19.02544592524343514, -5.153800228976328945, 113.5405762719810241 ) ) ;
#45742=CARTESIAN_POINT ( 'NONE',  ( -16.52544592524342804, 4.483927247898546575, 71.04057627198103830 ) ) ;
#45743=CARTESIAN_POINT ( 'NONE',  ( -15.72974639402197994, 15.80617190586746368, 70.62390960531436690 ) ) ;
#45745=CARTESIAN_POINT ( 'NONE',  ( 19.02544592524334988, 5.153800228976608722, 36.45942372801900433 ) ) ;
#45747=CARTESIAN_POINT ( 'NONE',  ( 9.474510206698971260, -16.51473224551069308, 67.91557627198102409 ) ) ;
#45748=CARTESIAN_POINT ( 'NONE',  ( -9.474510206698964154, 16.51473224551069663, 90.41557627198103830 ) ) ;
#45749=CARTESIAN_POINT ( 'NONE',  ( -14.29746914071037622, -8.314922557961029526, 49.16775706135234003 ) ) ;
#45751=CARTESIAN_POINT ( 'NONE',  ( 19.05341960407617918, -5.049401038297876454, 26.04275706135233293 ) ) ;
#45753=CARTESIAN_POINT ( 'NONE',  ( -14.34966873604972548, 8.224510206698743886, 88.33442372801901854 ) ) ;
#45755=CARTESIAN_POINT ( 'NONE',  ( 0.05219959533934541429, -16.53943276465976808, 85.00109039468568994 ) ) ;
#45756=CARTESIAN_POINT ( 'NONE',  ( -4.483927247898782831, 16.52544592524335698, 57.70942372801901143 ) ) ;
#45757=CARTESIAN_POINT ( 'NONE',  ( -13.89961937509957401, -13.97604488694547875, 29.37609039468565797 ) ) ;
#45758=CARTESIAN_POINT ( 'NONE',  ( 16.51473224551069308, 9.474510206698969483, 59.16557627198102409 ) ) ;
#45760=CARTESIAN_POINT ( 'NONE',  ( 21.52544592524334988, 5.823673210054432836, 71.45942372801901854 ) ) ;
#45761=CARTESIAN_POINT ( 'NONE',  ( 5.153800228976615827, -19.02544592524334988, 80.20942372801901854 ) ) ;
#45762=CARTESIAN_POINT ( 'NONE',  ( 0.05219959533937995610, -21.53943276465977519, 110.0010903946856757 ) ) ;
#45763=CARTESIAN_POINT ( 'NONE',  ( -9.564922557960796823, -16.46253265017161027, 47.08224293864769550 ) ) ;
#45765=CARTESIAN_POINT ( 'NONE',  ( -18.62759615963270932, 10.81492255796079327, 70.83224293864770971 ) ) ;
#45766=CARTESIAN_POINT ( 'NONE',  ( -21.53943276465977519, 0.05219959533907696930, 21.24890960531436690 ) ) ;
#45767=CARTESIAN_POINT ( 'NONE',  ( 12.06949235617757843, -12.14591786802309237, 113.1239096053143953 ) ) ;
#45768=CARTESIAN_POINT ( 'NONE',  ( 14.29746914071037800, 8.314922557961029526, 51.66775706135234714 ) ) ;
#45769=CARTESIAN_POINT ( 'NONE',  ( 16.55341960407611168, 4.379528057220329451, 28.95724293864769905 ) ) ;
#45771=CARTESIAN_POINT ( 'NONE',  ( -10.72451020669870658, -18.67979575497194134, 19.58442372801901143 ) ) ;
#45772=CARTESIAN_POINT ( 'NONE',  ( -16.55341960407611168, -4.379528057220339221, 46.45724293864769550 ) ) ;
#45775=CARTESIAN_POINT ( 'NONE',  ( -19.03943276465977164, -0.05219959533935918106, 103.7510903946856757 ) ) ;
#45776=CARTESIAN_POINT ( 'NONE',  ( 13.89961937509957401, 13.97604488694547697, 41.87609039468566152 ) ) ;
#45777=CARTESIAN_POINT ( 'NONE',  ( -8.224510206698948167, 14.34966873604960824, 45.41557627198103830 ) ) ;
#45778=CARTESIAN_POINT ( 'NONE',  ( -18.62759615963270932, 10.81492255796079327, 100.8322429386477097 ) ) ;
#45779=CARTESIAN_POINT ( 'NONE',  ( 16.79531203550651242, 7.028104445595491079, 33.75244988220442366 ) ) ;
#45780=CARTESIAN_POINT ( 'NONE',  ( 15.80617190586746368, 15.72974639402197994, 64.37390960531435269 ) ) ;
#45781=CARTESIAN_POINT ( 'NONE',  ( 16.51473224551069308, 9.474510206698969483, 79.16557627198103830 ) ) ;
#45782=CARTESIAN_POINT ( 'NONE',  ( -16.52544592524342804, 4.483927247898546575, 51.04057627198103120 ) ) ;
#45783=CARTESIAN_POINT ( 'NONE',  ( 5.153800228976335163, 19.02544592524342804, 99.79057627198102409 ) ) ;
#45784=CARTESIAN_POINT ( 'NONE',  ( -17.49999999999999645, 5.499999999999997335, 120.0000000000000142 ) ) ;
#45785=CARTESIAN_POINT ( 'NONE',  ( -16.46253265017146816, -9.564922557961047289, 54.16775706135234003 ) ) ;
#45786=CARTESIAN_POINT ( 'NONE',  ( 10.72451020669898902, -18.67979575497178502, 92.91557627198103830 ) ) ;
#45787=CARTESIAN_POINT ( 'NONE',  ( 19.02544592524343514, -5.153800228976328945, 43.54057627198103120 ) ) ;
#45788=CARTESIAN_POINT ( 'NONE',  ( -12.14591786802309592, -12.06949235617757132, 111.8739096053143669 ) ) ;
#45789=CARTESIAN_POINT ( 'NONE',  ( -0.05219959533937732626, 21.53943276465977519, 52.50109039468567573 ) ) ;
#45791=CARTESIAN_POINT ( 'NONE',  ( 8.314922557960818139, 14.29746914071049879, 24.58224293864768839 ) ) ;
#45792=CARTESIAN_POINT ( 'NONE',  ( 19.05341960407611168, 5.049401038298154454, 48.95724293864768129 ) ) ;
#45793=CARTESIAN_POINT ( 'NONE',  ( -5.153800228976328057, -19.02544592524343514, 97.29057627198099567 ) ) ;
#45794=CARTESIAN_POINT ( 'NONE',  ( 10.81492255796078972, 18.62759615963270932, 59.58224293864770260 ) ) ;
#45795=CARTESIAN_POINT ( 'NONE',  ( -19.02130022317637525, 5.499999999999598543, 45.78188669246576836 ) ) ;
#45796=CARTESIAN_POINT ( 'NONE',  ( -19.05341960407611168, -5.049401038298163336, 41.45724293864769550 ) ) ;
#45797=CARTESIAN_POINT ( 'NONE',  ( 10.81492255796078972, 18.62759615963270932, 49.58224293864769550 ) ) ;
#45798=CARTESIAN_POINT ( 'NONE',  ( -15.80617190586768217, 15.72974639402176855, 88.12609039468570415 ) ) ;
#45800=CARTESIAN_POINT ( 'NONE',  ( -14.34966873604972548, 8.224510206698743886, 88.33442372801901854 ) ) ;
#45801=CARTESIAN_POINT ( 'NONE',  ( 16.52544592524335698, 4.483927247898782831, 91.45942372801901854 ) ) ;
#45802=CARTESIAN_POINT ( 'NONE',  ( -13.97604488694527625, -13.89961937509977652, 66.87390960531436690 ) ) ;
#45805=CARTESIAN_POINT ( 'NONE',  ( -9.564922557961040184, 16.46253265017147172, 22.91775706135233648 ) ) ;
#45806=CARTESIAN_POINT ( 'NONE',  ( -12.14591786802326823, 12.06949235617739902, 88.12609039468570415 ) ) ;
#45807=CARTESIAN_POINT ( 'NONE',  ( 21.52544592524334988, 5.823673210054432836, 111.4594237280190328 ) ) ;
#45808=CARTESIAN_POINT ( 'NONE',  ( 9.564922557960805705, 16.46253265017160317, 79.58224293864769550 ) ) ;
#45809=CARTESIAN_POINT ( 'NONE',  ( 10.81492255796078972, 18.62759615963270932, 54.58224293864769550 ) ) ;
#45810=CARTESIAN_POINT ( 'NONE',  ( 4.379528057220092307, 16.55341960407617563, 22.29275706135235069 ) ) ;
#45811=CARTESIAN_POINT ( 'NONE',  ( 21.52544592524334988, 5.823673210054432836, 76.45942372801901854 ) ) ;
#45812=CARTESIAN_POINT ( 'NONE',  ( -8.314922557961024197, 14.29746914071037800, 62.91775706135236135 ) ) ;
#45813=CARTESIAN_POINT ( 'NONE',  ( -5.719274019375978568, 21.55341960407610458, 115.2072429386476955 ) ) ;
#45814=CARTESIAN_POINT ( 'NONE',  ( 19.02544592524334988, 5.153800228976608722, 106.4594237280190185 ) ) ;
#45815=CARTESIAN_POINT ( 'NONE',  ( 13.97604488694527802, 13.89961937509977652, 74.37390960531436690 ) ) ;
#45816=CARTESIAN_POINT ( 'NONE',  ( 0.05219959533934541429, -16.53943276465976808, 30.00109039468568284 ) ) ;
#45817=CARTESIAN_POINT ( 'NONE',  ( 16.46253265017160672, -9.564922557960803928, 38.33224293864768839 ) ) ;
#45818=CARTESIAN_POINT ( 'NONE',  ( -5.153800228976607833, 19.02544592524334988, 112.7094237280190043 ) ) ;
#45819=CARTESIAN_POINT ( 'NONE',  ( 14.29746914071049879, -8.314922557960816363, 78.33224293864770971 ) ) ;
#45820=CARTESIAN_POINT ( 'NONE',  ( -8.224510206698735004, -14.34966873604973081, 84.58442372801903275 ) ) ;
#45821=CARTESIAN_POINT ( 'NONE',  ( -21.52544592524334988, -5.823673210054445271, 33.95942372801901143 ) ) ;
#45822=CARTESIAN_POINT ( 'NONE',  ( -19.05341960407611168, -5.049401038298163336, 66.45724293864769550 ) ) ;
#45823=CARTESIAN_POINT ( 'NONE',  ( 19.02544592524343514, -5.153800228976328945, 63.54057627198103830 ) ) ;
#45824=CARTESIAN_POINT ( 'NONE',  ( 8.314922557961029526, -14.29746914071037800, 80.41775706135234714 ) ) ;
#45826=ORIENTED_EDGE ( 'NONE', *, *, #34324, .T. ) ;
#45828=CARTESIAN_POINT ( 'NONE',  ( 19.03943276465977164, 0.05219959533936151252, 26.25109039468566507 ) ) ;
#45829=CARTESIAN_POINT ( 'NONE',  ( -13.97604488694527625, -13.89961937509977652, 41.87390960531435979 ) ) ;
#45832=CARTESIAN_POINT ( 'NONE',  ( 0.05219959533934541429, -16.53943276465976808, 30.00109039468568284 ) ) ;
#45833=CARTESIAN_POINT ( 'NONE',  ( -19.03943276465977164, -0.05219959533935918106, 58.75109039468566863 ) ) ;
#45834=CARTESIAN_POINT ( 'NONE',  ( -8.314922557961024197, 14.29746914071037800, 42.91775706135235424 ) ) ;
#45835=CARTESIAN_POINT ( 'NONE',  ( 5.049401038298161559, -19.05341960407611168, 102.7072429386476955 ) ) ;
#45836=CARTESIAN_POINT ( 'NONE',  ( 13.89961937509977652, -13.97604488694527269, 63.12390960531435979 ) ) ;
#45837=CARTESIAN_POINT ( 'NONE',  ( -18.62759615963270932, 10.81492255796079327, 105.8322429386476955 ) ) ;
#45838=CARTESIAN_POINT ( 'NONE',  ( -16.46253265017160317, 9.564922557960807481, 95.83224293864769550 ) ) ;
#45840=CARTESIAN_POINT ( 'NONE',  ( -9.564922557960796823, -16.46253265017161027, 62.08224293864769550 ) ) ;
#45841=CARTESIAN_POINT ( 'NONE',  ( -12.14591786802309592, -12.06949235617757132, 26.87390960531435979 ) ) ;
#45842=CARTESIAN_POINT ( 'NONE',  ( -19.02544592524342804, 5.153800228976336051, 26.04057627198103120 ) ) ;
#45843=CARTESIAN_POINT ( 'NONE',  ( -19.05341960407617563, 5.049401038297882671, 33.54275706135231871 ) ) ;
#45844=CARTESIAN_POINT ( 'NONE',  ( 12.06949235617757843, -12.14591786802309237, 68.12390960531436690 ) ) ;
#45845=CARTESIAN_POINT ( 'NONE',  ( -0.05219959533937732626, 21.53943276465977519, 92.50109039468567573 ) ) ;
#45846=CARTESIAN_POINT ( 'NONE',  ( 13.97604488694527802, 13.89961937509977652, 44.37390960531435269 ) ) ;
#45847=CARTESIAN_POINT ( 'NONE',  ( 12.14591786802327356, -12.06949235617739191, 50.62609039468568994 ) ) ;
#45848=CARTESIAN_POINT ( 'NONE',  ( 14.34966873604960469, 8.224510206698951720, 39.16557627198102409 ) ) ;
#45849=CARTESIAN_POINT ( 'NONE',  ( -18.62759615963255300, -10.81492255796106328, 89.16775706135236135 ) ) ;
#45850=CARTESIAN_POINT ( 'NONE',  ( 5.049401038298161559, -19.05341960407611168, 77.70724293864765286 ) ) ;
#45851=CARTESIAN_POINT ( 'NONE',  ( 5.153800228976335163, 19.02544592524342804, 99.79057627198102409 ) ) ;
#45852=CARTESIAN_POINT ( 'NONE',  ( 8.224510206698953496, -14.34966873604960469, 112.9155762719810383 ) ) ;
#45853=CARTESIAN_POINT ( 'NONE',  ( -14.29746914071049879, 8.314922557960819915, 75.83224293864769550 ) ) ;
#45854=CARTESIAN_POINT ( 'NONE',  ( 18.62759615963271287, -10.81492255796078972, 88.33224293864769550 ) ) ;
#45855=CARTESIAN_POINT ( 'NONE',  ( 9.474510206698971260, -16.51473224551069308, 82.91557627198103830 ) ) ;
#45856=CARTESIAN_POINT ( 'NONE',  ( -15.80617190586745835, -15.72974639402198527, 101.8739096053143811 ) ) ;
#45857=CARTESIAN_POINT ( 'NONE',  ( -9.564922557961040184, 16.46253265017147172, 72.91775706135233293 ) ) ;
#45858=CARTESIAN_POINT ( 'NONE',  ( 18.39635199886966532, -5.500000000000095035, 48.51967076359998288 ) ) ;
#45859=CARTESIAN_POINT ( 'NONE',  ( -12.06949235617756955, 12.14591786802309770, 85.62390960531436690 ) ) ;
#45860=CARTESIAN_POINT ( 'NONE',  ( -9.564922557960796823, -16.46253265017161027, 52.08224293864768839 ) ) ;
#45861=CARTESIAN_POINT ( 'NONE',  ( -10.72451020669898014, 18.67979575497178502, 65.41557627198102409 ) ) ;
#45863=CARTESIAN_POINT ( 'NONE',  ( -14.29746914071049879, 8.314922557960819915, 25.83224293864769194 ) ) ;
#45865=CARTESIAN_POINT ( 'NONE',  ( -16.51473224551082808, 9.474510206698731452, 113.3344237280190043 ) ) ;
#45866=CARTESIAN_POINT ( 'NONE',  ( -16.53943276465976808, 0.05219959533911058130, 76.24890960531435269 ) ) ;
#45868=CARTESIAN_POINT ( 'NONE',  ( 0.05219959533909260263, 19.03943276465977164, 69.99890960531435269 ) ) ;
#45869=CARTESIAN_POINT ( 'NONE',  ( 5.049401038298161559, -19.05341960407611168, 27.70724293864769550 ) ) ;
#45870=CARTESIAN_POINT ( 'NONE',  ( -14.34966873604960291, -8.224510206698953496, 71.66557627198100988 ) ) ;
#45871=CARTESIAN_POINT ( 'NONE',  ( 5.049401038298161559, -19.05341960407611168, 112.7072429386476813 ) ) ;
#45872=CARTESIAN_POINT ( 'NONE',  ( -5.153800228976607833, 19.02544592524334988, 82.70942372801897591 ) ) ;
#45873=CARTESIAN_POINT ( 'NONE',  ( 0.05219959533909260263, 19.03943276465977164, 104.9989096053143669 ) ) ;
#45874=CARTESIAN_POINT ( 'NONE',  ( -21.53943276465977519, 0.05219959533907696930, 71.24890960531435269 ) ) ;
#45875=CARTESIAN_POINT ( 'NONE',  ( 12.14591786802327356, -12.06949235617739191, 70.62609039468567573 ) ) ;
#45876=CARTESIAN_POINT ( 'NONE',  ( 19.05341960407618274, -5.049401038297876454, 106.0427570613523471 ) ) ;
#45877=CARTESIAN_POINT ( 'NONE',  ( 9.564922557960805705, 16.46253265017160317, 59.58224293864769550 ) ) ;
#45878=CARTESIAN_POINT ( 'NONE',  ( 10.72451020669898902, -18.67979575497178502, 62.91557627198102409 ) ) ;
#45879=CARTESIAN_POINT ( 'NONE',  ( -19.03943276465977164, -0.05219959533935918106, 108.7510903946856615 ) ) ;
#45880=CARTESIAN_POINT ( 'NONE',  ( -12.06949235617756955, 12.14591786802309770, 35.62390960531437401 ) ) ;
#45881=CARTESIAN_POINT ( 'NONE',  ( -21.53943276465977519, -0.05219959533937600094, 58.75109039468568994 ) ) ;
#45882=EDGE_CURVE ( 'NONE', #15494, #63455, #152090, .T. ) ;
#45884=CARTESIAN_POINT ( 'NONE',  ( -12.06949235617739369, -12.14591786802326823, 79.37609039468567573 ) ) ;
#45885=CARTESIAN_POINT ( 'NONE',  ( 9.564922557960805705, 16.46253265017160317, 104.5822429386476955 ) ) ;
#45886=CARTESIAN_POINT ( 'NONE',  ( -15.49999999999999822, -5.500000000000000888, 118.0000000000000142 ) ) ;
#45888=CARTESIAN_POINT ( 'NONE',  ( 4.379528057220092307, 16.55341960407617563, 92.29275706135236135 ) ) ;
#45889=CARTESIAN_POINT ( 'NONE',  ( 12.06949235617739724, 12.14591786802326823, 46.87609039468568994 ) ) ;
#45890=CARTESIAN_POINT ( 'NONE',  ( 5.049401038298161559, -19.05341960407611168, 57.70724293864769550 ) ) ;
#45891=CARTESIAN_POINT ( 'NONE',  ( 19.05341960407611168, 5.049401038298154454, 73.95724293864768129 ) ) ;
#45892=CARTESIAN_POINT ( 'NONE',  ( -10.72451020669870658, -18.67979575497194134, 54.58442372801901143 ) ) ;
#45893=CARTESIAN_POINT ( 'NONE',  ( 12.06949235617739724, 12.14591786802326823, 66.87609039468568994 ) ) ;
#45894=CARTESIAN_POINT ( 'NONE',  ( 16.52544592524342804, -4.483927247898539470, 28.54057627198103120 ) ) ;
#45895=CARTESIAN_POINT ( 'NONE',  ( -5.153800228976328057, -19.02544592524343514, 42.29057627198101699 ) ) ;
#45896=CARTESIAN_POINT ( 'NONE',  ( -19.02544592524342804, 5.153800228976336051, 41.04057627198103120 ) ) ;
#45897=CARTESIAN_POINT ( 'NONE',  ( 4.379528057220092307, 16.55341960407617563, 27.29275706135234358 ) ) ;
#45898=CARTESIAN_POINT ( 'NONE',  ( 5.049401038297881783, 19.05341960407617563, 77.29275706135231871 ) ) ;
#45899=CARTESIAN_POINT ( 'NONE',  ( -16.55341960407611168, -4.379528057220339221, 101.4572429386476955 ) ) ;
#45900=CARTESIAN_POINT ( 'NONE',  ( -19.02544592524342804, 5.153800228976336051, 51.04057627198103120 ) ) ;
#45901=CARTESIAN_POINT ( 'NONE',  ( 5.049401038297881783, 19.05341960407617563, 82.29275706135229029 ) ) ;
#45903=CARTESIAN_POINT ( 'NONE',  ( -5.719274019375665041, -21.55341960407619695, 89.79275706135236135 ) ) ;
#45904=CARTESIAN_POINT ( 'NONE',  ( 16.53943276465976808, 0.05219959533934440121, 56.25109039468568284 ) ) ;
#45906=CARTESIAN_POINT ( 'NONE',  ( -21.52544592524343514, 5.823673210054127303, 51.04057627198103120 ) ) ;
#45907=CARTESIAN_POINT ( 'NONE',  ( 16.53943276465976808, 0.05219959533934440121, 41.25109039468568284 ) ) ;
#45908=CARTESIAN_POINT ( 'NONE',  ( -19.02544592524342804, 5.153800228976336939, 36.04057627198101699 ) ) ;
#45909=CARTESIAN_POINT ( 'NONE',  ( 16.46253265017146816, 9.564922557961045513, 41.66775706135234003 ) ) ;
#45910=CARTESIAN_POINT ( 'NONE',  ( 19.02544592524343514, -5.153800228976328945, 88.54057627198102409 ) ) ;
#45911=CARTESIAN_POINT ( 'NONE',  ( 19.02544592524343514, -5.153800228976328945, 48.54057627198103120 ) ) ;
#45913=CARTESIAN_POINT ( 'NONE',  ( 21.52544592524334988, 5.823673210054432836, 71.45942372801901854 ) ) ;
#45915=CARTESIAN_POINT ( 'NONE',  ( 5.049401038297881783, 19.05341960407617563, 37.29275706135232582 ) ) ;
#45916=CARTESIAN_POINT ( 'NONE',  ( 15.80617190586769283, -15.72974639402175789, 105.6260903946856899 ) ) ;
#45917=CARTESIAN_POINT ( 'NONE',  ( -14.29746914071049879, 8.314922557960819915, 35.83224293864768839 ) ) ;
#45918=CARTESIAN_POINT ( 'NONE',  ( -9.474510206698964154, 16.51473224551069663, 60.41557627198102409 ) ) ;
#45919=CARTESIAN_POINT ( 'NONE',  ( -16.46253265017160317, 9.564922557960807481, 105.8322429386476955 ) ) ;
#45920=CARTESIAN_POINT ( 'NONE',  ( -21.52544592524334988, -5.823673210054445271, 88.95942372801901854 ) ) ;
#45921=CARTESIAN_POINT ( 'NONE',  ( 9.564922557960805705, 16.46253265017160317, 64.58224293864769550 ) ) ;
#45922=CARTESIAN_POINT ( 'NONE',  ( -0.05219959533937732626, 21.53943276465977519, 77.50109039468567573 ) ) ;
#45923=CARTESIAN_POINT ( 'NONE',  ( 10.72451020669898902, -18.67979575497178502, 42.91557627198103120 ) ) ;
#45924=CARTESIAN_POINT ( 'NONE',  ( -18.62759615963255300, -10.81492255796106328, 29.16775706135234003 ) ) ;
#45925=CARTESIAN_POINT ( 'NONE',  ( -9.564922557961040184, 16.46253265017147172, 47.91775706135233293 ) ) ;
#45926=CARTESIAN_POINT ( 'NONE',  ( -13.97604488694527625, -13.89961937509977652, 31.87390960531435979 ) ) ;
#45927=CARTESIAN_POINT ( 'NONE',  ( -19.05341960407611168, -5.049401038298163336, 81.45724293864769550 ) ) ;
#45928=CARTESIAN_POINT ( 'NONE',  ( 16.55341960407618274, -4.379528057220086978, 31.04275706135234714 ) ) ;
#45929=CARTESIAN_POINT ( 'NONE',  ( 16.52544592524342804, -4.483927247898539470, 93.54057627198103830 ) ) ;
#45930=CARTESIAN_POINT ( 'NONE',  ( 19.03943276465977164, -0.05219959533909143690, 58.74890960531435979 ) ) ;
#45931=CARTESIAN_POINT ( 'NONE',  ( -10.81492255796078084, -18.62759615963271287, 32.08224293864769550 ) ) ;
#45932=CARTESIAN_POINT ( 'NONE',  ( 13.89961937509957401, 13.97604488694547697, 96.87609039468566152 ) ) ;
#45933=CARTESIAN_POINT ( 'NONE',  ( -21.52544592524343514, 5.823673210054127303, 106.0405762719810525 ) ) ;
#45934=CARTESIAN_POINT ( 'NONE',  ( 5.823673210054444382, -21.52544592524334988, 70.20942372801904696 ) ) ;
#45935=CARTESIAN_POINT ( 'NONE',  ( 8.224510206698742110, 14.34966873604972548, 67.08442372801901854 ) ) ;
#45936=CARTESIAN_POINT ( 'NONE',  ( 0.05219959533934541429, -16.53943276465976808, 65.00109039468568994 ) ) ;
#45937=CARTESIAN_POINT ( 'NONE',  ( 19.03943276465977164, -0.05219959533909143690, 58.74890960531435979 ) ) ;
#45938=CARTESIAN_POINT ( 'NONE',  ( -16.52544592524335698, -4.483927247898792601, 83.95942372801900433 ) ) ;
#45939=CARTESIAN_POINT ( 'NONE',  ( -19.02544592524334988, -5.153800228976617603, 48.95942372801900433 ) ) ;
#45940=CARTESIAN_POINT ( 'NONE',  ( -21.53943276465977519, -0.05219959533937600094, 23.75109039468567929 ) ) ;
#45941=CARTESIAN_POINT ( 'NONE',  ( 8.314922557960818139, 14.29746914071049879, 64.58224293864769550 ) ) ;
#45942=CARTESIAN_POINT ( 'NONE',  ( -19.03943276465977164, 0.05219959533909376836, 81.24890960531436690 ) ) ;
#45943=CARTESIAN_POINT ( 'NONE',  ( 16.53943276465976808, 0.05219959533934440121, 71.25109039468568994 ) ) ;
#45944=CARTESIAN_POINT ( 'NONE',  ( -21.53943276465977519, -0.05219959533937600094, 63.75109039468568284 ) ) ;
#45945=CARTESIAN_POINT ( 'NONE',  ( 8.224510206698742110, 14.34966873604972548, 22.08442372801901143 ) ) ;
#45946=CARTESIAN_POINT ( 'NONE',  ( -15.72974639402197994, 15.80617190586746368, 115.6239096053143669 ) ) ;
#45947=CARTESIAN_POINT ( 'NONE',  ( 16.52544592524342804, -4.483927247898539470, 58.54057627198103120 ) ) ;
#45948=VERTEX_POINT ( 'NONE', #30752 ) ;
#45949=CARTESIAN_POINT ( 'NONE',  ( 21.55341960407610458, 5.719274019375980345, 88.95724293864769550 ) ) ;
#45950=CARTESIAN_POINT ( 'NONE',  ( -16.52544592524342804, 4.483927247898546575, 41.04057627198103120 ) ) ;
#45953=CARTESIAN_POINT ( 'NONE',  ( -0.05219959533907301413, -21.53943276465977519, 112.4989096053143669 ) ) ;
#45954=CARTESIAN_POINT ( 'NONE',  ( -19.02544592524342804, 5.153800228976336051, 111.0405762719810099 ) ) ;
#45955=CARTESIAN_POINT ( 'NONE',  ( 15.72974639402176855, 15.80617190586768217, 36.87609039468568994 ) ) ;
#45956=CARTESIAN_POINT ( 'NONE',  ( -12.06949235617756955, 12.14591786802309770, 45.62390960531436690 ) ) ;
#45957=CARTESIAN_POINT ( 'NONE',  ( 9.474510206698971260, -16.51473224551069308, 62.91557627198102409 ) ) ;
#45958=CARTESIAN_POINT ( 'NONE',  ( -5.049401038297874678, -19.05341960407617918, 69.79275706135233293 ) ) ;
#45959=CARTESIAN_POINT ( 'NONE',  ( -13.89961937509977652, 13.97604488694528158, 95.62390960531436690 ) ) ;
#45960=EDGE_CURVE ( 'NONE', #132514, #55277, #124794, .T. ) ;
#45961=CARTESIAN_POINT ( 'NONE',  ( 21.55341960407610458, 5.719274019375980345, 48.95724293864770971 ) ) ;
#45963=CARTESIAN_POINT ( 'NONE',  ( 9.474510206698971260, -16.51473224551069308, 62.91557627198102409 ) ) ;
#45964=CARTESIAN_POINT ( 'NONE',  ( 14.34966873604972726, -8.224510206698740333, 35.83442372801901143 ) ) ;
#45965=CARTESIAN_POINT ( 'NONE',  ( -9.474510206698720793, -16.51473224551083518, 64.58442372801900433 ) ) ;
#45966=CARTESIAN_POINT ( 'NONE',  ( 15.80617190586746368, 15.72974639402197994, 109.3739096053143811 ) ) ;
#45967=CARTESIAN_POINT ( 'NONE',  ( -16.55341960407611168, -4.379528057220339221, 46.45724293864769550 ) ) ;
#45968=CARTESIAN_POINT ( 'NONE',  ( -13.89961937509977652, 13.97604488694528158, 95.62390960531436690 ) ) ;
#45969=CARTESIAN_POINT ( 'NONE',  ( 21.53943276465977519, -0.05219959533907433946, 78.74890960531436690 ) ) ;
#45970=CARTESIAN_POINT ( 'NONE',  ( 15.80617190586746368, 15.72974639402197994, 94.37390960531436690 ) ) ;
#45971=CARTESIAN_POINT ( 'NONE',  ( -4.379528057220086978, -16.55341960407618274, 39.79275706135235424 ) ) ;
#45972=CARTESIAN_POINT ( 'NONE',  ( 15.72974639402199770, -15.80617190586745480, 38.12390960531436690 ) ) ;
#45973=CARTESIAN_POINT ( 'NONE',  ( -15.72974639402176322, -15.80617190586768395, 94.37609039468568994 ) ) ;
#45974=CARTESIAN_POINT ( 'NONE',  ( -19.05341960407611168, -5.049401038298163336, 86.45724293864769550 ) ) ;
#45975=CARTESIAN_POINT ( 'NONE',  ( 0.05219959533909260263, 19.03943276465977164, 44.99890960531435979 ) ) ;
#45976=CARTESIAN_POINT ( 'NONE',  ( 13.89961937509977652, -13.97604488694527269, 93.12390960531436690 ) ) ;
#45977=CARTESIAN_POINT ( 'NONE',  ( -8.224510206698948167, 14.34966873604960824, 105.4155762719810383 ) ) ;
#45978=CARTESIAN_POINT ( 'NONE',  ( -16.46253265017160317, 9.564922557960807481, 70.83224293864770971 ) ) ;
#45979=CARTESIAN_POINT ( 'NONE',  ( -16.51473224551082808, 9.474510206698731452, 113.3344237280190043 ) ) ;
#45980=CARTESIAN_POINT ( 'NONE',  ( 18.22780087662126647, 5.499999999999818812, 41.48236817873107185 ) ) ;
#45981=CARTESIAN_POINT ( 'NONE',  ( -16.46253265017146816, -9.564922557961047289, 59.16775706135233293 ) ) ;
#45982=CARTESIAN_POINT ( 'NONE',  ( -0.05219959533937732626, 21.53943276465977519, 112.5010903946857042 ) ) ;
#45983=CARTESIAN_POINT ( 'NONE',  ( -18.62759615963270932, 10.81492255796079327, 35.83224293864768839 ) ) ;
#45984=CARTESIAN_POINT ( 'NONE',  ( 8.314922557961029526, -14.29746914071037800, 90.41775706135236135 ) ) ;
#45986=CARTESIAN_POINT ( 'NONE',  ( 13.89961937509957401, 13.97604488694547697, 71.87609039468567573 ) ) ;
#45987=CARTESIAN_POINT ( 'NONE',  ( 5.153800228976615827, -19.02544592524334988, 30.20942372801900433 ) ) ;
#45988=CARTESIAN_POINT ( 'NONE',  ( -17.26058549869089376, -6.457015423128631859, 46.37745837476068544 ) ) ;
#45989=CARTESIAN_POINT ( 'NONE',  ( 19.05341960407611168, 5.049401038298154454, 43.95724293864769550 ) ) ;
#45990=CARTESIAN_POINT ( 'NONE',  ( 14.34966873604960469, 8.224510206698951720, 34.16557627198102409 ) ) ;
#45991=CARTESIAN_POINT ( 'NONE',  ( -9.474510206698964154, 16.51473224551069663, 25.41557627198103120 ) ) ;
#45992=CARTESIAN_POINT ( 'NONE',  ( 4.379528057220339221, -16.55341960407611168, 27.70724293864769905 ) ) ;
#45993=LINE ( 'NONE', #118882, #119466 ) ;
#45994=CARTESIAN_POINT ( 'NONE',  ( 8.314922557961029526, -14.29746914071037800, 95.41775706135234714 ) ) ;
#45995=CARTESIAN_POINT ( 'NONE',  ( 19.02544592524343514, -5.153800228976328945, 38.54057627198103120 ) ) ;
#45996=CARTESIAN_POINT ( 'NONE',  ( -21.53943276465977519, -0.05219959533937600094, 103.7510903946857042 ) ) ;
#45997=CARTESIAN_POINT ( 'NONE',  ( 8.224510206698742110, 14.34966873604972548, 22.08442372801901143 ) ) ;
#45998=CARTESIAN_POINT ( 'NONE',  ( -10.81492255796105439, 18.62759615963255655, 72.91775706135234714 ) ) ;
#45999=CARTESIAN_POINT ( 'NONE',  ( 9.474510206698729675, 16.51473224551082808, 52.08442372801900433 ) ) ;
#46000=CARTESIAN_POINT ( 'NONE',  ( -0.05219959533909027116, -19.03943276465977164, 92.49890960531436690 ) ) ;
#46001=CARTESIAN_POINT ( 'NONE',  ( 16.46253265017160672, -9.564922557960803928, 88.33224293864769550 ) ) ;
#46002=CARTESIAN_POINT ( 'NONE',  ( -18.39443945427638738, 5.500000000000030198, 38.51745347608652281 ) ) ;
#46003=CARTESIAN_POINT ( 'NONE',  ( 10.81492255796078972, 18.62759615963270932, 104.5822429386477097 ) ) ;
#46004=CARTESIAN_POINT ( 'NONE',  ( -8.224510206698948167, 14.34966873604960824, 65.41557627198102409 ) ) ;
#46005=CARTESIAN_POINT ( 'NONE',  ( 10.81492255796078972, 18.62759615963270932, 59.58224293864770260 ) ) ;
#46006=CARTESIAN_POINT ( 'NONE',  ( -0.05219959533909027116, -19.03943276465977164, 57.49890960531435979 ) ) ;
#46007=CARTESIAN_POINT ( 'NONE',  ( -15.72974639402197994, 15.80617190586746368, 95.62390960531436690 ) ) ;
#46008=CARTESIAN_POINT ( 'NONE',  ( -14.34966873604972548, 8.224510206698743886, 93.33442372801901854 ) ) ;
#46009=ORIENTED_EDGE ( 'NONE', *, *, #31131, .T. ) ;
#46010=CARTESIAN_POINT ( 'NONE',  ( -5.153800228976328057, -19.02544592524343514, 42.29057627198101699 ) ) ;
#46011=CARTESIAN_POINT ( 'NONE',  ( 14.29746914071049879, -8.314922557960816363, 93.33224293864769550 ) ) ;
#46013=CARTESIAN_POINT ( 'NONE',  ( 13.89961937509977652, -13.97604488694527269, 53.12390960531434558 ) ) ;
#46014=CARTESIAN_POINT ( 'NONE',  ( 19.05341960407617918, -5.049401038297876454, 86.04275706135233293 ) ) ;
#46015=CARTESIAN_POINT ( 'NONE',  ( 8.314922557960818139, 14.29746914071049879, 89.58224293864768129 ) ) ;
#46016=CARTESIAN_POINT ( 'NONE',  ( -10.72451020669870658, -18.67979575497194134, 49.58442372801901143 ) ) ;
#46017=CARTESIAN_POINT ( 'NONE',  ( 19.05341960407611168, 5.049401038298154454, 33.95724293864769550 ) ) ;
#46018=CARTESIAN_POINT ( 'NONE',  ( 5.719274019375991003, -21.55341960407610458, 97.70724293864772392 ) ) ;
#46019=CARTESIAN_POINT ( 'NONE',  ( 8.314922557960818139, 14.29746914071049879, 94.58224293864769550 ) ) ;
#46021=CARTESIAN_POINT ( 'NONE',  ( -0.05219959533909027116, -19.03943276465977164, 62.49890960531435979 ) ) ;
#46022=CARTESIAN_POINT ( 'NONE',  ( 17.48853670773245028, 5.747243402303095827, 113.8332870025000716 ) ) ;
#46023=CARTESIAN_POINT ( 'NONE',  ( -5.153800228976607833, 19.02544592524334988, 97.70942372801900433 ) ) ;
#46024=CARTESIAN_POINT ( 'NONE',  ( 9.564922557960805705, 16.46253265017160317, 109.5822429386476955 ) ) ;
#46025=CARTESIAN_POINT ( 'NONE',  ( -0.05219959533937732626, 21.53943276465977519, 42.50109039468567573 ) ) ;
#46026=CARTESIAN_POINT ( 'NONE',  ( 13.97604488694527802, 13.89961937509977652, 79.37390960531435269 ) ) ;
#46027=CARTESIAN_POINT ( 'NONE',  ( -16.46253265017146816, -9.564922557961047289, 64.16775706135233293 ) ) ;
#46028=CARTESIAN_POINT ( 'NONE',  ( -19.02544592524342804, 5.153800228976336051, 61.04057627198103120 ) ) ;
#46029=B_SPLINE_CURVE_WITH_KNOTS ( 'NONE', 3,
 ( #92990, #154676, #16171, #126319, #976, #184030, #171839, #2978, #124329, #33326, #64657, #188016, #109165, #170845, #155669, #107167, #17165, #78818, #156672, #91984, #1985, #94987, #173839, #112147, #35305, #175819, #161641, #143462, #130280, #66631, #174820, #23135 ),
 .UNSPECIFIED., .F., .F.,
 ( 4, 2, 2, 2, 2, 2, 2, 2, 2, 2, 2, 2, 2, 2, 2, 4 ),
 ( 7.806255641895631925E-18, 0.0003712461730036880790, 0.0007424923460073683517, 0.001113738519011048516, 0.001484984692014728897, 0.002227477038022087057, 0.002598723211025766571, 0.002969969384029446085, 0.003341215557033124731, 0.003712461730036803811, 0.004083707903040482458, 0.004454954076044161104, 0.004826200249047840618, 0.005197446422051519264, 0.005568692595055198778, 0.005939938768058877425 ),
 .UNSPECIFIED. ) ;
#46030=CARTESIAN_POINT ( 'NONE',  ( 0.05219959533910956823, 16.53943276465976808, 74.99890960531435269 ) ) ;
#46031=CARTESIAN_POINT ( 'NONE',  ( -14.34966873604960291, -8.224510206698953496, 61.66557627198103120 ) ) ;
#46032=CARTESIAN_POINT ( 'NONE',  ( 0.05219959533909260263, 19.03943276465977164, 84.99890960531436690 ) ) ;
#46033=CARTESIAN_POINT ( 'NONE',  ( -10.81492255796078084, -18.62759615963271287, 97.08224293864770971 ) ) ;
#46034=CARTESIAN_POINT ( 'NONE',  ( -13.89961937509977652, 13.97604488694528158, 85.62390960531433848 ) ) ;
#46035=CARTESIAN_POINT ( 'NONE',  ( -19.02544592524334988, -5.153800228976617603, 28.95942372801900433 ) ) ;
#46036=CARTESIAN_POINT ( 'NONE',  ( -19.02544592524342804, 5.153800228976336051, 41.04057627198103120 ) ) ;
#46037=CARTESIAN_POINT ( 'NONE',  ( 12.14591786802309770, 12.06949235617756955, 34.37390960531435979 ) ) ;
#46038=CARTESIAN_POINT ( 'NONE',  ( -12.06949235617756955, 12.14591786802309770, 110.6239096053143669 ) ) ;
#46040=CARTESIAN_POINT ( 'NONE',  ( 10.81492255796106328, -18.62759615963255655, 35.41775706135234003 ) ) ;
#46041=CARTESIAN_POINT ( 'NONE',  ( -19.02544592524334988, -5.153800228976617603, 63.95942372801899012 ) ) ;
#46042=CARTESIAN_POINT ( 'NONE',  ( -12.14591786802309592, -12.06949235617757132, 31.87390960531435979 ) ) ;
#46043=CARTESIAN_POINT ( 'NONE',  ( -21.55341960407610458, -5.719274019375992779, 91.45724293864769550 ) ) ;
#46044=CARTESIAN_POINT ( 'NONE',  ( 15.80617190586746368, 15.72974639402197994, 24.37390960531435979 ) ) ;
#46045=CARTESIAN_POINT ( 'NONE',  ( 4.379528057220339221, -16.55341960407611168, 67.70724293864769550 ) ) ;
#46046=CARTESIAN_POINT ( 'NONE',  ( 19.03943276465977164, -0.05219959533909143690, 33.74890960531435979 ) ) ;
#46047=CARTESIAN_POINT ( 'NONE',  ( 9.474510206698729675, 16.51473224551082808, 32.08442372801900433 ) ) ;
#46048=CARTESIAN_POINT ( 'NONE',  ( -16.52544592524335698, -4.483927247898792601, 108.9594237280190185 ) ) ;
#46049=CARTESIAN_POINT ( 'NONE',  ( 4.483927247898790824, -16.52544592524335698, 55.20942372801902565 ) ) ;
#46050=CARTESIAN_POINT ( 'NONE',  ( 10.72451020669898902, -18.67979575497178502, 42.91557627198103120 ) ) ;
#46051=CARTESIAN_POINT ( 'NONE',  ( -5.823673210054431948, 21.52544592524334988, 112.7094237280190328 ) ) ;
#46052=CARTESIAN_POINT ( 'NONE',  ( 5.049401038298161559, -19.05341960407611168, 82.70724293864770971 ) ) ;
#46053=CARTESIAN_POINT ( 'NONE',  ( 12.14591786802327356, -12.06949235617739191, 55.62609039468568284 ) ) ;
#46054=CARTESIAN_POINT ( 'NONE',  ( 0.05219959533909260263, 19.03943276465977164, 29.99890960531435979 ) ) ;
#46055=CARTESIAN_POINT ( 'NONE',  ( 12.14591786802309770, 12.06949235617756955, 34.37390960531435979 ) ) ;
#46056=CARTESIAN_POINT ( 'NONE',  ( 19.05341960407611168, 5.049401038298154454, 108.9572429386477097 ) ) ;
#46057=CARTESIAN_POINT ( 'NONE',  ( 9.474510206698971260, -16.51473224551069308, 87.91557627198102409 ) ) ;
#46058=CARTESIAN_POINT ( 'NONE',  ( 5.049401038298161559, -19.05341960407611168, 102.7072429386476955 ) ) ;
#46059=CARTESIAN_POINT ( 'NONE',  ( 12.06949235617757843, -12.14591786802309237, 53.12390960531436690 ) ) ;
#46061=CARTESIAN_POINT ( 'NONE',  ( 8.224510206698953496, -14.34966873604960469, 27.91557627198103830 ) ) ;
#46063=CARTESIAN_POINT ( 'NONE',  ( 16.55341960407611168, 4.379528057220329451, 48.95724293864770971 ) ) ;
#46064=CARTESIAN_POINT ( 'NONE',  ( 16.52544592524335698, 4.483927247898782831, 41.45942372801901143 ) ) ;
#46065=PLANE ( 'NONE',  #70588 ) ;
#46066=CARTESIAN_POINT ( 'NONE',  ( 9.474510206698729675, 16.51473224551082808, 47.08442372801900433 ) ) ;
#46067=CARTESIAN_POINT ( 'NONE',  ( -5.049401038298153566, 19.05341960407611168, 85.20724293864766707 ) ) ;
#46068=CARTESIAN_POINT ( 'NONE',  ( 19.02544592524334988, 5.153800228976608722, 71.45942372801900433 ) ) ;
#46070=CARTESIAN_POINT ( 'NONE',  ( -5.153800228976607833, 19.02544592524334988, 52.70942372801900433 ) ) ;
#46071=CARTESIAN_POINT ( 'NONE',  ( 19.02544592524334988, 5.153800228976608722, 96.45942372801897591 ) ) ;
#46072=CARTESIAN_POINT ( 'NONE',  ( -16.53943276465976808, -0.05219959533934237506, 83.75109039468568994 ) ) ;
#46074=CARTESIAN_POINT ( 'NONE',  ( -19.05341960407611168, -5.049401038298163336, 21.45724293864768839 ) ) ;
#46075=CARTESIAN_POINT ( 'NONE',  ( -16.46253265017160317, 9.564922557960807481, 110.8322429386476955 ) ) ;
#46076=CARTESIAN_POINT ( 'NONE',  ( -10.81492255796105439, 18.62759615963255655, 42.91775706135235424 ) ) ;
#46077=CARTESIAN_POINT ( 'NONE',  ( -16.46253265017146816, -9.564922557961047289, 104.1677570613523329 ) ) ;
#46078=CARTESIAN_POINT ( 'NONE',  ( 17.49999999999999645, -5.076555817581239083, 106.3204850795022764 ) ) ;
#46079=CARTESIAN_POINT ( 'NONE',  ( -19.05341960407611168, -5.049401038298163336, 61.45724293864769550 ) ) ;
#46080=CARTESIAN_POINT ( 'NONE',  ( -0.05219959533909027116, -19.03943276465977164, 97.49890960531436690 ) ) ;
#46081=CARTESIAN_POINT ( 'NONE',  ( -16.53943276465976808, 0.05219959533911058130, 66.24890960531436690 ) ) ;
#46082=CARTESIAN_POINT ( 'NONE',  ( -19.02544592524342804, 5.153800228976336051, 61.04057627198103120 ) ) ;
#46083=CARTESIAN_POINT ( 'NONE',  ( -9.474510206698964154, 16.51473224551069663, 80.41557627198103830 ) ) ;
#46084=CARTESIAN_POINT ( 'NONE',  ( 16.51473224551083163, -9.474510206698727899, 75.83442372801900433 ) ) ;
#46085=CARTESIAN_POINT ( 'NONE',  ( 10.72451020669898902, -18.67979575497178502, 52.91557627198103830 ) ) ;
#46086=CARTESIAN_POINT ( 'NONE',  ( -8.224510206698948167, 14.34966873604960824, 115.4155762719810241 ) ) ;
#46087=CARTESIAN_POINT ( 'NONE',  ( 19.02544592524334988, 5.153800228976608722, 41.45942372801900433 ) ) ;
#46088=CARTESIAN_POINT ( 'NONE',  ( -0.05219959533909027116, -19.03943276465977164, 82.49890960531436690 ) ) ;
#46089=CARTESIAN_POINT ( 'NONE',  ( 21.52544592524344225, -5.823673210054117533, 78.54057627198103830 ) ) ;
#46090=CARTESIAN_POINT ( 'NONE',  ( -14.34966873604960291, -8.224510206698953496, 81.66557627198103830 ) ) ;
#46091=CARTESIAN_POINT ( 'NONE',  ( -16.46253265017146816, -9.564922557961047289, 29.16775706135232937 ) ) ;
#46092=CARTESIAN_POINT ( 'NONE',  ( 18.62759615963271287, -10.81492255796078972, 58.33224293864768839 ) ) ;
#46093=CARTESIAN_POINT ( 'NONE',  ( -21.55341960407610458, -5.719274019375992779, 36.45724293864768839 ) ) ;
#46094=CARTESIAN_POINT ( 'NONE',  ( 5.719274019375673035, 21.55341960407619339, 97.29275706135234714 ) ) ;
#46095=CARTESIAN_POINT ( 'NONE',  ( -5.153800228976328057, -19.02544592524343514, 62.29057627198100988 ) ) ;
#46096=CARTESIAN_POINT ( 'NONE',  ( 0.05219959533910956823, 16.53943276465976808, 109.9989096053143527 ) ) ;
#46097=CARTESIAN_POINT ( 'NONE',  ( -21.55341960407619339, 5.719274019375674811, 28.54275706135234358 ) ) ;
#46098=CARTESIAN_POINT ( 'NONE',  ( -19.20446147854528718, -5.499999999999909406, 39.38999695167677118 ) ) ;
#46099=CARTESIAN_POINT ( 'NONE',  ( -15.72974639402176322, -15.80617190586768395, 39.37609039468567573 ) ) ;
#46100=CARTESIAN_POINT ( 'NONE',  ( 19.03943276465977164, -0.05219959533909143690, 38.74890960531436690 ) ) ;
#46101=CARTESIAN_POINT ( 'NONE',  ( 15.72974639402199770, -15.80617190586745480, 108.1239096053143811 ) ) ;
#46102=CARTESIAN_POINT ( 'NONE',  ( 16.51473224551083163, -9.474510206698727899, 50.83442372801899722 ) ) ;
#46103=CARTESIAN_POINT ( 'NONE',  ( -19.03943276465977164, 0.05219959533909376836, 21.24890960531436335 ) ) ;
#46104=CARTESIAN_POINT ( 'NONE',  ( 9.474510206698971260, -16.51473224551069308, 22.91557627198102765 ) ) ;
#46105=CYLINDRICAL_SURFACE ( 'NONE', #62730, 2.500000000000002220 ) ;
#46106=CARTESIAN_POINT ( 'NONE',  ( -8.314922557961024197, 14.29746914071037800, 57.91775706135234714 ) ) ;
#46107=CARTESIAN_POINT ( 'NONE',  ( 19.03943276465977164, -0.05219959533909143690, 28.74890960531435624 ) ) ;
#46109=CARTESIAN_POINT ( 'NONE',  ( 0.05219959533909260263, 19.03943276465977164, 69.99890960531435269 ) ) ;
#46110=CARTESIAN_POINT ( 'NONE',  ( -16.52544592524342804, 4.483927247898546575, 101.0405762719810383 ) ) ;
#46112=CARTESIAN_POINT ( 'NONE',  ( -10.72451020669898014, 18.67979575497178502, 55.41557627198102409 ) ) ;
#46113=CARTESIAN_POINT ( 'NONE',  ( 12.06949235617739724, 12.14591786802326823, 41.87609039468568284 ) ) ;
#46114=CARTESIAN_POINT ( 'NONE',  ( 21.55341960407619695, -5.719274019375665929, 106.0427570613523471 ) ) ;
#46115=CARTESIAN_POINT ( 'NONE',  ( 19.03943276465977164, -0.05219959533909143690, 23.74890960531435269 ) ) ;
#46116=CARTESIAN_POINT ( 'NONE',  ( 12.14591786802309770, 12.06949235617756955, 24.37390960531435979 ) ) ;
#46117=CARTESIAN_POINT ( 'NONE',  ( -4.379528057220328563, 16.55341960407611168, 50.20724293864769550 ) ) ;
#46118=CARTESIAN_POINT ( 'NONE',  ( -9.564922557960796823, -16.46253265017161027, 47.08224293864769550 ) ) ;
#46119=CARTESIAN_POINT ( 'NONE',  ( 0.05219959533937995610, -21.53943276465977519, 90.00109039468567573 ) ) ;
#46120=CARTESIAN_POINT ( 'NONE',  ( 18.67979575497178502, 10.72451020669898547, 109.1655762719810383 ) ) ;
#46121=CARTESIAN_POINT ( 'NONE',  ( 5.719274019375673035, 21.55341960407619339, 72.29275706135236135 ) ) ;
#46122=CARTESIAN_POINT ( 'NONE',  ( 16.55341960407618274, -4.379528057220086978, 56.04275706135235424 ) ) ;
#46123=CARTESIAN_POINT ( 'NONE',  ( 4.379528057220339221, -16.55341960407611168, 77.70724293864770971 ) ) ;
#46124=CARTESIAN_POINT ( 'NONE',  ( -15.80617190586768217, 15.72974639402176855, 103.1260903946856757 ) ) ;
#46125=CARTESIAN_POINT ( 'NONE',  ( -16.55341960407611168, -4.379528057220339221, 21.45724293864769550 ) ) ;
#46126=CARTESIAN_POINT ( 'NONE',  ( -16.19135201231366850, 7.376712067591915556, 114.8131914594797394 ) ) ;
#46127=CARTESIAN_POINT ( 'NONE',  ( -16.52544592524335698, -4.483927247898792601, 33.95942372801901143 ) ) ;
#46128=CARTESIAN_POINT ( 'NONE',  ( -4.379528057220328563, 16.55341960407611168, 40.20724293864769550 ) ) ;
#46129=B_SPLINE_CURVE_WITH_KNOTS ( 'NONE', 3,
 ( #20044, #175725, #37204, #98860, #156582, #143369, #63572, #157574, #18077, #79732, #141401, #187928, #111060, #19067, #142392, #3871, #65550, #23046, #176740, #85705, #160555, #164562, #41216, #101878, #56373, #22045, #9882, #148388, #145374, #40198, #178735, #7858 ),
 .UNSPECIFIED., .F., .F.,
 ( 4, 2, 2, 2, 2, 2, 2, 2, 2, 2, 2, 2, 2, 2, 2, 4 ),
 ( 2.883244014823444873E-17, 0.0003712461730037120398, 0.0007424923460073952399, 0.001113738519011078440, 0.001484984692014761640, 0.002227477038022125221, 0.002598723211025809939, 0.002969969384029495525, 0.003341215557033180676, 0.003712461730036866261, 0.004083707903040550979, 0.004454954076044235697, 0.004826200249047921283, 0.005197446422051606868, 0.005568692595055292453, 0.005939938768058977171 ),
 .UNSPECIFIED. ) ;
#46130=CARTESIAN_POINT ( 'NONE',  ( -16.55341960407617563, 4.379528057220093196, 83.54275706135234714 ) ) ;
#46131=CARTESIAN_POINT ( 'NONE',  ( -13.89961937509977652, 13.97604488694528158, 105.6239096053143527 ) ) ;
#46132=CARTESIAN_POINT ( 'NONE',  ( -9.474510206698964154, 16.51473224551069663, 110.4155762719810383 ) ) ;
#46133=CARTESIAN_POINT ( 'NONE',  ( -21.52544592524334988, -5.823673210054445271, 93.95942372801903275 ) ) ;
#46134=CARTESIAN_POINT ( 'NONE',  ( 16.55341960407618274, -4.379528057220086978, 106.0427570613523471 ) ) ;
#46135=CARTESIAN_POINT ( 'NONE',  ( 16.53943276465976808, -0.05219959533910856209, 68.74890960531435269 ) ) ;
#46136=CARTESIAN_POINT ( 'NONE',  ( 9.564922557960805705, 16.46253265017160317, 79.58224293864769550 ) ) ;
#46138=CARTESIAN_POINT ( 'NONE',  ( 16.53943276465976808, 0.05219959533934440121, 46.25109039468567573 ) ) ;
#46139=CARTESIAN_POINT ( 'NONE',  ( -9.564922557960796823, -16.46253265017161027, 37.08224293864768839 ) ) ;
#46140=CARTESIAN_POINT ( 'NONE',  ( 9.474510206698971260, -16.51473224551069308, 92.91557627198103830 ) ) ;
#46141=CARTESIAN_POINT ( 'NONE',  ( -14.34966873604972548, 8.224510206698743886, 38.33442372801900433 ) ) ;
#46143=CARTESIAN_POINT ( 'NONE',  ( 13.89961937509957401, 13.97604488694547697, 31.87609039468566863 ) ) ;
#46144=CARTESIAN_POINT ( 'NONE',  ( 16.52544592524335698, 4.483927247898782831, 96.45942372801901854 ) ) ;
#46145=CARTESIAN_POINT ( 'NONE',  ( -9.564922557960796823, -16.46253265017161027, 37.08224293864768839 ) ) ;
#46146=CARTESIAN_POINT ( 'NONE',  ( -16.53943276465976808, -0.05219959533934237506, 78.75109039468568994 ) ) ;
#46147=CARTESIAN_POINT ( 'NONE',  ( 8.314922557961029526, -14.29746914071037800, 70.41775706135236135 ) ) ;
#46148=CARTESIAN_POINT ( 'NONE',  ( -13.89961937509957401, -13.97604488694547875, 84.37609039468567573 ) ) ;
#46149=CARTESIAN_POINT ( 'NONE',  ( 19.05341960407617918, -5.049401038297876454, 26.04275706135233293 ) ) ;
#46150=CARTESIAN_POINT ( 'NONE',  ( -9.564922557960796823, -16.46253265017161027, 52.08224293864768839 ) ) ;
#46151=CARTESIAN_POINT ( 'NONE',  ( -8.314922557960811034, -14.29746914071050412, 87.08224293864769550 ) ) ;
#46153=CARTESIAN_POINT ( 'NONE',  ( -13.89961937509957401, -13.97604488694547875, 54.37609039468565442 ) ) ;
#46154=CARTESIAN_POINT ( 'NONE',  ( 21.52544592524344225, -5.823673210054117533, 53.54057627198103120 ) ) ;
#46155=CARTESIAN_POINT ( 'NONE',  ( -19.03943276465977164, -0.05219959533935918106, 33.75109039468566863 ) ) ;
#46156=CARTESIAN_POINT ( 'NONE',  ( -19.05341960407611168, -5.049401038298163336, 101.4572429386476955 ) ) ;
#46157=CARTESIAN_POINT ( 'NONE',  ( -15.72974639402197994, 15.80617190586746368, 80.62390960531438111 ) ) ;
#46158=CARTESIAN_POINT ( 'NONE',  ( 9.474510206698971260, -16.51473224551069308, 112.9155762719810383 ) ) ;
#46159=CARTESIAN_POINT ( 'NONE',  ( -5.153800228976607833, 19.02544592524334988, 102.7094237280189759 ) ) ;
#46160=CARTESIAN_POINT ( 'NONE',  ( 9.474510206698971260, -16.51473224551069308, 112.9155762719810383 ) ) ;
#46161=CARTESIAN_POINT ( 'NONE',  ( 9.474510206698729675, 16.51473224551082808, 107.0844237280190043 ) ) ;
#46162=CARTESIAN_POINT ( 'NONE',  ( -16.46253265017160317, 9.564922557960807481, 35.83224293864768839 ) ) ;
#46163=CARTESIAN_POINT ( 'NONE',  ( -19.02544592524342804, 5.153800228976336051, 101.0405762719810241 ) ) ;
#46164=CARTESIAN_POINT ( 'NONE',  ( 21.55341960407610458, 5.719274019375980345, 73.95724293864769550 ) ) ;
#46165=CARTESIAN_POINT ( 'NONE',  ( -8.224510206698735004, -14.34966873604973081, 49.58442372801901143 ) ) ;
#46166=CARTESIAN_POINT ( 'NONE',  ( -21.53943276465977519, -0.05219959533937600094, 63.75109039468568284 ) ) ;
#46167=CARTESIAN_POINT ( 'NONE',  ( 19.02544592524334988, 5.153800228976608722, 101.4594237280189759 ) ) ;
#46168=CARTESIAN_POINT ( 'NONE',  ( 18.62759615963255655, 10.81492255796105972, 111.6677570613523613 ) ) ;
#46169=CARTESIAN_POINT ( 'NONE',  ( 12.14591786802327356, -12.06949235617739191, 105.6260903946856899 ) ) ;
#46171=CARTESIAN_POINT ( 'NONE',  ( 21.52544592524344225, -5.823673210054117533, 98.54057627198105251 ) ) ;
#46172=CARTESIAN_POINT ( 'NONE',  ( 12.14591786802309770, 12.06949235617756955, 39.37390960531436690 ) ) ;
#46173=CARTESIAN_POINT ( 'NONE',  ( 13.89961937509957401, 13.97604488694547697, 86.87609039468567573 ) ) ;
#46174=CARTESIAN_POINT ( 'NONE',  ( 18.62759615963255655, 10.81492255796105972, 56.66775706135235424 ) ) ;
#46175=CARTESIAN_POINT ( 'NONE',  ( -16.46253265017146816, -9.564922557961047289, 44.16775706135232582 ) ) ;
#46176=CARTESIAN_POINT ( 'NONE',  ( -4.379528057220328563, 16.55341960407611168, 100.2072429386476955 ) ) ;
#46177=CARTESIAN_POINT ( 'NONE',  ( 21.55341960407610458, 5.719274019375980345, 28.95724293864769905 ) ) ;
#46178=CARTESIAN_POINT ( 'NONE',  ( 4.379528057220339221, -16.55341960407611168, 32.70724293864770260 ) ) ;
#46179=CARTESIAN_POINT ( 'NONE',  ( -10.72451020669870658, -18.67979575497194134, 104.5844237280190185 ) ) ;
#46180=CARTESIAN_POINT ( 'NONE',  ( 14.29746914071037800, 8.314922557961029526, 56.66775706135235424 ) ) ;
#46181=CARTESIAN_POINT ( 'NONE',  ( -16.55341960407617563, 4.379528057220093196, 113.5427570613523756 ) ) ;
#46182=CARTESIAN_POINT ( 'NONE',  ( 18.67979575497194134, -10.72451020669871369, 60.83442372801901854 ) ) ;
#46183=CARTESIAN_POINT ( 'NONE',  ( -18.62759615963255300, -10.81492255796106328, 59.16775706135234714 ) ) ;
#46185=CARTESIAN_POINT ( 'NONE',  ( -13.89961937509977652, 13.97604488694528158, 30.62390960531435269 ) ) ;
#46186=CARTESIAN_POINT ( 'NONE',  ( 10.81492255796106328, -18.62759615963255655, 25.41775706135235779 ) ) ;
#46187=CARTESIAN_POINT ( 'NONE',  ( -12.06949235617756955, 12.14591786802309770, 105.6239096053143669 ) ) ;
#46188=CARTESIAN_POINT ( 'NONE',  ( 20.02699684519809509, -3.713461942911806979, 37.50000000000000000 ) ) ;
#46189=CARTESIAN_POINT ( 'NONE',  ( -4.483927247898539470, -16.52544592524342804, 77.29057627198102409 ) ) ;
#46190=CARTESIAN_POINT ( 'NONE',  ( -13.89961937509977652, 13.97604488694528158, 70.62390960531432427 ) ) ;
#46191=CARTESIAN_POINT ( 'NONE',  ( 12.14591786802309770, 12.06949235617756955, 24.37390960531435979 ) ) ;
#46192=CARTESIAN_POINT ( 'NONE',  ( 5.719274019375991003, -21.55341960407610458, 57.70724293864770260 ) ) ;
#46193=CARTESIAN_POINT ( 'NONE',  ( 16.55341960407611168, 4.379528057220329451, 88.95724293864769550 ) ) ;
#46194=CARTESIAN_POINT ( 'NONE',  ( -15.80617190586745835, -15.72974639402198527, 101.8739096053143811 ) ) ;
#46195=CARTESIAN_POINT ( 'NONE',  ( -13.97604488694527625, -13.89961937509977652, 96.87390960531433848 ) ) ;
#46196=CARTESIAN_POINT ( 'NONE',  ( 9.564922557960805705, 16.46253265017160317, 49.58224293864770260 ) ) ;
#46197=CARTESIAN_POINT ( 'NONE',  ( 19.03943276465977164, 0.05219959533936151252, 111.2510903946856757 ) ) ;
#46198=CARTESIAN_POINT ( 'NONE',  ( -21.53943276465977519, 0.05219959533907696930, 61.24890960531435979 ) ) ;
#46199=CARTESIAN_POINT ( 'NONE',  ( 18.62759615963255655, 10.81492255796105972, 81.66775706135236135 ) ) ;
#46200=CARTESIAN_POINT ( 'NONE',  ( -5.153800228976328057, -19.02544592524343514, 72.29057627198102409 ) ) ;
#46201=CARTESIAN_POINT ( 'NONE',  ( 9.564922557960805705, 16.46253265017160317, 99.58224293864770971 ) ) ;
#46202=CARTESIAN_POINT ( 'NONE',  ( 12.14591786802327356, -12.06949235617739191, 80.62609039468567573 ) ) ;
#46203=CARTESIAN_POINT ( 'NONE',  ( -18.62759615963255300, -10.81492255796106328, 54.16775706135235424 ) ) ;
#46204=CARTESIAN_POINT ( 'NONE',  ( -0.05219959533937732626, 21.53943276465977519, 87.50109039468568994 ) ) ;
#46205=CARTESIAN_POINT ( 'NONE',  ( -10.72451020669898014, 18.67979575497178502, 115.4155762719810241 ) ) ;
#46206=CARTESIAN_POINT ( 'NONE',  ( 14.29746914071037800, 8.314922557961029526, 81.66775706135236135 ) ) ;
#46207=CARTESIAN_POINT ( 'NONE',  ( 10.72451020669898902, -18.67979575497178502, 77.91557627198102409 ) ) ;
#46208=CARTESIAN_POINT ( 'NONE',  ( 16.51473224551083163, -9.474510206698727899, 40.83442372801900433 ) ) ;
#46209=CARTESIAN_POINT ( 'NONE',  ( -21.55341960407610458, -5.719274019375992779, 36.45724293864768839 ) ) ;
#46210=CARTESIAN_POINT ( 'NONE',  ( 0.05219959533909260263, 19.03943276465977164, 84.99890960531436690 ) ) ;
#46211=CARTESIAN_POINT ( 'NONE',  ( -14.34966873604960291, -8.224510206698953496, 21.66557627198102409 ) ) ;
#46213=CARTESIAN_POINT ( 'NONE',  ( -13.97604488694527625, -13.89961937509977652, 111.8739096053143243 ) ) ;
#46216=CARTESIAN_POINT ( 'NONE',  ( -5.049401038297874678, -19.05341960407617918, 99.79275706135234714 ) ) ;
#46217=CARTESIAN_POINT ( 'NONE',  ( 5.823673210054125526, 21.52544592524343514, 69.79057627198102409 ) ) ;
#46218=CARTESIAN_POINT ( 'NONE',  ( -0.05219959533910754901, -16.53943276465976808, 47.49890960531435979 ) ) ;
#46219=CARTESIAN_POINT ( 'NONE',  ( 9.564922557961047289, -16.46253265017146816, 110.4177570613523471 ) ) ;
#46220=CARTESIAN_POINT ( 'NONE',  ( 9.564922557960805705, 16.46253265017160317, 29.58224293864769550 ) ) ;
#46221=CARTESIAN_POINT ( 'NONE',  ( 0.05219959533936267826, -19.03943276465977164, 110.0010903946856757 ) ) ;
#46222=CARTESIAN_POINT ( 'NONE',  ( 15.80617190586746368, 15.72974639402197994, 94.37390960531436690 ) ) ;
#46223=CARTESIAN_POINT ( 'NONE',  ( 13.97604488694548053, -13.89961937509957401, 75.62609039468564731 ) ) ;
#46224=CARTESIAN_POINT ( 'NONE',  ( 4.379528057220092307, 16.55341960407617563, 82.29275706135234714 ) ) ;
#46225=CARTESIAN_POINT ( 'NONE',  ( -19.02544592524342804, 5.153800228976336051, 81.04057627198103830 ) ) ;
#46226=CARTESIAN_POINT ( 'NONE',  ( 8.224510206698953496, -14.34966873604960469, 82.91557627198103830 ) ) ;
#46227=CARTESIAN_POINT ( 'NONE',  ( -16.51473224551069308, -9.474510206698971260, 56.66557627198103120 ) ) ;
#46228=CARTESIAN_POINT ( 'NONE',  ( -16.53943276465976808, 0.05219959533911058130, 66.24890960531436690 ) ) ;
#46229=CARTESIAN_POINT ( 'NONE',  ( -9.564922557960796823, -16.46253265017161027, 27.08224293864769550 ) ) ;
#46231=CARTESIAN_POINT ( 'NONE',  ( -4.483927247898539470, -16.52544592524342804, 42.29057627198103120 ) ) ;
#46232=CARTESIAN_POINT ( 'NONE',  ( 9.564922557960805705, 16.46253265017160317, 79.58224293864769550 ) ) ;
#46234=CARTESIAN_POINT ( 'NONE',  ( 19.03943276465977164, 0.05219959533936151252, 56.25109039468566863 ) ) ;
#46235=CARTESIAN_POINT ( 'NONE',  ( -14.34966873604972548, 8.224510206698743886, 63.33442372801900433 ) ) ;
#46236=CARTESIAN_POINT ( 'NONE',  ( -21.52544592524343514, 5.823673210054127303, 66.04057627198103830 ) ) ;
#46237=CARTESIAN_POINT ( 'NONE',  ( 19.03943276465977164, 0.05219959533936151252, 26.25109039468566507 ) ) ;
#46238=CARTESIAN_POINT ( 'NONE',  ( 19.02544592524343514, -5.153800228976328945, 88.54057627198102409 ) ) ;
#46240=CARTESIAN_POINT ( 'NONE',  ( 15.80617190586746368, 15.72974639402197994, 24.37390960531435979 ) ) ;
#46241=CARTESIAN_POINT ( 'NONE',  ( 16.51473224551069308, 9.474510206698969483, 59.16557627198102409 ) ) ;
#46242=CARTESIAN_POINT ( 'NONE',  ( 21.55341960407619695, -5.719274019375665929, 56.04275706135235424 ) ) ;
#46243=CARTESIAN_POINT ( 'NONE',  ( -8.314922557960811034, -14.29746914071050412, 112.0822429386477097 ) ) ;
#46244=CARTESIAN_POINT ( 'NONE',  ( 15.72974639402199770, -15.80617190586745480, 103.1239096053143811 ) ) ;
#46245=CARTESIAN_POINT ( 'NONE',  ( 19.05341960407611168, 5.049401038298154454, 98.95724293864766707 ) ) ;
#46246=ORIENTED_EDGE ( 'NONE', *, *, #26316, .F. ) ;
#46247=CARTESIAN_POINT ( 'NONE',  ( -21.52544592524334988, -5.823673210054445271, 33.95942372801901143 ) ) ;
#46248=VERTEX_POINT ( 'NONE', #152108 ) ;
#46249=CARTESIAN_POINT ( 'NONE',  ( 9.474510206698971260, -16.51473224551069308, 97.91557627198102409 ) ) ;
#46252=CARTESIAN_POINT ( 'NONE',  ( -18.62759615963270932, 10.81492255796079327, 90.83224293864769550 ) ) ;
#46253=CARTESIAN_POINT ( 'NONE',  ( 9.564922557960805705, 16.46253265017160317, 44.58224293864769550 ) ) ;
#46254=CARTESIAN_POINT ( 'NONE',  ( -0.05219959533934338120, 16.53943276465976808, 27.50109039468567929 ) ) ;
#46256=CARTESIAN_POINT ( 'NONE',  ( -5.049401038298153566, 19.05341960407611168, 25.20724293864768484 ) ) ;
#46257=CARTESIAN_POINT ( 'NONE',  ( 0.05219959533937995610, -21.53943276465977519, 100.0010903946857042 ) ) ;
#46258=CARTESIAN_POINT ( 'NONE',  ( 0.05219959533909260263, 19.03943276465977164, 79.99890960531436690 ) ) ;
#46259=CARTESIAN_POINT ( 'NONE',  ( 10.72451020669871369, 18.67979575497193778, 47.08442372801901854 ) ) ;
#46260=CARTESIAN_POINT ( 'NONE',  ( 10.72451020669871369, 18.67979575497193778, 27.08442372801901854 ) ) ;
#46262=CARTESIAN_POINT ( 'NONE',  ( -9.564922557960796823, -16.46253265017161027, 97.08224293864769550 ) ) ;
#46264=CARTESIAN_POINT ( 'NONE',  ( 16.55341960407618274, -4.379528057220086978, 46.04275706135234714 ) ) ;
#46265=CARTESIAN_POINT ( 'NONE',  ( -14.29746914071037622, -8.314922557961029526, 74.16775706135231871 ) ) ;
#46266=CARTESIAN_POINT ( 'NONE',  ( -15.80617190586768217, 15.72974639402176855, 58.12609039468568994 ) ) ;
#46267=CARTESIAN_POINT ( 'NONE',  ( -10.81492255796105439, 18.62759615963255655, 77.91775706135231871 ) ) ;
#46269=CARTESIAN_POINT ( 'NONE',  ( -16.46253265017146816, -9.564922557961047289, 109.1677570613523471 ) ) ;
#46270=CARTESIAN_POINT ( 'NONE',  ( -16.51473224551069308, -9.474510206698971260, 71.66557627198102409 ) ) ;
#46271=CARTESIAN_POINT ( 'NONE',  ( -5.049401038298153566, 19.05341960407611168, 100.2072429386476955 ) ) ;
#46272=CARTESIAN_POINT ( 'NONE',  ( 4.379528057220339221, -16.55341960407611168, 107.7072429386476955 ) ) ;
#46273=CARTESIAN_POINT ( 'NONE',  ( -15.72974639402197994, 15.80617190586746368, 35.62390960531437401 ) ) ;
#46274=CARTESIAN_POINT ( 'NONE',  ( 0.05219959533934541429, -16.53943276465976808, 95.00109039468568994 ) ) ;
#46275=CARTESIAN_POINT ( 'NONE',  ( -12.06949235617756955, 12.14591786802309770, 70.62390960531436690 ) ) ;
#46276=CARTESIAN_POINT ( 'NONE',  ( -13.89961937509977652, 13.97604488694528158, 50.62390960531435979 ) ) ;
#46277=CARTESIAN_POINT ( 'NONE',  ( -21.53943276465977519, -0.05219959533937600094, 73.75109039468567573 ) ) ;
#46279=CARTESIAN_POINT ( 'NONE',  ( 9.474510206698729675, 16.51473224551082808, 102.0844237280190043 ) ) ;
#46280=CARTESIAN_POINT ( 'NONE',  ( -12.14591786802309592, -12.06949235617757132, 81.87390960531435269 ) ) ;
#46281=CARTESIAN_POINT ( 'NONE',  ( 21.52544592524334988, 5.823673210054432836, 26.45942372801901854 ) ) ;
#46282=CARTESIAN_POINT ( 'NONE',  ( -21.55341960407610458, -5.719274019375992779, 61.45724293864770260 ) ) ;
#46283=CARTESIAN_POINT ( 'NONE',  ( -16.31925111598456724, -7.325300261831553250, 104.8357546103274842 ) ) ;
#46285=CARTESIAN_POINT ( 'NONE',  ( 5.153800228976335163, 19.02544592524342804, 84.79057627198099567 ) ) ;
#46286=CARTESIAN_POINT ( 'NONE',  ( 16.53943276465976808, -0.05219959533910856209, 48.74890960531435979 ) ) ;
#46287=CARTESIAN_POINT ( 'NONE',  ( 14.29746914071049879, -8.314922557960816363, 28.33224293864769550 ) ) ;
#46288=CARTESIAN_POINT ( 'NONE',  ( -12.14591786802326823, 12.06949235617739902, 93.12609039468568994 ) ) ;
#46289=CARTESIAN_POINT ( 'NONE',  ( 19.02544592524334988, 5.153800228976608722, 46.45942372801899012 ) ) ;
#46290=CARTESIAN_POINT ( 'NONE',  ( 16.36317988757058117, 7.306389748694953390, 48.40210391636776421 ) ) ;
#46291=CARTESIAN_POINT ( 'NONE',  ( -5.049401038298153566, 19.05341960407611168, 110.2072429386476671 ) ) ;
#46292=CARTESIAN_POINT ( 'NONE',  ( 16.53943276465976808, -0.05219959533910856209, 73.74890960531433848 ) ) ;
#46293=CARTESIAN_POINT ( 'NONE',  ( 19.03943276465977164, 0.05219959533936151252, 46.25109039468566863 ) ) ;
#46294=CARTESIAN_POINT ( 'NONE',  ( -0.05219959533909027116, -19.03943276465977164, 32.49890960531435979 ) ) ;
#46295=CARTESIAN_POINT ( 'NONE',  ( -21.53943276465977519, 0.05219959533907696930, 41.24890960531435269 ) ) ;
#46296=CARTESIAN_POINT ( 'NONE',  ( 21.55341960407610458, 5.719274019375980345, 68.95724293864769550 ) ) ;
#46298=CARTESIAN_POINT ( 'NONE',  ( -0.05219959533910754901, -16.53943276465976808, 97.49890960531436690 ) ) ;
#46299=CARTESIAN_POINT ( 'NONE',  ( 12.14591786802327356, -12.06949235617739191, 55.62609039468568284 ) ) ;
#46300=EDGE_CURVE ( 'NONE', #160624, #46248, #45316, .T. ) ;
#46301=CARTESIAN_POINT ( 'NONE',  ( -12.06949235617756955, 12.14591786802309770, 90.62390960531436690 ) ) ;
#46302=CARTESIAN_POINT ( 'NONE',  ( 17.44270441346514389, -5.991230190323080684, 36.13664920735772768 ) ) ;
#46304=CARTESIAN_POINT ( 'NONE',  ( 15.80617190586746368, 15.72974639402197994, 39.37390960531436690 ) ) ;
#46307=CARTESIAN_POINT ( 'NONE',  ( 8.224510206698742110, 14.34966873604972548, 37.08442372801901143 ) ) ;
#46308=CARTESIAN_POINT ( 'NONE',  ( -8.314922557960811034, -14.29746914071050412, 27.08224293864769550 ) ) ;
#46309=CARTESIAN_POINT ( 'NONE',  ( -21.52544592524343514, 5.823673210054127303, 56.04057627198102409 ) ) ;
#46310=AXIS2_PLACEMENT_3D ( 'NONE', #71865, #133533, #72882 ) ;
#46311=CARTESIAN_POINT ( 'NONE',  ( 0.05219959533936267826, -19.03943276465977164, 80.00109039468567573 ) ) ;
#46312=CARTESIAN_POINT ( 'NONE',  ( -18.67979575497178146, -10.72451020669898902, 66.66557627198102409 ) ) ;
#46313=CARTESIAN_POINT ( 'NONE',  ( 15.72974639402176855, 15.80617190586768217, 76.87609039468567573 ) ) ;
#46315=CARTESIAN_POINT ( 'NONE',  ( -16.55341960407617563, 4.379528057220093196, 43.54275706135235424 ) ) ;
#46316=CARTESIAN_POINT ( 'NONE',  ( 5.049401038298161559, -19.05341960407611168, 42.70724293864767418 ) ) ;
#46317=CARTESIAN_POINT ( 'NONE',  ( -5.153800228976328057, -19.02544592524343514, 97.29057627198099567 ) ) ;
#46318=CARTESIAN_POINT ( 'NONE',  ( -13.97604488694527625, -13.89961937509977652, 36.87390960531436690 ) ) ;
#46319=CARTESIAN_POINT ( 'NONE',  ( -14.34966873604960291, -8.224510206698953496, 106.6655762719810383 ) ) ;
#46321=FACE_BOUND ( 'NONE', #104468, .T. ) ;
#46323=CARTESIAN_POINT ( 'NONE',  ( 4.483927247898790824, -16.52544592524335698, 75.20942372801901854 ) ) ;
#46324=CARTESIAN_POINT ( 'NONE',  ( -5.823673210054116645, -21.52544592524344225, 87.29057627198103830 ) ) ;
#46325=CARTESIAN_POINT ( 'NONE',  ( 19.02544592524343514, -5.153800228976328945, 53.54057627198102409 ) ) ;
#46326=CARTESIAN_POINT ( 'NONE',  ( -5.719274019375665041, -21.55341960407619695, 24.79275706135235779 ) ) ;
#46327=CARTESIAN_POINT ( 'NONE',  ( 0.05219959533909260263, 19.03943276465977164, 79.99890960531436690 ) ) ;
#46329=CARTESIAN_POINT ( 'NONE',  ( 0.05219959533937995610, -21.53943276465977519, 20.00109039468568639 ) ) ;
#46330=CARTESIAN_POINT ( 'NONE',  ( 19.05341960407611168, 5.049401038298154454, 23.95724293864769194 ) ) ;
#46331=CARTESIAN_POINT ( 'NONE',  ( -13.89961937509977652, 13.97604488694528158, 105.6239096053143527 ) ) ;
#46332=CARTESIAN_POINT ( 'NONE',  ( 9.564922557961047289, -16.46253265017146816, 75.41775706135234714 ) ) ;
#46333=CARTESIAN_POINT ( 'NONE',  ( -19.02544592524334988, -5.153800228976617603, 28.95942372801900433 ) ) ;
#46334=CARTESIAN_POINT ( 'NONE',  ( 21.53943276465977519, -0.05219959533907433946, 98.74890960531438111 ) ) ;
#46335=CARTESIAN_POINT ( 'NONE',  ( 9.474510206698729675, 16.51473224551082808, 37.08442372801899722 ) ) ;
#46336=CARTESIAN_POINT ( 'NONE',  ( 14.29746914071037800, 8.314922557961029526, 81.66775706135236135 ) ) ;
#46337=CARTESIAN_POINT ( 'NONE',  ( 13.97604488694527802, 13.89961937509977652, 109.3739096053143669 ) ) ;
#46338=CARTESIAN_POINT ( 'NONE',  ( 9.474510206698971260, -16.51473224551069308, 57.91557627198103120 ) ) ;
#46339=CARTESIAN_POINT ( 'NONE',  ( 18.67979575497194134, -10.72451020669871369, 60.83442372801901854 ) ) ;
#46340=CARTESIAN_POINT ( 'NONE',  ( 10.72451020669871369, 18.67979575497193778, 82.08442372801901854 ) ) ;
#46341=CARTESIAN_POINT ( 'NONE',  ( 0.05219959533909260263, 19.03943276465977164, 79.99890960531436690 ) ) ;
#46342=CARTESIAN_POINT ( 'NONE',  ( -15.80617190586768217, 15.72974639402176855, 43.12609039468568284 ) ) ;
#46343=CARTESIAN_POINT ( 'NONE',  ( 13.97604488694548053, -13.89961937509957401, 85.62609039468568994 ) ) ;
#46344=CARTESIAN_POINT ( 'NONE',  ( 19.05341960407611168, 5.049401038298154454, 53.95724293864770260 ) ) ;
#46345=CARTESIAN_POINT ( 'NONE',  ( 19.05341960407611168, 5.049401038298154454, 98.95724293864766707 ) ) ;
#46346=CARTESIAN_POINT ( 'NONE',  ( 5.153800228976335163, 19.02544592524342804, 59.79057627198100988 ) ) ;
#46347=CARTESIAN_POINT ( 'NONE',  ( 17.58332526062529411, -7.635886036038496805, 78.42334959558466778 ) ) ;
#46348=CARTESIAN_POINT ( 'NONE',  ( -13.97604488694527625, -13.89961937509977652, 46.87390960531435979 ) ) ;
#46349=CARTESIAN_POINT ( 'NONE',  ( -15.72974639402197994, 15.80617190586746368, 100.6239096053143811 ) ) ;
#46350=CARTESIAN_POINT ( 'NONE',  ( 12.14591786802327356, -12.06949235617739191, 85.62609039468568994 ) ) ;
#46352=CARTESIAN_POINT ( 'NONE',  ( 9.474510206698729675, 16.51473224551082808, 42.08442372801900433 ) ) ;
#46353=CARTESIAN_POINT ( 'NONE',  ( 9.474510206698971260, -16.51473224551069308, 62.91557627198102409 ) ) ;
#46354=CARTESIAN_POINT ( 'NONE',  ( 16.52544592524342804, -4.483927247898539470, 63.54057627198103830 ) ) ;
#46355=CARTESIAN_POINT ( 'NONE',  ( -8.224510206698948167, 14.34966873604960824, 90.41557627198103830 ) ) ;
#46356=CARTESIAN_POINT ( 'NONE',  ( 19.03943276465977164, -0.05219959533909143690, 113.7489096053143669 ) ) ;
#46357=CARTESIAN_POINT ( 'NONE',  ( 5.049401038298161559, -19.05341960407611168, 97.70724293864766707 ) ) ;
#46358=CARTESIAN_POINT ( 'NONE',  ( -19.03943276465977164, 0.05219959533909376836, 101.2489096053143669 ) ) ;
#46359=CARTESIAN_POINT ( 'NONE',  ( -19.05341960407617563, 5.049401038297882671, 23.54275706135233648 ) ) ;
#46360=CARTESIAN_POINT ( 'NONE',  ( -14.29746914071037622, -8.314922557961029526, 99.16775706135234714 ) ) ;
#46361=CARTESIAN_POINT ( 'NONE',  ( 5.153800228976335163, 19.02544592524342804, 74.79057627198103830 ) ) ;
#46362=CARTESIAN_POINT ( 'NONE',  ( -18.62759615963255300, -10.81492255796106328, 34.16775706135234714 ) ) ;
#46363=CARTESIAN_POINT ( 'NONE',  ( -21.55341960407610458, -5.719274019375992779, 26.45724293864768839 ) ) ;
#46364=CARTESIAN_POINT ( 'NONE',  ( 21.55341960407610458, 5.719274019375980345, 113.9572429386477239 ) ) ;
#46365=CARTESIAN_POINT ( 'NONE',  ( 21.53943276465977519, -0.05219959533907433946, 73.74890960531433848 ) ) ;
#46366=CARTESIAN_POINT ( 'NONE',  ( -5.049401038298153566, 19.05341960407611168, 50.20724293864770260 ) ) ;
#46367=CARTESIAN_POINT ( 'NONE',  ( -16.55341960407611168, -4.379528057220339221, 81.45724293864769550 ) ) ;
#46368=CARTESIAN_POINT ( 'NONE',  ( -19.02544592524334988, -5.153800228976617603, 48.95942372801900433 ) ) ;
#46369=CARTESIAN_POINT ( 'NONE',  ( 9.474510206698971260, -16.51473224551069308, 22.91557627198102765 ) ) ;
#46370=CARTESIAN_POINT ( 'NONE',  ( 19.03943276465977164, -0.05219959533909143690, 88.74890960531436690 ) ) ;
#46371=CARTESIAN_POINT ( 'NONE',  ( 9.474510206698971260, -16.51473224551069308, 77.91557627198103830 ) ) ;
#46373=CARTESIAN_POINT ( 'NONE',  ( 4.483927247898545687, 16.52544592524342804, 94.79057627198105251 ) ) ;
#46375=CARTESIAN_POINT ( 'NONE',  ( -4.379528057220086978, -16.55341960407618274, 104.7927570613523898 ) ) ;
#46376=CARTESIAN_POINT ( 'NONE',  ( 12.06949235617739724, 12.14591786802326823, 21.87609039468567573 ) ) ;
#46377=CARTESIAN_POINT ( 'NONE',  ( 5.719274019375673035, 21.55341960407619339, 97.29275706135234714 ) ) ;
#46378=CARTESIAN_POINT ( 'NONE',  ( -9.564922557960796823, -16.46253265017161027, 97.08224293864769550 ) ) ;
#46379=CARTESIAN_POINT ( 'NONE',  ( 18.62759615963255655, 10.81492255796105972, 21.66775706135235069 ) ) ;
#46380=CARTESIAN_POINT ( 'NONE',  ( -9.474510206698964154, 16.51473224551069663, 25.41557627198103120 ) ) ;
#46381=CARTESIAN_POINT ( 'NONE',  ( 12.14591786802327356, -12.06949235617739191, 30.62609039468567929 ) ) ;
#46382=EDGE_CURVE ( 'NONE', #93673, #115190, #134498, .T. ) ;
#46383=CARTESIAN_POINT ( 'NONE',  ( 19.05341960407617918, -5.049401038297876454, 101.0427570613523045 ) ) ;
#46385=CARTESIAN_POINT ( 'NONE',  ( 5.823673210054125526, 21.52544592524343514, 89.79057627198103830 ) ) ;
#46386=CARTESIAN_POINT ( 'NONE',  ( -19.05341960407617563, 5.049401038297882671, 63.54275706135234003 ) ) ;
#46387=CARTESIAN_POINT ( 'NONE',  ( -18.22780087662126647, -5.499999999999827693, 63.98236817873107185 ) ) ;
#46388=CARTESIAN_POINT ( 'NONE',  ( -21.52544592524334988, -5.823673210054445271, 23.95942372801901143 ) ) ;
#46390=CARTESIAN_POINT ( 'NONE',  ( 19.02544592524343514, -5.153800228976328945, 88.54057627198102409 ) ) ;
#46391=CARTESIAN_POINT ( 'NONE',  ( 14.29746914071037800, 8.314922557961029526, 51.66775706135234714 ) ) ;
#46393=CARTESIAN_POINT ( 'NONE',  ( -9.474510206698720793, -16.51473224551083518, 64.58442372801900433 ) ) ;
#46394=CARTESIAN_POINT ( 'NONE',  ( -21.53943276465977519, 0.05219959533907696930, 111.2489096053143669 ) ) ;
#46395=CARTESIAN_POINT ( 'NONE',  ( 16.52544592524342804, -4.483927247898539470, 73.54057627198102409 ) ) ;
#46396=CARTESIAN_POINT ( 'NONE',  ( 9.564922557960805705, 16.46253265017160317, 89.58224293864769550 ) ) ;
#46397=CARTESIAN_POINT ( 'NONE',  ( -4.379528057220086978, -16.55341960407618274, 49.79275706135234714 ) ) ;
#46398=CARTESIAN_POINT ( 'NONE',  ( -19.02544592524334988, -5.153800228976617603, 58.95942372801900433 ) ) ;
#46399=CARTESIAN_POINT ( 'NONE',  ( -18.62759615963255300, -10.81492255796106328, 64.16775706135234714 ) ) ;
#46400=CARTESIAN_POINT ( 'NONE',  ( 16.55341960407618274, -4.379528057220086978, 31.04275706135234714 ) ) ;
#46401=CARTESIAN_POINT ( 'NONE',  ( -19.02544592524342804, 5.153800228976336051, 66.04057627198103830 ) ) ;
#46402=CARTESIAN_POINT ( 'NONE',  ( -13.97604488694547697, 13.89961937509957934, 93.12609039468566152 ) ) ;
#46403=CARTESIAN_POINT ( 'NONE',  ( -4.379528057220086978, -16.55341960407618274, 49.79275706135234714 ) ) ;
#46404=CARTESIAN_POINT ( 'NONE',  ( -15.72974639402176322, -15.80617190586768395, 104.3760903946856899 ) ) ;
#46405=CARTESIAN_POINT ( 'NONE',  ( 0.05219959533936267826, -19.03943276465977164, 75.00109039468566152 ) ) ;
#46406=CARTESIAN_POINT ( 'NONE',  ( 19.03943276465977164, -0.05219959533909143690, 43.74890960531435979 ) ) ;
#46407=CARTESIAN_POINT ( 'NONE',  ( 21.55341960407610458, 5.719274019375980345, 68.95724293864769550 ) ) ;
#46408=CARTESIAN_POINT ( 'NONE',  ( -0.05219959533910754901, -16.53943276465976808, 72.49890960531435269 ) ) ;
#46409=CARTESIAN_POINT ( 'NONE',  ( 16.46253265017146816, 9.564922557961045513, 76.66775706135234714 ) ) ;
#46410=CARTESIAN_POINT ( 'NONE',  ( -18.56101223717332260, -5.500000000000061284, 71.44978406935676674 ) ) ;
#46411=CARTESIAN_POINT ( 'NONE',  ( -19.02544592524334988, -5.153800228976617603, 38.95942372801900433 ) ) ;
#46412=EDGE_CURVE ( 'NONE', #53443, #176653, #91117, .T. ) ;
#46413=CARTESIAN_POINT ( 'NONE',  ( -14.34966873604972548, 8.224510206698743886, 108.3344237280190185 ) ) ;
#46414=CARTESIAN_POINT ( 'NONE',  ( 14.29746914071049879, -8.314922557960816363, 68.33224293864769550 ) ) ;
#46415=CARTESIAN_POINT ( 'NONE',  ( 10.81492255796106328, -18.62759615963255655, 100.4177570613523471 ) ) ;
#46417=CARTESIAN_POINT ( 'NONE',  ( 0.05219959533907565091, 21.53943276465977519, 104.9989096053143669 ) ) ;
#46418=CARTESIAN_POINT ( 'NONE',  ( 5.153800228976335163, 19.02544592524342804, 59.79057627198100988 ) ) ;
#46419=CARTESIAN_POINT ( 'NONE',  ( -21.53943276465977519, -0.05219959533937600094, 83.75109039468568994 ) ) ;
#46420=CARTESIAN_POINT ( 'NONE',  ( -9.564922557960796823, -16.46253265017161027, 67.08224293864769550 ) ) ;
#46422=CARTESIAN_POINT ( 'NONE',  ( 16.51473224551069308, 9.474510206698969483, 24.16557627198102765 ) ) ;
#46423=CARTESIAN_POINT ( 'NONE',  ( -13.89961937509977652, 13.97604488694528158, 115.6239096053143669 ) ) ;
#46424=CARTESIAN_POINT ( 'NONE',  ( -0.05219959533910754901, -16.53943276465976808, 67.49890960531436690 ) ) ;
#46425=CARTESIAN_POINT ( 'NONE',  ( -5.153800228976328057, -19.02544592524343514, 27.29057627198103120 ) ) ;
#46426=CARTESIAN_POINT ( 'NONE',  ( 12.06949235617757843, -12.14591786802309237, 88.12390960531436690 ) ) ;
#46427=CARTESIAN_POINT ( 'NONE',  ( 21.53943276465977519, -0.05219959533907433946, 93.74890960531436690 ) ) ;
#46428=CARTESIAN_POINT ( 'NONE',  ( -0.05219959533937732626, 21.53943276465977519, 47.50109039468568994 ) ) ;
#46430=CARTESIAN_POINT ( 'NONE',  ( -16.52544592524335698, -4.483927247898792601, 53.95942372801900433 ) ) ;
#46431=CARTESIAN_POINT ( 'NONE',  ( 15.80617190586746368, 15.72974639402197994, 94.37390960531436690 ) ) ;
#46432=CARTESIAN_POINT ( 'NONE',  ( -5.153800228976607833, 19.02544592524334988, 22.70942372801899012 ) ) ;
#46433=CARTESIAN_POINT ( 'NONE',  ( -9.474510206698964154, 16.51473224551069663, 110.4155762719810383 ) ) ;
#46434=CARTESIAN_POINT ( 'NONE',  ( 15.80617190586769283, -15.72974639402175789, 45.62609039468567573 ) ) ;
#46435=CARTESIAN_POINT ( 'NONE',  ( 21.52544592524344225, -5.823673210054117533, 43.54057627198103830 ) ) ;
#46436=CARTESIAN_POINT ( 'NONE',  ( -8.314922557960811034, -14.29746914071050412, 27.08224293864769550 ) ) ;
#46437=CARTESIAN_POINT ( 'NONE',  ( -15.80617190586768217, 15.72974639402176855, 68.12609039468567573 ) ) ;
#46438=CARTESIAN_POINT ( 'NONE',  ( 21.55341960407619695, -5.719274019375665929, 91.04275706135236135 ) ) ;
#46439=CARTESIAN_POINT ( 'NONE',  ( -5.153800228976607833, 19.02544592524334988, 32.70942372801899722 ) ) ;
#46440=CARTESIAN_POINT ( 'NONE',  ( -14.29746914071037622, -8.314922557961029526, 84.16775706135234714 ) ) ;
#46441=CARTESIAN_POINT ( 'NONE',  ( 10.72451020669871369, 18.67979575497193778, 57.08442372801901854 ) ) ;
#46442=CARTESIAN_POINT ( 'NONE',  ( -5.153800228976328057, -19.02544592524343514, 47.29057627198102409 ) ) ;
#46443=CARTESIAN_POINT ( 'NONE',  ( 0.05219959533936267826, -19.03943276465977164, 25.00109039468566152 ) ) ;
#46444=CARTESIAN_POINT ( 'NONE',  ( 5.823673210054125526, 21.52544592524343514, 29.79057627198102409 ) ) ;
#46445=CARTESIAN_POINT ( 'NONE',  ( 21.55341960407610458, 5.719274019375980345, 113.9572429386477239 ) ) ;
#46446=CARTESIAN_POINT ( 'NONE',  ( 21.52544592524344225, -5.823673210054117533, 68.54057627198103830 ) ) ;
#46447=CARTESIAN_POINT ( 'NONE',  ( -16.53943276465976808, -0.05219959533934237506, 43.75109039468568284 ) ) ;
#46449=CARTESIAN_POINT ( 'NONE',  ( 10.81492255796078972, 18.62759615963270932, 74.58224293864768129 ) ) ;
#46450=CARTESIAN_POINT ( 'NONE',  ( -16.52544592524335698, -4.483927247898792601, 63.95942372801901854 ) ) ;
#46451=CARTESIAN_POINT ( 'NONE',  ( 12.06949235617757843, -12.14591786802309237, 63.12390960531435979 ) ) ;
#46453=CARTESIAN_POINT ( 'NONE',  ( 0.05219959533936267826, -19.03943276465977164, 110.0010903946856757 ) ) ;
#46455=CARTESIAN_POINT ( 'NONE',  ( 5.719274019375991003, -21.55341960407610458, 22.70724293864769194 ) ) ;
#46457=CARTESIAN_POINT ( 'NONE',  ( -12.14591786802326823, 12.06949235617739902, 43.12609039468568284 ) ) ;
#46458=CARTESIAN_POINT ( 'NONE',  ( -10.72451020669898014, 18.67979575497178502, 115.4155762719810241 ) ) ;
#46459=CARTESIAN_POINT ( 'NONE',  ( -18.67979575497178146, -10.72451020669898902, 26.66557627198103475 ) ) ;
#46460=CARTESIAN_POINT ( 'NONE',  ( 14.34966873604972726, -8.224510206698740333, 60.83442372801901854 ) ) ;
#46461=CARTESIAN_POINT ( 'NONE',  ( -19.03943276465977164, 0.05219959533909376836, 71.24890960531435269 ) ) ;
#46462=CARTESIAN_POINT ( 'NONE',  ( -5.823673210054431948, 21.52544592524334988, 42.70942372801901854 ) ) ;
#46463=CARTESIAN_POINT ( 'NONE',  ( 0.05219959533936267826, -19.03943276465977164, 105.0010903946856615 ) ) ;
#46464=CARTESIAN_POINT ( 'NONE',  ( 5.823673210054125526, 21.52544592524343514, 24.79057627198103120 ) ) ;
#46466=CARTESIAN_POINT ( 'NONE',  ( -19.03943276465977164, -0.05219959533935918106, 23.75109039468566152 ) ) ;
#46467=CARTESIAN_POINT ( 'NONE',  ( 12.06949235617739724, 12.14591786802326823, 36.87609039468568994 ) ) ;
#46468=CARTESIAN_POINT ( 'NONE',  ( 0.05219959533909260263, 19.03943276465977164, 94.99890960531436690 ) ) ;
#46469=CARTESIAN_POINT ( 'NONE',  ( -21.52544592524343514, 5.823673210054127303, 101.0405762719810383 ) ) ;
#46470=CARTESIAN_POINT ( 'NONE',  ( 0.05219959533909260263, 19.03943276465977164, 69.99890960531435269 ) ) ;
#46472=CARTESIAN_POINT ( 'NONE',  ( 8.314922557960818139, 14.29746914071049879, 79.58224293864769550 ) ) ;
#46473=CARTESIAN_POINT ( 'NONE',  ( 18.67979575497178502, 10.72451020669898547, 34.16557627198102409 ) ) ;
#46475=CARTESIAN_POINT ( 'NONE',  ( 8.314922557961029526, -14.29746914071037800, 60.41775706135235424 ) ) ;
#46476=CARTESIAN_POINT ( 'NONE',  ( 21.52544592524344225, -5.823673210054117533, 108.5405762719810241 ) ) ;
#46477=CARTESIAN_POINT ( 'NONE',  ( 5.153800228976615827, -19.02544592524334988, 80.20942372801901854 ) ) ;
#46478=CARTESIAN_POINT ( 'NONE',  ( 0.05219959533907565091, 21.53943276465977519, 34.99890960531435979 ) ) ;
#46479=CARTESIAN_POINT ( 'NONE',  ( -5.153800228976328057, -19.02544592524343514, 32.29057627198102409 ) ) ;
#46480=CARTESIAN_POINT ( 'NONE',  ( 18.62759615963271287, -10.81492255796078972, 68.33224293864769550 ) ) ;
#46481=CARTESIAN_POINT ( 'NONE',  ( 16.51473224551069308, 9.474510206698969483, 99.16557627198102409 ) ) ;
#46482=CARTESIAN_POINT ( 'NONE',  ( -21.55341960407619339, 5.719274019375674811, 98.54275706135234714 ) ) ;
#46483=CARTESIAN_POINT ( 'NONE',  ( -0.05219959533909027116, -19.03943276465977164, 57.49890960531435979 ) ) ;
#46484=CARTESIAN_POINT ( 'NONE',  ( 14.34966873604972726, -8.224510206698740333, 55.83442372801901854 ) ) ;
#46485=CARTESIAN_POINT ( 'NONE',  ( 19.03943276465977164, -0.05219959533909143690, 63.74890960531435979 ) ) ;
#46486=CARTESIAN_POINT ( 'NONE',  ( 5.823673210054444382, -21.52544592524334988, 80.20942372801901854 ) ) ;
#46488=CARTESIAN_POINT ( 'NONE',  ( 19.02544592524334988, 5.153800228976608722, 36.45942372801900433 ) ) ;
#46489=CARTESIAN_POINT ( 'NONE',  ( -9.564922557961040184, 16.46253265017147172, 37.91775706135233293 ) ) ;
#46490=CARTESIAN_POINT ( 'NONE',  ( -15.80617190586768217, 15.72974639402176855, 43.12609039468568284 ) ) ;
#46491=EDGE_CURVE ( 'NONE', #4215, #36339, #131967, .T. ) ;
#46493=CARTESIAN_POINT ( 'NONE',  ( -19.03943276465977164, -0.05219959533935918106, 33.75109039468566863 ) ) ;
#46494=CARTESIAN_POINT ( 'NONE',  ( 5.049401038298161559, -19.05341960407611168, 92.70724293864769550 ) ) ;
#46495=CARTESIAN_POINT ( 'NONE',  ( 19.05341960407611168, 5.049401038298154454, 63.95724293864769550 ) ) ;
#46496=CARTESIAN_POINT ( 'NONE',  ( -4.379528057220328563, 16.55341960407611168, 30.20724293864769550 ) ) ;
#46497=CARTESIAN_POINT ( 'NONE',  ( 10.72451020669898902, -18.67979575497178502, 22.91557627198102765 ) ) ;
#46498=CARTESIAN_POINT ( 'NONE',  ( 15.72974639402176855, 15.80617190586768217, 86.87609039468568994 ) ) ;
#46499=B_SPLINE_CURVE_WITH_KNOTS ( 'NONE', 3,
 ( #70242, #118750, #40902, #85389, #149085, #165252, #135904, #131910, #119738, #104564, #166246, #180439, #39890, #150078, #54071, #101557, #195603, #71240, #163249, #133912 ),
 .UNSPECIFIED., .F., .F.,
 ( 4, 2, 2, 2, 2, 2, 2, 2, 2, 4 ),
 ( 0.004000878361811928755, 0.004499404418915960331, 0.004997930476019991908, 0.005496456533124022617, 0.005994982590228054194, 0.006244245618780048732, 0.006493508647332044137, 0.006992034704436029743, 0.007490560761540015350, 0.007989086818644000956 ),
 .UNSPECIFIED. ) ;
#46501=CARTESIAN_POINT ( 'NONE',  ( 17.49999999999999645, 5.500000000000009770, 58.78230962303567253 ) ) ;
#46502=CARTESIAN_POINT ( 'NONE',  ( -0.05219959533937732626, 21.53943276465977519, 102.5010903946856899 ) ) ;
#46504=CARTESIAN_POINT ( 'NONE',  ( -5.049401038298153566, 19.05341960407611168, 30.20724293864768839 ) ) ;
#46505=CARTESIAN_POINT ( 'NONE',  ( 5.153800228976335163, 19.02544592524342804, 109.7905762719810099 ) ) ;
#46507=CARTESIAN_POINT ( 'NONE',  ( 30.00000000000000000, -1.163414459189985801E-14, 95.00000000000000000 ) ) ;
#46508=CARTESIAN_POINT ( 'NONE',  ( 12.06949235617739724, 12.14591786802326823, 46.87609039468568994 ) ) ;
#46509=B_SPLINE_CURVE_WITH_KNOTS ( 'NONE', 3,
 ( #25371, #176038, #37506, #55675, #145678, #99168 ),
 .UNSPECIFIED., .F., .F.,
 ( 4, 2, 4 ),
 ( 0.007228050697041520610, 0.007608510107494992694, 0.007988969517948463911 ),
 .UNSPECIFIED. ) ;
#46510=CARTESIAN_POINT ( 'NONE',  ( -0.05219959533907301413, -21.53943276465977519, 72.49890960531435269 ) ) ;
#46511=CARTESIAN_POINT ( 'NONE',  ( -12.14591786802309592, -12.06949235617757132, 36.87390960531435979 ) ) ;
#46512=CARTESIAN_POINT ( 'NONE',  ( 14.34966873604960469, 8.224510206698951720, 104.1655762719810241 ) ) ;
#46513=CARTESIAN_POINT ( 'NONE',  ( -19.03943276465977164, 0.05219959533909376836, 91.24890960531436690 ) ) ;
#46514=CARTESIAN_POINT ( 'NONE',  ( -16.51473224551082808, 9.474510206698731452, 23.33442372801900078 ) ) ;
#46515=CARTESIAN_POINT ( 'NONE',  ( 4.483927247898545687, 16.52544592524342804, 114.7905762719810383 ) ) ;
#46516=CARTESIAN_POINT ( 'NONE',  ( 0.05219959533937995610, -21.53943276465977519, 65.00109039468568994 ) ) ;
#46517=CARTESIAN_POINT ( 'NONE',  ( -13.97604488694527625, -13.89961937509977652, 111.8739096053143243 ) ) ;
#46518=CARTESIAN_POINT ( 'NONE',  ( 0.05219959533934541429, -16.53943276465976808, 105.0010903946856757 ) ) ;
#46519=CARTESIAN_POINT ( 'NONE',  ( 9.474510206698729675, 16.51473224551082808, 62.08442372801899722 ) ) ;
#46521=CARTESIAN_POINT ( 'NONE',  ( 5.719274019375991003, -21.55341960407610458, 22.70724293864769194 ) ) ;
#46522=CARTESIAN_POINT ( 'NONE',  ( 14.29746914071049879, -8.314922557960816363, 93.33224293864769550 ) ) ;
#46523=CARTESIAN_POINT ( 'NONE',  ( -9.564922557961040184, 16.46253265017147172, 52.91775706135233293 ) ) ;
#46524=CARTESIAN_POINT ( 'NONE',  ( 9.474510206698971260, -16.51473224551069308, 72.91557627198102409 ) ) ;
#46525=CARTESIAN_POINT ( 'NONE',  ( 16.53943276465976808, -0.05219959533910856209, 68.74890960531435269 ) ) ;
#46526=CARTESIAN_POINT ( 'NONE',  ( -0.05219959533936034679, 19.03943276465977164, 92.50109039468566152 ) ) ;
#46527=CARTESIAN_POINT ( 'NONE',  ( -5.823673210054116645, -21.52544592524344225, 52.29057627198102409 ) ) ;
#46529=CARTESIAN_POINT ( 'NONE',  ( 13.89961937509977652, -13.97604488694527269, 23.12390960531436335 ) ) ;
#46530=CARTESIAN_POINT ( 'NONE',  ( -16.61371651742602396, -7.165104196376045564, 31.14584930007003294 ) ) ;
#46531=CARTESIAN_POINT ( 'NONE',  ( -9.564922557960796823, -16.46253265017161027, 72.08224293864770971 ) ) ;
#46532=CARTESIAN_POINT ( 'NONE',  ( -15.80617190586745835, -15.72974639402198527, 76.87390960531439532 ) ) ;
#46533=VECTOR ( 'NONE', #87393, 1000.000000000000000 ) ;
#46534=CARTESIAN_POINT ( 'NONE',  ( -12.14591786802326823, 12.06949235617739902, 93.12609039468568994 ) ) ;
#46535=CARTESIAN_POINT ( 'NONE',  ( 19.03943276465977164, -0.05219959533909143690, 73.74890960531435269 ) ) ;
#46536=CARTESIAN_POINT ( 'NONE',  ( 5.153800228976615827, -19.02544592524334988, 65.20942372801900433 ) ) ;
#46537=CARTESIAN_POINT ( 'NONE',  ( 0.05219959533937995610, -21.53943276465977519, 85.00109039468568994 ) ) ;
#46538=CARTESIAN_POINT ( 'NONE',  ( 18.67979575497178502, 10.72451020669898547, 69.16557627198102409 ) ) ;
#46539=CARTESIAN_POINT ( 'NONE',  ( 10.81492255796078972, 18.62759615963270932, 24.58224293864768839 ) ) ;
#46540=CARTESIAN_POINT ( 'NONE',  ( 5.049401038298161559, -19.05341960407611168, 32.70724293864768129 ) ) ;
#46541=CARTESIAN_POINT ( 'NONE',  ( 16.53943276465976808, 0.05219959533934440121, 101.2510903946856757 ) ) ;
#46542=CARTESIAN_POINT ( 'NONE',  ( -9.564922557960796823, -16.46253265017161027, 47.08224293864769550 ) ) ;
#46543=CARTESIAN_POINT ( 'NONE',  ( -16.52544592524335698, -4.483927247898792601, 23.95942372801901143 ) ) ;
#46544=CARTESIAN_POINT ( 'NONE',  ( -9.564922557961040184, 16.46253265017147172, 82.91775706135233293 ) ) ;
#46545=CARTESIAN_POINT ( 'NONE',  ( 21.55341960407619695, -5.719274019375665929, 106.0427570613523471 ) ) ;
#46546=CARTESIAN_POINT ( 'NONE',  ( 14.34966873604960469, 8.224510206698951720, 64.16557627198102409 ) ) ;
#46547=CARTESIAN_POINT ( 'NONE',  ( -15.80617190586745835, -15.72974639402198527, 101.8739096053143811 ) ) ;
#46548=CARTESIAN_POINT ( 'NONE',  ( 5.719274019375991003, -21.55341960407610458, 102.7072429386476955 ) ) ;
#46550=CARTESIAN_POINT ( 'NONE',  ( 15.72974639402199770, -15.80617190586745480, 43.12390960531435269 ) ) ;
#46551=CARTESIAN_POINT ( 'NONE',  ( 4.483927247898790824, -16.52544592524335698, 85.20942372801901854 ) ) ;
#46552=CARTESIAN_POINT ( 'NONE',  ( 8.224510206698953496, -14.34966873604960469, 87.91557627198103830 ) ) ;
#46553=CARTESIAN_POINT ( 'NONE',  ( 19.05341960407611168, 5.049401038298154454, 58.95724293864768129 ) ) ;
#46554=CARTESIAN_POINT ( 'NONE',  ( -19.26498983726239089, 5.499999999999603872, 50.55319577422003618 ) ) ;
#46555=CARTESIAN_POINT ( 'NONE',  ( 0.05219959533934541429, -16.53943276465976808, 105.0010903946856757 ) ) ;
#46556=CARTESIAN_POINT ( 'NONE',  ( 21.55341960407619695, -5.719274019375665929, 31.04275706135234714 ) ) ;
#46557=CARTESIAN_POINT ( 'NONE',  ( 5.153800228976335163, 19.02544592524342804, 99.79057627198102409 ) ) ;
#46558=CARTESIAN_POINT ( 'NONE',  ( -21.53943276465977519, -0.05219959533937600094, 68.75109039468568994 ) ) ;
#46559=CARTESIAN_POINT ( 'NONE',  ( 9.474510206698971260, -16.51473224551069308, 22.91557627198102765 ) ) ;
#46560=CARTESIAN_POINT ( 'NONE',  ( -9.474510206698964154, 16.51473224551069663, 25.41557627198103120 ) ) ;
#46563=CARTESIAN_POINT ( 'NONE',  ( 15.80617190586769283, -15.72974639402175789, 65.62609039468568994 ) ) ;
#46564=CARTESIAN_POINT ( 'NONE',  ( -9.564922557960796823, -16.46253265017161027, 47.08224293864769550 ) ) ;
#46565=CARTESIAN_POINT ( 'NONE',  ( 16.51473224551069308, 9.474510206698969483, 84.16557627198102409 ) ) ;
#46566=CARTESIAN_POINT ( 'NONE',  ( 19.02544592524334988, 5.153800228976608722, 71.45942372801900433 ) ) ;
#46567=CARTESIAN_POINT ( 'NONE',  ( -18.67979575497193778, 10.72451020669871902, 48.33442372801902565 ) ) ;
#46568=CARTESIAN_POINT ( 'NONE',  ( 16.46253265017146816, 9.564922557961045513, 106.6677570613523471 ) ) ;
#46569=CARTESIAN_POINT ( 'NONE',  ( 5.049401038297881783, 19.05341960407617563, 72.29275706135234714 ) ) ;
#46570=CARTESIAN_POINT ( 'NONE',  ( -0.05219959533909027116, -19.03943276465977164, 37.49890960531436690 ) ) ;
#46571=CARTESIAN_POINT ( 'NONE',  ( -16.46253265017146816, -9.564922557961047289, 84.16775706135233293 ) ) ;
#46572=CARTESIAN_POINT ( 'NONE',  ( 16.53943276465976808, 0.05219959533934440121, 106.2510903946856757 ) ) ;
#46573=CARTESIAN_POINT ( 'NONE',  ( -16.51473224551082808, 9.474510206698731452, 78.33442372801900433 ) ) ;
#46574=CARTESIAN_POINT ( 'NONE',  ( -4.483927247898539470, -16.52544592524342804, 32.29057627198102409 ) ) ;
#46575=CARTESIAN_POINT ( 'NONE',  ( 16.46253265017146816, 9.564922557961045513, 51.66775706135233293 ) ) ;
#46576=CARTESIAN_POINT ( 'NONE',  ( 5.823673210054444382, -21.52544592524334988, 100.2094237280190043 ) ) ;
#46577=CARTESIAN_POINT ( 'NONE',  ( -16.46253265017146816, -9.564922557961047289, 19.16775706135233293 ) ) ;
#46578=CARTESIAN_POINT ( 'NONE',  ( 19.03943276465977164, -0.05219959533909143690, 23.74890960531435269 ) ) ;
#46579=CARTESIAN_POINT ( 'NONE',  ( 18.62759615963255655, 10.81492255796105972, 86.66775706135234714 ) ) ;
#46580=CARTESIAN_POINT ( 'NONE',  ( -16.55341960407617563, 4.379528057220093196, 38.54275706135234714 ) ) ;
#46581=CARTESIAN_POINT ( 'NONE',  ( -19.03943276465977164, 0.05219959533909376836, 91.24890960531436690 ) ) ;
#46583=CARTESIAN_POINT ( 'NONE',  ( -19.03943276465977164, 0.05219959533909376836, 81.24890960531436690 ) ) ;
#46586=CARTESIAN_POINT ( 'NONE',  ( -13.89961937509957401, -13.97604488694547875, 84.37609039468567573 ) ) ;
#46587=CARTESIAN_POINT ( 'NONE',  ( 9.564922557960805705, 16.46253265017160317, 109.5822429386476955 ) ) ;
#46588=CARTESIAN_POINT ( 'NONE',  ( 19.02544592524334988, 5.153800228976608722, 21.45942372801899012 ) ) ;
#46589=CARTESIAN_POINT ( 'NONE',  ( -19.02544592524334988, -5.153800228976617603, 103.9594237280190043 ) ) ;
#46590=CARTESIAN_POINT ( 'NONE',  ( 16.53943276465976808, -0.05219959533910856209, 93.74890960531436690 ) ) ;
#46591=CARTESIAN_POINT ( 'NONE',  ( -19.05341960407611168, -5.049401038298163336, 21.45724293864768839 ) ) ;
#46592=CARTESIAN_POINT ( 'NONE',  ( 15.80617190586746368, 15.72974639402197994, 59.37390960531436690 ) ) ;
#46594=CARTESIAN_POINT ( 'NONE',  ( -21.55341960407610458, -5.719274019375992779, 46.45724293864769550 ) ) ;
#46595=CARTESIAN_POINT ( 'NONE',  ( 12.14591786802309770, 12.06949235617756955, 114.3739096053143527 ) ) ;
#46597=CARTESIAN_POINT ( 'NONE',  ( 19.02544592524334988, 5.153800228976608722, 51.45942372801900433 ) ) ;
#46598=CARTESIAN_POINT ( 'NONE',  ( -8.314922557960811034, -14.29746914071050412, 42.08224293864769550 ) ) ;
#46599=CARTESIAN_POINT ( 'NONE',  ( -9.474510206698964154, 16.51473224551069663, 110.4155762719810383 ) ) ;
#46600=CARTESIAN_POINT ( 'NONE',  ( 10.81492255796106328, -18.62759615963255655, 75.41775706135233293 ) ) ;
#46601=CARTESIAN_POINT ( 'NONE',  ( 10.81492255796078972, 18.62759615963270932, 64.58224293864769550 ) ) ;
#46602=CARTESIAN_POINT ( 'NONE',  ( -15.72974639402176322, -15.80617190586768395, 54.37609039468568994 ) ) ;
#46603=CARTESIAN_POINT ( 'NONE',  ( -0.05219959533937732626, 21.53943276465977519, 57.50109039468568994 ) ) ;
#46604=CARTESIAN_POINT ( 'NONE',  ( 9.564922557960805705, 16.46253265017160317, 89.58224293864769550 ) ) ;
#46605=CARTESIAN_POINT ( 'NONE',  ( -4.379528057220086978, -16.55341960407618274, 79.79275706135236135 ) ) ;
#46606=CARTESIAN_POINT ( 'NONE',  ( -8.224510206698948167, 14.34966873604960824, 115.4155762719810241 ) ) ;
#46608=CARTESIAN_POINT ( 'NONE',  ( 12.06949235617757843, -12.14591786802309237, 68.12390960531436690 ) ) ;
#46609=CARTESIAN_POINT ( 'NONE',  ( 12.14591786802309770, 12.06949235617756955, 29.37390960531435269 ) ) ;
#46610=CARTESIAN_POINT ( 'NONE',  ( 5.049401038298161559, -19.05341960407611168, 67.70724293864769550 ) ) ;
#46611=CARTESIAN_POINT ( 'NONE',  ( 19.02544592524343514, -5.153800228976328945, 33.54057627198102409 ) ) ;
#46612=CARTESIAN_POINT ( 'NONE',  ( 0.05219959533907565091, 21.53943276465977519, 39.99890960531436690 ) ) ;
#46613=CARTESIAN_POINT ( 'NONE',  ( 9.474510206698729675, 16.51473224551082808, 32.08442372801900433 ) ) ;
#46616=CARTESIAN_POINT ( 'NONE',  ( 8.314922557960818139, 14.29746914071049879, 54.58224293864769550 ) ) ;
#46617=CARTESIAN_POINT ( 'NONE',  ( -18.62759615963270932, 10.81492255796079327, 30.83224293864770260 ) ) ;
#46618=CARTESIAN_POINT ( 'NONE',  ( 17.66907692000827979, 2.165031582823986778, 37.50000000000000000 ) ) ;
#46619=CARTESIAN_POINT ( 'NONE',  ( 8.314922557961029526, -14.29746914071037800, 70.41775706135236135 ) ) ;
#46620=CARTESIAN_POINT ( 'NONE',  ( -16.46253265017146816, -9.564922557961047289, 74.16775706135234714 ) ) ;
#46621=CARTESIAN_POINT ( 'NONE',  ( 14.34966873604960469, 8.224510206698951720, 44.16557627198103120 ) ) ;
#46623=CARTESIAN_POINT ( 'NONE',  ( -19.49190055781011921, -5.499999999999968026, 75.56116087098783396 ) ) ;
#46624=CARTESIAN_POINT ( 'NONE',  ( 16.55341960407611168, 4.379528057220329451, 23.95724293864769550 ) ) ;
#46625=CARTESIAN_POINT ( 'NONE',  ( -16.51473224551069308, -9.474510206698971260, 56.66557627198103120 ) ) ;
#46626=CARTESIAN_POINT ( 'NONE',  ( -5.153800228976328057, -19.02544592524343514, 57.29057627198103120 ) ) ;
#46627=CARTESIAN_POINT ( 'NONE',  ( 5.153800228976335163, 19.02544592524342804, 39.79057627198100988 ) ) ;
#46628=CARTESIAN_POINT ( 'NONE',  ( 10.72451020669871369, 18.67979575497193778, 47.08442372801901854 ) ) ;
#46629=CARTESIAN_POINT ( 'NONE',  ( -19.03943276465977164, 0.05219959533909376836, 61.24890960531436690 ) ) ;
#46630=CARTESIAN_POINT ( 'NONE',  ( 17.60769864724391098, -5.499999999999979572, 81.15024842019167295 ) ) ;
#46631=CARTESIAN_POINT ( 'NONE',  ( -13.97604488694527625, -13.89961937509977652, 41.87390960531435979 ) ) ;
#46632=CARTESIAN_POINT ( 'NONE',  ( -15.72974639402197994, 15.80617190586746368, 40.62390960531435269 ) ) ;
#46633=CARTESIAN_POINT ( 'NONE',  ( -5.823673210054431948, 21.52544592524334988, 77.70942372801900433 ) ) ;
#46634=CARTESIAN_POINT ( 'NONE',  ( -0.05219959533910754901, -16.53943276465976808, 112.4989096053143669 ) ) ;
#46635=CARTESIAN_POINT ( 'NONE',  ( 18.67979575497178502, 10.72451020669898547, 34.16557627198102409 ) ) ;
#46636=CARTESIAN_POINT ( 'NONE',  ( -12.06949235617739369, -12.14591786802326823, 94.37609039468568994 ) ) ;
#46637=CARTESIAN_POINT ( 'NONE',  ( -0.05219959533937732626, 21.53943276465977519, 102.5010903946856899 ) ) ;
#46638=CARTESIAN_POINT ( 'NONE',  ( 4.379528057220092307, 16.55341960407617563, 72.29275706135236135 ) ) ;
#46639=CARTESIAN_POINT ( 'NONE',  ( 19.03943276465977164, -0.05219959533909143690, 103.7489096053143669 ) ) ;
#46640=CARTESIAN_POINT ( 'NONE',  ( -4.379528057220086978, -16.55341960407618274, 49.79275706135234714 ) ) ;
#46641=CARTESIAN_POINT ( 'NONE',  ( -8.224510206698735004, -14.34966873604973081, 39.58442372801901143 ) ) ;
#46642=CARTESIAN_POINT ( 'NONE',  ( -12.06949235617739369, -12.14591786802326823, 99.37609039468568994 ) ) ;
#46643=CARTESIAN_POINT ( 'NONE',  ( -10.81492255796105439, 18.62759615963255655, 57.91775706135234714 ) ) ;
#46644=CARTESIAN_POINT ( 'NONE',  ( -8.314922557961024197, 14.29746914071037800, 22.91775706135235069 ) ) ;
#46645=CARTESIAN_POINT ( 'NONE',  ( -10.81492255796078084, -18.62759615963271287, 112.0822429386477097 ) ) ;
#46646=CARTESIAN_POINT ( 'NONE',  ( 14.34966873604972726, -8.224510206698740333, 25.83442372801901499 ) ) ;
#46647=CARTESIAN_POINT ( 'NONE',  ( 8.314922557961029526, -14.29746914071037800, 80.41775706135234714 ) ) ;
#46648=CARTESIAN_POINT ( 'NONE',  ( -17.48847506799950224, 5.747544572775299621, 45.82697437843291510 ) ) ;
#46649=CARTESIAN_POINT ( 'NONE',  ( 21.52544592524334988, 5.823673210054432836, 91.45942372801901854 ) ) ;
#46650=CARTESIAN_POINT ( 'NONE',  ( -13.89961937509957401, -13.97604488694547875, 89.37609039468563310 ) ) ;
#46652=CARTESIAN_POINT ( 'NONE',  ( 14.34966873604960469, 8.224510206698951720, 54.16557627198103120 ) ) ;
#46653=CARTESIAN_POINT ( 'NONE',  ( 4.379528057220339221, -16.55341960407611168, 37.70724293864769550 ) ) ;
#46654=CARTESIAN_POINT ( 'NONE',  ( -16.52544592524342804, 4.483927247898546575, 111.0405762719810525 ) ) ;
#46655=CARTESIAN_POINT ( 'NONE',  ( 5.153800228976615827, -19.02544592524334988, 50.20942372801897591 ) ) ;
#46657=CARTESIAN_POINT ( 'NONE',  ( 21.52544592524334988, 5.823673210054432836, 51.45942372801901854 ) ) ;
#46658=CARTESIAN_POINT ( 'NONE',  ( 13.97604488694548053, -13.89961937509957401, 105.6260903946856757 ) ) ;
#46660=CARTESIAN_POINT ( 'NONE',  ( 19.03943276465977164, -0.05219959533909143690, 108.7489096053143527 ) ) ;
#46661=CARTESIAN_POINT ( 'NONE',  ( 21.52544592524344225, -5.823673210054117533, 78.54057627198103830 ) ) ;
#46662=CARTESIAN_POINT ( 'NONE',  ( -13.97604488694547697, 13.89961937509957934, 98.12609039468566152 ) ) ;
#46663=CARTESIAN_POINT ( 'NONE',  ( -13.89961937509977652, 13.97604488694528158, 100.6239096053143669 ) ) ;
#46665=CARTESIAN_POINT ( 'NONE',  ( 0.05219959533910956823, 16.53943276465976808, 104.9989096053143669 ) ) ;
#46666=CARTESIAN_POINT ( 'NONE',  ( -0.05219959533937732626, 21.53943276465977519, 92.50109039468567573 ) ) ;
#46667=CARTESIAN_POINT ( 'NONE',  ( -13.89961937509977652, 13.97604488694528158, 25.62390960531434558 ) ) ;
#46668=CARTESIAN_POINT ( 'NONE',  ( -15.72974639402176322, -15.80617190586768395, 39.37609039468567573 ) ) ;
#46669=CARTESIAN_POINT ( 'NONE',  ( -5.719274019375665041, -21.55341960407619695, 89.79275706135236135 ) ) ;
#46670=CARTESIAN_POINT ( 'NONE',  ( 16.52544592524335698, 4.483927247898782831, 86.45942372801901854 ) ) ;
#46671=CARTESIAN_POINT ( 'NONE',  ( -21.52544592524334988, -5.823673210054445271, 48.95942372801902565 ) ) ;
#46672=CARTESIAN_POINT ( 'NONE',  ( 15.80617190586769283, -15.72974639402175789, 45.62609039468567573 ) ) ;
#46673=CARTESIAN_POINT ( 'NONE',  ( -5.049401038297874678, -19.05341960407617918, 64.79275706135233293 ) ) ;
#46674=CARTESIAN_POINT ( 'NONE',  ( 16.51473224551069308, 9.474510206698969483, 84.16557627198102409 ) ) ;
#46675=CARTESIAN_POINT ( 'NONE',  ( 16.53943276465976808, -0.05219959533910856209, 98.74890960531438111 ) ) ;
#46677=CARTESIAN_POINT ( 'NONE',  ( 5.823673210054125526, 21.52544592524343514, 84.79057627198102409 ) ) ;
#46678=CARTESIAN_POINT ( 'NONE',  ( -8.314922557960811034, -14.29746914071050412, 62.08224293864769550 ) ) ;
#46679=CARTESIAN_POINT ( 'NONE',  ( -15.72974639402176322, -15.80617190586768395, 109.3760903946857042 ) ) ;
#46680=CARTESIAN_POINT ( 'NONE',  ( 16.53943276465976808, -0.05219959533910856209, 88.74890960531436690 ) ) ;
#46681=CARTESIAN_POINT ( 'NONE',  ( 9.474510206698971260, -16.51473224551069308, 42.91557627198103120 ) ) ;
#46682=CARTESIAN_POINT ( 'NONE',  ( -0.05219959533936034679, 19.03943276465977164, 77.50109039468566152 ) ) ;
#46683=CARTESIAN_POINT ( 'NONE',  ( -8.224510206698948167, 14.34966873604960824, 30.41557627198101699 ) ) ;
#46684=CARTESIAN_POINT ( 'NONE',  ( -5.719274019375665041, -21.55341960407619695, 94.79275706135234714 ) ) ;
#46685=CARTESIAN_POINT ( 'NONE',  ( -16.51473224551069308, -9.474510206698971260, 86.66557627198102409 ) ) ;
#46686=CARTESIAN_POINT ( 'NONE',  ( -5.049401038297874678, -19.05341960407617918, 59.79275706135231871 ) ) ;
#46687=CARTESIAN_POINT ( 'NONE',  ( 21.52544592524344225, -5.823673210054117533, 63.54057627198103830 ) ) ;
#46688=CARTESIAN_POINT ( 'NONE',  ( 21.52544592524344225, -5.823673210054117533, 108.5405762719810241 ) ) ;
#46689=CARTESIAN_POINT ( 'NONE',  ( -13.89961937509957401, -13.97604488694547875, 109.3760903946856331 ) ) ;
#46690=CARTESIAN_POINT ( 'NONE',  ( 16.52544592524335698, 4.483927247898782831, 76.45942372801901854 ) ) ;
#46692=CARTESIAN_POINT ( 'NONE',  ( -18.62759615963270932, 10.81492255796079327, 115.8322429386477097 ) ) ;
#46693=CARTESIAN_POINT ( 'NONE',  ( 12.14591786802309770, 12.06949235617756955, 104.3739096053143669 ) ) ;
#46695=CARTESIAN_POINT ( 'NONE',  ( -8.314922557961024197, 14.29746914071037800, 47.91775706135234714 ) ) ;
#46696=CARTESIAN_POINT ( 'NONE',  ( -12.06949235617756955, 12.14591786802309770, 75.62390960531439532 ) ) ;
#46697=CARTESIAN_POINT ( 'NONE',  ( 5.719274019375991003, -21.55341960407610458, 72.70724293864769550 ) ) ;
#46698=CARTESIAN_POINT ( 'NONE',  ( 8.314922557961029526, -14.29746914071037800, 100.4177570613523471 ) ) ;
#46699=CARTESIAN_POINT ( 'NONE',  ( 14.34966873604972726, -8.224510206698740333, 35.83442372801901143 ) ) ;
#46700=CARTESIAN_POINT ( 'NONE',  ( -5.049401038298153566, 19.05341960407611168, 45.20724293864769550 ) ) ;
#46701=CARTESIAN_POINT ( 'NONE',  ( -14.29746914071037622, -8.314922557961029526, 84.16775706135234714 ) ) ;
#46702=CARTESIAN_POINT ( 'NONE',  ( 16.51473224551083163, -9.474510206698727899, 75.83442372801900433 ) ) ;
#46703=CARTESIAN_POINT ( 'NONE',  ( -10.81492255796078084, -18.62759615963271287, 72.08224293864769550 ) ) ;
#46704=CARTESIAN_POINT ( 'NONE',  ( -16.53943276465976808, -0.05219959533934237506, 103.7510903946857042 ) ) ;
#46705=CARTESIAN_POINT ( 'NONE',  ( 18.62759615963255655, 10.81492255796105972, 86.66775706135234714 ) ) ;
#46707=CARTESIAN_POINT ( 'NONE',  ( 15.72974639402199770, -15.80617190586745480, 63.12390960531435979 ) ) ;
#46708=CARTESIAN_POINT ( 'NONE',  ( 18.67979575497178502, 10.72451020669898547, 49.16557627198102409 ) ) ;
#46710=CARTESIAN_POINT ( 'NONE',  ( 8.224510206698742110, 14.34966873604972548, 82.08442372801901854 ) ) ;
#46711=CARTESIAN_POINT ( 'NONE',  ( 21.53943276465977519, -0.05219959533907433946, 43.74890960531435979 ) ) ;
#46713=CARTESIAN_POINT ( 'NONE',  ( -19.02544592524342804, 5.153800228976336051, 111.0405762719810099 ) ) ;
#46715=CARTESIAN_POINT ( 'NONE',  ( 16.46253265017160672, -9.564922557960803928, 23.33224293864769194 ) ) ;
#46716=CARTESIAN_POINT ( 'NONE',  ( -5.823673210054116645, -21.52544592524344225, 72.29057627198102409 ) ) ;
#46717=CARTESIAN_POINT ( 'NONE',  ( 0.05219959533934541429, -16.53943276465976808, 100.0010903946857042 ) ) ;
#46718=CARTESIAN_POINT ( 'NONE',  ( 10.72451020669871369, 18.67979575497193778, 47.08442372801901854 ) ) ;
#46719=CARTESIAN_POINT ( 'NONE',  ( -8.224510206698735004, -14.34966873604973081, 19.58442372801901143 ) ) ;
#46720=CARTESIAN_POINT ( 'NONE',  ( -0.05219959533909027116, -19.03943276465977164, 22.49890960531436690 ) ) ;
#46721=CARTESIAN_POINT ( 'NONE',  ( 5.049401038297881783, 19.05341960407617563, 112.2927570613523471 ) ) ;
#46722=CARTESIAN_POINT ( 'NONE',  ( 13.97604488694527802, 13.89961937509977652, 34.37390960531436690 ) ) ;
#46724=CARTESIAN_POINT ( 'NONE',  ( -13.97604488694527625, -13.89961937509977652, 101.8739096053143811 ) ) ;
#46726=CARTESIAN_POINT ( 'NONE',  ( -8.314922557961024197, 14.29746914071037800, 82.91775706135234714 ) ) ;
#46727=CARTESIAN_POINT ( 'NONE',  ( -0.05219959533936034679, 19.03943276465977164, 77.50109039468566152 ) ) ;
#46728=CARTESIAN_POINT ( 'NONE',  ( -9.564922557961040184, 16.46253265017147172, 22.91775706135233648 ) ) ;
#46729=CARTESIAN_POINT ( 'NONE',  ( -18.67979575497178146, -10.72451020669898902, 56.66557627198103830 ) ) ;
#46730=CARTESIAN_POINT ( 'NONE',  ( -0.05219959533934338120, 16.53943276465976808, 87.50109039468568994 ) ) ;
#46731=CARTESIAN_POINT ( 'NONE',  ( 9.474510206698729675, 16.51473224551082808, 92.08442372801900433 ) ) ;
#46732=CARTESIAN_POINT ( 'NONE',  ( 13.97604488694527802, 13.89961937509977652, 54.37390960531435979 ) ) ;
#46733=CARTESIAN_POINT ( 'NONE',  ( -13.89961937509977652, 13.97604488694528158, 85.62390960531433848 ) ) ;
#46735=CARTESIAN_POINT ( 'NONE',  ( 21.52544592524334988, 5.823673210054432836, 46.45942372801901854 ) ) ;
#46736=CARTESIAN_POINT ( 'NONE',  ( -13.97604488694527625, -13.89961937509977652, 41.87390960531435979 ) ) ;
#46737=CARTESIAN_POINT ( 'NONE',  ( -16.36317988757060249, -7.306389748694939179, 85.90210391636776421 ) ) ;
#46738=CARTESIAN_POINT ( 'NONE',  ( 19.03943276465977164, -0.05219959533909143690, 103.7489096053143669 ) ) ;
#46739=CARTESIAN_POINT ( 'NONE',  ( -12.06949235617756955, 12.14591786802309770, 70.62390960531436690 ) ) ;
#46740=CARTESIAN_POINT ( 'NONE',  ( -18.67979575497178146, -10.72451020669898902, 61.66557627198103120 ) ) ;
#46743=( BOUNDED_SURFACE ( )  B_SPLINE_SURFACE ( 3, 2, ( 
 ( #147779, #11269, #55754, #197275, #43584, #54754, #163953, #9265, #87091, #88081, #25451, #149767, #180132, #70931, #118439, #24439, #90074, #58738, #40594, #120407, #101243, #39584, #41601, #165941, #105250, #132598, #103266, #72942, #166936, #28439, #196296, #134612, #57766, #148776, #10265, #42595, #102265, #150775, #164946, #151757, #162932, #26439, #69931, #71924, #119436, #131595, #193280, #86088, #181121, #133594, #104258, #117428, #195286, #116428, #179126, #178116, #194288, #73935, #89083, #56767, #27441, #12270, #135604, #171891, #107218, #153730, #2035, #106232, #152733, #77877, #122392, #44576, #155718, #185069, #167915, #17215, #74913, #95036, #16225, #46557, #61707, #13250, #168889, #124384, #14223, #33378, #139544, #78867, #29415, #59732, #140547, #15226, #63715, #125390, #48557, #136576, #62701, #183095, #198256, #91046, #121401, #76885, #123377, #75893, #187087, #108219, #137568, #93042, #30394, #199251, #110210, #92041, #60718, #184081, #169899, #170893, #138556, #1029, #45565, #34, #186079, #47561, #109214, #31392, #154729, #32385, #94040, #49540, #128351, #83836, #126372, #66689, #145518, #112203, #97995, #192033, #6998, #111202, #159688, #189070, #190049, #142535, #81830, #38356, #65692, #64710, #79876, #160697, #175876, #68680, #51524, #188069, #53515, #115193, #50542, #97014, #130335, #172894, #96033, #21186, #127357, #34373, #99006, #113187, #157720, #22188, #18220, #156727, #82842, #174876, #5006, #141545, #173893, #67686, #19209, #176885, #144521, #3034, #80859, #4014, #35362, #158695, #20184, #143517, #36342, #6006, #129344, #191039, #52512, #114173, #37348, #102028, #10030, #162696, #104025, #133357, #100011, #179895, #194058, #161697, #88847, #178885, #27201, #181869, #195047, #57533, #117192, #26204, #39353, #101012, #87843, #149531, #134374, #40353, #163710, #86855, #193045, #54522, #177884, #41361, #85851, #150539, #12039, #84837, #55519, #24202, #25213, #118204, #148539, #103027, #71690, #147540, #56526, #116195, #120179, #73703, #70697, #135375, #131356, #69689, #164709, #196060, #197045, #9028, #11026, #72701, #58513, #23194, #119202, #180887, #42362, #165704, #146516, #8006, #132365, #124145, #169667, #108986, #125157, #107979, #13992, #74684, #47331, #89847, #199016, #1803, #92812, #800, #170667, #30162, #63481, #60485, #153498, #140313, #138334, #121169, #45337, #106989, #185844, #168662, #91806, #61481, #183849, #137336, #14995, #182863, #76655, #139320, #43348, #152503, #13019, #200014, #15994, #123152, #154499, #31162, #32155, #184840, #122160, #93812, #105019, #46325, #77652, #62473, #155492, #59494, #151530, #16984, #166703, #78638, #75659, #28206, #106002, #136350, #198026, #44344, #167689, #29186, #90820, #142301, #110968, #3781, #17988, #33149, #189819, #129105, #66454, #65458, #111967, #80624, #51291, #67447, #145282, #21953, #97762, #175635, #186856, #5772, #144283, #109980, #174645, #83603, #112952, #4767, #127121, #20945, #50311, #141310, #94807, #173659, #171660, #159449, #156486, #79641, #48325, #98768, #68444, #187840, #158467, #37109, #2799, #190804, #6765, #64477, #128116, #126144, #82602, #81597, #49309, #52278, #113936, #172652, #34140, #160462, #36110, #95799, #19955, #157485, #18978, #188827, #35126, #96778, #143281, #9792, #54288, #147298, #161463, #176648, #133119, #72460, #71454, #8787, #55280, #23956, #194808, #10792, #88610, #165471, #41125, #118971, #130098, #149298, #87612, #53276, #117964, #26967, #56282, #148298, #85611, #164475, #193815, #84601, #38124, #116951, #114955, #102789, #99778, #22953, #191795, #42130, #11803, #131117, #101784, #180654, #146280, #134134, #150306, #7767, #179655, #69450, #25969, #24969, #192806, #195823, #57294, #115960, #177648, #103791, #39116, #100772, #163472, #162455, #70457, #132122, #178643, #40106, #86615, #183620, #168435, #184605, #139083, #29931, #59260, #43115, #122917, #58281, #182628 ),
 ( #73467, #120929, #181635, #196814, #46086, #61245, #30927, #60255, #104783, #15754, #77413, #44113, #28954, #92575, #166471, #151298, #91570, #105771, #27969, #107741, #198789, #89609, #169422, #135140, #119950, #154263, #138097, #153258, #12787, #45103, #74452, #152277, #136118, #197794, #167458, #121926, #75429, #90595, #13761, #137103, #106760, #14760, #76421, #199778, #195469, #86264, #87268, #39758, #179305, #135779, #163113, #162110, #177301, #57942, #73121, #104436, #148952, #23607, #89261, #12447, #147954, #194459, #42774, #146945, #193457, #118618, #24616, #85253, #196472, #25623, #8434, #119613, #115612, #53937, #56944, #10442, #102438, #38773, #9441, #165121, #54934, #74109, #180308, #181296, #70106, #100429, #166120, #55930, #27622, #150953, #131775, #116606, #103442, #178294, #101421, #71106, #132772, #117605, #164125, #40769, #72102, #133775, #41776, #26613, #88256, #149943, #11449, #134790, #127280, #81757, #94969, #157645, #17146, #126301, #136748, #958, #187997, #49467, #34299, #140477, #78799, #187017, #90245, #151928, #75081, #141475, #186008, #188993, #112129, #182278, #93971, #62634, #1965, #18149, #155651, #79803, #110142, #124310, #48488, #13417, #20113, #50469, #170826, #173820, #28607, #167106, #171821, #95961, #35285, #47490, #33309, #2959, #96941, #158622, #111130, #64639, #172819, #63645, #125320, #19134, #32318, #80785, #156653, #197450, #109147, #142463, #58916, #3941, #65620, #120584, #43759, #105423, #25130, #84759, #21110, #39273, #38280, #40273, #147459, #85772, #143444, #82765, #24119, #23114, #7928, #176808, #51449, #162614, #4930, #113110, #144446, #178803, #146437, #69612, #8949, #66613, #131278, #114097, #174800, #70617, #189974, #98930, #101946, #192966, #100930, #132283, #130258, #163627, #160621, #53440, #128277, #99934, #5931, #145442, #6924, #193975, #68602, #191954, #161620, #83762, #37273, #115115, #67607, #54445, #55437, #36266, #52439, #97921, #116115, #177804, #117108, #159614, #129268, #190962, #175800, #22112, #171703, #128162, #189862, #111012, #141355, #156532, #108023, #1844, #19022, #109029, #66499, #172698, #50355, #843, #154541, #112014, #48368, #173703, #35171, #143325, #31203, #157528, #77694, #169710, #124188, #16036, #110025, #18031, #170708, #96826, #2842, #92854, #187883, #63526, #139362, #158510, #186897, #19997, #62516, #64520, #65503, #125201, #34183, #47374, #32198, #95844, #80668, #142344, #33192, #94851, #79685, #185889, #93855, #155532, #49350, #17027, #81641, #4811, #78680, #126187, #140356, #3824, #127164, #188872, #6810, #175679, #68488, #82645, #97806, #54330, #193857, #131161, #130143, #176694, #145328, #116001, #132166, #9835, #86655, #162498, #40150, #51336, #70498, #8830, #174690, #39158, #148339, #177690, #69496, #191840, #85655, #115000, #5817, #159495, #38168, #36154, #23999, #20990, #144328, #112996, #163513, #133160, #52324, #23000, #101826, #67493, #55322, #71494, #129150, #192851, #190847, #147342, #146323, #113981, #116993, #178688, #37153, #98813, #25012, #100815, #160507, #84646, #21997, #83650, #53321, #99823, #161508, #7812, #74495, #120971, #60294, #76462, #59302, #165514, #26010, #198830, #41168, #150350, #153300, #44153, #152317, #121968, #181677, #14801, #11847, #104825, #91612, #89654, #72504, #196857, #58323, #75469, #119991, #43158, #12829, #135183, #88654, #166514, #134179, #28012, #90635, #194852, #103833, #164517, #151340, #167500, #136161, #105813, #182669, #183660, #87653, #56325, #28995, #27010, #197836, #13803, #137142, #45145, #10834, #102831, #106801, #118007, #168475, #73512, #29973, #57339, #179696, #149338, #195866, #119014, #180697, #42173, #107779, #16785, #1600, #158271, #19760, #141112, #171463, #186653, #138139, #31955, #49115, #139123, #96582, #2601, #80426, #30965, #184644, #142099, #78435, #3584, #65262, #173458, #61287, #187644, #169464, #199819, #154303, #46125, #140109 ),
 ( #95599, #155295, #64279, #77452, #600, #125946, #110772, #172454, #63276, #124956, #48123, #92612, #15792, #62270, #79442, #123938, #126922, #50109, #122957, #93610, #185636, #109780, #156286, #32951, #17786, #94606, #47128, #33941, #108786, #170465, #188629, #157284, #111769, #18780, #34929, #129896, #177452, #70261, #20746, #114753, #22755, #116755, #193613, #7565, #84404, #146081, #36907, #21754, #54090, #113741, #162261, #53075, #8587, #51094, #191596, #131930, #98570, #69251, #178446, #55085, #35916, #130917, #175437, #176447, #67250, #6566, #163269, #190609, #189620, #4566, #85410, #100579, #39913, #37920, #112754, #101581, #81401, #160264, #83406, #143087, #174447, #82401, #192608, #52084, #66258, #127918, #115765, #97562, #159250, #23761, #38922, #144089, #147102, #5570, #128908, #99580, #145083, #68245, #161261, #179457, #132924, #88406, #9595, #135926, #71260, #56083, #24771, #136899, #106555, #25774, #196618, #75228, #194611, #43908, #183414, #86418, #166270, #102595, #120729, #119758, #121722, #28755, #167256, #148104, #164281, #105570, #104585, #89411, #58088, #117764, #90392, #40922, #87420, #149105, #60054, #27768, #151100, #152076, #10595, #12592, #195624, #72256, #13561, #133934, #180459, #44898, #74256, #182429, #198586, #11603, #57097, #41931, #134941, #118771, #181442, #103597, #26766, #150102, #165272, #73271, #42920, #197596, #59062, #62027, #78190, #45884, #16543, #64032, #65020, #77208, #137891, #139860, #140862, #93361, #17533, #94357, #172205, #199572, #126676, #2351, #357, #108541, #32705, #109534, #171216, #184403, #76212, #124706, #188380, #155048, #138877, #170220, #30722, #185390, #1349, #153052, #91361, #122713, #125702, #123692, #92369, #46881, #61041, #14554, #156036, #110524, #47881, #31713, #63029, #186404, #79193, #48869, #107537, #187401, #29728, #169213, #154055, #3345, #33690, #95353, #157038, #49857, #18535, #80182, #15550, #141854, #168232, #67007, #70014, #161016, #69003, #115520, #98316, #131683, #128666, #21503, #8339, #6322, #189377, #113497, #175192, #192363, #36658, #160016, #129654, #51838, #5323, #83164, #50854, #144838, #7319, #193364, #20500, #81164, #68002, #84157, #191350, #22510, #37668, #177208, #142846, #111523, #145837, #143844, #52828, #176199, #114497, #99333, #127677, #19519, #130669, #173208, #53846, #82148, #38681, #174205, #190362, #100337, #96341, #34684, #66009, #162016, #23512, #35673, #85159, #4325, #158028, #146845, #112512, #97321, #159007, #180214, #148858, #119520, #135684, #16061, #92878, #166024, #46391, #54840, #74014, #12351, #178202, #42679, #154565, #181202, #73024, #10349, #89165, #118525, #9350, #163016, #41684, #39666, #27524, #101328, #86174, #116515, #169734, #139385, #55838, #26520, #108049, #24523, #197356, #77719, #147864, #196379, #132683, #150857, #149849, #71015, #58820, #120488, #194371, #117512, #182179, #134696, #179209, #40676, #104340, #25533, #102346, #31229, #164035, #72006, #87177, #133679, #195371, #56850, #103348, #165027, #88165, #11353, #57848, #95873, #78708, #2871, #64549, #81670, #126214, #187910, #19049, #141383, #94880, #111042, #140385, #49379, #96854, #97834, #110052, #170732, #172729, #173732, #34210, #50384, #127192, #4842, #32223, #159522, #35201, #33220, #157556, #65532, #142373, #3853, #17053, #109055, #80696, #21019, #188904, #171732, #112044, #63553, #18059, #158538, #185914, #124217, #155559, #20028, #156561, #125227, #79714, #93881, #47399, #143353, #66528, #128191, #189889, #51364, #113025, #174717, #36180, #82674, #867, #62542, #1872, #186925, #48395, #101857, #67521, #132195, #41196, #70526, #162526, #38194, #178716, #7838, #98841, #52352, #69524, #129178, #55351, #190876, #175706, #144358, #56354, #26036, #145355, #116029, #194880, #114008, #163541, #102858, #5845, #85683, #22025, #40178, #39186, #164544, #148368, #86684, #37183, #83677, #99850, #8859, #25041 ),
 ( #146351, #131189, #24029, #84672, #161534, #54357, #6837, #192879, #9863, #160536, #53350, #68516, #177718, #117021, #100844, #193886, #71522, #133189, #130170, #191867, #118035, #176721, #147370, #179726, #115028, #23027, #103861, #195895, #44184, #184676, #74524, #58352, #89683, #150380, #104854, #121001, #72531, #10862, #42201, #45178, #43185, #11877, #166543, #119043, #134208, #90665, #30005, #167530, #28041, #12859, #181704, #152347, #168507, #46159, #122990, #198860, #76496, #87681, #106832, #91643, #57370, #75498, #107814, #13832, #105842, #151368, #122001, #136189, #165542, #180725, #197864, #27039, #60327, #88685, #73540, #149366, #199853, #169497, #135213, #59331, #138172, #196885, #153332, #120019, #182699, #29025, #137172, #183691, #14833, #61319, #34967, #173494, #112791, #170499, #124994, #95635, #50146, #47161, #139155, #111806, #92645, #633, #108820, #66295, #110809, #157323, #96619, #30996, #18818, #1637, #62303, #158308, #77486, #186689, #189658, #80462, #188667, #19796, #17823, #51131, #48159, #141150, #127954, #125983, #31989, #32989, #156323, #49151, #171500, #109817, #2639, #93647, #79481, #126958, #154334, #140145, #123973, #64315, #3620, #187681, #142136, #65299, #81437, #185670, #15825, #143123, #63314, #94642, #4603, #172491, #33979, #155332, #16820, #78471, #71301, #161299, #145121, #176485, #36946, #191634, #7603, #159286, #97598, #128945, #131968, #129935, #98608, #53114, #5607, #20783, #177491, #116793, #54128, #114792, #99619, #68284, #38960, #55124, #132964, #9634, #85449, #163311, #174485, #193652, #178485, #82438, #162299, #194653, #100617, #192645, #37961, #8627, #22795, #190646, #144126, #84441, #67287, #147139, #52122, #113778, #35952, #86458, #56123, #175474, #146119, #24809, #160302, #39951, #21792, #83443, #115801, #6605, #70299, #69289, #130955, #101622, #148143, #23799, #57137, #11646, #182469, #136941, #133975, #25813, #198630, #179498, #87459, #195666, #153094, #197637, #43950, #183457, #199616, #105612, #88449, #149146, #121764, #164320, #73312, #76254, #167300, #75271, #44943, #104625, #137932, #134983, #27811, #14598, #12632, #118813, #119799, #181484, #60096, #42962, #10636, #106598, #72296, #196661, #166314, #117805, #40963, #120768, #151141, #89452, #102635, #58130, #28796, #180499, #41971, #90435, #168274, #103638, #165316, #29771, #74297, #91406, #26809, #150144, #135966, #152121, #59103, #13603, #77249, #107580, #63073, #171261, #123735, #65061, #94400, #61082, #140909, #155090, #122755, #49899, #139903, #188422, #142886, #156081, #18577, #78232, #187444, #398, #62070, #48912, #110566, #95395, #1392, #124752, #47924, #154097, #15591, #138917, #2395, #46924, #111566, #173250, #45925, #16584, #185434, #186448, #79238, #109578, #64074, #32749, #108584, #17577, #170261, #81205, #34725, #31755, #96383, #92411, #157081, #125744, #169257, #184445, #93404, #172247, #33734, #158070, #19561, #80224, #141895, #3386, #126718, #30764, #177249, #36700, #85201, #176241, #131724, #174249, #114541, #193406, #160060, #145878, #39705, #54881, #159050, #7361, #98361, #37712, #190406, #129696, #86213, #113541, #112554, #127719, #8381, #23553, #116555, #99374, #35717, #101368, #163057, #21547, #144882, #178244, #97364, #143886, #69046, #175235, #83207, #161057, #82193, #52870, #100379, #24564, #6364, #20544, #22552, #38721, #191393, #53887, #130711, #70056, #5367, #4368, #162057, #68044, #84198, #192405, #115562, #146889, #67051, #128709, #66051, #189421, #50896, #51882, #149887, #10389, #165066, #181242, #132721, #71055, #102386, #105367, #103388, #72046, #26560, #179251, #194409, #150898, #90192, #27565, #88203, #73063, #41724, #12392, #28555, #106350, #183215, #58862, #136695, #147903, #167054, #151875, #55879, #135725, #44696, #74054, #166064, #11393, #182221, #134735, #164074, #117552, #196417, #40717, #120528, #25573, #87217, #9389, #59853, #29531, #148899 ),
 ( #133720, #195412, #57887, #197396, #13365, #56890, #118564, #75029, #180254, #119559, #42719, #168034, #89205, #43705, #198376, #104381, #121520, #61825, #122512, #95155, #137688, #46679, #49658, #140664, #48675, #156843, #77993, #111322, #108338, #1148, #188186, #186201, #169008, #93162, #154847, #172008, #16344, #139660, #109333, #31509, #45684, #32506, #123495, #124506, #77004, #62823, #173012, #156, #199373, #14348, #18338, #110327, #141661, #47683, #60837, #126488, #91164, #185188, #171015, #79993, #184202, #30512, #155837, #170019, #107335, #33496, #92164, #94158, #17334, #152853, #76013, #78990, #2156, #63834, #153850, #125507, #187204, #15348, #138676, #3153, #64826, #127479, #80977, #177010, #174995, #38479, #100136, #69809, #157838, #83962, #4131, #193163, #50657, #142652, #36460, #144643, #97128, #161817, #67809, #34491, #114301, #128468, #96149, #23312, #113304, #84956, #116310, #129464, #192161, #51640, #160823, #174008, #35479, #22311, #145642, #68804, #98117, #159814, #21309, #189184, #112318, #158812, #176003, #20300, #146638, #8131, #19329, #190164, #81948, #82966, #52636, #6126, #37472, #191163, #143640, #99133, #5123, #54635, #131476, #66805, #65810, #7122, #130463, #53641, #115318, #59614, #117310, #11151, #119319, #13139, #89964, #104144, #181006, #42481, #133477, #118323, #150660, #10149, #58629, #149653, #105138, #147661, #87965, #166824, #195169, #165826, #74801, #28325, #120295, #177999, #179006, #71809, #27323, #197163, #194173, #85971, #181988, #39466, #9148, #55637, #136464, #57653, #88970, #43470, #101127, #12158, #148661, #70815, #151644, #24322, #56650, #198144, #73823, #135493, #162813, #164829, #132484, #180016, #72825, #40474, #134494, #102146, #41483, #103148, #163831, #26325, #196181, #25333, #86974, #15110, #31274, #199133, #169781, #17101, #18105, #30276, #90932, #92925, #93927, #46437, #170780, #47445, #125275, #152618, #79759, #155606, #153614, #61593, #185960, #62587, #124265, #137454, #29302, #77764, #141430, #108096, #91922, #123262, #183963, #138443, #154611, #106118, #44464, #75776, #78753, #76771, #45450, #200124, #14109, #167802, #109101, #63599, #913, #184953, #16106, #139431, #32270, #1920, #2917, #156610, #140430, #110099, #121287, #186972, #48442, #60600, #171778, #182980, #33266, #94925, #122275, #107104, #168774, #19093, #172777, #128236, #49426, #175754, #111087, #95917, #64595, #179527, #149176, #65579, #36226, #117834, #34258, #86487, #25844, #126259, #5890, #142420, #163342, #159569, #164349, #71330, #35244, #157602, #132992, #80742, #20071, #87488, #114057, #24837, #194683, #51408, #187956, #81715, #174760, #3899, #21067, #127238, #66571, #189933, #148172, #113068, #97878, #82723, #4889, #158582, #144404, #188952, #67566, #9663, #50429, #173778, #112088, #129224, #37231, #190921, #101650, #52398, #56152, #96898, #143400, #40996, #102664, #151173, #75300, #152150, #13633, #26838, #118845, #167330, #107610, #197666, #181513, #12661, #73341, #27841, #43979, #195695, #134004, #165345, #168304, #166344, #135014, #89482, #42001, #57166, #136971, #153124, #90466, #74328, #135995, #104657, #198661, #91437, #169288, #45955, #121794, #199647, #10665, #29801, #14628, #180528, #60127, #30794, #183488, #28826, #59132, #44972, #120799, #88478, #103667, #182500, #150175, #106630, #11675, #196691, #72328, #122786, #92442, #58160, #105641, #61113, #119828, #76285, #42992, #137964, #184476, #31785, #49931, #48942, #50926, #158099, #96413, #35747, #93434, #47956, #18606, #173281, #170291, #62102, #34754, #15622, #123765, #155120, #189449, #33766, #80254, #19591, #154128, #141924, #77279, #81234, #142915, #4397, #110595, #185464, #112584, #174278, #109607, #94430, #66081, #46955, #16614, #3415, #63103, #108614, #127748, #78261, #32778, #17608, #138948, #428, #157110, #187473, #2426, #139934, #171291, #65090, #1423, #124781, #126749, #186479, #156111 ),
 ( #95426, #79268, #140939, #64106, #188451, #125773, #172277, #111596, #177283, #131757, #97393, #85235, #23587, #20573, #115594, #39739, #38754, #7395, #6395, #162092, #114576, #190436, #5397, #176275, #82225, #100411, #143916, #128740, #159079, #67080, #51912, #191425, #146925, #113571, #21578, #101401, #175265, #36731, #70088, #52901, #163094, #8416, #98393, #160092, #83236, #144912, #84232, #193439, #68074, #129728, #130745, #145910, #37746, #161089, #69079, #53920, #99406, #22584, #192438, #54915, #116587, #178276, #48600, #109257, #81875, #124427, #33422, #36385, #127403, #35404, #143567, #64752, #98039, #95081, #188111, #174921, #172937, #155761, #79916, #141588, #158738, #3076, #159736, #77920, #19254, #17259, #173936, #34416, #139587, #5049, #20227, #1072, #78912, #171933, #142578, #97055, #94082, #186123, #66735, #62747, #47603, #140589, #113231, #157764, #4057, #128395, #170936, #65735, #110252, #32428, #190092, #2079, #156769, #63758, #189112, #51567, #125432, #126414, #187128, #18263, #49583, #111246, #96075, #80901, #50585, #112245, #102073, #23238, #146561, #39397, #161743, #115239, #131402, #99052, #69734, #117239, #118250, #130381, #191084, #193090, #194103, #8056, #70743, #147588, #25258, #52557, #179941, #55565, #53561, #84882, #85900, #162742, #24250, #37394, #129388, #177930, #41408, #54566, #192079, #116238, #83882, #38401, #101057, #6052, #144566, #175923, #178932, #176931, #145564, #100058, #114218, #67730, #9073, #163758, #132411, #40402, #86901, #148584, #10076, #71734, #103073, #56576, #133404, #195093, #21233, #82888, #160741, #22233, #7042, #68724, #90862, #182906, #58558, #199059, #28253, #119248, #72751, #89892, #149577, #75700, #11073, #196108, #164755, #76700, #46365, #165752, #136394, #15039, #134422, #183895, #120224, #123194, #14035, #122203, #168705, #151575, #184883, #181914, #74730, #61525, #59537, #42407, #166749, #13064, #45380, #198071, #121216, #44390, #105065, #43394, #106045, #104070, #167731, #60528, #26250, #73748, #57578, #29229, #137380, #152547, #107033, #30207, #91849, #180932, #87891, #153542, #197091, #138376, #200056, #27245, #88894, #150586, #12085, #135420, #17320, #128452, #172996, #112302, #62808, #16329, #173992, #110312, #35461, #97112, #5107, #93147, #19312, #139646, #190148, #186186, #77979, #171994, #79979, #32491, #158795, #3137, #170003, #49644, #63819, #31494, #20284, #48660, #81930, #51623, #64812, #127462, #187189, #96133, #109319, #170999, #157822, #80960, #4114, #33482, #95140, #156829, #124490, #47667, #94144, #111307, #155823, #143622, #66788, #154831, #125492, #78975, #18322, #188171, #141647, #34474, #126473, #140650, #142636, #2140, #1134, #65793, #189168, #50640, #144626, #147643, #69791, #159796, #195152, #52620, #146621, #54618, #148643, #25316, #39450, #116293, #177983, #68786, #53623, #85955, #145625, #194157, #84940, #40456, #161801, #9132, #10132, #22294, #82948, #23296, #70798, #38462, #162797, #101111, #117294, #6109, #71793, #132466, #7105, #115299, #24306, #55621, #178989, #130444, #8113, #102130, #67791, #100118, #83945, #176992, #175985, #192142, #131459, #98098, #36443, #129447, #163814, #193146, #37453, #86958, #191146, #21291, #133462, #113288, #174979, #114282, #99114, #160806, #121270, #137436, #15095, #91905, #167786, #45434, #56633, #75759, #14092, #179999, #44447, #153597, #182964, #74785, #150644, #90916, #120279, #11134, #164812, #181971, #41466, #29285, #103131, #87948, #118307, #168758, #138429, #57637, #28308, #107087, #26308, #199116, #76754, #149636, #198128, #134478, #152602, #151628, #72808, #60583, #122259, #196163, #119303, #12141, #106101, #183948, #180987, #42464, #30261, #104127, #165809, #27306, #88953, #136447, #73805, #135477, #197146, #58612, #43453, #105121, #166808, #89948, #13122, #59596, #49410, #157587, #3884, #186957, #20056, #17086, #110084, #96884, #94910, #77750, #1905 ),
 ( #63585, #184938, #111073, #46423, #31259, #200110, #112074, #81700, #898, #171763, #50414, #108081, #19079, #158567, #61578, #141414, #139416, #95903, #156595, #123247, #65563, #142406, #169765, #62572, #93913, #64580, #80727, #16092, #92910, #127223, #154596, #124250, #185945, #35230, #79745, #126245, #188937, #47430, #187941, #170766, #109086, #173763, #32255, #155591, #78739, #172762, #140415, #125259, #48428, #33252, #18089, #2902, #34242, #38226, #21051, #145386, #6868, #24062, #68547, #130203, #161566, #83708, #37216, #53383, #82706, #191898, #39219, #40211, #52384, #113055, #115060, #116062, #176753, #192912, #69557, #147403, #174747, #101890, #177750, #175739, #99881, #7871, #84704, #146383, #98872, #23059, #132226, #97864, #131221, #114041, #54389, #5875, #160568, #100875, #128223, #66558, #159554, #162557, #22057, #67552, #85717, #36211, #189920, #8891, #70559, #193919, #55382, #117052, #178747, #163572, #25072, #143383, #4875, #51395, #144390, #129209, #190907, #44215, #9894, #74553, #183722, #12890, #104886, #180755, #45208, #181737, #164574, #88717, #150412, #167561, #11907, #73571, #166574, #27071, #42231, #196916, #26068, #135244, #182731, #106862, #195925, #56386, #58383, #59364, #120050, #136220, #197895, #90695, #118068, #168536, #121033, #119073, #43218, #151400, #28074, #89715, #103892, #105874, #75530, #41228, #29055, #57401, #152378, #149397, #165572, #13863, #71555, #133220, #102889, #137205, #198891, #10892, #60359, #179758, #194911, #122032, #86715, #148400, #87711, #72565, #134240, #94672, #110838, #188694, #65327, #141177, #18846, #30034, #49180, #187708, #153363, #17852, #126987, #156351, #48189, #124004, #64344, #93679, #184705, #138203, #155362, #14865, #2667, #76526, #61349, #91672, #142165, #111832, #31027, #1668, #80491, #199885, #172522, #50175, #123020, #171529, #107843, #126013, #125023, #46190, #34007, #95664, #169527, #92677, #185702, #79508, #157351, #154365, #15859, #3649, #77517, #139189, #664, #62334, #109844, #47191, #108851, #170531, #32021, #16851, #78502, #140175, #63346, #186719, #33017, #25594, #133741, #180276, #163082, #196439, #193427, #86234, #103410, #88225, #158334, #70077, #112818, #54902, #194430, #131745, #55901, #147924, #174511, #24586, #127982, #57909, #165088, #146913, #26582, #4631, #10410, #132742, #19823, #173521, #35978, #9410, #117574, #11416, #149909, #102408, #179274, #40738, #116576, #178265, #148921, #8402, #56911, #71076, #73086, #143150, #164095, #134757, #39728, #87238, #34992, #96646, #189685, #72068, #101389, #195436, #162080, #118586, #81464, #85222, #66321, #51158, #41746, #97625, #23574, #14369, #27588, #154868, #78013, #13386, #59875, #108362, #12413, #58883, #184224, #28577, #150920, #61847, #89226, #198397, #183236, #139681, #1168, #122533, #152874, #168055, #106373, #120549, #75050, #167075, #119581, #45705, #123516, #74075, #166085, #185209, #121541, #46700, #170040, #16365, #42741, #169029, #135746, #181264, #197417, #182242, #44717, #29552, #43727, #31530, #76035, #104403, #199394, #136716, #105388, #93183, #91185, #90213, #151896, #137710, #77025, #60858, #107356, #30534, #92187, #153871, #15369, #138697, #179, #141682, #49678, #155857, #17355, #140684, #4151, #48695, #2176, #64846, #126508, #143662, #188206, #111342, #80997, #3173, #156864, #173033, #63856, #34511, #158833, #159836, #172029, #32526, #96169, #35500, #157859, #112339, #189204, #66827, #94178, #21330, #97150, #95177, #19349, #127499, #65830, #50681, #18359, #142672, #51661, #79010, #174029, #33517, #20321, #125527, #80013, #81970, #47703, #186222, #187224, #5145, #128491, #110347, #190186, #113325, #109353, #175017, #36482, #98138, #82988, #144664, #62843, #124527, #171035, #164850, #41506, #117333, #195191, #6148, #25354, #163854, #129485, #194194, #103170, #132505, #24343, #100157, #40495, #69830, #160843, #114321, #131497, #191183, #179027 ) ),
 .UNSPECIFIED., .T., .F., .F. ) 
 B_SPLINE_SURFACE_WITH_KNOTS ( ( 4, 3, 4 ),
 ( 3, 2, 2, 2, 2, 2, 2, 2, 2, 2, 2, 2, 2, 2, 2, 2, 2, 2, 2, 2, 2, 2, 2, 2, 2, 2, 2, 2, 2, 2, 2, 2, 2, 2, 2, 2, 2, 2, 2, 2, 2, 2, 2, 2, 2, 2, 2, 2, 2, 2, 2, 2, 2, 2, 2, 2, 2, 2, 2, 2, 2, 2, 2, 2, 2, 2, 2, 2, 2, 2, 2, 2, 2, 2, 2, 2, 2, 2, 2, 2, 2, 2, 2, 2, 2, 2, 2, 2, 2, 2, 2, 2, 2, 2, 2, 2, 2, 2, 2, 2, 2, 2, 2, 2, 2, 2, 2, 2, 2, 2, 2, 2, 2, 2, 2, 2, 2, 2, 2, 2, 2, 2, 2, 2, 2, 2, 2, 2, 2, 2, 2, 2, 2, 2, 2, 2, 2, 2, 2, 2, 2, 2, 2, 2, 2, 2, 2, 2, 2, 2, 2, 2, 2, 2, 2, 2, 2, 2, 2, 2, 2, 2, 2, 2, 2, 2, 2, 2, 2, 2, 2, 2, 2, 2, 2, 2, 2, 2, 2, 2, 2, 2, 2, 2, 2, 2, 2, 2, 2, 2, 2, 2, 2, 2, 2, 2, 2, 2, 2, 2, 2, 2, 2, 2, 2, 2, 2, 2, 2, 2, 2, 2, 2, 2, 2, 2, 2, 2, 2, 2, 2, 2, 2, 2, 2, 2, 2, 2, 3 ),
 ( 0.000000000000000000, 0.5000000000000000000, 1.000000000000000000 ),
 ( 0.000000000000000000, 0.004385964912280701511, 0.008771929824561403022, 0.01315789473684210453, 0.01754385964912280604, 0.02192982456140350755, 0.02631578947368420907, 0.03070175438596491058, 0.03508771929824561209, 0.03947368421052631360, 0.04385964912280701511, 0.04824561403508771662, 0.05263157894736841813, 0.05701754385964911964, 0.06140350877192982115, 0.06578947368421052266, 0.07017543859649122417, 0.07456140350877192569, 0.07894736842105262720, 0.08333333333333332871, 0.08771929824561403022, 0.09210526315789473173, 0.09649122807017543324, 0.1008771929824561348, 0.1052631578947368363, 0.1096491228070175378, 0.1140350877192982393, 0.1184210526315789408, 0.1228070175438596423, 0.1271929824561403577, 0.1315789473684210453, 0.1359649122807017607, 0.1403508771929824483, 0.1447368421052631637, 0.1491228070175438514, 0.1535087719298245668, 0.1578947368421052544, 0.1622807017543859698, 0.1666666666666666574, 0.1710526315789473728, 0.1754385964912280604, 0.1798245614035087758, 0.1842105263157894635, 0.1885964912280701788, 0.1929824561403508665, 0.1973684210526315819, 0.2017543859649122695, 0.2061403508771929849, 0.2105263157894736725, 0.2149122807017543879, 0.2192982456140350755, 0.2236842105263157909, 0.2280701754385964786, 0.2324561403508771940, 0.2368421052631578816, 0.2412280701754385970, 0.2456140350877192846, 0.2500000000000000000, 0.2543859649122807154, 0.2587719298245614308, 0.2631578947368420907, 0.2675438596491228060, 0.2719298245614035214, 0.2763157894736842368, 0.2807017543859648967, 0.2850877192982456121, 0.2894736842105263275, 0.2938596491228070429, 0.2982456140350877027, 0.3026315789473684181, 0.3070175438596491335, 0.3114035087719298489, 0.3157894736842105088, 0.3201754385964912242, 0.3245614035087719396, 0.3289473684210526550, 0.3333333333333333148, 0.3377192982456140302, 0.3421052631578947456, 0.3464912280701754610, 0.3508771929824561209, 0.3552631578947368363, 0.3596491228070175517, 0.3640350877192982670, 0.3684210526315789269, 0.3728070175438596423, 0.3771929824561403577, 0.3815789473684210731, 0.3859649122807017330, 0.3903508771929824483, 0.3947368421052631637, 0.3991228070175438791, 0.4035087719298245390, 0.4078947368421052544, 0.4122807017543859698, 0.4166666666666666852, 0.4210526315789473450, 0.4254385964912280604, 0.4298245614035087758, 0.4342105263157894912, 0.4385964912280701511, 0.4429824561403508665, 0.4473684210526315819, 0.4517543859649122973, 0.4561403508771929571, 0.4605263157894736725, 0.4649122807017543879, 0.4692982456140351033, 0.4736842105263157632, 0.4780701754385964786, 0.4824561403508771940, 0.4868421052631579093, 0.4912280701754385692, 0.4956140350877192846, 0.5000000000000000000, 0.5043859649122807154, 0.5087719298245614308, 0.5131578947368421462, 0.5175438596491228616, 0.5219298245614034659, 0.5263157894736841813, 0.5307017543859648967, 0.5350877192982456121, 0.5394736842105263275, 0.5438596491228070429, 0.5482456140350877583, 0.5526315789473684736, 0.5570175438596490780, 0.5614035087719297934, 0.5657894736842105088, 0.5701754385964912242, 0.5745614035087719396, 0.5789473684210526550, 0.5833333333333333703, 0.5877192982456140857, 0.5921052631578946901, 0.5964912280701754055, 0.6008771929824561209, 0.6052631578947368363, 0.6096491228070175517, 0.6140350877192982670, 0.6184210526315789824, 0.6228070175438596978, 0.6271929824561403022, 0.6315789473684210176, 0.6359649122807017330, 0.6403508771929824483, 0.6447368421052631637, 0.6491228070175438791, 0.6535087719298245945, 0.6578947368421053099, 0.6622807017543859143, 0.6666666666666666297, 0.6710526315789473450, 0.6754385964912280604, 0.6798245614035087758, 0.6842105263157894912, 0.6885964912280702066, 0.6929824561403509220, 0.6973684210526315264, 0.7017543859649122417, 0.7061403508771929571, 0.7105263157894736725, 0.7149122807017543879, 0.7192982456140351033, 0.7236842105263158187, 0.7280701754385965341, 0.7324561403508771384, 0.7368421052631578538, 0.7412280701754385692, 0.7456140350877192846, 0.7500000000000000000, 0.7543859649122807154, 0.7587719298245614308, 0.7631578947368421462, 0.7675438596491228616, 0.7719298245614034659, 0.7763157894736841813, 0.7807017543859648967, 0.7850877192982456121, 0.7894736842105263275, 0.7938596491228070429, 0.7982456140350877583, 0.8026315789473684736, 0.8070175438596490780, 0.8114035087719297934, 0.8157894736842105088, 0.8201754385964912242, 0.8245614035087719396, 0.8289473684210526550, 0.8333333333333333703, 0.8377192982456140857, 0.8421052631578946901, 0.8464912280701754055, 0.8508771929824561209, 0.8552631578947368363, 0.8596491228070175517, 0.8640350877192982670, 0.8684210526315789824, 0.8728070175438596978, 0.8771929824561403022, 0.8815789473684210176, 0.8859649122807017330, 0.8903508771929824483, 0.8947368421052631637, 0.8991228070175438791, 0.9035087719298245945, 0.9078947368421053099, 0.9122807017543859143, 0.9166666666666666297, 0.9210526315789473450, 0.9254385964912280604, 0.9298245614035087758, 0.9342105263157894912, 0.9385964912280702066, 0.9429824561403509220, 0.9473684210526315264, 0.9517543859649122417, 0.9561403508771929571, 0.9605263157894736725, 0.9649122807017543879, 0.9692982456140351033, 0.9736842105263158187, 0.9780701754385965341, 0.9824561403508771384, 0.9868421052631578538, 0.9912280701754385692, 0.9956140350877192846, 1.000000000000000000 ),
 .UNSPECIFIED. ) 
 GEOMETRIC_REPRESENTATION_ITEM ( )  RATIONAL_B_SPLINE_SURFACE ( (
 ( 1.000000000000000000, 0.9659258262890683122, 1.000000000000000000, 0.9659258262890683122, 1.000000000000000000, 0.9659258262890683122, 1.000000000000000000, 0.9659258262890683122, 1.000000000000000000, 0.9659258262890683122, 1.000000000000000000, 0.9659258262890683122, 1.000000000000000000, 0.9659258262890683122, 1.000000000000000000, 0.9659258262890683122, 1.000000000000000000, 0.9659258262890683122, 1.000000000000000000, 0.9659258262890683122, 1.000000000000000000, 0.9659258262890683122, 1.000000000000000000, 0.9659258262890683122, 1.000000000000000000, 0.9659258262890683122, 1.000000000000000000, 0.9659258262890683122, 1.000000000000000000, 0.9659258262890683122, 1.000000000000000000, 0.9659258262890683122, 1.000000000000000000, 0.9659258262890683122, 1.000000000000000000, 0.9659258262890683122, 1.000000000000000000, 0.9659258262890683122, 1.000000000000000000, 0.9659258262890683122, 1.000000000000000000, 0.9659258262890683122, 1.000000000000000000, 0.9659258262890683122, 1.000000000000000000, 0.9659258262890683122, 1.000000000000000000, 0.9659258262890683122, 1.000000000000000000, 0.9659258262890683122, 1.000000000000000000, 0.9659258262890683122, 1.000000000000000000, 0.9659258262890683122, 1.000000000000000000, 0.9659258262890683122, 1.000000000000000000, 0.9659258262890683122, 1.000000000000000000, 0.9659258262890683122, 1.000000000000000000, 0.9659258262890683122, 1.000000000000000000, 0.9659258262890683122, 1.000000000000000000, 0.9659258262890683122, 1.000000000000000000, 0.9659258262890683122, 1.000000000000000000, 0.9659258262890683122, 1.000000000000000000, 0.9659258262890683122, 1.000000000000000000, 0.9659258262890683122, 1.000000000000000000, 0.9659258262890683122, 1.000000000000000000, 0.9659258262890683122, 1.000000000000000000, 0.9659258262890683122, 1.000000000000000000, 0.9659258262890683122, 1.000000000000000000, 0.9659258262890683122, 1.000000000000000000, 0.9659258262890683122, 1.000000000000000000, 0.9659258262890683122, 1.000000000000000000, 0.9659258262890683122, 1.000000000000000000, 0.9659258262890683122, 1.000000000000000000, 0.9659258262890683122, 1.000000000000000000, 0.9659258262890683122, 1.000000000000000000, 0.9659258262890683122, 1.000000000000000000, 0.9659258262890683122, 1.000000000000000000, 0.9659258262890683122, 1.000000000000000000, 0.9659258262890683122, 1.000000000000000000, 0.9659258262890683122, 1.000000000000000000, 0.9659258262890683122, 1.000000000000000000, 0.9659258262890683122, 1.000000000000000000, 0.9659258262890683122, 1.000000000000000000, 0.9659258262890683122, 1.000000000000000000, 0.9659258262890683122, 1.000000000000000000, 0.9659258262890683122, 1.000000000000000000, 0.9659258262890683122, 1.000000000000000000, 0.9659258262890683122, 1.000000000000000000, 0.9659258262890683122, 1.000000000000000000, 0.9659258262890683122, 1.000000000000000000, 0.9659258262890683122, 1.000000000000000000, 0.9659258262890683122, 1.000000000000000000, 0.9659258262890683122, 1.000000000000000000, 0.9659258262890683122, 1.000000000000000000, 0.9659258262890683122, 1.000000000000000000, 0.9659258262890683122, 1.000000000000000000, 0.9659258262890683122, 1.000000000000000000, 0.9659258262890683122, 1.000000000000000000, 0.9659258262890683122, 1.000000000000000000, 0.9659258262890683122, 1.000000000000000000, 0.9659258262890683122, 1.000000000000000000, 0.9659258262890683122, 1.000000000000000000, 0.9659258262890683122, 1.000000000000000000, 0.9659258262890683122, 1.000000000000000000, 0.9659258262890683122, 1.000000000000000000, 0.9659258262890683122, 1.000000000000000000, 0.9659258262890683122, 1.000000000000000000, 0.9659258262890683122, 1.000000000000000000, 0.9659258262890683122, 1.000000000000000000, 0.9659258262890683122, 1.000000000000000000, 0.9659258262890683122, 1.000000000000000000, 0.9659258262890683122, 1.000000000000000000, 0.9659258262890683122, 1.000000000000000000, 0.9659258262890683122, 1.000000000000000000, 0.9659258262890683122, 1.000000000000000000, 0.9659258262890683122, 1.000000000000000000, 0.9659258262890683122, 1.000000000000000000, 0.9659258262890683122, 1.000000000000000000, 0.9659258262890683122, 1.000000000000000000, 0.9659258262890683122, 1.000000000000000000, 0.9659258262890683122, 1.000000000000000000, 0.9659258262890683122, 1.000000000000000000, 0.9659258262890683122, 1.000000000000000000, 0.9659258262890683122, 1.000000000000000000, 0.9659258262890683122, 1.000000000000000000, 0.9659258262890683122, 1.000000000000000000, 0.9659258262890683122, 1.000000000000000000, 0.9659258262890683122, 1.000000000000000000, 0.9659258262890683122, 1.000000000000000000, 0.9659258262890683122, 1.000000000000000000, 0.9659258262890683122, 1.000000000000000000, 0.9659258262890683122, 1.000000000000000000, 0.9659258262890683122, 1.000000000000000000, 0.9659258262890683122, 1.000000000000000000, 0.9659258262890683122, 1.000000000000000000, 0.9659258262890683122, 1.000000000000000000, 0.9659258262890683122, 1.000000000000000000, 0.9659258262890683122, 1.000000000000000000, 0.9659258262890683122, 1.000000000000000000, 0.9659258262890683122, 1.000000000000000000, 0.9659258262890683122, 1.000000000000000000, 0.9659258262890683122, 1.000000000000000000, 0.9659258262890683122, 1.000000000000000000, 0.9659258262890683122, 1.000000000000000000, 0.9659258262890683122, 1.000000000000000000, 0.9659258262890683122, 1.000000000000000000, 0.9659258262890683122, 1.000000000000000000, 0.9659258262890683122, 1.000000000000000000, 0.9659258262890683122, 1.000000000000000000, 0.9659258262890683122, 1.000000000000000000, 0.9659258262890683122, 1.000000000000000000, 0.9659258262890683122, 1.000000000000000000, 0.9659258262890683122, 1.000000000000000000, 0.9659258262890683122, 1.000000000000000000, 0.9659258262890683122, 1.000000000000000000, 0.9659258262890683122, 1.000000000000000000, 0.9659258262890683122, 1.000000000000000000, 0.9659258262890683122, 1.000000000000000000, 0.9659258262890683122, 1.000000000000000000, 0.9659258262890683122, 1.000000000000000000, 0.9659258262890683122, 1.000000000000000000, 0.9659258262890683122, 1.000000000000000000, 0.9659258262890683122, 1.000000000000000000, 0.9659258262890683122, 1.000000000000000000, 0.9659258262890683122, 1.000000000000000000, 0.9659258262890683122, 1.000000000000000000, 0.9659258262890683122, 1.000000000000000000, 0.9659258262890683122, 1.000000000000000000, 0.9659258262890683122, 1.000000000000000000, 0.9659258262890683122, 1.000000000000000000, 0.9659258262890683122, 1.000000000000000000, 0.9659258262890683122, 1.000000000000000000, 0.9659258262890683122, 1.000000000000000000, 0.9659258262890683122, 1.000000000000000000, 0.9659258262890683122, 1.000000000000000000, 0.9659258262890683122, 1.000000000000000000, 0.9659258262890683122, 1.000000000000000000, 0.9659258262890683122, 1.000000000000000000, 0.9659258262890683122, 1.000000000000000000, 0.9659258262890683122, 1.000000000000000000, 0.9659258262890683122, 1.000000000000000000, 0.9659258262890683122, 1.000000000000000000, 0.9659258262890683122, 1.000000000000000000, 0.9659258262890683122, 1.000000000000000000, 0.9659258262890683122, 1.000000000000000000, 0.9659258262890683122, 1.000000000000000000, 0.9659258262890683122, 1.000000000000000000, 0.9659258262890683122, 1.000000000000000000, 0.9659258262890683122, 1.000000000000000000, 0.9659258262890683122, 1.000000000000000000, 0.9659258262890683122, 1.000000000000000000, 0.9659258262890683122, 1.000000000000000000, 0.9659258262890683122, 1.000000000000000000, 0.9659258262890683122, 1.000000000000000000, 0.9659258262890683122, 1.000000000000000000, 0.9659258262890683122, 1.000000000000000000, 0.9659258262890683122, 1.000000000000000000, 0.9659258262890683122, 1.000000000000000000, 0.9659258262890683122, 1.000000000000000000, 0.9659258262890683122, 1.000000000000000000, 0.9659258262890683122, 1.000000000000000000, 0.9659258262890683122, 1.000000000000000000, 0.9659258262890683122, 1.000000000000000000, 0.9659258262890683122, 1.000000000000000000, 0.9659258262890683122, 1.000000000000000000, 0.9659258262890683122, 1.000000000000000000, 0.9659258262890683122, 1.000000000000000000, 0.9659258262890683122, 1.000000000000000000, 0.9659258262890683122, 1.000000000000000000, 0.9659258262890683122, 1.000000000000000000, 0.9659258262890683122, 1.000000000000000000, 0.9659258262890683122, 1.000000000000000000, 0.9659258262890683122, 1.000000000000000000, 0.9659258262890683122, 1.000000000000000000, 0.9659258262890683122, 1.000000000000000000, 0.9659258262890683122, 1.000000000000000000, 0.9659258262890683122, 1.000000000000000000, 0.9659258262890683122, 1.000000000000000000, 0.9659258262890683122, 1.000000000000000000, 0.9659258262890683122, 1.000000000000000000, 0.9659258262890683122, 1.000000000000000000, 0.9659258262890683122, 1.000000000000000000, 0.9659258262890683122, 1.000000000000000000, 0.9659258262890683122, 1.000000000000000000, 0.9659258262890683122, 1.000000000000000000, 0.9659258262890683122, 1.000000000000000000, 0.9659258262890683122, 1.000000000000000000, 0.9659258262890683122, 1.000000000000000000, 0.9659258262890683122, 1.000000000000000000, 0.9659258262890683122, 1.000000000000000000, 0.9659258262890683122, 1.000000000000000000, 0.9659258262890683122, 1.000000000000000000, 0.9659258262890683122, 1.000000000000000000, 0.9659258262890683122, 1.000000000000000000, 0.9659258262890683122, 1.000000000000000000, 0.9659258262890683122, 1.000000000000000000, 0.9659258262890683122, 1.000000000000000000, 0.9659258262890683122, 1.000000000000000000, 0.9659258262890683122, 1.000000000000000000, 0.9659258262890683122, 1.000000000000000000, 0.9659258262890683122, 1.000000000000000000, 0.9659258262890683122, 1.000000000000000000, 0.9659258262890683122, 1.000000000000000000, 0.9659258262890683122, 1.000000000000000000, 0.9659258262890683122, 1.000000000000000000, 0.9659258262890683122, 1.000000000000000000, 0.9659258262890683122, 1.000000000000000000, 0.9659258262890683122, 1.000000000000000000, 0.9659258262890683122, 1.000000000000000000, 0.9659258262890683122, 1.000000000000000000, 0.9659258262890683122, 1.000000000000000000, 0.9659258262890683122, 1.000000000000000000, 0.9659258262890683122, 1.000000000000000000, 0.9659258262890683122, 1.000000000000000000, 0.9659258262890683122, 1.000000000000000000),
 ( 0.3333333333333333703, 0.3219752754296894559, 0.3333333333333333703, 0.3219752754296894559, 0.3333333333333333703, 0.3219752754296894559, 0.3333333333333333703, 0.3219752754296894559, 0.3333333333333333703, 0.3219752754296894559, 0.3333333333333333703, 0.3219752754296894559, 0.3333333333333333703, 0.3219752754296894559, 0.3333333333333333703, 0.3219752754296894559, 0.3333333333333333703, 0.3219752754296894559, 0.3333333333333333703, 0.3219752754296894559, 0.3333333333333333703, 0.3219752754296894559, 0.3333333333333333703, 0.3219752754296894559, 0.3333333333333333703, 0.3219752754296894559, 0.3333333333333333703, 0.3219752754296894559, 0.3333333333333333703, 0.3219752754296894559, 0.3333333333333333703, 0.3219752754296894559, 0.3333333333333333703, 0.3219752754296894559, 0.3333333333333333703, 0.3219752754296894559, 0.3333333333333333703, 0.3219752754296894559, 0.3333333333333333703, 0.3219752754296894559, 0.3333333333333333703, 0.3219752754296894559, 0.3333333333333333703, 0.3219752754296894559, 0.3333333333333333703, 0.3219752754296894559, 0.3333333333333333703, 0.3219752754296894559, 0.3333333333333333703, 0.3219752754296894559, 0.3333333333333333703, 0.3219752754296894559, 0.3333333333333333703, 0.3219752754296894559, 0.3333333333333333703, 0.3219752754296894559, 0.3333333333333333703, 0.3219752754296894559, 0.3333333333333333703, 0.3219752754296894559, 0.3333333333333333703, 0.3219752754296894559, 0.3333333333333333703, 0.3219752754296894559, 0.3333333333333333703, 0.3219752754296894559, 0.3333333333333333703, 0.3219752754296894559, 0.3333333333333333703, 0.3219752754296894559, 0.3333333333333333703, 0.3219752754296894559, 0.3333333333333333703, 0.3219752754296894559, 0.3333333333333333703, 0.3219752754296894559, 0.3333333333333333703, 0.3219752754296894559, 0.3333333333333333703, 0.3219752754296894559, 0.3333333333333333703, 0.3219752754296894559, 0.3333333333333333703, 0.3219752754296894559, 0.3333333333333333703, 0.3219752754296894559, 0.3333333333333333703, 0.3219752754296894559, 0.3333333333333333703, 0.3219752754296894559, 0.3333333333333333703, 0.3219752754296894559, 0.3333333333333333703, 0.3219752754296894559, 0.3333333333333333703, 0.3219752754296894559, 0.3333333333333333703, 0.3219752754296894559, 0.3333333333333333703, 0.3219752754296894559, 0.3333333333333333703, 0.3219752754296894559, 0.3333333333333333703, 0.3219752754296894559, 0.3333333333333333703, 0.3219752754296894559, 0.3333333333333333703, 0.3219752754296894559, 0.3333333333333333703, 0.3219752754296894559, 0.3333333333333333703, 0.3219752754296894559, 0.3333333333333333703, 0.3219752754296894559, 0.3333333333333333703, 0.3219752754296894559, 0.3333333333333333703, 0.3219752754296894559, 0.3333333333333333703, 0.3219752754296894559, 0.3333333333333333703, 0.3219752754296894559, 0.3333333333333333703, 0.3219752754296894559, 0.3333333333333333703, 0.3219752754296894559, 0.3333333333333333703, 0.3219752754296894559, 0.3333333333333333703, 0.3219752754296894559, 0.3333333333333333703, 0.3219752754296894559, 0.3333333333333333703, 0.3219752754296894559, 0.3333333333333333703, 0.3219752754296894559, 0.3333333333333333703, 0.3219752754296894559, 0.3333333333333333703, 0.3219752754296894559, 0.3333333333333333703, 0.3219752754296894559, 0.3333333333333333703, 0.3219752754296894559, 0.3333333333333333703, 0.3219752754296894559, 0.3333333333333333703, 0.3219752754296894559, 0.3333333333333333703, 0.3219752754296894559, 0.3333333333333333703, 0.3219752754296894559, 0.3333333333333333703, 0.3219752754296894559, 0.3333333333333333703, 0.3219752754296894559, 0.3333333333333333703, 0.3219752754296894559, 0.3333333333333333703, 0.3219752754296894559, 0.3333333333333333703, 0.3219752754296894559, 0.3333333333333333703, 0.3219752754296894559, 0.3333333333333333703, 0.3219752754296894559, 0.3333333333333333703, 0.3219752754296894559, 0.3333333333333333703, 0.3219752754296894559, 0.3333333333333333703, 0.3219752754296894559, 0.3333333333333333703, 0.3219752754296894559, 0.3333333333333333703, 0.3219752754296894559, 0.3333333333333333703, 0.3219752754296894559, 0.3333333333333333703, 0.3219752754296894559, 0.3333333333333333703, 0.3219752754296894559, 0.3333333333333333703, 0.3219752754296894559, 0.3333333333333333703, 0.3219752754296894559, 0.3333333333333333703, 0.3219752754296894559, 0.3333333333333333703, 0.3219752754296894559, 0.3333333333333333703, 0.3219752754296894559, 0.3333333333333333703, 0.3219752754296894559, 0.3333333333333333703, 0.3219752754296894559, 0.3333333333333333703, 0.3219752754296894559, 0.3333333333333333703, 0.3219752754296894559, 0.3333333333333333703, 0.3219752754296894559, 0.3333333333333333703, 0.3219752754296894559, 0.3333333333333333703, 0.3219752754296894559, 0.3333333333333333703, 0.3219752754296894559, 0.3333333333333333703, 0.3219752754296894559, 0.3333333333333333703, 0.3219752754296894559, 0.3333333333333333703, 0.3219752754296894559, 0.3333333333333333703, 0.3219752754296894559, 0.3333333333333333703, 0.3219752754296894559, 0.3333333333333333703, 0.3219752754296894559, 0.3333333333333333703, 0.3219752754296894559, 0.3333333333333333703, 0.3219752754296894559, 0.3333333333333333703, 0.3219752754296894559, 0.3333333333333333703, 0.3219752754296894559, 0.3333333333333333703, 0.3219752754296894559, 0.3333333333333333703, 0.3219752754296894559, 0.3333333333333333703, 0.3219752754296894559, 0.3333333333333333703, 0.3219752754296894559, 0.3333333333333333703, 0.3219752754296894559, 0.3333333333333333703, 0.3219752754296894559, 0.3333333333333333703, 0.3219752754296894559, 0.3333333333333333703, 0.3219752754296894559, 0.3333333333333333703, 0.3219752754296894559, 0.3333333333333333703, 0.3219752754296894559, 0.3333333333333333703, 0.3219752754296894559, 0.3333333333333333703, 0.3219752754296894559, 0.3333333333333333703, 0.3219752754296894559, 0.3333333333333333703, 0.3219752754296894559, 0.3333333333333333703, 0.3219752754296894559, 0.3333333333333333703, 0.3219752754296894559, 0.3333333333333333703, 0.3219752754296894559, 0.3333333333333333703, 0.3219752754296894559, 0.3333333333333333703, 0.3219752754296894559, 0.3333333333333333703, 0.3219752754296894559, 0.3333333333333333703, 0.3219752754296894559, 0.3333333333333333703, 0.3219752754296894559, 0.3333333333333333703, 0.3219752754296894559, 0.3333333333333333703, 0.3219752754296894559, 0.3333333333333333703, 0.3219752754296894559, 0.3333333333333333703, 0.3219752754296894559, 0.3333333333333333703, 0.3219752754296894559, 0.3333333333333333703, 0.3219752754296894559, 0.3333333333333333703, 0.3219752754296894559, 0.3333333333333333703, 0.3219752754296894559, 0.3333333333333333703, 0.3219752754296894559, 0.3333333333333333703, 0.3219752754296894559, 0.3333333333333333703, 0.3219752754296894559, 0.3333333333333333703, 0.3219752754296894559, 0.3333333333333333703, 0.3219752754296894559, 0.3333333333333333703, 0.3219752754296894559, 0.3333333333333333703, 0.3219752754296894559, 0.3333333333333333703, 0.3219752754296894559, 0.3333333333333333703, 0.3219752754296894559, 0.3333333333333333703, 0.3219752754296894559, 0.3333333333333333703, 0.3219752754296894559, 0.3333333333333333703, 0.3219752754296894559, 0.3333333333333333703, 0.3219752754296894559, 0.3333333333333333703, 0.3219752754296894559, 0.3333333333333333703, 0.3219752754296894559, 0.3333333333333333703, 0.3219752754296894559, 0.3333333333333333703, 0.3219752754296894559, 0.3333333333333333703, 0.3219752754296894559, 0.3333333333333333703, 0.3219752754296894559, 0.3333333333333333703, 0.3219752754296894559, 0.3333333333333333703, 0.3219752754296894559, 0.3333333333333333703, 0.3219752754296894559, 0.3333333333333333703, 0.3219752754296894559, 0.3333333333333333703, 0.3219752754296894559, 0.3333333333333333703, 0.3219752754296894559, 0.3333333333333333703, 0.3219752754296894559, 0.3333333333333333703, 0.3219752754296894559, 0.3333333333333333703, 0.3219752754296894559, 0.3333333333333333703, 0.3219752754296894559, 0.3333333333333333703, 0.3219752754296894559, 0.3333333333333333703, 0.3219752754296894559, 0.3333333333333333703, 0.3219752754296894559, 0.3333333333333333703, 0.3219752754296894559, 0.3333333333333333703, 0.3219752754296894559, 0.3333333333333333703, 0.3219752754296894559, 0.3333333333333333703, 0.3219752754296894559, 0.3333333333333333703, 0.3219752754296894559, 0.3333333333333333703, 0.3219752754296894559, 0.3333333333333333703, 0.3219752754296894559, 0.3333333333333333703, 0.3219752754296894559, 0.3333333333333333703, 0.3219752754296894559, 0.3333333333333333703, 0.3219752754296894559, 0.3333333333333333703, 0.3219752754296894559, 0.3333333333333333703, 0.3219752754296894559, 0.3333333333333333703, 0.3219752754296894559, 0.3333333333333333703, 0.3219752754296894559, 0.3333333333333333703, 0.3219752754296894559, 0.3333333333333333703, 0.3219752754296894559, 0.3333333333333333703, 0.3219752754296894559, 0.3333333333333333703, 0.3219752754296894559, 0.3333333333333333703, 0.3219752754296894559, 0.3333333333333333703, 0.3219752754296894559, 0.3333333333333333703, 0.3219752754296894559, 0.3333333333333333703, 0.3219752754296894559, 0.3333333333333333703, 0.3219752754296894559, 0.3333333333333333703, 0.3219752754296894559, 0.3333333333333333703, 0.3219752754296894559, 0.3333333333333333703, 0.3219752754296894559, 0.3333333333333333703, 0.3219752754296894559, 0.3333333333333333703, 0.3219752754296894559, 0.3333333333333333703, 0.3219752754296894559, 0.3333333333333333703, 0.3219752754296894559, 0.3333333333333333703, 0.3219752754296894559, 0.3333333333333333703, 0.3219752754296894559, 0.3333333333333333703, 0.3219752754296894559, 0.3333333333333333703, 0.3219752754296894559, 0.3333333333333333703, 0.3219752754296894559, 0.3333333333333333703, 0.3219752754296894559, 0.3333333333333333703, 0.3219752754296894559, 0.3333333333333333703, 0.3219752754296894559, 0.3333333333333333703, 0.3219752754296894559, 0.3333333333333333703, 0.3219752754296894559, 0.3333333333333333703, 0.3219752754296894559, 0.3333333333333333703, 0.3219752754296894559, 0.3333333333333333703, 0.3219752754296894559, 0.3333333333333333703, 0.3219752754296894559, 0.3333333333333333703, 0.3219752754296894559, 0.3333333333333333703, 0.3219752754296894559, 0.3333333333333333703, 0.3219752754296894559, 0.3333333333333333703, 0.3219752754296894559, 0.3333333333333333703, 0.3219752754296894559, 0.3333333333333333703, 0.3219752754296894559, 0.3333333333333333703, 0.3219752754296894559, 0.3333333333333333703, 0.3219752754296894559, 0.3333333333333333703),
 ( 0.3333333333333333703, 0.3219752754296894559, 0.3333333333333333703, 0.3219752754296894559, 0.3333333333333333703, 0.3219752754296894559, 0.3333333333333333703, 0.3219752754296894559, 0.3333333333333333703, 0.3219752754296894559, 0.3333333333333333703, 0.3219752754296894559, 0.3333333333333333703, 0.3219752754296894559, 0.3333333333333333703, 0.3219752754296894559, 0.3333333333333333703, 0.3219752754296894559, 0.3333333333333333703, 0.3219752754296894559, 0.3333333333333333703, 0.3219752754296894559, 0.3333333333333333703, 0.3219752754296894559, 0.3333333333333333703, 0.3219752754296894559, 0.3333333333333333703, 0.3219752754296894559, 0.3333333333333333703, 0.3219752754296894559, 0.3333333333333333703, 0.3219752754296894559, 0.3333333333333333703, 0.3219752754296894559, 0.3333333333333333703, 0.3219752754296894559, 0.3333333333333333703, 0.3219752754296894559, 0.3333333333333333703, 0.3219752754296894559, 0.3333333333333333703, 0.3219752754296894559, 0.3333333333333333703, 0.3219752754296894559, 0.3333333333333333703, 0.3219752754296894559, 0.3333333333333333703, 0.3219752754296894559, 0.3333333333333333703, 0.3219752754296894559, 0.3333333333333333703, 0.3219752754296894559, 0.3333333333333333703, 0.3219752754296894559, 0.3333333333333333703, 0.3219752754296894559, 0.3333333333333333703, 0.3219752754296894559, 0.3333333333333333703, 0.3219752754296894559, 0.3333333333333333703, 0.3219752754296894559, 0.3333333333333333703, 0.3219752754296894559, 0.3333333333333333703, 0.3219752754296894559, 0.3333333333333333703, 0.3219752754296894559, 0.3333333333333333703, 0.3219752754296894559, 0.3333333333333333703, 0.3219752754296894559, 0.3333333333333333703, 0.3219752754296894559, 0.3333333333333333703, 0.3219752754296894559, 0.3333333333333333703, 0.3219752754296894559, 0.3333333333333333703, 0.3219752754296894559, 0.3333333333333333703, 0.3219752754296894559, 0.3333333333333333703, 0.3219752754296894559, 0.3333333333333333703, 0.3219752754296894559, 0.3333333333333333703, 0.3219752754296894559, 0.3333333333333333703, 0.3219752754296894559, 0.3333333333333333703, 0.3219752754296894559, 0.3333333333333333703, 0.3219752754296894559, 0.3333333333333333703, 0.3219752754296894559, 0.3333333333333333703, 0.3219752754296894559, 0.3333333333333333703, 0.3219752754296894559, 0.3333333333333333703, 0.3219752754296894559, 0.3333333333333333703, 0.3219752754296894559, 0.3333333333333333703, 0.3219752754296894559, 0.3333333333333333703, 0.3219752754296894559, 0.3333333333333333703, 0.3219752754296894559, 0.3333333333333333703, 0.3219752754296894559, 0.3333333333333333703, 0.3219752754296894559, 0.3333333333333333703, 0.3219752754296894559, 0.3333333333333333703, 0.3219752754296894559, 0.3333333333333333703, 0.3219752754296894559, 0.3333333333333333703, 0.3219752754296894559, 0.3333333333333333703, 0.3219752754296894559, 0.3333333333333333703, 0.3219752754296894559, 0.3333333333333333703, 0.3219752754296894559, 0.3333333333333333703, 0.3219752754296894559, 0.3333333333333333703, 0.3219752754296894559, 0.3333333333333333703, 0.3219752754296894559, 0.3333333333333333703, 0.3219752754296894559, 0.3333333333333333703, 0.3219752754296894559, 0.3333333333333333703, 0.3219752754296894559, 0.3333333333333333703, 0.3219752754296894559, 0.3333333333333333703, 0.3219752754296894559, 0.3333333333333333703, 0.3219752754296894559, 0.3333333333333333703, 0.3219752754296894559, 0.3333333333333333703, 0.3219752754296894559, 0.3333333333333333703, 0.3219752754296894559, 0.3333333333333333703, 0.3219752754296894559, 0.3333333333333333703, 0.3219752754296894559, 0.3333333333333333703, 0.3219752754296894559, 0.3333333333333333703, 0.3219752754296894559, 0.3333333333333333703, 0.3219752754296894559, 0.3333333333333333703, 0.3219752754296894559, 0.3333333333333333703, 0.3219752754296894559, 0.3333333333333333703, 0.3219752754296894559, 0.3333333333333333703, 0.3219752754296894559, 0.3333333333333333703, 0.3219752754296894559, 0.3333333333333333703, 0.3219752754296894559, 0.3333333333333333703, 0.3219752754296894559, 0.3333333333333333703, 0.3219752754296894559, 0.3333333333333333703, 0.3219752754296894559, 0.3333333333333333703, 0.3219752754296894559, 0.3333333333333333703, 0.3219752754296894559, 0.3333333333333333703, 0.3219752754296894559, 0.3333333333333333703, 0.3219752754296894559, 0.3333333333333333703, 0.3219752754296894559, 0.3333333333333333703, 0.3219752754296894559, 0.3333333333333333703, 0.3219752754296894559, 0.3333333333333333703, 0.3219752754296894559, 0.3333333333333333703, 0.3219752754296894559, 0.3333333333333333703, 0.3219752754296894559, 0.3333333333333333703, 0.3219752754296894559, 0.3333333333333333703, 0.3219752754296894559, 0.3333333333333333703, 0.3219752754296894559, 0.3333333333333333703, 0.3219752754296894559, 0.3333333333333333703, 0.3219752754296894559, 0.3333333333333333703, 0.3219752754296894559, 0.3333333333333333703, 0.3219752754296894559, 0.3333333333333333703, 0.3219752754296894559, 0.3333333333333333703, 0.3219752754296894559, 0.3333333333333333703, 0.3219752754296894559, 0.3333333333333333703, 0.3219752754296894559, 0.3333333333333333703, 0.3219752754296894559, 0.3333333333333333703, 0.3219752754296894559, 0.3333333333333333703, 0.3219752754296894559, 0.3333333333333333703, 0.3219752754296894559, 0.3333333333333333703, 0.3219752754296894559, 0.3333333333333333703, 0.3219752754296894559, 0.3333333333333333703, 0.3219752754296894559, 0.3333333333333333703, 0.3219752754296894559, 0.3333333333333333703, 0.3219752754296894559, 0.3333333333333333703, 0.3219752754296894559, 0.3333333333333333703, 0.3219752754296894559, 0.3333333333333333703, 0.3219752754296894559, 0.3333333333333333703, 0.3219752754296894559, 0.3333333333333333703, 0.3219752754296894559, 0.3333333333333333703, 0.3219752754296894559, 0.3333333333333333703, 0.3219752754296894559, 0.3333333333333333703, 0.3219752754296894559, 0.3333333333333333703, 0.3219752754296894559, 0.3333333333333333703, 0.3219752754296894559, 0.3333333333333333703, 0.3219752754296894559, 0.3333333333333333703, 0.3219752754296894559, 0.3333333333333333703, 0.3219752754296894559, 0.3333333333333333703, 0.3219752754296894559, 0.3333333333333333703, 0.3219752754296894559, 0.3333333333333333703, 0.3219752754296894559, 0.3333333333333333703, 0.3219752754296894559, 0.3333333333333333703, 0.3219752754296894559, 0.3333333333333333703, 0.3219752754296894559, 0.3333333333333333703, 0.3219752754296894559, 0.3333333333333333703, 0.3219752754296894559, 0.3333333333333333703, 0.3219752754296894559, 0.3333333333333333703, 0.3219752754296894559, 0.3333333333333333703, 0.3219752754296894559, 0.3333333333333333703, 0.3219752754296894559, 0.3333333333333333703, 0.3219752754296894559, 0.3333333333333333703, 0.3219752754296894559, 0.3333333333333333703, 0.3219752754296894559, 0.3333333333333333703, 0.3219752754296894559, 0.3333333333333333703, 0.3219752754296894559, 0.3333333333333333703, 0.3219752754296894559, 0.3333333333333333703, 0.3219752754296894559, 0.3333333333333333703, 0.3219752754296894559, 0.3333333333333333703, 0.3219752754296894559, 0.3333333333333333703, 0.3219752754296894559, 0.3333333333333333703, 0.3219752754296894559, 0.3333333333333333703, 0.3219752754296894559, 0.3333333333333333703, 0.3219752754296894559, 0.3333333333333333703, 0.3219752754296894559, 0.3333333333333333703, 0.3219752754296894559, 0.3333333333333333703, 0.3219752754296894559, 0.3333333333333333703, 0.3219752754296894559, 0.3333333333333333703, 0.3219752754296894559, 0.3333333333333333703, 0.3219752754296894559, 0.3333333333333333703, 0.3219752754296894559, 0.3333333333333333703, 0.3219752754296894559, 0.3333333333333333703, 0.3219752754296894559, 0.3333333333333333703, 0.3219752754296894559, 0.3333333333333333703, 0.3219752754296894559, 0.3333333333333333703, 0.3219752754296894559, 0.3333333333333333703, 0.3219752754296894559, 0.3333333333333333703, 0.3219752754296894559, 0.3333333333333333703, 0.3219752754296894559, 0.3333333333333333703, 0.3219752754296894559, 0.3333333333333333703, 0.3219752754296894559, 0.3333333333333333703, 0.3219752754296894559, 0.3333333333333333703, 0.3219752754296894559, 0.3333333333333333703, 0.3219752754296894559, 0.3333333333333333703, 0.3219752754296894559, 0.3333333333333333703, 0.3219752754296894559, 0.3333333333333333703, 0.3219752754296894559, 0.3333333333333333703, 0.3219752754296894559, 0.3333333333333333703, 0.3219752754296894559, 0.3333333333333333703, 0.3219752754296894559, 0.3333333333333333703, 0.3219752754296894559, 0.3333333333333333703, 0.3219752754296894559, 0.3333333333333333703, 0.3219752754296894559, 0.3333333333333333703, 0.3219752754296894559, 0.3333333333333333703, 0.3219752754296894559, 0.3333333333333333703, 0.3219752754296894559, 0.3333333333333333703, 0.3219752754296894559, 0.3333333333333333703, 0.3219752754296894559, 0.3333333333333333703, 0.3219752754296894559, 0.3333333333333333703, 0.3219752754296894559, 0.3333333333333333703, 0.3219752754296894559, 0.3333333333333333703, 0.3219752754296894559, 0.3333333333333333703, 0.3219752754296894559, 0.3333333333333333703, 0.3219752754296894559, 0.3333333333333333703, 0.3219752754296894559, 0.3333333333333333703, 0.3219752754296894559, 0.3333333333333333703, 0.3219752754296894559, 0.3333333333333333703, 0.3219752754296894559, 0.3333333333333333703, 0.3219752754296894559, 0.3333333333333333703, 0.3219752754296894559, 0.3333333333333333703, 0.3219752754296894559, 0.3333333333333333703, 0.3219752754296894559, 0.3333333333333333703, 0.3219752754296894559, 0.3333333333333333703, 0.3219752754296894559, 0.3333333333333333703, 0.3219752754296894559, 0.3333333333333333703, 0.3219752754296894559, 0.3333333333333333703, 0.3219752754296894559, 0.3333333333333333703, 0.3219752754296894559, 0.3333333333333333703, 0.3219752754296894559, 0.3333333333333333703, 0.3219752754296894559, 0.3333333333333333703, 0.3219752754296894559, 0.3333333333333333703, 0.3219752754296894559, 0.3333333333333333703, 0.3219752754296894559, 0.3333333333333333703, 0.3219752754296894559, 0.3333333333333333703, 0.3219752754296894559, 0.3333333333333333703, 0.3219752754296894559, 0.3333333333333333703, 0.3219752754296894559, 0.3333333333333333703, 0.3219752754296894559, 0.3333333333333333703, 0.3219752754296894559, 0.3333333333333333703, 0.3219752754296894559, 0.3333333333333333703, 0.3219752754296894559, 0.3333333333333333703, 0.3219752754296894559, 0.3333333333333333703, 0.3219752754296894559, 0.3333333333333333703, 0.3219752754296894559, 0.3333333333333333703),
 ( 1.000000000000000000, 0.9659258262890683122, 1.000000000000000000, 0.9659258262890683122, 1.000000000000000000, 0.9659258262890683122, 1.000000000000000000, 0.9659258262890683122, 1.000000000000000000, 0.9659258262890683122, 1.000000000000000000, 0.9659258262890683122, 1.000000000000000000, 0.9659258262890683122, 1.000000000000000000, 0.9659258262890683122, 1.000000000000000000, 0.9659258262890683122, 1.000000000000000000, 0.9659258262890683122, 1.000000000000000000, 0.9659258262890683122, 1.000000000000000000, 0.9659258262890683122, 1.000000000000000000, 0.9659258262890683122, 1.000000000000000000, 0.9659258262890683122, 1.000000000000000000, 0.9659258262890683122, 1.000000000000000000, 0.9659258262890683122, 1.000000000000000000, 0.9659258262890683122, 1.000000000000000000, 0.9659258262890683122, 1.000000000000000000, 0.9659258262890683122, 1.000000000000000000, 0.9659258262890683122, 1.000000000000000000, 0.9659258262890683122, 1.000000000000000000, 0.9659258262890683122, 1.000000000000000000, 0.9659258262890683122, 1.000000000000000000, 0.9659258262890683122, 1.000000000000000000, 0.9659258262890683122, 1.000000000000000000, 0.9659258262890683122, 1.000000000000000000, 0.9659258262890683122, 1.000000000000000000, 0.9659258262890683122, 1.000000000000000000, 0.9659258262890683122, 1.000000000000000000, 0.9659258262890683122, 1.000000000000000000, 0.9659258262890683122, 1.000000000000000000, 0.9659258262890683122, 1.000000000000000000, 0.9659258262890683122, 1.000000000000000000, 0.9659258262890683122, 1.000000000000000000, 0.9659258262890683122, 1.000000000000000000, 0.9659258262890683122, 1.000000000000000000, 0.9659258262890683122, 1.000000000000000000, 0.9659258262890683122, 1.000000000000000000, 0.9659258262890683122, 1.000000000000000000, 0.9659258262890683122, 1.000000000000000000, 0.9659258262890683122, 1.000000000000000000, 0.9659258262890683122, 1.000000000000000000, 0.9659258262890683122, 1.000000000000000000, 0.9659258262890683122, 1.000000000000000000, 0.9659258262890683122, 1.000000000000000000, 0.9659258262890683122, 1.000000000000000000, 0.9659258262890683122, 1.000000000000000000, 0.9659258262890683122, 1.000000000000000000, 0.9659258262890683122, 1.000000000000000000, 0.9659258262890683122, 1.000000000000000000, 0.9659258262890683122, 1.000000000000000000, 0.9659258262890683122, 1.000000000000000000, 0.9659258262890683122, 1.000000000000000000, 0.9659258262890683122, 1.000000000000000000, 0.9659258262890683122, 1.000000000000000000, 0.9659258262890683122, 1.000000000000000000, 0.9659258262890683122, 1.000000000000000000, 0.9659258262890683122, 1.000000000000000000, 0.9659258262890683122, 1.000000000000000000, 0.9659258262890683122, 1.000000000000000000, 0.9659258262890683122, 1.000000000000000000, 0.9659258262890683122, 1.000000000000000000, 0.9659258262890683122, 1.000000000000000000, 0.9659258262890683122, 1.000000000000000000, 0.9659258262890683122, 1.000000000000000000, 0.9659258262890683122, 1.000000000000000000, 0.9659258262890683122, 1.000000000000000000, 0.9659258262890683122, 1.000000000000000000, 0.9659258262890683122, 1.000000000000000000, 0.9659258262890683122, 1.000000000000000000, 0.9659258262890683122, 1.000000000000000000, 0.9659258262890683122, 1.000000000000000000, 0.9659258262890683122, 1.000000000000000000, 0.9659258262890683122, 1.000000000000000000, 0.9659258262890683122, 1.000000000000000000, 0.9659258262890683122, 1.000000000000000000, 0.9659258262890683122, 1.000000000000000000, 0.9659258262890683122, 1.000000000000000000, 0.9659258262890683122, 1.000000000000000000, 0.9659258262890683122, 1.000000000000000000, 0.9659258262890683122, 1.000000000000000000, 0.9659258262890683122, 1.000000000000000000, 0.9659258262890683122, 1.000000000000000000, 0.9659258262890683122, 1.000000000000000000, 0.9659258262890683122, 1.000000000000000000, 0.9659258262890683122, 1.000000000000000000, 0.9659258262890683122, 1.000000000000000000, 0.9659258262890683122, 1.000000000000000000, 0.9659258262890683122, 1.000000000000000000, 0.9659258262890683122, 1.000000000000000000, 0.9659258262890683122, 1.000000000000000000, 0.9659258262890683122, 1.000000000000000000, 0.9659258262890683122, 1.000000000000000000, 0.9659258262890683122, 1.000000000000000000, 0.9659258262890683122, 1.000000000000000000, 0.9659258262890683122, 1.000000000000000000, 0.9659258262890683122, 1.000000000000000000, 0.9659258262890683122, 1.000000000000000000, 0.9659258262890683122, 1.000000000000000000, 0.9659258262890683122, 1.000000000000000000, 0.9659258262890683122, 1.000000000000000000, 0.9659258262890683122, 1.000000000000000000, 0.9659258262890683122, 1.000000000000000000, 0.9659258262890683122, 1.000000000000000000, 0.9659258262890683122, 1.000000000000000000, 0.9659258262890683122, 1.000000000000000000, 0.9659258262890683122, 1.000000000000000000, 0.9659258262890683122, 1.000000000000000000, 0.9659258262890683122, 1.000000000000000000, 0.9659258262890683122, 1.000000000000000000, 0.9659258262890683122, 1.000000000000000000, 0.9659258262890683122, 1.000000000000000000, 0.9659258262890683122, 1.000000000000000000, 0.9659258262890683122, 1.000000000000000000, 0.9659258262890683122, 1.000000000000000000, 0.9659258262890683122, 1.000000000000000000, 0.9659258262890683122, 1.000000000000000000, 0.9659258262890683122, 1.000000000000000000, 0.9659258262890683122, 1.000000000000000000, 0.9659258262890683122, 1.000000000000000000, 0.9659258262890683122, 1.000000000000000000, 0.9659258262890683122, 1.000000000000000000, 0.9659258262890683122, 1.000000000000000000, 0.9659258262890683122, 1.000000000000000000, 0.9659258262890683122, 1.000000000000000000, 0.9659258262890683122, 1.000000000000000000, 0.9659258262890683122, 1.000000000000000000, 0.9659258262890683122, 1.000000000000000000, 0.9659258262890683122, 1.000000000000000000, 0.9659258262890683122, 1.000000000000000000, 0.9659258262890683122, 1.000000000000000000, 0.9659258262890683122, 1.000000000000000000, 0.9659258262890683122, 1.000000000000000000, 0.9659258262890683122, 1.000000000000000000, 0.9659258262890683122, 1.000000000000000000, 0.9659258262890683122, 1.000000000000000000, 0.9659258262890683122, 1.000000000000000000, 0.9659258262890683122, 1.000000000000000000, 0.9659258262890683122, 1.000000000000000000, 0.9659258262890683122, 1.000000000000000000, 0.9659258262890683122, 1.000000000000000000, 0.9659258262890683122, 1.000000000000000000, 0.9659258262890683122, 1.000000000000000000, 0.9659258262890683122, 1.000000000000000000, 0.9659258262890683122, 1.000000000000000000, 0.9659258262890683122, 1.000000000000000000, 0.9659258262890683122, 1.000000000000000000, 0.9659258262890683122, 1.000000000000000000, 0.9659258262890683122, 1.000000000000000000, 0.9659258262890683122, 1.000000000000000000, 0.9659258262890683122, 1.000000000000000000, 0.9659258262890683122, 1.000000000000000000, 0.9659258262890683122, 1.000000000000000000, 0.9659258262890683122, 1.000000000000000000, 0.9659258262890683122, 1.000000000000000000, 0.9659258262890683122, 1.000000000000000000, 0.9659258262890683122, 1.000000000000000000, 0.9659258262890683122, 1.000000000000000000, 0.9659258262890683122, 1.000000000000000000, 0.9659258262890683122, 1.000000000000000000, 0.9659258262890683122, 1.000000000000000000, 0.9659258262890683122, 1.000000000000000000, 0.9659258262890683122, 1.000000000000000000, 0.9659258262890683122, 1.000000000000000000, 0.9659258262890683122, 1.000000000000000000, 0.9659258262890683122, 1.000000000000000000, 0.9659258262890683122, 1.000000000000000000, 0.9659258262890683122, 1.000000000000000000, 0.9659258262890683122, 1.000000000000000000, 0.9659258262890683122, 1.000000000000000000, 0.9659258262890683122, 1.000000000000000000, 0.9659258262890683122, 1.000000000000000000, 0.9659258262890683122, 1.000000000000000000, 0.9659258262890683122, 1.000000000000000000, 0.9659258262890683122, 1.000000000000000000, 0.9659258262890683122, 1.000000000000000000, 0.9659258262890683122, 1.000000000000000000, 0.9659258262890683122, 1.000000000000000000, 0.9659258262890683122, 1.000000000000000000, 0.9659258262890683122, 1.000000000000000000, 0.9659258262890683122, 1.000000000000000000, 0.9659258262890683122, 1.000000000000000000, 0.9659258262890683122, 1.000000000000000000, 0.9659258262890683122, 1.000000000000000000, 0.9659258262890683122, 1.000000000000000000, 0.9659258262890683122, 1.000000000000000000, 0.9659258262890683122, 1.000000000000000000, 0.9659258262890683122, 1.000000000000000000, 0.9659258262890683122, 1.000000000000000000, 0.9659258262890683122, 1.000000000000000000, 0.9659258262890683122, 1.000000000000000000, 0.9659258262890683122, 1.000000000000000000, 0.9659258262890683122, 1.000000000000000000, 0.9659258262890683122, 1.000000000000000000, 0.9659258262890683122, 1.000000000000000000, 0.9659258262890683122, 1.000000000000000000, 0.9659258262890683122, 1.000000000000000000, 0.9659258262890683122, 1.000000000000000000, 0.9659258262890683122, 1.000000000000000000, 0.9659258262890683122, 1.000000000000000000, 0.9659258262890683122, 1.000000000000000000, 0.9659258262890683122, 1.000000000000000000, 0.9659258262890683122, 1.000000000000000000, 0.9659258262890683122, 1.000000000000000000, 0.9659258262890683122, 1.000000000000000000, 0.9659258262890683122, 1.000000000000000000, 0.9659258262890683122, 1.000000000000000000, 0.9659258262890683122, 1.000000000000000000, 0.9659258262890683122, 1.000000000000000000, 0.9659258262890683122, 1.000000000000000000, 0.9659258262890683122, 1.000000000000000000, 0.9659258262890683122, 1.000000000000000000, 0.9659258262890683122, 1.000000000000000000, 0.9659258262890683122, 1.000000000000000000, 0.9659258262890683122, 1.000000000000000000, 0.9659258262890683122, 1.000000000000000000, 0.9659258262890683122, 1.000000000000000000, 0.9659258262890683122, 1.000000000000000000, 0.9659258262890683122, 1.000000000000000000, 0.9659258262890683122, 1.000000000000000000, 0.9659258262890683122, 1.000000000000000000, 0.9659258262890683122, 1.000000000000000000, 0.9659258262890683122, 1.000000000000000000, 0.9659258262890683122, 1.000000000000000000, 0.9659258262890683122, 1.000000000000000000, 0.9659258262890683122, 1.000000000000000000, 0.9659258262890683122, 1.000000000000000000, 0.9659258262890683122, 1.000000000000000000),
 ( 0.3333333333333333703, 0.3219752754296894559, 0.3333333333333333703, 0.3219752754296894559, 0.3333333333333333703, 0.3219752754296894559, 0.3333333333333333703, 0.3219752754296894559, 0.3333333333333333703, 0.3219752754296894559, 0.3333333333333333703, 0.3219752754296894559, 0.3333333333333333703, 0.3219752754296894559, 0.3333333333333333703, 0.3219752754296894559, 0.3333333333333333703, 0.3219752754296894559, 0.3333333333333333703, 0.3219752754296894559, 0.3333333333333333703, 0.3219752754296894559, 0.3333333333333333703, 0.3219752754296894559, 0.3333333333333333703, 0.3219752754296894559, 0.3333333333333333703, 0.3219752754296894559, 0.3333333333333333703, 0.3219752754296894559, 0.3333333333333333703, 0.3219752754296894559, 0.3333333333333333703, 0.3219752754296894559, 0.3333333333333333703, 0.3219752754296894559, 0.3333333333333333703, 0.3219752754296894559, 0.3333333333333333703, 0.3219752754296894559, 0.3333333333333333703, 0.3219752754296894559, 0.3333333333333333703, 0.3219752754296894559, 0.3333333333333333703, 0.3219752754296894559, 0.3333333333333333703, 0.3219752754296894559, 0.3333333333333333703, 0.3219752754296894559, 0.3333333333333333703, 0.3219752754296894559, 0.3333333333333333703, 0.3219752754296894559, 0.3333333333333333703, 0.3219752754296894559, 0.3333333333333333703, 0.3219752754296894559, 0.3333333333333333703, 0.3219752754296894559, 0.3333333333333333703, 0.3219752754296894559, 0.3333333333333333703, 0.3219752754296894559, 0.3333333333333333703, 0.3219752754296894559, 0.3333333333333333703, 0.3219752754296894559, 0.3333333333333333703, 0.3219752754296894559, 0.3333333333333333703, 0.3219752754296894559, 0.3333333333333333703, 0.3219752754296894559, 0.3333333333333333703, 0.3219752754296894559, 0.3333333333333333703, 0.3219752754296894559, 0.3333333333333333703, 0.3219752754296894559, 0.3333333333333333703, 0.3219752754296894559, 0.3333333333333333703, 0.3219752754296894559, 0.3333333333333333703, 0.3219752754296894559, 0.3333333333333333703, 0.3219752754296894559, 0.3333333333333333703, 0.3219752754296894559, 0.3333333333333333703, 0.3219752754296894559, 0.3333333333333333703, 0.3219752754296894559, 0.3333333333333333703, 0.3219752754296894559, 0.3333333333333333703, 0.3219752754296894559, 0.3333333333333333703, 0.3219752754296894559, 0.3333333333333333703, 0.3219752754296894559, 0.3333333333333333703, 0.3219752754296894559, 0.3333333333333333703, 0.3219752754296894559, 0.3333333333333333703, 0.3219752754296894559, 0.3333333333333333703, 0.3219752754296894559, 0.3333333333333333703, 0.3219752754296894559, 0.3333333333333333703, 0.3219752754296894559, 0.3333333333333333703, 0.3219752754296894559, 0.3333333333333333703, 0.3219752754296894559, 0.3333333333333333703, 0.3219752754296894559, 0.3333333333333333703, 0.3219752754296894559, 0.3333333333333333703, 0.3219752754296894559, 0.3333333333333333703, 0.3219752754296894559, 0.3333333333333333703, 0.3219752754296894559, 0.3333333333333333703, 0.3219752754296894559, 0.3333333333333333703, 0.3219752754296894559, 0.3333333333333333703, 0.3219752754296894559, 0.3333333333333333703, 0.3219752754296894559, 0.3333333333333333703, 0.3219752754296894559, 0.3333333333333333703, 0.3219752754296894559, 0.3333333333333333703, 0.3219752754296894559, 0.3333333333333333703, 0.3219752754296894559, 0.3333333333333333703, 0.3219752754296894559, 0.3333333333333333703, 0.3219752754296894559, 0.3333333333333333703, 0.3219752754296894559, 0.3333333333333333703, 0.3219752754296894559, 0.3333333333333333703, 0.3219752754296894559, 0.3333333333333333703, 0.3219752754296894559, 0.3333333333333333703, 0.3219752754296894559, 0.3333333333333333703, 0.3219752754296894559, 0.3333333333333333703, 0.3219752754296894559, 0.3333333333333333703, 0.3219752754296894559, 0.3333333333333333703, 0.3219752754296894559, 0.3333333333333333703, 0.3219752754296894559, 0.3333333333333333703, 0.3219752754296894559, 0.3333333333333333703, 0.3219752754296894559, 0.3333333333333333703, 0.3219752754296894559, 0.3333333333333333703, 0.3219752754296894559, 0.3333333333333333703, 0.3219752754296894559, 0.3333333333333333703, 0.3219752754296894559, 0.3333333333333333703, 0.3219752754296894559, 0.3333333333333333703, 0.3219752754296894559, 0.3333333333333333703, 0.3219752754296894559, 0.3333333333333333703, 0.3219752754296894559, 0.3333333333333333703, 0.3219752754296894559, 0.3333333333333333703, 0.3219752754296894559, 0.3333333333333333703, 0.3219752754296894559, 0.3333333333333333703, 0.3219752754296894559, 0.3333333333333333703, 0.3219752754296894559, 0.3333333333333333703, 0.3219752754296894559, 0.3333333333333333703, 0.3219752754296894559, 0.3333333333333333703, 0.3219752754296894559, 0.3333333333333333703, 0.3219752754296894559, 0.3333333333333333703, 0.3219752754296894559, 0.3333333333333333703, 0.3219752754296894559, 0.3333333333333333703, 0.3219752754296894559, 0.3333333333333333703, 0.3219752754296894559, 0.3333333333333333703, 0.3219752754296894559, 0.3333333333333333703, 0.3219752754296894559, 0.3333333333333333703, 0.3219752754296894559, 0.3333333333333333703, 0.3219752754296894559, 0.3333333333333333703, 0.3219752754296894559, 0.3333333333333333703, 0.3219752754296894559, 0.3333333333333333703, 0.3219752754296894559, 0.3333333333333333703, 0.3219752754296894559, 0.3333333333333333703, 0.3219752754296894559, 0.3333333333333333703, 0.3219752754296894559, 0.3333333333333333703, 0.3219752754296894559, 0.3333333333333333703, 0.3219752754296894559, 0.3333333333333333703, 0.3219752754296894559, 0.3333333333333333703, 0.3219752754296894559, 0.3333333333333333703, 0.3219752754296894559, 0.3333333333333333703, 0.3219752754296894559, 0.3333333333333333703, 0.3219752754296894559, 0.3333333333333333703, 0.3219752754296894559, 0.3333333333333333703, 0.3219752754296894559, 0.3333333333333333703, 0.3219752754296894559, 0.3333333333333333703, 0.3219752754296894559, 0.3333333333333333703, 0.3219752754296894559, 0.3333333333333333703, 0.3219752754296894559, 0.3333333333333333703, 0.3219752754296894559, 0.3333333333333333703, 0.3219752754296894559, 0.3333333333333333703, 0.3219752754296894559, 0.3333333333333333703, 0.3219752754296894559, 0.3333333333333333703, 0.3219752754296894559, 0.3333333333333333703, 0.3219752754296894559, 0.3333333333333333703, 0.3219752754296894559, 0.3333333333333333703, 0.3219752754296894559, 0.3333333333333333703, 0.3219752754296894559, 0.3333333333333333703, 0.3219752754296894559, 0.3333333333333333703, 0.3219752754296894559, 0.3333333333333333703, 0.3219752754296894559, 0.3333333333333333703, 0.3219752754296894559, 0.3333333333333333703, 0.3219752754296894559, 0.3333333333333333703, 0.3219752754296894559, 0.3333333333333333703, 0.3219752754296894559, 0.3333333333333333703, 0.3219752754296894559, 0.3333333333333333703, 0.3219752754296894559, 0.3333333333333333703, 0.3219752754296894559, 0.3333333333333333703, 0.3219752754296894559, 0.3333333333333333703, 0.3219752754296894559, 0.3333333333333333703, 0.3219752754296894559, 0.3333333333333333703, 0.3219752754296894559, 0.3333333333333333703, 0.3219752754296894559, 0.3333333333333333703, 0.3219752754296894559, 0.3333333333333333703, 0.3219752754296894559, 0.3333333333333333703, 0.3219752754296894559, 0.3333333333333333703, 0.3219752754296894559, 0.3333333333333333703, 0.3219752754296894559, 0.3333333333333333703, 0.3219752754296894559, 0.3333333333333333703, 0.3219752754296894559, 0.3333333333333333703, 0.3219752754296894559, 0.3333333333333333703, 0.3219752754296894559, 0.3333333333333333703, 0.3219752754296894559, 0.3333333333333333703, 0.3219752754296894559, 0.3333333333333333703, 0.3219752754296894559, 0.3333333333333333703, 0.3219752754296894559, 0.3333333333333333703, 0.3219752754296894559, 0.3333333333333333703, 0.3219752754296894559, 0.3333333333333333703, 0.3219752754296894559, 0.3333333333333333703, 0.3219752754296894559, 0.3333333333333333703, 0.3219752754296894559, 0.3333333333333333703, 0.3219752754296894559, 0.3333333333333333703, 0.3219752754296894559, 0.3333333333333333703, 0.3219752754296894559, 0.3333333333333333703, 0.3219752754296894559, 0.3333333333333333703, 0.3219752754296894559, 0.3333333333333333703, 0.3219752754296894559, 0.3333333333333333703, 0.3219752754296894559, 0.3333333333333333703, 0.3219752754296894559, 0.3333333333333333703, 0.3219752754296894559, 0.3333333333333333703, 0.3219752754296894559, 0.3333333333333333703, 0.3219752754296894559, 0.3333333333333333703, 0.3219752754296894559, 0.3333333333333333703, 0.3219752754296894559, 0.3333333333333333703, 0.3219752754296894559, 0.3333333333333333703, 0.3219752754296894559, 0.3333333333333333703, 0.3219752754296894559, 0.3333333333333333703, 0.3219752754296894559, 0.3333333333333333703, 0.3219752754296894559, 0.3333333333333333703, 0.3219752754296894559, 0.3333333333333333703, 0.3219752754296894559, 0.3333333333333333703, 0.3219752754296894559, 0.3333333333333333703, 0.3219752754296894559, 0.3333333333333333703, 0.3219752754296894559, 0.3333333333333333703, 0.3219752754296894559, 0.3333333333333333703, 0.3219752754296894559, 0.3333333333333333703, 0.3219752754296894559, 0.3333333333333333703, 0.3219752754296894559, 0.3333333333333333703, 0.3219752754296894559, 0.3333333333333333703, 0.3219752754296894559, 0.3333333333333333703, 0.3219752754296894559, 0.3333333333333333703, 0.3219752754296894559, 0.3333333333333333703, 0.3219752754296894559, 0.3333333333333333703, 0.3219752754296894559, 0.3333333333333333703, 0.3219752754296894559, 0.3333333333333333703, 0.3219752754296894559, 0.3333333333333333703, 0.3219752754296894559, 0.3333333333333333703, 0.3219752754296894559, 0.3333333333333333703, 0.3219752754296894559, 0.3333333333333333703, 0.3219752754296894559, 0.3333333333333333703, 0.3219752754296894559, 0.3333333333333333703, 0.3219752754296894559, 0.3333333333333333703, 0.3219752754296894559, 0.3333333333333333703, 0.3219752754296894559, 0.3333333333333333703, 0.3219752754296894559, 0.3333333333333333703, 0.3219752754296894559, 0.3333333333333333703, 0.3219752754296894559, 0.3333333333333333703, 0.3219752754296894559, 0.3333333333333333703, 0.3219752754296894559, 0.3333333333333333703, 0.3219752754296894559, 0.3333333333333333703, 0.3219752754296894559, 0.3333333333333333703, 0.3219752754296894559, 0.3333333333333333703, 0.3219752754296894559, 0.3333333333333333703, 0.3219752754296894559, 0.3333333333333333703, 0.3219752754296894559, 0.3333333333333333703, 0.3219752754296894559, 0.3333333333333333703, 0.3219752754296894559, 0.3333333333333333703),
 ( 0.3333333333333333703, 0.3219752754296894559, 0.3333333333333333703, 0.3219752754296894559, 0.3333333333333333703, 0.3219752754296894559, 0.3333333333333333703, 0.3219752754296894559, 0.3333333333333333703, 0.3219752754296894559, 0.3333333333333333703, 0.3219752754296894559, 0.3333333333333333703, 0.3219752754296894559, 0.3333333333333333703, 0.3219752754296894559, 0.3333333333333333703, 0.3219752754296894559, 0.3333333333333333703, 0.3219752754296894559, 0.3333333333333333703, 0.3219752754296894559, 0.3333333333333333703, 0.3219752754296894559, 0.3333333333333333703, 0.3219752754296894559, 0.3333333333333333703, 0.3219752754296894559, 0.3333333333333333703, 0.3219752754296894559, 0.3333333333333333703, 0.3219752754296894559, 0.3333333333333333703, 0.3219752754296894559, 0.3333333333333333703, 0.3219752754296894559, 0.3333333333333333703, 0.3219752754296894559, 0.3333333333333333703, 0.3219752754296894559, 0.3333333333333333703, 0.3219752754296894559, 0.3333333333333333703, 0.3219752754296894559, 0.3333333333333333703, 0.3219752754296894559, 0.3333333333333333703, 0.3219752754296894559, 0.3333333333333333703, 0.3219752754296894559, 0.3333333333333333703, 0.3219752754296894559, 0.3333333333333333703, 0.3219752754296894559, 0.3333333333333333703, 0.3219752754296894559, 0.3333333333333333703, 0.3219752754296894559, 0.3333333333333333703, 0.3219752754296894559, 0.3333333333333333703, 0.3219752754296894559, 0.3333333333333333703, 0.3219752754296894559, 0.3333333333333333703, 0.3219752754296894559, 0.3333333333333333703, 0.3219752754296894559, 0.3333333333333333703, 0.3219752754296894559, 0.3333333333333333703, 0.3219752754296894559, 0.3333333333333333703, 0.3219752754296894559, 0.3333333333333333703, 0.3219752754296894559, 0.3333333333333333703, 0.3219752754296894559, 0.3333333333333333703, 0.3219752754296894559, 0.3333333333333333703, 0.3219752754296894559, 0.3333333333333333703, 0.3219752754296894559, 0.3333333333333333703, 0.3219752754296894559, 0.3333333333333333703, 0.3219752754296894559, 0.3333333333333333703, 0.3219752754296894559, 0.3333333333333333703, 0.3219752754296894559, 0.3333333333333333703, 0.3219752754296894559, 0.3333333333333333703, 0.3219752754296894559, 0.3333333333333333703, 0.3219752754296894559, 0.3333333333333333703, 0.3219752754296894559, 0.3333333333333333703, 0.3219752754296894559, 0.3333333333333333703, 0.3219752754296894559, 0.3333333333333333703, 0.3219752754296894559, 0.3333333333333333703, 0.3219752754296894559, 0.3333333333333333703, 0.3219752754296894559, 0.3333333333333333703, 0.3219752754296894559, 0.3333333333333333703, 0.3219752754296894559, 0.3333333333333333703, 0.3219752754296894559, 0.3333333333333333703, 0.3219752754296894559, 0.3333333333333333703, 0.3219752754296894559, 0.3333333333333333703, 0.3219752754296894559, 0.3333333333333333703, 0.3219752754296894559, 0.3333333333333333703, 0.3219752754296894559, 0.3333333333333333703, 0.3219752754296894559, 0.3333333333333333703, 0.3219752754296894559, 0.3333333333333333703, 0.3219752754296894559, 0.3333333333333333703, 0.3219752754296894559, 0.3333333333333333703, 0.3219752754296894559, 0.3333333333333333703, 0.3219752754296894559, 0.3333333333333333703, 0.3219752754296894559, 0.3333333333333333703, 0.3219752754296894559, 0.3333333333333333703, 0.3219752754296894559, 0.3333333333333333703, 0.3219752754296894559, 0.3333333333333333703, 0.3219752754296894559, 0.3333333333333333703, 0.3219752754296894559, 0.3333333333333333703, 0.3219752754296894559, 0.3333333333333333703, 0.3219752754296894559, 0.3333333333333333703, 0.3219752754296894559, 0.3333333333333333703, 0.3219752754296894559, 0.3333333333333333703, 0.3219752754296894559, 0.3333333333333333703, 0.3219752754296894559, 0.3333333333333333703, 0.3219752754296894559, 0.3333333333333333703, 0.3219752754296894559, 0.3333333333333333703, 0.3219752754296894559, 0.3333333333333333703, 0.3219752754296894559, 0.3333333333333333703, 0.3219752754296894559, 0.3333333333333333703, 0.3219752754296894559, 0.3333333333333333703, 0.3219752754296894559, 0.3333333333333333703, 0.3219752754296894559, 0.3333333333333333703, 0.3219752754296894559, 0.3333333333333333703, 0.3219752754296894559, 0.3333333333333333703, 0.3219752754296894559, 0.3333333333333333703, 0.3219752754296894559, 0.3333333333333333703, 0.3219752754296894559, 0.3333333333333333703, 0.3219752754296894559, 0.3333333333333333703, 0.3219752754296894559, 0.3333333333333333703, 0.3219752754296894559, 0.3333333333333333703, 0.3219752754296894559, 0.3333333333333333703, 0.3219752754296894559, 0.3333333333333333703, 0.3219752754296894559, 0.3333333333333333703, 0.3219752754296894559, 0.3333333333333333703, 0.3219752754296894559, 0.3333333333333333703, 0.3219752754296894559, 0.3333333333333333703, 0.3219752754296894559, 0.3333333333333333703, 0.3219752754296894559, 0.3333333333333333703, 0.3219752754296894559, 0.3333333333333333703, 0.3219752754296894559, 0.3333333333333333703, 0.3219752754296894559, 0.3333333333333333703, 0.3219752754296894559, 0.3333333333333333703, 0.3219752754296894559, 0.3333333333333333703, 0.3219752754296894559, 0.3333333333333333703, 0.3219752754296894559, 0.3333333333333333703, 0.3219752754296894559, 0.3333333333333333703, 0.3219752754296894559, 0.3333333333333333703, 0.3219752754296894559, 0.3333333333333333703, 0.3219752754296894559, 0.3333333333333333703, 0.3219752754296894559, 0.3333333333333333703, 0.3219752754296894559, 0.3333333333333333703, 0.3219752754296894559, 0.3333333333333333703, 0.3219752754296894559, 0.3333333333333333703, 0.3219752754296894559, 0.3333333333333333703, 0.3219752754296894559, 0.3333333333333333703, 0.3219752754296894559, 0.3333333333333333703, 0.3219752754296894559, 0.3333333333333333703, 0.3219752754296894559, 0.3333333333333333703, 0.3219752754296894559, 0.3333333333333333703, 0.3219752754296894559, 0.3333333333333333703, 0.3219752754296894559, 0.3333333333333333703, 0.3219752754296894559, 0.3333333333333333703, 0.3219752754296894559, 0.3333333333333333703, 0.3219752754296894559, 0.3333333333333333703, 0.3219752754296894559, 0.3333333333333333703, 0.3219752754296894559, 0.3333333333333333703, 0.3219752754296894559, 0.3333333333333333703, 0.3219752754296894559, 0.3333333333333333703, 0.3219752754296894559, 0.3333333333333333703, 0.3219752754296894559, 0.3333333333333333703, 0.3219752754296894559, 0.3333333333333333703, 0.3219752754296894559, 0.3333333333333333703, 0.3219752754296894559, 0.3333333333333333703, 0.3219752754296894559, 0.3333333333333333703, 0.3219752754296894559, 0.3333333333333333703, 0.3219752754296894559, 0.3333333333333333703, 0.3219752754296894559, 0.3333333333333333703, 0.3219752754296894559, 0.3333333333333333703, 0.3219752754296894559, 0.3333333333333333703, 0.3219752754296894559, 0.3333333333333333703, 0.3219752754296894559, 0.3333333333333333703, 0.3219752754296894559, 0.3333333333333333703, 0.3219752754296894559, 0.3333333333333333703, 0.3219752754296894559, 0.3333333333333333703, 0.3219752754296894559, 0.3333333333333333703, 0.3219752754296894559, 0.3333333333333333703, 0.3219752754296894559, 0.3333333333333333703, 0.3219752754296894559, 0.3333333333333333703, 0.3219752754296894559, 0.3333333333333333703, 0.3219752754296894559, 0.3333333333333333703, 0.3219752754296894559, 0.3333333333333333703, 0.3219752754296894559, 0.3333333333333333703, 0.3219752754296894559, 0.3333333333333333703, 0.3219752754296894559, 0.3333333333333333703, 0.3219752754296894559, 0.3333333333333333703, 0.3219752754296894559, 0.3333333333333333703, 0.3219752754296894559, 0.3333333333333333703, 0.3219752754296894559, 0.3333333333333333703, 0.3219752754296894559, 0.3333333333333333703, 0.3219752754296894559, 0.3333333333333333703, 0.3219752754296894559, 0.3333333333333333703, 0.3219752754296894559, 0.3333333333333333703, 0.3219752754296894559, 0.3333333333333333703, 0.3219752754296894559, 0.3333333333333333703, 0.3219752754296894559, 0.3333333333333333703, 0.3219752754296894559, 0.3333333333333333703, 0.3219752754296894559, 0.3333333333333333703, 0.3219752754296894559, 0.3333333333333333703, 0.3219752754296894559, 0.3333333333333333703, 0.3219752754296894559, 0.3333333333333333703, 0.3219752754296894559, 0.3333333333333333703, 0.3219752754296894559, 0.3333333333333333703, 0.3219752754296894559, 0.3333333333333333703, 0.3219752754296894559, 0.3333333333333333703, 0.3219752754296894559, 0.3333333333333333703, 0.3219752754296894559, 0.3333333333333333703, 0.3219752754296894559, 0.3333333333333333703, 0.3219752754296894559, 0.3333333333333333703, 0.3219752754296894559, 0.3333333333333333703, 0.3219752754296894559, 0.3333333333333333703, 0.3219752754296894559, 0.3333333333333333703, 0.3219752754296894559, 0.3333333333333333703, 0.3219752754296894559, 0.3333333333333333703, 0.3219752754296894559, 0.3333333333333333703, 0.3219752754296894559, 0.3333333333333333703, 0.3219752754296894559, 0.3333333333333333703, 0.3219752754296894559, 0.3333333333333333703, 0.3219752754296894559, 0.3333333333333333703, 0.3219752754296894559, 0.3333333333333333703, 0.3219752754296894559, 0.3333333333333333703, 0.3219752754296894559, 0.3333333333333333703, 0.3219752754296894559, 0.3333333333333333703, 0.3219752754296894559, 0.3333333333333333703, 0.3219752754296894559, 0.3333333333333333703, 0.3219752754296894559, 0.3333333333333333703, 0.3219752754296894559, 0.3333333333333333703, 0.3219752754296894559, 0.3333333333333333703, 0.3219752754296894559, 0.3333333333333333703, 0.3219752754296894559, 0.3333333333333333703, 0.3219752754296894559, 0.3333333333333333703, 0.3219752754296894559, 0.3333333333333333703, 0.3219752754296894559, 0.3333333333333333703, 0.3219752754296894559, 0.3333333333333333703, 0.3219752754296894559, 0.3333333333333333703, 0.3219752754296894559, 0.3333333333333333703, 0.3219752754296894559, 0.3333333333333333703, 0.3219752754296894559, 0.3333333333333333703, 0.3219752754296894559, 0.3333333333333333703, 0.3219752754296894559, 0.3333333333333333703, 0.3219752754296894559, 0.3333333333333333703, 0.3219752754296894559, 0.3333333333333333703, 0.3219752754296894559, 0.3333333333333333703, 0.3219752754296894559, 0.3333333333333333703, 0.3219752754296894559, 0.3333333333333333703, 0.3219752754296894559, 0.3333333333333333703, 0.3219752754296894559, 0.3333333333333333703, 0.3219752754296894559, 0.3333333333333333703, 0.3219752754296894559, 0.3333333333333333703, 0.3219752754296894559, 0.3333333333333333703, 0.3219752754296894559, 0.3333333333333333703, 0.3219752754296894559, 0.3333333333333333703),
 ( 1.000000000000000000, 0.9659258262890683122, 1.000000000000000000, 0.9659258262890683122, 1.000000000000000000, 0.9659258262890683122, 1.000000000000000000, 0.9659258262890683122, 1.000000000000000000, 0.9659258262890683122, 1.000000000000000000, 0.9659258262890683122, 1.000000000000000000, 0.9659258262890683122, 1.000000000000000000, 0.9659258262890683122, 1.000000000000000000, 0.9659258262890683122, 1.000000000000000000, 0.9659258262890683122, 1.000000000000000000, 0.9659258262890683122, 1.000000000000000000, 0.9659258262890683122, 1.000000000000000000, 0.9659258262890683122, 1.000000000000000000, 0.9659258262890683122, 1.000000000000000000, 0.9659258262890683122, 1.000000000000000000, 0.9659258262890683122, 1.000000000000000000, 0.9659258262890683122, 1.000000000000000000, 0.9659258262890683122, 1.000000000000000000, 0.9659258262890683122, 1.000000000000000000, 0.9659258262890683122, 1.000000000000000000, 0.9659258262890683122, 1.000000000000000000, 0.9659258262890683122, 1.000000000000000000, 0.9659258262890683122, 1.000000000000000000, 0.9659258262890683122, 1.000000000000000000, 0.9659258262890683122, 1.000000000000000000, 0.9659258262890683122, 1.000000000000000000, 0.9659258262890683122, 1.000000000000000000, 0.9659258262890683122, 1.000000000000000000, 0.9659258262890683122, 1.000000000000000000, 0.9659258262890683122, 1.000000000000000000, 0.9659258262890683122, 1.000000000000000000, 0.9659258262890683122, 1.000000000000000000, 0.9659258262890683122, 1.000000000000000000, 0.9659258262890683122, 1.000000000000000000, 0.9659258262890683122, 1.000000000000000000, 0.9659258262890683122, 1.000000000000000000, 0.9659258262890683122, 1.000000000000000000, 0.9659258262890683122, 1.000000000000000000, 0.9659258262890683122, 1.000000000000000000, 0.9659258262890683122, 1.000000000000000000, 0.9659258262890683122, 1.000000000000000000, 0.9659258262890683122, 1.000000000000000000, 0.9659258262890683122, 1.000000000000000000, 0.9659258262890683122, 1.000000000000000000, 0.9659258262890683122, 1.000000000000000000, 0.9659258262890683122, 1.000000000000000000, 0.9659258262890683122, 1.000000000000000000, 0.9659258262890683122, 1.000000000000000000, 0.9659258262890683122, 1.000000000000000000, 0.9659258262890683122, 1.000000000000000000, 0.9659258262890683122, 1.000000000000000000, 0.9659258262890683122, 1.000000000000000000, 0.9659258262890683122, 1.000000000000000000, 0.9659258262890683122, 1.000000000000000000, 0.9659258262890683122, 1.000000000000000000, 0.9659258262890683122, 1.000000000000000000, 0.9659258262890683122, 1.000000000000000000, 0.9659258262890683122, 1.000000000000000000, 0.9659258262890683122, 1.000000000000000000, 0.9659258262890683122, 1.000000000000000000, 0.9659258262890683122, 1.000000000000000000, 0.9659258262890683122, 1.000000000000000000, 0.9659258262890683122, 1.000000000000000000, 0.9659258262890683122, 1.000000000000000000, 0.9659258262890683122, 1.000000000000000000, 0.9659258262890683122, 1.000000000000000000, 0.9659258262890683122, 1.000000000000000000, 0.9659258262890683122, 1.000000000000000000, 0.9659258262890683122, 1.000000000000000000, 0.9659258262890683122, 1.000000000000000000, 0.9659258262890683122, 1.000000000000000000, 0.9659258262890683122, 1.000000000000000000, 0.9659258262890683122, 1.000000000000000000, 0.9659258262890683122, 1.000000000000000000, 0.9659258262890683122, 1.000000000000000000, 0.9659258262890683122, 1.000000000000000000, 0.9659258262890683122, 1.000000000000000000, 0.9659258262890683122, 1.000000000000000000, 0.9659258262890683122, 1.000000000000000000, 0.9659258262890683122, 1.000000000000000000, 0.9659258262890683122, 1.000000000000000000, 0.9659258262890683122, 1.000000000000000000, 0.9659258262890683122, 1.000000000000000000, 0.9659258262890683122, 1.000000000000000000, 0.9659258262890683122, 1.000000000000000000, 0.9659258262890683122, 1.000000000000000000, 0.9659258262890683122, 1.000000000000000000, 0.9659258262890683122, 1.000000000000000000, 0.9659258262890683122, 1.000000000000000000, 0.9659258262890683122, 1.000000000000000000, 0.9659258262890683122, 1.000000000000000000, 0.9659258262890683122, 1.000000000000000000, 0.9659258262890683122, 1.000000000000000000, 0.9659258262890683122, 1.000000000000000000, 0.9659258262890683122, 1.000000000000000000, 0.9659258262890683122, 1.000000000000000000, 0.9659258262890683122, 1.000000000000000000, 0.9659258262890683122, 1.000000000000000000, 0.9659258262890683122, 1.000000000000000000, 0.9659258262890683122, 1.000000000000000000, 0.9659258262890683122, 1.000000000000000000, 0.9659258262890683122, 1.000000000000000000, 0.9659258262890683122, 1.000000000000000000, 0.9659258262890683122, 1.000000000000000000, 0.9659258262890683122, 1.000000000000000000, 0.9659258262890683122, 1.000000000000000000, 0.9659258262890683122, 1.000000000000000000, 0.9659258262890683122, 1.000000000000000000, 0.9659258262890683122, 1.000000000000000000, 0.9659258262890683122, 1.000000000000000000, 0.9659258262890683122, 1.000000000000000000, 0.9659258262890683122, 1.000000000000000000, 0.9659258262890683122, 1.000000000000000000, 0.9659258262890683122, 1.000000000000000000, 0.9659258262890683122, 1.000000000000000000, 0.9659258262890683122, 1.000000000000000000, 0.9659258262890683122, 1.000000000000000000, 0.9659258262890683122, 1.000000000000000000, 0.9659258262890683122, 1.000000000000000000, 0.9659258262890683122, 1.000000000000000000, 0.9659258262890683122, 1.000000000000000000, 0.9659258262890683122, 1.000000000000000000, 0.9659258262890683122, 1.000000000000000000, 0.9659258262890683122, 1.000000000000000000, 0.9659258262890683122, 1.000000000000000000, 0.9659258262890683122, 1.000000000000000000, 0.9659258262890683122, 1.000000000000000000, 0.9659258262890683122, 1.000000000000000000, 0.9659258262890683122, 1.000000000000000000, 0.9659258262890683122, 1.000000000000000000, 0.9659258262890683122, 1.000000000000000000, 0.9659258262890683122, 1.000000000000000000, 0.9659258262890683122, 1.000000000000000000, 0.9659258262890683122, 1.000000000000000000, 0.9659258262890683122, 1.000000000000000000, 0.9659258262890683122, 1.000000000000000000, 0.9659258262890683122, 1.000000000000000000, 0.9659258262890683122, 1.000000000000000000, 0.9659258262890683122, 1.000000000000000000, 0.9659258262890683122, 1.000000000000000000, 0.9659258262890683122, 1.000000000000000000, 0.9659258262890683122, 1.000000000000000000, 0.9659258262890683122, 1.000000000000000000, 0.9659258262890683122, 1.000000000000000000, 0.9659258262890683122, 1.000000000000000000, 0.9659258262890683122, 1.000000000000000000, 0.9659258262890683122, 1.000000000000000000, 0.9659258262890683122, 1.000000000000000000, 0.9659258262890683122, 1.000000000000000000, 0.9659258262890683122, 1.000000000000000000, 0.9659258262890683122, 1.000000000000000000, 0.9659258262890683122, 1.000000000000000000, 0.9659258262890683122, 1.000000000000000000, 0.9659258262890683122, 1.000000000000000000, 0.9659258262890683122, 1.000000000000000000, 0.9659258262890683122, 1.000000000000000000, 0.9659258262890683122, 1.000000000000000000, 0.9659258262890683122, 1.000000000000000000, 0.9659258262890683122, 1.000000000000000000, 0.9659258262890683122, 1.000000000000000000, 0.9659258262890683122, 1.000000000000000000, 0.9659258262890683122, 1.000000000000000000, 0.9659258262890683122, 1.000000000000000000, 0.9659258262890683122, 1.000000000000000000, 0.9659258262890683122, 1.000000000000000000, 0.9659258262890683122, 1.000000000000000000, 0.9659258262890683122, 1.000000000000000000, 0.9659258262890683122, 1.000000000000000000, 0.9659258262890683122, 1.000000000000000000, 0.9659258262890683122, 1.000000000000000000, 0.9659258262890683122, 1.000000000000000000, 0.9659258262890683122, 1.000000000000000000, 0.9659258262890683122, 1.000000000000000000, 0.9659258262890683122, 1.000000000000000000, 0.9659258262890683122, 1.000000000000000000, 0.9659258262890683122, 1.000000000000000000, 0.9659258262890683122, 1.000000000000000000, 0.9659258262890683122, 1.000000000000000000, 0.9659258262890683122, 1.000000000000000000, 0.9659258262890683122, 1.000000000000000000, 0.9659258262890683122, 1.000000000000000000, 0.9659258262890683122, 1.000000000000000000, 0.9659258262890683122, 1.000000000000000000, 0.9659258262890683122, 1.000000000000000000, 0.9659258262890683122, 1.000000000000000000, 0.9659258262890683122, 1.000000000000000000, 0.9659258262890683122, 1.000000000000000000, 0.9659258262890683122, 1.000000000000000000, 0.9659258262890683122, 1.000000000000000000, 0.9659258262890683122, 1.000000000000000000, 0.9659258262890683122, 1.000000000000000000, 0.9659258262890683122, 1.000000000000000000, 0.9659258262890683122, 1.000000000000000000, 0.9659258262890683122, 1.000000000000000000, 0.9659258262890683122, 1.000000000000000000, 0.9659258262890683122, 1.000000000000000000, 0.9659258262890683122, 1.000000000000000000, 0.9659258262890683122, 1.000000000000000000, 0.9659258262890683122, 1.000000000000000000, 0.9659258262890683122, 1.000000000000000000, 0.9659258262890683122, 1.000000000000000000, 0.9659258262890683122, 1.000000000000000000, 0.9659258262890683122, 1.000000000000000000, 0.9659258262890683122, 1.000000000000000000, 0.9659258262890683122, 1.000000000000000000, 0.9659258262890683122, 1.000000000000000000, 0.9659258262890683122, 1.000000000000000000, 0.9659258262890683122, 1.000000000000000000, 0.9659258262890683122, 1.000000000000000000, 0.9659258262890683122, 1.000000000000000000, 0.9659258262890683122, 1.000000000000000000, 0.9659258262890683122, 1.000000000000000000, 0.9659258262890683122, 1.000000000000000000, 0.9659258262890683122, 1.000000000000000000, 0.9659258262890683122, 1.000000000000000000, 0.9659258262890683122, 1.000000000000000000, 0.9659258262890683122, 1.000000000000000000, 0.9659258262890683122, 1.000000000000000000, 0.9659258262890683122, 1.000000000000000000, 0.9659258262890683122, 1.000000000000000000, 0.9659258262890683122, 1.000000000000000000, 0.9659258262890683122, 1.000000000000000000, 0.9659258262890683122, 1.000000000000000000, 0.9659258262890683122, 1.000000000000000000, 0.9659258262890683122, 1.000000000000000000, 0.9659258262890683122, 1.000000000000000000, 0.9659258262890683122, 1.000000000000000000, 0.9659258262890683122, 1.000000000000000000) ) ) 
 REPRESENTATION_ITEM ( '' )  SURFACE ( )  );
#46744=CARTESIAN_POINT ( 'NONE',  ( 0.05219959533936267826, -19.03943276465977164, 45.00109039468566863 ) ) ;
#46746=CARTESIAN_POINT ( 'NONE',  ( 5.153800228976335163, 19.02544592524342804, 64.79057627198100988 ) ) ;
#46747=CARTESIAN_POINT ( 'NONE',  ( 13.97604488694527802, 13.89961937509977652, 79.37390960531435269 ) ) ;
#46748=CARTESIAN_POINT ( 'NONE',  ( 8.314922557961029526, -14.29746914071037800, 55.41775706135234714 ) ) ;
#46749=CARTESIAN_POINT ( 'NONE',  ( 18.22780087662122384, -5.500000000000022204, 81.01540105326105845 ) ) ;
#46750=CARTESIAN_POINT ( 'NONE',  ( -17.48847506799969409, 5.747544572773746197, 110.8269743784328512 ) ) ;
#46751=CARTESIAN_POINT ( 'NONE',  ( 12.14591786802327356, -12.06949235617739191, 85.62609039468568994 ) ) ;
#46753=CARTESIAN_POINT ( 'NONE',  ( 4.379528057220092307, 16.55341960407617563, 82.29275706135234714 ) ) ;
#46754=CARTESIAN_POINT ( 'NONE',  ( 16.53943276465976808, 0.05219959533934440121, 51.25109039468568994 ) ) ;
#46755=CARTESIAN_POINT ( 'NONE',  ( -9.474510206698720793, -16.51473224551083518, 29.58442372801900433 ) ) ;
#46756=CARTESIAN_POINT ( 'NONE',  ( 5.153800228976335163, 19.02544592524342804, 49.79057627198100988 ) ) ;
#46758=CARTESIAN_POINT ( 'NONE',  ( -21.52544592524334988, -5.823673210054445271, 48.95942372801902565 ) ) ;
#46759=CARTESIAN_POINT ( 'NONE',  ( -13.89961937509957401, -13.97604488694547875, 79.37609039468567573 ) ) ;
#46760=CARTESIAN_POINT ( 'NONE',  ( -10.81492255796105439, 18.62759615963255655, 102.9177570613523756 ) ) ;
#46761=CARTESIAN_POINT ( 'NONE',  ( 9.474510206698971260, -16.51473224551069308, 32.91557627198102409 ) ) ;
#46763=CARTESIAN_POINT ( 'NONE',  ( 18.67979575497178502, 10.72451020669898547, 69.16557627198102409 ) ) ;
#46764=CARTESIAN_POINT ( 'NONE',  ( 13.97604488694527802, 13.89961937509977652, 114.3739096053143669 ) ) ;
#46765=CARTESIAN_POINT ( 'NONE',  ( 16.46253265017160672, -9.564922557960803928, 23.33224293864769194 ) ) ;
#46766=CARTESIAN_POINT ( 'NONE',  ( 4.379528057220092307, 16.55341960407617563, 32.29275706135235424 ) ) ;
#46767=CARTESIAN_POINT ( 'NONE',  ( 16.53943276465976808, -0.05219959533910856209, 33.74890960531436690 ) ) ;
#46769=CARTESIAN_POINT ( 'NONE',  ( 5.823673210054444382, -21.52544592524334988, 20.20942372801900788 ) ) ;
#46770=CARTESIAN_POINT ( 'NONE',  ( 0.05219959533910956823, 16.53943276465976808, 39.99890960531436690 ) ) ;
#46772=CARTESIAN_POINT ( 'NONE',  ( 5.153800228976615827, -19.02544592524334988, 105.2094237280190185 ) ) ;
#46773=CARTESIAN_POINT ( 'NONE',  ( 16.51473224551083163, -9.474510206698727899, 20.83442372801899722 ) ) ;
#46774=CARTESIAN_POINT ( 'NONE',  ( 8.224510206698953496, -14.34966873604960469, 37.91557627198102409 ) ) ;
#46775=CARTESIAN_POINT ( 'NONE',  ( -0.05219959533907301413, -21.53943276465977519, 107.4989096053143669 ) ) ;
#46777=CARTESIAN_POINT ( 'NONE',  ( 21.52544592524344225, -5.823673210054117533, 68.54057627198103830 ) ) ;
#46778=CARTESIAN_POINT ( 'NONE',  ( 0.05219959533909260263, 19.03943276465977164, 74.99890960531435269 ) ) ;
#46779=CARTESIAN_POINT ( 'NONE',  ( -8.314922557960811034, -14.29746914071050412, 52.08224293864768839 ) ) ;
#46780=CARTESIAN_POINT ( 'NONE',  ( -5.153800228976328057, -19.02544592524343514, 87.29057627198103830 ) ) ;
#46782=CARTESIAN_POINT ( 'NONE',  ( 9.474510206698729675, 16.51473224551082808, 52.08442372801900433 ) ) ;
#46783=CARTESIAN_POINT ( 'NONE',  ( -18.62759615963270932, 10.81492255796079327, 95.83224293864770971 ) ) ;
#46784=CARTESIAN_POINT ( 'NONE',  ( -12.14591786802309592, -12.06949235617757132, 101.8739096053143811 ) ) ;
#46785=CARTESIAN_POINT ( 'NONE',  ( 18.67979575497194134, -10.72451020669871369, 50.83442372801901143 ) ) ;
#46787=CARTESIAN_POINT ( 'NONE',  ( 14.34966873604960469, 8.224510206698951720, 29.16557627198103120 ) ) ;
#46788=CARTESIAN_POINT ( 'NONE',  ( 16.51473224551069308, 9.474510206698969483, 39.16557627198103120 ) ) ;
#46789=CARTESIAN_POINT ( 'NONE',  ( 13.97604488694527802, 13.89961937509977652, 94.37390960531436690 ) ) ;
#46790=CARTESIAN_POINT ( 'NONE',  ( 10.81492255796078972, 18.62759615963270932, 54.58224293864769550 ) ) ;
#46791=CARTESIAN_POINT ( 'NONE',  ( 5.049401038297881783, 19.05341960407617918, 92.29275706135234714 ) ) ;
#46792=CARTESIAN_POINT ( 'NONE',  ( 5.153800228976335163, 19.02544592524342804, 34.79057627198102409 ) ) ;
#46793=CARTESIAN_POINT ( 'NONE',  ( 21.55341960407610458, 5.719274019375980345, 53.95724293864770260 ) ) ;
#46794=CARTESIAN_POINT ( 'NONE',  ( -21.53943276465977519, -0.05219959533937600094, 68.75109039468568994 ) ) ;
#46796=CARTESIAN_POINT ( 'NONE',  ( 0.05219959533934541429, -16.53943276465976808, 85.00109039468568994 ) ) ;
#46797=CARTESIAN_POINT ( 'NONE',  ( -5.153800228976328057, -19.02544592524343514, 52.29057627198100988 ) ) ;
#46798=CARTESIAN_POINT ( 'NONE',  ( -5.049401038298153566, 19.05341960407611168, 60.20724293864768129 ) ) ;
#46799=ORIENTED_EDGE ( 'NONE', *, *, #148993, .F. ) ;
#46800=CARTESIAN_POINT ( 'NONE',  ( -5.153800228976607833, 19.02544592524334988, 32.70942372801899722 ) ) ;
#46801=CARTESIAN_POINT ( 'NONE',  ( -12.14591786802326823, 12.06949235617739902, 73.12609039468567573 ) ) ;
#46802=CARTESIAN_POINT ( 'NONE',  ( -21.55341960407619339, 5.719274019375674811, 98.54275706135234714 ) ) ;
#46803=CARTESIAN_POINT ( 'NONE',  ( -16.46253265017160317, 9.564922557960807481, 70.83224293864770971 ) ) ;
#46804=CARTESIAN_POINT ( 'NONE',  ( 10.72451020669898902, -18.67979575497178502, 32.91557627198102409 ) ) ;
#46805=CARTESIAN_POINT ( 'NONE',  ( -13.89961937509957401, -13.97604488694547875, 104.3760903946856757 ) ) ;
#46806=CARTESIAN_POINT ( 'NONE',  ( 15.72974639402176855, 15.80617190586768217, 81.87609039468568994 ) ) ;
#46807=CARTESIAN_POINT ( 'NONE',  ( 16.52544592524335698, 4.483927247898782831, 46.45942372801901854 ) ) ;
#46808=CARTESIAN_POINT ( 'NONE',  ( -15.72974639402197994, 15.80617190586746368, 95.62390960531436690 ) ) ;
#46809=CARTESIAN_POINT ( 'NONE',  ( -5.153800228976607833, 19.02544592524334988, 107.7094237280189759 ) ) ;
#46810=CARTESIAN_POINT ( 'NONE',  ( 9.564922557960805705, 16.46253265017160317, 79.58224293864769550 ) ) ;
#46811=CARTESIAN_POINT ( 'NONE',  ( -14.29746914071037622, -8.314922557961029526, 34.16775706135234714 ) ) ;
#46812=CARTESIAN_POINT ( 'NONE',  ( 13.97604488694527802, 13.89961937509977652, 39.37390960531435269 ) ) ;
#46813=CARTESIAN_POINT ( 'NONE',  ( 16.51473224551083163, -9.474510206698727899, 110.8344237280190043 ) ) ;
#46814=CARTESIAN_POINT ( 'NONE',  ( 12.14591786802309770, 12.06949235617756955, 84.37390960531438111 ) ) ;
#46815=CARTESIAN_POINT ( 'NONE',  ( 16.52544592524335698, 4.483927247898782831, 86.45942372801901854 ) ) ;
#46816=CARTESIAN_POINT ( 'NONE',  ( 21.53943276465977519, 0.05219959533937863772, 36.25109039468567573 ) ) ;
#46817=CARTESIAN_POINT ( 'NONE',  ( -16.46253265017160317, 9.564922557960807481, 55.83224293864769550 ) ) ;
#46818=CARTESIAN_POINT ( 'NONE',  ( -19.03943276465977164, 0.05219959533909376836, 66.24890960531436690 ) ) ;
#46819=CARTESIAN_POINT ( 'NONE',  ( 16.55341960407618274, -4.379528057220086978, 91.04275706135236135 ) ) ;
#46822=VERTEX_POINT ( 'NONE', #55986 ) ;
#46823=CARTESIAN_POINT ( 'NONE',  ( 16.51473224551083163, -9.474510206698727899, 20.83442372801899722 ) ) ;
#46824=CARTESIAN_POINT ( 'NONE',  ( -19.05341960407611168, -5.049401038298163336, 41.45724293864769550 ) ) ;
#46825=CARTESIAN_POINT ( 'NONE',  ( 16.51473224551069308, 9.474510206698969483, 109.1655762719810383 ) ) ;
#46827=CARTESIAN_POINT ( 'NONE',  ( -14.29746914071037622, -8.314922557961029526, 34.16775706135234714 ) ) ;
#46828=CARTESIAN_POINT ( 'NONE',  ( -16.51473224551082808, 9.474510206698731452, 63.33442372801900433 ) ) ;
#46829=CARTESIAN_POINT ( 'NONE',  ( 12.14591786802327356, -12.06949235617739191, 40.62609039468567573 ) ) ;
#46830=CARTESIAN_POINT ( 'NONE',  ( 19.03943276465977164, -0.05219959533909143690, 43.74890960531435979 ) ) ;
#46831=CARTESIAN_POINT ( 'NONE',  ( 16.46253265017160672, -9.564922557960803928, 103.3322429386476955 ) ) ;
#46832=CARTESIAN_POINT ( 'NONE',  ( 5.049401038298161559, -19.05341960407611168, 67.70724293864769550 ) ) ;
#46833=CARTESIAN_POINT ( 'NONE',  ( 5.823673210054125526, 21.52544592524343514, 99.79057627198103830 ) ) ;
#46834=CARTESIAN_POINT ( 'NONE',  ( -0.05219959533909027116, -19.03943276465977164, 92.49890960531436690 ) ) ;
#46836=CARTESIAN_POINT ( 'NONE',  ( 0.05219959533909260263, 19.03943276465977164, 59.99890960531436690 ) ) ;
#46837=CARTESIAN_POINT ( 'NONE',  ( -12.14591786802326823, 12.06949235617739902, 108.1260903946856757 ) ) ;
#46838=CARTESIAN_POINT ( 'NONE',  ( 16.46253265017160672, -9.564922557960803928, 28.33224293864769550 ) ) ;
#46839=CARTESIAN_POINT ( 'NONE',  ( -19.05341960407617563, 5.049401038297882671, 23.54275706135233648 ) ) ;
#46841=CARTESIAN_POINT ( 'NONE',  ( -14.34966873604960291, -8.224510206698953496, 61.66557627198103120 ) ) ;
#46842=CARTESIAN_POINT ( 'NONE',  ( 21.52544592524334988, 5.823673210054432836, 101.4594237280190185 ) ) ;
#46843=CARTESIAN_POINT ( 'NONE',  ( -9.564922557960796823, -16.46253265017161027, 37.08224293864768839 ) ) ;
#46844=CARTESIAN_POINT ( 'NONE',  ( 14.29746914071049879, -8.314922557960816363, 43.33224293864769550 ) ) ;
#46845=CARTESIAN_POINT ( 'NONE',  ( 21.53943276465977519, 0.05219959533937863772, 96.25109039468568994 ) ) ;
#46846=CARTESIAN_POINT ( 'NONE',  ( 19.03943276465977164, -0.05219959533909143690, 83.74890960531436690 ) ) ;
#46847=CARTESIAN_POINT ( 'NONE',  ( -9.474510206698964154, 16.51473224551069663, 90.41557627198103830 ) ) ;
#46848=CARTESIAN_POINT ( 'NONE',  ( -14.34966873604960291, -8.224510206698953496, 111.6655762719810525 ) ) ;
#46849=CARTESIAN_POINT ( 'NONE',  ( 16.55341960407611168, 4.379528057220329451, 73.95724293864769550 ) ) ;
#46850=CARTESIAN_POINT ( 'NONE',  ( 10.72451020669898902, -18.67979575497178502, 87.91557627198103830 ) ) ;
#46851=CARTESIAN_POINT ( 'NONE',  ( 13.97604488694527802, 13.89961937509977652, 69.37390960531436690 ) ) ;
#46852=CARTESIAN_POINT ( 'NONE',  ( 10.72451020669898902, -18.67979575497178502, 82.91557627198103830 ) ) ;
#46854=CARTESIAN_POINT ( 'NONE',  ( -16.46253265017146816, -9.564922557961047289, 79.16775706135234714 ) ) ;
#46855=CARTESIAN_POINT ( 'NONE',  ( 5.153800228976617603, -19.02544592524335343, 65.20942372801899012 ) ) ;
#46856=CARTESIAN_POINT ( 'NONE',  ( -4.483927247898539470, -16.52544592524342804, 87.29057627198103830 ) ) ;
#46857=CARTESIAN_POINT ( 'NONE',  ( 19.05341960407611168, 5.049401038298154454, 63.95724293864769550 ) ) ;
#46858=CARTESIAN_POINT ( 'NONE',  ( 0.05219959533907565091, 21.53943276465977519, 64.99890960531435269 ) ) ;
#46859=CARTESIAN_POINT ( 'NONE',  ( -17.60691670004652565, -5.499999999999996447, 84.13333313366439370 ) ) ;
#46860=CARTESIAN_POINT ( 'NONE',  ( 4.379528057220092307, 16.55341960407617563, 112.2927570613523471 ) ) ;
#46861=CARTESIAN_POINT ( 'NONE',  ( 4.483927247898790824, -16.52544592524335698, 25.20942372801901854 ) ) ;
#46862=CARTESIAN_POINT ( 'NONE',  ( 0.05219959533910956823, 16.53943276465976808, 74.99890960531435269 ) ) ;
#46863=CARTESIAN_POINT ( 'NONE',  ( -18.89770734986048950, -5.499999999999954703, 94.10214472496637939 ) ) ;
#46864=CARTESIAN_POINT ( 'NONE',  ( -13.97604488694527625, -13.89961937509977652, 76.87390960531433848 ) ) ;
#46865=CARTESIAN_POINT ( 'NONE',  ( -9.474510206698964154, 16.51473224551069663, 30.41557627198102054 ) ) ;
#46866=CARTESIAN_POINT ( 'NONE',  ( 16.52544592524342804, -4.483927247898539470, 68.54057627198103830 ) ) ;
#46867=CARTESIAN_POINT ( 'NONE',  ( -5.153800228976328057, -19.02544592524343514, 112.2905762719810099 ) ) ;
#46868=CARTESIAN_POINT ( 'NONE',  ( 19.03943276465977164, 0.05219959533936151252, 86.25109039468567573 ) ) ;
#46869=CARTESIAN_POINT ( 'NONE',  ( -13.89961937509977652, 13.97604488694528158, 80.62390960531436690 ) ) ;
#46871=CARTESIAN_POINT ( 'NONE',  ( 0.05219959533909260263, 19.03943276465977164, 89.99890960531436690 ) ) ;
#46872=CARTESIAN_POINT ( 'NONE',  ( -15.80617190586745835, -15.72974639402198527, 76.87390960531439532 ) ) ;
#46873=CARTESIAN_POINT ( 'NONE',  ( -8.224510206698735004, -14.34966873604973081, 69.58442372801900433 ) ) ;
#46874=CARTESIAN_POINT ( 'NONE',  ( -19.03943276465977164, 0.05219959533909376836, 56.24890960531435979 ) ) ;
#46875=CARTESIAN_POINT ( 'NONE',  ( 21.53943276465977519, -0.05219959533907433946, 68.74890960531435269 ) ) ;
#46876=CARTESIAN_POINT ( 'NONE',  ( -21.52544592524334988, -5.823673210054445271, 73.95942372801901854 ) ) ;
#46877=CARTESIAN_POINT ( 'NONE',  ( 19.05341960407617918, -5.049401038297876454, 91.04275706135234714 ) ) ;
#46878=CARTESIAN_POINT ( 'NONE',  ( -4.483927247898539470, -16.52544592524342804, 42.29057627198103120 ) ) ;
#46879=CARTESIAN_POINT ( 'NONE',  ( 10.81492255796106328, -18.62759615963255655, 40.41775706135234714 ) ) ;
#46881=CARTESIAN_POINT ( 'NONE',  ( 12.06949235617739724, 12.14591786802326823, 71.87609039468568994 ) ) ;
#46882=CARTESIAN_POINT ( 'NONE',  ( -16.51473224551069308, -9.474510206698971260, 106.6655762719810383 ) ) ;
#46885=CARTESIAN_POINT ( 'NONE',  ( 0.05219959533934541429, -16.53943276465976808, 90.00109039468567573 ) ) ;
#46886=CARTESIAN_POINT ( 'NONE',  ( -12.06949235617739369, -12.14591786802326823, 49.37609039468569705 ) ) ;
#46887=CARTESIAN_POINT ( 'NONE',  ( -19.05341960407611168, -5.049401038298163336, 61.45724293864769550 ) ) ;
#46888=CARTESIAN_POINT ( 'NONE',  ( 9.474510206698971260, -16.51473224551069308, 77.91557627198103830 ) ) ;
#46889=CARTESIAN_POINT ( 'NONE',  ( -5.719274019375665041, -21.55341960407619695, 59.79275706135234714 ) ) ;
#46890=CARTESIAN_POINT ( 'NONE',  ( -12.06949235617739369, -12.14591786802326823, 64.37609039468568994 ) ) ;
#46891=CARTESIAN_POINT ( 'NONE',  ( -12.14591786802309592, -12.06949235617757132, 26.87390960531435979 ) ) ;
#46892=CARTESIAN_POINT ( 'NONE',  ( -9.564922557960796823, -16.46253265017161027, 37.08224293864768839 ) ) ;
#46893=CARTESIAN_POINT ( 'NONE',  ( 5.153800228976335163, 19.02544592524342804, 29.79057627198102409 ) ) ;
#46894=CARTESIAN_POINT ( 'NONE',  ( -16.52544592524335698, -4.483927247898792601, 23.95942372801901143 ) ) ;
#46896=CARTESIAN_POINT ( 'NONE',  ( -13.97604488694547697, 13.89961937509957934, 83.12609039468564731 ) ) ;
#46897=CARTESIAN_POINT ( 'NONE',  ( 4.379528057220339221, -16.55341960407611168, 82.70724293864770971 ) ) ;
#46898=CARTESIAN_POINT ( 'NONE',  ( -9.474510206698964154, 16.51473224551069663, 45.41557627198103120 ) ) ;
#46899=CARTESIAN_POINT ( 'NONE',  ( 16.51473224551083163, -9.474510206698727899, 90.83442372801900433 ) ) ;
#46901=CARTESIAN_POINT ( 'NONE',  ( -21.55341960407619339, 5.719274019375674811, 93.54275706135234714 ) ) ;
#46902=CARTESIAN_POINT ( 'NONE',  ( -4.483927247898782831, 16.52544592524335698, 47.70942372801902565 ) ) ;
#46903=CARTESIAN_POINT ( 'NONE',  ( 16.62475595723696387, 7.163666690055258357, 36.97286648189536606 ) ) ;
#46904=CARTESIAN_POINT ( 'NONE',  ( -15.72974639402197994, 15.80617190586746368, 50.62390960531435979 ) ) ;
#46905=CARTESIAN_POINT ( 'NONE',  ( -0.05219959533934338120, 16.53943276465976808, 42.50109039468567573 ) ) ;
#46906=CARTESIAN_POINT ( 'NONE',  ( 13.97604488694527802, 13.89961937509977830, 34.37390960531435979 ) ) ;
#46907=CARTESIAN_POINT ( 'NONE',  ( -13.97604488694547697, 13.89961937509957934, 48.12609039468566863 ) ) ;
#46908=CARTESIAN_POINT ( 'NONE',  ( 16.46253265017160672, -9.564922557960803928, 83.33224293864768129 ) ) ;
#46909=CARTESIAN_POINT ( 'NONE',  ( -13.97604488694527625, -13.89961937509977652, 51.87390960531436690 ) ) ;
#46912=CARTESIAN_POINT ( 'NONE',  ( 19.05341960407611168, 5.049401038298154454, 63.95724293864769550 ) ) ;
#46914=CARTESIAN_POINT ( 'NONE',  ( -9.564922557961040184, 16.46253265017147172, 37.91775706135233293 ) ) ;
#46915=CARTESIAN_POINT ( 'NONE',  ( 0.05219959533937995610, -21.53943276465977519, 105.0010903946856757 ) ) ;
#46916=CARTESIAN_POINT ( 'NONE',  ( 0.05219959533910956823, 16.53943276465976808, 39.99890960531436690 ) ) ;
#46917=CARTESIAN_POINT ( 'NONE',  ( -9.564922557960796823, -16.46253265017161027, 47.08224293864769550 ) ) ;
#46918=CARTESIAN_POINT ( 'NONE',  ( -19.02544592524342804, 5.153800228976336051, 111.0405762719810099 ) ) ;
#46919=CARTESIAN_POINT ( 'NONE',  ( -15.72974639402176322, -15.80617190586768395, 79.37609039468567573 ) ) ;
#46920=CARTESIAN_POINT ( 'NONE',  ( -19.02544592524342804, 5.153800228976336051, 51.04057627198103120 ) ) ;
#46921=CARTESIAN_POINT ( 'NONE',  ( 10.81492255796106328, -18.62759615963255655, 85.41775706135236135 ) ) ;
#46922=CARTESIAN_POINT ( 'NONE',  ( -15.72974639402197994, 15.80617190586746368, 35.62390960531437401 ) ) ;
#46923=CARTESIAN_POINT ( 'NONE',  ( -0.05219959533937732626, 21.53943276465977519, 22.50109039468567573 ) ) ;
#46924=CARTESIAN_POINT ( 'NONE',  ( -19.05341960407617563, 5.049401038297882671, 48.54275706135233293 ) ) ;
#46925=CARTESIAN_POINT ( 'NONE',  ( 9.564922557960805705, 16.46253265017160317, 34.58224293864770260 ) ) ;
#46926=CARTESIAN_POINT ( 'NONE',  ( -9.564922557960796823, -16.46253265017161027, 77.08224293864769550 ) ) ;
#46927=CARTESIAN_POINT ( 'NONE',  ( 13.89961937509957401, 13.97604488694547697, 111.8760903946856757 ) ) ;
#46928=CARTESIAN_POINT ( 'NONE',  ( -4.483927247898539470, -16.52544592524342804, 87.29057627198103830 ) ) ;
#46929=CARTESIAN_POINT ( 'NONE',  ( -13.97604488694527625, -13.89961937509977652, 51.87390960531436690 ) ) ;
#46930=CARTESIAN_POINT ( 'NONE',  ( -5.823673210054116645, -21.52544592524344225, 32.29057627198102409 ) ) ;
#46931=CARTESIAN_POINT ( 'NONE',  ( 19.05341960407617918, -5.049401038297876454, 96.04275706135231871 ) ) ;
#46932=CARTESIAN_POINT ( 'NONE',  ( 5.823673210054125526, 21.52544592524343514, 99.79057627198103830 ) ) ;
#46933=CARTESIAN_POINT ( 'NONE',  ( 15.72974639402176855, 15.80617190586768217, 61.87609039468568284 ) ) ;
#46934=CARTESIAN_POINT ( 'NONE',  ( 0.05219959533934541429, -16.53943276465976808, 60.00109039468568284 ) ) ;
#46935=CARTESIAN_POINT ( 'NONE',  ( 8.314922557961029526, -14.29746914071037800, 70.41775706135236135 ) ) ;
#46936=CARTESIAN_POINT ( 'NONE',  ( 9.564922557960805705, 16.46253265017160317, 64.58224293864769550 ) ) ;
#46937=CARTESIAN_POINT ( 'NONE',  ( -0.05219959533934338120, 16.53943276465976808, 92.50109039468567573 ) ) ;
#46938=CARTESIAN_POINT ( 'NONE',  ( -21.53943276465977519, 0.05219959533907696930, 111.2489096053143669 ) ) ;
#46939=CARTESIAN_POINT ( 'NONE',  ( -14.34966873604960291, -8.224510206698953496, 71.66557627198100988 ) ) ;
#46940=CARTESIAN_POINT ( 'NONE',  ( 19.03943276465977164, -0.05219959533909143690, 83.74890960531436690 ) ) ;
#46941=CARTESIAN_POINT ( 'NONE',  ( 12.14591786802327356, -12.06949235617739191, 70.62609039468567573 ) ) ;
#46942=CARTESIAN_POINT ( 'NONE',  ( 15.72974639402176855, 15.80617190586768217, 61.87609039468568284 ) ) ;
#46943=CARTESIAN_POINT ( 'NONE',  ( -9.474510206698720793, -16.51473224551083518, 109.5844237280190043 ) ) ;
#46944=CARTESIAN_POINT ( 'NONE',  ( -15.72974639402197994, 15.80617190586746368, 110.6239096053143669 ) ) ;
#46945=CARTESIAN_POINT ( 'NONE',  ( 8.224510206698953496, -14.34966873604960469, 62.91557627198102409 ) ) ;
#46947=CARTESIAN_POINT ( 'NONE',  ( -17.49999999999999645, 5.499999999999992895, 68.71769037696435589 ) ) ;
#46948=CARTESIAN_POINT ( 'NONE',  ( 21.52544592524344225, -5.823673210054117533, 83.54057627198102409 ) ) ;
#46949=CARTESIAN_POINT ( 'NONE',  ( -14.29746914071049879, 8.314922557960819915, 45.83224293864769550 ) ) ;
#46952=CARTESIAN_POINT ( 'NONE',  ( 21.52544592524334988, 5.823673210054432836, 21.45942372801901499 ) ) ;
#46954=CARTESIAN_POINT ( 'NONE',  ( -21.55341960407610458, -5.719274019375992779, 21.45724293864769550 ) ) ;
#46955=CARTESIAN_POINT ( 'NONE',  ( -15.80617190586768217, 15.72974639402176855, 23.12609039468567573 ) ) ;
#46956=CARTESIAN_POINT ( 'NONE',  ( 14.29746914071049879, -8.314922557960816363, 53.33224293864769550 ) ) ;
#46957=CARTESIAN_POINT ( 'NONE',  ( 0.05219959533934541429, -16.53943276465976808, 65.00109039468568994 ) ) ;
#46958=CARTESIAN_POINT ( 'NONE',  ( 19.03943276465977164, -0.05219959533909143690, 58.74890960531435979 ) ) ;
#46959=CARTESIAN_POINT ( 'NONE',  ( -13.89961937509957401, -13.97604488694547875, 64.37609039468567573 ) ) ;
#46960=CARTESIAN_POINT ( 'NONE',  ( 0.05219959533909260263, 19.03943276465977164, 74.99890960531435269 ) ) ;
#46961=CARTESIAN_POINT ( 'NONE',  ( 5.823673210054125526, 21.52544592524343514, 34.79057627198103120 ) ) ;
#46963=CARTESIAN_POINT ( 'NONE',  ( 16.51473224551069308, 9.474510206698969483, 59.16557627198102409 ) ) ;
#46964=CARTESIAN_POINT ( 'NONE',  ( -16.53943276465976808, -0.05219959533934237506, 28.75109039468567929 ) ) ;
#46965=CARTESIAN_POINT ( 'NONE',  ( 9.564922557961047289, -16.46253265017146816, 65.41775706135233293 ) ) ;
#46966=CARTESIAN_POINT ( 'NONE',  ( -21.53943276465977519, -0.05219959533937600094, 23.75109039468567929 ) ) ;
#46967=CARTESIAN_POINT ( 'NONE',  ( 16.52544592524342804, -4.483927247898539470, 28.54057627198103120 ) ) ;
#46968=CARTESIAN_POINT ( 'NONE',  ( 16.51473224551069308, 9.474510206698969483, 89.16557627198103830 ) ) ;
#46969=CARTESIAN_POINT ( 'NONE',  ( -21.55341960407610458, -5.719274019375992779, 61.45724293864770260 ) ) ;
#46970=CARTESIAN_POINT ( 'NONE',  ( -15.80617190586745835, -15.72974639402198527, 91.87390960531436690 ) ) ;
#46971=CARTESIAN_POINT ( 'NONE',  ( 0.05219959533934541429, -16.53943276465976808, 35.00109039468568284 ) ) ;
#46972=CARTESIAN_POINT ( 'NONE',  ( 0.05219959533907565091, 21.53943276465977519, 39.99890960531436690 ) ) ;
#46973=CARTESIAN_POINT ( 'NONE',  ( -18.62759615963255300, -10.81492255796106328, 89.16775706135236135 ) ) ;
#46974=CARTESIAN_POINT ( 'NONE',  ( -5.153800228976328057, -19.02544592524343514, 82.29057627198103830 ) ) ;
#46975=CARTESIAN_POINT ( 'NONE',  ( -9.474510206698964154, 16.51473224551069663, 45.41557627198103120 ) ) ;
#46976=CARTESIAN_POINT ( 'NONE',  ( -9.474510206698964154, 16.51473224551069663, 95.41557627198102409 ) ) ;
#46977=CARTESIAN_POINT ( 'NONE',  ( -16.55341960407611168, -4.379528057220339221, 101.4572429386476955 ) ) ;
#46978=CARTESIAN_POINT ( 'NONE',  ( 19.05341960407611168, 5.049401038298154454, 58.95724293864768129 ) ) ;
#46979=CARTESIAN_POINT ( 'NONE',  ( -4.379528057220086978, -16.55341960407618274, 24.79275706135235779 ) ) ;
#46980=CARTESIAN_POINT ( 'NONE',  ( 17.50000000000001066, 3.345213924137313555, 32.91231376905654571 ) ) ;
#46981=CARTESIAN_POINT ( 'NONE',  ( 21.52544592524334988, 5.823673210054432836, 101.4594237280190185 ) ) ;
#46982=CARTESIAN_POINT ( 'NONE',  ( 5.153800228976335163, 19.02544592524342804, 109.7905762719810099 ) ) ;
#46983=B_SPLINE_CURVE_WITH_KNOTS ( 'NONE', 3,
 ( #100339, #194373, #39668, #131685, #180216, #42681 ),
 .UNSPECIFIED., .F., .F.,
 ( 4, 2, 4 ),
 ( 0.003239945802372296794, 0.003620412082092151589, 0.004000878361812006817 ),
 .UNSPECIFIED. ) ;
#46984=CARTESIAN_POINT ( 'NONE',  ( 14.34966873604972726, -8.224510206698740333, 95.83442372801903275 ) ) ;
#46986=CARTESIAN_POINT ( 'NONE',  ( -19.03943276465977164, -0.05219959533935918106, 68.75109039468566152 ) ) ;
#46987=CARTESIAN_POINT ( 'NONE',  ( 13.97604488694548053, -13.89961937509957401, 25.62609039468566507 ) ) ;
#46989=CARTESIAN_POINT ( 'NONE',  ( -13.89961937509977652, 13.97604488694528158, 25.62390960531434558 ) ) ;
#46990=CARTESIAN_POINT ( 'NONE',  ( -4.483927247898539470, -16.52544592524342804, 32.29057627198102409 ) ) ;
#46991=CARTESIAN_POINT ( 'NONE',  ( -17.26172910966780094, -6.454744622555835143, 109.1935309135077716 ) ) ;
#46992=CARTESIAN_POINT ( 'NONE',  ( -16.55341960407617563, 4.379528057220093196, 113.5427570613523756 ) ) ;
#46993=CARTESIAN_POINT ( 'NONE',  ( 17.40805194822030444, 6.112264579159358391, 66.66628727489390371 ) ) ;
#46994=CARTESIAN_POINT ( 'NONE',  ( 12.06949235617739724, 12.14591786802326823, 91.87609039468568994 ) ) ;
#46995=CARTESIAN_POINT ( 'NONE',  ( -5.153800228976328057, -19.02544592524343514, 32.29057627198102409 ) ) ;
#46996=CARTESIAN_POINT ( 'NONE',  ( 15.80617190586769283, -15.72974639402175789, 105.6260903946856899 ) ) ;
#46997=CARTESIAN_POINT ( 'NONE',  ( 16.55341960407618274, -4.379528057220086978, 21.04275706135234714 ) ) ;
#46998=CARTESIAN_POINT ( 'NONE',  ( 5.719274019375673035, 21.55341960407619339, 72.29275706135236135 ) ) ;
#46999=CARTESIAN_POINT ( 'NONE',  ( -16.46253265017146816, -9.564922557961047289, 49.16775706135233293 ) ) ;
#47000=CARTESIAN_POINT ( 'NONE',  ( 13.89961937509977652, -13.97604488694527269, 98.12390960531433848 ) ) ;
#47001=CARTESIAN_POINT ( 'NONE',  ( -19.02544592524342804, 5.153800228976336051, 71.04057627198099567 ) ) ;
#47002=CARTESIAN_POINT ( 'NONE',  ( 17.26172910966777962, 6.454744622555869782, 71.69353091350775742 ) ) ;
#47003=CARTESIAN_POINT ( 'NONE',  ( 5.823673210054125526, 21.52544592524343514, 94.79057627198105251 ) ) ;
#47005=CARTESIAN_POINT ( 'NONE',  ( -8.224510206698948167, 14.34966873604960824, 60.41557627198102409 ) ) ;
#47006=CARTESIAN_POINT ( 'NONE',  ( 15.80617190586746368, 15.72974639402197994, 59.37390960531436690 ) ) ;
#47007=CARTESIAN_POINT ( 'NONE',  ( 9.474510206698971260, -16.51473224551069308, 57.91557627198103120 ) ) ;
#47008=CARTESIAN_POINT ( 'NONE',  ( 18.62759615963271287, -10.81492255796078972, 88.33224293864769550 ) ) ;
#47009=CARTESIAN_POINT ( 'NONE',  ( -16.55341960407617563, 4.379528057220093196, 78.54275706135236135 ) ) ;
#47010=ORIENTED_EDGE ( 'NONE', *, *, #56442, .T. ) ;
#47011=CARTESIAN_POINT ( 'NONE',  ( -19.03943276465977164, 0.05219959533909376836, 41.24890960531435269 ) ) ;
#47012=CARTESIAN_POINT ( 'NONE',  ( -8.314922557960811034, -14.29746914071050412, 82.08224293864768129 ) ) ;
#47014=CARTESIAN_POINT ( 'NONE',  ( 16.51473224551069308, 9.474510206698969483, 49.16557627198102409 ) ) ;
#47015=CARTESIAN_POINT ( 'NONE',  ( 14.29746914071049879, -8.314922557960816363, 113.3322429386476955 ) ) ;
#47016=CARTESIAN_POINT ( 'NONE',  ( 19.05341960407617918, -5.049401038297876454, 61.04275706135232582 ) ) ;
#47017=CARTESIAN_POINT ( 'NONE',  ( -16.52544592524342804, 4.483927247898546575, 81.04057627198102409 ) ) ;
#47018=CARTESIAN_POINT ( 'NONE',  ( -15.72974639402176322, -15.80617190586768395, 44.37609039468567573 ) ) ;
#47019=CARTESIAN_POINT ( 'NONE',  ( 9.474510206698971260, -16.51473224551069308, 37.91557627198102409 ) ) ;
#47020=CARTESIAN_POINT ( 'NONE',  ( -10.81492255796078084, -18.62759615963271287, 102.0822429386476955 ) ) ;
#47021=CARTESIAN_POINT ( 'NONE',  ( 14.29746914071049879, -8.314922557960816363, 83.33224293864769550 ) ) ;
#47023=CARTESIAN_POINT ( 'NONE',  ( 16.51473224551069308, 9.474510206698969483, 64.16557627198102409 ) ) ;
#47026=CARTESIAN_POINT ( 'NONE',  ( -13.97604488694547697, 13.89961937509957934, 93.12609039468566152 ) ) ;
#47027=CARTESIAN_POINT ( 'NONE',  ( -16.46253265017160317, 9.564922557960807481, 95.83224293864769550 ) ) ;
#47028=CARTESIAN_POINT ( 'NONE',  ( 21.52544592524334988, 5.823673210054432836, 41.45942372801901143 ) ) ;
#47029=CARTESIAN_POINT ( 'NONE',  ( 9.564922557960805705, 16.46253265017160317, 89.58224293864769550 ) ) ;
#47030=CARTESIAN_POINT ( 'NONE',  ( 5.153800228976615827, -19.02544592524334988, 70.20942372801899012 ) ) ;
#47031=CARTESIAN_POINT ( 'NONE',  ( 19.02544592524343514, -5.153800228976328945, 38.54057627198103120 ) ) ;
#47033=CARTESIAN_POINT ( 'NONE',  ( 16.52544592524342804, -4.483927247898539470, 73.54057627198102409 ) ) ;
#47034=CARTESIAN_POINT ( 'NONE',  ( -14.34966873604960291, -8.224510206698953496, 71.66557627198100988 ) ) ;
#47035=CARTESIAN_POINT ( 'NONE',  ( 19.02544592524343514, -5.153800228976328945, 88.54057627198102409 ) ) ;
#47036=CARTESIAN_POINT ( 'NONE',  ( 10.81492255796078972, 18.62759615963270932, 104.5822429386477097 ) ) ;
#47037=CARTESIAN_POINT ( 'NONE',  ( -19.02544592524342804, 5.153800228976336051, 91.04057627198100988 ) ) ;
#47038=CARTESIAN_POINT ( 'NONE',  ( -13.97604488694547697, 13.89961937509957934, 33.12609039468566863 ) ) ;
#47039=CARTESIAN_POINT ( 'NONE',  ( -16.46253265017160317, 9.564922557960807481, 35.83224293864768839 ) ) ;
#47040=CARTESIAN_POINT ( 'NONE',  ( -0.05219959533910754901, -16.53943276465976808, 27.49890960531435269 ) ) ;
#47041=CARTESIAN_POINT ( 'NONE',  ( -16.53943276465976808, 0.05219959533911058130, 116.2489096053143669 ) ) ;
#47042=CARTESIAN_POINT ( 'NONE',  ( 16.51473224551083163, -9.474510206698727899, 105.8344237280190043 ) ) ;
#47044=CARTESIAN_POINT ( 'NONE',  ( -0.05219959533937732626, 21.53943276465977519, 27.50109039468567929 ) ) ;
#47045=CARTESIAN_POINT ( 'NONE',  ( -0.05219959533936034679, 19.03943276465977164, 72.50109039468566152 ) ) ;
#47046=CARTESIAN_POINT ( 'NONE',  ( 16.55341960407611168, 4.379528057220329451, 28.95724293864769905 ) ) ;
#47047=CARTESIAN_POINT ( 'NONE',  ( -21.53943276465977519, 0.05219959533907696930, 91.24890960531436690 ) ) ;
#47048=CARTESIAN_POINT ( 'NONE',  ( -5.049401038298153566, 19.05341960407611168, 110.2072429386476671 ) ) ;
#47049=CARTESIAN_POINT ( 'NONE',  ( 0.05219959533910956823, 16.53943276465976808, 64.99890960531435269 ) ) ;
#47050=CARTESIAN_POINT ( 'NONE',  ( 13.89961937509977652, -13.97604488694527269, 23.12390960531436335 ) ) ;
#47051=CARTESIAN_POINT ( 'NONE',  ( -19.05341960407617563, 5.049401038297882671, 23.54275706135233648 ) ) ;
#47052=CARTESIAN_POINT ( 'NONE',  ( 4.483927247898790824, -16.52544592524335698, 85.20942372801901854 ) ) ;
#47053=CARTESIAN_POINT ( 'NONE',  ( 0.05219959533934541429, -16.53943276465976808, 60.00109039468568284 ) ) ;
#47054=CARTESIAN_POINT ( 'NONE',  ( 10.72451020669898902, -18.67979575497178502, 22.91557627198102765 ) ) ;
#47055=CARTESIAN_POINT ( 'NONE',  ( -21.55341960407619339, 5.719274019375674811, 108.5427570613523756 ) ) ;
#47056=CARTESIAN_POINT ( 'NONE',  ( 9.474510206698971260, -16.51473224551069308, 72.91557627198102409 ) ) ;
#47057=CARTESIAN_POINT ( 'NONE',  ( 16.55341960407618274, -4.379528057220086978, 56.04275706135235424 ) ) ;
#47058=CARTESIAN_POINT ( 'NONE',  ( 5.049401038298161559, -19.05341960407611168, 27.70724293864769550 ) ) ;
#47059=CARTESIAN_POINT ( 'NONE',  ( -12.06949235617756955, 12.14591786802309770, 40.62390960531435269 ) ) ;
#47060=CARTESIAN_POINT ( 'NONE',  ( -17.49999999999999289, 5.500000000000032863, 70.79690382534172954 ) ) ;
#47061=CARTESIAN_POINT ( 'NONE',  ( -9.564922557960796823, -16.46253265017161027, 102.0822429386477097 ) ) ;
#47062=CARTESIAN_POINT ( 'NONE',  ( 16.51473224551069308, 9.474510206698969483, 74.16557627198103830 ) ) ;
#47063=CARTESIAN_POINT ( 'NONE',  ( -16.46253265017160317, 9.564922557960807481, 110.8322429386476955 ) ) ;
#47064=CARTESIAN_POINT ( 'NONE',  ( -16.52544592524342804, 4.483927247898546575, 56.04057627198102409 ) ) ;
#47065=CARTESIAN_POINT ( 'NONE',  ( -8.224510206698948167, 14.34966873604960824, 35.41557627198102409 ) ) ;
#47066=CARTESIAN_POINT ( 'NONE',  ( 0.05219959533910956823, 16.53943276465976808, 49.99890960531437401 ) ) ;
#47067=CARTESIAN_POINT ( 'NONE',  ( 8.314922557961029526, -14.29746914071037800, 45.41775706135234003 ) ) ;
#47068=CARTESIAN_POINT ( 'NONE',  ( -18.09918380851992481, -5.500000000000040856, 56.48618307335612343 ) ) ;
#47069=CARTESIAN_POINT ( 'NONE',  ( -0.05219959533936034679, 19.03943276465977164, 52.50109039468566863 ) ) ;
#47070=CARTESIAN_POINT ( 'NONE',  ( -16.46253265017160317, 9.564922557960807481, 70.83224293864770971 ) ) ;
#47071=CARTESIAN_POINT ( 'NONE',  ( -19.02544592524334988, -5.153800228976617603, 48.95942372801900433 ) ) ;
#47072=CARTESIAN_POINT ( 'NONE',  ( 19.03943276465977164, 0.05219959533936151252, 56.25109039468566863 ) ) ;
#47073=CARTESIAN_POINT ( 'NONE',  ( -13.89961937509957401, -13.97604488694547875, 94.37609039468566152 ) ) ;
#47074=CARTESIAN_POINT ( 'NONE',  ( -14.34966873604972548, 8.224510206698743886, 88.33442372801901854 ) ) ;
#47076=CARTESIAN_POINT ( 'NONE',  ( 16.51473224551069308, 9.474510206698969483, 24.16557627198102765 ) ) ;
#47077=CARTESIAN_POINT ( 'NONE',  ( -0.05219959533909027116, -19.03943276465977164, 107.4989096053143527 ) ) ;
#47078=CARTESIAN_POINT ( 'NONE',  ( 10.72451020669871369, 18.67979575497193778, 47.08442372801901854 ) ) ;
#47079=CARTESIAN_POINT ( 'NONE',  ( 19.02544592524334988, 5.153800228976608722, 106.4594237280190185 ) ) ;
#47080=CARTESIAN_POINT ( 'NONE',  ( 17.50000000000002132, -4.049696124445863354, 106.6803967066595078 ) ) ;
#47081=CARTESIAN_POINT ( 'NONE',  ( -13.97604488694527625, -13.89961937509977652, 61.87390960531435979 ) ) ;
#47082=CARTESIAN_POINT ( 'NONE',  ( -13.89961937509977652, 13.97604488694528158, 100.6239096053143669 ) ) ;
#47083=CARTESIAN_POINT ( 'NONE',  ( 16.55341960407611168, 4.379528057220329451, 58.95724293864770971 ) ) ;
#47084=CARTESIAN_POINT ( 'NONE',  ( 9.474510206698971260, -16.51473224551069308, 62.91557627198102409 ) ) ;
#47085=CARTESIAN_POINT ( 'NONE',  ( 5.049401038298161559, -19.05341960407611168, 57.70724293864769550 ) ) ;
#47086=CARTESIAN_POINT ( 'NONE',  ( -9.564922557961040184, 16.46253265017147172, 77.91775706135234714 ) ) ;
#47087=CARTESIAN_POINT ( 'NONE',  ( 5.719274019375991003, -21.55341960407610458, 52.70724293864769550 ) ) ;
#47088=CARTESIAN_POINT ( 'NONE',  ( -19.03943276465977164, -0.05219959533935918106, 38.75109039468566152 ) ) ;
#47089=CARTESIAN_POINT ( 'NONE',  ( 19.03943276465977164, -0.05219959533909143690, 83.74890960531436690 ) ) ;
#47090=CARTESIAN_POINT ( 'NONE',  ( 10.81492255796078972, 18.62759615963270932, 79.58224293864769550 ) ) ;
#47091=CARTESIAN_POINT ( 'NONE',  ( 8.224510206698953496, -14.34966873604960469, 77.91557627198102409 ) ) ;
#47092=CARTESIAN_POINT ( 'NONE',  ( 19.03943276465977164, 0.05219959533936151252, 31.25109039468566863 ) ) ;
#47093=CARTESIAN_POINT ( 'NONE',  ( 21.53943276465977519, -0.05219959533907433946, 63.74890960531435979 ) ) ;
#47095=CARTESIAN_POINT ( 'NONE',  ( -15.72974639402197994, 15.80617190586746368, 40.62390960531435269 ) ) ;
#47096=CARTESIAN_POINT ( 'NONE',  ( 5.049401038298161559, -19.05341960407611168, 67.70724293864769550 ) ) ;
#47097=CARTESIAN_POINT ( 'NONE',  ( -16.52544592524342804, 4.483927247898546575, 111.0405762719810525 ) ) ;
#47098=CARTESIAN_POINT ( 'NONE',  ( 5.719274019375673035, 21.55341960407619339, 32.29275706135235424 ) ) ;
#47099=CARTESIAN_POINT ( 'NONE',  ( 9.564922557960805705, 16.46253265017160317, 114.5822429386476955 ) ) ;
#47100=CARTESIAN_POINT ( 'NONE',  ( 21.53943276465977519, 0.05219959533937863772, 41.25109039468568284 ) ) ;
#47101=CARTESIAN_POINT ( 'NONE',  ( -19.02544592524342804, 5.153800228976336051, 31.04057627198102409 ) ) ;
#47102=CARTESIAN_POINT ( 'NONE',  ( -21.55341960407610458, -5.719274019375992779, 111.4572429386476813 ) ) ;
#47104=CARTESIAN_POINT ( 'NONE',  ( -9.564922557961040184, 16.46253265017147172, 42.91775706135234003 ) ) ;
#47106=CARTESIAN_POINT ( 'NONE',  ( -16.51473224551069308, -9.474510206698971260, 26.66557627198103120 ) ) ;
#47108=CARTESIAN_POINT ( 'NONE',  ( 16.55341960407618274, -4.379528057220086978, 56.04275706135235424 ) ) ;
#47109=CARTESIAN_POINT ( 'NONE',  ( -13.89961937509977652, 13.97604488694528158, 30.62390960531435269 ) ) ;
#47111=CARTESIAN_POINT ( 'NONE',  ( 0.05219959533909260263, 19.03943276465977164, 74.99890960531435269 ) ) ;
#47112=CARTESIAN_POINT ( 'NONE',  ( 4.483927247898545687, 16.52544592524342804, 109.7905762719810383 ) ) ;
#47113=CARTESIAN_POINT ( 'NONE',  ( 18.67979575497178502, 10.72451020669898547, 59.16557627198103120 ) ) ;
#47114=CARTESIAN_POINT ( 'NONE',  ( 12.14591786802309770, 12.06949235617756955, 84.37390960531438111 ) ) ;
#47115=CARTESIAN_POINT ( 'NONE',  ( 12.06949235617739724, 12.14591786802326823, 31.87609039468567929 ) ) ;
#47116=CARTESIAN_POINT ( 'NONE',  ( -10.81492255796105439, 18.62759615963255655, 92.91775706135236135 ) ) ;
#47117=CARTESIAN_POINT ( 'NONE',  ( -16.51473224551069308, -9.474510206698971260, 21.66557627198102765 ) ) ;
#47119=CARTESIAN_POINT ( 'NONE',  ( 14.34966873604972726, -8.224510206698740333, 105.8344237280190328 ) ) ;
#47120=CARTESIAN_POINT ( 'NONE',  ( 16.52544592524342804, -4.483927247898539470, 53.54057627198103120 ) ) ;
#47121=CARTESIAN_POINT ( 'NONE',  ( 9.474510206698971260, -16.51473224551069308, 52.91557627198102409 ) ) ;
#47122=CARTESIAN_POINT ( 'NONE',  ( 21.55341960407619695, -5.719274019375665929, 91.04275706135236135 ) ) ;
#47123=CARTESIAN_POINT ( 'NONE',  ( 0.05219959533907565091, 21.53943276465977519, 104.9989096053143669 ) ) ;
#47124=CARTESIAN_POINT ( 'NONE',  ( -21.55341960407619339, 5.719274019375674811, 73.54275706135234714 ) ) ;
#47125=CARTESIAN_POINT ( 'NONE',  ( -12.14591786802326823, 12.06949235617739902, 48.12609039468568284 ) ) ;
#47126=CARTESIAN_POINT ( 'NONE',  ( 16.52544592524342804, -4.483927247898539470, 78.54057627198103830 ) ) ;
#47127=CARTESIAN_POINT ( 'NONE',  ( 18.67979575497194134, -10.72451020669871369, 85.83442372801901854 ) ) ;
#47128=CARTESIAN_POINT ( 'NONE',  ( -14.34966873604972548, 8.224510206698743886, 108.3344237280190185 ) ) ;
#47129=CARTESIAN_POINT ( 'NONE',  ( -17.05116617787822975, 6.768360034955819948, 113.6567555325920296 ) ) ;
#47130=CARTESIAN_POINT ( 'NONE',  ( -16.53943276465976808, -0.05219959533934237506, 43.75109039468568284 ) ) ;
#47131=CARTESIAN_POINT ( 'NONE',  ( 8.314922557960818139, 14.29746914071049879, 44.58224293864769550 ) ) ;
#47132=CARTESIAN_POINT ( 'NONE',  ( -8.314922557961024197, 14.29746914071037800, 82.91775706135234714 ) ) ;
#47133=CARTESIAN_POINT ( 'NONE',  ( -0.05219959533909027116, -19.03943276465977164, 102.4989096053143669 ) ) ;
#47134=CARTESIAN_POINT ( 'NONE',  ( -19.03943276465977164, 0.05219959533909376836, 116.2489096053143669 ) ) ;
#47135=CARTESIAN_POINT ( 'NONE',  ( -0.05219959533937732626, 21.53943276465977519, 97.50109039468567573 ) ) ;
#47136=CARTESIAN_POINT ( 'NONE',  ( 12.06949235617739724, 12.14591786802326823, 96.87609039468568994 ) ) ;
#47137=CARTESIAN_POINT ( 'NONE',  ( -8.224510206698948167, 14.34966873604960824, 75.41557627198102409 ) ) ;
#47138=CARTESIAN_POINT ( 'NONE',  ( -19.02544592524342804, 5.153800228976336051, 86.04057627198103830 ) ) ;
#47139=VERTEX_POINT ( 'NONE', #145984 ) ;
#47140=CARTESIAN_POINT ( 'NONE',  ( 16.52544592524335698, 4.483927247898782831, 21.45942372801901499 ) ) ;
#47141=CARTESIAN_POINT ( 'NONE',  ( -19.03943276465977164, 0.05219959533909376836, 31.24890960531435979 ) ) ;
#47142=CARTESIAN_POINT ( 'NONE',  ( -0.05219959533909027116, -19.03943276465977164, 87.49890960531436690 ) ) ;
#47143=CARTESIAN_POINT ( 'NONE',  ( -16.52544592524335698, -4.483927247898792601, 28.95942372801902209 ) ) ;
#47145=CARTESIAN_POINT ( 'NONE',  ( -9.564922557961040184, 16.46253265017147172, 32.91775706135233293 ) ) ;
#47146=CARTESIAN_POINT ( 'NONE',  ( -12.14591786802326823, 12.06949235617739902, 88.12609039468570415 ) ) ;
#47147=CARTESIAN_POINT ( 'NONE',  ( -16.51473224551069308, -9.474510206698971260, 31.66557627198102054 ) ) ;
#47148=CARTESIAN_POINT ( 'NONE',  ( -4.379528057220086978, -16.55341960407618274, 74.79275706135234714 ) ) ;
#47149=CARTESIAN_POINT ( 'NONE',  ( -16.53943276465976808, -0.05219959533934237506, 68.75109039468568994 ) ) ;
#47150=CARTESIAN_POINT ( 'NONE',  ( -19.05341960407617563, 5.049401038297882671, 78.54275706135233293 ) ) ;
#47151=CARTESIAN_POINT ( 'NONE',  ( -10.81492255796105439, 18.62759615963255655, 112.9177570613523329 ) ) ;
#47152=CARTESIAN_POINT ( 'NONE',  ( -5.153800228976328057, -19.02544592524343514, 52.29057627198100988 ) ) ;
#47153=CARTESIAN_POINT ( 'NONE',  ( -5.049401038298153566, 19.05341960407611168, 90.20724293864766707 ) ) ;
#47154=CARTESIAN_POINT ( 'NONE',  ( -4.379528057220328563, 16.55341960407611168, 90.20724293864770971 ) ) ;
#47155=CARTESIAN_POINT ( 'NONE',  ( -5.049401038297874678, -19.05341960407617918, 49.79275706135231871 ) ) ;
#47156=CARTESIAN_POINT ( 'NONE',  ( 0.05219959533907565091, 21.53943276465977519, 44.99890960531435979 ) ) ;
#47157=CARTESIAN_POINT ( 'NONE',  ( -19.05341960407617563, 5.049401038297882671, 33.54275706135231871 ) ) ;
#47158=CARTESIAN_POINT ( 'NONE',  ( 0.05219959533909260263, 19.03943276465977164, 99.99890960531436690 ) ) ;
#47159=CARTESIAN_POINT ( 'NONE',  ( -15.72974639402197994, 15.80617190586746368, 75.62390960531439532 ) ) ;
#47160=CARTESIAN_POINT ( 'NONE',  ( -5.153800228976328057, -19.02544592524343514, 112.2905762719810099 ) ) ;
#47161=CARTESIAN_POINT ( 'NONE',  ( -19.05341960407617563, 5.049401038297882671, 93.54275706135234714 ) ) ;
#47162=CARTESIAN_POINT ( 'NONE',  ( -17.50000000000014566, 3.292511757969728947, 110.0652027021053243 ) ) ;
#47163=CARTESIAN_POINT ( 'NONE',  ( -19.03943276465977164, -0.05219959533935918106, 108.7510903946856615 ) ) ;
#47164=CARTESIAN_POINT ( 'NONE',  ( 0.05219959533909260263, 19.03943276465977164, 29.99890960531435979 ) ) ;
#47165=CARTESIAN_POINT ( 'NONE',  ( -0.05219959533909027116, -19.03943276465977164, 97.49890960531436690 ) ) ;
#47166=CARTESIAN_POINT ( 'NONE',  ( 15.80617190586746368, 15.72974639402197994, 74.37390960531436690 ) ) ;
#47167=CARTESIAN_POINT ( 'NONE',  ( 8.224510206698742110, 14.34966873604972548, 47.08442372801901854 ) ) ;
#47168=CARTESIAN_POINT ( 'NONE',  ( 10.81492255796106328, -18.62759615963255655, 50.41775706135235424 ) ) ;
#47169=CARTESIAN_POINT ( 'NONE',  ( 13.97604488694548053, -13.89961937509957401, 90.62609039468567573 ) ) ;
#47170=CARTESIAN_POINT ( 'NONE',  ( -21.53943276465977519, -0.05219959533937600094, 103.7510903946857042 ) ) ;
#47171=CARTESIAN_POINT ( 'NONE',  ( 4.379528057220092307, 16.55341960407617563, 112.2927570613523471 ) ) ;
#47172=CARTESIAN_POINT ( 'NONE',  ( 16.51473224551069308, 9.474510206698969483, 99.16557627198102409 ) ) ;
#47173=CARTESIAN_POINT ( 'NONE',  ( 8.314922557960818139, 14.29746914071049879, 94.58224293864769550 ) ) ;
#47174=CARTESIAN_POINT ( 'NONE',  ( -8.224510206698948167, 14.34966873604960824, 40.41557627198103120 ) ) ;
#47175=CARTESIAN_POINT ( 'NONE',  ( 0.05219959533936267826, -19.03943276465977164, 70.00109039468566152 ) ) ;
#47176=CARTESIAN_POINT ( 'NONE',  ( 5.823673210054444382, -21.52544592524334988, 60.20942372801902565 ) ) ;
#47177=CARTESIAN_POINT ( 'NONE',  ( -13.97604488694547697, 13.89961937509957934, 23.12609039468565442 ) ) ;
#47178=CARTESIAN_POINT ( 'NONE',  ( 4.483927247898545687, 16.52544592524342804, 109.7905762719810383 ) ) ;
#47179=CARTESIAN_POINT ( 'NONE',  ( -21.52544592524343514, 5.823673210054127303, 31.04057627198102409 ) ) ;
#47180=CARTESIAN_POINT ( 'NONE',  ( 12.06949235617739724, 12.14591786802326823, 111.8760903946856615 ) ) ;
#47181=CARTESIAN_POINT ( 'NONE',  ( -10.72451020669870658, -18.67979575497194134, 99.58442372801900433 ) ) ;
#47182=CARTESIAN_POINT ( 'NONE',  ( -12.06949235617739369, -12.14591786802326823, 54.37609039468568994 ) ) ;
#47183=CARTESIAN_POINT ( 'NONE',  ( -16.53943276465976808, 0.05219959533911058130, 26.24890960531435624 ) ) ;
#47184=CARTESIAN_POINT ( 'NONE',  ( 18.67979575497194134, -10.72451020669871369, 65.83442372801900433 ) ) ;
#47185=CARTESIAN_POINT ( 'NONE',  ( -21.55341960407619339, 5.719274019375674811, 58.54275706135235424 ) ) ;
#47186=CARTESIAN_POINT ( 'NONE',  ( 9.564922557960805705, 16.46253265017160317, 29.58224293864769550 ) ) ;
#47187=CARTESIAN_POINT ( 'NONE',  ( -18.62759615963255300, -10.81492255796106328, 24.16775706135235424 ) ) ;
#47188=CARTESIAN_POINT ( 'NONE',  ( -8.224510206698948167, 14.34966873604960824, 100.4155762719810241 ) ) ;
#47189=CARTESIAN_POINT ( 'NONE',  ( 13.89961937509977652, -13.97604488694527269, 28.12390960531435624 ) ) ;
#47190=CARTESIAN_POINT ( 'NONE',  ( -16.53943276465976808, 0.05219959533911058130, 81.24890960531436690 ) ) ;
#47191=CARTESIAN_POINT ( 'NONE',  ( -5.153800228976328057, -19.02544592524343514, 67.29057627198102409 ) ) ;
#47192=CARTESIAN_POINT ( 'NONE',  ( 8.224510206698953496, -14.34966873604960469, 22.91557627198102765 ) ) ;
#47193=CARTESIAN_POINT ( 'NONE',  ( 18.67979575497178502, 10.72451020669898547, 54.16557627198103120 ) ) ;
#47194=CARTESIAN_POINT ( 'NONE',  ( -16.55341960407611168, -4.379528057220339221, 91.45724293864769550 ) ) ;
#47196=CARTESIAN_POINT ( 'NONE',  ( -21.55341960407610458, -5.719274019375992779, 96.45724293864770971 ) ) ;
#47197=CARTESIAN_POINT ( 'NONE',  ( 19.02544592524343514, -5.153800228976328945, 98.54057627198100988 ) ) ;
#47198=CARTESIAN_POINT ( 'NONE',  ( 16.46253265017160672, -9.564922557960803928, 58.33224293864769550 ) ) ;
#47199=CARTESIAN_POINT ( 'NONE',  ( -13.97604488694547697, 13.89961937509957934, 108.1260903946856331 ) ) ;
#47200=CARTESIAN_POINT ( 'NONE',  ( -5.719274019375978568, 21.55341960407610458, 40.20724293864769550 ) ) ;
#47201=CARTESIAN_POINT ( 'NONE',  ( -10.81492255796105439, 18.62759615963255655, 87.91775706135234714 ) ) ;
#47202=CARTESIAN_POINT ( 'NONE',  ( -0.05219959533909027116, -19.03943276465977164, 67.49890960531436690 ) ) ;
#47203=EDGE_CURVE ( 'NONE', #111651, #194969, #33125, .T. ) ;
#47204=CARTESIAN_POINT ( 'NONE',  ( -5.049401038298153566, 19.05341960407611168, 105.2072429386476671 ) ) ;
#47205=CARTESIAN_POINT ( 'NONE',  ( -12.06949235617739369, -12.14591786802326823, 74.37609039468568994 ) ) ;
#47206=CARTESIAN_POINT ( 'NONE',  ( -18.67979575497193778, 10.72451020669871902, 63.33442372801900433 ) ) ;
#47207=CARTESIAN_POINT ( 'NONE',  ( 5.719274019375673035, 21.55341960407619339, 92.29275706135236135 ) ) ;
#47208=CARTESIAN_POINT ( 'NONE',  ( -15.72974639402197994, 15.80617190586746368, 95.62390960531436690 ) ) ;
#47209=CARTESIAN_POINT ( 'NONE',  ( -5.823673210054431948, 21.52544592524334988, 37.70942372801900433 ) ) ;
#47210=CARTESIAN_POINT ( 'NONE',  ( -4.379528057220086978, -16.55341960407618274, 74.79275706135234714 ) ) ;
#47211=CARTESIAN_POINT ( 'NONE',  ( -21.52544592524343514, 5.823673210054127303, 76.04057627198102409 ) ) ;
#47212=CARTESIAN_POINT ( 'NONE',  ( 13.89961937509957401, 13.97604488694547697, 31.87609039468566863 ) ) ;
#47213=CARTESIAN_POINT ( 'NONE',  ( 10.81492255796078972, 18.62759615963270932, 44.58224293864769550 ) ) ;
#47214=CARTESIAN_POINT ( 'NONE',  ( 9.474510206698971260, -16.51473224551069308, 82.91557627198103830 ) ) ;
#47215=CARTESIAN_POINT ( 'NONE',  ( 14.34966873604960469, 8.224510206698951720, 24.16557627198103120 ) ) ;
#47216=CARTESIAN_POINT ( 'NONE',  ( -16.18388926212242396, 7.379444403734377822, 64.56046848633850743 ) ) ;
#47217=CARTESIAN_POINT ( 'NONE',  ( -16.46253265017160317, 9.564922557960807481, 105.8322429386476955 ) ) ;
#47219=CARTESIAN_POINT ( 'NONE',  ( -16.46253265017146816, -9.564922557961047289, 94.16775706135233293 ) ) ;
#47220=CARTESIAN_POINT ( 'NONE',  ( 21.52544592524344225, -5.823673210054117533, 73.54057627198102409 ) ) ;
#47221=CARTESIAN_POINT ( 'NONE',  ( 12.06949235617757843, -12.14591786802309237, 43.12390960531435269 ) ) ;
#47222=CARTESIAN_POINT ( 'NONE',  ( -13.97604488694547697, 13.89961937509957934, 108.1260903946856331 ) ) ;
#47223=CARTESIAN_POINT ( 'NONE',  ( -5.153800228976328057, -19.02544592524343514, 37.29057627198102409 ) ) ;
#47224=CARTESIAN_POINT ( 'NONE',  ( 9.564922557961047289, -16.46253265017146816, 105.4177570613523471 ) ) ;
#47225=CARTESIAN_POINT ( 'NONE',  ( -18.67979575497178146, -10.72451020669898902, 106.6655762719810383 ) ) ;
#47226=CARTESIAN_POINT ( 'NONE',  ( -13.97604488694547697, 13.89961937509957934, 73.12609039468568994 ) ) ;
#47227=CARTESIAN_POINT ( 'NONE',  ( -14.34966873604972548, 8.224510206698743886, 83.33442372801903275 ) ) ;
#47228=CARTESIAN_POINT ( 'NONE',  ( 19.05341960407611168, 5.049401038298154454, 68.95724293864769550 ) ) ;
#47229=CARTESIAN_POINT ( 'NONE',  ( -16.55341960407611168, -4.379528057220339221, 76.45724293864769550 ) ) ;
#47230=CARTESIAN_POINT ( 'NONE',  ( -9.564922557960796823, -16.46253265017161027, 67.08224293864769550 ) ) ;
#47231=CARTESIAN_POINT ( 'NONE',  ( -14.29746914071049879, 8.314922557960819915, 65.83224293864769550 ) ) ;
#47232=CARTESIAN_POINT ( 'NONE',  ( 19.02544592524343514, -5.153800228976328945, 23.54057627198102054 ) ) ;
#47234=CARTESIAN_POINT ( 'NONE',  ( -12.06949235617756955, 12.14591786802309770, 45.62390960531436690 ) ) ;
#47235=CARTESIAN_POINT ( 'NONE',  ( -9.564922557960796823, -16.46253265017161027, 82.08224293864768129 ) ) ;
#47237=CARTESIAN_POINT ( 'NONE',  ( 13.97604488694548053, -13.89961937509957401, 45.62609039468566863 ) ) ;
#47238=CARTESIAN_POINT ( 'NONE',  ( 16.53943276465976808, 0.05219959533934440121, 66.25109039468567573 ) ) ;
#47240=CARTESIAN_POINT ( 'NONE',  ( 0.05219959533907565091, 21.53943276465977519, 64.99890960531435269 ) ) ;
#47241=CARTESIAN_POINT ( 'NONE',  ( 0.05219959533936267826, -19.03943276465977164, 20.00109039468567218 ) ) ;
#47242=CARTESIAN_POINT ( 'NONE',  ( -16.51473224551069308, -9.474510206698971260, 91.66557627198103830 ) ) ;
#47244=CARTESIAN_POINT ( 'NONE',  ( 18.62759615963271287, -10.81492255796078972, 33.33224293864769550 ) ) ;
#47245=CARTESIAN_POINT ( 'NONE',  ( 5.153800228976335163, 19.02544592524342804, 64.79057627198100988 ) ) ;
#47246=CARTESIAN_POINT ( 'NONE',  ( -21.55341960407619339, 5.719274019375674811, 33.54275706135234714 ) ) ;
#47248=CARTESIAN_POINT ( 'NONE',  ( 12.14591786802309770, 12.06949235617756955, 109.3739096053143811 ) ) ;
#47249=CARTESIAN_POINT ( 'NONE',  ( -15.80617190586745835, -15.72974639402198527, 101.8739096053143811 ) ) ;
#47250=CARTESIAN_POINT ( 'NONE',  ( 5.049401038298161559, -19.05341960407611168, 97.70724293864766707 ) ) ;
#47252=CARTESIAN_POINT ( 'NONE',  ( 15.80617190586769283, -15.72974639402175789, 30.62609039468567929 ) ) ;
#47253=VERTEX_POINT ( 'NONE', #23659 ) ;
#47254=CARTESIAN_POINT ( 'NONE',  ( 13.97604488694527802, 13.89961937509977652, 89.37390960531436690 ) ) ;
#47255=CARTESIAN_POINT ( 'NONE',  ( 18.87580814761074777, -5.500000000000045297, 83.37172394265758157 ) ) ;
#47256=CARTESIAN_POINT ( 'NONE',  ( -21.53943276465977519, 0.05219959533907696930, 91.24890960531436690 ) ) ;
#47257=CARTESIAN_POINT ( 'NONE',  ( -0.05219959533909027116, -19.03943276465977164, 47.49890960531435979 ) ) ;
#47258=CARTESIAN_POINT ( 'NONE',  ( -5.153800228976607833, 19.02544592524334988, 112.7094237280190043 ) ) ;
#47260=CARTESIAN_POINT ( 'NONE',  ( 19.05341960407611168, 5.049401038298154454, 33.95724293864769550 ) ) ;
#47261=CARTESIAN_POINT ( 'NONE',  ( 15.72974639402176855, 15.80617190586768217, 81.87609039468568994 ) ) ;
#47262=CARTESIAN_POINT ( 'NONE',  ( -19.03943276465977164, 0.05219959533909376836, 76.24890960531435269 ) ) ;
#47263=CARTESIAN_POINT ( 'NONE',  ( 10.72451020669871369, 18.67979575497193778, 42.08442372801901854 ) ) ;
#47264=CARTESIAN_POINT ( 'NONE',  ( -15.80617190586768217, 15.72974639402176855, 23.12609039468567573 ) ) ;
#47266=CARTESIAN_POINT ( 'NONE',  ( 5.049401038298161559, -19.05341960407611168, 97.70724293864766707 ) ) ;
#47267=CARTESIAN_POINT ( 'NONE',  ( 19.19724070472091526, 5.500000000000158096, 63.56193348274384647 ) ) ;
#47268=CARTESIAN_POINT ( 'NONE',  ( -4.379528057220086978, -16.55341960407618274, 34.79275706135235424 ) ) ;
#47269=CARTESIAN_POINT ( 'NONE',  ( 4.483927247898790824, -16.52544592524335698, 70.20942372801904696 ) ) ;
#47270=CARTESIAN_POINT ( 'NONE',  ( 10.72451020669871369, 18.67979575497193778, 42.08442372801901854 ) ) ;
#47271=CARTESIAN_POINT ( 'NONE',  ( 21.52544592524334988, 5.823673210054432836, 81.45942372801900433 ) ) ;
#47273=CARTESIAN_POINT ( 'NONE',  ( 5.153800228976615827, -19.02544592524334988, 110.2094237280189901 ) ) ;
#47274=CARTESIAN_POINT ( 'NONE',  ( 19.03943276465977164, -0.05219959533909143690, 58.74890960531435979 ) ) ;
#47275=CARTESIAN_POINT ( 'NONE',  ( 19.05341960407611168, 5.049401038298154454, 103.9572429386476671 ) ) ;
#47277=CARTESIAN_POINT ( 'NONE',  ( -8.224510206698948167, 14.34966873604960824, 110.4155762719810383 ) ) ;
#47278=CARTESIAN_POINT ( 'NONE',  ( 16.53943276465976808, -0.05219959533910856209, 108.7489096053143669 ) ) ;
#47279=CARTESIAN_POINT ( 'NONE',  ( 18.62759615963271287, -10.81492255796078972, 28.33224293864769550 ) ) ;
#47280=CARTESIAN_POINT ( 'NONE',  ( 12.14591786802327356, -12.06949235617739191, 80.62609039468567573 ) ) ;
#47281=CARTESIAN_POINT ( 'NONE',  ( -8.314922557960811034, -14.29746914071050412, 67.08224293864770971 ) ) ;
#47282=CARTESIAN_POINT ( 'NONE',  ( -13.97604488694527625, -13.89961937509977652, 56.87390960531434558 ) ) ;
#47283=CARTESIAN_POINT ( 'NONE',  ( 10.72451020669871369, 18.67979575497193778, 72.08442372801899012 ) ) ;
#47284=CARTESIAN_POINT ( 'NONE',  ( 18.62759615963255655, 10.81492255796105972, 66.66775706135234714 ) ) ;
#47285=CARTESIAN_POINT ( 'NONE',  ( -19.05341960407617563, 5.049401038297882671, 103.5427570613523329 ) ) ;
#47286=CARTESIAN_POINT ( 'NONE',  ( -8.314922557960811034, -14.29746914071050412, 72.08224293864769550 ) ) ;
#47287=CARTESIAN_POINT ( 'NONE',  ( 21.52544592524334988, 5.823673210054432836, 31.45942372801901854 ) ) ;
#47288=CARTESIAN_POINT ( 'NONE',  ( -5.823673210054116645, -21.52544592524344225, 57.29057627198103120 ) ) ;
#47291=CARTESIAN_POINT ( 'NONE',  ( -16.51473224551069308, -9.474510206698971260, 66.66557627198102409 ) ) ;
#47292=CARTESIAN_POINT ( 'NONE',  ( -16.52544592524342804, 4.483927247898546575, 46.04057627198103830 ) ) ;
#47293=CARTESIAN_POINT ( 'NONE',  ( 16.52544592524335698, 4.483927247898782831, 111.4594237280190328 ) ) ;
#47294=CARTESIAN_POINT ( 'NONE',  ( -16.52544592524335698, -4.483927247898792601, 98.95942372801903275 ) ) ;
#47295=CARTESIAN_POINT ( 'NONE',  ( -13.97604488694547697, 13.89961937509957934, 53.12609039468565442 ) ) ;
#47296=CARTESIAN_POINT ( 'NONE',  ( 17.40861289039005300, 6.110651285853281323, 48.87232470827434128 ) ) ;
#47297=CARTESIAN_POINT ( 'NONE',  ( -0.05219959533909027116, -19.03943276465977164, 102.4989096053143669 ) ) ;
#47299=CARTESIAN_POINT ( 'NONE',  ( -16.52544592524342804, 4.483927247898546575, 81.04057627198102409 ) ) ;
#47300=CARTESIAN_POINT ( 'NONE',  ( -9.474510206698720793, -16.51473224551083518, 49.58442372801899722 ) ) ;
#47301=CARTESIAN_POINT ( 'NONE',  ( 19.03943276465977164, -0.05219959533909143690, 38.74890960531436690 ) ) ;
#47302=CARTESIAN_POINT ( 'NONE',  ( 15.72974639402199770, -15.80617190586745480, 33.12390960531435979 ) ) ;
#47303=CARTESIAN_POINT ( 'NONE',  ( 21.53943276465977519, -0.05219959533907433946, 58.74890960531436690 ) ) ;
#47304=ORIENTED_EDGE ( 'NONE', *, *, #5230, .F. ) ;
#47305=CARTESIAN_POINT ( 'NONE',  ( 4.379528057220339221, -16.55341960407611168, 92.70724293864770971 ) ) ;
#47306=CARTESIAN_POINT ( 'NONE',  ( -12.14591786802326823, 12.06949235617739902, 53.12609039468568284 ) ) ;
#47307=CARTESIAN_POINT ( 'NONE',  ( 12.06949235617757843, -12.14591786802309237, 88.12390960531436690 ) ) ;
#47309=CARTESIAN_POINT ( 'NONE',  ( -17.48847506799968698, 5.747544572773789717, 50.82697437843282273 ) ) ;
#47310=CARTESIAN_POINT ( 'NONE',  ( -19.02544592524342804, 5.153800228976336051, 111.0405762719810099 ) ) ;
#47311=CARTESIAN_POINT ( 'NONE',  ( 17.60728821186566151, -5.500000000000016875, 78.36690927743003954 ) ) ;
#47312=CARTESIAN_POINT ( 'NONE',  ( 18.22780087662122739, 5.500000000000000888, 86.48236817873107896 ) ) ;
#47314=CARTESIAN_POINT ( 'NONE',  ( -16.55341960407617563, 4.379528057220093196, 43.54275706135235424 ) ) ;
#47315=CARTESIAN_POINT ( 'NONE',  ( -8.314922557960811034, -14.29746914071050412, 32.08224293864769550 ) ) ;
#47316=CARTESIAN_POINT ( 'NONE',  ( -15.72974639402197994, 15.80617190586746368, 50.62390960531435979 ) ) ;
#47317=CARTESIAN_POINT ( 'NONE',  ( -19.05341960407617563, 5.049401038297882671, 88.54275706135230450 ) ) ;
#47318=CARTESIAN_POINT ( 'NONE',  ( 15.72974639402199770, -15.80617190586745480, 43.12390960531435269 ) ) ;
#47319=CARTESIAN_POINT ( 'NONE',  ( 21.52544592524334988, 5.823673210054432836, 81.45942372801900433 ) ) ;
#47321=CARTESIAN_POINT ( 'NONE',  ( 16.55341960407618274, -4.379528057220086978, 51.04275706135234714 ) ) ;
#47322=CARTESIAN_POINT ( 'NONE',  ( 19.05341960407611168, 5.049401038298154454, 38.95724293864767418 ) ) ;
#47323=CARTESIAN_POINT ( 'NONE',  ( -9.564922557960796823, -16.46253265017161027, 107.0822429386476955 ) ) ;
#47324=CARTESIAN_POINT ( 'NONE',  ( 5.153800228976335163, 19.02544592524342804, 34.79057627198102409 ) ) ;
#47325=CARTESIAN_POINT ( 'NONE',  ( -8.224510206698948167, 14.34966873604960824, 100.4155762719810241 ) ) ;
#47327=CARTESIAN_POINT ( 'NONE',  ( -9.474510206698964154, 16.51473224551069663, 105.4155762719810383 ) ) ;
#47329=CARTESIAN_POINT ( 'NONE',  ( -4.483927247898782831, 16.52544592524335698, 62.70942372801902565 ) ) ;
#47330=CARTESIAN_POINT ( 'NONE',  ( -18.62759615963270932, 10.81492255796079327, 90.83224293864769550 ) ) ;
#47331=CARTESIAN_POINT ( 'NONE',  ( -16.51473224551069308, -9.474510206698971260, 61.66557627198103120 ) ) ;
#47332=CARTESIAN_POINT ( 'NONE',  ( -0.05219959533937732626, 21.53943276465977519, 22.50109039468567573 ) ) ;
#47333=CARTESIAN_POINT ( 'NONE',  ( 9.474510206698971260, -16.51473224551069308, 82.91557627198103830 ) ) ;
#47335=ORIENTED_EDGE ( 'NONE', *, *, #26374, .T. ) ;
#47336=CARTESIAN_POINT ( 'NONE',  ( 10.81492255796078972, 18.62759615963270932, 114.5822429386477097 ) ) ;
#47337=CARTESIAN_POINT ( 'NONE',  ( 19.02544592524343514, -5.153800228976328945, 23.54057627198102054 ) ) ;
#47338=CARTESIAN_POINT ( 'NONE',  ( -16.51473224551069308, -9.474510206698971260, 111.6655762719810383 ) ) ;
#47339=CARTESIAN_POINT ( 'NONE',  ( -5.153800228976607833, 19.02544592524334988, 77.70942372801900433 ) ) ;
#47340=CARTESIAN_POINT ( 'NONE',  ( -16.46253265017146816, -9.564922557961047289, 29.16775706135232937 ) ) ;
#47341=CARTESIAN_POINT ( 'NONE',  ( 10.72451020669898902, -18.67979575497178502, 97.91557627198103830 ) ) ;
#47342=CARTESIAN_POINT ( 'NONE',  ( -19.02544592524334988, -5.153800228976617603, 38.95942372801900433 ) ) ;
#47343=CARTESIAN_POINT ( 'NONE',  ( -8.314922557961024197, 14.29746914071037800, 72.91775706135234714 ) ) ;
#47344=CARTESIAN_POINT ( 'NONE',  ( 9.474510206698971260, -16.51473224551069308, 107.9155762719810383 ) ) ;
#47345=CARTESIAN_POINT ( 'NONE',  ( -9.474510206698964154, 16.51473224551069663, 60.41557627198102409 ) ) ;
#47347=CARTESIAN_POINT ( 'NONE',  ( -15.80617190586768217, 15.72974639402176855, 68.12609039468567573 ) ) ;
#47348=CARTESIAN_POINT ( 'NONE',  ( -10.72451020669870658, -18.67979575497194134, 84.58442372801903275 ) ) ;
#47349=CARTESIAN_POINT ( 'NONE',  ( 19.03943276465977164, -0.05219959533909143690, 73.74890960531435269 ) ) ;
#47350=CARTESIAN_POINT ( 'NONE',  ( -18.62759615963255300, -10.81492255796106328, 49.16775706135234003 ) ) ;
#47352=CARTESIAN_POINT ( 'NONE',  ( -19.03943276465977164, -0.05219959533935918106, 88.75109039468567573 ) ) ;
#47353=CARTESIAN_POINT ( 'NONE',  ( 19.05341960407611168, 5.049401038298154454, 48.95724293864768129 ) ) ;
#47354=CARTESIAN_POINT ( 'NONE',  ( 16.51473224551069308, 9.474510206698969483, 99.16557627198102409 ) ) ;
#47355=CARTESIAN_POINT ( 'NONE',  ( -16.51473224551069308, -9.474510206698971260, 66.66557627198102409 ) ) ;
#47356=CARTESIAN_POINT ( 'NONE',  ( -5.153800228976328057, -19.02544592524343514, 107.2905762719810383 ) ) ;
#47357=CARTESIAN_POINT ( 'NONE',  ( 19.03943276465977164, -0.05219959533909143690, 48.74890960531435979 ) ) ;
#47358=CARTESIAN_POINT ( 'NONE',  ( -18.67979575497178146, -10.72451020669898902, 101.6655762719810383 ) ) ;
#47359=CARTESIAN_POINT ( 'NONE',  ( -16.52544592524335698, -4.483927247898792601, 78.95942372801901854 ) ) ;
#47361=CARTESIAN_POINT ( 'NONE',  ( -9.564922557961040184, 16.46253265017147172, 47.91775706135233293 ) ) ;
#47362=CARTESIAN_POINT ( 'NONE',  ( 19.02544592524343514, -5.153800228976328945, 63.54057627198103830 ) ) ;
#47363=CARTESIAN_POINT ( 'NONE',  ( -8.314922557960811034, -14.29746914071050412, 52.08224293864768839 ) ) ;
#47364=CARTESIAN_POINT ( 'NONE',  ( 16.55341960407611168, 4.379528057220329451, 88.95724293864769550 ) ) ;
#47365=CARTESIAN_POINT ( 'NONE',  ( -13.97604488694527625, -13.89961937509977652, 106.8739096053143669 ) ) ;
#47366=CARTESIAN_POINT ( 'NONE',  ( -9.474510206698964154, 16.51473224551069663, 85.41557627198102409 ) ) ;
#47367=CARTESIAN_POINT ( 'NONE',  ( -5.153800228976328057, -19.02544592524343514, 107.2905762719810383 ) ) ;
#47368=CARTESIAN_POINT ( 'NONE',  ( 21.52544592524334988, 5.823673210054432836, 106.4594237280190328 ) ) ;
#47369=CARTESIAN_POINT ( 'NONE',  ( 16.55341960407618274, -4.379528057220086978, 91.04275706135236135 ) ) ;
#47370=CARTESIAN_POINT ( 'NONE',  ( 16.46253265017160672, -9.564922557960803928, 73.33224293864769550 ) ) ;
#47371=CARTESIAN_POINT ( 'NONE',  ( 0.05219959533937995610, -21.53943276465977519, 45.00109039468568284 ) ) ;
#47372=CARTESIAN_POINT ( 'NONE',  ( 0.05219959533907565091, 21.53943276465977519, 29.99890960531435979 ) ) ;
#47373=CARTESIAN_POINT ( 'NONE',  ( 10.72451020669898902, -18.67979575497178502, 102.9155762719810383 ) ) ;
#47374=CARTESIAN_POINT ( 'NONE',  ( 12.06949235617757843, -12.14591786802309237, 58.12390960531435979 ) ) ;
#47375=CARTESIAN_POINT ( 'NONE',  ( -19.03943276465977164, 0.05219959533909376836, 61.24890960531436690 ) ) ;
#47376=CARTESIAN_POINT ( 'NONE',  ( -8.314922557960811034, -14.29746914071050412, 87.08224293864769550 ) ) ;
#47377=CARTESIAN_POINT ( 'NONE',  ( -9.564922557961040184, 16.46253265017147172, 47.91775706135233293 ) ) ;
#47378=CARTESIAN_POINT ( 'NONE',  ( 4.483927247898545687, 16.52544592524342804, 109.7905762719810383 ) ) ;
#47379=CARTESIAN_POINT ( 'NONE',  ( 4.379528057220092307, 16.55341960407617563, 72.29275706135236135 ) ) ;
#47380=CARTESIAN_POINT ( 'NONE',  ( -9.564922557960796823, -16.46253265017161027, 62.08224293864769550 ) ) ;
#47382=CARTESIAN_POINT ( 'NONE',  ( -4.483927247898539470, -16.52544592524342804, 92.29057627198103830 ) ) ;
#47383=CARTESIAN_POINT ( 'NONE',  ( 15.72974639402199770, -15.80617190586745480, 38.12390960531436690 ) ) ;
#47385=CARTESIAN_POINT ( 'NONE',  ( 12.14591786802327356, -12.06949235617739191, 100.6260903946857184 ) ) ;
#47386=CARTESIAN_POINT ( 'NONE',  ( 0.05219959533934541429, -16.53943276465976808, 30.00109039468568284 ) ) ;
#47387=CARTESIAN_POINT ( 'NONE',  ( 0.05219959533937995610, -21.53943276465977519, 95.00109039468568994 ) ) ;
#47388=CARTESIAN_POINT ( 'NONE',  ( 9.474510206698971260, -16.51473224551069308, 82.91557627198103830 ) ) ;
#47389=CARTESIAN_POINT ( 'NONE',  ( 10.81492255796106328, -18.62759615963255655, 20.41775706135234714 ) ) ;
#47390=CARTESIAN_POINT ( 'NONE',  ( 19.05341960407611168, 5.049401038298154454, 33.95724293864769550 ) ) ;
#47392=CARTESIAN_POINT ( 'NONE',  ( 0.05219959533934541429, -16.53943276465976808, 35.00109039468568284 ) ) ;
#47393=CARTESIAN_POINT ( 'NONE',  ( 16.46253265017146816, 9.564922557961045513, 96.66775706135233293 ) ) ;
#47394=CARTESIAN_POINT ( 'NONE',  ( 5.823673210054125526, 21.52544592524343514, 84.79057627198102409 ) ) ;
#47395=CARTESIAN_POINT ( 'NONE',  ( 19.05341960407617918, -5.049401038297876454, 66.04275706135233293 ) ) ;
#47396=CARTESIAN_POINT ( 'NONE',  ( 21.53943276465977519, 0.05219959533937863772, 21.25109039468567218 ) ) ;
#47397=CARTESIAN_POINT ( 'NONE',  ( -13.97604488694527625, -13.89961937509977830, 71.87390960531435269 ) ) ;
#47398=CARTESIAN_POINT ( 'NONE',  ( -13.97604488694527625, -13.89961937509977652, 71.87390960531433848 ) ) ;
#47399=CARTESIAN_POINT ( 'NONE',  ( -8.224510206698735004, -14.34966873604973081, 29.58442372801901854 ) ) ;
#47401=CARTESIAN_POINT ( 'NONE',  ( -5.049401038297874678, -19.05341960407617918, 54.79275706135234003 ) ) ;
#47402=CARTESIAN_POINT ( 'NONE',  ( -18.62759615963255300, -10.81492255796106328, 24.16775706135235424 ) ) ;
#47403=CARTESIAN_POINT ( 'NONE',  ( -8.224510206698948167, 14.34966873604960824, 75.41557627198102409 ) ) ;
#47404=CARTESIAN_POINT ( 'NONE',  ( 19.05341960407611168, 5.049401038298154454, 83.95724293864766707 ) ) ;
#47405=CARTESIAN_POINT ( 'NONE',  ( 12.14591786802327356, -12.06949235617739191, 40.62609039468567573 ) ) ;
#47406=CARTESIAN_POINT ( 'NONE',  ( 16.46253265017146816, 9.564922557961045513, 51.66775706135233293 ) ) ;
#47407=CARTESIAN_POINT ( 'NONE',  ( -15.80617190586768217, 15.72974639402176855, 68.12609039468567573 ) ) ;
#47408=CARTESIAN_POINT ( 'NONE',  ( -16.53943276465976808, -0.05219959533934237506, 23.75109039468567929 ) ) ;
#47409=CARTESIAN_POINT ( 'NONE',  ( 5.049401038298161559, -19.05341960407611168, 67.70724293864769550 ) ) ;
#47410=CARTESIAN_POINT ( 'NONE',  ( -13.97604488694547697, 13.89961937509957934, 88.12609039468563310 ) ) ;
#47411=CARTESIAN_POINT ( 'NONE',  ( -8.314922557961024197, 14.29746914071037800, 57.91775706135234714 ) ) ;
#47412=CARTESIAN_POINT ( 'NONE',  ( 10.72451020669871369, 18.67979575497193778, 102.0844237280190185 ) ) ;
#47413=CARTESIAN_POINT ( 'NONE',  ( -13.89961937509957401, -13.97604488694547875, 64.37609039468567573 ) ) ;
#47414=CARTESIAN_POINT ( 'NONE',  ( 9.564922557960805705, 16.46253265017160317, 49.58224293864770260 ) ) ;
#47415=CARTESIAN_POINT ( 'NONE',  ( 15.72974639402199770, -15.80617190586745480, 68.12390960531436690 ) ) ;
#47416=CARTESIAN_POINT ( 'NONE',  ( -16.55341960407611168, -4.379528057220339221, 66.45724293864768129 ) ) ;
#47417=CARTESIAN_POINT ( 'NONE',  ( -19.05341960407617563, 5.049401038297882671, 73.54275706135233293 ) ) ;
#47418=CARTESIAN_POINT ( 'NONE',  ( -18.87255363501903105, -5.500000000000063061, 71.32513748171827217 ) ) ;
#47419=CARTESIAN_POINT ( 'NONE',  ( -0.05219959533936034679, 19.03943276465977164, 42.50109039468566152 ) ) ;
#47420=CARTESIAN_POINT ( 'NONE',  ( -8.224510206698735004, -14.34966873604973081, 99.58442372801900433 ) ) ;
#47421=CARTESIAN_POINT ( 'NONE',  ( 16.55341960407611168, 4.379528057220329451, 63.95724293864770260 ) ) ;
#47422=CARTESIAN_POINT ( 'NONE',  ( -21.53943276465977519, -0.05219959533937600094, 98.75109039468568994 ) ) ;
#47424=CARTESIAN_POINT ( 'NONE',  ( 10.72451020669898902, -18.67979575497178502, 92.91557627198103830 ) ) ;
#47425=CARTESIAN_POINT ( 'NONE',  ( -16.51473224551069308, -9.474510206698971260, 61.66557627198103120 ) ) ;
#47426=CARTESIAN_POINT ( 'NONE',  ( -5.823673210054431948, 21.52544592524334988, 72.70942372801901854 ) ) ;
#47427=CARTESIAN_POINT ( 'NONE',  ( -19.03943276465977164, 0.05219959533909376836, 51.24890960531436690 ) ) ;
#47428=ORIENTED_EDGE ( 'NONE', *, *, #196038, .F. ) ;
#47429=CARTESIAN_POINT ( 'NONE',  ( -13.97604488694527625, -13.89961937509977652, 21.87390960531435979 ) ) ;
#47430=CARTESIAN_POINT ( 'NONE',  ( 19.02544592524343514, -5.153800228976328945, 108.5405762719810383 ) ) ;
#47431=CARTESIAN_POINT ( 'NONE',  ( -14.34966873604960291, -8.224510206698953496, 71.66557627198100988 ) ) ;
#47432=CARTESIAN_POINT ( 'NONE',  ( -13.89961937509977652, 13.97604488694528158, 30.62390960531435269 ) ) ;
#47433=CARTESIAN_POINT ( 'NONE',  ( 14.34966873604960469, 8.224510206698951720, 79.16557627198103830 ) ) ;
#47434=CARTESIAN_POINT ( 'NONE',  ( 21.55341960407610458, 5.719274019375980345, 98.95724293864770971 ) ) ;
#47435=CARTESIAN_POINT ( 'NONE',  ( -5.719274019375665041, -21.55341960407619695, 34.79275706135235424 ) ) ;
#47437=CARTESIAN_POINT ( 'NONE',  ( -4.379528057220086978, -16.55341960407618274, 54.79275706135235424 ) ) ;
#47438=CARTESIAN_POINT ( 'NONE',  ( -10.72451020669898014, 18.67979575497178502, 85.41557627198102409 ) ) ;
#47439=CARTESIAN_POINT ( 'NONE',  ( 16.46253265017146816, 9.564922557961045513, 21.66775706135233648 ) ) ;
#47440=CARTESIAN_POINT ( 'NONE',  ( -13.97604488694527625, -13.89961937509977652, 101.8739096053143811 ) ) ;
#47441=CARTESIAN_POINT ( 'NONE',  ( -18.62759615963255300, -10.81492255796106328, 39.16775706135235424 ) ) ;
#47442=EDGE_CURVE ( 'NONE', #7679, #165187, #136569, .T. ) ;
#47443=CARTESIAN_POINT ( 'NONE',  ( 21.53943276465977519, -0.05219959533907433946, 38.74890960531435979 ) ) ;
#47444=CARTESIAN_POINT ( 'NONE',  ( 12.06949235617757843, -12.14591786802309237, 28.12390960531435979 ) ) ;
#47445=CARTESIAN_POINT ( 'NONE',  ( -5.823673210054431948, 21.52544592524334988, 67.70942372801901854 ) ) ;
#47446=CARTESIAN_POINT ( 'NONE',  ( -10.72451020669870658, -18.67979575497194134, 94.58442372801901854 ) ) ;
#47447=CARTESIAN_POINT ( 'NONE',  ( 5.153800228976615827, -19.02544592524334988, 25.20942372801900433 ) ) ;
#47448=CARTESIAN_POINT ( 'NONE',  ( -14.29746914071037622, -8.314922557961029526, 94.16775706135237556 ) ) ;
#47449=CARTESIAN_POINT ( 'NONE',  ( -18.62759615963255300, -10.81492255796106328, 59.16775706135234714 ) ) ;
#47450=CARTESIAN_POINT ( 'NONE',  ( 0.05219959533909260263, 19.03943276465977164, 39.99890960531436690 ) ) ;
#47451=CARTESIAN_POINT ( 'NONE',  ( 5.153800228976615827, -19.02544592524334988, 25.20942372801900433 ) ) ;
#47452=CARTESIAN_POINT ( 'NONE',  ( -10.72451020669898014, 18.67979575497178502, 25.41557627198103120 ) ) ;
#47453=CARTESIAN_POINT ( 'NONE',  ( 10.72451020669898902, -18.67979575497178502, 112.9155762719810383 ) ) ;
#47454=CARTESIAN_POINT ( 'NONE',  ( -18.62759615963270932, 10.81492255796079327, 80.83224293864769550 ) ) ;
#47455=CARTESIAN_POINT ( 'NONE',  ( 16.55341960407618274, -4.379528057220086978, 36.04275706135234714 ) ) ;
#47457=CARTESIAN_POINT ( 'NONE',  ( -21.53943276465977519, 0.05219959533907696930, 81.24890960531436690 ) ) ;
#47458=CARTESIAN_POINT ( 'NONE',  ( -4.379528057220086978, -16.55341960407618274, 64.79275706135234714 ) ) ;
#47459=CARTESIAN_POINT ( 'NONE',  ( -4.379528057220328563, 16.55341960407611168, 60.20724293864768839 ) ) ;
#47461=CARTESIAN_POINT ( 'NONE',  ( 19.05341960407617918, -5.049401038297876454, 96.04275706135231871 ) ) ;
#47463=CARTESIAN_POINT ( 'NONE',  ( 12.14591786802327356, -12.06949235617739191, 35.62609039468568994 ) ) ;
#47464=CARTESIAN_POINT ( 'NONE',  ( 18.67979575497178502, 10.72451020669898547, 109.1655762719810383 ) ) ;
#47465=CARTESIAN_POINT ( 'NONE',  ( 15.80617190586746368, 15.72974639402197994, 74.37390960531436690 ) ) ;
#47466=CARTESIAN_POINT ( 'NONE',  ( 0.05219959533907565091, 21.53943276465977519, 34.99890960531435979 ) ) ;
#47467=CARTESIAN_POINT ( 'NONE',  ( 16.55341960407618274, -4.379528057220086978, 56.04275706135235424 ) ) ;
#47468=CARTESIAN_POINT ( 'NONE',  ( -13.97604488694527625, -13.89961937509977652, 66.87390960531436690 ) ) ;
#47469=CARTESIAN_POINT ( 'NONE',  ( 0.05219959533937995610, -21.53943276465977519, 45.00109039468568284 ) ) ;
#47470=CARTESIAN_POINT ( 'NONE',  ( 13.97604488694548053, -13.89961937509957401, 110.6260903946856615 ) ) ;
#47471=CARTESIAN_POINT ( 'NONE',  ( 10.81492255796078972, 18.62759615963270932, 29.58224293864769905 ) ) ;
#47472=CARTESIAN_POINT ( 'NONE',  ( -13.89961937509957401, -13.97604488694547875, 29.37609039468565797 ) ) ;
#47473=CARTESIAN_POINT ( 'NONE',  ( -12.06949235617739369, -12.14591786802326823, 44.37609039468567573 ) ) ;
#47474=CARTESIAN_POINT ( 'NONE',  ( -19.02544592524342804, 5.153800228976336051, 101.0405762719810241 ) ) ;
#47475=CARTESIAN_POINT ( 'NONE',  ( 10.81492255796078972, 18.62759615963270932, 109.5822429386476955 ) ) ;
#47476=CARTESIAN_POINT ( 'NONE',  ( 0.05219959533909260263, 19.03943276465977164, 74.99890960531435269 ) ) ;
#47477=CARTESIAN_POINT ( 'NONE',  ( -17.50000000000000355, 5.622605283950871780, 23.68792689403890606 ) ) ;
#47478=CARTESIAN_POINT ( 'NONE',  ( 8.224510206698953496, -14.34966873604960469, 82.91557627198103830 ) ) ;
#47479=CARTESIAN_POINT ( 'NONE',  ( -21.53943276465977519, 0.05219959533907696930, 21.24890960531436690 ) ) ;
#47480=CARTESIAN_POINT ( 'NONE',  ( 19.03943276465977164, -0.05219959533909143690, 23.74890960531435269 ) ) ;
#47481=CARTESIAN_POINT ( 'NONE',  ( 21.55341960407610458, 5.719274019375980345, 103.9572429386476813 ) ) ;
#47482=CARTESIAN_POINT ( 'NONE',  ( 16.51473224551083163, -9.474510206698727899, 65.83442372801900433 ) ) ;
#47483=CARTESIAN_POINT ( 'NONE',  ( -21.52544592524343514, 5.823673210054127303, 31.04057627198102409 ) ) ;
#47484=CARTESIAN_POINT ( 'NONE',  ( -13.89961937509977652, 13.97604488694528158, 25.62390960531434558 ) ) ;
#47485=CARTESIAN_POINT ( 'NONE',  ( -10.72451020669898014, 18.67979575497178502, 70.41557627198102409 ) ) ;
#47487=CARTESIAN_POINT ( 'NONE',  ( 9.474510206698971260, -16.51473224551069308, 92.91557627198103830 ) ) ;
#47488=CARTESIAN_POINT ( 'NONE',  ( -5.823673210054431948, 21.52544592524334988, 92.70942372801901854 ) ) ;
#47489=CARTESIAN_POINT ( 'NONE',  ( -19.02544592524342804, 5.153800228976336051, 51.04057627198103120 ) ) ;
#47490=CARTESIAN_POINT ( 'NONE',  ( -4.379528057220328563, 16.55341960407611168, 85.20724293864770971 ) ) ;
#47491=CARTESIAN_POINT ( 'NONE',  ( 14.34966873604972726, -8.224510206698740333, 40.83442372801901854 ) ) ;
#47492=CARTESIAN_POINT ( 'NONE',  ( 16.46253265017160672, -9.564922557960803928, 58.33224293864769550 ) ) ;
#47493=CARTESIAN_POINT ( 'NONE',  ( -5.823673210054431948, 21.52544592524334988, 77.70942372801900433 ) ) ;
#47495=CARTESIAN_POINT ( 'NONE',  ( 19.02544592524334988, 5.153800228976608722, 26.45942372801899722 ) ) ;
#47496=CARTESIAN_POINT ( 'NONE',  ( 16.51473224551083163, -9.474510206698727899, 35.83442372801899722 ) ) ;
#47497=CARTESIAN_POINT ( 'NONE',  ( 21.55341960407619695, -5.719274019375665929, 31.04275706135234714 ) ) ;
#47500=CARTESIAN_POINT ( 'NONE',  ( 0.05219959533936267826, -19.03943276465977164, 35.00109039468566863 ) ) ;
#47501=CARTESIAN_POINT ( 'NONE',  ( 13.97604488694527802, 13.89961937509977652, 84.37390960531433848 ) ) ;
#47502=CARTESIAN_POINT ( 'NONE',  ( 0.05219959533909260263, 19.03943276465977164, 69.99890960531435269 ) ) ;
#47503=CARTESIAN_POINT ( 'NONE',  ( 8.224510206698953496, -14.34966873604960469, 27.91557627198103830 ) ) ;
#47504=CARTESIAN_POINT ( 'NONE',  ( 16.46253265017160672, -9.564922557960803928, 113.3322429386476955 ) ) ;
#47505=CARTESIAN_POINT ( 'NONE',  ( -0.05219959533937732626, 21.53943276465977519, 87.50109039468568994 ) ) ;
#47507=CARTESIAN_POINT ( 'NONE',  ( 17.49999999999999645, 5.500000000000000888, 28.78230962303566542 ) ) ;
#47508=CARTESIAN_POINT ( 'NONE',  ( -18.67979575497193778, 10.72451020669871902, 93.33442372801901854 ) ) ;
#47509=CARTESIAN_POINT ( 'NONE',  ( 17.50000000000000000, 5.499999999999992895, 61.70309617465829177 ) ) ;
#47510=CARTESIAN_POINT ( 'NONE',  ( 19.03943276465977164, -0.05219959533909143690, 98.74890960531436690 ) ) ;
#47512=CARTESIAN_POINT ( 'NONE',  ( 12.14591786802327356, -12.06949235617739191, 45.62609039468567573 ) ) ;
#47513=CARTESIAN_POINT ( 'NONE',  ( 5.823673210054125526, 21.52544592524343514, 74.79057627198105251 ) ) ;
#47514=CARTESIAN_POINT ( 'NONE',  ( 16.52544592524342804, -4.483927247898539470, 23.54057627198102765 ) ) ;
#47515=CARTESIAN_POINT ( 'NONE',  ( 16.52544592524342804, -4.483927247898539470, 113.5405762719810383 ) ) ;
#47516=CARTESIAN_POINT ( 'NONE',  ( 16.51473224551069308, 9.474510206698969483, 94.16557627198103830 ) ) ;
#47517=CARTESIAN_POINT ( 'NONE',  ( -15.80617190586768217, 15.72974639402176855, 113.1260903946856899 ) ) ;
#47518=CARTESIAN_POINT ( 'NONE',  ( 0.05219959533910956823, 16.53943276465976808, 109.9989096053143527 ) ) ;
#47519=CARTESIAN_POINT ( 'NONE',  ( 10.72451020669871369, 18.67979575497193778, 67.08442372801901854 ) ) ;
#47520=CARTESIAN_POINT ( 'NONE',  ( -9.474510206698964154, 16.51473224551069663, 110.4155762719810383 ) ) ;
#47521=CARTESIAN_POINT ( 'NONE',  ( -12.14591786802326823, 12.06949235617739902, 108.1260903946856757 ) ) ;
#47522=CARTESIAN_POINT ( 'NONE',  ( -13.97604488694547697, 13.89961937509957934, 58.12609039468566863 ) ) ;
#47523=CARTESIAN_POINT ( 'NONE',  ( -9.564922557961040184, 16.46253265017147172, 67.91775706135233293 ) ) ;
#47524=CARTESIAN_POINT ( 'NONE',  ( -13.97604488694527625, -13.89961937509977652, 111.8739096053143243 ) ) ;
#47525=CARTESIAN_POINT ( 'NONE',  ( 8.314922557960818139, 14.29746914071049879, 94.58224293864769550 ) ) ;
#47526=CARTESIAN_POINT ( 'NONE',  ( -0.05219959533936034679, 19.03943276465977164, 57.50109039468566863 ) ) ;
#47528=CARTESIAN_POINT ( 'NONE',  ( 5.049401038298161559, -19.05341960407611168, 82.70724293864770971 ) ) ;
#47529=CARTESIAN_POINT ( 'NONE',  ( 12.14591786802309770, 12.06949235617756955, 64.37390960531435269 ) ) ;
#47530=CARTESIAN_POINT ( 'NONE',  ( -19.02544592524334988, -5.153800228976617603, 93.95942372801900433 ) ) ;
#47531=CARTESIAN_POINT ( 'NONE',  ( -21.55341960407610458, -5.719274019375992779, 51.45724293864770260 ) ) ;
#47534=CARTESIAN_POINT ( 'NONE',  ( 12.14591786802309770, 12.06949235617756955, 114.3739096053143527 ) ) ;
#47535=CARTESIAN_POINT ( 'NONE',  ( -16.81555441253549432, -7.025013491695499823, 29.36314554665745646 ) ) ;
#47536=CARTESIAN_POINT ( 'NONE',  ( 13.97604488694527802, 13.89961937509977652, 69.37390960531436690 ) ) ;
#47537=CARTESIAN_POINT ( 'NONE',  ( -21.55341960407610458, -5.719274019375992779, 71.45724293864769550 ) ) ;
#47538=CARTESIAN_POINT ( 'NONE',  ( 16.55341960407618274, -4.379528057220086978, 91.04275706135236135 ) ) ;
#47539=CARTESIAN_POINT ( 'NONE',  ( -16.46253265017160317, 9.564922557960807481, 75.83224293864769550 ) ) ;
#47540=CARTESIAN_POINT ( 'NONE',  ( -9.564922557961040184, 16.46253265017147172, 62.91775706135233293 ) ) ;
#47541=CARTESIAN_POINT ( 'NONE',  ( -15.80617190586768217, 15.72974639402176855, 83.12609039468568994 ) ) ;
#47542=CARTESIAN_POINT ( 'NONE',  ( 5.823673210054125526, 21.52544592524343514, 64.79057627198103830 ) ) ;
#47543=CARTESIAN_POINT ( 'NONE',  ( 5.823673210054125526, 21.52544592524343514, 24.79057627198103120 ) ) ;
#47544=CARTESIAN_POINT ( 'NONE',  ( 19.03943276465977164, -0.05219959533909143690, 38.74890960531436690 ) ) ;
#47545=CARTESIAN_POINT ( 'NONE',  ( 12.14591786802327356, -12.06949235617739191, 100.6260903946857184 ) ) ;
#47546=CARTESIAN_POINT ( 'NONE',  ( -9.474510206698964154, 16.51473224551069663, 55.41557627198103120 ) ) ;
#47547=CARTESIAN_POINT ( 'NONE',  ( 12.06949235617739724, 12.14591786802326823, 26.87609039468567218 ) ) ;
#47548=CARTESIAN_POINT ( 'NONE',  ( 16.46253265017146816, 9.564922557961045513, 81.66775706135233293 ) ) ;
#47549=CARTESIAN_POINT ( 'NONE',  ( 21.53943276465977519, 0.05219959533937863772, 96.25109039468568994 ) ) ;
#47550=CARTESIAN_POINT ( 'NONE',  ( 14.34966873604960469, 8.224510206698951720, 54.16557627198103120 ) ) ;
#47551=CARTESIAN_POINT ( 'NONE',  ( -21.55341960407610458, -5.719274019375992779, 101.4572429386476955 ) ) ;
#47552=CARTESIAN_POINT ( 'NONE',  ( 10.72451020669898902, -18.67979575497178502, 102.9155762719810383 ) ) ;
#47554=CARTESIAN_POINT ( 'NONE',  ( 5.823673210054125526, 21.52544592524343514, 49.79057627198102409 ) ) ;
#47555=CARTESIAN_POINT ( 'NONE',  ( -8.224510206698735004, -14.34966873604973081, 74.58442372801901854 ) ) ;
#47556=CARTESIAN_POINT ( 'NONE',  ( -12.06949235617756955, 12.14591786802309770, 90.62390960531436690 ) ) ;
#47557=CARTESIAN_POINT ( 'NONE',  ( 13.89961937509977652, -13.97604488694527269, 43.12390960531434558 ) ) ;
#47559=CARTESIAN_POINT ( 'NONE',  ( 0.05219959533934541429, -16.53943276465976808, 110.0010903946856757 ) ) ;
#47560=CARTESIAN_POINT ( 'NONE',  ( -15.80617190586768217, 15.72974639402176855, 38.12609039468567573 ) ) ;
#47561=CARTESIAN_POINT ( 'NONE',  ( -19.02544592524342804, 5.153800228976336051, 91.04057627198100988 ) ) ;
#47562=CARTESIAN_POINT ( 'NONE',  ( 15.72974639402176855, 15.80617190586768217, 61.87609039468568284 ) ) ;
#47563=CARTESIAN_POINT ( 'NONE',  ( 17.50000000000000000, -5.499999999999992895, 51.21769037696435589 ) ) ;
#47567=CARTESIAN_POINT ( 'NONE',  ( -10.81492255796105439, 18.62759615963255655, 52.91775706135235424 ) ) ;
#47568=CARTESIAN_POINT ( 'NONE',  ( 19.05341960407611168, 5.049401038298154454, 53.95724293864770260 ) ) ;
#47570=CARTESIAN_POINT ( 'NONE',  ( -13.89961937509977652, 13.97604488694528158, 85.62390960531433848 ) ) ;
#47571=CARTESIAN_POINT ( 'NONE',  ( -5.153800228976607833, 19.02544592524334988, 72.70942372801900433 ) ) ;
#47572=CARTESIAN_POINT ( 'NONE',  ( 18.62759615963255655, 10.81492255796105972, 46.66775706135234714 ) ) ;
#47573=CARTESIAN_POINT ( 'NONE',  ( 13.97604488694548053, -13.89961937509957401, 65.62609039468567573 ) ) ;
#47574=CARTESIAN_POINT ( 'NONE',  ( 9.564922557960805705, 16.46253265017160317, 39.58224293864768839 ) ) ;
#47575=CARTESIAN_POINT ( 'NONE',  ( 8.224510206698742110, 14.34966873604972548, 102.0844237280190185 ) ) ;
#47576=CARTESIAN_POINT ( 'NONE',  ( 13.89961937509957401, 13.97604488694547697, 71.87609039468567573 ) ) ;
#47577=CARTESIAN_POINT ( 'NONE',  ( 4.483927247898545687, 16.52544592524342804, 29.79057627198102409 ) ) ;
#47578=CARTESIAN_POINT ( 'NONE',  ( -13.89961937509957401, -13.97604488694547875, 44.37609039468566863 ) ) ;
#47579=CARTESIAN_POINT ( 'NONE',  ( 18.62759615963255655, 10.81492255796105972, 111.6677570613523613 ) ) ;
#47580=CARTESIAN_POINT ( 'NONE',  ( 16.46253265017146816, 9.564922557961045513, 31.66775706135232937 ) ) ;
#47581=CARTESIAN_POINT ( 'NONE',  ( 19.05341960407611168, 5.049401038298154454, 33.95724293864769550 ) ) ;
#47582=CARTESIAN_POINT ( 'NONE',  ( -5.719274019375665041, -21.55341960407619695, 94.79275706135234714 ) ) ;
#47583=CARTESIAN_POINT ( 'NONE',  ( -14.29746914071037622, -8.314922557961029526, 39.16775706135235424 ) ) ;
#47584=CARTESIAN_POINT ( 'NONE',  ( -5.153800228976328057, -19.02544592524343514, 92.29057627198099567 ) ) ;
#47586=CARTESIAN_POINT ( 'NONE',  ( -5.049401038298153566, 19.05341960407611168, 75.20724293864769550 ) ) ;
#47588=CARTESIAN_POINT ( 'NONE',  ( 13.97604488694548053, -13.89961937509957401, 90.62609039468567573 ) ) ;
#47589=CARTESIAN_POINT ( 'NONE',  ( 9.564922557960805705, 16.46253265017160317, 104.5822429386476955 ) ) ;
#47590=CARTESIAN_POINT ( 'NONE',  ( -0.05219959533937732626, 21.53943276465977519, 97.50109039468567573 ) ) ;
#47591=CARTESIAN_POINT ( 'NONE',  ( 0.05219959533910956823, 16.53943276465976808, 94.99890960531436690 ) ) ;
#47592=CARTESIAN_POINT ( 'NONE',  ( -19.03943276465977164, 0.05219959533909376836, 26.24890960531435624 ) ) ;
#47593=CARTESIAN_POINT ( 'NONE',  ( -21.53943276465977519, 0.05219959533907696930, 56.24890960531436690 ) ) ;
#47594=CARTESIAN_POINT ( 'NONE',  ( 18.62759615963271287, -10.81492255796078972, 38.33224293864768839 ) ) ;
#47595=CARTESIAN_POINT ( 'NONE',  ( -0.05219959533909027116, -19.03943276465977164, 27.49890960531435624 ) ) ;
#47596=CARTESIAN_POINT ( 'NONE',  ( 17.50000000000000000, -5.500000000000000888, 120.0000000000000142 ) ) ;
#47597=CARTESIAN_POINT ( 'NONE',  ( 19.05341960407617918, -5.049401038297876454, 61.04275706135232582 ) ) ;
#47598=CARTESIAN_POINT ( 'NONE',  ( -4.379528057220328563, 16.55341960407611168, 45.20724293864769550 ) ) ;
#47599=CARTESIAN_POINT ( 'NONE',  ( 16.51473224551069308, 9.474510206698969483, 114.1655762719810241 ) ) ;
#47600=CARTESIAN_POINT ( 'NONE',  ( -18.62759615963255300, -10.81492255796106328, 84.16775706135234714 ) ) ;
#47601=CARTESIAN_POINT ( 'NONE',  ( 18.62759615963271287, -10.81492255796078972, 68.33224293864769550 ) ) ;
#47602=CARTESIAN_POINT ( 'NONE',  ( 10.72451020669871369, 18.67979575497193778, 47.08442372801901854 ) ) ;
#47603=CARTESIAN_POINT ( 'NONE',  ( -10.72451020669898014, 18.67979575497178502, 95.41557627198102409 ) ) ;
#47604=CARTESIAN_POINT ( 'NONE',  ( 18.67979575497194134, -10.72451020669871369, 45.83442372801901854 ) ) ;
#47605=CARTESIAN_POINT ( 'NONE',  ( -13.97604488694527625, -13.89961937509977652, 26.87390960531434558 ) ) ;
#47606=CARTESIAN_POINT ( 'NONE',  ( -0.05219959533909027116, -19.03943276465977164, 77.49890960531435269 ) ) ;
#47607=CARTESIAN_POINT ( 'NONE',  ( -12.14591786802326823, 12.06949235617739902, 78.12609039468570415 ) ) ;
#47608=CARTESIAN_POINT ( 'NONE',  ( 4.379528057220339221, -16.55341960407611168, 102.7072429386476955 ) ) ;
#47609=FACE_OUTER_BOUND ( 'NONE', #188300, .T. ) ;
#47610=CARTESIAN_POINT ( 'NONE',  ( -16.52544592524342804, 4.483927247898546575, 51.04057627198103120 ) ) ;
#47611=CARTESIAN_POINT ( 'NONE',  ( 4.379528057220092307, 16.55341960407617563, 107.2927570613523471 ) ) ;
#47612=CARTESIAN_POINT ( 'NONE',  ( -16.51473224551069308, -9.474510206698971260, 71.66557627198102409 ) ) ;
#47613=CARTESIAN_POINT ( 'NONE',  ( 19.05341960407611168, 5.049401038298154454, 33.95724293864769550 ) ) ;
#47614=CARTESIAN_POINT ( 'NONE',  ( 21.52544592524344225, -5.823673210054117533, 48.54057627198103120 ) ) ;
#47615=CARTESIAN_POINT ( 'NONE',  ( 13.89961937509957401, 13.97604488694547697, 36.87609039468565442 ) ) ;
#47617=CARTESIAN_POINT ( 'NONE',  ( 16.53943276465976808, -0.05219959533910856209, 53.74890960531437401 ) ) ;
#47618=CARTESIAN_POINT ( 'NONE',  ( 21.53943276465977519, -0.05219959533907433946, 28.74890960531435624 ) ) ;
#47619=CARTESIAN_POINT ( 'NONE',  ( 18.67979575497194134, -10.72451020669871369, 65.83442372801900433 ) ) ;
#47621=CARTESIAN_POINT ( 'NONE',  ( 14.29746914071037800, 8.314922557961029526, 66.66775706135234714 ) ) ;
#47622=CARTESIAN_POINT ( 'NONE',  ( 13.89961937509957401, 13.97604488694547697, 56.87609039468564731 ) ) ;
#47623=CARTESIAN_POINT ( 'NONE',  ( -16.55341960407611168, -4.379528057220339221, 41.45724293864769550 ) ) ;
#47624=DIRECTION ( 'NONE',  ( 0.000000000000000000, -1.000000000000000000, -0.000000000000000000 ) ) ;
#47625=CARTESIAN_POINT ( 'NONE',  ( 16.55341960407611168, 4.379528057220329451, 28.95724293864769905 ) ) ;
#47626=CARTESIAN_POINT ( 'NONE',  ( 16.46253265017160672, -9.564922557960803928, 38.33224293864768839 ) ) ;
#47627=CARTESIAN_POINT ( 'NONE',  ( -19.05341960407611168, -5.049401038298163336, 56.45724293864768129 ) ) ;
#47628=CARTESIAN_POINT ( 'NONE',  ( -8.224510206698948167, 14.34966873604960824, 115.4155762719810241 ) ) ;
#47629=CARTESIAN_POINT ( 'NONE',  ( 18.67979575497194134, -10.72451020669871369, 35.83442372801901143 ) ) ;
#47630=CARTESIAN_POINT ( 'NONE',  ( -19.03943276465977164, 0.05219959533909376836, 56.24890960531435979 ) ) ;
#47632=CARTESIAN_POINT ( 'NONE',  ( 13.89961937509977652, -13.97604488694527269, 48.12390960531435979 ) ) ;
#47634=CARTESIAN_POINT ( 'NONE',  ( -5.719274019375978568, 21.55341960407610458, 35.20724293864768839 ) ) ;
#47635=CARTESIAN_POINT ( 'NONE',  ( 5.823673210054444382, -21.52544592524334988, 55.20942372801902565 ) ) ;
#47636=CARTESIAN_POINT ( 'NONE',  ( 4.379528057220339221, -16.55341960407611168, 112.7072429386476955 ) ) ;
#47637=CARTESIAN_POINT ( 'NONE',  ( -21.53943276465977519, 0.05219959533907696930, 31.24890960531435979 ) ) ;
#47639=CARTESIAN_POINT ( 'NONE',  ( 12.06949235617739724, 12.14591786802326823, 96.87609039468568994 ) ) ;
#47640=CARTESIAN_POINT ( 'NONE',  ( 21.52544592524334988, 5.823673210054432836, 111.4594237280190328 ) ) ;
#47642=CARTESIAN_POINT ( 'NONE',  ( -8.314922557961024197, 14.29746914071037800, 62.91775706135236135 ) ) ;
#47643=CARTESIAN_POINT ( 'NONE',  ( 0.05219959533909260263, 19.03943276465977164, 109.9989096053143669 ) ) ;
#47645=CARTESIAN_POINT ( 'NONE',  ( -14.29746914071037622, -8.314922557961029526, 49.16775706135234003 ) ) ;
#47646=CARTESIAN_POINT ( 'NONE',  ( 12.14591786802327356, -12.06949235617739191, 25.62609039468567929 ) ) ;
#47647=CARTESIAN_POINT ( 'NONE',  ( 12.06949235617739724, 12.14591786802326823, 96.87609039468568994 ) ) ;
#47648=CARTESIAN_POINT ( 'NONE',  ( 5.719274019375673035, 21.55341960407619339, 52.29275706135236135 ) ) ;
#47649=CARTESIAN_POINT ( 'NONE',  ( -16.55341960407617563, 4.379528057220093196, 28.54275706135234358 ) ) ;
#47650=CARTESIAN_POINT ( 'NONE',  ( 18.67979575497178502, 10.72451020669898547, 114.1655762719810383 ) ) ;
#47651=CARTESIAN_POINT ( 'NONE',  ( 4.379528057220092307, 16.55341960407617563, 22.29275706135235069 ) ) ;
#47652=CARTESIAN_POINT ( 'NONE',  ( -12.14591786802326823, 12.06949235617739902, 88.12609039468570415 ) ) ;
#47654=CARTESIAN_POINT ( 'NONE',  ( 21.53943276465977519, 0.05219959533937863772, 86.25109039468568994 ) ) ;
#47655=CARTESIAN_POINT ( 'NONE',  ( -16.51473224551082808, 9.474510206698731452, 83.33442372801899012 ) ) ;
#47656=CARTESIAN_POINT ( 'NONE',  ( -12.14591786802309592, -12.06949235617757132, 41.87390960531435979 ) ) ;
#47657=CARTESIAN_POINT ( 'NONE',  ( -0.05219959533910754901, -16.53943276465976808, 42.49890960531435979 ) ) ;
#47658=CARTESIAN_POINT ( 'NONE',  ( 4.379528057220339221, -16.55341960407611168, 112.7072429386476955 ) ) ;
#47659=CARTESIAN_POINT ( 'NONE',  ( 0.05219959533936267826, -19.03943276465977164, 45.00109039468566863 ) ) ;
#47661=CARTESIAN_POINT ( 'NONE',  ( 18.62759615963255655, 10.81492255796105972, 51.66775706135234714 ) ) ;
#47662=CARTESIAN_POINT ( 'NONE',  ( -9.474510206698720793, -16.51473224551083518, 104.5844237280190043 ) ) ;
#47663=CARTESIAN_POINT ( 'NONE',  ( 9.474510206698971260, -16.51473224551069308, 107.9155762719810383 ) ) ;
#47664=CARTESIAN_POINT ( 'NONE',  ( 18.62759615963271287, -10.81492255796078972, 53.33224293864769550 ) ) ;
#47665=CARTESIAN_POINT ( 'NONE',  ( -5.049401038297874678, -19.05341960407617918, 94.79275706135230450 ) ) ;
#47666=CARTESIAN_POINT ( 'NONE',  ( 5.153800228976335163, 19.02544592524342804, 89.79057627198102409 ) ) ;
#47667=CARTESIAN_POINT ( 'NONE',  ( 15.80617190586746368, 15.72974639402197994, 54.37390960531435979 ) ) ;
#47668=CARTESIAN_POINT ( 'NONE',  ( 12.06949235617757843, -12.14591786802309237, 113.1239096053143953 ) ) ;
#47669=CARTESIAN_POINT ( 'NONE',  ( 9.564922557960805705, 16.46253265017160317, 64.58224293864769550 ) ) ;
#47670=CARTESIAN_POINT ( 'NONE',  ( -19.03943276465977164, 0.05219959533909376836, 26.24890960531435624 ) ) ;
#47672=CARTESIAN_POINT ( 'NONE',  ( -21.52544592524334988, -5.823673210054445271, 33.95942372801901143 ) ) ;
#47673=CARTESIAN_POINT ( 'NONE',  ( 15.80617190586769283, -15.72974639402175789, 85.62609039468568994 ) ) ;
#47674=CARTESIAN_POINT ( 'NONE',  ( 8.314922557961029526, -14.29746914071037800, 90.41775706135236135 ) ) ;
#47675=CARTESIAN_POINT ( 'NONE',  ( -15.80617190586768217, 15.72974639402176855, 28.12609039468568284 ) ) ;
#47676=CARTESIAN_POINT ( 'NONE',  ( -5.823673210054431948, 21.52544592524334988, 42.70942372801901854 ) ) ;
#47677=CARTESIAN_POINT ( 'NONE',  ( -0.05219959533936034679, 19.03943276465977164, 62.50109039468566863 ) ) ;
#47678=CARTESIAN_POINT ( 'NONE',  ( -0.05219959533909027116, -19.03943276465977164, 72.49890960531435269 ) ) ;
#47679=CARTESIAN_POINT ( 'NONE',  ( -18.62759615963255300, -10.81492255796106328, 84.16775706135234714 ) ) ;
#47681=CARTESIAN_POINT ( 'NONE',  ( -0.05219959533907301413, -21.53943276465977519, 87.49890960531436690 ) ) ;
#47682=CARTESIAN_POINT ( 'NONE',  ( -14.34966873604960291, -8.224510206698953496, 66.66557627198102409 ) ) ;
#47683=CARTESIAN_POINT ( 'NONE',  ( -5.823673210054431948, 21.52544592524334988, 102.7094237280190185 ) ) ;
#47684=CARTESIAN_POINT ( 'NONE',  ( -16.55341960407611168, -4.379528057220339221, 81.45724293864769550 ) ) ;
#47685=CARTESIAN_POINT ( 'NONE',  ( 0.05219959533909260263, 19.03943276465977164, 34.99890960531435979 ) ) ;
#47686=CARTESIAN_POINT ( 'NONE',  ( -16.51473224551082808, 9.474510206698731452, 73.33442372801900433 ) ) ;
#47687=CARTESIAN_POINT ( 'NONE',  ( 4.483927247898545687, 16.52544592524342804, 29.79057627198102409 ) ) ;
#47688=CARTESIAN_POINT ( 'NONE',  ( 18.67979575497194134, -10.72451020669871369, 90.83442372801901854 ) ) ;
#47689=CARTESIAN_POINT ( 'NONE',  ( 19.03943276465977164, -0.05219959533909143690, 93.74890960531435269 ) ) ;
#47690=CARTESIAN_POINT ( 'NONE',  ( -0.05219959533936034679, 19.03943276465977164, 62.50109039468566863 ) ) ;
#47691=CARTESIAN_POINT ( 'NONE',  ( 18.67979575497178502, 10.72451020669898547, 64.16557627198102409 ) ) ;
#47692=CARTESIAN_POINT ( 'NONE',  ( 5.823673210054125526, 21.52544592524343514, 114.7905762719810383 ) ) ;
#47693=CARTESIAN_POINT ( 'NONE',  ( 5.153800228976615827, -19.02544592524334988, 105.2094237280190185 ) ) ;
#47694=CARTESIAN_POINT ( 'NONE',  ( -16.52544592524335698, -4.483927247898792601, 78.95942372801901854 ) ) ;
#47696=CARTESIAN_POINT ( 'NONE',  ( -18.62759615963255300, -10.81492255796106328, 19.16775706135234714 ) ) ;
#47697=CARTESIAN_POINT ( 'NONE',  ( 16.55341960407611168, 4.379528057220329451, 98.95724293864770971 ) ) ;
#47699=CARTESIAN_POINT ( 'NONE',  ( 16.55341960407618274, -4.379528057220086978, 51.04275706135234714 ) ) ;
#47700=CARTESIAN_POINT ( 'NONE',  ( 5.719274019375991003, -21.55341960407610458, 67.70724293864769550 ) ) ;
#47701=CARTESIAN_POINT ( 'NONE',  ( -0.05219959533934338120, 16.53943276465976808, 107.5010903946856899 ) ) ;
#47702=CARTESIAN_POINT ( 'NONE',  ( -14.34966873604972548, 8.224510206698743886, 33.33442372801900433 ) ) ;
#47703=CARTESIAN_POINT ( 'NONE',  ( 19.03943276465977164, -0.05219959533909143690, 28.74890960531435624 ) ) ;
#47704=CARTESIAN_POINT ( 'NONE',  ( 4.379528057220092307, 16.55341960407617563, 82.29275706135234714 ) ) ;
#47705=CARTESIAN_POINT ( 'NONE',  ( -13.89961937509957401, -13.97604488694547875, 69.37609039468564731 ) ) ;
#47706=CARTESIAN_POINT ( 'NONE',  ( 5.719274019375991003, -21.55341960407610458, 77.70724293864770971 ) ) ;
#47707=CARTESIAN_POINT ( 'NONE',  ( 12.06949235617739724, 12.14591786802326823, 96.87609039468568994 ) ) ;
#47708=CARTESIAN_POINT ( 'NONE',  ( 5.719274019375673035, 21.55341960407619339, 87.29275706135236135 ) ) ;
#47709=CARTESIAN_POINT ( 'NONE',  ( -0.05219959533907301413, -21.53943276465977519, 62.49890960531436690 ) ) ;
#47710=CARTESIAN_POINT ( 'NONE',  ( 21.55341960407610458, 5.719274019375980345, 48.95724293864770971 ) ) ;
#47711=ORIENTED_EDGE ( 'NONE', *, *, #82905, .T. ) ;
#47712=CARTESIAN_POINT ( 'NONE',  ( -16.53943276465976808, -0.05219959533934237506, 83.75109039468568994 ) ) ;
#47713=CARTESIAN_POINT ( 'NONE',  ( 5.719274019375991003, -21.55341960407610458, 42.70724293864770260 ) ) ;
#47715=CARTESIAN_POINT ( 'NONE',  ( 19.02544592524343514, -5.153800228976328945, 113.5405762719810241 ) ) ;
#47716=CARTESIAN_POINT ( 'NONE',  ( -19.02544592524342804, 5.153800228976336051, 31.04057627198102409 ) ) ;
#47717=CARTESIAN_POINT ( 'NONE',  ( 0.05219959533907565091, 21.53943276465977519, 64.99890960531435269 ) ) ;
#47718=CARTESIAN_POINT ( 'NONE',  ( -4.379528057220086978, -16.55341960407618274, 99.79275706135234714 ) ) ;
#47719=CARTESIAN_POINT ( 'NONE',  ( -10.81492255796105439, 18.62759615963255655, 42.91775706135235424 ) ) ;
#47720=CARTESIAN_POINT ( 'NONE',  ( -19.03943276465977164, -0.05219959533935918106, 108.7510903946856615 ) ) ;
#47721=CARTESIAN_POINT ( 'NONE',  ( -16.51473224551069308, -9.474510206698971260, 21.66557627198102765 ) ) ;
#47722=CARTESIAN_POINT ( 'NONE',  ( -12.06949235617739369, -12.14591786802326823, 19.37609039468568639 ) ) ;
#47723=CARTESIAN_POINT ( 'NONE',  ( 19.03943276465977164, -0.05219959533909143690, 43.74890960531435979 ) ) ;
#47725=CARTESIAN_POINT ( 'NONE',  ( 9.564922557960805705, 16.46253265017160317, 89.58224293864769550 ) ) ;
#47726=CARTESIAN_POINT ( 'NONE',  ( 8.224510206698742110, 14.34966873604972548, 82.08442372801901854 ) ) ;
#47727=CARTESIAN_POINT ( 'NONE',  ( 9.564922557961047289, -16.46253265017146816, 75.41775706135234714 ) ) ;
#47728=CARTESIAN_POINT ( 'NONE',  ( -5.049401038297874678, -19.05341960407617918, 19.79275706135233293 ) ) ;
#47729=CARTESIAN_POINT ( 'NONE',  ( -0.05219959533907301413, -21.53943276465977519, 67.49890960531436690 ) ) ;
#47730=CARTESIAN_POINT ( 'NONE',  ( -8.314922557961024197, 14.29746914071037800, 82.91775706135234714 ) ) ;
#47731=CARTESIAN_POINT ( 'NONE',  ( -19.03943276465977164, -0.05219959533935918106, 78.75109039468567573 ) ) ;
#47732=CARTESIAN_POINT ( 'NONE',  ( 9.474510206698971260, -16.51473224551069308, 42.91557627198103120 ) ) ;
#47733=CARTESIAN_POINT ( 'NONE',  ( 16.46253265017160672, -9.564922557960803928, 78.33224293864769550 ) ) ;
#47734=CARTESIAN_POINT ( 'NONE',  ( -21.55341960407619339, 5.719274019375674811, 53.54275706135234714 ) ) ;
#47735=CARTESIAN_POINT ( 'NONE',  ( 9.474510206698971260, -16.51473224551069308, 47.91557627198102409 ) ) ;
#47736=CARTESIAN_POINT ( 'NONE',  ( 19.02544592524334988, 5.153800228976608722, 76.45942372801897591 ) ) ;
#47738=CARTESIAN_POINT ( 'NONE',  ( -9.474510206698964154, 16.51473224551069663, 110.4155762719810383 ) ) ;
#47739=CARTESIAN_POINT ( 'NONE',  ( 4.483927247898545687, 16.52544592524342804, 59.79057627198103120 ) ) ;
#47740=CARTESIAN_POINT ( 'NONE',  ( 18.67979575497178502, 10.72451020669898547, 54.16557627198103120 ) ) ;
#47742=CARTESIAN_POINT ( 'NONE',  ( 9.474510206698729675, 16.51473224551082808, 42.08442372801900433 ) ) ;
#47744=CARTESIAN_POINT ( 'NONE',  ( 19.03943276465977164, -0.05219959533909143690, 63.74890960531435979 ) ) ;
#47745=CARTESIAN_POINT ( 'NONE',  ( 9.564922557960805705, 16.46253265017160317, 74.58224293864769550 ) ) ;
#47746=CARTESIAN_POINT ( 'NONE',  ( -4.483927247898782831, 16.52544592524335698, 47.70942372801902565 ) ) ;
#47747=CARTESIAN_POINT ( 'NONE',  ( -18.09918380851993192, -5.500000000000040856, 66.48618307335613054 ) ) ;
#47749=CARTESIAN_POINT ( 'NONE',  ( -4.483927247898782831, 16.52544592524335698, 82.70942372801900433 ) ) ;
#47750=FACE_OUTER_BOUND ( 'NONE', #144784, .T. ) ;
#47751=CARTESIAN_POINT ( 'NONE',  ( -16.55341960407617563, 4.379528057220093196, 68.54275706135234714 ) ) ;
#47752=CARTESIAN_POINT ( 'NONE',  ( -14.29746914071037622, -8.314922557961029526, 39.16775706135235424 ) ) ;
#47753=CARTESIAN_POINT ( 'NONE',  ( 19.02544592524334988, 5.153800228976608722, 26.45942372801899722 ) ) ;
#47754=CARTESIAN_POINT ( 'NONE',  ( 16.51473224551069308, 9.474510206698969483, 54.16557627198103120 ) ) ;
#47756=CARTESIAN_POINT ( 'NONE',  ( 5.823673210054444382, -21.52544592524334988, 55.20942372801902565 ) ) ;
#47757=CARTESIAN_POINT ( 'NONE',  ( 9.564922557961047289, -16.46253265017146816, 65.41775706135233293 ) ) ;
#47758=CARTESIAN_POINT ( 'NONE',  ( 18.62759615963255655, 10.81492255796105972, 106.6677570613523756 ) ) ;
#47759=CARTESIAN_POINT ( 'NONE',  ( -13.97604488694527625, -13.89961937509977652, 31.87390960531435979 ) ) ;
#47761=CARTESIAN_POINT ( 'NONE',  ( 0.05219959533907565091, 21.53943276465977519, 49.99890960531437401 ) ) ;
#47762=CIRCLE ( 'NONE', #80070, 2.000000000000000000 ) ;
#47763=CARTESIAN_POINT ( 'NONE',  ( 0.05219959533909260263, 19.03943276465977164, 114.9989096053143669 ) ) ;
#47764=CARTESIAN_POINT ( 'NONE',  ( -12.06949235617756955, 12.14591786802309770, 100.6239096053143811 ) ) ;
#47765=CARTESIAN_POINT ( 'NONE',  ( 16.55341960407618274, -4.379528057220086978, 31.04275706135234714 ) ) ;
#47766=CARTESIAN_POINT ( 'NONE',  ( -12.06949235617756955, 12.14591786802309770, 35.62390960531437401 ) ) ;
#47768=CARTESIAN_POINT ( 'NONE',  ( -21.55341960407610458, -5.719274019375992779, 111.4572429386476813 ) ) ;
#47769=CARTESIAN_POINT ( 'NONE',  ( -16.53943276465976808, 0.05219959533911058130, 36.24890960531435979 ) ) ;
#47770=CARTESIAN_POINT ( 'NONE',  ( 9.564922557960805705, 16.46253265017160317, 109.5822429386476955 ) ) ;
#47771=CARTESIAN_POINT ( 'NONE',  ( 16.51473224551083163, -9.474510206698727899, 110.8344237280190043 ) ) ;
#47772=CARTESIAN_POINT ( 'NONE',  ( 9.564922557961047289, -16.46253265017146816, 25.41775706135234003 ) ) ;
#47773=CARTESIAN_POINT ( 'NONE',  ( -16.53943276465976808, 0.05219959533911058130, 36.24890960531435979 ) ) ;
#47774=CARTESIAN_POINT ( 'NONE',  ( -21.53943276465977519, 0.05219959533907696930, 101.2489096053143669 ) ) ;
#47775=CARTESIAN_POINT ( 'NONE',  ( 17.40805194822031865, 6.112264579159358391, 31.66628727489388595 ) ) ;
#47776=CARTESIAN_POINT ( 'NONE',  ( -15.80617190586745835, -15.72974639402198527, 66.87390960531436690 ) ) ;
#47777=CARTESIAN_POINT ( 'NONE',  ( -5.153800228976328057, -19.02544592524343514, 82.29057627198103830 ) ) ;
#47778=CARTESIAN_POINT ( 'NONE',  ( 16.55341960407611168, 4.379528057220329451, 43.95724293864769550 ) ) ;
#47779=CARTESIAN_POINT ( 'NONE',  ( 13.97604488694527802, 13.89961937509977652, 94.37390960531436690 ) ) ;
#47781=CARTESIAN_POINT ( 'NONE',  ( -19.03943276465977164, -0.05219959533935918106, 58.75109039468566863 ) ) ;
#47782=CARTESIAN_POINT ( 'NONE',  ( 21.55341960407610458, 5.719274019375980345, 98.95724293864770971 ) ) ;
#47783=CARTESIAN_POINT ( 'NONE',  ( 16.55341960407611168, 4.379528057220329451, 93.95724293864770971 ) ) ;
#47784=CARTESIAN_POINT ( 'NONE',  ( 10.81492255796106328, -18.62759615963255655, 35.41775706135234003 ) ) ;
#47787=CARTESIAN_POINT ( 'NONE',  ( -4.379528057220328563, 16.55341960407611168, 30.20724293864769550 ) ) ;
#47788=CARTESIAN_POINT ( 'NONE',  ( 13.97604488694527802, 13.89961937509977652, 34.37390960531436690 ) ) ;
#47789=CARTESIAN_POINT ( 'NONE',  ( -19.05341960407611168, -5.049401038298163336, 81.45724293864769550 ) ) ;
#47790=CARTESIAN_POINT ( 'NONE',  ( 21.55341960407610458, 5.719274019375980345, 63.95724293864770260 ) ) ;
#47792=CARTESIAN_POINT ( 'NONE',  ( -19.02544592524342804, 5.153800228976336051, 36.04057627198100988 ) ) ;
#47793=CARTESIAN_POINT ( 'NONE',  ( 21.55341960407610458, 5.719274019375980345, 48.95724293864770971 ) ) ;
#47795=CARTESIAN_POINT ( 'NONE',  ( 10.72451020669871369, 18.67979575497193778, 72.08442372801899012 ) ) ;
#47797=CARTESIAN_POINT ( 'NONE',  ( -12.06949235617739369, -12.14591786802326823, 64.37609039468568994 ) ) ;
#47798=CARTESIAN_POINT ( 'NONE',  ( -9.564922557960796823, -16.46253265017161027, 52.08224293864768839 ) ) ;
#47799=CARTESIAN_POINT ( 'NONE',  ( 19.03943276465977164, -0.05219959533909143690, 58.74890960531435979 ) ) ;
#47801=CARTESIAN_POINT ( 'NONE',  ( 9.564922557961047289, -16.46253265017146816, 20.41775706135233293 ) ) ;
#47802=CARTESIAN_POINT ( 'NONE',  ( 16.55341960407618274, -4.379528057220086978, 76.04275706135237556 ) ) ;
#47803=CARTESIAN_POINT ( 'NONE',  ( 10.81492255796106328, -18.62759615963255655, 95.41775706135234714 ) ) ;
#47804=CARTESIAN_POINT ( 'NONE',  ( 0.05219959533909260263, 19.03943276465977164, 79.99890960531436690 ) ) ;
#47805=CARTESIAN_POINT ( 'NONE',  ( 21.55341960407610458, 5.719274019375980345, 38.95724293864768839 ) ) ;
#47806=CARTESIAN_POINT ( 'NONE',  ( -19.05341960407617563, 5.049401038297882671, 113.5427570613523471 ) ) ;
#47807=CARTESIAN_POINT ( 'NONE',  ( 18.62759615963255655, 10.81492255796105972, 81.66775706135236135 ) ) ;
#47808=CARTESIAN_POINT ( 'NONE',  ( -14.34966873604972548, 8.224510206698743886, 43.33442372801901143 ) ) ;
#47809=CARTESIAN_POINT ( 'NONE',  ( 21.55341960407610458, 5.719274019375980345, 93.95724293864770971 ) ) ;
#47810=CARTESIAN_POINT ( 'NONE',  ( -13.89961937509957401, -13.97604488694547875, 109.3760903946856331 ) ) ;
#47811=CARTESIAN_POINT ( 'NONE',  ( -5.153800228976328057, -19.02544592524343514, 77.29057627198099567 ) ) ;
#47813=CARTESIAN_POINT ( 'NONE',  ( -9.564922557961040184, 16.46253265017147172, 112.9177570613523329 ) ) ;
#47814=CARTESIAN_POINT ( 'NONE',  ( -16.46253265017160317, 9.564922557960807481, 40.83224293864769550 ) ) ;
#47815=CARTESIAN_POINT ( 'NONE',  ( -16.53943276465976808, -0.05219959533934237506, 23.75109039468567929 ) ) ;
#47816=CARTESIAN_POINT ( 'NONE',  ( -16.52544592524342804, 4.483927247898546575, 66.04057627198103830 ) ) ;
#47817=CARTESIAN_POINT ( 'NONE',  ( 8.314922557961029526, -14.29746914071037800, 75.41775706135233293 ) ) ;
#47818=CARTESIAN_POINT ( 'NONE',  ( 18.62759615963255655, 10.81492255796105972, 26.66775706135235424 ) ) ;
#47819=CARTESIAN_POINT ( 'NONE',  ( -19.02544592524342804, 5.153800228976336051, 46.04057627198101699 ) ) ;
#47820=CARTESIAN_POINT ( 'NONE',  ( -13.97604488694527625, -13.89961937509977652, 66.87390960531436690 ) ) ;
#47821=CARTESIAN_POINT ( 'NONE',  ( 4.483927247898790824, -16.52544592524335698, 70.20942372801904696 ) ) ;
#47823=ORIENTED_EDGE ( 'NONE', *, *, #186744, .T. ) ;
#47824=CARTESIAN_POINT ( 'NONE',  ( -0.05219959533936034679, 19.03943276465977164, 22.50109039468566152 ) ) ;
#47825=CARTESIAN_POINT ( 'NONE',  ( 0.05219959533909260263, 19.03943276465977164, 34.99890960531435979 ) ) ;
#47826=CARTESIAN_POINT ( 'NONE',  ( 5.153800228976335163, 19.02544592524342804, 104.7905762719809957 ) ) ;
#47827=ORIENTED_EDGE ( 'NONE', *, *, #116452, .F. ) ;
#47828=CARTESIAN_POINT ( 'NONE',  ( 8.314922557961029526, -14.29746914071037800, 35.41775706135234003 ) ) ;
#47829=CARTESIAN_POINT ( 'NONE',  ( 5.153800228976615827, -19.02544592524334988, 55.20942372801899722 ) ) ;
#47830=CARTESIAN_POINT ( 'NONE',  ( -0.05219959533934338120, 16.53943276465976808, 37.50109039468568284 ) ) ;
#47831=CARTESIAN_POINT ( 'NONE',  ( -13.97604488694527625, -13.89961937509977652, 36.87390960531436690 ) ) ;
#47832=CARTESIAN_POINT ( 'NONE',  ( -9.474510206698964154, 16.51473224551069663, 110.4155762719810383 ) ) ;
#47833=CARTESIAN_POINT ( 'NONE',  ( 13.89961937509977652, -13.97604488694527269, 58.12390960531436690 ) ) ;
#47834=CARTESIAN_POINT ( 'NONE',  ( 18.62759615963271287, -10.81492255796078972, 103.3322429386476955 ) ) ;
#47835=CARTESIAN_POINT ( 'NONE',  ( 9.564922557960805705, 16.46253265017160317, 89.58224293864769550 ) ) ;
#47836=CARTESIAN_POINT ( 'NONE',  ( 16.51473224551069308, 9.474510206698969483, 109.1655762719810383 ) ) ;
#47837=CARTESIAN_POINT ( 'NONE',  ( 19.05341960407611168, 5.049401038298154454, 58.95724293864768129 ) ) ;
#47838=CARTESIAN_POINT ( 'NONE',  ( 4.483927247898790824, -16.52544592524335698, 110.2094237280190185 ) ) ;
#47839=CARTESIAN_POINT ( 'NONE',  ( -18.22780087662122028, 5.500000000000031086, 93.51540105326107266 ) ) ;
#47840=CARTESIAN_POINT ( 'NONE',  ( -9.474510206698720793, -16.51473224551083518, 99.58442372801900433 ) ) ;
#47841=CARTESIAN_POINT ( 'NONE',  ( 5.153800228976615827, -19.02544592524334988, 20.20942372801899722 ) ) ;
#47842=CARTESIAN_POINT ( 'NONE',  ( 4.483927247898545687, 16.52544592524342804, 54.79057627198104541 ) ) ;
#47843=CARTESIAN_POINT ( 'NONE',  ( -18.67979575497193778, 10.72451020669871902, 93.33442372801901854 ) ) ;
#47844=CARTESIAN_POINT ( 'NONE',  ( -5.049401038298153566, 19.05341960407611168, 40.20724293864768839 ) ) ;
#47845=CARTESIAN_POINT ( 'NONE',  ( -8.224510206698948167, 14.34966873604960824, 25.41557627198103120 ) ) ;
#47846=CARTESIAN_POINT ( 'NONE',  ( -21.52544592524334988, -5.823673210054445271, 88.95942372801901854 ) ) ;
#47847=CARTESIAN_POINT ( 'NONE',  ( -19.02544592524342804, 5.153800228976336051, 76.04057627198102409 ) ) ;
#47848=CARTESIAN_POINT ( 'NONE',  ( 0.05219959533909260263, 19.03943276465977164, 89.99890960531436690 ) ) ;
#47849=CARTESIAN_POINT ( 'NONE',  ( 8.224510206698953496, -14.34966873604960469, 97.91557627198103830 ) ) ;
#47850=CARTESIAN_POINT ( 'NONE',  ( 14.29746914071049879, -8.314922557960816363, 63.33224293864770260 ) ) ;
#47851=CARTESIAN_POINT ( 'NONE',  ( 18.62759615963271287, -10.81492255796078972, 68.33224293864769550 ) ) ;
#47852=CARTESIAN_POINT ( 'NONE',  ( 0.05219959533909260263, 19.03943276465977164, 79.99890960531436690 ) ) ;
#47853=CARTESIAN_POINT ( 'NONE',  ( 21.53943276465977519, -0.05219959533907433946, 88.74890960531436690 ) ) ;
#47854=CARTESIAN_POINT ( 'NONE',  ( 16.51473224551083163, -9.474510206698727899, 80.83442372801899012 ) ) ;
#47856=CARTESIAN_POINT ( 'NONE',  ( 8.224510206698953496, -14.34966873604960469, 92.91557627198103830 ) ) ;
#47857=CARTESIAN_POINT ( 'NONE',  ( 5.153800228976335163, 19.02544592524342804, 54.79057627198103120 ) ) ;
#47858=CARTESIAN_POINT ( 'NONE',  ( 5.823673210054125526, 21.52544592524343514, 64.79057627198103830 ) ) ;
#47859=CARTESIAN_POINT ( 'NONE',  ( 16.19135201231362586, -7.376712067592066546, 27.31319145947968607 ) ) ;
#47860=CARTESIAN_POINT ( 'NONE',  ( -14.34966873604972548, 8.224510206698743886, 113.3344237280190328 ) ) ;
#47862=CARTESIAN_POINT ( 'NONE',  ( 9.474510206698729675, 16.51473224551082808, 112.0844237280190043 ) ) ;
#47863=CARTESIAN_POINT ( 'NONE',  ( 4.483927247898545687, 16.52544592524342804, 79.79057627198102409 ) ) ;
#47864=CARTESIAN_POINT ( 'NONE',  ( -19.25918095147779852, -5.499999999999533706, 94.45284276293934056 ) ) ;
#47865=CARTESIAN_POINT ( 'NONE',  ( 13.89961937509977652, -13.97604488694527269, 73.12390960531436690 ) ) ;
#47866=CARTESIAN_POINT ( 'NONE',  ( 16.46253265017160672, -9.564922557960803928, 38.33224293864768839 ) ) ;
#47867=CARTESIAN_POINT ( 'NONE',  ( 12.06949235617757843, -12.14591786802309237, 63.12390960531435979 ) ) ;
#47868=CARTESIAN_POINT ( 'NONE',  ( 19.03943276465977164, -0.05219959533909143690, 98.74890960531436690 ) ) ;
#47869=CARTESIAN_POINT ( 'NONE',  ( -19.03943276465977164, -0.05219959533935918106, 93.75109039468566152 ) ) ;
#47870=CARTESIAN_POINT ( 'NONE',  ( 19.03943276465977164, -0.05219959533909143690, 68.74890960531436690 ) ) ;
#47871=CARTESIAN_POINT ( 'NONE',  ( 19.05341960407611168, 5.049401038298154454, 88.95724293864769550 ) ) ;
#47872=CARTESIAN_POINT ( 'NONE',  ( 0.05219959533907565091, 21.53943276465977519, 74.99890960531435269 ) ) ;
#47873=CARTESIAN_POINT ( 'NONE',  ( -12.06949235617739369, -12.14591786802326823, 69.37609039468567573 ) ) ;
#47874=CARTESIAN_POINT ( 'NONE',  ( -5.049401038297874678, -19.05341960407618274, 109.7927570613523329 ) ) ;
#47875=CARTESIAN_POINT ( 'NONE',  ( 16.46253265017160672, -9.564922557960803928, 63.33224293864769550 ) ) ;
#47876=CARTESIAN_POINT ( 'NONE',  ( 15.72974639402199770, -15.80617190586745480, 73.12390960531436690 ) ) ;
#47877=CARTESIAN_POINT ( 'NONE',  ( 19.03943276465977164, 0.05219959533936151252, 91.25109039468566152 ) ) ;
#47878=CARTESIAN_POINT ( 'NONE',  ( -16.52544592524342804, 4.483927247898546575, 41.04057627198103120 ) ) ;
#47879=CARTESIAN_POINT ( 'NONE',  ( -21.52544592524334988, -5.823673210054445271, 43.95942372801902565 ) ) ;
#47881=CARTESIAN_POINT ( 'NONE',  ( 14.34966873604972726, -8.224510206698740333, 70.83442372801901854 ) ) ;
#47882=CARTESIAN_POINT ( 'NONE',  ( 19.02544592524343514, -5.153800228976328945, 108.5405762719810383 ) ) ;
#47883=CARTESIAN_POINT ( 'NONE',  ( -19.03943276465977164, 0.05219959533909376836, 106.2489096053143669 ) ) ;
#47885=CARTESIAN_POINT ( 'NONE',  ( -8.314922557961024197, 14.29746914071037800, 87.91775706135234714 ) ) ;
#47886=CARTESIAN_POINT ( 'NONE',  ( 12.14591786802327356, -12.06949235617739191, 45.62609039468567573 ) ) ;
#47887=CARTESIAN_POINT ( 'NONE',  ( -5.049401038298153566, 19.05341960407611168, 55.20724293864769550 ) ) ;
#47888=CARTESIAN_POINT ( 'NONE',  ( -16.51473224551069308, -9.474510206698971260, 56.66557627198103120 ) ) ;
#47889=CARTESIAN_POINT ( 'NONE',  ( -15.80617190586768217, 15.72974639402176855, 48.12609039468568284 ) ) ;
#47890=CARTESIAN_POINT ( 'NONE',  ( 8.314922557961029526, -14.29746914071037800, 60.41775706135235424 ) ) ;
#47891=CARTESIAN_POINT ( 'NONE',  ( 0.05219959533910956823, 16.53943276465976808, 39.99890960531436690 ) ) ;
#47892=CARTESIAN_POINT ( 'NONE',  ( -5.049401038298153566, 19.05341960407611168, 45.20724293864769550 ) ) ;
#47893=CARTESIAN_POINT ( 'NONE',  ( -19.03943276465977164, 0.05219959533909376836, 31.24890960531435979 ) ) ;
#47894=CARTESIAN_POINT ( 'NONE',  ( -16.53943276465976808, -0.05219959533934237506, 33.75109039468568284 ) ) ;
#47895=CARTESIAN_POINT ( 'NONE',  ( 19.03943276465977164, 0.05219959533936151252, 76.25109039468566152 ) ) ;
#47896=CARTESIAN_POINT ( 'NONE',  ( -16.55341960407611168, -4.379528057220339221, 81.45724293864769550 ) ) ;
#47897=CARTESIAN_POINT ( 'NONE',  ( -13.97604488694527625, -13.89961937509977652, 51.87390960531436690 ) ) ;
#47898=CARTESIAN_POINT ( 'NONE',  ( -19.05341960407617563, 5.049401038297882671, 83.54275706135233293 ) ) ;
#47900=CARTESIAN_POINT ( 'NONE',  ( 21.52544592524334988, 5.823673210054432836, 86.45942372801901854 ) ) ;
#47901=CARTESIAN_POINT ( 'NONE',  ( -14.34966873604972548, 8.224510206698743886, 58.33442372801901143 ) ) ;
#47902=CARTESIAN_POINT ( 'NONE',  ( 16.79531203550649820, 7.028104445595489302, 38.75244988220443787 ) ) ;
#47903=CARTESIAN_POINT ( 'NONE',  ( -10.72451020669898014, 18.67979575497178502, 45.41557627198103830 ) ) ;
#47904=CARTESIAN_POINT ( 'NONE',  ( -14.34966873604972548, 8.224510206698743886, 43.33442372801901143 ) ) ;
#47906=CARTESIAN_POINT ( 'NONE',  ( 13.97604488694548053, -13.89961937509957401, 25.62609039468566507 ) ) ;
#47907=CARTESIAN_POINT ( 'NONE',  ( -19.05341960407611168, -5.049401038298163336, 71.45724293864766707 ) ) ;
#47909=CARTESIAN_POINT ( 'NONE',  ( 19.05341960407611168, 5.049401038298154454, 53.95724293864770260 ) ) ;
#47911=CARTESIAN_POINT ( 'NONE',  ( -16.46253265017160317, 9.564922557960807481, 65.83224293864769550 ) ) ;
#47912=CARTESIAN_POINT ( 'NONE',  ( -18.56399227203345603, -5.499999999999828582, 53.97830131249904184 ) ) ;
#47913=CARTESIAN_POINT ( 'NONE',  ( 19.02544592524334988, 5.153800228976608722, 31.45942372801900433 ) ) ;
#47914=CARTESIAN_POINT ( 'NONE',  ( 21.55341960407619695, -5.719274019375665929, 111.0427570613523613 ) ) ;
#47915=CARTESIAN_POINT ( 'NONE',  ( 12.14591786802309770, 12.06949235617756955, 34.37390960531435979 ) ) ;
#47916=CARTESIAN_POINT ( 'NONE',  ( -16.46253265017160317, 9.564922557960807481, 45.83224293864769550 ) ) ;
#47917=CARTESIAN_POINT ( 'NONE',  ( 13.89961937509977652, -13.97604488694527269, 103.1239096053143527 ) ) ;
#47918=CARTESIAN_POINT ( 'NONE',  ( 21.52544592524334988, 5.823673210054432836, 76.45942372801901854 ) ) ;
#47919=CARTESIAN_POINT ( 'NONE',  ( 9.564922557960805705, 16.46253265017160317, 54.58224293864769550 ) ) ;
#47920=CARTESIAN_POINT ( 'NONE',  ( 21.55341960407619695, -5.719274019375665929, 81.04275706135236135 ) ) ;
#47921=CARTESIAN_POINT ( 'NONE',  ( -21.55341960407610458, -5.719274019375992779, 21.45724293864769550 ) ) ;
#47922=CARTESIAN_POINT ( 'NONE',  ( 9.474510206698971260, -16.51473224551069308, 32.91557627198102409 ) ) ;
#47923=CARTESIAN_POINT ( 'NONE',  ( -5.719274019375665041, -21.55341960407619695, 29.79275706135234358 ) ) ;
#47924=CARTESIAN_POINT ( 'NONE',  ( -9.474510206698720793, -16.51473224551083518, 49.58442372801899722 ) ) ;
#47925=CARTESIAN_POINT ( 'NONE',  ( 0.05219959533909260263, 19.03943276465977164, 34.99890960531435979 ) ) ;
#47926=CARTESIAN_POINT ( 'NONE',  ( 5.049401038298161559, -19.05341960407611168, 77.70724293864765286 ) ) ;
#47927=CARTESIAN_POINT ( 'NONE',  ( 19.02544592524334988, 5.153800228976608722, 111.4594237280190043 ) ) ;
#47928=CARTESIAN_POINT ( 'NONE',  ( 16.55341960407611168, 4.379528057220329451, 73.95724293864769550 ) ) ;
#47929=CARTESIAN_POINT ( 'NONE',  ( 15.80617190586746368, 15.72974639402197994, 34.37390960531435979 ) ) ;
#47930=CARTESIAN_POINT ( 'NONE',  ( 16.51473224551083163, -9.474510206698727899, 105.8344237280190043 ) ) ;
#47931=CARTESIAN_POINT ( 'NONE',  ( 21.52544592524344225, -5.823673210054117533, 98.54057627198105251 ) ) ;
#47932=CARTESIAN_POINT ( 'NONE',  ( -18.67979575497193778, 10.72451020669871902, 58.33442372801901143 ) ) ;
#47933=CARTESIAN_POINT ( 'NONE',  ( 16.52544592524335698, 4.483927247898782831, 51.45942372801901854 ) ) ;
#47934=CARTESIAN_POINT ( 'NONE',  ( -14.29746914071037622, -8.314922557961029526, 59.16775706135234714 ) ) ;
#47935=CARTESIAN_POINT ( 'NONE',  ( -18.67979575497178146, -10.72451020669898902, 66.66557627198102409 ) ) ;
#47936=EDGE_LOOP ( 'NONE', ( #45535, #23772 ) ) ;
#47937=( BOUNDED_SURFACE ( )  B_SPLINE_SURFACE ( 3, 2, ( 
 ( #91823, #157250, #18744, #60503, #45355, #122178, #183870, #173422, #34892, #107007, #153516, #15013, #200032, #49080, #61500, #71224, #68211, #35882, #99546, #114720, #39874, #86383, #101541, #98536, #175403, #38889, #177418, #132887, #23724, #161228, #5537, #55050, #67216, #100546, #20711, #22722, #144055, #193578, #36871, #84370, #24733, #128874, #85373, #176412, #160229, #7531, #129863, #162225, #82367, #148067, #146047, #147066, #83373, #130884, #9558, #159216, #131894, #190574, #69216, #163233, #117725, #194576, #52050, #113706, #54057, #56046, #37888, #191561, #97529, #8549, #21720, #192573, #70226, #115731, #116721, #178410, #53040, #145050, #6531, #74220, #14517, #58052, #153018, #61008, #13527, #12554, #87384, #150063, #198550, #90357, #76178, #137858, #135888, #25738, #165236, #133896, #199538, #179420, #166231, #41895, #40885, #59027, #26730, #102558, #72221, #43871, #42884, #164243, #197560, #10557, #152042, #134905, #149069, #75193, #120694, #60020, #182393, #195587, #57059, #136864, #11568, #118734, #180422, #121687, #105536, #28720, #73234, #103561, #183383, #88369, #91326, #196582, #119723, #181406, #44865, #104549, #27731, #89374, #151063, #167222, #106520, #168198, #29695, #32670, #93328, #4291, #125667, #123658, #107503, #156001, #126642, #17498, #138844, #111487, #30685, #33655, #46846, #187365, #62993, #324, #61992, #185355, #108506, #110487, #170185, #49823, #172170, #173172, #157001, #1314, #140826, #79155, #48834, #139825, #34648, #142811, #96307, #122680, #94323, #92336, #154022, #81130, #186368, #141818, #95316, #45850, #109500, #31679, #155013, #16509, #78157, #124671, #18499, #47847, #171182, #15517, #188344, #77174, #80147, #64984, #2315, #169179, #63997, #157993, #3311, #19485, #184369, #116479, #145803, #53809, #54804, #84124, #147830, #7286, #127642, #23476, #189342, #177172, #158973, #69980, #100302, #66972, #20465, #38645, #36623, #50820, #112477, #128632, #86139, #129621, #115484, #99296, #8303, #174170, #82115, #143806, #101293, #68970, #161980, #35640, #130634, #97286, #191316, #65972, #193330, #5289, #192328, #85125, #51803, #178168, #24488, #190326, #146809, #144805, #159981, #113462, #131648, #175156, #39633, #162983, #98280, #21467, #83129, #6288, #67967, #52793, #114461, #176163, #37633, #160982, #22476, #149815, #120455, #72991, #9316, #165990, #132649, #181168, #179175, #89133, #42645, #25498, #40643, #104307, #71972, #70981, #117477, #148825, #194337, #26489, #27490, #134660, #12318, #102312, #87141, #10315, #55805, #150821, #73983, #133646, #135652, #195337, #196346, #164002, #56817, #103315, #118491, #180182, #119486, #41651, #164995, #197323, #58786, #88131, #11321, #57814, #119260, #151587, #42420, #30221, #135433, #122218, #41421, #181927, #73761, #43408, #87904, #137393, #180944, #149590, #166764, #27259, #138389, #59551, #57590, #103087, #89904, #60542, #13076, #72765, #45394, #164768, #167745, #104083, #121229, #197104, #134435, #196120, #165765, #88909, #44405, #150600, #183909, #106059, #107047, #90876, #58571, #74743, #136406, #182920, #120236, #168719, #76714, #91863, #56590, #28266, #26263, #11088, #15053, #105078, #75715, #29243, #179954, #198084, #12098, #152560, #14049, #199073, #153556, #118264, #157546, #139376, #125218, #188893, #92869, #49368, #140375, #124205, #171722, #32215, #2861, #184898, #50373, #48386, #64539, #47390, #94870, #112033, #123208, #95863, #154556, #33211, #65522, #81660, #127182, #16051, #169725, #18050, #158529, #1862, #155550, #35190, #79703, #126205, #858, #63544, #186915, #141374, #110043, #17044, #93871, #20017, #170723, #3843, #78698, #173722, #200071, #34201, #156551, #108039, #187901, #19040, #111032, #96844, #61539, #172719, #46380, #185905, #77710, #31218, #62532, #80687, #109045, #142363, #23017, #190865, #25031, #36171, #7829, #6827, #178707, #99841, #174707, #54348, #98830, #189879, #116019 ),
 ( #115017, #51354, #113014, #101845, #68505, #162517, #146341, #66518, #130160, #5835, #52342, #67511, #160524, #37172, #177709, #22015, #83667, #97823, #147361, #159512, #131180, #85674, #129168, #21008, #82663, #8849, #144347, #39176, #70517, #193876, #84663, #192869, #132185, #161525, #143343, #69515, #4831, #100834, #176711, #113998, #175696, #163531, #191857, #24019, #55342, #128180, #53339, #145345, #38185, #117012, #40169, #180717, #120993, #165535, #42193, #56344, #90657, #179716, #74516, #29017, #10855, #133181, #194871, #152339, #118026, #59324, #13825, #137164, #166536, #136182, #75491, #104845, #168499, #28033, #148358, #44176, #9854, #197857, #41188, #198853, #182691, #87674, #102851, #105835, #57361, #71513, #164536, #149358, #106825, #150373, #167522, #120012, #60317, #26029, #72524, #134199, #121994, #89674, #183684, #195887, #151361, #119035, #11868, #86675, #45169, #103854, #12850, #27031, #88677, #73533, #135205, #196877, #58344, #181697, #43178, #153324, #79472, #92637, #124984, #15817, #3612, #108812, #95627, #14826, #155324, #47154, #16812, #61312, #110801, #154328, #122982, #140136, #625, #111797, #32980, #30989, #76487, #63305, #33970, #186681, #46151, #18809, #138164, #141140, #77478, #94634, #170491, #107805, #169489, #139148, #62296, #17815, #123964, #157312, #2630, #80454, #64307, #31982, #48151, #109808, #156313, #93638, #142127, #50138, #65291, #29997, #171491, #125974, #185662, #126950, #78462, #91636, #1628, #187673, #188658, #199846, #184669, #49143, #172482, #176475, #114782, #70289, #161289, #36936, #143115, #192635, #4594, #37949, #158299, #98599, #81429, #130945, #112782, #160292, #162288, #66287, #22783, #113769, #97590, #145111, #5598, #99609, #19788, #23788, #21783, #84431, #20774, #68273, #85438, #96610, #69278, #127946, #6594, #38949, #55113, #100606, #189648, #51123, #191624, #131957, #175465, #128936, #8616, #53103, #146108, #174475, #83434, #129924, #7592, #54117, #190637, #67278, #193641, #144118, #177480, #52112, #147129, #173485, #115791, #34958, #35944, #159278, #82430, #30486, #93134, #154819, #150132, #163300, #102624, #71289, #16317, #77967, #103627, #179488, #139634, #196648, #164310, #1122, #9624, #184176, #180489, #116783, #73301, #148133, #92137, #72286, #24799, #153824, #58118, #130, #134971, #178474, #132954, #15319, #87449, #101610, #86447, #76978, #194642, #138649, #45658, #11634, #57127, #122485, #107309, #169991, #133963, #56112, #10625, #168982, #61799, #123469, #39941, #117793, #108311, #40952, #185161, #25803, #46652, #118801, #149134, #195655, #41961, #165303, #31482, #26796, #88438, #50631, #113278, #97102, #141637, #80950, #19302, #189158, #79969, #174969, #82938, #190138, #144616, #34464, #170986, #32479, #21281, #126463, #81920, #65783, #186174, #49634, #125483, #171984, #187179, #18312, #156820, #158786, #3127, #64802, #94132, #66780, #155811, #112292, #5097, #48650, #109307, #17309, #128441, #78964, #35451, #51613, #36433, #142625, #173982, #98088, #4104, #62796, #127452, #124478, #20274, #47656, #143613, #140639, #159786, #2129, #63810, #110302, #33472, #95130, #188161, #111297, #172986, #96123, #157812, #194148, #39442, #148633, #191136, #160796, #99104, #41457, #24297, #55612, #114271, #70789, #175975, #131450, #26298, #133453, #37444, #132457, #178980, #192133, #85945, #6100, #117286, #40447, #102121, #176983, #129437, #163805, #68777, #101102, #53614, #179990, #84931, #71783, #52609, #193137, #23287, #54610, #22284, #86949, #130434, #83935, #116284, #38453, #87939, #9123, #7095, #145616, #162788, #10123, #147634, #115290, #25307, #195143, #56624, #100108, #161792, #146612, #103122, #118298, #164803, #8104, #67780, #69782, #177974, #169755, #76745, #57627, #75749, #122249, #135467, #167777, #149626, #137426, #199106, #60573, #120268, #72799, #183939, #12130, #44437, #197135, #123237, #28298, #15084, #134469, #74776 ),
 ( #153586, #182954, #165799, #138420, #119294, #45424, #73794, #152592, #89938, #27296, #88943, #58602, #150634, #107077, #181960, #200100, #168749, #61568, #30252, #151619, #29275, #106091, #91895, #166797, #184928, #31250, #46413, #11124, #121260, #180977, #42453, #108071, #13112, #196154, #14083, #104117, #136438, #43442, #105111, #198119, #59586, #90907, #127211, #171753, #186946, #62563, #96872, #185935, #80716, #35219, #17075, #139406, #888, #158556, #124240, #65552, #20046, #143371, #172750, #142394, #81689, #111062, #174737, #34231, #154586, #50403, #16082, #3873, #47420, #4863, #188925, #93902, #109076, #112063, #63574, #77740, #170755, #155580, #113045, #156584, #173751, #32244, #18079, #66548, #78729, #128212, #33242, #140405, #64570, #125248, #95893, #1894, #189909, #141403, #157576, #48417, #187930, #51384, #110073, #92900, #94900, #126235, #79734, #2891, #49399, #19069, #5865, #54379, #194901, #176742, #191888, #71544, #116051, #39209, #175727, #38215, #161555, #177740, #23048, #53372, #130192, #56375, #6858, #40200, #115050, #9884, #118058, #70549, #69547, #144378, #68537, #55372, #147393, #133210, #36200, #131211, #82694, #22047, #190897, #97854, #159543, #84693, #98862, #21041, #100865, #83698, #67541, #129199, #162547, #99871, #52373, #192902, #114030, #8881, #146373, #37206, #132216, #24051, #117042, #85707, #160557, #145376, #193908, #7860, #178737, #101880, #163562, #25062, #86705, #148390, #12879, #120039, #59353, #182719, #30025, #135233, #26058, #73560, #29045, #167550, #198880, #76516, #72552, #121022, #136209, #57390, #14855, #11897, #179748, #43207, #58372, #183712, #91663, #45198, #42221, #119063, #44204, #105863, #138192, #90685, #104874, #149386, #60347, #10882, #152367, #164564, #166563, #87701, #134230, #122021, #195915, #13852, #180745, #28062, #103882, #137194, #165562, #89703, #168527, #27059, #75519, #181726, #88705, #151389, #196905, #106852, #150401, #153353, #74544, #199875, #197884, #61339, #41218, #102879, #18838, #15848, #156343, #188687, #4623, #50167, #77507, #92667, #141170, #81457, #63337, #78493, #158327, #2659, #126005, #62324, #125014, #48181, #64336, #109837, #140166, #16843, #143143, #93668, #126978, #1659, #96639, #123010, #157343, #17843, #31017, #155353, #142157, #33999, #19816, #184696, #79501, #169517, #108841, #139178, #46180, #107833, #171520, #185692, #154355, #187701, #170522, #654, #123994, #49171, #186710, #47182, #110830, #32011, #95655, #33009, #94664, #80483, #172514, #3641, #65319, #111825, #173513, #34986, #36967, #51150, #174504, #23820, #82458, #85470, #130975, #99639, #6625, #146139, #69309, #116815, #21813, #112811, #160322, #115822, #54149, #147159, #163333, #159308, #7625, #22815, #144146, #101642, #98628, #66314, #129955, #145142, #70321, #178506, #131988, #128966, #5630, #192666, #177512, #24829, #38982, #191655, #35971, #97618, #86479, #53134, #8647, #100638, #189678, #114813, #190666, #175494, #52142, #83465, #68304, #162319, #176505, #37982, #20803, #193673, #67307, #55144, #39972, #113799, #161322, #84461, #148164, #127975, #182489, #136962, #60117, #89473, #197657, #198651, #27832, #91427, #151164, #71321, #167321, #132984, #120789, #102655, #13624, #43970, #10656, #164340, #105632, #180519, #194675, #56144, #72319, #29791, #73332, #59123, #42982, #152141, #117825, #25835, #87479, #44963, #12652, #28817, #179518, #74319, #40987, #135004, #9655, #121785, #149166, #135986, #90457, #195686, #75291, #133995, #183479, #106621, #168295, #41992, #57157, #118836, #103658, #165336, #26828, #88469, #150166, #11666, #196682, #104647, #58151, #119819, #181504, #166334, #126737, #188440, #186468, #199636, #138937, #107600, #49919, #111584, #139923, #15611, #173269, #32767, #417, #34743, #45945, #17597, #16603, #153114, #109596, #184466, #64094, #108603, #61103, #125762, #94419, #33755, #171279, #14618, #169278, #187462, #123754 ),
 ( #3404, #156099, #140928, #141913, #79256, #76275, #2414, #137953, #110584, #122776, #48930, #30784, #157099, #172265, #154118, #92431, #95414, #185453, #77268, #62091, #46943, #170280, #78250, #18595, #47945, #80243, #31774, #93422, #155109, #1412, #65079, #63091, #124770, #161078, #66071, #21566, #116577, #23575, #4386, #22573, #69067, #82214, #114565, #96402, #84220, #145899, #7383, #67070, #19581, #130734, #192426, #129717, #85223, #144901, #175254, #162081, #81224, #83226, #113560, #6384, #127737, #177271, #20563, #189439, #68063, #128729, #178266, #99395, #97383, #142905, #191414, #100400, #52890, #112574, #146914, #50916, #53908, #143905, #115583, #36720, #174268, #35736, #159069, #5387, #38742, #190425, #8403, #70078, #131746, #193428, #98382, #176262, #37733, #54904, #160079, #158089, #51901, #167077, #121543, #11418, #147925, #9411, #198399, #103412, #58885, #42743, #163083, #26584, #102410, #148923, #164097, #195438, #133743, #74077, #118588, #56913, #71077, #43729, #132743, #27590, #182244, #25596, #39729, #89228, #166087, #150922, #10412, #24587, #12415, #135748, #73088, #28579, #88227, #180278, #105391, #86235, #165090, #41748, #149911, #194431, #120551, #87240, #55902, #134759, #72070, #101390, #104405, #40740, #117575, #196441, #90215, #57911, #179275, #151898, #119583, #197419, #181266, #13388, #75052, #136718, #59877, #45707, #122535, #171037, #169031, #110349, #32528, #33519, #17357, #61849, #1170, #139683, #109355, #181, #95179, #3175, #172031, #64848, #154870, #91187, #152876, #141684, #46702, #2178, #186224, #106375, #170042, #107358, #92189, #30537, #138699, #77027, #79012, #123518, #185211, #14371, #187226, #76037, #94180, #125529, #153873, #29554, #137712, #48697, #199396, #155859, #156866, #18362, #62845, #140686, #80015, #124529, #183238, #47705, #44719, #63858, #168057, #60860, #184226, #15371, #108364, #31532, #93185, #16367, #78015, #188208, #173035, #127501, #149419, #190188, #117074, #162580, #71576, #111344, #81000, #19351, #164596, #147426, #178770, #34513, #193941, #96171, #51663, #10915, #56410, #157861, #55404, #101912, #112341, #8913, #87734, #113327, #148422, #132250, #49680, #175020, #189206, #35502, #50683, #81972, #20323, #163594, #5147, #143665, #142674, #133242, #4153, #40236, #194934, #174031, #65832, #97152, #118091, #158835, #25095, #179781, #41250, #70581, #86737, #102912, #9917, #126510, #26090, #66829, #128493, #39240, #100896, #24084, #85739, #106880, #73591, #27092, #45226, #43239, #134262, #119095, #135264, #92695, #136238, #60376, #105891, #14884, #57422, #88738, #165594, #107862, #90711, #122048, #180777, #137222, #42252, #197912, #154383, #199903, #103914, #198908, #168553, #58403, #152394, #72588, #183739, #30051, #91692, #104906, #195949, #153383, #76545, #167578, #61367, #121055, #151419, #138221, #150432, #59382, #89733, #182750, #11927, #123038, #196935, #120069, #44234, #166594, #181757, #75547, #28094, #12906, #29072, #184724, #13880, #74570, #46208, #169547, #31046, #140195, #18867, #156370, #93698, #32041, #78521, #155381, #3670, #1688, #143173, #65348, #66344, #50199, #94692, #34028, #172543, #142186, #33037, #128006, #36000, #4653, #97647, #187729, #124024, #185722, #127008, #188716, #186738, #139208, #111855, #173545, #49200, #189708, #64364, #17874, #81486, #683, #141198, #79528, #2687, #47212, #96669, #63365, #108871, #126033, #48209, #15878, #80513, #16870, #62354, #110858, #19845, #95686, #125042, #51181, #170551, #35014, #109863, #158357, #157373, #171548, #112841, #174533, #77536, #147186, #145171, #86506, #8676, #9684, #193702, #38012, #177541, #115851, #85498, #176536, #71349, #179546, #148190, #41016, #131003, #67335, #128997, #117853, #22843, #178532, #162347, #82489, #146168, #21842, #68333, #83494, #114842, #53164, #55172, #99668, #161352, #190695, #163361, #52170, #70348, #101671, #6655, #5659, #113827 ),
 ( #144173, #132015, #175522, #24857, #116842, #160352, #36997, #39999, #129983, #20833, #98658, #191683, #159336, #84490, #133013, #192695, #194703, #7653, #69337, #54178, #56172, #39010, #100665, #23848, #167347, #72348, #27860, #122804, #29819, #10684, #28844, #75317, #88500, #120818, #102682, #90485, #181530, #196708, #134022, #106650, #195714, #152167, #44990, #26858, #149194, #57187, #168322, #118863, #136988, #91455, #153143, #182518, #13650, #14645, #43998, #184494, #105660, #164367, #60144, #25862, #198677, #180546, #76305, #121812, #103685, #42020, #183507, #73361, #87506, #165364, #150196, #11694, #166363, #137983, #136011, #199666, #135033, #58178, #119845, #61131, #43009, #104676, #89501, #151190, #12678, #74345, #197683, #59148, #154148, #172295, #18624, #31803, #64126, #45973, #33784, #95444, #157128, #16633, #169305, #80271, #141941, #79287, #34774, #94449, #124800, #111615, #30811, #171310, #63121, #32797, #77298, #126766, #170310, #138968, #156129, #78280, #127766, #48959, #46973, #92460, #140957, #49951, #2444, #62121, #96431, #15640, #3432, #93452, #110613, #186498, #123784, #185483, #108632, #155140, #65108, #139953, #173300, #188470, #158117, #19609, #47974, #125791, #187493, #81251, #109626, #142933, #66100, #4414, #107627, #17628, #446, #1443, #147952, #52917, #8432, #192453, #112602, #176290, #51929, #98412, #113589, #144929, #83254, #23605, #35764, #6410, #38770, #177299, #70104, #86262, #82243, #69094, #145928, #67098, #24614, #21596, #189466, #114593, #68091, #193455, #39756, #54931, #175283, #128757, #53935, #130761, #9438, #100427, #37762, #159097, #131773, #20591, #115610, #174294, #99424, #97410, #146942, #190454, #161106, #178292, #143934, #162108, #129744, #36748, #22601, #191441, #85251, #5415, #101419, #84248, #116604, #160108, #7411, #163111, #71103, #50944, #25621, #166118, #198431, #14401, #59904, #87265, #102436, #150951, #91213, #73119, #88254, #168085, #12445, #135777, #72100, #134788, #57940, #74107, #119611, #149941, #27620, #152904, #75079, #117603, #11447, #106403, #132770, #167104, #89259, #40767, #103439, #151926, #43757, #29582, #194457, #197448, #179303, #118616, #148950, #55928, #164123, #181294, #195467, #10440, #58914, #180306, #133773, #56942, #120582, #196470, #41774, #182276, #165119, #105421, #42772, #26611, #28605, #90243, #13415, #136746, #104434, #121572, #183267, #44747, #199425, #122566, #140718, #169063, #2208, #171067, #1202, #170073, #186256, #47734, #172062, #185243, #109387, #76066, #63889, #60890, #17388, #107390, #48726, #125560, #15401, #30569, #79044, #123549, #184256, #45738, #153906, #141713, #154900, #94211, #62879, #187257, #92220, #77058, #138730, #18393, #32557, #155890, #210, #110379, #61879, #16399, #137741, #46735, #78045, #108396, #31564, #33549, #93215, #139714, #124559, #95211, #156897, #80044, #77533, #110855, #35997, #158353, #680, #94689, #189705, #97644, #50196, #49197, #124021, #186735, #35011, #127005, #51178, #112838, #172540, #62351, #1685, #170547, #174530, #15875, #2684, #78518, #139205, #95683, #63362, #185719, #108868, #80510, #79525, #47209, #34025, #32038, #188713, #171545, #93695, #111852, #157370, #96666, #18864, #155378, #16867, #173542, #48206, #140192, #125039, #19842, #109860, #81483, #142183, #3667, #156367, #65345, #143170, #66341, #33033, #17871, #141195, #4650, #128003, #64361, #126030, #187726, #39007, #115848, #36994, #194700, #191680, #159333, #22840, #38009, #163358, #9681, #24854, #21838, #98655, #162344, #100662, #56169, #147183, #84487, #128994, #178529, #190692, #23845, #71346, #114839, #5656, #53161, #8672, #70345, #39996, #117850, #52167, #85495, #177537, #160349, #179543, #176533, #20830, #146164, #99664, #86503, #133009, #148187, #83491, #145168, #132012, #193699, #41012, #55168, #7650, #113824, #101668, #175519, #116839, #144170, #69334, #67332, #82486, #6652, #131000 ),
 ( #68330, #129980, #161349, #192692, #54175, #120815, #152164, #10680, #167344, #72345, #27857, #122801, #29816, #134019, #28841, #75314, #88496, #182515, #102679, #90482, #13647, #59145, #183504, #168319, #136985, #198674, #136008, #91452, #151187, #181527, #153140, #87503, #89497, #119842, #12675, #195711, #44987, #26855, #57183, #74342, #73357, #184491, #105656, #103682, #149191, #197680, #106647, #43994, #118860, #14642, #180543, #60141, #150193, #121808, #43006, #42017, #165361, #11691, #135030, #76302, #137980, #199662, #61128, #164364, #25859, #196705, #58175, #104673, #166359, #154145, #3429, #62118, #65105, #110609, #79284, #186495, #125788, #15637, #64123, #4411, #47971, #1440, #81248, #187490, #48956, #185480, #109623, #155136, #171307, #172292, #107624, #140954, #66096, #188466, #30808, #124797, #19606, #127763, #80268, #2441, #77294, #16630, #126763, #157125, #142930, #45970, #33781, #92457, #31800, #443, #169302, #138965, #32793, #108629, #123781, #95441, #93449, #46970, #170307, #18621, #94446, #78277, #141938, #156126, #17625, #139950, #49948, #111612, #173297, #34771, #96428, #63118, #158114, #23602, #160105, #174291, #97407, #146939, #5412, #8429, #53932, #22598, #129741, #69091, #192450, #39753, #144926, #35761, #83251, #38767, #177296, #70101, #86259, #82240, #130758, #145925, #67095, #24611, #21592, #189463, #52914, #68088, #193452, #101415, #54928, #51926, #128754, #115607, #100424, #147949, #162105, #114590, #159094, #131770, #20588, #85248, #143930, #176287, #190451, #116601, #113586, #37759, #178289, #175280, #163108, #191438, #36745, #161103, #6407, #9435, #98409, #71100, #99420, #50941, #84245, #7408, #112599, #58670, #31315, #28368, #168816, #953, #17142, #62629, #90006, #169824, #14151, #29345, #105180, #139473, #151689, #123303, #77804, #59656, #182031, #43514, #124306, #166866, #108140, #186004, #47485, #15151, #184996, #109142, #153656, #132767, #76813, #197207, #92968, #120336, #46480, #13180, #170821, #154654, #136506, #74843, #16149, #106162, #198186, #121330, #183022, #155647, #199176, #32313, #30320, #93967, #44506, #167844, #90974, #152661, #138484, #75818, #137496, #200165, #60643, #122317, #184008, #45491, #107146, #61635, #91963, #64634, #96936, #78794, #66608, #4926, #35281, #159607, #144441, #143439, #174796, #112124, #67603, #127275, #157641, #5927, #63640, #3936, #95956, #65616, #110138, #21106, #2955, #171817, #188989, #49463, #160617, #81752, #79798, #125316, #173816, #82761, #158618, #94964, #129263, #187012, #189970, #126296, #128272, #19130, #156649, #18145, #48482, #51445, #33305, #141471, #190958, #113105, #52435, #36262, #80780, #20108, #97916, #114093, #142458, #175794, #98926, #37268, #140473, #50465, #187993, #111125, #1961, #172815, #34295, #25124, #145437, #8943, #84755, #131273, #146433, #177799, #116111, #86768, #191949, #147455, #42282, #149446, #130254, #148451, #194962, #7923, #40268, #22108, #9946, #71605, #178799, #102939, #87761, #133271, #118120, #55433, #10942, #70612, #100925, #72615, #6920, #132279, #39269, #193970, #53435, #164624, #69608, #115110, #117104, #192961, #103940, #56439, #23109, #68598, #101942, #26118, #163623, #38276, #134290, #176803, #179808, #54440, #41277, #162610, #99930, #161615, #24114, #195977, #85768, #57449, #119122, #180803, #83758, #199934, #44262, #183769, #122077, #91721, #182779, #15909, #185755, #92726, #47244, #137252, #73618, #135289, #124056, #29100, #184755, #168582, #88766, #152422, #28122, #74598, #89761, #121084, #59410, #61397, #105919, #167605, #196961, #169581, #58429, #153415, #107894, #151447, #11954, #120096, #31079, #181784, #138250, #154415, #77567, #45255, #14914, #139239, #106909, #165620, #30080, #27119, #123069, #150459, #76575, #43265, #714, #46240, #166620, #104933, #62386, #136266, #12934, #197941, #90739, #13910, #75576, #198938, #60405, #51211, #93728, #63395, #1719 ),
 ( #187760, #127039, #65379, #35044, #126063, #159368, #129025, #36030, #190726, #80543, #16900, #78551, #67366, #172573, #128036, #111885, #32072, #95717, #171578, #17904, #33067, #64395, #2718, #143203, #49230, #110888, #140226, #112872, #125072, #96698, #174563, #94722, #155410, #186769, #97679, #48239, #81516, #20865, #82522, #188746, #158387, #144204, #50231, #108902, #173575, #170581, #66376, #109894, #19876, #156400, #5690, #4684, #79559, #141227, #189738, #34059, #157404, #18897, #142217, #3700, #115879, #40026, #85527, #194731, #37028, #6684, #145201, #87535, #70376, #101699, #160383, #116870, #21873, #177569, #72376, #179574, #83523, #178561, #24886, #38041, #132044, #52199, #163389, #86535, #8706, #133041, #117883, #148219, #9713, #147215, #41044, #100693, #131035, #102709, #98689, #39037, #69366, #162374, #68362, #56201, #176566, #130013, #23876, #22872, #134050, #55201, #53196, #191712, #193733, #164398, #71377, #114871, #25890, #99697, #149222, #161381, #10713, #192724, #84519, #113857, #175553, #146196, #7682, #54208, #180575, #103713, #153171, #11721, #14673, #60171, #28871, #136037, #75345, #198704, #46001, #151217, #42049, #89529, #45018, #183534, #76334, #92488, #88529, #137014, #152194, #73389, #30841, #27887, #195742, #59177, #74372, #199695, #107656, #61160, #58204, #135061, #121840, #106678, #154177, #168351, #120846, #165393, #138011, #26886, #29847, #150225, #182545, #196737, #122832, #119873, #44027, #184521, #181558, #91484, #197712, #43036, #167375, #12706, #169333, #104702, #15668, #105688, #77327, #166391, #90512, #57216, #118890, #13678, #31831, #172323, #4441, #20621, #66129, #93481, #108660, #157158, #97440, #79315, #94476, #174323, #18653, #141971, #78308, #140984, #48001, #2472, #80299, #474, #33812, #159125, #81279, #123812, #17655, #112631, #138995, #173328, #95472, #47001, #109655, #158145, #49979, #35793, #62148, #3460, #185510, #124827, #155168, #170338, #16660, #125818, #1470, #139981, #65137, #186527, #63148, #171337, #126794, #64154, #32825, #188500, #187521, #48987, #156157, #34803, #111643, #96458, #19637, #110642, #142961, #127794, #189494, #50972, #146971, #115638, #22629, #162135, #85279, #132799, #37789, #128785, #176319, #131804, #70132, #101448, #179333, #175311, #23631, #38798, #160137, #117634, #114620, #82271, #145957, #161133, #86291, #194486, #147981, #144956, #21625, #8459, #193483, #40796, #54960, #7438, #51957, #163140, #113617, #116632, #67127, #69122, #190485, #39784, #83282, #130789, #71133, #36777, #178321, #84276, #6437, #53963, #99453, #24643, #98442, #55958, #192480, #9470, #129771, #177327, #102465, #5443, #164153, #68119, #100455, #143963, #191467, #52945, #180334, #195495, #43785, #184280, #166145, #181321, #60917, #105449, #28633, #165148, #27648, #134817, #89287, #167133, #87295, #120610, #45763, #168109, #10468, #104462, #199449, #107415, #59931, #58941, #133803, #196497, #44775, #136773, #122592, #25650, #182304, #72129, #11476, #41802, #148979, #56969, #12472, #88282, #118642, #90270, #73147, #103469, #26639, #151953, #150978, #149970, #13442, #74133, #135804, #57967, #121598, #198459, #75106, #106428, #183293, #119638, #42800, #29606, #197475, #91238, #152928, #14425, #76090, #137765, #77085, #126562, #185269, #188262, #33573, #2231, #109413, #48751, #172086, #19403, #124585, #15426, #62904, #18418, #156921, #49736, #65886, #61903, #110404, #125583, #46761, #4208, #1226, #169088, #32583, #47759, #173090, #81052, #34568, #31589, #108420, #95235, #80067, #127560, #141737, #94236, #138754, #111404, #236, #3227, #153932, #155917, #123574, #96224, #170095, #17412, #157913, #93239, #64901, #171092, #154924, #140743, #186280, #142728, #16422, #189262, #79069, #50737, #78069, #63913, #30594, #92247, #139737, #187281, #145720, #178079, #194252, #39546, #66883, #82026, #130545, #70896, #52711, #67884, #147742, #192243, #115400 ) ),
 .UNSPECIFIED., .T., .F., .T. ) 
 B_SPLINE_SURFACE_WITH_KNOTS ( ( 4, 3, 4 ),
 ( 3, 2, 2, 2, 2, 2, 2, 2, 2, 2, 2, 2, 2, 2, 2, 2, 2, 2, 2, 2, 2, 2, 2, 2, 2, 2, 2, 2, 2, 2, 2, 2, 2, 2, 2, 2, 2, 2, 2, 2, 2, 2, 2, 2, 2, 2, 2, 2, 2, 2, 2, 2, 2, 2, 2, 2, 2, 2, 2, 2, 2, 2, 2, 2, 2, 2, 2, 2, 2, 2, 2, 2, 2, 2, 2, 2, 2, 2, 2, 2, 2, 2, 2, 2, 2, 2, 2, 2, 2, 2, 2, 2, 2, 2, 2, 2, 2, 2, 2, 2, 2, 2, 2, 2, 2, 2, 2, 2, 2, 2, 2, 2, 2, 2, 2, 2, 2, 2, 2, 2, 2, 2, 2, 2, 2, 2, 2, 2, 2, 2, 2, 2, 2, 2, 2, 2, 2, 2, 2, 2, 2, 2, 2, 2, 2, 2, 2, 2, 2, 2, 2, 2, 2, 2, 2, 2, 2, 2, 2, 2, 2, 2, 2, 2, 2, 2, 2, 2, 2, 2, 2, 2, 2, 2, 2, 2, 2, 2, 2, 2, 2, 2, 2, 2, 2, 2, 2, 2, 2, 2, 2, 2, 2, 2, 2, 2, 2, 2, 2, 2, 2, 2, 2, 2, 2, 2, 2, 2, 2, 2, 2, 2, 2, 2, 2, 2, 2, 2, 2, 2, 2, 2, 2, 2, 2, 2, 2, 2, 3 ),
 ( 0.000000000000000000, 0.5000000000000000000, 1.000000000000000000 ),
 ( 0.000000000000000000, 0.004385964912280701511, 0.008771929824561403022, 0.01315789473684210453, 0.01754385964912280604, 0.02192982456140350755, 0.02631578947368420907, 0.03070175438596491058, 0.03508771929824561209, 0.03947368421052631360, 0.04385964912280701511, 0.04824561403508771662, 0.05263157894736841813, 0.05701754385964911964, 0.06140350877192982115, 0.06578947368421052266, 0.07017543859649122417, 0.07456140350877192569, 0.07894736842105262720, 0.08333333333333332871, 0.08771929824561403022, 0.09210526315789473173, 0.09649122807017543324, 0.1008771929824561348, 0.1052631578947368363, 0.1096491228070175378, 0.1140350877192982393, 0.1184210526315789408, 0.1228070175438596423, 0.1271929824561403577, 0.1315789473684210453, 0.1359649122807017607, 0.1403508771929824483, 0.1447368421052631637, 0.1491228070175438514, 0.1535087719298245668, 0.1578947368421052544, 0.1622807017543859698, 0.1666666666666666574, 0.1710526315789473728, 0.1754385964912280604, 0.1798245614035087758, 0.1842105263157894635, 0.1885964912280701788, 0.1929824561403508665, 0.1973684210526315819, 0.2017543859649122695, 0.2061403508771929849, 0.2105263157894736725, 0.2149122807017543879, 0.2192982456140350755, 0.2236842105263157909, 0.2280701754385964786, 0.2324561403508771940, 0.2368421052631578816, 0.2412280701754385970, 0.2456140350877192846, 0.2500000000000000000, 0.2543859649122807154, 0.2587719298245614308, 0.2631578947368420907, 0.2675438596491228060, 0.2719298245614035214, 0.2763157894736842368, 0.2807017543859648967, 0.2850877192982456121, 0.2894736842105263275, 0.2938596491228070429, 0.2982456140350877027, 0.3026315789473684181, 0.3070175438596491335, 0.3114035087719298489, 0.3157894736842105088, 0.3201754385964912242, 0.3245614035087719396, 0.3289473684210526550, 0.3333333333333333148, 0.3377192982456140302, 0.3421052631578947456, 0.3464912280701754610, 0.3508771929824561209, 0.3552631578947368363, 0.3596491228070175517, 0.3640350877192982670, 0.3684210526315789269, 0.3728070175438596423, 0.3771929824561403577, 0.3815789473684210731, 0.3859649122807017330, 0.3903508771929824483, 0.3947368421052631637, 0.3991228070175438791, 0.4035087719298245390, 0.4078947368421052544, 0.4122807017543859698, 0.4166666666666666852, 0.4210526315789473450, 0.4254385964912280604, 0.4298245614035087758, 0.4342105263157894912, 0.4385964912280701511, 0.4429824561403508665, 0.4473684210526315819, 0.4517543859649122973, 0.4561403508771929571, 0.4605263157894736725, 0.4649122807017543879, 0.4692982456140351033, 0.4736842105263157632, 0.4780701754385964786, 0.4824561403508771940, 0.4868421052631579093, 0.4912280701754385692, 0.4956140350877192846, 0.5000000000000000000, 0.5043859649122807154, 0.5087719298245614308, 0.5131578947368421462, 0.5175438596491228616, 0.5219298245614034659, 0.5263157894736841813, 0.5307017543859648967, 0.5350877192982456121, 0.5394736842105263275, 0.5438596491228070429, 0.5482456140350877583, 0.5526315789473684736, 0.5570175438596490780, 0.5614035087719297934, 0.5657894736842105088, 0.5701754385964912242, 0.5745614035087719396, 0.5789473684210526550, 0.5833333333333333703, 0.5877192982456140857, 0.5921052631578946901, 0.5964912280701754055, 0.6008771929824561209, 0.6052631578947368363, 0.6096491228070175517, 0.6140350877192982670, 0.6184210526315789824, 0.6228070175438596978, 0.6271929824561403022, 0.6315789473684210176, 0.6359649122807017330, 0.6403508771929824483, 0.6447368421052631637, 0.6491228070175438791, 0.6535087719298245945, 0.6578947368421053099, 0.6622807017543859143, 0.6666666666666666297, 0.6710526315789473450, 0.6754385964912280604, 0.6798245614035087758, 0.6842105263157894912, 0.6885964912280702066, 0.6929824561403509220, 0.6973684210526315264, 0.7017543859649122417, 0.7061403508771929571, 0.7105263157894736725, 0.7149122807017543879, 0.7192982456140351033, 0.7236842105263158187, 0.7280701754385965341, 0.7324561403508771384, 0.7368421052631578538, 0.7412280701754385692, 0.7456140350877192846, 0.7500000000000000000, 0.7543859649122807154, 0.7587719298245614308, 0.7631578947368421462, 0.7675438596491228616, 0.7719298245614034659, 0.7763157894736841813, 0.7807017543859648967, 0.7850877192982456121, 0.7894736842105263275, 0.7938596491228070429, 0.7982456140350877583, 0.8026315789473684736, 0.8070175438596490780, 0.8114035087719297934, 0.8157894736842105088, 0.8201754385964912242, 0.8245614035087719396, 0.8289473684210526550, 0.8333333333333333703, 0.8377192982456140857, 0.8421052631578946901, 0.8464912280701754055, 0.8508771929824561209, 0.8552631578947368363, 0.8596491228070175517, 0.8640350877192982670, 0.8684210526315789824, 0.8728070175438596978, 0.8771929824561403022, 0.8815789473684210176, 0.8859649122807017330, 0.8903508771929824483, 0.8947368421052631637, 0.8991228070175438791, 0.9035087719298245945, 0.9078947368421053099, 0.9122807017543859143, 0.9166666666666666297, 0.9210526315789473450, 0.9254385964912280604, 0.9298245614035087758, 0.9342105263157894912, 0.9385964912280702066, 0.9429824561403509220, 0.9473684210526315264, 0.9517543859649122417, 0.9561403508771929571, 0.9605263157894736725, 0.9649122807017543879, 0.9692982456140351033, 0.9736842105263158187, 0.9780701754385965341, 0.9824561403508771384, 0.9868421052631578538, 0.9912280701754385692, 0.9956140350877192846, 1.000000000000000000 ),
 .UNSPECIFIED. ) 
 GEOMETRIC_REPRESENTATION_ITEM ( )  RATIONAL_B_SPLINE_SURFACE ( (
 ( 1.000000000000000000, 0.9659258262890683122, 1.000000000000000000, 0.9659258262890683122, 1.000000000000000000, 0.9659258262890683122, 1.000000000000000000, 0.9659258262890683122, 1.000000000000000000, 0.9659258262890683122, 1.000000000000000000, 0.9659258262890683122, 1.000000000000000000, 0.9659258262890683122, 1.000000000000000000, 0.9659258262890683122, 1.000000000000000000, 0.9659258262890683122, 1.000000000000000000, 0.9659258262890683122, 1.000000000000000000, 0.9659258262890683122, 1.000000000000000000, 0.9659258262890683122, 1.000000000000000000, 0.9659258262890683122, 1.000000000000000000, 0.9659258262890683122, 1.000000000000000000, 0.9659258262890683122, 1.000000000000000000, 0.9659258262890683122, 1.000000000000000000, 0.9659258262890683122, 1.000000000000000000, 0.9659258262890683122, 1.000000000000000000, 0.9659258262890683122, 1.000000000000000000, 0.9659258262890683122, 1.000000000000000000, 0.9659258262890683122, 1.000000000000000000, 0.9659258262890683122, 1.000000000000000000, 0.9659258262890683122, 1.000000000000000000, 0.9659258262890683122, 1.000000000000000000, 0.9659258262890683122, 1.000000000000000000, 0.9659258262890683122, 1.000000000000000000, 0.9659258262890683122, 1.000000000000000000, 0.9659258262890683122, 1.000000000000000000, 0.9659258262890683122, 1.000000000000000000, 0.9659258262890683122, 1.000000000000000000, 0.9659258262890683122, 1.000000000000000000, 0.9659258262890683122, 1.000000000000000000, 0.9659258262890683122, 1.000000000000000000, 0.9659258262890683122, 1.000000000000000000, 0.9659258262890683122, 1.000000000000000000, 0.9659258262890683122, 1.000000000000000000, 0.9659258262890683122, 1.000000000000000000, 0.9659258262890683122, 1.000000000000000000, 0.9659258262890683122, 1.000000000000000000, 0.9659258262890683122, 1.000000000000000000, 0.9659258262890683122, 1.000000000000000000, 0.9659258262890683122, 1.000000000000000000, 0.9659258262890683122, 1.000000000000000000, 0.9659258262890683122, 1.000000000000000000, 0.9659258262890683122, 1.000000000000000000, 0.9659258262890683122, 1.000000000000000000, 0.9659258262890683122, 1.000000000000000000, 0.9659258262890683122, 1.000000000000000000, 0.9659258262890683122, 1.000000000000000000, 0.9659258262890683122, 1.000000000000000000, 0.9659258262890683122, 1.000000000000000000, 0.9659258262890683122, 1.000000000000000000, 0.9659258262890683122, 1.000000000000000000, 0.9659258262890683122, 1.000000000000000000, 0.9659258262890683122, 1.000000000000000000, 0.9659258262890683122, 1.000000000000000000, 0.9659258262890683122, 1.000000000000000000, 0.9659258262890683122, 1.000000000000000000, 0.9659258262890683122, 1.000000000000000000, 0.9659258262890683122, 1.000000000000000000, 0.9659258262890683122, 1.000000000000000000, 0.9659258262890683122, 1.000000000000000000, 0.9659258262890683122, 1.000000000000000000, 0.9659258262890683122, 1.000000000000000000, 0.9659258262890683122, 1.000000000000000000, 0.9659258262890683122, 1.000000000000000000, 0.9659258262890683122, 1.000000000000000000, 0.9659258262890683122, 1.000000000000000000, 0.9659258262890683122, 1.000000000000000000, 0.9659258262890683122, 1.000000000000000000, 0.9659258262890683122, 1.000000000000000000, 0.9659258262890683122, 1.000000000000000000, 0.9659258262890683122, 1.000000000000000000, 0.9659258262890683122, 1.000000000000000000, 0.9659258262890683122, 1.000000000000000000, 0.9659258262890683122, 1.000000000000000000, 0.9659258262890683122, 1.000000000000000000, 0.9659258262890683122, 1.000000000000000000, 0.9659258262890683122, 1.000000000000000000, 0.9659258262890683122, 1.000000000000000000, 0.9659258262890683122, 1.000000000000000000, 0.9659258262890683122, 1.000000000000000000, 0.9659258262890683122, 1.000000000000000000, 0.9659258262890683122, 1.000000000000000000, 0.9659258262890683122, 1.000000000000000000, 0.9659258262890683122, 1.000000000000000000, 0.9659258262890683122, 1.000000000000000000, 0.9659258262890683122, 1.000000000000000000, 0.9659258262890683122, 1.000000000000000000, 0.9659258262890683122, 1.000000000000000000, 0.9659258262890683122, 1.000000000000000000, 0.9659258262890683122, 1.000000000000000000, 0.9659258262890683122, 1.000000000000000000, 0.9659258262890683122, 1.000000000000000000, 0.9659258262890683122, 1.000000000000000000, 0.9659258262890683122, 1.000000000000000000, 0.9659258262890683122, 1.000000000000000000, 0.9659258262890683122, 1.000000000000000000, 0.9659258262890683122, 1.000000000000000000, 0.9659258262890683122, 1.000000000000000000, 0.9659258262890683122, 1.000000000000000000, 0.9659258262890683122, 1.000000000000000000, 0.9659258262890683122, 1.000000000000000000, 0.9659258262890683122, 1.000000000000000000, 0.9659258262890683122, 1.000000000000000000, 0.9659258262890683122, 1.000000000000000000, 0.9659258262890683122, 1.000000000000000000, 0.9659258262890683122, 1.000000000000000000, 0.9659258262890683122, 1.000000000000000000, 0.9659258262890683122, 1.000000000000000000, 0.9659258262890683122, 1.000000000000000000, 0.9659258262890683122, 1.000000000000000000, 0.9659258262890683122, 1.000000000000000000, 0.9659258262890683122, 1.000000000000000000, 0.9659258262890683122, 1.000000000000000000, 0.9659258262890683122, 1.000000000000000000, 0.9659258262890683122, 1.000000000000000000, 0.9659258262890683122, 1.000000000000000000, 0.9659258262890683122, 1.000000000000000000, 0.9659258262890683122, 1.000000000000000000, 0.9659258262890683122, 1.000000000000000000, 0.9659258262890683122, 1.000000000000000000, 0.9659258262890683122, 1.000000000000000000, 0.9659258262890683122, 1.000000000000000000, 0.9659258262890683122, 1.000000000000000000, 0.9659258262890683122, 1.000000000000000000, 0.9659258262890683122, 1.000000000000000000, 0.9659258262890683122, 1.000000000000000000, 0.9659258262890683122, 1.000000000000000000, 0.9659258262890683122, 1.000000000000000000, 0.9659258262890683122, 1.000000000000000000, 0.9659258262890683122, 1.000000000000000000, 0.9659258262890683122, 1.000000000000000000, 0.9659258262890683122, 1.000000000000000000, 0.9659258262890683122, 1.000000000000000000, 0.9659258262890683122, 1.000000000000000000, 0.9659258262890683122, 1.000000000000000000, 0.9659258262890683122, 1.000000000000000000, 0.9659258262890683122, 1.000000000000000000, 0.9659258262890683122, 1.000000000000000000, 0.9659258262890683122, 1.000000000000000000, 0.9659258262890683122, 1.000000000000000000, 0.9659258262890683122, 1.000000000000000000, 0.9659258262890683122, 1.000000000000000000, 0.9659258262890683122, 1.000000000000000000, 0.9659258262890683122, 1.000000000000000000, 0.9659258262890683122, 1.000000000000000000, 0.9659258262890683122, 1.000000000000000000, 0.9659258262890683122, 1.000000000000000000, 0.9659258262890683122, 1.000000000000000000, 0.9659258262890683122, 1.000000000000000000, 0.9659258262890683122, 1.000000000000000000, 0.9659258262890683122, 1.000000000000000000, 0.9659258262890683122, 1.000000000000000000, 0.9659258262890683122, 1.000000000000000000, 0.9659258262890683122, 1.000000000000000000, 0.9659258262890683122, 1.000000000000000000, 0.9659258262890683122, 1.000000000000000000, 0.9659258262890683122, 1.000000000000000000, 0.9659258262890683122, 1.000000000000000000, 0.9659258262890683122, 1.000000000000000000, 0.9659258262890683122, 1.000000000000000000, 0.9659258262890683122, 1.000000000000000000, 0.9659258262890683122, 1.000000000000000000, 0.9659258262890683122, 1.000000000000000000, 0.9659258262890683122, 1.000000000000000000, 0.9659258262890683122, 1.000000000000000000, 0.9659258262890683122, 1.000000000000000000, 0.9659258262890683122, 1.000000000000000000, 0.9659258262890683122, 1.000000000000000000, 0.9659258262890683122, 1.000000000000000000, 0.9659258262890683122, 1.000000000000000000, 0.9659258262890683122, 1.000000000000000000, 0.9659258262890683122, 1.000000000000000000, 0.9659258262890683122, 1.000000000000000000, 0.9659258262890683122, 1.000000000000000000, 0.9659258262890683122, 1.000000000000000000, 0.9659258262890683122, 1.000000000000000000, 0.9659258262890683122, 1.000000000000000000, 0.9659258262890683122, 1.000000000000000000, 0.9659258262890683122, 1.000000000000000000, 0.9659258262890683122, 1.000000000000000000, 0.9659258262890683122, 1.000000000000000000, 0.9659258262890683122, 1.000000000000000000, 0.9659258262890683122, 1.000000000000000000, 0.9659258262890683122, 1.000000000000000000, 0.9659258262890683122, 1.000000000000000000, 0.9659258262890683122, 1.000000000000000000, 0.9659258262890683122, 1.000000000000000000, 0.9659258262890683122, 1.000000000000000000, 0.9659258262890683122, 1.000000000000000000, 0.9659258262890683122, 1.000000000000000000, 0.9659258262890683122, 1.000000000000000000, 0.9659258262890683122, 1.000000000000000000, 0.9659258262890683122, 1.000000000000000000, 0.9659258262890683122, 1.000000000000000000, 0.9659258262890683122, 1.000000000000000000, 0.9659258262890683122, 1.000000000000000000, 0.9659258262890683122, 1.000000000000000000, 0.9659258262890683122, 1.000000000000000000, 0.9659258262890683122, 1.000000000000000000, 0.9659258262890683122, 1.000000000000000000, 0.9659258262890683122, 1.000000000000000000, 0.9659258262890683122, 1.000000000000000000, 0.9659258262890683122, 1.000000000000000000, 0.9659258262890683122, 1.000000000000000000, 0.9659258262890683122, 1.000000000000000000, 0.9659258262890683122, 1.000000000000000000, 0.9659258262890683122, 1.000000000000000000, 0.9659258262890683122, 1.000000000000000000, 0.9659258262890683122, 1.000000000000000000, 0.9659258262890683122, 1.000000000000000000, 0.9659258262890683122, 1.000000000000000000, 0.9659258262890683122, 1.000000000000000000, 0.9659258262890683122, 1.000000000000000000, 0.9659258262890683122, 1.000000000000000000, 0.9659258262890683122, 1.000000000000000000, 0.9659258262890683122, 1.000000000000000000, 0.9659258262890683122, 1.000000000000000000, 0.9659258262890683122, 1.000000000000000000, 0.9659258262890683122, 1.000000000000000000, 0.9659258262890683122, 1.000000000000000000, 0.9659258262890683122, 1.000000000000000000, 0.9659258262890683122, 1.000000000000000000, 0.9659258262890683122, 1.000000000000000000, 0.9659258262890683122, 1.000000000000000000, 0.9659258262890683122, 1.000000000000000000, 0.9659258262890683122, 1.000000000000000000),
 ( 0.3333333333333333703, 0.3219752754296894559, 0.3333333333333333703, 0.3219752754296894559, 0.3333333333333333703, 0.3219752754296894559, 0.3333333333333333703, 0.3219752754296894559, 0.3333333333333333703, 0.3219752754296894559, 0.3333333333333333703, 0.3219752754296894559, 0.3333333333333333703, 0.3219752754296894559, 0.3333333333333333703, 0.3219752754296894559, 0.3333333333333333703, 0.3219752754296894559, 0.3333333333333333703, 0.3219752754296894559, 0.3333333333333333703, 0.3219752754296894559, 0.3333333333333333703, 0.3219752754296894559, 0.3333333333333333703, 0.3219752754296894559, 0.3333333333333333703, 0.3219752754296894559, 0.3333333333333333703, 0.3219752754296894559, 0.3333333333333333703, 0.3219752754296894559, 0.3333333333333333703, 0.3219752754296894559, 0.3333333333333333703, 0.3219752754296894559, 0.3333333333333333703, 0.3219752754296894559, 0.3333333333333333703, 0.3219752754296894559, 0.3333333333333333703, 0.3219752754296894559, 0.3333333333333333703, 0.3219752754296894559, 0.3333333333333333703, 0.3219752754296894559, 0.3333333333333333703, 0.3219752754296894559, 0.3333333333333333703, 0.3219752754296894559, 0.3333333333333333703, 0.3219752754296894559, 0.3333333333333333703, 0.3219752754296894559, 0.3333333333333333703, 0.3219752754296894559, 0.3333333333333333703, 0.3219752754296894559, 0.3333333333333333703, 0.3219752754296894559, 0.3333333333333333703, 0.3219752754296894559, 0.3333333333333333703, 0.3219752754296894559, 0.3333333333333333703, 0.3219752754296894559, 0.3333333333333333703, 0.3219752754296894559, 0.3333333333333333703, 0.3219752754296894559, 0.3333333333333333703, 0.3219752754296894559, 0.3333333333333333703, 0.3219752754296894559, 0.3333333333333333703, 0.3219752754296894559, 0.3333333333333333703, 0.3219752754296894559, 0.3333333333333333703, 0.3219752754296894559, 0.3333333333333333703, 0.3219752754296894559, 0.3333333333333333703, 0.3219752754296894559, 0.3333333333333333703, 0.3219752754296894559, 0.3333333333333333703, 0.3219752754296894559, 0.3333333333333333703, 0.3219752754296894559, 0.3333333333333333703, 0.3219752754296894559, 0.3333333333333333703, 0.3219752754296894559, 0.3333333333333333703, 0.3219752754296894559, 0.3333333333333333703, 0.3219752754296894559, 0.3333333333333333703, 0.3219752754296894559, 0.3333333333333333703, 0.3219752754296894559, 0.3333333333333333703, 0.3219752754296894559, 0.3333333333333333703, 0.3219752754296894559, 0.3333333333333333703, 0.3219752754296894559, 0.3333333333333333703, 0.3219752754296894559, 0.3333333333333333703, 0.3219752754296894559, 0.3333333333333333703, 0.3219752754296894559, 0.3333333333333333703, 0.3219752754296894559, 0.3333333333333333703, 0.3219752754296894559, 0.3333333333333333703, 0.3219752754296894559, 0.3333333333333333703, 0.3219752754296894559, 0.3333333333333333703, 0.3219752754296894559, 0.3333333333333333703, 0.3219752754296894559, 0.3333333333333333703, 0.3219752754296894559, 0.3333333333333333703, 0.3219752754296894559, 0.3333333333333333703, 0.3219752754296894559, 0.3333333333333333703, 0.3219752754296894559, 0.3333333333333333703, 0.3219752754296894559, 0.3333333333333333703, 0.3219752754296894559, 0.3333333333333333703, 0.3219752754296894559, 0.3333333333333333703, 0.3219752754296894559, 0.3333333333333333703, 0.3219752754296894559, 0.3333333333333333703, 0.3219752754296894559, 0.3333333333333333703, 0.3219752754296894559, 0.3333333333333333703, 0.3219752754296894559, 0.3333333333333333703, 0.3219752754296894559, 0.3333333333333333703, 0.3219752754296894559, 0.3333333333333333703, 0.3219752754296894559, 0.3333333333333333703, 0.3219752754296894559, 0.3333333333333333703, 0.3219752754296894559, 0.3333333333333333703, 0.3219752754296894559, 0.3333333333333333703, 0.3219752754296894559, 0.3333333333333333703, 0.3219752754296894559, 0.3333333333333333703, 0.3219752754296894559, 0.3333333333333333703, 0.3219752754296894559, 0.3333333333333333703, 0.3219752754296894559, 0.3333333333333333703, 0.3219752754296894559, 0.3333333333333333703, 0.3219752754296894559, 0.3333333333333333703, 0.3219752754296894559, 0.3333333333333333703, 0.3219752754296894559, 0.3333333333333333703, 0.3219752754296894559, 0.3333333333333333703, 0.3219752754296894559, 0.3333333333333333703, 0.3219752754296894559, 0.3333333333333333703, 0.3219752754296894559, 0.3333333333333333703, 0.3219752754296894559, 0.3333333333333333703, 0.3219752754296894559, 0.3333333333333333703, 0.3219752754296894559, 0.3333333333333333703, 0.3219752754296894559, 0.3333333333333333703, 0.3219752754296894559, 0.3333333333333333703, 0.3219752754296894559, 0.3333333333333333703, 0.3219752754296894559, 0.3333333333333333703, 0.3219752754296894559, 0.3333333333333333703, 0.3219752754296894559, 0.3333333333333333703, 0.3219752754296894559, 0.3333333333333333703, 0.3219752754296894559, 0.3333333333333333703, 0.3219752754296894559, 0.3333333333333333703, 0.3219752754296894559, 0.3333333333333333703, 0.3219752754296894559, 0.3333333333333333703, 0.3219752754296894559, 0.3333333333333333703, 0.3219752754296894559, 0.3333333333333333703, 0.3219752754296894559, 0.3333333333333333703, 0.3219752754296894559, 0.3333333333333333703, 0.3219752754296894559, 0.3333333333333333703, 0.3219752754296894559, 0.3333333333333333703, 0.3219752754296894559, 0.3333333333333333703, 0.3219752754296894559, 0.3333333333333333703, 0.3219752754296894559, 0.3333333333333333703, 0.3219752754296894559, 0.3333333333333333703, 0.3219752754296894559, 0.3333333333333333703, 0.3219752754296894559, 0.3333333333333333703, 0.3219752754296894559, 0.3333333333333333703, 0.3219752754296894559, 0.3333333333333333703, 0.3219752754296894559, 0.3333333333333333703, 0.3219752754296894559, 0.3333333333333333703, 0.3219752754296894559, 0.3333333333333333703, 0.3219752754296894559, 0.3333333333333333703, 0.3219752754296894559, 0.3333333333333333703, 0.3219752754296894559, 0.3333333333333333703, 0.3219752754296894559, 0.3333333333333333703, 0.3219752754296894559, 0.3333333333333333703, 0.3219752754296894559, 0.3333333333333333703, 0.3219752754296894559, 0.3333333333333333703, 0.3219752754296894559, 0.3333333333333333703, 0.3219752754296894559, 0.3333333333333333703, 0.3219752754296894559, 0.3333333333333333703, 0.3219752754296894559, 0.3333333333333333703, 0.3219752754296894559, 0.3333333333333333703, 0.3219752754296894559, 0.3333333333333333703, 0.3219752754296894559, 0.3333333333333333703, 0.3219752754296894559, 0.3333333333333333703, 0.3219752754296894559, 0.3333333333333333703, 0.3219752754296894559, 0.3333333333333333703, 0.3219752754296894559, 0.3333333333333333703, 0.3219752754296894559, 0.3333333333333333703, 0.3219752754296894559, 0.3333333333333333703, 0.3219752754296894559, 0.3333333333333333703, 0.3219752754296894559, 0.3333333333333333703, 0.3219752754296894559, 0.3333333333333333703, 0.3219752754296894559, 0.3333333333333333703, 0.3219752754296894559, 0.3333333333333333703, 0.3219752754296894559, 0.3333333333333333703, 0.3219752754296894559, 0.3333333333333333703, 0.3219752754296894559, 0.3333333333333333703, 0.3219752754296894559, 0.3333333333333333703, 0.3219752754296894559, 0.3333333333333333703, 0.3219752754296894559, 0.3333333333333333703, 0.3219752754296894559, 0.3333333333333333703, 0.3219752754296894559, 0.3333333333333333703, 0.3219752754296894559, 0.3333333333333333703, 0.3219752754296894559, 0.3333333333333333703, 0.3219752754296894559, 0.3333333333333333703, 0.3219752754296894559, 0.3333333333333333703, 0.3219752754296894559, 0.3333333333333333703, 0.3219752754296894559, 0.3333333333333333703, 0.3219752754296894559, 0.3333333333333333703, 0.3219752754296894559, 0.3333333333333333703, 0.3219752754296894559, 0.3333333333333333703, 0.3219752754296894559, 0.3333333333333333703, 0.3219752754296894559, 0.3333333333333333703, 0.3219752754296894559, 0.3333333333333333703, 0.3219752754296894559, 0.3333333333333333703, 0.3219752754296894559, 0.3333333333333333703, 0.3219752754296894559, 0.3333333333333333703, 0.3219752754296894559, 0.3333333333333333703, 0.3219752754296894559, 0.3333333333333333703, 0.3219752754296894559, 0.3333333333333333703, 0.3219752754296894559, 0.3333333333333333703, 0.3219752754296894559, 0.3333333333333333703, 0.3219752754296894559, 0.3333333333333333703, 0.3219752754296894559, 0.3333333333333333703, 0.3219752754296894559, 0.3333333333333333703, 0.3219752754296894559, 0.3333333333333333703, 0.3219752754296894559, 0.3333333333333333703, 0.3219752754296894559, 0.3333333333333333703, 0.3219752754296894559, 0.3333333333333333703, 0.3219752754296894559, 0.3333333333333333703, 0.3219752754296894559, 0.3333333333333333703, 0.3219752754296894559, 0.3333333333333333703, 0.3219752754296894559, 0.3333333333333333703, 0.3219752754296894559, 0.3333333333333333703, 0.3219752754296894559, 0.3333333333333333703, 0.3219752754296894559, 0.3333333333333333703, 0.3219752754296894559, 0.3333333333333333703, 0.3219752754296894559, 0.3333333333333333703, 0.3219752754296894559, 0.3333333333333333703, 0.3219752754296894559, 0.3333333333333333703, 0.3219752754296894559, 0.3333333333333333703, 0.3219752754296894559, 0.3333333333333333703, 0.3219752754296894559, 0.3333333333333333703, 0.3219752754296894559, 0.3333333333333333703, 0.3219752754296894559, 0.3333333333333333703, 0.3219752754296894559, 0.3333333333333333703, 0.3219752754296894559, 0.3333333333333333703, 0.3219752754296894559, 0.3333333333333333703, 0.3219752754296894559, 0.3333333333333333703, 0.3219752754296894559, 0.3333333333333333703, 0.3219752754296894559, 0.3333333333333333703, 0.3219752754296894559, 0.3333333333333333703, 0.3219752754296894559, 0.3333333333333333703, 0.3219752754296894559, 0.3333333333333333703, 0.3219752754296894559, 0.3333333333333333703, 0.3219752754296894559, 0.3333333333333333703, 0.3219752754296894559, 0.3333333333333333703, 0.3219752754296894559, 0.3333333333333333703, 0.3219752754296894559, 0.3333333333333333703, 0.3219752754296894559, 0.3333333333333333703, 0.3219752754296894559, 0.3333333333333333703, 0.3219752754296894559, 0.3333333333333333703, 0.3219752754296894559, 0.3333333333333333703, 0.3219752754296894559, 0.3333333333333333703, 0.3219752754296894559, 0.3333333333333333703, 0.3219752754296894559, 0.3333333333333333703, 0.3219752754296894559, 0.3333333333333333703, 0.3219752754296894559, 0.3333333333333333703, 0.3219752754296894559, 0.3333333333333333703, 0.3219752754296894559, 0.3333333333333333703, 0.3219752754296894559, 0.3333333333333333703, 0.3219752754296894559, 0.3333333333333333703),
 ( 0.3333333333333333703, 0.3219752754296894559, 0.3333333333333333703, 0.3219752754296894559, 0.3333333333333333703, 0.3219752754296894559, 0.3333333333333333703, 0.3219752754296894559, 0.3333333333333333703, 0.3219752754296894559, 0.3333333333333333703, 0.3219752754296894559, 0.3333333333333333703, 0.3219752754296894559, 0.3333333333333333703, 0.3219752754296894559, 0.3333333333333333703, 0.3219752754296894559, 0.3333333333333333703, 0.3219752754296894559, 0.3333333333333333703, 0.3219752754296894559, 0.3333333333333333703, 0.3219752754296894559, 0.3333333333333333703, 0.3219752754296894559, 0.3333333333333333703, 0.3219752754296894559, 0.3333333333333333703, 0.3219752754296894559, 0.3333333333333333703, 0.3219752754296894559, 0.3333333333333333703, 0.3219752754296894559, 0.3333333333333333703, 0.3219752754296894559, 0.3333333333333333703, 0.3219752754296894559, 0.3333333333333333703, 0.3219752754296894559, 0.3333333333333333703, 0.3219752754296894559, 0.3333333333333333703, 0.3219752754296894559, 0.3333333333333333703, 0.3219752754296894559, 0.3333333333333333703, 0.3219752754296894559, 0.3333333333333333703, 0.3219752754296894559, 0.3333333333333333703, 0.3219752754296894559, 0.3333333333333333703, 0.3219752754296894559, 0.3333333333333333703, 0.3219752754296894559, 0.3333333333333333703, 0.3219752754296894559, 0.3333333333333333703, 0.3219752754296894559, 0.3333333333333333703, 0.3219752754296894559, 0.3333333333333333703, 0.3219752754296894559, 0.3333333333333333703, 0.3219752754296894559, 0.3333333333333333703, 0.3219752754296894559, 0.3333333333333333703, 0.3219752754296894559, 0.3333333333333333703, 0.3219752754296894559, 0.3333333333333333703, 0.3219752754296894559, 0.3333333333333333703, 0.3219752754296894559, 0.3333333333333333703, 0.3219752754296894559, 0.3333333333333333703, 0.3219752754296894559, 0.3333333333333333703, 0.3219752754296894559, 0.3333333333333333703, 0.3219752754296894559, 0.3333333333333333703, 0.3219752754296894559, 0.3333333333333333703, 0.3219752754296894559, 0.3333333333333333703, 0.3219752754296894559, 0.3333333333333333703, 0.3219752754296894559, 0.3333333333333333703, 0.3219752754296894559, 0.3333333333333333703, 0.3219752754296894559, 0.3333333333333333703, 0.3219752754296894559, 0.3333333333333333703, 0.3219752754296894559, 0.3333333333333333703, 0.3219752754296894559, 0.3333333333333333703, 0.3219752754296894559, 0.3333333333333333703, 0.3219752754296894559, 0.3333333333333333703, 0.3219752754296894559, 0.3333333333333333703, 0.3219752754296894559, 0.3333333333333333703, 0.3219752754296894559, 0.3333333333333333703, 0.3219752754296894559, 0.3333333333333333703, 0.3219752754296894559, 0.3333333333333333703, 0.3219752754296894559, 0.3333333333333333703, 0.3219752754296894559, 0.3333333333333333703, 0.3219752754296894559, 0.3333333333333333703, 0.3219752754296894559, 0.3333333333333333703, 0.3219752754296894559, 0.3333333333333333703, 0.3219752754296894559, 0.3333333333333333703, 0.3219752754296894559, 0.3333333333333333703, 0.3219752754296894559, 0.3333333333333333703, 0.3219752754296894559, 0.3333333333333333703, 0.3219752754296894559, 0.3333333333333333703, 0.3219752754296894559, 0.3333333333333333703, 0.3219752754296894559, 0.3333333333333333703, 0.3219752754296894559, 0.3333333333333333703, 0.3219752754296894559, 0.3333333333333333703, 0.3219752754296894559, 0.3333333333333333703, 0.3219752754296894559, 0.3333333333333333703, 0.3219752754296894559, 0.3333333333333333703, 0.3219752754296894559, 0.3333333333333333703, 0.3219752754296894559, 0.3333333333333333703, 0.3219752754296894559, 0.3333333333333333703, 0.3219752754296894559, 0.3333333333333333703, 0.3219752754296894559, 0.3333333333333333703, 0.3219752754296894559, 0.3333333333333333703, 0.3219752754296894559, 0.3333333333333333703, 0.3219752754296894559, 0.3333333333333333703, 0.3219752754296894559, 0.3333333333333333703, 0.3219752754296894559, 0.3333333333333333703, 0.3219752754296894559, 0.3333333333333333703, 0.3219752754296894559, 0.3333333333333333703, 0.3219752754296894559, 0.3333333333333333703, 0.3219752754296894559, 0.3333333333333333703, 0.3219752754296894559, 0.3333333333333333703, 0.3219752754296894559, 0.3333333333333333703, 0.3219752754296894559, 0.3333333333333333703, 0.3219752754296894559, 0.3333333333333333703, 0.3219752754296894559, 0.3333333333333333703, 0.3219752754296894559, 0.3333333333333333703, 0.3219752754296894559, 0.3333333333333333703, 0.3219752754296894559, 0.3333333333333333703, 0.3219752754296894559, 0.3333333333333333703, 0.3219752754296894559, 0.3333333333333333703, 0.3219752754296894559, 0.3333333333333333703, 0.3219752754296894559, 0.3333333333333333703, 0.3219752754296894559, 0.3333333333333333703, 0.3219752754296894559, 0.3333333333333333703, 0.3219752754296894559, 0.3333333333333333703, 0.3219752754296894559, 0.3333333333333333703, 0.3219752754296894559, 0.3333333333333333703, 0.3219752754296894559, 0.3333333333333333703, 0.3219752754296894559, 0.3333333333333333703, 0.3219752754296894559, 0.3333333333333333703, 0.3219752754296894559, 0.3333333333333333703, 0.3219752754296894559, 0.3333333333333333703, 0.3219752754296894559, 0.3333333333333333703, 0.3219752754296894559, 0.3333333333333333703, 0.3219752754296894559, 0.3333333333333333703, 0.3219752754296894559, 0.3333333333333333703, 0.3219752754296894559, 0.3333333333333333703, 0.3219752754296894559, 0.3333333333333333703, 0.3219752754296894559, 0.3333333333333333703, 0.3219752754296894559, 0.3333333333333333703, 0.3219752754296894559, 0.3333333333333333703, 0.3219752754296894559, 0.3333333333333333703, 0.3219752754296894559, 0.3333333333333333703, 0.3219752754296894559, 0.3333333333333333703, 0.3219752754296894559, 0.3333333333333333703, 0.3219752754296894559, 0.3333333333333333703, 0.3219752754296894559, 0.3333333333333333703, 0.3219752754296894559, 0.3333333333333333703, 0.3219752754296894559, 0.3333333333333333703, 0.3219752754296894559, 0.3333333333333333703, 0.3219752754296894559, 0.3333333333333333703, 0.3219752754296894559, 0.3333333333333333703, 0.3219752754296894559, 0.3333333333333333703, 0.3219752754296894559, 0.3333333333333333703, 0.3219752754296894559, 0.3333333333333333703, 0.3219752754296894559, 0.3333333333333333703, 0.3219752754296894559, 0.3333333333333333703, 0.3219752754296894559, 0.3333333333333333703, 0.3219752754296894559, 0.3333333333333333703, 0.3219752754296894559, 0.3333333333333333703, 0.3219752754296894559, 0.3333333333333333703, 0.3219752754296894559, 0.3333333333333333703, 0.3219752754296894559, 0.3333333333333333703, 0.3219752754296894559, 0.3333333333333333703, 0.3219752754296894559, 0.3333333333333333703, 0.3219752754296894559, 0.3333333333333333703, 0.3219752754296894559, 0.3333333333333333703, 0.3219752754296894559, 0.3333333333333333703, 0.3219752754296894559, 0.3333333333333333703, 0.3219752754296894559, 0.3333333333333333703, 0.3219752754296894559, 0.3333333333333333703, 0.3219752754296894559, 0.3333333333333333703, 0.3219752754296894559, 0.3333333333333333703, 0.3219752754296894559, 0.3333333333333333703, 0.3219752754296894559, 0.3333333333333333703, 0.3219752754296894559, 0.3333333333333333703, 0.3219752754296894559, 0.3333333333333333703, 0.3219752754296894559, 0.3333333333333333703, 0.3219752754296894559, 0.3333333333333333703, 0.3219752754296894559, 0.3333333333333333703, 0.3219752754296894559, 0.3333333333333333703, 0.3219752754296894559, 0.3333333333333333703, 0.3219752754296894559, 0.3333333333333333703, 0.3219752754296894559, 0.3333333333333333703, 0.3219752754296894559, 0.3333333333333333703, 0.3219752754296894559, 0.3333333333333333703, 0.3219752754296894559, 0.3333333333333333703, 0.3219752754296894559, 0.3333333333333333703, 0.3219752754296894559, 0.3333333333333333703, 0.3219752754296894559, 0.3333333333333333703, 0.3219752754296894559, 0.3333333333333333703, 0.3219752754296894559, 0.3333333333333333703, 0.3219752754296894559, 0.3333333333333333703, 0.3219752754296894559, 0.3333333333333333703, 0.3219752754296894559, 0.3333333333333333703, 0.3219752754296894559, 0.3333333333333333703, 0.3219752754296894559, 0.3333333333333333703, 0.3219752754296894559, 0.3333333333333333703, 0.3219752754296894559, 0.3333333333333333703, 0.3219752754296894559, 0.3333333333333333703, 0.3219752754296894559, 0.3333333333333333703, 0.3219752754296894559, 0.3333333333333333703, 0.3219752754296894559, 0.3333333333333333703, 0.3219752754296894559, 0.3333333333333333703, 0.3219752754296894559, 0.3333333333333333703, 0.3219752754296894559, 0.3333333333333333703, 0.3219752754296894559, 0.3333333333333333703, 0.3219752754296894559, 0.3333333333333333703, 0.3219752754296894559, 0.3333333333333333703, 0.3219752754296894559, 0.3333333333333333703, 0.3219752754296894559, 0.3333333333333333703, 0.3219752754296894559, 0.3333333333333333703, 0.3219752754296894559, 0.3333333333333333703, 0.3219752754296894559, 0.3333333333333333703, 0.3219752754296894559, 0.3333333333333333703, 0.3219752754296894559, 0.3333333333333333703, 0.3219752754296894559, 0.3333333333333333703, 0.3219752754296894559, 0.3333333333333333703, 0.3219752754296894559, 0.3333333333333333703, 0.3219752754296894559, 0.3333333333333333703, 0.3219752754296894559, 0.3333333333333333703, 0.3219752754296894559, 0.3333333333333333703, 0.3219752754296894559, 0.3333333333333333703, 0.3219752754296894559, 0.3333333333333333703, 0.3219752754296894559, 0.3333333333333333703, 0.3219752754296894559, 0.3333333333333333703, 0.3219752754296894559, 0.3333333333333333703, 0.3219752754296894559, 0.3333333333333333703, 0.3219752754296894559, 0.3333333333333333703, 0.3219752754296894559, 0.3333333333333333703, 0.3219752754296894559, 0.3333333333333333703, 0.3219752754296894559, 0.3333333333333333703, 0.3219752754296894559, 0.3333333333333333703, 0.3219752754296894559, 0.3333333333333333703, 0.3219752754296894559, 0.3333333333333333703, 0.3219752754296894559, 0.3333333333333333703, 0.3219752754296894559, 0.3333333333333333703, 0.3219752754296894559, 0.3333333333333333703, 0.3219752754296894559, 0.3333333333333333703, 0.3219752754296894559, 0.3333333333333333703, 0.3219752754296894559, 0.3333333333333333703, 0.3219752754296894559, 0.3333333333333333703, 0.3219752754296894559, 0.3333333333333333703, 0.3219752754296894559, 0.3333333333333333703, 0.3219752754296894559, 0.3333333333333333703, 0.3219752754296894559, 0.3333333333333333703, 0.3219752754296894559, 0.3333333333333333703, 0.3219752754296894559, 0.3333333333333333703, 0.3219752754296894559, 0.3333333333333333703),
 ( 1.000000000000000000, 0.9659258262890683122, 1.000000000000000000, 0.9659258262890683122, 1.000000000000000000, 0.9659258262890683122, 1.000000000000000000, 0.9659258262890683122, 1.000000000000000000, 0.9659258262890683122, 1.000000000000000000, 0.9659258262890683122, 1.000000000000000000, 0.9659258262890683122, 1.000000000000000000, 0.9659258262890683122, 1.000000000000000000, 0.9659258262890683122, 1.000000000000000000, 0.9659258262890683122, 1.000000000000000000, 0.9659258262890683122, 1.000000000000000000, 0.9659258262890683122, 1.000000000000000000, 0.9659258262890683122, 1.000000000000000000, 0.9659258262890683122, 1.000000000000000000, 0.9659258262890683122, 1.000000000000000000, 0.9659258262890683122, 1.000000000000000000, 0.9659258262890683122, 1.000000000000000000, 0.9659258262890683122, 1.000000000000000000, 0.9659258262890683122, 1.000000000000000000, 0.9659258262890683122, 1.000000000000000000, 0.9659258262890683122, 1.000000000000000000, 0.9659258262890683122, 1.000000000000000000, 0.9659258262890683122, 1.000000000000000000, 0.9659258262890683122, 1.000000000000000000, 0.9659258262890683122, 1.000000000000000000, 0.9659258262890683122, 1.000000000000000000, 0.9659258262890683122, 1.000000000000000000, 0.9659258262890683122, 1.000000000000000000, 0.9659258262890683122, 1.000000000000000000, 0.9659258262890683122, 1.000000000000000000, 0.9659258262890683122, 1.000000000000000000, 0.9659258262890683122, 1.000000000000000000, 0.9659258262890683122, 1.000000000000000000, 0.9659258262890683122, 1.000000000000000000, 0.9659258262890683122, 1.000000000000000000, 0.9659258262890683122, 1.000000000000000000, 0.9659258262890683122, 1.000000000000000000, 0.9659258262890683122, 1.000000000000000000, 0.9659258262890683122, 1.000000000000000000, 0.9659258262890683122, 1.000000000000000000, 0.9659258262890683122, 1.000000000000000000, 0.9659258262890683122, 1.000000000000000000, 0.9659258262890683122, 1.000000000000000000, 0.9659258262890683122, 1.000000000000000000, 0.9659258262890683122, 1.000000000000000000, 0.9659258262890683122, 1.000000000000000000, 0.9659258262890683122, 1.000000000000000000, 0.9659258262890683122, 1.000000000000000000, 0.9659258262890683122, 1.000000000000000000, 0.9659258262890683122, 1.000000000000000000, 0.9659258262890683122, 1.000000000000000000, 0.9659258262890683122, 1.000000000000000000, 0.9659258262890683122, 1.000000000000000000, 0.9659258262890683122, 1.000000000000000000, 0.9659258262890683122, 1.000000000000000000, 0.9659258262890683122, 1.000000000000000000, 0.9659258262890683122, 1.000000000000000000, 0.9659258262890683122, 1.000000000000000000, 0.9659258262890683122, 1.000000000000000000, 0.9659258262890683122, 1.000000000000000000, 0.9659258262890683122, 1.000000000000000000, 0.9659258262890683122, 1.000000000000000000, 0.9659258262890683122, 1.000000000000000000, 0.9659258262890683122, 1.000000000000000000, 0.9659258262890683122, 1.000000000000000000, 0.9659258262890683122, 1.000000000000000000, 0.9659258262890683122, 1.000000000000000000, 0.9659258262890683122, 1.000000000000000000, 0.9659258262890683122, 1.000000000000000000, 0.9659258262890683122, 1.000000000000000000, 0.9659258262890683122, 1.000000000000000000, 0.9659258262890683122, 1.000000000000000000, 0.9659258262890683122, 1.000000000000000000, 0.9659258262890683122, 1.000000000000000000, 0.9659258262890683122, 1.000000000000000000, 0.9659258262890683122, 1.000000000000000000, 0.9659258262890683122, 1.000000000000000000, 0.9659258262890683122, 1.000000000000000000, 0.9659258262890683122, 1.000000000000000000, 0.9659258262890683122, 1.000000000000000000, 0.9659258262890683122, 1.000000000000000000, 0.9659258262890683122, 1.000000000000000000, 0.9659258262890683122, 1.000000000000000000, 0.9659258262890683122, 1.000000000000000000, 0.9659258262890683122, 1.000000000000000000, 0.9659258262890683122, 1.000000000000000000, 0.9659258262890683122, 1.000000000000000000, 0.9659258262890683122, 1.000000000000000000, 0.9659258262890683122, 1.000000000000000000, 0.9659258262890683122, 1.000000000000000000, 0.9659258262890683122, 1.000000000000000000, 0.9659258262890683122, 1.000000000000000000, 0.9659258262890683122, 1.000000000000000000, 0.9659258262890683122, 1.000000000000000000, 0.9659258262890683122, 1.000000000000000000, 0.9659258262890683122, 1.000000000000000000, 0.9659258262890683122, 1.000000000000000000, 0.9659258262890683122, 1.000000000000000000, 0.9659258262890683122, 1.000000000000000000, 0.9659258262890683122, 1.000000000000000000, 0.9659258262890683122, 1.000000000000000000, 0.9659258262890683122, 1.000000000000000000, 0.9659258262890683122, 1.000000000000000000, 0.9659258262890683122, 1.000000000000000000, 0.9659258262890683122, 1.000000000000000000, 0.9659258262890683122, 1.000000000000000000, 0.9659258262890683122, 1.000000000000000000, 0.9659258262890683122, 1.000000000000000000, 0.9659258262890683122, 1.000000000000000000, 0.9659258262890683122, 1.000000000000000000, 0.9659258262890683122, 1.000000000000000000, 0.9659258262890683122, 1.000000000000000000, 0.9659258262890683122, 1.000000000000000000, 0.9659258262890683122, 1.000000000000000000, 0.9659258262890683122, 1.000000000000000000, 0.9659258262890683122, 1.000000000000000000, 0.9659258262890683122, 1.000000000000000000, 0.9659258262890683122, 1.000000000000000000, 0.9659258262890683122, 1.000000000000000000, 0.9659258262890683122, 1.000000000000000000, 0.9659258262890683122, 1.000000000000000000, 0.9659258262890683122, 1.000000000000000000, 0.9659258262890683122, 1.000000000000000000, 0.9659258262890683122, 1.000000000000000000, 0.9659258262890683122, 1.000000000000000000, 0.9659258262890683122, 1.000000000000000000, 0.9659258262890683122, 1.000000000000000000, 0.9659258262890683122, 1.000000000000000000, 0.9659258262890683122, 1.000000000000000000, 0.9659258262890683122, 1.000000000000000000, 0.9659258262890683122, 1.000000000000000000, 0.9659258262890683122, 1.000000000000000000, 0.9659258262890683122, 1.000000000000000000, 0.9659258262890683122, 1.000000000000000000, 0.9659258262890683122, 1.000000000000000000, 0.9659258262890683122, 1.000000000000000000, 0.9659258262890683122, 1.000000000000000000, 0.9659258262890683122, 1.000000000000000000, 0.9659258262890683122, 1.000000000000000000, 0.9659258262890683122, 1.000000000000000000, 0.9659258262890683122, 1.000000000000000000, 0.9659258262890683122, 1.000000000000000000, 0.9659258262890683122, 1.000000000000000000, 0.9659258262890683122, 1.000000000000000000, 0.9659258262890683122, 1.000000000000000000, 0.9659258262890683122, 1.000000000000000000, 0.9659258262890683122, 1.000000000000000000, 0.9659258262890683122, 1.000000000000000000, 0.9659258262890683122, 1.000000000000000000, 0.9659258262890683122, 1.000000000000000000, 0.9659258262890683122, 1.000000000000000000, 0.9659258262890683122, 1.000000000000000000, 0.9659258262890683122, 1.000000000000000000, 0.9659258262890683122, 1.000000000000000000, 0.9659258262890683122, 1.000000000000000000, 0.9659258262890683122, 1.000000000000000000, 0.9659258262890683122, 1.000000000000000000, 0.9659258262890683122, 1.000000000000000000, 0.9659258262890683122, 1.000000000000000000, 0.9659258262890683122, 1.000000000000000000, 0.9659258262890683122, 1.000000000000000000, 0.9659258262890683122, 1.000000000000000000, 0.9659258262890683122, 1.000000000000000000, 0.9659258262890683122, 1.000000000000000000, 0.9659258262890683122, 1.000000000000000000, 0.9659258262890683122, 1.000000000000000000, 0.9659258262890683122, 1.000000000000000000, 0.9659258262890683122, 1.000000000000000000, 0.9659258262890683122, 1.000000000000000000, 0.9659258262890683122, 1.000000000000000000, 0.9659258262890683122, 1.000000000000000000, 0.9659258262890683122, 1.000000000000000000, 0.9659258262890683122, 1.000000000000000000, 0.9659258262890683122, 1.000000000000000000, 0.9659258262890683122, 1.000000000000000000, 0.9659258262890683122, 1.000000000000000000, 0.9659258262890683122, 1.000000000000000000, 0.9659258262890683122, 1.000000000000000000, 0.9659258262890683122, 1.000000000000000000, 0.9659258262890683122, 1.000000000000000000, 0.9659258262890683122, 1.000000000000000000, 0.9659258262890683122, 1.000000000000000000, 0.9659258262890683122, 1.000000000000000000, 0.9659258262890683122, 1.000000000000000000, 0.9659258262890683122, 1.000000000000000000, 0.9659258262890683122, 1.000000000000000000, 0.9659258262890683122, 1.000000000000000000, 0.9659258262890683122, 1.000000000000000000, 0.9659258262890683122, 1.000000000000000000, 0.9659258262890683122, 1.000000000000000000, 0.9659258262890683122, 1.000000000000000000, 0.9659258262890683122, 1.000000000000000000, 0.9659258262890683122, 1.000000000000000000, 0.9659258262890683122, 1.000000000000000000, 0.9659258262890683122, 1.000000000000000000, 0.9659258262890683122, 1.000000000000000000, 0.9659258262890683122, 1.000000000000000000, 0.9659258262890683122, 1.000000000000000000, 0.9659258262890683122, 1.000000000000000000, 0.9659258262890683122, 1.000000000000000000, 0.9659258262890683122, 1.000000000000000000, 0.9659258262890683122, 1.000000000000000000, 0.9659258262890683122, 1.000000000000000000, 0.9659258262890683122, 1.000000000000000000, 0.9659258262890683122, 1.000000000000000000, 0.9659258262890683122, 1.000000000000000000, 0.9659258262890683122, 1.000000000000000000, 0.9659258262890683122, 1.000000000000000000, 0.9659258262890683122, 1.000000000000000000, 0.9659258262890683122, 1.000000000000000000, 0.9659258262890683122, 1.000000000000000000, 0.9659258262890683122, 1.000000000000000000, 0.9659258262890683122, 1.000000000000000000, 0.9659258262890683122, 1.000000000000000000, 0.9659258262890683122, 1.000000000000000000, 0.9659258262890683122, 1.000000000000000000, 0.9659258262890683122, 1.000000000000000000, 0.9659258262890683122, 1.000000000000000000, 0.9659258262890683122, 1.000000000000000000, 0.9659258262890683122, 1.000000000000000000, 0.9659258262890683122, 1.000000000000000000, 0.9659258262890683122, 1.000000000000000000, 0.9659258262890683122, 1.000000000000000000, 0.9659258262890683122, 1.000000000000000000, 0.9659258262890683122, 1.000000000000000000, 0.9659258262890683122, 1.000000000000000000, 0.9659258262890683122, 1.000000000000000000, 0.9659258262890683122, 1.000000000000000000),
 ( 0.3333333333333333703, 0.3219752754296894559, 0.3333333333333333703, 0.3219752754296894559, 0.3333333333333333703, 0.3219752754296894559, 0.3333333333333333703, 0.3219752754296894559, 0.3333333333333333703, 0.3219752754296894559, 0.3333333333333333703, 0.3219752754296894559, 0.3333333333333333703, 0.3219752754296894559, 0.3333333333333333703, 0.3219752754296894559, 0.3333333333333333703, 0.3219752754296894559, 0.3333333333333333703, 0.3219752754296894559, 0.3333333333333333703, 0.3219752754296894559, 0.3333333333333333703, 0.3219752754296894559, 0.3333333333333333703, 0.3219752754296894559, 0.3333333333333333703, 0.3219752754296894559, 0.3333333333333333703, 0.3219752754296894559, 0.3333333333333333703, 0.3219752754296894559, 0.3333333333333333703, 0.3219752754296894559, 0.3333333333333333703, 0.3219752754296894559, 0.3333333333333333703, 0.3219752754296894559, 0.3333333333333333703, 0.3219752754296894559, 0.3333333333333333703, 0.3219752754296894559, 0.3333333333333333703, 0.3219752754296894559, 0.3333333333333333703, 0.3219752754296894559, 0.3333333333333333703, 0.3219752754296894559, 0.3333333333333333703, 0.3219752754296894559, 0.3333333333333333703, 0.3219752754296894559, 0.3333333333333333703, 0.3219752754296894559, 0.3333333333333333703, 0.3219752754296894559, 0.3333333333333333703, 0.3219752754296894559, 0.3333333333333333703, 0.3219752754296894559, 0.3333333333333333703, 0.3219752754296894559, 0.3333333333333333703, 0.3219752754296894559, 0.3333333333333333703, 0.3219752754296894559, 0.3333333333333333703, 0.3219752754296894559, 0.3333333333333333703, 0.3219752754296894559, 0.3333333333333333703, 0.3219752754296894559, 0.3333333333333333703, 0.3219752754296894559, 0.3333333333333333703, 0.3219752754296894559, 0.3333333333333333703, 0.3219752754296894559, 0.3333333333333333703, 0.3219752754296894559, 0.3333333333333333703, 0.3219752754296894559, 0.3333333333333333703, 0.3219752754296894559, 0.3333333333333333703, 0.3219752754296894559, 0.3333333333333333703, 0.3219752754296894559, 0.3333333333333333703, 0.3219752754296894559, 0.3333333333333333703, 0.3219752754296894559, 0.3333333333333333703, 0.3219752754296894559, 0.3333333333333333703, 0.3219752754296894559, 0.3333333333333333703, 0.3219752754296894559, 0.3333333333333333703, 0.3219752754296894559, 0.3333333333333333703, 0.3219752754296894559, 0.3333333333333333703, 0.3219752754296894559, 0.3333333333333333703, 0.3219752754296894559, 0.3333333333333333703, 0.3219752754296894559, 0.3333333333333333703, 0.3219752754296894559, 0.3333333333333333703, 0.3219752754296894559, 0.3333333333333333703, 0.3219752754296894559, 0.3333333333333333703, 0.3219752754296894559, 0.3333333333333333703, 0.3219752754296894559, 0.3333333333333333703, 0.3219752754296894559, 0.3333333333333333703, 0.3219752754296894559, 0.3333333333333333703, 0.3219752754296894559, 0.3333333333333333703, 0.3219752754296894559, 0.3333333333333333703, 0.3219752754296894559, 0.3333333333333333703, 0.3219752754296894559, 0.3333333333333333703, 0.3219752754296894559, 0.3333333333333333703, 0.3219752754296894559, 0.3333333333333333703, 0.3219752754296894559, 0.3333333333333333703, 0.3219752754296894559, 0.3333333333333333703, 0.3219752754296894559, 0.3333333333333333703, 0.3219752754296894559, 0.3333333333333333703, 0.3219752754296894559, 0.3333333333333333703, 0.3219752754296894559, 0.3333333333333333703, 0.3219752754296894559, 0.3333333333333333703, 0.3219752754296894559, 0.3333333333333333703, 0.3219752754296894559, 0.3333333333333333703, 0.3219752754296894559, 0.3333333333333333703, 0.3219752754296894559, 0.3333333333333333703, 0.3219752754296894559, 0.3333333333333333703, 0.3219752754296894559, 0.3333333333333333703, 0.3219752754296894559, 0.3333333333333333703, 0.3219752754296894559, 0.3333333333333333703, 0.3219752754296894559, 0.3333333333333333703, 0.3219752754296894559, 0.3333333333333333703, 0.3219752754296894559, 0.3333333333333333703, 0.3219752754296894559, 0.3333333333333333703, 0.3219752754296894559, 0.3333333333333333703, 0.3219752754296894559, 0.3333333333333333703, 0.3219752754296894559, 0.3333333333333333703, 0.3219752754296894559, 0.3333333333333333703, 0.3219752754296894559, 0.3333333333333333703, 0.3219752754296894559, 0.3333333333333333703, 0.3219752754296894559, 0.3333333333333333703, 0.3219752754296894559, 0.3333333333333333703, 0.3219752754296894559, 0.3333333333333333703, 0.3219752754296894559, 0.3333333333333333703, 0.3219752754296894559, 0.3333333333333333703, 0.3219752754296894559, 0.3333333333333333703, 0.3219752754296894559, 0.3333333333333333703, 0.3219752754296894559, 0.3333333333333333703, 0.3219752754296894559, 0.3333333333333333703, 0.3219752754296894559, 0.3333333333333333703, 0.3219752754296894559, 0.3333333333333333703, 0.3219752754296894559, 0.3333333333333333703, 0.3219752754296894559, 0.3333333333333333703, 0.3219752754296894559, 0.3333333333333333703, 0.3219752754296894559, 0.3333333333333333703, 0.3219752754296894559, 0.3333333333333333703, 0.3219752754296894559, 0.3333333333333333703, 0.3219752754296894559, 0.3333333333333333703, 0.3219752754296894559, 0.3333333333333333703, 0.3219752754296894559, 0.3333333333333333703, 0.3219752754296894559, 0.3333333333333333703, 0.3219752754296894559, 0.3333333333333333703, 0.3219752754296894559, 0.3333333333333333703, 0.3219752754296894559, 0.3333333333333333703, 0.3219752754296894559, 0.3333333333333333703, 0.3219752754296894559, 0.3333333333333333703, 0.3219752754296894559, 0.3333333333333333703, 0.3219752754296894559, 0.3333333333333333703, 0.3219752754296894559, 0.3333333333333333703, 0.3219752754296894559, 0.3333333333333333703, 0.3219752754296894559, 0.3333333333333333703, 0.3219752754296894559, 0.3333333333333333703, 0.3219752754296894559, 0.3333333333333333703, 0.3219752754296894559, 0.3333333333333333703, 0.3219752754296894559, 0.3333333333333333703, 0.3219752754296894559, 0.3333333333333333703, 0.3219752754296894559, 0.3333333333333333703, 0.3219752754296894559, 0.3333333333333333703, 0.3219752754296894559, 0.3333333333333333703, 0.3219752754296894559, 0.3333333333333333703, 0.3219752754296894559, 0.3333333333333333703, 0.3219752754296894559, 0.3333333333333333703, 0.3219752754296894559, 0.3333333333333333703, 0.3219752754296894559, 0.3333333333333333703, 0.3219752754296894559, 0.3333333333333333703, 0.3219752754296894559, 0.3333333333333333703, 0.3219752754296894559, 0.3333333333333333703, 0.3219752754296894559, 0.3333333333333333703, 0.3219752754296894559, 0.3333333333333333703, 0.3219752754296894559, 0.3333333333333333703, 0.3219752754296894559, 0.3333333333333333703, 0.3219752754296894559, 0.3333333333333333703, 0.3219752754296894559, 0.3333333333333333703, 0.3219752754296894559, 0.3333333333333333703, 0.3219752754296894559, 0.3333333333333333703, 0.3219752754296894559, 0.3333333333333333703, 0.3219752754296894559, 0.3333333333333333703, 0.3219752754296894559, 0.3333333333333333703, 0.3219752754296894559, 0.3333333333333333703, 0.3219752754296894559, 0.3333333333333333703, 0.3219752754296894559, 0.3333333333333333703, 0.3219752754296894559, 0.3333333333333333703, 0.3219752754296894559, 0.3333333333333333703, 0.3219752754296894559, 0.3333333333333333703, 0.3219752754296894559, 0.3333333333333333703, 0.3219752754296894559, 0.3333333333333333703, 0.3219752754296894559, 0.3333333333333333703, 0.3219752754296894559, 0.3333333333333333703, 0.3219752754296894559, 0.3333333333333333703, 0.3219752754296894559, 0.3333333333333333703, 0.3219752754296894559, 0.3333333333333333703, 0.3219752754296894559, 0.3333333333333333703, 0.3219752754296894559, 0.3333333333333333703, 0.3219752754296894559, 0.3333333333333333703, 0.3219752754296894559, 0.3333333333333333703, 0.3219752754296894559, 0.3333333333333333703, 0.3219752754296894559, 0.3333333333333333703, 0.3219752754296894559, 0.3333333333333333703, 0.3219752754296894559, 0.3333333333333333703, 0.3219752754296894559, 0.3333333333333333703, 0.3219752754296894559, 0.3333333333333333703, 0.3219752754296894559, 0.3333333333333333703, 0.3219752754296894559, 0.3333333333333333703, 0.3219752754296894559, 0.3333333333333333703, 0.3219752754296894559, 0.3333333333333333703, 0.3219752754296894559, 0.3333333333333333703, 0.3219752754296894559, 0.3333333333333333703, 0.3219752754296894559, 0.3333333333333333703, 0.3219752754296894559, 0.3333333333333333703, 0.3219752754296894559, 0.3333333333333333703, 0.3219752754296894559, 0.3333333333333333703, 0.3219752754296894559, 0.3333333333333333703, 0.3219752754296894559, 0.3333333333333333703, 0.3219752754296894559, 0.3333333333333333703, 0.3219752754296894559, 0.3333333333333333703, 0.3219752754296894559, 0.3333333333333333703, 0.3219752754296894559, 0.3333333333333333703, 0.3219752754296894559, 0.3333333333333333703, 0.3219752754296894559, 0.3333333333333333703, 0.3219752754296894559, 0.3333333333333333703, 0.3219752754296894559, 0.3333333333333333703, 0.3219752754296894559, 0.3333333333333333703, 0.3219752754296894559, 0.3333333333333333703, 0.3219752754296894559, 0.3333333333333333703, 0.3219752754296894559, 0.3333333333333333703, 0.3219752754296894559, 0.3333333333333333703, 0.3219752754296894559, 0.3333333333333333703, 0.3219752754296894559, 0.3333333333333333703, 0.3219752754296894559, 0.3333333333333333703, 0.3219752754296894559, 0.3333333333333333703, 0.3219752754296894559, 0.3333333333333333703, 0.3219752754296894559, 0.3333333333333333703, 0.3219752754296894559, 0.3333333333333333703, 0.3219752754296894559, 0.3333333333333333703, 0.3219752754296894559, 0.3333333333333333703, 0.3219752754296894559, 0.3333333333333333703, 0.3219752754296894559, 0.3333333333333333703, 0.3219752754296894559, 0.3333333333333333703, 0.3219752754296894559, 0.3333333333333333703, 0.3219752754296894559, 0.3333333333333333703, 0.3219752754296894559, 0.3333333333333333703, 0.3219752754296894559, 0.3333333333333333703, 0.3219752754296894559, 0.3333333333333333703, 0.3219752754296894559, 0.3333333333333333703, 0.3219752754296894559, 0.3333333333333333703, 0.3219752754296894559, 0.3333333333333333703, 0.3219752754296894559, 0.3333333333333333703, 0.3219752754296894559, 0.3333333333333333703, 0.3219752754296894559, 0.3333333333333333703, 0.3219752754296894559, 0.3333333333333333703, 0.3219752754296894559, 0.3333333333333333703, 0.3219752754296894559, 0.3333333333333333703, 0.3219752754296894559, 0.3333333333333333703, 0.3219752754296894559, 0.3333333333333333703, 0.3219752754296894559, 0.3333333333333333703, 0.3219752754296894559, 0.3333333333333333703),
 ( 0.3333333333333333703, 0.3219752754296894559, 0.3333333333333333703, 0.3219752754296894559, 0.3333333333333333703, 0.3219752754296894559, 0.3333333333333333703, 0.3219752754296894559, 0.3333333333333333703, 0.3219752754296894559, 0.3333333333333333703, 0.3219752754296894559, 0.3333333333333333703, 0.3219752754296894559, 0.3333333333333333703, 0.3219752754296894559, 0.3333333333333333703, 0.3219752754296894559, 0.3333333333333333703, 0.3219752754296894559, 0.3333333333333333703, 0.3219752754296894559, 0.3333333333333333703, 0.3219752754296894559, 0.3333333333333333703, 0.3219752754296894559, 0.3333333333333333703, 0.3219752754296894559, 0.3333333333333333703, 0.3219752754296894559, 0.3333333333333333703, 0.3219752754296894559, 0.3333333333333333703, 0.3219752754296894559, 0.3333333333333333703, 0.3219752754296894559, 0.3333333333333333703, 0.3219752754296894559, 0.3333333333333333703, 0.3219752754296894559, 0.3333333333333333703, 0.3219752754296894559, 0.3333333333333333703, 0.3219752754296894559, 0.3333333333333333703, 0.3219752754296894559, 0.3333333333333333703, 0.3219752754296894559, 0.3333333333333333703, 0.3219752754296894559, 0.3333333333333333703, 0.3219752754296894559, 0.3333333333333333703, 0.3219752754296894559, 0.3333333333333333703, 0.3219752754296894559, 0.3333333333333333703, 0.3219752754296894559, 0.3333333333333333703, 0.3219752754296894559, 0.3333333333333333703, 0.3219752754296894559, 0.3333333333333333703, 0.3219752754296894559, 0.3333333333333333703, 0.3219752754296894559, 0.3333333333333333703, 0.3219752754296894559, 0.3333333333333333703, 0.3219752754296894559, 0.3333333333333333703, 0.3219752754296894559, 0.3333333333333333703, 0.3219752754296894559, 0.3333333333333333703, 0.3219752754296894559, 0.3333333333333333703, 0.3219752754296894559, 0.3333333333333333703, 0.3219752754296894559, 0.3333333333333333703, 0.3219752754296894559, 0.3333333333333333703, 0.3219752754296894559, 0.3333333333333333703, 0.3219752754296894559, 0.3333333333333333703, 0.3219752754296894559, 0.3333333333333333703, 0.3219752754296894559, 0.3333333333333333703, 0.3219752754296894559, 0.3333333333333333703, 0.3219752754296894559, 0.3333333333333333703, 0.3219752754296894559, 0.3333333333333333703, 0.3219752754296894559, 0.3333333333333333703, 0.3219752754296894559, 0.3333333333333333703, 0.3219752754296894559, 0.3333333333333333703, 0.3219752754296894559, 0.3333333333333333703, 0.3219752754296894559, 0.3333333333333333703, 0.3219752754296894559, 0.3333333333333333703, 0.3219752754296894559, 0.3333333333333333703, 0.3219752754296894559, 0.3333333333333333703, 0.3219752754296894559, 0.3333333333333333703, 0.3219752754296894559, 0.3333333333333333703, 0.3219752754296894559, 0.3333333333333333703, 0.3219752754296894559, 0.3333333333333333703, 0.3219752754296894559, 0.3333333333333333703, 0.3219752754296894559, 0.3333333333333333703, 0.3219752754296894559, 0.3333333333333333703, 0.3219752754296894559, 0.3333333333333333703, 0.3219752754296894559, 0.3333333333333333703, 0.3219752754296894559, 0.3333333333333333703, 0.3219752754296894559, 0.3333333333333333703, 0.3219752754296894559, 0.3333333333333333703, 0.3219752754296894559, 0.3333333333333333703, 0.3219752754296894559, 0.3333333333333333703, 0.3219752754296894559, 0.3333333333333333703, 0.3219752754296894559, 0.3333333333333333703, 0.3219752754296894559, 0.3333333333333333703, 0.3219752754296894559, 0.3333333333333333703, 0.3219752754296894559, 0.3333333333333333703, 0.3219752754296894559, 0.3333333333333333703, 0.3219752754296894559, 0.3333333333333333703, 0.3219752754296894559, 0.3333333333333333703, 0.3219752754296894559, 0.3333333333333333703, 0.3219752754296894559, 0.3333333333333333703, 0.3219752754296894559, 0.3333333333333333703, 0.3219752754296894559, 0.3333333333333333703, 0.3219752754296894559, 0.3333333333333333703, 0.3219752754296894559, 0.3333333333333333703, 0.3219752754296894559, 0.3333333333333333703, 0.3219752754296894559, 0.3333333333333333703, 0.3219752754296894559, 0.3333333333333333703, 0.3219752754296894559, 0.3333333333333333703, 0.3219752754296894559, 0.3333333333333333703, 0.3219752754296894559, 0.3333333333333333703, 0.3219752754296894559, 0.3333333333333333703, 0.3219752754296894559, 0.3333333333333333703, 0.3219752754296894559, 0.3333333333333333703, 0.3219752754296894559, 0.3333333333333333703, 0.3219752754296894559, 0.3333333333333333703, 0.3219752754296894559, 0.3333333333333333703, 0.3219752754296894559, 0.3333333333333333703, 0.3219752754296894559, 0.3333333333333333703, 0.3219752754296894559, 0.3333333333333333703, 0.3219752754296894559, 0.3333333333333333703, 0.3219752754296894559, 0.3333333333333333703, 0.3219752754296894559, 0.3333333333333333703, 0.3219752754296894559, 0.3333333333333333703, 0.3219752754296894559, 0.3333333333333333703, 0.3219752754296894559, 0.3333333333333333703, 0.3219752754296894559, 0.3333333333333333703, 0.3219752754296894559, 0.3333333333333333703, 0.3219752754296894559, 0.3333333333333333703, 0.3219752754296894559, 0.3333333333333333703, 0.3219752754296894559, 0.3333333333333333703, 0.3219752754296894559, 0.3333333333333333703, 0.3219752754296894559, 0.3333333333333333703, 0.3219752754296894559, 0.3333333333333333703, 0.3219752754296894559, 0.3333333333333333703, 0.3219752754296894559, 0.3333333333333333703, 0.3219752754296894559, 0.3333333333333333703, 0.3219752754296894559, 0.3333333333333333703, 0.3219752754296894559, 0.3333333333333333703, 0.3219752754296894559, 0.3333333333333333703, 0.3219752754296894559, 0.3333333333333333703, 0.3219752754296894559, 0.3333333333333333703, 0.3219752754296894559, 0.3333333333333333703, 0.3219752754296894559, 0.3333333333333333703, 0.3219752754296894559, 0.3333333333333333703, 0.3219752754296894559, 0.3333333333333333703, 0.3219752754296894559, 0.3333333333333333703, 0.3219752754296894559, 0.3333333333333333703, 0.3219752754296894559, 0.3333333333333333703, 0.3219752754296894559, 0.3333333333333333703, 0.3219752754296894559, 0.3333333333333333703, 0.3219752754296894559, 0.3333333333333333703, 0.3219752754296894559, 0.3333333333333333703, 0.3219752754296894559, 0.3333333333333333703, 0.3219752754296894559, 0.3333333333333333703, 0.3219752754296894559, 0.3333333333333333703, 0.3219752754296894559, 0.3333333333333333703, 0.3219752754296894559, 0.3333333333333333703, 0.3219752754296894559, 0.3333333333333333703, 0.3219752754296894559, 0.3333333333333333703, 0.3219752754296894559, 0.3333333333333333703, 0.3219752754296894559, 0.3333333333333333703, 0.3219752754296894559, 0.3333333333333333703, 0.3219752754296894559, 0.3333333333333333703, 0.3219752754296894559, 0.3333333333333333703, 0.3219752754296894559, 0.3333333333333333703, 0.3219752754296894559, 0.3333333333333333703, 0.3219752754296894559, 0.3333333333333333703, 0.3219752754296894559, 0.3333333333333333703, 0.3219752754296894559, 0.3333333333333333703, 0.3219752754296894559, 0.3333333333333333703, 0.3219752754296894559, 0.3333333333333333703, 0.3219752754296894559, 0.3333333333333333703, 0.3219752754296894559, 0.3333333333333333703, 0.3219752754296894559, 0.3333333333333333703, 0.3219752754296894559, 0.3333333333333333703, 0.3219752754296894559, 0.3333333333333333703, 0.3219752754296894559, 0.3333333333333333703, 0.3219752754296894559, 0.3333333333333333703, 0.3219752754296894559, 0.3333333333333333703, 0.3219752754296894559, 0.3333333333333333703, 0.3219752754296894559, 0.3333333333333333703, 0.3219752754296894559, 0.3333333333333333703, 0.3219752754296894559, 0.3333333333333333703, 0.3219752754296894559, 0.3333333333333333703, 0.3219752754296894559, 0.3333333333333333703, 0.3219752754296894559, 0.3333333333333333703, 0.3219752754296894559, 0.3333333333333333703, 0.3219752754296894559, 0.3333333333333333703, 0.3219752754296894559, 0.3333333333333333703, 0.3219752754296894559, 0.3333333333333333703, 0.3219752754296894559, 0.3333333333333333703, 0.3219752754296894559, 0.3333333333333333703, 0.3219752754296894559, 0.3333333333333333703, 0.3219752754296894559, 0.3333333333333333703, 0.3219752754296894559, 0.3333333333333333703, 0.3219752754296894559, 0.3333333333333333703, 0.3219752754296894559, 0.3333333333333333703, 0.3219752754296894559, 0.3333333333333333703, 0.3219752754296894559, 0.3333333333333333703, 0.3219752754296894559, 0.3333333333333333703, 0.3219752754296894559, 0.3333333333333333703, 0.3219752754296894559, 0.3333333333333333703, 0.3219752754296894559, 0.3333333333333333703, 0.3219752754296894559, 0.3333333333333333703, 0.3219752754296894559, 0.3333333333333333703, 0.3219752754296894559, 0.3333333333333333703, 0.3219752754296894559, 0.3333333333333333703, 0.3219752754296894559, 0.3333333333333333703, 0.3219752754296894559, 0.3333333333333333703, 0.3219752754296894559, 0.3333333333333333703, 0.3219752754296894559, 0.3333333333333333703, 0.3219752754296894559, 0.3333333333333333703, 0.3219752754296894559, 0.3333333333333333703, 0.3219752754296894559, 0.3333333333333333703, 0.3219752754296894559, 0.3333333333333333703, 0.3219752754296894559, 0.3333333333333333703, 0.3219752754296894559, 0.3333333333333333703, 0.3219752754296894559, 0.3333333333333333703, 0.3219752754296894559, 0.3333333333333333703, 0.3219752754296894559, 0.3333333333333333703, 0.3219752754296894559, 0.3333333333333333703, 0.3219752754296894559, 0.3333333333333333703, 0.3219752754296894559, 0.3333333333333333703, 0.3219752754296894559, 0.3333333333333333703, 0.3219752754296894559, 0.3333333333333333703, 0.3219752754296894559, 0.3333333333333333703, 0.3219752754296894559, 0.3333333333333333703, 0.3219752754296894559, 0.3333333333333333703, 0.3219752754296894559, 0.3333333333333333703, 0.3219752754296894559, 0.3333333333333333703, 0.3219752754296894559, 0.3333333333333333703, 0.3219752754296894559, 0.3333333333333333703, 0.3219752754296894559, 0.3333333333333333703, 0.3219752754296894559, 0.3333333333333333703, 0.3219752754296894559, 0.3333333333333333703, 0.3219752754296894559, 0.3333333333333333703, 0.3219752754296894559, 0.3333333333333333703, 0.3219752754296894559, 0.3333333333333333703, 0.3219752754296894559, 0.3333333333333333703, 0.3219752754296894559, 0.3333333333333333703, 0.3219752754296894559, 0.3333333333333333703, 0.3219752754296894559, 0.3333333333333333703, 0.3219752754296894559, 0.3333333333333333703, 0.3219752754296894559, 0.3333333333333333703, 0.3219752754296894559, 0.3333333333333333703, 0.3219752754296894559, 0.3333333333333333703, 0.3219752754296894559, 0.3333333333333333703, 0.3219752754296894559, 0.3333333333333333703),
 ( 1.000000000000000000, 0.9659258262890683122, 1.000000000000000000, 0.9659258262890683122, 1.000000000000000000, 0.9659258262890683122, 1.000000000000000000, 0.9659258262890683122, 1.000000000000000000, 0.9659258262890683122, 1.000000000000000000, 0.9659258262890683122, 1.000000000000000000, 0.9659258262890683122, 1.000000000000000000, 0.9659258262890683122, 1.000000000000000000, 0.9659258262890683122, 1.000000000000000000, 0.9659258262890683122, 1.000000000000000000, 0.9659258262890683122, 1.000000000000000000, 0.9659258262890683122, 1.000000000000000000, 0.9659258262890683122, 1.000000000000000000, 0.9659258262890683122, 1.000000000000000000, 0.9659258262890683122, 1.000000000000000000, 0.9659258262890683122, 1.000000000000000000, 0.9659258262890683122, 1.000000000000000000, 0.9659258262890683122, 1.000000000000000000, 0.9659258262890683122, 1.000000000000000000, 0.9659258262890683122, 1.000000000000000000, 0.9659258262890683122, 1.000000000000000000, 0.9659258262890683122, 1.000000000000000000, 0.9659258262890683122, 1.000000000000000000, 0.9659258262890683122, 1.000000000000000000, 0.9659258262890683122, 1.000000000000000000, 0.9659258262890683122, 1.000000000000000000, 0.9659258262890683122, 1.000000000000000000, 0.9659258262890683122, 1.000000000000000000, 0.9659258262890683122, 1.000000000000000000, 0.9659258262890683122, 1.000000000000000000, 0.9659258262890683122, 1.000000000000000000, 0.9659258262890683122, 1.000000000000000000, 0.9659258262890683122, 1.000000000000000000, 0.9659258262890683122, 1.000000000000000000, 0.9659258262890683122, 1.000000000000000000, 0.9659258262890683122, 1.000000000000000000, 0.9659258262890683122, 1.000000000000000000, 0.9659258262890683122, 1.000000000000000000, 0.9659258262890683122, 1.000000000000000000, 0.9659258262890683122, 1.000000000000000000, 0.9659258262890683122, 1.000000000000000000, 0.9659258262890683122, 1.000000000000000000, 0.9659258262890683122, 1.000000000000000000, 0.9659258262890683122, 1.000000000000000000, 0.9659258262890683122, 1.000000000000000000, 0.9659258262890683122, 1.000000000000000000, 0.9659258262890683122, 1.000000000000000000, 0.9659258262890683122, 1.000000000000000000, 0.9659258262890683122, 1.000000000000000000, 0.9659258262890683122, 1.000000000000000000, 0.9659258262890683122, 1.000000000000000000, 0.9659258262890683122, 1.000000000000000000, 0.9659258262890683122, 1.000000000000000000, 0.9659258262890683122, 1.000000000000000000, 0.9659258262890683122, 1.000000000000000000, 0.9659258262890683122, 1.000000000000000000, 0.9659258262890683122, 1.000000000000000000, 0.9659258262890683122, 1.000000000000000000, 0.9659258262890683122, 1.000000000000000000, 0.9659258262890683122, 1.000000000000000000, 0.9659258262890683122, 1.000000000000000000, 0.9659258262890683122, 1.000000000000000000, 0.9659258262890683122, 1.000000000000000000, 0.9659258262890683122, 1.000000000000000000, 0.9659258262890683122, 1.000000000000000000, 0.9659258262890683122, 1.000000000000000000, 0.9659258262890683122, 1.000000000000000000, 0.9659258262890683122, 1.000000000000000000, 0.9659258262890683122, 1.000000000000000000, 0.9659258262890683122, 1.000000000000000000, 0.9659258262890683122, 1.000000000000000000, 0.9659258262890683122, 1.000000000000000000, 0.9659258262890683122, 1.000000000000000000, 0.9659258262890683122, 1.000000000000000000, 0.9659258262890683122, 1.000000000000000000, 0.9659258262890683122, 1.000000000000000000, 0.9659258262890683122, 1.000000000000000000, 0.9659258262890683122, 1.000000000000000000, 0.9659258262890683122, 1.000000000000000000, 0.9659258262890683122, 1.000000000000000000, 0.9659258262890683122, 1.000000000000000000, 0.9659258262890683122, 1.000000000000000000, 0.9659258262890683122, 1.000000000000000000, 0.9659258262890683122, 1.000000000000000000, 0.9659258262890683122, 1.000000000000000000, 0.9659258262890683122, 1.000000000000000000, 0.9659258262890683122, 1.000000000000000000, 0.9659258262890683122, 1.000000000000000000, 0.9659258262890683122, 1.000000000000000000, 0.9659258262890683122, 1.000000000000000000, 0.9659258262890683122, 1.000000000000000000, 0.9659258262890683122, 1.000000000000000000, 0.9659258262890683122, 1.000000000000000000, 0.9659258262890683122, 1.000000000000000000, 0.9659258262890683122, 1.000000000000000000, 0.9659258262890683122, 1.000000000000000000, 0.9659258262890683122, 1.000000000000000000, 0.9659258262890683122, 1.000000000000000000, 0.9659258262890683122, 1.000000000000000000, 0.9659258262890683122, 1.000000000000000000, 0.9659258262890683122, 1.000000000000000000, 0.9659258262890683122, 1.000000000000000000, 0.9659258262890683122, 1.000000000000000000, 0.9659258262890683122, 1.000000000000000000, 0.9659258262890683122, 1.000000000000000000, 0.9659258262890683122, 1.000000000000000000, 0.9659258262890683122, 1.000000000000000000, 0.9659258262890683122, 1.000000000000000000, 0.9659258262890683122, 1.000000000000000000, 0.9659258262890683122, 1.000000000000000000, 0.9659258262890683122, 1.000000000000000000, 0.9659258262890683122, 1.000000000000000000, 0.9659258262890683122, 1.000000000000000000, 0.9659258262890683122, 1.000000000000000000, 0.9659258262890683122, 1.000000000000000000, 0.9659258262890683122, 1.000000000000000000, 0.9659258262890683122, 1.000000000000000000, 0.9659258262890683122, 1.000000000000000000, 0.9659258262890683122, 1.000000000000000000, 0.9659258262890683122, 1.000000000000000000, 0.9659258262890683122, 1.000000000000000000, 0.9659258262890683122, 1.000000000000000000, 0.9659258262890683122, 1.000000000000000000, 0.9659258262890683122, 1.000000000000000000, 0.9659258262890683122, 1.000000000000000000, 0.9659258262890683122, 1.000000000000000000, 0.9659258262890683122, 1.000000000000000000, 0.9659258262890683122, 1.000000000000000000, 0.9659258262890683122, 1.000000000000000000, 0.9659258262890683122, 1.000000000000000000, 0.9659258262890683122, 1.000000000000000000, 0.9659258262890683122, 1.000000000000000000, 0.9659258262890683122, 1.000000000000000000, 0.9659258262890683122, 1.000000000000000000, 0.9659258262890683122, 1.000000000000000000, 0.9659258262890683122, 1.000000000000000000, 0.9659258262890683122, 1.000000000000000000, 0.9659258262890683122, 1.000000000000000000, 0.9659258262890683122, 1.000000000000000000, 0.9659258262890683122, 1.000000000000000000, 0.9659258262890683122, 1.000000000000000000, 0.9659258262890683122, 1.000000000000000000, 0.9659258262890683122, 1.000000000000000000, 0.9659258262890683122, 1.000000000000000000, 0.9659258262890683122, 1.000000000000000000, 0.9659258262890683122, 1.000000000000000000, 0.9659258262890683122, 1.000000000000000000, 0.9659258262890683122, 1.000000000000000000, 0.9659258262890683122, 1.000000000000000000, 0.9659258262890683122, 1.000000000000000000, 0.9659258262890683122, 1.000000000000000000, 0.9659258262890683122, 1.000000000000000000, 0.9659258262890683122, 1.000000000000000000, 0.9659258262890683122, 1.000000000000000000, 0.9659258262890683122, 1.000000000000000000, 0.9659258262890683122, 1.000000000000000000, 0.9659258262890683122, 1.000000000000000000, 0.9659258262890683122, 1.000000000000000000, 0.9659258262890683122, 1.000000000000000000, 0.9659258262890683122, 1.000000000000000000, 0.9659258262890683122, 1.000000000000000000, 0.9659258262890683122, 1.000000000000000000, 0.9659258262890683122, 1.000000000000000000, 0.9659258262890683122, 1.000000000000000000, 0.9659258262890683122, 1.000000000000000000, 0.9659258262890683122, 1.000000000000000000, 0.9659258262890683122, 1.000000000000000000, 0.9659258262890683122, 1.000000000000000000, 0.9659258262890683122, 1.000000000000000000, 0.9659258262890683122, 1.000000000000000000, 0.9659258262890683122, 1.000000000000000000, 0.9659258262890683122, 1.000000000000000000, 0.9659258262890683122, 1.000000000000000000, 0.9659258262890683122, 1.000000000000000000, 0.9659258262890683122, 1.000000000000000000, 0.9659258262890683122, 1.000000000000000000, 0.9659258262890683122, 1.000000000000000000, 0.9659258262890683122, 1.000000000000000000, 0.9659258262890683122, 1.000000000000000000, 0.9659258262890683122, 1.000000000000000000, 0.9659258262890683122, 1.000000000000000000, 0.9659258262890683122, 1.000000000000000000, 0.9659258262890683122, 1.000000000000000000, 0.9659258262890683122, 1.000000000000000000, 0.9659258262890683122, 1.000000000000000000, 0.9659258262890683122, 1.000000000000000000, 0.9659258262890683122, 1.000000000000000000, 0.9659258262890683122, 1.000000000000000000, 0.9659258262890683122, 1.000000000000000000, 0.9659258262890683122, 1.000000000000000000, 0.9659258262890683122, 1.000000000000000000, 0.9659258262890683122, 1.000000000000000000, 0.9659258262890683122, 1.000000000000000000, 0.9659258262890683122, 1.000000000000000000, 0.9659258262890683122, 1.000000000000000000, 0.9659258262890683122, 1.000000000000000000, 0.9659258262890683122, 1.000000000000000000, 0.9659258262890683122, 1.000000000000000000, 0.9659258262890683122, 1.000000000000000000, 0.9659258262890683122, 1.000000000000000000, 0.9659258262890683122, 1.000000000000000000, 0.9659258262890683122, 1.000000000000000000, 0.9659258262890683122, 1.000000000000000000, 0.9659258262890683122, 1.000000000000000000, 0.9659258262890683122, 1.000000000000000000, 0.9659258262890683122, 1.000000000000000000, 0.9659258262890683122, 1.000000000000000000, 0.9659258262890683122, 1.000000000000000000, 0.9659258262890683122, 1.000000000000000000, 0.9659258262890683122, 1.000000000000000000, 0.9659258262890683122, 1.000000000000000000, 0.9659258262890683122, 1.000000000000000000, 0.9659258262890683122, 1.000000000000000000, 0.9659258262890683122, 1.000000000000000000, 0.9659258262890683122, 1.000000000000000000, 0.9659258262890683122, 1.000000000000000000, 0.9659258262890683122, 1.000000000000000000, 0.9659258262890683122, 1.000000000000000000, 0.9659258262890683122, 1.000000000000000000, 0.9659258262890683122, 1.000000000000000000, 0.9659258262890683122, 1.000000000000000000, 0.9659258262890683122, 1.000000000000000000, 0.9659258262890683122, 1.000000000000000000, 0.9659258262890683122, 1.000000000000000000, 0.9659258262890683122, 1.000000000000000000, 0.9659258262890683122, 1.000000000000000000, 0.9659258262890683122, 1.000000000000000000, 0.9659258262890683122, 1.000000000000000000) ) ) 
 REPRESENTATION_ITEM ( '' )  SURFACE ( )  );
#47938=CARTESIAN_POINT ( 'NONE',  ( -16.46253265017160317, 9.564922557960807481, 45.83224293864769550 ) ) ;
#47939=CARTESIAN_POINT ( 'NONE',  ( -8.314922557961024197, 14.29746914071037800, 92.91775706135236135 ) ) ;
#47941=CARTESIAN_POINT ( 'NONE',  ( 10.81492255796078972, 18.62759615963270932, 99.58224293864770971 ) ) ;
#47942=CARTESIAN_POINT ( 'NONE',  ( -12.14591786802309592, -12.06949235617757132, 46.87390960531435979 ) ) ;
#47943=CARTESIAN_POINT ( 'NONE',  ( -19.05341960407611168, -5.049401038298163336, 86.45724293864769550 ) ) ;
#47944=CARTESIAN_POINT ( 'NONE',  ( 0.05219959533934541429, -16.53943276465976808, 80.00109039468568994 ) ) ;
#47945=CARTESIAN_POINT ( 'NONE',  ( -19.03943276465977164, -0.05219959533935918106, 108.7510903946856615 ) ) ;
#47946=CARTESIAN_POINT ( 'NONE',  ( -21.52544592524334988, -5.823673210054445271, 18.95942372801901143 ) ) ;
#47947=CARTESIAN_POINT ( 'NONE',  ( 14.29746914071049879, -8.314922557960816363, 43.33224293864769550 ) ) ;
#47949=CARTESIAN_POINT ( 'NONE',  ( -17.12812012977029141, 6.668231424565931320, 68.64051240676857901 ) ) ;
#47950=CARTESIAN_POINT ( 'NONE',  ( -21.55341960407610458, -5.719274019375992779, 86.45724293864770971 ) ) ;
#47951=CARTESIAN_POINT ( 'NONE',  ( -4.379528057220328563, 16.55341960407611168, 30.20724293864769550 ) ) ;
#47953=CARTESIAN_POINT ( 'NONE',  ( -17.13100169013299379, -6.664070546373171311, 54.23210164300153480 ) ) ;
#47954=CARTESIAN_POINT ( 'NONE',  ( 10.81492255796078972, 18.62759615963270932, 114.5822429386477097 ) ) ;
#47955=CARTESIAN_POINT ( 'NONE',  ( -13.89961937509977652, 13.97604488694528158, 110.6239096053143243 ) ) ;
#47956=CARTESIAN_POINT ( 'NONE',  ( -21.55341960407619339, 5.719274019375674811, 28.54275706135234358 ) ) ;
#47957=CARTESIAN_POINT ( 'NONE',  ( -16.53943276465976808, 0.05219959533911058130, 56.24890960531436690 ) ) ;
#47958=CARTESIAN_POINT ( 'NONE',  ( 8.224510206698742110, 14.34966873604972548, 42.08442372801901854 ) ) ;
#47959=CARTESIAN_POINT ( 'NONE',  ( 5.153800228976335163, 19.02544592524342804, 59.79057627198100988 ) ) ;
#47960=CARTESIAN_POINT ( 'NONE',  ( -9.474510206698720793, -16.51473224551083518, 49.58442372801899722 ) ) ;
#47961=CARTESIAN_POINT ( 'NONE',  ( 19.03943276465977164, -0.05219959533909143690, 73.74890960531435269 ) ) ;
#47962=CARTESIAN_POINT ( 'NONE',  ( -18.62759615963270932, 10.81492255796079327, 35.83224293864768839 ) ) ;
#47964=CARTESIAN_POINT ( 'NONE',  ( -0.05219959533909027116, -19.03943276465977164, 42.49890960531435269 ) ) ;
#47965=CARTESIAN_POINT ( 'NONE',  ( -4.379528057220086978, -16.55341960407618274, 19.79275706135235069 ) ) ;
#47966=CARTESIAN_POINT ( 'NONE',  ( 19.02544592524334988, 5.153800228976608722, 66.45942372801899012 ) ) ;
#47967=CARTESIAN_POINT ( 'NONE',  ( 18.62759615963271287, -10.81492255796078972, 98.33224293864769550 ) ) ;
#47968=CARTESIAN_POINT ( 'NONE',  ( -12.06949235617756955, 12.14591786802309770, 35.62390960531437401 ) ) ;
#47969=CARTESIAN_POINT ( 'NONE',  ( -16.46253265017160317, 9.564922557960807481, 90.83224293864769550 ) ) ;
#47970=CARTESIAN_POINT ( 'NONE',  ( 18.62759615963271287, -10.81492255796078972, 53.33224293864769550 ) ) ;
#47971=CARTESIAN_POINT ( 'NONE',  ( 10.81492255796078972, 18.62759615963270932, 99.58224293864770971 ) ) ;
#47972=CARTESIAN_POINT ( 'NONE',  ( -8.224510206698735004, -14.34966873604973081, 24.58442372801901499 ) ) ;
#47973=CARTESIAN_POINT ( 'NONE',  ( -21.52544592524343514, 5.823673210054127303, 36.04057627198102409 ) ) ;
#47974=CARTESIAN_POINT ( 'NONE',  ( -10.72451020669870658, -18.67979575497194134, 84.58442372801903275 ) ) ;
#47975=CARTESIAN_POINT ( 'NONE',  ( 9.564922557960805705, 16.46253265017160317, 89.58224293864769550 ) ) ;
#47976=CARTESIAN_POINT ( 'NONE',  ( 5.153800228976335163, 19.02544592524342804, 34.79057627198102409 ) ) ;
#47977=CARTESIAN_POINT ( 'NONE',  ( 19.03943276465977164, -0.05219959533909143690, 88.74890960531436690 ) ) ;
#47978=CARTESIAN_POINT ( 'NONE',  ( 16.53943276465976808, -0.05219959533910856209, 98.74890960531438111 ) ) ;
#47979=CARTESIAN_POINT ( 'NONE',  ( -5.153800228976328057, -19.02544592524343514, 67.29057627198102409 ) ) ;
#47980=CARTESIAN_POINT ( 'NONE',  ( -16.52544592524335698, -4.483927247898792601, 28.95942372801902209 ) ) ;
#47981=CARTESIAN_POINT ( 'NONE',  ( 17.40861289039007431, -6.110651285853167636, 86.12767529172568004 ) ) ;
#47982=CARTESIAN_POINT ( 'NONE',  ( -0.05219959533937732626, 21.53943276465977519, 92.50109039468567573 ) ) ;
#47983=CARTESIAN_POINT ( 'NONE',  ( 5.049401038298161559, -19.05341960407611168, 107.7072429386476955 ) ) ;
#47984=CARTESIAN_POINT ( 'NONE',  ( 12.06949235617739724, 12.14591786802326823, 86.87609039468568994 ) ) ;
#47985=PLANE ( 'NONE',  #113166 ) ;
#47986=CARTESIAN_POINT ( 'NONE',  ( -0.05219959533936034679, 19.03943276465977164, 72.50109039468566152 ) ) ;
#47987=CARTESIAN_POINT ( 'NONE',  ( 0.05219959533936267826, -19.03943276465977164, 35.00109039468566863 ) ) ;
#47988=CARTESIAN_POINT ( 'NONE',  ( 18.22780087662123805, -5.499999999999976019, 93.51763182126896368 ) ) ;
#47989=CARTESIAN_POINT ( 'NONE',  ( 19.05341960407611168, 5.049401038298154454, 23.95724293864769194 ) ) ;
#47990=CARTESIAN_POINT ( 'NONE',  ( -16.55341960407611168, -4.379528057220339221, 41.45724293864769550 ) ) ;
#47991=CARTESIAN_POINT ( 'NONE',  ( -16.51473224551069308, -9.474510206698971260, 21.66557627198102765 ) ) ;
#47992=CARTESIAN_POINT ( 'NONE',  ( -14.29746914071049879, 8.314922557960819915, 30.83224293864770260 ) ) ;
#47993=CARTESIAN_POINT ( 'NONE',  ( -19.49190055781010855, -5.499999999999973355, 85.56116087098779133 ) ) ;
#47994=CARTESIAN_POINT ( 'NONE',  ( 16.53943276465976808, 0.05219959533934440121, 101.2510903946856757 ) ) ;
#47995=CARTESIAN_POINT ( 'NONE',  ( 0.05219959533909260263, 19.03943276465977164, 34.99890960531435979 ) ) ;
#47996=CARTESIAN_POINT ( 'NONE',  ( -18.62759615963255300, -10.81492255796106328, 94.16775706135237556 ) ) ;
#47997=CARTESIAN_POINT ( 'NONE',  ( 5.153800228976615827, -19.02544592524334988, 105.2094237280190185 ) ) ;
#47998=CARTESIAN_POINT ( 'NONE',  ( 5.823673210054444382, -21.52544592524334988, 85.20942372801901854 ) ) ;
#47999=CARTESIAN_POINT ( 'NONE',  ( 5.153800228976615827, -19.02544592524334988, 55.20942372801899722 ) ) ;
#48000=CARTESIAN_POINT ( 'NONE',  ( -19.03943276465977164, 0.05219959533909376836, 91.24890960531436690 ) ) ;
#48001=CARTESIAN_POINT ( 'NONE',  ( 19.03943276465977164, -0.05219959533909143690, 73.74890960531435269 ) ) ;
#48002=CARTESIAN_POINT ( 'NONE',  ( 17.05116617787822975, 6.768360034955830606, 73.84324446740798464 ) ) ;
#48003=CARTESIAN_POINT ( 'NONE',  ( -12.06949235617756955, 12.14591786802309770, 70.62390960531436690 ) ) ;
#48004=CARTESIAN_POINT ( 'NONE',  ( 21.52544592524344225, -5.823673210054117533, 63.54057627198103830 ) ) ;
#48005=CARTESIAN_POINT ( 'NONE',  ( -13.89961937509977652, 13.97604488694528158, 60.62390960531436690 ) ) ;
#48006=CARTESIAN_POINT ( 'NONE',  ( 0.05219959533907565091, 21.53943276465977519, 79.99890960531435269 ) ) ;
#48007=CARTESIAN_POINT ( 'NONE',  ( 8.224510206698742110, 14.34966873604972548, 72.08442372801899012 ) ) ;
#48008=ORIENTED_EDGE ( 'NONE', *, *, #165748, .F. ) ;
#48009=CARTESIAN_POINT ( 'NONE',  ( -5.049401038298153566, 19.05341960407611168, 50.20724293864770260 ) ) ;
#48010=CARTESIAN_POINT ( 'NONE',  ( 12.14591786802309770, 12.06949235617756955, 84.37390960531438111 ) ) ;
#48012=CARTESIAN_POINT ( 'NONE',  ( -9.564922557960796823, -16.46253265017161027, 57.08224293864769550 ) ) ;
#48013=CARTESIAN_POINT ( 'NONE',  ( -8.224510206698948167, 14.34966873604960824, 110.4155762719810383 ) ) ;
#48014=CARTESIAN_POINT ( 'NONE',  ( -19.02544592524334988, -5.153800228976617603, 68.95942372801896170 ) ) ;
#48015=CARTESIAN_POINT ( 'NONE',  ( 16.53943276465976808, -0.05219959533910856209, 88.74890960531436690 ) ) ;
#48016=CARTESIAN_POINT ( 'NONE',  ( -15.72974639402176322, -15.80617190586768395, 39.37609039468567573 ) ) ;
#48017=CARTESIAN_POINT ( 'NONE',  ( 5.153800228976335163, 19.02544592524342804, 39.79057627198100988 ) ) ;
#48018=CARTESIAN_POINT ( 'NONE',  ( 5.823673210054125526, 21.52544592524343514, 99.79057627198103830 ) ) ;
#48019=CARTESIAN_POINT ( 'NONE',  ( -4.483927247898539470, -16.52544592524342804, 87.29057627198103830 ) ) ;
#48021=CARTESIAN_POINT ( 'NONE',  ( 9.474510206698971260, -16.51473224551069308, 42.91557627198103120 ) ) ;
#48022=CARTESIAN_POINT ( 'NONE',  ( 19.49190055781009079, 5.500000000000041744, 48.06116087098784817 ) ) ;
#48023=CARTESIAN_POINT ( 'NONE',  ( -5.049401038297874678, -19.05341960407617918, 99.79275706135234714 ) ) ;
#48024=CARTESIAN_POINT ( 'NONE',  ( 19.03943276465977164, -0.05219959533909143690, 103.7489096053143669 ) ) ;
#48025=CARTESIAN_POINT ( 'NONE',  ( -21.52544592524334988, -5.823673210054445271, 33.95942372801901143 ) ) ;
#48026=CARTESIAN_POINT ( 'NONE',  ( 19.03943276465977164, -0.05219959533909143690, 78.74890960531436690 ) ) ;
#48027=CARTESIAN_POINT ( 'NONE',  ( 16.51473224551083163, -9.474510206698727899, 70.83442372801900433 ) ) ;
#48028=CARTESIAN_POINT ( 'NONE',  ( 9.474510206698971260, -16.51473224551069308, 47.91557627198102409 ) ) ;
#48029=CARTESIAN_POINT ( 'NONE',  ( -8.224510206698948167, 14.34966873604960824, 75.41557627198102409 ) ) ;
#48030=CARTESIAN_POINT ( 'NONE',  ( -12.14591786802309592, -12.06949235617757132, 66.87390960531436690 ) ) ;
#48031=CARTESIAN_POINT ( 'NONE',  ( -5.153800228976328057, -19.02544592524343514, 77.29057627198099567 ) ) ;
#48032=CARTESIAN_POINT ( 'NONE',  ( 18.62759615963271287, -10.81492255796078972, 103.3322429386476955 ) ) ;
#48033=CARTESIAN_POINT ( 'NONE',  ( -9.474510206698964154, 16.51473224551069663, 70.41557627198102409 ) ) ;
#48034=EDGE_CURVE ( 'NONE', #95422, #115310, #189981, .T. ) ;
#48035=CARTESIAN_POINT ( 'NONE',  ( -15.80617190586768217, 15.72974639402176855, 113.1260903946856899 ) ) ;
#48036=CARTESIAN_POINT ( 'NONE',  ( 5.049401038298161559, -19.05341960407611168, 37.70724293864768839 ) ) ;
#48037=CARTESIAN_POINT ( 'NONE',  ( 12.14591786802327356, -12.06949235617739191, 105.6260903946856899 ) ) ;
#48038=CARTESIAN_POINT ( 'NONE',  ( 4.483927247898545687, 16.52544592524342804, 114.7905762719810383 ) ) ;
#48039=CARTESIAN_POINT ( 'NONE',  ( 19.05341960407617918, -5.049401038297876454, 101.0427570613523045 ) ) ;
#48041=CARTESIAN_POINT ( 'NONE',  ( 21.55341960407619695, -5.719274019375665929, 31.04275706135234714 ) ) ;
#48042=CARTESIAN_POINT ( 'NONE',  ( 16.51473224551083163, -9.474510206698727899, 60.83442372801900433 ) ) ;
#48043=CARTESIAN_POINT ( 'NONE',  ( 16.53943276465976808, 0.05219959533934440121, 111.2510903946856899 ) ) ;
#48044=CARTESIAN_POINT ( 'NONE',  ( -10.81492255796078084, -18.62759615963271287, 67.08224293864770971 ) ) ;
#48045=CARTESIAN_POINT ( 'NONE',  ( -13.97604488694527625, -13.89961937509977652, 111.8739096053143243 ) ) ;
#48046=CARTESIAN_POINT ( 'NONE',  ( -14.34966873604960291, -8.224510206698953496, 51.66557627198102409 ) ) ;
#48047=CARTESIAN_POINT ( 'NONE',  ( -9.474510206698964154, 16.51473224551069663, 25.41557627198103120 ) ) ;
#48048=CARTESIAN_POINT ( 'NONE',  ( 19.05341960407611168, 5.049401038298154454, 43.95724293864769550 ) ) ;
#48049=CARTESIAN_POINT ( 'NONE',  ( 5.153800228976615827, -19.02544592524334988, 25.20942372801900433 ) ) ;
#48050=CARTESIAN_POINT ( 'NONE',  ( -14.34966873604972548, 8.224510206698743886, 83.33442372801903275 ) ) ;
#48051=CARTESIAN_POINT ( 'NONE',  ( 8.224510206698742110, 14.34966873604972548, 62.08442372801901143 ) ) ;
#48052=CARTESIAN_POINT ( 'NONE',  ( 13.97604488694527802, 13.89961937509977652, 114.3739096053143669 ) ) ;
#48053=CARTESIAN_POINT ( 'NONE',  ( 18.67979575497194134, -10.72451020669871369, 110.8344237280190043 ) ) ;
#48054=CARTESIAN_POINT ( 'NONE',  ( 5.153800228976335163, 19.02544592524342804, 84.79057627198099567 ) ) ;
#48055=CARTESIAN_POINT ( 'NONE',  ( -4.483927247898782831, 16.52544592524335698, 57.70942372801901143 ) ) ;
#48056=CARTESIAN_POINT ( 'NONE',  ( -0.05219959533910754901, -16.53943276465976808, 112.4989096053143669 ) ) ;
#48057=CARTESIAN_POINT ( 'NONE',  ( -16.53943276465976808, -0.05219959533934237506, 108.7510903946857042 ) ) ;
#48059=CARTESIAN_POINT ( 'NONE',  ( -15.80617190586768217, 15.72974639402176855, 73.12609039468567573 ) ) ;
#48060=CARTESIAN_POINT ( 'NONE',  ( 13.89961937509977652, -13.97604488694527269, 98.12390960531433848 ) ) ;
#48061=CARTESIAN_POINT ( 'NONE',  ( -5.153800228976328057, -19.02544592524343514, 72.29057627198102409 ) ) ;
#48062=CARTESIAN_POINT ( 'NONE',  ( -9.564922557960796823, -16.46253265017161027, 107.0822429386476955 ) ) ;
#48063=CARTESIAN_POINT ( 'NONE',  ( 16.53943276465976808, -0.05219959533910856209, 53.74890960531437401 ) ) ;
#48064=CARTESIAN_POINT ( 'NONE',  ( 16.53943276465976808, 0.05219959533934440121, 106.2510903946856757 ) ) ;
#48065=CARTESIAN_POINT ( 'NONE',  ( -14.34966873604960291, -8.224510206698953496, 51.66557627198102409 ) ) ;
#48066=CARTESIAN_POINT ( 'NONE',  ( -14.34966873604972548, 8.224510206698743886, 43.33442372801901143 ) ) ;
#48068=CARTESIAN_POINT ( 'NONE',  ( 0.05219959533936267826, -19.03943276465977164, 35.00109039468566863 ) ) ;
#48069=CARTESIAN_POINT ( 'NONE',  ( -9.564922557960796823, -16.46253265017161027, 72.08224293864770971 ) ) ;
#48070=CARTESIAN_POINT ( 'NONE',  ( -9.474510206698720793, -16.51473224551083518, 54.58442372801899722 ) ) ;
#48071=CARTESIAN_POINT ( 'NONE',  ( 13.89961937509957401, 13.97604488694547697, 56.87609039468564731 ) ) ;
#48072=CARTESIAN_POINT ( 'NONE',  ( -13.97604488694547697, 13.89961937509957934, 103.1260903946856473 ) ) ;
#48073=CARTESIAN_POINT ( 'NONE',  ( 16.55341960407618274, -4.379528057220086978, 86.04275706135236135 ) ) ;
#48074=CARTESIAN_POINT ( 'NONE',  ( -16.51473224551069308, -9.474510206698971260, 31.66557627198102054 ) ) ;
#48075=CARTESIAN_POINT ( 'NONE',  ( 9.474510206698971260, -16.51473224551069308, 102.9155762719810241 ) ) ;
#48076=CARTESIAN_POINT ( 'NONE',  ( 21.55341960407619695, -5.719274019375665929, 41.04275706135236135 ) ) ;
#48077=CARTESIAN_POINT ( 'NONE',  ( 5.049401038297881783, 19.05341960407617563, 87.29275706135234714 ) ) ;
#48079=CARTESIAN_POINT ( 'NONE',  ( -13.89961937509977652, 13.97604488694528158, 55.62390960531434558 ) ) ;
#48080=CARTESIAN_POINT ( 'NONE',  ( 13.89961937509977652, -13.97604488694527269, 98.12390960531433848 ) ) ;
#48081=CARTESIAN_POINT ( 'NONE',  ( -8.224510206698948167, 14.34966873604960824, 60.41557627198102409 ) ) ;
#48082=CARTESIAN_POINT ( 'NONE',  ( 5.049401038298161559, -19.05341960407611168, 47.70724293864770260 ) ) ;
#48083=CARTESIAN_POINT ( 'NONE',  ( -13.89961937509977652, 13.97604488694528158, 65.62390960531436690 ) ) ;
#48084=CARTESIAN_POINT ( 'NONE',  ( -5.153800228976607833, 19.02544592524334988, 67.70942372801900433 ) ) ;
#48085=CARTESIAN_POINT ( 'NONE',  ( -16.46253265017146816, -9.564922557961047289, 49.16775706135233293 ) ) ;
#48086=CARTESIAN_POINT ( 'NONE',  ( 16.51473224551069308, 9.474510206698969483, 84.16557627198102409 ) ) ;
#48087=CARTESIAN_POINT ( 'NONE',  ( -5.719274019375978568, 21.55341960407610458, 75.20724293864769550 ) ) ;
#48088=CARTESIAN_POINT ( 'NONE',  ( -0.05219959533910754901, -16.53943276465976808, 72.49890960531435269 ) ) ;
#48089=CARTESIAN_POINT ( 'NONE',  ( -16.46253265017146816, -9.564922557961047289, 39.16775706135234003 ) ) ;
#48090=CARTESIAN_POINT ( 'NONE',  ( -21.55341960407610458, -5.719274019375992779, 46.45724293864769550 ) ) ;
#48091=CARTESIAN_POINT ( 'NONE',  ( -15.72974639402197994, 15.80617190586746368, 45.62390960531436690 ) ) ;
#48092=CARTESIAN_POINT ( 'NONE',  ( -0.05219959533909027116, -19.03943276465977164, 62.49890960531435979 ) ) ;
#48093=CARTESIAN_POINT ( 'NONE',  ( -9.474510206698964154, 16.51473224551069663, 45.41557627198103120 ) ) ;
#48094=CARTESIAN_POINT ( 'NONE',  ( 8.224510206698953496, -14.34966873604960469, 107.9155762719810241 ) ) ;
#48095=CARTESIAN_POINT ( 'NONE',  ( 5.823673210054444382, -21.52544592524334988, 20.20942372801900788 ) ) ;
#48096=CARTESIAN_POINT ( 'NONE',  ( -9.474510206698964154, 16.51473224551069663, 115.4155762719810241 ) ) ;
#48097=CARTESIAN_POINT ( 'NONE',  ( 5.719274019375673035, 21.55341960407619339, 22.29275706135235069 ) ) ;
#48098=CARTESIAN_POINT ( 'NONE',  ( 19.02544592524343514, -5.153800228976328945, 33.54057627198102409 ) ) ;
#48099=CARTESIAN_POINT ( 'NONE',  ( -15.72974639402197994, 15.80617190586746368, 100.6239096053143811 ) ) ;
#48100=CARTESIAN_POINT ( 'NONE',  ( -16.46253265017146816, -9.564922557961047289, 44.16775706135232582 ) ) ;
#48102=CARTESIAN_POINT ( 'NONE',  ( -5.049401038298153566, 19.05341960407611168, 25.20724293864768484 ) ) ;
#48104=CARTESIAN_POINT ( 'NONE',  ( -12.06949235617739369, -12.14591786802326823, 64.37609039468568994 ) ) ;
#48105=CARTESIAN_POINT ( 'NONE',  ( -19.03943276465977164, 0.05219959533909376836, 31.24890960531435979 ) ) ;
#48107=CARTESIAN_POINT ( 'NONE',  ( 9.474510206698971260, -16.51473224551069308, 77.91557627198103830 ) ) ;
#48108=CARTESIAN_POINT ( 'NONE',  ( -4.379528057220328563, 16.55341960407611168, 110.2072429386477239 ) ) ;
#48109=CARTESIAN_POINT ( 'NONE',  ( 18.62759615963271287, -10.81492255796078972, 48.33224293864770260 ) ) ;
#48110=CARTESIAN_POINT ( 'NONE',  ( 12.06949235617757843, -12.14591786802309237, 83.12390960531436690 ) ) ;
#48111=CARTESIAN_POINT ( 'NONE',  ( -4.483927247898782831, 16.52544592524335698, 27.70942372801901854 ) ) ;
#48112=CARTESIAN_POINT ( 'NONE',  ( -21.55341960407619339, 5.719274019375674811, 83.54275706135234714 ) ) ;
#48113=CARTESIAN_POINT ( 'NONE',  ( 13.89961937509977652, -13.97604488694527269, 23.12390960531436335 ) ) ;
#48114=CARTESIAN_POINT ( 'NONE',  ( -4.379528057220086978, -16.55341960407618274, 109.7927570613523613 ) ) ;
#48115=CARTESIAN_POINT ( 'NONE',  ( -4.379528057220328563, 16.55341960407611168, 60.20724293864768839 ) ) ;
#48116=CARTESIAN_POINT ( 'NONE',  ( -16.51473224551069308, -9.474510206698971260, 51.66557627198102409 ) ) ;
#48117=CARTESIAN_POINT ( 'NONE',  ( -15.80617190586768217, 15.72974639402176855, 93.12609039468568994 ) ) ;
#48118=CARTESIAN_POINT ( 'NONE',  ( 10.81492255796078972, 18.62759615963270932, 114.5822429386477097 ) ) ;
#48119=CARTESIAN_POINT ( 'NONE',  ( 18.62759615963255655, 10.81492255796105972, 71.66775706135234714 ) ) ;
#48120=CARTESIAN_POINT ( 'NONE',  ( 14.29746914071037800, 8.314922557961029526, 36.66775706135234714 ) ) ;
#48121=CARTESIAN_POINT ( 'NONE',  ( -8.314922557960811034, -14.29746914071050412, 72.08224293864769550 ) ) ;
#48122=CARTESIAN_POINT ( 'NONE',  ( 21.52544592524334988, 5.823673210054432836, 91.45942372801901854 ) ) ;
#48123=CARTESIAN_POINT ( 'NONE',  ( 14.29746914071037800, 8.314922557961029526, 111.6677570613523613 ) ) ;
#48124=CARTESIAN_POINT ( 'NONE',  ( 17.72696623605160227, -5.500000000000079048, 61.09811031808416004 ) ) ;
#48125=CARTESIAN_POINT ( 'NONE',  ( -16.55341960407617563, 4.379528057220093196, 38.54275706135234714 ) ) ;
#48126=CARTESIAN_POINT ( 'NONE',  ( -14.29746914071049879, 8.314922557960819915, 45.83224293864769550 ) ) ;
#48127=CARTESIAN_POINT ( 'NONE',  ( -8.314922557961024197, 14.29746914071037800, 87.91775706135234714 ) ) ;
#48128=CARTESIAN_POINT ( 'NONE',  ( -9.564922557960796823, -16.46253265017161027, 102.0822429386477097 ) ) ;
#48129=CARTESIAN_POINT ( 'NONE',  ( -5.049401038298153566, 19.05341960407611168, 100.2072429386476955 ) ) ;
#48130=CARTESIAN_POINT ( 'NONE',  ( -21.53943276465977519, -0.05219959533937600094, 98.75109039468568994 ) ) ;
#48131=CARTESIAN_POINT ( 'NONE',  ( -14.34966873604972548, 8.224510206698743886, 108.3344237280190185 ) ) ;
#48132=CARTESIAN_POINT ( 'NONE',  ( 12.06949235617757843, -12.14591786802309237, 78.12390960531436690 ) ) ;
#48133=CARTESIAN_POINT ( 'NONE',  ( -9.564922557960796823, -16.46253265017161027, 87.08224293864769550 ) ) ;
#48135=CARTESIAN_POINT ( 'NONE',  ( 8.224510206698742110, 14.34966873604972548, 22.08442372801901143 ) ) ;
#48136=CARTESIAN_POINT ( 'NONE',  ( 19.02544592524343514, -5.153800228976328945, 33.54057627198102409 ) ) ;
#48137=CARTESIAN_POINT ( 'NONE',  ( -13.97604488694527625, -13.89961937509977652, 96.87390960531433848 ) ) ;
#48138=CARTESIAN_POINT ( 'NONE',  ( 8.224510206698742110, 14.34966873604972548, 32.08442372801901854 ) ) ;
#48140=CARTESIAN_POINT ( 'NONE',  ( 9.564922557961047289, -16.46253265017146816, 35.41775706135233293 ) ) ;
#48141=CARTESIAN_POINT ( 'NONE',  ( 4.379528057220092307, 16.55341960407617563, 97.29275706135234714 ) ) ;
#48142=CARTESIAN_POINT ( 'NONE',  ( -0.05219959533936034679, 19.03943276465977164, 107.5010903946856615 ) ) ;
#48143=CARTESIAN_POINT ( 'NONE',  ( -5.153800228976328057, -19.02544592524343514, 37.29057627198102409 ) ) ;
#48144=CARTESIAN_POINT ( 'NONE',  ( 16.52544592524335698, 4.483927247898782831, 86.45942372801901854 ) ) ;
#48145=CARTESIAN_POINT ( 'NONE',  ( 16.55341960407618274, -4.379528057220086978, 71.04275706135234714 ) ) ;
#48146=CARTESIAN_POINT ( 'NONE',  ( -19.05341960407611168, -5.049401038298163336, 41.45724293864769550 ) ) ;
#48147=CARTESIAN_POINT ( 'NONE',  ( -9.564922557961040184, 16.46253265017147172, 72.91775706135233293 ) ) ;
#48148=CARTESIAN_POINT ( 'NONE',  ( -5.823673210054431948, 21.52544592524334988, 112.7094237280190328 ) ) ;
#48149=CARTESIAN_POINT ( 'NONE',  ( 9.474510206698971260, -16.51473224551069308, 52.91557627198102409 ) ) ;
#48150=CARTESIAN_POINT ( 'NONE',  ( -19.05341960407611168, -5.049401038298163336, 96.45724293864769550 ) ) ;
#48151=CARTESIAN_POINT ( 'NONE',  ( 14.29746914071049879, -8.314922557960816363, 83.33224293864769550 ) ) ;
#48152=CARTESIAN_POINT ( 'NONE',  ( -9.474510206698720793, -16.51473224551083518, 59.58442372801900433 ) ) ;
#48153=CARTESIAN_POINT ( 'NONE',  ( -15.72974639402197994, 15.80617190586746368, 45.62390960531436690 ) ) ;
#48154=CARTESIAN_POINT ( 'NONE',  ( -16.51473224551082808, 9.474510206698731452, 23.33442372801900078 ) ) ;
#48155=CARTESIAN_POINT ( 'NONE',  ( -0.05219959533909027116, -19.03943276465977164, 87.49890960531436690 ) ) ;
#48156=CARTESIAN_POINT ( 'NONE',  ( -9.474510206698720793, -16.51473224551083518, 19.58442372801899722 ) ) ;
#48157=CARTESIAN_POINT ( 'NONE',  ( 10.81492255796078972, 18.62759615963270932, 64.58224293864769550 ) ) ;
#48158=CARTESIAN_POINT ( 'NONE',  ( 5.049401038298161559, -19.05341960407611168, 112.7072429386476813 ) ) ;
#48159=CARTESIAN_POINT ( 'NONE',  ( -19.03943276465977164, -0.05219959533935918106, 88.75109039468567573 ) ) ;
#48160=CARTESIAN_POINT ( 'NONE',  ( -17.50000000000000000, 3.345213924137382389, 109.5876862309435040 ) ) ;
#48161=CARTESIAN_POINT ( 'NONE',  ( 19.05341960407617918, -5.049401038297876454, 106.0427570613523471 ) ) ;
#48162=CARTESIAN_POINT ( 'NONE',  ( 13.89961937509977652, -13.97604488694527269, 23.12390960531436335 ) ) ;
#48163=CARTESIAN_POINT ( 'NONE',  ( -19.03943276465977164, 0.05219959533909376836, 101.2489096053143669 ) ) ;
#48164=CARTESIAN_POINT ( 'NONE',  ( 18.62759615963271287, -10.81492255796078972, 73.33224293864769550 ) ) ;
#48166=CARTESIAN_POINT ( 'NONE',  ( 4.483927247898790824, -16.52544592524335698, 45.20942372801901854 ) ) ;
#48167=CARTESIAN_POINT ( 'NONE',  ( 21.55341960407619695, -5.719274019375665929, 51.04275706135234714 ) ) ;
#48168=CARTESIAN_POINT ( 'NONE',  ( 21.52544592524334988, 5.823673210054432836, 101.4594237280190185 ) ) ;
#48169=CARTESIAN_POINT ( 'NONE',  ( 12.14591786802327356, -12.06949235617739191, 90.62609039468567573 ) ) ;
#48170=CARTESIAN_POINT ( 'NONE',  ( 19.03943276465977164, -0.05219959533909143690, 93.74890960531435269 ) ) ;
#48171=CARTESIAN_POINT ( 'NONE',  ( 16.53943276465976808, -0.05219959533910856209, 93.74890960531436690 ) ) ;
#48172=CARTESIAN_POINT ( 'NONE',  ( -4.483927247898539470, -16.52544592524342804, 42.29057627198103120 ) ) ;
#48173=CARTESIAN_POINT ( 'NONE',  ( 16.51473224551083163, -9.474510206698727899, 65.83442372801900433 ) ) ;
#48175=CARTESIAN_POINT ( 'NONE',  ( 18.62759615963255655, 10.81492255796105972, 51.66775706135234714 ) ) ;
#48176=CARTESIAN_POINT ( 'NONE',  ( -19.05341960407617563, 5.049401038297882671, 28.54275706135232937 ) ) ;
#48177=CARTESIAN_POINT ( 'NONE',  ( 0.05219959533910956823, 16.53943276465976808, 89.99890960531438111 ) ) ;
#48178=CARTESIAN_POINT ( 'NONE',  ( -18.67979575497178146, -10.72451020669898902, 31.66557627198102054 ) ) ;
#48179=CARTESIAN_POINT ( 'NONE',  ( 14.29746914071049879, -8.314922557960816363, 28.33224293864769550 ) ) ;
#48180=CARTESIAN_POINT ( 'NONE',  ( 15.80617190586769283, -15.72974639402175789, 95.62609039468568994 ) ) ;
#48181=CARTESIAN_POINT ( 'NONE',  ( 16.52544592524335698, 4.483927247898782831, 61.45942372801901854 ) ) ;
#48182=CARTESIAN_POINT ( 'NONE',  ( 8.314922557961029526, -14.29746914071037800, 110.4177570613523756 ) ) ;
#48183=CARTESIAN_POINT ( 'NONE',  ( 21.55341960407619695, -5.719274019375665929, 56.04275706135235424 ) ) ;
#48185=CARTESIAN_POINT ( 'NONE',  ( 21.52544592524334988, 5.823673210054432836, 36.45942372801901143 ) ) ;
#48186=CARTESIAN_POINT ( 'NONE',  ( 16.53943276465976808, -0.05219959533910856209, 98.74890960531438111 ) ) ;
#48187=CARTESIAN_POINT ( 'NONE',  ( -5.049401038298153566, 19.05341960407611168, 30.20724293864768839 ) ) ;
#48188=CARTESIAN_POINT ( 'NONE',  ( -8.224510206698948167, 14.34966873604960824, 65.41557627198102409 ) ) ;
#48189=CARTESIAN_POINT ( 'NONE',  ( -16.46253265017160317, 9.564922557960807481, 75.83224293864769550 ) ) ;
#48190=CARTESIAN_POINT ( 'NONE',  ( 16.53943276465976808, 0.05219959533934440121, 106.2510903946856757 ) ) ;
#48192=CARTESIAN_POINT ( 'NONE',  ( 18.62759615963271287, -10.81492255796078972, 58.33224293864768839 ) ) ;
#48193=CARTESIAN_POINT ( 'NONE',  ( -12.06949235617756955, 12.14591786802309770, 85.62390960531436690 ) ) ;
#48194=CARTESIAN_POINT ( 'NONE',  ( 15.72974639402199770, -15.80617190586745480, 98.12390960531436690 ) ) ;
#48195=CARTESIAN_POINT ( 'NONE',  ( 9.474510206698971260, -16.51473224551069308, 97.91557627198102409 ) ) ;
#48196=CARTESIAN_POINT ( 'NONE',  ( 16.51473224551069308, 9.474510206698969483, 54.16557627198103120 ) ) ;
#48197=CARTESIAN_POINT ( 'NONE',  ( -13.89961937509957401, -13.97604488694547875, 104.3760903946856757 ) ) ;
#48198=CARTESIAN_POINT ( 'NONE',  ( 18.62759615963271287, -10.81492255796078972, 38.33224293864768839 ) ) ;
#48199=CARTESIAN_POINT ( 'NONE',  ( 21.53943276465977519, 0.05219959533937863772, 71.25109039468568994 ) ) ;
#48200=CARTESIAN_POINT ( 'NONE',  ( 16.51473224551069308, 9.474510206698969483, 64.16557627198102409 ) ) ;
#48201=CARTESIAN_POINT ( 'NONE',  ( -19.02544592524342804, 5.153800228976336051, 96.04057627198103830 ) ) ;
#48202=CARTESIAN_POINT ( 'NONE',  ( -16.55341960407617563, 4.379528057220093196, 58.54275706135235424 ) ) ;
#48203=CARTESIAN_POINT ( 'NONE',  ( 21.53943276465977519, 0.05219959533937863772, 41.25109039468568284 ) ) ;
#48204=CARTESIAN_POINT ( 'NONE',  ( 21.55341960407619695, -5.719274019375665929, 86.04275706135236135 ) ) ;
#48205=CARTESIAN_POINT ( 'NONE',  ( 15.80617190586746368, 15.72974639402197994, 104.3739096053143669 ) ) ;
#48206=CARTESIAN_POINT ( 'NONE',  ( 0.05219959533937995610, -21.53943276465977519, 35.00109039468568284 ) ) ;
#48207=CARTESIAN_POINT ( 'NONE',  ( 4.483927247898790824, -16.52544592524335698, 80.20942372801901854 ) ) ;
#48208=CARTESIAN_POINT ( 'NONE',  ( 5.823673210054125526, 21.52544592524343514, 74.79057627198105251 ) ) ;
#48209=CARTESIAN_POINT ( 'NONE',  ( 16.51473224551083163, -9.474510206698727899, 30.83442372801900433 ) ) ;
#48210=CARTESIAN_POINT ( 'NONE',  ( 9.564922557960805705, 16.46253265017160317, 74.58224293864769550 ) ) ;
#48211=CARTESIAN_POINT ( 'NONE',  ( 0.05219959533910956823, 16.53943276465976808, 24.99890960531435624 ) ) ;
#48213=CARTESIAN_POINT ( 'NONE',  ( -9.474510206698964154, 16.51473224551069663, 100.4155762719810241 ) ) ;
#48215=CARTESIAN_POINT ( 'NONE',  ( -16.46253265017146816, -9.564922557961047289, 79.16775706135234714 ) ) ;
#48216=CARTESIAN_POINT ( 'NONE',  ( -5.823673210054116645, -21.52544592524344225, 57.29057627198103120 ) ) ;
#48217=CARTESIAN_POINT ( 'NONE',  ( 16.52544592524342804, -4.483927247898539470, 38.54057627198103120 ) ) ;
#48218=CARTESIAN_POINT ( 'NONE',  ( -12.14591786802326823, 12.06949235617739902, 23.12609039468567573 ) ) ;
#48219=CARTESIAN_POINT ( 'NONE',  ( -9.474510206698964154, 16.51473224551069663, 30.41557627198102054 ) ) ;
#48220=CARTESIAN_POINT ( 'NONE',  ( -16.46253265017146816, -9.564922557961047289, 104.1677570613523329 ) ) ;
#48221=CARTESIAN_POINT ( 'NONE',  ( -21.53943276465977519, 0.05219959533907696930, 96.24890960531435269 ) ) ;
#48222=CARTESIAN_POINT ( 'NONE',  ( 0.05219959533936267826, -19.03943276465977164, 75.00109039468566152 ) ) ;
#48223=CARTESIAN_POINT ( 'NONE',  ( 8.314922557961029526, -14.29746914071037800, 85.41775706135236135 ) ) ;
#48224=CARTESIAN_POINT ( 'NONE',  ( 0.05219959533909260263, 19.03943276465977164, 69.99890960531435269 ) ) ;
#48225=CARTESIAN_POINT ( 'NONE',  ( -14.29746914071049879, 8.314922557960819915, 70.83224293864770971 ) ) ;
#48226=CARTESIAN_POINT ( 'NONE',  ( 5.153800228976335163, 19.02544592524342804, 64.79057627198100988 ) ) ;
#48227=CARTESIAN_POINT ( 'NONE',  ( 16.53943276465976808, -0.05219959533910856209, 63.74890960531435979 ) ) ;
#48230=CARTESIAN_POINT ( 'NONE',  ( -8.224510206698948167, 14.34966873604960824, 35.41557627198102409 ) ) ;
#48231=CARTESIAN_POINT ( 'NONE',  ( -16.46253265017160317, 9.564922557960807481, 75.83224293864769550 ) ) ;
#48233=CARTESIAN_POINT ( 'NONE',  ( 9.564922557961047289, -16.46253265017146816, 45.41775706135232582 ) ) ;
#48234=CARTESIAN_POINT ( 'NONE',  ( -8.314922557961024197, 14.29746914071037800, 62.91775706135236135 ) ) ;
#48235=CARTESIAN_POINT ( 'NONE',  ( 21.53943276465977519, -0.05219959533907433946, 63.74890960531435979 ) ) ;
#48236=CARTESIAN_POINT ( 'NONE',  ( -16.46253265017146816, -9.564922557961047289, 24.16775706135233648 ) ) ;
#48237=CARTESIAN_POINT ( 'NONE',  ( 9.564922557960805705, 16.46253265017160317, 79.58224293864769550 ) ) ;
#48239=CARTESIAN_POINT ( 'NONE',  ( 19.05341960407611168, 5.049401038298154454, 108.9572429386477097 ) ) ;
#48240=CARTESIAN_POINT ( 'NONE',  ( 19.03943276465977164, -0.05219959533909143690, 63.74890960531435979 ) ) ;
#48241=CARTESIAN_POINT ( 'NONE',  ( -10.81492255796105439, 18.62759615963255655, 32.91775706135234714 ) ) ;
#48242=CARTESIAN_POINT ( 'NONE',  ( 12.06949235617757843, -12.14591786802309237, 113.1239096053143953 ) ) ;
#48244=CARTESIAN_POINT ( 'NONE',  ( -18.67979575497178146, -10.72451020669898902, 96.66557627198102409 ) ) ;
#48245=CARTESIAN_POINT ( 'NONE',  ( 16.51473224551069308, 9.474510206698969483, 84.16557627198102409 ) ) ;
#48247=CARTESIAN_POINT ( 'NONE',  ( 15.72974639402176855, 15.80617190586768217, 21.87609039468567573 ) ) ;
#48249=CARTESIAN_POINT ( 'NONE',  ( -16.51473224551069308, -9.474510206698971260, 81.66557627198103830 ) ) ;
#48250=LINE ( 'NONE', #17913, #68957 ) ;
#48251=CARTESIAN_POINT ( 'NONE',  ( -21.52544592524343514, 5.823673210054127303, 96.04057627198102409 ) ) ;
#48252=CARTESIAN_POINT ( 'NONE',  ( -13.89961937509977652, 13.97604488694528158, 40.62390960531435979 ) ) ;
#48253=CARTESIAN_POINT ( 'NONE',  ( 19.05341960407617918, -5.049401038297876454, 101.0427570613523045 ) ) ;
#48255=CARTESIAN_POINT ( 'NONE',  ( -9.474510206698964154, 16.51473224551069663, 25.41557627198103120 ) ) ;
#48256=CARTESIAN_POINT ( 'NONE',  ( -21.52544592524334988, -5.823673210054445271, 88.95942372801901854 ) ) ;
#48257=CARTESIAN_POINT ( 'NONE',  ( -13.97604488694527625, -13.89961937509977652, 81.87390960531436690 ) ) ;
#48258=CARTESIAN_POINT ( 'NONE',  ( 21.55341960407619695, -5.719274019375665929, 41.04275706135236135 ) ) ;
#48260=CARTESIAN_POINT ( 'NONE',  ( 21.52544592524334988, 5.823673210054432836, 26.45942372801901854 ) ) ;
#48262=CARTESIAN_POINT ( 'NONE',  ( 16.46253265017160672, -9.564922557960803928, 88.33224293864769550 ) ) ;
#48263=CARTESIAN_POINT ( 'NONE',  ( 19.25176906914649422, 5.499999999999733546, 63.49927264242280245 ) ) ;
#48264=CARTESIAN_POINT ( 'NONE',  ( -4.483927247898782831, 16.52544592524335698, 42.70942372801901854 ) ) ;
#48265=CARTESIAN_POINT ( 'NONE',  ( -21.53943276465977519, 0.05219959533907696930, 46.24890960531435979 ) ) ;
#48266=CARTESIAN_POINT ( 'NONE',  ( -0.05219959533937732626, 21.53943276465977519, 47.50109039468568994 ) ) ;
#48267=CARTESIAN_POINT ( 'NONE',  ( 15.80617190586769283, -15.72974639402175789, 70.62609039468567573 ) ) ;
#48269=CARTESIAN_POINT ( 'NONE',  ( 9.474510206698729675, 16.51473224551082808, 107.0844237280190043 ) ) ;
#48270=CARTESIAN_POINT ( 'NONE',  ( -16.51473224551069308, -9.474510206698971260, 56.66557627198103120 ) ) ;
#48271=CARTESIAN_POINT ( 'NONE',  ( -13.89961937509977652, 13.97604488694528158, 80.62390960531436690 ) ) ;
#48272=CARTESIAN_POINT ( 'NONE',  ( -8.314922557960811034, -14.29746914071050412, 102.0822429386476955 ) ) ;
#48273=CARTESIAN_POINT ( 'NONE',  ( 4.483927247898545687, 16.52544592524342804, 109.7905762719810383 ) ) ;
#48274=CARTESIAN_POINT ( 'NONE',  ( 0.05219959533909260263, 19.03943276465977164, 114.9989096053143669 ) ) ;
#48275=CARTESIAN_POINT ( 'NONE',  ( -12.14591786802326823, 12.06949235617739902, 78.12609039468570415 ) ) ;
#48276=CARTESIAN_POINT ( 'NONE',  ( -12.14591786802309592, -12.06949235617757132, 71.87390960531438111 ) ) ;
#48277=CARTESIAN_POINT ( 'NONE',  ( 16.46253265017160672, -9.564922557960803928, 53.33224293864768839 ) ) ;
#48278=CARTESIAN_POINT ( 'NONE',  ( 10.81492255796106328, -18.62759615963255655, 80.41775706135234714 ) ) ;
#48279=CARTESIAN_POINT ( 'NONE',  ( 18.67979575497194134, -10.72451020669871369, 65.83442372801900433 ) ) ;
#48280=CARTESIAN_POINT ( 'NONE',  ( 19.05341960407617918, -5.049401038297876454, 101.0427570613523045 ) ) ;
#48281=CARTESIAN_POINT ( 'NONE',  ( -12.14591786802309592, -12.06949235617757132, 66.87390960531436690 ) ) ;
#48282=CARTESIAN_POINT ( 'NONE',  ( 10.72451020669871369, 18.67979575497193778, 22.08442372801901143 ) ) ;
#48283=CARTESIAN_POINT ( 'NONE',  ( -21.52544592524343514, 5.823673210054127303, 61.04057627198103120 ) ) ;
#48284=DIRECTION ( 'NONE',  ( 0.000000000000000000, 0.000000000000000000, -1.000000000000000000 ) ) ;
#48286=CARTESIAN_POINT ( 'NONE',  ( 19.02544592524343514, -5.153800228976328945, 68.54057627198103830 ) ) ;
#48287=CARTESIAN_POINT ( 'NONE',  ( -4.379528057220328563, 16.55341960407611168, 35.20724293864768839 ) ) ;
#48288=CARTESIAN_POINT ( 'NONE',  ( -16.52544592524342804, 4.483927247898546575, 26.04057627198103475 ) ) ;
#48289=CARTESIAN_POINT ( 'NONE',  ( -12.14591786802326823, 12.06949235617739902, 98.12609039468570415 ) ) ;
#48290=CARTESIAN_POINT ( 'NONE',  ( 16.51473224551083163, -9.474510206698727899, 50.83442372801899722 ) ) ;
#48292=CARTESIAN_POINT ( 'NONE',  ( 5.153800228976335163, 19.02544592524342804, 109.7905762719810099 ) ) ;
#48293=CARTESIAN_POINT ( 'NONE',  ( -16.53943276465976808, 0.05219959533911058130, 71.24890960531435269 ) ) ;
#48294=CARTESIAN_POINT ( 'NONE',  ( -19.03943276465977164, -0.05219959533935918106, 48.75109039468566863 ) ) ;
#48295=CARTESIAN_POINT ( 'NONE',  ( 16.61371651742600264, -7.165104196376133494, 101.3541506999299884 ) ) ;
#48296=CARTESIAN_POINT ( 'NONE',  ( 9.474510206698971260, -16.51473224551069308, 112.9155762719810383 ) ) ;
#48297=CARTESIAN_POINT ( 'NONE',  ( -5.823673210054116645, -21.52544592524344225, 57.29057627198103120 ) ) ;
#48298=CARTESIAN_POINT ( 'NONE',  ( -8.224510206698948167, 14.34966873604960824, 100.4155762719810241 ) ) ;
#48299=CARTESIAN_POINT ( 'NONE',  ( 16.55341960407618274, -4.379528057220086978, 46.04275706135234714 ) ) ;
#48300=CARTESIAN_POINT ( 'NONE',  ( -14.34966873604960291, -8.224510206698953496, 91.66557627198103830 ) ) ;
#48301=CARTESIAN_POINT ( 'NONE',  ( 17.26058549869089731, -6.457015423128600773, 36.12254162523932877 ) ) ;
#48302=CARTESIAN_POINT ( 'NONE',  ( -17.12812012977025589, 6.668231424566045007, 48.64051240676857901 ) ) ;
#48303=CARTESIAN_POINT ( 'NONE',  ( -21.53943276465977519, 0.05219959533907696930, 26.24890960531435624 ) ) ;
#48308=CARTESIAN_POINT ( 'NONE',  ( -16.53943276465976808, -0.05219959533934237506, 43.75109039468568284 ) ) ;
#48309=CARTESIAN_POINT ( 'NONE',  ( 4.483927247898545687, 16.52544592524342804, 24.79057627198103120 ) ) ;
#48310=CARTESIAN_POINT ( 'NONE',  ( 15.80617190586746368, 15.72974639402197994, 59.37390960531436690 ) ) ;
#48311=CARTESIAN_POINT ( 'NONE',  ( 9.564922557961047289, -16.46253265017146816, 90.41775706135234714 ) ) ;
#48312=CARTESIAN_POINT ( 'NONE',  ( 18.67979575497178502, 10.72451020669898547, 49.16557627198102409 ) ) ;
#48313=CARTESIAN_POINT ( 'NONE',  ( -21.53943276465977519, -0.05219959533937600094, 78.75109039468568994 ) ) ;
#48315=CARTESIAN_POINT ( 'NONE',  ( 16.53943276465976808, 0.05219959533934440121, 41.25109039468568284 ) ) ;
#48316=CARTESIAN_POINT ( 'NONE',  ( -5.153800228976328057, -19.02544592524343514, 37.29057627198102409 ) ) ;
#48317=CARTESIAN_POINT ( 'NONE',  ( -16.51473224551069308, -9.474510206698971260, 106.6655762719810383 ) ) ;
#48318=CARTESIAN_POINT ( 'NONE',  ( -19.05341960407611168, -5.049401038298163336, 41.45724293864769550 ) ) ;
#48319=CARTESIAN_POINT ( 'NONE',  ( 8.224510206698953496, -14.34966873604960469, 97.91557627198103830 ) ) ;
#48321=CARTESIAN_POINT ( 'NONE',  ( 9.564922557960805705, 16.46253265017160317, 94.58224293864769550 ) ) ;
#48323=CARTESIAN_POINT ( 'NONE',  ( 8.314922557961029526, -14.29746914071037800, 50.41775706135235424 ) ) ;
#48324=CARTESIAN_POINT ( 'NONE',  ( -15.80617190586745835, -15.72974639402198527, 96.87390960531436690 ) ) ;
#48325=CARTESIAN_POINT ( 'NONE',  ( -0.05219959533909027116, -19.03943276465977164, 42.49890960531435269 ) ) ;
#48326=CARTESIAN_POINT ( 'NONE',  ( -5.823673210054431948, 21.52544592524334988, 27.70942372801901854 ) ) ;
#48327=CARTESIAN_POINT ( 'NONE',  ( -16.51473224551069308, -9.474510206698971260, 81.66557627198103830 ) ) ;
#48328=CARTESIAN_POINT ( 'NONE',  ( -9.474510206698964154, 16.51473224551069663, 115.4155762719810241 ) ) ;
#48330=CARTESIAN_POINT ( 'NONE',  ( 12.06949235617739724, 12.14591786802326823, 41.87609039468568284 ) ) ;
#48331=CARTESIAN_POINT ( 'NONE',  ( 18.62759615963255655, 10.81492255796105972, 21.66775706135235069 ) ) ;
#48332=CARTESIAN_POINT ( 'NONE',  ( -16.53943276465976808, 0.05219959533911058130, 116.2489096053143669 ) ) ;
#48333=CARTESIAN_POINT ( 'NONE',  ( -9.474510206698964154, 16.51473224551069663, 90.41557627198103830 ) ) ;
#48334=CARTESIAN_POINT ( 'NONE',  ( -5.049401038297874678, -19.05341960407617918, 69.79275706135233293 ) ) ;
#48335=CARTESIAN_POINT ( 'NONE',  ( -5.049401038297874678, -19.05341960407617918, 29.79275706135232227 ) ) ;
#48336=CARTESIAN_POINT ( 'NONE',  ( -21.52544592524343514, 5.823673210054127303, 91.04057627198103830 ) ) ;
#48337=CARTESIAN_POINT ( 'NONE',  ( -19.03943276465977164, -0.05219959533935918106, 33.75109039468566863 ) ) ;
#48338=CARTESIAN_POINT ( 'NONE',  ( 4.379528057220092307, 16.55341960407617563, 72.29275706135236135 ) ) ;
#48339=CARTESIAN_POINT ( 'NONE',  ( -16.51473224551069308, -9.474510206698971260, 111.6655762719810383 ) ) ;
#48340=CARTESIAN_POINT ( 'NONE',  ( -9.564922557960796823, -16.46253265017161027, 62.08224293864769550 ) ) ;
#48342=CARTESIAN_POINT ( 'NONE',  ( -5.823673210054431948, 21.52544592524334988, 67.70942372801901854 ) ) ;
#48343=CARTESIAN_POINT ( 'NONE',  ( 10.72451020669871369, 18.67979575497193778, 62.08442372801901143 ) ) ;
#48344=CARTESIAN_POINT ( 'NONE',  ( -9.474510206698964154, 16.51473224551069663, 80.41557627198103830 ) ) ;
#48345=CARTESIAN_POINT ( 'NONE',  ( 15.80617190586769283, -15.72974639402175789, 45.62609039468567573 ) ) ;
#48346=CARTESIAN_POINT ( 'NONE',  ( 19.02544592524334988, 5.153800228976608722, 81.45942372801897591 ) ) ;
#48347=CARTESIAN_POINT ( 'NONE',  ( -19.02544592524342804, 5.153800228976336051, 51.04057627198103120 ) ) ;
#48348=CARTESIAN_POINT ( 'NONE',  ( 9.564922557960805705, 16.46253265017160317, 99.58224293864770971 ) ) ;
#48349=CARTESIAN_POINT ( 'NONE',  ( -13.89961937509977652, 13.97604488694528158, 65.62390960531436690 ) ) ;
#48350=CARTESIAN_POINT ( 'NONE',  ( 19.05341960407611168, 5.049401038298154454, 108.9572429386477097 ) ) ;
#48351=CARTESIAN_POINT ( 'NONE',  ( 19.05341960407611168, 5.049401038298154454, 53.95724293864770260 ) ) ;
#48352=CARTESIAN_POINT ( 'NONE',  ( -5.719274019375978568, 21.55341960407610458, 100.2072429386476955 ) ) ;
#48353=CARTESIAN_POINT ( 'NONE',  ( -0.05219959533934338120, 16.53943276465976808, 72.50109039468568994 ) ) ;
#48355=CARTESIAN_POINT ( 'NONE',  ( -19.05341960407617563, 5.049401038297882671, 28.54275706135232937 ) ) ;
#48356=CARTESIAN_POINT ( 'NONE',  ( 13.89961937509977652, -13.97604488694527269, 68.12390960531436690 ) ) ;
#48357=CARTESIAN_POINT ( 'NONE',  ( 8.314922557960818139, 14.29746914071049879, 64.58224293864769550 ) ) ;
#48358=CARTESIAN_POINT ( 'NONE',  ( 16.55341960407611168, 4.379528057220329451, 93.95724293864770971 ) ) ;
#48359=CARTESIAN_POINT ( 'NONE',  ( -16.51473224551069308, -9.474510206698971260, 101.6655762719810241 ) ) ;
#48360=CARTESIAN_POINT ( 'NONE',  ( 5.153800228976335163, 19.02544592524342804, 94.79057627198103830 ) ) ;
#48361=CARTESIAN_POINT ( 'NONE',  ( -21.52544592524334988, -5.823673210054445271, 48.95942372801902565 ) ) ;
#48362=CARTESIAN_POINT ( 'NONE',  ( 16.46253265017160672, -9.564922557960803928, 108.3322429386476955 ) ) ;
#48363=CARTESIAN_POINT ( 'NONE',  ( 13.89961937509957401, 13.97604488694547697, 21.87609039468566152 ) ) ;
#48364=CARTESIAN_POINT ( 'NONE',  ( -16.53943276465976808, -0.05219959533934237506, 78.75109039468568994 ) ) ;
#48365=CARTESIAN_POINT ( 'NONE',  ( -21.53943276465977519, -0.05219959533937600094, 43.75109039468568284 ) ) ;
#48366=CARTESIAN_POINT ( 'NONE',  ( -0.05219959533907301413, -21.53943276465977519, 37.49890960531436690 ) ) ;
#48367=CARTESIAN_POINT ( 'NONE',  ( -5.719274019375978568, 21.55341960407610458, 105.2072429386477097 ) ) ;
#48368=CARTESIAN_POINT ( 'NONE',  ( 16.53943276465976808, -0.05219959533910856209, 63.74890960531435979 ) ) ;
#48369=CARTESIAN_POINT ( 'NONE',  ( -16.46253265017160317, 9.564922557960807481, 55.83224293864769550 ) ) ;
#48370=CARTESIAN_POINT ( 'NONE',  ( -4.483927247898539470, -16.52544592524342804, 82.29057627198103830 ) ) ;
#48371=CARTESIAN_POINT ( 'NONE',  ( 5.719274019375991003, -21.55341960407610458, 47.70724293864770260 ) ) ;
#48372=CARTESIAN_POINT ( 'NONE',  ( 16.46253265017146816, 9.564922557961045513, 46.66775706135233293 ) ) ;
#48373=CARTESIAN_POINT ( 'NONE',  ( -19.05341960407611168, -5.049401038298163336, 21.45724293864768839 ) ) ;
#48375=CARTESIAN_POINT ( 'NONE',  ( -0.05219959533934338120, 16.53943276465976808, 62.50109039468568284 ) ) ;
#48376=CARTESIAN_POINT ( 'NONE',  ( -19.03943276465977164, 0.05219959533909376836, 71.24890960531435269 ) ) ;
#48378=CARTESIAN_POINT ( 'NONE',  ( 8.224510206698953496, -14.34966873604960469, 87.91557627198103830 ) ) ;
#48379=CARTESIAN_POINT ( 'NONE',  ( 21.52544592524344225, -5.823673210054117533, 33.54057627198102409 ) ) ;
#48380=CARTESIAN_POINT ( 'NONE',  ( 16.55341960407618274, -4.379528057220086978, 111.0427570613523613 ) ) ;
#48381=CARTESIAN_POINT ( 'NONE',  ( 14.29746914071037800, 8.314922557961029526, 21.66775706135235069 ) ) ;
#48382=CARTESIAN_POINT ( 'NONE',  ( 5.823673210054444382, -21.52544592524334988, 95.20942372801903275 ) ) ;
#48383=CARTESIAN_POINT ( 'NONE',  ( -9.564922557960796823, -16.46253265017161027, 92.08224293864769550 ) ) ;
#48384=CARTESIAN_POINT ( 'NONE',  ( 21.53943276465977519, -0.05219959533907433946, 113.7489096053143527 ) ) ;
#48385=CARTESIAN_POINT ( 'NONE',  ( 14.29746914071037800, 8.314922557961029526, 61.66775706135235424 ) ) ;
#48386=CARTESIAN_POINT ( 'NONE',  ( 13.97604488694527802, 13.89961937509977652, 34.37390960531436690 ) ) ;
#48387=CARTESIAN_POINT ( 'NONE',  ( -16.53943276465976808, -0.05219959533934237506, 28.75109039468567929 ) ) ;
#48388=CARTESIAN_POINT ( 'NONE',  ( 19.03943276465977164, 0.05219959533936151252, 101.2510903946856757 ) ) ;
#48389=CARTESIAN_POINT ( 'NONE',  ( -15.80617190586745835, -15.72974639402198527, 96.87390960531436690 ) ) ;
#48390=CARTESIAN_POINT ( 'NONE',  ( -9.474510206698720793, -16.51473224551083518, 64.58442372801900433 ) ) ;
#48391=CARTESIAN_POINT ( 'NONE',  ( 18.22780087662122384, -5.500000000000022204, 86.01540105326108687 ) ) ;
#48392=CARTESIAN_POINT ( 'NONE',  ( 21.55341960407610458, 5.719274019375980345, 113.9572429386477239 ) ) ;
#48394=CARTESIAN_POINT ( 'NONE',  ( 19.05341960407611168, 5.049401038298154454, 78.95724293864769550 ) ) ;
#48395=CARTESIAN_POINT ( 'NONE',  ( 14.29746914071037800, 8.314922557961029526, 26.66775706135235424 ) ) ;
#48397=CARTESIAN_POINT ( 'NONE',  ( -9.564922557961040184, 16.46253265017147172, 62.91775706135233293 ) ) ;
#48398=CARTESIAN_POINT ( 'NONE',  ( -5.823673210054116645, -21.52544592524344225, 112.2905762719810241 ) ) ;
#48399=CARTESIAN_POINT ( 'NONE',  ( 8.224510206698953496, -14.34966873604960469, 77.91557627198102409 ) ) ;
#48400=CARTESIAN_POINT ( 'NONE',  ( 13.89961937509977652, -13.97604488694527269, 78.12390960531433848 ) ) ;
#48401=CARTESIAN_POINT ( 'NONE',  ( 14.29746914071037800, 8.314922557961029526, 41.66775706135235424 ) ) ;
#48402=CARTESIAN_POINT ( 'NONE',  ( 19.03943276465977164, 0.05219959533936151252, 36.25109039468567573 ) ) ;
#48403=CARTESIAN_POINT ( 'NONE',  ( -10.81492255796105439, 18.62759615963255655, 57.91775706135234714 ) ) ;
#48404=CARTESIAN_POINT ( 'NONE',  ( -19.02544592524334988, -5.153800228976617603, 108.9594237280189759 ) ) ;
#48405=CARTESIAN_POINT ( 'NONE',  ( -19.03943276465977164, 0.05219959533909376836, 56.24890960531435979 ) ) ;
#48407=CARTESIAN_POINT ( 'NONE',  ( 5.153800228976615827, -19.02544592524334988, 80.20942372801901854 ) ) ;
#48408=CARTESIAN_POINT ( 'NONE',  ( 4.483927247898790824, -16.52544592524335698, 55.20942372801902565 ) ) ;
#48409=CARTESIAN_POINT ( 'NONE',  ( 0.05219959533937995610, -21.53943276465977519, 100.0010903946857042 ) ) ;
#48410=CARTESIAN_POINT ( 'NONE',  ( -16.51473224551082808, 9.474510206698731452, 68.33442372801900433 ) ) ;
#48411=CARTESIAN_POINT ( 'NONE',  ( -5.049401038298153566, 19.05341960407611168, 45.20724293864769550 ) ) ;
#48412=CARTESIAN_POINT ( 'NONE',  ( -5.719274019375978568, 21.55341960407610458, 65.20724293864768129 ) ) ;
#48413=CARTESIAN_POINT ( 'NONE',  ( 14.29746914071049879, -8.314922557960816363, 63.33224293864770260 ) ) ;
#48414=CARTESIAN_POINT ( 'NONE',  ( 19.05341960407617918, -5.049401038297876454, 71.04275706135234714 ) ) ;
#48416=CARTESIAN_POINT ( 'NONE',  ( -19.05341960407617563, 5.049401038297882671, 38.54275706135233293 ) ) ;
#48417=CARTESIAN_POINT ( 'NONE',  ( -16.52544592524335698, -4.483927247898792601, 93.95942372801903275 ) ) ;
#48418=CARTESIAN_POINT ( 'NONE',  ( 8.224510206698953496, -14.34966873604960469, 52.91557627198103830 ) ) ;
#48419=CARTESIAN_POINT ( 'NONE',  ( 15.72974639402176855, 15.80617190586768217, 86.87609039468568994 ) ) ;
#48421=CARTESIAN_POINT ( 'NONE',  ( 21.55341960407610458, 5.719274019375980345, 98.95724293864770971 ) ) ;
#48422=CARTESIAN_POINT ( 'NONE',  ( 5.153800228976335163, 19.02544592524342804, 54.79057627198103120 ) ) ;
#48423=CARTESIAN_POINT ( 'NONE',  ( 10.72451020669871369, 18.67979575497193778, 67.08442372801901854 ) ) ;
#48424=CARTESIAN_POINT ( 'NONE',  ( 19.03943276465977164, -0.05219959533909143690, 43.74890960531435979 ) ) ;
#48426=CARTESIAN_POINT ( 'NONE',  ( -19.02544592524342804, 5.153800228976336051, 66.04057627198103830 ) ) ;
#48427=CARTESIAN_POINT ( 'NONE',  ( -16.51473224551069308, -9.474510206698971260, 21.66557627198102765 ) ) ;
#48428=CARTESIAN_POINT ( 'NONE',  ( -19.03943276465977164, 0.05219959533909376836, 106.2489096053143669 ) ) ;
#48429=CARTESIAN_POINT ( 'NONE',  ( 4.379528057220339221, -16.55341960407611168, 57.70724293864770260 ) ) ;
#48430=CARTESIAN_POINT ( 'NONE',  ( 16.51473224551069308, 9.474510206698969483, 34.16557627198102409 ) ) ;
#48431=CARTESIAN_POINT ( 'NONE',  ( -8.224510206698948167, 14.34966873604960824, 80.41557627198103830 ) ) ;
#48432=CARTESIAN_POINT ( 'NONE',  ( 18.67979575497178502, 10.72451020669898547, 94.16557627198103830 ) ) ;
#48433=CARTESIAN_POINT ( 'NONE',  ( 15.80617190586769283, -15.72974639402175789, 30.62609039468567929 ) ) ;
#48434=CARTESIAN_POINT ( 'NONE',  ( -5.153800228976328057, -19.02544592524343514, 22.29057627198102765 ) ) ;
#48435=CARTESIAN_POINT ( 'NONE',  ( -8.224510206698735004, -14.34966873604973081, 49.58442372801901143 ) ) ;
#48436=CARTESIAN_POINT ( 'NONE',  ( 5.719274019375991003, -21.55341960407610458, 77.70724293864770971 ) ) ;
#48437=CARTESIAN_POINT ( 'NONE',  ( 10.81492255796106328, -18.62759615963255655, 105.4177570613523613 ) ) ;
#48438=CARTESIAN_POINT ( 'NONE',  ( 9.564922557960805705, 16.46253265017160317, 104.5822429386476955 ) ) ;
#48439=CARTESIAN_POINT ( 'NONE',  ( -5.823673210054431948, 21.52544592524334988, 47.70942372801902565 ) ) ;
#48440=CARTESIAN_POINT ( 'NONE',  ( 15.80617190586746368, 15.72974639402197994, 39.37390960531436690 ) ) ;
#48441=CARTESIAN_POINT ( 'NONE',  ( -4.483927247898782831, 16.52544592524335698, 97.70942372801904696 ) ) ;
#48442=CARTESIAN_POINT ( 'NONE',  ( -21.53943276465977519, -0.05219959533937600094, 58.75109039468568994 ) ) ;
#48443=CARTESIAN_POINT ( 'NONE',  ( 10.72451020669871369, 18.67979575497193778, 87.08442372801901854 ) ) ;
#48444=CARTESIAN_POINT ( 'NONE',  ( 9.564922557961047289, -16.46253265017146816, 35.41775706135233293 ) ) ;
#48445=CARTESIAN_POINT ( 'NONE',  ( 0.05219959533934541429, -16.53943276465976808, 85.00109039468568994 ) ) ;
#48446=CARTESIAN_POINT ( 'NONE',  ( -21.53943276465977519, -0.05219959533937600094, 38.75109039468567573 ) ) ;
#48447=CARTESIAN_POINT ( 'NONE',  ( -16.46253265017160317, 9.564922557960807481, 45.83224293864769550 ) ) ;
#48448=CARTESIAN_POINT ( 'NONE',  ( 21.55341960407619695, -5.719274019375665929, 111.0427570613523613 ) ) ;
#48449=CARTESIAN_POINT ( 'NONE',  ( -19.03943276465977164, 0.05219959533909376836, 116.2489096053143669 ) ) ;
#48450=CARTESIAN_POINT ( 'NONE',  ( -5.719274019375665041, -21.55341960407619695, 24.79275706135235779 ) ) ;
#48451=CIRCLE ( 'NONE', #138775, 2.500000000000002220 ) ;
#48452=CARTESIAN_POINT ( 'NONE',  ( -10.81492255796078084, -18.62759615963271287, 77.08224293864769550 ) ) ;
#48454=CARTESIAN_POINT ( 'NONE',  ( -15.80617190586745835, -15.72974639402198527, 81.87390960531435269 ) ) ;
#48455=CARTESIAN_POINT ( 'NONE',  ( 4.483927247898790824, -16.52544592524335698, 60.20942372801902565 ) ) ;
#48456=CARTESIAN_POINT ( 'NONE',  ( -8.224510206698948167, 14.34966873604960824, 65.41557627198102409 ) ) ;
#48458=CARTESIAN_POINT ( 'NONE',  ( 9.564922557961047289, -16.46253265017146816, 90.41775706135234714 ) ) ;
#48460=CARTESIAN_POINT ( 'NONE',  ( 8.314922557961029526, -14.29746914071037800, 40.41775706135234714 ) ) ;
#48461=CARTESIAN_POINT ( 'NONE',  ( 15.72974639402199770, -15.80617190586745480, 93.12390960531436690 ) ) ;
#48462=CARTESIAN_POINT ( 'NONE',  ( -10.81492255796078084, -18.62759615963271287, 77.08224293864769550 ) ) ;
#48463=CARTESIAN_POINT ( 'NONE',  ( 15.80617190586746368, 15.72974639402197994, 24.37390960531435979 ) ) ;
#48464=CARTESIAN_POINT ( 'NONE',  ( 16.53943276465976808, 0.05219959533934440121, 56.25109039468568284 ) ) ;
#48465=CARTESIAN_POINT ( 'NONE',  ( -16.51473224551069308, -9.474510206698971260, 76.66557627198103830 ) ) ;
#48466=CARTESIAN_POINT ( 'NONE',  ( -15.72974639402176322, -15.80617190586768395, 39.37609039468567573 ) ) ;
#48467=CARTESIAN_POINT ( 'NONE',  ( -0.05219959533936034679, 19.03943276465977164, 107.5010903946856615 ) ) ;
#48468=CARTESIAN_POINT ( 'NONE',  ( 19.03943276465977164, -0.05219959533909143690, 113.7489096053143669 ) ) ;
#48469=CARTESIAN_POINT ( 'NONE',  ( 19.02544592524334988, 5.153800228976608722, 31.45942372801900433 ) ) ;
#48470=CARTESIAN_POINT ( 'NONE',  ( -16.52544592524335698, -4.483927247898792601, 38.95942372801901854 ) ) ;
#48471=CARTESIAN_POINT ( 'NONE',  ( 5.049401038298161559, -19.05341960407611168, 97.70724293864766707 ) ) ;
#48472=CARTESIAN_POINT ( 'NONE',  ( 5.823673210054125526, 21.52544592524343514, 99.79057627198103830 ) ) ;
#48473=CARTESIAN_POINT ( 'NONE',  ( 16.46253265017160672, -9.564922557960803928, 58.33224293864769550 ) ) ;
#48475=CARTESIAN_POINT ( 'NONE',  ( -8.314922557960811034, -14.29746914071050412, 77.08224293864769550 ) ) ;
#48476=CARTESIAN_POINT ( 'NONE',  ( 13.97604488694527802, 13.89961937509977652, 114.3739096053143669 ) ) ;
#48477=CARTESIAN_POINT ( 'NONE',  ( 19.05341960407611168, 5.049401038298154454, 23.95724293864769194 ) ) ;
#48478=CARTESIAN_POINT ( 'NONE',  ( 5.719274019375991003, -21.55341960407610458, 97.70724293864772392 ) ) ;
#48479=CARTESIAN_POINT ( 'NONE',  ( 9.474510206698729675, 16.51473224551082808, 57.08442372801900433 ) ) ;
#48480=CARTESIAN_POINT ( 'NONE',  ( 16.51473224551069308, 9.474510206698969483, 114.1655762719810241 ) ) ;
#48481=CARTESIAN_POINT ( 'NONE',  ( 19.05341960407611168, 5.049401038298154454, 28.95724293864769550 ) ) ;
#48482=CARTESIAN_POINT ( 'NONE',  ( 18.62759615963271287, -10.81492255796078972, 53.33224293864769550 ) ) ;
#48484=CARTESIAN_POINT ( 'NONE',  ( 19.05341960407611168, 5.049401038298154454, 98.95724293864766707 ) ) ;
#48485=CARTESIAN_POINT ( 'NONE',  ( -18.62759615963255300, -10.81492255796106328, 74.16775706135231871 ) ) ;
#48486=CARTESIAN_POINT ( 'NONE',  ( -5.153800228976328057, -19.02544592524343514, 47.29057627198102409 ) ) ;
#48488=CARTESIAN_POINT ( 'NONE',  ( -0.05219959533910754901, -16.53943276465976808, 87.49890960531436690 ) ) ;
#48489=CARTESIAN_POINT ( 'NONE',  ( 16.52544592524335698, 4.483927247898782831, 31.45942372801901854 ) ) ;
#48490=CARTESIAN_POINT ( 'NONE',  ( -18.62759615963255300, -10.81492255796106328, 64.16775706135234714 ) ) ;
#48491=ORIENTED_EDGE ( 'NONE', *, *, #10333, .T. ) ;
#48492=CARTESIAN_POINT ( 'NONE',  ( -13.89961937509957401, -13.97604488694547875, 24.37609039468565442 ) ) ;
#48493=CARTESIAN_POINT ( 'NONE',  ( 19.02544592524334988, 5.153800228976608722, 81.45942372801897591 ) ) ;
#48494=CARTESIAN_POINT ( 'NONE',  ( 19.02544592524334988, 5.153800228976608722, 41.45942372801900433 ) ) ;
#48496=CARTESIAN_POINT ( 'NONE',  ( -5.823673210054431948, 21.52544592524334988, 37.70942372801900433 ) ) ;
#48497=CARTESIAN_POINT ( 'NONE',  ( 17.59860650958989936, 7.585241751807028088, 54.07662985737508876 ) ) ;
#48498=CARTESIAN_POINT ( 'NONE',  ( -13.89961937509957401, -13.97604488694547875, 39.37609039468566152 ) ) ;
#48499=CARTESIAN_POINT ( 'NONE',  ( 13.89961937509977652, -13.97604488694527269, 63.12390960531435979 ) ) ;
#48500=CARTESIAN_POINT ( 'NONE',  ( 4.379528057220339221, -16.55341960407611168, 27.70724293864769905 ) ) ;
#48501=CARTESIAN_POINT ( 'NONE',  ( -5.719274019375978568, 21.55341960407610458, 25.20724293864769550 ) ) ;
#48502=CARTESIAN_POINT ( 'NONE',  ( 15.72974639402176855, 15.80617190586768217, 91.87609039468568994 ) ) ;
#48505=CARTESIAN_POINT ( 'NONE',  ( 18.67979575497194134, -10.72451020669871369, 85.83442372801901854 ) ) ;
#48507=CARTESIAN_POINT ( 'NONE',  ( 16.46253265017160672, -9.564922557960803928, 103.3322429386476955 ) ) ;
#48509=CARTESIAN_POINT ( 'NONE',  ( -16.51473224551069308, -9.474510206698971260, 56.66557627198103120 ) ) ;
#48510=CARTESIAN_POINT ( 'NONE',  ( 21.53943276465977519, -0.05219959533907433946, 63.74890960531435979 ) ) ;
#48511=CARTESIAN_POINT ( 'NONE',  ( -16.52544592524342804, 4.483927247898546575, 31.04057627198102409 ) ) ;
#48512=CARTESIAN_POINT ( 'NONE',  ( -16.55341960407611168, -4.379528057220339221, 111.4572429386476813 ) ) ;
#48513=CARTESIAN_POINT ( 'NONE',  ( -5.153800228976328057, -19.02544592524343514, 97.29057627198099567 ) ) ;
#48514=CARTESIAN_POINT ( 'NONE',  ( -16.51473224551082808, 9.474510206698731452, 28.33442372801900433 ) ) ;
#48515=CARTESIAN_POINT ( 'NONE',  ( -12.06949235617756955, 12.14591786802309770, 100.6239096053143811 ) ) ;
#48516=CARTESIAN_POINT ( 'NONE',  ( 21.52544592524334988, 5.823673210054432836, 71.45942372801901854 ) ) ;
#48517=CARTESIAN_POINT ( 'NONE',  ( 16.46253265017160672, -9.564922557960803928, 98.33224293864769550 ) ) ;
#48518=CARTESIAN_POINT ( 'NONE',  ( -12.14591786802326823, 12.06949235617739902, 113.1260903946856899 ) ) ;
#48519=CARTESIAN_POINT ( 'NONE',  ( 19.05341960407617918, -5.049401038297876454, 61.04275706135232582 ) ) ;
#48521=CARTESIAN_POINT ( 'NONE',  ( 5.049401038298161559, -19.05341960407611168, 107.7072429386476955 ) ) ;
#48522=CARTESIAN_POINT ( 'NONE',  ( -16.52544592524342804, 4.483927247898546575, 71.04057627198103830 ) ) ;
#48523=CARTESIAN_POINT ( 'NONE',  ( -19.02544592524334988, -5.153800228976617603, 58.95942372801900433 ) ) ;
#48524=CARTESIAN_POINT ( 'NONE',  ( 13.89961937509977652, -13.97604488694527269, 58.12390960531436690 ) ) ;
#48525=CARTESIAN_POINT ( 'NONE',  ( -0.05219959533910754901, -16.53943276465976808, 62.49890960531436690 ) ) ;
#48526=CARTESIAN_POINT ( 'NONE',  ( -9.564922557961040184, 16.46253265017147172, 87.91775706135233293 ) ) ;
#48527=CARTESIAN_POINT ( 'NONE',  ( -18.62759615963270932, 10.81492255796079327, 45.83224293864769550 ) ) ;
#48529=CARTESIAN_POINT ( 'NONE',  ( 5.049401038298161559, -19.05341960407611168, 22.70724293864769194 ) ) ;
#48530=CARTESIAN_POINT ( 'NONE',  ( -16.20579543436681647, -7.371946100354982434, 30.56520834171878320 ) ) ;
#48531=CARTESIAN_POINT ( 'NONE',  ( 5.153800228976335163, 19.02544592524342804, 69.79057627198103830 ) ) ;
#48532=CARTESIAN_POINT ( 'NONE',  ( -21.55341960407610458, -5.719274019375992779, 61.45724293864770260 ) ) ;
#48533=CARTESIAN_POINT ( 'NONE',  ( 4.483927247898790824, -16.52544592524335698, 90.20942372801903275 ) ) ;
#48534=CARTESIAN_POINT ( 'NONE',  ( 19.05341960407611168, 5.049401038298154454, 73.95724293864768129 ) ) ;
#48535=CARTESIAN_POINT ( 'NONE',  ( -0.05219959533936034679, 19.03943276465977164, 52.50109039468566863 ) ) ;
#48536=CARTESIAN_POINT ( 'NONE',  ( -5.719274019375665041, -21.55341960407619695, 84.79275706135234714 ) ) ;
#48537=CARTESIAN_POINT ( 'NONE',  ( -15.80617190586745835, -15.72974639402198527, 61.87390960531436690 ) ) ;
#48538=CARTESIAN_POINT ( 'NONE',  ( 0.05219959533909260263, 19.03943276465977164, 104.9989096053143669 ) ) ;
#48539=CARTESIAN_POINT ( 'NONE',  ( -13.89961937509977652, 13.97604488694528158, 35.62390960531435269 ) ) ;
#48540=CARTESIAN_POINT ( 'NONE',  ( 8.314922557961029526, -14.29746914071037800, 105.4177570613523613 ) ) ;
#48541=CARTESIAN_POINT ( 'NONE',  ( -19.03943276465977164, -0.05219959533935918106, 113.7510903946856757 ) ) ;
#48542=CARTESIAN_POINT ( 'NONE',  ( 19.25176906914651553, 5.499999999999744205, 78.49927264242278113 ) ) ;
#48543=CARTESIAN_POINT ( 'NONE',  ( 15.80617190586769283, -15.72974639402175789, 90.62609039468567573 ) ) ;
#48544=CARTESIAN_POINT ( 'NONE',  ( -8.224510206698948167, 14.34966873604960824, 60.41557627198102409 ) ) ;
#48545=CARTESIAN_POINT ( 'NONE',  ( 12.06949235617757843, -12.14591786802309237, 68.12390960531436690 ) ) ;
#48546=CARTESIAN_POINT ( 'NONE',  ( 15.80617190586746368, 15.72974639402197994, 89.37390960531435269 ) ) ;
#48547=CARTESIAN_POINT ( 'NONE',  ( -10.72451020669898014, 18.67979575497178502, 95.41557627198102409 ) ) ;
#48549=CARTESIAN_POINT ( 'NONE',  ( 21.52544592524344225, -5.823673210054117533, 48.54057627198103120 ) ) ;
#48550=CARTESIAN_POINT ( 'NONE',  ( 4.379528057220092307, 16.55341960407617563, 67.29275706135234714 ) ) ;
#48551=CARTESIAN_POINT ( 'NONE',  ( -8.314922557960811034, -14.29746914071050412, 97.08224293864770971 ) ) ;
#48552=CARTESIAN_POINT ( 'NONE',  ( -13.97604488694527625, -13.89961937509977652, 41.87390960531435979 ) ) ;
#48555=CARTESIAN_POINT ( 'NONE',  ( 4.483927247898790824, -16.52544592524335698, 100.2094237280190043 ) ) ;
#48556=CARTESIAN_POINT ( 'NONE',  ( 5.823673210054444382, -21.52544592524334988, 30.20942372801902565 ) ) ;
#48557=CARTESIAN_POINT ( 'NONE',  ( -16.51473224551069308, -9.474510206698971260, 96.66557627198102409 ) ) ;
#48558=CARTESIAN_POINT ( 'NONE',  ( -21.53943276465977519, -0.05219959533937600094, 63.75109039468568284 ) ) ;
#48560=CARTESIAN_POINT ( 'NONE',  ( 19.03943276465977164, -0.05219959533909143690, 28.74890960531435624 ) ) ;
#48562=CARTESIAN_POINT ( 'NONE',  ( 18.62759615963255655, 10.81492255796105972, 56.66775706135235424 ) ) ;
#48563=CARTESIAN_POINT ( 'NONE',  ( 9.474510206698971260, -16.51473224551069308, 47.91557627198102409 ) ) ;
#48564=CARTESIAN_POINT ( 'NONE',  ( 9.474510206698971260, -16.51473224551069308, 22.91557627198102765 ) ) ;
#48565=CARTESIAN_POINT ( 'NONE',  ( -9.564922557960796823, -16.46253265017161027, 92.08224293864769550 ) ) ;
#48566=CARTESIAN_POINT ( 'NONE',  ( 19.02544592524334988, 5.153800228976608722, 66.45942372801899012 ) ) ;
#48567=CARTESIAN_POINT ( 'NONE',  ( -10.81492255796105439, 18.62759615963255655, 27.91775706135234358 ) ) ;
#48568=CARTESIAN_POINT ( 'NONE',  ( 19.03943276465977164, 0.05219959533936151252, 61.25109039468566863 ) ) ;
#48569=CARTESIAN_POINT ( 'NONE',  ( 13.89961937509977652, -13.97604488694527269, 43.12390960531434558 ) ) ;
#48570=CARTESIAN_POINT ( 'NONE',  ( -12.14591786802326823, 12.06949235617739902, 108.1260903946856757 ) ) ;
#48571=CARTESIAN_POINT ( 'NONE',  ( -5.049401038297874678, -19.05341960407617918, 74.79275706135231871 ) ) ;
#48572=CARTESIAN_POINT ( 'NONE',  ( -12.14591786802309592, -12.06949235617757132, 21.87390960531436690 ) ) ;
#48573=CARTESIAN_POINT ( 'NONE',  ( 5.153800228976615827, -19.02544592524334988, 45.20942372801901143 ) ) ;
#48574=CARTESIAN_POINT ( 'NONE',  ( -5.153800228976328057, -19.02544592524343514, 102.2905762719810383 ) ) ;
#48575=CARTESIAN_POINT ( 'NONE',  ( 21.52544592524334988, 5.823673210054432836, 106.4594237280190328 ) ) ;
#48576=CARTESIAN_POINT ( 'NONE',  ( 9.474510206698729675, 16.51473224551082808, 22.08442372801899722 ) ) ;
#48577=CARTESIAN_POINT ( 'NONE',  ( -19.05341960407611168, -5.049401038298163336, 31.45724293864769550 ) ) ;
#48578=CARTESIAN_POINT ( 'NONE',  ( 21.52544592524334988, 5.823673210054432836, 91.45942372801901854 ) ) ;
#48579=CARTESIAN_POINT ( 'NONE',  ( 4.379528057220092307, 16.55341960407617563, 37.29275706135235424 ) ) ;
#48580=CARTESIAN_POINT ( 'NONE',  ( -16.51473224551069308, -9.474510206698971260, 96.66557627198102409 ) ) ;
#48583=CARTESIAN_POINT ( 'NONE',  ( -9.474510206698964154, 16.51473224551069663, 75.41557627198103830 ) ) ;
#48585=CARTESIAN_POINT ( 'NONE',  ( -16.51473224551082808, 9.474510206698731452, 68.33442372801900433 ) ) ;
#48586=CARTESIAN_POINT ( 'NONE',  ( 19.05341960407611168, 5.049401038298154454, 108.9572429386477097 ) ) ;
#48587=CARTESIAN_POINT ( 'NONE',  ( 15.72974639402176855, 15.80617190586768217, 96.87609039468568994 ) ) ;
#48588=CARTESIAN_POINT ( 'NONE',  ( 8.314922557960818139, 14.29746914071049879, 94.58224293864769550 ) ) ;
#48589=CARTESIAN_POINT ( 'NONE',  ( 0.05219959533909260263, 19.03943276465977164, 24.99890960531435269 ) ) ;
#48590=CARTESIAN_POINT ( 'NONE',  ( 21.55341960407610458, 5.719274019375980345, 43.95724293864769550 ) ) ;
#48591=CARTESIAN_POINT ( 'NONE',  ( 10.81492255796078972, 18.62759615963270932, 34.58224293864770260 ) ) ;
#48592=CARTESIAN_POINT ( 'NONE',  ( 14.29746914071049879, -8.314922557960816363, 103.3322429386476955 ) ) ;
#48594=CARTESIAN_POINT ( 'NONE',  ( 19.05341960407617918, -5.049401038297876454, 56.04275706135234714 ) ) ;
#48595=CARTESIAN_POINT ( 'NONE',  ( -16.53943276465976808, 0.05219959533911058130, 46.24890960531435979 ) ) ;
#48596=CARTESIAN_POINT ( 'NONE',  ( -19.03943276465977164, 0.05219959533909376836, 111.2489096053143669 ) ) ;
#48597=CARTESIAN_POINT ( 'NONE',  ( 21.55341960407619695, -5.719274019375665929, 86.04275706135236135 ) ) ;
#48598=CARTESIAN_POINT ( 'NONE',  ( -15.72974639402197994, 15.80617190586746368, 75.62390960531439532 ) ) ;
#48599=CARTESIAN_POINT ( 'NONE',  ( -10.81492255796105439, 18.62759615963255655, 42.91775706135235424 ) ) ;
#48600=CARTESIAN_POINT ( 'NONE',  ( 18.62759615963271287, -10.81492255796078972, 103.3322429386476955 ) ) ;
#48601=CARTESIAN_POINT ( 'NONE',  ( -10.72451020669870658, -18.67979575497194134, 49.58442372801901143 ) ) ;
#48602=CARTESIAN_POINT ( 'NONE',  ( -16.51473224551069308, -9.474510206698971260, 21.66557627198102765 ) ) ;
#48603=CARTESIAN_POINT ( 'NONE',  ( 16.46253265017160672, -9.564922557960803928, 83.33224293864768129 ) ) ;
#48604=CARTESIAN_POINT ( 'NONE',  ( -12.06949235617739369, -12.14591786802326823, 84.37609039468570415 ) ) ;
#48605=CARTESIAN_POINT ( 'NONE',  ( -12.06949235617756955, 12.14591786802309770, 100.6239096053143811 ) ) ;
#48606=CARTESIAN_POINT ( 'NONE',  ( 9.474510206698971260, -16.51473224551069308, 107.9155762719810383 ) ) ;
#48607=CARTESIAN_POINT ( 'NONE',  ( -4.483927247898539470, -16.52544592524342804, 57.29057627198103120 ) ) ;
#48608=CARTESIAN_POINT ( 'NONE',  ( -16.55341960407617563, 4.379528057220093196, 113.5427570613523756 ) ) ;
#48609=CARTESIAN_POINT ( 'NONE',  ( -9.474510206698964154, 16.51473224551069663, 70.41557627198102409 ) ) ;
#48610=CARTESIAN_POINT ( 'NONE',  ( 0.05219959533909260263, 19.03943276465977164, 34.99890960531435979 ) ) ;
#48611=CARTESIAN_POINT ( 'NONE',  ( 0.05219959533907565091, 21.53943276465977519, 49.99890960531437401 ) ) ;
#48612=CARTESIAN_POINT ( 'NONE',  ( -9.564922557961040184, 16.46253265017147172, 32.91775706135233293 ) ) ;
#48613=CARTESIAN_POINT ( 'NONE',  ( -17.49999999999999645, -5.499999999999992895, 49.20309617465830598 ) ) ;
#48614=CARTESIAN_POINT ( 'NONE',  ( -12.06949235617756955, 12.14591786802309770, 30.62390960531436335 ) ) ;
#48615=CARTESIAN_POINT ( 'NONE',  ( -0.05219959533909027116, -19.03943276465977164, 102.4989096053143669 ) ) ;
#48617=CARTESIAN_POINT ( 'NONE',  ( -10.72451020669870658, -18.67979575497194134, 54.58442372801901143 ) ) ;
#48618=CARTESIAN_POINT ( 'NONE',  ( -0.05219959533909027116, -19.03943276465977164, 112.4989096053143669 ) ) ;
#48619=CARTESIAN_POINT ( 'NONE',  ( -16.52544592524335698, -4.483927247898792601, 58.95942372801902565 ) ) ;
#48620=CARTESIAN_POINT ( 'NONE',  ( 16.51473224551083163, -9.474510206698727899, 65.83442372801900433 ) ) ;
#48621=CARTESIAN_POINT ( 'NONE',  ( 16.55341960407611168, 4.379528057220329451, 28.95724293864769905 ) ) ;
#48622=CARTESIAN_POINT ( 'NONE',  ( -19.39720447994793773, -5.500000000000083489, 74.66317477297180005 ) ) ;
#48623=CARTESIAN_POINT ( 'NONE',  ( 8.314922557961029526, -14.29746914071037800, 100.4177570613523471 ) ) ;
#48624=CARTESIAN_POINT ( 'NONE',  ( 19.02544592524343514, -5.153800228976328945, 43.54057627198103120 ) ) ;
#48625=CARTESIAN_POINT ( 'NONE',  ( 0.05219959533909260263, 19.03943276465977164, 54.99890960531435979 ) ) ;
#48626=CARTESIAN_POINT ( 'NONE',  ( -19.05341960407611168, -5.049401038298163336, 26.45724293864769550 ) ) ;
#48627=CARTESIAN_POINT ( 'NONE',  ( 5.719274019375673035, 21.55341960407619339, 27.29275706135234358 ) ) ;
#48628=CARTESIAN_POINT ( 'NONE',  ( -19.02544592524342804, 5.153800228976336051, 51.04057627198103120 ) ) ;
#48630=CARTESIAN_POINT ( 'NONE',  ( -19.02544592524342804, 5.153800228976336051, 41.04057627198103120 ) ) ;
#48631=CARTESIAN_POINT ( 'NONE',  ( 15.72974639402199770, -15.80617190586745480, 28.12390960531435979 ) ) ;
#48632=CARTESIAN_POINT ( 'NONE',  ( -18.67979575497193778, 10.72451020669871902, 53.33442372801901854 ) ) ;
#48633=CARTESIAN_POINT ( 'NONE',  ( 16.55341960407611168, 4.379528057220329451, 113.9572429386477239 ) ) ;
#48634=CARTESIAN_POINT ( 'NONE',  ( -5.823673210054116645, -21.52544592524344225, 27.29057627198103120 ) ) ;
#48635=CARTESIAN_POINT ( 'NONE',  ( -16.53943276465976808, -0.05219959533934237506, 73.75109039468567573 ) ) ;
#48636=CARTESIAN_POINT ( 'NONE',  ( -10.81492255796105439, 18.62759615963255655, 102.9177570613523756 ) ) ;
#48637=CARTESIAN_POINT ( 'NONE',  ( -16.55341960407617563, 4.379528057220093196, 53.54275706135234714 ) ) ;
#48638=CARTESIAN_POINT ( 'NONE',  ( -13.97604488694527625, -13.89961937509977652, 91.87390960531432427 ) ) ;
#48639=CARTESIAN_POINT ( 'NONE',  ( 12.14591786802327356, -12.06949235617739191, 40.62609039468567573 ) ) ;
#48640=CARTESIAN_POINT ( 'NONE',  ( 16.55341960407618274, -4.379528057220086978, 31.04275706135234714 ) ) ;
#48641=CARTESIAN_POINT ( 'NONE',  ( 12.06949235617739724, 12.14591786802326823, 91.87609039468568994 ) ) ;
#48642=CARTESIAN_POINT ( 'NONE',  ( -21.55341960407619339, 5.719274019375674811, 53.54275706135234714 ) ) ;
#48643=CARTESIAN_POINT ( 'NONE',  ( 5.049401038297881783, 19.05341960407617563, 102.2927570613523045 ) ) ;
#48644=CARTESIAN_POINT ( 'NONE',  ( 5.823673210054125526, 21.52544592524343514, 109.7905762719810383 ) ) ;
#48645=CARTESIAN_POINT ( 'NONE',  ( -16.55341960407611168, -4.379528057220339221, 106.4572429386477097 ) ) ;
#48646=CARTESIAN_POINT ( 'NONE',  ( -5.153800228976607833, 19.02544592524334988, 107.7094237280189759 ) ) ;
#48647=CARTESIAN_POINT ( 'NONE',  ( 16.55341960407618274, -4.379528057220086978, 91.04275706135236135 ) ) ;
#48648=CARTESIAN_POINT ( 'NONE',  ( -17.48853670773247870, 5.747243402302952830, 43.66671299749993551 ) ) ;
#48649=CARTESIAN_POINT ( 'NONE',  ( -0.05219959533936034679, 19.03943276465977164, 82.50109039468567573 ) ) ;
#48650=CARTESIAN_POINT ( 'NONE',  ( -4.379528057220328563, 16.55341960407611168, 45.20724293864769550 ) ) ;
#48651=CARTESIAN_POINT ( 'NONE',  ( 14.34966873604960469, 8.224510206698951720, 44.16557627198103120 ) ) ;
#48652=CARTESIAN_POINT ( 'NONE',  ( -14.34966873604960291, -8.224510206698953496, 106.6655762719810383 ) ) ;
#48653=CARTESIAN_POINT ( 'NONE',  ( 19.03943276465977164, 0.05219959533936151252, 46.25109039468566863 ) ) ;
#48654=CARTESIAN_POINT ( 'NONE',  ( -17.44279575226822843, 5.990770900252461395, 90.83557567514318976 ) ) ;
#48655=CARTESIAN_POINT ( 'NONE',  ( 21.55341960407619695, -5.719274019375665929, 41.04275706135236135 ) ) ;
#48656=CARTESIAN_POINT ( 'NONE',  ( 9.564922557961047289, -16.46253265017146816, 105.4177570613523471 ) ) ;
#48658=CARTESIAN_POINT ( 'NONE',  ( -0.05219959533909027116, -19.03943276465977164, 92.49890960531436690 ) ) ;
#48659=CARTESIAN_POINT ( 'NONE',  ( 19.02544592524343514, -5.153800228976328945, 83.54057627198100988 ) ) ;
#48660=CARTESIAN_POINT ( 'NONE',  ( 5.719274019375991003, -21.55341960407610458, 57.70724293864770260 ) ) ;
#48661=CARTESIAN_POINT ( 'NONE',  ( -12.14591786802309592, -12.06949235617757132, 111.8739096053143669 ) ) ;
#48662=CARTESIAN_POINT ( 'NONE',  ( 16.51473224551069308, 9.474510206698969483, 69.16557627198102409 ) ) ;
#48663=CARTESIAN_POINT ( 'NONE',  ( -19.05341960407611168, -5.049401038298163336, 26.45724293864769550 ) ) ;
#48664=CARTESIAN_POINT ( 'NONE',  ( 5.823673210054444382, -21.52544592524334988, 40.20942372801901854 ) ) ;
#48665=CARTESIAN_POINT ( 'NONE',  ( -21.53943276465977519, -0.05219959533937600094, 73.75109039468567573 ) ) ;
#48666=CARTESIAN_POINT ( 'NONE',  ( -16.55341960407617563, 4.379528057220093196, 88.54275706135236135 ) ) ;
#48668=CARTESIAN_POINT ( 'NONE',  ( -18.62759615963255300, -10.81492255796106328, 24.16775706135235424 ) ) ;
#48669=CARTESIAN_POINT ( 'NONE',  ( -21.52544592524334988, -5.823673210054445271, 23.95942372801901143 ) ) ;
#48670=CARTESIAN_POINT ( 'NONE',  ( 19.02544592524334988, 5.153800228976608722, 56.45942372801898301 ) ) ;
#48671=CARTESIAN_POINT ( 'NONE',  ( 19.03943276465977164, -0.05219959533909143690, 78.74890960531436690 ) ) ;
#48672=CARTESIAN_POINT ( 'NONE',  ( 0.05219959533937995610, -21.53943276465977519, 90.00109039468567573 ) ) ;
#48673=CARTESIAN_POINT ( 'NONE',  ( -21.55341960407610458, -5.719274019375992779, 86.45724293864770971 ) ) ;
#48674=CARTESIAN_POINT ( 'NONE',  ( 8.224510206698953496, -14.34966873604960469, 47.91557627198102409 ) ) ;
#48675=CARTESIAN_POINT ( 'NONE',  ( -21.53943276465977519, -0.05219959533937600094, 108.7510903946857042 ) ) ;
#48676=CARTESIAN_POINT ( 'NONE',  ( 16.53943276465976808, -0.05219959533910856209, 83.74890960531435269 ) ) ;
#48677=CARTESIAN_POINT ( 'NONE',  ( 4.483927247898545687, 16.52544592524342804, 114.7905762719810383 ) ) ;
#48678=CARTESIAN_POINT ( 'NONE',  ( 9.474510206698729675, 16.51473224551082808, 72.08442372801900433 ) ) ;
#48679=CARTESIAN_POINT ( 'NONE',  ( -12.14591786802309592, -12.06949235617757132, 41.87390960531435979 ) ) ;
#48680=CARTESIAN_POINT ( 'NONE',  ( -5.719274019375665041, -21.55341960407619695, 84.79275706135234714 ) ) ;
#48681=CARTESIAN_POINT ( 'NONE',  ( 0.05219959533909260263, 19.03943276465977164, 94.99890960531436690 ) ) ;
#48682=CARTESIAN_POINT ( 'NONE',  ( -16.46253265017146816, -9.564922557961047289, 59.16775706135233293 ) ) ;
#48683=CARTESIAN_POINT ( 'NONE',  ( -21.53943276465977519, 0.05219959533907696930, 61.24890960531435979 ) ) ;
#48684=CARTESIAN_POINT ( 'NONE',  ( -0.05219959533907301413, -21.53943276465977519, 112.4989096053143669 ) ) ;
#48685=CARTESIAN_POINT ( 'NONE',  ( 4.379528057220092307, 16.55341960407617563, 22.29275706135235069 ) ) ;
#48686=CARTESIAN_POINT ( 'NONE',  ( 12.14591786802327356, -12.06949235617739191, 75.62609039468567573 ) ) ;
#48687=CARTESIAN_POINT ( 'NONE',  ( -21.52544592524334988, -5.823673210054445271, 28.95942372801902209 ) ) ;
#48688=CARTESIAN_POINT ( 'NONE',  ( 14.34966873604960469, 8.224510206698951720, 109.1655762719810383 ) ) ;
#48690=CARTESIAN_POINT ( 'NONE',  ( 0.05219959533934541429, -16.53943276465976808, 30.00109039468568284 ) ) ;
#48691=PRODUCT_DEFINITION ( 'UNKNOWN', '', #82349, #3893 ) ;
#48692=CARTESIAN_POINT ( 'NONE',  ( -18.67979575497178146, -10.72451020669898902, 56.66557627198103830 ) ) ;
#48693=CARTESIAN_POINT ( 'NONE',  ( -12.06949235617739369, -12.14591786802326823, 99.37609039468568994 ) ) ;
#48694=CARTESIAN_POINT ( 'NONE',  ( 8.314922557961029526, -14.29746914071037800, 40.41775706135234714 ) ) ;
#48695=CARTESIAN_POINT ( 'NONE',  ( -5.153800228976328057, -19.02544592524343514, 37.29057627198102409 ) ) ;
#48696=CARTESIAN_POINT ( 'NONE',  ( 16.52544592524335698, 4.483927247898782831, 86.45942372801901854 ) ) ;
#48697=CARTESIAN_POINT ( 'NONE',  ( 19.02544592524334988, 5.153800228976608722, 71.45942372801900433 ) ) ;
#48698=CARTESIAN_POINT ( 'NONE',  ( 21.53943276465977519, -0.05219959533907433946, 58.74890960531436690 ) ) ;
#48699=CARTESIAN_POINT ( 'NONE',  ( 16.55341960407618274, -4.379528057220086978, 101.0427570613523756 ) ) ;
#48700=CARTESIAN_POINT ( 'NONE',  ( 5.719274019375673035, 21.55341960407619339, 77.29275706135234714 ) ) ;
#48701=CARTESIAN_POINT ( 'NONE',  ( -21.55341960407610458, -5.719274019375992779, 56.45724293864768839 ) ) ;
#48702=CARTESIAN_POINT ( 'NONE',  ( -21.55341960407610458, -5.719274019375992779, 46.45724293864769550 ) ) ;
#48703=CARTESIAN_POINT ( 'NONE',  ( 4.483927247898790824, -16.52544592524335698, 80.20942372801901854 ) ) ;
#48704=CARTESIAN_POINT ( 'NONE',  ( -15.72974639402197994, 15.80617190586746368, 40.62390960531435269 ) ) ;
#48706=CARTESIAN_POINT ( 'NONE',  ( 13.97604488694527802, 13.89961937509977652, 99.37390960531436690 ) ) ;
#48708=CARTESIAN_POINT ( 'NONE',  ( -9.564922557960796823, -16.46253265017161027, 22.08224293864768839 ) ) ;
#48709=CARTESIAN_POINT ( 'NONE',  ( 5.719274019375991003, -21.55341960407610458, 67.70724293864769550 ) ) ;
#48710=CARTESIAN_POINT ( 'NONE',  ( -14.29746914071037622, -8.314922557961029526, 109.1677570613523613 ) ) ;
#48711=CARTESIAN_POINT ( 'NONE',  ( -21.52544592524334988, -5.823673210054445271, 48.95942372801902565 ) ) ;
#48712=CARTESIAN_POINT ( 'NONE',  ( 19.05341960407617918, -5.049401038297876454, 101.0427570613523045 ) ) ;
#48713=CARTESIAN_POINT ( 'NONE',  ( 14.34966873604960469, 8.224510206698951720, 109.1655762719810383 ) ) ;
#48714=CARTESIAN_POINT ( 'NONE',  ( -16.51473224551082808, 9.474510206698731452, 108.3344237280190043 ) ) ;
#48715=CARTESIAN_POINT ( 'NONE',  ( 0.05219959533909260263, 19.03943276465977164, 39.99890960531436690 ) ) ;
#48717=CARTESIAN_POINT ( 'NONE',  ( -5.153800228976328057, -19.02544592524343514, 87.29057627198103830 ) ) ;
#48718=CARTESIAN_POINT ( 'NONE',  ( -16.53943276465976808, -0.05219959533934237506, 78.75109039468568994 ) ) ;
#48719=CARTESIAN_POINT ( 'NONE',  ( -9.474510206698720793, -16.51473224551083518, 74.58442372801900433 ) ) ;
#48720=CARTESIAN_POINT ( 'NONE',  ( 10.72451020669871369, 18.67979575497193778, 107.0844237280190043 ) ) ;
#48721=CARTESIAN_POINT ( 'NONE',  ( 21.52544592524344225, -5.823673210054117533, 63.54057627198103830 ) ) ;
#48722=CARTESIAN_POINT ( 'NONE',  ( -12.06949235617739369, -12.14591786802326823, 84.37609039468570415 ) ) ;
#48723=CARTESIAN_POINT ( 'NONE',  ( 9.564922557961047289, -16.46253265017146816, 75.41775706135234714 ) ) ;
#48724=CARTESIAN_POINT ( 'NONE',  ( 19.05341960407611168, 5.049401038298154454, 38.95724293864767418 ) ) ;
#48725=CARTESIAN_POINT ( 'NONE',  ( -5.153800228976328057, -19.02544592524343514, 72.29057627198102409 ) ) ;
#48726=CARTESIAN_POINT ( 'NONE',  ( 18.62759615963255655, 10.81492255796105972, 51.66775706135234714 ) ) ;
#48727=CARTESIAN_POINT ( 'NONE',  ( 5.049401038298161559, -19.05341960407611168, 52.70724293864767418 ) ) ;
#48728=CARTESIAN_POINT ( 'NONE',  ( 5.153800228976615827, -19.02544592524334988, 70.20942372801899012 ) ) ;
#48730=CARTESIAN_POINT ( 'NONE',  ( 16.46253265017160672, -9.564922557960803928, 103.3322429386476955 ) ) ;
#48731=CARTESIAN_POINT ( 'NONE',  ( -14.34966873604960291, -8.224510206698953496, 66.66557627198102409 ) ) ;
#48732=CARTESIAN_POINT ( 'NONE',  ( -21.55341960407610458, -5.719274019375992779, 56.45724293864768839 ) ) ;
#48734=CARTESIAN_POINT ( 'NONE',  ( -13.97604488694547697, 13.89961937509957934, 28.12609039468565797 ) ) ;
#48736=CARTESIAN_POINT ( 'NONE',  ( 19.02544592524343514, -5.153800228976328945, 68.54057627198103830 ) ) ;
#48737=CARTESIAN_POINT ( 'NONE',  ( 9.564922557960805705, 16.46253265017160317, 79.58224293864769550 ) ) ;
#48738=CARTESIAN_POINT ( 'NONE',  ( 4.379528057220092307, 16.55341960407617563, 57.29275706135234714 ) ) ;
#48739=CARTESIAN_POINT ( 'NONE',  ( 5.153800228976617603, -19.02544592524335343, 80.20942372801900433 ) ) ;
#48740=CARTESIAN_POINT ( 'NONE',  ( -17.13100169013301510, 6.664070546373130455, 110.7678983569984723 ) ) ;
#48741=CARTESIAN_POINT ( 'NONE',  ( 4.379528057220092307, 16.55341960407617563, 87.29275706135236135 ) ) ;
#48743=CARTESIAN_POINT ( 'NONE',  ( -14.34966873604972548, 8.224510206698743886, 63.33442372801900433 ) ) ;
#48745=CARTESIAN_POINT ( 'NONE',  ( 8.224510206698742110, 14.34966873604972548, 37.08442372801901143 ) ) ;
#48746=CARTESIAN_POINT ( 'NONE',  ( -19.02544592524342804, 5.153800228976336051, 56.04057627198100988 ) ) ;
#48748=CARTESIAN_POINT ( 'NONE',  ( -15.72974639402176322, -15.80617190586768395, 59.37609039468568284 ) ) ;
#48749=CARTESIAN_POINT ( 'NONE',  ( -9.564922557961040184, 16.46253265017147172, 67.91775706135233293 ) ) ;
#48750=CARTESIAN_POINT ( 'NONE',  ( -15.72974639402176322, -15.80617190586768395, 109.3760903946857042 ) ) ;
#48751=CARTESIAN_POINT ( 'NONE',  ( -13.89961937509977652, 13.97604488694528158, 35.62390960531435269 ) ) ;
#48752=CARTESIAN_POINT ( 'NONE',  ( -17.49999999999999645, -5.500000000000005329, 31.28230962303567253 ) ) ;
#48753=CARTESIAN_POINT ( 'NONE',  ( 21.52544592524344225, -5.823673210054117533, 48.54057627198103120 ) ) ;
#48754=CARTESIAN_POINT ( 'NONE',  ( 18.62759615963271287, -10.81492255796078972, 23.33224293864769194 ) ) ;
#48755=CARTESIAN_POINT ( 'NONE',  ( -8.224510206698948167, 14.34966873604960824, 100.4155762719810241 ) ) ;
#48756=CARTESIAN_POINT ( 'NONE',  ( 14.34966873604972726, -8.224510206698740333, 35.83442372801901143 ) ) ;
#48757=CARTESIAN_POINT ( 'NONE',  ( 8.224510206698953496, -14.34966873604960469, 32.91557627198102409 ) ) ;
#48759=CARTESIAN_POINT ( 'NONE',  ( -15.72974639402176322, -15.80617190586768395, 19.37609039468568639 ) ) ;
#48760=CARTESIAN_POINT ( 'NONE',  ( -0.05219959533910754901, -16.53943276465976808, 37.49890960531436690 ) ) ;
#48762=CARTESIAN_POINT ( 'NONE',  ( -9.564922557961040184, 16.46253265017147172, 97.91775706135233293 ) ) ;
#48763=CARTESIAN_POINT ( 'NONE',  ( -0.05219959533936034679, 19.03943276465977164, 32.50109039468566863 ) ) ;
#48764=CARTESIAN_POINT ( 'NONE',  ( -14.29746914071049879, 8.314922557960819915, 30.83224293864770260 ) ) ;
#48765=CARTESIAN_POINT ( 'NONE',  ( -15.72974639402197994, 15.80617190586746368, 100.6239096053143811 ) ) ;
#48767=CARTESIAN_POINT ( 'NONE',  ( 21.53943276465977519, -0.05219959533907433946, 68.74890960531435269 ) ) ;
#48768=CARTESIAN_POINT ( 'NONE',  ( 13.89961937509977652, -13.97604488694527269, 78.12390960531433848 ) ) ;
#48769=CARTESIAN_POINT ( 'NONE',  ( 14.34966873604960469, 8.224510206698951720, 49.16557627198102409 ) ) ;
#48770=CARTESIAN_POINT ( 'NONE',  ( -19.03943276465977164, 0.05219959533909376836, 96.24890960531436690 ) ) ;
#48772=CARTESIAN_POINT ( 'NONE',  ( 16.46253265017146816, 9.564922557961045513, 46.66775706135233293 ) ) ;
#48773=CARTESIAN_POINT ( 'NONE',  ( -18.62759615963270932, 10.81492255796079327, 90.83224293864769550 ) ) ;
#48774=CARTESIAN_POINT ( 'NONE',  ( 14.34966873604960469, 8.224510206698951720, 99.16557627198100988 ) ) ;
#48775=CARTESIAN_POINT ( 'NONE',  ( 21.53943276465977519, 0.05219959533937863772, 41.25109039468568284 ) ) ;
#48778=CARTESIAN_POINT ( 'NONE',  ( 8.314922557961029526, -14.29746914071037800, 105.4177570613523613 ) ) ;
#48779=CARTESIAN_POINT ( 'NONE',  ( -19.02544592524342804, 5.153800228976336051, 31.04057627198102409 ) ) ;
#48780=CARTESIAN_POINT ( 'NONE',  ( -13.89961937509977652, 13.97604488694528158, 90.62390960531432427 ) ) ;
#48781=CARTESIAN_POINT ( 'NONE',  ( 10.72451020669898902, -18.67979575497178502, 57.91557627198103120 ) ) ;
#48783=CARTESIAN_POINT ( 'NONE',  ( -5.153800228976328057, -19.02544592524343514, 37.29057627198102409 ) ) ;
#48784=CARTESIAN_POINT ( 'NONE',  ( -8.314922557960811034, -14.29746914071050412, 42.08224293864769550 ) ) ;
#48785=CARTESIAN_POINT ( 'NONE',  ( 5.719274019375673035, 21.55341960407619339, 67.29275706135234714 ) ) ;
#48787=CARTESIAN_POINT ( 'NONE',  ( 8.224510206698742110, 14.34966873604972548, 67.08442372801901854 ) ) ;
#48788=CARTESIAN_POINT ( 'NONE',  ( -19.03943276465977164, 0.05219959533909376836, 51.24890960531436690 ) ) ;
#48789=CARTESIAN_POINT ( 'NONE',  ( -19.03943276465977164, 0.05219959533909376836, 66.24890960531436690 ) ) ;
#48791=CARTESIAN_POINT ( 'NONE',  ( -15.72974639402176322, -15.80617190586768395, 104.3760903946856899 ) ) ;
#48792=CARTESIAN_POINT ( 'NONE',  ( 12.14591786802327356, -12.06949235617739191, 70.62609039468567573 ) ) ;
#48793=CARTESIAN_POINT ( 'NONE',  ( -21.53943276465977519, -0.05219959533937600094, 93.75109039468567573 ) ) ;
#48794=CARTESIAN_POINT ( 'NONE',  ( 9.474510206698971260, -16.51473224551069308, 67.91557627198102409 ) ) ;
#48795=CARTESIAN_POINT ( 'NONE',  ( -21.55341960407610458, -5.719274019375992779, 36.45724293864768839 ) ) ;
#48796=CARTESIAN_POINT ( 'NONE',  ( 16.46253265017146816, 9.564922557961045513, 101.6677570613523329 ) ) ;
#48797=CARTESIAN_POINT ( 'NONE',  ( 21.52544592524334988, 5.823673210054432836, 86.45942372801901854 ) ) ;
#48798=CARTESIAN_POINT ( 'NONE',  ( 8.314922557961029526, -14.29746914071037800, 55.41775706135234714 ) ) ;
#48799=CARTESIAN_POINT ( 'NONE',  ( 18.62759615963271287, -10.81492255796078972, 98.33224293864769550 ) ) ;
#48800=CARTESIAN_POINT ( 'NONE',  ( -0.05219959533936034679, 19.03943276465977164, 97.50109039468567573 ) ) ;
#48801=CARTESIAN_POINT ( 'NONE',  ( 16.46253265017160672, -9.564922557960803928, 83.33224293864768129 ) ) ;
#48802=CARTESIAN_POINT ( 'NONE',  ( 19.05341960407617918, -5.049401038297876454, 106.0427570613523471 ) ) ;
#48803=CARTESIAN_POINT ( 'NONE',  ( 8.224510206698742110, 14.34966873604972548, 22.08442372801901143 ) ) ;
#48804=CARTESIAN_POINT ( 'NONE',  ( -12.06949235617756955, 12.14591786802309770, 60.62390960531437401 ) ) ;
#48805=CARTESIAN_POINT ( 'NONE',  ( -16.55341960407617563, 4.379528057220093196, 68.54275706135234714 ) ) ;
#48806=CARTESIAN_POINT ( 'NONE',  ( -5.719274019375665041, -21.55341960407619695, 29.79275706135234358 ) ) ;
#48807=CARTESIAN_POINT ( 'NONE',  ( -9.564922557960796823, -16.46253265017161027, 47.08224293864769550 ) ) ;
#48808=CARTESIAN_POINT ( 'NONE',  ( 9.474510206698971260, -16.51473224551069308, 72.91557627198102409 ) ) ;
#48809=CARTESIAN_POINT ( 'NONE',  ( -0.05219959533934338120, 16.53943276465976808, 72.50109039468568994 ) ) ;
#48812=VERTEX_POINT ( 'NONE', #176876 ) ;
#48813=CARTESIAN_POINT ( 'NONE',  ( 10.81492255796106328, -18.62759615963255655, 110.4177570613523756 ) ) ;
#48814=CARTESIAN_POINT ( 'NONE',  ( 9.564922557960805705, 16.46253265017160317, 34.58224293864770260 ) ) ;
#48816=CARTESIAN_POINT ( 'NONE',  ( 4.483927247898790824, -16.52544592524335698, 35.20942372801901854 ) ) ;
#48817=CARTESIAN_POINT ( 'NONE',  ( -16.46253265017146816, -9.564922557961047289, 44.16775706135232582 ) ) ;
#48818=CARTESIAN_POINT ( 'NONE',  ( 8.224510206698742110, 14.34966873604972548, 47.08442372801901854 ) ) ;
#48819=CARTESIAN_POINT ( 'NONE',  ( 5.153800228976335163, 19.02544592524342804, 49.79057627198100988 ) ) ;
#48820=CARTESIAN_POINT ( 'NONE',  ( 13.97604488694527802, 13.89961937509977652, 64.37390960531436690 ) ) ;
#48821=CARTESIAN_POINT ( 'NONE',  ( 10.81492255796078972, 18.62759615963270932, 89.58224293864768129 ) ) ;
#48822=CARTESIAN_POINT ( 'NONE',  ( -5.049401038298153566, 19.05341960407611168, 80.20724293864769550 ) ) ;
#48823=CARTESIAN_POINT ( 'NONE',  ( 0.05219959533909260263, 19.03943276465977164, 109.9989096053143669 ) ) ;
#48824=CARTESIAN_POINT ( 'NONE',  ( -13.89961937509977652, 13.97604488694528158, 60.62390960531436690 ) ) ;
#48826=CARTESIAN_POINT ( 'NONE',  ( 16.46253265017146816, 9.564922557961045513, 101.6677570613523329 ) ) ;
#48827=CARTESIAN_POINT ( 'NONE',  ( 10.81492255796078972, 18.62759615963270932, 79.58224293864769550 ) ) ;
#48828=CARTESIAN_POINT ( 'NONE',  ( -9.474510206698720793, -16.51473224551083518, 29.58442372801900433 ) ) ;
#48829=CARTESIAN_POINT ( 'NONE',  ( -4.483927247898539470, -16.52544592524342804, 67.29057627198103830 ) ) ;
#48830=CARTESIAN_POINT ( 'NONE',  ( -21.55341960407619339, 5.719274019375674811, 88.54275706135236135 ) ) ;
#48831=CARTESIAN_POINT ( 'NONE',  ( -8.224510206698948167, 14.34966873604960824, 115.4155762719810241 ) ) ;
#48832=CARTESIAN_POINT ( 'NONE',  ( 4.483927247898545687, 16.52544592524342804, 29.79057627198102409 ) ) ;
#48833=CARTESIAN_POINT ( 'NONE',  ( 10.81492255796106328, -18.62759615963255655, 95.41775706135234714 ) ) ;
#48834=CARTESIAN_POINT ( 'NONE',  ( -9.474510206698964154, 16.51473224551069663, 80.41557627198103830 ) ) ;
#48835=CARTESIAN_POINT ( 'NONE',  ( 5.719274019375673035, 21.55341960407619339, 42.29275706135235424 ) ) ;
#48836=CARTESIAN_POINT ( 'NONE',  ( 13.89961937509977652, -13.97604488694527269, 78.12390960531433848 ) ) ;
#48837=CARTESIAN_POINT ( 'NONE',  ( 0.05219959533910956823, 16.53943276465976808, 99.99890960531436690 ) ) ;
#48838=CARTESIAN_POINT ( 'NONE',  ( 14.29746914071049879, -8.314922557960816363, 58.33224293864768839 ) ) ;
#48839=CARTESIAN_POINT ( 'NONE',  ( -10.72451020669898014, 18.67979575497178502, 70.41557627198102409 ) ) ;
#48840=CARTESIAN_POINT ( 'NONE',  ( 16.46253265017160672, -9.564922557960803928, 68.33224293864770971 ) ) ;
#48841=CARTESIAN_POINT ( 'NONE',  ( -15.72974639402197994, 15.80617190586746368, 80.62390960531438111 ) ) ;
#48842=CARTESIAN_POINT ( 'NONE',  ( 13.97604488694548053, -13.89961937509957401, 80.62609039468567573 ) ) ;
#48843=CARTESIAN_POINT ( 'NONE',  ( -19.03943276465977164, -0.05219959533935918106, 33.75109039468566863 ) ) ;
#48844=CARTESIAN_POINT ( 'NONE',  ( -16.53943276465976808, 0.05219959533911058130, 71.24890960531435269 ) ) ;
#48845=CARTESIAN_POINT ( 'NONE',  ( 15.72974639402199770, -15.80617190586745480, 53.12390960531436690 ) ) ;
#48847=CARTESIAN_POINT ( 'NONE',  ( -12.06949235617739369, -12.14591786802326823, 99.37609039468568994 ) ) ;
#48849=CARTESIAN_POINT ( 'NONE',  ( -19.02544592524334988, -5.153800228976617603, 103.9594237280190043 ) ) ;
#48850=CARTESIAN_POINT ( 'NONE',  ( 14.29746914071049879, -8.314922557960816363, 78.33224293864770971 ) ) ;
#48851=CARTESIAN_POINT ( 'NONE',  ( -17.50000000000147793, 3.254303733634561269, 35.02395893071405197 ) ) ;
#48852=CARTESIAN_POINT ( 'NONE',  ( -19.05341960407611168, -5.049401038298163336, 71.45724293864766707 ) ) ;
#48853=CARTESIAN_POINT ( 'NONE',  ( -13.97604488694527625, -13.89961937509977652, 36.87390960531436690 ) ) ;
#48854=CARTESIAN_POINT ( 'NONE',  ( -14.34966873604960291, -8.224510206698953496, 61.66557627198103120 ) ) ;
#48855=CARTESIAN_POINT ( 'NONE',  ( -0.05219959533909027116, -19.03943276465977164, 97.49890960531436690 ) ) ;
#48856=CARTESIAN_POINT ( 'NONE',  ( 16.51473224551083163, -9.474510206698727899, 95.83442372801900433 ) ) ;
#48857=CARTESIAN_POINT ( 'NONE',  ( -9.474510206698964154, 16.51473224551069663, 60.41557627198102409 ) ) ;
#48858=CARTESIAN_POINT ( 'NONE',  ( -14.29746914071037622, -8.314922557961029526, 24.16775706135235424 ) ) ;
#48859=CARTESIAN_POINT ( 'NONE',  ( -5.153800228976328057, -19.02544592524343514, 92.29057627198099567 ) ) ;
#48860=CARTESIAN_POINT ( 'NONE',  ( -18.67979575497178146, -10.72451020669898902, 66.66557627198102409 ) ) ;
#48861=CARTESIAN_POINT ( 'NONE',  ( -4.483927247898782831, 16.52544592524335698, 52.70942372801902565 ) ) ;
#48862=CARTESIAN_POINT ( 'NONE',  ( -17.26058549869103942, 6.457015423128297016, 93.62254162523932166 ) ) ;
#48863=CARTESIAN_POINT ( 'NONE',  ( 0.05219959533909260263, 19.03943276465977164, 64.99890960531436690 ) ) ;
#48864=CARTESIAN_POINT ( 'NONE',  ( -15.72974639402197994, 15.80617190586746368, 65.62390960531436690 ) ) ;
#48865=CARTESIAN_POINT ( 'NONE',  ( -9.564922557961040184, 16.46253265017147172, 92.91775706135233293 ) ) ;
#48866=CARTESIAN_POINT ( 'NONE',  ( -4.483927247898782831, 16.52544592524335698, 112.7094237280190328 ) ) ;
#48867=CARTESIAN_POINT ( 'NONE',  ( 18.62759615963255655, 10.81492255796105972, 51.66775706135234714 ) ) ;
#48869=CARTESIAN_POINT ( 'NONE',  ( -4.379528057220086978, -16.55341960407618274, 69.79275706135234714 ) ) ;
#48870=CARTESIAN_POINT ( 'NONE',  ( 19.02544592524343514, -5.153800228976328945, 103.5405762719809957 ) ) ;
#48871=CARTESIAN_POINT ( 'NONE',  ( 18.87075004821566537, -5.499999999999866773, 41.17408112101043116 ) ) ;
#48872=CARTESIAN_POINT ( 'NONE',  ( -16.21995358207307092, -7.366697692864072167, 35.06448998487840640 ) ) ;
#48873=CARTESIAN_POINT ( 'NONE',  ( 14.34966873604972726, -8.224510206698740333, 90.83442372801901854 ) ) ;
#48874=CARTESIAN_POINT ( 'NONE',  ( 14.29746914071037800, 8.314922557961029526, 36.66775706135234714 ) ) ;
#48875=CARTESIAN_POINT ( 'NONE',  ( -9.474510206698964154, 16.51473224551069663, 50.41557627198102409 ) ) ;
#48876=CARTESIAN_POINT ( 'NONE',  ( -5.153800228976328057, -19.02544592524343514, 47.29057627198102409 ) ) ;
#48877=CARTESIAN_POINT ( 'NONE',  ( -5.153800228976328057, -19.02544592524343514, 57.29057627198103120 ) ) ;
#48878=CARTESIAN_POINT ( 'NONE',  ( 15.72974639402176855, 15.80617190586768217, 46.87609039468568994 ) ) ;
#48879=CARTESIAN_POINT ( 'NONE',  ( -12.14591786802326823, 12.06949235617739902, 58.12609039468568994 ) ) ;
#48880=CARTESIAN_POINT ( 'NONE',  ( -12.14591786802309592, -12.06949235617757132, 31.87390960531435979 ) ) ;
#48881=CARTESIAN_POINT ( 'NONE',  ( -16.51473224551069308, -9.474510206698971260, 46.66557627198102409 ) ) ;
#48882=CARTESIAN_POINT ( 'NONE',  ( -13.89961937509977652, 13.97604488694528158, 40.62390960531435979 ) ) ;
#48883=CARTESIAN_POINT ( 'NONE',  ( 14.34966873604972726, -8.224510206698740333, 30.83442372801902209 ) ) ;
#48884=CARTESIAN_POINT ( 'NONE',  ( -0.05219959533936034679, 19.03943276465977164, 87.50109039468567573 ) ) ;
#48885=CARTESIAN_POINT ( 'NONE',  ( 4.483927247898545687, 16.52544592524342804, 89.79057627198103830 ) ) ;
#48886=CARTESIAN_POINT ( 'NONE',  ( 0.05219959533909260263, 19.03943276465977164, 49.99890960531435979 ) ) ;
#48887=CARTESIAN_POINT ( 'NONE',  ( 13.89961937509957401, 13.97604488694547697, 91.87609039468567573 ) ) ;
#48889=CARTESIAN_POINT ( 'NONE',  ( 21.52544592524334988, 5.823673210054432836, 71.45942372801901854 ) ) ;
#48890=CARTESIAN_POINT ( 'NONE',  ( -0.05219959533934338120, 16.53943276465976808, 57.50109039468568994 ) ) ;
#48892=CARTESIAN_POINT ( 'NONE',  ( -5.823673210054116645, -21.52544592524344225, 47.29057627198103120 ) ) ;
#48893=CARTESIAN_POINT ( 'NONE',  ( 14.34966873604972726, -8.224510206698740333, 40.83442372801901854 ) ) ;
#48894=CARTESIAN_POINT ( 'NONE',  ( 16.51473224551069308, 9.474510206698969483, 24.16557627198102765 ) ) ;
#48895=CARTESIAN_POINT ( 'NONE',  ( 13.89961937509957401, 13.97604488694547697, 26.87609039468566507 ) ) ;
#48897=CARTESIAN_POINT ( 'NONE',  ( -9.564922557960796823, -16.46253265017161027, 47.08224293864769550 ) ) ;
#48898=DIRECTION ( 'NONE',  ( 0.000000000000000000, 0.000000000000000000, -1.000000000000000000 ) ) ;
#48899=CARTESIAN_POINT ( 'NONE',  ( 16.51473224551069308, 9.474510206698969483, 74.16557627198103830 ) ) ;
#48900=CARTESIAN_POINT ( 'NONE',  ( 17.50000000000000000, -3.805241302050221819, 112.8735247278258953 ) ) ;
#48901=CARTESIAN_POINT ( 'NONE',  ( 5.719274019375673035, 21.55341960407619339, 112.2927570613523471 ) ) ;
#48902=CARTESIAN_POINT ( 'NONE',  ( -12.06949235617756955, 12.14591786802309770, 35.62390960531437401 ) ) ;
#48903=CARTESIAN_POINT ( 'NONE',  ( 0.05219959533909260263, 19.03943276465977164, 39.99890960531436690 ) ) ;
#48905=CARTESIAN_POINT ( 'NONE',  ( -13.97604488694527625, -13.89961937509977652, 106.8739096053143669 ) ) ;
#48906=CARTESIAN_POINT ( 'NONE',  ( -10.72451020669870658, -18.67979575497194134, 74.58442372801901854 ) ) ;
#48907=CARTESIAN_POINT ( 'NONE',  ( 0.05219959533909260263, 19.03943276465977164, 54.99890960531435979 ) ) ;
#48908=CARTESIAN_POINT ( 'NONE',  ( -21.55341960407619339, 5.719274019375674811, 68.54275706135234714 ) ) ;
#48909=CARTESIAN_POINT ( 'NONE',  ( -9.474510206698964154, 16.51473224551069663, 115.4155762719810241 ) ) ;
#48910=CARTESIAN_POINT ( 'NONE',  ( -19.05341960407611168, -5.049401038298163336, 31.45724293864769550 ) ) ;
#48911=CARTESIAN_POINT ( 'NONE',  ( -5.823673210054431948, 21.52544592524334988, 22.70942372801901499 ) ) ;
#48912=CARTESIAN_POINT ( 'NONE',  ( 13.97604488694548053, -13.89961937509957401, 50.62609039468566152 ) ) ;
#48913=CARTESIAN_POINT ( 'NONE',  ( -5.049401038298153566, 19.05341960407611168, 25.20724293864768484 ) ) ;
#48914=CARTESIAN_POINT ( 'NONE',  ( 5.153800228976335163, 19.02544592524342804, 74.79057627198103830 ) ) ;
#48915=CARTESIAN_POINT ( 'NONE',  ( 5.049401038297881783, 19.05341960407617563, 107.2927570613523187 ) ) ;
#48916=CARTESIAN_POINT ( 'NONE',  ( -4.379528057220328563, 16.55341960407611168, 70.20724293864769550 ) ) ;
#48917=CARTESIAN_POINT ( 'NONE',  ( -5.719274019375978568, 21.55341960407610458, 35.20724293864768839 ) ) ;
#48918=CARTESIAN_POINT ( 'NONE',  ( 13.89961937509957401, 13.97604488694547697, 106.8760903946856757 ) ) ;
#48919=CARTESIAN_POINT ( 'NONE',  ( 18.62759615963271287, -10.81492255796078972, 103.3322429386476955 ) ) ;
#48920=CARTESIAN_POINT ( 'NONE',  ( -18.62759615963255300, -10.81492255796106328, 54.16775706135235424 ) ) ;
#48921=CARTESIAN_POINT ( 'NONE',  ( 4.483927247898790824, -16.52544592524335698, 55.20942372801902565 ) ) ;
#48922=CARTESIAN_POINT ( 'NONE',  ( -4.379528057220086978, -16.55341960407618274, 59.79275706135234714 ) ) ;
#48923=CARTESIAN_POINT ( 'NONE',  ( -21.55341960407610458, -5.719274019375992779, 71.45724293864769550 ) ) ;
#48924=CARTESIAN_POINT ( 'NONE',  ( 9.564922557960805705, 16.46253265017160317, 44.58224293864769550 ) ) ;
#48925=CARTESIAN_POINT ( 'NONE',  ( -4.483927247898782831, 16.52544592524335698, 72.70942372801901854 ) ) ;
#48926=CARTESIAN_POINT ( 'NONE',  ( 21.53943276465977519, -0.05219959533907433946, 98.74890960531438111 ) ) ;
#48927=CARTESIAN_POINT ( 'NONE',  ( 4.483927247898545687, 16.52544592524342804, 54.79057627198104541 ) ) ;
#48928=CARTESIAN_POINT ( 'NONE',  ( 13.89961937509977652, -13.97604488694527269, 73.12390960531436690 ) ) ;
#48929=CARTESIAN_POINT ( 'NONE',  ( 14.34966873604972726, -8.224510206698740333, 80.83442372801901854 ) ) ;
#48930=CARTESIAN_POINT ( 'NONE',  ( 16.46253265017146816, 9.564922557961045513, 111.6677570613523329 ) ) ;
#48931=CARTESIAN_POINT ( 'NONE',  ( -10.81492255796078084, -18.62759615963271287, 107.0822429386476955 ) ) ;
#48932=CARTESIAN_POINT ( 'NONE',  ( 12.14591786802309770, 12.06949235617756955, 39.37390960531436690 ) ) ;
#48933=EDGE_CURVE ( 'NONE', #2480, #102413, #98244, .T. ) ;
#48934=ORIENTED_EDGE ( 'NONE', *, *, #136064, .T. ) ;
#48935=CARTESIAN_POINT ( 'NONE',  ( -16.19135201231366139, 7.376712067591930655, 74.81319145947973936 ) ) ;
#48936=CARTESIAN_POINT ( 'NONE',  ( 10.81492255796078972, 18.62759615963270932, 89.58224293864768129 ) ) ;
#48937=CARTESIAN_POINT ( 'NONE',  ( 14.29746914071049879, -8.314922557960816363, 23.33224293864769194 ) ) ;
#48940=CARTESIAN_POINT ( 'NONE',  ( 10.81492255796078972, 18.62759615963270932, 99.58224293864770971 ) ) ;
#48941=CARTESIAN_POINT ( 'NONE',  ( -0.05219959533909027116, -19.03943276465977164, 112.4989096053143669 ) ) ;
#48942=CARTESIAN_POINT ( 'NONE',  ( -5.719274019375665041, -21.55341960407619695, 29.79275706135234358 ) ) ;
#48943=CARTESIAN_POINT ( 'NONE',  ( 12.06949235617757843, -12.14591786802309237, 48.12390960531436690 ) ) ;
#48944=CARTESIAN_POINT ( 'NONE',  ( -0.05219959533934338120, 16.53943276465976808, 47.50109039468568994 ) ) ;
#48945=CARTESIAN_POINT ( 'NONE',  ( 5.153800228976335163, 19.02544592524342804, 54.79057627198103120 ) ) ;
#48946=CARTESIAN_POINT ( 'NONE',  ( 19.05341960407617918, -5.049401038297876454, 51.04275706135231871 ) ) ;
#48947=CARTESIAN_POINT ( 'NONE',  ( 9.474510206698971260, -16.51473224551069308, 82.91557627198103830 ) ) ;
#48948=CARTESIAN_POINT ( 'NONE',  ( 21.55341960407610458, 5.719274019375980345, 38.95724293864768839 ) ) ;
#48949=CARTESIAN_POINT ( 'NONE',  ( 5.153800228976335163, 19.02544592524342804, 64.79057627198102409 ) ) ;
#48950=CARTESIAN_POINT ( 'NONE',  ( -14.34966873604972548, 8.224510206698743886, 28.33442372801902209 ) ) ;
#48951=CARTESIAN_POINT ( 'NONE',  ( -19.02544592524334988, -5.153800228976617603, 68.95942372801896170 ) ) ;
#48952=CARTESIAN_POINT ( 'NONE',  ( -5.719274019375978568, 21.55341960407610458, 100.2072429386476955 ) ) ;
#48953=CARTESIAN_POINT ( 'NONE',  ( -16.52544592524342804, 4.483927247898546575, 36.04057627198102409 ) ) ;
#48954=CARTESIAN_POINT ( 'NONE',  ( 5.049401038298161559, -19.05341960407611168, 82.70724293864770971 ) ) ;
#48955=CARTESIAN_POINT ( 'NONE',  ( 18.67979575497178502, 10.72451020669898547, 64.16557627198102409 ) ) ;
#48956=CARTESIAN_POINT ( 'NONE',  ( 21.53943276465977519, -0.05219959533907433946, 98.74890960531438111 ) ) ;
#48957=CARTESIAN_POINT ( 'NONE',  ( -4.483927247898782831, 16.52544592524335698, 22.70942372801901499 ) ) ;
#48958=CARTESIAN_POINT ( 'NONE',  ( 10.81492255796078972, 18.62759615963270932, 29.58224293864769905 ) ) ;
#48959=CARTESIAN_POINT ( 'NONE',  ( -15.72974639402176322, -15.80617190586768395, 89.37609039468568994 ) ) ;
#48960=CARTESIAN_POINT ( 'NONE',  ( -13.89961937509977652, 13.97604488694528158, 80.62390960531436690 ) ) ;
#48961=CARTESIAN_POINT ( 'NONE',  ( 16.46253265017160672, -9.564922557960803928, 23.33224293864769194 ) ) ;
#48962=CARTESIAN_POINT ( 'NONE',  ( 16.46253265017160672, -9.564922557960803928, 78.33224293864769550 ) ) ;
#48963=CARTESIAN_POINT ( 'NONE',  ( 4.483927247898545687, 16.52544592524342804, 109.7905762719810383 ) ) ;
#48964=CARTESIAN_POINT ( 'NONE',  ( 5.153800228976335163, 19.02544592524342804, 64.79057627198100988 ) ) ;
#48965=CARTESIAN_POINT ( 'NONE',  ( 4.483927247898790824, -16.52544592524335698, 25.20942372801901854 ) ) ;
#48966=CARTESIAN_POINT ( 'NONE',  ( 17.49999999999998224, 3.512728167237055388, 32.27190004818874769 ) ) ;
#48967=CARTESIAN_POINT ( 'NONE',  ( 16.51473224551069308, 9.474510206698969483, 74.16557627198103830 ) ) ;
#48968=CARTESIAN_POINT ( 'NONE',  ( 15.72974639402176855, 15.80617190586768217, 101.8760903946857042 ) ) ;
#48969=CARTESIAN_POINT ( 'NONE',  ( 18.62759615963271287, -10.81492255796078972, 23.33224293864769194 ) ) ;
#48970=CARTESIAN_POINT ( 'NONE',  ( 4.379528057220092307, 16.55341960407617563, 97.29275706135234714 ) ) ;
#48972=CARTESIAN_POINT ( 'NONE',  ( 19.02544592524334988, 5.153800228976608722, 66.45942372801899012 ) ) ;
#48973=CARTESIAN_POINT ( 'NONE',  ( -21.55341960407619339, 5.719274019375674811, 113.5427570613523756 ) ) ;
#48975=CARTESIAN_POINT ( 'NONE',  ( 9.564922557960805705, 16.46253265017160317, 34.58224293864770260 ) ) ;
#48976=CARTESIAN_POINT ( 'NONE',  ( 12.14591786802309770, 12.06949235617756955, 34.37390960531435979 ) ) ;
#48978=CARTESIAN_POINT ( 'NONE',  ( -14.29746914071037622, -8.314922557961029526, 109.1677570613523613 ) ) ;
#48980=CARTESIAN_POINT ( 'NONE',  ( 4.379528057220092307, 16.55341960407617563, 87.29275706135236135 ) ) ;
#48981=CARTESIAN_POINT ( 'NONE',  ( -13.89961937509977652, 13.97604488694528158, 35.62390960531435269 ) ) ;
#48982=CARTESIAN_POINT ( 'NONE',  ( -5.719274019375665041, -21.55341960407619695, 94.79275706135234714 ) ) ;
#48983=CARTESIAN_POINT ( 'NONE',  ( 16.46253265017146816, 9.564922557961045513, 96.66775706135233293 ) ) ;
#48984=CARTESIAN_POINT ( 'NONE',  ( 18.67979575497194134, -10.72451020669871369, 80.83442372801901854 ) ) ;
#48985=CARTESIAN_POINT ( 'NONE',  ( 0.05219959533936267826, -19.03943276465977164, 55.00109039468566863 ) ) ;
#48986=CARTESIAN_POINT ( 'NONE',  ( 16.51473224551069308, 9.474510206698969483, 79.16557627198103830 ) ) ;
#48987=CARTESIAN_POINT ( 'NONE',  ( -19.02544592524342804, 5.153800228976336051, 66.04057627198103830 ) ) ;
#48989=CARTESIAN_POINT ( 'NONE',  ( -8.224510206698948167, 14.34966873604960824, 70.41557627198102409 ) ) ;
#48990=CARTESIAN_POINT ( 'NONE',  ( -5.719274019375978568, 21.55341960407610458, 65.20724293864768129 ) ) ;
#48991=CARTESIAN_POINT ( 'NONE',  ( 19.03943276465977164, -0.05219959533909143690, 43.74890960531435979 ) ) ;
#48992=CARTESIAN_POINT ( 'NONE',  ( 21.55341960407610458, 5.719274019375980345, 83.95724293864770971 ) ) ;
#48993=CARTESIAN_POINT ( 'NONE',  ( -16.53943276465976808, -0.05219959533934237506, 73.75109039468567573 ) ) ;
#48995=CARTESIAN_POINT ( 'NONE',  ( -16.51473224551069308, -9.474510206698971260, 51.66557627198102409 ) ) ;
#48996=CARTESIAN_POINT ( 'NONE',  ( -8.224510206698948167, 14.34966873604960824, 85.41557627198102409 ) ) ;
#48998=CARTESIAN_POINT ( 'NONE',  ( -5.049401038298153566, 19.05341960407611168, 45.20724293864769550 ) ) ;
#48999=CARTESIAN_POINT ( 'NONE',  ( 0.05219959533909260263, 19.03943276465977164, 24.99890960531435269 ) ) ;
#49000=CARTESIAN_POINT ( 'NONE',  ( 0.05219959533936267826, -19.03943276465977164, 65.00109039468567573 ) ) ;
#49001=CARTESIAN_POINT ( 'NONE',  ( 4.379528057220339221, -16.55341960407611168, 77.70724293864770971 ) ) ;
#49002=CARTESIAN_POINT ( 'NONE',  ( -5.823673210054431948, 21.52544592524334988, 42.70942372801901854 ) ) ;
#49004=CARTESIAN_POINT ( 'NONE',  ( 5.153800228976335163, 19.02544592524342804, 29.79057627198102409 ) ) ;
#49005=CARTESIAN_POINT ( 'NONE',  ( 10.81492255796078972, 18.62759615963270932, 99.58224293864770971 ) ) ;
#49007=CARTESIAN_POINT ( 'NONE',  ( -0.05219959533910754901, -16.53943276465976808, 82.49890960531436690 ) ) ;
#49009=CARTESIAN_POINT ( 'NONE',  ( -9.474510206698964154, 16.51473224551069663, 40.41557627198103120 ) ) ;
#49011=CARTESIAN_POINT ( 'NONE',  ( 13.89961937509957401, 13.97604488694547697, 76.87609039468566152 ) ) ;
#49012=CARTESIAN_POINT ( 'NONE',  ( 21.53943276465977519, 0.05219959533937863772, 31.25109039468568639 ) ) ;
#49013=CARTESIAN_POINT ( 'NONE',  ( -16.51473224551069308, -9.474510206698971260, 66.66557627198102409 ) ) ;
#49014=CARTESIAN_POINT ( 'NONE',  ( -16.46253265017146816, -9.564922557961047289, 59.16775706135233293 ) ) ;
#49015=CARTESIAN_POINT ( 'NONE',  ( 16.46253265017160672, -9.564922557960803928, 43.33224293864769550 ) ) ;
#49016=CARTESIAN_POINT ( 'NONE',  ( -4.379528057220328563, 16.55341960407611168, 60.20724293864768839 ) ) ;
#49017=CARTESIAN_POINT ( 'NONE',  ( -4.483927247898539470, -16.52544592524342804, 62.29057627198102409 ) ) ;
#49018=CARTESIAN_POINT ( 'NONE',  ( -19.02544592524342804, 5.153800228976336051, 71.04057627198099567 ) ) ;
#49019=CARTESIAN_POINT ( 'NONE',  ( -0.05219959533907301413, -21.53943276465977519, 102.4989096053143811 ) ) ;
#49020=CARTESIAN_POINT ( 'NONE',  ( 5.153800228976335163, 19.02544592524342804, 74.79057627198103830 ) ) ;
#49021=CARTESIAN_POINT ( 'NONE',  ( -13.97604488694547697, 13.89961937509957934, 23.12609039468565442 ) ) ;
#49022=CARTESIAN_POINT ( 'NONE',  ( 0.05219959533909260263, 19.03943276465977164, 34.99890960531435979 ) ) ;
#49023=CARTESIAN_POINT ( 'NONE',  ( -8.314922557960811034, -14.29746914071050412, 22.08224293864769194 ) ) ;
#49024=CARTESIAN_POINT ( 'NONE',  ( 16.52544592524342804, -4.483927247898539470, 98.54057627198105251 ) ) ;
#49025=CARTESIAN_POINT ( 'NONE',  ( -13.89961937509957401, -13.97604488694547875, 104.3760903946856757 ) ) ;
#49027=CARTESIAN_POINT ( 'NONE',  ( 5.823673210054444382, -21.52544592524334988, 30.20942372801902565 ) ) ;
#49028=CARTESIAN_POINT ( 'NONE',  ( -16.51473224551082808, 9.474510206698731452, 58.33442372801900433 ) ) ;
#49029=CARTESIAN_POINT ( 'NONE',  ( 16.52544592524335698, 4.483927247898782831, 111.4594237280190328 ) ) ;
#49030=CARTESIAN_POINT ( 'NONE',  ( -15.72974639402197994, 15.80617190586746368, 70.62390960531436690 ) ) ;
#49031=CARTESIAN_POINT ( 'NONE',  ( 9.474510206698971260, -16.51473224551069308, 107.9155762719810383 ) ) ;
#49032=CARTESIAN_POINT ( 'NONE',  ( -8.224510206698948167, 14.34966873604960824, 50.41557627198103120 ) ) ;
#49033=CARTESIAN_POINT ( 'NONE',  ( 9.474510206698971260, -16.51473224551069308, 27.91557627198103120 ) ) ;
#49034=CARTESIAN_POINT ( 'NONE',  ( -9.474510206698964154, 16.51473224551069663, 30.41557627198102054 ) ) ;
#49035=CARTESIAN_POINT ( 'NONE',  ( -16.46253265017146816, -9.564922557961047289, 29.16775706135232937 ) ) ;
#49036=CARTESIAN_POINT ( 'NONE',  ( -14.34966873604972548, 8.224510206698743886, 93.33442372801901854 ) ) ;
#49037=CARTESIAN_POINT ( 'NONE',  ( -10.81492255796105439, 18.62759615963255655, 42.91775706135235424 ) ) ;
#49038=CARTESIAN_POINT ( 'NONE',  ( -8.314922557961024197, 14.29746914071037800, 42.91775706135235424 ) ) ;
#49039=CARTESIAN_POINT ( 'NONE',  ( -10.81492255796078084, -18.62759615963271287, 22.08224293864769194 ) ) ;
#49040=CARTESIAN_POINT ( 'NONE',  ( -13.89961937509977652, 13.97604488694528158, 55.62390960531434558 ) ) ;
#49041=CARTESIAN_POINT ( 'NONE',  ( -10.72451020669870658, -18.67979575497194134, 94.58442372801901854 ) ) ;
#49042=CARTESIAN_POINT ( 'NONE',  ( 16.46253265017160672, -9.564922557960803928, 78.33224293864769550 ) ) ;
#49043=CARTESIAN_POINT ( 'NONE',  ( 16.52544592524335698, 4.483927247898782831, 66.45942372801903275 ) ) ;
#49044=CARTESIAN_POINT ( 'NONE',  ( 12.06949235617757843, -12.14591786802309237, 103.1239096053143811 ) ) ;
#49045=CARTESIAN_POINT ( 'NONE',  ( -12.14591786802309592, -12.06949235617757132, 21.87390960531436690 ) ) ;
#49046=CARTESIAN_POINT ( 'NONE',  ( 17.50000000000000000, -5.500000000000001776, 106.2176903769643417 ) ) ;
#49047=CARTESIAN_POINT ( 'NONE',  ( 10.81492255796106328, -18.62759615963255655, 75.41775706135233293 ) ) ;
#49048=CARTESIAN_POINT ( 'NONE',  ( -9.474510206698964154, 16.51473224551069663, 85.41557627198102409 ) ) ;
#49049=CARTESIAN_POINT ( 'NONE',  ( 16.46253265017160672, -9.564922557960803928, 83.33224293864768129 ) ) ;
#49050=CARTESIAN_POINT ( 'NONE',  ( 0.05219959533909260263, 19.03943276465977164, 109.9989096053143669 ) ) ;
#49051=CARTESIAN_POINT ( 'NONE',  ( 16.53943276465976808, -0.05219959533910856209, 63.74890960531435979 ) ) ;
#49052=CARTESIAN_POINT ( 'NONE',  ( 16.55341960407618274, -4.379528057220086978, 111.0427570613523613 ) ) ;
#49053=ORIENTED_EDGE ( 'NONE', *, *, #163318, .T. ) ;
#49054=CARTESIAN_POINT ( 'NONE',  ( 14.34966873604960469, 8.224510206698951720, 44.16557627198103120 ) ) ;
#49055=CARTESIAN_POINT ( 'NONE',  ( -14.34966873604972548, 8.224510206698743886, 38.33442372801900433 ) ) ;
#49056=CARTESIAN_POINT ( 'NONE',  ( 17.50000000000000000, 5.499999999999992895, 56.70309617465829888 ) ) ;
#49057=CARTESIAN_POINT ( 'NONE',  ( 19.05341960407617918, -5.049401038297876454, 36.04275706135234003 ) ) ;
#49058=CARTESIAN_POINT ( 'NONE',  ( 9.564922557960805705, 16.46253265017160317, 74.58224293864769550 ) ) ;
#49059=CARTESIAN_POINT ( 'NONE',  ( 19.05341960407617918, -5.049401038297876454, 56.04275706135234714 ) ) ;
#49061=CARTESIAN_POINT ( 'NONE',  ( -30.00000000000000000, -5.204748896376250896E-15, 42.49999999999999289 ) ) ;
#49062=CARTESIAN_POINT ( 'NONE',  ( -13.89961937509957401, -13.97604488694547875, 79.37609039468567573 ) ) ;
#49063=CARTESIAN_POINT ( 'NONE',  ( -14.29746914071037622, -8.314922557961029526, 79.16775706135234714 ) ) ;
#49065=CARTESIAN_POINT ( 'NONE',  ( -9.474510206698964154, 16.51473224551069663, 105.4155762719810383 ) ) ;
#49066=CARTESIAN_POINT ( 'NONE',  ( 5.719274019375673035, 21.55341960407619339, 42.29275706135235424 ) ) ;
#49067=CARTESIAN_POINT ( 'NONE',  ( -9.474510206698720793, -16.51473224551083518, 94.58442372801900433 ) ) ;
#49068=CARTESIAN_POINT ( 'NONE',  ( 17.05587630539785238, 6.762274262135713698, 86.75819690962691766 ) ) ;
#49069=CARTESIAN_POINT ( 'NONE',  ( 16.46253265017160672, -9.564922557960803928, 48.33224293864769550 ) ) ;
#49070=CARTESIAN_POINT ( 'NONE',  ( 9.564922557960805705, 16.46253265017160317, 104.5822429386476955 ) ) ;
#49071=CARTESIAN_POINT ( 'NONE',  ( 0.05219959533910956823, 16.53943276465976808, 59.99890960531436690 ) ) ;
#49072=CARTESIAN_POINT ( 'NONE',  ( -9.564922557960796823, -16.46253265017161027, 52.08224293864768839 ) ) ;
#49073=CARTESIAN_POINT ( 'NONE',  ( -0.05219959533909027116, -19.03943276465977164, 62.49890960531435979 ) ) ;
#49074=CARTESIAN_POINT ( 'NONE',  ( -5.049401038297874678, -19.05341960407617918, 59.79275706135231871 ) ) ;
#49075=CARTESIAN_POINT ( 'NONE',  ( 9.474510206698729675, 16.51473224551082808, 27.08442372801900433 ) ) ;
#49076=CARTESIAN_POINT ( 'NONE',  ( -19.05341960407611168, -5.049401038298163336, 61.45724293864769550 ) ) ;
#49077=CARTESIAN_POINT ( 'NONE',  ( 18.62759615963271287, -10.81492255796078972, 78.33224293864770971 ) ) ;
#49078=CARTESIAN_POINT ( 'NONE',  ( 8.314922557960818139, 14.29746914071049879, 64.58224293864769550 ) ) ;
#49079=CARTESIAN_POINT ( 'NONE',  ( 19.02544592524334988, 5.153800228976608722, 41.45942372801900433 ) ) ;
#49080=CARTESIAN_POINT ( 'NONE',  ( 19.02544592524343514, -5.153800228976328945, 113.5405762719810241 ) ) ;
#49081=CARTESIAN_POINT ( 'NONE',  ( -10.81492255796078084, -18.62759615963271287, 47.08224293864770260 ) ) ;
#49082=CARTESIAN_POINT ( 'NONE',  ( 21.53943276465977519, -0.05219959533907433946, 28.74890960531435624 ) ) ;
#49083=CARTESIAN_POINT ( 'NONE',  ( -19.02544592524342804, 5.153800228976336051, 71.04057627198099567 ) ) ;
#49084=CARTESIAN_POINT ( 'NONE',  ( -19.05341960407611168, -5.049401038298163336, 41.45724293864769550 ) ) ;
#49085=CARTESIAN_POINT ( 'NONE',  ( -14.29746914071049879, 8.314922557960819915, 105.8322429386476955 ) ) ;
#49086=CARTESIAN_POINT ( 'NONE',  ( 15.80617190586746368, 15.72974639402197994, 104.3739096053143669 ) ) ;
#49088=CARTESIAN_POINT ( 'NONE',  ( 21.52544592524334988, 5.823673210054432836, 21.45942372801901499 ) ) ;
#49089=CARTESIAN_POINT ( 'NONE',  ( 5.049401038298161559, -19.05341960407611168, 27.70724293864769550 ) ) ;
#49090=CARTESIAN_POINT ( 'NONE',  ( 10.72451020669898902, -18.67979575497178502, 102.9155762719810383 ) ) ;
#49091=CARTESIAN_POINT ( 'NONE',  ( 9.564922557961047289, -16.46253265017146816, 45.41775706135232582 ) ) ;
#49092=CARTESIAN_POINT ( 'NONE',  ( -19.05341960407611168, -5.049401038298163336, 21.45724293864768839 ) ) ;
#49093=CARTESIAN_POINT ( 'NONE',  ( 0.05219959533909260263, 19.03943276465977164, 29.99890960531435979 ) ) ;
#49095=CARTESIAN_POINT ( 'NONE',  ( 16.55341960407618274, -4.379528057220086978, 51.04275706135234714 ) ) ;
#49096=CARTESIAN_POINT ( 'NONE',  ( 5.049401038298161559, -19.05341960407611168, 32.70724293864768129 ) ) ;
#49098=CARTESIAN_POINT ( 'NONE',  ( -9.474510206698964154, 16.51473224551069663, 75.41557627198103830 ) ) ;
#49099=CARTESIAN_POINT ( 'NONE',  ( -0.05219959533910754901, -16.53943276465976808, 112.4989096053143669 ) ) ;
#49100=CARTESIAN_POINT ( 'NONE',  ( -18.62759615963270932, 10.81492255796079327, 50.83224293864770971 ) ) ;
#49101=CARTESIAN_POINT ( 'NONE',  ( 8.314922557960818139, 14.29746914071049879, 74.58224293864768129 ) ) ;
#49102=CARTESIAN_POINT ( 'NONE',  ( -12.06949235617739369, -12.14591786802326823, 39.37609039468567573 ) ) ;
#49103=CARTESIAN_POINT ( 'NONE',  ( 5.823673210054444382, -21.52544592524334988, 80.20942372801901854 ) ) ;
#49104=CARTESIAN_POINT ( 'NONE',  ( -0.05219959533909027116, -19.03943276465977164, 22.49890960531436690 ) ) ;
#49105=CARTESIAN_POINT ( 'NONE',  ( -8.224510206698735004, -14.34966873604973081, 109.5844237280190328 ) ) ;
#49106=CARTESIAN_POINT ( 'NONE',  ( 0.05219959533910956823, 16.53943276465976808, 54.99890960531435269 ) ) ;
#49107=CARTESIAN_POINT ( 'NONE',  ( 19.02544592524343514, -5.153800228976328945, 48.54057627198103120 ) ) ;
#49108=CARTESIAN_POINT ( 'NONE',  ( -5.823673210054431948, 21.52544592524334988, 102.7094237280190185 ) ) ;
#49109=CARTESIAN_POINT ( 'NONE',  ( -10.81492255796078084, -18.62759615963271287, 112.0822429386477097 ) ) ;
#49110=( BOUNDED_CURVE ( )  B_SPLINE_CURVE ( 2, ( #59359, #121028, #659, #45203, #107838, #198886, #31022, #60354, #106857, #27066, #77512, #139184, #62329 ),
 .UNSPECIFIED., .F., .F. ) 
 B_SPLINE_CURVE_WITH_KNOTS ( ( 3, 2, 2, 2, 2, 2, 3 ),
 ( 0.5550620153744135754, 0.5570175438596490780, 0.5614035087719297934, 0.5657894736842105088, 0.5701754385964912242, 0.5745614035087719396, 0.5764712521719174143 ),
 .UNSPECIFIED. ) 
 CURVE ( )  GEOMETRIC_REPRESENTATION_ITEM ( )  RATIONAL_B_SPLINE_CURVE ( ( 0.9831626618144004848, 0.9848076720550091867, 1.000000000000000000, 0.9659258262890683122, 1.000000000000000000, 0.9659258262890683122, 1.000000000000000000, 0.9659258262890683122, 1.000000000000000000, 0.9659258262890683122, 1.000000000000000000, 0.9851625545550091179, 0.9832469066685282089 ) ) 
 REPRESENTATION_ITEM ( '' )  );
#49111=CARTESIAN_POINT ( 'NONE',  ( -10.72451020669870658, -18.67979575497194134, 69.58442372801900433 ) ) ;
#49112=CARTESIAN_POINT ( 'NONE',  ( 16.55341960407618274, -4.379528057220086978, 46.04275706135234714 ) ) ;
#49113=CARTESIAN_POINT ( 'NONE',  ( 12.06949235617757843, -12.14591786802309237, 78.12390960531436690 ) ) ;
#49114=CARTESIAN_POINT ( 'NONE',  ( -15.72974639402176322, -15.80617190586768395, 84.37609039468570415 ) ) ;
#49115=CARTESIAN_POINT ( 'NONE',  ( 0.05219959533910956823, 16.53943276465976808, 24.99890960531435624 ) ) ;
#49118=CARTESIAN_POINT ( 'NONE',  ( 12.14591786802309770, 12.06949235617756955, 39.37390960531436690 ) ) ;
#49119=CARTESIAN_POINT ( 'NONE',  ( -0.05219959533934338120, 16.53943276465976808, 67.50109039468568994 ) ) ;
#49120=CARTESIAN_POINT ( 'NONE',  ( -5.153800228976328057, -19.02544592524343514, 92.29057627198099567 ) ) ;
#49121=CARTESIAN_POINT ( 'NONE',  ( -9.564922557960796823, -16.46253265017161027, 107.0822429386476955 ) ) ;
#49122=CARTESIAN_POINT ( 'NONE',  ( -21.53943276465977519, -0.05219959533937600094, 103.7510903946857042 ) ) ;
#49123=CARTESIAN_POINT ( 'NONE',  ( 8.314922557961029526, -14.29746914071037800, 105.4177570613523613 ) ) ;
#49124=CARTESIAN_POINT ( 'NONE',  ( 8.314922557960818139, 14.29746914071049879, 79.58224293864769550 ) ) ;
#49125=CARTESIAN_POINT ( 'NONE',  ( 13.97604488694527802, 13.89961937509977652, 79.37390960531435269 ) ) ;
#49127=CARTESIAN_POINT ( 'NONE',  ( -16.55341960407617563, 4.379528057220093196, 28.54275706135234358 ) ) ;
#49128=CARTESIAN_POINT ( 'NONE',  ( 16.46253265017160672, -9.564922557960803928, 28.33224293864769550 ) ) ;
#49129=CARTESIAN_POINT ( 'NONE',  ( 16.51473224551069308, 9.474510206698969483, 94.16557627198103830 ) ) ;
#49130=CARTESIAN_POINT ( 'NONE',  ( 14.34966873604972726, -8.224510206698740333, 30.83442372801902209 ) ) ;
#49132=CARTESIAN_POINT ( 'NONE',  ( -5.049401038297874678, -19.05341960407617918, 39.79275706135232582 ) ) ;
#49133=CARTESIAN_POINT ( 'NONE',  ( -0.05219959533934338120, 16.53943276465976808, 97.50109039468567573 ) ) ;
#49134=CARTESIAN_POINT ( 'NONE',  ( 13.97604488694548053, -13.89961937509957401, 100.6260903946856615 ) ) ;
#49135=CARTESIAN_POINT ( 'NONE',  ( -19.03943276465977164, 0.05219959533909376836, 36.24890960531436690 ) ) ;
#49136=CARTESIAN_POINT ( 'NONE',  ( -4.483927247898782831, 16.52544592524335698, 82.70942372801900433 ) ) ;
#49137=CARTESIAN_POINT ( 'NONE',  ( 16.52544592524335698, 4.483927247898782831, 61.45942372801901854 ) ) ;
#49139=CARTESIAN_POINT ( 'NONE',  ( -13.97604488694547697, 13.89961937509957934, 63.12609039468566152 ) ) ;
#49140=CARTESIAN_POINT ( 'NONE',  ( 18.67979575497194134, -10.72451020669871369, 105.8344237280190328 ) ) ;
#49141=CARTESIAN_POINT ( 'NONE',  ( 0.05219959533909260263, 19.03943276465977164, 49.99890960531435979 ) ) ;
#49142=CARTESIAN_POINT ( 'NONE',  ( 5.049401038298161559, -19.05341960407611168, 87.70724293864769550 ) ) ;
#49143=CARTESIAN_POINT ( 'NONE',  ( 12.14591786802309770, 12.06949235617756955, 79.37390960531436690 ) ) ;
#49144=CARTESIAN_POINT ( 'NONE',  ( 19.02544592524334988, 5.153800228976608722, 61.45942372801900433 ) ) ;
#49145=CARTESIAN_POINT ( 'NONE',  ( 18.67979575497178502, 10.72451020669898547, 54.16557627198103120 ) ) ;
#49146=CARTESIAN_POINT ( 'NONE',  ( 5.823673210054444382, -21.52544592524334988, 105.2094237280190328 ) ) ;
#49147=CARTESIAN_POINT ( 'NONE',  ( 13.97604488694527802, 13.89961937509977652, 94.37390960531436690 ) ) ;
#49148=CARTESIAN_POINT ( 'NONE',  ( 19.03943276465977164, 0.05219959533936151252, 21.25109039468565797 ) ) ;
#49149=CARTESIAN_POINT ( 'NONE',  ( 10.72451020669898902, -18.67979575497178502, 67.91557627198102409 ) ) ;
#49150=CARTESIAN_POINT ( 'NONE',  ( 16.51473224551069308, 9.474510206698969483, 109.1655762719810383 ) ) ;
#49151=CARTESIAN_POINT ( 'NONE',  ( 5.049401038297881783, 19.05341960407617563, 87.29275706135234714 ) ) ;
#49152=CARTESIAN_POINT ( 'NONE',  ( -17.50000000000147438, 3.254303733634575924, 110.0239589307140307 ) ) ;
#49153=CARTESIAN_POINT ( 'NONE',  ( -5.049401038297874678, -19.05341960407617918, 109.7927570613523187 ) ) ;
#49154=CARTESIAN_POINT ( 'NONE',  ( -13.89961937509977652, 13.97604488694528158, 25.62390960531434558 ) ) ;
#49155=CARTESIAN_POINT ( 'NONE',  ( 16.51473224551069308, 9.474510206698969483, 104.1655762719810241 ) ) ;
#49156=CARTESIAN_POINT ( 'NONE',  ( -5.823673210054116645, -21.52544592524344225, 82.29057627198103830 ) ) ;
#49157=CARTESIAN_POINT ( 'NONE',  ( -4.483927247898782831, 16.52544592524335698, 47.70942372801902565 ) ) ;
#49158=CARTESIAN_POINT ( 'NONE',  ( -15.80617190586768217, 15.72974639402176855, 53.12609039468568284 ) ) ;
#49159=CARTESIAN_POINT ( 'NONE',  ( -5.719274019375665041, -21.55341960407619695, 99.79275706135234714 ) ) ;
#49160=CARTESIAN_POINT ( 'NONE',  ( -4.379528057220086978, -16.55341960407618274, 99.79275706135234714 ) ) ;
#49161=CARTESIAN_POINT ( 'NONE',  ( -16.46253265017160317, 9.564922557960807481, 85.83224293864769550 ) ) ;
#49162=CARTESIAN_POINT ( 'NONE',  ( -12.14591786802309592, -12.06949235617757132, 91.87390960531436690 ) ) ;
#49163=CARTESIAN_POINT ( 'NONE',  ( -4.483927247898539470, -16.52544592524342804, 32.29057627198102409 ) ) ;
#49164=CARTESIAN_POINT ( 'NONE',  ( 9.474510206698729675, 16.51473224551082808, 72.08442372801900433 ) ) ;
#49165=CARTESIAN_POINT ( 'NONE',  ( 21.55341960407619695, -5.719274019375665929, 51.04275706135234714 ) ) ;
#49166=CARTESIAN_POINT ( 'NONE',  ( -19.03943276465977164, -0.05219959533935918106, 28.75109039468566507 ) ) ;
#49167=CARTESIAN_POINT ( 'NONE',  ( -4.483927247898539470, -16.52544592524342804, 87.29057627198103830 ) ) ;
#49168=CARTESIAN_POINT ( 'NONE',  ( 5.719274019375991003, -21.55341960407610458, 22.70724293864769194 ) ) ;
#49169=CARTESIAN_POINT ( 'NONE',  ( 4.483927247898545687, 16.52544592524342804, 29.79057627198102409 ) ) ;
#49170=CARTESIAN_POINT ( 'NONE',  ( 5.719274019375673035, 21.55341960407619339, 82.29275706135234714 ) ) ;
#49171=CARTESIAN_POINT ( 'NONE',  ( -4.379528057220086978, -16.55341960407618274, 54.79275706135235424 ) ) ;
#49172=CARTESIAN_POINT ( 'NONE',  ( 16.55341960407618274, -4.379528057220086978, 101.0427570613523756 ) ) ;
#49173=CARTESIAN_POINT ( 'NONE',  ( -18.67979575497193778, 10.72451020669871902, 53.33442372801901854 ) ) ;
#49176=CARTESIAN_POINT ( 'NONE',  ( -21.53943276465977519, -0.05219959533937600094, 28.75109039468567929 ) ) ;
#49177=CARTESIAN_POINT ( 'NONE',  ( 0.05219959533910956823, 16.53943276465976808, 104.9989096053143669 ) ) ;
#49178=CARTESIAN_POINT ( 'NONE',  ( 20.28951144177218424, -1.856485852971755390, 37.50000000000002842 ) ) ;
#49179=CARTESIAN_POINT ( 'NONE',  ( 16.52544592524342804, -4.483927247898539470, 63.54057627198103830 ) ) ;
#49180=CARTESIAN_POINT ( 'NONE',  ( -9.564922557960796823, -16.46253265017161027, 77.08224293864769550 ) ) ;
#49181=CARTESIAN_POINT ( 'NONE',  ( -4.483927247898782831, 16.52544592524335698, 107.7094237280190328 ) ) ;
#49182=CARTESIAN_POINT ( 'NONE',  ( 0.05219959533909260263, 19.03943276465977164, 39.99890960531436690 ) ) ;
#49183=CARTESIAN_POINT ( 'NONE',  ( -18.62759615963270932, 10.81492255796079327, 50.83224293864770971 ) ) ;
#49184=CARTESIAN_POINT ( 'NONE',  ( -4.379528057220328563, 16.55341960407611168, 90.20724293864770971 ) ) ;
#49185=CARTESIAN_POINT ( 'NONE',  ( 21.55341960407610458, 5.719274019375980345, 93.95724293864770971 ) ) ;
#49186=CARTESIAN_POINT ( 'NONE',  ( -16.46253265017160317, 9.564922557960807481, 105.8322429386476955 ) ) ;
#49187=CARTESIAN_POINT ( 'NONE',  ( 0.05219959533909260263, 19.03943276465977164, 54.99890960531435979 ) ) ;
#49188=CARTESIAN_POINT ( 'NONE',  ( 19.05341960407617918, -5.049401038297876454, 96.04275706135231871 ) ) ;
#49189=CARTESIAN_POINT ( 'NONE',  ( -21.55341960407610458, -5.719274019375992779, 41.45724293864769550 ) ) ;
#49190=CARTESIAN_POINT ( 'NONE',  ( 5.823673210054444382, -21.52544592524334988, 65.20942372801901854 ) ) ;
#49191=CARTESIAN_POINT ( 'NONE',  ( -0.05219959533909027116, -19.03943276465977164, 57.49890960531435979 ) ) ;
#49192=CARTESIAN_POINT ( 'NONE',  ( -16.51473224551069308, -9.474510206698971260, 91.66557627198103830 ) ) ;
#49193=CARTESIAN_POINT ( 'NONE',  ( -8.314922557961024197, 14.29746914071037800, 62.91775706135236135 ) ) ;
#49194=CARTESIAN_POINT ( 'NONE',  ( -10.81492255796105439, 18.62759615963255655, 42.91775706135235424 ) ) ;
#49195=CARTESIAN_POINT ( 'NONE',  ( 15.72974639402176855, 15.80617190586768217, 91.87609039468568994 ) ) ;
#49196=CARTESIAN_POINT ( 'NONE',  ( -15.72974639402197994, 15.80617190586746368, 100.6239096053143811 ) ) ;
#49197=CARTESIAN_POINT ( 'NONE',  ( 5.719274019375673035, 21.55341960407619339, 42.29275706135235424 ) ) ;
#49198=CARTESIAN_POINT ( 'NONE',  ( 16.55341960407618274, -4.379528057220086978, 61.04275706135234714 ) ) ;
#49199=CARTESIAN_POINT ( 'NONE',  ( -15.72974639402197994, 15.80617190586746368, 60.62390960531437401 ) ) ;
#49200=CARTESIAN_POINT ( 'NONE',  ( -19.03943276465977164, -0.05219959533935918106, 33.75109039468566863 ) ) ;
#49201=CARTESIAN_POINT ( 'NONE',  ( -5.049401038298153566, 19.05341960407611168, 70.20724293864769550 ) ) ;
#49202=CARTESIAN_POINT ( 'NONE',  ( 16.53943276465976808, 0.05219959533934440121, 111.2510903946856899 ) ) ;
#49204=CARTESIAN_POINT ( 'NONE',  ( -13.97604488694527625, -13.89961937509977652, 106.8739096053143669 ) ) ;
#49206=CARTESIAN_POINT ( 'NONE',  ( -13.89961937509957401, -13.97604488694547875, 84.37609039468567573 ) ) ;
#49207=CARTESIAN_POINT ( 'NONE',  ( -10.81492255796078084, -18.62759615963271287, 62.08224293864769550 ) ) ;
#49208=CARTESIAN_POINT ( 'NONE',  ( 14.34966873604960469, 8.224510206698951720, 39.16557627198102409 ) ) ;
#49209=CARTESIAN_POINT ( 'NONE',  ( -13.97604488694547697, 13.89961937509957934, 113.1260903946856757 ) ) ;
#49210=CARTESIAN_POINT ( 'NONE',  ( 19.05341960407611168, 5.049401038298154454, 28.95724293864769550 ) ) ;
#49211=CARTESIAN_POINT ( 'NONE',  ( -9.474510206698720793, -16.51473224551083518, 109.5844237280190043 ) ) ;
#49212=CARTESIAN_POINT ( 'NONE',  ( 21.52544592524344225, -5.823673210054117533, 98.54057627198105251 ) ) ;
#49213=CARTESIAN_POINT ( 'NONE',  ( 16.51473224551083163, -9.474510206698727899, 75.83442372801900433 ) ) ;
#49214=CARTESIAN_POINT ( 'NONE',  ( 4.483927247898790824, -16.52544592524335698, 85.20942372801901854 ) ) ;
#49215=CARTESIAN_POINT ( 'NONE',  ( -13.97604488694527625, -13.89961937509977652, 66.87390960531436690 ) ) ;
#49216=CARTESIAN_POINT ( 'NONE',  ( -16.52544592524342804, 4.483927247898546575, 76.04057627198102409 ) ) ;
#49217=CARTESIAN_POINT ( 'NONE',  ( -16.46253265017160317, 9.564922557960807481, 50.83224293864770260 ) ) ;
#49218=CARTESIAN_POINT ( 'NONE',  ( 16.55341960407611168, 4.379528057220329451, 53.95724293864770260 ) ) ;
#49221=CARTESIAN_POINT ( 'NONE',  ( 14.34966873604960469, 8.224510206698951720, 24.16557627198103120 ) ) ;
#49222=CARTESIAN_POINT ( 'NONE',  ( -16.46253265017160317, 9.564922557960807481, 80.83224293864769550 ) ) ;
#49224=CARTESIAN_POINT ( 'NONE',  ( -5.153800228976607833, 19.02544592524334988, 37.70942372801899722 ) ) ;
#49225=CARTESIAN_POINT ( 'NONE',  ( -12.06949235617739369, -12.14591786802326823, 44.37609039468567573 ) ) ;
#49226=CARTESIAN_POINT ( 'NONE',  ( 15.80617190586746368, 15.72974639402197994, 59.37390960531436690 ) ) ;
#49227=CARTESIAN_POINT ( 'NONE',  ( -5.153800228976607833, 19.02544592524334988, 27.70942372801899722 ) ) ;
#49228=CARTESIAN_POINT ( 'NONE',  ( 19.05341960407611168, 5.049401038298154454, 68.95724293864769550 ) ) ;
#49230=CARTESIAN_POINT ( 'NONE',  ( -19.03943276465977164, 0.05219959533909376836, 111.2489096053143669 ) ) ;
#49231=CARTESIAN_POINT ( 'NONE',  ( -18.62759615963255300, -10.81492255796106328, 34.16775706135234714 ) ) ;
#49232=CARTESIAN_POINT ( 'NONE',  ( -0.05219959533910754901, -16.53943276465976808, 107.4989096053143669 ) ) ;
#49233=CARTESIAN_POINT ( 'NONE',  ( 0.05219959533907565091, 21.53943276465977519, 94.99890960531436690 ) ) ;
#49234=CARTESIAN_POINT ( 'NONE',  ( -13.97604488694527625, -13.89961937509977652, 76.87390960531433848 ) ) ;
#49236=CARTESIAN_POINT ( 'NONE',  ( 5.719274019375673035, 21.55341960407619339, 27.29275706135234358 ) ) ;
#49238=CARTESIAN_POINT ( 'NONE',  ( -16.51473224551069308, -9.474510206698971260, 86.66557627198102409 ) ) ;
#49239=CARTESIAN_POINT ( 'NONE',  ( 19.46398650005391318, -5.499999999999942268, 82.68269651486370719 ) ) ;
#49240=CARTESIAN_POINT ( 'NONE',  ( 5.153800228976335163, 19.02544592524342804, 39.79057627198100988 ) ) ;
#49241=CARTESIAN_POINT ( 'NONE',  ( 16.51473224551083163, -9.474510206698727899, 105.8344237280190043 ) ) ;
#49243=CARTESIAN_POINT ( 'NONE',  ( -0.05219959533909027116, -19.03943276465977164, 22.49890960531436690 ) ) ;
#49244=CARTESIAN_POINT ( 'NONE',  ( 21.55341960407619695, -5.719274019375665929, 91.04275706135236135 ) ) ;
#49245=CARTESIAN_POINT ( 'NONE',  ( 9.474510206698971260, -16.51473224551069308, 77.91557627198103830 ) ) ;
#49246=CARTESIAN_POINT ( 'NONE',  ( 15.72974639402176855, 15.80617190586768217, 51.87609039468568284 ) ) ;
#49247=CARTESIAN_POINT ( 'NONE',  ( -21.53943276465977519, -0.05219959533937600094, 23.75109039468567929 ) ) ;
#49249=CARTESIAN_POINT ( 'NONE',  ( -13.97604488694527625, -13.89961937509977652, 91.87390960531432427 ) ) ;
#49251=CARTESIAN_POINT ( 'NONE',  ( -14.34966873604972548, 8.224510206698743886, 33.33442372801900433 ) ) ;
#49252=CARTESIAN_POINT ( 'NONE',  ( -0.05219959533907301413, -21.53943276465977519, 47.49890960531435979 ) ) ;
#49253=CARTESIAN_POINT ( 'NONE',  ( 18.62759615963255655, 10.81492255796105972, 81.66775706135236135 ) ) ;
#49254=CARTESIAN_POINT ( 'NONE',  ( -17.49999999999999645, -5.500000000000000888, 24.20309617465829533 ) ) ;
#49255=CARTESIAN_POINT ( 'NONE',  ( -19.05341960407617563, 5.049401038297882671, 113.5427570613523471 ) ) ;
#49256=CARTESIAN_POINT ( 'NONE',  ( 0.05219959533909260263, 19.03943276465977164, 59.99890960531436690 ) ) ;
#49257=CARTESIAN_POINT ( 'NONE',  ( 13.97604488694527802, 13.89961937509977652, 84.37390960531433848 ) ) ;
#49258=CARTESIAN_POINT ( 'NONE',  ( -14.34966873604960291, -8.224510206698953496, 111.6655762719810525 ) ) ;
#49259=CARTESIAN_POINT ( 'NONE',  ( -4.379528057220328563, 16.55341960407611168, 110.2072429386477239 ) ) ;
#49260=CARTESIAN_POINT ( 'NONE',  ( -0.05219959533909027116, -19.03943276465977164, 107.4989096053143527 ) ) ;
#49261=CARTESIAN_POINT ( 'NONE',  ( 14.29746914071037800, 8.314922557961029526, 76.66775706135234714 ) ) ;
#49262=CARTESIAN_POINT ( 'NONE',  ( -4.379528057220328563, 16.55341960407611168, 55.20724293864770260 ) ) ;
#49263=CARTESIAN_POINT ( 'NONE',  ( -16.51473224551069308, -9.474510206698971260, 56.66557627198103120 ) ) ;
#49264=CARTESIAN_POINT ( 'NONE',  ( 18.62759615963255655, 10.81492255796105972, 81.66775706135236135 ) ) ;
#49265=CARTESIAN_POINT ( 'NONE',  ( 5.823673210054444382, -21.52544592524334988, 75.20942372801901854 ) ) ;
#49266=CARTESIAN_POINT ( 'NONE',  ( 13.97604488694548053, -13.89961937509957401, 90.62609039468567573 ) ) ;
#49267=CARTESIAN_POINT ( 'NONE',  ( -14.29746914071049879, 8.314922557960819915, 65.83224293864769550 ) ) ;
#49268=CARTESIAN_POINT ( 'NONE',  ( -21.53943276465977519, 0.05219959533907696930, 116.2489096053143669 ) ) ;
#49269=CARTESIAN_POINT ( 'NONE',  ( -18.67979575497178146, -10.72451020669898902, 61.66557627198103120 ) ) ;
#49272=CARTESIAN_POINT ( 'NONE',  ( -5.049401038298153566, 19.05341960407611168, 65.20724293864765286 ) ) ;
#49273=CARTESIAN_POINT ( 'NONE',  ( 8.314922557960818139, 14.29746914071049879, 34.58224293864770260 ) ) ;
#49274=CARTESIAN_POINT ( 'NONE',  ( 14.34966873604972726, -8.224510206698740333, 110.8344237280190043 ) ) ;
#49275=CARTESIAN_POINT ( 'NONE',  ( 16.53943276465976808, 0.05219959533934440121, 96.25109039468568994 ) ) ;
#49276=CARTESIAN_POINT ( 'NONE',  ( -5.049401038297874678, -19.05341960407617918, 49.79275706135231871 ) ) ;
#49278=CARTESIAN_POINT ( 'NONE',  ( -16.46253265017160317, 9.564922557960807481, 95.83224293864769550 ) ) ;
#49279=CARTESIAN_POINT ( 'NONE',  ( 16.53943276465976808, -0.05219959533910856209, 58.74890960531436690 ) ) ;
#49281=CARTESIAN_POINT ( 'NONE',  ( -5.823673210054116645, -21.52544592524344225, 22.29057627198102765 ) ) ;
#49282=CARTESIAN_POINT ( 'NONE',  ( 10.72451020669898902, -18.67979575497178502, 47.91557627198102409 ) ) ;
#49283=VERTEX_POINT ( 'NONE', #71680 ) ;
#49284=CARTESIAN_POINT ( 'NONE',  ( -0.05219959533910754901, -16.53943276465976808, 92.49890960531436690 ) ) ;
#49285=CARTESIAN_POINT ( 'NONE',  ( 16.55341960407618274, -4.379528057220086978, 51.04275706135234714 ) ) ;
#49286=CARTESIAN_POINT ( 'NONE',  ( 16.52544592524342804, -4.483927247898539470, 83.54057627198102409 ) ) ;
#49287=CARTESIAN_POINT ( 'NONE',  ( -19.52837319214027900, 5.499999999999901412, 64.60471352585541638 ) ) ;
#49288=CARTESIAN_POINT ( 'NONE',  ( 19.03943276465977164, 0.05219959533936151252, 76.25109039468566152 ) ) ;
#49289=CARTESIAN_POINT ( 'NONE',  ( 0.05219959533909260263, 19.03943276465977164, 114.9989096053143669 ) ) ;
#49291=CARTESIAN_POINT ( 'NONE',  ( 16.46253265017160672, -9.564922557960803928, 43.33224293864769550 ) ) ;
#49292=CARTESIAN_POINT ( 'NONE',  ( -8.224510206698735004, -14.34966873604973081, 39.58442372801901143 ) ) ;
#49293=CARTESIAN_POINT ( 'NONE',  ( -16.52544592524342804, 4.483927247898546575, 36.04057627198102409 ) ) ;
#49294=CARTESIAN_POINT ( 'NONE',  ( 5.719274019375991003, -21.55341960407610458, 52.70724293864769550 ) ) ;
#49295=CARTESIAN_POINT ( 'NONE',  ( -19.02544592524334988, -5.153800228976617603, 78.95942372801900433 ) ) ;
#49296=CARTESIAN_POINT ( 'NONE',  ( -15.80617190586745835, -15.72974639402198527, 46.87390960531435979 ) ) ;
#49297=CARTESIAN_POINT ( 'NONE',  ( 10.81492255796106328, -18.62759615963255655, 85.41775706135236135 ) ) ;
#49299=CARTESIAN_POINT ( 'NONE',  ( 4.379528057220092307, 16.55341960407617563, 32.29275706135235424 ) ) ;
#49300=CARTESIAN_POINT ( 'NONE',  ( -19.02544592524342804, 5.153800228976336051, 36.04057627198100988 ) ) ;
#49301=CARTESIAN_POINT ( 'NONE',  ( -16.46253265017160317, 9.564922557960807481, 85.83224293864769550 ) ) ;
#49303=CARTESIAN_POINT ( 'NONE',  ( -0.05219959533909027116, -19.03943276465977164, 37.49890960531436690 ) ) ;
#49304=CARTESIAN_POINT ( 'NONE',  ( 14.34966873604960469, 8.224510206698951720, 99.16557627198100988 ) ) ;
#49305=CARTESIAN_POINT ( 'NONE',  ( 5.153800228976335163, 19.02544592524342804, 104.7905762719809957 ) ) ;
#49306=VERTEX_POINT ( 'NONE', #36333 ) ;
#49307=CARTESIAN_POINT ( 'NONE',  ( -16.53943276465976808, -0.05219959533934237506, 58.75109039468568994 ) ) ;
#49308=CARTESIAN_POINT ( 'NONE',  ( 15.72974639402199770, -15.80617190586745480, 93.12390960531436690 ) ) ;
#49309=CARTESIAN_POINT ( 'NONE',  ( 9.564922557960805705, 16.46253265017160317, 39.58224293864768839 ) ) ;
#49310=CARTESIAN_POINT ( 'NONE',  ( 18.67979575497194134, -10.72451020669871369, 25.83442372801901499 ) ) ;
#49311=CARTESIAN_POINT ( 'NONE',  ( -9.564922557960796823, -16.46253265017161027, 77.08224293864769550 ) ) ;
#49312=CARTESIAN_POINT ( 'NONE',  ( 19.02544592524343514, -5.153800228976328945, 108.5405762719810383 ) ) ;
#49314=CARTESIAN_POINT ( 'NONE',  ( 0.05219959533934541429, -16.53943276465976808, 30.00109039468568284 ) ) ;
#49315=CARTESIAN_POINT ( 'NONE',  ( -18.62759615963270932, 10.81492255796079327, 110.8322429386476955 ) ) ;
#49316=CARTESIAN_POINT ( 'NONE',  ( 16.52544592524342804, -4.483927247898539470, 108.5405762719810241 ) ) ;
#49317=CARTESIAN_POINT ( 'NONE',  ( 5.153800228976335163, 19.02544592524342804, 99.79057627198102409 ) ) ;
#49318=CARTESIAN_POINT ( 'NONE',  ( -19.05341960407617563, 5.049401038297882671, 68.54275706135230450 ) ) ;
#49319=CARTESIAN_POINT ( 'NONE',  ( 0.05219959533936267826, -19.03943276465977164, 25.00109039468566152 ) ) ;
#49320=CARTESIAN_POINT ( 'NONE',  ( -18.67979575497178146, -10.72451020669898902, 91.66557627198103830 ) ) ;
#49321=CARTESIAN_POINT ( 'NONE',  ( -13.97604488694547697, 13.89961937509957934, 28.12609039468565797 ) ) ;
#49322=CARTESIAN_POINT ( 'NONE',  ( 14.34966873604972726, -8.224510206698740333, 80.83442372801901854 ) ) ;
#49323=CARTESIAN_POINT ( 'NONE',  ( 9.564922557960805705, 16.46253265017160317, 104.5822429386476955 ) ) ;
#49324=CARTESIAN_POINT ( 'NONE',  ( -19.02544592524342804, 5.153800228976336051, 51.04057627198103120 ) ) ;
#49325=CARTESIAN_POINT ( 'NONE',  ( 21.52544592524334988, 5.823673210054432836, 56.45942372801902565 ) ) ;
#49326=CARTESIAN_POINT ( 'NONE',  ( -15.80617190586768217, 15.72974639402176855, 68.12609039468567573 ) ) ;
#49327=CARTESIAN_POINT ( 'NONE',  ( 0.05219959533909260263, 19.03943276465977164, 69.99890960531435269 ) ) ;
#49328=CARTESIAN_POINT ( 'NONE',  ( 5.823673210054444382, -21.52544592524334988, 55.20942372801902565 ) ) ;
#49329=CARTESIAN_POINT ( 'NONE',  ( 13.89961937509957401, 13.97604488694547697, 86.87609039468567573 ) ) ;
#49330=CARTESIAN_POINT ( 'NONE',  ( 0.05219959533909260263, 19.03943276465977164, 54.99890960531435979 ) ) ;
#49331=CARTESIAN_POINT ( 'NONE',  ( 4.483927247898790824, -16.52544592524335698, 90.20942372801903275 ) ) ;
#49332=CARTESIAN_POINT ( 'NONE',  ( -19.02544592524342804, 5.153800228976336051, 71.04057627198099567 ) ) ;
#49333=CARTESIAN_POINT ( 'NONE',  ( 16.51473224551069308, 9.474510206698969483, 54.16557627198103120 ) ) ;
#49334=CARTESIAN_POINT ( 'NONE',  ( -10.81492255796078084, -18.62759615963271287, 92.08224293864769550 ) ) ;
#49335=CARTESIAN_POINT ( 'NONE',  ( -8.224510206698735004, -14.34966873604973081, 74.58442372801901854 ) ) ;
#49337=CARTESIAN_POINT ( 'NONE',  ( 9.564922557961047289, -16.46253265017146816, 25.41775706135234003 ) ) ;
#49338=CARTESIAN_POINT ( 'NONE',  ( 5.153800228976335163, 19.02544592524342804, 69.79057627198103830 ) ) ;
#49339=CARTESIAN_POINT ( 'NONE',  ( 8.314922557960818139, 14.29746914071049879, 54.58224293864769550 ) ) ;
#49340=CARTESIAN_POINT ( 'NONE',  ( -12.06949235617756955, 12.14591786802309770, 90.62390960531436690 ) ) ;
#49341=CARTESIAN_POINT ( 'NONE',  ( -13.89961937509977652, 13.97604488694528158, 95.62390960531436690 ) ) ;
#49342=CARTESIAN_POINT ( 'NONE',  ( -16.46253265017160317, 9.564922557960807481, 95.83224293864769550 ) ) ;
#49343=CARTESIAN_POINT ( 'NONE',  ( -15.72974639402176322, -15.80617190586768395, 49.37609039468569705 ) ) ;
#49344=CARTESIAN_POINT ( 'NONE',  ( -13.97604488694527625, -13.89961937509977652, 106.8739096053143669 ) ) ;
#49345=CARTESIAN_POINT ( 'NONE',  ( 16.51473224551083163, -9.474510206698727899, 20.83442372801899722 ) ) ;
#49346=CARTESIAN_POINT ( 'NONE',  ( -16.52544592524335698, -4.483927247898792601, 73.95942372801901854 ) ) ;
#49347=CARTESIAN_POINT ( 'NONE',  ( 21.53943276465977519, 0.05219959533937863772, 41.25109039468568284 ) ) ;
#49348=CARTESIAN_POINT ( 'NONE',  ( -18.67979575497178146, -10.72451020669898902, 36.66557627198103120 ) ) ;
#49349=CARTESIAN_POINT ( 'NONE',  ( -10.81492255796078084, -18.62759615963271287, 97.08224293864770971 ) ) ;
#49350=CARTESIAN_POINT ( 'NONE',  ( -14.29746914071049879, 8.314922557960819915, 55.83224293864770260 ) ) ;
#49351=CARTESIAN_POINT ( 'NONE',  ( -19.02544592524342804, 5.153800228976336051, 61.04057627198103120 ) ) ;
#49352=CARTESIAN_POINT ( 'NONE',  ( -16.53943276465976808, 0.05219959533911058130, 81.24890960531436690 ) ) ;
#49353=CARTESIAN_POINT ( 'NONE',  ( -0.05219959533907301413, -21.53943276465977519, 37.49890960531436690 ) ) ;
#49354=CARTESIAN_POINT ( 'NONE',  ( -13.97604488694547697, 13.89961937509957934, 43.12609039468566152 ) ) ;
#49355=CARTESIAN_POINT ( 'NONE',  ( -16.55341960407611168, -4.379528057220339221, 111.4572429386476813 ) ) ;
#49357=CARTESIAN_POINT ( 'NONE',  ( -0.05219959533934338120, 16.53943276465976808, 67.50109039468568994 ) ) ;
#49358=CARTESIAN_POINT ( 'NONE',  ( -16.46253265017160317, 9.564922557960807481, 65.83224293864769550 ) ) ;
#49360=CARTESIAN_POINT ( 'NONE',  ( 16.52544592524342804, -4.483927247898539470, 88.54057627198103830 ) ) ;
#49361=CARTESIAN_POINT ( 'NONE',  ( -10.72451020669898014, 18.67979575497178502, 40.41557627198103120 ) ) ;
#49362=CARTESIAN_POINT ( 'NONE',  ( 16.52544592524335698, 4.483927247898782831, 111.4594237280190328 ) ) ;
#49363=CARTESIAN_POINT ( 'NONE',  ( -19.05341960407617563, 5.049401038297882671, 103.5427570613523329 ) ) ;
#49364=CARTESIAN_POINT ( 'NONE',  ( 5.719274019375673035, 21.55341960407619339, 82.29275706135234714 ) ) ;
#49365=CARTESIAN_POINT ( 'NONE',  ( 0.05219959533909260263, 19.03943276465977164, 84.99890960531436690 ) ) ;
#49366=CARTESIAN_POINT ( 'NONE',  ( -18.62759615963270932, 10.81492255796079327, 110.8322429386476955 ) ) ;
#49367=CARTESIAN_POINT ( 'NONE',  ( 8.314922557961029526, -14.29746914071037800, 50.41775706135235424 ) ) ;
#49368=CARTESIAN_POINT ( 'NONE',  ( -19.02544592524342804, 5.153800228976336051, 36.04057627198100988 ) ) ;
#49371=CARTESIAN_POINT ( 'NONE',  ( 8.314922557961029526, -14.29746914071037800, 35.41775706135234003 ) ) ;
#49372=CARTESIAN_POINT ( 'NONE',  ( 16.51473224551083163, -9.474510206698727899, 95.83442372801900433 ) ) ;
#49373=CARTESIAN_POINT ( 'NONE',  ( 21.53943276465977519, -0.05219959533907433946, 88.74890960531436690 ) ) ;
#49374=CARTESIAN_POINT ( 'NONE',  ( -9.474510206698720793, -16.51473224551083518, 54.58442372801899722 ) ) ;
#49376=CARTESIAN_POINT ( 'NONE',  ( -10.72451020669898014, 18.67979575497178502, 100.4155762719810241 ) ) ;
#49378=CARTESIAN_POINT ( 'NONE',  ( -5.049401038298153566, 19.05341960407611168, 75.20724293864769550 ) ) ;
#49379=CARTESIAN_POINT ( 'NONE',  ( 4.379528057220092307, 16.55341960407617563, 37.29275706135235424 ) ) ;
#49380=CARTESIAN_POINT ( 'NONE',  ( -18.22780087662123805, 5.499999999999981348, 96.01763182126897789 ) ) ;
#49381=CARTESIAN_POINT ( 'NONE',  ( 19.02544592524334988, 5.153800228976608722, 66.45942372801899012 ) ) ;
#49382=CARTESIAN_POINT ( 'NONE',  ( -15.72974639402197994, 15.80617190586746368, 115.6239096053143669 ) ) ;
#49383=CARTESIAN_POINT ( 'NONE',  ( 16.55341960407611168, 4.379528057220329451, 63.95724293864770260 ) ) ;
#49384=CARTESIAN_POINT ( 'NONE',  ( 9.564922557960805705, 16.46253265017160317, 69.58224293864770971 ) ) ;
#49385=CARTESIAN_POINT ( 'NONE',  ( -8.224510206698735004, -14.34966873604973081, 34.58442372801900433 ) ) ;
#49386=CARTESIAN_POINT ( 'NONE',  ( -0.05219959533936034679, 19.03943276465977164, 47.50109039468566863 ) ) ;
#49387=CARTESIAN_POINT ( 'NONE',  ( -21.55341960407619339, 5.719274019375674811, 48.54275706135234714 ) ) ;
#49388=CARTESIAN_POINT ( 'NONE',  ( -5.153800228976607833, 19.02544592524334988, 102.7094237280189759 ) ) ;
#49389=CARTESIAN_POINT ( 'NONE',  ( 9.564922557960805705, 16.46253265017160317, 49.58224293864770260 ) ) ;
#49390=CARTESIAN_POINT ( 'NONE',  ( -13.97604488694547697, 13.89961937509957934, 83.12609039468564731 ) ) ;
#49391=CARTESIAN_POINT ( 'NONE',  ( 0.05219959533937995610, -21.53943276465977519, 90.00109039468567573 ) ) ;
#49392=CARTESIAN_POINT ( 'NONE',  ( -13.97604488694547697, 13.89961937509957934, 63.12609039468566152 ) ) ;
#49393=CARTESIAN_POINT ( 'NONE',  ( 19.02544592524343514, -5.153800228976328945, 38.54057627198103120 ) ) ;
#49394=CARTESIAN_POINT ( 'NONE',  ( -5.823673210054116645, -21.52544592524344225, 52.29057627198102409 ) ) ;
#49395=CARTESIAN_POINT ( 'NONE',  ( -0.05219959533910754901, -16.53943276465976808, 67.49890960531436690 ) ) ;
#49396=CARTESIAN_POINT ( 'NONE',  ( 16.51473224551083163, -9.474510206698727899, 65.83442372801900433 ) ) ;
#49398=CARTESIAN_POINT ( 'NONE',  ( 16.46253265017146816, 9.564922557961045513, 31.66775706135232937 ) ) ;
#49399=CARTESIAN_POINT ( 'NONE',  ( 8.224510206698742110, 14.34966873604972548, 92.08442372801901854 ) ) ;
#49400=CARTESIAN_POINT ( 'NONE',  ( 14.34966873604960469, 8.224510206698951720, 59.16557627198103120 ) ) ;
#49401=CARTESIAN_POINT ( 'NONE',  ( -5.823673210054431948, 21.52544592524334988, 82.70942372801900433 ) ) ;
#49403=CARTESIAN_POINT ( 'NONE',  ( -15.72974639402197994, 15.80617190586746368, 100.6239096053143811 ) ) ;
#49404=CARTESIAN_POINT ( 'NONE',  ( 16.46253265017160672, -9.564922557960803928, 48.33224293864769550 ) ) ;
#49405=CARTESIAN_POINT ( 'NONE',  ( -10.72451020669870658, -18.67979575497194134, 64.58442372801900433 ) ) ;
#49406=CARTESIAN_POINT ( 'NONE',  ( -13.89961937509977652, 13.97604488694528158, 45.62390960531433848 ) ) ;
#49407=EDGE_LOOP ( 'NONE', ( #187767, #6471, #4772, #33611 ) ) ;
#49408=CARTESIAN_POINT ( 'NONE',  ( 5.049401038298161559, -19.05341960407611168, 67.70724293864769550 ) ) ;
#49409=CARTESIAN_POINT ( 'NONE',  ( -16.53943276465976808, 0.05219959533911058130, 111.2489096053143669 ) ) ;
#49410=CARTESIAN_POINT ( 'NONE',  ( 18.62759615963271287, -10.81492255796078972, 23.33224293864769194 ) ) ;
#49411=CARTESIAN_POINT ( 'NONE',  ( 4.483927247898545687, 16.52544592524342804, 54.79057627198104541 ) ) ;
#49412=CARTESIAN_POINT ( 'NONE',  ( 0.05219959533909260263, 19.03943276465977164, 29.99890960531435979 ) ) ;
#49413=CARTESIAN_POINT ( 'NONE',  ( 0.05219959533910956823, 16.53943276465976808, 84.99890960531436690 ) ) ;
#49414=CARTESIAN_POINT ( 'NONE',  ( 10.72451020669898902, -18.67979575497178502, 102.9155762719810383 ) ) ;
#49415=B_SPLINE_CURVE_WITH_KNOTS ( 'NONE', 3,
 ( #4229, #65908, #98216, #99234, #80088, #52733, #174108, #36561, #127581, #5224, #35578, #82050, #159919, #21408, #156940, #114400, #144740, #176101, #160921, #95257 ),
 .UNSPECIFIED., .F., .F.,
 ( 4, 2, 2, 2, 2, 2, 2, 2, 2, 4 ),
 ( 0.004000878361812020695, 0.004499404418916028853, 0.004997930476020036143, 0.005496456533124044301, 0.005994982590228051592, 0.006244245618780055671, 0.006493508647332038933, 0.006992034704436043621, 0.007490560761540048310, 0.007989086818644052998 ),
 .UNSPECIFIED. ) ;
#49416=CARTESIAN_POINT ( 'NONE',  ( -10.81492255796105439, 18.62759615963255655, 37.91775706135235424 ) ) ;
#49417=CARTESIAN_POINT ( 'NONE',  ( 16.46253265017160672, -9.564922557960803928, 23.33224293864769194 ) ) ;
#49418=CARTESIAN_POINT ( 'NONE',  ( -4.379528057220086978, -16.55341960407618274, 39.79275706135235424 ) ) ;
#49419=CARTESIAN_POINT ( 'NONE',  ( 15.80617190586746368, 15.72974639402197994, 89.37390960531435269 ) ) ;
#49420=CARTESIAN_POINT ( 'NONE',  ( -13.89961937509957401, -13.97604488694547875, 19.37609039468566507 ) ) ;
#49421=CARTESIAN_POINT ( 'NONE',  ( 19.05341960407611168, 5.049401038298154454, 88.95724293864769550 ) ) ;
#49422=CARTESIAN_POINT ( 'NONE',  ( -10.72451020669870658, -18.67979575497194134, 44.58442372801901854 ) ) ;
#49424=CARTESIAN_POINT ( 'NONE',  ( 0.05219959533907565091, 21.53943276465977519, 29.99890960531435979 ) ) ;
#49425=CARTESIAN_POINT ( 'NONE',  ( 16.53943276465976808, 0.05219959533934440121, 101.2510903946856757 ) ) ;
#49426=CARTESIAN_POINT ( 'NONE',  ( 21.53943276465977519, 0.05219959533937863772, 56.25109039468568284 ) ) ;
#49427=CARTESIAN_POINT ( 'NONE',  ( -21.52544592524334988, -5.823673210054445271, 83.95942372801900433 ) ) ;
#49428=CARTESIAN_POINT ( 'NONE',  ( 5.049401038297881783, 19.05341960407617563, 27.29275706135232937 ) ) ;
#49429=CARTESIAN_POINT ( 'NONE',  ( 8.224510206698742110, 14.34966873604972548, 87.08442372801901854 ) ) ;
#49430=CARTESIAN_POINT ( 'NONE',  ( 5.823673210054444382, -21.52544592524334988, 40.20942372801901854 ) ) ;
#49431=CARTESIAN_POINT ( 'NONE',  ( -19.05341960407611168, -5.049401038298163336, 51.45724293864770260 ) ) ;
#49432=CARTESIAN_POINT ( 'NONE',  ( 21.53943276465977519, 0.05219959533937863772, 101.2510903946856757 ) ) ;
#49433=CARTESIAN_POINT ( 'NONE',  ( -19.03943276465977164, 0.05219959533909376836, 106.2489096053143669 ) ) ;
#49434=CARTESIAN_POINT ( 'NONE',  ( -21.52544592524334988, -5.823673210054445271, 23.95942372801901143 ) ) ;
#49435=CARTESIAN_POINT ( 'NONE',  ( 15.72974639402199770, -15.80617190586745480, 78.12390960531436690 ) ) ;
#49437=CARTESIAN_POINT ( 'NONE',  ( -10.72451020669898014, 18.67979575497178502, 65.41557627198102409 ) ) ;
#49438=CARTESIAN_POINT ( 'NONE',  ( 16.55341960407618274, -4.379528057220086978, 51.04275706135234714 ) ) ;
#49439=CARTESIAN_POINT ( 'NONE',  ( -16.55341960407611168, -4.379528057220339221, 61.45724293864770260 ) ) ;
#49440=CARTESIAN_POINT ( 'NONE',  ( -0.05219959533936034679, 19.03943276465977164, 87.50109039468567573 ) ) ;
#49442=CARTESIAN_POINT ( 'NONE',  ( 8.224510206698742110, 14.34966873604972548, 32.08442372801901854 ) ) ;
#49443=CARTESIAN_POINT ( 'NONE',  ( -18.62759615963270932, 10.81492255796079327, 100.8322429386477097 ) ) ;
#49444=CARTESIAN_POINT ( 'NONE',  ( -21.55341960407610458, -5.719274019375992779, 71.45724293864769550 ) ) ;
#49445=CARTESIAN_POINT ( 'NONE',  ( 19.02544592524343514, -5.153800228976328945, 108.5405762719810383 ) ) ;
#49446=CARTESIAN_POINT ( 'NONE',  ( 16.52544592524335698, 4.483927247898782831, 61.45942372801901854 ) ) ;
#49447=CARTESIAN_POINT ( 'NONE',  ( -5.153800228976328057, -19.02544592524343514, 77.29057627198099567 ) ) ;
#49448=CARTESIAN_POINT ( 'NONE',  ( -21.55341960407619339, 5.719274019375674811, 48.54275706135234714 ) ) ;
#49449=CARTESIAN_POINT ( 'NONE',  ( -16.46253265017146816, -9.564922557961047289, 109.1677570613523471 ) ) ;
#49450=CARTESIAN_POINT ( 'NONE',  ( -0.05219959533909027116, -19.03943276465977164, 102.4989096053143669 ) ) ;
#49452=CARTESIAN_POINT ( 'NONE',  ( 16.51473224551069308, 9.474510206698969483, 99.16557627198102409 ) ) ;
#49453=CARTESIAN_POINT ( 'NONE',  ( 0.05219959533907565091, 21.53943276465977519, 104.9989096053143669 ) ) ;
#49454=CARTESIAN_POINT ( 'NONE',  ( -13.97604488694527625, -13.89961937509977652, 61.87390960531435979 ) ) ;
#49455=FACE_OUTER_BOUND ( 'NONE', #173897, .T. ) ;
#49456=CARTESIAN_POINT ( 'NONE',  ( -16.52544592524342804, 4.483927247898546575, 76.04057627198102409 ) ) ;
#49457=CARTESIAN_POINT ( 'NONE',  ( -21.55341960407610458, -5.719274019375992779, 21.45724293864769550 ) ) ;
#49458=CARTESIAN_POINT ( 'NONE',  ( 13.97604488694527802, 13.89961937509977652, 24.37390960531435624 ) ) ;
#49459=CARTESIAN_POINT ( 'NONE',  ( 18.62759615963271287, -10.81492255796078972, 108.3322429386477097 ) ) ;
#49460=CARTESIAN_POINT ( 'NONE',  ( -16.46253265017146816, -9.564922557961047289, 59.16775706135233293 ) ) ;
#49461=CARTESIAN_POINT ( 'NONE',  ( 10.72451020669898902, -18.67979575497178502, 22.91557627198102765 ) ) ;
#49462=CARTESIAN_POINT ( 'NONE',  ( 19.05341960407611168, 5.049401038298154454, 23.95724293864769194 ) ) ;
#49463=CARTESIAN_POINT ( 'NONE',  ( -15.80617190586745835, -15.72974639402198527, 56.87390960531436690 ) ) ;
#49464=CARTESIAN_POINT ( 'NONE',  ( -9.564922557960796823, -16.46253265017161027, 102.0822429386477097 ) ) ;
#49465=CARTESIAN_POINT ( 'NONE',  ( -5.823673210054431948, 21.52544592524334988, 77.70942372801900433 ) ) ;
#49466=CARTESIAN_POINT ( 'NONE',  ( -5.049401038298153566, 19.05341960407611168, 45.20724293864769550 ) ) ;
#49467=CARTESIAN_POINT ( 'NONE',  ( -12.14591786802309592, -12.06949235617757132, 91.87390960531436690 ) ) ;
#49468=CARTESIAN_POINT ( 'NONE',  ( -12.14591786802326823, 12.06949235617739902, 38.12609039468567573 ) ) ;
#49469=CARTESIAN_POINT ( 'NONE',  ( 21.55341960407619695, -5.719274019375665929, 61.04275706135234714 ) ) ;
#49470=ORIENTED_EDGE ( 'NONE', *, *, #193512, .T. ) ;
#49471=CARTESIAN_POINT ( 'NONE',  ( 16.51473224551083163, -9.474510206698727899, 25.83442372801900078 ) ) ;
#49472=CARTESIAN_POINT ( 'NONE',  ( 5.049401038297881783, 19.05341960407617563, 82.29275706135229029 ) ) ;
#49473=CARTESIAN_POINT ( 'NONE',  ( 9.474510206698729675, 16.51473224551082808, 37.08442372801899722 ) ) ;
#49474=CARTESIAN_POINT ( 'NONE',  ( -18.09918380851993547, -5.499999999999988454, 91.48618307335611632 ) ) ;
#49475=CARTESIAN_POINT ( 'NONE',  ( -0.05219959533937732626, 21.53943276465977519, 32.50109039468568284 ) ) ;
#49477=CARTESIAN_POINT ( 'NONE',  ( 0.05219959533936267826, -19.03943276465977164, 30.00109039468566863 ) ) ;
#49478=CARTESIAN_POINT ( 'NONE',  ( 0.05219959533909260263, 19.03943276465977164, 54.99890960531435979 ) ) ;
#49479=CARTESIAN_POINT ( 'NONE',  ( -13.89961937509957401, -13.97604488694547875, 34.37609039468566863 ) ) ;
#49480=CARTESIAN_POINT ( 'NONE',  ( 12.06949235617739724, 12.14591786802326823, 106.8760903946856899 ) ) ;
#49481=CARTESIAN_POINT ( 'NONE',  ( -21.55341960407610458, -5.719274019375992779, 21.45724293864769550 ) ) ;
#49482=CARTESIAN_POINT ( 'NONE',  ( 10.72451020669871369, 18.67979575497193778, 92.08442372801901854 ) ) ;
#49485=CARTESIAN_POINT ( 'NONE',  ( -18.67979575497193778, 10.72451020669871902, 78.33442372801901854 ) ) ;
#49488=CARTESIAN_POINT ( 'NONE',  ( -13.97604488694527625, -13.89961937509977652, 101.8739096053143811 ) ) ;
#49491=CARTESIAN_POINT ( 'NONE',  ( -19.05341960407611168, -5.049401038298163336, 46.45724293864768129 ) ) ;
#49492=CARTESIAN_POINT ( 'NONE',  ( -5.719274019375978568, 21.55341960407610458, 60.20724293864768839 ) ) ;
#49493=CARTESIAN_POINT ( 'NONE',  ( -16.52544592524342804, 4.483927247898546575, 26.04057627198103475 ) ) ;
#49494=CARTESIAN_POINT ( 'NONE',  ( 4.483927247898545687, 16.52544592524342804, 99.79057627198103830 ) ) ;
#49495=CARTESIAN_POINT ( 'NONE',  ( -9.474510206698964154, 16.51473224551069663, 100.4155762719810241 ) ) ;
#49496=CARTESIAN_POINT ( 'NONE',  ( -13.97604488694547697, 13.89961937509957934, 23.12609039468565442 ) ) ;
#49497=CARTESIAN_POINT ( 'NONE',  ( -14.34966873604960291, -8.224510206698953496, 106.6655762719810383 ) ) ;
#49498=CARTESIAN_POINT ( 'NONE',  ( 21.53943276465977519, 0.05219959533937863772, 51.25109039468568994 ) ) ;
#49499=CARTESIAN_POINT ( 'NONE',  ( -14.29746914071037622, -8.314922557961029526, 104.1677570613523471 ) ) ;
#49500=CARTESIAN_POINT ( 'NONE',  ( -0.05219959533936034679, 19.03943276465977164, 67.50109039468566152 ) ) ;
#49501=CARTESIAN_POINT ( 'NONE',  ( 13.89961937509977652, -13.97604488694527269, 113.1239096053143527 ) ) ;
#49502=CARTESIAN_POINT ( 'NONE',  ( -12.14591786802309592, -12.06949235617757132, 81.87390960531435269 ) ) ;
#49503=CARTESIAN_POINT ( 'NONE',  ( 19.03943276465977164, 0.05219959533936151252, 61.25109039468566863 ) ) ;
#49504=CARTESIAN_POINT ( 'NONE',  ( -9.564922557960796823, -16.46253265017161027, 57.08224293864769550 ) ) ;
#49505=CARTESIAN_POINT ( 'NONE',  ( -4.483927247898539470, -16.52544592524342804, 67.29057627198103830 ) ) ;
#49506=CARTESIAN_POINT ( 'NONE',  ( 13.89961937509957401, 13.97604488694547697, 96.87609039468566152 ) ) ;
#49507=CARTESIAN_POINT ( 'NONE',  ( -18.67979575497178146, -10.72451020669898902, 41.66557627198103120 ) ) ;
#49509=CARTESIAN_POINT ( 'NONE',  ( -8.314922557960811034, -14.29746914071050412, 97.08224293864770971 ) ) ;
#49510=CARTESIAN_POINT ( 'NONE',  ( -17.05116617787826172, -6.768360034955703597, 31.34324446740801307 ) ) ;
#49511=CARTESIAN_POINT ( 'NONE',  ( 5.049401038298161559, -19.05341960407611168, 62.70724293864769550 ) ) ;
#49512=CARTESIAN_POINT ( 'NONE',  ( 21.52544592524344225, -5.823673210054117533, 63.54057627198103830 ) ) ;
#49513=CARTESIAN_POINT ( 'NONE',  ( -9.564922557960796823, -16.46253265017161027, 42.08224293864769550 ) ) ;
#49514=CARTESIAN_POINT ( 'NONE',  ( -4.483927247898782831, 16.52544592524335698, 92.70942372801901854 ) ) ;
#49515=CARTESIAN_POINT ( 'NONE',  ( -13.89961937509977652, 13.97604488694528158, 70.62390960531432427 ) ) ;
#49516=CARTESIAN_POINT ( 'NONE',  ( -9.564922557961040184, 16.46253265017147172, 52.91775706135233293 ) ) ;
#49517=CARTESIAN_POINT ( 'NONE',  ( 15.72974639402176855, 15.80617190586768217, 76.87609039468567573 ) ) ;
#49518=CARTESIAN_POINT ( 'NONE',  ( -21.53943276465977519, 0.05219959533907696930, 46.24890960531435979 ) ) ;
#49519=CARTESIAN_POINT ( 'NONE',  ( 5.049401038298161559, -19.05341960407611168, 102.7072429386476955 ) ) ;
#49520=CARTESIAN_POINT ( 'NONE',  ( -19.02544592524342804, 5.153800228976336051, 26.04057627198103120 ) ) ;
#49521=CARTESIAN_POINT ( 'NONE',  ( 12.06949235617739724, 12.14591786802326823, 86.87609039468568994 ) ) ;
#49522=CARTESIAN_POINT ( 'NONE',  ( -9.474510206698720793, -16.51473224551083518, 109.5844237280190043 ) ) ;
#49523=CARTESIAN_POINT ( 'NONE',  ( -16.51473224551069308, -9.474510206698971260, 26.66557627198103120 ) ) ;
#49525=CARTESIAN_POINT ( 'NONE',  ( -21.53943276465977519, -0.05219959533937600094, 93.75109039468567573 ) ) ;
#49526=CARTESIAN_POINT ( 'NONE',  ( 14.29746914071049879, -8.314922557960816363, 58.33224293864768839 ) ) ;
#49527=CARTESIAN_POINT ( 'NONE',  ( 12.06949235617757843, -12.14591786802309237, 73.12390960531436690 ) ) ;
#49528=CARTESIAN_POINT ( 'NONE',  ( -10.81492255796078084, -18.62759615963271287, 97.08224293864770971 ) ) ;
#49529=CARTESIAN_POINT ( 'NONE',  ( -0.05219959533907301413, -21.53943276465977519, 87.49890960531436690 ) ) ;
#49531=CARTESIAN_POINT ( 'NONE',  ( 10.72451020669898902, -18.67979575497178502, 42.91557627198103120 ) ) ;
#49533=CARTESIAN_POINT ( 'NONE',  ( -16.55341960407617563, 4.379528057220093196, 68.54275706135234714 ) ) ;
#49534=CARTESIAN_POINT ( 'NONE',  ( -8.314922557960811034, -14.29746914071050412, 92.08224293864769550 ) ) ;
#49535=CARTESIAN_POINT ( 'NONE',  ( -5.049401038298153566, 19.05341960407611168, 40.20724293864768839 ) ) ;
#49536=( NAMED_UNIT ( * ) SI_UNIT ( $, .STERADIAN. ) SOLID_ANGLE_UNIT ( ) );
#49538=CARTESIAN_POINT ( 'NONE',  ( 8.224510206698742110, 14.34966873604972548, 92.08442372801901854 ) ) ;
#49539=CARTESIAN_POINT ( 'NONE',  ( -21.53943276465977519, -0.05219959533937600094, 28.75109039468567929 ) ) ;
#49540=CARTESIAN_POINT ( 'NONE',  ( 5.153800228976335163, 19.02544592524342804, 89.79057627198102409 ) ) ;
#49541=CARTESIAN_POINT ( 'NONE',  ( -15.72974639402176322, -15.80617190586768395, 74.37609039468568994 ) ) ;
#49545=CARTESIAN_POINT ( 'NONE',  ( 0.05219959533937995610, -21.53943276465977519, 60.00109039468568284 ) ) ;
#49546=CARTESIAN_POINT ( 'NONE',  ( -19.02544592524342804, 5.153800228976336051, 41.04057627198103120 ) ) ;
#49547=CARTESIAN_POINT ( 'NONE',  ( -9.564922557960796823, -16.46253265017161027, 112.0822429386476955 ) ) ;
#49548=CARTESIAN_POINT ( 'NONE',  ( -0.05219959533909027116, -19.03943276465977164, 92.49890960531436690 ) ) ;
#49549=CARTESIAN_POINT ( 'NONE',  ( 5.153800228976615827, -19.02544592524334988, 65.20942372801900433 ) ) ;
#49550=CARTESIAN_POINT ( 'NONE',  ( -21.52544592524334988, -5.823673210054445271, 23.95942372801901143 ) ) ;
#49551=CARTESIAN_POINT ( 'NONE',  ( -19.05341960407617563, 5.049401038297882671, 58.54275706135234003 ) ) ;
#49552=CARTESIAN_POINT ( 'NONE',  ( -19.02544592524342804, 5.153800228976336051, 41.04057627198103120 ) ) ;
#49553=CARTESIAN_POINT ( 'NONE',  ( 16.55341960407618274, -4.379528057220086978, 111.0427570613523613 ) ) ;
#49554=CARTESIAN_POINT ( 'NONE',  ( 19.02544592524334988, 5.153800228976608722, 61.45942372801900433 ) ) ;
#49555=CARTESIAN_POINT ( 'NONE',  ( 16.55341960407611168, 4.379528057220329451, 23.95724293864769550 ) ) ;
#49556=CARTESIAN_POINT ( 'NONE',  ( -9.564922557961040184, 16.46253265017147172, 52.91775706135233293 ) ) ;
#49557=CARTESIAN_POINT ( 'NONE',  ( -16.51473224551069308, -9.474510206698971260, 96.66557627198102409 ) ) ;
#49558=CARTESIAN_POINT ( 'NONE',  ( -0.05219959533937732626, 21.53943276465977519, 107.5010903946856899 ) ) ;
#49559=CARTESIAN_POINT ( 'NONE',  ( 15.72974639402176855, 15.80617190586768217, 111.8760903946856615 ) ) ;
#49561=CARTESIAN_POINT ( 'NONE',  ( -5.719274019375665041, -21.55341960407619695, 84.79275706135234714 ) ) ;
#49562=CARTESIAN_POINT ( 'NONE',  ( -12.14591786802326823, 12.06949235617739902, 28.12609039468568284 ) ) ;
#49563=CARTESIAN_POINT ( 'NONE',  ( 19.02544592524343514, -5.153800228976328945, 93.54057627198102409 ) ) ;
#49566=B_SPLINE_CURVE_WITH_KNOTS ( 'NONE', 3,
 ( #1288, #14490, #61967, #108480, #139799, #62965 ),
 .UNSPECIFIED., .F., .F.,
 ( 4, 2, 4 ),
 ( 0.007228050697041494589, 0.007608510107494984021, 0.007988969517948474319 ),
 .UNSPECIFIED. ) ;
#49567=CARTESIAN_POINT ( 'NONE',  ( -0.05219959533909027116, -19.03943276465977164, 72.49890960531435269 ) ) ;
#49569=CARTESIAN_POINT ( 'NONE',  ( 13.97604488694548053, -13.89961937509957401, 70.62609039468567573 ) ) ;
#49570=CARTESIAN_POINT ( 'NONE',  ( -13.89961937509977652, 13.97604488694528158, 105.6239096053143527 ) ) ;
#49571=CARTESIAN_POINT ( 'NONE',  ( -10.81492255796105439, 18.62759615963255655, 102.9177570613523756 ) ) ;
#49572=CARTESIAN_POINT ( 'NONE',  ( 12.14591786802309770, 12.06949235617756955, 104.3739096053143669 ) ) ;
#49573=CARTESIAN_POINT ( 'NONE',  ( -15.80617190586745835, -15.72974639402198527, 41.87390960531435979 ) ) ;
#49574=CARTESIAN_POINT ( 'NONE',  ( -0.05219959533907301413, -21.53943276465977519, 42.49890960531435979 ) ) ;
#49575=CARTESIAN_POINT ( 'NONE',  ( -14.34966873604960291, -8.224510206698953496, 101.6655762719810383 ) ) ;
#49577=CARTESIAN_POINT ( 'NONE',  ( -16.51473224551082808, 9.474510206698731452, 53.33442372801900433 ) ) ;
#49578=CARTESIAN_POINT ( 'NONE',  ( 12.14591786802309770, 12.06949235617756955, 29.37390960531435269 ) ) ;
#49579=CARTESIAN_POINT ( 'NONE',  ( -19.05341960407611168, -5.049401038298163336, 106.4572429386476955 ) ) ;
#49580=CARTESIAN_POINT ( 'NONE',  ( -18.67979575497193778, 10.72451020669871902, 83.33442372801903275 ) ) ;
#49581=CARTESIAN_POINT ( 'NONE',  ( -21.55341960407610458, -5.719274019375992779, 76.45724293864769550 ) ) ;
#49582=CARTESIAN_POINT ( 'NONE',  ( 21.52544592524334988, 5.823673210054432836, 41.45942372801901143 ) ) ;
#49583=CARTESIAN_POINT ( 'NONE',  ( -21.53943276465977519, 0.05219959533907696930, 91.24890960531436690 ) ) ;
#49584=CARTESIAN_POINT ( 'NONE',  ( 10.81492255796106328, -18.62759615963255655, 50.41775706135235424 ) ) ;
#49585=CARTESIAN_POINT ( 'NONE',  ( 5.049401038298161559, -19.05341960407611168, 32.70724293864768129 ) ) ;
#49586=CARTESIAN_POINT ( 'NONE',  ( 5.049401038298161559, -19.05341960407611168, 82.70724293864770971 ) ) ;
#49587=CARTESIAN_POINT ( 'NONE',  ( -4.379528057220086978, -16.55341960407618274, 84.79275706135234714 ) ) ;
#49588=CARTESIAN_POINT ( 'NONE',  ( 8.314922557960818139, 14.29746914071049879, 99.58224293864770971 ) ) ;
#49589=CARTESIAN_POINT ( 'NONE',  ( 16.46253265017160672, -9.564922557960803928, 103.3322429386476955 ) ) ;
#49590=CARTESIAN_POINT ( 'NONE',  ( 4.483927247898545687, 16.52544592524342804, 54.79057627198104541 ) ) ;
#49591=CARTESIAN_POINT ( 'NONE',  ( -14.34966873604972548, 8.224510206698743886, 108.3344237280190185 ) ) ;
#49592=CARTESIAN_POINT ( 'NONE',  ( -19.03943276465977164, 0.05219959533909376836, 51.24890960531436690 ) ) ;
#49593=CARTESIAN_POINT ( 'NONE',  ( 19.03943276465977164, -0.05219959533909143690, 33.74890960531435979 ) ) ;
#49594=CARTESIAN_POINT ( 'NONE',  ( 0.05219959533907565091, 21.53943276465977519, 44.99890960531435979 ) ) ;
#49595=CARTESIAN_POINT ( 'NONE',  ( 16.51473224551083163, -9.474510206698727899, 25.83442372801900078 ) ) ;
#49597=CARTESIAN_POINT ( 'NONE',  ( -4.379528057220328563, 16.55341960407611168, 40.20724293864769550 ) ) ;
#49598=CARTESIAN_POINT ( 'NONE',  ( 15.72974639402176855, 15.80617190586768217, 41.87609039468568284 ) ) ;
#49600=CARTESIAN_POINT ( 'NONE',  ( 16.55341960407618274, -4.379528057220086978, 61.04275706135234714 ) ) ;
#49602=CARTESIAN_POINT ( 'NONE',  ( -13.97604488694547697, 13.89961937509957934, 63.12609039468566152 ) ) ;
#49603=CARTESIAN_POINT ( 'NONE',  ( 12.06949235617757843, -12.14591786802309237, 28.12390960531435979 ) ) ;
#49604=CARTESIAN_POINT ( 'NONE',  ( -19.52851543214745789, -5.499999999999945821, 75.39357721762580411 ) ) ;
#49605=CARTESIAN_POINT ( 'NONE',  ( 8.224510206698742110, 14.34966873604972548, 107.0844237280190043 ) ) ;
#49606=CARTESIAN_POINT ( 'NONE',  ( 9.564922557960805705, 16.46253265017160317, 39.58224293864768839 ) ) ;
#49607=CARTESIAN_POINT ( 'NONE',  ( 13.97604488694527802, 13.89961937509977652, 64.37390960531436690 ) ) ;
#49608=CARTESIAN_POINT ( 'NONE',  ( 19.05341960407611168, 5.049401038298154454, 23.95724293864769194 ) ) ;
#49609=CARTESIAN_POINT ( 'NONE',  ( 21.53943276465977519, 0.05219959533937863772, 31.25109039468568639 ) ) ;
#49610=CARTESIAN_POINT ( 'NONE',  ( -19.03943276465977164, 0.05219959533909376836, 41.24890960531435269 ) ) ;
#49612=CARTESIAN_POINT ( 'NONE',  ( 5.153800228976335163, 19.02544592524342804, 49.79057627198100988 ) ) ;
#49613=CARTESIAN_POINT ( 'NONE',  ( -18.67979575497178146, -10.72451020669898902, 26.66557627198103475 ) ) ;
#49614=ADVANCED_FACE ( 'NONE', ( #59485 ), #90811, .F. ) ;
#49615=CARTESIAN_POINT ( 'NONE',  ( 21.55341960407619695, -5.719274019375665929, 56.04275706135235424 ) ) ;
#49616=CARTESIAN_POINT ( 'NONE',  ( 16.52544592524342804, -4.483927247898539470, 98.54057627198105251 ) ) ;
#49617=CARTESIAN_POINT ( 'NONE',  ( -9.474510206698964154, 16.51473224551069663, 115.4155762719810241 ) ) ;
#49619=CARTESIAN_POINT ( 'NONE',  ( 12.14591786802327356, -12.06949235617739191, 80.62609039468567573 ) ) ;
#49620=CARTESIAN_POINT ( 'NONE',  ( 18.62759615963255655, 10.81492255796105972, 91.66775706135234714 ) ) ;
#49621=CARTESIAN_POINT ( 'NONE',  ( -4.483927247898782831, 16.52544592524335698, 57.70942372801901143 ) ) ;
#49622=CARTESIAN_POINT ( 'NONE',  ( -19.05341960407611168, -5.049401038298163336, 96.45724293864769550 ) ) ;
#49623=CARTESIAN_POINT ( 'NONE',  ( -14.34966873604972548, 8.224510206698743886, 38.33442372801900433 ) ) ;
#49624=CARTESIAN_POINT ( 'NONE',  ( -0.05219959533934338120, 16.53943276465976808, 22.50109039468567573 ) ) ;
#49625=CARTESIAN_POINT ( 'NONE',  ( -4.483927247898782831, 16.52544592524335698, 102.7094237280190185 ) ) ;
#49626=CARTESIAN_POINT ( 'NONE',  ( 15.80617190586769283, -15.72974639402175789, 50.62609039468568994 ) ) ;
#49627=CARTESIAN_POINT ( 'NONE',  ( 9.564922557961047289, -16.46253265017146816, 100.4177570613523329 ) ) ;
#49628=CARTESIAN_POINT ( 'NONE',  ( -15.72974639402197994, 15.80617190586746368, 115.6239096053143669 ) ) ;
#49629=CARTESIAN_POINT ( 'NONE',  ( 14.34966873604960469, 8.224510206698951720, 109.1655762719810383 ) ) ;
#49630=CARTESIAN_POINT ( 'NONE',  ( -0.05219959533936034679, 19.03943276465977164, 102.5010903946856757 ) ) ;
#49631=CARTESIAN_POINT ( 'NONE',  ( -16.52544592524335698, -4.483927247898792601, 68.95942372801901854 ) ) ;
#49633=CARTESIAN_POINT ( 'NONE',  ( 16.51473224551083163, -9.474510206698727899, 70.83442372801900433 ) ) ;
#49634=CARTESIAN_POINT ( 'NONE',  ( 12.06949235617757843, -12.14591786802309237, 48.12390960531436690 ) ) ;
#49635=CARTESIAN_POINT ( 'NONE',  ( -4.379528057220328563, 16.55341960407611168, 45.20724293864769550 ) ) ;
#49636=CARTESIAN_POINT ( 'NONE',  ( 16.52544592524342804, -4.483927247898539470, 93.54057627198103830 ) ) ;
#49637=CARTESIAN_POINT ( 'NONE',  ( -16.46253265017146816, -9.564922557961047289, 29.16775706135232937 ) ) ;
#49639=CARTESIAN_POINT ( 'NONE',  ( -15.80617190586768217, 15.72974639402176855, 43.12609039468568284 ) ) ;
#49640=CARTESIAN_POINT ( 'NONE',  ( -16.46253265017146816, -9.564922557961047289, 99.16775706135233293 ) ) ;
#49642=CARTESIAN_POINT ( 'NONE',  ( -19.03943276465977164, 0.05219959533909376836, 86.24890960531436690 ) ) ;
#49643=CARTESIAN_POINT ( 'NONE',  ( -5.153800228976328057, -19.02544592524343514, 92.29057627198099567 ) ) ;
#49644=CARTESIAN_POINT ( 'NONE',  ( 21.52544592524344225, -5.823673210054117533, 58.54057627198103120 ) ) ;
#49645=CARTESIAN_POINT ( 'NONE',  ( -12.06949235617756955, 12.14591786802309770, 90.62390960531436690 ) ) ;
#49646=CARTESIAN_POINT ( 'NONE',  ( 9.564922557960805705, 16.46253265017160317, 74.58224293864769550 ) ) ;
#49647=CARTESIAN_POINT ( 'NONE',  ( 13.89961937509977652, -13.97604488694527269, 23.12390960531436335 ) ) ;
#49648=CARTESIAN_POINT ( 'NONE',  ( -18.62759615963255300, -10.81492255796106328, 39.16775706135235424 ) ) ;
#49649=CARTESIAN_POINT ( 'NONE',  ( -21.52544592524334988, -5.823673210054445271, 73.95942372801901854 ) ) ;
#49650=CARTESIAN_POINT ( 'NONE',  ( 8.224510206698742110, 14.34966873604972548, 97.08442372801904696 ) ) ;
#49651=CARTESIAN_POINT ( 'NONE',  ( -21.55341960407619339, 5.719274019375674811, 33.54275706135234714 ) ) ;
#49652=CARTESIAN_POINT ( 'NONE',  ( 5.719274019375673035, 21.55341960407619339, 27.29275706135234358 ) ) ;
#49653=CARTESIAN_POINT ( 'NONE',  ( 16.51473224551083163, -9.474510206698727899, 55.83442372801899722 ) ) ;
#49654=CARTESIAN_POINT ( 'NONE',  ( 5.153800228976335163, 19.02544592524342804, 74.79057627198103830 ) ) ;
#49655=CARTESIAN_POINT ( 'NONE',  ( -10.72451020669870658, -18.67979575497194134, 79.58442372801903275 ) ) ;
#49656=CARTESIAN_POINT ( 'NONE',  ( 18.62759615963271287, -10.81492255796078972, 78.33224293864770971 ) ) ;
#49657=CARTESIAN_POINT ( 'NONE',  ( -8.314922557960811034, -14.29746914071050412, 57.08224293864769550 ) ) ;
#49658=CARTESIAN_POINT ( 'NONE',  ( -18.62759615963255300, -10.81492255796106328, 109.1677570613523613 ) ) ;
#49659=CARTESIAN_POINT ( 'NONE',  ( 9.474510206698729675, 16.51473224551082808, 32.08442372801900433 ) ) ;
#49660=CARTESIAN_POINT ( 'NONE',  ( -4.483927247898539470, -16.52544592524342804, 77.29057627198102409 ) ) ;
#49661=CARTESIAN_POINT ( 'NONE',  ( -5.153800228976328057, -19.02544592524343514, 27.29057627198103120 ) ) ;
#49662=CARTESIAN_POINT ( 'NONE',  ( -9.564922557961040184, 16.46253265017147172, 67.91775706135233293 ) ) ;
#49663=CARTESIAN_POINT ( 'NONE',  ( -12.06949235617756955, 12.14591786802309770, 35.62390960531437401 ) ) ;
#49664=CARTESIAN_POINT ( 'NONE',  ( 21.55341960407619695, -5.719274019375665929, 76.04275706135237556 ) ) ;
#49665=CARTESIAN_POINT ( 'NONE',  ( -5.049401038298153566, 19.05341960407611168, 75.20724293864769550 ) ) ;
#49666=CARTESIAN_POINT ( 'NONE',  ( 9.474510206698729675, 16.51473224551082808, 47.08442372801900433 ) ) ;
#49667=CARTESIAN_POINT ( 'NONE',  ( -18.67979575497178146, -10.72451020669898902, 61.66557627198103120 ) ) ;
#49668=CARTESIAN_POINT ( 'NONE',  ( -18.67979575497178146, -10.72451020669898902, 111.6655762719810525 ) ) ;
#49669=CARTESIAN_POINT ( 'NONE',  ( -5.153800228976607833, 19.02544592524334988, 107.7094237280189759 ) ) ;
#49670=CARTESIAN_POINT ( 'NONE',  ( -16.53943276465976808, -0.05219959533934237506, 73.75109039468567573 ) ) ;
#49672=CARTESIAN_POINT ( 'NONE',  ( 21.55341960407610458, 5.719274019375980345, 108.9572429386476955 ) ) ;
#49673=CARTESIAN_POINT ( 'NONE',  ( 8.314922557960818139, 14.29746914071049879, 104.5822429386477097 ) ) ;
#49675=CARTESIAN_POINT ( 'NONE',  ( -16.52544592524335698, -4.483927247898792601, 38.95942372801901854 ) ) ;
#49676=CARTESIAN_POINT ( 'NONE',  ( -10.72451020669898014, 18.67979575497178502, 60.41557627198102409 ) ) ;
#49677=CARTESIAN_POINT ( 'NONE',  ( -16.53943276465976808, -0.05219959533934237506, 103.7510903946857042 ) ) ;
#49678=CARTESIAN_POINT ( 'NONE',  ( 16.46253265017160672, -9.564922557960803928, 38.33224293864768839 ) ) ;
#49679=CARTESIAN_POINT ( 'NONE',  ( 4.379528057220092307, 16.55341960407617563, 67.29275706135234714 ) ) ;
#49680=CARTESIAN_POINT ( 'NONE',  ( 16.51473224551083163, -9.474510206698727899, 60.83442372801900433 ) ) ;
#49681=CARTESIAN_POINT ( 'NONE',  ( 21.55341960407619695, -5.719274019375665929, 46.04275706135234714 ) ) ;
#49682=CARTESIAN_POINT ( 'NONE',  ( 15.80617190586746368, 15.72974639402197994, 59.37390960531436690 ) ) ;
#49683=CARTESIAN_POINT ( 'NONE',  ( 16.55341960407618274, -4.379528057220086978, 96.04275706135236135 ) ) ;
#49684=CARTESIAN_POINT ( 'NONE',  ( -15.72974639402176322, -15.80617190586768395, 89.37609039468568994 ) ) ;
#49685=CARTESIAN_POINT ( 'NONE',  ( -10.81492255796078084, -18.62759615963271287, 47.08224293864770260 ) ) ;
#49686=CARTESIAN_POINT ( 'NONE',  ( -21.53943276465977519, 0.05219959533907696930, 31.24890960531435979 ) ) ;
#49687=ORIENTED_EDGE ( 'NONE', *, *, #78467, .T. ) ;
#49689=CARTESIAN_POINT ( 'NONE',  ( 4.483927247898790824, -16.52544592524335698, 75.20942372801901854 ) ) ;
#49690=CARTESIAN_POINT ( 'NONE',  ( -21.55341960407610458, -5.719274019375992779, 46.45724293864769550 ) ) ;
#49691=EDGE_LOOP ( 'NONE', ( #104651, #47711, #14714, #37751, #160204, #100824, #32649, #121405 ) ) ;
#49692=CARTESIAN_POINT ( 'NONE',  ( 19.03943276465977164, -0.05219959533909143690, 93.74890960531435269 ) ) ;
#49694=CARTESIAN_POINT ( 'NONE',  ( 5.153800228976335163, 19.02544592524342804, 29.79057627198102409 ) ) ;
#49695=CARTESIAN_POINT ( 'NONE',  ( 15.72974639402199770, -15.80617190586745480, 58.12390960531435979 ) ) ;
#49696=CARTESIAN_POINT ( 'NONE',  ( -16.52544592524335698, -4.483927247898792601, 88.95942372801901854 ) ) ;
#49697=CARTESIAN_POINT ( 'NONE',  ( -18.62759615963255300, -10.81492255796106328, 44.16775706135234714 ) ) ;
#49698=CARTESIAN_POINT ( 'NONE',  ( 19.03943276465977164, 0.05219959533936151252, 106.2510903946856615 ) ) ;
#49699=CARTESIAN_POINT ( 'NONE',  ( 16.53943276465976808, -0.05219959533910856209, 108.7489096053143669 ) ) ;
#49700=CARTESIAN_POINT ( 'NONE',  ( -19.03943276465977164, -0.05219959533935918106, 108.7510903946856615 ) ) ;
#49701=CARTESIAN_POINT ( 'NONE',  ( -5.153800228976328057, -19.02544592524343514, 37.29057627198102409 ) ) ;
#49702=CARTESIAN_POINT ( 'NONE',  ( 17.50000000000002132, -5.499999999999878320, 63.29690382534172954 ) ) ;
#49703=CARTESIAN_POINT ( 'NONE',  ( 19.02544592524343514, -5.153800228976328945, 93.54057627198102409 ) ) ;
#49704=CARTESIAN_POINT ( 'NONE',  ( 16.55341960407618274, -4.379528057220086978, 81.04275706135236135 ) ) ;
#49705=CARTESIAN_POINT ( 'NONE',  ( 5.823673210054444382, -21.52544592524334988, 110.2094237280190185 ) ) ;
#49706=CARTESIAN_POINT ( 'NONE',  ( 10.81492255796078972, 18.62759615963270932, 59.58224293864770260 ) ) ;
#49708=CARTESIAN_POINT ( 'NONE',  ( 16.55341960407618274, -4.379528057220086978, 91.04275706135236135 ) ) ;
#49710=CARTESIAN_POINT ( 'NONE',  ( 19.02544592524334988, 5.153800228976608722, 76.45942372801897591 ) ) ;
#49711=CARTESIAN_POINT ( 'NONE',  ( 16.51473224551069308, 9.474510206698969483, 34.16557627198102409 ) ) ;
#49712=CARTESIAN_POINT ( 'NONE',  ( 5.153800228976335163, 19.02544592524342804, 74.79057627198103830 ) ) ;
#49713=CARTESIAN_POINT ( 'NONE',  ( -13.89961937509977652, 13.97604488694528158, 30.62390960531435269 ) ) ;
#49714=CARTESIAN_POINT ( 'NONE',  ( -9.564922557961040184, 16.46253265017147172, 77.91775706135234714 ) ) ;
#49716=CARTESIAN_POINT ( 'NONE',  ( 19.02544592524343514, -5.153800228976328945, 108.5405762719810383 ) ) ;
#49717=CARTESIAN_POINT ( 'NONE',  ( -16.53943276465976808, 0.05219959533911058130, 61.24890960531435979 ) ) ;
#49718=CARTESIAN_POINT ( 'NONE',  ( -5.823673210054116645, -21.52544592524344225, 67.29057627198103830 ) ) ;
#49719=DIRECTION ( 'NONE',  ( -1.000000000000000000, -0.000000000000000000, -0.000000000000000000 ) ) ;
#49720=CARTESIAN_POINT ( 'NONE',  ( 19.05341960407617918, -5.049401038297876454, 31.04275706135232227 ) ) ;
#49722=CARTESIAN_POINT ( 'NONE',  ( 16.51473224551069308, 9.474510206698969483, 59.16557627198102409 ) ) ;
#49723=CARTESIAN_POINT ( 'NONE',  ( 5.153800228976335163, 19.02544592524342804, 79.79057627198102409 ) ) ;
#49724=CARTESIAN_POINT ( 'NONE',  ( 16.55341960407618274, -4.379528057220086978, 51.04275706135234714 ) ) ;
#49725=CARTESIAN_POINT ( 'NONE',  ( -19.19724070472095079, -5.500000000000031086, 101.0619334827438109 ) ) ;
#49726=CARTESIAN_POINT ( 'NONE',  ( -16.18388926212237422, 7.379444403734519931, 109.5604684863385074 ) ) ;
#49727=CARTESIAN_POINT ( 'NONE',  ( 16.52544592524335698, 4.483927247898782831, 76.45942372801901854 ) ) ;
#49729=CARTESIAN_POINT ( 'NONE',  ( 4.483927247898790824, -16.52544592524335698, 60.20942372801902565 ) ) ;
#49730=CARTESIAN_POINT ( 'NONE',  ( 14.29746914071037800, 8.314922557961029526, 46.66775706135234714 ) ) ;
#49731=CARTESIAN_POINT ( 'NONE',  ( -13.89961937509977652, 13.97604488694528158, 55.62390960531434558 ) ) ;
#49733=CARTESIAN_POINT ( 'NONE',  ( 18.67979575497194134, -10.72451020669871369, 50.83442372801901143 ) ) ;
#49734=CARTESIAN_POINT ( 'NONE',  ( 0.05219959533936267826, -19.03943276465977164, 65.00109039468567573 ) ) ;
#49735=CARTESIAN_POINT ( 'NONE',  ( 10.81492255796106328, -18.62759615963255655, 105.4177570613523613 ) ) ;
#49736=CARTESIAN_POINT ( 'NONE',  ( 19.05341960407611168, 5.049401038298154454, 33.95724293864769550 ) ) ;
#49737=CARTESIAN_POINT ( 'NONE',  ( 16.73912658984721702, 7.076536648759412351, 23.72892465253222127 ) ) ;
#49738=CARTESIAN_POINT ( 'NONE',  ( -5.719274019375978568, 21.55341960407610458, 55.20724293864770260 ) ) ;
#49739=CARTESIAN_POINT ( 'NONE',  ( -5.153800228976328057, -19.02544592524343514, 102.2905762719810383 ) ) ;
#49740=CARTESIAN_POINT ( 'NONE',  ( 4.483927247898545687, 16.52544592524342804, 99.79057627198103830 ) ) ;
#49741=CARTESIAN_POINT ( 'NONE',  ( 12.06949235617739724, 12.14591786802326823, 36.87609039468568994 ) ) ;
#49742=CARTESIAN_POINT ( 'NONE',  ( -14.29746914071049879, 8.314922557960819915, 35.83224293864768839 ) ) ;
#49744=CARTESIAN_POINT ( 'NONE',  ( 18.62759615963271287, -10.81492255796078972, 103.3322429386476955 ) ) ;
#49745=CARTESIAN_POINT ( 'NONE',  ( -14.34966873604960291, -8.224510206698953496, 36.66557627198103120 ) ) ;
#49747=CARTESIAN_POINT ( 'NONE',  ( -13.89961937509957401, -13.97604488694547875, 89.37609039468563310 ) ) ;
#49748=CARTESIAN_POINT ( 'NONE',  ( 19.02544592524334988, 5.153800228976608722, 31.45942372801900433 ) ) ;
#49749=CARTESIAN_POINT ( 'NONE',  ( -16.52544592524342804, 4.483927247898546575, 26.04057627198103475 ) ) ;
#49750=CARTESIAN_POINT ( 'NONE',  ( -18.67979575497178146, -10.72451020669898902, 106.6655762719810383 ) ) ;
#49751=CARTESIAN_POINT ( 'NONE',  ( 5.719274019375991003, -21.55341960407610458, 47.70724293864770260 ) ) ;
#49753=CARTESIAN_POINT ( 'NONE',  ( -0.05219959533909027116, -19.03943276465977164, 82.49890960531436690 ) ) ;
#49754=CARTESIAN_POINT ( 'NONE',  ( 16.53943276465976808, -0.05219959533910856209, 33.74890960531436690 ) ) ;
#49755=CARTESIAN_POINT ( 'NONE',  ( 0.05219959533909260263, 19.03943276465977164, 94.99890960531436690 ) ) ;
#49757=CARTESIAN_POINT ( 'NONE',  ( 17.59860650958989936, 7.585241751807028088, 79.07662985737508166 ) ) ;
#49758=CARTESIAN_POINT ( 'NONE',  ( -0.05219959533936034679, 19.03943276465977164, 47.50109039468566863 ) ) ;
#49759=CARTESIAN_POINT ( 'NONE',  ( -10.81492255796078084, -18.62759615963271287, 82.08224293864768129 ) ) ;
#49760=B_SPLINE_CURVE_WITH_KNOTS ( 'NONE', 3,
 ( #108435, #123590, #186295, #120624, #47775, #62920, #106443, #124600, #139754, #171108, #15443, #169103, #143485, #91252, #153947, #60933, #109428, #13456, #59946, #90284, #16437, #45779, #78086, #158662, #136788, #35328, #20153, #137781, #121613, #75120, #251, #107431 ),
 .UNSPECIFIED., .F., .F.,
 ( 4, 2, 2, 2, 2, 2, 2, 2, 2, 2, 2, 2, 2, 2, 2, 4 ),
 ( 2.281672496420497557E-17, 0.0003712461730037045046, 0.0007424923460073861326, 0.001113738519011067598, 0.001484984692014749497, 0.002227477038022112645, 0.002598723211025787388, 0.002969969384029461697, 0.003341215557033136441, 0.003712461730036810750, 0.004083707903040485060, 0.004454954076044158502, 0.004826200249047832812, 0.005197446422051507989, 0.005568692595055182298, 0.005939938768058856608 ),
 .UNSPECIFIED. ) ;
#49761=CARTESIAN_POINT ( 'NONE',  ( -12.06949235617756955, 12.14591786802309770, 95.62390960531436690 ) ) ;
#49763=CARTESIAN_POINT ( 'NONE',  ( -0.05219959533937732626, 21.53943276465977519, 42.50109039468567573 ) ) ;
#49766=CARTESIAN_POINT ( 'NONE',  ( 16.55341960407618274, -4.379528057220086978, 111.0427570613523613 ) ) ;
#49767=CARTESIAN_POINT ( 'NONE',  ( -0.05219959533909027116, -19.03943276465977164, 42.49890960531435269 ) ) ;
#49768=CARTESIAN_POINT ( 'NONE',  ( -19.03943276465977164, 0.05219959533909376836, 91.24890960531436690 ) ) ;
#49769=CARTESIAN_POINT ( 'NONE',  ( -19.53037848336980886, 5.499999999999904077, 44.85532783611448338 ) ) ;
#49770=CARTESIAN_POINT ( 'NONE',  ( 9.474510206698971260, -16.51473224551069308, 32.91557627198102409 ) ) ;
#49771=CARTESIAN_POINT ( 'NONE',  ( 8.314922557960818139, 14.29746914071049879, 44.58224293864769550 ) ) ;
#49772=CARTESIAN_POINT ( 'NONE',  ( 21.53943276465977519, 0.05219959533937863772, 71.25109039468568994 ) ) ;
#49774=CARTESIAN_POINT ( 'NONE',  ( -12.14591786802326823, 12.06949235617739902, 68.12609039468567573 ) ) ;
#49775=CARTESIAN_POINT ( 'NONE',  ( -13.89961937509977652, 13.97604488694528158, 50.62390960531435979 ) ) ;
#49776=CARTESIAN_POINT ( 'NONE',  ( -0.05219959533909027116, -19.03943276465977164, 67.49890960531436690 ) ) ;
#49778=CARTESIAN_POINT ( 'NONE',  ( 21.53943276465977519, 0.05219959533937863772, 106.2510903946856757 ) ) ;
#49779=CARTESIAN_POINT ( 'NONE',  ( -16.53943276465976808, -0.05219959533934237506, 68.75109039468568994 ) ) ;
#49780=CARTESIAN_POINT ( 'NONE',  ( -0.05219959533937732626, 21.53943276465977519, 97.50109039468567573 ) ) ;
#49781=CARTESIAN_POINT ( 'NONE',  ( -5.153800228976328057, -19.02544592524343514, 62.29057627198100988 ) ) ;
#49782=CARTESIAN_POINT ( 'NONE',  ( -0.05219959533907301413, -21.53943276465977519, 37.49890960531436690 ) ) ;
#49783=CARTESIAN_POINT ( 'NONE',  ( 13.97604488694548053, -13.89961937509957401, 105.6260903946856757 ) ) ;
#49784=CARTESIAN_POINT ( 'NONE',  ( -18.67979575497193778, 10.72451020669871902, 63.33442372801900433 ) ) ;
#49785=CARTESIAN_POINT ( 'NONE',  ( 12.06949235617739724, 12.14591786802326823, 51.87609039468568284 ) ) ;
#49786=CARTESIAN_POINT ( 'NONE',  ( -15.72974639402197994, 15.80617190586746368, 105.6239096053143669 ) ) ;
#49787=CARTESIAN_POINT ( 'NONE',  ( -9.474510206698720793, -16.51473224551083518, 94.58442372801900433 ) ) ;
#49788=CARTESIAN_POINT ( 'NONE',  ( 13.97604488694527802, 13.89961937509977652, 79.37390960531435269 ) ) ;
#49789=CARTESIAN_POINT ( 'NONE',  ( -16.46253265017146816, -9.564922557961047289, 104.1677570613523329 ) ) ;
#49790=CARTESIAN_POINT ( 'NONE',  ( -16.51473224551082808, 9.474510206698731452, 113.3344237280190043 ) ) ;
#49791=CARTESIAN_POINT ( 'NONE',  ( -0.05219959533910754901, -16.53943276465976808, 67.49890960531436690 ) ) ;
#49792=B_SPLINE_CURVE_WITH_KNOTS ( 'NONE', 3,
 ( #139261, #199955, #168603, #137277, #108924, #47267, #48263, #156424, #107918, #30103, #109917, #737, #1741, #170604, #138272, #172594, #91743, #17925, #63419, #61420 ),
 .UNSPECIFIED., .F., .F.,
 ( 4, 2, 2, 2, 2, 2, 2, 2, 2, 4 ),
 ( 0.000000000000000000, 0.0004987090165372609933, 0.0009974180330745219866, 0.001246772541343152537, 0.001496127049611783088, 0.001994836066149048310, 0.002493545082686314182, 0.002742899590954939095, 0.002992254099223564442, 0.003989672132298079273 ),
 .UNSPECIFIED. ) ;
#49793=CARTESIAN_POINT ( 'NONE',  ( 14.34966873604972726, -8.224510206698740333, 75.83442372801900433 ) ) ;
#49794=CARTESIAN_POINT ( 'NONE',  ( -18.67979575497178146, -10.72451020669898902, 111.6655762719810525 ) ) ;
#49795=CARTESIAN_POINT ( 'NONE',  ( -9.564922557960796823, -16.46253265017161027, 52.08224293864768839 ) ) ;
#49796=CARTESIAN_POINT ( 'NONE',  ( -16.46253265017160317, 9.564922557960807481, 65.83224293864769550 ) ) ;
#49798=CARTESIAN_POINT ( 'NONE',  ( 12.06949235617739724, 12.14591786802326823, 71.87609039468568994 ) ) ;
#49799=CYLINDRICAL_SURFACE ( 'NONE', #133806, 2.000000000000000000 ) ;
#49800=ORIENTED_EDGE ( 'NONE', *, *, #69228, .F. ) ;
#49801=CARTESIAN_POINT ( 'NONE',  ( -21.53943276465977519, -0.05219959533937600094, 113.7510903946856757 ) ) ;
#49802=CARTESIAN_POINT ( 'NONE',  ( -9.564922557960796823, -16.46253265017161027, 37.08224293864768839 ) ) ;
#49804=CARTESIAN_POINT ( 'NONE',  ( 16.51473224551083163, -9.474510206698727899, 105.8344237280190043 ) ) ;
#49805=CARTESIAN_POINT ( 'NONE',  ( -13.89961937509957401, -13.97604488694547875, 39.37609039468566152 ) ) ;
#49806=CARTESIAN_POINT ( 'NONE',  ( -8.314922557961024197, 14.29746914071037800, 22.91775706135235069 ) ) ;
#49807=CARTESIAN_POINT ( 'NONE',  ( 0.05219959533909260263, 19.03943276465977164, 44.99890960531435979 ) ) ;
#49808=CARTESIAN_POINT ( 'NONE',  ( 13.89961937509977652, -13.97604488694527269, 68.12390960531436690 ) ) ;
#49809=CARTESIAN_POINT ( 'NONE',  ( -18.62759615963270932, 10.81492255796079327, 80.83224293864769550 ) ) ;
#49810=CARTESIAN_POINT ( 'NONE',  ( -5.153800228976328057, -19.02544592524343514, 107.2905762719810383 ) ) ;
#49811=CARTESIAN_POINT ( 'NONE',  ( 13.89961937509977652, -13.97604488694527269, 48.12390960531435979 ) ) ;
#49813=CARTESIAN_POINT ( 'NONE',  ( -19.02544592524334988, -5.153800228976617603, 93.95942372801900433 ) ) ;
#49814=CARTESIAN_POINT ( 'NONE',  ( -14.34966873604960291, -8.224510206698953496, 71.66557627198100988 ) ) ;
#49815=CARTESIAN_POINT ( 'NONE',  ( 19.03943276465977164, 0.05219959533936151252, 31.25109039468566863 ) ) ;
#49817=CARTESIAN_POINT ( 'NONE',  ( 16.55341960407611168, 4.379528057220329451, 58.95724293864770971 ) ) ;
#49818=CARTESIAN_POINT ( 'NONE',  ( -21.53943276465977519, -0.05219959533937600094, 83.75109039468568994 ) ) ;
#49819=CARTESIAN_POINT ( 'NONE',  ( 19.03943276465977164, -0.05219959533909143690, 28.74890960531435624 ) ) ;
#49820=CARTESIAN_POINT ( 'NONE',  ( -21.55341960407619339, 5.719274019375674811, 93.54275706135234714 ) ) ;
#49821=CARTESIAN_POINT ( 'NONE',  ( -16.52544592524342804, 4.483927247898546575, 31.04057627198102409 ) ) ;
#49822=CARTESIAN_POINT ( 'NONE',  ( -21.53943276465977519, -0.05219959533937600094, 78.75109039468568994 ) ) ;
#49823=CARTESIAN_POINT ( 'NONE',  ( -13.97604488694527625, -13.89961937509977652, 81.87390960531436690 ) ) ;
#49824=CARTESIAN_POINT ( 'NONE',  ( 0.05219959533937995610, -21.53943276465977519, 40.00109039468567573 ) ) ;
#49825=CARTESIAN_POINT ( 'NONE',  ( -13.89961937509977652, 13.97604488694528158, 80.62390960531436690 ) ) ;
#49826=CARTESIAN_POINT ( 'NONE',  ( 16.52544592524342804, -4.483927247898539470, 98.54057627198105251 ) ) ;
#49827=CARTESIAN_POINT ( 'NONE',  ( 8.314922557960818139, 14.29746914071049879, 59.58224293864770260 ) ) ;
#49828=CARTESIAN_POINT ( 'NONE',  ( 21.55341960407610458, 5.719274019375980345, 68.95724293864769550 ) ) ;
#49829=CARTESIAN_POINT ( 'NONE',  ( -19.03943276465977164, 0.05219959533909376836, 71.24890960531435269 ) ) ;
#49830=CARTESIAN_POINT ( 'NONE',  ( -21.52544592524343514, 5.823673210054127303, 91.04057627198103830 ) ) ;
#49831=CARTESIAN_POINT ( 'NONE',  ( 5.049401038297881783, 19.05341960407617563, 77.29275706135231871 ) ) ;
#49832=CARTESIAN_POINT ( 'NONE',  ( 5.049401038297881783, 19.05341960407617918, 27.29275706135232582 ) ) ;
#49833=CARTESIAN_POINT ( 'NONE',  ( 4.483927247898545687, 16.52544592524342804, 74.79057627198105251 ) ) ;
#49834=CARTESIAN_POINT ( 'NONE',  ( 18.67979575497178502, 10.72451020669898547, 49.16557627198102409 ) ) ;
#49836=CARTESIAN_POINT ( 'NONE',  ( 12.14591786802327356, -12.06949235617739191, 95.62609039468568994 ) ) ;
#49838=CARTESIAN_POINT ( 'NONE',  ( -16.51473224551082808, 9.474510206698731452, 98.33442372801900433 ) ) ;
#49839=CARTESIAN_POINT ( 'NONE',  ( -0.05219959533910754901, -16.53943276465976808, 72.49890960531435269 ) ) ;
#49840=CARTESIAN_POINT ( 'NONE',  ( -18.39639308325438449, -5.500000000000017764, 96.48252246182198633 ) ) ;
#49841=CARTESIAN_POINT ( 'NONE',  ( 5.049401038298161559, -19.05341960407611168, 57.70724293864769550 ) ) ;
#49842=CARTESIAN_POINT ( 'NONE',  ( -14.34966873604960291, -8.224510206698953496, 56.66557627198103830 ) ) ;
#49843=CARTESIAN_POINT ( 'NONE',  ( -16.51473224551069308, -9.474510206698971260, 106.6655762719810383 ) ) ;
#49844=CARTESIAN_POINT ( 'NONE',  ( -19.03943276465977164, -0.05219959533935918106, 88.75109039468567573 ) ) ;
#49845=CARTESIAN_POINT ( 'NONE',  ( 9.564922557960805705, 16.46253265017160317, 59.58224293864769550 ) ) ;
#49846=CARTESIAN_POINT ( 'NONE',  ( -13.97604488694527625, -13.89961937509977652, 81.87390960531436690 ) ) ;
#49847=CARTESIAN_POINT ( 'NONE',  ( -0.05219959533909027116, -19.03943276465977164, 87.49890960531436690 ) ) ;
#49848=CARTESIAN_POINT ( 'NONE',  ( 15.72974639402199770, -15.80617190586745480, 68.12390960531436690 ) ) ;
#49849=CARTESIAN_POINT ( 'NONE',  ( 12.06949235617739724, 12.14591786802326823, 51.87609039468568284 ) ) ;
#49851=CARTESIAN_POINT ( 'NONE',  ( -13.97604488694527625, -13.89961937509977652, 56.87390960531434558 ) ) ;
#49852=CARTESIAN_POINT ( 'NONE',  ( 21.53943276465977519, -0.05219959533907433946, 73.74890960531433848 ) ) ;
#49853=CARTESIAN_POINT ( 'NONE',  ( -13.97604488694547697, 13.89961937509957934, 98.12609039468566152 ) ) ;
#49854=CARTESIAN_POINT ( 'NONE',  ( 16.55341960407611168, 4.379528057220329451, 23.95724293864769550 ) ) ;
#49855=CARTESIAN_POINT ( 'NONE',  ( -21.55341960407619339, 5.719274019375674811, 43.54275706135235424 ) ) ;
#49856=CARTESIAN_POINT ( 'NONE',  ( -19.03943276465977164, -0.05219959533935918106, 43.75109039468566863 ) ) ;
#49857=CARTESIAN_POINT ( 'NONE',  ( -4.483927247898782831, 16.52544592524335698, 67.70942372801901854 ) ) ;
#49858=CARTESIAN_POINT ( 'NONE',  ( 8.224510206698742110, 14.34966873604972548, 97.08442372801904696 ) ) ;
#49859=CARTESIAN_POINT ( 'NONE',  ( -17.49999999999999645, 5.499999999999992895, 73.71769037696435589 ) ) ;
#49860=CARTESIAN_POINT ( 'NONE',  ( -16.53943276465976808, -0.05219959533934237506, 83.75109039468568994 ) ) ;
#49861=CARTESIAN_POINT ( 'NONE',  ( 0.05219959533934541429, -16.53943276465976808, 40.00109039468567573 ) ) ;
#49862=CARTESIAN_POINT ( 'NONE',  ( 16.46253265017160672, -9.564922557960803928, 43.33224293864769550 ) ) ;
#49863=CARTESIAN_POINT ( 'NONE',  ( -19.05341960407611168, -5.049401038298163336, 56.45724293864768129 ) ) ;
#49864=CARTESIAN_POINT ( 'NONE',  ( -13.89961937509977652, 13.97604488694528158, 55.62390960531434558 ) ) ;
#49865=CARTESIAN_POINT ( 'NONE',  ( -21.53943276465977519, -0.05219959533937600094, 48.75109039468568284 ) ) ;
#49866=CARTESIAN_POINT ( 'NONE',  ( 0.05219959533934541429, -16.53943276465976808, 50.00109039468568994 ) ) ;
#49867=CARTESIAN_POINT ( 'NONE',  ( 16.55341960407611168, 4.379528057220329451, 23.95724293864769550 ) ) ;
#49868=CARTESIAN_POINT ( 'NONE',  ( 0.05219959533909260263, 19.03943276465977164, 34.99890960531435979 ) ) ;
#49869=CARTESIAN_POINT ( 'NONE',  ( 9.474510206698971260, -16.51473224551069308, 32.91557627198102409 ) ) ;
#49870=CARTESIAN_POINT ( 'NONE',  ( 0.05219959533934541429, -16.53943276465976808, 25.00109039468567218 ) ) ;
#49872=CARTESIAN_POINT ( 'NONE',  ( -9.564922557961040184, 16.46253265017147172, 87.91775706135233293 ) ) ;
#49873=CARTESIAN_POINT ( 'NONE',  ( -4.483927247898539470, -16.52544592524342804, 87.29057627198103830 ) ) ;
#49874=CARTESIAN_POINT ( 'NONE',  ( 5.153800228976335163, 19.02544592524342804, 39.79057627198100988 ) ) ;
#49875=CARTESIAN_POINT ( 'NONE',  ( 19.05341960407617918, -5.049401038297876454, 71.04275706135234714 ) ) ;
#49876=CARTESIAN_POINT ( 'NONE',  ( 17.31728774477272736, 6.344390552232407998, 76.68093348310681279 ) ) ;
#49877=CARTESIAN_POINT ( 'NONE',  ( 18.67979575497194134, -10.72451020669871369, 70.83442372801901854 ) ) ;
#49878=CARTESIAN_POINT ( 'NONE',  ( 14.29746914071037800, 8.314922557961029526, 46.66775706135234714 ) ) ;
#49879=CARTESIAN_POINT ( 'NONE',  ( 16.38665767535053774, 7.295008042176047702, 37.23599135785455871 ) ) ;
#49880=CARTESIAN_POINT ( 'NONE',  ( -5.823673210054116645, -21.52544592524344225, 32.29057627198102409 ) ) ;
#49881=CARTESIAN_POINT ( 'NONE',  ( 12.06949235617739724, 12.14591786802326823, 21.87609039468567573 ) ) ;
#49882=CARTESIAN_POINT ( 'NONE',  ( 19.03943276465977164, -0.05219959533909143690, 28.74890960531435624 ) ) ;
#49883=CARTESIAN_POINT ( 'NONE',  ( -5.049401038297874678, -19.05341960407617918, 34.79275706135233293 ) ) ;
#49885=CARTESIAN_POINT ( 'NONE',  ( 5.153800228976335163, 19.02544592524342804, 34.79057627198102409 ) ) ;
#49886=CARTESIAN_POINT ( 'NONE',  ( -5.049401038298153566, 19.05341960407611168, 70.20724293864769550 ) ) ;
#49887=CARTESIAN_POINT ( 'NONE',  ( 17.50000000000000000, -3.471454075611709822, 111.9833258114436063 ) ) ;
#49888=CARTESIAN_POINT ( 'NONE',  ( -5.719274019375665041, -21.55341960407619695, 109.7927570613523613 ) ) ;
#49889=CARTESIAN_POINT ( 'NONE',  ( 16.52544592524342804, -4.483927247898539470, 33.54057627198102409 ) ) ;
#49890=CARTESIAN_POINT ( 'NONE',  ( -9.564922557960796823, -16.46253265017161027, 37.08224293864768839 ) ) ;
#49892=CARTESIAN_POINT ( 'NONE',  ( -19.02544592524342804, 5.153800228976336051, 91.04057627198100988 ) ) ;
#49893=CARTESIAN_POINT ( 'NONE',  ( 0.05219959533937995610, -21.53943276465977519, 65.00109039468568994 ) ) ;
#49894=CARTESIAN_POINT ( 'NONE',  ( -19.02544592524342804, 5.153800228976336051, 46.04057627198101699 ) ) ;
#49895=CARTESIAN_POINT ( 'NONE',  ( 21.52544592524334988, 5.823673210054432836, 61.45942372801901854 ) ) ;
#49896=CARTESIAN_POINT ( 'NONE',  ( 5.823673210054125526, 21.52544592524343514, 29.79057627198102409 ) ) ;
#49897=CARTESIAN_POINT ( 'NONE',  ( 5.153800228976335163, 19.02544592524342804, 29.79057627198102409 ) ) ;
#49898=CARTESIAN_POINT ( 'NONE',  ( 5.719274019375673035, 21.55341960407619339, 22.29275706135235069 ) ) ;
#49899=CARTESIAN_POINT ( 'NONE',  ( -5.153800228976607833, 19.02544592524334988, 52.70942372801900433 ) ) ;
#49900=CARTESIAN_POINT ( 'NONE',  ( -16.52544592524342804, 4.483927247898546575, 116.0405762719810383 ) ) ;
#49901=CARTESIAN_POINT ( 'NONE',  ( 13.97604488694527802, 13.89961937509977652, 59.37390960531434558 ) ) ;
#49902=CARTESIAN_POINT ( 'NONE',  ( -8.224510206698735004, -14.34966873604973081, 19.58442372801901143 ) ) ;
#49904=CARTESIAN_POINT ( 'NONE',  ( 16.52544592524342804, -4.483927247898539470, 78.54057627198103830 ) ) ;
#49905=CARTESIAN_POINT ( 'NONE',  ( 21.53943276465977519, -0.05219959533907433946, 28.74890960531435624 ) ) ;
#49906=CARTESIAN_POINT ( 'NONE',  ( 0.05219959533936267826, -19.03943276465977164, 100.0010903946856757 ) ) ;
#49907=CARTESIAN_POINT ( 'NONE',  ( -5.719274019375978568, 21.55341960407610458, 105.2072429386477097 ) ) ;
#49908=CARTESIAN_POINT ( 'NONE',  ( 10.72451020669871369, 18.67979575497193778, 52.08442372801901854 ) ) ;
#49909=CARTESIAN_POINT ( 'NONE',  ( -16.53943276465976808, -0.05219959533934237506, 53.75109039468568994 ) ) ;
#49910=CARTESIAN_POINT ( 'NONE',  ( 4.379528057220092307, 16.55341960407617563, 57.29275706135234714 ) ) ;
#49911=CARTESIAN_POINT ( 'NONE',  ( -21.55341960407610458, -5.719274019375992779, 56.45724293864768839 ) ) ;
#49913=CARTESIAN_POINT ( 'NONE',  ( 13.97604488694527802, 13.89961937509977652, 49.37390960531434558 ) ) ;
#49914=CARTESIAN_POINT ( 'NONE',  ( 12.06949235617739724, 12.14591786802326823, 71.87609039468568994 ) ) ;
#49915=CARTESIAN_POINT ( 'NONE',  ( 15.72974639402199770, -15.80617190586745480, 108.1239096053143811 ) ) ;
#49916=CARTESIAN_POINT ( 'NONE',  ( -16.53943276465976808, 0.05219959533911058130, 46.24890960531435979 ) ) ;
#49917=CARTESIAN_POINT ( 'NONE',  ( -16.51473224551069308, -9.474510206698971260, 76.66557627198103830 ) ) ;
#49918=CARTESIAN_POINT ( 'NONE',  ( -12.06949235617739369, -12.14591786802326823, 79.37609039468567573 ) ) ;
#49919=CARTESIAN_POINT ( 'NONE',  ( -16.53943276465976808, -0.05219959533934237506, 23.75109039468567929 ) ) ;
#49920=CARTESIAN_POINT ( 'NONE',  ( 18.67979575497178502, 10.72451020669898547, 99.16557627198100988 ) ) ;
#49921=CARTESIAN_POINT ( 'NONE',  ( -16.52544592524342804, 4.483927247898546575, 51.04057627198103120 ) ) ;
#49923=CARTESIAN_POINT ( 'NONE',  ( 19.52217212775660116, -5.499999999999906741, 92.43993709005263781 ) ) ;
#49925=CARTESIAN_POINT ( 'NONE',  ( -10.72451020669898014, 18.67979575497178502, 85.41557627198102409 ) ) ;
#49926=CARTESIAN_POINT ( 'NONE',  ( 8.314922557960818139, 14.29746914071049879, 24.58224293864768839 ) ) ;
#49928=CARTESIAN_POINT ( 'NONE',  ( -16.20579543436680936, -7.371946100354977105, 55.56520834171877254 ) ) ;
#49929=CARTESIAN_POINT ( 'NONE',  ( -18.67979575497178146, -10.72451020669898902, 106.6655762719810383 ) ) ;
#49930=CARTESIAN_POINT ( 'NONE',  ( -0.05219959533909027116, -19.03943276465977164, 97.49890960531436690 ) ) ;
#49931=CARTESIAN_POINT ( 'NONE',  ( 0.05219959533937995610, -21.53943276465977519, 30.00109039468568284 ) ) ;
#49932=CARTESIAN_POINT ( 'NONE',  ( 4.379528057220339221, -16.55341960407611168, 37.70724293864769550 ) ) ;
#49934=CARTESIAN_POINT ( 'NONE',  ( -16.52544592524335698, -4.483927247898792601, 43.95942372801902565 ) ) ;
#49935=CARTESIAN_POINT ( 'NONE',  ( 5.153800228976335163, 19.02544592524342804, 49.79057627198100988 ) ) ;
#49936=CARTESIAN_POINT ( 'NONE',  ( 16.46253265017146816, 9.564922557961045513, 56.66775706135233293 ) ) ;
#49937=CARTESIAN_POINT ( 'NONE',  ( 13.97604488694527802, 13.89961937509977652, 79.37390960531435269 ) ) ;
#49939=CARTESIAN_POINT ( 'NONE',  ( -0.05219959533907301413, -21.53943276465977519, 32.49890960531435979 ) ) ;
#49941=CARTESIAN_POINT ( 'NONE',  ( 16.52544592524335698, 4.483927247898782831, 26.45942372801901854 ) ) ;
#49942=CARTESIAN_POINT ( 'NONE',  ( 19.05341960407617918, -5.049401038297876454, 56.04275706135234714 ) ) ;
#49943=CARTESIAN_POINT ( 'NONE',  ( -21.53943276465977519, 0.05219959533907696930, 96.24890960531435269 ) ) ;
#49945=CARTESIAN_POINT ( 'NONE',  ( -16.52544592524342804, 4.483927247898546575, 31.04057627198102409 ) ) ;
#49946=CARTESIAN_POINT ( 'NONE',  ( -19.03943276465977164, 0.05219959533909376836, 76.24890960531435269 ) ) ;
#49947=CARTESIAN_POINT ( 'NONE',  ( 21.53943276465977519, -0.05219959533907433946, 58.74890960531436690 ) ) ;
#49948=CARTESIAN_POINT ( 'NONE',  ( 0.05219959533907565091, 21.53943276465977519, 89.99890960531438111 ) ) ;
#49949=CARTESIAN_POINT ( 'NONE',  ( -16.52544592524335698, -4.483927247898792601, 18.95942372801901143 ) ) ;
#49950=CARTESIAN_POINT ( 'NONE',  ( 21.53943276465977519, -0.05219959533907433946, 23.74890960531435269 ) ) ;
#49951=CARTESIAN_POINT ( 'NONE',  ( -21.55341960407619339, 5.719274019375674811, 88.54275706135236135 ) ) ;
#49952=CARTESIAN_POINT ( 'NONE',  ( -0.05219959533909027116, -19.03943276465977164, 92.49890960531436690 ) ) ;
#49953=CARTESIAN_POINT ( 'NONE',  ( -13.97604488694527625, -13.89961937509977652, 26.87390960531434558 ) ) ;
#49954=CARTESIAN_POINT ( 'NONE',  ( 16.51473224551069308, 9.474510206698969483, 89.16557627198103830 ) ) ;
#49955=CARTESIAN_POINT ( 'NONE',  ( 4.379528057220339221, -16.55341960407611168, 107.7072429386476955 ) ) ;
#49956=CARTESIAN_POINT ( 'NONE',  ( 16.46253265017160672, -9.564922557960803928, 63.33224293864769550 ) ) ;
#49957=CARTESIAN_POINT ( 'NONE',  ( 9.564922557961047289, -16.46253265017146816, 110.4177570613523471 ) ) ;
#49958=CARTESIAN_POINT ( 'NONE',  ( 17.31747979337957233, -6.344076630960846508, 86.12055131934816643 ) ) ;
#49959=CARTESIAN_POINT ( 'NONE',  ( -19.03943276465977164, 0.05219959533909376836, 71.24890960531435269 ) ) ;
#49960=CARTESIAN_POINT ( 'NONE',  ( 10.81492255796106328, -18.62759615963255655, 100.4177570613523471 ) ) ;
#49961=CARTESIAN_POINT ( 'NONE',  ( 0.05219959533907565091, 21.53943276465977519, 24.99890960531435624 ) ) ;
#49962=CARTESIAN_POINT ( 'NONE',  ( -8.314922557961024197, 14.29746914071037800, 97.91775706135236135 ) ) ;
#49964=CARTESIAN_POINT ( 'NONE',  ( 9.564922557961047289, -16.46253265017146816, 75.41775706135234714 ) ) ;
#49965=CARTESIAN_POINT ( 'NONE',  ( -16.46253265017146816, -9.564922557961047289, 19.16775706135233293 ) ) ;
#49967=CARTESIAN_POINT ( 'NONE',  ( 19.03943276465977164, -0.05219959533909143690, 23.74890960531435269 ) ) ;
#49968=CARTESIAN_POINT ( 'NONE',  ( -16.52544592524342804, 4.483927247898546575, 26.04057627198103475 ) ) ;
#49969=FACE_OUTER_BOUND ( 'NONE', #79263, .T. ) ;
#49970=CARTESIAN_POINT ( 'NONE',  ( 12.14591786802327356, -12.06949235617739191, 100.6260903946857184 ) ) ;
#49972=CARTESIAN_POINT ( 'NONE',  ( 12.14591786802327356, -12.06949235617739191, 75.62609039468567573 ) ) ;
#49973=CARTESIAN_POINT ( 'NONE',  ( -5.049401038298153566, 19.05341960407611168, 35.20724293864768839 ) ) ;
#49974=CARTESIAN_POINT ( 'NONE',  ( 5.719274019375673035, 21.55341960407619339, 92.29275706135236135 ) ) ;
#49975=CARTESIAN_POINT ( 'NONE',  ( 16.51473224551083163, -9.474510206698727899, 100.8344237280190043 ) ) ;
#49976=CARTESIAN_POINT ( 'NONE',  ( -21.53943276465977519, -0.05219959533937600094, 73.75109039468567573 ) ) ;
#49977=CARTESIAN_POINT ( 'NONE',  ( -13.97604488694547697, 13.89961937509957934, 48.12609039468566863 ) ) ;
#49978=CARTESIAN_POINT ( 'NONE',  ( 9.474510206698971260, -16.51473224551069308, 72.91557627198102409 ) ) ;
#49979=CARTESIAN_POINT ( 'NONE',  ( -9.474510206698964154, 16.51473224551069663, 70.41557627198102409 ) ) ;
#49981=CARTESIAN_POINT ( 'NONE',  ( 14.29746914071049879, -8.314922557960816363, 53.33224293864769550 ) ) ;
#49982=CARTESIAN_POINT ( 'NONE',  ( -15.80617190586745835, -15.72974639402198527, 51.87390960531437401 ) ) ;
#49983=CARTESIAN_POINT ( 'NONE',  ( 0.05219959533909260263, 19.03943276465977164, 44.99890960531435979 ) ) ;
#49984=CARTESIAN_POINT ( 'NONE',  ( 10.72451020669898902, -18.67979575497178502, 82.91557627198103830 ) ) ;
#49985=CARTESIAN_POINT ( 'NONE',  ( 16.55341960407618274, -4.379528057220086978, 71.04275706135234714 ) ) ;
#49987=CARTESIAN_POINT ( 'NONE',  ( -14.29746914071049879, 8.314922557960819915, 75.83224293864769550 ) ) ;
#49989=CARTESIAN_POINT ( 'NONE',  ( 16.52544592524335698, 4.483927247898782831, 41.45942372801901143 ) ) ;
#49990=CARTESIAN_POINT ( 'NONE',  ( -16.51473224551069308, -9.474510206698971260, 26.66557627198103120 ) ) ;
#49991=CARTESIAN_POINT ( 'NONE',  ( -19.05341960407617563, 5.049401038297882671, 63.54275706135234003 ) ) ;
#49992=CARTESIAN_POINT ( 'NONE',  ( 16.53943276465976808, -0.05219959533910856209, 73.74890960531433848 ) ) ;
#49993=CARTESIAN_POINT ( 'NONE',  ( -18.67979575497193778, 10.72451020669871902, 48.33442372801902565 ) ) ;
#49994=CARTESIAN_POINT ( 'NONE',  ( 16.51473224551069308, 9.474510206698969483, 29.16557627198103475 ) ) ;
#49995=CARTESIAN_POINT ( 'NONE',  ( -0.05219959533907301413, -21.53943276465977519, 92.49890960531436690 ) ) ;
#49996=CARTESIAN_POINT ( 'NONE',  ( -13.97604488694527625, -13.89961937509977652, 111.8739096053143243 ) ) ;
#49997=CARTESIAN_POINT ( 'NONE',  ( 14.34966873604960469, 8.224510206698951720, 89.16557627198102409 ) ) ;
#49999=CARTESIAN_POINT ( 'NONE',  ( 16.46253265017160672, -9.564922557960803928, 48.33224293864769550 ) ) ;
#50001=CARTESIAN_POINT ( 'NONE',  ( 19.05341960407617918, -5.049401038297876454, 76.04275706135230450 ) ) ;
#50002=CARTESIAN_POINT ( 'NONE',  ( -15.80617190586768217, 15.72974639402176855, 28.12609039468568284 ) ) ;
#50003=CARTESIAN_POINT ( 'NONE',  ( -5.049401038298153566, 19.05341960407611168, 70.20724293864769550 ) ) ;
#50004=CARTESIAN_POINT ( 'NONE',  ( -13.97604488694547697, 13.89961937509957934, 58.12609039468566863 ) ) ;
#50005=CARTESIAN_POINT ( 'NONE',  ( 19.03943276465977164, -0.05219959533909143690, 38.74890960531436690 ) ) ;
#50006=CARTESIAN_POINT ( 'NONE',  ( -0.05219959533910754901, -16.53943276465976808, 57.49890960531435979 ) ) ;
#50007=CARTESIAN_POINT ( 'NONE',  ( -8.224510206698948167, 14.34966873604960824, 50.41557627198103120 ) ) ;
#50008=CARTESIAN_POINT ( 'NONE',  ( -5.153800228976328057, -19.02544592524343514, 82.29057627198103830 ) ) ;
#50010=CARTESIAN_POINT ( 'NONE',  ( -21.53943276465977519, 0.05219959533907696930, 96.24890960531435269 ) ) ;
#50011=CARTESIAN_POINT ( 'NONE',  ( 13.89961937509977652, -13.97604488694527269, 78.12390960531433848 ) ) ;
#50012=CARTESIAN_POINT ( 'NONE',  ( -18.62759615963270932, 10.81492255796079327, 75.83224293864769550 ) ) ;
#50013=CARTESIAN_POINT ( 'NONE',  ( -19.03943276465977164, -0.05219959533935918106, 23.75109039468566152 ) ) ;
#50014=CARTESIAN_POINT ( 'NONE',  ( -16.46253265017160317, 9.564922557960807481, 40.83224293864769550 ) ) ;
#50015=CARTESIAN_POINT ( 'NONE',  ( -16.55341960407617563, 4.379528057220093196, 103.5427570613523613 ) ) ;
#50016=CARTESIAN_POINT ( 'NONE',  ( -16.53943276465976808, 0.05219959533911058130, 96.24890960531435269 ) ) ;
#50017=CARTESIAN_POINT ( 'NONE',  ( -5.153800228976607833, 19.02544592524334988, 107.7094237280189759 ) ) ;
#50018=VERTEX_POINT ( 'NONE', #2788 ) ;
#50019=CARTESIAN_POINT ( 'NONE',  ( -0.05219959533937732626, 21.53943276465977519, 37.50109039468568284 ) ) ;
#50020=CARTESIAN_POINT ( 'NONE',  ( 9.474510206698729675, 16.51473224551082808, 57.08442372801900433 ) ) ;
#50021=CARTESIAN_POINT ( 'NONE',  ( -8.224510206698735004, -14.34966873604973081, 109.5844237280190328 ) ) ;
#50022=CARTESIAN_POINT ( 'NONE',  ( -0.05219959533907301413, -21.53943276465977519, 67.49890960531436690 ) ) ;
#50023=CARTESIAN_POINT ( 'NONE',  ( 19.02544592524343514, -5.153800228976328945, 108.5405762719810383 ) ) ;
#50024=CARTESIAN_POINT ( 'NONE',  ( -12.06949235617756955, 12.14591786802309770, 55.62390960531436690 ) ) ;
#50025=CARTESIAN_POINT ( 'NONE',  ( -13.89961937509977652, 13.97604488694528158, 25.62390960531434558 ) ) ;
#50026=CARTESIAN_POINT ( 'NONE',  ( 16.46253265017160672, -9.564922557960803928, 28.33224293864769550 ) ) ;
#50027=CARTESIAN_POINT ( 'NONE',  ( 10.81492255796106328, -18.62759615963255655, 105.4177570613523613 ) ) ;
#50028=CARTESIAN_POINT ( 'NONE',  ( -14.34966873604972548, 8.224510206698743886, 88.33442372801901854 ) ) ;
#50029=CARTESIAN_POINT ( 'NONE',  ( -10.81492255796105439, 18.62759615963255655, 47.91775706135234714 ) ) ;
#50030=CARTESIAN_POINT ( 'NONE',  ( 12.14591786802327356, -12.06949235617739191, 40.62609039468567573 ) ) ;
#50031=CARTESIAN_POINT ( 'NONE',  ( 21.52544592524344225, -5.823673210054117533, 28.54057627198103120 ) ) ;
#50032=CARTESIAN_POINT ( 'NONE',  ( -0.05219959533909027116, -19.03943276465977164, 57.49890960531435979 ) ) ;
#50033=CARTESIAN_POINT ( 'NONE',  ( -5.719274019375665041, -21.55341960407619695, 94.79275706135234714 ) ) ;
#50034=CARTESIAN_POINT ( 'NONE',  ( 19.03943276465977164, -0.05219959533909143690, 73.74890960531435269 ) ) ;
#50036=CARTESIAN_POINT ( 'NONE',  ( -16.53943276465976808, -0.05219959533934237506, 58.75109039468568994 ) ) ;
#50037=CARTESIAN_POINT ( 'NONE',  ( -14.29746914071049879, 8.314922557960819915, 100.8322429386477097 ) ) ;
#50038=CARTESIAN_POINT ( 'NONE',  ( 16.52544592524335698, 4.483927247898782831, 111.4594237280190328 ) ) ;
#50039=CARTESIAN_POINT ( 'NONE',  ( 16.51473224551069308, 9.474510206698969483, 49.16557627198102409 ) ) ;
#50040=CARTESIAN_POINT ( 'NONE',  ( 21.55341960407619695, -5.719274019375665929, 51.04275706135234714 ) ) ;
#50041=CARTESIAN_POINT ( 'NONE',  ( 13.89961937509977652, -13.97604488694527269, 93.12390960531436690 ) ) ;
#50042=CARTESIAN_POINT ( 'NONE',  ( 5.153800228976335163, 19.02544592524342804, 74.79057627198103830 ) ) ;
#50043=CARTESIAN_POINT ( 'NONE',  ( 5.153800228976335163, 19.02544592524342804, 109.7905762719810099 ) ) ;
#50045=CARTESIAN_POINT ( 'NONE',  ( 14.29746914071049879, -8.314922557960816363, 43.33224293864769550 ) ) ;
#50046=CARTESIAN_POINT ( 'NONE',  ( -14.34966873604972548, 8.224510206698743886, 113.3344237280190328 ) ) ;
#50047=CARTESIAN_POINT ( 'NONE',  ( 12.14591786802309770, 12.06949235617756955, 34.37390960531435979 ) ) ;
#50050=CARTESIAN_POINT ( 'NONE',  ( -16.51473224551082808, 9.474510206698731452, 38.33442372801899722 ) ) ;
#50051=CARTESIAN_POINT ( 'NONE',  ( -9.474510206698964154, 16.51473224551069663, 75.41557627198103830 ) ) ;
#50052=CARTESIAN_POINT ( 'NONE',  ( -5.153800228976607833, 19.02544592524334988, 52.70942372801900433 ) ) ;
#50054=CARTESIAN_POINT ( 'NONE',  ( -16.51473224551069308, -9.474510206698971260, 66.66557627198102409 ) ) ;
#50055=CARTESIAN_POINT ( 'NONE',  ( -13.97604488694547697, 13.89961937509957934, 88.12609039468563310 ) ) ;
#50056=CARTESIAN_POINT ( 'NONE',  ( 4.379528057220092307, 16.55341960407617563, 72.29275706135236135 ) ) ;
#50059=CARTESIAN_POINT ( 'NONE',  ( 16.51473224551069308, 9.474510206698969483, 104.1655762719810241 ) ) ;
#50060=CARTESIAN_POINT ( 'NONE',  ( 15.80617190586769283, -15.72974639402175789, 25.62609039468567929 ) ) ;
#50061=CARTESIAN_POINT ( 'NONE',  ( -16.51473224551082808, 9.474510206698731452, 88.33442372801900433 ) ) ;
#50062=CARTESIAN_POINT ( 'NONE',  ( 17.48847506799967633, 5.747544572773806593, 86.67302562156719148 ) ) ;
#50063=CARTESIAN_POINT ( 'NONE',  ( 19.02544592524343514, -5.153800228976328945, 43.54057627198103120 ) ) ;
#50064=CARTESIAN_POINT ( 'NONE',  ( 9.474510206698971260, -16.51473224551069308, 87.91557627198102409 ) ) ;
#50065=CARTESIAN_POINT ( 'NONE',  ( 14.29746914071049879, -8.314922557960816363, 63.33224293864770260 ) ) ;
#50066=CARTESIAN_POINT ( 'NONE',  ( -16.46253265017160317, 9.564922557960807481, 50.83224293864770260 ) ) ;
#50067=CARTESIAN_POINT ( 'NONE',  ( 19.02544592524343514, -5.153800228976328945, 58.54057627198102409 ) ) ;
#50068=CARTESIAN_POINT ( 'NONE',  ( 13.89961937509957401, 13.97604488694547697, 66.87609039468567573 ) ) ;
#50069=CARTESIAN_POINT ( 'NONE',  ( -5.153800228976607833, 19.02544592524334988, 27.70942372801899722 ) ) ;
#50070=CARTESIAN_POINT ( 'NONE',  ( 5.153800228976335163, 19.02544592524342804, 59.79057627198100988 ) ) ;
#50071=CARTESIAN_POINT ( 'NONE',  ( 10.81492255796078972, 18.62759615963270932, 64.58224293864769550 ) ) ;
#50072=CARTESIAN_POINT ( 'NONE',  ( -16.52544592524342804, 4.483927247898546575, 66.04057627198103830 ) ) ;
#50073=CARTESIAN_POINT ( 'NONE',  ( 9.474510206698729675, 16.51473224551082808, 37.08442372801899722 ) ) ;
#50074=CARTESIAN_POINT ( 'NONE',  ( 18.22780087662122384, -5.500000000000022204, 86.01540105326108687 ) ) ;
#50075=CARTESIAN_POINT ( 'NONE',  ( -21.55341960407610458, -5.719274019375992779, 51.45724293864770260 ) ) ;
#50076=CARTESIAN_POINT ( 'NONE',  ( 15.72974639402199770, -15.80617190586745480, 28.12390960531435979 ) ) ;
#50077=CARTESIAN_POINT ( 'NONE',  ( 5.153800228976335163, 19.02544592524342804, 54.79057627198103120 ) ) ;
#50078=CARTESIAN_POINT ( 'NONE',  ( 16.51473224551069308, 9.474510206698969483, 39.16557627198103120 ) ) ;
#50079=CARTESIAN_POINT ( 'NONE',  ( -0.05219959533910754901, -16.53943276465976808, 107.4989096053143669 ) ) ;
#50080=CARTESIAN_POINT ( 'NONE',  ( -21.53943276465977519, 0.05219959533907696930, 106.2489096053143811 ) ) ;
#50082=CARTESIAN_POINT ( 'NONE',  ( 21.53943276465977519, 0.05219959533937863772, 31.25109039468568639 ) ) ;
#50083=CARTESIAN_POINT ( 'NONE',  ( -8.224510206698948167, 14.34966873604960824, 110.4155762719810383 ) ) ;
#50084=CARTESIAN_POINT ( 'NONE',  ( 18.62759615963255655, 10.81492255796105972, 81.66775706135236135 ) ) ;
#50085=CARTESIAN_POINT ( 'NONE',  ( -0.05219959533907301413, -21.53943276465977519, 87.49890960531436690 ) ) ;
#50086=CARTESIAN_POINT ( 'NONE',  ( 19.02544592524334988, 5.153800228976608722, 36.45942372801900433 ) ) ;
#50087=CARTESIAN_POINT ( 'NONE',  ( 16.51473224551069308, 9.474510206698969483, 29.16557627198103475 ) ) ;
#50090=CARTESIAN_POINT ( 'NONE',  ( 0.05219959533934541429, -16.53943276465976808, 45.00109039468568284 ) ) ;
#50091=CARTESIAN_POINT ( 'NONE',  ( 4.379528057220339221, -16.55341960407611168, 112.7072429386476955 ) ) ;
#50093=CARTESIAN_POINT ( 'NONE',  ( -9.564922557960796823, -16.46253265017161027, 72.08224293864770971 ) ) ;
#50094=CARTESIAN_POINT ( 'NONE',  ( 16.53943276465976808, -0.05219959533910856209, 93.74890960531436690 ) ) ;
#50095=CARTESIAN_POINT ( 'NONE',  ( -21.55341960407610458, -5.719274019375992779, 46.45724293864769550 ) ) ;
#50096=CARTESIAN_POINT ( 'NONE',  ( 16.53943276465976808, -0.05219959533910856209, 83.74890960531435269 ) ) ;
#50097=CARTESIAN_POINT ( 'NONE',  ( 8.314922557961029526, -14.29746914071037800, 35.41775706135234003 ) ) ;
#50098=CARTESIAN_POINT ( 'NONE',  ( 21.52544592524334988, 5.823673210054432836, 91.45942372801901854 ) ) ;
#50099=CARTESIAN_POINT ( 'NONE',  ( -9.564922557961040184, 16.46253265017147172, 62.91775706135233293 ) ) ;
#50100=CARTESIAN_POINT ( 'NONE',  ( -4.379528057220086978, -16.55341960407618274, 99.79275706135234714 ) ) ;
#50101=CARTESIAN_POINT ( 'NONE',  ( -8.314922557960811034, -14.29746914071050412, 42.08224293864769550 ) ) ;
#50102=CARTESIAN_POINT ( 'NONE',  ( 13.89961937509977652, -13.97604488694527269, 48.12390960531435979 ) ) ;
#50103=CARTESIAN_POINT ( 'NONE',  ( -0.05219959533937732626, 21.53943276465977519, 97.50109039468567573 ) ) ;
#50104=CARTESIAN_POINT ( 'NONE',  ( -21.52544592524343514, 5.823673210054127303, 111.0405762719810525 ) ) ;
#50105=CARTESIAN_POINT ( 'NONE',  ( -21.55341960407619339, 5.719274019375674811, 53.54275706135234714 ) ) ;
#50106=CARTESIAN_POINT ( 'NONE',  ( -16.55341960407617563, 4.379528057220093196, 43.54275706135235424 ) ) ;
#50107=CARTESIAN_POINT ( 'NONE',  ( 8.314922557960818139, 14.29746914071049879, 64.58224293864769550 ) ) ;
#50108=CARTESIAN_POINT ( 'NONE',  ( 5.823673210054444382, -21.52544592524334988, 85.20942372801901854 ) ) ;
#50109=CARTESIAN_POINT ( 'NONE',  ( 4.483927247898790824, -16.52544592524335698, 110.2094237280190185 ) ) ;
#50110=CARTESIAN_POINT ( 'NONE',  ( 16.20579543436696213, -7.371946100355080134, 46.93479165828048849 ) ) ;
#50111=DIRECTION ( 'NONE',  ( -0.000000000000000000, 0.000000000000000000, -1.000000000000000000 ) ) ;
#50112=CARTESIAN_POINT ( 'NONE',  ( 16.55341960407611168, 4.379528057220329451, 33.95724293864769550 ) ) ;
#50113=CARTESIAN_POINT ( 'NONE',  ( 0.05219959533934541429, -16.53943276465976808, 80.00109039468568994 ) ) ;
#50114=CARTESIAN_POINT ( 'NONE',  ( -5.049401038298153566, 19.05341960407611168, 80.20724293864769550 ) ) ;
#50115=CARTESIAN_POINT ( 'NONE',  ( -13.97604488694527625, -13.89961937509977652, 96.87390960531433848 ) ) ;
#50116=CARTESIAN_POINT ( 'NONE',  ( -21.52544592524334988, -5.823673210054445271, 88.95942372801901854 ) ) ;
#50117=CARTESIAN_POINT ( 'NONE',  ( -16.55341960407617563, 4.379528057220093196, 83.54275706135234714 ) ) ;
#50118=CARTESIAN_POINT ( 'NONE',  ( 4.483927247898545687, 16.52544592524342804, 79.79057627198102409 ) ) ;
#50119=CARTESIAN_POINT ( 'NONE',  ( 16.46253265017160672, -9.564922557960803928, 73.33224293864769550 ) ) ;
#50121=CARTESIAN_POINT ( 'NONE',  ( -14.29746914071037622, -8.314922557961029526, 24.16775706135235424 ) ) ;
#50122=CARTESIAN_POINT ( 'NONE',  ( -5.153800228976328057, -19.02544592524343514, 22.29057627198102765 ) ) ;
#50123=CARTESIAN_POINT ( 'NONE',  ( 13.89961937509977652, -13.97604488694527269, 98.12390960531433848 ) ) ;
#50124=CARTESIAN_POINT ( 'NONE',  ( 14.34966873604972726, -8.224510206698740333, 25.83442372801901499 ) ) ;
#50126=CARTESIAN_POINT ( 'NONE',  ( -13.89961937509957401, -13.97604488694547875, 24.37609039468565442 ) ) ;
#50127=CARTESIAN_POINT ( 'NONE',  ( -14.29746914071037622, -8.314922557961029526, 94.16775706135237556 ) ) ;
#50128=CARTESIAN_POINT ( 'NONE',  ( 9.564922557961047289, -16.46253265017146816, 105.4177570613523471 ) ) ;
#50129=CARTESIAN_POINT ( 'NONE',  ( 16.52544592524342804, -4.483927247898539470, 113.5405762719810383 ) ) ;
#50130=CARTESIAN_POINT ( 'NONE',  ( 4.379528057220092307, 16.55341960407617563, 77.29275706135234714 ) ) ;
#50131=CARTESIAN_POINT ( 'NONE',  ( -16.55341960407617563, 4.379528057220093196, 73.54275706135234714 ) ) ;
#50133=CARTESIAN_POINT ( 'NONE',  ( -5.153800228976607833, 19.02544592524334988, 72.70942372801900433 ) ) ;
#50135=CARTESIAN_POINT ( 'NONE',  ( -21.53943276465977519, -0.05219959533937600094, 113.7510903946856757 ) ) ;
#50136=CARTESIAN_POINT ( 'NONE',  ( 16.51473224551069308, 9.474510206698969483, 54.16557627198103120 ) ) ;
#50137=CARTESIAN_POINT ( 'NONE',  ( 13.89961937509977652, -13.97604488694527269, 78.12390960531433848 ) ) ;
#50138=CARTESIAN_POINT ( 'NONE',  ( -4.483927247898539470, -16.52544592524342804, 82.29057627198103830 ) ) ;
#50139=CARTESIAN_POINT ( 'NONE',  ( 19.05341960407617918, -5.049401038297876454, 61.04275706135232582 ) ) ;
#50140=CARTESIAN_POINT ( 'NONE',  ( -21.52544592524343514, 5.823673210054127303, 46.04057627198103830 ) ) ;
#50141=CARTESIAN_POINT ( 'NONE',  ( 15.80617190586769283, -15.72974639402175789, 105.6260903946856899 ) ) ;
#50142=CARTESIAN_POINT ( 'NONE',  ( 13.97604488694527802, 13.89961937509977652, 89.37390960531436690 ) ) ;
#50143=CARTESIAN_POINT ( 'NONE',  ( 0.05219959533937995610, -21.53943276465977519, 105.0010903946856757 ) ) ;
#50144=CARTESIAN_POINT ( 'NONE',  ( 21.52544592524344225, -5.823673210054117533, 58.54057627198103120 ) ) ;
#50145=CARTESIAN_POINT ( 'NONE',  ( 19.02544592524343514, -5.153800228976328945, 103.5405762719809957 ) ) ;
#50146=CARTESIAN_POINT ( 'NONE',  ( -19.03943276465977164, -0.05219959533935918106, 93.75109039468566152 ) ) ;
#50147=CARTESIAN_POINT ( 'NONE',  ( -0.05219959533909027116, -19.03943276465977164, 107.4989096053143527 ) ) ;
#50148=ADVANCED_FACE ( 'NONE', ( #81585 ), #184828, .T. ) ;
#50149=CARTESIAN_POINT ( 'NONE',  ( -19.02544592524334988, -5.153800228976617603, 103.9594237280190043 ) ) ;
#50150=CARTESIAN_POINT ( 'NONE',  ( 12.14591786802309770, 12.06949235617756955, 114.3739096053143527 ) ) ;
#50151=CARTESIAN_POINT ( 'NONE',  ( -13.97604488694527625, -13.89961937509977652, 86.87390960531436690 ) ) ;
#50152=CARTESIAN_POINT ( 'NONE',  ( -15.80617190586745835, -15.72974639402198527, 76.87390960531439532 ) ) ;
#50153=CARTESIAN_POINT ( 'NONE',  ( 0.05219959533934541429, -16.53943276465976808, 40.00109039468567573 ) ) ;
#50154=CARTESIAN_POINT ( 'NONE',  ( -18.67979575497193778, 10.72451020669871902, 48.33442372801902565 ) ) ;
#50155=CARTESIAN_POINT ( 'NONE',  ( -18.67979575497193778, 10.72451020669871902, 103.3344237280190043 ) ) ;
#50156=CARTESIAN_POINT ( 'NONE',  ( 16.53943276465976808, 0.05219959533934440121, 96.25109039468568994 ) ) ;
#50157=CARTESIAN_POINT ( 'NONE',  ( -19.05341960407611168, -5.049401038298163336, 91.45724293864766707 ) ) ;
#50158=CARTESIAN_POINT ( 'NONE',  ( -8.224510206698948167, 14.34966873604960824, 95.41557627198102409 ) ) ;
#50159=CARTESIAN_POINT ( 'NONE',  ( -12.14591786802326823, 12.06949235617739902, 113.1260903946856899 ) ) ;
#50160=CARTESIAN_POINT ( 'NONE',  ( -16.46253265017146816, -9.564922557961047289, 69.16775706135233293 ) ) ;
#50161=CARTESIAN_POINT ( 'NONE',  ( -10.72451020669870658, -18.67979575497194134, 44.58442372801901854 ) ) ;
#50163=CARTESIAN_POINT ( 'NONE',  ( 16.55341960407611168, 4.379528057220329451, 88.95724293864769550 ) ) ;
#50164=CARTESIAN_POINT ( 'NONE',  ( -13.89961937509977652, 13.97604488694528158, 115.6239096053143669 ) ) ;
#50165=CARTESIAN_POINT ( 'NONE',  ( 14.29746914071049879, -8.314922557960816363, 23.33224293864769194 ) ) ;
#50166=CARTESIAN_POINT ( 'NONE',  ( -18.62759615963255300, -10.81492255796106328, 89.16775706135236135 ) ) ;
#50167=CARTESIAN_POINT ( 'NONE',  ( -16.52544592524335698, -4.483927247898792601, 63.95942372801901854 ) ) ;
#50168=CARTESIAN_POINT ( 'NONE',  ( 16.52544592524335698, 4.483927247898782831, 111.4594237280190328 ) ) ;
#50169=CARTESIAN_POINT ( 'NONE',  ( -5.823673210054431948, 21.52544592524334988, 37.70942372801900433 ) ) ;
#50171=CARTESIAN_POINT ( 'NONE',  ( 15.72974639402176855, 15.80617190586768217, 31.87609039468567929 ) ) ;
#50172=CARTESIAN_POINT ( 'NONE',  ( 16.53943276465976808, -0.05219959533910856209, 103.7489096053143669 ) ) ;
#50173=CARTESIAN_POINT ( 'NONE',  ( -13.97604488694527625, -13.89961937509977652, 26.87390960531434558 ) ) ;
#50174=CARTESIAN_POINT ( 'NONE',  ( -14.34966873604960291, -8.224510206698953496, 61.66557627198103120 ) ) ;
#50175=CARTESIAN_POINT ( 'NONE',  ( -13.97604488694527625, -13.89961937509977652, 71.87390960531433848 ) ) ;
#50176=CARTESIAN_POINT ( 'NONE',  ( 16.55341960407618274, -4.379528057220086978, 101.0427570613523756 ) ) ;
#50177=CARTESIAN_POINT ( 'NONE',  ( 19.02544592524343514, -5.153800228976328945, 38.54057627198103120 ) ) ;
#50178=CARTESIAN_POINT ( 'NONE',  ( 21.52544592524344225, -5.823673210054117533, 43.54057627198103830 ) ) ;
#50179=CARTESIAN_POINT ( 'NONE',  ( -14.34966873604960291, -8.224510206698953496, 91.66557627198103830 ) ) ;
#50181=CARTESIAN_POINT ( 'NONE',  ( 15.80617190586746368, 15.72974639402197994, 89.37390960531435269 ) ) ;
#50182=CARTESIAN_POINT ( 'NONE',  ( -19.05341960407611168, -5.049401038298163336, 86.45724293864769550 ) ) ;
#50183=CARTESIAN_POINT ( 'NONE',  ( -19.03943276465977164, 0.05219959533909376836, 46.24890960531435979 ) ) ;
#50184=CARTESIAN_POINT ( 'NONE',  ( -19.05341960407617563, 5.049401038297882671, 88.54275706135230450 ) ) ;
#50185=CARTESIAN_POINT ( 'NONE',  ( -18.62759615963270932, 10.81492255796079327, 50.83224293864770971 ) ) ;
#50186=CARTESIAN_POINT ( 'NONE',  ( -5.719274019375665041, -21.55341960407619695, 74.79275706135234714 ) ) ;
#50187=CARTESIAN_POINT ( 'NONE',  ( -5.049401038298153566, 19.05341960407611168, 50.20724293864770260 ) ) ;
#50188=CARTESIAN_POINT ( 'NONE',  ( 16.51473224551069308, 9.474510206698969483, 79.16557627198103830 ) ) ;
#50190=CARTESIAN_POINT ( 'NONE',  ( -12.14591786802326823, 12.06949235617739902, 58.12609039468568994 ) ) ;
#50191=CARTESIAN_POINT ( 'NONE',  ( -21.55341960407619339, 5.719274019375674811, 48.54275706135234714 ) ) ;
#50193=CARTESIAN_POINT ( 'NONE',  ( -15.72974639402176322, -15.80617190586768395, 79.37609039468567573 ) ) ;
#50194=CARTESIAN_POINT ( 'NONE',  ( -19.05341960407611168, -5.049401038298163336, 111.4572429386476671 ) ) ;
#50195=CARTESIAN_POINT ( 'NONE',  ( 15.80617190586746368, 15.72974639402197994, 94.37390960531436690 ) ) ;
#50196=CARTESIAN_POINT ( 'NONE',  ( -0.05219959533937732626, 21.53943276465977519, 42.50109039468567573 ) ) ;
#50197=CARTESIAN_POINT ( 'NONE',  ( -8.224510206698735004, -14.34966873604973081, 69.58442372801900433 ) ) ;
#50198=CARTESIAN_POINT ( 'NONE',  ( 10.81492255796078972, 18.62759615963270932, 59.58224293864770260 ) ) ;
#50199=CARTESIAN_POINT ( 'NONE',  ( -5.153800228976607833, 19.02544592524334988, 37.70942372801899722 ) ) ;
#50200=AXIS2_PLACEMENT_3D ( 'NONE', #36288, #112152, #53464 ) ;
#50201=CARTESIAN_POINT ( 'NONE',  ( 19.05341960407611168, 5.049401038298154454, 73.95724293864768129 ) ) ;
#50202=CARTESIAN_POINT ( 'NONE',  ( 12.06949235617739724, 12.14591786802326823, 106.8760903946856899 ) ) ;
#50204=CARTESIAN_POINT ( 'NONE',  ( -9.564922557960796823, -16.46253265017161027, 107.0822429386476955 ) ) ;
#50206=CARTESIAN_POINT ( 'NONE',  ( -19.03943276465977164, -0.05219959533935918106, 78.75109039468567573 ) ) ;
#50208=CARTESIAN_POINT ( 'NONE',  ( -18.62759615963270932, 10.81492255796079327, 55.83224293864770260 ) ) ;
#50209=CARTESIAN_POINT ( 'NONE',  ( -4.379528057220328563, 16.55341960407611168, 35.20724293864768839 ) ) ;
#50210=CARTESIAN_POINT ( 'NONE',  ( -16.46253265017146816, -9.564922557961047289, 94.16775706135233293 ) ) ;
#50211=CARTESIAN_POINT ( 'NONE',  ( 13.89961937509977652, -13.97604488694527269, 28.12390960531435624 ) ) ;
#50212=CARTESIAN_POINT ( 'NONE',  ( -13.97604488694547697, 13.89961937509957934, 113.1260903946856757 ) ) ;
#50213=CARTESIAN_POINT ( 'NONE',  ( -5.719274019375978568, 21.55341960407610458, 85.20724293864770971 ) ) ;
#50214=CARTESIAN_POINT ( 'NONE',  ( 9.564922557961047289, -16.46253265017146816, 55.41775706135234003 ) ) ;
#50215=CARTESIAN_POINT ( 'NONE',  ( -0.05219959533934338120, 16.53943276465976808, 82.50109039468568994 ) ) ;
#50216=CARTESIAN_POINT ( 'NONE',  ( -13.89961937509977652, 13.97604488694528158, 65.62390960531436690 ) ) ;
#50217=CARTESIAN_POINT ( 'NONE',  ( -14.34966873604960291, -8.224510206698953496, 76.66557627198103830 ) ) ;
#50218=CARTESIAN_POINT ( 'NONE',  ( -0.05219959533909027116, -19.03943276465977164, 47.49890960531435979 ) ) ;
#50219=CARTESIAN_POINT ( 'NONE',  ( 12.14591786802309770, 12.06949235617756955, 49.37390960531436690 ) ) ;
#50222=CARTESIAN_POINT ( 'NONE',  ( -12.14591786802309592, -12.06949235617757132, 26.87390960531435979 ) ) ;
#50223=CARTESIAN_POINT ( 'NONE',  ( 0.05219959533909260263, 19.03943276465977164, 74.99890960531435269 ) ) ;
#50225=CARTESIAN_POINT ( 'NONE',  ( 19.03943276465977164, 0.05219959533936151252, 36.25109039468567573 ) ) ;
#50226=CARTESIAN_POINT ( 'NONE',  ( -4.483927247898782831, 16.52544592524335698, 52.70942372801902565 ) ) ;
#50227=CARTESIAN_POINT ( 'NONE',  ( -15.72974639402197994, 15.80617190586746368, 50.62390960531435979 ) ) ;
#50228=CARTESIAN_POINT ( 'NONE',  ( -10.81492255796105439, 18.62759615963255655, 112.9177570613523329 ) ) ;
#50229=CARTESIAN_POINT ( 'NONE',  ( -19.03943276465977164, 0.05219959533909376836, 76.24890960531435269 ) ) ;
#50230=CARTESIAN_POINT ( 'NONE',  ( -5.049401038298153566, 19.05341960407611168, 115.2072429386477097 ) ) ;
#50231=CARTESIAN_POINT ( 'NONE',  ( -0.05219959533909027116, -19.03943276465977164, 107.4989096053143527 ) ) ;
#50232=CARTESIAN_POINT ( 'NONE',  ( -5.719274019375665041, -21.55341960407619695, 44.79275706135234714 ) ) ;
#50233=CARTESIAN_POINT ( 'NONE',  ( -4.483927247898539470, -16.52544592524342804, 112.2905762719810241 ) ) ;
#50234=CARTESIAN_POINT ( 'NONE',  ( -18.62759615963270932, 10.81492255796079327, 100.8322429386477097 ) ) ;
#50235=CARTESIAN_POINT ( 'NONE',  ( -19.03943276465977164, 0.05219959533909376836, 76.24890960531435269 ) ) ;
#50237=CARTESIAN_POINT ( 'NONE',  ( -0.05219959533937732626, 21.53943276465977519, 32.50109039468568284 ) ) ;
#50239=CARTESIAN_POINT ( 'NONE',  ( 19.05341960407611168, 5.049401038298154454, 83.95724293864766707 ) ) ;
#50240=CARTESIAN_POINT ( 'NONE',  ( 19.52837319214028611, -5.499999999999892530, 82.10471352585541638 ) ) ;
#50241=CARTESIAN_POINT ( 'NONE',  ( -16.53943276465976808, 0.05219959533911058130, 116.2489096053143669 ) ) ;
#50242=CARTESIAN_POINT ( 'NONE',  ( -13.89961937509977652, 13.97604488694528158, 30.62390960531435269 ) ) ;
#50243=CARTESIAN_POINT ( 'NONE',  ( -19.02544592524334988, -5.153800228976617603, 103.9594237280190043 ) ) ;
#50245=CARTESIAN_POINT ( 'NONE',  ( -8.224510206698948167, 14.34966873604960824, 115.4155762719810241 ) ) ;
#50246=CARTESIAN_POINT ( 'NONE',  ( 10.81492255796106328, -18.62759615963255655, 80.41775706135234714 ) ) ;
#50247=CARTESIAN_POINT ( 'NONE',  ( -19.05341960407611168, -5.049401038298163336, 56.45724293864768129 ) ) ;
#50248=CARTESIAN_POINT ( 'NONE',  ( -0.05219959533937732626, 21.53943276465977519, 27.50109039468567929 ) ) ;
#50249=CARTESIAN_POINT ( 'NONE',  ( 10.72451020669871369, 18.67979575497193778, 32.08442372801901854 ) ) ;
#50251=CARTESIAN_POINT ( 'NONE',  ( 19.05341960407611168, 5.049401038298154454, 83.95724293864766707 ) ) ;
#50253=CARTESIAN_POINT ( 'NONE',  ( -8.224510206698735004, -14.34966873604973081, 29.58442372801901854 ) ) ;
#50254=CARTESIAN_POINT ( 'NONE',  ( 21.55341960407610458, 5.719274019375980345, 38.95724293864768839 ) ) ;
#50255=CARTESIAN_POINT ( 'NONE',  ( -18.62759615963255300, -10.81492255796106328, 74.16775706135231871 ) ) ;
#50256=CARTESIAN_POINT ( 'NONE',  ( -16.51473224551069308, -9.474510206698971260, 106.6655762719810383 ) ) ;
#50257=CARTESIAN_POINT ( 'NONE',  ( -19.03943276465977164, -0.05219959533935918106, 93.75109039468566152 ) ) ;
#50258=CARTESIAN_POINT ( 'NONE',  ( -19.02544592524342804, 5.153800228976336051, 61.04057627198103120 ) ) ;
#50259=CARTESIAN_POINT ( 'NONE',  ( -5.049401038298153566, 19.05341960407611168, 85.20724293864766707 ) ) ;
#50260=CARTESIAN_POINT ( 'NONE',  ( 16.52544592524342804, -4.483927247898539470, 88.54057627198103830 ) ) ;
#50261=CARTESIAN_POINT ( 'NONE',  ( 16.52544592524342804, -4.483927247898539470, 103.5405762719810383 ) ) ;
#50262=CARTESIAN_POINT ( 'NONE',  ( -13.89961937509977652, 13.97604488694528158, 105.6239096053143527 ) ) ;
#50263=CARTESIAN_POINT ( 'NONE',  ( 14.34966873604972726, -8.224510206698740333, 75.83442372801900433 ) ) ;
#50264=CARTESIAN_POINT ( 'NONE',  ( 4.483927247898545687, 16.52544592524342804, 54.79057627198104541 ) ) ;
#50265=CARTESIAN_POINT ( 'NONE',  ( 9.564922557960805705, 16.46253265017160317, 44.58224293864769550 ) ) ;
#50266=CARTESIAN_POINT ( 'NONE',  ( -5.719274019375665041, -21.55341960407619695, 69.79275706135234714 ) ) ;
#50267=CARTESIAN_POINT ( 'NONE',  ( 13.97604488694548053, -13.89961937509957401, 95.62609039468563310 ) ) ;
#50268=CARTESIAN_POINT ( 'NONE',  ( 8.314922557960818139, 14.29746914071049879, 64.58224293864769550 ) ) ;
#50269=CARTESIAN_POINT ( 'NONE',  ( 18.62759615963255655, 10.81492255796105972, 21.66775706135235069 ) ) ;
#50270=CARTESIAN_POINT ( 'NONE',  ( -15.72974639402197994, 15.80617190586746368, 50.62390960531435979 ) ) ;
#50273=CARTESIAN_POINT ( 'NONE',  ( 19.05341960407611168, 5.049401038298154454, 73.95724293864768129 ) ) ;
#50274=CARTESIAN_POINT ( 'NONE',  ( -12.14591786802309592, -12.06949235617757132, 36.87390960531435979 ) ) ;
#50275=CARTESIAN_POINT ( 'NONE',  ( 12.06949235617739724, 12.14591786802326823, 111.8760903946856615 ) ) ;
#50276=CARTESIAN_POINT ( 'NONE',  ( 4.379528057220092307, 16.55341960407617563, 87.29275706135236135 ) ) ;
#50277=CARTESIAN_POINT ( 'NONE',  ( 5.153800228976615827, -19.02544592524334988, 35.20942372801899722 ) ) ;
#50280=CARTESIAN_POINT ( 'NONE',  ( -13.97604488694527625, -13.89961937509977652, 96.87390960531433848 ) ) ;
#50281=CARTESIAN_POINT ( 'NONE',  ( -8.314922557960811034, -14.29746914071050412, 67.08224293864770971 ) ) ;
#50282=CARTESIAN_POINT ( 'NONE',  ( 0.05219959533909260263, 19.03943276465977164, 24.99890960531435269 ) ) ;
#50283=CARTESIAN_POINT ( 'NONE',  ( -18.67979575497178146, -10.72451020669898902, 21.66557627198102409 ) ) ;
#50284=CARTESIAN_POINT ( 'NONE',  ( -5.719274019375978568, 21.55341960407610458, 50.20724293864769550 ) ) ;
#50286=CARTESIAN_POINT ( 'NONE',  ( 16.53943276465976808, -0.05219959533910856209, 78.74890960531436690 ) ) ;
#50287=CARTESIAN_POINT ( 'NONE',  ( -16.52544592524335698, -4.483927247898792601, 33.95942372801901143 ) ) ;
#50288=CARTESIAN_POINT ( 'NONE',  ( 12.06949235617757843, -12.14591786802309237, 83.12390960531436690 ) ) ;
#50289=CARTESIAN_POINT ( 'NONE',  ( -17.49999999999999645, -5.500000000000000888, 120.0000000000000142 ) ) ;
#50290=CARTESIAN_POINT ( 'NONE',  ( -19.02544592524334988, -5.153800228976617603, 83.95942372801901854 ) ) ;
#50291=CARTESIAN_POINT ( 'NONE',  ( -5.719274019375978568, 21.55341960407610458, 25.20724293864769550 ) ) ;
#50294=CARTESIAN_POINT ( 'NONE',  ( 4.379528057220092307, 16.55341960407617563, 27.29275706135234358 ) ) ;
#50295=CARTESIAN_POINT ( 'NONE',  ( 16.52544592524342804, -4.483927247898539470, 33.54057627198102409 ) ) ;
#50296=CARTESIAN_POINT ( 'NONE',  ( 19.02544592524334988, 5.153800228976608722, 66.45942372801899012 ) ) ;
#50297=CARTESIAN_POINT ( 'NONE',  ( 5.719274019375991003, -21.55341960407610458, 47.70724293864770260 ) ) ;
#50298=CARTESIAN_POINT ( 'NONE',  ( -18.67979575497193778, 10.72451020669871902, 68.33442372801900433 ) ) ;
#50300=CARTESIAN_POINT ( 'NONE',  ( -12.14591786802326823, 12.06949235617739902, 33.12609039468569705 ) ) ;
#50301=CARTESIAN_POINT ( 'NONE',  ( -13.89961937509977652, 13.97604488694528158, 25.62390960531434558 ) ) ;
#50302=CARTESIAN_POINT ( 'NONE',  ( 16.46253265017160672, -9.564922557960803928, 83.33224293864768129 ) ) ;
#50303=CARTESIAN_POINT ( 'NONE',  ( 19.03943276465977164, -0.05219959533909143690, 28.74890960531435624 ) ) ;
#50304=CARTESIAN_POINT ( 'NONE',  ( 16.55341960407611168, 4.379528057220329451, 98.95724293864770971 ) ) ;
#50306=CARTESIAN_POINT ( 'NONE',  ( 16.51473224551069308, 9.474510206698969483, 104.1655762719810241 ) ) ;
#50307=ORIENTED_EDGE ( 'NONE', *, *, #199845, .T. ) ;
#50308=CARTESIAN_POINT ( 'NONE',  ( -4.483927247898782831, 16.52544592524335698, 57.70942372801901143 ) ) ;
#50309=CARTESIAN_POINT ( 'NONE',  ( 16.51473224551083163, -9.474510206698727899, 110.8344237280190043 ) ) ;
#50310=CARTESIAN_POINT ( 'NONE',  ( 18.62759615963271287, -10.81492255796078972, 73.33224293864769550 ) ) ;
#50311=CARTESIAN_POINT ( 'NONE',  ( 16.51473224551069308, 9.474510206698969483, 44.16557627198103120 ) ) ;
#50312=CARTESIAN_POINT ( 'NONE',  ( 16.51473224551083163, -9.474510206698727899, 70.83442372801900433 ) ) ;
#50313=CARTESIAN_POINT ( 'NONE',  ( 10.72451020669898902, -18.67979575497178502, 107.9155762719810241 ) ) ;
#50314=CARTESIAN_POINT ( 'NONE',  ( -13.97604488694527625, -13.89961937509977652, 66.87390960531436690 ) ) ;
#50315=CARTESIAN_POINT ( 'NONE',  ( -9.474510206698964154, 16.51473224551069663, 100.4155762719810241 ) ) ;
#50316=EDGE_CURVE ( 'NONE', #133003, #43212, #23073, .T. ) ;
#50317=ORIENTED_EDGE ( 'NONE', *, *, #157780, .F. ) ;
#50318=CARTESIAN_POINT ( 'NONE',  ( 16.55341960407618274, -4.379528057220086978, 36.04275706135234714 ) ) ;
#50319=CARTESIAN_POINT ( 'NONE',  ( 10.72451020669898902, -18.67979575497178502, 97.91557627198103830 ) ) ;
#50320=CARTESIAN_POINT ( 'NONE',  ( -12.06949235617756955, 12.14591786802309770, 110.6239096053143669 ) ) ;
#50321=CARTESIAN_POINT ( 'NONE',  ( 19.03943276465977164, -0.05219959533909143690, 88.74890960531436690 ) ) ;
#50322=CARTESIAN_POINT ( 'NONE',  ( -16.51473224551082808, 9.474510206698731452, 78.33442372801900433 ) ) ;
#50323=CARTESIAN_POINT ( 'NONE',  ( -15.72974639402197994, 15.80617190586746368, 80.62390960531438111 ) ) ;
#50324=CARTESIAN_POINT ( 'NONE',  ( 4.379528057220339221, -16.55341960407611168, 47.70724293864770260 ) ) ;
#50325=CARTESIAN_POINT ( 'NONE',  ( -21.53943276465977519, -0.05219959533937600094, 113.7510903946856757 ) ) ;
#50326=CARTESIAN_POINT ( 'NONE',  ( -4.483927247898782831, 16.52544592524335698, 77.70942372801900433 ) ) ;
#50327=CARTESIAN_POINT ( 'NONE',  ( 19.05341960407611168, 5.049401038298154454, 88.95724293864769550 ) ) ;
#50328=CARTESIAN_POINT ( 'NONE',  ( -13.97604488694527625, -13.89961937509977652, 51.87390960531436690 ) ) ;
#50329=CARTESIAN_POINT ( 'NONE',  ( -15.80617190586768217, 15.72974639402176855, 58.12609039468568994 ) ) ;
#50330=CARTESIAN_POINT ( 'NONE',  ( 5.823673210054444382, -21.52544592524334988, 70.20942372801904696 ) ) ;
#50331=CARTESIAN_POINT ( 'NONE',  ( -9.564922557960796823, -16.46253265017161027, 67.08224293864769550 ) ) ;
#50332=CARTESIAN_POINT ( 'NONE',  ( -5.719274019375665041, -21.55341960407619695, 34.79275706135235424 ) ) ;
#50333=CARTESIAN_POINT ( 'NONE',  ( 16.46253265017146816, 9.564922557961045513, 91.66775706135234714 ) ) ;
#50334=CARTESIAN_POINT ( 'NONE',  ( -16.46253265017160317, 9.564922557960807481, 35.83224293864768839 ) ) ;
#50335=CARTESIAN_POINT ( 'NONE',  ( -4.379528057220086978, -16.55341960407618274, 84.79275706135234714 ) ) ;
#50336=CARTESIAN_POINT ( 'NONE',  ( -0.05219959533909027116, -19.03943276465977164, 62.49890960531435979 ) ) ;
#50337=CARTESIAN_POINT ( 'NONE',  ( 9.474510206698971260, -16.51473224551069308, 107.9155762719810383 ) ) ;
#50338=CARTESIAN_POINT ( 'NONE',  ( -9.564922557960796823, -16.46253265017161027, 37.08224293864768839 ) ) ;
#50339=CARTESIAN_POINT ( 'NONE',  ( -10.72451020669898014, 18.67979575497178502, 80.41557627198103830 ) ) ;
#50340=CARTESIAN_POINT ( 'NONE',  ( -4.483927247898782831, 16.52544592524335698, 77.70942372801900433 ) ) ;
#50342=CARTESIAN_POINT ( 'NONE',  ( -13.97604488694547697, 13.89961937509957934, 33.12609039468566863 ) ) ;
#50343=CARTESIAN_POINT ( 'NONE',  ( 19.05341960407611168, 5.049401038298154454, 68.95724293864769550 ) ) ;
#50344=CARTESIAN_POINT ( 'NONE',  ( -14.34966873604960291, -8.224510206698953496, 46.66557627198102409 ) ) ;
#50345=CARTESIAN_POINT ( 'NONE',  ( -16.53943276465976808, 0.05219959533911058130, 81.24890960531436690 ) ) ;
#50346=CARTESIAN_POINT ( 'NONE',  ( -19.02544592524342804, 5.153800228976336051, 101.0405762719810241 ) ) ;
#50347=CARTESIAN_POINT ( 'NONE',  ( 19.02544592524343514, -5.153800228976328945, 93.54057627198102409 ) ) ;
#50348=CARTESIAN_POINT ( 'NONE',  ( -21.55341960407619339, 5.719274019375674811, 48.54275706135234714 ) ) ;
#50349=CARTESIAN_POINT ( 'NONE',  ( 16.51473224551069308, 9.474510206698969483, 109.1655762719810383 ) ) ;
#50350=CARTESIAN_POINT ( 'NONE',  ( -21.52544592524334988, -5.823673210054445271, 108.9594237280190185 ) ) ;
#50351=CARTESIAN_POINT ( 'NONE',  ( -14.29746914071037622, -8.314922557961029526, 79.16775706135234714 ) ) ;
#50352=CARTESIAN_POINT ( 'NONE',  ( 10.72451020669871369, 18.67979575497193778, 27.08442372801901854 ) ) ;
#50353=CARTESIAN_POINT ( 'NONE',  ( 13.89961937509977652, -13.97604488694527269, 108.1239096053143669 ) ) ;
#50354=CARTESIAN_POINT ( 'NONE',  ( 5.719274019375991003, -21.55341960407610458, 107.7072429386476955 ) ) ;
#50355=CARTESIAN_POINT ( 'NONE',  ( 8.314922557960818139, 14.29746914071049879, 64.58224293864769550 ) ) ;
#50356=CARTESIAN_POINT ( 'NONE',  ( 5.049401038298161559, -19.05341960407611168, 47.70724293864770260 ) ) ;
#50357=CARTESIAN_POINT ( 'NONE',  ( -4.379528057220328563, 16.55341960407611168, 80.20724293864769550 ) ) ;
#50358=CARTESIAN_POINT ( 'NONE',  ( 5.823673210054125526, 21.52544592524343514, 29.79057627198102409 ) ) ;
#50359=CARTESIAN_POINT ( 'NONE',  ( 19.05341960407617918, -5.049401038297876454, 26.04275706135233293 ) ) ;
#50360=CARTESIAN_POINT ( 'NONE',  ( 16.46253265017160672, -9.564922557960803928, 23.33224293864769194 ) ) ;
#50362=CARTESIAN_POINT ( 'NONE',  ( 14.34966873604972726, -8.224510206698740333, 60.83442372801901854 ) ) ;
#50363=CARTESIAN_POINT ( 'NONE',  ( 9.564922557960805705, 16.46253265017160317, 64.58224293864769550 ) ) ;
#50365=CARTESIAN_POINT ( 'NONE',  ( 14.29746914071049879, -8.314922557960816363, 88.33224293864769550 ) ) ;
#50366=CARTESIAN_POINT ( 'NONE',  ( -10.81492255796078084, -18.62759615963271287, 37.08224293864768129 ) ) ;
#50367=CARTESIAN_POINT ( 'NONE',  ( -12.14591786802326823, 12.06949235617739902, 113.1260903946856899 ) ) ;
#50368=CARTESIAN_POINT ( 'NONE',  ( 0.05219959533936267826, -19.03943276465977164, 110.0010903946856757 ) ) ;
#50369=CARTESIAN_POINT ( 'NONE',  ( -10.81492255796105439, 18.62759615963255655, 77.91775706135231871 ) ) ;
#50370=CARTESIAN_POINT ( 'NONE',  ( 16.46253265017160672, -9.564922557960803928, 83.33224293864768129 ) ) ;
#50371=CARTESIAN_POINT ( 'NONE',  ( -10.81492255796078084, -18.62759615963271287, 107.0822429386476955 ) ) ;
#50372=CARTESIAN_POINT ( 'NONE',  ( 8.224510206698742110, 14.34966873604972548, 57.08442372801901854 ) ) ;
#50373=CARTESIAN_POINT ( 'NONE',  ( 9.564922557960805705, 16.46253265017160317, 34.58224293864770260 ) ) ;
#50375=CARTESIAN_POINT ( 'NONE',  ( 16.55341960407618274, -4.379528057220086978, 31.04275706135234714 ) ) ;
#50376=CARTESIAN_POINT ( 'NONE',  ( -19.02544592524334988, -5.153800228976617603, 93.95942372801900433 ) ) ;
#50377=CARTESIAN_POINT ( 'NONE',  ( 5.719274019375991003, -21.55341960407610458, 87.70724293864769550 ) ) ;
#50378=CARTESIAN_POINT ( 'NONE',  ( 16.51473224551083163, -9.474510206698727899, 50.83442372801899722 ) ) ;
#50379=CARTESIAN_POINT ( 'NONE',  ( 19.01533133064925352, -5.499999999999441336, 86.26586590595742621 ) ) ;
#50380=CARTESIAN_POINT ( 'NONE',  ( 21.55341960407610458, 5.719274019375980345, 103.9572429386476813 ) ) ;
#50382=CARTESIAN_POINT ( 'NONE',  ( 13.97604488694527802, 13.89961937509977652, 74.37390960531436690 ) ) ;
#50384=CARTESIAN_POINT ( 'NONE',  ( 12.14591786802327356, -12.06949235617739191, 35.62609039468568994 ) ) ;
#50386=CARTESIAN_POINT ( 'NONE',  ( -15.72974639402176322, -15.80617190586768395, 19.37609039468568639 ) ) ;
#50387=CARTESIAN_POINT ( 'NONE',  ( 14.29746914071049879, -8.314922557960816363, 68.33224293864769550 ) ) ;
#50388=CARTESIAN_POINT ( 'NONE',  ( -19.02544592524342804, 5.153800228976336051, 66.04057627198103830 ) ) ;
#50389=CARTESIAN_POINT ( 'NONE',  ( -8.314922557961024197, 14.29746914071037800, 37.91775706135235424 ) ) ;
#50390=CARTESIAN_POINT ( 'NONE',  ( 5.153800228976615827, -19.02544592524334988, 45.20942372801901143 ) ) ;
#50391=CARTESIAN_POINT ( 'NONE',  ( -15.80617190586768217, 15.72974639402176855, 48.12609039468568284 ) ) ;
#50392=CARTESIAN_POINT ( 'NONE',  ( -9.564922557961040184, 16.46253265017147172, 107.9177570613523471 ) ) ;
#50393=CARTESIAN_POINT ( 'NONE',  ( -13.89961937509977652, 13.97604488694528158, 60.62390960531436690 ) ) ;
#50394=CARTESIAN_POINT ( 'NONE',  ( 5.153800228976615827, -19.02544592524334988, 85.20942372801900433 ) ) ;
#50395=CARTESIAN_POINT ( 'NONE',  ( -21.55341960407619339, 5.719274019375674811, 83.54275706135234714 ) ) ;
#50396=CARTESIAN_POINT ( 'NONE',  ( -19.03943276465977164, -0.05219959533935918106, 63.75109039468566863 ) ) ;
#50397=CARTESIAN_POINT ( 'NONE',  ( 5.049401038298161559, -19.05341960407611168, 37.70724293864768839 ) ) ;
#50398=CARTESIAN_POINT ( 'NONE',  ( -21.52544592524343514, 5.823673210054127303, 61.04057627198103120 ) ) ;
#50399=CARTESIAN_POINT ( 'NONE',  ( -12.06949235617756955, 12.14591786802309770, 60.62390960531437401 ) ) ;
#50400=CARTESIAN_POINT ( 'NONE',  ( 13.97604488694548053, -13.89961937509957401, 70.62609039468567573 ) ) ;
#50402=CARTESIAN_POINT ( 'NONE',  ( 9.474510206698729675, 16.51473224551082808, 27.08442372801900433 ) ) ;
#50403=CARTESIAN_POINT ( 'NONE',  ( 4.483927247898790824, -16.52544592524335698, 100.2094237280190043 ) ) ;
#50404=CARTESIAN_POINT ( 'NONE',  ( -16.55341960407611168, -4.379528057220339221, 51.45724293864770260 ) ) ;
#50405=CARTESIAN_POINT ( 'NONE',  ( -10.81492255796105439, 18.62759615963255655, 87.91775706135234714 ) ) ;
#50407=CARTESIAN_POINT ( 'NONE',  ( 21.55341960407619695, -5.719274019375665929, 91.04275706135236135 ) ) ;
#50408=CARTESIAN_POINT ( 'NONE',  ( -10.72451020669898014, 18.67979575497178502, 90.41557627198103830 ) ) ;
#50409=CARTESIAN_POINT ( 'NONE',  ( 9.564922557960805705, 16.46253265017160317, 49.58224293864770260 ) ) ;
#50410=CARTESIAN_POINT ( 'NONE',  ( -18.67979575497193778, 10.72451020669871902, 68.33442372801900433 ) ) ;
#50411=CARTESIAN_POINT ( 'NONE',  ( 19.03943276465977164, -0.05219959533909143690, 48.74890960531435979 ) ) ;
#50412=CARTESIAN_POINT ( 'NONE',  ( -0.05219959533909027116, -19.03943276465977164, 62.49890960531435979 ) ) ;
#50413=CARTESIAN_POINT ( 'NONE',  ( 12.06949235617757843, -12.14591786802309237, 103.1239096053143811 ) ) ;
#50414=CARTESIAN_POINT ( 'NONE',  ( 16.51473224551069308, 9.474510206698969483, 114.1655762719810241 ) ) ;
#50416=CARTESIAN_POINT ( 'NONE',  ( 14.29746914071049879, -8.314922557960816363, 58.33224293864768839 ) ) ;
#50417=CARTESIAN_POINT ( 'NONE',  ( -16.51473224551069308, -9.474510206698971260, 36.66557627198102409 ) ) ;
#50418=CARTESIAN_POINT ( 'NONE',  ( -4.379528057220328563, 16.55341960407611168, 70.20724293864769550 ) ) ;
#50419=CARTESIAN_POINT ( 'NONE',  ( 15.72974639402199770, -15.80617190586745480, 98.12390960531436690 ) ) ;
#50420=CARTESIAN_POINT ( 'NONE',  ( 10.72451020669871369, 18.67979575497193778, 42.08442372801901854 ) ) ;
#50422=CARTESIAN_POINT ( 'NONE',  ( -12.14591786802326823, 12.06949235617739902, 33.12609039468569705 ) ) ;
#50423=CARTESIAN_POINT ( 'NONE',  ( 5.823673210054125526, 21.52544592524343514, 79.79057627198102409 ) ) ;
#50424=CARTESIAN_POINT ( 'NONE',  ( 10.81492255796106328, -18.62759615963255655, 110.4177570613523756 ) ) ;
#50425=CARTESIAN_POINT ( 'NONE',  ( -5.153800228976328057, -19.02544592524343514, 87.29057627198103830 ) ) ;
#50426=CARTESIAN_POINT ( 'NONE',  ( -21.53943276465977519, -0.05219959533937600094, 43.75109039468568284 ) ) ;
#50427=CARTESIAN_POINT ( 'NONE',  ( 10.81492255796078972, 18.62759615963270932, 34.58224293864770260 ) ) ;
#50428=CARTESIAN_POINT ( 'NONE',  ( 16.55341960407618274, -4.379528057220086978, 106.0427570613523471 ) ) ;
#50429=CARTESIAN_POINT ( 'NONE',  ( 21.53943276465977519, 0.05219959533937863772, 46.25109039468567573 ) ) ;
#50430=CARTESIAN_POINT ( 'NONE',  ( 10.81492255796106328, -18.62759615963255655, 90.41775706135236135 ) ) ;
#50431=CARTESIAN_POINT ( 'NONE',  ( -5.719274019375665041, -21.55341960407619695, 109.7927570613523613 ) ) ;
#50432=CARTESIAN_POINT ( 'NONE',  ( 4.483927247898790824, -16.52544592524335698, 85.20942372801901854 ) ) ;
#50433=CARTESIAN_POINT ( 'NONE',  ( -21.53943276465977519, -0.05219959533937600094, 43.75109039468568284 ) ) ;
#50434=CARTESIAN_POINT ( 'NONE',  ( 13.89961937509977652, -13.97604488694527269, 33.12390960531434558 ) ) ;
#50435=CARTESIAN_POINT ( 'NONE',  ( 15.72974639402176855, 15.80617190586768217, 101.8760903946857042 ) ) ;
#50436=CARTESIAN_POINT ( 'NONE',  ( 9.474510206698971260, -16.51473224551069308, 102.9155762719810241 ) ) ;
#50437=CARTESIAN_POINT ( 'NONE',  ( -15.72974639402197994, 15.80617190586746368, 100.6239096053143811 ) ) ;
#50439=CARTESIAN_POINT ( 'NONE',  ( -5.823673210054116645, -21.52544592524344225, 72.29057627198102409 ) ) ;
#50440=CARTESIAN_POINT ( 'NONE',  ( 0.05219959533934541429, -16.53943276465976808, 50.00109039468568994 ) ) ;
#50441=CARTESIAN_POINT ( 'NONE',  ( -14.34966873604960291, -8.224510206698953496, 66.66557627198102409 ) ) ;
#50442=CARTESIAN_POINT ( 'NONE',  ( 18.93472913878447983, -5.500000000000005329, 101.2198988386846423 ) ) ;
#50443=CARTESIAN_POINT ( 'NONE',  ( 5.049401038297881783, 19.05341960407617563, 87.29275706135234714 ) ) ;
#50445=CARTESIAN_POINT ( 'NONE',  ( -8.314922557961024197, 14.29746914071037800, 27.91775706135234358 ) ) ;
#50446=CARTESIAN_POINT ( 'NONE',  ( -10.81492255796078084, -18.62759615963271287, 92.08224293864769550 ) ) ;
#50447=CARTESIAN_POINT ( 'NONE',  ( -21.52544592524343514, 5.823673210054127303, 76.04057627198102409 ) ) ;
#50448=CARTESIAN_POINT ( 'NONE',  ( 13.97604488694527802, 13.89961937509977652, 109.3739096053143669 ) ) ;
#50449=CARTESIAN_POINT ( 'NONE',  ( 8.224510206698742110, 14.34966873604972548, 62.08442372801901143 ) ) ;
#50450=CARTESIAN_POINT ( 'NONE',  ( -19.05341960407611168, -5.049401038298163336, 76.45724293864769550 ) ) ;
#50451=CARTESIAN_POINT ( 'NONE',  ( 21.52544592524334988, 5.823673210054432836, 31.45942372801901854 ) ) ;
#50452=CARTESIAN_POINT ( 'NONE',  ( -5.153800228976607833, 19.02544592524334988, 102.7094237280189759 ) ) ;
#50453=CARTESIAN_POINT ( 'NONE',  ( -9.564922557960796823, -16.46253265017161027, 107.0822429386476955 ) ) ;
#50454=CARTESIAN_POINT ( 'NONE',  ( -13.97604488694527625, -13.89961937509977652, 81.87390960531436690 ) ) ;
#50455=CARTESIAN_POINT ( 'NONE',  ( 15.80617190586746368, 15.72974639402197994, 84.37390960531438111 ) ) ;
#50456=CARTESIAN_POINT ( 'NONE',  ( -19.03943276465977164, 0.05219959533909376836, 56.24890960531435979 ) ) ;
#50458=CARTESIAN_POINT ( 'NONE',  ( -8.224510206698948167, 14.34966873604960824, 65.41557627198102409 ) ) ;
#50459=CARTESIAN_POINT ( 'NONE',  ( 9.564922557960805705, 16.46253265017160317, 114.5822429386476955 ) ) ;
#50461=CARTESIAN_POINT ( 'NONE',  ( 15.80617190586746368, 15.72974639402197994, 104.3739096053143669 ) ) ;
#50462=CARTESIAN_POINT ( 'NONE',  ( -9.564922557961040184, 16.46253265017147172, 67.91775706135233293 ) ) ;
#50463=CARTESIAN_POINT ( 'NONE',  ( 5.153800228976335163, 19.02544592524342804, 114.7905762719810241 ) ) ;
#50465=CARTESIAN_POINT ( 'NONE',  ( 5.823673210054125526, 21.52544592524343514, 49.79057627198102409 ) ) ;
#50466=CARTESIAN_POINT ( 'NONE',  ( -5.153800228976328057, -19.02544592524343514, 92.29057627198099567 ) ) ;
#50467=CARTESIAN_POINT ( 'NONE',  ( 15.80617190586769283, -15.72974639402175789, 75.62609039468567573 ) ) ;
#50468=CARTESIAN_POINT ( 'NONE',  ( 16.46253265017160672, -9.564922557960803928, 48.33224293864769550 ) ) ;
#50469=CARTESIAN_POINT ( 'NONE',  ( -12.14591786802309592, -12.06949235617757132, 86.87390960531438111 ) ) ;
#50470=CARTESIAN_POINT ( 'NONE',  ( 14.29746914071037800, 8.314922557961029526, 36.66775706135234714 ) ) ;
#50471=CARTESIAN_POINT ( 'NONE',  ( 21.53943276465977519, 0.05219959533937863772, 61.25109039468567573 ) ) ;
#50473=CARTESIAN_POINT ( 'NONE',  ( 9.564922557961047289, -16.46253265017146816, 30.41775706135232937 ) ) ;
#50474=CARTESIAN_POINT ( 'NONE',  ( 16.46253265017146816, 9.564922557961045513, 81.66775706135233293 ) ) ;
#50475=CARTESIAN_POINT ( 'NONE',  ( -18.22780087662123094, -5.499999999999984901, 91.48459894673894155 ) ) ;
#50476=CARTESIAN_POINT ( 'NONE',  ( 15.72974639402176855, 15.80617190586768217, 41.87609039468568284 ) ) ;
#50478=CARTESIAN_POINT ( 'NONE',  ( -0.05219959533936034679, 19.03943276465977164, 27.50109039468566507 ) ) ;
#50479=CARTESIAN_POINT ( 'NONE',  ( -5.153800228976328057, -19.02544592524343514, 62.29057627198100988 ) ) ;
#50480=CARTESIAN_POINT ( 'NONE',  ( -13.89961937509957401, -13.97604488694547875, 29.37609039468565797 ) ) ;
#50481=CARTESIAN_POINT ( 'NONE',  ( -14.34966873604972548, 8.224510206698743886, 98.33442372801901854 ) ) ;
#50482=CARTESIAN_POINT ( 'NONE',  ( -13.89961937509977652, 13.97604488694528158, 115.6239096053143669 ) ) ;
#50483=CARTESIAN_POINT ( 'NONE',  ( 21.52544592524334988, 5.823673210054432836, 81.45942372801900433 ) ) ;
#50485=CARTESIAN_POINT ( 'NONE',  ( -17.50000000000003197, -3.305555262949710915, 35.37482847843423883 ) ) ;
#50486=CARTESIAN_POINT ( 'NONE',  ( 21.52544592524334988, 5.823673210054432836, 91.45942372801901854 ) ) ;
#50488=CARTESIAN_POINT ( 'NONE',  ( 19.03943276465977164, -0.05219959533909143690, 103.7489096053143669 ) ) ;
#50490=CARTESIAN_POINT ( 'NONE',  ( -16.46253265017160317, 9.564922557960807481, 50.83224293864770260 ) ) ;
#50491=CARTESIAN_POINT ( 'NONE',  ( -5.719274019375978568, 21.55341960407610458, 55.20724293864770260 ) ) ;
#50492=CARTESIAN_POINT ( 'NONE',  ( 14.29746914071049879, -8.314922557960816363, 33.33224293864769550 ) ) ;
#50493=CARTESIAN_POINT ( 'NONE',  ( 16.55341960407611168, 4.379528057220329451, 93.95724293864770971 ) ) ;
#50494=CARTESIAN_POINT ( 'NONE',  ( -5.153800228976328057, -19.02544592524343514, 82.29057627198103830 ) ) ;
#50495=CARTESIAN_POINT ( 'NONE',  ( -19.03943276465977164, -0.05219959533935918106, 28.75109039468566507 ) ) ;
#50496=CARTESIAN_POINT ( 'NONE',  ( 9.474510206698971260, -16.51473224551069308, 32.91557627198102409 ) ) ;
#50497=CARTESIAN_POINT ( 'NONE',  ( 12.06949235617757843, -12.14591786802309237, 98.12390960531436690 ) ) ;
#50498=CARTESIAN_POINT ( 'NONE',  ( -15.72974639402176322, -15.80617190586768395, 59.37609039468568284 ) ) ;
#50499=CARTESIAN_POINT ( 'NONE',  ( -21.52544592524343514, 5.823673210054127303, 91.04057627198103830 ) ) ;
#50500=CARTESIAN_POINT ( 'NONE',  ( 19.02544592524334988, 5.153800228976608722, 61.45942372801900433 ) ) ;
#50502=CARTESIAN_POINT ( 'NONE',  ( 9.474510206698971260, -16.51473224551069308, 112.9155762719810383 ) ) ;
#50503=CARTESIAN_POINT ( 'NONE',  ( -0.05219959533910754901, -16.53943276465976808, 77.49890960531433848 ) ) ;
#50505=CARTESIAN_POINT ( 'NONE',  ( -19.02544592524334988, -5.153800228976617603, 48.95942372801900433 ) ) ;
#50506=CARTESIAN_POINT ( 'NONE',  ( 5.049401038298161559, -19.05341960407611168, 67.70724293864769550 ) ) ;
#50507=CARTESIAN_POINT ( 'NONE',  ( 8.224510206698953496, -14.34966873604960469, 67.91557627198102409 ) ) ;
#50508=CARTESIAN_POINT ( 'NONE',  ( 5.153800228976615827, -19.02544592524334988, 75.20942372801896170 ) ) ;
#50510=CARTESIAN_POINT ( 'NONE',  ( 21.55341960407610458, 5.719274019375980345, 33.95724293864769550 ) ) ;
#50511=ORIENTED_EDGE ( 'NONE', *, *, #182922, .T. ) ;
#50512=CARTESIAN_POINT ( 'NONE',  ( -12.14591786802309592, -12.06949235617757132, 101.8739096053143811 ) ) ;
#50514=CARTESIAN_POINT ( 'NONE',  ( -0.05219959533909027116, -19.03943276465977164, 57.49890960531435979 ) ) ;
#50515=CARTESIAN_POINT ( 'NONE',  ( 15.72974639402199770, -15.80617190586745480, 63.12390960531435979 ) ) ;
#50516=CARTESIAN_POINT ( 'NONE',  ( -19.03943276465977164, 0.05219959533909376836, 41.24890960531435269 ) ) ;
#50517=CARTESIAN_POINT ( 'NONE',  ( 8.224510206698742110, 14.34966873604972548, 77.08442372801901854 ) ) ;
#50518=CARTESIAN_POINT ( 'NONE',  ( -16.51473224551069308, -9.474510206698971260, 76.66557627198103830 ) ) ;
#50519=CARTESIAN_POINT ( 'NONE',  ( 5.153800228976615827, -19.02544592524334988, 55.20942372801899722 ) ) ;
#50520=CARTESIAN_POINT ( 'NONE',  ( -21.52544592524334988, -5.823673210054445271, 68.95942372801901854 ) ) ;
#50521=CARTESIAN_POINT ( 'NONE',  ( 10.81492255796078972, 18.62759615963270932, 49.58224293864769550 ) ) ;
#50522=CARTESIAN_POINT ( 'NONE',  ( -13.97604488694527625, -13.89961937509977652, 111.8739096053143243 ) ) ;
#50523=CARTESIAN_POINT ( 'NONE',  ( 16.53943276465976808, -0.05219959533910856209, 113.7489096053143527 ) ) ;
#50524=CARTESIAN_POINT ( 'NONE',  ( 16.53943276465976808, 0.05219959533934440121, 81.25109039468568994 ) ) ;
#50525=CARTESIAN_POINT ( 'NONE',  ( -19.03943276465977164, -0.05219959533935918106, 108.7510903946856615 ) ) ;
#50528=CARTESIAN_POINT ( 'NONE',  ( 15.72974639402176855, 15.80617190586768217, 91.87609039468568994 ) ) ;
#50529=CARTESIAN_POINT ( 'NONE',  ( -4.379528057220328563, 16.55341960407611168, 45.20724293864769550 ) ) ;
#50530=CARTESIAN_POINT ( 'NONE',  ( -12.14591786802309592, -12.06949235617757132, 66.87390960531436690 ) ) ;
#50531=CARTESIAN_POINT ( 'NONE',  ( -21.55341960407610458, -5.719274019375992779, 96.45724293864770971 ) ) ;
#50532=CARTESIAN_POINT ( 'NONE',  ( -5.823673210054116645, -21.52544592524344225, 82.29057627198103830 ) ) ;
#50534=CARTESIAN_POINT ( 'NONE',  ( 18.67979575497178502, 10.72451020669898547, 34.16557627198102409 ) ) ;
#50535=CARTESIAN_POINT ( 'NONE',  ( -14.34966873604972548, 8.224510206698743886, 63.33442372801900433 ) ) ;
#50536=CARTESIAN_POINT ( 'NONE',  ( 14.34966873604960469, 8.224510206698951720, 94.16557627198103830 ) ) ;
#50537=CARTESIAN_POINT ( 'NONE',  ( 5.153800228976335163, 19.02544592524342804, 39.79057627198100988 ) ) ;
#50540=CARTESIAN_POINT ( 'NONE',  ( 16.52544592524335698, 4.483927247898782831, 96.45942372801901854 ) ) ;
#50541=CARTESIAN_POINT ( 'NONE',  ( 5.719274019375673035, 21.55341960407619339, 37.29275706135235424 ) ) ;
#50542=CARTESIAN_POINT ( 'NONE',  ( 16.51473224551069308, 9.474510206698969483, 84.16557627198102409 ) ) ;
#50543=CARTESIAN_POINT ( 'NONE',  ( -21.55341960407619339, 5.719274019375674811, 68.54275706135234714 ) ) ;
#50544=CARTESIAN_POINT ( 'NONE',  ( 19.02544592524343514, -5.153800228976328945, 108.5405762719810383 ) ) ;
#50547=ORIENTED_EDGE ( 'NONE', *, *, #33328, .F. ) ;
#50548=CARTESIAN_POINT ( 'NONE',  ( -18.62759615963255300, -10.81492255796106328, 59.16775706135234714 ) ) ;
#50549=CARTESIAN_POINT ( 'NONE',  ( -13.97604488694527625, -13.89961937509977652, 41.87390960531435979 ) ) ;
#50550=CARTESIAN_POINT ( 'NONE',  ( -13.89961937509977652, 13.97604488694528158, 115.6239096053143669 ) ) ;
#50551=CARTESIAN_POINT ( 'NONE',  ( 9.474510206698729675, 16.51473224551082808, 72.08442372801900433 ) ) ;
#50552=CARTESIAN_POINT ( 'NONE',  ( 5.719274019375673035, 21.55341960407619339, 27.29275706135234358 ) ) ;
#50553=CARTESIAN_POINT ( 'NONE',  ( 0.05219959533936267826, -19.03943276465977164, 65.00109039468567573 ) ) ;
#50554=CARTESIAN_POINT ( 'NONE',  ( -13.89961937509977652, 13.97604488694528158, 25.62390960531434558 ) ) ;
#50555=CARTESIAN_POINT ( 'NONE',  ( 0.05219959533934541429, -16.53943276465976808, 95.00109039468568994 ) ) ;
#50556=CARTESIAN_POINT ( 'NONE',  ( -19.02544592524334988, -5.153800228976617603, 58.95942372801900433 ) ) ;
#50557=CARTESIAN_POINT ( 'NONE',  ( -0.05219959533934338120, 16.53943276465976808, 112.5010903946857042 ) ) ;
#50558=CARTESIAN_POINT ( 'NONE',  ( 19.05341960407617918, -5.049401038297876454, 46.04275706135233293 ) ) ;
#50559=CARTESIAN_POINT ( 'NONE',  ( -9.474510206698964154, 16.51473224551069663, 85.41557627198102409 ) ) ;
#50561=CARTESIAN_POINT ( 'NONE',  ( 5.823673210054444382, -21.52544592524334988, 95.20942372801903275 ) ) ;
#50562=CARTESIAN_POINT ( 'NONE',  ( 0.05219959533937995610, -21.53943276465977519, 105.0010903946856757 ) ) ;
#50563=DIRECTION ( 'NONE',  ( 0.000000000000000000, 0.000000000000000000, 1.000000000000000000 ) ) ;
#50564=CARTESIAN_POINT ( 'NONE',  ( -10.81492255796105439, 18.62759615963255655, 87.91775706135234714 ) ) ;
#50565=CARTESIAN_POINT ( 'NONE',  ( 12.06949235617739724, 12.14591786802326823, 31.87609039468567929 ) ) ;
#50566=CARTESIAN_POINT ( 'NONE',  ( 0.05219959533909260263, 19.03943276465977164, 84.99890960531436690 ) ) ;
#50567=CARTESIAN_POINT ( 'NONE',  ( 5.823673210054125526, 21.52544592524343514, 29.79057627198102409 ) ) ;
#50569=CARTESIAN_POINT ( 'NONE',  ( -0.05219959533909027116, -19.03943276465977164, 77.49890960531435269 ) ) ;
#50570=CARTESIAN_POINT ( 'NONE',  ( -19.39056639909673407, -5.500000000000056843, 40.78948781074345931 ) ) ;
#50571=CARTESIAN_POINT ( 'NONE',  ( -16.51473224551082808, 9.474510206698731452, 73.33442372801900433 ) ) ;
#50572=CARTESIAN_POINT ( 'NONE',  ( -5.049401038298153566, 19.05341960407611168, 105.2072429386476671 ) ) ;
#50573=CARTESIAN_POINT ( 'NONE',  ( 15.72974639402176855, 15.80617190586768217, 101.8760903946857042 ) ) ;
#50574=CARTESIAN_POINT ( 'NONE',  ( -16.53943276465976808, 0.05219959533911058130, 96.24890960531435269 ) ) ;
#50575=CARTESIAN_POINT ( 'NONE',  ( -18.67979575497178146, -10.72451020669898902, 51.66557627198102409 ) ) ;
#50576=CARTESIAN_POINT ( 'NONE',  ( 10.72451020669898902, -18.67979575497178502, 32.91557627198102409 ) ) ;
#50577=CARTESIAN_POINT ( 'NONE',  ( -16.52544592524342804, 4.483927247898546575, 101.0405762719810383 ) ) ;
#50578=CARTESIAN_POINT ( 'NONE',  ( 17.58332526062528345, 7.635886036038587399, 46.57665040441534643 ) ) ;
#50579=CARTESIAN_POINT ( 'NONE',  ( -0.05219959533936034679, 19.03943276465977164, 52.50109039468566863 ) ) ;
#50580=CARTESIAN_POINT ( 'NONE',  ( -8.224510206698948167, 14.34966873604960824, 30.41557627198101699 ) ) ;
#50581=CARTESIAN_POINT ( 'NONE',  ( 13.89961937509977652, -13.97604488694527269, 98.12390960531433848 ) ) ;
#50582=CARTESIAN_POINT ( 'NONE',  ( 21.53943276465977519, 0.05219959533937863772, 86.25109039468568994 ) ) ;
#50583=CARTESIAN_POINT ( 'NONE',  ( -10.72451020669898014, 18.67979575497178502, 55.41557627198102409 ) ) ;
#50584=CARTESIAN_POINT ( 'NONE',  ( -21.52544592524334988, -5.823673210054445271, 48.95942372801902565 ) ) ;
#50585=CARTESIAN_POINT ( 'NONE',  ( -10.72451020669898014, 18.67979575497178502, 90.41557627198103830 ) ) ;
#50586=CARTESIAN_POINT ( 'NONE',  ( -21.52544592524334988, -5.823673210054445271, 43.95942372801902565 ) ) ;
#50587=CARTESIAN_POINT ( 'NONE',  ( 5.153800228976335163, 19.02544592524342804, 24.79057627198102765 ) ) ;
#50588=CARTESIAN_POINT ( 'NONE',  ( -0.05219959533909027116, -19.03943276465977164, 87.49890960531436690 ) ) ;
#50589=CARTESIAN_POINT ( 'NONE',  ( 14.29746914071037800, 8.314922557961029526, 81.66775706135236135 ) ) ;
#50590=CARTESIAN_POINT ( 'NONE',  ( -16.52544592524342804, 4.483927247898546575, 101.0405762719810383 ) ) ;
#50591=CARTESIAN_POINT ( 'NONE',  ( -19.03943276465977164, 0.05219959533909376836, 111.2489096053143669 ) ) ;
#50592=CARTESIAN_POINT ( 'NONE',  ( 16.53943276465976808, -0.05219959533910856209, 58.74890960531436690 ) ) ;
#50593=CARTESIAN_POINT ( 'NONE',  ( -4.379528057220328563, 16.55341960407611168, 25.20724293864769550 ) ) ;
#50594=CARTESIAN_POINT ( 'NONE',  ( -16.46253265017160317, 9.564922557960807481, 55.83224293864769550 ) ) ;
#50595=CARTESIAN_POINT ( 'NONE',  ( -19.02544592524342804, 5.153800228976336051, 26.04057627198103120 ) ) ;
#50596=CARTESIAN_POINT ( 'NONE',  ( -18.67979575497178146, -10.72451020669898902, 51.66557627198102409 ) ) ;
#50597=CARTESIAN_POINT ( 'NONE',  ( -5.153800228976607833, 19.02544592524334988, 22.70942372801899012 ) ) ;
#50598=CARTESIAN_POINT ( 'NONE',  ( -17.44270441346512968, -5.991230190323103777, 41.36335079264229364 ) ) ;
#50599=CARTESIAN_POINT ( 'NONE',  ( -12.14591786802309592, -12.06949235617757132, 41.87390960531435979 ) ) ;
#50600=CARTESIAN_POINT ( 'NONE',  ( 5.823673210054444382, -21.52544592524334988, 50.20942372801901854 ) ) ;
#50602=CARTESIAN_POINT ( 'NONE',  ( -14.29746914071037622, -8.314922557961029526, 64.16775706135234714 ) ) ;
#50603=CARTESIAN_POINT ( 'NONE',  ( -5.049401038297874678, -19.05341960407617918, 59.79275706135231871 ) ) ;
#50604=CARTESIAN_POINT ( 'NONE',  ( -8.224510206698948167, 14.34966873604960824, 30.41557627198101699 ) ) ;
#50605=CARTESIAN_POINT ( 'NONE',  ( -12.14591786802326823, 12.06949235617739902, 113.1260903946856899 ) ) ;
#50606=CARTESIAN_POINT ( 'NONE',  ( -5.049401038298153566, 19.05341960407611168, 40.20724293864768839 ) ) ;
#50607=CARTESIAN_POINT ( 'NONE',  ( -9.564922557960796823, -16.46253265017161027, 62.08224293864769550 ) ) ;
#50608=CARTESIAN_POINT ( 'NONE',  ( -16.53943276465976808, 0.05219959533911058130, 116.2489096053143669 ) ) ;
#50609=CARTESIAN_POINT ( 'NONE',  ( 21.52544592524334988, 5.823673210054432836, 36.45942372801901143 ) ) ;
#50610=CARTESIAN_POINT ( 'NONE',  ( 19.02544592524343514, -5.153800228976328945, 48.54057627198103120 ) ) ;
#50611=CARTESIAN_POINT ( 'NONE',  ( -9.474510206698964154, 16.51473224551069663, 115.4155762719810241 ) ) ;
#50612=CARTESIAN_POINT ( 'NONE',  ( -16.46253265017160317, 9.564922557960807481, 45.83224293864769550 ) ) ;
#50613=CARTESIAN_POINT ( 'NONE',  ( -5.049401038298153566, 19.05341960407611168, 115.2072429386477097 ) ) ;
#50614=CARTESIAN_POINT ( 'NONE',  ( 0.05219959533937995610, -21.53943276465977519, 65.00109039468568994 ) ) ;
#50615=CARTESIAN_POINT ( 'NONE',  ( 0.05219959533910956823, 16.53943276465976808, 99.99890960531436690 ) ) ;
#50616=CARTESIAN_POINT ( 'NONE',  ( -5.153800228976328057, -19.02544592524343514, 107.2905762719810383 ) ) ;
#50617=CARTESIAN_POINT ( 'NONE',  ( -0.05219959533934338120, 16.53943276465976808, 82.50109039468568994 ) ) ;
#50618=CARTESIAN_POINT ( 'NONE',  ( -21.52544592524334988, -5.823673210054445271, 98.95942372801903275 ) ) ;
#50619=CARTESIAN_POINT ( 'NONE',  ( -14.34966873604972548, 8.224510206698743886, 48.33442372801902565 ) ) ;
#50620=CARTESIAN_POINT ( 'NONE',  ( -16.51473224551069308, -9.474510206698971260, 101.6655762719810241 ) ) ;
#50621=CARTESIAN_POINT ( 'NONE',  ( 16.53943276465976808, 0.05219959533934440121, 41.25109039468568284 ) ) ;
#50622=CARTESIAN_POINT ( 'NONE',  ( 8.224510206698742110, 14.34966873604972548, 22.08442372801901143 ) ) ;
#50623=CARTESIAN_POINT ( 'NONE',  ( -8.224510206698735004, -14.34966873604973081, 84.58442372801903275 ) ) ;
#50624=CARTESIAN_POINT ( 'NONE',  ( -5.153800228976607833, 19.02544592524334988, 112.7094237280190043 ) ) ;
#50625=CARTESIAN_POINT ( 'NONE',  ( 21.55341960407610458, 5.719274019375980345, 93.95724293864770971 ) ) ;
#50626=CARTESIAN_POINT ( 'NONE',  ( -0.05219959533910754901, -16.53943276465976808, 107.4989096053143669 ) ) ;
#50627=CARTESIAN_POINT ( 'NONE',  ( -13.89961937509957401, -13.97604488694547875, 99.37609039468567573 ) ) ;
#50628=CARTESIAN_POINT ( 'NONE',  ( -8.314922557961024197, 14.29746914071037800, 72.91775706135234714 ) ) ;
#50630=CARTESIAN_POINT ( 'NONE',  ( 13.97604488694548053, -13.89961937509957401, 65.62609039468567573 ) ) ;
#50631=CARTESIAN_POINT ( 'NONE',  ( -4.483927247898539470, -16.52544592524342804, 52.29057627198102409 ) ) ;
#50632=CARTESIAN_POINT ( 'NONE',  ( -4.483927247898539470, -16.52544592524342804, 27.29057627198103120 ) ) ;
#50633=CARTESIAN_POINT ( 'NONE',  ( 16.53943276465976808, -0.05219959533910856209, 88.74890960531436690 ) ) ;
#50634=CARTESIAN_POINT ( 'NONE',  ( -5.153800228976607833, 19.02544592524334988, 27.70942372801899722 ) ) ;
#50635=CARTESIAN_POINT ( 'NONE',  ( -0.05219959533937732626, 21.53943276465977519, 32.50109039468568284 ) ) ;
#50636=CARTESIAN_POINT ( 'NONE',  ( 16.46253265017146816, 9.564922557961045513, 91.66775706135234714 ) ) ;
#50638=CARTESIAN_POINT ( 'NONE',  ( -13.89961937509977652, 13.97604488694528158, 90.62390960531432427 ) ) ;
#50639=CARTESIAN_POINT ( 'NONE',  ( 19.02544592524343514, -5.153800228976328945, 93.54057627198102409 ) ) ;
#50640=CARTESIAN_POINT ( 'NONE',  ( -5.719274019375978568, 21.55341960407610458, 50.20724293864769550 ) ) ;
#50641=CARTESIAN_POINT ( 'NONE',  ( 4.379528057220339221, -16.55341960407611168, 97.70724293864772392 ) ) ;
#50642=CARTESIAN_POINT ( 'NONE',  ( 19.02544592524343514, -5.153800228976328945, 68.54057627198103830 ) ) ;
#50643=CARTESIAN_POINT ( 'NONE',  ( -13.97604488694527625, -13.89961937509977652, 31.87390960531435979 ) ) ;
#50645=CARTESIAN_POINT ( 'NONE',  ( -5.719274019375665041, -21.55341960407619695, 34.79275706135235424 ) ) ;
#50646=CARTESIAN_POINT ( 'NONE',  ( 21.53943276465977519, 0.05219959533937863772, 81.25109039468568994 ) ) ;
#50647=CARTESIAN_POINT ( 'NONE',  ( -9.474510206698964154, 16.51473224551069663, 55.41557627198103120 ) ) ;
#50648=CARTESIAN_POINT ( 'NONE',  ( 8.314922557961029526, -14.29746914071037800, 75.41775706135233293 ) ) ;
#50649=CARTESIAN_POINT ( 'NONE',  ( -0.05219959533937732626, 21.53943276465977519, 32.50109039468568284 ) ) ;
#50650=CARTESIAN_POINT ( 'NONE',  ( 21.53943276465977519, 0.05219959533937863772, 26.25109039468567573 ) ) ;
#50651=CARTESIAN_POINT ( 'NONE',  ( 16.46253265017146816, 9.564922557961045513, 46.66775706135233293 ) ) ;
#50652=CARTESIAN_POINT ( 'NONE',  ( 16.46253265017160672, -9.564922557960803928, 78.33224293864769550 ) ) ;
#50653=CARTESIAN_POINT ( 'NONE',  ( -16.51473224551082808, 9.474510206698731452, 28.33442372801900433 ) ) ;
#50654=CARTESIAN_POINT ( 'NONE',  ( -21.55341960407619339, 5.719274019375674811, 78.54275706135236135 ) ) ;
#50655=CARTESIAN_POINT ( 'NONE',  ( -18.62759615963270932, 10.81492255796079327, 75.83224293864769550 ) ) ;
#50656=CARTESIAN_POINT ( 'NONE',  ( -12.06949235617756955, 12.14591786802309770, 55.62390960531436690 ) ) ;
#50657=CARTESIAN_POINT ( 'NONE',  ( -10.72451020669870658, -18.67979575497194134, 94.58442372801901854 ) ) ;
#50658=CARTESIAN_POINT ( 'NONE',  ( 16.51473224551083163, -9.474510206698727899, 25.83442372801900078 ) ) ;
#50659=CARTESIAN_POINT ( 'NONE',  ( -8.314922557960811034, -14.29746914071050412, 67.08224293864770971 ) ) ;
#50660=CARTESIAN_POINT ( 'NONE',  ( 5.049401038298161559, -19.05341960407611168, 22.70724293864769194 ) ) ;
#50661=CARTESIAN_POINT ( 'NONE',  ( -19.05341960407617563, 5.049401038297882671, 68.54275706135230450 ) ) ;
#50662=CARTESIAN_POINT ( 'NONE',  ( 0.05219959533910956823, 16.53943276465976808, 34.99890960531435979 ) ) ;
#50664=CARTESIAN_POINT ( 'NONE',  ( 21.53943276465977519, 0.05219959533937863772, 81.25109039468568994 ) ) ;
#50665=CARTESIAN_POINT ( 'NONE',  ( 16.46253265017160672, -9.564922557960803928, 73.33224293864769550 ) ) ;
#50666=CARTESIAN_POINT ( 'NONE',  ( -5.153800228976607833, 19.02544592524334988, 52.70942372801900433 ) ) ;
#50667=CARTESIAN_POINT ( 'NONE',  ( 15.72974639402199770, -15.80617190586745480, 53.12390960531436690 ) ) ;
#50668=CARTESIAN_POINT ( 'NONE',  ( -5.719274019375665041, -21.55341960407619695, 39.79275706135235424 ) ) ;
#50669=CARTESIAN_POINT ( 'NONE',  ( -10.81492255796078084, -18.62759615963271287, 107.0822429386476955 ) ) ;
#50670=CARTESIAN_POINT ( 'NONE',  ( 13.89961937509957401, 13.97604488694547697, 111.8760903946856757 ) ) ;
#50671=CARTESIAN_POINT ( 'NONE',  ( 4.483927247898790824, -16.52544592524335698, 65.20942372801901854 ) ) ;
#50672=CARTESIAN_POINT ( 'NONE',  ( 17.05116617787826527, 6.768360034955703597, 63.84324446740807701 ) ) ;
#50673=CARTESIAN_POINT ( 'NONE',  ( 5.823673210054125526, 21.52544592524343514, 104.7905762719810241 ) ) ;
#50674=CARTESIAN_POINT ( 'NONE',  ( -14.29746914071049879, 8.314922557960819915, 100.8322429386477097 ) ) ;
#50675=CARTESIAN_POINT ( 'NONE',  ( 20.49784845243110709, -1.163414459189985801E-14, 95.00000000000000000 ) ) ;
#50676=CARTESIAN_POINT ( 'NONE',  ( -4.379528057220086978, -16.55341960407618274, 39.79275706135235424 ) ) ;
#50679=CARTESIAN_POINT ( 'NONE',  ( 18.62759615963271287, -10.81492255796078972, 68.33224293864769550 ) ) ;
#50680=CARTESIAN_POINT ( 'NONE',  ( -12.06949235617739369, -12.14591786802326823, 104.3760903946856899 ) ) ;
#50681=CARTESIAN_POINT ( 'NONE',  ( -19.02544592524342804, 5.153800228976336051, 31.04057627198102409 ) ) ;
#50682=CARTESIAN_POINT ( 'NONE',  ( -14.29746914071037622, -8.314922557961029526, 69.16775706135234714 ) ) ;
#50683=CARTESIAN_POINT ( 'NONE',  ( 0.05219959533936267826, -19.03943276465977164, 60.00109039468566863 ) ) ;
#50684=CARTESIAN_POINT ( 'NONE',  ( -0.05219959533937732626, 21.53943276465977519, 37.50109039468568284 ) ) ;
#50686=CARTESIAN_POINT ( 'NONE',  ( 18.62759615963271287, -10.81492255796078972, 53.33224293864769550 ) ) ;
#50687=CARTESIAN_POINT ( 'NONE',  ( -8.224510206698735004, -14.34966873604973081, 99.58442372801900433 ) ) ;
#50688=CARTESIAN_POINT ( 'NONE',  ( -21.55341960407619339, 5.719274019375674811, 63.54275706135234003 ) ) ;
#50689=CARTESIAN_POINT ( 'NONE',  ( -18.62759615963270932, 10.81492255796079327, 55.83224293864770260 ) ) ;
#50690=CARTESIAN_POINT ( 'NONE',  ( 21.52544592524344225, -5.823673210054117533, 28.54057627198103120 ) ) ;
#50692=CARTESIAN_POINT ( 'NONE',  ( -8.224510206698735004, -14.34966873604973081, 79.58442372801903275 ) ) ;
#50693=CARTESIAN_POINT ( 'NONE',  ( 10.72451020669898902, -18.67979575497178502, 27.91557627198103830 ) ) ;
#50695=CARTESIAN_POINT ( 'NONE',  ( 19.03943276465977164, -0.05219959533909143690, 98.74890960531436690 ) ) ;
#50696=CARTESIAN_POINT ( 'NONE',  ( -16.53943276465976808, -0.05219959533934237506, 108.7510903946857042 ) ) ;
#50697=CARTESIAN_POINT ( 'NONE',  ( -14.29746914071049879, 8.314922557960819915, 105.8322429386476955 ) ) ;
#50698=CARTESIAN_POINT ( 'NONE',  ( -21.55341960407610458, -5.719274019375992779, 66.45724293864768129 ) ) ;
#50699=CARTESIAN_POINT ( 'NONE',  ( -0.05219959533934338120, 16.53943276465976808, 97.50109039468567573 ) ) ;
#50700=CARTESIAN_POINT ( 'NONE',  ( 18.62759615963255655, 10.81492255796105972, 41.66775706135235424 ) ) ;
#50701=CARTESIAN_POINT ( 'NONE',  ( -13.97604488694547697, 13.89961937509957934, 103.1260903946856473 ) ) ;
#50702=CARTESIAN_POINT ( 'NONE',  ( -16.52544592524342804, 4.483927247898546575, 101.0405762719810383 ) ) ;
#50703=CARTESIAN_POINT ( 'NONE',  ( 19.03943276465977164, 0.05219959533936151252, 106.2510903946856615 ) ) ;
#50705=CARTESIAN_POINT ( 'NONE',  ( 13.89961937509977652, -13.97604488694527269, 23.12390960531436335 ) ) ;
#50707=CARTESIAN_POINT ( 'NONE',  ( 16.46253265017160672, -9.564922557960803928, 88.33224293864769550 ) ) ;
#50708=CARTESIAN_POINT ( 'NONE',  ( 14.29746914071037800, 8.314922557961029526, 71.66775706135234714 ) ) ;
#50709=CARTESIAN_POINT ( 'NONE',  ( -5.823673210054431948, 21.52544592524334988, 107.7094237280190328 ) ) ;
#50710=CARTESIAN_POINT ( 'NONE',  ( 10.72451020669898902, -18.67979575497178502, 62.91557627198102409 ) ) ;
#50711=CARTESIAN_POINT ( 'NONE',  ( -14.29746914071037622, -8.314922557961029526, 84.16775706135234714 ) ) ;
#50712=CARTESIAN_POINT ( 'NONE',  ( -5.049401038297874678, -19.05341960407617918, 79.79275706135233293 ) ) ;
#50713=CARTESIAN_POINT ( 'NONE',  ( -9.474510206698964154, 16.51473224551069663, 30.41557627198102054 ) ) ;
#50714=CARTESIAN_POINT ( 'NONE',  ( -5.153800228976328057, -19.02544592524343514, 77.29057627198099567 ) ) ;
#50715=CARTESIAN_POINT ( 'NONE',  ( -13.89961937509977652, 13.97604488694528158, 35.62390960531435269 ) ) ;
#50716=CARTESIAN_POINT ( 'NONE',  ( 16.46253265017146816, 9.564922557961045513, 66.66775706135233293 ) ) ;
#50718=CARTESIAN_POINT ( 'NONE',  ( -9.564922557960796823, -16.46253265017161027, 97.08224293864769550 ) ) ;
#50719=CARTESIAN_POINT ( 'NONE',  ( -16.53943276465976808, 0.05219959533911058130, 46.24890960531435979 ) ) ;
#50720=CARTESIAN_POINT ( 'NONE',  ( -15.72974639402197994, 15.80617190586746368, 65.62390960531436690 ) ) ;
#50721=CARTESIAN_POINT ( 'NONE',  ( 17.50000000000000355, -7.500000000000000888, 22.00000000000000711 ) ) ;
#50722=CARTESIAN_POINT ( 'NONE',  ( -19.05341960407617563, 5.049401038297882671, 33.54275706135231871 ) ) ;
#50724=CARTESIAN_POINT ( 'NONE',  ( -5.049401038298153566, 19.05341960407611168, 50.20724293864770260 ) ) ;
#50725=CARTESIAN_POINT ( 'NONE',  ( -13.97604488694527625, -13.89961937509977652, 71.87390960531433848 ) ) ;
#50726=CARTESIAN_POINT ( 'NONE',  ( -8.224510206698735004, -14.34966873604973081, 44.58442372801901854 ) ) ;
#50729=CARTESIAN_POINT ( 'NONE',  ( 14.34966873604972726, -8.224510206698740333, 70.83442372801901854 ) ) ;
#50730=CARTESIAN_POINT ( 'NONE',  ( 5.719274019375991003, -21.55341960407610458, 97.70724293864772392 ) ) ;
#50731=CARTESIAN_POINT ( 'NONE',  ( 12.06949235617739724, 12.14591786802326823, 41.87609039468568284 ) ) ;
#50732=CARTESIAN_POINT ( 'NONE',  ( 0.05219959533909260263, 19.03943276465977164, 44.99890960531435979 ) ) ;
#50734=CARTESIAN_POINT ( 'NONE',  ( 15.80617190586769283, -15.72974639402175789, 50.62609039468568994 ) ) ;
#50735=CARTESIAN_POINT ( 'NONE',  ( -19.05341960407617563, 5.049401038297882671, 58.54275706135234003 ) ) ;
#50736=CARTESIAN_POINT ( 'NONE',  ( 0.05219959533937995610, -21.53943276465977519, 95.00109039468568994 ) ) ;
#50737=CARTESIAN_POINT ( 'NONE',  ( -5.049401038298153566, 19.05341960407611168, 25.20724293864768484 ) ) ;
#50739=CARTESIAN_POINT ( 'NONE',  ( -0.05219959533907301413, -21.53943276465977519, 52.49890960531435979 ) ) ;
#50740=CARTESIAN_POINT ( 'NONE',  ( 16.46253265017160672, -9.564922557960803928, 98.33224293864769550 ) ) ;
#50741=CARTESIAN_POINT ( 'NONE',  ( 4.483927247898545687, 16.52544592524342804, 104.7905762719810241 ) ) ;
#50742=CARTESIAN_POINT ( 'NONE',  ( -16.55341960407617563, 4.379528057220093196, 33.54275706135234714 ) ) ;
#50744=CARTESIAN_POINT ( 'NONE',  ( -16.53943276465976808, -0.05219959533934237506, 108.7510903946857042 ) ) ;
#50746=CARTESIAN_POINT ( 'NONE',  ( -10.81492255796078084, -18.62759615963271287, 97.08224293864770971 ) ) ;
#50747=CARTESIAN_POINT ( 'NONE',  ( -8.314922557960811034, -14.29746914071050412, 42.08224293864769550 ) ) ;
#50748=CARTESIAN_POINT ( 'NONE',  ( 19.05341960407611168, 5.049401038298154454, 108.9572429386477097 ) ) ;
#50749=CARTESIAN_POINT ( 'NONE',  ( 5.153800228976615827, -19.02544592524334988, 100.2094237280190043 ) ) ;
#50750=CARTESIAN_POINT ( 'NONE',  ( 10.81492255796106328, -18.62759615963255655, 110.4177570613523756 ) ) ;
#50751=CARTESIAN_POINT ( 'NONE',  ( -16.52544592524342804, 4.483927247898546575, 36.04057627198102409 ) ) ;
#50752=CARTESIAN_POINT ( 'NONE',  ( -21.53943276465977519, 0.05219959533907696930, 91.24890960531436690 ) ) ;
#50753=CARTESIAN_POINT ( 'NONE',  ( -15.80617190586745835, -15.72974639402198527, 46.87390960531435979 ) ) ;
#50754=CARTESIAN_POINT ( 'NONE',  ( 13.89961937509977652, -13.97604488694527269, 63.12390960531435979 ) ) ;
#50755=CARTESIAN_POINT ( 'NONE',  ( 14.29746914071049879, -8.314922557960816363, 33.33224293864769550 ) ) ;
#50756=CARTESIAN_POINT ( 'NONE',  ( 19.02544592524343514, -5.153800228976328945, 93.54057627198102409 ) ) ;
#50757=B_SPLINE_CURVE_WITH_KNOTS ( 'NONE', 3,
 ( #174547, #129010, #98672, #162360, #55186, #67350, #6668, #160366, #68346, #36014, #84504, #114856, #192709, #40012, #23861, #178546, #176550, #85512, #147200, #120832, #59164, #75332, #71362, #104689, #91470, #164383, #149208, #13665, #42035, #26872, #180561, #10699 ),
 .UNSPECIFIED., .F., .F.,
 ( 4, 2, 2, 2, 2, 2, 2, 2, 2, 2, 2, 2, 2, 2, 2, 4 ),
 ( 0.000000000000000000, 0.0003712461730036594018, 0.0007424923460073188037, 0.001113738519010978260, 0.001484984692014637607, 0.002227477038021972566, 0.002598723211025655115, 0.002969969384029337665, 0.003341215557033020214, 0.003712461730036702330, 0.004083707903040385313, 0.004454954076044067429, 0.004826200249047749545, 0.005197446422051432528, 0.005568692595055114644, 0.005939938768058796760 ),
 .UNSPECIFIED. ) ;
#50758=ORIENTED_EDGE ( 'NONE', *, *, #70314, .T. ) ;
#50759=CARTESIAN_POINT ( 'NONE',  ( 18.39639308325435252, 5.500000000000036415, 58.98252246182193659 ) ) ;
#50760=CARTESIAN_POINT ( 'NONE',  ( -5.153800228976607833, 19.02544592524334988, 47.70942372801900433 ) ) ;
#50761=CARTESIAN_POINT ( 'NONE',  ( -10.81492255796078084, -18.62759615963271287, 77.08224293864769550 ) ) ;
#50762=CARTESIAN_POINT ( 'NONE',  ( -8.224510206698948167, 14.34966873604960824, 95.41557627198102409 ) ) ;
#50763=CARTESIAN_POINT ( 'NONE',  ( 15.80617190586769283, -15.72974639402175789, 40.62609039468567573 ) ) ;
#50765=CARTESIAN_POINT ( 'NONE',  ( 14.29746914071037800, 8.314922557961029526, 111.6677570613523613 ) ) ;
#50766=CARTESIAN_POINT ( 'NONE',  ( -5.153800228976328057, -19.02544592524343514, 42.29057627198101699 ) ) ;
#50767=CARTESIAN_POINT ( 'NONE',  ( 13.97604488694527802, 13.89961937509977652, 89.37390960531436690 ) ) ;
#50768=CARTESIAN_POINT ( 'NONE',  ( -19.05341960407611168, -5.049401038298163336, 26.45724293864769550 ) ) ;
#50769=CARTESIAN_POINT ( 'NONE',  ( 16.55341960407611168, 4.379528057220329451, 38.95724293864768839 ) ) ;
#50770=CARTESIAN_POINT ( 'NONE',  ( -0.05219959533937732626, 21.53943276465977519, 67.50109039468568994 ) ) ;
#50772=CARTESIAN_POINT ( 'NONE',  ( -4.483927247898782831, 16.52544592524335698, 67.70942372801901854 ) ) ;
#50773=CARTESIAN_POINT ( 'NONE',  ( 19.02544592524343514, -5.153800228976328945, 63.54057627198103830 ) ) ;
#50774=CARTESIAN_POINT ( 'NONE',  ( 0.05219959533909260263, 19.03943276465977164, 49.99890960531435979 ) ) ;
#50776=CARTESIAN_POINT ( 'NONE',  ( -5.823673210054431948, 21.52544592524334988, 107.7094237280190328 ) ) ;
#50777=CARTESIAN_POINT ( 'NONE',  ( 8.314922557961029526, -14.29746914071037800, 80.41775706135234714 ) ) ;
#50778=CARTESIAN_POINT ( 'NONE',  ( -0.05219959533937732626, 21.53943276465977519, 102.5010903946856899 ) ) ;
#50779=CARTESIAN_POINT ( 'NONE',  ( 15.80617190586746368, 15.72974639402197994, 34.37390960531435979 ) ) ;
#50780=CARTESIAN_POINT ( 'NONE',  ( -16.51473224551082808, 9.474510206698731452, 113.3344237280190043 ) ) ;
#50781=CARTESIAN_POINT ( 'NONE',  ( -0.05219959533937732626, 21.53943276465977519, 62.50109039468568284 ) ) ;
#50782=CARTESIAN_POINT ( 'NONE',  ( -4.483927247898782831, 16.52544592524335698, 47.70942372801902565 ) ) ;
#50783=CARTESIAN_POINT ( 'NONE',  ( -21.53943276465977519, 0.05219959533907696930, 101.2489096053143669 ) ) ;
#50784=CARTESIAN_POINT ( 'NONE',  ( -9.564922557961040184, 16.46253265017147172, 102.9177570613523329 ) ) ;
#50785=CARTESIAN_POINT ( 'NONE',  ( 5.049401038298161559, -19.05341960407611168, 62.70724293864769550 ) ) ;
#50786=CARTESIAN_POINT ( 'NONE',  ( -9.474510206698720793, -16.51473224551083518, 109.5844237280190043 ) ) ;
#50788=CARTESIAN_POINT ( 'NONE',  ( 5.049401038297881783, 19.05341960407617563, 102.2927570613523045 ) ) ;
#50789=CARTESIAN_POINT ( 'NONE',  ( -14.34966873604960291, -8.224510206698953496, 66.66557627198102409 ) ) ;
#50790=CARTESIAN_POINT ( 'NONE',  ( 4.483927247898790824, -16.52544592524335698, 75.20942372801901854 ) ) ;
#50791=CARTESIAN_POINT ( 'NONE',  ( 0.05219959533907565091, 21.53943276465977519, 109.9989096053143527 ) ) ;
#50792=CARTESIAN_POINT ( 'NONE',  ( 5.153800228976335163, 19.02544592524342804, 54.79057627198103120 ) ) ;
#50793=CARTESIAN_POINT ( 'NONE',  ( -5.049401038298153566, 19.05341960407611168, 55.20724293864769550 ) ) ;
#50794=CARTESIAN_POINT ( 'NONE',  ( -14.29746914071037622, -8.314922557961029526, 74.16775706135231871 ) ) ;
#50797=CARTESIAN_POINT ( 'NONE',  ( -21.55341960407619339, 5.719274019375674811, 108.5427570613523756 ) ) ;
#50798=CARTESIAN_POINT ( 'NONE',  ( 13.97604488694527802, 13.89961937509977652, 29.37390960531435979 ) ) ;
#50800=CARTESIAN_POINT ( 'NONE',  ( 9.474510206698729675, 16.51473224551082808, 107.0844237280190043 ) ) ;
#50801=CARTESIAN_POINT ( 'NONE',  ( 0.05219959533907565091, 21.53943276465977519, 49.99890960531437401 ) ) ;
#50802=CARTESIAN_POINT ( 'NONE',  ( -19.05341960407617563, 5.049401038297882671, 48.54275706135233293 ) ) ;
#50803=CARTESIAN_POINT ( 'NONE',  ( -16.52544592524335698, -4.483927247898792601, 28.95942372801902209 ) ) ;
#50804=CARTESIAN_POINT ( 'NONE',  ( -19.05341960407611168, -5.049401038298163336, 46.45724293864768129 ) ) ;
#50805=CARTESIAN_POINT ( 'NONE',  ( 16.51473224551069308, 9.474510206698969483, 49.16557627198102409 ) ) ;
#50806=CARTESIAN_POINT ( 'NONE',  ( -5.823673210054116645, -21.52544592524344225, 82.29057627198103830 ) ) ;
#50807=CARTESIAN_POINT ( 'NONE',  ( 19.02544592524343514, -5.153800228976328945, 113.5405762719810241 ) ) ;
#50808=CARTESIAN_POINT ( 'NONE',  ( 16.51473224551069308, 9.474510206698969483, 49.16557627198102409 ) ) ;
#50809=CARTESIAN_POINT ( 'NONE',  ( -18.10062525802553779, 5.500000000000031086, 93.51383468041922242 ) ) ;
#50810=CARTESIAN_POINT ( 'NONE',  ( -13.89961937509957401, -13.97604488694547875, 94.37609039468566152 ) ) ;
#50811=CARTESIAN_POINT ( 'NONE',  ( 8.314922557960818139, 14.29746914071049879, 64.58224293864769550 ) ) ;
#50813=CARTESIAN_POINT ( 'NONE',  ( 9.564922557961047289, -16.46253265017146816, 20.41775706135233293 ) ) ;
#50814=CARTESIAN_POINT ( 'NONE',  ( -16.53943276465976808, 0.05219959533911058130, 66.24890960531436690 ) ) ;
#50815=CARTESIAN_POINT ( 'NONE',  ( 18.67979575497194134, -10.72451020669871369, 80.83442372801901854 ) ) ;
#50816=CARTESIAN_POINT ( 'NONE',  ( 9.564922557960805705, 16.46253265017160317, 29.58224293864769550 ) ) ;
#50817=CARTESIAN_POINT ( 'NONE',  ( -15.72974639402176322, -15.80617190586768395, 94.37609039468568994 ) ) ;
#50818=CARTESIAN_POINT ( 'NONE',  ( 16.53943276465976808, -0.05219959533910856209, 23.74890960531435269 ) ) ;
#50819=CARTESIAN_POINT ( 'NONE',  ( -18.62759615963255300, -10.81492255796106328, 79.16775706135234714 ) ) ;
#50820=CARTESIAN_POINT ( 'NONE',  ( 13.97604488694527802, 13.89961937509977652, 69.37390960531436690 ) ) ;
#50821=CARTESIAN_POINT ( 'NONE',  ( -15.72974639402176322, -15.80617190586768395, 39.37609039468567573 ) ) ;
#50822=CARTESIAN_POINT ( 'NONE',  ( -19.03943276465977164, 0.05219959533909376836, 81.24890960531436690 ) ) ;
#50823=CARTESIAN_POINT ( 'NONE',  ( 12.06949235617757843, -12.14591786802309237, 88.12390960531436690 ) ) ;
#50824=CARTESIAN_POINT ( 'NONE',  ( 12.14591786802309770, 12.06949235617756955, 64.37390960531435269 ) ) ;
#50825=CARTESIAN_POINT ( 'NONE',  ( -5.719274019375978568, 21.55341960407610458, 70.20724293864769550 ) ) ;
#50826=CARTESIAN_POINT ( 'NONE',  ( 16.51473224551069308, 9.474510206698969483, 79.16557627198103830 ) ) ;
#50827=CARTESIAN_POINT ( 'NONE',  ( 10.72451020669898902, -18.67979575497178502, 87.91557627198103830 ) ) ;
#50828=CARTESIAN_POINT ( 'NONE',  ( -0.05219959533936034679, 19.03943276465977164, 67.50109039468566152 ) ) ;
#50829=CARTESIAN_POINT ( 'NONE',  ( 9.564922557961047289, -16.46253265017146816, 35.41775706135233293 ) ) ;
#50830=CARTESIAN_POINT ( 'NONE',  ( 8.314922557960818139, 14.29746914071049879, 74.58224293864768129 ) ) ;
#50831=CARTESIAN_POINT ( 'NONE',  ( -5.823673210054116645, -21.52544592524344225, 52.29057627198102409 ) ) ;
#50832=CARTESIAN_POINT ( 'NONE',  ( -18.22780087662121673, -5.500000000000063061, 41.48459894673893444 ) ) ;
#50833=CARTESIAN_POINT ( 'NONE',  ( -0.05219959533934338120, 16.53943276465976808, 102.5010903946856899 ) ) ;
#50835=CARTESIAN_POINT ( 'NONE',  ( 19.03943276465977164, 0.05219959533936151252, 101.2510903946856757 ) ) ;
#50836=CARTESIAN_POINT ( 'NONE',  ( -8.224510206698948167, 14.34966873604960824, 70.41557627198102409 ) ) ;
#50837=CARTESIAN_POINT ( 'NONE',  ( -17.50000000000002132, 3.345213924137298012, 34.58768623094346140 ) ) ;
#50838=CARTESIAN_POINT ( 'NONE',  ( 19.02544592524343514, -5.153800228976328945, 63.54057627198103830 ) ) ;
#50839=CARTESIAN_POINT ( 'NONE',  ( -4.483927247898539470, -16.52544592524342804, 57.29057627198103120 ) ) ;
#50840=CARTESIAN_POINT ( 'NONE',  ( 13.89961937509977652, -13.97604488694527269, 103.1239096053143527 ) ) ;
#50841=CARTESIAN_POINT ( 'NONE',  ( 0.05219959533936267826, -19.03943276465977164, 75.00109039468566152 ) ) ;
#50842=CARTESIAN_POINT ( 'NONE',  ( 19.05341960407611168, 5.049401038298154454, 63.95724293864769550 ) ) ;
#50843=CARTESIAN_POINT ( 'NONE',  ( -9.474510206698964154, 16.51473224551069663, 90.41557627198103830 ) ) ;
#50844=CARTESIAN_POINT ( 'NONE',  ( -5.153800228976328057, -19.02544592524343514, 87.29057627198103830 ) ) ;
#50845=CARTESIAN_POINT ( 'NONE',  ( 18.62759615963271287, -10.81492255796078972, 63.33224293864770260 ) ) ;
#50846=CARTESIAN_POINT ( 'NONE',  ( 16.52544592524335698, 4.483927247898782831, 51.45942372801901854 ) ) ;
#50848=CARTESIAN_POINT ( 'NONE',  ( -19.02544592524342804, 5.153800228976336051, 51.04057627198103120 ) ) ;
#50849=CARTESIAN_POINT ( 'NONE',  ( -5.823673210054116645, -21.52544592524344225, 52.29057627198102409 ) ) ;
#50850=CARTESIAN_POINT ( 'NONE',  ( -5.153800228976607833, 19.02544592524334988, 92.70942372801901854 ) ) ;
#50851=CARTESIAN_POINT ( 'NONE',  ( 8.314922557960818139, 14.29746914071049879, 24.58224293864768839 ) ) ;
#50852=CARTESIAN_POINT ( 'NONE',  ( -5.823673210054431948, 21.52544592524334988, 42.70942372801901854 ) ) ;
#50853=CARTESIAN_POINT ( 'NONE',  ( 16.51473224551083163, -9.474510206698727899, 35.83442372801899722 ) ) ;
#50854=CARTESIAN_POINT ( 'NONE',  ( 8.224510206698742110, 14.34966873604972548, 62.08442372801901143 ) ) ;
#50855=CARTESIAN_POINT ( 'NONE',  ( 4.379528057220092307, 16.55341960407617563, 97.29275706135234714 ) ) ;
#50856=CARTESIAN_POINT ( 'NONE',  ( -17.72696623605163424, 5.499999999999871214, 53.59811031808416715 ) ) ;
#50857=CARTESIAN_POINT ( 'NONE',  ( 8.224510206698742110, 14.34966873604972548, 77.08442372801901854 ) ) ;
#50858=CARTESIAN_POINT ( 'NONE',  ( 12.14591786802327356, -12.06949235617739191, 35.62609039468568994 ) ) ;
#50859=CARTESIAN_POINT ( 'NONE',  ( 5.049401038298161559, -19.05341960407611168, 42.70724293864767418 ) ) ;
#50860=CARTESIAN_POINT ( 'NONE',  ( -19.05341960407611168, -5.049401038298163336, 46.45724293864768129 ) ) ;
#50861=CARTESIAN_POINT ( 'NONE',  ( 9.564922557960805705, 16.46253265017160317, 59.58224293864769550 ) ) ;
#50862=CARTESIAN_POINT ( 'NONE',  ( -5.823673210054431948, 21.52544592524334988, 42.70942372801901854 ) ) ;
#50863=CARTESIAN_POINT ( 'NONE',  ( -14.34966873604972548, 8.224510206698743886, 53.33442372801901854 ) ) ;
#50864=CARTESIAN_POINT ( 'NONE',  ( -8.314922557961024197, 14.29746914071037800, 107.9177570613523471 ) ) ;
#50865=CARTESIAN_POINT ( 'NONE',  ( 13.89961937509977652, -13.97604488694527269, 33.12390960531434558 ) ) ;
#50866=CARTESIAN_POINT ( 'NONE',  ( -21.55341960407619339, 5.719274019375674811, 108.5427570613523756 ) ) ;
#50867=CARTESIAN_POINT ( 'NONE',  ( 13.97604488694548053, -13.89961937509957401, 105.6260903946856757 ) ) ;
#50868=CARTESIAN_POINT ( 'NONE',  ( -16.46253265017146816, -9.564922557961047289, 64.16775706135233293 ) ) ;
#50869=CARTESIAN_POINT ( 'NONE',  ( -16.55341960407611168, -4.379528057220339221, 76.45724293864769550 ) ) ;
#50870=CARTESIAN_POINT ( 'NONE',  ( 16.46253265017160672, -9.564922557960803928, 43.33224293864769550 ) ) ;
#50871=CARTESIAN_POINT ( 'NONE',  ( -5.153800228976607833, 19.02544592524334988, 67.70942372801900433 ) ) ;
#50872=CARTESIAN_POINT ( 'NONE',  ( 17.40861289039003168, -6.110651285853313297, 91.12767529172569425 ) ) ;
#50873=CARTESIAN_POINT ( 'NONE',  ( 5.719274019375673035, 21.55341960407619339, 72.29275706135236135 ) ) ;
#50874=CARTESIAN_POINT ( 'NONE',  ( 16.53943276465976808, 0.05219959533934440121, 41.25109039468568284 ) ) ;
#50875=CARTESIAN_POINT ( 'NONE',  ( -17.50000000000001066, 4.658240926743144605, 23.94470417816805963 ) ) ;
#50876=CARTESIAN_POINT ( 'NONE',  ( 0.05219959533907565091, 21.53943276465977519, 34.99890960531435979 ) ) ;
#50877=CARTESIAN_POINT ( 'NONE',  ( 16.52544592524335698, 4.483927247898782831, 21.45942372801901499 ) ) ;
#50878=CARTESIAN_POINT ( 'NONE',  ( -19.05341960407611168, -5.049401038298164224, 26.45724293864769550 ) ) ;
#50879=CARTESIAN_POINT ( 'NONE',  ( -5.153800228976607833, 19.02544592524334988, 32.70942372801899722 ) ) ;
#50881=CARTESIAN_POINT ( 'NONE',  ( 16.46253265017160672, -9.564922557960803928, 33.33224293864770260 ) ) ;
#50883=CARTESIAN_POINT ( 'NONE',  ( 13.89961937509977652, -13.97604488694527269, 68.12390960531436690 ) ) ;
#50884=CARTESIAN_POINT ( 'NONE',  ( -19.46398650005391318, 5.499999999999953815, 100.1826965148636646 ) ) ;
#50885=CARTESIAN_POINT ( 'NONE',  ( -5.153800228976607833, 19.02544592524334988, 22.70942372801899012 ) ) ;
#50886=CARTESIAN_POINT ( 'NONE',  ( -4.483927247898782831, 16.52544592524335698, 112.7094237280190328 ) ) ;
#50887=CARTESIAN_POINT ( 'NONE',  ( 13.97604488694527802, 13.89961937509977652, 44.37390960531435269 ) ) ;
#50888=CARTESIAN_POINT ( 'NONE',  ( 5.153800228976335163, 19.02544592524342804, 89.79057627198102409 ) ) ;
#50889=CARTESIAN_POINT ( 'NONE',  ( -21.55341960407619339, 5.719274019375674811, 68.54275706135234714 ) ) ;
#50890=CARTESIAN_POINT ( 'NONE',  ( -19.03943276465977164, 0.05219959533909376836, 51.24890960531436690 ) ) ;
#50891=CARTESIAN_POINT ( 'NONE',  ( 10.72451020669871369, 18.67979575497193778, 62.08442372801901143 ) ) ;
#50892=CARTESIAN_POINT ( 'NONE',  ( 19.03943276465977164, 0.05219959533936151252, 96.25109039468567573 ) ) ;
#50893=CARTESIAN_POINT ( 'NONE',  ( -18.62759615963270932, 10.81492255796079327, 25.83224293864769194 ) ) ;
#50894=CARTESIAN_POINT ( 'NONE',  ( 19.05341960407611168, 5.049401038298154454, 38.95724293864767418 ) ) ;
#50895=CARTESIAN_POINT ( 'NONE',  ( 10.81492255796078972, 18.62759615963270932, 109.5822429386476955 ) ) ;
#50896=CARTESIAN_POINT ( 'NONE',  ( -19.03943276465977164, -0.05219959533935918106, 28.75109039468566507 ) ) ;
#50897=CARTESIAN_POINT ( 'NONE',  ( -8.224510206698948167, 14.34966873604960824, 105.4155762719810383 ) ) ;
#50898=CARTESIAN_POINT ( 'NONE',  ( -5.049401038298153566, 19.05341960407611168, 65.20724293864765286 ) ) ;
#50899=CARTESIAN_POINT ( 'NONE',  ( 9.474510206698729675, 16.51473224551082808, 112.0844237280190043 ) ) ;
#50900=CARTESIAN_POINT ( 'NONE',  ( 14.29746914071049879, -8.314922557960816363, 73.33224293864769550 ) ) ;
#50901=CARTESIAN_POINT ( 'NONE',  ( -5.823673210054116645, -21.52544592524344225, 27.29057627198103120 ) ) ;
#50902=CARTESIAN_POINT ( 'NONE',  ( 9.564922557961047289, -16.46253265017146816, 90.41775706135234714 ) ) ;
#50903=CARTESIAN_POINT ( 'NONE',  ( 10.72451020669898902, -18.67979575497178502, 87.91557627198103830 ) ) ;
#50904=CARTESIAN_POINT ( 'NONE',  ( -18.67979575497193778, 10.72451020669871902, 53.33442372801901854 ) ) ;
#50905=CARTESIAN_POINT ( 'NONE',  ( -12.14591786802326823, 12.06949235617739902, 58.12609039468568994 ) ) ;
#50906=CARTESIAN_POINT ( 'NONE',  ( -4.483927247898782831, 16.52544592524335698, 52.70942372801902565 ) ) ;
#50907=CARTESIAN_POINT ( 'NONE',  ( 21.55341960407619695, -5.719274019375665929, 51.04275706135234714 ) ) ;
#50908=CARTESIAN_POINT ( 'NONE',  ( 10.81492255796078972, 18.62759615963270932, 49.58224293864769550 ) ) ;
#50909=CARTESIAN_POINT ( 'NONE',  ( -16.46253265017160317, 9.564922557960807481, 50.83224293864770260 ) ) ;
#50911=CARTESIAN_POINT ( 'NONE',  ( -12.14591786802326823, 12.06949235617739902, 73.12609039468567573 ) ) ;
#50913=CARTESIAN_POINT ( 'NONE',  ( -10.72451020669898014, 18.67979575497178502, 105.4155762719810383 ) ) ;
#50914=CARTESIAN_POINT ( 'NONE',  ( -0.05219959533910754901, -16.53943276465976808, 47.49890960531435979 ) ) ;
#50915=CARTESIAN_POINT ( 'NONE',  ( -14.29746914071037622, -8.314922557961029526, 64.16775706135234714 ) ) ;
#50916=CARTESIAN_POINT ( 'NONE',  ( -13.97604488694547697, 13.89961937509957934, 98.12609039468566152 ) ) ;
#50917=CARTESIAN_POINT ( 'NONE',  ( 10.72451020669898902, -18.67979575497178502, 92.91557627198103830 ) ) ;
#50918=CARTESIAN_POINT ( 'NONE',  ( -4.483927247898539470, -16.52544592524342804, 47.29057627198103120 ) ) ;
#50919=ORIENTED_EDGE ( 'NONE', *, *, #55537, .T. ) ;
#50920=CARTESIAN_POINT ( 'NONE',  ( -17.05116617787824751, 6.768360034955817284, 73.65675553259202957 ) ) ;
#50921=CARTESIAN_POINT ( 'NONE',  ( 0.05219959533907565091, 21.53943276465977519, 74.99890960531435269 ) ) ;
#50922=CARTESIAN_POINT ( 'NONE',  ( -8.314922557961024197, 14.29746914071037800, 112.9177570613523329 ) ) ;
#50923=VERTEX_POINT ( 'NONE', #152990 ) ;
#50925=CARTESIAN_POINT ( 'NONE',  ( -15.72974639402197994, 15.80617190586746368, 95.62390960531436690 ) ) ;
#50926=CARTESIAN_POINT ( 'NONE',  ( -10.72451020669870658, -18.67979575497194134, 29.58442372801901854 ) ) ;
#50927=CARTESIAN_POINT ( 'NONE',  ( 4.483927247898545687, 16.52544592524342804, 44.79057627198103120 ) ) ;
#50928=CARTESIAN_POINT ( 'NONE',  ( 4.379528057220092307, 16.55341960407617563, 47.29275706135234003 ) ) ;
#50930=CARTESIAN_POINT ( 'NONE',  ( -16.51473224551069308, -9.474510206698971260, 51.66557627198102409 ) ) ;
#50931=CARTESIAN_POINT ( 'NONE',  ( -9.474510206698964154, 16.51473224551069663, 80.41557627198103830 ) ) ;
#50933=CARTESIAN_POINT ( 'NONE',  ( 0.05219959533907565091, 21.53943276465977519, 34.99890960531435979 ) ) ;
#50934=CARTESIAN_POINT ( 'NONE',  ( 9.564922557960805705, 16.46253265017160317, 64.58224293864769550 ) ) ;
#50935=CARTESIAN_POINT ( 'NONE',  ( -0.05219959533934338120, 16.53943276465976808, 27.50109039468567929 ) ) ;
#50936=CARTESIAN_POINT ( 'NONE',  ( -19.03943276465977164, -0.05219959533935918106, 48.75109039468566863 ) ) ;
#50937=CARTESIAN_POINT ( 'NONE',  ( -5.823673210054116645, -21.52544592524344225, 102.2905762719810383 ) ) ;
#50938=CARTESIAN_POINT ( 'NONE',  ( 16.55341960407611168, 4.379528057220329451, 33.95724293864769550 ) ) ;
#50939=CARTESIAN_POINT ( 'NONE',  ( -19.05341960407611168, -5.049401038298163336, 76.45724293864769550 ) ) ;
#50940=CARTESIAN_POINT ( 'NONE',  ( -18.62759615963270932, 10.81492255796079327, 65.83224293864769550 ) ) ;
#50941=CARTESIAN_POINT ( 'NONE',  ( -21.52544592524343514, 5.823673210054127303, 76.04057627198102409 ) ) ;
#50942=CARTESIAN_POINT ( 'NONE',  ( -4.483927247898782831, 16.52544592524335698, 27.70942372801901854 ) ) ;
#50943=CARTESIAN_POINT ( 'NONE',  ( 21.52544592524344225, -5.823673210054117533, 23.54057627198102765 ) ) ;
#50944=CARTESIAN_POINT ( 'NONE',  ( -21.52544592524334988, -5.823673210054445271, 68.95942372801901854 ) ) ;
#50945=CARTESIAN_POINT ( 'NONE',  ( 19.02544592524343514, -5.153800228976328945, 78.54057627198099567 ) ) ;
#50946=CARTESIAN_POINT ( 'NONE',  ( 9.564922557960805705, 16.46253265017160317, 34.58224293864770260 ) ) ;
#50947=CARTESIAN_POINT ( 'NONE',  ( 13.89961937509977652, -13.97604488694527269, 88.12390960531438111 ) ) ;
#50948=CARTESIAN_POINT ( 'NONE',  ( 16.53943276465976808, -0.05219959533910856209, 88.74890960531436690 ) ) ;
#50949=ORIENTED_EDGE ( 'NONE', *, *, #85306, .T. ) ;
#50950=CARTESIAN_POINT ( 'NONE',  ( 5.153800228976615827, -19.02544592524334988, 100.2094237280190043 ) ) ;
#50952=CARTESIAN_POINT ( 'NONE',  ( 13.97604488694527802, 13.89961937509977652, 69.37390960531436690 ) ) ;
#50953=CARTESIAN_POINT ( 'NONE',  ( -21.52544592524334988, -5.823673210054445271, 93.95942372801903275 ) ) ;
#50954=CARTESIAN_POINT ( 'NONE',  ( 15.72974639402199770, -15.80617190586745480, 23.12390960531436335 ) ) ;
#50955=CARTESIAN_POINT ( 'NONE',  ( 8.224510206698742110, 14.34966873604972548, 72.08442372801899012 ) ) ;
#50957=CARTESIAN_POINT ( 'NONE',  ( 5.049401038297881783, 19.05341960407617563, 57.29275706135231871 ) ) ;
#50958=CARTESIAN_POINT ( 'NONE',  ( 5.719274019375673035, 21.55341960407619339, 107.2927570613523471 ) ) ;
#50960=CARTESIAN_POINT ( 'NONE',  ( -13.89961937509977652, 13.97604488694528158, 30.62390960531435269 ) ) ;
#50961=CARTESIAN_POINT ( 'NONE',  ( -8.314922557961024197, 14.29746914071037800, 112.9177570613523329 ) ) ;
#50963=CARTESIAN_POINT ( 'NONE',  ( 16.53943276465976808, 0.05219959533934440121, 106.2510903946856757 ) ) ;
#50964=CARTESIAN_POINT ( 'NONE',  ( -19.39056639909675894, -5.499999999999976019, 85.78948781074340957 ) ) ;
#50965=CARTESIAN_POINT ( 'NONE',  ( 14.29746914071037800, 8.314922557961029526, 81.66775706135236135 ) ) ;
#50966=CARTESIAN_POINT ( 'NONE',  ( -19.02544592524342804, 5.153800228976336051, 26.04057627198103120 ) ) ;
#50967=CARTESIAN_POINT ( 'NONE',  ( 18.67979575497194134, -10.72451020669871369, 90.83442372801901854 ) ) ;
#50968=CARTESIAN_POINT ( 'NONE',  ( -0.05219959533936034679, 19.03943276465977164, 102.5010903946856757 ) ) ;
#50969=CARTESIAN_POINT ( 'NONE',  ( -10.81492255796105439, 18.62759615963255655, 62.91775706135236135 ) ) ;
#50970=CARTESIAN_POINT ( 'NONE',  ( -19.03943276465977164, -0.05219959533935918106, 43.75109039468566863 ) ) ;
#50971=CARTESIAN_POINT ( 'NONE',  ( -19.02544592524342804, 5.153800228976336051, 81.04057627198103830 ) ) ;
#50972=CARTESIAN_POINT ( 'NONE',  ( 19.05341960407611168, 5.049401038298154454, 63.95724293864769550 ) ) ;
#50973=CARTESIAN_POINT ( 'NONE',  ( 18.67979575497178502, 10.72451020669898547, 54.16557627198103120 ) ) ;
#50974=CARTESIAN_POINT ( 'NONE',  ( 5.153800228976335163, 19.02544592524342804, 44.79057627198103830 ) ) ;
#50975=CARTESIAN_POINT ( 'NONE',  ( 14.29746914071037800, 8.314922557961029526, 81.66775706135236135 ) ) ;
#50977=VERTEX_POINT ( 'NONE', #153994 ) ;
#50978=CARTESIAN_POINT ( 'NONE',  ( -14.29746914071049879, 8.314922557960819915, 80.83224293864769550 ) ) ;
#50980=CARTESIAN_POINT ( 'NONE',  ( 4.379528057220092307, 16.55341960407617563, 42.29275706135235424 ) ) ;
#50981=CARTESIAN_POINT ( 'NONE',  ( 4.483927247898545687, 16.52544592524342804, 99.79057627198103830 ) ) ;
#50982=CARTESIAN_POINT ( 'NONE',  ( 13.89961937509957401, 13.97604488694547697, 61.87609039468566863 ) ) ;
#50983=CARTESIAN_POINT ( 'NONE',  ( -4.483927247898539470, -16.52544592524342804, 77.29057627198102409 ) ) ;
#50984=CARTESIAN_POINT ( 'NONE',  ( 18.62759615963255655, 10.81492255796105972, 31.66775706135234358 ) ) ;
#50986=CARTESIAN_POINT ( 'NONE',  ( 18.62759615963271287, -10.81492255796078972, 93.33224293864769550 ) ) ;
#50987=CARTESIAN_POINT ( 'NONE',  ( -5.153800228976328057, -19.02544592524343514, 97.29057627198099567 ) ) ;
#50988=CARTESIAN_POINT ( 'NONE',  ( 4.483927247898545687, 16.52544592524342804, 69.79057627198102409 ) ) ;
#50990=CARTESIAN_POINT ( 'NONE',  ( 16.46253265017160672, -9.564922557960803928, 43.33224293864769550 ) ) ;
#50992=CARTESIAN_POINT ( 'NONE',  ( -19.02544592524334988, -5.153800228976617603, 83.95942372801901854 ) ) ;
#50993=CARTESIAN_POINT ( 'NONE',  ( 0.05219959533937995610, -21.53943276465977519, 20.00109039468568639 ) ) ;
#50994=CARTESIAN_POINT ( 'NONE',  ( -19.03943276465977164, 0.05219959533909376836, 66.24890960531436690 ) ) ;
#50995=CARTESIAN_POINT ( 'NONE',  ( 5.153800228976615827, -19.02544592524334988, 50.20942372801897591 ) ) ;
#50996=CARTESIAN_POINT ( 'NONE',  ( -19.03943276465977164, 0.05219959533909376836, 46.24890960531435979 ) ) ;
#50997=CARTESIAN_POINT ( 'NONE',  ( 12.14591786802309770, 12.06949235617756955, 69.37390960531436690 ) ) ;
#50998=CARTESIAN_POINT ( 'NONE',  ( 12.06949235617757843, -12.14591786802309237, 58.12390960531435979 ) ) ;
#50999=CARTESIAN_POINT ( 'NONE',  ( 5.153800228976335163, 19.02544592524342804, 74.79057627198103830 ) ) ;
#51000=CARTESIAN_POINT ( 'NONE',  ( -5.823673210054116645, -21.52544592524344225, 82.29057627198103830 ) ) ;
#51001=CARTESIAN_POINT ( 'NONE',  ( -19.03943276465977164, 0.05219959533909376836, 71.24890960531435269 ) ) ;
#51002=CARTESIAN_POINT ( 'NONE',  ( 21.52544592524344225, -5.823673210054117533, 73.54057627198102409 ) ) ;
#51003=CARTESIAN_POINT ( 'NONE',  ( 5.719274019375673035, 21.55341960407619339, 112.2927570613523471 ) ) ;
#51004=CARTESIAN_POINT ( 'NONE',  ( 19.03943276465977164, -0.05219959533909143690, 28.74890960531435624 ) ) ;
#51005=CARTESIAN_POINT ( 'NONE',  ( -14.34966873604972548, 8.224510206698743886, 108.3344237280190185 ) ) ;
#51006=CARTESIAN_POINT ( 'NONE',  ( 14.29746914071049879, -8.314922557960816363, 93.33224293864769550 ) ) ;
#51007=CARTESIAN_POINT ( 'NONE',  ( -9.564922557961040184, 16.46253265017147172, 102.9177570613523329 ) ) ;
#51009=CARTESIAN_POINT ( 'NONE',  ( -21.52544592524334988, -5.823673210054445271, 23.95942372801901143 ) ) ;
#51010=CARTESIAN_POINT ( 'NONE',  ( 16.51473224551083163, -9.474510206698727899, 55.83442372801899722 ) ) ;
#51011=CARTESIAN_POINT ( 'NONE',  ( 14.29746914071049879, -8.314922557960816363, 28.33224293864769550 ) ) ;
#51012=CARTESIAN_POINT ( 'NONE',  ( 5.823673210054125526, 21.52544592524343514, 69.79057627198102409 ) ) ;
#51013=CARTESIAN_POINT ( 'NONE',  ( 19.05341960407611168, 5.049401038298154454, 98.95724293864766707 ) ) ;
#51014=CARTESIAN_POINT ( 'NONE',  ( -14.29746914071049879, 8.314922557960819915, 60.83224293864769550 ) ) ;
#51015=CARTESIAN_POINT ( 'NONE',  ( -18.87075004821565472, 5.499999999999873879, 48.67408112101043827 ) ) ;
#51016=CARTESIAN_POINT ( 'NONE',  ( -5.049401038298153566, 19.05341960407611168, 35.20724293864768839 ) ) ;
#51017=CARTESIAN_POINT ( 'NONE',  ( -15.80617190586768217, 15.72974639402176855, 103.1260903946856757 ) ) ;
#51018=CARTESIAN_POINT ( 'NONE',  ( 16.52544592524335698, 4.483927247898782831, 91.45942372801901854 ) ) ;
#51019=CARTESIAN_POINT ( 'NONE',  ( 15.80617190586769283, -15.72974639402175789, 40.62609039468567573 ) ) ;
#51020=CARTESIAN_POINT ( 'NONE',  ( -4.483927247898782831, 16.52544592524335698, 37.70942372801900433 ) ) ;
#51021=CARTESIAN_POINT ( 'NONE',  ( -10.72451020669898014, 18.67979575497178502, 25.41557627198103120 ) ) ;
#51022=CARTESIAN_POINT ( 'NONE',  ( -16.46253265017160317, 9.564922557960807481, 50.83224293864770260 ) ) ;
#51023=CARTESIAN_POINT ( 'NONE',  ( -5.153800228976328057, -19.02544592524343514, 62.29057627198100988 ) ) ;
#51024=CARTESIAN_POINT ( 'NONE',  ( -16.55341960407617563, 4.379528057220093196, 48.54275706135234714 ) ) ;
#51025=CARTESIAN_POINT ( 'NONE',  ( -16.55341960407611168, -4.379528057220339221, 101.4572429386476955 ) ) ;
#51026=CARTESIAN_POINT ( 'NONE',  ( -16.55341960407617563, 4.379528057220093196, 108.5427570613523756 ) ) ;
#51027=CARTESIAN_POINT ( 'NONE',  ( -5.049401038298153566, 19.05341960407611168, 50.20724293864770260 ) ) ;
#51028=CARTESIAN_POINT ( 'NONE',  ( -10.81492255796105439, 18.62759615963255655, 52.91775706135235424 ) ) ;
#51029=CARTESIAN_POINT ( 'NONE',  ( -0.05219959533909027116, -19.03943276465977164, 97.49890960531436690 ) ) ;
#51030=CARTESIAN_POINT ( 'NONE',  ( -13.97604488694527625, -13.89961937509977652, 81.87390960531436690 ) ) ;
#51031=CARTESIAN_POINT ( 'NONE',  ( -0.05219959533909027116, -19.03943276465977164, 102.4989096053143669 ) ) ;
#51032=CARTESIAN_POINT ( 'NONE',  ( -16.53943276465976808, 0.05219959533911058130, 41.24890960531435269 ) ) ;
#51033=CARTESIAN_POINT ( 'NONE',  ( -0.05219959533934338120, 16.53943276465976808, 107.5010903946856899 ) ) ;
#51034=CARTESIAN_POINT ( 'NONE',  ( 16.52544592524342804, -4.483927247898539470, 43.54057627198103830 ) ) ;
#51036=CARTESIAN_POINT ( 'NONE',  ( -19.02544592524334988, -5.153800228976617603, 38.95942372801900433 ) ) ;
#51037=CARTESIAN_POINT ( 'NONE',  ( -19.05341960407611168, -5.049401038298163336, 71.45724293864766707 ) ) ;
#51038=CARTESIAN_POINT ( 'NONE',  ( 13.89961937509957401, 13.97604488694547697, 46.87609039468565442 ) ) ;
#51041=CARTESIAN_POINT ( 'NONE',  ( -19.03943276465977164, -0.05219959533935918106, 83.75109039468567573 ) ) ;
#51042=CARTESIAN_POINT ( 'NONE',  ( -8.224510206698735004, -14.34966873604973081, 64.58442372801900433 ) ) ;
#51043=CARTESIAN_POINT ( 'NONE',  ( 16.61371651742600619, 7.165104196376149481, 93.64584930007004004 ) ) ;
#51044=CARTESIAN_POINT ( 'NONE',  ( -5.049401038298153566, 19.05341960407611168, 100.2072429386476955 ) ) ;
#51045=CARTESIAN_POINT ( 'NONE',  ( 10.72451020669871369, 18.67979575497193778, 27.08442372801901854 ) ) ;
#51046=CARTESIAN_POINT ( 'NONE',  ( -9.474510206698720793, -16.51473224551083518, 89.58442372801900433 ) ) ;
#51047=FACE_OUTER_BOUND ( 'NONE', #128586, .T. ) ;
#51048=CARTESIAN_POINT ( 'NONE',  ( -16.46253265017160317, 9.564922557960807481, 45.83224293864769550 ) ) ;
#51049=CARTESIAN_POINT ( 'NONE',  ( -13.89961937509977652, 13.97604488694528158, 90.62390960531432427 ) ) ;
#51050=CARTESIAN_POINT ( 'NONE',  ( -14.34966873604960291, -8.224510206698953496, 46.66557627198102409 ) ) ;
#51051=CARTESIAN_POINT ( 'NONE',  ( -5.153800228976328057, -19.02544592524343514, 52.29057627198100988 ) ) ;
#51052=CARTESIAN_POINT ( 'NONE',  ( -13.97604488694547697, 13.89961937509957934, 68.12609039468563310 ) ) ;
#51053=CARTESIAN_POINT ( 'NONE',  ( -5.049401038297874678, -19.05341960407617918, 34.79275706135233293 ) ) ;
#51054=CARTESIAN_POINT ( 'NONE',  ( 9.564922557960805705, 16.46253265017160317, 59.58224293864769550 ) ) ;
#51055=CARTESIAN_POINT ( 'NONE',  ( -15.80617190586745835, -15.72974639402198527, 61.87390960531436690 ) ) ;
#51056=CARTESIAN_POINT ( 'NONE',  ( -16.55341960407611168, -4.379528057220339221, 71.45724293864769550 ) ) ;
#51057=CARTESIAN_POINT ( 'NONE',  ( 15.72974639402176855, 15.80617190586768217, 111.8760903946856615 ) ) ;
#51059=CARTESIAN_POINT ( 'NONE',  ( 0.05219959533909260263, 19.03943276465977164, 114.9989096053143669 ) ) ;
#51060=CARTESIAN_POINT ( 'NONE',  ( -0.05219959533909027116, -19.03943276465977164, 52.49890960531436690 ) ) ;
#51061=CARTESIAN_POINT ( 'NONE',  ( 9.564922557960805705, 16.46253265017160317, 34.58224293864770260 ) ) ;
#51062=CARTESIAN_POINT ( 'NONE',  ( -16.55341960407611168, -4.379528057220339221, 101.4572429386476955 ) ) ;
#51063=VECTOR ( 'NONE', #9170, 1000.000000000000000 ) ;
#51064=CARTESIAN_POINT ( 'NONE',  ( -21.52544592524343514, 5.823673210054127303, 106.0405762719810525 ) ) ;
#51065=CARTESIAN_POINT ( 'NONE',  ( 13.97604488694527802, 13.89961937509977652, 114.3739096053143669 ) ) ;
#51066=CARTESIAN_POINT ( 'NONE',  ( 10.72451020669871369, 18.67979575497193778, 32.08442372801901854 ) ) ;
#51067=CARTESIAN_POINT ( 'NONE',  ( 13.97604488694527802, 13.89961937509977652, 99.37390960531436690 ) ) ;
#51068=CARTESIAN_POINT ( 'NONE',  ( -19.05341960407611168, -5.049401038298163336, 21.45724293864768839 ) ) ;
#51069=CARTESIAN_POINT ( 'NONE',  ( -10.81492255796105439, 18.62759615963255655, 72.91775706135234714 ) ) ;
#51070=CARTESIAN_POINT ( 'NONE',  ( 21.52544592524344225, -5.823673210054117533, 98.54057627198105251 ) ) ;
#51074=CARTESIAN_POINT ( 'NONE',  ( 12.06949235617739724, 12.14591786802326823, 51.87609039468568284 ) ) ;
#51075=CARTESIAN_POINT ( 'NONE',  ( 16.52544592524342804, -4.483927247898539470, 113.5405762719810383 ) ) ;
#51077=CARTESIAN_POINT ( 'NONE',  ( 19.02544592524343514, -5.153800228976328945, 58.54057627198102409 ) ) ;
#51078=CARTESIAN_POINT ( 'NONE',  ( 8.224510206698953496, -14.34966873604960469, 92.91557627198103830 ) ) ;
#51079=EDGE_CURVE ( 'NONE', #92102, #72646, #49566, .T. ) ;
#51080=CARTESIAN_POINT ( 'NONE',  ( -5.719274019375978568, 21.55341960407610458, 45.20724293864769550 ) ) ;
#51081=CARTESIAN_POINT ( 'NONE',  ( 16.55341960407611168, 4.379528057220329451, 63.95724293864770260 ) ) ;
#51082=CARTESIAN_POINT ( 'NONE',  ( -13.97604488694547697, 13.89961937509957934, 113.1260903946856757 ) ) ;
#51083=CARTESIAN_POINT ( 'NONE',  ( -5.719274019375665041, -21.55341960407619695, 84.79275706135234714 ) ) ;
#51084=CARTESIAN_POINT ( 'NONE',  ( 16.21995358207303539, -7.366697692864228486, 77.43551001512156517 ) ) ;
#51085=CARTESIAN_POINT ( 'NONE',  ( -4.379528057220086978, -16.55341960407618274, 94.79275706135234714 ) ) ;
#51086=CARTESIAN_POINT ( 'NONE',  ( 8.314922557960818139, 14.29746914071049879, 39.58224293864769550 ) ) ;
#51087=CARTESIAN_POINT ( 'NONE',  ( 19.02544592524343514, -5.153800228976328945, 33.54057627198102409 ) ) ;
#51088=CARTESIAN_POINT ( 'NONE',  ( -5.049401038298153566, 19.05341960407611168, 85.20724293864766707 ) ) ;
#51089=CARTESIAN_POINT ( 'NONE',  ( 18.67979575497178502, 10.72451020669898547, 99.16557627198100988 ) ) ;
#51090=CARTESIAN_POINT ( 'NONE',  ( -12.14591786802326823, 12.06949235617739902, 38.12609039468567573 ) ) ;
#51091=CARTESIAN_POINT ( 'NONE',  ( 12.06949235617757843, -12.14591786802309237, 63.12390960531435979 ) ) ;
#51092=CARTESIAN_POINT ( 'NONE',  ( 5.823673210054444382, -21.52544592524334988, 80.20942372801901854 ) ) ;
#51093=VECTOR ( 'NONE', #21931, 1000.000000000000000 ) ;
#51094=CARTESIAN_POINT ( 'NONE',  ( -4.483927247898782831, 16.52544592524335698, 102.7094237280190185 ) ) ;
#51097=CARTESIAN_POINT ( 'NONE',  ( -12.14591786802309592, -12.06949235617757132, 26.87390960531435979 ) ) ;
#51098=CARTESIAN_POINT ( 'NONE',  ( 16.55341960407618274, -4.379528057220086978, 76.04275706135237556 ) ) ;
#51099=CARTESIAN_POINT ( 'NONE',  ( -5.153800228976328057, -19.02544592524343514, 87.29057627198103830 ) ) ;
#51100=CARTESIAN_POINT ( 'NONE',  ( -16.51473224551069308, -9.474510206698971260, 106.6655762719810383 ) ) ;
#51101=CARTESIAN_POINT ( 'NONE',  ( -10.72451020669870658, -18.67979575497194134, 89.58442372801901854 ) ) ;
#51102=CARTESIAN_POINT ( 'NONE',  ( 14.29746914071037800, 8.314922557961029526, 86.66775706135234714 ) ) ;
#51103=CARTESIAN_POINT ( 'NONE',  ( -4.379528057220328563, 16.55341960407611168, 65.20724293864768129 ) ) ;
#51104=CARTESIAN_POINT ( 'NONE',  ( 13.97604488694527802, 13.89961937509977652, 64.37390960531436690 ) ) ;
#51105=ORIENTED_EDGE ( 'NONE', *, *, #115652, .F. ) ;
#51106=CARTESIAN_POINT ( 'NONE',  ( 16.53943276465976808, 0.05219959533934440121, 31.25109039468568639 ) ) ;
#51107=( BOUNDED_SURFACE ( )  B_SPLINE_SURFACE ( 3, 2, ( 
 ( #78875, #142542, #140554, #50550, #112210, #143525, #66695, #4021, #62709, #109221, #65699, #128359, #2042, #190055, #3041, #141552, #113194, #93049, #126379, #188076, #49547, #174883, #172902, #1036, #170900, #189077, #34380, #154736, #186086, #25220, #146522, #129351, #40360, #86862, #148546, #162704, #22195, #132372, #56533, #83844, #177891, #53522, #145526, #116202, #70704, #8013, #84844, #36349, #99013, #24209, #159696, #10037, #160704, #7005, #68687, #178892, #71697, #85858, #192041, #69696, #147547, #176892, #131363, #23201, #117200, #130342, #175884, #98002, #115200, #39361, #193052, #38363, #133364, #191046, #102035, #195055, #118211, #9035, #100018, #194065, #21193, #161705, #101019, #54529, #55526, #163718, #82849, #144528, #6014, #67693, #52519, #114180, #37355, #26793, #183440, #104611, #136925, #27796, #195652, #137917, #30747, #12618, #28779, #44925, #120754, #88435, #41958, #76239, #107563, #166299, #105595, #119785, #198612, #92396, #135952, #184430, #197622, #89437, #57124, #151125, #150129, #154082, #74282, #182453, #60080, #199600, #29754, #59087, #90418, #43934, #15576, #196645, #167281, #45910, #168258, #61067, #153078, #103624, #165300, #180486, #73298, #122739, #152103, #13587, #75254, #134968, #118798, #121748, #169241, #106581, #133960, #91389, #14580, #11631, #58115, #181469, #42947, #2379, #46908, #100101, #93388, #113270, #170246, #31740, #130427, #17560, #79220, #51606, #160789, #83928, #161785, #140890, #21274, #32731, #7088, #66773, #128434, #155074, #77234, #22277, #176976, #190131, #191128, #159779, #82931, #144609, #62055, #94383, #108569, #138903, #16569, #67773, #383, #192126, #174962, #68769, #38446, #6094, #123720, #156062, #185417, #36426, #78216, #139886, #129430, #98081, #53607, #1375, #115283, #52602, #63054, #145609, #124734, #186431, #114264, #47907, #175968, #109561, #171242, #37437, #99097, #9115, #103115, #57619, #195136, #71776, #23280, #85938, #149619, #146604, #84924, #41450, #72792, #147627, #165793, #197129, #134462, #178973, #56617, #11117, #163798, #118291, #10116, #104111, #70782, #162781, #8097, #132450, #164796, #179982, #40440, #120262, #194141, #55605, #196147, #88937, #54603, #102113, #177967, #39435, #43436, #26291, #87932, #119287, #27290, #24289, #12124, #181954, #150628, #73788, #180970, #42447, #25300, #86942, #105105, #135460, #58596, #69775, #131443, #148626, #117279, #193130, #116277, #133446, #101095, #154580, #16076, #1887, #90900, #198113, #182948, #89932, #60567, #108065, #93896, #138414, #139400, #59580, #28292, #63568, #151613, #13105, #74770, #136432, #882, #76739, #155574, #29269, #31244, #152586, #124233, #185929, #109070, #170749, #77734, #121254, #44431, #62557, #140399, #106085, #47414, #200094, #137420, #17069, #166791, #45418, #61562, #14077, #199100, #169749, #122243, #167771, #32238, #125242, #107071, #123231, #78723, #153580, #75743, #183933, #186940, #48411, #168742, #184922, #30246, #92894, #91889, #15078, #46406, #112057, #80710, #33236, #127205, #2885, #130187, #65546, #96867, #174732, #114025, #5860, #142388, #66543, #158551, #191883, #172744, #81684, #160552, #144373, #175722, #129194, #79728, #141397, #156578, #49393, #37201, #3867, #188919, #50397, #111056, #94894, #113040, #98857, #173745, #52368, #143366, #35214, #68532, #67536, #128207, #22042, #20041, #64564, #110067, #126229, #4858, #187924, #34225, #83693, #189904, #51379, #36195, #190892, #145371, #171747, #97849, #159538, #21036, #6853, #82689, #18073, #95887, #157570, #19063, #150397, #40195, #164559, #133205, #56370, #118053, #38210, #8876, #84688, #53367, #192897, #41213, #73556, #165558, #117037, #42217, #11893, #179743, #176737, #132212, #54374, #102874, #26053, #99866, #103878, #70544, #135229, #25057, #27055, #146368, #162542, #115045, #87697, #161550, #116046, #149382, #10878, #88701, #85702, #23043, #72548, #7855, #134226, #69542 ),
 ( #195911, #131206, #177735, #57386, #119059, #39204, #147388, #100860, #180741, #24046, #193903, #55367, #178732, #101875, #163557, #86700, #148385, #9879, #71539, #194896, #183708, #151385, #104870, #139174, #170518, #167546, #168523, #182715, #199871, #93664, #198876, #47178, #60343, #29041, #120035, #13848, #89699, #16839, #152363, #45194, #61335, #650, #92663, #90681, #153348, #106848, #78489, #59349, #30021, #108837, #31013, #62320, #15844, #166559, #28058, #43203, #136205, #123990, #75515, #137189, #122017, #197880, #181721, #123006, #185688, #91659, #32007, #14850, #76512, #155349, #154351, #138188, #196901, #184692, #12875, #58368, #74540, #46176, #121017, #44200, #105859, #107829, #169513, #77503, #20799, #144142, #21809, #80479, #81453, #95651, #67303, #65315, #3637, #17839, #160318, #82454, #36963, #126974, #51146, #19812, #143139, #4619, #125010, #157339, #171516, #140162, #79497, #127971, #1654, #52138, #188683, #128962, #98624, #66310, #64332, #33005, #156339, #63332, #33995, #189674, #190662, #111821, #112807, #94660, #186706, #175490, #48177, #109833, #141166, #2655, #174500, #50163, #113795, #126000, #35967, #187697, #97614, #159304, #5626, #49167, #110826, #172510, #18834, #142153, #173509, #34982, #96635, #158323, #54145, #72315, #83461, #162315, #116811, #130971, #103654, #39968, #6621, #37978, #148160, #70317, #10652, #84457, #133991, #193669, #176501, #87475, #195682, #57153, #9651, #69305, #179514, #165332, #192662, #24825, #100634, #115818, #163329, #117821, #55140, #131984, #145138, #146135, #71317, #68300, #129951, #101638, #132980, #7621, #25831, #118832, #194671, #38978, #178502, #56140, #23816, #86475, #40982, #164336, #177508, #22811, #191651, #85466, #102651, #149162, #147155, #180515, #8643, #41988, #53130, #114809, #99635, #161318, #181500, #42978, #46939, #121781, #198647, #168291, #169274, #27828, #15607, #185449, #92427, #77264, #137949, #76271, #28813, #90453, #123750, #199632, #122772, #154113, #138933, #167317, #151160, #60113, #184462, #59119, #413, #14614, #61099, #62087, #152137, #104643, #108599, #30780, #26824, #13620, #45941, #106617, #29787, #91423, #11662, #182485, #58147, #88465, #166330, #107596, #150162, #73328, #75287, #135000, #196678, #153110, #119815, #105628, #89469, #12648, #74315, #135982, #197653, #43966, #120785, #183475, #136958, #44959, #79253, #128727, #96399, #155105, #32764, #158086, #19578, #143903, #2411, #5385, #34740, #63087, #81221, #140925, #173266, #64091, #31770, #174266, #67068, #48927, #65076, #142902, #157096, #124766, #78246, #112572, #190423, #125759, #141910, #156096, #4384, #51899, #172262, #20561, #33752, #187459, #93418, #110581, #186464, #170276, #95411, #18592, #66069, #35734, #127735, #80240, #126734, #3401, #16598, #94416, #188437, #82212, #189437, #97381, #50914, #139919, #1408, #47942, #109593, #159067, #49916, #111581, #171276, #17594, #36718, #116574, #179272, #69065, #55899, #85220, #115581, #72066, #147922, #131743, #25592, #38740, #83224, #133739, #129715, #146911, #6382, #68061, #164093, #53906, #177269, #8400, #194428, #117572, #195434, #100398, #54900, #130732, #40736, #162078, #191412, #175252, #148919, #98380, #160077, #21564, #144899, #9408, #23572, #102406, #176260, #178263, #37731, #71074, #132740, #87236, #10408, #24584, #52888, #114563, #101387, #113558, #99393, #161076, #70075, #84218, #22571, #145897, #192424, #193425, #7381, #39726, #163080, #86232, #11414, #121539, #43725, #184222, #57907, #45703, #167073, #149907, #60856, #107354, #169027, #183234, #42739, #152872, #77023, #104401, #198395, #74073, #166083, #136714, #91183, #28575, #105386, #56909, #119579, #44715, #180274, #118584, #75048, #106371, #181262, #199392, #30532, #168053, #12411, #90211, #29550, #197415, #151894, #13384, #137708, #27586, #196437, #41744, #89224, #59873, #14367, #135744, #153869, #150918, #58881, #76033, #122531 ),
 ( #120547, #92185, #15367, #138695, #103408, #165086, #26580, #88223, #73084, #182240, #134755, #32524, #17353, #171033, #1166, #123514, #3172, #65829, #155855, #142671, #172027, #2174, #158832, #34510, #18357, #112338, #125525, #170038, #20320, #62841, #47701, #111341, #127498, #31528, #79008, #154866, #16363, #81969, #95175, #33515, #141681, #4150, #124525, #189203, #177, #50680, #174028, #173032, #49677, #63854, #187222, #97149, #96168, #157858, #35499, #61845, #140682, #186220, #156862, #19348, #94176, #185207, #188205, #80996, #46698, #109351, #93181, #78011, #108360, #48693, #64845, #139679, #80012, #110345, #126507, #5144, #179026, #66826, #128490, #190185, #51660, #178019, #53662, #132504, #6147, #8152, #67828, #101147, #162833, #85992, #147682, #54656, #113324, #98137, #131496, #117332, #82987, #24342, #115340, #114320, #194193, #143661, #22331, #177030, #191182, #163853, #100156, #175016, #159835, #69829, #130484, #70836, #144663, #55658, #38500, #36481, #9169, #40494, #102166, #193183, #129484, #39487, #25353, #52657, #84976, #160842, #176022, #23332, #21329, #161838, #192181, #37491, #99153, #116330, #83982, #145661, #146658, #7142, #68825, #32039, #63363, #139206, #45223, #61365, #15876, #30049, #123036, #76543, #170548, #11171, #26345, #148681, #134516, #31044, #46206, #106878, #186736, #109861, #1686, #153381, #78519, #48207, #92693, #10169, #168551, #87985, #681, #154381, #71829, #140193, #91690, #171546, #184722, #125040, #118343, #196202, #86994, #77534, #133498, #149673, #62352, #124022, #195190, #119341, #56670, #185720, #180037, #47210, #57674, #108869, #183737, #41505, #93696, #103169, #14882, #107860, #155379, #138219, #164849, #72847, #16868, #199901, #169545, #4651, #18865, #35998, #129981, #35012, #83492, #96667, #3668, #156368, #50197, #126031, #53162, #188714, #19843, #97645, #36995, #128995, #65346, #189706, #81484, #114840, #95684, #66342, #145169, #67333, #98656, #52168, #2685, #64362, #79526, #172541, #160350, #127006, #111853, #173543, #34026, #17872, #159334, #21839, #158354, #175520, #128004, #143171, #191681, #190693, #51179, #6653, #112839, #187727, #33034, #49198, #174531, #110856, #157371, #68331, #20831, #82487, #144171, #113825, #94690, #141196, #5657, #80511, #142184, #103683, #101669, #39997, #54176, #196706, #118861, #73358, #163359, #87504, #56170, #179544, #41013, #161350, #132013, #7651, #176534, #115849, #164365, #58176, #116840, #117851, #193700, #165362, #24855, #86504, #177538, #38010, #180544, #135031, #148188, #149192, #102680, #25860, #10681, #22841, #55169, #69335, #99665, #39008, #72346, #84488, #88497, #9682, #26856, #146165, #134020, #131001, #178530, #100663, #195712, #57184, #192693, #150194, #71347, #162345, #133010, #11692, #23846, #85496, #147184, #42018, #8673, #70346, #194701, #169303, #93450, #152165, #155137, #184492, #12676, #30809, #90483, #122802, #13648, #181528, #123782, #16631, #198675, #14643, #92458, #106648, #74343, #27858, #62119, #78278, #75315, #91453, #105657, #45971, #139951, #121809, #170308, #183505, #136986, #43007, #60142, #136009, #1441, #44988, #168320, #107625, #185481, #15638, #29817, #76303, #153141, #119843, #182516, #137981, #31801, #154146, #46971, #138966, #89498, #151188, #166360, #59146, #108630, #199663, #61129, #77295, #120816, #104674, #444, #197681, #43995, #167345, #28842, #65106, #21593, #97408, #81249, #175281, #188467, #32794, #83252, #79285, #96429, #156127, #17626, #113587, #3430, #126764, #34772, #143931, #67096, #50942, #112600, #98410, #187491, #94447, #140955, #186496, #157126, #4412, #190452, #158115, #35762, #2442, #124798, #160106, #47972, #109624, #171308, #64124, #159095, #173298, #51927, #125789, #127764, #48957, #20589, #82241, #5413, #128755, #174292, #110610, #172293, #36746, #144927, #33782, #63119, #19607, #95442, #18622, #80269, #141939, #142931, #49949, #111613 ),
 ( #189464, #66097, #102434, #26609, #192451, #147950, #23603, #53933, #86260, #40765, #178290, #54929, #6408, #69092, #132768, #129742, #68089, #24612, #55926, #130759, #148948, #180304, #117600, #162106, #39754, #194455, #146940, #101416, #193453, #87263, #115608, #145926, #191439, #177297, #9436, #163109, #85249, #103437, #38768, #100425, #179301, #72098, #37760, #8430, #161104, #22599, #88252, #71101, #164121, #25619, #10438, #7409, #195465, #165117, #133770, #56940, #118614, #41772, #70102, #131771, #52915, #114591, #176288, #99421, #84246, #116602, #74104, #183264, #45735, #182272, #207, #135774, #91210, #167101, #197445, #29579, #184253, #121569, #198427, #149938, #12442, #76063, #73116, #11444, #168082, #199422, #58911, #92217, #123546, #60887, #105418, #44744, #137738, #90240, #106400, #136743, #30566, #120579, #89256, #134785, #43754, #152901, #14397, #28602, #46731, #151923, #13412, #122563, #15398, #181291, #75076, #104431, #166114, #170070, #107387, #169060, #153903, #77055, #150948, #138727, #108393, #61876, #185240, #31561, #196467, #59901, #57937, #119608, #42769, #27617, #158863, #20352, #33546, #17385, #126536, #189234, #125557, #143693, #81026, #142702, #128520, #79040, #124556, #109384, #16396, #187254, #34540, #82000, #64875, #65860, #186253, #154897, #190215, #78042, #139711, #1199, #62875, #127531, #3201, #5176, #155887, #157888, #140715, #50712, #112370, #35530, #97178, #4181, #47731, #171064, #174062, #66858, #32554, #51694, #188235, #63886, #113356, #93212, #172059, #49710, #2205, #175048, #111374, #94208, #48723, #19377, #80041, #110376, #95207, #156894, #173063, #18390, #141710, #96199, #148713, #162869, #22365, #132537, #56703, #8189, #117365, #40530, #118376, #177064, #178053, #192215, #163890, #161872, #100190, #114351, #36513, #179061, #133530, #23366, #147716, #116364, #39521, #101181, #21361, #53698, #67858, #98168, #176056, #24377, #159868, #10201, #85012, #25386, #195222, #86028, #83019, #115375, #37523, #9204, #70869, #144693, #87028, #38534, #6178, #69864, #71861, #129513, #145695, #191213, #194226, #52688, #99186, #55691, #102201, #160875, #68860, #84017, #7177, #130519, #146692, #131533, #193217, #54691, #41539, #184018, #76822, #58677, #74852, #90982, #166874, #134547, #88017, #122326, #153666, #150711, #151697, #165877, #183031, #138493, #182039, #30331, #43522, #12210, #103202, #197215, #72879, #200175, #135543, #28375, #44514, #45500, #75827, #73873, #136514, #90013, #61644, #42533, #13188, #91972, #14159, #107155, #199185, #149705, #11204, #26378, #119375, #168825, #120344, #105187, #198195, #181057, #164883, #106170, #15162, #59665, #180070, #121338, #167853, #196236, #137505, #29353, #57705, #152670, #104196, #27374, #89020, #60653, #154663, #16159, #19141, #17152, #78805, #34305, #170832, #155657, #109153, #139482, #185005, #156660, #95967, #32324, #172826, #187023, #140484, #127286, #126307, #171827, #80791, #1971, #31326, #188999, #77813, #48494, #964, #62640, #142469, #63652, #125326, #110148, #111136, #157651, #123312, #33315, #18155, #94975, #3947, #79809, #141482, #124316, #46489, #65626, #108151, #2965, #49473, #64645, #188003, #169833, #186015, #92978, #47496, #93977, #43176, #91634, #123961, #15815, #167520, #92635, #623, #106823, #27029, #182689, #104843, #153322, #168497, #88674, #154326, #120991, #62294, #75489, #77476, #135203, #12848, #185659, #29995, #150370, #166534, #14824, #76485, #139146, #136180, #103852, #138162, #196875, #199843, #74514, #61310, #197855, #165533, #107803, #11866, #44174, #198851, #122980, #90655, #58342, #73531, #46149, #120010, #59322, #137162, #89672, #184667, #181695, #105833, #28031, #29015, #152337, #151359, #13823, #60315, #121991, #183682, #45167, #169487, #30987, #143112, #17812, #3609, #33967, #128933, #109805, #18806, #97587, #81426, #112779, #66284, #16809, #78459, #93635, #186678, #111794, #171488 ),
 ( #50135, #31979, #2627, #140133, #47151, #48148, #34955, #67275, #159275, #110798, #35941, #144115, #173482, #170488, #125971, #32977, #96607, #158296, #155320, #20771, #64304, #5595, #80451, #82427, #1625, #156310, #108809, #19785, #63301, #94631, #4591, #127943, #124981, #79468, #141137, #189645, #187670, #51120, #49140, #174472, #172479, #95624, #157309, #142124, #65288, #126947, #188655, #177477, #145108, #98596, #132951, #164307, #161286, #162285, #176472, #193638, #87446, #192632, #40949, #54114, #22780, #113766, #7589, #83431, #10622, #146105, #38946, #55110, #194639, #86444, #84428, #147126, #100603, #72283, #53100, #23785, #102621, #24796, #56109, #9621, #160289, #21780, #36933, #129921, #117790, #69275, #130942, #115788, #191621, #175462, #116780, #179485, #85435, #25800, #8613, #70286, #149131, #148130, #131954, #190634, #178471, #6591, #52109, #68270, #39938, #114779, #37946, #99606, #101607, #163297, #71286, #187201, #186198, #81945, #48672, #190161, #3149, #143636, #62819, #140661, #51637, #157835, #16341, #94155, #19326, #80973, #5120, #63831, #66802, #96146, #124503, #142649, #2153, #34488, #125503, #93159, #35476, #128465, #110324, #126485, #4128, #18335, #47679, #139657, #174005, #113301, #172005, #64823, #17331, #65807, #31506, #33493, #154844, #95151, #156840, #77990, #79990, #109330, #1145, #141658, #188183, #127475, #97125, #189181, #49655, #111319, #173009, #171012, #155834, #50654, #32503, #112315, #158808, #20297, #78986, #6123, #21306, #114297, #179003, #7119, #192157, #145639, #175999, #98114, #177996, #40471, #130460, #117307, #146635, #177007, #133474, #9145, #193160, #86971, #100133, #144640, #195166, #191160, #8127, #67806, #129461, #25329, #115315, #38476, #69805, #39463, #148658, #161814, #68801, #116307, #53638, #102143, #23309, #84953, #52633, #56647, #163828, #71806, #131473, #85968, #54632, #101124, #162810, #159811, #24319, #37469, #174992, #99130, #147657, #36456, #10146, #70812, #82963, #160820, #132481, #22308, #194170, #83959, #55634, #182977, #103144, #15107, #197160, #13136, #29299, #105135, #72822, #26322, #60597, #91918, #88967, #89961, #104141, #121284, #76768, #120292, #168770, #181985, #150657, #41480, #135490, #11148, #138440, #73820, #166821, #44461, #122272, #14105, #12155, #74798, #28322, #200121, #181002, #151641, #30273, #152615, #183960, #137451, #87962, #149650, #164826, #57650, #45447, #58625, #43467, #136460, #119316, #134491, #106115, #107100, #198141, #153611, #59611, #167799, #118320, #75773, #90929, #180013, #199130, #196178, #42478, #165823, #27320, #154608, #16103, #112085, #1917, #63596, #33263, #64592, #35241, #125271, #32267, #2913, #17097, #188949, #186969, #48439, #139427, #81711, #3896, #158578, #110096, #172774, #141427, #126256, #187953, #46434, #78750, #92922, #61590, #909, #49422, #143397, #173775, #171774, #50426, #20068, #111084, #184949, #140427, #62584, #34255, #95914, #108093, #96895, #94922, #123258, #156607, #169777, #77761, #170777, #31271, #157598, #124262, #185957, #19090, #80738, #47441, #93924, #109098, #142417, #155602, #65575, #18102, #127235, #79756, #66568, #8902, #116072, #54400, #6880, #68558, #101901, #177760, #100885, #70570, #132238, #145397, #129221, #38236, #162568, #37228, #55393, #192922, #39229, #40224, #190918, #36222, #21064, #128233, #98885, #146393, #193930, #176764, #24072, #97874, #189930, #163583, #51405, #113065, #174757, #159566, #85727, #115072, #160579, #82719, #161576, #117063, #147414, #178758, #25083, #86726, #4886, #144401, #5887, #67563, #52395, #114052, #175751, #99891, #22068, #83719, #130214, #191909, #23069, #53394, #84715, #7882, #69567, #131234, #15620, #137962, #78259, #149408, #139932, #61111, #41239, #155118, #1421, #63100, #77277, #134251, #46952, #171289, #195938, #92440, #165584, #57412, #30792, #185462, #122784, #199645, #148411, #10903, #138946, #71566 ),
 ( #31783, #72577, #87723, #9906, #119085, #154126, #107608, #103903, #47954, #180766, #42242, #62100, #16612, #179770, #29799, #102900, #164585, #32776, #45953, #184474, #426, #93432, #91435, #124779, #109605, #186477, #133231, #123763, #194922, #153122, #14626, #108612, #76283, #56398, #169286, #170289, #26079, #118080, #36730, #191424, #81233, #5396, #174277, #97392, #159078, #79265, #49929, #125771, #94428, #33764, #82224, #114575, #6394, #158098, #83235, #52900, #20572, #17606, #173279, #95424, #143914, #67079, #140937, #144911, #111593, #176273, #66080, #68073, #187471, #3413, #156109, #128739, #2424, #157108, #190435, #51911, #129727, #126747, #64104, #113570, #48940, #175264, #65088, #98392, #188449, #110593, #160090, #172275, #34752, #189448, #21577, #142914, #18604, #80252, #141922, #96411, #19590, #127746, #4396, #50925, #112583, #35746, #88237, #39738, #8414, #161088, #54914, #130744, #57922, #193438, #24597, #102419, #41757, #133755, #70087, #194440, #86245, #119593, #100410, #9421, #149922, #72081, #103422, #56923, #7394, #69078, #84231, #177282, #165101, #131756, #116586, #178275, #38753, #22583, #40750, #26594, #101400, #180289, #71086, #163093, #196452, #195449, #55911, #11428, #147935, #192436, #37745, #53919, #132753, #115593, #162091, #73098, #117585, #179285, #164106, #25605, #134769, #87249, #148933, #99405, #23586, #85234, #146924, #145909, #10423, #118599, #108379, #152887, #153887, #74089, #42753, #16381, #104416, #166099, #27601, #89239, #15384, #91197, #136729, #135759, #137724, #93198, #138712, #193, #123531, #185225, #92203, #150933, #197430, #169045, #154883, #120562, #61862, #14382, #151910, #170055, #181276, #59888, #76048, #28589, #1183, #199408, #12426, #58896, #45720, #168068, #31546, #182256, #78028, #60872, #43741, #46716, #139697, #62860, #107373, #167088, #77041, #105402, #90226, #122549, #198411, #13399, #184239, #75063, #30551, #29566, #121554, #183250, #44731, #106387, #186239, #142688, #174048, #48709, #66844, #98153, #35517, #80028, #96186, #50698, #64861, #157875, #111360, #5161, #110362, #63872, #47717, #172044, #65846, #81013, #141697, #21346, #187239, #33531, #97165, #190202, #155873, #3188, #79025, #140700, #144679, #19364, #4168, #127516, #128507, #125543, #113342, #83004, #51680, #175034, #158850, #20338, #126523, #188222, #6164, #81987, #143680, #36499, #159853, #49695, #95193, #189220, #124542, #109368, #171050, #32540, #94193, #34526, #173049, #2190, #112357, #17370, #156879, #18376, #10189, #71849, #179047, #37508, #22350, #55677, #41526, #7162, #25373, #178038, #38519, #56690, #67844, #146677, #101166, #115359, #88005, #24361, #191199, #84001, #132523, #54675, #195210, #68845, #118364, #39506, #160860, #133518, #180057, #103189, #194212, #53682, #163874, #149693, #177049, #9189, #84996, #100175, #147701, #102186, #162854, #116349, #129499, #130504, #117351, #52674, #114337, #86012, #40515, #192200, #164870, #26365, #87015, #23351, #70854, #148701, #8172, #176040, #99170, #145680, #161857, #69848, #131516, #193202, #152655, #167838, #166860, #108133, #73861, #58664, #122311, #76807, #42520, #28362, #165865, #27361, #31308, #106156, #183016, #14145, #153650, #12196, #200159, #169817, #138478, #61629, #184002, #60637, #13174, #74837, #92961, #45485, #107140, #123297, #184989, #151682, #135530, #44500, #168810, #43508, #46473, #199170, #30314, #11191, #197201, #104183, #89007, #134535, #105174, #75812, #72866, #29339, #91957, #150698, #196223, #57693, #119361, #137490, #181045, #90968, #15145, #120330, #182025, #90000, #136500, #198180, #59650, #121324, #188983, #64628, #110132, #109136, #111119, #66602, #112118, #173810, #96930, #158612, #65610, #124299, #170815, #142452, #128266, #93961, #35275, #126290, #125310, #143433, #154647, #33299, #187987, #1955, #174790, #172808, #77797, #32307, #19124, #141465, #81746, #155641, #4919, #49457, #47479 ),
 ( #17136, #80774, #3930, #189964, #187006, #51439, #127270, #78788, #50459, #48476, #157635, #171811, #16142, #20102, #113099, #94958, #34289, #36256, #2949, #140465, #62621, #139466, #946, #156642, #95950, #63634, #185996, #18138, #79792, #148444, #99923, #68591, #21098, #115104, #190951, #118112, #53427, #84748, #162603, #101934, #193963, #130247, #54434, #146426, #179801, #160611, #69600, #9939, #132272, #163616, #117097, #67597, #129256, #144434, #37261, #25117, #191942, #176796, #38269, #98919, #82754, #100918, #86761, #161608, #40261, #131267, #23102, #56432, #55426, #7916, #52428, #97909, #192955, #116104, #24107, #71598, #178792, #177792, #39262, #85761, #159600, #22101, #147448, #133264, #194955, #5920, #114086, #175787, #83751, #145430, #6913, #8936, #70605, #58422, #11947, #42275, #164617, #44254, #106901, #196954, #183761, #12926, #43258, #199926, #75568, #59402, #153407, #166613, #10935, #61389, #57442, #74590, #134282, #195970, #91713, #181777, #104926, #136258, #105911, #14905, #28115, #73611, #182770, #120089, #168574, #89753, #151439, #119115, #123061, #45247, #138242, #197934, #152414, #121076, #167597, #29092, #26111, #90731, #72608, #41270, #180796, #13902, #102932, #76567, #137244, #30072, #87754, #198929, #149439, #60397, #103933, #122069, #165613, #27112, #88758, #150451, #135282, #156392, #35036, #15901, #93720, #143196, #110880, #169573, #47235, #172565, #34051, #158379, #16892, #19868, #49222, #77559, #95708, #155402, #187752, #78543, #46232, #188738, #81508, #63387, #79550, #157396, #171570, #139231, #92718, #127031, #4676, #140218, #17896, #170573, #18889, #66368, #186761, #96691, #48231, #1711, #107886, #184747, #50223, #31070, #33059, #80535, #64387, #142209, #3692, #154407, #125064, #706, #62378, #124048, #65371, #185747, #108894, #109886, #173567, #32064, #111877, #94714, #141219, #2710, #126055, #192716, #112864, #178553, #145192, #86527, #99689, #40019, #159360, #37020, #148211, #54200, #174555, #190718, #115872, #177561, #101692, #160374, #163381, #39030, #20857, #100685, #98681, #131027, #21865, #189730, #132036, #24878, #6675, #22864, #162367, #114863, #82514, #36022, #70368, #9705, #83515, #161373, #113849, #23868, #128028, #130004, #51203, #191704, #68353, #97671, #53188, #144196, #5682, #176558, #38033, #85519, #193725, #147207, #84511, #146189, #7674, #67358, #52191, #69358, #129018, #8698, #55193, #116862, #175545, #102702, #117876, #10706, #75339, #103706, #88522, #42042, #72369, #194723, #74365, #137009, #26879, #13672, #43030, #73382, #29840, #105682, #89521, #183528, #196730, #41036, #91477, #87528, #104696, #164390, #25883, #121834, #11715, #135054, #166384, #136031, #45011, #58198, #165386, #12699, #150218, #198699, #119866, #181551, #149215, #134043, #60165, #27880, #151211, #197705, #195736, #56193, #59171, #106671, #120840, #168344, #182539, #44021, #153165, #167368, #28866, #71369, #90506, #57209, #133033, #118884, #152188, #180568, #179566, #65131, #155162, #16654, #186521, #17649, #188494, #78301, #185504, #156151, #170332, #141965, #139975, #1464, #92482, #34797, #157152, #111637, #63142, #125812, #94470, #79309, #140978, #199688, #31825, #45995, #14666, #154171, #2466, #96452, #126788, #124821, #3454, #173322, #64148, #138004, #93475, #15662, #187515, #48981, #61153, #49973, #47995, #76327, #109649, #122825, #107650, #123806, #184515, #110636, #169327, #77321, #172317, #33806, #30834, #46995, #138989, #95466, #467, #18647, #108654, #80293, #171331, #62142, #32819, #57719, #39534, #55705, #71875, #147729, #112625, #66123, #103216, #134562, #131547, #132551, #146706, #163904, #119389, #162883, #11218, #24392, #193232, #81273, #178066, #50966, #181072, #116377, #9216, #25400, #164898, #56718, #54705, #117378, #70883, #42547, #20615, #194239, #72894, #195235, #26392, #180084, #127788, #189488, #4435, #41553, #174317, #35787, #97434 ) ),
 .UNSPECIFIED., .T., .F., .T. ) 
 B_SPLINE_SURFACE_WITH_KNOTS ( ( 4, 3, 4 ),
 ( 3, 2, 2, 2, 2, 2, 2, 2, 2, 2, 2, 2, 2, 2, 2, 2, 2, 2, 2, 2, 2, 2, 2, 2, 2, 2, 2, 2, 2, 2, 2, 2, 2, 2, 2, 2, 2, 2, 2, 2, 2, 2, 2, 2, 2, 2, 2, 2, 2, 2, 2, 2, 2, 2, 2, 2, 2, 2, 2, 2, 2, 2, 2, 2, 2, 2, 2, 2, 2, 2, 2, 2, 2, 2, 2, 2, 2, 2, 2, 2, 2, 2, 2, 2, 2, 2, 2, 2, 2, 2, 2, 2, 2, 2, 2, 2, 2, 2, 2, 2, 2, 2, 2, 2, 2, 2, 2, 2, 2, 2, 2, 2, 2, 2, 2, 2, 2, 2, 2, 2, 2, 2, 2, 2, 2, 2, 2, 2, 2, 2, 2, 2, 2, 2, 2, 2, 2, 2, 2, 2, 2, 2, 2, 2, 2, 2, 2, 2, 2, 2, 2, 2, 2, 2, 2, 2, 2, 2, 2, 2, 2, 2, 2, 2, 2, 2, 2, 2, 2, 2, 2, 2, 2, 2, 2, 2, 2, 2, 2, 2, 2, 2, 2, 2, 2, 2, 2, 2, 2, 2, 2, 2, 2, 2, 2, 2, 2, 2, 2, 2, 2, 2, 2, 2, 2, 2, 2, 2, 2, 2, 2, 2, 2, 2, 2, 2, 2, 2, 2, 2, 2, 2, 2, 2, 2, 2, 2, 2, 3 ),
 ( 0.000000000000000000, 0.5000000000000000000, 1.000000000000000000 ),
 ( 0.000000000000000000, 0.004385964912280701511, 0.008771929824561403022, 0.01315789473684210453, 0.01754385964912280604, 0.02192982456140350755, 0.02631578947368420907, 0.03070175438596491058, 0.03508771929824561209, 0.03947368421052631360, 0.04385964912280701511, 0.04824561403508771662, 0.05263157894736841813, 0.05701754385964911964, 0.06140350877192982115, 0.06578947368421052266, 0.07017543859649122417, 0.07456140350877192569, 0.07894736842105262720, 0.08333333333333332871, 0.08771929824561403022, 0.09210526315789473173, 0.09649122807017543324, 0.1008771929824561348, 0.1052631578947368363, 0.1096491228070175378, 0.1140350877192982393, 0.1184210526315789408, 0.1228070175438596423, 0.1271929824561403577, 0.1315789473684210453, 0.1359649122807017607, 0.1403508771929824483, 0.1447368421052631637, 0.1491228070175438514, 0.1535087719298245668, 0.1578947368421052544, 0.1622807017543859698, 0.1666666666666666574, 0.1710526315789473728, 0.1754385964912280604, 0.1798245614035087758, 0.1842105263157894635, 0.1885964912280701788, 0.1929824561403508665, 0.1973684210526315819, 0.2017543859649122695, 0.2061403508771929849, 0.2105263157894736725, 0.2149122807017543879, 0.2192982456140350755, 0.2236842105263157909, 0.2280701754385964786, 0.2324561403508771940, 0.2368421052631578816, 0.2412280701754385970, 0.2456140350877192846, 0.2500000000000000000, 0.2543859649122807154, 0.2587719298245614308, 0.2631578947368420907, 0.2675438596491228060, 0.2719298245614035214, 0.2763157894736842368, 0.2807017543859648967, 0.2850877192982456121, 0.2894736842105263275, 0.2938596491228070429, 0.2982456140350877027, 0.3026315789473684181, 0.3070175438596491335, 0.3114035087719298489, 0.3157894736842105088, 0.3201754385964912242, 0.3245614035087719396, 0.3289473684210526550, 0.3333333333333333148, 0.3377192982456140302, 0.3421052631578947456, 0.3464912280701754610, 0.3508771929824561209, 0.3552631578947368363, 0.3596491228070175517, 0.3640350877192982670, 0.3684210526315789269, 0.3728070175438596423, 0.3771929824561403577, 0.3815789473684210731, 0.3859649122807017330, 0.3903508771929824483, 0.3947368421052631637, 0.3991228070175438791, 0.4035087719298245390, 0.4078947368421052544, 0.4122807017543859698, 0.4166666666666666852, 0.4210526315789473450, 0.4254385964912280604, 0.4298245614035087758, 0.4342105263157894912, 0.4385964912280701511, 0.4429824561403508665, 0.4473684210526315819, 0.4517543859649122973, 0.4561403508771929571, 0.4605263157894736725, 0.4649122807017543879, 0.4692982456140351033, 0.4736842105263157632, 0.4780701754385964786, 0.4824561403508771940, 0.4868421052631579093, 0.4912280701754385692, 0.4956140350877192846, 0.5000000000000000000, 0.5043859649122807154, 0.5087719298245614308, 0.5131578947368421462, 0.5175438596491228616, 0.5219298245614034659, 0.5263157894736841813, 0.5307017543859648967, 0.5350877192982456121, 0.5394736842105263275, 0.5438596491228070429, 0.5482456140350877583, 0.5526315789473684736, 0.5570175438596490780, 0.5614035087719297934, 0.5657894736842105088, 0.5701754385964912242, 0.5745614035087719396, 0.5789473684210526550, 0.5833333333333333703, 0.5877192982456140857, 0.5921052631578946901, 0.5964912280701754055, 0.6008771929824561209, 0.6052631578947368363, 0.6096491228070175517, 0.6140350877192982670, 0.6184210526315789824, 0.6228070175438596978, 0.6271929824561403022, 0.6315789473684210176, 0.6359649122807017330, 0.6403508771929824483, 0.6447368421052631637, 0.6491228070175438791, 0.6535087719298245945, 0.6578947368421053099, 0.6622807017543859143, 0.6666666666666666297, 0.6710526315789473450, 0.6754385964912280604, 0.6798245614035087758, 0.6842105263157894912, 0.6885964912280702066, 0.6929824561403509220, 0.6973684210526315264, 0.7017543859649122417, 0.7061403508771929571, 0.7105263157894736725, 0.7149122807017543879, 0.7192982456140351033, 0.7236842105263158187, 0.7280701754385965341, 0.7324561403508771384, 0.7368421052631578538, 0.7412280701754385692, 0.7456140350877192846, 0.7500000000000000000, 0.7543859649122807154, 0.7587719298245614308, 0.7631578947368421462, 0.7675438596491228616, 0.7719298245614034659, 0.7763157894736841813, 0.7807017543859648967, 0.7850877192982456121, 0.7894736842105263275, 0.7938596491228070429, 0.7982456140350877583, 0.8026315789473684736, 0.8070175438596490780, 0.8114035087719297934, 0.8157894736842105088, 0.8201754385964912242, 0.8245614035087719396, 0.8289473684210526550, 0.8333333333333333703, 0.8377192982456140857, 0.8421052631578946901, 0.8464912280701754055, 0.8508771929824561209, 0.8552631578947368363, 0.8596491228070175517, 0.8640350877192982670, 0.8684210526315789824, 0.8728070175438596978, 0.8771929824561403022, 0.8815789473684210176, 0.8859649122807017330, 0.8903508771929824483, 0.8947368421052631637, 0.8991228070175438791, 0.9035087719298245945, 0.9078947368421053099, 0.9122807017543859143, 0.9166666666666666297, 0.9210526315789473450, 0.9254385964912280604, 0.9298245614035087758, 0.9342105263157894912, 0.9385964912280702066, 0.9429824561403509220, 0.9473684210526315264, 0.9517543859649122417, 0.9561403508771929571, 0.9605263157894736725, 0.9649122807017543879, 0.9692982456140351033, 0.9736842105263158187, 0.9780701754385965341, 0.9824561403508771384, 0.9868421052631578538, 0.9912280701754385692, 0.9956140350877192846, 1.000000000000000000 ),
 .UNSPECIFIED. ) 
 GEOMETRIC_REPRESENTATION_ITEM ( )  RATIONAL_B_SPLINE_SURFACE ( (
 ( 1.000000000000000000, 0.9659258262890683122, 1.000000000000000000, 0.9659258262890683122, 1.000000000000000000, 0.9659258262890683122, 1.000000000000000000, 0.9659258262890683122, 1.000000000000000000, 0.9659258262890683122, 1.000000000000000000, 0.9659258262890683122, 1.000000000000000000, 0.9659258262890683122, 1.000000000000000000, 0.9659258262890683122, 1.000000000000000000, 0.9659258262890683122, 1.000000000000000000, 0.9659258262890683122, 1.000000000000000000, 0.9659258262890683122, 1.000000000000000000, 0.9659258262890683122, 1.000000000000000000, 0.9659258262890683122, 1.000000000000000000, 0.9659258262890683122, 1.000000000000000000, 0.9659258262890683122, 1.000000000000000000, 0.9659258262890683122, 1.000000000000000000, 0.9659258262890683122, 1.000000000000000000, 0.9659258262890683122, 1.000000000000000000, 0.9659258262890683122, 1.000000000000000000, 0.9659258262890683122, 1.000000000000000000, 0.9659258262890683122, 1.000000000000000000, 0.9659258262890683122, 1.000000000000000000, 0.9659258262890683122, 1.000000000000000000, 0.9659258262890683122, 1.000000000000000000, 0.9659258262890683122, 1.000000000000000000, 0.9659258262890683122, 1.000000000000000000, 0.9659258262890683122, 1.000000000000000000, 0.9659258262890683122, 1.000000000000000000, 0.9659258262890683122, 1.000000000000000000, 0.9659258262890683122, 1.000000000000000000, 0.9659258262890683122, 1.000000000000000000, 0.9659258262890683122, 1.000000000000000000, 0.9659258262890683122, 1.000000000000000000, 0.9659258262890683122, 1.000000000000000000, 0.9659258262890683122, 1.000000000000000000, 0.9659258262890683122, 1.000000000000000000, 0.9659258262890683122, 1.000000000000000000, 0.9659258262890683122, 1.000000000000000000, 0.9659258262890683122, 1.000000000000000000, 0.9659258262890683122, 1.000000000000000000, 0.9659258262890683122, 1.000000000000000000, 0.9659258262890683122, 1.000000000000000000, 0.9659258262890683122, 1.000000000000000000, 0.9659258262890683122, 1.000000000000000000, 0.9659258262890683122, 1.000000000000000000, 0.9659258262890683122, 1.000000000000000000, 0.9659258262890683122, 1.000000000000000000, 0.9659258262890683122, 1.000000000000000000, 0.9659258262890683122, 1.000000000000000000, 0.9659258262890683122, 1.000000000000000000, 0.9659258262890683122, 1.000000000000000000, 0.9659258262890683122, 1.000000000000000000, 0.9659258262890683122, 1.000000000000000000, 0.9659258262890683122, 1.000000000000000000, 0.9659258262890683122, 1.000000000000000000, 0.9659258262890683122, 1.000000000000000000, 0.9659258262890683122, 1.000000000000000000, 0.9659258262890683122, 1.000000000000000000, 0.9659258262890683122, 1.000000000000000000, 0.9659258262890683122, 1.000000000000000000, 0.9659258262890683122, 1.000000000000000000, 0.9659258262890683122, 1.000000000000000000, 0.9659258262890683122, 1.000000000000000000, 0.9659258262890683122, 1.000000000000000000, 0.9659258262890683122, 1.000000000000000000, 0.9659258262890683122, 1.000000000000000000, 0.9659258262890683122, 1.000000000000000000, 0.9659258262890683122, 1.000000000000000000, 0.9659258262890683122, 1.000000000000000000, 0.9659258262890683122, 1.000000000000000000, 0.9659258262890683122, 1.000000000000000000, 0.9659258262890683122, 1.000000000000000000, 0.9659258262890683122, 1.000000000000000000, 0.9659258262890683122, 1.000000000000000000, 0.9659258262890683122, 1.000000000000000000, 0.9659258262890683122, 1.000000000000000000, 0.9659258262890683122, 1.000000000000000000, 0.9659258262890683122, 1.000000000000000000, 0.9659258262890683122, 1.000000000000000000, 0.9659258262890683122, 1.000000000000000000, 0.9659258262890683122, 1.000000000000000000, 0.9659258262890683122, 1.000000000000000000, 0.9659258262890683122, 1.000000000000000000, 0.9659258262890683122, 1.000000000000000000, 0.9659258262890683122, 1.000000000000000000, 0.9659258262890683122, 1.000000000000000000, 0.9659258262890683122, 1.000000000000000000, 0.9659258262890683122, 1.000000000000000000, 0.9659258262890683122, 1.000000000000000000, 0.9659258262890683122, 1.000000000000000000, 0.9659258262890683122, 1.000000000000000000, 0.9659258262890683122, 1.000000000000000000, 0.9659258262890683122, 1.000000000000000000, 0.9659258262890683122, 1.000000000000000000, 0.9659258262890683122, 1.000000000000000000, 0.9659258262890683122, 1.000000000000000000, 0.9659258262890683122, 1.000000000000000000, 0.9659258262890683122, 1.000000000000000000, 0.9659258262890683122, 1.000000000000000000, 0.9659258262890683122, 1.000000000000000000, 0.9659258262890683122, 1.000000000000000000, 0.9659258262890683122, 1.000000000000000000, 0.9659258262890683122, 1.000000000000000000, 0.9659258262890683122, 1.000000000000000000, 0.9659258262890683122, 1.000000000000000000, 0.9659258262890683122, 1.000000000000000000, 0.9659258262890683122, 1.000000000000000000, 0.9659258262890683122, 1.000000000000000000, 0.9659258262890683122, 1.000000000000000000, 0.9659258262890683122, 1.000000000000000000, 0.9659258262890683122, 1.000000000000000000, 0.9659258262890683122, 1.000000000000000000, 0.9659258262890683122, 1.000000000000000000, 0.9659258262890683122, 1.000000000000000000, 0.9659258262890683122, 1.000000000000000000, 0.9659258262890683122, 1.000000000000000000, 0.9659258262890683122, 1.000000000000000000, 0.9659258262890683122, 1.000000000000000000, 0.9659258262890683122, 1.000000000000000000, 0.9659258262890683122, 1.000000000000000000, 0.9659258262890683122, 1.000000000000000000, 0.9659258262890683122, 1.000000000000000000, 0.9659258262890683122, 1.000000000000000000, 0.9659258262890683122, 1.000000000000000000, 0.9659258262890683122, 1.000000000000000000, 0.9659258262890683122, 1.000000000000000000, 0.9659258262890683122, 1.000000000000000000, 0.9659258262890683122, 1.000000000000000000, 0.9659258262890683122, 1.000000000000000000, 0.9659258262890683122, 1.000000000000000000, 0.9659258262890683122, 1.000000000000000000, 0.9659258262890683122, 1.000000000000000000, 0.9659258262890683122, 1.000000000000000000, 0.9659258262890683122, 1.000000000000000000, 0.9659258262890683122, 1.000000000000000000, 0.9659258262890683122, 1.000000000000000000, 0.9659258262890683122, 1.000000000000000000, 0.9659258262890683122, 1.000000000000000000, 0.9659258262890683122, 1.000000000000000000, 0.9659258262890683122, 1.000000000000000000, 0.9659258262890683122, 1.000000000000000000, 0.9659258262890683122, 1.000000000000000000, 0.9659258262890683122, 1.000000000000000000, 0.9659258262890683122, 1.000000000000000000, 0.9659258262890683122, 1.000000000000000000, 0.9659258262890683122, 1.000000000000000000, 0.9659258262890683122, 1.000000000000000000, 0.9659258262890683122, 1.000000000000000000, 0.9659258262890683122, 1.000000000000000000, 0.9659258262890683122, 1.000000000000000000, 0.9659258262890683122, 1.000000000000000000, 0.9659258262890683122, 1.000000000000000000, 0.9659258262890683122, 1.000000000000000000, 0.9659258262890683122, 1.000000000000000000, 0.9659258262890683122, 1.000000000000000000, 0.9659258262890683122, 1.000000000000000000, 0.9659258262890683122, 1.000000000000000000, 0.9659258262890683122, 1.000000000000000000, 0.9659258262890683122, 1.000000000000000000, 0.9659258262890683122, 1.000000000000000000, 0.9659258262890683122, 1.000000000000000000, 0.9659258262890683122, 1.000000000000000000, 0.9659258262890683122, 1.000000000000000000, 0.9659258262890683122, 1.000000000000000000, 0.9659258262890683122, 1.000000000000000000, 0.9659258262890683122, 1.000000000000000000, 0.9659258262890683122, 1.000000000000000000, 0.9659258262890683122, 1.000000000000000000, 0.9659258262890683122, 1.000000000000000000, 0.9659258262890683122, 1.000000000000000000, 0.9659258262890683122, 1.000000000000000000, 0.9659258262890683122, 1.000000000000000000, 0.9659258262890683122, 1.000000000000000000, 0.9659258262890683122, 1.000000000000000000, 0.9659258262890683122, 1.000000000000000000, 0.9659258262890683122, 1.000000000000000000, 0.9659258262890683122, 1.000000000000000000, 0.9659258262890683122, 1.000000000000000000, 0.9659258262890683122, 1.000000000000000000, 0.9659258262890683122, 1.000000000000000000, 0.9659258262890683122, 1.000000000000000000, 0.9659258262890683122, 1.000000000000000000, 0.9659258262890683122, 1.000000000000000000, 0.9659258262890683122, 1.000000000000000000, 0.9659258262890683122, 1.000000000000000000, 0.9659258262890683122, 1.000000000000000000, 0.9659258262890683122, 1.000000000000000000, 0.9659258262890683122, 1.000000000000000000, 0.9659258262890683122, 1.000000000000000000, 0.9659258262890683122, 1.000000000000000000, 0.9659258262890683122, 1.000000000000000000, 0.9659258262890683122, 1.000000000000000000, 0.9659258262890683122, 1.000000000000000000, 0.9659258262890683122, 1.000000000000000000, 0.9659258262890683122, 1.000000000000000000, 0.9659258262890683122, 1.000000000000000000, 0.9659258262890683122, 1.000000000000000000, 0.9659258262890683122, 1.000000000000000000, 0.9659258262890683122, 1.000000000000000000, 0.9659258262890683122, 1.000000000000000000, 0.9659258262890683122, 1.000000000000000000, 0.9659258262890683122, 1.000000000000000000, 0.9659258262890683122, 1.000000000000000000, 0.9659258262890683122, 1.000000000000000000, 0.9659258262890683122, 1.000000000000000000, 0.9659258262890683122, 1.000000000000000000, 0.9659258262890683122, 1.000000000000000000, 0.9659258262890683122, 1.000000000000000000, 0.9659258262890683122, 1.000000000000000000, 0.9659258262890683122, 1.000000000000000000, 0.9659258262890683122, 1.000000000000000000, 0.9659258262890683122, 1.000000000000000000, 0.9659258262890683122, 1.000000000000000000, 0.9659258262890683122, 1.000000000000000000, 0.9659258262890683122, 1.000000000000000000, 0.9659258262890683122, 1.000000000000000000, 0.9659258262890683122, 1.000000000000000000, 0.9659258262890683122, 1.000000000000000000, 0.9659258262890683122, 1.000000000000000000, 0.9659258262890683122, 1.000000000000000000, 0.9659258262890683122, 1.000000000000000000, 0.9659258262890683122, 1.000000000000000000, 0.9659258262890683122, 1.000000000000000000, 0.9659258262890683122, 1.000000000000000000, 0.9659258262890683122, 1.000000000000000000, 0.9659258262890683122, 1.000000000000000000, 0.9659258262890683122, 1.000000000000000000, 0.9659258262890683122, 1.000000000000000000),
 ( 0.3333333333333333703, 0.3219752754296894559, 0.3333333333333333703, 0.3219752754296894559, 0.3333333333333333703, 0.3219752754296894559, 0.3333333333333333703, 0.3219752754296894559, 0.3333333333333333703, 0.3219752754296894559, 0.3333333333333333703, 0.3219752754296894559, 0.3333333333333333703, 0.3219752754296894559, 0.3333333333333333703, 0.3219752754296894559, 0.3333333333333333703, 0.3219752754296894559, 0.3333333333333333703, 0.3219752754296894559, 0.3333333333333333703, 0.3219752754296894559, 0.3333333333333333703, 0.3219752754296894559, 0.3333333333333333703, 0.3219752754296894559, 0.3333333333333333703, 0.3219752754296894559, 0.3333333333333333703, 0.3219752754296894559, 0.3333333333333333703, 0.3219752754296894559, 0.3333333333333333703, 0.3219752754296894559, 0.3333333333333333703, 0.3219752754296894559, 0.3333333333333333703, 0.3219752754296894559, 0.3333333333333333703, 0.3219752754296894559, 0.3333333333333333703, 0.3219752754296894559, 0.3333333333333333703, 0.3219752754296894559, 0.3333333333333333703, 0.3219752754296894559, 0.3333333333333333703, 0.3219752754296894559, 0.3333333333333333703, 0.3219752754296894559, 0.3333333333333333703, 0.3219752754296894559, 0.3333333333333333703, 0.3219752754296894559, 0.3333333333333333703, 0.3219752754296894559, 0.3333333333333333703, 0.3219752754296894559, 0.3333333333333333703, 0.3219752754296894559, 0.3333333333333333703, 0.3219752754296894559, 0.3333333333333333703, 0.3219752754296894559, 0.3333333333333333703, 0.3219752754296894559, 0.3333333333333333703, 0.3219752754296894559, 0.3333333333333333703, 0.3219752754296894559, 0.3333333333333333703, 0.3219752754296894559, 0.3333333333333333703, 0.3219752754296894559, 0.3333333333333333703, 0.3219752754296894559, 0.3333333333333333703, 0.3219752754296894559, 0.3333333333333333703, 0.3219752754296894559, 0.3333333333333333703, 0.3219752754296894559, 0.3333333333333333703, 0.3219752754296894559, 0.3333333333333333703, 0.3219752754296894559, 0.3333333333333333703, 0.3219752754296894559, 0.3333333333333333703, 0.3219752754296894559, 0.3333333333333333703, 0.3219752754296894559, 0.3333333333333333703, 0.3219752754296894559, 0.3333333333333333703, 0.3219752754296894559, 0.3333333333333333703, 0.3219752754296894559, 0.3333333333333333703, 0.3219752754296894559, 0.3333333333333333703, 0.3219752754296894559, 0.3333333333333333703, 0.3219752754296894559, 0.3333333333333333703, 0.3219752754296894559, 0.3333333333333333703, 0.3219752754296894559, 0.3333333333333333703, 0.3219752754296894559, 0.3333333333333333703, 0.3219752754296894559, 0.3333333333333333703, 0.3219752754296894559, 0.3333333333333333703, 0.3219752754296894559, 0.3333333333333333703, 0.3219752754296894559, 0.3333333333333333703, 0.3219752754296894559, 0.3333333333333333703, 0.3219752754296894559, 0.3333333333333333703, 0.3219752754296894559, 0.3333333333333333703, 0.3219752754296894559, 0.3333333333333333703, 0.3219752754296894559, 0.3333333333333333703, 0.3219752754296894559, 0.3333333333333333703, 0.3219752754296894559, 0.3333333333333333703, 0.3219752754296894559, 0.3333333333333333703, 0.3219752754296894559, 0.3333333333333333703, 0.3219752754296894559, 0.3333333333333333703, 0.3219752754296894559, 0.3333333333333333703, 0.3219752754296894559, 0.3333333333333333703, 0.3219752754296894559, 0.3333333333333333703, 0.3219752754296894559, 0.3333333333333333703, 0.3219752754296894559, 0.3333333333333333703, 0.3219752754296894559, 0.3333333333333333703, 0.3219752754296894559, 0.3333333333333333703, 0.3219752754296894559, 0.3333333333333333703, 0.3219752754296894559, 0.3333333333333333703, 0.3219752754296894559, 0.3333333333333333703, 0.3219752754296894559, 0.3333333333333333703, 0.3219752754296894559, 0.3333333333333333703, 0.3219752754296894559, 0.3333333333333333703, 0.3219752754296894559, 0.3333333333333333703, 0.3219752754296894559, 0.3333333333333333703, 0.3219752754296894559, 0.3333333333333333703, 0.3219752754296894559, 0.3333333333333333703, 0.3219752754296894559, 0.3333333333333333703, 0.3219752754296894559, 0.3333333333333333703, 0.3219752754296894559, 0.3333333333333333703, 0.3219752754296894559, 0.3333333333333333703, 0.3219752754296894559, 0.3333333333333333703, 0.3219752754296894559, 0.3333333333333333703, 0.3219752754296894559, 0.3333333333333333703, 0.3219752754296894559, 0.3333333333333333703, 0.3219752754296894559, 0.3333333333333333703, 0.3219752754296894559, 0.3333333333333333703, 0.3219752754296894559, 0.3333333333333333703, 0.3219752754296894559, 0.3333333333333333703, 0.3219752754296894559, 0.3333333333333333703, 0.3219752754296894559, 0.3333333333333333703, 0.3219752754296894559, 0.3333333333333333703, 0.3219752754296894559, 0.3333333333333333703, 0.3219752754296894559, 0.3333333333333333703, 0.3219752754296894559, 0.3333333333333333703, 0.3219752754296894559, 0.3333333333333333703, 0.3219752754296894559, 0.3333333333333333703, 0.3219752754296894559, 0.3333333333333333703, 0.3219752754296894559, 0.3333333333333333703, 0.3219752754296894559, 0.3333333333333333703, 0.3219752754296894559, 0.3333333333333333703, 0.3219752754296894559, 0.3333333333333333703, 0.3219752754296894559, 0.3333333333333333703, 0.3219752754296894559, 0.3333333333333333703, 0.3219752754296894559, 0.3333333333333333703, 0.3219752754296894559, 0.3333333333333333703, 0.3219752754296894559, 0.3333333333333333703, 0.3219752754296894559, 0.3333333333333333703, 0.3219752754296894559, 0.3333333333333333703, 0.3219752754296894559, 0.3333333333333333703, 0.3219752754296894559, 0.3333333333333333703, 0.3219752754296894559, 0.3333333333333333703, 0.3219752754296894559, 0.3333333333333333703, 0.3219752754296894559, 0.3333333333333333703, 0.3219752754296894559, 0.3333333333333333703, 0.3219752754296894559, 0.3333333333333333703, 0.3219752754296894559, 0.3333333333333333703, 0.3219752754296894559, 0.3333333333333333703, 0.3219752754296894559, 0.3333333333333333703, 0.3219752754296894559, 0.3333333333333333703, 0.3219752754296894559, 0.3333333333333333703, 0.3219752754296894559, 0.3333333333333333703, 0.3219752754296894559, 0.3333333333333333703, 0.3219752754296894559, 0.3333333333333333703, 0.3219752754296894559, 0.3333333333333333703, 0.3219752754296894559, 0.3333333333333333703, 0.3219752754296894559, 0.3333333333333333703, 0.3219752754296894559, 0.3333333333333333703, 0.3219752754296894559, 0.3333333333333333703, 0.3219752754296894559, 0.3333333333333333703, 0.3219752754296894559, 0.3333333333333333703, 0.3219752754296894559, 0.3333333333333333703, 0.3219752754296894559, 0.3333333333333333703, 0.3219752754296894559, 0.3333333333333333703, 0.3219752754296894559, 0.3333333333333333703, 0.3219752754296894559, 0.3333333333333333703, 0.3219752754296894559, 0.3333333333333333703, 0.3219752754296894559, 0.3333333333333333703, 0.3219752754296894559, 0.3333333333333333703, 0.3219752754296894559, 0.3333333333333333703, 0.3219752754296894559, 0.3333333333333333703, 0.3219752754296894559, 0.3333333333333333703, 0.3219752754296894559, 0.3333333333333333703, 0.3219752754296894559, 0.3333333333333333703, 0.3219752754296894559, 0.3333333333333333703, 0.3219752754296894559, 0.3333333333333333703, 0.3219752754296894559, 0.3333333333333333703, 0.3219752754296894559, 0.3333333333333333703, 0.3219752754296894559, 0.3333333333333333703, 0.3219752754296894559, 0.3333333333333333703, 0.3219752754296894559, 0.3333333333333333703, 0.3219752754296894559, 0.3333333333333333703, 0.3219752754296894559, 0.3333333333333333703, 0.3219752754296894559, 0.3333333333333333703, 0.3219752754296894559, 0.3333333333333333703, 0.3219752754296894559, 0.3333333333333333703, 0.3219752754296894559, 0.3333333333333333703, 0.3219752754296894559, 0.3333333333333333703, 0.3219752754296894559, 0.3333333333333333703, 0.3219752754296894559, 0.3333333333333333703, 0.3219752754296894559, 0.3333333333333333703, 0.3219752754296894559, 0.3333333333333333703, 0.3219752754296894559, 0.3333333333333333703, 0.3219752754296894559, 0.3333333333333333703, 0.3219752754296894559, 0.3333333333333333703, 0.3219752754296894559, 0.3333333333333333703, 0.3219752754296894559, 0.3333333333333333703, 0.3219752754296894559, 0.3333333333333333703, 0.3219752754296894559, 0.3333333333333333703, 0.3219752754296894559, 0.3333333333333333703, 0.3219752754296894559, 0.3333333333333333703, 0.3219752754296894559, 0.3333333333333333703, 0.3219752754296894559, 0.3333333333333333703, 0.3219752754296894559, 0.3333333333333333703, 0.3219752754296894559, 0.3333333333333333703, 0.3219752754296894559, 0.3333333333333333703, 0.3219752754296894559, 0.3333333333333333703, 0.3219752754296894559, 0.3333333333333333703, 0.3219752754296894559, 0.3333333333333333703, 0.3219752754296894559, 0.3333333333333333703, 0.3219752754296894559, 0.3333333333333333703, 0.3219752754296894559, 0.3333333333333333703, 0.3219752754296894559, 0.3333333333333333703, 0.3219752754296894559, 0.3333333333333333703, 0.3219752754296894559, 0.3333333333333333703, 0.3219752754296894559, 0.3333333333333333703, 0.3219752754296894559, 0.3333333333333333703, 0.3219752754296894559, 0.3333333333333333703, 0.3219752754296894559, 0.3333333333333333703, 0.3219752754296894559, 0.3333333333333333703, 0.3219752754296894559, 0.3333333333333333703, 0.3219752754296894559, 0.3333333333333333703, 0.3219752754296894559, 0.3333333333333333703, 0.3219752754296894559, 0.3333333333333333703, 0.3219752754296894559, 0.3333333333333333703, 0.3219752754296894559, 0.3333333333333333703, 0.3219752754296894559, 0.3333333333333333703, 0.3219752754296894559, 0.3333333333333333703, 0.3219752754296894559, 0.3333333333333333703, 0.3219752754296894559, 0.3333333333333333703, 0.3219752754296894559, 0.3333333333333333703, 0.3219752754296894559, 0.3333333333333333703, 0.3219752754296894559, 0.3333333333333333703, 0.3219752754296894559, 0.3333333333333333703, 0.3219752754296894559, 0.3333333333333333703, 0.3219752754296894559, 0.3333333333333333703, 0.3219752754296894559, 0.3333333333333333703, 0.3219752754296894559, 0.3333333333333333703, 0.3219752754296894559, 0.3333333333333333703, 0.3219752754296894559, 0.3333333333333333703, 0.3219752754296894559, 0.3333333333333333703, 0.3219752754296894559, 0.3333333333333333703, 0.3219752754296894559, 0.3333333333333333703, 0.3219752754296894559, 0.3333333333333333703, 0.3219752754296894559, 0.3333333333333333703, 0.3219752754296894559, 0.3333333333333333703, 0.3219752754296894559, 0.3333333333333333703, 0.3219752754296894559, 0.3333333333333333703, 0.3219752754296894559, 0.3333333333333333703),
 ( 0.3333333333333333703, 0.3219752754296894559, 0.3333333333333333703, 0.3219752754296894559, 0.3333333333333333703, 0.3219752754296894559, 0.3333333333333333703, 0.3219752754296894559, 0.3333333333333333703, 0.3219752754296894559, 0.3333333333333333703, 0.3219752754296894559, 0.3333333333333333703, 0.3219752754296894559, 0.3333333333333333703, 0.3219752754296894559, 0.3333333333333333703, 0.3219752754296894559, 0.3333333333333333703, 0.3219752754296894559, 0.3333333333333333703, 0.3219752754296894559, 0.3333333333333333703, 0.3219752754296894559, 0.3333333333333333703, 0.3219752754296894559, 0.3333333333333333703, 0.3219752754296894559, 0.3333333333333333703, 0.3219752754296894559, 0.3333333333333333703, 0.3219752754296894559, 0.3333333333333333703, 0.3219752754296894559, 0.3333333333333333703, 0.3219752754296894559, 0.3333333333333333703, 0.3219752754296894559, 0.3333333333333333703, 0.3219752754296894559, 0.3333333333333333703, 0.3219752754296894559, 0.3333333333333333703, 0.3219752754296894559, 0.3333333333333333703, 0.3219752754296894559, 0.3333333333333333703, 0.3219752754296894559, 0.3333333333333333703, 0.3219752754296894559, 0.3333333333333333703, 0.3219752754296894559, 0.3333333333333333703, 0.3219752754296894559, 0.3333333333333333703, 0.3219752754296894559, 0.3333333333333333703, 0.3219752754296894559, 0.3333333333333333703, 0.3219752754296894559, 0.3333333333333333703, 0.3219752754296894559, 0.3333333333333333703, 0.3219752754296894559, 0.3333333333333333703, 0.3219752754296894559, 0.3333333333333333703, 0.3219752754296894559, 0.3333333333333333703, 0.3219752754296894559, 0.3333333333333333703, 0.3219752754296894559, 0.3333333333333333703, 0.3219752754296894559, 0.3333333333333333703, 0.3219752754296894559, 0.3333333333333333703, 0.3219752754296894559, 0.3333333333333333703, 0.3219752754296894559, 0.3333333333333333703, 0.3219752754296894559, 0.3333333333333333703, 0.3219752754296894559, 0.3333333333333333703, 0.3219752754296894559, 0.3333333333333333703, 0.3219752754296894559, 0.3333333333333333703, 0.3219752754296894559, 0.3333333333333333703, 0.3219752754296894559, 0.3333333333333333703, 0.3219752754296894559, 0.3333333333333333703, 0.3219752754296894559, 0.3333333333333333703, 0.3219752754296894559, 0.3333333333333333703, 0.3219752754296894559, 0.3333333333333333703, 0.3219752754296894559, 0.3333333333333333703, 0.3219752754296894559, 0.3333333333333333703, 0.3219752754296894559, 0.3333333333333333703, 0.3219752754296894559, 0.3333333333333333703, 0.3219752754296894559, 0.3333333333333333703, 0.3219752754296894559, 0.3333333333333333703, 0.3219752754296894559, 0.3333333333333333703, 0.3219752754296894559, 0.3333333333333333703, 0.3219752754296894559, 0.3333333333333333703, 0.3219752754296894559, 0.3333333333333333703, 0.3219752754296894559, 0.3333333333333333703, 0.3219752754296894559, 0.3333333333333333703, 0.3219752754296894559, 0.3333333333333333703, 0.3219752754296894559, 0.3333333333333333703, 0.3219752754296894559, 0.3333333333333333703, 0.3219752754296894559, 0.3333333333333333703, 0.3219752754296894559, 0.3333333333333333703, 0.3219752754296894559, 0.3333333333333333703, 0.3219752754296894559, 0.3333333333333333703, 0.3219752754296894559, 0.3333333333333333703, 0.3219752754296894559, 0.3333333333333333703, 0.3219752754296894559, 0.3333333333333333703, 0.3219752754296894559, 0.3333333333333333703, 0.3219752754296894559, 0.3333333333333333703, 0.3219752754296894559, 0.3333333333333333703, 0.3219752754296894559, 0.3333333333333333703, 0.3219752754296894559, 0.3333333333333333703, 0.3219752754296894559, 0.3333333333333333703, 0.3219752754296894559, 0.3333333333333333703, 0.3219752754296894559, 0.3333333333333333703, 0.3219752754296894559, 0.3333333333333333703, 0.3219752754296894559, 0.3333333333333333703, 0.3219752754296894559, 0.3333333333333333703, 0.3219752754296894559, 0.3333333333333333703, 0.3219752754296894559, 0.3333333333333333703, 0.3219752754296894559, 0.3333333333333333703, 0.3219752754296894559, 0.3333333333333333703, 0.3219752754296894559, 0.3333333333333333703, 0.3219752754296894559, 0.3333333333333333703, 0.3219752754296894559, 0.3333333333333333703, 0.3219752754296894559, 0.3333333333333333703, 0.3219752754296894559, 0.3333333333333333703, 0.3219752754296894559, 0.3333333333333333703, 0.3219752754296894559, 0.3333333333333333703, 0.3219752754296894559, 0.3333333333333333703, 0.3219752754296894559, 0.3333333333333333703, 0.3219752754296894559, 0.3333333333333333703, 0.3219752754296894559, 0.3333333333333333703, 0.3219752754296894559, 0.3333333333333333703, 0.3219752754296894559, 0.3333333333333333703, 0.3219752754296894559, 0.3333333333333333703, 0.3219752754296894559, 0.3333333333333333703, 0.3219752754296894559, 0.3333333333333333703, 0.3219752754296894559, 0.3333333333333333703, 0.3219752754296894559, 0.3333333333333333703, 0.3219752754296894559, 0.3333333333333333703, 0.3219752754296894559, 0.3333333333333333703, 0.3219752754296894559, 0.3333333333333333703, 0.3219752754296894559, 0.3333333333333333703, 0.3219752754296894559, 0.3333333333333333703, 0.3219752754296894559, 0.3333333333333333703, 0.3219752754296894559, 0.3333333333333333703, 0.3219752754296894559, 0.3333333333333333703, 0.3219752754296894559, 0.3333333333333333703, 0.3219752754296894559, 0.3333333333333333703, 0.3219752754296894559, 0.3333333333333333703, 0.3219752754296894559, 0.3333333333333333703, 0.3219752754296894559, 0.3333333333333333703, 0.3219752754296894559, 0.3333333333333333703, 0.3219752754296894559, 0.3333333333333333703, 0.3219752754296894559, 0.3333333333333333703, 0.3219752754296894559, 0.3333333333333333703, 0.3219752754296894559, 0.3333333333333333703, 0.3219752754296894559, 0.3333333333333333703, 0.3219752754296894559, 0.3333333333333333703, 0.3219752754296894559, 0.3333333333333333703, 0.3219752754296894559, 0.3333333333333333703, 0.3219752754296894559, 0.3333333333333333703, 0.3219752754296894559, 0.3333333333333333703, 0.3219752754296894559, 0.3333333333333333703, 0.3219752754296894559, 0.3333333333333333703, 0.3219752754296894559, 0.3333333333333333703, 0.3219752754296894559, 0.3333333333333333703, 0.3219752754296894559, 0.3333333333333333703, 0.3219752754296894559, 0.3333333333333333703, 0.3219752754296894559, 0.3333333333333333703, 0.3219752754296894559, 0.3333333333333333703, 0.3219752754296894559, 0.3333333333333333703, 0.3219752754296894559, 0.3333333333333333703, 0.3219752754296894559, 0.3333333333333333703, 0.3219752754296894559, 0.3333333333333333703, 0.3219752754296894559, 0.3333333333333333703, 0.3219752754296894559, 0.3333333333333333703, 0.3219752754296894559, 0.3333333333333333703, 0.3219752754296894559, 0.3333333333333333703, 0.3219752754296894559, 0.3333333333333333703, 0.3219752754296894559, 0.3333333333333333703, 0.3219752754296894559, 0.3333333333333333703, 0.3219752754296894559, 0.3333333333333333703, 0.3219752754296894559, 0.3333333333333333703, 0.3219752754296894559, 0.3333333333333333703, 0.3219752754296894559, 0.3333333333333333703, 0.3219752754296894559, 0.3333333333333333703, 0.3219752754296894559, 0.3333333333333333703, 0.3219752754296894559, 0.3333333333333333703, 0.3219752754296894559, 0.3333333333333333703, 0.3219752754296894559, 0.3333333333333333703, 0.3219752754296894559, 0.3333333333333333703, 0.3219752754296894559, 0.3333333333333333703, 0.3219752754296894559, 0.3333333333333333703, 0.3219752754296894559, 0.3333333333333333703, 0.3219752754296894559, 0.3333333333333333703, 0.3219752754296894559, 0.3333333333333333703, 0.3219752754296894559, 0.3333333333333333703, 0.3219752754296894559, 0.3333333333333333703, 0.3219752754296894559, 0.3333333333333333703, 0.3219752754296894559, 0.3333333333333333703, 0.3219752754296894559, 0.3333333333333333703, 0.3219752754296894559, 0.3333333333333333703, 0.3219752754296894559, 0.3333333333333333703, 0.3219752754296894559, 0.3333333333333333703, 0.3219752754296894559, 0.3333333333333333703, 0.3219752754296894559, 0.3333333333333333703, 0.3219752754296894559, 0.3333333333333333703, 0.3219752754296894559, 0.3333333333333333703, 0.3219752754296894559, 0.3333333333333333703, 0.3219752754296894559, 0.3333333333333333703, 0.3219752754296894559, 0.3333333333333333703, 0.3219752754296894559, 0.3333333333333333703, 0.3219752754296894559, 0.3333333333333333703, 0.3219752754296894559, 0.3333333333333333703, 0.3219752754296894559, 0.3333333333333333703, 0.3219752754296894559, 0.3333333333333333703, 0.3219752754296894559, 0.3333333333333333703, 0.3219752754296894559, 0.3333333333333333703, 0.3219752754296894559, 0.3333333333333333703, 0.3219752754296894559, 0.3333333333333333703, 0.3219752754296894559, 0.3333333333333333703, 0.3219752754296894559, 0.3333333333333333703, 0.3219752754296894559, 0.3333333333333333703, 0.3219752754296894559, 0.3333333333333333703, 0.3219752754296894559, 0.3333333333333333703, 0.3219752754296894559, 0.3333333333333333703, 0.3219752754296894559, 0.3333333333333333703, 0.3219752754296894559, 0.3333333333333333703, 0.3219752754296894559, 0.3333333333333333703, 0.3219752754296894559, 0.3333333333333333703, 0.3219752754296894559, 0.3333333333333333703, 0.3219752754296894559, 0.3333333333333333703, 0.3219752754296894559, 0.3333333333333333703, 0.3219752754296894559, 0.3333333333333333703, 0.3219752754296894559, 0.3333333333333333703, 0.3219752754296894559, 0.3333333333333333703, 0.3219752754296894559, 0.3333333333333333703, 0.3219752754296894559, 0.3333333333333333703, 0.3219752754296894559, 0.3333333333333333703, 0.3219752754296894559, 0.3333333333333333703, 0.3219752754296894559, 0.3333333333333333703, 0.3219752754296894559, 0.3333333333333333703, 0.3219752754296894559, 0.3333333333333333703, 0.3219752754296894559, 0.3333333333333333703, 0.3219752754296894559, 0.3333333333333333703, 0.3219752754296894559, 0.3333333333333333703, 0.3219752754296894559, 0.3333333333333333703, 0.3219752754296894559, 0.3333333333333333703, 0.3219752754296894559, 0.3333333333333333703, 0.3219752754296894559, 0.3333333333333333703, 0.3219752754296894559, 0.3333333333333333703, 0.3219752754296894559, 0.3333333333333333703, 0.3219752754296894559, 0.3333333333333333703, 0.3219752754296894559, 0.3333333333333333703, 0.3219752754296894559, 0.3333333333333333703, 0.3219752754296894559, 0.3333333333333333703, 0.3219752754296894559, 0.3333333333333333703, 0.3219752754296894559, 0.3333333333333333703, 0.3219752754296894559, 0.3333333333333333703, 0.3219752754296894559, 0.3333333333333333703, 0.3219752754296894559, 0.3333333333333333703),
 ( 1.000000000000000000, 0.9659258262890683122, 1.000000000000000000, 0.9659258262890683122, 1.000000000000000000, 0.9659258262890683122, 1.000000000000000000, 0.9659258262890683122, 1.000000000000000000, 0.9659258262890683122, 1.000000000000000000, 0.9659258262890683122, 1.000000000000000000, 0.9659258262890683122, 1.000000000000000000, 0.9659258262890683122, 1.000000000000000000, 0.9659258262890683122, 1.000000000000000000, 0.9659258262890683122, 1.000000000000000000, 0.9659258262890683122, 1.000000000000000000, 0.9659258262890683122, 1.000000000000000000, 0.9659258262890683122, 1.000000000000000000, 0.9659258262890683122, 1.000000000000000000, 0.9659258262890683122, 1.000000000000000000, 0.9659258262890683122, 1.000000000000000000, 0.9659258262890683122, 1.000000000000000000, 0.9659258262890683122, 1.000000000000000000, 0.9659258262890683122, 1.000000000000000000, 0.9659258262890683122, 1.000000000000000000, 0.9659258262890683122, 1.000000000000000000, 0.9659258262890683122, 1.000000000000000000, 0.9659258262890683122, 1.000000000000000000, 0.9659258262890683122, 1.000000000000000000, 0.9659258262890683122, 1.000000000000000000, 0.9659258262890683122, 1.000000000000000000, 0.9659258262890683122, 1.000000000000000000, 0.9659258262890683122, 1.000000000000000000, 0.9659258262890683122, 1.000000000000000000, 0.9659258262890683122, 1.000000000000000000, 0.9659258262890683122, 1.000000000000000000, 0.9659258262890683122, 1.000000000000000000, 0.9659258262890683122, 1.000000000000000000, 0.9659258262890683122, 1.000000000000000000, 0.9659258262890683122, 1.000000000000000000, 0.9659258262890683122, 1.000000000000000000, 0.9659258262890683122, 1.000000000000000000, 0.9659258262890683122, 1.000000000000000000, 0.9659258262890683122, 1.000000000000000000, 0.9659258262890683122, 1.000000000000000000, 0.9659258262890683122, 1.000000000000000000, 0.9659258262890683122, 1.000000000000000000, 0.9659258262890683122, 1.000000000000000000, 0.9659258262890683122, 1.000000000000000000, 0.9659258262890683122, 1.000000000000000000, 0.9659258262890683122, 1.000000000000000000, 0.9659258262890683122, 1.000000000000000000, 0.9659258262890683122, 1.000000000000000000, 0.9659258262890683122, 1.000000000000000000, 0.9659258262890683122, 1.000000000000000000, 0.9659258262890683122, 1.000000000000000000, 0.9659258262890683122, 1.000000000000000000, 0.9659258262890683122, 1.000000000000000000, 0.9659258262890683122, 1.000000000000000000, 0.9659258262890683122, 1.000000000000000000, 0.9659258262890683122, 1.000000000000000000, 0.9659258262890683122, 1.000000000000000000, 0.9659258262890683122, 1.000000000000000000, 0.9659258262890683122, 1.000000000000000000, 0.9659258262890683122, 1.000000000000000000, 0.9659258262890683122, 1.000000000000000000, 0.9659258262890683122, 1.000000000000000000, 0.9659258262890683122, 1.000000000000000000, 0.9659258262890683122, 1.000000000000000000, 0.9659258262890683122, 1.000000000000000000, 0.9659258262890683122, 1.000000000000000000, 0.9659258262890683122, 1.000000000000000000, 0.9659258262890683122, 1.000000000000000000, 0.9659258262890683122, 1.000000000000000000, 0.9659258262890683122, 1.000000000000000000, 0.9659258262890683122, 1.000000000000000000, 0.9659258262890683122, 1.000000000000000000, 0.9659258262890683122, 1.000000000000000000, 0.9659258262890683122, 1.000000000000000000, 0.9659258262890683122, 1.000000000000000000, 0.9659258262890683122, 1.000000000000000000, 0.9659258262890683122, 1.000000000000000000, 0.9659258262890683122, 1.000000000000000000, 0.9659258262890683122, 1.000000000000000000, 0.9659258262890683122, 1.000000000000000000, 0.9659258262890683122, 1.000000000000000000, 0.9659258262890683122, 1.000000000000000000, 0.9659258262890683122, 1.000000000000000000, 0.9659258262890683122, 1.000000000000000000, 0.9659258262890683122, 1.000000000000000000, 0.9659258262890683122, 1.000000000000000000, 0.9659258262890683122, 1.000000000000000000, 0.9659258262890683122, 1.000000000000000000, 0.9659258262890683122, 1.000000000000000000, 0.9659258262890683122, 1.000000000000000000, 0.9659258262890683122, 1.000000000000000000, 0.9659258262890683122, 1.000000000000000000, 0.9659258262890683122, 1.000000000000000000, 0.9659258262890683122, 1.000000000000000000, 0.9659258262890683122, 1.000000000000000000, 0.9659258262890683122, 1.000000000000000000, 0.9659258262890683122, 1.000000000000000000, 0.9659258262890683122, 1.000000000000000000, 0.9659258262890683122, 1.000000000000000000, 0.9659258262890683122, 1.000000000000000000, 0.9659258262890683122, 1.000000000000000000, 0.9659258262890683122, 1.000000000000000000, 0.9659258262890683122, 1.000000000000000000, 0.9659258262890683122, 1.000000000000000000, 0.9659258262890683122, 1.000000000000000000, 0.9659258262890683122, 1.000000000000000000, 0.9659258262890683122, 1.000000000000000000, 0.9659258262890683122, 1.000000000000000000, 0.9659258262890683122, 1.000000000000000000, 0.9659258262890683122, 1.000000000000000000, 0.9659258262890683122, 1.000000000000000000, 0.9659258262890683122, 1.000000000000000000, 0.9659258262890683122, 1.000000000000000000, 0.9659258262890683122, 1.000000000000000000, 0.9659258262890683122, 1.000000000000000000, 0.9659258262890683122, 1.000000000000000000, 0.9659258262890683122, 1.000000000000000000, 0.9659258262890683122, 1.000000000000000000, 0.9659258262890683122, 1.000000000000000000, 0.9659258262890683122, 1.000000000000000000, 0.9659258262890683122, 1.000000000000000000, 0.9659258262890683122, 1.000000000000000000, 0.9659258262890683122, 1.000000000000000000, 0.9659258262890683122, 1.000000000000000000, 0.9659258262890683122, 1.000000000000000000, 0.9659258262890683122, 1.000000000000000000, 0.9659258262890683122, 1.000000000000000000, 0.9659258262890683122, 1.000000000000000000, 0.9659258262890683122, 1.000000000000000000, 0.9659258262890683122, 1.000000000000000000, 0.9659258262890683122, 1.000000000000000000, 0.9659258262890683122, 1.000000000000000000, 0.9659258262890683122, 1.000000000000000000, 0.9659258262890683122, 1.000000000000000000, 0.9659258262890683122, 1.000000000000000000, 0.9659258262890683122, 1.000000000000000000, 0.9659258262890683122, 1.000000000000000000, 0.9659258262890683122, 1.000000000000000000, 0.9659258262890683122, 1.000000000000000000, 0.9659258262890683122, 1.000000000000000000, 0.9659258262890683122, 1.000000000000000000, 0.9659258262890683122, 1.000000000000000000, 0.9659258262890683122, 1.000000000000000000, 0.9659258262890683122, 1.000000000000000000, 0.9659258262890683122, 1.000000000000000000, 0.9659258262890683122, 1.000000000000000000, 0.9659258262890683122, 1.000000000000000000, 0.9659258262890683122, 1.000000000000000000, 0.9659258262890683122, 1.000000000000000000, 0.9659258262890683122, 1.000000000000000000, 0.9659258262890683122, 1.000000000000000000, 0.9659258262890683122, 1.000000000000000000, 0.9659258262890683122, 1.000000000000000000, 0.9659258262890683122, 1.000000000000000000, 0.9659258262890683122, 1.000000000000000000, 0.9659258262890683122, 1.000000000000000000, 0.9659258262890683122, 1.000000000000000000, 0.9659258262890683122, 1.000000000000000000, 0.9659258262890683122, 1.000000000000000000, 0.9659258262890683122, 1.000000000000000000, 0.9659258262890683122, 1.000000000000000000, 0.9659258262890683122, 1.000000000000000000, 0.9659258262890683122, 1.000000000000000000, 0.9659258262890683122, 1.000000000000000000, 0.9659258262890683122, 1.000000000000000000, 0.9659258262890683122, 1.000000000000000000, 0.9659258262890683122, 1.000000000000000000, 0.9659258262890683122, 1.000000000000000000, 0.9659258262890683122, 1.000000000000000000, 0.9659258262890683122, 1.000000000000000000, 0.9659258262890683122, 1.000000000000000000, 0.9659258262890683122, 1.000000000000000000, 0.9659258262890683122, 1.000000000000000000, 0.9659258262890683122, 1.000000000000000000, 0.9659258262890683122, 1.000000000000000000, 0.9659258262890683122, 1.000000000000000000, 0.9659258262890683122, 1.000000000000000000, 0.9659258262890683122, 1.000000000000000000, 0.9659258262890683122, 1.000000000000000000, 0.9659258262890683122, 1.000000000000000000, 0.9659258262890683122, 1.000000000000000000, 0.9659258262890683122, 1.000000000000000000, 0.9659258262890683122, 1.000000000000000000, 0.9659258262890683122, 1.000000000000000000, 0.9659258262890683122, 1.000000000000000000, 0.9659258262890683122, 1.000000000000000000, 0.9659258262890683122, 1.000000000000000000, 0.9659258262890683122, 1.000000000000000000, 0.9659258262890683122, 1.000000000000000000, 0.9659258262890683122, 1.000000000000000000, 0.9659258262890683122, 1.000000000000000000, 0.9659258262890683122, 1.000000000000000000, 0.9659258262890683122, 1.000000000000000000, 0.9659258262890683122, 1.000000000000000000, 0.9659258262890683122, 1.000000000000000000, 0.9659258262890683122, 1.000000000000000000, 0.9659258262890683122, 1.000000000000000000, 0.9659258262890683122, 1.000000000000000000, 0.9659258262890683122, 1.000000000000000000, 0.9659258262890683122, 1.000000000000000000, 0.9659258262890683122, 1.000000000000000000, 0.9659258262890683122, 1.000000000000000000, 0.9659258262890683122, 1.000000000000000000, 0.9659258262890683122, 1.000000000000000000, 0.9659258262890683122, 1.000000000000000000, 0.9659258262890683122, 1.000000000000000000, 0.9659258262890683122, 1.000000000000000000, 0.9659258262890683122, 1.000000000000000000, 0.9659258262890683122, 1.000000000000000000, 0.9659258262890683122, 1.000000000000000000, 0.9659258262890683122, 1.000000000000000000, 0.9659258262890683122, 1.000000000000000000, 0.9659258262890683122, 1.000000000000000000, 0.9659258262890683122, 1.000000000000000000, 0.9659258262890683122, 1.000000000000000000, 0.9659258262890683122, 1.000000000000000000, 0.9659258262890683122, 1.000000000000000000, 0.9659258262890683122, 1.000000000000000000, 0.9659258262890683122, 1.000000000000000000, 0.9659258262890683122, 1.000000000000000000, 0.9659258262890683122, 1.000000000000000000, 0.9659258262890683122, 1.000000000000000000, 0.9659258262890683122, 1.000000000000000000, 0.9659258262890683122, 1.000000000000000000, 0.9659258262890683122, 1.000000000000000000, 0.9659258262890683122, 1.000000000000000000, 0.9659258262890683122, 1.000000000000000000, 0.9659258262890683122, 1.000000000000000000),
 ( 0.3333333333333333703, 0.3219752754296894559, 0.3333333333333333703, 0.3219752754296894559, 0.3333333333333333703, 0.3219752754296894559, 0.3333333333333333703, 0.3219752754296894559, 0.3333333333333333703, 0.3219752754296894559, 0.3333333333333333703, 0.3219752754296894559, 0.3333333333333333703, 0.3219752754296894559, 0.3333333333333333703, 0.3219752754296894559, 0.3333333333333333703, 0.3219752754296894559, 0.3333333333333333703, 0.3219752754296894559, 0.3333333333333333703, 0.3219752754296894559, 0.3333333333333333703, 0.3219752754296894559, 0.3333333333333333703, 0.3219752754296894559, 0.3333333333333333703, 0.3219752754296894559, 0.3333333333333333703, 0.3219752754296894559, 0.3333333333333333703, 0.3219752754296894559, 0.3333333333333333703, 0.3219752754296894559, 0.3333333333333333703, 0.3219752754296894559, 0.3333333333333333703, 0.3219752754296894559, 0.3333333333333333703, 0.3219752754296894559, 0.3333333333333333703, 0.3219752754296894559, 0.3333333333333333703, 0.3219752754296894559, 0.3333333333333333703, 0.3219752754296894559, 0.3333333333333333703, 0.3219752754296894559, 0.3333333333333333703, 0.3219752754296894559, 0.3333333333333333703, 0.3219752754296894559, 0.3333333333333333703, 0.3219752754296894559, 0.3333333333333333703, 0.3219752754296894559, 0.3333333333333333703, 0.3219752754296894559, 0.3333333333333333703, 0.3219752754296894559, 0.3333333333333333703, 0.3219752754296894559, 0.3333333333333333703, 0.3219752754296894559, 0.3333333333333333703, 0.3219752754296894559, 0.3333333333333333703, 0.3219752754296894559, 0.3333333333333333703, 0.3219752754296894559, 0.3333333333333333703, 0.3219752754296894559, 0.3333333333333333703, 0.3219752754296894559, 0.3333333333333333703, 0.3219752754296894559, 0.3333333333333333703, 0.3219752754296894559, 0.3333333333333333703, 0.3219752754296894559, 0.3333333333333333703, 0.3219752754296894559, 0.3333333333333333703, 0.3219752754296894559, 0.3333333333333333703, 0.3219752754296894559, 0.3333333333333333703, 0.3219752754296894559, 0.3333333333333333703, 0.3219752754296894559, 0.3333333333333333703, 0.3219752754296894559, 0.3333333333333333703, 0.3219752754296894559, 0.3333333333333333703, 0.3219752754296894559, 0.3333333333333333703, 0.3219752754296894559, 0.3333333333333333703, 0.3219752754296894559, 0.3333333333333333703, 0.3219752754296894559, 0.3333333333333333703, 0.3219752754296894559, 0.3333333333333333703, 0.3219752754296894559, 0.3333333333333333703, 0.3219752754296894559, 0.3333333333333333703, 0.3219752754296894559, 0.3333333333333333703, 0.3219752754296894559, 0.3333333333333333703, 0.3219752754296894559, 0.3333333333333333703, 0.3219752754296894559, 0.3333333333333333703, 0.3219752754296894559, 0.3333333333333333703, 0.3219752754296894559, 0.3333333333333333703, 0.3219752754296894559, 0.3333333333333333703, 0.3219752754296894559, 0.3333333333333333703, 0.3219752754296894559, 0.3333333333333333703, 0.3219752754296894559, 0.3333333333333333703, 0.3219752754296894559, 0.3333333333333333703, 0.3219752754296894559, 0.3333333333333333703, 0.3219752754296894559, 0.3333333333333333703, 0.3219752754296894559, 0.3333333333333333703, 0.3219752754296894559, 0.3333333333333333703, 0.3219752754296894559, 0.3333333333333333703, 0.3219752754296894559, 0.3333333333333333703, 0.3219752754296894559, 0.3333333333333333703, 0.3219752754296894559, 0.3333333333333333703, 0.3219752754296894559, 0.3333333333333333703, 0.3219752754296894559, 0.3333333333333333703, 0.3219752754296894559, 0.3333333333333333703, 0.3219752754296894559, 0.3333333333333333703, 0.3219752754296894559, 0.3333333333333333703, 0.3219752754296894559, 0.3333333333333333703, 0.3219752754296894559, 0.3333333333333333703, 0.3219752754296894559, 0.3333333333333333703, 0.3219752754296894559, 0.3333333333333333703, 0.3219752754296894559, 0.3333333333333333703, 0.3219752754296894559, 0.3333333333333333703, 0.3219752754296894559, 0.3333333333333333703, 0.3219752754296894559, 0.3333333333333333703, 0.3219752754296894559, 0.3333333333333333703, 0.3219752754296894559, 0.3333333333333333703, 0.3219752754296894559, 0.3333333333333333703, 0.3219752754296894559, 0.3333333333333333703, 0.3219752754296894559, 0.3333333333333333703, 0.3219752754296894559, 0.3333333333333333703, 0.3219752754296894559, 0.3333333333333333703, 0.3219752754296894559, 0.3333333333333333703, 0.3219752754296894559, 0.3333333333333333703, 0.3219752754296894559, 0.3333333333333333703, 0.3219752754296894559, 0.3333333333333333703, 0.3219752754296894559, 0.3333333333333333703, 0.3219752754296894559, 0.3333333333333333703, 0.3219752754296894559, 0.3333333333333333703, 0.3219752754296894559, 0.3333333333333333703, 0.3219752754296894559, 0.3333333333333333703, 0.3219752754296894559, 0.3333333333333333703, 0.3219752754296894559, 0.3333333333333333703, 0.3219752754296894559, 0.3333333333333333703, 0.3219752754296894559, 0.3333333333333333703, 0.3219752754296894559, 0.3333333333333333703, 0.3219752754296894559, 0.3333333333333333703, 0.3219752754296894559, 0.3333333333333333703, 0.3219752754296894559, 0.3333333333333333703, 0.3219752754296894559, 0.3333333333333333703, 0.3219752754296894559, 0.3333333333333333703, 0.3219752754296894559, 0.3333333333333333703, 0.3219752754296894559, 0.3333333333333333703, 0.3219752754296894559, 0.3333333333333333703, 0.3219752754296894559, 0.3333333333333333703, 0.3219752754296894559, 0.3333333333333333703, 0.3219752754296894559, 0.3333333333333333703, 0.3219752754296894559, 0.3333333333333333703, 0.3219752754296894559, 0.3333333333333333703, 0.3219752754296894559, 0.3333333333333333703, 0.3219752754296894559, 0.3333333333333333703, 0.3219752754296894559, 0.3333333333333333703, 0.3219752754296894559, 0.3333333333333333703, 0.3219752754296894559, 0.3333333333333333703, 0.3219752754296894559, 0.3333333333333333703, 0.3219752754296894559, 0.3333333333333333703, 0.3219752754296894559, 0.3333333333333333703, 0.3219752754296894559, 0.3333333333333333703, 0.3219752754296894559, 0.3333333333333333703, 0.3219752754296894559, 0.3333333333333333703, 0.3219752754296894559, 0.3333333333333333703, 0.3219752754296894559, 0.3333333333333333703, 0.3219752754296894559, 0.3333333333333333703, 0.3219752754296894559, 0.3333333333333333703, 0.3219752754296894559, 0.3333333333333333703, 0.3219752754296894559, 0.3333333333333333703, 0.3219752754296894559, 0.3333333333333333703, 0.3219752754296894559, 0.3333333333333333703, 0.3219752754296894559, 0.3333333333333333703, 0.3219752754296894559, 0.3333333333333333703, 0.3219752754296894559, 0.3333333333333333703, 0.3219752754296894559, 0.3333333333333333703, 0.3219752754296894559, 0.3333333333333333703, 0.3219752754296894559, 0.3333333333333333703, 0.3219752754296894559, 0.3333333333333333703, 0.3219752754296894559, 0.3333333333333333703, 0.3219752754296894559, 0.3333333333333333703, 0.3219752754296894559, 0.3333333333333333703, 0.3219752754296894559, 0.3333333333333333703, 0.3219752754296894559, 0.3333333333333333703, 0.3219752754296894559, 0.3333333333333333703, 0.3219752754296894559, 0.3333333333333333703, 0.3219752754296894559, 0.3333333333333333703, 0.3219752754296894559, 0.3333333333333333703, 0.3219752754296894559, 0.3333333333333333703, 0.3219752754296894559, 0.3333333333333333703, 0.3219752754296894559, 0.3333333333333333703, 0.3219752754296894559, 0.3333333333333333703, 0.3219752754296894559, 0.3333333333333333703, 0.3219752754296894559, 0.3333333333333333703, 0.3219752754296894559, 0.3333333333333333703, 0.3219752754296894559, 0.3333333333333333703, 0.3219752754296894559, 0.3333333333333333703, 0.3219752754296894559, 0.3333333333333333703, 0.3219752754296894559, 0.3333333333333333703, 0.3219752754296894559, 0.3333333333333333703, 0.3219752754296894559, 0.3333333333333333703, 0.3219752754296894559, 0.3333333333333333703, 0.3219752754296894559, 0.3333333333333333703, 0.3219752754296894559, 0.3333333333333333703, 0.3219752754296894559, 0.3333333333333333703, 0.3219752754296894559, 0.3333333333333333703, 0.3219752754296894559, 0.3333333333333333703, 0.3219752754296894559, 0.3333333333333333703, 0.3219752754296894559, 0.3333333333333333703, 0.3219752754296894559, 0.3333333333333333703, 0.3219752754296894559, 0.3333333333333333703, 0.3219752754296894559, 0.3333333333333333703, 0.3219752754296894559, 0.3333333333333333703, 0.3219752754296894559, 0.3333333333333333703, 0.3219752754296894559, 0.3333333333333333703, 0.3219752754296894559, 0.3333333333333333703, 0.3219752754296894559, 0.3333333333333333703, 0.3219752754296894559, 0.3333333333333333703, 0.3219752754296894559, 0.3333333333333333703, 0.3219752754296894559, 0.3333333333333333703, 0.3219752754296894559, 0.3333333333333333703, 0.3219752754296894559, 0.3333333333333333703, 0.3219752754296894559, 0.3333333333333333703, 0.3219752754296894559, 0.3333333333333333703, 0.3219752754296894559, 0.3333333333333333703, 0.3219752754296894559, 0.3333333333333333703, 0.3219752754296894559, 0.3333333333333333703, 0.3219752754296894559, 0.3333333333333333703, 0.3219752754296894559, 0.3333333333333333703, 0.3219752754296894559, 0.3333333333333333703, 0.3219752754296894559, 0.3333333333333333703, 0.3219752754296894559, 0.3333333333333333703, 0.3219752754296894559, 0.3333333333333333703, 0.3219752754296894559, 0.3333333333333333703, 0.3219752754296894559, 0.3333333333333333703, 0.3219752754296894559, 0.3333333333333333703, 0.3219752754296894559, 0.3333333333333333703, 0.3219752754296894559, 0.3333333333333333703, 0.3219752754296894559, 0.3333333333333333703, 0.3219752754296894559, 0.3333333333333333703, 0.3219752754296894559, 0.3333333333333333703, 0.3219752754296894559, 0.3333333333333333703, 0.3219752754296894559, 0.3333333333333333703, 0.3219752754296894559, 0.3333333333333333703, 0.3219752754296894559, 0.3333333333333333703, 0.3219752754296894559, 0.3333333333333333703, 0.3219752754296894559, 0.3333333333333333703, 0.3219752754296894559, 0.3333333333333333703, 0.3219752754296894559, 0.3333333333333333703, 0.3219752754296894559, 0.3333333333333333703, 0.3219752754296894559, 0.3333333333333333703, 0.3219752754296894559, 0.3333333333333333703, 0.3219752754296894559, 0.3333333333333333703, 0.3219752754296894559, 0.3333333333333333703, 0.3219752754296894559, 0.3333333333333333703, 0.3219752754296894559, 0.3333333333333333703, 0.3219752754296894559, 0.3333333333333333703, 0.3219752754296894559, 0.3333333333333333703, 0.3219752754296894559, 0.3333333333333333703, 0.3219752754296894559, 0.3333333333333333703, 0.3219752754296894559, 0.3333333333333333703),
 ( 0.3333333333333333703, 0.3219752754296894559, 0.3333333333333333703, 0.3219752754296894559, 0.3333333333333333703, 0.3219752754296894559, 0.3333333333333333703, 0.3219752754296894559, 0.3333333333333333703, 0.3219752754296894559, 0.3333333333333333703, 0.3219752754296894559, 0.3333333333333333703, 0.3219752754296894559, 0.3333333333333333703, 0.3219752754296894559, 0.3333333333333333703, 0.3219752754296894559, 0.3333333333333333703, 0.3219752754296894559, 0.3333333333333333703, 0.3219752754296894559, 0.3333333333333333703, 0.3219752754296894559, 0.3333333333333333703, 0.3219752754296894559, 0.3333333333333333703, 0.3219752754296894559, 0.3333333333333333703, 0.3219752754296894559, 0.3333333333333333703, 0.3219752754296894559, 0.3333333333333333703, 0.3219752754296894559, 0.3333333333333333703, 0.3219752754296894559, 0.3333333333333333703, 0.3219752754296894559, 0.3333333333333333703, 0.3219752754296894559, 0.3333333333333333703, 0.3219752754296894559, 0.3333333333333333703, 0.3219752754296894559, 0.3333333333333333703, 0.3219752754296894559, 0.3333333333333333703, 0.3219752754296894559, 0.3333333333333333703, 0.3219752754296894559, 0.3333333333333333703, 0.3219752754296894559, 0.3333333333333333703, 0.3219752754296894559, 0.3333333333333333703, 0.3219752754296894559, 0.3333333333333333703, 0.3219752754296894559, 0.3333333333333333703, 0.3219752754296894559, 0.3333333333333333703, 0.3219752754296894559, 0.3333333333333333703, 0.3219752754296894559, 0.3333333333333333703, 0.3219752754296894559, 0.3333333333333333703, 0.3219752754296894559, 0.3333333333333333703, 0.3219752754296894559, 0.3333333333333333703, 0.3219752754296894559, 0.3333333333333333703, 0.3219752754296894559, 0.3333333333333333703, 0.3219752754296894559, 0.3333333333333333703, 0.3219752754296894559, 0.3333333333333333703, 0.3219752754296894559, 0.3333333333333333703, 0.3219752754296894559, 0.3333333333333333703, 0.3219752754296894559, 0.3333333333333333703, 0.3219752754296894559, 0.3333333333333333703, 0.3219752754296894559, 0.3333333333333333703, 0.3219752754296894559, 0.3333333333333333703, 0.3219752754296894559, 0.3333333333333333703, 0.3219752754296894559, 0.3333333333333333703, 0.3219752754296894559, 0.3333333333333333703, 0.3219752754296894559, 0.3333333333333333703, 0.3219752754296894559, 0.3333333333333333703, 0.3219752754296894559, 0.3333333333333333703, 0.3219752754296894559, 0.3333333333333333703, 0.3219752754296894559, 0.3333333333333333703, 0.3219752754296894559, 0.3333333333333333703, 0.3219752754296894559, 0.3333333333333333703, 0.3219752754296894559, 0.3333333333333333703, 0.3219752754296894559, 0.3333333333333333703, 0.3219752754296894559, 0.3333333333333333703, 0.3219752754296894559, 0.3333333333333333703, 0.3219752754296894559, 0.3333333333333333703, 0.3219752754296894559, 0.3333333333333333703, 0.3219752754296894559, 0.3333333333333333703, 0.3219752754296894559, 0.3333333333333333703, 0.3219752754296894559, 0.3333333333333333703, 0.3219752754296894559, 0.3333333333333333703, 0.3219752754296894559, 0.3333333333333333703, 0.3219752754296894559, 0.3333333333333333703, 0.3219752754296894559, 0.3333333333333333703, 0.3219752754296894559, 0.3333333333333333703, 0.3219752754296894559, 0.3333333333333333703, 0.3219752754296894559, 0.3333333333333333703, 0.3219752754296894559, 0.3333333333333333703, 0.3219752754296894559, 0.3333333333333333703, 0.3219752754296894559, 0.3333333333333333703, 0.3219752754296894559, 0.3333333333333333703, 0.3219752754296894559, 0.3333333333333333703, 0.3219752754296894559, 0.3333333333333333703, 0.3219752754296894559, 0.3333333333333333703, 0.3219752754296894559, 0.3333333333333333703, 0.3219752754296894559, 0.3333333333333333703, 0.3219752754296894559, 0.3333333333333333703, 0.3219752754296894559, 0.3333333333333333703, 0.3219752754296894559, 0.3333333333333333703, 0.3219752754296894559, 0.3333333333333333703, 0.3219752754296894559, 0.3333333333333333703, 0.3219752754296894559, 0.3333333333333333703, 0.3219752754296894559, 0.3333333333333333703, 0.3219752754296894559, 0.3333333333333333703, 0.3219752754296894559, 0.3333333333333333703, 0.3219752754296894559, 0.3333333333333333703, 0.3219752754296894559, 0.3333333333333333703, 0.3219752754296894559, 0.3333333333333333703, 0.3219752754296894559, 0.3333333333333333703, 0.3219752754296894559, 0.3333333333333333703, 0.3219752754296894559, 0.3333333333333333703, 0.3219752754296894559, 0.3333333333333333703, 0.3219752754296894559, 0.3333333333333333703, 0.3219752754296894559, 0.3333333333333333703, 0.3219752754296894559, 0.3333333333333333703, 0.3219752754296894559, 0.3333333333333333703, 0.3219752754296894559, 0.3333333333333333703, 0.3219752754296894559, 0.3333333333333333703, 0.3219752754296894559, 0.3333333333333333703, 0.3219752754296894559, 0.3333333333333333703, 0.3219752754296894559, 0.3333333333333333703, 0.3219752754296894559, 0.3333333333333333703, 0.3219752754296894559, 0.3333333333333333703, 0.3219752754296894559, 0.3333333333333333703, 0.3219752754296894559, 0.3333333333333333703, 0.3219752754296894559, 0.3333333333333333703, 0.3219752754296894559, 0.3333333333333333703, 0.3219752754296894559, 0.3333333333333333703, 0.3219752754296894559, 0.3333333333333333703, 0.3219752754296894559, 0.3333333333333333703, 0.3219752754296894559, 0.3333333333333333703, 0.3219752754296894559, 0.3333333333333333703, 0.3219752754296894559, 0.3333333333333333703, 0.3219752754296894559, 0.3333333333333333703, 0.3219752754296894559, 0.3333333333333333703, 0.3219752754296894559, 0.3333333333333333703, 0.3219752754296894559, 0.3333333333333333703, 0.3219752754296894559, 0.3333333333333333703, 0.3219752754296894559, 0.3333333333333333703, 0.3219752754296894559, 0.3333333333333333703, 0.3219752754296894559, 0.3333333333333333703, 0.3219752754296894559, 0.3333333333333333703, 0.3219752754296894559, 0.3333333333333333703, 0.3219752754296894559, 0.3333333333333333703, 0.3219752754296894559, 0.3333333333333333703, 0.3219752754296894559, 0.3333333333333333703, 0.3219752754296894559, 0.3333333333333333703, 0.3219752754296894559, 0.3333333333333333703, 0.3219752754296894559, 0.3333333333333333703, 0.3219752754296894559, 0.3333333333333333703, 0.3219752754296894559, 0.3333333333333333703, 0.3219752754296894559, 0.3333333333333333703, 0.3219752754296894559, 0.3333333333333333703, 0.3219752754296894559, 0.3333333333333333703, 0.3219752754296894559, 0.3333333333333333703, 0.3219752754296894559, 0.3333333333333333703, 0.3219752754296894559, 0.3333333333333333703, 0.3219752754296894559, 0.3333333333333333703, 0.3219752754296894559, 0.3333333333333333703, 0.3219752754296894559, 0.3333333333333333703, 0.3219752754296894559, 0.3333333333333333703, 0.3219752754296894559, 0.3333333333333333703, 0.3219752754296894559, 0.3333333333333333703, 0.3219752754296894559, 0.3333333333333333703, 0.3219752754296894559, 0.3333333333333333703, 0.3219752754296894559, 0.3333333333333333703, 0.3219752754296894559, 0.3333333333333333703, 0.3219752754296894559, 0.3333333333333333703, 0.3219752754296894559, 0.3333333333333333703, 0.3219752754296894559, 0.3333333333333333703, 0.3219752754296894559, 0.3333333333333333703, 0.3219752754296894559, 0.3333333333333333703, 0.3219752754296894559, 0.3333333333333333703, 0.3219752754296894559, 0.3333333333333333703, 0.3219752754296894559, 0.3333333333333333703, 0.3219752754296894559, 0.3333333333333333703, 0.3219752754296894559, 0.3333333333333333703, 0.3219752754296894559, 0.3333333333333333703, 0.3219752754296894559, 0.3333333333333333703, 0.3219752754296894559, 0.3333333333333333703, 0.3219752754296894559, 0.3333333333333333703, 0.3219752754296894559, 0.3333333333333333703, 0.3219752754296894559, 0.3333333333333333703, 0.3219752754296894559, 0.3333333333333333703, 0.3219752754296894559, 0.3333333333333333703, 0.3219752754296894559, 0.3333333333333333703, 0.3219752754296894559, 0.3333333333333333703, 0.3219752754296894559, 0.3333333333333333703, 0.3219752754296894559, 0.3333333333333333703, 0.3219752754296894559, 0.3333333333333333703, 0.3219752754296894559, 0.3333333333333333703, 0.3219752754296894559, 0.3333333333333333703, 0.3219752754296894559, 0.3333333333333333703, 0.3219752754296894559, 0.3333333333333333703, 0.3219752754296894559, 0.3333333333333333703, 0.3219752754296894559, 0.3333333333333333703, 0.3219752754296894559, 0.3333333333333333703, 0.3219752754296894559, 0.3333333333333333703, 0.3219752754296894559, 0.3333333333333333703, 0.3219752754296894559, 0.3333333333333333703, 0.3219752754296894559, 0.3333333333333333703, 0.3219752754296894559, 0.3333333333333333703, 0.3219752754296894559, 0.3333333333333333703, 0.3219752754296894559, 0.3333333333333333703, 0.3219752754296894559, 0.3333333333333333703, 0.3219752754296894559, 0.3333333333333333703, 0.3219752754296894559, 0.3333333333333333703, 0.3219752754296894559, 0.3333333333333333703, 0.3219752754296894559, 0.3333333333333333703, 0.3219752754296894559, 0.3333333333333333703, 0.3219752754296894559, 0.3333333333333333703, 0.3219752754296894559, 0.3333333333333333703, 0.3219752754296894559, 0.3333333333333333703, 0.3219752754296894559, 0.3333333333333333703, 0.3219752754296894559, 0.3333333333333333703, 0.3219752754296894559, 0.3333333333333333703, 0.3219752754296894559, 0.3333333333333333703, 0.3219752754296894559, 0.3333333333333333703, 0.3219752754296894559, 0.3333333333333333703, 0.3219752754296894559, 0.3333333333333333703, 0.3219752754296894559, 0.3333333333333333703, 0.3219752754296894559, 0.3333333333333333703, 0.3219752754296894559, 0.3333333333333333703, 0.3219752754296894559, 0.3333333333333333703, 0.3219752754296894559, 0.3333333333333333703, 0.3219752754296894559, 0.3333333333333333703, 0.3219752754296894559, 0.3333333333333333703, 0.3219752754296894559, 0.3333333333333333703, 0.3219752754296894559, 0.3333333333333333703, 0.3219752754296894559, 0.3333333333333333703, 0.3219752754296894559, 0.3333333333333333703, 0.3219752754296894559, 0.3333333333333333703, 0.3219752754296894559, 0.3333333333333333703, 0.3219752754296894559, 0.3333333333333333703, 0.3219752754296894559, 0.3333333333333333703, 0.3219752754296894559, 0.3333333333333333703, 0.3219752754296894559, 0.3333333333333333703, 0.3219752754296894559, 0.3333333333333333703, 0.3219752754296894559, 0.3333333333333333703, 0.3219752754296894559, 0.3333333333333333703, 0.3219752754296894559, 0.3333333333333333703, 0.3219752754296894559, 0.3333333333333333703, 0.3219752754296894559, 0.3333333333333333703, 0.3219752754296894559, 0.3333333333333333703),
 ( 1.000000000000000000, 0.9659258262890683122, 1.000000000000000000, 0.9659258262890683122, 1.000000000000000000, 0.9659258262890683122, 1.000000000000000000, 0.9659258262890683122, 1.000000000000000000, 0.9659258262890683122, 1.000000000000000000, 0.9659258262890683122, 1.000000000000000000, 0.9659258262890683122, 1.000000000000000000, 0.9659258262890683122, 1.000000000000000000, 0.9659258262890683122, 1.000000000000000000, 0.9659258262890683122, 1.000000000000000000, 0.9659258262890683122, 1.000000000000000000, 0.9659258262890683122, 1.000000000000000000, 0.9659258262890683122, 1.000000000000000000, 0.9659258262890683122, 1.000000000000000000, 0.9659258262890683122, 1.000000000000000000, 0.9659258262890683122, 1.000000000000000000, 0.9659258262890683122, 1.000000000000000000, 0.9659258262890683122, 1.000000000000000000, 0.9659258262890683122, 1.000000000000000000, 0.9659258262890683122, 1.000000000000000000, 0.9659258262890683122, 1.000000000000000000, 0.9659258262890683122, 1.000000000000000000, 0.9659258262890683122, 1.000000000000000000, 0.9659258262890683122, 1.000000000000000000, 0.9659258262890683122, 1.000000000000000000, 0.9659258262890683122, 1.000000000000000000, 0.9659258262890683122, 1.000000000000000000, 0.9659258262890683122, 1.000000000000000000, 0.9659258262890683122, 1.000000000000000000, 0.9659258262890683122, 1.000000000000000000, 0.9659258262890683122, 1.000000000000000000, 0.9659258262890683122, 1.000000000000000000, 0.9659258262890683122, 1.000000000000000000, 0.9659258262890683122, 1.000000000000000000, 0.9659258262890683122, 1.000000000000000000, 0.9659258262890683122, 1.000000000000000000, 0.9659258262890683122, 1.000000000000000000, 0.9659258262890683122, 1.000000000000000000, 0.9659258262890683122, 1.000000000000000000, 0.9659258262890683122, 1.000000000000000000, 0.9659258262890683122, 1.000000000000000000, 0.9659258262890683122, 1.000000000000000000, 0.9659258262890683122, 1.000000000000000000, 0.9659258262890683122, 1.000000000000000000, 0.9659258262890683122, 1.000000000000000000, 0.9659258262890683122, 1.000000000000000000, 0.9659258262890683122, 1.000000000000000000, 0.9659258262890683122, 1.000000000000000000, 0.9659258262890683122, 1.000000000000000000, 0.9659258262890683122, 1.000000000000000000, 0.9659258262890683122, 1.000000000000000000, 0.9659258262890683122, 1.000000000000000000, 0.9659258262890683122, 1.000000000000000000, 0.9659258262890683122, 1.000000000000000000, 0.9659258262890683122, 1.000000000000000000, 0.9659258262890683122, 1.000000000000000000, 0.9659258262890683122, 1.000000000000000000, 0.9659258262890683122, 1.000000000000000000, 0.9659258262890683122, 1.000000000000000000, 0.9659258262890683122, 1.000000000000000000, 0.9659258262890683122, 1.000000000000000000, 0.9659258262890683122, 1.000000000000000000, 0.9659258262890683122, 1.000000000000000000, 0.9659258262890683122, 1.000000000000000000, 0.9659258262890683122, 1.000000000000000000, 0.9659258262890683122, 1.000000000000000000, 0.9659258262890683122, 1.000000000000000000, 0.9659258262890683122, 1.000000000000000000, 0.9659258262890683122, 1.000000000000000000, 0.9659258262890683122, 1.000000000000000000, 0.9659258262890683122, 1.000000000000000000, 0.9659258262890683122, 1.000000000000000000, 0.9659258262890683122, 1.000000000000000000, 0.9659258262890683122, 1.000000000000000000, 0.9659258262890683122, 1.000000000000000000, 0.9659258262890683122, 1.000000000000000000, 0.9659258262890683122, 1.000000000000000000, 0.9659258262890683122, 1.000000000000000000, 0.9659258262890683122, 1.000000000000000000, 0.9659258262890683122, 1.000000000000000000, 0.9659258262890683122, 1.000000000000000000, 0.9659258262890683122, 1.000000000000000000, 0.9659258262890683122, 1.000000000000000000, 0.9659258262890683122, 1.000000000000000000, 0.9659258262890683122, 1.000000000000000000, 0.9659258262890683122, 1.000000000000000000, 0.9659258262890683122, 1.000000000000000000, 0.9659258262890683122, 1.000000000000000000, 0.9659258262890683122, 1.000000000000000000, 0.9659258262890683122, 1.000000000000000000, 0.9659258262890683122, 1.000000000000000000, 0.9659258262890683122, 1.000000000000000000, 0.9659258262890683122, 1.000000000000000000, 0.9659258262890683122, 1.000000000000000000, 0.9659258262890683122, 1.000000000000000000, 0.9659258262890683122, 1.000000000000000000, 0.9659258262890683122, 1.000000000000000000, 0.9659258262890683122, 1.000000000000000000, 0.9659258262890683122, 1.000000000000000000, 0.9659258262890683122, 1.000000000000000000, 0.9659258262890683122, 1.000000000000000000, 0.9659258262890683122, 1.000000000000000000, 0.9659258262890683122, 1.000000000000000000, 0.9659258262890683122, 1.000000000000000000, 0.9659258262890683122, 1.000000000000000000, 0.9659258262890683122, 1.000000000000000000, 0.9659258262890683122, 1.000000000000000000, 0.9659258262890683122, 1.000000000000000000, 0.9659258262890683122, 1.000000000000000000, 0.9659258262890683122, 1.000000000000000000, 0.9659258262890683122, 1.000000000000000000, 0.9659258262890683122, 1.000000000000000000, 0.9659258262890683122, 1.000000000000000000, 0.9659258262890683122, 1.000000000000000000, 0.9659258262890683122, 1.000000000000000000, 0.9659258262890683122, 1.000000000000000000, 0.9659258262890683122, 1.000000000000000000, 0.9659258262890683122, 1.000000000000000000, 0.9659258262890683122, 1.000000000000000000, 0.9659258262890683122, 1.000000000000000000, 0.9659258262890683122, 1.000000000000000000, 0.9659258262890683122, 1.000000000000000000, 0.9659258262890683122, 1.000000000000000000, 0.9659258262890683122, 1.000000000000000000, 0.9659258262890683122, 1.000000000000000000, 0.9659258262890683122, 1.000000000000000000, 0.9659258262890683122, 1.000000000000000000, 0.9659258262890683122, 1.000000000000000000, 0.9659258262890683122, 1.000000000000000000, 0.9659258262890683122, 1.000000000000000000, 0.9659258262890683122, 1.000000000000000000, 0.9659258262890683122, 1.000000000000000000, 0.9659258262890683122, 1.000000000000000000, 0.9659258262890683122, 1.000000000000000000, 0.9659258262890683122, 1.000000000000000000, 0.9659258262890683122, 1.000000000000000000, 0.9659258262890683122, 1.000000000000000000, 0.9659258262890683122, 1.000000000000000000, 0.9659258262890683122, 1.000000000000000000, 0.9659258262890683122, 1.000000000000000000, 0.9659258262890683122, 1.000000000000000000, 0.9659258262890683122, 1.000000000000000000, 0.9659258262890683122, 1.000000000000000000, 0.9659258262890683122, 1.000000000000000000, 0.9659258262890683122, 1.000000000000000000, 0.9659258262890683122, 1.000000000000000000, 0.9659258262890683122, 1.000000000000000000, 0.9659258262890683122, 1.000000000000000000, 0.9659258262890683122, 1.000000000000000000, 0.9659258262890683122, 1.000000000000000000, 0.9659258262890683122, 1.000000000000000000, 0.9659258262890683122, 1.000000000000000000, 0.9659258262890683122, 1.000000000000000000, 0.9659258262890683122, 1.000000000000000000, 0.9659258262890683122, 1.000000000000000000, 0.9659258262890683122, 1.000000000000000000, 0.9659258262890683122, 1.000000000000000000, 0.9659258262890683122, 1.000000000000000000, 0.9659258262890683122, 1.000000000000000000, 0.9659258262890683122, 1.000000000000000000, 0.9659258262890683122, 1.000000000000000000, 0.9659258262890683122, 1.000000000000000000, 0.9659258262890683122, 1.000000000000000000, 0.9659258262890683122, 1.000000000000000000, 0.9659258262890683122, 1.000000000000000000, 0.9659258262890683122, 1.000000000000000000, 0.9659258262890683122, 1.000000000000000000, 0.9659258262890683122, 1.000000000000000000, 0.9659258262890683122, 1.000000000000000000, 0.9659258262890683122, 1.000000000000000000, 0.9659258262890683122, 1.000000000000000000, 0.9659258262890683122, 1.000000000000000000, 0.9659258262890683122, 1.000000000000000000, 0.9659258262890683122, 1.000000000000000000, 0.9659258262890683122, 1.000000000000000000, 0.9659258262890683122, 1.000000000000000000, 0.9659258262890683122, 1.000000000000000000, 0.9659258262890683122, 1.000000000000000000, 0.9659258262890683122, 1.000000000000000000, 0.9659258262890683122, 1.000000000000000000, 0.9659258262890683122, 1.000000000000000000, 0.9659258262890683122, 1.000000000000000000, 0.9659258262890683122, 1.000000000000000000, 0.9659258262890683122, 1.000000000000000000, 0.9659258262890683122, 1.000000000000000000, 0.9659258262890683122, 1.000000000000000000, 0.9659258262890683122, 1.000000000000000000, 0.9659258262890683122, 1.000000000000000000, 0.9659258262890683122, 1.000000000000000000, 0.9659258262890683122, 1.000000000000000000, 0.9659258262890683122, 1.000000000000000000, 0.9659258262890683122, 1.000000000000000000, 0.9659258262890683122, 1.000000000000000000, 0.9659258262890683122, 1.000000000000000000, 0.9659258262890683122, 1.000000000000000000, 0.9659258262890683122, 1.000000000000000000, 0.9659258262890683122, 1.000000000000000000, 0.9659258262890683122, 1.000000000000000000, 0.9659258262890683122, 1.000000000000000000, 0.9659258262890683122, 1.000000000000000000, 0.9659258262890683122, 1.000000000000000000, 0.9659258262890683122, 1.000000000000000000, 0.9659258262890683122, 1.000000000000000000, 0.9659258262890683122, 1.000000000000000000, 0.9659258262890683122, 1.000000000000000000, 0.9659258262890683122, 1.000000000000000000, 0.9659258262890683122, 1.000000000000000000, 0.9659258262890683122, 1.000000000000000000, 0.9659258262890683122, 1.000000000000000000, 0.9659258262890683122, 1.000000000000000000, 0.9659258262890683122, 1.000000000000000000, 0.9659258262890683122, 1.000000000000000000, 0.9659258262890683122, 1.000000000000000000, 0.9659258262890683122, 1.000000000000000000, 0.9659258262890683122, 1.000000000000000000, 0.9659258262890683122, 1.000000000000000000, 0.9659258262890683122, 1.000000000000000000, 0.9659258262890683122, 1.000000000000000000, 0.9659258262890683122, 1.000000000000000000, 0.9659258262890683122, 1.000000000000000000, 0.9659258262890683122, 1.000000000000000000, 0.9659258262890683122, 1.000000000000000000, 0.9659258262890683122, 1.000000000000000000, 0.9659258262890683122, 1.000000000000000000, 0.9659258262890683122, 1.000000000000000000, 0.9659258262890683122, 1.000000000000000000, 0.9659258262890683122, 1.000000000000000000, 0.9659258262890683122, 1.000000000000000000) ) ) 
 REPRESENTATION_ITEM ( '' )  SURFACE ( )  );
#51108=CARTESIAN_POINT ( 'NONE',  ( 0.05219959533909260263, 19.03943276465977164, 24.99890960531435269 ) ) ;
#51109=CARTESIAN_POINT ( 'NONE',  ( -9.564922557960796823, -16.46253265017161027, 82.08224293864768129 ) ) ;
#51110=CARTESIAN_POINT ( 'NONE',  ( 16.51473224551083163, -9.474510206698727899, 110.8344237280190043 ) ) ;
#51112=CARTESIAN_POINT ( 'NONE',  ( 19.05341960407617918, -5.049401038297876454, 21.04275706135232582 ) ) ;
#51113=CARTESIAN_POINT ( 'NONE',  ( -0.05219959533934338120, 16.53943276465976808, 77.50109039468567573 ) ) ;
#51114=CARTESIAN_POINT ( 'NONE',  ( -9.564922557961040184, 16.46253265017147172, 112.9177570613523329 ) ) ;
#51115=CARTESIAN_POINT ( 'NONE',  ( 12.06949235617757843, -12.14591786802309237, 113.1239096053143953 ) ) ;
#51116=CARTESIAN_POINT ( 'NONE',  ( -8.314922557961024197, 14.29746914071037800, 72.91775706135234714 ) ) ;
#51117=CARTESIAN_POINT ( 'NONE',  ( -14.29746914071037622, -8.314922557961029526, 49.16775706135234003 ) ) ;
#51118=CARTESIAN_POINT ( 'NONE',  ( 13.89961937509977652, -13.97604488694527269, 23.12390960531436335 ) ) ;
#51119=CARTESIAN_POINT ( 'NONE',  ( -16.46253265017146816, -9.564922557961047289, 74.16775706135234714 ) ) ;
#51120=CARTESIAN_POINT ( 'NONE',  ( 21.55341960407619695, -5.719274019375665929, 106.0427570613523471 ) ) ;
#51121=CARTESIAN_POINT ( 'NONE',  ( -5.049401038298153566, 19.05341960407611168, 30.20724293864768839 ) ) ;
#51122=CARTESIAN_POINT ( 'NONE',  ( -16.46253265017160317, 9.564922557960807481, 75.83224293864769550 ) ) ;
#51123=CARTESIAN_POINT ( 'NONE',  ( -16.52544592524342804, 4.483927247898546575, 71.04057627198103830 ) ) ;
#51124=CARTESIAN_POINT ( 'NONE',  ( 0.05219959533936267826, -19.03943276465977164, 40.00109039468566152 ) ) ;
#51125=CARTESIAN_POINT ( 'NONE',  ( -18.67979575497178146, -10.72451020669898902, 41.66557627198103120 ) ) ;
#51126=CARTESIAN_POINT ( 'NONE',  ( -21.53943276465977519, -0.05219959533937600094, 108.7510903946857042 ) ) ;
#51127=CARTESIAN_POINT ( 'NONE',  ( -13.89961937509977652, 13.97604488694528158, 95.62390960531436690 ) ) ;
#51128=CARTESIAN_POINT ( 'NONE',  ( 15.72974639402176855, 15.80617190586768217, 101.8760903946857042 ) ) ;
#51129=CARTESIAN_POINT ( 'NONE',  ( -5.823673210054116645, -21.52544592524344225, 67.29057627198103830 ) ) ;
#51130=CARTESIAN_POINT ( 'NONE',  ( -16.46253265017160317, 9.564922557960807481, 95.83224293864769550 ) ) ;
#51131=CARTESIAN_POINT ( 'NONE',  ( -19.02544592524334988, -5.153800228976617603, 88.95942372801897591 ) ) ;
#51132=CARTESIAN_POINT ( 'NONE',  ( 19.05341960407611168, 5.049401038298154454, 103.9572429386476671 ) ) ;
#51133=CARTESIAN_POINT ( 'NONE',  ( -9.474510206698720793, -16.51473224551083518, 94.58442372801900433 ) ) ;
#51134=CARTESIAN_POINT ( 'NONE',  ( -4.483927247898539470, -16.52544592524342804, 112.2905762719810241 ) ) ;
#51135=CARTESIAN_POINT ( 'NONE',  ( 13.97604488694527802, 13.89961937509977652, 84.37390960531433848 ) ) ;
#51136=CARTESIAN_POINT ( 'NONE',  ( -21.55341960407610458, -5.719274019375992779, 61.45724293864770260 ) ) ;
#51137=CARTESIAN_POINT ( 'NONE',  ( 16.55341960407618274, -4.379528057220086978, 31.04275706135234714 ) ) ;
#51138=CARTESIAN_POINT ( 'NONE',  ( -21.55341960407619339, 5.719274019375674811, 53.54275706135234714 ) ) ;
#51139=CARTESIAN_POINT ( 'NONE',  ( 21.55341960407619695, -5.719274019375665929, 91.04275706135236135 ) ) ;
#51140=CARTESIAN_POINT ( 'NONE',  ( 0.05219959533934541429, -16.53943276465976808, 100.0010903946857042 ) ) ;
#51141=CARTESIAN_POINT ( 'NONE',  ( 5.153800228976335163, 19.02544592524342804, 84.79057627198099567 ) ) ;
#51142=CARTESIAN_POINT ( 'NONE',  ( 12.06949235617757843, -12.14591786802309237, 88.12390960531436690 ) ) ;
#51143=CARTESIAN_POINT ( 'NONE',  ( -14.29746914071037622, -8.314922557961029526, 109.1677570613523613 ) ) ;
#51144=CARTESIAN_POINT ( 'NONE',  ( -0.05219959533936034679, 19.03943276465977164, 62.50109039468566863 ) ) ;
#51145=CARTESIAN_POINT ( 'NONE',  ( -21.52544592524334988, -5.823673210054445271, 43.95942372801902565 ) ) ;
#51146=CARTESIAN_POINT ( 'NONE',  ( -14.29746914071049879, 8.314922557960819915, 95.83224293864770971 ) ) ;
#51147=CARTESIAN_POINT ( 'NONE',  ( -19.03943276465977164, 0.05219959533909376836, 106.2489096053143669 ) ) ;
#51148=CARTESIAN_POINT ( 'NONE',  ( 4.379528057220339221, -16.55341960407611168, 27.70724293864769905 ) ) ;
#51149=CARTESIAN_POINT ( 'NONE',  ( 5.823673210054444382, -21.52544592524334988, 85.20942372801901854 ) ) ;
#51150=CARTESIAN_POINT ( 'NONE',  ( 16.52544592524335698, 4.483927247898782831, 51.45942372801901854 ) ) ;
#51151=CARTESIAN_POINT ( 'NONE',  ( -15.72974639402176322, -15.80617190586768395, 39.37609039468567573 ) ) ;
#51153=CARTESIAN_POINT ( 'NONE',  ( -21.52544592524334988, -5.823673210054445271, 18.95942372801901143 ) ) ;
#51154=CARTESIAN_POINT ( 'NONE',  ( 0.05219959533910956823, 16.53943276465976808, 89.99890960531438111 ) ) ;
#51156=CARTESIAN_POINT ( 'NONE',  ( -19.01529144963331674, -5.500000000000165201, 51.23431955728442233 ) ) ;
#51157=CARTESIAN_POINT ( 'NONE',  ( 16.55341960407611168, 4.379528057220329451, 63.95724293864770260 ) ) ;
#51158=CARTESIAN_POINT ( 'NONE',  ( 5.049401038298161559, -19.05341960407611168, 52.70724293864767418 ) ) ;
#51159=CARTESIAN_POINT ( 'NONE',  ( 14.29746914071037800, 8.314922557961029526, 111.6677570613523613 ) ) ;
#51160=CARTESIAN_POINT ( 'NONE',  ( -5.153800228976328057, -19.02544592524343514, 42.29057627198101699 ) ) ;
#51161=CARTESIAN_POINT ( 'NONE',  ( -0.05219959533907301413, -21.53943276465977519, 37.49890960531436690 ) ) ;
#51162=CARTESIAN_POINT ( 'NONE',  ( 8.314922557960818139, 14.29746914071049879, 84.58224293864769550 ) ) ;
#51163=CARTESIAN_POINT ( 'NONE',  ( 10.81492255796078972, 18.62759615963270932, 94.58224293864769550 ) ) ;
#51164=CARTESIAN_POINT ( 'NONE',  ( 13.97604488694527802, 13.89961937509977652, 84.37390960531433848 ) ) ;
#51165=CARTESIAN_POINT ( 'NONE',  ( 19.02544592524343514, -5.153800228976328945, 38.54057627198103120 ) ) ;
#51166=CARTESIAN_POINT ( 'NONE',  ( -5.153800228976607833, 19.02544592524334988, 87.70942372801897591 ) ) ;
#51167=ADVANCED_FACE ( 'NONE', ( #176139 ), #49799, .T. ) ;
#51168=CARTESIAN_POINT ( 'NONE',  ( 10.72451020669898902, -18.67979575497178502, 47.91557627198102409 ) ) ;
#51169=CARTESIAN_POINT ( 'NONE',  ( -15.80617190586768217, 15.72974639402176855, 73.12609039468567573 ) ) ;
#51170=CARTESIAN_POINT ( 'NONE',  ( -19.03943276465977164, 0.05219959533909376836, 51.24890960531436690 ) ) ;
#51171=CARTESIAN_POINT ( 'NONE',  ( 19.05341960407611168, 5.049401038298154454, 78.95724293864769550 ) ) ;
#51172=ORIENTED_EDGE ( 'NONE', *, *, #45882, .F. ) ;
#51173=CARTESIAN_POINT ( 'NONE',  ( 8.314922557961029526, -14.29746914071037800, 65.41775706135234714 ) ) ;
#51174=CARTESIAN_POINT ( 'NONE',  ( -18.67979575497193778, 10.72451020669871902, 48.33442372801902565 ) ) ;
#51175=CARTESIAN_POINT ( 'NONE',  ( -18.67979575497193778, 10.72451020669871902, 73.33442372801901854 ) ) ;
#51176=CARTESIAN_POINT ( 'NONE',  ( 5.153800228976335163, 19.02544592524342804, 114.7905762719810241 ) ) ;
#51177=CARTESIAN_POINT ( 'NONE',  ( 18.62759615963271287, -10.81492255796078972, 98.33224293864769550 ) ) ;
#51178=CARTESIAN_POINT ( 'NONE',  ( 21.53943276465977519, 0.05219959533937863772, 41.25109039468568284 ) ) ;
#51179=CARTESIAN_POINT ( 'NONE',  ( 8.224510206698742110, 14.34966873604972548, 62.08442372801901143 ) ) ;
#51180=CARTESIAN_POINT ( 'NONE',  ( 21.52544592524344225, -5.823673210054117533, 58.54057627198103120 ) ) ;
#51181=CARTESIAN_POINT ( 'NONE',  ( -19.02544592524334988, -5.153800228976617603, 28.95942372801900433 ) ) ;
#51182=CARTESIAN_POINT ( 'NONE',  ( -19.02544592524342804, 5.153800228976336051, 66.04057627198103830 ) ) ;
#51183=CARTESIAN_POINT ( 'NONE',  ( 16.53943276465976808, 0.05219959533934440121, 101.2510903946856757 ) ) ;
#51185=CARTESIAN_POINT ( 'NONE',  ( 13.97604488694527802, 13.89961937509977652, 99.37390960531436690 ) ) ;
#51187=CARTESIAN_POINT ( 'NONE',  ( -19.02544592524334988, -5.153800228976617603, 78.95942372801900433 ) ) ;
#51188=CARTESIAN_POINT ( 'NONE',  ( 0.05219959533907565091, 21.53943276465977519, 59.99890960531436690 ) ) ;
#51189=CARTESIAN_POINT ( 'NONE',  ( 12.06949235617757843, -12.14591786802309237, 33.12390960531435979 ) ) ;
#51190=CARTESIAN_POINT ( 'NONE',  ( 19.02544592524334988, 5.153800228976608722, 101.4594237280189759 ) ) ;
#51192=CARTESIAN_POINT ( 'NONE',  ( -16.51473224551082808, 9.474510206698731452, 103.3344237280190043 ) ) ;
#51193=CARTESIAN_POINT ( 'NONE',  ( -18.62759615963270932, 10.81492255796079327, 85.83224293864768129 ) ) ;
#51194=CARTESIAN_POINT ( 'NONE',  ( 19.03943276465977164, 0.05219959533936151252, 61.25109039468566863 ) ) ;
#51196=CARTESIAN_POINT ( 'NONE',  ( 9.474510206698971260, -16.51473224551069308, 62.91557627198102409 ) ) ;
#51197=CARTESIAN_POINT ( 'NONE',  ( -16.53943276465976808, 0.05219959533911058130, 61.24890960531435979 ) ) ;
#51198=CARTESIAN_POINT ( 'NONE',  ( 19.02544592524343514, -5.153800228976328945, 48.54057627198103120 ) ) ;
#51199=CARTESIAN_POINT ( 'NONE',  ( 8.314922557960818139, 14.29746914071049879, 49.58224293864769550 ) ) ;
#51202=CARTESIAN_POINT ( 'NONE',  ( 4.379528057220339221, -16.55341960407611168, 27.70724293864769905 ) ) ;
#51203=CARTESIAN_POINT ( 'NONE',  ( -16.51473224551069308, -9.474510206698971260, 61.66557627198103120 ) ) ;
#51205=CARTESIAN_POINT ( 'NONE',  ( -5.049401038297874678, -19.05341960407617918, 34.79275706135233293 ) ) ;
#51206=CARTESIAN_POINT ( 'NONE',  ( 12.14591786802327356, -12.06949235617739191, 45.62609039468567573 ) ) ;
#51207=CARTESIAN_POINT ( 'NONE',  ( 15.72974639402199770, -15.80617190586745480, 48.12390960531436690 ) ) ;
#51208=CARTESIAN_POINT ( 'NONE',  ( 15.80617190586769283, -15.72974639402175789, 110.6260903946857042 ) ) ;
#51209=CARTESIAN_POINT ( 'NONE',  ( -16.46253265017160317, 9.564922557960807481, 80.83224293864769550 ) ) ;
#51211=CARTESIAN_POINT ( 'NONE',  ( -15.80617190586745835, -15.72974639402198527, 21.87390960531436690 ) ) ;
#51212=CARTESIAN_POINT ( 'NONE',  ( -15.72974639402176322, -15.80617190586768395, 44.37609039468567573 ) ) ;
#51213=CARTESIAN_POINT ( 'NONE',  ( 8.314922557960818139, 14.29746914071049879, 94.58224293864769550 ) ) ;
#51214=CARTESIAN_POINT ( 'NONE',  ( -15.80617190586745835, -15.72974639402198527, 91.87390960531436690 ) ) ;
#51215=CARTESIAN_POINT ( 'NONE',  ( 19.03943276465977164, -0.05219959533909143690, 78.74890960531436690 ) ) ;
#51217=CARTESIAN_POINT ( 'NONE',  ( 9.474510206698971260, -16.51473224551069308, 87.91557627198102409 ) ) ;
#51218=CARTESIAN_POINT ( 'NONE',  ( 0.05219959533937995610, -21.53943276465977519, 20.00109039468568639 ) ) ;
#51220=CARTESIAN_POINT ( 'NONE',  ( -13.89961937509977652, 13.97604488694528158, 80.62390960531436690 ) ) ;
#51222=CARTESIAN_POINT ( 'NONE',  ( -9.564922557960796823, -16.46253265017161027, 27.08224293864769550 ) ) ;
#51223=CARTESIAN_POINT ( 'NONE',  ( 16.51473224551069308, 9.474510206698969483, 39.16557627198103120 ) ) ;
#51224=CARTESIAN_POINT ( 'NONE',  ( 9.564922557961047289, -16.46253265017146816, 110.4177570613523471 ) ) ;
#51226=CARTESIAN_POINT ( 'NONE',  ( -8.224510206698948167, 14.34966873604960824, 105.4155762719810383 ) ) ;
#51227=CARTESIAN_POINT ( 'NONE',  ( -10.81492255796105439, 18.62759615963255655, 82.91775706135234714 ) ) ;
#51228=CARTESIAN_POINT ( 'NONE',  ( -16.51473224551069308, -9.474510206698971260, 61.66557627198103120 ) ) ;
#51229=CARTESIAN_POINT ( 'NONE',  ( 5.719274019375673035, 21.55341960407619339, 27.29275706135234358 ) ) ;
#51230=CARTESIAN_POINT ( 'NONE',  ( -21.52544592524343514, 5.823673210054127303, 106.0405762719810525 ) ) ;
#51232=CARTESIAN_POINT ( 'NONE',  ( -9.564922557960796823, -16.46253265017161027, 92.08224293864769550 ) ) ;
#51233=LINE ( 'NONE', #100715, #21054 ) ;
#51234=CARTESIAN_POINT ( 'NONE',  ( 12.14591786802327356, -12.06949235617739191, 20.62609039468568639 ) ) ;
#51235=CARTESIAN_POINT ( 'NONE',  ( -21.53943276465977519, 0.05219959533907696930, 41.24890960531435269 ) ) ;
#51236=CARTESIAN_POINT ( 'NONE',  ( -15.72974639402176322, -15.80617190586768395, 59.37609039468568284 ) ) ;
#51237=CARTESIAN_POINT ( 'NONE',  ( -16.46253265017160317, 9.564922557960807481, 110.8322429386476955 ) ) ;
#51238=CARTESIAN_POINT ( 'NONE',  ( -0.05219959533936034679, 19.03943276465977164, 92.50109039468566152 ) ) ;
#51239=CARTESIAN_POINT ( 'NONE',  ( 5.153800228976335163, 19.02544592524342804, 59.79057627198100988 ) ) ;
#51240=CARTESIAN_POINT ( 'NONE',  ( -9.564922557960796823, -16.46253265017161027, 87.08224293864769550 ) ) ;
#51242=CARTESIAN_POINT ( 'NONE',  ( 8.314922557960818139, 14.29746914071049879, 89.58224293864768129 ) ) ;
#51243=CARTESIAN_POINT ( 'NONE',  ( 14.34966873604960469, 8.224510206698951720, 89.16557627198102409 ) ) ;
#51244=CARTESIAN_POINT ( 'NONE',  ( 9.564922557960805705, 16.46253265017160317, 109.5822429386476955 ) ) ;
#51245=CARTESIAN_POINT ( 'NONE',  ( -12.06949235617756955, 12.14591786802309770, 50.62390960531435979 ) ) ;
#51246=CARTESIAN_POINT ( 'NONE',  ( 19.03943276465977164, -0.05219959533909143690, 43.74890960531435979 ) ) ;
#51247=CARTESIAN_POINT ( 'NONE',  ( 5.823673210054444382, -21.52544592524334988, 65.20942372801901854 ) ) ;
#51248=CARTESIAN_POINT ( 'NONE',  ( -5.153800228976607833, 19.02544592524334988, 87.70942372801897591 ) ) ;
#51249=CARTESIAN_POINT ( 'NONE',  ( -0.05219959533910754901, -16.53943276465976808, 57.49890960531435979 ) ) ;
#51250=CARTESIAN_POINT ( 'NONE',  ( 10.81492255796106328, -18.62759615963255655, 20.41775706135234714 ) ) ;
#51251=CARTESIAN_POINT ( 'NONE',  ( -18.67979575497178146, -10.72451020669898902, 51.66557627198102409 ) ) ;
#51252=FACE_OUTER_BOUND ( 'NONE', #88537, .T. ) ;
#51254=CARTESIAN_POINT ( 'NONE',  ( 13.89961937509977652, -13.97604488694527269, 58.12390960531436690 ) ) ;
#51255=CARTESIAN_POINT ( 'NONE',  ( 16.52544592524342804, -4.483927247898539470, 33.54057627198102409 ) ) ;
#51256=CARTESIAN_POINT ( 'NONE',  ( 0.05219959533934541429, -16.53943276465976808, 100.0010903946857042 ) ) ;
#51257=CARTESIAN_POINT ( 'NONE',  ( 14.34966873604972726, -8.224510206698740333, 85.83442372801901854 ) ) ;
#51258=CARTESIAN_POINT ( 'NONE',  ( -9.564922557961040184, 16.46253265017147172, 37.91775706135233293 ) ) ;
#51259=CARTESIAN_POINT ( 'NONE',  ( -17.49999999999999289, 5.500000000000032863, 70.79690382534172954 ) ) ;
#51260=CARTESIAN_POINT ( 'NONE',  ( -5.153800228976328057, -19.02544592524343514, 92.29057627198099567 ) ) ;
#51261=CARTESIAN_POINT ( 'NONE',  ( -19.02544592524342804, 5.153800228976336051, 56.04057627198100988 ) ) ;
#51262=CARTESIAN_POINT ( 'NONE',  ( -8.224510206698948167, 14.34966873604960824, 65.41557627198102409 ) ) ;
#51263=CARTESIAN_POINT ( 'NONE',  ( 17.40861289039002813, -6.110651285853312409, 101.1276752917256658 ) ) ;
#51264=CARTESIAN_POINT ( 'NONE',  ( -5.049401038298153566, 19.05341960407611168, 115.2072429386477097 ) ) ;
#51265=CARTESIAN_POINT ( 'NONE',  ( 10.81492255796078972, 18.62759615963270932, 49.58224293864769550 ) ) ;
#51266=CARTESIAN_POINT ( 'NONE',  ( -14.29746914071049879, 8.314922557960819915, 80.83224293864769550 ) ) ;
#51267=CARTESIAN_POINT ( 'NONE',  ( -12.06949235617739369, -12.14591786802326823, 39.37609039468567573 ) ) ;
#51268=CARTESIAN_POINT ( 'NONE',  ( 14.34966873604960469, 8.224510206698951720, 84.16557627198103830 ) ) ;
#51270=CARTESIAN_POINT ( 'NONE',  ( -18.39635199886966177, 5.500000000000102141, 66.01967076359997577 ) ) ;
#51271=CARTESIAN_POINT ( 'NONE',  ( -16.51473224551082808, 9.474510206698731452, 83.33442372801899012 ) ) ;
#51272=CARTESIAN_POINT ( 'NONE',  ( 21.55341960407610458, 5.719274019375980345, 23.95724293864769550 ) ) ;
#51274=CARTESIAN_POINT ( 'NONE',  ( 19.27311148717737055, 5.499999999999991118, 101.9602859708923575 ) ) ;
#51275=CARTESIAN_POINT ( 'NONE',  ( -12.06949235617739369, -12.14591786802326823, 24.37609039468567573 ) ) ;
#51276=CARTESIAN_POINT ( 'NONE',  ( 12.06949235617757843, -12.14591786802309237, 23.12390960531436335 ) ) ;
#51277=CARTESIAN_POINT ( 'NONE',  ( -13.89961937509957401, -13.97604488694547875, 74.37609039468566152 ) ) ;
#51278=CARTESIAN_POINT ( 'NONE',  ( 21.53943276465977519, -0.05219959533907433946, 48.74890960531435979 ) ) ;
#51279=CARTESIAN_POINT ( 'NONE',  ( 10.72451020669871369, 18.67979575497193778, 62.08442372801901143 ) ) ;
#51281=CARTESIAN_POINT ( 'NONE',  ( 12.14591786802327356, -12.06949235617739191, 30.62609039468567929 ) ) ;
#51282=CARTESIAN_POINT ( 'NONE',  ( -5.153800228976328057, -19.02544592524343514, 27.29057627198103120 ) ) ;
#51283=CARTESIAN_POINT ( 'NONE',  ( 19.03943276465977164, -0.05219959533909143690, 88.74890960531436690 ) ) ;
#51285=CARTESIAN_POINT ( 'NONE',  ( -16.53943276465976808, 0.05219959533911058130, 86.24890960531436690 ) ) ;
#51287=CARTESIAN_POINT ( 'NONE',  ( 13.89961937509977652, -13.97604488694527269, 103.1239096053143527 ) ) ;
#51289=CARTESIAN_POINT ( 'NONE',  ( 9.564922557961047289, -16.46253265017146816, 100.4177570613523329 ) ) ;
#51290=CARTESIAN_POINT ( 'NONE',  ( -5.823673210054116645, -21.52544592524344225, 82.29057627198103830 ) ) ;
#51291=CARTESIAN_POINT ( 'NONE',  ( -0.05219959533909027116, -19.03943276465977164, 47.49890960531435979 ) ) ;
#51292=CARTESIAN_POINT ( 'NONE',  ( -5.049401038297874678, -19.05341960407617918, 64.79275706135233293 ) ) ;
#51293=CARTESIAN_POINT ( 'NONE',  ( -21.52544592524343514, 5.823673210054127303, 116.0405762719810383 ) ) ;
#51294=CARTESIAN_POINT ( 'NONE',  ( 16.51473224551069308, 9.474510206698969483, 64.16557627198102409 ) ) ;
#51295=CARTESIAN_POINT ( 'NONE',  ( -19.03943276465977164, 0.05219959533909376836, 111.2489096053143669 ) ) ;
#51297=CARTESIAN_POINT ( 'NONE',  ( 0.05219959533934541429, -16.53943276465976808, 35.00109039468568284 ) ) ;
#51298=CARTESIAN_POINT ( 'NONE',  ( 5.719274019375991003, -21.55341960407610458, 97.70724293864772392 ) ) ;
#51299=CARTESIAN_POINT ( 'NONE',  ( 12.14591786802309770, 12.06949235617756955, 109.3739096053143811 ) ) ;
#51300=CARTESIAN_POINT ( 'NONE',  ( 0.05219959533909260263, 19.03943276465977164, 89.99890960531436690 ) ) ;
#51301=CARTESIAN_POINT ( 'NONE',  ( 16.46253265017146816, 9.564922557961045513, 61.66775706135234003 ) ) ;
#51302=CARTESIAN_POINT ( 'NONE',  ( -18.67979575497178146, -10.72451020669898902, 86.66557627198102409 ) ) ;
#51303=CARTESIAN_POINT ( 'NONE',  ( -14.34966873604960291, -8.224510206698953496, 46.66557627198102409 ) ) ;
#51304=CARTESIAN_POINT ( 'NONE',  ( -19.05341960407617563, 5.049401038297882671, 28.54275706135232937 ) ) ;
#51305=CARTESIAN_POINT ( 'NONE',  ( 14.34966873604972726, -8.224510206698740333, 60.83442372801901854 ) ) ;
#51306=CARTESIAN_POINT ( 'NONE',  ( -19.03943276465977164, 0.05219959533909376836, 91.24890960531436690 ) ) ;
#51308=CARTESIAN_POINT ( 'NONE',  ( 16.46253265017160672, -9.564922557960803928, 43.33224293864769550 ) ) ;
#51309=CARTESIAN_POINT ( 'NONE',  ( 0.05219959533937995610, -21.53943276465977519, 50.00109039468568994 ) ) ;
#51310=CARTESIAN_POINT ( 'NONE',  ( 0.05219959533937995610, -21.53943276465977519, 70.00109039468568994 ) ) ;
#51311=CARTESIAN_POINT ( 'NONE',  ( -19.05341960407611168, -5.049401038298163336, 61.45724293864769550 ) ) ;
#51312=CARTESIAN_POINT ( 'NONE',  ( -15.72974639402176322, -15.80617190586768395, 29.37609039468568284 ) ) ;
#51313=CARTESIAN_POINT ( 'NONE',  ( 19.05341960407617918, -5.049401038297876454, 81.04275706135231871 ) ) ;
#51314=CARTESIAN_POINT ( 'NONE',  ( 9.564922557960805705, 16.46253265017160317, 34.58224293864770260 ) ) ;
#51315=CARTESIAN_POINT ( 'NONE',  ( -12.06949235617739369, -12.14591786802326823, 84.37609039468570415 ) ) ;
#51316=CARTESIAN_POINT ( 'NONE',  ( 9.564922557960805705, 16.46253265017160317, 54.58224293864769550 ) ) ;
#51318=CARTESIAN_POINT ( 'NONE',  ( 19.05341960407611168, 5.049401038298154454, 33.95724293864769550 ) ) ;
#51320=CARTESIAN_POINT ( 'NONE',  ( 10.72451020669898902, -18.67979575497178502, 92.91557627198103830 ) ) ;
#51321=CARTESIAN_POINT ( 'NONE',  ( 16.55341960407618274, -4.379528057220086978, 76.04275706135237556 ) ) ;
#51323=CARTESIAN_POINT ( 'NONE',  ( 9.474510206698729675, 16.51473224551082808, 27.08442372801900433 ) ) ;
#51324=CARTESIAN_POINT ( 'NONE',  ( 13.97604488694527802, 13.89961937509977652, 59.37390960531434558 ) ) ;
#51325=CARTESIAN_POINT ( 'NONE',  ( 12.14591786802309770, 12.06949235617756955, 49.37390960531436690 ) ) ;
#51326=CARTESIAN_POINT ( 'NONE',  ( 14.29746914071049879, -8.314922557960816363, 83.33224293864769550 ) ) ;
#51328=CARTESIAN_POINT ( 'NONE',  ( -19.03943276465977164, 0.05219959533909376836, 101.2489096053143669 ) ) ;
#51329=CARTESIAN_POINT ( 'NONE',  ( 5.049401038298161559, -19.05341960407611168, 82.70724293864770971 ) ) ;
#51330=CARTESIAN_POINT ( 'NONE',  ( 10.81492255796106328, -18.62759615963255655, 55.41775706135234714 ) ) ;
#51331=CARTESIAN_POINT ( 'NONE',  ( 16.51473224551069308, 9.474510206698969483, 99.16557627198102409 ) ) ;
#51332=CARTESIAN_POINT ( 'NONE',  ( -21.55341960407619339, 5.719274019375674811, 103.5427570613523613 ) ) ;
#51333=CARTESIAN_POINT ( 'NONE',  ( -16.52544592524335698, -4.483927247898792601, 83.95942372801900433 ) ) ;
#51334=CARTESIAN_POINT ( 'NONE',  ( -5.823673210054431948, 21.52544592524334988, 22.70942372801901499 ) ) ;
#51335=CARTESIAN_POINT ( 'NONE',  ( -21.53943276465977519, 0.05219959533907696930, 101.2489096053143669 ) ) ;
#51336=CARTESIAN_POINT ( 'NONE',  ( -4.379528057220328563, 16.55341960407611168, 50.20724293864769550 ) ) ;
#51337=CARTESIAN_POINT ( 'NONE',  ( -16.51473224551069308, -9.474510206698971260, 36.66557627198102409 ) ) ;
#51338=CARTESIAN_POINT ( 'NONE',  ( 14.34966873604960469, 8.224510206698951720, 64.16557627198102409 ) ) ;
#51339=CARTESIAN_POINT ( 'NONE',  ( 15.80617190586746368, 15.72974639402197994, 29.37390960531435269 ) ) ;
#51340=CARTESIAN_POINT ( 'NONE',  ( -9.474510206698720793, -16.51473224551083518, 24.58442372801900078 ) ) ;
#51341=CARTESIAN_POINT ( 'NONE',  ( -14.29746914071049879, 8.314922557960819915, 105.8322429386476955 ) ) ;
#51343=CARTESIAN_POINT ( 'NONE',  ( 14.29746914071037800, 8.314922557961029526, 66.66775706135234714 ) ) ;
#51344=CARTESIAN_POINT ( 'NONE',  ( 5.153800228976335163, 19.02544592524342804, 69.79057627198103830 ) ) ;
#51345=CARTESIAN_POINT ( 'NONE',  ( -16.90269667309137347, -6.687378500144563809, 21.20804624429822383 ) ) ;
#51346=CARTESIAN_POINT ( 'NONE',  ( 12.06949235617757843, -12.14591786802309237, 83.12390960531436690 ) ) ;
#51347=CARTESIAN_POINT ( 'NONE',  ( -5.719274019375978568, 21.55341960407610458, 40.20724293864769550 ) ) ;
#51348=CARTESIAN_POINT ( 'NONE',  ( -8.224510206698735004, -14.34966873604973081, 89.58442372801901854 ) ) ;
#51349=CARTESIAN_POINT ( 'NONE',  ( -5.153800228976607833, 19.02544592524334988, 112.7094237280190043 ) ) ;
#51350=CARTESIAN_POINT ( 'NONE',  ( 18.67979575497194134, -10.72451020669871369, 80.83442372801901854 ) ) ;
#51351=CARTESIAN_POINT ( 'NONE',  ( 5.049401038298161559, -19.05341960407611168, 92.70724293864769550 ) ) ;
#51352=CARTESIAN_POINT ( 'NONE',  ( -5.719274019375978568, 21.55341960407610458, 100.2072429386476955 ) ) ;
#51353=CARTESIAN_POINT ( 'NONE',  ( 14.29746914071037800, 8.314922557961029526, 51.66775706135234714 ) ) ;
#51354=CARTESIAN_POINT ( 'NONE',  ( -16.52544592524342804, 4.483927247898546575, 116.0405762719810383 ) ) ;
#51355=CARTESIAN_POINT ( 'NONE',  ( -0.05219959533936034679, 19.03943276465977164, 112.5010903946856757 ) ) ;
#51356=CARTESIAN_POINT ( 'NONE',  ( 9.474510206698729675, 16.51473224551082808, 87.08442372801900433 ) ) ;
#51357=CARTESIAN_POINT ( 'NONE',  ( -21.52544592524343514, 5.823673210054127303, 71.04057627198103830 ) ) ;
#51358=CARTESIAN_POINT ( 'NONE',  ( -5.049401038297874678, -19.05341960407617918, 54.79275706135234003 ) ) ;
#51360=CARTESIAN_POINT ( 'NONE',  ( 5.823673210054125526, 21.52544592524343514, 104.7905762719810241 ) ) ;
#51361=CARTESIAN_POINT ( 'NONE',  ( 17.49999999999998934, 4.013004640162652237, 27.05394279005593461 ) ) ;
#51362=CARTESIAN_POINT ( 'NONE',  ( 9.474510206698971260, -16.51473224551069308, 72.91557627198102409 ) ) ;
#51364=CARTESIAN_POINT ( 'NONE',  ( -16.55341960407617563, 4.379528057220093196, 28.54275706135234358 ) ) ;
#51366=CARTESIAN_POINT ( 'NONE',  ( 10.72451020669898902, -18.67979575497178502, 97.91557627198103830 ) ) ;
#51367=CARTESIAN_POINT ( 'NONE',  ( 12.14591786802309770, 12.06949235617756955, 69.37390960531436690 ) ) ;
#51368=CARTESIAN_POINT ( 'NONE',  ( -16.51473224551069308, -9.474510206698971260, 71.66557627198102409 ) ) ;
#51369=CARTESIAN_POINT ( 'NONE',  ( 15.80617190586769283, -15.72974639402175789, 85.62609039468568994 ) ) ;
#51370=CARTESIAN_POINT ( 'NONE',  ( 16.53943276465976808, 0.05219959533934440121, 36.25109039468567573 ) ) ;
#51371=CARTESIAN_POINT ( 'NONE',  ( -16.46253265017146816, -9.564922557961047289, 39.16775706135234003 ) ) ;
#51372=CARTESIAN_POINT ( 'NONE',  ( -21.53943276465977519, -0.05219959533937600094, 48.75109039468568284 ) ) ;
#51373=CARTESIAN_POINT ( 'NONE',  ( 5.823673210054125526, 21.52544592524343514, 64.79057627198103830 ) ) ;
#51374=CARTESIAN_POINT ( 'NONE',  ( 0.05219959533936267826, -19.03943276465977164, 105.0010903946856615 ) ) ;
#51375=CARTESIAN_POINT ( 'NONE',  ( -9.564922557960796823, -16.46253265017161027, 52.08224293864768839 ) ) ;
#51376=CARTESIAN_POINT ( 'NONE',  ( -19.02544592524334988, -5.153800228976617603, 78.95942372801900433 ) ) ;
#51377=CARTESIAN_POINT ( 'NONE',  ( -10.72451020669870658, -18.67979575497194134, 79.58442372801903275 ) ) ;
#51378=CARTESIAN_POINT ( 'NONE',  ( -9.564922557961040184, 16.46253265017147172, 62.91775706135233293 ) ) ;
#51379=CARTESIAN_POINT ( 'NONE',  ( 13.89961937509977652, -13.97604488694527269, 33.12390960531434558 ) ) ;
#51380=CARTESIAN_POINT ( 'NONE',  ( -21.52544592524343514, 5.823673210054127303, 56.04057627198102409 ) ) ;
#51381=CARTESIAN_POINT ( 'NONE',  ( 8.314922557960818139, 14.29746914071049879, 69.58224293864769550 ) ) ;
#51383=CARTESIAN_POINT ( 'NONE',  ( -5.049401038297874678, -19.05341960407617918, 24.79275706135233648 ) ) ;
#51384=CARTESIAN_POINT ( 'NONE',  ( -16.55341960407617563, 4.379528057220093196, 93.54275706135234714 ) ) ;
#51385=CARTESIAN_POINT ( 'NONE',  ( -8.224510206698948167, 14.34966873604960824, 55.41557627198102409 ) ) ;
#51386=CARTESIAN_POINT ( 'NONE',  ( -21.55341960407619339, 5.719274019375674811, 88.54275706135236135 ) ) ;
#51387=CARTESIAN_POINT ( 'NONE',  ( -10.81492255796105439, 18.62759615963255655, 82.91775706135234714 ) ) ;
#51388=CARTESIAN_POINT ( 'NONE',  ( -5.823673210054116645, -21.52544592524344225, 97.29057627198105251 ) ) ;
#51389=CARTESIAN_POINT ( 'NONE',  ( 19.02544592524343514, -5.153800228976328945, 53.54057627198102409 ) ) ;
#51390=CARTESIAN_POINT ( 'NONE',  ( -21.55341960407619339, 5.719274019375674811, 63.54275706135234003 ) ) ;
#51391=CARTESIAN_POINT ( 'NONE',  ( -0.05219959533909027116, -19.03943276465977164, 52.49890960531436690 ) ) ;
#51393=CARTESIAN_POINT ( 'NONE',  ( 9.564922557960805705, 16.46253265017160317, 64.58224293864769550 ) ) ;
#51394=CARTESIAN_POINT ( 'NONE',  ( -16.52544592524342804, 4.483927247898546575, 106.0405762719810525 ) ) ;
#51395=CARTESIAN_POINT ( 'NONE',  ( 5.049401038298161559, -19.05341960407611168, 92.70724293864769550 ) ) ;
#51396=CARTESIAN_POINT ( 'NONE',  ( -8.224510206698948167, 14.34966873604960824, 60.41557627198102409 ) ) ;
#51397=CARTESIAN_POINT ( 'NONE',  ( -9.564922557960796823, -16.46253265017161027, 22.08224293864768839 ) ) ;
#51398=CARTESIAN_POINT ( 'NONE',  ( -21.52544592524343514, 5.823673210054127303, 81.04057627198102409 ) ) ;
#51399=CARTESIAN_POINT ( 'NONE',  ( 21.52544592524334988, 5.823673210054432836, 41.45942372801901143 ) ) ;
#51401=CARTESIAN_POINT ( 'NONE',  ( -14.34966873604972548, 8.224510206698743886, 38.33442372801900433 ) ) ;
#51402=CARTESIAN_POINT ( 'NONE',  ( 0.05219959533907565091, 21.53943276465977519, 84.99890960531436690 ) ) ;
#51403=CARTESIAN_POINT ( 'NONE',  ( -18.67979575497193778, 10.72451020669871902, 108.3344237280190185 ) ) ;
#51404=CARTESIAN_POINT ( 'NONE',  ( -13.97604488694527625, -13.89961937509977652, 96.87390960531433848 ) ) ;
#51405=CARTESIAN_POINT ( 'NONE',  ( 15.80617190586769283, -15.72974639402175789, 30.62609039468567929 ) ) ;
#51406=CARTESIAN_POINT ( 'NONE',  ( 15.80617190586746368, 15.72974639402197994, 34.37390960531435979 ) ) ;
#51407=CARTESIAN_POINT ( 'NONE',  ( 0.05219959533934541429, -16.53943276465976808, 105.0010903946856757 ) ) ;
#51408=CARTESIAN_POINT ( 'NONE',  ( 5.823673210054444382, -21.52544592524334988, 50.20942372801901854 ) ) ;
#51409=CARTESIAN_POINT ( 'NONE',  ( 18.67979575497194134, -10.72451020669871369, 90.83442372801901854 ) ) ;
#51410=CARTESIAN_POINT ( 'NONE',  ( -15.80617190586768217, 15.72974639402176855, 108.1260903946856757 ) ) ;
#51411=CARTESIAN_POINT ( 'NONE',  ( 8.314922557961029526, -14.29746914071037800, 80.41775706135234714 ) ) ;
#51412=CARTESIAN_POINT ( 'NONE',  ( -5.719274019375665041, -21.55341960407619695, 39.79275706135235424 ) ) ;
#51413=CARTESIAN_POINT ( 'NONE',  ( 5.049401038298161559, -19.05341960407611168, 32.70724293864768129 ) ) ;
#51414=CARTESIAN_POINT ( 'NONE',  ( 0.05219959533937995610, -21.53943276465977519, 100.0010903946857042 ) ) ;
#51415=CARTESIAN_POINT ( 'NONE',  ( -0.05219959533909027116, -19.03943276465977164, 112.4989096053143669 ) ) ;
#51416=CARTESIAN_POINT ( 'NONE',  ( -18.62759615963270932, 10.81492255796079327, 105.8322429386476955 ) ) ;
#51417=DIRECTION ( 'NONE',  ( -0.5150380737757255245, 0.000000000000000000, 0.8571673013836856869 ) ) ;
#51418=CARTESIAN_POINT ( 'NONE',  ( -15.80617190586745835, -15.72974639402198527, 66.87390960531436690 ) ) ;
#51419=CARTESIAN_POINT ( 'NONE',  ( 16.53943276465976808, 0.05219959533934440121, 46.25109039468567573 ) ) ;
#51420=CARTESIAN_POINT ( 'NONE',  ( 14.29746914071049879, -8.314922557960816363, 53.33224293864769550 ) ) ;
#51422=CARTESIAN_POINT ( 'NONE',  ( -13.97604488694547697, 13.89961937509957934, 93.12609039468566152 ) ) ;
#51424=CARTESIAN_POINT ( 'NONE',  ( 14.34966873604972726, -8.224510206698740333, 25.83442372801901499 ) ) ;
#51425=CARTESIAN_POINT ( 'NONE',  ( -21.53943276465977519, 0.05219959533907696930, 101.2489096053143669 ) ) ;
#51426=CARTESIAN_POINT ( 'NONE',  ( -18.67979575497178146, -10.72451020669898902, 71.66557627198100988 ) ) ;
#51427=CARTESIAN_POINT ( 'NONE',  ( 13.89961937509977652, -13.97604488694527269, 108.1239096053143669 ) ) ;
#51428=CARTESIAN_POINT ( 'NONE',  ( 16.55341960407618274, -4.379528057220086978, 41.04275706135236135 ) ) ;
#51429=CARTESIAN_POINT ( 'NONE',  ( 19.02544592524343514, -5.153800228976328945, 63.54057627198103830 ) ) ;
#51430=CARTESIAN_POINT ( 'NONE',  ( -10.81492255796105439, 18.62759615963255655, 32.91775706135234714 ) ) ;
#51431=CARTESIAN_POINT ( 'NONE',  ( 13.97604488694548053, -13.89961937509957401, 95.62609039468563310 ) ) ;
#51433=CARTESIAN_POINT ( 'NONE',  ( -19.05341960407611168, -5.049401038298163336, 106.4572429386476955 ) ) ;
#51434=CARTESIAN_POINT ( 'NONE',  ( 5.153800228976335163, 19.02544592524342804, 84.79057627198099567 ) ) ;
#51435=CARTESIAN_POINT ( 'NONE',  ( 21.52544592524344225, -5.823673210054117533, 93.54057627198103830 ) ) ;
#51436=CARTESIAN_POINT ( 'NONE',  ( 9.474510206698971260, -16.51473224551069308, 52.91557627198102409 ) ) ;
#51437=CARTESIAN_POINT ( 'NONE',  ( -17.12812012977024523, -6.668231424566068988, 61.35948759323143520 ) ) ;
#51438=CARTESIAN_POINT ( 'NONE',  ( 14.34966873604960469, 8.224510206698951720, 69.16557627198102409 ) ) ;
#51439=CARTESIAN_POINT ( 'NONE',  ( -5.049401038298153566, 19.05341960407611168, 115.2072429386477097 ) ) ;
#51441=CARTESIAN_POINT ( 'NONE',  ( 18.67979575497178502, 10.72451020669898547, 89.16557627198102409 ) ) ;
#51442=CARTESIAN_POINT ( 'NONE',  ( -19.03943276465977164, -0.05219959533935918106, 48.75109039468566863 ) ) ;
#51443=CARTESIAN_POINT ( 'NONE',  ( 9.564922557960805705, 16.46253265017160317, 114.5822429386476955 ) ) ;
#51445=CARTESIAN_POINT ( 'NONE',  ( 15.72974639402199770, -15.80617190586745480, 53.12390960531436690 ) ) ;
#51446=CARTESIAN_POINT ( 'NONE',  ( -16.46253265017160317, 9.564922557960807481, 80.83224293864769550 ) ) ;
#51447=CARTESIAN_POINT ( 'NONE',  ( 0.05219959533937995610, -21.53943276465977519, 85.00109039468568994 ) ) ;
#51448=CARTESIAN_POINT ( 'NONE',  ( 13.89961937509977652, -13.97604488694527269, 43.12390960531434558 ) ) ;
#51449=CARTESIAN_POINT ( 'NONE',  ( -0.05219959533910754901, -16.53943276465976808, 77.49890960531433848 ) ) ;
#51450=CARTESIAN_POINT ( 'NONE',  ( -12.14591786802326823, 12.06949235617739902, 23.12609039468567573 ) ) ;
#51451=CARTESIAN_POINT ( 'NONE',  ( 15.72974639402176855, 15.80617190586768217, 66.87609039468568994 ) ) ;
#51453=CARTESIAN_POINT ( 'NONE',  ( -16.46253265017146816, -9.564922557961047289, 29.16775706135232937 ) ) ;
#51454=CARTESIAN_POINT ( 'NONE',  ( -5.153800228976607833, 19.02544592524334988, 77.70942372801900433 ) ) ;
#51456=CARTESIAN_POINT ( 'NONE',  ( -10.72451020669870658, -18.67979575497194134, 29.58442372801901854 ) ) ;
#51457=LINE ( 'NONE', #191962, #117329 ) ;
#51458=CARTESIAN_POINT ( 'NONE',  ( -10.72451020669870658, -18.67979575497194134, 109.5844237280190328 ) ) ;
#51459=CARTESIAN_POINT ( 'NONE',  ( 5.049401038298161559, -19.05341960407611168, 52.70724293864767418 ) ) ;
#51460=CARTESIAN_POINT ( 'NONE',  ( -0.05219959533936034679, 19.03943276465977164, 27.50109039468566507 ) ) ;
#51461=CARTESIAN_POINT ( 'NONE',  ( 12.06949235617739724, 12.14591786802326823, 101.8760903946857042 ) ) ;
#51462=CARTESIAN_POINT ( 'NONE',  ( 13.97604488694527802, 13.89961937509977652, 104.3739096053143385 ) ) ;
#51463=CARTESIAN_POINT ( 'NONE',  ( -5.823673210054431948, 21.52544592524334988, 67.70942372801901854 ) ) ;
#51467=CARTESIAN_POINT ( 'NONE',  ( 5.823673210054444382, -21.52544592524334988, 85.20942372801901854 ) ) ;
#51468=CARTESIAN_POINT ( 'NONE',  ( -21.52544592524334988, -5.823673210054445271, 103.9594237280190185 ) ) ;
#51470=CARTESIAN_POINT ( 'NONE',  ( 13.97604488694527802, 13.89961937509977652, 94.37390960531436690 ) ) ;
#51471=CARTESIAN_POINT ( 'NONE',  ( -16.46253265017146816, -9.564922557961047289, 19.16775706135233293 ) ) ;
#51473=CARTESIAN_POINT ( 'NONE',  ( -0.05219959533909027116, -19.03943276465977164, 42.49890960531435269 ) ) ;
#51474=CARTESIAN_POINT ( 'NONE',  ( 15.72974639402199770, -15.80617190586745480, 53.12390960531436690 ) ) ;
#51475=CARTESIAN_POINT ( 'NONE',  ( -8.224510206698948167, 14.34966873604960824, 25.41557627198103120 ) ) ;
#51476=CARTESIAN_POINT ( 'NONE',  ( 16.53943276465976808, -0.05219959533910856209, 98.74890960531438111 ) ) ;
#51477=CARTESIAN_POINT ( 'NONE',  ( -19.03943276465977164, 0.05219959533909376836, 86.24890960531436690 ) ) ;
#51478=CARTESIAN_POINT ( 'NONE',  ( 0.05219959533937995610, -21.53943276465977519, 105.0010903946856757 ) ) ;
#51479=CARTESIAN_POINT ( 'NONE',  ( 0.05219959533909260263, 19.03943276465977164, 39.99890960531436690 ) ) ;
#51480=CARTESIAN_POINT ( 'NONE',  ( 16.55341960407611168, 4.379528057220329451, 98.95724293864770971 ) ) ;
#51481=CARTESIAN_POINT ( 'NONE',  ( 18.62759615963255655, 10.81492255796105972, 61.66775706135235424 ) ) ;
#51482=CARTESIAN_POINT ( 'NONE',  ( 10.81492255796078972, 18.62759615963270932, 84.58224293864769550 ) ) ;
#51483=CARTESIAN_POINT ( 'NONE',  ( -16.51473224551082808, 9.474510206698731452, 53.33442372801900433 ) ) ;
#51485=CARTESIAN_POINT ( 'NONE',  ( 13.97604488694527802, 13.89961937509977652, 104.3739096053143385 ) ) ;
#51486=CARTESIAN_POINT ( 'NONE',  ( 8.224510206698953496, -14.34966873604960469, 77.91557627198102409 ) ) ;
#51487=CARTESIAN_POINT ( 'NONE',  ( -9.474510206698720793, -16.51473224551083518, 44.58442372801900433 ) ) ;
#51488=CARTESIAN_POINT ( 'NONE',  ( 5.153800228976335163, 19.02544592524342804, 59.79057627198100988 ) ) ;
#51490=CARTESIAN_POINT ( 'NONE',  ( 8.224510206698953496, -14.34966873604960469, 57.91557627198103120 ) ) ;
#51491=CARTESIAN_POINT ( 'NONE',  ( -9.564922557961040184, 16.46253265017147172, 77.91775706135234714 ) ) ;
#51492=CARTESIAN_POINT ( 'NONE',  ( 18.22780087662122384, -5.500000000000022204, 91.01540105326107266 ) ) ;
#51493=CARTESIAN_POINT ( 'NONE',  ( -5.823673210054116645, -21.52544592524344225, 32.29057627198102409 ) ) ;
#51495=CARTESIAN_POINT ( 'NONE',  ( 0.05219959533910956823, 16.53943276465976808, 94.99890960531436690 ) ) ;
#51497=CARTESIAN_POINT ( 'NONE',  ( -5.153800228976328057, -19.02544592524343514, 57.29057627198103120 ) ) ;
#51498=CARTESIAN_POINT ( 'NONE',  ( -18.62759615963270932, 10.81492255796079327, 65.83224293864769550 ) ) ;
#51499=CARTESIAN_POINT ( 'NONE',  ( 5.049401038298161559, -19.05341960407611168, 27.70724293864769550 ) ) ;
#51500=CARTESIAN_POINT ( 'NONE',  ( 14.34966873604972726, -8.224510206698740333, 75.83442372801900433 ) ) ;
#51501=CARTESIAN_POINT ( 'NONE',  ( 5.049401038298161559, -19.05341960407611168, 57.70724293864769550 ) ) ;
#51502=CARTESIAN_POINT ( 'NONE',  ( -19.02544592524334988, -5.153800228976617603, 58.95942372801900433 ) ) ;
#51503=CARTESIAN_POINT ( 'NONE',  ( 0.05219959533937995610, -21.53943276465977519, 70.00109039468568994 ) ) ;
#51504=CARTESIAN_POINT ( 'NONE',  ( 18.67979575497178502, 10.72451020669898547, 49.16557627198102409 ) ) ;
#51505=CARTESIAN_POINT ( 'NONE',  ( 4.483927247898545687, 16.52544592524342804, 114.7905762719810383 ) ) ;
#51506=CARTESIAN_POINT ( 'NONE',  ( -0.05219959533934338120, 16.53943276465976808, 92.50109039468567573 ) ) ;
#51507=CARTESIAN_POINT ( 'NONE',  ( 13.97604488694548053, -13.89961937509957401, 100.6260903946856615 ) ) ;
#51508=CARTESIAN_POINT ( 'NONE',  ( -15.49999999999999822, -5.500000000000000888, 22.00000000000000711 ) ) ;
#51509=CARTESIAN_POINT ( 'NONE',  ( 16.52216118717208104, 7.221426719304520958, 53.57599021046992505 ) ) ;
#51510=CARTESIAN_POINT ( 'NONE',  ( -5.823673210054431948, 21.52544592524334988, 102.7094237280190185 ) ) ;
#51511=CARTESIAN_POINT ( 'NONE',  ( 4.379528057220339221, -16.55341960407611168, 42.70724293864770260 ) ) ;
#51512=CARTESIAN_POINT ( 'NONE',  ( -14.34966873604960291, -8.224510206698953496, 61.66557627198103120 ) ) ;
#51513=CARTESIAN_POINT ( 'NONE',  ( -18.67979575497178146, -10.72451020669898902, 91.66557627198103830 ) ) ;
#51514=CARTESIAN_POINT ( 'NONE',  ( 5.823673210054125526, 21.52544592524343514, 89.79057627198103830 ) ) ;
#51516=CARTESIAN_POINT ( 'NONE',  ( 21.53943276465977519, -0.05219959533907433946, 28.74890960531435624 ) ) ;
#51517=CARTESIAN_POINT ( 'NONE',  ( -4.483927247898782831, 16.52544592524335698, 72.70942372801901854 ) ) ;
#51518=CARTESIAN_POINT ( 'NONE',  ( -16.53943276465976808, 0.05219959533911058130, 76.24890960531435269 ) ) ;
#51519=CARTESIAN_POINT ( 'NONE',  ( -16.46253265017160317, 9.564922557960807481, 50.83224293864770260 ) ) ;
#51522=CARTESIAN_POINT ( 'NONE',  ( -4.483927247898782831, 16.52544592524335698, 97.70942372801904696 ) ) ;
#51523=CARTESIAN_POINT ( 'NONE',  ( 21.52544592524334988, 5.823673210054432836, 26.45942372801901854 ) ) ;
#51524=CARTESIAN_POINT ( 'NONE',  ( 0.05219959533909260263, 19.03943276465977164, 84.99890960531436690 ) ) ;
#51525=CARTESIAN_POINT ( 'NONE',  ( -5.719274019375665041, -21.55341960407619695, 49.79275706135234714 ) ) ;
#51526=CARTESIAN_POINT ( 'NONE',  ( 5.153800228976335163, 19.02544592524342804, 114.7905762719810241 ) ) ;
#51528=EDGE_LOOP ( 'NONE', ( #52381, #44726, #70373, #76520 ) ) ;
#51529=CARTESIAN_POINT ( 'NONE',  ( -21.52544592524334988, -5.823673210054445271, 48.95942372801902565 ) ) ;
#51530=CARTESIAN_POINT ( 'NONE',  ( -9.564922557960796823, -16.46253265017161027, 42.08224293864769550 ) ) ;
#51531=CARTESIAN_POINT ( 'NONE',  ( -9.564922557960796823, -16.46253265017161027, 22.08224293864768839 ) ) ;
#51532=CARTESIAN_POINT ( 'NONE',  ( 13.89961937509957401, 13.97604488694547697, 56.87609039468564731 ) ) ;
#51533=CARTESIAN_POINT ( 'NONE',  ( -18.62759615963255300, -10.81492255796106328, 34.16775706135234714 ) ) ;
#51534=CARTESIAN_POINT ( 'NONE',  ( -5.153800228976607833, 19.02544592524334988, 52.70942372801900433 ) ) ;
#51535=CARTESIAN_POINT ( 'NONE',  ( -19.05341960407611168, -5.049401038298163336, 21.45724293864768839 ) ) ;
#51536=CARTESIAN_POINT ( 'NONE',  ( 12.06949235617739724, 12.14591786802326823, 96.87609039468568994 ) ) ;
#51537=CARTESIAN_POINT ( 'NONE',  ( -13.97604488694547697, 13.89961937509957934, 58.12609039468566863 ) ) ;
#51538=CARTESIAN_POINT ( 'NONE',  ( 14.29746914071037800, 8.314922557961029526, 111.6677570613523613 ) ) ;
#51540=CARTESIAN_POINT ( 'NONE',  ( -13.97604488694527625, -13.89961937509977652, 86.87390960531436690 ) ) ;
#51541=CARTESIAN_POINT ( 'NONE',  ( 10.72451020669871369, 18.67979575497193778, 87.08442372801901854 ) ) ;
#51542=CARTESIAN_POINT ( 'NONE',  ( -21.53943276465977519, -0.05219959533937600094, 103.7510903946857042 ) ) ;
#51544=CARTESIAN_POINT ( 'NONE',  ( -5.049401038298153566, 19.05341960407611168, 100.2072429386476955 ) ) ;
#51545=CARTESIAN_POINT ( 'NONE',  ( 21.53943276465977519, 0.05219959533937863772, 71.25109039468568994 ) ) ;
#51546=CARTESIAN_POINT ( 'NONE',  ( 12.14591786802327356, -12.06949235617739191, 20.62609039468568639 ) ) ;
#51547=CARTESIAN_POINT ( 'NONE',  ( 9.474510206698971260, -16.51473224551069308, 72.91557627198102409 ) ) ;
#51548=CARTESIAN_POINT ( 'NONE',  ( -10.81492255796078084, -18.62759615963271287, 27.08224293864769550 ) ) ;
#51549=CARTESIAN_POINT ( 'NONE',  ( 9.474510206698971260, -16.51473224551069308, 97.91557627198102409 ) ) ;
#51551=CARTESIAN_POINT ( 'NONE',  ( -13.97604488694527625, -13.89961937509977652, 66.87390960531436690 ) ) ;
#51552=CARTESIAN_POINT ( 'NONE',  ( 8.314922557961029526, -14.29746914071037800, 110.4177570613523756 ) ) ;
#51554=CARTESIAN_POINT ( 'NONE',  ( 13.97604488694548053, -13.89961937509957401, 75.62609039468564731 ) ) ;
#51555=CARTESIAN_POINT ( 'NONE',  ( -16.51473224551069308, -9.474510206698971260, 96.66557627198102409 ) ) ;
#51556=CARTESIAN_POINT ( 'NONE',  ( -14.29746914071049879, 8.314922557960819915, 90.83224293864769550 ) ) ;
#51557=CARTESIAN_POINT ( 'NONE',  ( 15.72974639402199770, -15.80617190586745480, 48.12390960531436690 ) ) ;
#51558=CARTESIAN_POINT ( 'NONE',  ( 5.823673210054125526, 21.52544592524343514, 24.79057627198103120 ) ) ;
#51559=CARTESIAN_POINT ( 'NONE',  ( -4.379528057220328563, 16.55341960407611168, 105.2072429386477097 ) ) ;
#51561=CARTESIAN_POINT ( 'NONE',  ( -13.89961937509957401, -13.97604488694547875, 39.37609039468566152 ) ) ;
#51562=CARTESIAN_POINT ( 'NONE',  ( -16.53943276465976808, 0.05219959533911058130, 26.24890960531435624 ) ) ;
#51563=CARTESIAN_POINT ( 'NONE',  ( -16.51473224551069308, -9.474510206698971260, 101.6655762719810241 ) ) ;
#51564=CARTESIAN_POINT ( 'NONE',  ( 18.67979575497194134, -10.72451020669871369, 70.83442372801901854 ) ) ;
#51565=CARTESIAN_POINT ( 'NONE',  ( -15.80617190586745835, -15.72974639402198527, 61.87390960531436690 ) ) ;
#51566=CARTESIAN_POINT ( 'NONE',  ( -21.53943276465977519, -0.05219959533937600094, 43.75109039468568284 ) ) ;
#51567=CARTESIAN_POINT ( 'NONE',  ( -5.823673210054116645, -21.52544592524344225, 92.29057627198103830 ) ) ;
#51568=CARTESIAN_POINT ( 'NONE',  ( 21.52544592524334988, 5.823673210054432836, 41.45942372801901143 ) ) ;
#51569=CARTESIAN_POINT ( 'NONE',  ( -8.314922557960811034, -14.29746914071050412, 107.0822429386476955 ) ) ;
#51570=CARTESIAN_POINT ( 'NONE',  ( 13.97604488694548053, -13.89961937509957401, 65.62609039468567573 ) ) ;
#51571=CARTESIAN_POINT ( 'NONE',  ( 16.51473224551069308, 9.474510206698969483, 59.16557627198102409 ) ) ;
#51572=CARTESIAN_POINT ( 'NONE',  ( -14.34966873604960291, -8.224510206698953496, 111.6655762719810525 ) ) ;
#51573=CARTESIAN_POINT ( 'NONE',  ( 5.049401038298161559, -19.05341960407611168, 112.7072429386476813 ) ) ;
#51574=CARTESIAN_POINT ( 'NONE',  ( -4.379528057220328563, 16.55341960407611168, 40.20724293864769550 ) ) ;
#51575=CARTESIAN_POINT ( 'NONE',  ( -4.379528057220086978, -16.55341960407618274, 109.7927570613523613 ) ) ;
#51576=CARTESIAN_POINT ( 'NONE',  ( 19.05341960407611168, 5.049401038298154454, 53.95724293864770260 ) ) ;
#51577=CARTESIAN_POINT ( 'NONE',  ( -9.474510206698964154, 16.51473224551069663, 25.41557627198103120 ) ) ;
#51578=CARTESIAN_POINT ( 'NONE',  ( -9.474510206698720793, -16.51473224551083518, 19.58442372801899722 ) ) ;
#51580=CARTESIAN_POINT ( 'NONE',  ( -14.29746914071049879, 8.314922557960819915, 40.83224293864769550 ) ) ;
#51581=CARTESIAN_POINT ( 'NONE',  ( 0.05219959533937995610, -21.53943276465977519, 45.00109039468568284 ) ) ;
#51583=CARTESIAN_POINT ( 'NONE',  ( 0.05219959533934541429, -16.53943276465976808, 60.00109039468568284 ) ) ;
#51584=CARTESIAN_POINT ( 'NONE',  ( 14.29746914071049879, -8.314922557960816363, 28.33224293864769550 ) ) ;
#51585=CARTESIAN_POINT ( 'NONE',  ( -12.14591786802326823, 12.06949235617739902, 103.1260903946856757 ) ) ;
#51586=CARTESIAN_POINT ( 'NONE',  ( -5.153800228976328057, -19.02544592524343514, 32.29057627198102409 ) ) ;
#51587=CARTESIAN_POINT ( 'NONE',  ( -0.05219959533909027116, -19.03943276465977164, 42.49890960531435269 ) ) ;
#51588=CARTESIAN_POINT ( 'NONE',  ( -16.52544592524342804, 4.483927247898546575, 116.0405762719810383 ) ) ;
#51589=CARTESIAN_POINT ( 'NONE',  ( -10.72451020669870658, -18.67979575497194134, 29.58442372801901854 ) ) ;
#51590=CARTESIAN_POINT ( 'NONE',  ( -19.02544592524342804, 5.153800228976336051, 46.04057627198101699 ) ) ;
#51591=CARTESIAN_POINT ( 'NONE',  ( 18.22780087662122384, -5.500000000000022204, 81.01540105326105845 ) ) ;
#51592=CARTESIAN_POINT ( 'NONE',  ( 16.51473224551069308, 9.474510206698969483, 39.16557627198103120 ) ) ;
#51593=CARTESIAN_POINT ( 'NONE',  ( -5.823673210054116645, -21.52544592524344225, 27.29057627198103120 ) ) ;
#51595=CARTESIAN_POINT ( 'NONE',  ( -5.719274019375665041, -21.55341960407619695, 59.79275706135234714 ) ) ;
#51596=CARTESIAN_POINT ( 'NONE',  ( 4.483927247898545687, 16.52544592524342804, 104.7905762719810241 ) ) ;
#51597=CARTESIAN_POINT ( 'NONE',  ( 0.05219959533909260263, 19.03943276465977164, 104.9989096053143669 ) ) ;
#51598=CARTESIAN_POINT ( 'NONE',  ( -4.379528057220086978, -16.55341960407618274, 79.79275706135236135 ) ) ;
#51599=CARTESIAN_POINT ( 'NONE',  ( -15.80617190586768217, 15.72974639402176855, 98.12609039468570415 ) ) ;
#51600=CARTESIAN_POINT ( 'NONE',  ( 4.379528057220092307, 16.55341960407617563, 47.29275706135234003 ) ) ;
#51601=CARTESIAN_POINT ( 'NONE',  ( -16.46253265017160317, 9.564922557960807481, 95.83224293864769550 ) ) ;
#51602=CARTESIAN_POINT ( 'NONE',  ( -12.14591786802326823, 12.06949235617739902, 43.12609039468568284 ) ) ;
#51603=CARTESIAN_POINT ( 'NONE',  ( -14.29746914071037622, -8.314922557961029526, 24.16775706135235424 ) ) ;
#51604=CARTESIAN_POINT ( 'NONE',  ( -14.29746914071037622, -8.314922557961029526, 79.16775706135234714 ) ) ;
#51605=CARTESIAN_POINT ( 'NONE',  ( -13.89961937509957401, -13.97604488694547875, 104.3760903946856757 ) ) ;
#51606=CARTESIAN_POINT ( 'NONE',  ( -19.05341960407611168, -5.049401038298163336, 81.45724293864769550 ) ) ;
#51607=CARTESIAN_POINT ( 'NONE',  ( 0.05219959533907565091, 21.53943276465977519, 94.99890960531436690 ) ) ;
#51608=CARTESIAN_POINT ( 'NONE',  ( -4.483927247898539470, -16.52544592524342804, 107.2905762719810525 ) ) ;
#51609=CARTESIAN_POINT ( 'NONE',  ( -13.97604488694547697, 13.89961937509957934, 108.1260903946856331 ) ) ;
#51610=CARTESIAN_POINT ( 'NONE',  ( 12.06949235617739724, 12.14591786802326823, 71.87609039468568994 ) ) ;
#51611=CARTESIAN_POINT ( 'NONE',  ( -17.05116617787848554, 6.768360034955530402, 43.65675553259193720 ) ) ;
#51612=CARTESIAN_POINT ( 'NONE',  ( -19.03943276465977164, -0.05219959533935918106, 73.75109039468566152 ) ) ;
#51613=CARTESIAN_POINT ( 'NONE',  ( 16.55341960407611168, 4.379528057220329451, 43.95724293864769550 ) ) ;
#51614=CARTESIAN_POINT ( 'NONE',  ( -8.314922557960811034, -14.29746914071050412, 87.08224293864769550 ) ) ;
#51615=CARTESIAN_POINT ( 'NONE',  ( 13.97604488694548053, -13.89961937509957401, 30.62609039468566863 ) ) ;
#51616=CARTESIAN_POINT ( 'NONE',  ( -17.13100169013301155, 6.664070546373155324, 90.76789835699851494 ) ) ;
#51617=CARTESIAN_POINT ( 'NONE',  ( -5.823673210054431948, 21.52544592524334988, 37.70942372801900433 ) ) ;
#51618=CARTESIAN_POINT ( 'NONE',  ( -0.05219959533936034679, 19.03943276465977164, 102.5010903946856757 ) ) ;
#51620=CARTESIAN_POINT ( 'NONE',  ( -5.153800228976328057, -19.02544592524343514, 97.29057627198099567 ) ) ;
#51621=CARTESIAN_POINT ( 'NONE',  ( -5.049401038297874678, -19.05341960407617918, 19.79275706135233293 ) ) ;
#51622=CARTESIAN_POINT ( 'NONE',  ( 19.05341960407611168, 5.049401038298154454, 93.95724293864769550 ) ) ;
#51623=CARTESIAN_POINT ( 'NONE',  ( -5.823673210054116645, -21.52544592524344225, 57.29057627198103120 ) ) ;
#51624=CARTESIAN_POINT ( 'NONE',  ( -12.06949235617756955, 12.14591786802309770, 95.62390960531436690 ) ) ;
#51625=CARTESIAN_POINT ( 'NONE',  ( 5.049401038298161559, -19.05341960407611168, 62.70724293864769550 ) ) ;
#51626=CARTESIAN_POINT ( 'NONE',  ( -4.379528057220328563, 16.55341960407611168, 110.2072429386477239 ) ) ;
#51627=CARTESIAN_POINT ( 'NONE',  ( 18.62759615963255655, 10.81492255796105972, 26.66775706135235424 ) ) ;
#51629=CARTESIAN_POINT ( 'NONE',  ( -21.52544592524334988, -5.823673210054445271, 78.95942372801901854 ) ) ;
#51630=CARTESIAN_POINT ( 'NONE',  ( 19.05341960407611168, 5.049401038298154454, 38.95724293864767418 ) ) ;
#51631=CARTESIAN_POINT ( 'NONE',  ( -4.379528057220086978, -16.55341960407618274, 79.79275706135236135 ) ) ;
#51632=CARTESIAN_POINT ( 'NONE',  ( -21.55341960407619339, 5.719274019375674811, 28.54275706135234358 ) ) ;
#51633=CARTESIAN_POINT ( 'NONE',  ( 5.823673210054444382, -21.52544592524334988, 30.20942372801902565 ) ) ;
#51634=CARTESIAN_POINT ( 'NONE',  ( -9.564922557961040184, 16.46253265017147172, 52.91775706135233293 ) ) ;
#51635=CARTESIAN_POINT ( 'NONE',  ( -5.153800228976328057, -19.02544592524343514, 67.29057627198102409 ) ) ;
#51636=CARTESIAN_POINT ( 'NONE',  ( 19.05341960407617918, -5.049401038297876454, 26.04275706135233293 ) ) ;
#51637=CARTESIAN_POINT ( 'NONE',  ( -21.53943276465977519, -0.05219959533937600094, 88.75109039468567573 ) ) ;
#51638=CARTESIAN_POINT ( 'NONE',  ( 18.67979575497178502, 10.72451020669898547, 64.16557627198102409 ) ) ;
#51639=CARTESIAN_POINT ( 'NONE',  ( -14.34966873604960291, -8.224510206698953496, 56.66557627198103830 ) ) ;
#51640=CARTESIAN_POINT ( 'NONE',  ( 21.55341960407619695, -5.719274019375665929, 91.04275706135236135 ) ) ;
#51641=CARTESIAN_POINT ( 'NONE',  ( -13.97604488694547697, 13.89961937509957934, 23.12609039468565442 ) ) ;
#51642=CARTESIAN_POINT ( 'NONE',  ( -16.52544592524342804, 4.483927247898546575, 71.04057627198103830 ) ) ;
#51643=CARTESIAN_POINT ( 'NONE',  ( 19.03943276465977164, -0.05219959533909143690, 23.74890960531435269 ) ) ;
#51644=CARTESIAN_POINT ( 'NONE',  ( -9.564922557961040184, 16.46253265017147172, 62.91775706135233293 ) ) ;
#51645=CARTESIAN_POINT ( 'NONE',  ( -16.52544592524335698, -4.483927247898792601, 108.9594237280190185 ) ) ;
#51646=CARTESIAN_POINT ( 'NONE',  ( 21.52544592524334988, 5.823673210054432836, 86.45942372801901854 ) ) ;
#51647=CARTESIAN_POINT ( 'NONE',  ( -5.153800228976328057, -19.02544592524343514, 82.29057627198103830 ) ) ;
#51648=CARTESIAN_POINT ( 'NONE',  ( 5.153800228976615827, -19.02544592524334988, 45.20942372801901143 ) ) ;
#51649=CARTESIAN_POINT ( 'NONE',  ( -5.823673210054116645, -21.52544592524344225, 57.29057627198103120 ) ) ;
#51650=CARTESIAN_POINT ( 'NONE',  ( 0.05219959533937995610, -21.53943276465977519, 50.00109039468568994 ) ) ;
#51651=CARTESIAN_POINT ( 'NONE',  ( -21.53943276465977519, 0.05219959533907696930, 101.2489096053143669 ) ) ;
#51652=CARTESIAN_POINT ( 'NONE',  ( -16.51473224551082808, 9.474510206698731452, 93.33442372801900433 ) ) ;
#51653=CARTESIAN_POINT ( 'NONE',  ( 16.55341960407618274, -4.379528057220086978, 61.04275706135234714 ) ) ;
#51654=CARTESIAN_POINT ( 'NONE',  ( -17.97161686093721400, 5.500000000000146549, 55.99637206859166128 ) ) ;
#51655=CARTESIAN_POINT ( 'NONE',  ( 0.05219959533907565091, 21.53943276465977519, 109.9989096053143527 ) ) ;
#51656=CARTESIAN_POINT ( 'NONE',  ( -8.224510206698948167, 14.34966873604960824, 95.41557627198102409 ) ) ;
#51657=CARTESIAN_POINT ( 'NONE',  ( -17.44279575226822132, -5.990770900252460507, 99.16442432485683867 ) ) ;
#51658=CARTESIAN_POINT ( 'NONE',  ( 12.14591786802327356, -12.06949235617739191, 30.62609039468567929 ) ) ;
#51659=CARTESIAN_POINT ( 'NONE',  ( -18.67979575497178146, -10.72451020669898902, 61.66557627198103120 ) ) ;
#51660=CARTESIAN_POINT ( 'NONE',  ( 8.224510206698742110, 14.34966873604972548, 97.08442372801904696 ) ) ;
#51661=CARTESIAN_POINT ( 'NONE',  ( -9.474510206698964154, 16.51473224551069663, 30.41557627198102054 ) ) ;
#51662=CARTESIAN_POINT ( 'NONE',  ( 8.314922557961029526, -14.29746914071037800, 60.41775706135235424 ) ) ;
#51663=CARTESIAN_POINT ( 'NONE',  ( -16.51473224551082808, 9.474510206698731452, 63.33442372801900433 ) ) ;
#51664=CARTESIAN_POINT ( 'NONE',  ( 21.55341960407619695, -5.719274019375665929, 41.04275706135236135 ) ) ;
#51665=CARTESIAN_POINT ( 'NONE',  ( 10.72451020669898902, -18.67979575497178502, 57.91557627198103120 ) ) ;
#51666=CARTESIAN_POINT ( 'NONE',  ( 14.29746914071037800, 8.314922557961029526, 86.66775706135234714 ) ) ;
#51667=CARTESIAN_POINT ( 'NONE',  ( 15.80617190586769283, -15.72974639402175789, 70.62609039468567573 ) ) ;
#51669=CARTESIAN_POINT ( 'NONE',  ( 21.53943276465977519, -0.05219959533907433946, 53.74890960531437401 ) ) ;
#51670=CARTESIAN_POINT ( 'NONE',  ( -21.53943276465977519, 0.05219959533907696930, 36.24890960531435979 ) ) ;
#51672=ORIENTED_EDGE ( 'NONE', *, *, #194116, .T. ) ;
#51673=CARTESIAN_POINT ( 'NONE',  ( -16.55341960407617563, 4.379528057220093196, 63.54275706135234003 ) ) ;
#51674=CARTESIAN_POINT ( 'NONE',  ( 15.72974639402199770, -15.80617190586745480, 28.12390960531435979 ) ) ;
#51676=CARTESIAN_POINT ( 'NONE',  ( -0.05219959533909027116, -19.03943276465977164, 97.49890960531436690 ) ) ;
#51677=CARTESIAN_POINT ( 'NONE',  ( -4.483927247898539470, -16.52544592524342804, 22.29057627198102765 ) ) ;
#51679=CARTESIAN_POINT ( 'NONE',  ( -0.05219959533910754901, -16.53943276465976808, 112.4989096053143669 ) ) ;
#51680=CARTESIAN_POINT ( 'NONE',  ( -10.72451020669898014, 18.67979575497178502, 60.41557627198102409 ) ) ;
#51681=CARTESIAN_POINT ( 'NONE',  ( -5.049401038298153566, 19.05341960407611168, 40.20724293864768839 ) ) ;
#51682=CARTESIAN_POINT ( 'NONE',  ( -12.06949235617739369, -12.14591786802326823, 84.37609039468570415 ) ) ;
#51683=CARTESIAN_POINT ( 'NONE',  ( 5.719274019375673035, 21.55341960407619339, 37.29275706135235424 ) ) ;
#51684=CARTESIAN_POINT ( 'NONE',  ( -13.89961937509957401, -13.97604488694547875, 104.3760903946856757 ) ) ;
#51685=CARTESIAN_POINT ( 'NONE',  ( -4.379528057220328563, 16.55341960407611168, 100.2072429386476955 ) ) ;
#51686=CARTESIAN_POINT ( 'NONE',  ( 0.05219959533909260263, 19.03943276465977164, 59.99890960531436690 ) ) ;
#51687=CARTESIAN_POINT ( 'NONE',  ( -5.153800228976328057, -19.02544592524343514, 22.29057627198102765 ) ) ;
#51689=CARTESIAN_POINT ( 'NONE',  ( -16.46253265017160317, 9.564922557960807481, 85.83224293864769550 ) ) ;
#51690=CARTESIAN_POINT ( 'NONE',  ( 12.06949235617739724, 12.14591786802326823, 81.87609039468568994 ) ) ;
#51691=CARTESIAN_POINT ( 'NONE',  ( -21.52544592524334988, -5.823673210054445271, 108.9594237280190185 ) ) ;
#51692=CARTESIAN_POINT ( 'NONE',  ( 21.53943276465977519, -0.05219959533907433946, 53.74890960531437401 ) ) ;
#51693=CARTESIAN_POINT ( 'NONE',  ( -12.06949235617739369, -12.14591786802326823, 74.37609039468568994 ) ) ;
#51694=CARTESIAN_POINT ( 'NONE',  ( -5.153800228976607833, 19.02544592524334988, 77.70942372801900433 ) ) ;
#51695=CARTESIAN_POINT ( 'NONE',  ( 13.89961937509977652, -13.97604488694527269, 43.12390960531434558 ) ) ;
#51696=CARTESIAN_POINT ( 'NONE',  ( 0.05219959533909260263, 19.03943276465977164, 74.99890960531435269 ) ) ;
#51697=CARTESIAN_POINT ( 'NONE',  ( 16.51473224551069308, 9.474510206698969483, 39.16557627198103120 ) ) ;
#51698=CARTESIAN_POINT ( 'NONE',  ( -9.474510206698720793, -16.51473224551083518, 69.58442372801901854 ) ) ;
#51699=CARTESIAN_POINT ( 'NONE',  ( 9.564922557960805705, 16.46253265017160317, 114.5822429386476955 ) ) ;
#51700=CARTESIAN_POINT ( 'NONE',  ( 5.153800228976335163, 19.02544592524342804, 94.79057627198103830 ) ) ;
#51701=CARTESIAN_POINT ( 'NONE',  ( -12.14591786802309592, -12.06949235617757132, 56.87390960531436690 ) ) ;
#51702=CARTESIAN_POINT ( 'NONE',  ( 21.53943276465977519, -0.05219959533907433946, 43.74890960531435979 ) ) ;
#51703=DIRECTION ( 'NONE',  ( 0.000000000000000000, 0.000000000000000000, 1.000000000000000000 ) ) ;
#51704=CARTESIAN_POINT ( 'NONE',  ( 19.02544592524334988, 5.153800228976608722, 31.45942372801900433 ) ) ;
#51705=CARTESIAN_POINT ( 'NONE',  ( -17.49999999999999645, -5.624438216177581218, 79.18329655085355512 ) ) ;
#51706=CARTESIAN_POINT ( 'NONE',  ( -5.153800228976328057, -19.02544592524343514, 52.29057627198100988 ) ) ;
#51707=CARTESIAN_POINT ( 'NONE',  ( 8.314922557961029526, -14.29746914071037800, 40.41775706135234714 ) ) ;
#51710=CARTESIAN_POINT ( 'NONE',  ( -12.14591786802326823, 12.06949235617739902, 78.12609039468570415 ) ) ;
#51711=CARTESIAN_POINT ( 'NONE',  ( 0.05219959533907565091, 21.53943276465977519, 99.99890960531436690 ) ) ;
#51712=CARTESIAN_POINT ( 'NONE',  ( -8.224510206698735004, -14.34966873604973081, 39.58442372801901143 ) ) ;
#51713=CARTESIAN_POINT ( 'NONE',  ( -16.51473224551069308, -9.474510206698971260, 46.66557627198102409 ) ) ;
#51715=CARTESIAN_POINT ( 'NONE',  ( -18.67979575497193778, 10.72451020669871902, 43.33442372801901143 ) ) ;
#51716=CARTESIAN_POINT ( 'NONE',  ( -19.02544592524334988, -5.153800228976617603, 63.95942372801899012 ) ) ;
#51717=CARTESIAN_POINT ( 'NONE',  ( 5.823673210054444382, -21.52544592524334988, 100.2094237280190043 ) ) ;
#51719=CARTESIAN_POINT ( 'NONE',  ( 12.14591786802309770, 12.06949235617756955, 39.37390960531436690 ) ) ;
#51720=CARTESIAN_POINT ( 'NONE',  ( 18.89770734986050726, 5.499999999999904077, 41.60214472496639360 ) ) ;
#51721=CARTESIAN_POINT ( 'NONE',  ( 18.62759615963271287, -10.81492255796078972, 58.33224293864768839 ) ) ;
#51723=CARTESIAN_POINT ( 'NONE',  ( 5.153800228976335163, 19.02544592524342804, 109.7905762719810099 ) ) ;
#51724=CARTESIAN_POINT ( 'NONE',  ( 4.379528057220339221, -16.55341960407611168, 102.7072429386476955 ) ) ;
#51725=CARTESIAN_POINT ( 'NONE',  ( 8.224510206698742110, 14.34966873604972548, 27.08442372801901854 ) ) ;
#51726=CARTESIAN_POINT ( 'NONE',  ( -0.05219959533934338120, 16.53943276465976808, 112.5010903946857042 ) ) ;
#51727=ORIENTED_EDGE ( 'NONE', *, *, #26464, .F. ) ;
#51728=CARTESIAN_POINT ( 'NONE',  ( -19.05341960407611168, -5.049401038298163336, 101.4572429386476955 ) ) ;
#51729=CARTESIAN_POINT ( 'NONE',  ( 15.72974639402199770, -15.80617190586745480, 108.1239096053143811 ) ) ;
#51730=CARTESIAN_POINT ( 'NONE',  ( -16.55341960407611168, -4.379528057220339221, 26.45724293864768839 ) ) ;
#51731=CARTESIAN_POINT ( 'NONE',  ( -16.51473224551069308, -9.474510206698971260, 111.6655762719810383 ) ) ;
#51732=CARTESIAN_POINT ( 'NONE',  ( 5.049401038297881783, 19.05341960407617563, 97.29275706135233293 ) ) ;
#51733=CARTESIAN_POINT ( 'NONE',  ( 15.72974639402176855, 15.80617190586768217, 101.8760903946857042 ) ) ;
#51734=CARTESIAN_POINT ( 'NONE',  ( -8.314922557960811034, -14.29746914071050412, 32.08224293864769550 ) ) ;
#51735=CARTESIAN_POINT ( 'NONE',  ( -18.62759615963270932, 10.81492255796079327, 85.83224293864768129 ) ) ;
#51736=CARTESIAN_POINT ( 'NONE',  ( 21.55341960407610458, 5.719274019375980345, 53.95724293864770260 ) ) ;
#51737=CARTESIAN_POINT ( 'NONE',  ( 13.97604488694527802, 13.89961937509977652, 64.37390960531436690 ) ) ;
#51738=CARTESIAN_POINT ( 'NONE',  ( 8.314922557960818139, 14.29746914071049879, 39.58224293864769550 ) ) ;
#51739=CARTESIAN_POINT ( 'NONE',  ( -19.02544592524342804, 5.153800228976336051, 76.04057627198102409 ) ) ;
#51741=CARTESIAN_POINT ( 'NONE',  ( 18.56101223717331905, 5.499999999999942268, 58.94978406935675252 ) ) ;
#51742=CARTESIAN_POINT ( 'NONE',  ( -19.03943276465977164, -0.05219959533935918106, 38.75109039468566152 ) ) ;
#51743=CARTESIAN_POINT ( 'NONE',  ( -18.62759615963270932, 10.81492255796079327, 85.83224293864768129 ) ) ;
#51744=CARTESIAN_POINT ( 'NONE',  ( 8.314922557960818139, 14.29746914071049879, 89.58224293864768129 ) ) ;
#51745=CARTESIAN_POINT ( 'NONE',  ( -21.52544592524334988, -5.823673210054445271, 38.95942372801901854 ) ) ;
#51747=CARTESIAN_POINT ( 'NONE',  ( 16.55341960407618274, -4.379528057220086978, 101.0427570613523756 ) ) ;
#51748=CARTESIAN_POINT ( 'NONE',  ( -16.46253265017160317, 9.564922557960807481, 25.83224293864769194 ) ) ;
#51749=CARTESIAN_POINT ( 'NONE',  ( -19.03943276465977164, 0.05219959533909376836, 86.24890960531436690 ) ) ;
#51751=CARTESIAN_POINT ( 'NONE',  ( 14.34966873604960469, 8.224510206698951720, 49.16557627198102409 ) ) ;
#51752=CARTESIAN_POINT ( 'NONE',  ( 15.80617190586769283, -15.72974639402175789, 60.62609039468567573 ) ) ;
#51754=CARTESIAN_POINT ( 'NONE',  ( 16.46253265017160672, -9.564922557960803928, 38.33224293864768839 ) ) ;
#51755=CARTESIAN_POINT ( 'NONE',  ( -0.05219959533909027116, -19.03943276465977164, 47.49890960531435979 ) ) ;
#51757=CARTESIAN_POINT ( 'NONE',  ( -15.80617190586768217, 15.72974639402176855, 103.1260903946856757 ) ) ;
#51758=CARTESIAN_POINT ( 'NONE',  ( 12.06949235617739724, 12.14591786802326823, 66.87609039468568994 ) ) ;
#51759=CARTESIAN_POINT ( 'NONE',  ( -21.52544592524334988, -5.823673210054445271, 83.95942372801900433 ) ) ;
#51760=CARTESIAN_POINT ( 'NONE',  ( -15.80617190586745835, -15.72974639402198527, 21.87390960531436690 ) ) ;
#51761=CARTESIAN_POINT ( 'NONE',  ( -13.97604488694547697, 13.89961937509957934, 93.12609039468566152 ) ) ;
#51762=CARTESIAN_POINT ( 'NONE',  ( 15.80617190586769283, -15.72974639402175789, 75.62609039468567573 ) ) ;
#51763=CARTESIAN_POINT ( 'NONE',  ( 14.34966873604972726, -8.224510206698740333, 30.83442372801902209 ) ) ;
#51764=CARTESIAN_POINT ( 'NONE',  ( 5.719274019375991003, -21.55341960407610458, 92.70724293864770971 ) ) ;
#51765=CARTESIAN_POINT ( 'NONE',  ( -19.03943276465977164, -0.05219959533935918106, 103.7510903946856757 ) ) ;
#51766=CARTESIAN_POINT ( 'NONE',  ( 19.02544592524343514, -5.153800228976328945, 63.54057627198103830 ) ) ;
#51767=CARTESIAN_POINT ( 'NONE',  ( 13.97604488694548053, -13.89961937509957401, 105.6260903946856757 ) ) ;
#51769=CARTESIAN_POINT ( 'NONE',  ( -19.05341960407617563, 5.049401038297882671, 98.54275706135233293 ) ) ;
#51770=CARTESIAN_POINT ( 'NONE',  ( -0.05219959533910754901, -16.53943276465976808, 47.49890960531435979 ) ) ;
#51771=CARTESIAN_POINT ( 'NONE',  ( 19.05341960407617918, -5.049401038297876454, 76.04275706135230450 ) ) ;
#51772=CARTESIAN_POINT ( 'NONE',  ( -4.379528057220086978, -16.55341960407618274, 74.79275706135234714 ) ) ;
#51773=CARTESIAN_POINT ( 'NONE',  ( 10.81492255796078972, 18.62759615963270932, 114.5822429386477097 ) ) ;
#51774=CARTESIAN_POINT ( 'NONE',  ( -19.05341960407611168, -5.049401038298163336, 41.45724293864769550 ) ) ;
#51775=CARTESIAN_POINT ( 'NONE',  ( -9.564922557960796823, -16.46253265017161027, 62.08224293864769550 ) ) ;
#51776=CARTESIAN_POINT ( 'NONE',  ( -8.314922557961024197, 14.29746914071037800, 72.91775706135234714 ) ) ;
#51779=CARTESIAN_POINT ( 'NONE',  ( -9.474510206698964154, 16.51473224551069663, 105.4155762719810383 ) ) ;
#51782=CARTESIAN_POINT ( 'NONE',  ( 9.474510206698729675, 16.51473224551082808, 112.0844237280190043 ) ) ;
#51783=CARTESIAN_POINT ( 'NONE',  ( -18.62759615963270932, 10.81492255796079327, 55.83224293864770260 ) ) ;
#51784=CARTESIAN_POINT ( 'NONE',  ( 16.51473224551083163, -9.474510206698727899, 45.83442372801900433 ) ) ;
#51785=CARTESIAN_POINT ( 'NONE',  ( -12.14591786802326823, 12.06949235617739902, 28.12609039468568284 ) ) ;
#51786=CARTESIAN_POINT ( 'NONE',  ( 19.03943276465977164, -0.05219959533909143690, 33.74890960531435979 ) ) ;
#51787=CARTESIAN_POINT ( 'NONE',  ( 19.02544592524343514, -5.153800228976328945, 53.54057627198102409 ) ) ;
#51788=CARTESIAN_POINT ( 'NONE',  ( 18.67979575497178502, 10.72451020669898547, 89.16557627198102409 ) ) ;
#51789=CARTESIAN_POINT ( 'NONE',  ( -19.02544592524342804, 5.153800228976336051, 106.0405762719810241 ) ) ;
#51791=CARTESIAN_POINT ( 'NONE',  ( 19.02544592524343514, -5.153800228976328945, 53.54057627198102409 ) ) ;
#51792=LINE ( 'NONE', #111477, #188855 ) ;
#51793=CARTESIAN_POINT ( 'NONE',  ( -16.51473224551082808, 9.474510206698731452, 103.3344237280190043 ) ) ;
#51794=CARTESIAN_POINT ( 'NONE',  ( -16.53943276465976808, 0.05219959533911058130, 66.24890960531436690 ) ) ;
#51795=CARTESIAN_POINT ( 'NONE',  ( 5.823673210054444382, -21.52544592524334988, 105.2094237280190328 ) ) ;
#51796=CARTESIAN_POINT ( 'NONE',  ( -0.05219959533907301413, -21.53943276465977519, 92.49890960531436690 ) ) ;
#51797=CARTESIAN_POINT ( 'NONE',  ( -15.72974639402176322, -15.80617190586768395, 84.37609039468570415 ) ) ;
#51798=CARTESIAN_POINT ( 'NONE',  ( 5.049401038298161559, -19.05341960407611168, 22.70724293864769194 ) ) ;
#51799=CARTESIAN_POINT ( 'NONE',  ( -10.81492255796105439, 18.62759615963255655, 77.91775706135231871 ) ) ;
#51800=CARTESIAN_POINT ( 'NONE',  ( 16.51473224551069308, 9.474510206698969483, 104.1655762719810241 ) ) ;
#51801=CARTESIAN_POINT ( 'NONE',  ( 4.483927247898545687, 16.52544592524342804, 24.79057627198103120 ) ) ;
#51802=CARTESIAN_POINT ( 'NONE',  ( 5.719274019375673035, 21.55341960407619339, 72.29275706135236135 ) ) ;
#51803=CARTESIAN_POINT ( 'NONE',  ( 9.564922557960805705, 16.46253265017160317, 64.58224293864769550 ) ) ;
#51804=CARTESIAN_POINT ( 'NONE',  ( -10.81492255796105439, 18.62759615963255655, 47.91775706135234714 ) ) ;
#51805=CARTESIAN_POINT ( 'NONE',  ( 13.97604488694527802, 13.89961937509977652, 79.37390960531435269 ) ) ;
#51806=CARTESIAN_POINT ( 'NONE',  ( -12.14591786802309592, -12.06949235617757132, 91.87390960531436690 ) ) ;
#51807=CARTESIAN_POINT ( 'NONE',  ( 8.224510206698953496, -14.34966873604960469, 62.91557627198102409 ) ) ;
#51808=CARTESIAN_POINT ( 'NONE',  ( -5.719274019375978568, 21.55341960407610458, 75.20724293864769550 ) ) ;
#51809=CARTESIAN_POINT ( 'NONE',  ( 19.05341960407611168, 5.049401038298154454, 63.95724293864769550 ) ) ;
#51810=CARTESIAN_POINT ( 'NONE',  ( 15.80617190586746368, 15.72974639402197994, 74.37390960531436690 ) ) ;
#51811=CARTESIAN_POINT ( 'NONE',  ( 19.02544592524334988, 5.153800228976608722, 66.45942372801899012 ) ) ;
#51812=CARTESIAN_POINT ( 'NONE',  ( 19.03943276465977164, 0.05219959533936151252, 31.25109039468566863 ) ) ;
#51813=CARTESIAN_POINT ( 'NONE',  ( 4.379528057220339221, -16.55341960407611168, 77.70724293864770971 ) ) ;
#51814=CARTESIAN_POINT ( 'NONE',  ( -15.80617190586745835, -15.72974639402198527, 46.87390960531435979 ) ) ;
#51815=CARTESIAN_POINT ( 'NONE',  ( 17.26172910966779384, 6.454744622555852906, 101.6935309135077716 ) ) ;
#51816=CARTESIAN_POINT ( 'NONE',  ( -4.483927247898782831, 16.52544592524335698, 97.70942372801904696 ) ) ;
#51818=CARTESIAN_POINT ( 'NONE',  ( -13.89961937509957401, -13.97604488694547875, 99.37609039468567573 ) ) ;
#51819=CARTESIAN_POINT ( 'NONE',  ( -14.34966873604960291, -8.224510206698953496, 71.66557627198100988 ) ) ;
#51821=CARTESIAN_POINT ( 'NONE',  ( -13.89961937509977652, 13.97604488694528158, 65.62390960531436690 ) ) ;
#51822=CARTESIAN_POINT ( 'NONE',  ( -4.379528057220328563, 16.55341960407611168, 55.20724293864770260 ) ) ;
#51823=CARTESIAN_POINT ( 'NONE',  ( 16.51473224551069308, 9.474510206698969483, 104.1655762719810241 ) ) ;
#51824=CARTESIAN_POINT ( 'NONE',  ( 13.89961937509957401, 13.97604488694547697, 71.87609039468567573 ) ) ;
#51825=CARTESIAN_POINT ( 'NONE',  ( -16.46253265017160317, 9.564922557960807481, 65.83224293864769550 ) ) ;
#51826=CARTESIAN_POINT ( 'NONE',  ( -19.02544592524342804, 5.153800228976336051, 91.04057627198100988 ) ) ;
#51828=CARTESIAN_POINT ( 'NONE',  ( 13.89961937509977652, -13.97604488694527269, 68.12390960531436690 ) ) ;
#51829=CARTESIAN_POINT ( 'NONE',  ( 10.72451020669898902, -18.67979575497178502, 67.91557627198102409 ) ) ;
#51830=CARTESIAN_POINT ( 'NONE',  ( 12.06949235617739724, 12.14591786802326823, 61.87609039468568284 ) ) ;
#51831=CARTESIAN_POINT ( 'NONE',  ( 17.97214573761834089, 5.499999999999959144, 98.96970049038660022 ) ) ;
#51832=CARTESIAN_POINT ( 'NONE',  ( 19.02544592524343514, -5.153800228976328945, 48.54057627198103120 ) ) ;
#51833=CARTESIAN_POINT ( 'NONE',  ( 18.62759615963271287, -10.81492255796078972, 48.33224293864770260 ) ) ;
#51834=CARTESIAN_POINT ( 'NONE',  ( -16.51473224551082808, 9.474510206698731452, 78.33442372801900433 ) ) ;
#51835=CARTESIAN_POINT ( 'NONE',  ( 16.55341960407611168, 4.379528057220329451, 28.95724293864769905 ) ) ;
#51836=CARTESIAN_POINT ( 'NONE',  ( -21.55341960407619339, 5.719274019375674811, 38.54275706135234714 ) ) ;
#51837=CARTESIAN_POINT ( 'NONE',  ( 19.05341960407617918, -5.049401038297876454, 31.04275706135232227 ) ) ;
#51838=CARTESIAN_POINT ( 'NONE',  ( -4.483927247898782831, 16.52544592524335698, 62.70942372801902565 ) ) ;
#51839=CARTESIAN_POINT ( 'NONE',  ( 12.06949235617739724, 12.14591786802326823, 96.87609039468568994 ) ) ;
#51840=CARTESIAN_POINT ( 'NONE',  ( 19.01533133064921088, -5.499999999999425349, 41.26586590595739068 ) ) ;
#51841=CARTESIAN_POINT ( 'NONE',  ( -8.314922557961024197, 14.29746914071037800, 82.91775706135234714 ) ) ;
#51842=CARTESIAN_POINT ( 'NONE',  ( 15.80617190586746368, 15.72974639402197994, 24.37390960531435979 ) ) ;
#51843=CARTESIAN_POINT ( 'NONE',  ( -14.34966873604972548, 8.224510206698743886, 38.33442372801900433 ) ) ;
#51844=CARTESIAN_POINT ( 'NONE',  ( -19.02544592524342804, 5.153800228976336051, 51.04057627198103120 ) ) ;
#51845=CARTESIAN_POINT ( 'NONE',  ( 13.89961937509977652, -13.97604488694527269, 53.12390960531434558 ) ) ;
#51846=CARTESIAN_POINT ( 'NONE',  ( 19.02544592524343514, -5.153800228976328945, 63.54057627198103830 ) ) ;
#51847=CARTESIAN_POINT ( 'NONE',  ( 21.52544592524334988, 5.823673210054432836, 46.45942372801901854 ) ) ;
#51848=CARTESIAN_POINT ( 'NONE',  ( 12.06949235617739724, 12.14591786802326823, 46.87609039468568994 ) ) ;
#51849=CARTESIAN_POINT ( 'NONE',  ( -16.52544592524342804, 4.483927247898546575, 26.04057627198103475 ) ) ;
#51850=CARTESIAN_POINT ( 'NONE',  ( 13.97604488694527802, 13.89961937509977652, 29.37390960531435979 ) ) ;
#51851=CARTESIAN_POINT ( 'NONE',  ( -5.823673210054431948, 21.52544592524334988, 112.7094237280190328 ) ) ;
#51852=CARTESIAN_POINT ( 'NONE',  ( -16.46253265017146816, -9.564922557961047289, 104.1677570613523329 ) ) ;
#51853=CARTESIAN_POINT ( 'NONE',  ( -19.03943276465977164, -0.05219959533935918106, 68.75109039468566152 ) ) ;
#51854=CARTESIAN_POINT ( 'NONE',  ( -8.224510206698948167, 14.34966873604960824, 65.41557627198102409 ) ) ;
#51855=CARTESIAN_POINT ( 'NONE',  ( -9.564922557960796823, -16.46253265017161027, 32.08224293864769550 ) ) ;
#51856=CARTESIAN_POINT ( 'NONE',  ( -9.564922557961040184, 16.46253265017147172, 67.91775706135233293 ) ) ;
#51858=CARTESIAN_POINT ( 'NONE',  ( 21.52544592524334988, 5.823673210054432836, 81.45942372801900433 ) ) ;
#51859=CARTESIAN_POINT ( 'NONE',  ( -14.29746914071037622, -8.314922557961029526, 34.16775706135234714 ) ) ;
#51861=CARTESIAN_POINT ( 'NONE',  ( -5.823673210054116645, -21.52544592524344225, 42.29057627198103120 ) ) ;
#51862=CARTESIAN_POINT ( 'NONE',  ( 14.29746914071037800, 8.314922557961029526, 21.66775706135235069 ) ) ;
#51863=CARTESIAN_POINT ( 'NONE',  ( 13.97604488694527802, 13.89961937509977830, 24.37390960531435269 ) ) ;
#51864=CARTESIAN_POINT ( 'NONE',  ( -9.564922557961040184, 16.46253265017147172, 27.91775706135232582 ) ) ;
#51866=CARTESIAN_POINT ( 'NONE',  ( 16.51473224551069308, 9.474510206698969483, 39.16557627198103120 ) ) ;
#51868=CARTESIAN_POINT ( 'NONE',  ( -5.153800228976328057, -19.02544592524343514, 52.29057627198100988 ) ) ;
#51869=CARTESIAN_POINT ( 'NONE',  ( -18.39443945427638738, 5.500000000000031974, 98.51745347608651571 ) ) ;
#51871=CARTESIAN_POINT ( 'NONE',  ( 16.51473224551083163, -9.474510206698727899, 25.83442372801900078 ) ) ;
#51872=CARTESIAN_POINT ( 'NONE',  ( 4.379528057220092307, 16.55341960407617563, 112.2927570613523471 ) ) ;
#51873=CARTESIAN_POINT ( 'NONE',  ( -19.02544592524342804, 5.153800228976336051, 36.04057627198100988 ) ) ;
#51874=CARTESIAN_POINT ( 'NONE',  ( -9.564922557960796823, -16.46253265017161027, 97.08224293864769550 ) ) ;
#51875=CARTESIAN_POINT ( 'NONE',  ( 10.81492255796106328, -18.62759615963255655, 70.41775706135236135 ) ) ;
#51876=CARTESIAN_POINT ( 'NONE',  ( -5.153800228976328057, -19.02544592524343514, 32.29057627198102409 ) ) ;
#51877=CARTESIAN_POINT ( 'NONE',  ( -18.62759615963255300, -10.81492255796106328, 69.16775706135234714 ) ) ;
#51878=CARTESIAN_POINT ( 'NONE',  ( 19.05341960407617918, -5.049401038297876454, 96.04275706135231871 ) ) ;
#51879=CARTESIAN_POINT ( 'NONE',  ( -21.55341960407610458, -5.719274019375992779, 26.45724293864768839 ) ) ;
#51880=CARTESIAN_POINT ( 'NONE',  ( -5.153800228976328057, -19.02544592524343514, 42.29057627198101699 ) ) ;
#51881=CARTESIAN_POINT ( 'NONE',  ( 10.81492255796078972, 18.62759615963270932, 104.5822429386477097 ) ) ;
#51882=CARTESIAN_POINT ( 'NONE',  ( -19.05341960407617563, 5.049401038297882671, 28.54275706135232937 ) ) ;
#51883=CARTESIAN_POINT ( 'NONE',  ( -14.29746914071049879, 8.314922557960819915, 105.8322429386476955 ) ) ;
#51884=CARTESIAN_POINT ( 'NONE',  ( -13.89961937509977652, 13.97604488694528158, 65.62390960531436690 ) ) ;
#51885=CARTESIAN_POINT ( 'NONE',  ( -0.05219959533936034679, 19.03943276465977164, 92.50109039468566152 ) ) ;
#51886=CARTESIAN_POINT ( 'NONE',  ( 8.224510206698953496, -14.34966873604960469, 77.91557627198102409 ) ) ;
#51887=CARTESIAN_POINT ( 'NONE',  ( -0.05219959533907301413, -21.53943276465977519, 27.49890960531435269 ) ) ;
#51888=CARTESIAN_POINT ( 'NONE',  ( 5.049401038297881783, 19.05341960407617563, 82.29275706135229029 ) ) ;
#51889=CARTESIAN_POINT ( 'NONE',  ( -18.67979575497178146, -10.72451020669898902, 86.66557627198102409 ) ) ;
#51890=CARTESIAN_POINT ( 'NONE',  ( -5.719274019375665041, -21.55341960407619695, 39.79275706135235424 ) ) ;
#51891=CARTESIAN_POINT ( 'NONE',  ( 16.55341960407618274, -4.379528057220086978, 46.04275706135234714 ) ) ;
#51892=CARTESIAN_POINT ( 'NONE',  ( 8.224510206698742110, 14.34966873604972548, 57.08442372801901854 ) ) ;
#51893=CARTESIAN_POINT ( 'NONE',  ( -5.719274019375665041, -21.55341960407619695, 54.79275706135235424 ) ) ;
#51894=CARTESIAN_POINT ( 'NONE',  ( 21.55341960407610458, 5.719274019375980345, 58.95724293864770971 ) ) ;
#51895=CARTESIAN_POINT ( 'NONE',  ( -5.049401038298153566, 19.05341960407611168, 45.20724293864769550 ) ) ;
#51897=CARTESIAN_POINT ( 'NONE',  ( -14.34966873604972548, 8.224510206698743886, 73.33442372801901854 ) ) ;
#51898=CARTESIAN_POINT ( 'NONE',  ( -15.80617190586745835, -15.72974639402198527, 96.87390960531436690 ) ) ;
#51899=CARTESIAN_POINT ( 'NONE',  ( -4.483927247898539470, -16.52544592524342804, 52.29057627198102409 ) ) ;
#51900=CARTESIAN_POINT ( 'NONE',  ( 8.224510206698742110, 14.34966873604972548, 57.08442372801901854 ) ) ;
#51901=CARTESIAN_POINT ( 'NONE',  ( -19.03943276465977164, -0.05219959533935918106, 93.75109039468566152 ) ) ;
#51902=CARTESIAN_POINT ( 'NONE',  ( -18.62759615963270932, 10.81492255796079327, 95.83224293864770971 ) ) ;
#51903=CARTESIAN_POINT ( 'NONE',  ( -16.52544592524342804, 4.483927247898546575, 46.04057627198103830 ) ) ;
#51905=CARTESIAN_POINT ( 'NONE',  ( -4.483927247898782831, 16.52544592524335698, 77.70942372801900433 ) ) ;
#51906=CARTESIAN_POINT ( 'NONE',  ( 19.02130022317636815, -5.499999999999793943, 93.28188669246577547 ) ) ;
#51907=CARTESIAN_POINT ( 'NONE',  ( -10.81492255796078084, -18.62759615963271287, 72.08224293864769550 ) ) ;
#51908=CARTESIAN_POINT ( 'NONE',  ( -12.14591786802309592, -12.06949235617757132, 21.87390960531436690 ) ) ;
#51911=CARTESIAN_POINT ( 'NONE',  ( -15.72974639402197994, 15.80617190586746368, 100.6239096053143811 ) ) ;
#51912=CARTESIAN_POINT ( 'NONE',  ( 0.05219959533907565091, 21.53943276465977519, 109.9989096053143527 ) ) ;
#51913=CARTESIAN_POINT ( 'NONE',  ( 16.52544592524342804, -4.483927247898539470, 33.54057627198102409 ) ) ;
#51914=CARTESIAN_POINT ( 'NONE',  ( -4.483927247898782831, 16.52544592524335698, 52.70942372801902565 ) ) ;
#51915=CARTESIAN_POINT ( 'NONE',  ( 19.03943276465977164, -0.05219959533909143690, 43.74890960531435979 ) ) ;
#51916=CARTESIAN_POINT ( 'NONE',  ( -16.51473224551069308, -9.474510206698971260, 71.66557627198102409 ) ) ;
#51918=CARTESIAN_POINT ( 'NONE',  ( 19.02544592524343514, -5.153800228976328945, 113.5405762719810241 ) ) ;
#51920=CARTESIAN_POINT ( 'NONE',  ( 16.51473224551083163, -9.474510206698727899, 110.8344237280190043 ) ) ;
#51921=CARTESIAN_POINT ( 'NONE',  ( 16.46253265017146816, 9.564922557961045513, 51.66775706135233293 ) ) ;
#51922=CARTESIAN_POINT ( 'NONE',  ( 15.72974639402199770, -15.80617190586745480, 88.12390960531436690 ) ) ;
#51923=CARTESIAN_POINT ( 'NONE',  ( -14.29746914071037622, -8.314922557961029526, 109.1677570613523613 ) ) ;
#51924=CARTESIAN_POINT ( 'NONE',  ( -5.153800228976328057, -19.02544592524343514, 77.29057627198099567 ) ) ;
#51925=CARTESIAN_POINT ( 'NONE',  ( -21.52544592524343514, 5.823673210054127303, 41.04057627198103120 ) ) ;
#51926=CARTESIAN_POINT ( 'NONE',  ( -15.80617190586745835, -15.72974639402198527, 81.87390960531435269 ) ) ;
#51927=CARTESIAN_POINT ( 'NONE',  ( -14.34966873604972548, 8.224510206698743886, 23.33442372801901499 ) ) ;
#51928=CARTESIAN_POINT ( 'NONE',  ( 21.52544592524344225, -5.823673210054117533, 28.54057627198103120 ) ) ;
#51929=CARTESIAN_POINT ( 'NONE',  ( 18.67979575497194134, -10.72451020669871369, 80.83442372801901854 ) ) ;
#51930=CARTESIAN_POINT ( 'NONE',  ( -16.51473224551069308, -9.474510206698971260, 76.66557627198103830 ) ) ;
#51931=CARTESIAN_POINT ( 'NONE',  ( -5.049401038298153566, 19.05341960407611168, 25.20724293864768484 ) ) ;
#51932=CARTESIAN_POINT ( 'NONE',  ( -13.89961937509977652, 13.97604488694528158, 85.62390960531433848 ) ) ;
#51933=CARTESIAN_POINT ( 'NONE',  ( 0.05219959533910956823, 16.53943276465976808, 89.99890960531438111 ) ) ;
#51935=CARTESIAN_POINT ( 'NONE',  ( 9.474510206698729675, 16.51473224551082808, 102.0844237280190043 ) ) ;
#51937=CARTESIAN_POINT ( 'NONE',  ( 19.02544592524343514, -5.153800228976328945, 78.54057627198099567 ) ) ;
#51938=CARTESIAN_POINT ( 'NONE',  ( 15.80617190586769283, -15.72974639402175789, 80.62609039468567573 ) ) ;
#51939=CARTESIAN_POINT ( 'NONE',  ( -9.474510206698964154, 16.51473224551069663, 100.4155762719810241 ) ) ;
#51940=CARTESIAN_POINT ( 'NONE',  ( -4.379528057220086978, -16.55341960407618274, 79.79275706135236135 ) ) ;
#51941=CARTESIAN_POINT ( 'NONE',  ( -17.48853670773247160, -5.747243402303015891, 76.33328700250010002 ) ) ;
#51942=CARTESIAN_POINT ( 'NONE',  ( 13.89961937509957401, 13.97604488694547697, 51.87609039468566863 ) ) ;
#51943=CARTESIAN_POINT ( 'NONE',  ( -16.51473224551082808, 9.474510206698731452, 23.33442372801900078 ) ) ;
#51947=CARTESIAN_POINT ( 'NONE',  ( 16.53943276465976808, -0.05219959533910856209, 23.74890960531435269 ) ) ;
#51949=CARTESIAN_POINT ( 'NONE',  ( 12.06949235617739724, 12.14591786802326823, 111.8760903946856615 ) ) ;
#51951=CARTESIAN_POINT ( 'NONE',  ( -8.314922557961024197, 14.29746914071037800, 87.91775706135234714 ) ) ;
#51952=CARTESIAN_POINT ( 'NONE',  ( 15.80617190586769283, -15.72974639402175789, 95.62609039468568994 ) ) ;
#51953=CARTESIAN_POINT ( 'NONE',  ( 5.153800228976615827, -19.02544592524334988, 100.2094237280190043 ) ) ;
#51954=CARTESIAN_POINT ( 'NONE',  ( 18.62759615963255655, 10.81492255796105972, 66.66775706135234714 ) ) ;
#51955=CARTESIAN_POINT ( 'NONE',  ( 0.05219959533936267826, -19.03943276465977164, 45.00109039468566863 ) ) ;
#51956=CARTESIAN_POINT ( 'NONE',  ( -13.97604488694527625, -13.89961937509977652, 76.87390960531433848 ) ) ;
#51957=CARTESIAN_POINT ( 'NONE',  ( -9.564922557960796823, -16.46253265017161027, 57.08224293864769550 ) ) ;
#51958=CARTESIAN_POINT ( 'NONE',  ( -18.87580814761071935, 5.500000000000042633, 40.87172394265763842 ) ) ;
#51959=CARTESIAN_POINT ( 'NONE',  ( -10.81492255796078084, -18.62759615963271287, 97.08224293864770971 ) ) ;
#51960=CARTESIAN_POINT ( 'NONE',  ( 18.62759615963271287, -10.81492255796078972, 48.33224293864770260 ) ) ;
#51961=CARTESIAN_POINT ( 'NONE',  ( -5.153800228976328057, -19.02544592524343514, 47.29057627198102409 ) ) ;
#51962=CARTESIAN_POINT ( 'NONE',  ( 12.14591786802327356, -12.06949235617739191, 60.62609039468567573 ) ) ;
#51965=CARTESIAN_POINT ( 'NONE',  ( -21.55341960407619339, 5.719274019375674811, 48.54275706135234714 ) ) ;
#51966=CARTESIAN_POINT ( 'NONE',  ( 14.29746914071049879, -8.314922557960816363, 68.33224293864769550 ) ) ;
#51968=CARTESIAN_POINT ( 'NONE',  ( -12.14591786802326823, 12.06949235617739902, 43.12609039468568284 ) ) ;
#51969=CARTESIAN_POINT ( 'NONE',  ( -4.379528057220328563, 16.55341960407611168, 100.2072429386476955 ) ) ;
#51970=CARTESIAN_POINT ( 'NONE',  ( -19.05341960407617563, 5.049401038297882671, 48.54275706135233293 ) ) ;
#51971=CARTESIAN_POINT ( 'NONE',  ( -4.379528057220328563, 16.55341960407611168, 65.20724293864768129 ) ) ;
#51972=CARTESIAN_POINT ( 'NONE',  ( 21.52544592524334988, 5.823673210054432836, 26.45942372801901854 ) ) ;
#51973=CARTESIAN_POINT ( 'NONE',  ( -0.05219959533909027116, -19.03943276465977164, 27.49890960531435624 ) ) ;
#51974=CARTESIAN_POINT ( 'NONE',  ( 0.05219959533907565091, 21.53943276465977519, 89.99890960531438111 ) ) ;
#51976=CARTESIAN_POINT ( 'NONE',  ( -13.89961937509977652, 13.97604488694528158, 105.6239096053143527 ) ) ;
#51977=CARTESIAN_POINT ( 'NONE',  ( -14.29746914071049879, 8.314922557960819915, 75.83224293864769550 ) ) ;
#51980=CARTESIAN_POINT ( 'NONE',  ( -13.97604488694547697, 13.89961937509957934, 83.12609039468564731 ) ) ;
#51981=CARTESIAN_POINT ( 'NONE',  ( -10.72451020669870658, -18.67979575497194134, 19.58442372801901143 ) ) ;
#51982=CARTESIAN_POINT ( 'NONE',  ( 13.97604488694527802, 13.89961937509977652, 74.37390960531436690 ) ) ;
#51983=CARTESIAN_POINT ( 'NONE',  ( 16.51473224551083163, -9.474510206698727899, 55.83442372801899722 ) ) ;
#51984=CARTESIAN_POINT ( 'NONE',  ( 19.03943276465977164, -0.05219959533909143690, 28.74890960531435624 ) ) ;
#51985=CARTESIAN_POINT ( 'NONE',  ( 8.224510206698953496, -14.34966873604960469, 57.91557627198103120 ) ) ;
#51986=CARTESIAN_POINT ( 'NONE',  ( 4.483927247898545687, 16.52544592524342804, 59.79057627198103120 ) ) ;
#51987=CARTESIAN_POINT ( 'NONE',  ( 19.03943276465977164, -0.05219959533909143690, 78.74890960531436690 ) ) ;
#51988=CARTESIAN_POINT ( 'NONE',  ( 18.62759615963271287, -10.81492255796078972, 93.33224293864769550 ) ) ;
#51989=CARTESIAN_POINT ( 'NONE',  ( 9.474510206698971260, -16.51473224551069308, 72.91557627198102409 ) ) ;
#51990=CARTESIAN_POINT ( 'NONE',  ( 18.62759615963271287, -10.81492255796078972, 78.33224293864770971 ) ) ;
#51991=CARTESIAN_POINT ( 'NONE',  ( 19.05341960407617918, -5.049401038297876454, 21.04275706135232582 ) ) ;
#51992=CARTESIAN_POINT ( 'NONE',  ( 16.46253265017160672, -9.564922557960803928, 28.33224293864769550 ) ) ;
#51993=CARTESIAN_POINT ( 'NONE',  ( 16.52544592524335698, 4.483927247898782831, 111.4594237280190328 ) ) ;
#51994=CARTESIAN_POINT ( 'NONE',  ( 0.05219959533910956823, 16.53943276465976808, 89.99890960531438111 ) ) ;
#51995=CARTESIAN_POINT ( 'NONE',  ( -5.153800228976607833, 19.02544592524334988, 92.70942372801901854 ) ) ;
#51996=ORIENTED_EDGE ( 'NONE', *, *, #69172, .T. ) ;
#51997=CARTESIAN_POINT ( 'NONE',  ( -21.53943276465977519, 0.05219959533907696930, 116.2489096053143669 ) ) ;
#51998=CARTESIAN_POINT ( 'NONE',  ( 19.05341960407617918, -5.049401038297876454, 51.04275706135231871 ) ) ;
#51999=CARTESIAN_POINT ( 'NONE',  ( -4.379528057220086978, -16.55341960407618274, 104.7927570613523898 ) ) ;
#52000=CARTESIAN_POINT ( 'NONE',  ( -19.02544592524334988, -5.153800228976617603, 38.95942372801900433 ) ) ;
#52001=CARTESIAN_POINT ( 'NONE',  ( -5.153800228976328057, -19.02544592524343514, 97.29057627198099567 ) ) ;
#52002=CARTESIAN_POINT ( 'NONE',  ( -12.14591786802309592, -12.06949235617757132, 51.87390960531437401 ) ) ;
#52003=CARTESIAN_POINT ( 'NONE',  ( -19.52217212775657984, 5.500000000000114575, 49.93993709005260939 ) ) ;
#52004=CARTESIAN_POINT ( 'NONE',  ( -19.05341960407611168, -5.049401038298163336, 31.45724293864769550 ) ) ;
#52005=CARTESIAN_POINT ( 'NONE',  ( -18.62759615963255300, -10.81492255796106328, 109.1677570613523613 ) ) ;
#52006=CARTESIAN_POINT ( 'NONE',  ( 4.483927247898790824, -16.52544592524335698, 80.20942372801901854 ) ) ;
#52007=CARTESIAN_POINT ( 'NONE',  ( 21.53943276465977519, 0.05219959533937863772, 36.25109039468567573 ) ) ;
#52008=CARTESIAN_POINT ( 'NONE',  ( 8.224510206698742110, 14.34966873604972548, 47.08442372801901854 ) ) ;
#52009=CARTESIAN_POINT ( 'NONE',  ( -16.51473224551069308, -9.474510206698971260, 101.6655762719810241 ) ) ;
#52010=CARTESIAN_POINT ( 'NONE',  ( -19.05341960407611168, -5.049401038298163336, 51.45724293864770260 ) ) ;
#52011=CARTESIAN_POINT ( 'NONE',  ( 16.51473224551069308, 9.474510206698969483, 69.16557627198102409 ) ) ;
#52012=CARTESIAN_POINT ( 'NONE',  ( -8.224510206698735004, -14.34966873604973081, 44.58442372801901854 ) ) ;
#52013=CARTESIAN_POINT ( 'NONE',  ( -16.53943276465976808, 0.05219959533911058130, 106.2489096053143811 ) ) ;
#52014=CARTESIAN_POINT ( 'NONE',  ( 4.379528057220339221, -16.55341960407611168, 22.70724293864769194 ) ) ;
#52016=CARTESIAN_POINT ( 'NONE',  ( -21.52544592524334988, -5.823673210054445271, 53.95942372801900433 ) ) ;
#52017=CARTESIAN_POINT ( 'NONE',  ( 9.474510206698971260, -16.51473224551069308, 87.91557627198102409 ) ) ;
#52018=CARTESIAN_POINT ( 'NONE',  ( 0.05219959533909260263, 19.03943276465977164, 64.99890960531436690 ) ) ;
#52019=CARTESIAN_POINT ( 'NONE',  ( -13.97604488694527625, -13.89961937509977652, 91.87390960531432427 ) ) ;
#52020=CARTESIAN_POINT ( 'NONE',  ( -8.224510206698948167, 14.34966873604960824, 45.41557627198103830 ) ) ;
#52021=CARTESIAN_POINT ( 'NONE',  ( -12.06949235617739369, -12.14591786802326823, 109.3760903946857042 ) ) ;
#52022=CARTESIAN_POINT ( 'NONE',  ( -0.05219959533910754901, -16.53943276465976808, 37.49890960531436690 ) ) ;
#52025=CARTESIAN_POINT ( 'NONE',  ( -19.03943276465977164, 0.05219959533909376836, 66.24890960531436690 ) ) ;
#52026=CARTESIAN_POINT ( 'NONE',  ( -19.02544592524334988, -5.153800228976617603, 33.95942372801897591 ) ) ;
#52029=CARTESIAN_POINT ( 'NONE',  ( -16.46253265017146816, -9.564922557961047289, 84.16775706135233293 ) ) ;
#52030=CARTESIAN_POINT ( 'NONE',  ( 4.379528057220092307, 16.55341960407617563, 67.29275706135234714 ) ) ;
#52033=CARTESIAN_POINT ( 'NONE',  ( -13.89961937509977652, 13.97604488694528158, 90.62390960531432427 ) ) ;
#52034=CARTESIAN_POINT ( 'NONE',  ( -10.72451020669870658, -18.67979575497194134, 29.58442372801901854 ) ) ;
#52035=CARTESIAN_POINT ( 'NONE',  ( 9.474510206698729675, 16.51473224551082808, 87.08442372801900433 ) ) ;
#52036=CARTESIAN_POINT ( 'NONE',  ( 5.049401038298161559, -19.05341960407611168, 112.7072429386476813 ) ) ;
#52037=CARTESIAN_POINT ( 'NONE',  ( -5.153800228976328057, -19.02544592524343514, 52.29057627198100988 ) ) ;
#52038=EDGE_CURVE ( 'NONE', #65463, #45569, #36368, .T. ) ;
#52039=CARTESIAN_POINT ( 'NONE',  ( 19.05341960407611168, 5.049401038298154454, 93.95724293864769550 ) ) ;
#52040=CARTESIAN_POINT ( 'NONE',  ( -4.379528057220328563, 16.55341960407611168, 50.20724293864769550 ) ) ;
#52041=CARTESIAN_POINT ( 'NONE',  ( 0.05219959533909260263, 19.03943276465977164, 54.99890960531435979 ) ) ;
#52042=CARTESIAN_POINT ( 'NONE',  ( 16.46253265017146816, 9.564922557961045513, 61.66775706135234003 ) ) ;
#52044=CARTESIAN_POINT ( 'NONE',  ( 0.05219959533910956823, 16.53943276465976808, 84.99890960531436690 ) ) ;
#52045=CARTESIAN_POINT ( 'NONE',  ( -16.51473224551082808, 9.474510206698731452, 33.33442372801899722 ) ) ;
#52046=CARTESIAN_POINT ( 'NONE',  ( 0.05219959533909260263, 19.03943276465977164, 64.99890960531436690 ) ) ;
#52047=CARTESIAN_POINT ( 'NONE',  ( 15.72974639402199770, -15.80617190586745480, 68.12390960531436690 ) ) ;
#52048=CARTESIAN_POINT ( 'NONE',  ( -12.14591786802309592, -12.06949235617757132, 61.87390960531436690 ) ) ;
#52049=CARTESIAN_POINT ( 'NONE',  ( -9.564922557961040184, 16.46253265017147172, 27.91775706135232582 ) ) ;
#52050=CARTESIAN_POINT ( 'NONE',  ( 16.46253265017160672, -9.564922557960803928, 103.3322429386476955 ) ) ;
#52051=CARTESIAN_POINT ( 'NONE',  ( -10.81492255796078084, -18.62759615963271287, 27.08224293864769550 ) ) ;
#52052=CARTESIAN_POINT ( 'NONE',  ( -9.564922557960796823, -16.46253265017161027, 52.08224293864768839 ) ) ;
#52053=CARTESIAN_POINT ( 'NONE',  ( 9.564922557960805705, 16.46253265017160317, 44.58224293864769550 ) ) ;
#52054=CARTESIAN_POINT ( 'NONE',  ( 4.379528057220339221, -16.55341960407611168, 102.7072429386476955 ) ) ;
#52055=CARTESIAN_POINT ( 'NONE',  ( 21.52544592524344225, -5.823673210054117533, 113.5405762719810383 ) ) ;
#52056=CARTESIAN_POINT ( 'NONE',  ( -13.97604488694527625, -13.89961937509977652, 101.8739096053143811 ) ) ;
#52057=CARTESIAN_POINT ( 'NONE',  ( 21.53943276465977519, 0.05219959533937863772, 26.25109039468567573 ) ) ;
#52058=CARTESIAN_POINT ( 'NONE',  ( -9.474510206698964154, 16.51473224551069663, 105.4155762719810383 ) ) ;
#52059=CARTESIAN_POINT ( 'NONE',  ( 19.05341960407611168, 5.049401038298154454, 23.95724293864769194 ) ) ;
#52060=CARTESIAN_POINT ( 'NONE',  ( -10.72451020669870658, -18.67979575497194134, 79.58442372801903275 ) ) ;
#52061=CARTESIAN_POINT ( 'NONE',  ( 10.81492255796078972, 18.62759615963270932, 99.58224293864770971 ) ) ;
#52063=CARTESIAN_POINT ( 'NONE',  ( 18.22780087662123805, -5.499999999999989342, 53.51763182126895657 ) ) ;
#52064=CARTESIAN_POINT ( 'NONE',  ( 0.05219959533909260263, 19.03943276465977164, 59.99890960531436690 ) ) ;
#52065=CARTESIAN_POINT ( 'NONE',  ( 16.53943276465976808, 0.05219959533934440121, 51.25109039468568994 ) ) ;
#52066=CARTESIAN_POINT ( 'NONE',  ( -16.55341960407611168, -4.379528057220339221, 101.4572429386476955 ) ) ;
#52067=CARTESIAN_POINT ( 'NONE',  ( 19.52837319214024703, -5.500000000000095923, 52.10471352585538796 ) ) ;
#52068=CARTESIAN_POINT ( 'NONE',  ( 19.03943276465977164, -0.05219959533909143690, 63.74890960531435979 ) ) ;
#52069=CARTESIAN_POINT ( 'NONE',  ( 16.52544592524342804, -4.483927247898539470, 93.54057627198103830 ) ) ;
#52070=CARTESIAN_POINT ( 'NONE',  ( -5.823673210054116645, -21.52544592524344225, 42.29057627198103120 ) ) ;
#52072=CARTESIAN_POINT ( 'NONE',  ( 12.06949235617757843, -12.14591786802309237, 68.12390960531436690 ) ) ;
#52073=CARTESIAN_POINT ( 'NONE',  ( 14.34966873604972726, -8.224510206698740333, 20.83442372801901143 ) ) ;
#52074=CARTESIAN_POINT ( 'NONE',  ( -21.52544592524334988, -5.823673210054445271, 78.95942372801901854 ) ) ;
#52076=CARTESIAN_POINT ( 'NONE',  ( -8.314922557961024197, 14.29746914071037800, 102.9177570613523756 ) ) ;
#52077=CARTESIAN_POINT ( 'NONE',  ( 8.224510206698953496, -14.34966873604960469, 47.91557627198102409 ) ) ;
#52078=CARTESIAN_POINT ( 'NONE',  ( 13.97604488694527802, 13.89961937509977652, 44.37390960531435269 ) ) ;
#52079=CARTESIAN_POINT ( 'NONE',  ( 16.46253265017160672, -9.564922557960803928, 83.33224293864768129 ) ) ;
#52080=CARTESIAN_POINT ( 'NONE',  ( -18.67979575497178146, -10.72451020669898902, 91.66557627198103830 ) ) ;
#52081=CARTESIAN_POINT ( 'NONE',  ( 16.52544592524335698, 4.483927247898782831, 41.45942372801901143 ) ) ;
#52082=CARTESIAN_POINT ( 'NONE',  ( -16.53943276465976808, 0.05219959533911058130, 71.24890960531435269 ) ) ;
#52083=CARTESIAN_POINT ( 'NONE',  ( 10.72451020669871369, 18.67979575497193778, 77.08442372801901854 ) ) ;
#52084=CARTESIAN_POINT ( 'NONE',  ( 16.52544592524335698, 4.483927247898782831, 96.45942372801901854 ) ) ;
#52085=CARTESIAN_POINT ( 'NONE',  ( 17.50000000001358558, -5.500000000000039968, 48.29690382535059001 ) ) ;
#52087=CARTESIAN_POINT ( 'NONE',  ( -12.14591786802309592, -12.06949235617757132, 21.87390960531436690 ) ) ;
#52088=CARTESIAN_POINT ( 'NONE',  ( -14.34966873604972548, 8.224510206698743886, 78.33442372801901854 ) ) ;
#52089=CARTESIAN_POINT ( 'NONE',  ( -5.049401038298153566, 19.05341960407611168, 90.20724293864766707 ) ) ;
#52090=CARTESIAN_POINT ( 'NONE',  ( -0.05219959533909027116, -19.03943276465977164, 102.4989096053143669 ) ) ;
#52091=CARTESIAN_POINT ( 'NONE',  ( -0.05219959533937732626, 21.53943276465977519, 82.50109039468568994 ) ) ;
#52092=CARTESIAN_POINT ( 'NONE',  ( 4.483927247898790824, -16.52544592524335698, 90.20942372801903275 ) ) ;
#52093=CARTESIAN_POINT ( 'NONE',  ( 14.34966873604960469, 8.224510206698951720, 54.16557627198103120 ) ) ;
#52094=CARTESIAN_POINT ( 'NONE',  ( -0.05219959533909027116, -19.03943276465977164, 62.49890960531435979 ) ) ;
#52095=ORIENTED_EDGE ( 'NONE', *, *, #109475, .T. ) ;
#52096=CARTESIAN_POINT ( 'NONE',  ( -5.049401038297874678, -19.05341960407617918, 104.7927570613523471 ) ) ;
#52097=CARTESIAN_POINT ( 'NONE',  ( 14.29746914071049879, -8.314922557960816363, 113.3322429386476955 ) ) ;
#52098=CARTESIAN_POINT ( 'NONE',  ( 19.05341960407611168, 5.049401038298154454, 83.95724293864766707 ) ) ;
#52099=CARTESIAN_POINT ( 'NONE',  ( -16.46253265017146816, -9.564922557961047289, 109.1677570613523471 ) ) ;
#52101=CARTESIAN_POINT ( 'NONE',  ( -16.51473224551082808, 9.474510206698731452, 28.33442372801900433 ) ) ;
#52102=CARTESIAN_POINT ( 'NONE',  ( 4.483927247898790824, -16.52544592524335698, 85.20942372801901854 ) ) ;
#52103=CARTESIAN_POINT ( 'NONE',  ( 9.474510206698729675, 16.51473224551082808, 112.0844237280190043 ) ) ;
#52104=CARTESIAN_POINT ( 'NONE',  ( 4.483927247898545687, 16.52544592524342804, 109.7905762719810383 ) ) ;
#52105=CARTESIAN_POINT ( 'NONE',  ( 8.224510206698742110, 14.34966873604972548, 62.08442372801901143 ) ) ;
#52106=CARTESIAN_POINT ( 'NONE',  ( -16.52544592524335698, -4.483927247898792601, 48.95942372801902565 ) ) ;
#52108=CARTESIAN_POINT ( 'NONE',  ( -19.02544592524334988, -5.153800228976617603, 63.95942372801899012 ) ) ;
#52109=CARTESIAN_POINT ( 'NONE',  ( -0.05219959533937732626, 21.53943276465977519, 92.50109039468567573 ) ) ;
#52110=CARTESIAN_POINT ( 'NONE',  ( 19.05341960407611168, 5.049401038298154454, 28.95724293864769550 ) ) ;
#52111=CARTESIAN_POINT ( 'NONE',  ( -0.05219959533909027116, -19.03943276465977164, 72.49890960531435269 ) ) ;
#52112=CARTESIAN_POINT ( 'NONE',  ( -4.483927247898539470, -16.52544592524342804, 67.29057627198103830 ) ) ;
#52113=CARTESIAN_POINT ( 'NONE',  ( -10.72451020669870658, -18.67979575497194134, 94.58442372801901854 ) ) ;
#52115=CARTESIAN_POINT ( 'NONE',  ( -19.05341960407617563, 5.049401038297882671, 43.54275706135232582 ) ) ;
#52116=CARTESIAN_POINT ( 'NONE',  ( -15.72974639402197994, 15.80617190586746368, 35.62390960531437401 ) ) ;
#52117=CARTESIAN_POINT ( 'NONE',  ( -15.72974639402176322, -15.80617190586768395, 109.3760903946857042 ) ) ;
#52118=CARTESIAN_POINT ( 'NONE',  ( 16.51473224551069308, 9.474510206698969483, 74.16557627198103830 ) ) ;
#52119=CARTESIAN_POINT ( 'NONE',  ( -0.05219959533937732626, 21.53943276465977519, 102.5010903946856899 ) ) ;
#52120=CARTESIAN_POINT ( 'NONE',  ( -10.72451020669898014, 18.67979575497178502, 70.41557627198102409 ) ) ;
#52121=CARTESIAN_POINT ( 'NONE',  ( -16.46253265017160317, 9.564922557960807481, 100.8322429386477097 ) ) ;
#52122=CARTESIAN_POINT ( 'NONE',  ( -0.05219959533936034679, 19.03943276465977164, 72.50109039468566152 ) ) ;
#52123=CARTESIAN_POINT ( 'NONE',  ( -19.05341960407611168, -5.049401038298163336, 101.4572429386476955 ) ) ;
#52124=CARTESIAN_POINT ( 'NONE',  ( 5.153800228976615827, -19.02544592524334988, 90.20942372801900433 ) ) ;
#52125=CARTESIAN_POINT ( 'NONE',  ( -12.14591786802326823, 12.06949235617739902, 58.12609039468568994 ) ) ;
#52126=CARTESIAN_POINT ( 'NONE',  ( -0.05219959533909027116, -19.03943276465977164, 22.49890960531436690 ) ) ;
#52127=CARTESIAN_POINT ( 'NONE',  ( 19.03943276465977164, -0.05219959533909143690, 88.74890960531436690 ) ) ;
#52128=CARTESIAN_POINT ( 'NONE',  ( 15.80617190586746368, 15.72974639402197994, 59.37390960531436690 ) ) ;
#52129=CARTESIAN_POINT ( 'NONE',  ( -12.14591786802326823, 12.06949235617739902, 28.12609039468568284 ) ) ;
#52130=CARTESIAN_POINT ( 'NONE',  ( -15.80617190586768217, 15.72974639402176855, 33.12609039468569705 ) ) ;
#52131=CARTESIAN_POINT ( 'NONE',  ( 10.72451020669871369, 18.67979575497193778, 82.08442372801901854 ) ) ;
#52132=CARTESIAN_POINT ( 'NONE',  ( -8.314922557961024197, 14.29746914071037800, 102.9177570613523756 ) ) ;
#52133=CARTESIAN_POINT ( 'NONE',  ( 13.97604488694527802, 13.89961937509977652, 84.37390960531433848 ) ) ;
#52134=CARTESIAN_POINT ( 'NONE',  ( 16.52544592524342804, -4.483927247898539470, 78.54057627198103830 ) ) ;
#52135=CARTESIAN_POINT ( 'NONE',  ( -16.53943276465976808, 0.05219959533911058130, 21.24890960531436690 ) ) ;
#52136=CARTESIAN_POINT ( 'NONE',  ( 13.89961937509957401, 13.97604488694547697, 56.87609039468564731 ) ) ;
#52137=CARTESIAN_POINT ( 'NONE',  ( -10.81492255796105439, 18.62759615963255655, 42.91775706135235424 ) ) ;
#52138=CARTESIAN_POINT ( 'NONE',  ( 16.52544592524342804, -4.483927247898539470, 93.54057627198103830 ) ) ;
#52139=CARTESIAN_POINT ( 'NONE',  ( -16.46253265017160317, 9.564922557960807481, 110.8322429386476955 ) ) ;
#52140=CARTESIAN_POINT ( 'NONE',  ( -14.34966873604972548, 8.224510206698743886, 108.3344237280190185 ) ) ;
#52141=CARTESIAN_POINT ( 'NONE',  ( 21.55341960407619695, -5.719274019375665929, 86.04275706135236135 ) ) ;
#52142=CARTESIAN_POINT ( 'NONE',  ( 14.29746914071037800, 8.314922557961029526, 41.66775706135235424 ) ) ;
#52143=CARTESIAN_POINT ( 'NONE',  ( -18.62759615963255300, -10.81492255796106328, 39.16775706135235424 ) ) ;
#52144=VERTEX_POINT ( 'NONE', #193071 ) ;
#52145=CARTESIAN_POINT ( 'NONE',  ( -18.67979575497193778, 10.72451020669871902, 23.33442372801901499 ) ) ;
#52146=CARTESIAN_POINT ( 'NONE',  ( -16.53943276465976808, 0.05219959533911058130, 91.24890960531436690 ) ) ;
#52147=CARTESIAN_POINT ( 'NONE',  ( -19.35543954521081034, -5.499999999999584332, 49.58901960356452321 ) ) ;
#52148=CARTESIAN_POINT ( 'NONE',  ( -14.29746914071049879, 8.314922557960819915, 60.83224293864769550 ) ) ;
#52149=CARTESIAN_POINT ( 'NONE',  ( -16.52544592524335698, -4.483927247898792601, 103.9594237280190185 ) ) ;
#52150=CARTESIAN_POINT ( 'NONE',  ( 9.474510206698971260, -16.51473224551069308, 42.91557627198103120 ) ) ;
#52151=CARTESIAN_POINT ( 'NONE',  ( 18.67979575497178502, 10.72451020669898547, 39.16557627198102409 ) ) ;
#52152=CARTESIAN_POINT ( 'NONE',  ( -8.314922557960811034, -14.29746914071050412, 82.08224293864768129 ) ) ;
#52153=CARTESIAN_POINT ( 'NONE',  ( 5.719274019375991003, -21.55341960407610458, 77.70724293864770971 ) ) ;
#52154=CARTESIAN_POINT ( 'NONE',  ( 19.05341960407611168, 5.049401038298154454, 83.95724293864766707 ) ) ;
#52155=CARTESIAN_POINT ( 'NONE',  ( 19.02544592524343514, -5.153800228976328945, 33.54057627198102409 ) ) ;
#52156=CARTESIAN_POINT ( 'NONE',  ( -19.03943276465977164, -0.05219959533935918106, 98.75109039468567573 ) ) ;
#52157=CARTESIAN_POINT ( 'NONE',  ( 5.823673210054125526, 21.52544592524343514, 34.79057627198103120 ) ) ;
#52158=CARTESIAN_POINT ( 'NONE',  ( -15.80617190586768217, 15.72974639402176855, 53.12609039468568284 ) ) ;
#52159=CARTESIAN_POINT ( 'NONE',  ( 19.03943276465977164, -0.05219959533909143690, 58.74890960531435979 ) ) ;
#52160=CARTESIAN_POINT ( 'NONE',  ( 9.474510206698971260, -16.51473224551069308, 87.91557627198102409 ) ) ;
#52162=CARTESIAN_POINT ( 'NONE',  ( -4.483927247898782831, 16.52544592524335698, 47.70942372801902565 ) ) ;
#52163=CARTESIAN_POINT ( 'NONE',  ( 10.81492255796106328, -18.62759615963255655, 40.41775706135234714 ) ) ;
#52164=CARTESIAN_POINT ( 'NONE',  ( 5.823673210054444382, -21.52544592524334988, 75.20942372801901854 ) ) ;
#52165=CARTESIAN_POINT ( 'NONE',  ( -5.823673210054116645, -21.52544592524344225, 22.29057627198102765 ) ) ;
#52166=CARTESIAN_POINT ( 'NONE',  ( -10.72451020669898014, 18.67979575497178502, 85.41557627198102409 ) ) ;
#52167=CARTESIAN_POINT ( 'NONE',  ( -10.72451020669870658, -18.67979575497194134, 24.58442372801901499 ) ) ;
#52168=CARTESIAN_POINT ( 'NONE',  ( 16.55341960407618274, -4.379528057220086978, 66.04275706135236135 ) ) ;
#52169=CARTESIAN_POINT ( 'NONE',  ( 15.72974639402199770, -15.80617190586745480, 58.12390960531435979 ) ) ;
#52170=CARTESIAN_POINT ( 'NONE',  ( -5.049401038297874678, -19.05341960407617918, 19.79275706135233293 ) ) ;
#52171=CARTESIAN_POINT ( 'NONE',  ( 16.46253265017160672, -9.564922557960803928, 73.33224293864769550 ) ) ;
#52172=CARTESIAN_POINT ( 'NONE',  ( -12.14591786802326823, 12.06949235617739902, 103.1260903946856757 ) ) ;
#52173=CARTESIAN_POINT ( 'NONE',  ( -17.49999999999999645, -5.076555817581251517, 106.1795149204977378 ) ) ;
#52174=CARTESIAN_POINT ( 'NONE',  ( -19.02544592524342804, 5.153800228976336051, 86.04057627198103830 ) ) ;
#52175=CARTESIAN_POINT ( 'NONE',  ( 13.89961937509957401, 13.97604488694547697, 86.87609039468567573 ) ) ;
#52176=CARTESIAN_POINT ( 'NONE',  ( 18.67979575497178502, 10.72451020669898547, 59.16557627198103120 ) ) ;
#52177=CARTESIAN_POINT ( 'NONE',  ( -16.55341960407617563, 4.379528057220093196, 113.5427570613523756 ) ) ;
#52178=CARTESIAN_POINT ( 'NONE',  ( -19.02544592524334988, -5.153800228976617603, 98.95942372801900433 ) ) ;
#52179=CARTESIAN_POINT ( 'NONE',  ( -5.049401038298153566, 19.05341960407611168, 40.20724293864768839 ) ) ;
#52180=CARTESIAN_POINT ( 'NONE',  ( 13.97604488694548053, -13.89961937509957401, 90.62609039468567573 ) ) ;
#52181=CARTESIAN_POINT ( 'NONE',  ( 0.05219959533907565091, 21.53943276465977519, 89.99890960531438111 ) ) ;
#52182=CARTESIAN_POINT ( 'NONE',  ( -13.89961937509957401, -13.97604488694547875, 54.37609039468565442 ) ) ;
#52184=CARTESIAN_POINT ( 'NONE',  ( 16.51473224551069308, 9.474510206698969483, 49.16557627198102409 ) ) ;
#52185=CARTESIAN_POINT ( 'NONE',  ( -0.05219959533910754901, -16.53943276465976808, 57.49890960531435979 ) ) ;
#52186=CARTESIAN_POINT ( 'NONE',  ( -9.564922557960796823, -16.46253265017161027, 47.08224293864769550 ) ) ;
#52187=CARTESIAN_POINT ( 'NONE',  ( -16.55341960407611168, -4.379528057220339221, 56.45724293864768839 ) ) ;
#52188=CARTESIAN_POINT ( 'NONE',  ( -15.49999999999999822, -7.500000000000000888, 22.00000000000000711 ) ) ;
#52190=CARTESIAN_POINT ( 'NONE',  ( 4.483927247898545687, 16.52544592524342804, 34.79057627198103120 ) ) ;
#52191=CARTESIAN_POINT ( 'NONE',  ( 16.46253265017160672, -9.564922557960803928, 58.33224293864769550 ) ) ;
#52192=CARTESIAN_POINT ( 'NONE',  ( -0.05219959533936034679, 19.03943276465977164, 72.50109039468566152 ) ) ;
#52193=CARTESIAN_POINT ( 'NONE',  ( 5.153800228976615827, -19.02544592524334988, 40.20942372801898301 ) ) ;
#52194=CARTESIAN_POINT ( 'NONE',  ( -8.224510206698735004, -14.34966873604973081, 49.58442372801901143 ) ) ;
#52195=CARTESIAN_POINT ( 'NONE',  ( -21.53943276465977519, 0.05219959533907696930, 46.24890960531435979 ) ) ;
#52196=CARTESIAN_POINT ( 'NONE',  ( -5.719274019375665041, -21.55341960407619695, 109.7927570613523613 ) ) ;
#52197=CARTESIAN_POINT ( 'NONE',  ( 5.153800228976335163, 19.02544592524342804, 74.79057627198103830 ) ) ;
#52198=CARTESIAN_POINT ( 'NONE',  ( -17.49999999999999645, -5.500000000000000888, 120.0000000000000142 ) ) ;
#52199=CARTESIAN_POINT ( 'NONE',  ( 13.97604488694527802, 13.89961937509977652, 99.37390960531436690 ) ) ;
#52201=CARTESIAN_POINT ( 'NONE',  ( -21.53943276465977519, -0.05219959533937600094, 23.75109039468567929 ) ) ;
#52202=CARTESIAN_POINT ( 'NONE',  ( -12.14591786802309592, -12.06949235617757132, 86.87390960531438111 ) ) ;
#52203=CARTESIAN_POINT ( 'NONE',  ( 5.719274019375991003, -21.55341960407610458, 92.70724293864770971 ) ) ;
#52204=CARTESIAN_POINT ( 'NONE',  ( 9.564922557960805705, 16.46253265017160317, 79.58224293864769550 ) ) ;
#52205=CARTESIAN_POINT ( 'NONE',  ( 16.46253265017160672, -9.564922557960803928, 83.33224293864768129 ) ) ;
#52206=CARTESIAN_POINT ( 'NONE',  ( -5.823673210054116645, -21.52544592524344225, 112.2905762719810241 ) ) ;
#52208=CARTESIAN_POINT ( 'NONE',  ( 19.05341960407611168, 5.049401038298154454, 73.95724293864768129 ) ) ;
#52211=CARTESIAN_POINT ( 'NONE',  ( -19.03943276465977164, 0.05219959533909376836, 21.24890960531436335 ) ) ;
#52212=CARTESIAN_POINT ( 'NONE',  ( -19.03943276465977164, 0.05219959533909376836, 31.24890960531435979 ) ) ;
#52213=CARTESIAN_POINT ( 'NONE',  ( -0.05219959533936034679, 19.03943276465977164, 92.50109039468566152 ) ) ;
#52214=CARTESIAN_POINT ( 'NONE',  ( 12.06949235617757843, -12.14591786802309237, 108.1239096053143811 ) ) ;
#52215=CARTESIAN_POINT ( 'NONE',  ( -5.719274019375665041, -21.55341960407619695, 69.79275706135234714 ) ) ;
#52216=CARTESIAN_POINT ( 'NONE',  ( -16.51473224551069308, -9.474510206698971260, 66.66557627198102409 ) ) ;
#52217=CARTESIAN_POINT ( 'NONE',  ( -18.62759615963255300, -10.81492255796106328, 39.16775706135235424 ) ) ;
#52218=CARTESIAN_POINT ( 'NONE',  ( 21.55341960407610458, 5.719274019375980345, 113.9572429386477239 ) ) ;
#52220=CARTESIAN_POINT ( 'NONE',  ( -9.474510206698964154, 16.51473224551069663, 85.41557627198102409 ) ) ;
#52222=CARTESIAN_POINT ( 'NONE',  ( -0.05219959533934338120, 16.53943276465976808, 27.50109039468567929 ) ) ;
#52223=CARTESIAN_POINT ( 'NONE',  ( 5.823673210054125526, 21.52544592524343514, 34.79057627198103120 ) ) ;
#52224=CARTESIAN_POINT ( 'NONE',  ( 15.72974639402176855, 15.80617190586768217, 61.87609039468568284 ) ) ;
#52225=CARTESIAN_POINT ( 'NONE',  ( 13.89961937509977652, -13.97604488694527269, 108.1239096053143669 ) ) ;
#52226=CARTESIAN_POINT ( 'NONE',  ( -13.97604488694547697, 13.89961937509957934, 103.1260903946856473 ) ) ;
#52227=CARTESIAN_POINT ( 'NONE',  ( -19.05341960407611168, -5.049401038298163336, 51.45724293864770260 ) ) ;
#52228=CARTESIAN_POINT ( 'NONE',  ( -13.97604488694527625, -13.89961937509977652, 81.87390960531436690 ) ) ;
#52229=CARTESIAN_POINT ( 'NONE',  ( 4.483927247898545687, 16.52544592524342804, 94.79057627198105251 ) ) ;
#52231=CARTESIAN_POINT ( 'NONE',  ( -14.29746914071049879, 8.314922557960819915, 85.83224293864768129 ) ) ;
#52232=CARTESIAN_POINT ( 'NONE',  ( -9.564922557960796823, -16.46253265017161027, 107.0822429386476955 ) ) ;
#52233=CARTESIAN_POINT ( 'NONE',  ( -8.224510206698948167, 14.34966873604960824, 60.41557627198102409 ) ) ;
#52234=CARTESIAN_POINT ( 'NONE',  ( -13.97604488694527625, -13.89961937509977652, 41.87390960531435979 ) ) ;
#52235=CARTESIAN_POINT ( 'NONE',  ( -21.55341960407619339, 5.719274019375674811, 58.54275706135235424 ) ) ;
#52236=CARTESIAN_POINT ( 'NONE',  ( -19.05341960407617563, 5.049401038297882671, 93.54275706135234714 ) ) ;
#52237=CARTESIAN_POINT ( 'NONE',  ( 16.53943276465976808, -0.05219959533910856209, 48.74890960531435979 ) ) ;
#52238=CARTESIAN_POINT ( 'NONE',  ( -15.72974639402197994, 15.80617190586746368, 115.6239096053143669 ) ) ;
#52239=CARTESIAN_POINT ( 'NONE',  ( 10.81492255796078972, 18.62759615963270932, 44.58224293864769550 ) ) ;
#52240=CARTESIAN_POINT ( 'NONE',  ( 9.474510206698971260, -16.51473224551069308, 112.9155762719810383 ) ) ;
#52242=CARTESIAN_POINT ( 'NONE',  ( 19.03943276465977164, -0.05219959533909143690, 53.74890960531436690 ) ) ;
#52243=CARTESIAN_POINT ( 'NONE',  ( -16.52544592524342804, 4.483927247898546575, 31.04057627198102409 ) ) ;
#52244=CARTESIAN_POINT ( 'NONE',  ( 16.55341960407618274, -4.379528057220086978, 96.04275706135236135 ) ) ;
#52245=CARTESIAN_POINT ( 'NONE',  ( 4.483927247898790824, -16.52544592524335698, 90.20942372801903275 ) ) ;
#52246=CARTESIAN_POINT ( 'NONE',  ( 5.049401038297881783, 19.05341960407617563, 42.29275706135234003 ) ) ;
#52247=CARTESIAN_POINT ( 'NONE',  ( -17.40805194822030799, 6.112264579159339739, 70.83371272510613892 ) ) ;
#52248=CARTESIAN_POINT ( 'NONE',  ( 16.46253265017160672, -9.564922557960803928, 88.33224293864769550 ) ) ;
#52249=CARTESIAN_POINT ( 'NONE',  ( -16.51473224551069308, -9.474510206698971260, 56.66557627198103120 ) ) ;
#52250=CARTESIAN_POINT ( 'NONE',  ( -0.05219959533910754901, -16.53943276465976808, 62.49890960531436690 ) ) ;
#52251=CARTESIAN_POINT ( 'NONE',  ( 9.474510206698971260, -16.51473224551069308, 22.91557627198102765 ) ) ;
#52252=CARTESIAN_POINT ( 'NONE',  ( 18.67979575497178502, 10.72451020669898547, 29.16557627198103120 ) ) ;
#52253=CARTESIAN_POINT ( 'NONE',  ( 5.823673210054125526, 21.52544592524343514, 39.79057627198103830 ) ) ;
#52254=CARTESIAN_POINT ( 'NONE',  ( -12.06949235617756955, 12.14591786802309770, 90.62390960531436690 ) ) ;
#52255=CARTESIAN_POINT ( 'NONE',  ( 16.55341960407618274, -4.379528057220086978, 41.04275706135236135 ) ) ;
#52256=CARTESIAN_POINT ( 'NONE',  ( 16.55341960407611168, 4.379528057220329451, 83.95724293864770971 ) ) ;
#52258=CARTESIAN_POINT ( 'NONE',  ( -19.03943276465977164, -0.05219959533935918106, 83.75109039468567573 ) ) ;
#52259=CARTESIAN_POINT ( 'NONE',  ( 13.89961937509977652, -13.97604488694527269, 108.1239096053143669 ) ) ;
#52262=CARTESIAN_POINT ( 'NONE',  ( 12.14591786802327356, -12.06949235617739191, 30.62609039468567929 ) ) ;
#52263=CARTESIAN_POINT ( 'NONE',  ( 8.224510206698742110, 14.34966873604972548, 112.0844237280190185 ) ) ;
#52264=CARTESIAN_POINT ( 'NONE',  ( 19.05341960407617918, -5.049401038297876454, 66.04275706135233293 ) ) ;
#52265=CARTESIAN_POINT ( 'NONE',  ( -21.55341960407610458, -5.719274019375992779, 41.45724293864769550 ) ) ;
#52266=CARTESIAN_POINT ( 'NONE',  ( -15.72974639402176322, -15.80617190586768395, 64.37609039468568994 ) ) ;
#52268=CARTESIAN_POINT ( 'NONE',  ( 8.314922557961029526, -14.29746914071037800, 35.41775706135234003 ) ) ;
#52269=CARTESIAN_POINT ( 'NONE',  ( -5.153800228976328057, -19.02544592524343514, 22.29057627198102765 ) ) ;
#52270=CARTESIAN_POINT ( 'NONE',  ( -19.05341960407611168, -5.049401038298163336, 86.45724293864769550 ) ) ;
#52272=CARTESIAN_POINT ( 'NONE',  ( -4.483927247898539470, -16.52544592524342804, 87.29057627198103830 ) ) ;
#52274=CARTESIAN_POINT ( 'NONE',  ( 13.97604488694527802, 13.89961937509977652, 89.37390960531436690 ) ) ;
#52276=CARTESIAN_POINT ( 'NONE',  ( -19.02544592524334988, -5.153800228976617603, 108.9594237280189759 ) ) ;
#52277=CARTESIAN_POINT ( 'NONE',  ( -0.05219959533907301413, -21.53943276465977519, 82.49890960531436690 ) ) ;
#52278=CARTESIAN_POINT ( 'NONE',  ( 13.97604488694527802, 13.89961937509977652, 39.37390960531435269 ) ) ;
#52279=CARTESIAN_POINT ( 'NONE',  ( -19.05341960407617563, 5.049401038297882671, 63.54275706135234003 ) ) ;
#52280=CARTESIAN_POINT ( 'NONE',  ( -18.62759615963270932, 10.81492255796079327, 115.8322429386477097 ) ) ;
#52281=CARTESIAN_POINT ( 'NONE',  ( 16.46253265017160672, -9.564922557960803928, 63.33224293864769550 ) ) ;
#52282=CARTESIAN_POINT ( 'NONE',  ( -5.049401038298153566, 19.05341960407611168, 105.2072429386476671 ) ) ;
#52284=CARTESIAN_POINT ( 'NONE',  ( 12.06949235617739724, 12.14591786802326823, 36.87609039468568994 ) ) ;
#52286=CARTESIAN_POINT ( 'NONE',  ( 5.823673210054125526, 21.52544592524343514, 109.7905762719810383 ) ) ;
#52287=CARTESIAN_POINT ( 'NONE',  ( 16.53943276465976808, -0.05219959533910856209, 108.7489096053143669 ) ) ;
#52288=CARTESIAN_POINT ( 'NONE',  ( 13.89961937509977652, -13.97604488694527269, 88.12390960531438111 ) ) ;
#52289=CARTESIAN_POINT ( 'NONE',  ( -9.474510206698720793, -16.51473224551083518, 64.58442372801900433 ) ) ;
#52290=CARTESIAN_POINT ( 'NONE',  ( -15.80617190586745835, -15.72974639402198527, 81.87390960531435269 ) ) ;
#52291=CARTESIAN_POINT ( 'NONE',  ( -12.14591786802309592, -12.06949235617757132, 46.87390960531435979 ) ) ;
#52292=CARTESIAN_POINT ( 'NONE',  ( -13.89961937509957401, -13.97604488694547875, 19.37609039468566507 ) ) ;
#52293=CARTESIAN_POINT ( 'NONE',  ( 12.14591786802327356, -12.06949235617739191, 65.62609039468568994 ) ) ;
#52294=CARTESIAN_POINT ( 'NONE',  ( -5.153800228976328057, -19.02544592524343514, 87.29057627198103830 ) ) ;
#52295=CARTESIAN_POINT ( 'NONE',  ( 13.89961937509977652, -13.97604488694527269, 48.12390960531435979 ) ) ;
#52296=CARTESIAN_POINT ( 'NONE',  ( 5.823673210054444382, -21.52544592524334988, 50.20942372801901854 ) ) ;
#52297=CARTESIAN_POINT ( 'NONE',  ( -10.81492255796105439, 18.62759615963255655, 72.91775706135234714 ) ) ;
#52298=CARTESIAN_POINT ( 'NONE',  ( 19.05341960407611168, 5.049401038298154454, 58.95724293864768129 ) ) ;
#52299=CARTESIAN_POINT ( 'NONE',  ( 5.823673210054444382, -21.52544592524334988, 40.20942372801901854 ) ) ;
#52300=CARTESIAN_POINT ( 'NONE',  ( -0.05219959533936034679, 19.03943276465977164, 77.50109039468566152 ) ) ;
#52301=EDGE_CURVE ( 'NONE', #189322, #81647, #70599, .T. ) ;
#52302=CARTESIAN_POINT ( 'NONE',  ( -9.474510206698720793, -16.51473224551083518, 69.58442372801901854 ) ) ;
#52303=CARTESIAN_POINT ( 'NONE',  ( 16.51473224551069308, 9.474510206698969483, 44.16557627198103120 ) ) ;
#52304=CARTESIAN_POINT ( 'NONE',  ( -16.52544592524335698, -4.483927247898792601, 88.95942372801901854 ) ) ;
#52305=CARTESIAN_POINT ( 'NONE',  ( -16.51473224551069308, -9.474510206698971260, 46.66557627198102409 ) ) ;
#52307=CARTESIAN_POINT ( 'NONE',  ( -9.564922557960796823, -16.46253265017161027, 97.08224293864769550 ) ) ;
#52308=CARTESIAN_POINT ( 'NONE',  ( 5.049401038298161559, -19.05341960407611168, 37.70724293864768839 ) ) ;
#52309=CARTESIAN_POINT ( 'NONE',  ( 21.55341960407610458, 5.719274019375980345, 83.95724293864770971 ) ) ;
#52310=CARTESIAN_POINT ( 'NONE',  ( 16.52544592524335698, 4.483927247898782831, 56.45942372801902565 ) ) ;
#52311=CARTESIAN_POINT ( 'NONE',  ( -0.05219959533936034679, 19.03943276465977164, 27.50109039468566507 ) ) ;
#52312=CARTESIAN_POINT ( 'NONE',  ( -13.97604488694527625, -13.89961937509977652, 56.87390960531434558 ) ) ;
#52313=CARTESIAN_POINT ( 'NONE',  ( 16.55341960407611168, 4.379528057220329451, 38.95724293864768839 ) ) ;
#52314=CARTESIAN_POINT ( 'NONE',  ( -12.14591786802309592, -12.06949235617757132, 86.87390960531438111 ) ) ;
#52315=CARTESIAN_POINT ( 'NONE',  ( 5.153800228976335163, 19.02544592524342804, 89.79057627198102409 ) ) ;
#52316=CARTESIAN_POINT ( 'NONE',  ( 16.51473224551069308, 9.474510206698969483, 79.16557627198103830 ) ) ;
#52317=CARTESIAN_POINT ( 'NONE',  ( 21.55341960407619695, -5.719274019375665929, 31.04275706135234714 ) ) ;
#52318=CARTESIAN_POINT ( 'NONE',  ( -9.474510206698964154, 16.51473224551069663, 90.41557627198103830 ) ) ;
#52319=CARTESIAN_POINT ( 'NONE',  ( 15.72974639402176855, 15.80617190586768217, 101.8760903946857042 ) ) ;
#52320=CARTESIAN_POINT ( 'NONE',  ( 4.379528057220092307, 16.55341960407617563, 82.29275706135234714 ) ) ;
#52322=CARTESIAN_POINT ( 'NONE',  ( 10.72451020669871369, 18.67979575497193778, 32.08442372801901854 ) ) ;
#52323=CARTESIAN_POINT ( 'NONE',  ( -18.62759615963270932, 10.81492255796079327, 90.83224293864769550 ) ) ;
#52324=CARTESIAN_POINT ( 'NONE',  ( -14.29746914071049879, 8.314922557960819915, 45.83224293864769550 ) ) ;
#52325=CARTESIAN_POINT ( 'NONE',  ( -19.02544592524342804, 5.153800228976336051, 36.04057627198100988 ) ) ;
#52326=CARTESIAN_POINT ( 'NONE',  ( 12.14591786802309770, 12.06949235617756955, 69.37390960531436690 ) ) ;
#52327=CARTESIAN_POINT ( 'NONE',  ( 18.67979575497178502, 10.72451020669898547, 29.16557627198103120 ) ) ;
#52328=CARTESIAN_POINT ( 'NONE',  ( 5.153800228976615827, -19.02544592524334988, 25.20942372801900433 ) ) ;
#52329=CARTESIAN_POINT ( 'NONE',  ( -16.53943276465976808, 0.05219959533911058130, 96.24890960531435269 ) ) ;
#52330=CARTESIAN_POINT ( 'NONE',  ( 19.02544592524343514, -5.153800228976328945, 108.5405762719810383 ) ) ;
#52332=CARTESIAN_POINT ( 'NONE',  ( 0.05219959533934541429, -16.53943276465976808, 50.00109039468568994 ) ) ;
#52333=CARTESIAN_POINT ( 'NONE',  ( -5.153800228976328057, -19.02544592524343514, 57.29057627198103120 ) ) ;
#52335=CARTESIAN_POINT ( 'NONE',  ( -21.53943276465977519, 0.05219959533907696930, 21.24890960531436690 ) ) ;
#52336=CARTESIAN_POINT ( 'NONE',  ( 8.314922557961029526, -14.29746914071037800, 90.41775706135236135 ) ) ;
#52337=CARTESIAN_POINT ( 'NONE',  ( -9.474510206698720793, -16.51473224551083518, 109.5844237280190043 ) ) ;
#52338=CARTESIAN_POINT ( 'NONE',  ( 21.53943276465977519, 0.05219959533937863772, 86.25109039468568994 ) ) ;
#52339=CARTESIAN_POINT ( 'NONE',  ( 19.03943276465977164, -0.05219959533909143690, 78.74890960531436690 ) ) ;
#52340=CARTESIAN_POINT ( 'NONE',  ( 5.719274019375991003, -21.55341960407610458, 107.7072429386476955 ) ) ;
#52341=CARTESIAN_POINT ( 'NONE',  ( -14.29746914071037622, -8.314922557961029526, 54.16775706135235424 ) ) ;
#52342=CARTESIAN_POINT ( 'NONE',  ( 14.34966873604960469, 8.224510206698951720, 114.1655762719810383 ) ) ;
#52343=CARTESIAN_POINT ( 'NONE',  ( 8.314922557961029526, -14.29746914071037800, 20.41775706135234714 ) ) ;
#52344=CARTESIAN_POINT ( 'NONE',  ( 19.03943276465977164, 0.05219959533936151252, 86.25109039468567573 ) ) ;
#52345=CARTESIAN_POINT ( 'NONE',  ( -18.62759615963270932, 10.81492255796079327, 70.83224293864770971 ) ) ;
#52346=CARTESIAN_POINT ( 'NONE',  ( 13.97604488694548053, -13.89961937509957401, 50.62609039468566152 ) ) ;
#52347=DIRECTION ( 'NONE',  ( -1.000000000000000000, -0.000000000000000000, -0.000000000000000000 ) ) ;
#52348=CARTESIAN_POINT ( 'NONE',  ( -10.72451020669898014, 18.67979575497178502, 105.4155762719810383 ) ) ;
#52349=LINE ( 'NONE', #162523, #104880 ) ;
#52350=CARTESIAN_POINT ( 'NONE',  ( -19.02544592524342804, 5.153800228976336051, 71.04057627198099567 ) ) ;
#52352=CARTESIAN_POINT ( 'NONE',  ( -12.06949235617739369, -12.14591786802326823, 24.37609039468567573 ) ) ;
#52354=CARTESIAN_POINT ( 'NONE',  ( -18.67979575497178146, -10.72451020669898902, 106.6655762719810383 ) ) ;
#52355=CARTESIAN_POINT ( 'NONE',  ( -16.55341960407611168, -4.379528057220339221, 66.45724293864768129 ) ) ;
#52356=CARTESIAN_POINT ( 'NONE',  ( -19.05341960407611168, -5.049401038298163336, 71.45724293864766707 ) ) ;
#52357=CARTESIAN_POINT ( 'NONE',  ( -21.52544592524334988, -5.823673210054445271, 68.95942372801901854 ) ) ;
#52358=CARTESIAN_POINT ( 'NONE',  ( -12.14591786802326823, 12.06949235617739902, 23.12609039468567573 ) ) ;
#52359=CARTESIAN_POINT ( 'NONE',  ( 9.474510206698729675, 16.51473224551082808, 37.08442372801899722 ) ) ;
#52360=CARTESIAN_POINT ( 'NONE',  ( 15.80617190586769283, -15.72974639402175789, 50.62609039468568994 ) ) ;
#52361=CARTESIAN_POINT ( 'NONE',  ( 15.72974639402176855, 15.80617190586768217, 21.87609039468567573 ) ) ;
#52362=CARTESIAN_POINT ( 'NONE',  ( 21.53943276465977519, -0.05219959533907433946, 63.74890960531435979 ) ) ;
#52363=CARTESIAN_POINT ( 'NONE',  ( 0.05219959533936267826, -19.03943276465977164, 110.0010903946856757 ) ) ;
#52364=CARTESIAN_POINT ( 'NONE',  ( -16.51473224551069308, -9.474510206698971260, 41.66557627198103120 ) ) ;
#52365=CARTESIAN_POINT ( 'NONE',  ( -19.03943276465977164, -0.05219959533935918106, 68.75109039468566152 ) ) ;
#52366=CARTESIAN_POINT ( 'NONE',  ( -5.719274019375665041, -21.55341960407619695, 84.79275706135234714 ) ) ;
#52367=CARTESIAN_POINT ( 'NONE',  ( 19.02544592524334988, 5.153800228976608722, 56.45942372801898301 ) ) ;
#52368=CARTESIAN_POINT ( 'NONE',  ( -19.05341960407611168, -5.049401038298163336, 36.45724293864766707 ) ) ;
#52369=CARTESIAN_POINT ( 'NONE',  ( 5.823673210054125526, 21.52544592524343514, 59.79057627198103120 ) ) ;
#52370=CARTESIAN_POINT ( 'NONE',  ( 8.314922557960818139, 14.29746914071049879, 49.58224293864769550 ) ) ;
#52372=CARTESIAN_POINT ( 'NONE',  ( -13.97604488694547697, 13.89961937509957934, 33.12609039468566863 ) ) ;
#52373=CARTESIAN_POINT ( 'NONE',  ( -0.05219959533934338120, 16.53943276465976808, 82.50109039468568994 ) ) ;
#52374=CARTESIAN_POINT ( 'NONE',  ( 8.224510206698953496, -14.34966873604960469, 47.91557627198102409 ) ) ;
#52375=CARTESIAN_POINT ( 'NONE',  ( 5.719274019375673035, 21.55341960407619339, 87.29275706135236135 ) ) ;
#52376=CARTESIAN_POINT ( 'NONE',  ( -21.55341960407619339, 5.719274019375674811, 83.54275706135234714 ) ) ;
#52377=CARTESIAN_POINT ( 'NONE',  ( -18.67979575497178146, -10.72451020669898902, 81.66557627198103830 ) ) ;
#52378=CARTESIAN_POINT ( 'NONE',  ( -16.51473224551069308, -9.474510206698971260, 46.66557627198102409 ) ) ;
#52379=CARTESIAN_POINT ( 'NONE',  ( 21.52544592524334988, 5.823673210054432836, 61.45942372801901854 ) ) ;
#52380=CARTESIAN_POINT ( 'NONE',  ( 19.03943276465977164, -0.05219959533909143690, 33.74890960531435979 ) ) ;
#52381=ORIENTED_EDGE ( 'NONE', *, *, #81680, .F. ) ;
#52382=CARTESIAN_POINT ( 'NONE',  ( 13.89961937509977652, -13.97604488694527269, 53.12390960531434558 ) ) ;
#52383=CARTESIAN_POINT ( 'NONE',  ( -0.05219959533910754901, -16.53943276465976808, 112.4989096053143669 ) ) ;
#52384=CARTESIAN_POINT ( 'NONE',  ( -9.564922557960796823, -16.46253265017161027, 102.0822429386477097 ) ) ;
#52385=CARTESIAN_POINT ( 'NONE',  ( 16.52544592524342804, -4.483927247898539470, 53.54057627198103120 ) ) ;
#52386=CARTESIAN_POINT ( 'NONE',  ( -0.05219959533910754901, -16.53943276465976808, 112.4989096053143669 ) ) ;
#52387=CARTESIAN_POINT ( 'NONE',  ( 10.72451020669898902, -18.67979575497178502, 87.91557627198103830 ) ) ;
#52388=CARTESIAN_POINT ( 'NONE',  ( 18.62759615963271287, -10.81492255796078972, 113.3322429386476955 ) ) ;
#52390=CARTESIAN_POINT ( 'NONE',  ( -8.224510206698735004, -14.34966873604973081, 39.58442372801901143 ) ) ;
#52392=CARTESIAN_POINT ( 'NONE',  ( -21.55341960407610458, -5.719274019375992779, 71.45724293864769550 ) ) ;
#52393=CARTESIAN_POINT ( 'NONE',  ( -21.52544592524334988, -5.823673210054445271, 103.9594237280190185 ) ) ;
#52394=CARTESIAN_POINT ( 'NONE',  ( -13.97604488694527625, -13.89961937509977652, 91.87390960531432427 ) ) ;
#52395=CARTESIAN_POINT ( 'NONE',  ( 15.72974639402176855, 15.80617190586768217, 26.87609039468567218 ) ) ;
#52396=CARTESIAN_POINT ( 'NONE',  ( -5.719274019375978568, 21.55341960407610458, 35.20724293864768839 ) ) ;
#52397=CARTESIAN_POINT ( 'NONE',  ( 16.53943276465976808, 0.05219959533934440121, 106.2510903946856757 ) ) ;
#52398=CARTESIAN_POINT ( 'NONE',  ( -5.719274019375665041, -21.55341960407619695, 44.79275706135234714 ) ) ;
#52399=CARTESIAN_POINT ( 'NONE',  ( -5.719274019375665041, -21.55341960407619695, 84.79275706135234714 ) ) ;
#52400=CARTESIAN_POINT ( 'NONE',  ( 13.89961937509957401, 13.97604488694547697, 21.87609039468566152 ) ) ;
#52401=CARTESIAN_POINT ( 'NONE',  ( -12.06949235617739369, -12.14591786802326823, 74.37609039468568994 ) ) ;
#52402=CARTESIAN_POINT ( 'NONE',  ( -15.80617190586768217, 15.72974639402176855, 38.12609039468567573 ) ) ;
#52403=CARTESIAN_POINT ( 'NONE',  ( -9.474510206698964154, 16.51473224551069663, 35.41557627198102409 ) ) ;
#52404=CARTESIAN_POINT ( 'NONE',  ( 18.62759615963255655, 10.81492255796105972, 96.66775706135234714 ) ) ;
#52405=CARTESIAN_POINT ( 'NONE',  ( -5.049401038298153566, 19.05341960407611168, 110.2072429386476671 ) ) ;
#52406=CARTESIAN_POINT ( 'NONE',  ( 18.67979575497178502, 10.72451020669898547, 104.1655762719810241 ) ) ;
#52408=CARTESIAN_POINT ( 'NONE',  ( 10.72451020669898902, -18.67979575497178502, 67.91557627198102409 ) ) ;
#52409=CARTESIAN_POINT ( 'NONE',  ( -12.14591786802326823, 12.06949235617739902, 58.12609039468568994 ) ) ;
#52410=CARTESIAN_POINT ( 'NONE',  ( -4.483927247898539470, -16.52544592524342804, 52.29057627198102409 ) ) ;
#52412=CARTESIAN_POINT ( 'NONE',  ( 5.049401038297881783, 19.05341960407617563, 82.29275706135229029 ) ) ;
#52413=CARTESIAN_POINT ( 'NONE',  ( -16.36317988757056696, 7.306389748694939179, 104.0978960836323211 ) ) ;
#52414=CARTESIAN_POINT ( 'NONE',  ( -0.05219959533934338120, 16.53943276465976808, 27.50109039468567929 ) ) ;
#52415=CARTESIAN_POINT ( 'NONE',  ( 21.52544592524344225, -5.823673210054117533, 98.54057627198105251 ) ) ;
#52416=CARTESIAN_POINT ( 'NONE',  ( -4.379528057220328563, 16.55341960407611168, 70.20724293864769550 ) ) ;
#52417=CARTESIAN_POINT ( 'NONE',  ( -19.02544592524342804, 5.153800228976336051, 116.0405762719810383 ) ) ;
#52418=CARTESIAN_POINT ( 'NONE',  ( -16.55341960407617563, 4.379528057220093196, 38.54275706135234714 ) ) ;
#52419=CARTESIAN_POINT ( 'NONE',  ( 19.02544592524343514, -5.153800228976328945, 58.54057627198102409 ) ) ;
#52420=CARTESIAN_POINT ( 'NONE',  ( -18.67979575497193778, 10.72451020669871902, 23.33442372801901499 ) ) ;
#52421=CARTESIAN_POINT ( 'NONE',  ( 19.02544592524334988, 5.153800228976608722, 91.45942372801900433 ) ) ;
#52422=CARTESIAN_POINT ( 'NONE',  ( 13.89961937509977652, -13.97604488694527269, 113.1239096053143527 ) ) ;
#52423=CARTESIAN_POINT ( 'NONE',  ( 16.46253265017160672, -9.564922557960803928, 88.33224293864769550 ) ) ;
#52424=CARTESIAN_POINT ( 'NONE',  ( 18.67979575497178502, 10.72451020669898547, 89.16557627198102409 ) ) ;
#52425=CARTESIAN_POINT ( 'NONE',  ( -19.02544592524342804, 5.153800228976336051, 66.04057627198103830 ) ) ;
#52427=CARTESIAN_POINT ( 'NONE',  ( 16.53943276465976808, -0.05219959533910856209, 68.74890960531435269 ) ) ;
#52428=CARTESIAN_POINT ( 'NONE',  ( -16.51473224551069308, -9.474510206698971260, 101.6655762719810241 ) ) ;
#52430=CARTESIAN_POINT ( 'NONE',  ( 9.474510206698729675, 16.51473224551082808, 77.08442372801900433 ) ) ;
#52431=CARTESIAN_POINT ( 'NONE',  ( 5.823673210054125526, 21.52544592524343514, 89.79057627198103830 ) ) ;
#52432=CARTESIAN_POINT ( 'NONE',  ( -9.474510206698720793, -16.51473224551083518, 44.58442372801900433 ) ) ;
#52433=CARTESIAN_POINT ( 'NONE',  ( -21.53943276465977519, 0.05219959533907696930, 21.24890960531436690 ) ) ;
#52435=CARTESIAN_POINT ( 'NONE',  ( -10.81492255796078084, -18.62759615963271287, 52.08224293864768839 ) ) ;
#52436=CARTESIAN_POINT ( 'NONE',  ( -9.474510206698964154, 16.51473224551069663, 85.41557627198102409 ) ) ;
#52437=CARTESIAN_POINT ( 'NONE',  ( 5.823673210054444382, -21.52544592524334988, 75.20942372801901854 ) ) ;
#52438=CARTESIAN_POINT ( 'NONE',  ( -9.474510206698964154, 16.51473224551069663, 40.41557627198103120 ) ) ;
#52439=CARTESIAN_POINT ( 'NONE',  ( 14.34966873604960469, 8.224510206698951720, 69.16557627198102409 ) ) ;
#52440=CARTESIAN_POINT ( 'NONE',  ( -16.53943276465976808, -0.05219959533934237506, 28.75109039468567929 ) ) ;
#52441=CARTESIAN_POINT ( 'NONE',  ( -0.05219959533937732626, 21.53943276465977519, 67.50109039468568994 ) ) ;
#52442=ORIENTED_EDGE ( 'NONE', *, *, #11302, .T. ) ;
#52443=LINE ( 'NONE', #86776, #107634 ) ;
#52444=CARTESIAN_POINT ( 'NONE',  ( -13.97604488694547697, 13.89961937509957934, 83.12609039468564731 ) ) ;
#52446=CARTESIAN_POINT ( 'NONE',  ( 17.50000000000000000, 5.499999999999997335, 111.7030961746582847 ) ) ;
#52447=CARTESIAN_POINT ( 'NONE',  ( -10.72451020669898014, 18.67979575497178502, 115.4155762719810241 ) ) ;
#52449=CARTESIAN_POINT ( 'NONE',  ( -15.80617190586768217, 15.72974639402176855, 108.1260903946856757 ) ) ;
#52450=CARTESIAN_POINT ( 'NONE',  ( -0.05219959533909027116, -19.03943276465977164, 62.49890960531435979 ) ) ;
#52451=CARTESIAN_POINT ( 'NONE',  ( -21.53943276465977519, -0.05219959533937600094, 113.7510903946856757 ) ) ;
#52452=CARTESIAN_POINT ( 'NONE',  ( -12.14591786802326823, 12.06949235617739902, 108.1260903946856757 ) ) ;
#52453=CARTESIAN_POINT ( 'NONE',  ( -19.02544592524342804, 5.153800228976336051, 96.04057627198103830 ) ) ;
#52454=CARTESIAN_POINT ( 'NONE',  ( 10.72451020669871369, 18.67979575497193778, 77.08442372801901854 ) ) ;
#52456=CARTESIAN_POINT ( 'NONE',  ( -17.49999999999996447, -3.471454075611972723, 35.51667418855652869 ) ) ;
#52457=CARTESIAN_POINT ( 'NONE',  ( 15.80617190586769283, -15.72974639402175789, 75.62609039468567573 ) ) ;
#52458=CARTESIAN_POINT ( 'NONE',  ( -21.55341960407619339, 5.719274019375674811, 103.5427570613523613 ) ) ;
#52460=CARTESIAN_POINT ( 'NONE',  ( -5.153800228976328057, -19.02544592524343514, 82.29057627198103830 ) ) ;
#52461=CARTESIAN_POINT ( 'NONE',  ( -9.474510206698720793, -16.51473224551083518, 24.58442372801900078 ) ) ;
#52463=CARTESIAN_POINT ( 'NONE',  ( -19.02544592524342804, 5.153800228976336051, 36.04057627198100988 ) ) ;
#52464=CARTESIAN_POINT ( 'NONE',  ( -10.81492255796078084, -18.62759615963271287, 57.08224293864769550 ) ) ;
#52465=CARTESIAN_POINT ( 'NONE',  ( -14.29746914071037622, -8.314922557961029526, 109.1677570613523613 ) ) ;
#52466=CARTESIAN_POINT ( 'NONE',  ( -8.314922557960811034, -14.29746914071050412, 102.0822429386476955 ) ) ;
#52467=CARTESIAN_POINT ( 'NONE',  ( 5.153800228976335163, 19.02544592524342804, 79.79057627198102409 ) ) ;
#52468=CARTESIAN_POINT ( 'NONE',  ( -18.67979575497193778, 10.72451020669871902, 98.33442372801901854 ) ) ;
#52469=CARTESIAN_POINT ( 'NONE',  ( -13.97604488694527625, -13.89961937509977652, 31.87390960531435979 ) ) ;
#52470=CARTESIAN_POINT ( 'NONE',  ( 8.224510206698953496, -14.34966873604960469, 102.9155762719810383 ) ) ;
#52471=CARTESIAN_POINT ( 'NONE',  ( 0.05219959533937995610, -21.53943276465977519, 50.00109039468568994 ) ) ;
#52472=CARTESIAN_POINT ( 'NONE',  ( -18.67979575497178146, -10.72451020669898902, 81.66557627198103830 ) ) ;
#52473=CARTESIAN_POINT ( 'NONE',  ( -5.153800228976607833, 19.02544592524334988, 47.70942372801900433 ) ) ;
#52475=CARTESIAN_POINT ( 'NONE',  ( 19.03943276465977164, -0.05219959533909143690, 98.74890960531436690 ) ) ;
#52476=CARTESIAN_POINT ( 'NONE',  ( -4.379528057220328563, 16.55341960407611168, 80.20724293864769550 ) ) ;
#52477=CARTESIAN_POINT ( 'NONE',  ( -19.02544592524334988, -5.153800228976617603, 43.95942372801899012 ) ) ;
#52478=CARTESIAN_POINT ( 'NONE',  ( 19.05341960407611168, 5.049401038298154454, 58.95724293864768129 ) ) ;
#52479=CARTESIAN_POINT ( 'NONE',  ( -16.52544592524342804, 4.483927247898546575, 46.04057627198103830 ) ) ;
#52480=CARTESIAN_POINT ( 'NONE',  ( -9.564922557961040184, 16.46253265017147172, 72.91775706135233293 ) ) ;
#52481=CARTESIAN_POINT ( 'NONE',  ( 0.05219959533936267826, -19.03943276465977164, 90.00109039468567573 ) ) ;
#52482=CARTESIAN_POINT ( 'NONE',  ( -5.719274019375978568, 21.55341960407610458, 40.20724293864769550 ) ) ;
#52483=CARTESIAN_POINT ( 'NONE',  ( -16.53943276465976808, 0.05219959533911058130, 101.2489096053143669 ) ) ;
#52485=CARTESIAN_POINT ( 'NONE',  ( -19.05341960407611168, -5.049401038298163336, 56.45724293864768129 ) ) ;
#52486=CARTESIAN_POINT ( 'NONE',  ( -21.52544592524343514, 5.823673210054127303, 66.04057627198103830 ) ) ;
#52487=CARTESIAN_POINT ( 'NONE',  ( -16.46253265017160317, 9.564922557960807481, 30.83224293864769550 ) ) ;
#52488=CARTESIAN_POINT ( 'NONE',  ( 4.483927247898790824, -16.52544592524335698, 80.20942372801901854 ) ) ;
#52489=CARTESIAN_POINT ( 'NONE',  ( 5.153800228976335163, 19.02544592524342804, 54.79057627198103120 ) ) ;
#52490=CARTESIAN_POINT ( 'NONE',  ( -13.89961937509957401, -13.97604488694547875, 54.37609039468565442 ) ) ;
#52491=CARTESIAN_POINT ( 'NONE',  ( -18.62759615963255300, -10.81492255796106328, 69.16775706135234714 ) ) ;
#52492=CARTESIAN_POINT ( 'NONE',  ( -10.72451020669898014, 18.67979575497178502, 45.41557627198103830 ) ) ;
#52493=CARTESIAN_POINT ( 'NONE',  ( -8.224510206698948167, 14.34966873604960824, 115.4155762719810241 ) ) ;
#52494=CARTESIAN_POINT ( 'NONE',  ( 4.483927247898790824, -16.52544592524335698, 85.20942372801901854 ) ) ;
#52495=CARTESIAN_POINT ( 'NONE',  ( -16.46253265017146816, -9.564922557961047289, 99.16775706135233293 ) ) ;
#52496=CARTESIAN_POINT ( 'NONE',  ( -0.05219959533909027116, -19.03943276465977164, 27.49890960531435624 ) ) ;
#52498=CARTESIAN_POINT ( 'NONE',  ( -18.62759615963270932, 10.81492255796079327, 60.83224293864769550 ) ) ;
#52499=CARTESIAN_POINT ( 'NONE',  ( -21.52544592524334988, -5.823673210054445271, 78.95942372801901854 ) ) ;
#52500=CARTESIAN_POINT ( 'NONE',  ( 4.379528057220339221, -16.55341960407611168, 47.70724293864770260 ) ) ;
#52501=CARTESIAN_POINT ( 'NONE',  ( -14.29746914071049879, 8.314922557960819915, 50.83224293864770971 ) ) ;
#52502=CARTESIAN_POINT ( 'NONE',  ( -5.719274019375978568, 21.55341960407610458, 80.20724293864769550 ) ) ;
#52503=CARTESIAN_POINT ( 'NONE',  ( 5.823673210054125526, 21.52544592524343514, 84.79057627198102409 ) ) ;
#52505=CARTESIAN_POINT ( 'NONE',  ( -18.62759615963270932, 10.81492255796079327, 35.83224293864768839 ) ) ;
#52506=CARTESIAN_POINT ( 'NONE',  ( 16.55341960407618274, -4.379528057220086978, 66.04275706135236135 ) ) ;
#52507=CARTESIAN_POINT ( 'NONE',  ( 8.224510206698953496, -14.34966873604960469, 82.91557627198103830 ) ) ;
#52508=CARTESIAN_POINT ( 'NONE',  ( -13.89961937509977652, 13.97604488694528158, 30.62390960531435269 ) ) ;
#52510=CARTESIAN_POINT ( 'NONE',  ( 0.05219959533934541429, -16.53943276465976808, 90.00109039468567573 ) ) ;
#52511=CARTESIAN_POINT ( 'NONE',  ( -18.67979575497178146, -10.72451020669898902, 111.6655762719810525 ) ) ;
#52512=CARTESIAN_POINT ( 'NONE',  ( -9.564922557960796823, -16.46253265017161027, 77.08224293864769550 ) ) ;
#52513=CARTESIAN_POINT ( 'NONE',  ( -18.62759615963255300, -10.81492255796106328, 54.16775706135235424 ) ) ;
#52514=CARTESIAN_POINT ( 'NONE',  ( -5.049401038298153566, 19.05341960407611168, 110.2072429386476671 ) ) ;
#52517=CARTESIAN_POINT ( 'NONE',  ( 18.62759615963255655, 10.81492255796105972, 41.66775706135235424 ) ) ;
#52518=CARTESIAN_POINT ( 'NONE',  ( 5.153800228976335163, 19.02544592524342804, 39.79057627198100988 ) ) ;
#52519=CARTESIAN_POINT ( 'NONE',  ( -0.05219959533909027116, -19.03943276465977164, 97.49890960531436690 ) ) ;
#52520=CARTESIAN_POINT ( 'NONE',  ( -9.474510206698720793, -16.51473224551083518, 49.58442372801899722 ) ) ;
#52521=CARTESIAN_POINT ( 'NONE',  ( 10.72451020669871369, 18.67979575497193778, 32.08442372801901854 ) ) ;
#52522=CARTESIAN_POINT ( 'NONE',  ( 5.049401038297881783, 19.05341960407617563, 52.29275706135234003 ) ) ;
#52523=CARTESIAN_POINT ( 'NONE',  ( 13.97604488694527802, 13.89961937509977652, 24.37390960531435624 ) ) ;
#52524=CARTESIAN_POINT ( 'NONE',  ( -16.53943276465976808, -0.05219959533934237506, 88.75109039468567573 ) ) ;
#52525=CARTESIAN_POINT ( 'NONE',  ( 5.049401038297881783, 19.05341960407617563, 67.29275706135234714 ) ) ;
#52526=CARTESIAN_POINT ( 'NONE',  ( 16.53943276465976808, 0.05219959533934440121, 101.2510903946856757 ) ) ;
#52528=CARTESIAN_POINT ( 'NONE',  ( 13.97604488694527802, 13.89961937509977652, 79.37390960531435269 ) ) ;
#52529=CARTESIAN_POINT ( 'NONE',  ( -10.72451020669870658, -18.67979575497194134, 94.58442372801901854 ) ) ;
#52530=CARTESIAN_POINT ( 'NONE',  ( 15.72974639402176855, 15.80617190586768217, 101.8760903946857042 ) ) ;
#52531=CARTESIAN_POINT ( 'NONE',  ( -0.05219959533909027116, -19.03943276465977164, 22.49890960531436690 ) ) ;
#52532=CARTESIAN_POINT ( 'NONE',  ( -19.02544592524342804, 5.153800228976336051, 96.04057627198103830 ) ) ;
#52533=CARTESIAN_POINT ( 'NONE',  ( -21.53943276465977519, -0.05219959533937600094, 78.75109039468568994 ) ) ;
#52534=CARTESIAN_POINT ( 'NONE',  ( -16.53943276465976808, -0.05219959533934237506, 18.75109039468568639 ) ) ;
#52536=CARTESIAN_POINT ( 'NONE',  ( -9.474510206698964154, 16.51473224551069663, 75.41557627198103830 ) ) ;
#52537=CARTESIAN_POINT ( 'NONE',  ( 15.80617190586746368, 15.72974639402197994, 29.37390960531435269 ) ) ;
#52538=CARTESIAN_POINT ( 'NONE',  ( -19.02544592524342804, 5.153800228976336051, 91.04057627198100988 ) ) ;
#52539=CARTESIAN_POINT ( 'NONE',  ( 17.58332526062524437, 7.635886036038643354, 86.57665040441534643 ) ) ;
#52540=CARTESIAN_POINT ( 'NONE',  ( 9.474510206698971260, -16.51473224551069308, 72.91557627198102409 ) ) ;
#52541=CARTESIAN_POINT ( 'NONE',  ( -13.97604488694527625, -13.89961937509977652, 71.87390960531433848 ) ) ;
#52542=CARTESIAN_POINT ( 'NONE',  ( 0.05219959533934541429, -16.53943276465976808, 105.0010903946856757 ) ) ;
#52543=CARTESIAN_POINT ( 'NONE',  ( -16.52216118717252158, 7.221426719304241182, 98.92400978952971968 ) ) ;
#52544=CARTESIAN_POINT ( 'NONE',  ( -9.564922557961040184, 16.46253265017147172, 77.91775706135234714 ) ) ;
#52545=CARTESIAN_POINT ( 'NONE',  ( -13.89961937509977652, 13.97604488694528158, 95.62390960531436690 ) ) ;
#52546=CARTESIAN_POINT ( 'NONE',  ( -16.53943276465976808, 0.05219959533911058130, 81.24890960531436690 ) ) ;
#52547=CARTESIAN_POINT ( 'NONE',  ( -5.719274019375978568, 21.55341960407610458, 50.20724293864769550 ) ) ;
#52548=CARTESIAN_POINT ( 'NONE',  ( -10.81492255796078084, -18.62759615963271287, 22.08224293864769194 ) ) ;
#52549=CARTESIAN_POINT ( 'NONE',  ( -8.314922557960811034, -14.29746914071050412, 112.0822429386477097 ) ) ;
#52551=CARTESIAN_POINT ( 'NONE',  ( 13.89961937509957401, 13.97604488694547697, 41.87609039468566152 ) ) ;
#52552=CARTESIAN_POINT ( 'NONE',  ( -4.483927247898539470, -16.52544592524342804, 22.29057627198102765 ) ) ;
#52553=CARTESIAN_POINT ( 'NONE',  ( 0.05219959533909260263, 19.03943276465977164, 104.9989096053143669 ) ) ;
#52554=CARTESIAN_POINT ( 'NONE',  ( 18.67979575497194134, -10.72451020669871369, 60.83442372801901854 ) ) ;
#52555=CARTESIAN_POINT ( 'NONE',  ( 10.81492255796078972, 18.62759615963270932, 59.58224293864770260 ) ) ;
#52556=CARTESIAN_POINT ( 'NONE',  ( 5.719274019375673035, 21.55341960407619339, 37.29275706135235424 ) ) ;
#52557=CARTESIAN_POINT ( 'NONE',  ( -21.52544592524343514, 5.823673210054127303, 86.04057627198102409 ) ) ;
#52558=CARTESIAN_POINT ( 'NONE',  ( -21.52544592524334988, -5.823673210054445271, 38.95942372801901854 ) ) ;
#52559=CARTESIAN_POINT ( 'NONE',  ( 12.14591786802309770, 12.06949235617756955, 114.3739096053143527 ) ) ;
#52561=CARTESIAN_POINT ( 'NONE',  ( -19.02544592524334988, -5.153800228976617603, 63.95942372801899012 ) ) ;
#52562=CARTESIAN_POINT ( 'NONE',  ( 0.05219959533909260263, 19.03943276465977164, 49.99890960531435979 ) ) ;
#52563=CARTESIAN_POINT ( 'NONE',  ( -8.224510206698948167, 14.34966873604960824, 85.41557627198102409 ) ) ;
#52564=CARTESIAN_POINT ( 'NONE',  ( -19.02544592524342804, 5.153800228976336051, 101.0405762719810241 ) ) ;
#52565=CARTESIAN_POINT ( 'NONE',  ( 9.564922557960805705, 16.46253265017160317, 114.5822429386476955 ) ) ;
#52566=CARTESIAN_POINT ( 'NONE',  ( -16.46253265017160317, 9.564922557960807481, 25.83224293864769194 ) ) ;
#52567=CARTESIAN_POINT ( 'NONE',  ( -4.483927247898539470, -16.52544592524342804, 37.29057627198102409 ) ) ;
#52568=CARTESIAN_POINT ( 'NONE',  ( 0.05219959533934541429, -16.53943276465976808, 105.0010903946856757 ) ) ;
#52569=CARTESIAN_POINT ( 'NONE',  ( 9.564922557960805705, 16.46253265017160317, 49.58224293864770260 ) ) ;
#52570=CARTESIAN_POINT ( 'NONE',  ( 12.06949235617757843, -12.14591786802309237, 113.1239096053143953 ) ) ;
#52571=CARTESIAN_POINT ( 'NONE',  ( 0.05219959533936267826, -19.03943276465977164, 20.00109039468567218 ) ) ;
#52572=CARTESIAN_POINT ( 'NONE',  ( 13.97604488694527802, 13.89961937509977652, 109.3739096053143669 ) ) ;
#52573=CARTESIAN_POINT ( 'NONE',  ( -0.05219959533910754901, -16.53943276465976808, 22.49890960531436335 ) ) ;
#52574=CARTESIAN_POINT ( 'NONE',  ( 18.62759615963255655, 10.81492255796105972, 41.66775706135235424 ) ) ;
#52576=CARTESIAN_POINT ( 'NONE',  ( -16.55341960407617563, 4.379528057220093196, 53.54275706135234714 ) ) ;
#52577=CARTESIAN_POINT ( 'NONE',  ( 4.379528057220339221, -16.55341960407611168, 32.70724293864770260 ) ) ;
#52578=CARTESIAN_POINT ( 'NONE',  ( -12.06949235617739369, -12.14591786802326823, 109.3760903946857042 ) ) ;
#52579=CARTESIAN_POINT ( 'NONE',  ( 16.53943276465976808, 0.05219959533934440121, 26.25109039468567573 ) ) ;
#52580=CARTESIAN_POINT ( 'NONE',  ( 19.03943276465977164, -0.05219959533909143690, 43.74890960531435979 ) ) ;
#52581=AXIS2_PLACEMENT_3D ( 'NONE', #112983, #73243, #134914 ) ;
#52582=CARTESIAN_POINT ( 'NONE',  ( -14.29746914071049879, 8.314922557960819915, 110.8322429386476955 ) ) ;
#52583=CARTESIAN_POINT ( 'NONE',  ( -10.72451020669870658, -18.67979575497194134, 24.58442372801901499 ) ) ;
#52584=CARTESIAN_POINT ( 'NONE',  ( -16.51473224551069308, -9.474510206698971260, 41.66557627198103120 ) ) ;
#52586=CARTESIAN_POINT ( 'NONE',  ( -5.153800228976328057, -19.02544592524343514, 27.29057627198103120 ) ) ;
#52587=CARTESIAN_POINT ( 'NONE',  ( 21.52544592524344225, -5.823673210054117533, 28.54057627198103120 ) ) ;
#52588=CARTESIAN_POINT ( 'NONE',  ( -16.20579543436676317, -7.371946100355211584, 35.56520834171877254 ) ) ;
#52589=CARTESIAN_POINT ( 'NONE',  ( -16.46253265017160317, 9.564922557960807481, 95.83224293864769550 ) ) ;
#52590=CARTESIAN_POINT ( 'NONE',  ( -21.53943276465977519, -0.05219959533937600094, 43.75109039468568284 ) ) ;
#52591=CARTESIAN_POINT ( 'NONE',  ( -4.483927247898539470, -16.52544592524342804, 107.2905762719810525 ) ) ;
#52592=CARTESIAN_POINT ( 'NONE',  ( -19.03943276465977164, 0.05219959533909376836, 116.2489096053143669 ) ) ;
#52594=CARTESIAN_POINT ( 'NONE',  ( -4.483927247898782831, 16.52544592524335698, 82.70942372801900433 ) ) ;
#52595=CARTESIAN_POINT ( 'NONE',  ( 21.53943276465977519, 0.05219959533937863772, 91.25109039468568994 ) ) ;
#52596=CARTESIAN_POINT ( 'NONE',  ( -14.34966873604972548, 8.224510206698743886, 58.33442372801901143 ) ) ;
#52597=CARTESIAN_POINT ( 'NONE',  ( 5.049401038298161559, -19.05341960407611168, 92.70724293864769550 ) ) ;
#52598=CARTESIAN_POINT ( 'NONE',  ( -14.29746914071037622, -8.314922557961029526, 39.16775706135235424 ) ) ;
#52599=CARTESIAN_POINT ( 'NONE',  ( -0.05219959533936034679, 19.03943276465977164, 102.5010903946856757 ) ) ;
#52600=CARTESIAN_POINT ( 'NONE',  ( -16.53943276465976808, -0.05219959533934237506, 78.75109039468568994 ) ) ;
#52601=CARTESIAN_POINT ( 'NONE',  ( -16.46253265017146816, -9.564922557961047289, 94.16775706135233293 ) ) ;
#52602=CARTESIAN_POINT ( 'NONE',  ( 5.049401038298161559, -19.05341960407611168, 72.70724293864768129 ) ) ;
#52603=CARTESIAN_POINT ( 'NONE',  ( 5.719274019375991003, -21.55341960407610458, 97.70724293864772392 ) ) ;
#52604=CARTESIAN_POINT ( 'NONE',  ( 16.52544592524342804, -4.483927247898539470, 103.5405762719810383 ) ) ;
#52605=CARTESIAN_POINT ( 'NONE',  ( 0.05219959533936267826, -19.03943276465977164, 100.0010903946856757 ) ) ;
#52606=CARTESIAN_POINT ( 'NONE',  ( 14.34966873604972726, -8.224510206698740333, 75.83442372801900433 ) ) ;
#52607=CARTESIAN_POINT ( 'NONE',  ( -16.18388926212245948, 7.379444403734574109, 44.56046848633771162 ) ) ;
#52608=CARTESIAN_POINT ( 'NONE',  ( 16.51473224551083163, -9.474510206698727899, 65.83442372801900433 ) ) ;
#52609=CARTESIAN_POINT ( 'NONE',  ( -8.314922557960811034, -14.29746914071050412, 32.08224293864769550 ) ) ;
#52610=CARTESIAN_POINT ( 'NONE',  ( 16.52544592524342804, -4.483927247898539470, 88.54057627198103830 ) ) ;
#52611=CARTESIAN_POINT ( 'NONE',  ( 9.564922557961047289, -16.46253265017146816, 30.41775706135232937 ) ) ;
#52613=CARTESIAN_POINT ( 'NONE',  ( -21.55341960407619339, 5.719274019375674811, 43.54275706135235424 ) ) ;
#52614=CARTESIAN_POINT ( 'NONE',  ( -16.46253265017146816, -9.564922557961047289, 94.16775706135233293 ) ) ;
#52615=DIRECTION ( 'NONE',  ( 3.469446951953611033E-15, 0.000000000000000000, -1.000000000000000000 ) ) ;
#52616=CARTESIAN_POINT ( 'NONE',  ( -0.05219959533909027116, -19.03943276465977164, 87.49890960531436690 ) ) ;
#52617=B_SPLINE_CURVE_WITH_KNOTS ( 'NONE', 3,
 ( #104855, #56355, #72532, #74525, #119044, #73541 ),
 .UNSPECIFIED., .F., .F.,
 ( 4, 2, 4 ),
 ( 0.003989672132298145192, 0.004372778065220570172, 0.004755883998142995152 ),
 .UNSPECIFIED. ) ;
#52618=CARTESIAN_POINT ( 'NONE',  ( 18.67979575497194134, -10.72451020669871369, 100.8344237280190185 ) ) ;
#52619=CARTESIAN_POINT ( 'NONE',  ( -19.03943276465977164, 0.05219959533909376836, 81.24890960531436690 ) ) ;
#52620=CARTESIAN_POINT ( 'NONE',  ( 21.55341960407610458, 5.719274019375980345, 48.95724293864770971 ) ) ;
#52621=CARTESIAN_POINT ( 'NONE',  ( -12.14591786802309592, -12.06949235617757132, 91.87390960531436690 ) ) ;
#52622=CARTESIAN_POINT ( 'NONE',  ( -19.05341960407611168, -5.049401038298163336, 51.45724293864770260 ) ) ;
#52623=CARTESIAN_POINT ( 'NONE',  ( 12.14591786802309770, 12.06949235617756955, 114.3739096053143527 ) ) ;
#52624=CARTESIAN_POINT ( 'NONE',  ( -5.719274019375665041, -21.55341960407619695, 19.79275706135235069 ) ) ;
#52625=CARTESIAN_POINT ( 'NONE',  ( 0.05219959533937995610, -21.53943276465977519, 60.00109039468568284 ) ) ;
#52626=CARTESIAN_POINT ( 'NONE',  ( 19.02544592524343514, -5.153800228976328945, 38.54057627198103120 ) ) ;
#52627=CARTESIAN_POINT ( 'NONE',  ( -0.05219959533934338120, 16.53943276465976808, 72.50109039468568994 ) ) ;
#52628=CARTESIAN_POINT ( 'NONE',  ( -15.80617190586745835, -15.72974639402198527, 111.8739096053143669 ) ) ;
#52629=CARTESIAN_POINT ( 'NONE',  ( -5.823673210054431948, 21.52544592524334988, 27.70942372801901854 ) ) ;
#52630=CARTESIAN_POINT ( 'NONE',  ( 19.02544592524334988, 5.153800228976608722, 51.45942372801900433 ) ) ;
#52631=CARTESIAN_POINT ( 'NONE',  ( -13.89961937509977652, 13.97604488694528158, 70.62390960531432427 ) ) ;
#52632=CARTESIAN_POINT ( 'NONE',  ( 13.97604488694548053, -13.89961937509957401, 35.62609039468567573 ) ) ;
#52633=CARTESIAN_POINT ( 'NONE',  ( -18.62759615963255300, -10.81492255796106328, 69.16775706135234714 ) ) ;
#52634=CARTESIAN_POINT ( 'NONE',  ( 5.823673210054125526, 21.52544592524343514, 74.79057627198105251 ) ) ;
#52635=CARTESIAN_POINT ( 'NONE',  ( 0.05219959533910956823, 16.53943276465976808, 49.99890960531437401 ) ) ;
#52636=CARTESIAN_POINT ( 'NONE',  ( 18.62759615963255655, 10.81492255796105972, 86.66775706135234714 ) ) ;
#52637=CARTESIAN_POINT ( 'NONE',  ( -16.51473224551082808, 9.474510206698731452, 33.33442372801899722 ) ) ;
#52638=CARTESIAN_POINT ( 'NONE',  ( 4.483927247898545687, 16.52544592524342804, 69.79057627198102409 ) ) ;
#52639=CARTESIAN_POINT ( 'NONE',  ( -16.53943276465976808, 0.05219959533911058130, 116.2489096053143669 ) ) ;
#52640=CARTESIAN_POINT ( 'NONE',  ( 0.05219959533936267826, -19.03943276465977164, 55.00109039468566863 ) ) ;
#52641=CARTESIAN_POINT ( 'NONE',  ( 16.52544592524342804, -4.483927247898539470, 23.54057627198102765 ) ) ;
#52642=CARTESIAN_POINT ( 'NONE',  ( 10.72451020669871369, 18.67979575497193778, 82.08442372801901854 ) ) ;
#52644=CARTESIAN_POINT ( 'NONE',  ( -19.03943276465977164, -0.05219959533935918106, 43.75109039468566863 ) ) ;
#52645=CARTESIAN_POINT ( 'NONE',  ( -10.72451020669898014, 18.67979575497178502, 55.41557627198102409 ) ) ;
#52646=CARTESIAN_POINT ( 'NONE',  ( -21.55341960407619339, 5.719274019375674811, 43.54275706135235424 ) ) ;
#52647=CARTESIAN_POINT ( 'NONE',  ( -21.52544592524343514, 5.823673210054127303, 96.04057627198102409 ) ) ;
#52648=CARTESIAN_POINT ( 'NONE',  ( 9.474510206698729675, 16.51473224551082808, 92.08442372801900433 ) ) ;
#52649=CARTESIAN_POINT ( 'NONE',  ( 4.379528057220092307, 16.55341960407617563, 72.29275706135236135 ) ) ;
#52651=CARTESIAN_POINT ( 'NONE',  ( 15.80617190586746368, 15.72974639402197994, 109.3739096053143811 ) ) ;
#52652=CARTESIAN_POINT ( 'NONE',  ( -16.52544592524342804, 4.483927247898546575, 86.04057627198102409 ) ) ;
#52653=B_SPLINE_CURVE_WITH_KNOTS ( 'NONE', 3,
 ( #179807, #104932, #25123, #181783, #121083, #55432 ),
 .UNSPECIFIED., .F., .F.,
 ( 4, 2, 4 ),
 ( 0.003989672132298160805, 0.004372778065220584917, 0.004755883998143008162 ),
 .UNSPECIFIED. ) ;
#52655=CARTESIAN_POINT ( 'NONE',  ( -4.483927247898782831, 16.52544592524335698, 37.70942372801900433 ) ) ;
#52656=CARTESIAN_POINT ( 'NONE',  ( -5.719274019375978568, 21.55341960407610458, 55.20724293864770260 ) ) ;
#52657=CARTESIAN_POINT ( 'NONE',  ( -12.14591786802326823, 12.06949235617739902, 88.12609039468570415 ) ) ;
#52659=EDGE_CURVE ( 'NONE', #151905, #176032, #114200, .T. ) ;
#52660=CARTESIAN_POINT ( 'NONE',  ( -4.483927247898782831, 16.52544592524335698, 72.70942372801901854 ) ) ;
#52661=CARTESIAN_POINT ( 'NONE',  ( 15.72974639402176855, 15.80617190586768217, 41.87609039468568284 ) ) ;
#52662=CARTESIAN_POINT ( 'NONE',  ( -15.80617190586745835, -15.72974639402198527, 56.87390960531436690 ) ) ;
#52663=CARTESIAN_POINT ( 'NONE',  ( -14.29746914071037622, -8.314922557961029526, 89.16775706135236135 ) ) ;
#52664=CARTESIAN_POINT ( 'NONE',  ( 10.81492255796106328, -18.62759615963255655, 75.41775706135233293 ) ) ;
#52665=CARTESIAN_POINT ( 'NONE',  ( 15.80617190586746368, 15.72974639402197994, 49.37390960531436690 ) ) ;
#52666=CARTESIAN_POINT ( 'NONE',  ( -5.719274019375978568, 21.55341960407610458, 35.20724293864768839 ) ) ;
#52668=CARTESIAN_POINT ( 'NONE',  ( -16.55341960407617563, 4.379528057220093196, 68.54275706135234714 ) ) ;
#52669=CARTESIAN_POINT ( 'NONE',  ( 21.53943276465977519, -0.05219959533907433946, 28.74890960531435624 ) ) ;
#52670=CARTESIAN_POINT ( 'NONE',  ( -5.049401038298153566, 19.05341960407611168, 105.2072429386476671 ) ) ;
#52671=CARTESIAN_POINT ( 'NONE',  ( 4.379528057220339221, -16.55341960407611168, 22.70724293864769194 ) ) ;
#52673=CARTESIAN_POINT ( 'NONE',  ( 8.314922557960818139, 14.29746914071049879, 114.5822429386477097 ) ) ;
#52674=CARTESIAN_POINT ( 'NONE',  ( -15.72974639402197994, 15.80617190586746368, 45.62390960531436690 ) ) ;
#52675=CARTESIAN_POINT ( 'NONE',  ( 19.03943276465977164, -0.05219959533909143690, 43.74890960531435979 ) ) ;
#52676=CARTESIAN_POINT ( 'NONE',  ( -14.29746914071037622, -8.314922557961029526, 94.16775706135237556 ) ) ;
#52677=CARTESIAN_POINT ( 'NONE',  ( 21.55341960407619695, -5.719274019375665929, 36.04275706135234714 ) ) ;
#52678=CARTESIAN_POINT ( 'NONE',  ( -16.46253265017146816, -9.564922557961047289, 84.16775706135233293 ) ) ;
#52679=CARTESIAN_POINT ( 'NONE',  ( -8.224510206698948167, 14.34966873604960824, 100.4155762719810241 ) ) ;
#52680=CARTESIAN_POINT ( 'NONE',  ( 16.51473224551069308, 9.474510206698969483, 54.16557627198103120 ) ) ;
#52681=CARTESIAN_POINT ( 'NONE',  ( -19.03943276465977164, 0.05219959533909376836, 31.24890960531435979 ) ) ;
#52682=CARTESIAN_POINT ( 'NONE',  ( 18.22780087662125226, -5.499999999999864997, 61.01540105326109398 ) ) ;
#52683=CARTESIAN_POINT ( 'NONE',  ( 0.05219959533909260263, 19.03943276465977164, 74.99890960531435269 ) ) ;
#52684=CARTESIAN_POINT ( 'NONE',  ( 4.379528057220092307, 16.55341960407617563, 67.29275706135234714 ) ) ;
#52685=CARTESIAN_POINT ( 'NONE',  ( 15.72974639402176855, 15.80617190586768217, 111.8760903946856615 ) ) ;
#52686=CARTESIAN_POINT ( 'NONE',  ( 21.52544592524344225, -5.823673210054117533, 53.54057627198103120 ) ) ;
#52687=CARTESIAN_POINT ( 'NONE',  ( -4.379528057220086978, -16.55341960407618274, 69.79275706135234714 ) ) ;
#52688=CARTESIAN_POINT ( 'NONE',  ( -5.153800228976607833, 19.02544592524334988, 62.70942372801899722 ) ) ;
#52689=CARTESIAN_POINT ( 'NONE',  ( -5.719274019375665041, -21.55341960407619695, 69.79275706135234714 ) ) ;
#52690=CARTESIAN_POINT ( 'NONE',  ( -16.46253265017160317, 9.564922557960807481, 70.83224293864770971 ) ) ;
#52691=CARTESIAN_POINT ( 'NONE',  ( 9.564922557960805705, 16.46253265017160317, 34.58224293864770260 ) ) ;
#52692=CARTESIAN_POINT ( 'NONE',  ( -19.03943276465977164, -0.05219959533935918106, 58.75109039468566863 ) ) ;
#52693=CARTESIAN_POINT ( 'NONE',  ( 5.153800228976335163, 19.02544592524342804, 114.7905762719810241 ) ) ;
#52694=CARTESIAN_POINT ( 'NONE',  ( -9.564922557960796823, -16.46253265017161027, 102.0822429386477097 ) ) ;
#52695=CARTESIAN_POINT ( 'NONE',  ( -12.14591786802309592, -12.06949235617757132, 51.87390960531437401 ) ) ;
#52696=CARTESIAN_POINT ( 'NONE',  ( 10.72451020669898902, -18.67979575497178502, 42.91557627198103120 ) ) ;
#52698=CARTESIAN_POINT ( 'NONE',  ( 5.049401038297881783, 19.05341960407617563, 32.29275706135233293 ) ) ;
#52700=CARTESIAN_POINT ( 'NONE',  ( 13.97604488694527802, 13.89961937509977652, 44.37390960531435269 ) ) ;
#52701=CARTESIAN_POINT ( 'NONE',  ( -19.49671883438227127, -5.500000000000030198, 99.89279849105680853 ) ) ;
#52703=CARTESIAN_POINT ( 'NONE',  ( 12.06949235617739724, 12.14591786802326823, 76.87609039468567573 ) ) ;
#52704=CARTESIAN_POINT ( 'NONE',  ( 5.823673210054125526, 21.52544592524343514, 99.79057627198103830 ) ) ;
#52705=CARTESIAN_POINT ( 'NONE',  ( -19.03943276465977164, 0.05219959533909376836, 41.24890960531435269 ) ) ;
#52707=CARTESIAN_POINT ( 'NONE',  ( -10.81492255796105439, 18.62759615963255655, 37.91775706135235424 ) ) ;
#52708=CARTESIAN_POINT ( 'NONE',  ( 9.564922557961047289, -16.46253265017146816, 55.41775706135234003 ) ) ;
#52709=CARTESIAN_POINT ( 'NONE',  ( 16.46253265017160672, -9.564922557960803928, 53.33224293864768839 ) ) ;
#52710=CARTESIAN_POINT ( 'NONE',  ( 10.81492255796106328, -18.62759615963255655, 95.41775706135234714 ) ) ;
#52711=CARTESIAN_POINT ( 'NONE',  ( -9.564922557960796823, -16.46253265017161027, 22.08224293864768839 ) ) ;
#52712=CARTESIAN_POINT ( 'NONE',  ( -12.14591786802309592, -12.06949235617757132, 46.87390960531435979 ) ) ;
#52714=CARTESIAN_POINT ( 'NONE',  ( 15.80617190586746368, 15.72974639402197994, 44.37390960531435979 ) ) ;
#52716=CARTESIAN_POINT ( 'NONE',  ( -19.02544592524342804, 5.153800228976336051, 106.0405762719810241 ) ) ;
#52717=CARTESIAN_POINT ( 'NONE',  ( 12.14591786802309770, 12.06949235617756955, 89.37390960531435269 ) ) ;
#52718=CARTESIAN_POINT ( 'NONE',  ( 12.06949235617739724, 12.14591786802326823, 26.87609039468567218 ) ) ;
#52719=CARTESIAN_POINT ( 'NONE',  ( -8.314922557961024197, 14.29746914071037800, 107.9177570613523471 ) ) ;
#52720=ORIENTED_EDGE ( 'NONE', *, *, #125362, .F. ) ;
#52721=CARTESIAN_POINT ( 'NONE',  ( 19.02544592524343514, -5.153800228976328945, 98.54057627198100988 ) ) ;
#52722=CARTESIAN_POINT ( 'NONE',  ( -5.823673210054116645, -21.52544592524344225, 107.2905762719810525 ) ) ;
#52724=CARTESIAN_POINT ( 'NONE',  ( -4.483927247898539470, -16.52544592524342804, 32.29057627198102409 ) ) ;
#52725=CARTESIAN_POINT ( 'NONE',  ( 19.03943276465977164, -0.05219959533909143690, 103.7489096053143669 ) ) ;
#52726=CARTESIAN_POINT ( 'NONE',  ( 16.51473224551083163, -9.474510206698727899, 90.83442372801900433 ) ) ;
#52727=CARTESIAN_POINT ( 'NONE',  ( -21.53943276465977519, -0.05219959533937600094, 113.7510903946856757 ) ) ;
#52728=CARTESIAN_POINT ( 'NONE',  ( 15.72974639402199770, -15.80617190586745480, 93.12390960531436690 ) ) ;
#52729=CARTESIAN_POINT ( 'NONE',  ( 18.67979575497178502, 10.72451020669898547, 49.16557627198102409 ) ) ;
#52730=CARTESIAN_POINT ( 'NONE',  ( -13.97604488694527625, -13.89961937509977652, 61.87390960531435979 ) ) ;
#52731=CARTESIAN_POINT ( 'NONE',  ( 16.53943276465976808, -0.05219959533910856209, 38.74890960531435979 ) ) ;
#52732=CARTESIAN_POINT ( 'NONE',  ( 19.02544592524343514, -5.153800228976328945, 78.54057627198099567 ) ) ;
#52733=CARTESIAN_POINT ( 'NONE',  ( 19.25663599770057388, -5.499999999999650058, 61.49419308057201050 ) ) ;
#52734=CARTESIAN_POINT ( 'NONE',  ( -0.05219959533936034679, 19.03943276465977164, 42.50109039468566152 ) ) ;
#52735=CARTESIAN_POINT ( 'NONE',  ( -0.05219959533910754901, -16.53943276465976808, 92.49890960531436690 ) ) ;
#52736=CARTESIAN_POINT ( 'NONE',  ( 5.823673210054444382, -21.52544592524334988, 25.20942372801901854 ) ) ;
#52738=CARTESIAN_POINT ( 'NONE',  ( -0.05219959533934338120, 16.53943276465976808, 112.5010903946857042 ) ) ;
#52739=CARTESIAN_POINT ( 'NONE',  ( 0.05219959533910956823, 16.53943276465976808, 114.9989096053143669 ) ) ;
#52740=CARTESIAN_POINT ( 'NONE',  ( 9.474510206698971260, -16.51473224551069308, 77.91557627198103830 ) ) ;
#52742=CARTESIAN_POINT ( 'NONE',  ( 8.314922557960818139, 14.29746914071049879, 49.58224293864769550 ) ) ;
#52743=CARTESIAN_POINT ( 'NONE',  ( 5.823673210054444382, -21.52544592524334988, 55.20942372801902565 ) ) ;
#52745=CARTESIAN_POINT ( 'NONE',  ( -19.03943276465977164, 0.05219959533909376836, 41.24890960531435269 ) ) ;
#52746=CARTESIAN_POINT ( 'NONE',  ( -19.02544592524342804, 5.153800228976336051, 46.04057627198101699 ) ) ;
#52748=CARTESIAN_POINT ( 'NONE',  ( -21.55341960407619339, 5.719274019375674811, 98.54275706135234714 ) ) ;
#52749=CARTESIAN_POINT ( 'NONE',  ( 0.05219959533934541429, -16.53943276465976808, 60.00109039468568284 ) ) ;
#52750=CARTESIAN_POINT ( 'NONE',  ( 0.05219959533937995610, -21.53943276465977519, 85.00109039468568994 ) ) ;
#52751=CARTESIAN_POINT ( 'NONE',  ( -15.80617190586745835, -15.72974639402198527, 26.87390960531435979 ) ) ;
#52752=CARTESIAN_POINT ( 'NONE',  ( 0.05219959533936267826, -19.03943276465977164, 100.0010903946856757 ) ) ;
#52753=CARTESIAN_POINT ( 'NONE',  ( -10.72451020669870658, -18.67979575497194134, 74.58442372801901854 ) ) ;
#52754=CARTESIAN_POINT ( 'NONE',  ( 14.34966873604972726, -8.224510206698740333, 40.83442372801901854 ) ) ;
#52755=CARTESIAN_POINT ( 'NONE',  ( 18.62759615963271287, -10.81492255796078972, 88.33224293864769550 ) ) ;
#52756=CARTESIAN_POINT ( 'NONE',  ( 13.89961937509957401, 13.97604488694547697, 101.8760903946856331 ) ) ;
#52757=CARTESIAN_POINT ( 'NONE',  ( -16.51473224551069308, -9.474510206698971260, 66.66557627198102409 ) ) ;
#52758=CARTESIAN_POINT ( 'NONE',  ( 13.89961937509957401, 13.97604488694547697, 101.8760903946856331 ) ) ;
#52759=CARTESIAN_POINT ( 'NONE',  ( -5.153800228976607833, 19.02544592524334988, 97.70942372801900433 ) ) ;
#52760=CARTESIAN_POINT ( 'NONE',  ( 14.29746914071049879, -8.314922557960816363, 48.33224293864770260 ) ) ;
#52762=CARTESIAN_POINT ( 'NONE',  ( -5.153800228976607833, 19.02544592524334988, 72.70942372801900433 ) ) ;
#52763=CARTESIAN_POINT ( 'NONE',  ( 12.06949235617739724, 12.14591786802326823, 66.87609039468568994 ) ) ;
#52764=CARTESIAN_POINT ( 'NONE',  ( -18.67979575497193778, 10.72451020669871902, 23.33442372801901499 ) ) ;
#52765=CARTESIAN_POINT ( 'NONE',  ( -13.89961937509977652, 13.97604488694528158, 40.62390960531435979 ) ) ;
#52766=CARTESIAN_POINT ( 'NONE',  ( 19.05341960407611168, 5.049401038298154454, 58.95724293864768129 ) ) ;
#52767=CARTESIAN_POINT ( 'NONE',  ( -16.53943276465976808, -0.05219959533934237506, 63.75109039468568284 ) ) ;
#52770=CARTESIAN_POINT ( 'NONE',  ( 9.564922557960805705, 16.46253265017160317, 99.58224293864770971 ) ) ;
#52771=CARTESIAN_POINT ( 'NONE',  ( 16.51473224551069308, 9.474510206698969483, 29.16557627198103475 ) ) ;
#52773=CARTESIAN_POINT ( 'NONE',  ( -13.97604488694547697, 13.89961937509957934, 108.1260903946856331 ) ) ;
#52774=CARTESIAN_POINT ( 'NONE',  ( 21.53943276465977519, -0.05219959533907433946, 43.74890960531435979 ) ) ;
#52775=CARTESIAN_POINT ( 'NONE',  ( -13.97604488694547697, 13.89961937509957934, 43.12609039468566152 ) ) ;
#52776=CARTESIAN_POINT ( 'NONE',  ( 12.06949235617739724, 12.14591786802326823, 31.87609039468567929 ) ) ;
#52777=CARTESIAN_POINT ( 'NONE',  ( 5.153800228976335163, 19.02544592524342804, 34.79057627198102409 ) ) ;
#52778=CARTESIAN_POINT ( 'NONE',  ( -13.97604488694527625, -13.89961937509977652, 46.87390960531435979 ) ) ;
#52779=CARTESIAN_POINT ( 'NONE',  ( 5.719274019375991003, -21.55341960407610458, 92.70724293864770971 ) ) ;
#52780=CARTESIAN_POINT ( 'NONE',  ( 9.564922557960805705, 16.46253265017160317, 99.58224293864770971 ) ) ;
#52781=CARTESIAN_POINT ( 'NONE',  ( -9.474510206698964154, 16.51473224551069663, 50.41557627198102409 ) ) ;
#52783=CARTESIAN_POINT ( 'NONE',  ( 13.97604488694548053, -13.89961937509957401, 80.62609039468567573 ) ) ;
#52784=CARTESIAN_POINT ( 'NONE',  ( -8.224510206698948167, 14.34966873604960824, 65.41557627198102409 ) ) ;
#52785=CARTESIAN_POINT ( 'NONE',  ( 18.67979575497194134, -10.72451020669871369, 110.8344237280190043 ) ) ;
#52786=CARTESIAN_POINT ( 'NONE',  ( 21.53943276465977519, -0.05219959533907433946, 98.74890960531438111 ) ) ;
#52787=CARTESIAN_POINT ( 'NONE',  ( -10.72451020669870658, -18.67979575497194134, 79.58442372801903275 ) ) ;
#52788=CARTESIAN_POINT ( 'NONE',  ( 5.719274019375673035, 21.55341960407619339, 77.29275706135234714 ) ) ;
#52789=EDGE_CURVE ( 'NONE', #55277, #127622, #85731, .T. ) ;
#52790=CARTESIAN_POINT ( 'NONE',  ( 19.03943276465977164, -0.05219959533909143690, 113.7489096053143669 ) ) ;
#52791=CARTESIAN_POINT ( 'NONE',  ( -16.52544592524335698, -4.483927247898792601, 108.9594237280190185 ) ) ;
#52792=CARTESIAN_POINT ( 'NONE',  ( 15.72974639402176855, 15.80617190586768217, 81.87609039468568994 ) ) ;
#52793=CARTESIAN_POINT ( 'NONE',  ( -19.02544592524342804, 5.153800228976336051, 61.04057627198103120 ) ) ;
#52794=CARTESIAN_POINT ( 'NONE',  ( -0.05219959533937732626, 21.53943276465977519, 42.50109039468567573 ) ) ;
#52795=CARTESIAN_POINT ( 'NONE',  ( -16.46253265017160317, 9.564922557960807481, 85.83224293864769550 ) ) ;
#52796=CARTESIAN_POINT ( 'NONE',  ( -14.34966873604960291, -8.224510206698953496, 86.66557627198102409 ) ) ;
#52797=CARTESIAN_POINT ( 'NONE',  ( 14.34966873604960469, 8.224510206698951720, 49.16557627198102409 ) ) ;
#52798=CARTESIAN_POINT ( 'NONE',  ( -5.823673210054116645, -21.52544592524344225, 57.29057627198103120 ) ) ;
#52800=CARTESIAN_POINT ( 'NONE',  ( -13.89961937509977652, 13.97604488694528158, 55.62390960531434558 ) ) ;
#52801=CARTESIAN_POINT ( 'NONE',  ( 10.81492255796078972, 18.62759615963270932, 74.58224293864768129 ) ) ;
#52802=CARTESIAN_POINT ( 'NONE',  ( -9.474510206698720793, -16.51473224551083518, 64.58442372801900433 ) ) ;
#52803=CARTESIAN_POINT ( 'NONE',  ( 19.02544592524335343, 5.153800228976608722, 26.45942372801899722 ) ) ;
#52804=CARTESIAN_POINT ( 'NONE',  ( 14.29746914071049879, -8.314922557960816363, 73.33224293864769550 ) ) ;
#52805=CARTESIAN_POINT ( 'NONE',  ( -18.67979575497178146, -10.72451020669898902, 56.66557627198103830 ) ) ;
#52807=CARTESIAN_POINT ( 'NONE',  ( -17.49999999999999645, -5.500000000000000888, 120.0000000000000142 ) ) ;
#52808=CARTESIAN_POINT ( 'NONE',  ( 0.05219959533934541429, -16.53943276465976808, 95.00109039468568994 ) ) ;
#52810=CARTESIAN_POINT ( 'NONE',  ( -9.474510206698720793, -16.51473224551083518, 89.58442372801900433 ) ) ;
#52811=CARTESIAN_POINT ( 'NONE',  ( -14.29746914071049879, 8.314922557960819915, 65.83224293864769550 ) ) ;
#52813=CARTESIAN_POINT ( 'NONE',  ( 5.153800228976335163, 19.02544592524342804, 59.79057627198100988 ) ) ;
#52814=CARTESIAN_POINT ( 'NONE',  ( -14.29746914071049879, 8.314922557960819915, 55.83224293864770260 ) ) ;
#52815=CARTESIAN_POINT ( 'NONE',  ( 0.05219959533909260263, 19.03943276465977164, 89.99890960531436690 ) ) ;
#52816=CARTESIAN_POINT ( 'NONE',  ( -16.46253265017146816, -9.564922557961047289, 79.16775706135234714 ) ) ;
#52817=CARTESIAN_POINT ( 'NONE',  ( 19.02544592524343514, -5.153800228976328945, 48.54057627198103120 ) ) ;
#52818=CARTESIAN_POINT ( 'NONE',  ( -16.46253265017160317, 9.564922557960807481, 90.83224293864769550 ) ) ;
#52819=CARTESIAN_POINT ( 'NONE',  ( -5.153800228976328057, -19.02544592524343514, 67.29057627198102409 ) ) ;
#52820=CARTESIAN_POINT ( 'NONE',  ( -0.05219959533907301413, -21.53943276465977519, 67.49890960531436690 ) ) ;
#52821=CARTESIAN_POINT ( 'NONE',  ( 14.29746914071037800, 8.314922557961029526, 56.66775706135235424 ) ) ;
#52823=CARTESIAN_POINT ( 'NONE',  ( 19.05341960407611168, 5.049401038298154454, 53.95724293864770260 ) ) ;
#52824=CARTESIAN_POINT ( 'NONE',  ( 10.72451020669898902, -18.67979575497178502, 57.91557627198103120 ) ) ;
#52825=CARTESIAN_POINT ( 'NONE',  ( -13.89961937509957401, -13.97604488694547875, 79.37609039468567573 ) ) ;
#52826=CARTESIAN_POINT ( 'NONE',  ( 0.05219959533910956823, 16.53943276465976808, 29.99890960531435979 ) ) ;
#52827=CARTESIAN_POINT ( 'NONE',  ( -16.51473224551082808, 9.474510206698731452, 38.33442372801899722 ) ) ;
#52828=CARTESIAN_POINT ( 'NONE',  ( -16.53943276465976808, -0.05219959533934237506, 58.75109039468568994 ) ) ;
#52829=CARTESIAN_POINT ( 'NONE',  ( 0.05219959533934541429, -16.53943276465976808, 100.0010903946857042 ) ) ;
#52830=CARTESIAN_POINT ( 'NONE',  ( 18.56453257813361901, -5.500000000000039080, 43.49000423690687711 ) ) ;
#52831=CARTESIAN_POINT ( 'NONE',  ( 16.55341960407618274, -4.379528057220086978, 86.04275706135236135 ) ) ;
#52832=CARTESIAN_POINT ( 'NONE',  ( -19.03943276465977164, 0.05219959533909376836, 116.2489096053143669 ) ) ;
#52833=CARTESIAN_POINT ( 'NONE',  ( -9.474510206698964154, 16.51473224551069663, 40.41557627198103120 ) ) ;
#52834=CARTESIAN_POINT ( 'NONE',  ( -19.03943276465977164, 0.05219959533909376836, 46.24890960531435979 ) ) ;
#52835=CARTESIAN_POINT ( 'NONE',  ( -16.51473224551069308, -9.474510206698971260, 41.66557627198103120 ) ) ;
#52836=CARTESIAN_POINT ( 'NONE',  ( -15.72974639402176322, -15.80617190586768395, 34.37609039468568284 ) ) ;
#52837=CARTESIAN_POINT ( 'NONE',  ( 4.379528057220092307, 16.55341960407617563, 47.29275706135234003 ) ) ;
#52838=CARTESIAN_POINT ( 'NONE',  ( -16.53943276465976808, -0.05219959533934237506, 113.7510903946856757 ) ) ;
#52839=CARTESIAN_POINT ( 'NONE',  ( 16.51473224551069308, 9.474510206698969483, 24.16557627198102765 ) ) ;
#52840=CARTESIAN_POINT ( 'NONE',  ( 13.89961937509957401, 13.97604488694547697, 21.87609039468566152 ) ) ;
#52841=CARTESIAN_POINT ( 'NONE',  ( -19.03943276465977164, -0.05219959533935918106, 113.7510903946856757 ) ) ;
#52842=CARTESIAN_POINT ( 'NONE',  ( 9.564922557961047289, -16.46253265017146816, 70.41775706135233293 ) ) ;
#52843=CARTESIAN_POINT ( 'NONE',  ( -12.06949235617756955, 12.14591786802309770, 70.62390960531436690 ) ) ;
#52844=CARTESIAN_POINT ( 'NONE',  ( 19.02544592524343514, -5.153800228976328945, 43.54057627198103120 ) ) ;
#52845=CARTESIAN_POINT ( 'NONE',  ( -19.03943276465977164, -0.05219959533935918106, 68.75109039468566152 ) ) ;
#52846=CARTESIAN_POINT ( 'NONE',  ( -10.81492255796105439, 18.62759615963255655, 72.91775706135234714 ) ) ;
#52847=CARTESIAN_POINT ( 'NONE',  ( -8.314922557961024197, 14.29746914071037800, 42.91775706135235424 ) ) ;
#52848=CARTESIAN_POINT ( 'NONE',  ( 19.53037848336980886, -5.499999999999891642, 57.35532783611445495 ) ) ;
#52849=CARTESIAN_POINT ( 'NONE',  ( -0.05219959533907301413, -21.53943276465977519, 42.49890960531435979 ) ) ;
#52850=CARTESIAN_POINT ( 'NONE',  ( -8.224510206698735004, -14.34966873604973081, 24.58442372801901499 ) ) ;
#52851=CARTESIAN_POINT ( 'NONE',  ( 17.72517630440434999, -5.499999999999972466, 98.42175719257214439 ) ) ;
#52852=CARTESIAN_POINT ( 'NONE',  ( -5.719274019375665041, -21.55341960407619695, 104.7927570613523898 ) ) ;
#52854=CARTESIAN_POINT ( 'NONE',  ( 19.05341960407611168, 5.049401038298154454, 43.95724293864769550 ) ) ;
#52855=CARTESIAN_POINT ( 'NONE',  ( -17.49999999999999645, 5.499999999999997335, 120.0000000000000142 ) ) ;
#52856=CARTESIAN_POINT ( 'NONE',  ( 13.89961937509977652, -13.97604488694527269, 58.12390960531436690 ) ) ;
#52857=CARTESIAN_POINT ( 'NONE',  ( 10.72451020669871369, 18.67979575497193778, 62.08442372801901143 ) ) ;
#52858=CARTESIAN_POINT ( 'NONE',  ( 18.67979575497194134, -10.72451020669871369, 110.8344237280190043 ) ) ;
#52859=CARTESIAN_POINT ( 'NONE',  ( -14.34966873604960291, -8.224510206698953496, 26.66557627198103475 ) ) ;
#52860=CARTESIAN_POINT ( 'NONE',  ( 16.51473224551069308, 9.474510206698969483, 29.16557627198103475 ) ) ;
#52861=CARTESIAN_POINT ( 'NONE',  ( 9.474510206698971260, -16.51473224551069308, 87.91557627198102409 ) ) ;
#52862=CARTESIAN_POINT ( 'NONE',  ( -18.67979575497193778, 10.72451020669871902, 53.33442372801901854 ) ) ;
#52863=CARTESIAN_POINT ( 'NONE',  ( 19.05341960407611168, 5.049401038298154454, 33.95724293864769550 ) ) ;
#52865=CARTESIAN_POINT ( 'NONE',  ( -5.719274019375665041, -21.55341960407619695, 69.79275706135234714 ) ) ;
#52866=CARTESIAN_POINT ( 'NONE',  ( -9.474510206698720793, -16.51473224551083518, 89.58442372801900433 ) ) ;
#52867=CARTESIAN_POINT ( 'NONE',  ( -9.474510206698964154, 16.51473224551069663, 110.4155762719810383 ) ) ;
#52868=CARTESIAN_POINT ( 'NONE',  ( -14.29746914071049879, 8.314922557960819915, 115.8322429386477097 ) ) ;
#52869=CARTESIAN_POINT ( 'NONE',  ( -5.823673210054116645, -21.52544592524344225, 112.2905762719810241 ) ) ;
#52870=CARTESIAN_POINT ( 'NONE',  ( -19.05341960407617563, 5.049401038297882671, 33.54275706135231871 ) ) ;
#52871=CARTESIAN_POINT ( 'NONE',  ( -12.06949235617756955, 12.14591786802309770, 115.6239096053143669 ) ) ;
#52872=CARTESIAN_POINT ( 'NONE',  ( 19.05341960407611168, 5.049401038298154454, 58.95724293864768129 ) ) ;
#52873=CARTESIAN_POINT ( 'NONE',  ( -19.03943276465977164, -0.05219959533935918106, 103.7510903946856757 ) ) ;
#52874=CARTESIAN_POINT ( 'NONE',  ( -16.55341960407611168, -4.379528057220339221, 61.45724293864770260 ) ) ;
#52875=CARTESIAN_POINT ( 'NONE',  ( 5.153800228976615827, -19.02544592524334988, 30.20942372801900433 ) ) ;
#52876=CARTESIAN_POINT ( 'NONE',  ( -21.55341960407610458, -5.719274019375992779, 21.45724293864769550 ) ) ;
#52877=CARTESIAN_POINT ( 'NONE',  ( 5.153800228976615827, -19.02544592524334988, 90.20942372801900433 ) ) ;
#52878=CARTESIAN_POINT ( 'NONE',  ( 18.62759615963271287, -10.81492255796078972, 98.33224293864769550 ) ) ;
#52879=CARTESIAN_POINT ( 'NONE',  ( -21.53943276465977519, -0.05219959533937600094, 38.75109039468567573 ) ) ;
#52880=CARTESIAN_POINT ( 'NONE',  ( 14.29746914071037800, 8.314922557961029526, 36.66775706135234714 ) ) ;
#52881=CARTESIAN_POINT ( 'NONE',  ( 12.06949235617739724, 12.14591786802326823, 46.87609039468568994 ) ) ;
#52882=CARTESIAN_POINT ( 'NONE',  ( -0.05219959533937732626, 21.53943276465977519, 47.50109039468568994 ) ) ;
#52883=CARTESIAN_POINT ( 'NONE',  ( -21.53943276465977519, 0.05219959533907696930, 56.24890960531436690 ) ) ;
#52884=CARTESIAN_POINT ( 'NONE',  ( -19.02544592524342804, 5.153800228976336051, 36.04057627198100988 ) ) ;
#52886=CARTESIAN_POINT ( 'NONE',  ( 4.379528057220092307, 16.55341960407617563, 77.29275706135234714 ) ) ;
#52887=CARTESIAN_POINT ( 'NONE',  ( 5.719274019375991003, -21.55341960407610458, 92.70724293864770971 ) ) ;
#52888=CARTESIAN_POINT ( 'NONE',  ( -8.224510206698948167, 14.34966873604960824, 35.41557627198102409 ) ) ;
#52889=CARTESIAN_POINT ( 'NONE',  ( 4.483927247898790824, -16.52544592524335698, 65.20942372801901854 ) ) ;
#52890=CARTESIAN_POINT ( 'NONE',  ( -19.03943276465977164, -0.05219959533935918106, 98.75109039468567573 ) ) ;
#52891=CARTESIAN_POINT ( 'NONE',  ( -10.81492255796078084, -18.62759615963271287, 92.08224293864769550 ) ) ;
#52892=CARTESIAN_POINT ( 'NONE',  ( -16.52544592524342804, 4.483927247898546575, 26.04057627198103475 ) ) ;
#52894=CARTESIAN_POINT ( 'NONE',  ( -0.05219959533934338120, 16.53943276465976808, 72.50109039468568994 ) ) ;
#52896=CARTESIAN_POINT ( 'NONE',  ( 5.823673210054125526, 21.52544592524343514, 69.79057627198102409 ) ) ;
#52897=CARTESIAN_POINT ( 'NONE',  ( -14.34966873604972548, 8.224510206698743886, 103.3344237280190043 ) ) ;
#52898=ORIENTED_EDGE ( 'NONE', *, *, #195051, .F. ) ;
#52899=CARTESIAN_POINT ( 'NONE',  ( 18.87255363501903815, 5.499999999999949374, 88.82513748171831480 ) ) ;
#52900=CARTESIAN_POINT ( 'NONE',  ( 5.823673210054125526, 21.52544592524343514, 104.7905762719810241 ) ) ;
#52901=CARTESIAN_POINT ( 'NONE',  ( 15.72974639402199770, -15.80617190586745480, 108.1239096053143811 ) ) ;
#52902=CARTESIAN_POINT ( 'NONE',  ( 0.05219959533910956823, 16.53943276465976808, 34.99890960531435979 ) ) ;
#52903=CARTESIAN_POINT ( 'NONE',  ( 14.29746914071037800, 8.314922557961029526, 36.66775706135234714 ) ) ;
#52904=CARTESIAN_POINT ( 'NONE',  ( 5.049401038298161559, -19.05341960407611168, 52.70724293864767418 ) ) ;
#52905=CARTESIAN_POINT ( 'NONE',  ( -19.05341960407611168, -5.049401038298163336, 61.45724293864769550 ) ) ;
#52907=CARTESIAN_POINT ( 'NONE',  ( -9.474510206698964154, 16.51473224551069663, 110.4155762719810383 ) ) ;
#52909=CARTESIAN_POINT ( 'NONE',  ( -13.89961937509957401, -13.97604488694547875, 109.3760903946856331 ) ) ;
#52910=CARTESIAN_POINT ( 'NONE',  ( 0.05219959533936267826, -19.03943276465977164, 55.00109039468566863 ) ) ;
#52911=CARTESIAN_POINT ( 'NONE',  ( 0.05219959533907565091, 21.53943276465977519, 84.99890960531436690 ) ) ;
#52912=CARTESIAN_POINT ( 'NONE',  ( -14.34966873604972548, 8.224510206698743886, 108.3344237280190185 ) ) ;
#52913=CARTESIAN_POINT ( 'NONE',  ( -10.81492255796078084, -18.62759615963271287, 42.08224293864769550 ) ) ;
#52914=CARTESIAN_POINT ( 'NONE',  ( 10.72451020669898902, -18.67979575497178502, 82.91557627198103830 ) ) ;
#52915=CARTESIAN_POINT ( 'NONE',  ( 19.03943276465977164, 0.05219959533936151252, 101.2510903946856757 ) ) ;
#52916=CARTESIAN_POINT ( 'NONE',  ( 19.03943276465977164, -0.05219959533909143690, 113.7489096053143669 ) ) ;
#52917=CARTESIAN_POINT ( 'NONE',  ( 15.72974639402176855, 15.80617190586768217, 81.87609039468568994 ) ) ;
#52918=CARTESIAN_POINT ( 'NONE',  ( -19.05341960407611168, -5.049401038298163336, 71.45724293864766707 ) ) ;
#52919=CARTESIAN_POINT ( 'NONE',  ( -19.05341960407611168, -5.049401038298163336, 21.45724293864768839 ) ) ;
#52920=CARTESIAN_POINT ( 'NONE',  ( 16.46253265017160672, -9.564922557960803928, 73.33224293864769550 ) ) ;
#52921=CARTESIAN_POINT ( 'NONE',  ( -8.224510206698948167, 14.34966873604960824, 90.41557627198103830 ) ) ;
#52923=CARTESIAN_POINT ( 'NONE',  ( -5.153800228976607833, 19.02544592524334988, 102.7094237280189759 ) ) ;
#52926=CARTESIAN_POINT ( 'NONE',  ( -19.05341960407611168, -5.049401038298163336, 76.45724293864769550 ) ) ;
#52927=CARTESIAN_POINT ( 'NONE',  ( -21.53943276465977519, -0.05219959533937600094, 78.75109039468568994 ) ) ;
#52928=CARTESIAN_POINT ( 'NONE',  ( 9.564922557960805705, 16.46253265017160317, 94.58224293864769550 ) ) ;
#52929=CARTESIAN_POINT ( 'NONE',  ( 14.29746914071037800, 8.314922557961029526, 71.66775706135234714 ) ) ;
#52930=CARTESIAN_POINT ( 'NONE',  ( -17.31747979337950838, -6.344076630960982399, 76.37944868065184778 ) ) ;
#52931=CARTESIAN_POINT ( 'NONE',  ( -13.97604488694547697, 13.89961937509957934, 58.12609039468566863 ) ) ;
#52932=CARTESIAN_POINT ( 'NONE',  ( -5.153800228976607833, 19.02544592524334988, 22.70942372801899012 ) ) ;
#52934=CARTESIAN_POINT ( 'NONE',  ( -19.03943276465977164, 0.05219959533909376836, 116.2489096053143669 ) ) ;
#52936=CARTESIAN_POINT ( 'NONE',  ( 16.55341960407611168, 4.379528057220329451, 23.95724293864769550 ) ) ;
#52938=CARTESIAN_POINT ( 'NONE',  ( 16.52544592524335698, 4.483927247898782831, 106.4594237280190328 ) ) ;
#52939=CARTESIAN_POINT ( 'NONE',  ( 17.05116617787824751, 6.768360034955832383, 68.84324446740802728 ) ) ;
#52940=CARTESIAN_POINT ( 'NONE',  ( -16.52544592524335698, -4.483927247898792601, 83.95942372801900433 ) ) ;
#52941=CARTESIAN_POINT ( 'NONE',  ( -5.823673210054431948, 21.52544592524334988, 82.70942372801900433 ) ) ;
#52942=CARTESIAN_POINT ( 'NONE',  ( 16.51473224551083163, -9.474510206698727899, 90.83442372801900433 ) ) ;
#52943=CARTESIAN_POINT ( 'NONE',  ( -5.049401038297874678, -19.05341960407617918, 39.79275706135232582 ) ) ;
#52944=CARTESIAN_POINT ( 'NONE',  ( 16.46253265017160672, -9.564922557960803928, 78.33224293864769550 ) ) ;
#52945=CARTESIAN_POINT ( 'NONE',  ( -13.89961937509977652, 13.97604488694528158, 50.62390960531435979 ) ) ;
#52946=CARTESIAN_POINT ( 'NONE',  ( -19.46398650005389541, 5.499999999999947597, 40.18269651486372851 ) ) ;
#52947=CARTESIAN_POINT ( 'NONE',  ( 18.67979575497178502, 10.72451020669898547, 89.16557627198102409 ) ) ;
#52949=CARTESIAN_POINT ( 'NONE',  ( -21.53943276465977519, 0.05219959533907696930, 51.24890960531436690 ) ) ;
#52950=CARTESIAN_POINT ( 'NONE',  ( 16.51473224551069308, 9.474510206698969483, 49.16557627198102409 ) ) ;
#52951=CARTESIAN_POINT ( 'NONE',  ( 16.52544592524335698, 4.483927247898782831, 61.45942372801901854 ) ) ;
#52953=CARTESIAN_POINT ( 'NONE',  ( -18.62759615963255300, -10.81492255796106328, 44.16775706135234714 ) ) ;
#52954=CARTESIAN_POINT ( 'NONE',  ( 8.224510206698953496, -14.34966873604960469, 62.91557627198102409 ) ) ;
#52956=CARTESIAN_POINT ( 'NONE',  ( -16.55341960407617563, 4.379528057220093196, 43.54275706135235424 ) ) ;
#52957=CARTESIAN_POINT ( 'NONE',  ( 8.314922557960818139, 14.29746914071049879, 104.5822429386477097 ) ) ;
#52958=CARTESIAN_POINT ( 'NONE',  ( -5.049401038297874678, -19.05341960407617918, 49.79275706135231871 ) ) ;
#52959=CARTESIAN_POINT ( 'NONE',  ( -8.224510206698948167, 14.34966873604960824, 60.41557627198102409 ) ) ;
#52960=CARTESIAN_POINT ( 'NONE',  ( 0.05219959533937995610, -21.53943276465977519, 35.00109039468568284 ) ) ;
#52961=CARTESIAN_POINT ( 'NONE',  ( 19.02544592524343514, -5.153800228976328945, 28.54057627198102409 ) ) ;
#52962=CARTESIAN_POINT ( 'NONE',  ( -5.719274019375978568, 21.55341960407610458, 85.20724293864770971 ) ) ;
#52963=CARTESIAN_POINT ( 'NONE',  ( 16.46253265017160672, -9.564922557960803928, 108.3322429386476955 ) ) ;
#52964=CARTESIAN_POINT ( 'NONE',  ( -14.29746914071049879, 8.314922557960819915, 80.83224293864769550 ) ) ;
#52965=CARTESIAN_POINT ( 'NONE',  ( 16.46253265017160672, -9.564922557960803928, 113.3322429386476955 ) ) ;
#52967=CARTESIAN_POINT ( 'NONE',  ( -0.05219959533936034679, 19.03943276465977164, 77.50109039468566152 ) ) ;
#52968=CARTESIAN_POINT ( 'NONE',  ( 5.823673210054444382, -21.52544592524334988, 20.20942372801900788 ) ) ;
#52969=CARTESIAN_POINT ( 'NONE',  ( 16.51473224551069308, 9.474510206698969483, 64.16557627198102409 ) ) ;
#52970=CARTESIAN_POINT ( 'NONE',  ( -19.05341960407617563, 5.049401038297882671, 58.54275706135234003 ) ) ;
#52971=CARTESIAN_POINT ( 'NONE',  ( -5.153800228976328057, -19.02544592524343514, 32.29057627198102409 ) ) ;
#52972=CARTESIAN_POINT ( 'NONE',  ( 18.67979575497194134, -10.72451020669871369, 80.83442372801901854 ) ) ;
#52973=CARTESIAN_POINT ( 'NONE',  ( -8.314922557960811034, -14.29746914071050412, 62.08224293864769550 ) ) ;
#52974=CARTESIAN_POINT ( 'NONE',  ( 12.14591786802309770, 12.06949235617756955, 54.37390960531435979 ) ) ;
#52975=CARTESIAN_POINT ( 'NONE',  ( -16.51473224551069308, -9.474510206698971260, 66.66557627198102409 ) ) ;
#52976=CARTESIAN_POINT ( 'NONE',  ( -21.52544592524343514, 5.823673210054127303, 86.04057627198102409 ) ) ;
#52977=CARTESIAN_POINT ( 'NONE',  ( -13.89961937509977652, 13.97604488694528158, 55.62390960531434558 ) ) ;
#52979=CARTESIAN_POINT ( 'NONE',  ( -10.72451020669898014, 18.67979575497178502, 75.41557627198102409 ) ) ;
#52980=CARTESIAN_POINT ( 'NONE',  ( -18.62759615963255300, -10.81492255796106328, 99.16775706135234714 ) ) ;
#52981=CARTESIAN_POINT ( 'NONE',  ( -18.22780087662121673, -5.500000000000063061, 46.48459894673893444 ) ) ;
#52982=CARTESIAN_POINT ( 'NONE',  ( -16.55341960407617563, 4.379528057220093196, 98.54275706135234714 ) ) ;
#52983=CARTESIAN_POINT ( 'NONE',  ( -14.29746914071049879, 8.314922557960819915, 100.8322429386477097 ) ) ;
#52985=CARTESIAN_POINT ( 'NONE',  ( -19.03943276465977164, -0.05219959533935918106, 93.75109039468566152 ) ) ;
#52987=CARTESIAN_POINT ( 'NONE',  ( 18.67979575497178502, 10.72451020669898547, 109.1655762719810383 ) ) ;
#52988=CARTESIAN_POINT ( 'NONE',  ( 13.97604488694548053, -13.89961937509957401, 55.62609039468566863 ) ) ;
#52989=CARTESIAN_POINT ( 'NONE',  ( 12.06949235617739724, 12.14591786802326823, 96.87609039468568994 ) ) ;
#52990=CARTESIAN_POINT ( 'NONE',  ( -9.564922557961040184, 16.46253265017147172, 27.91775706135232582 ) ) ;
#52991=CARTESIAN_POINT ( 'NONE',  ( 5.049401038298161559, -19.05341960407611168, 102.7072429386476955 ) ) ;
#52992=CARTESIAN_POINT ( 'NONE',  ( -21.52544592524343514, 5.823673210054127303, 61.04057627198103120 ) ) ;
#52993=CARTESIAN_POINT ( 'NONE',  ( 9.474510206698971260, -16.51473224551069308, 22.91557627198102765 ) ) ;
#52994=CARTESIAN_POINT ( 'NONE',  ( -0.05219959533909027116, -19.03943276465977164, 37.49890960531436690 ) ) ;
#52995=CARTESIAN_POINT ( 'NONE',  ( -15.72974639402176322, -15.80617190586768395, 104.3760903946856899 ) ) ;
#52996=CARTESIAN_POINT ( 'NONE',  ( 16.52544592524335698, 4.483927247898782831, 76.45942372801901854 ) ) ;
#52997=CARTESIAN_POINT ( 'NONE',  ( -10.81492255796105439, 18.62759615963255655, 32.91775706135234714 ) ) ;
#52998=CARTESIAN_POINT ( 'NONE',  ( 12.06949235617739724, 12.14591786802326823, 41.87609039468568284 ) ) ;
#52999=CARTESIAN_POINT ( 'NONE',  ( -5.049401038298153566, 19.05341960407611168, 105.2072429386476671 ) ) ;
#53000=CARTESIAN_POINT ( 'NONE',  ( 13.89961937509977652, -13.97604488694527269, 48.12390960531435979 ) ) ;
#53001=CARTESIAN_POINT ( 'NONE',  ( 19.02544592524343514, -5.153800228976328945, 68.54057627198103830 ) ) ;
#53002=CARTESIAN_POINT ( 'NONE',  ( 8.224510206698742110, 14.34966873604972548, 47.08442372801901854 ) ) ;
#53003=CARTESIAN_POINT ( 'NONE',  ( 8.314922557960818139, 14.29746914071049879, 89.58224293864768129 ) ) ;
#53004=CARTESIAN_POINT ( 'NONE',  ( -0.05219959533934338120, 16.53943276465976808, 102.5010903946856899 ) ) ;
#53006=CARTESIAN_POINT ( 'NONE',  ( -15.80617190586768217, 15.72974639402176855, 53.12609039468568284 ) ) ;
#53007=CARTESIAN_POINT ( 'NONE',  ( 5.049401038298161559, -19.05341960407611168, 82.70724293864770971 ) ) ;
#53008=CARTESIAN_POINT ( 'NONE',  ( -16.46253265017160317, 9.564922557960807481, 60.83224293864769550 ) ) ;
#53009=CARTESIAN_POINT ( 'NONE',  ( 5.153800228976335163, 19.02544592524342804, 89.79057627198102409 ) ) ;
#53010=CARTESIAN_POINT ( 'NONE',  ( 12.14591786802309770, 12.06949235617756955, 49.37390960531436690 ) ) ;
#53011=CARTESIAN_POINT ( 'NONE',  ( -16.52544592524335698, -4.483927247898792601, 93.95942372801903275 ) ) ;
#53012=CARTESIAN_POINT ( 'NONE',  ( 4.379528057220339221, -16.55341960407611168, 22.70724293864769194 ) ) ;
#53013=EDGE_LOOP ( 'NONE', ( #28443, #55238, #95964, #102661 ) ) ;
#53014=CARTESIAN_POINT ( 'NONE',  ( 0.05219959533936267826, -19.03943276465977164, 50.00109039468566863 ) ) ;
#53015=CARTESIAN_POINT ( 'NONE',  ( -19.02544592524342804, 5.153800228976336051, 116.0405762719810383 ) ) ;
#53016=CARTESIAN_POINT ( 'NONE',  ( 16.46253265017160672, -9.564922557960803928, 68.33224293864770971 ) ) ;
#53017=CARTESIAN_POINT ( 'NONE',  ( -19.02544592524334988, -5.153800228976617603, 38.95942372801900433 ) ) ;
#53020=CARTESIAN_POINT ( 'NONE',  ( 19.02544592524334988, 5.153800228976608722, 86.45942372801900433 ) ) ;
#53021=CARTESIAN_POINT ( 'NONE',  ( -4.379528057220086978, -16.55341960407618274, 69.79275706135234714 ) ) ;
#53022=CARTESIAN_POINT ( 'NONE',  ( 17.31728774477273802, 6.344390552232390235, 91.68093348310684121 ) ) ;
#53023=CARTESIAN_POINT ( 'NONE',  ( -16.51473224551069308, -9.474510206698971260, 91.66557627198103830 ) ) ;
#53024=CARTESIAN_POINT ( 'NONE',  ( -10.72451020669870658, -18.67979575497194134, 34.58442372801900433 ) ) ;
#53025=CARTESIAN_POINT ( 'NONE',  ( 16.46253265017146816, 9.564922557961045513, 81.66775706135233293 ) ) ;
#53026=CARTESIAN_POINT ( 'NONE',  ( 17.12812012977029497, 6.668231424565951748, 88.85948759323147783 ) ) ;
#53027=CARTESIAN_POINT ( 'NONE',  ( -19.05341960407611168, -5.049401038298163336, 51.45724293864770260 ) ) ;
#53028=CARTESIAN_POINT ( 'NONE',  ( -19.03943276465977164, 0.05219959533909376836, 91.24890960531436690 ) ) ;
#53029=CARTESIAN_POINT ( 'NONE',  ( 12.06949235617757843, -12.14591786802309237, 48.12390960531436690 ) ) ;
#53030=CARTESIAN_POINT ( 'NONE',  ( 16.46253265017160672, -9.564922557960803928, 33.33224293864770260 ) ) ;
#53031=CARTESIAN_POINT ( 'NONE',  ( -9.564922557961040184, 16.46253265017147172, 52.91775706135233293 ) ) ;
#53032=CARTESIAN_POINT ( 'NONE',  ( 4.379528057220339221, -16.55341960407611168, 92.70724293864770971 ) ) ;
#53033=CARTESIAN_POINT ( 'NONE',  ( -13.97604488694547697, 13.89961937509957934, 33.12609039468566863 ) ) ;
#53034=CARTESIAN_POINT ( 'NONE',  ( 16.51473224551069308, 9.474510206698969483, 64.16557627198102409 ) ) ;
#53037=CARTESIAN_POINT ( 'NONE',  ( -15.72974639402197994, 15.80617190586746368, 65.62390960531436690 ) ) ;
#53038=CARTESIAN_POINT ( 'NONE',  ( -8.224510206698948167, 14.34966873604960824, 55.41557627198102409 ) ) ;
#53039=CARTESIAN_POINT ( 'NONE',  ( 9.564922557961047289, -16.46253265017146816, 25.41775706135234003 ) ) ;
#53040=CARTESIAN_POINT ( 'NONE',  ( -9.474510206698964154, 16.51473224551069663, 100.4155762719810241 ) ) ;
#53041=CARTESIAN_POINT ( 'NONE',  ( 21.55341960407610458, 5.719274019375980345, 23.95724293864769550 ) ) ;
#53042=CARTESIAN_POINT ( 'NONE',  ( 16.46253265017160672, -9.564922557960803928, 48.33224293864769550 ) ) ;
#53043=CARTESIAN_POINT ( 'NONE',  ( 0.05219959533909260263, 19.03943276465977164, 24.99890960531435269 ) ) ;
#53044=CARTESIAN_POINT ( 'NONE',  ( -4.483927247898539470, -16.52544592524342804, 97.29057627198105251 ) ) ;
#53045=CARTESIAN_POINT ( 'NONE',  ( -0.05219959533907301413, -21.53943276465977519, 107.4989096053143669 ) ) ;
#53046=CARTESIAN_POINT ( 'NONE',  ( -13.89961937509977652, 13.97604488694528158, 100.6239096053143669 ) ) ;
#53047=CARTESIAN_POINT ( 'NONE',  ( -0.05219959533907301413, -21.53943276465977519, 107.4989096053143669 ) ) ;
#53048=CARTESIAN_POINT ( 'NONE',  ( 16.51473224551069308, 9.474510206698969483, 99.16557627198102409 ) ) ;
#53049=CARTESIAN_POINT ( 'NONE',  ( -8.314922557960811034, -14.29746914071050412, 112.0822429386477097 ) ) ;
#53050=CARTESIAN_POINT ( 'NONE',  ( 21.53943276465977519, 0.05219959533937863772, 81.25109039468568994 ) ) ;
#53051=CARTESIAN_POINT ( 'NONE',  ( 5.823673210054125526, 21.52544592524343514, 89.79057627198103830 ) ) ;
#53052=CARTESIAN_POINT ( 'NONE',  ( 16.81555441253553695, -7.025013491695474954, 108.1368544533426501 ) ) ;
#53054=CARTESIAN_POINT ( 'NONE',  ( 17.59860650958989936, 7.585241751807028088, 59.07662985737508166 ) ) ;
#53055=CARTESIAN_POINT ( 'NONE',  ( 16.53943276465976808, 0.05219959533934440121, 41.25109039468568284 ) ) ;
#53056=CARTESIAN_POINT ( 'NONE',  ( 0.05219959533910956823, 16.53943276465976808, 104.9989096053143669 ) ) ;
#53058=CARTESIAN_POINT ( 'NONE',  ( -17.49999999999998579, -3.850315288878773945, 110.7337086939655251 ) ) ;
#53059=CARTESIAN_POINT ( 'NONE',  ( 16.51473224551069308, 9.474510206698969483, 54.16557627198103120 ) ) ;
#53060=CARTESIAN_POINT ( 'NONE',  ( -4.379528057220328563, 16.55341960407611168, 90.20724293864770971 ) ) ;
#53061=CARTESIAN_POINT ( 'NONE',  ( 15.80617190586746368, 15.72974639402197994, 39.37390960531436690 ) ) ;
#53062=CARTESIAN_POINT ( 'NONE',  ( 12.06949235617757843, -12.14591786802309237, 63.12390960531435979 ) ) ;
#53063=CARTESIAN_POINT ( 'NONE',  ( 16.55341960407618274, -4.379528057220086978, 21.04275706135234714 ) ) ;
#53064=CARTESIAN_POINT ( 'NONE',  ( -5.823673210054431948, 21.52544592524334988, 77.70942372801900433 ) ) ;
#53067=CARTESIAN_POINT ( 'NONE',  ( 14.34966873604972726, -8.224510206698740333, 95.83442372801903275 ) ) ;
#53068=CARTESIAN_POINT ( 'NONE',  ( -8.224510206698948167, 14.34966873604960824, 45.41557627198103830 ) ) ;
#53069=CARTESIAN_POINT ( 'NONE',  ( 9.474510206698971260, -16.51473224551069308, 32.91557627198102409 ) ) ;
#53070=CARTESIAN_POINT ( 'NONE',  ( -9.564922557960796823, -16.46253265017161027, 87.08224293864769550 ) ) ;
#53071=CARTESIAN_POINT ( 'NONE',  ( 5.823673210054125526, 21.52544592524343514, 94.79057627198105251 ) ) ;
#53072=CARTESIAN_POINT ( 'NONE',  ( 14.29746914071037800, 8.314922557961029526, 26.66775706135235424 ) ) ;
#53073=CARTESIAN_POINT ( 'NONE',  ( -8.314922557960811034, -14.29746914071050412, 67.08224293864770971 ) ) ;
#53074=CARTESIAN_POINT ( 'NONE',  ( -21.53943276465977519, -0.05219959533937600094, 78.75109039468568994 ) ) ;
#53075=CARTESIAN_POINT ( 'NONE',  ( -12.14591786802326823, 12.06949235617739902, 103.1260903946856757 ) ) ;
#53076=CARTESIAN_POINT ( 'NONE',  ( 16.31925111598406630, -7.325300261831833915, 47.66424538967169156 ) ) ;
#53077=CARTESIAN_POINT ( 'NONE',  ( -18.56101223717332260, -5.499999999999952927, 66.44978406935679516 ) ) ;
#53078=CARTESIAN_POINT ( 'NONE',  ( -14.34966873604960291, -8.224510206698953496, 21.66557627198102409 ) ) ;
#53079=CARTESIAN_POINT ( 'NONE',  ( -8.224510206698735004, -14.34966873604973081, 74.58442372801901854 ) ) ;
#53080=CARTESIAN_POINT ( 'NONE',  ( 13.89961937509977652, -13.97604488694527269, 83.12390960531436690 ) ) ;
#53081=CARTESIAN_POINT ( 'NONE',  ( -5.153800228976328057, -19.02544592524343514, 82.29057627198103830 ) ) ;
#53082=CARTESIAN_POINT ( 'NONE',  ( 21.55341960407619695, -5.719274019375665929, 81.04275706135236135 ) ) ;
#53083=CARTESIAN_POINT ( 'NONE',  ( -8.314922557961024197, 14.29746914071037800, 87.91775706135234714 ) ) ;
#53084=CARTESIAN_POINT ( 'NONE',  ( 0.05219959533910956823, 16.53943276465976808, 54.99890960531435269 ) ) ;
#53085=CARTESIAN_POINT ( 'NONE',  ( 16.46253265017160672, -9.564922557960803928, 63.33224293864769550 ) ) ;
#53087=CARTESIAN_POINT ( 'NONE',  ( -16.52544592524335698, -4.483927247898792601, 18.95942372801901143 ) ) ;
#53088=CARTESIAN_POINT ( 'NONE',  ( 16.52544592524342804, -4.483927247898539470, 113.5405762719810383 ) ) ;
#53089=CARTESIAN_POINT ( 'NONE',  ( 5.049401038298161559, -19.05341960407611168, 82.70724293864770971 ) ) ;
#53090=CARTESIAN_POINT ( 'NONE',  ( -16.53943276465976808, -0.05219959533934237506, 23.75109039468567929 ) ) ;
#53092=CARTESIAN_POINT ( 'NONE',  ( 19.02544592524334988, 5.153800228976608722, 26.45942372801899722 ) ) ;
#53093=CARTESIAN_POINT ( 'NONE',  ( 12.06949235617739724, 12.14591786802326823, 86.87609039468568994 ) ) ;
#53094=CARTESIAN_POINT ( 'NONE',  ( -5.153800228976607833, 19.02544592524334988, 97.70942372801900433 ) ) ;
#53095=CARTESIAN_POINT ( 'NONE',  ( 14.29746914071049879, -8.314922557960816363, 113.3322429386476955 ) ) ;
#53096=CARTESIAN_POINT ( 'NONE',  ( 12.14591786802327356, -12.06949235617739191, 65.62609039468568994 ) ) ;
#53097=CARTESIAN_POINT ( 'NONE',  ( 8.224510206698742110, 14.34966873604972548, 57.08442372801901854 ) ) ;
#53099=CARTESIAN_POINT ( 'NONE',  ( 16.51473224551083163, -9.474510206698727899, 50.83442372801899722 ) ) ;
#53100=CARTESIAN_POINT ( 'NONE',  ( -18.67979575497193778, 10.72451020669871902, 98.33442372801901854 ) ) ;
#53101=CARTESIAN_POINT ( 'NONE',  ( 16.46253265017160672, -9.564922557960803928, 28.33224293864769550 ) ) ;
#53102=CARTESIAN_POINT ( 'NONE',  ( -5.153800228976328057, -19.02544592524343514, 82.29057627198103830 ) ) ;
#53103=CARTESIAN_POINT ( 'NONE',  ( 4.483927247898545687, 16.52544592524342804, 69.79057627198102409 ) ) ;
#53104=AXIS2_PLACEMENT_3D ( 'NONE', #19944, #170656, #108975 ) ;
#53105=CARTESIAN_POINT ( 'NONE',  ( -21.52544592524334988, -5.823673210054445271, 93.95942372801903275 ) ) ;
#53106=CARTESIAN_POINT ( 'NONE',  ( -5.153800228976607833, 19.02544592524334988, 62.70942372801899722 ) ) ;
#53107=CARTESIAN_POINT ( 'NONE',  ( -9.474510206698720793, -16.51473224551083518, 39.58442372801899722 ) ) ;
#53108=CARTESIAN_POINT ( 'NONE',  ( 0.05219959533907565091, 21.53943276465977519, 34.99890960531435979 ) ) ;
#53109=CARTESIAN_POINT ( 'NONE',  ( -15.72974639402176322, -15.80617190586768395, 94.37609039468568994 ) ) ;
#53110=CARTESIAN_POINT ( 'NONE',  ( 5.049401038298161559, -19.05341960407611168, 77.70724293864765286 ) ) ;
#53111=CARTESIAN_POINT ( 'NONE',  ( -5.719274019375665041, -21.55341960407619695, 104.7927570613523898 ) ) ;
#53112=CARTESIAN_POINT ( 'NONE',  ( 18.62759615963271287, -10.81492255796078972, 53.33224293864769550 ) ) ;
#53113=CARTESIAN_POINT ( 'NONE',  ( -0.05219959533909027116, -19.03943276465977164, 97.49890960531436690 ) ) ;
#53114=CARTESIAN_POINT ( 'NONE',  ( -19.02544592524334988, -5.153800228976617603, 78.95942372801900433 ) ) ;
#53115=CARTESIAN_POINT ( 'NONE',  ( -5.049401038298153566, 19.05341960407611168, 105.2072429386476671 ) ) ;
#53116=CARTESIAN_POINT ( 'NONE',  ( 16.46253265017146816, 9.564922557961045513, 101.6677570613523329 ) ) ;
#53117=CARTESIAN_POINT ( 'NONE',  ( -16.53943276465976808, -0.05219959533934237506, 48.75109039468568284 ) ) ;
#53118=CARTESIAN_POINT ( 'NONE',  ( 14.29746914071049879, -8.314922557960816363, 108.3322429386477097 ) ) ;
#53119=CARTESIAN_POINT ( 'NONE',  ( 9.474510206698971260, -16.51473224551069308, 77.91557627198103830 ) ) ;
#53120=CARTESIAN_POINT ( 'NONE',  ( 10.81492255796078972, 18.62759615963270932, 59.58224293864770260 ) ) ;
#53121=CARTESIAN_POINT ( 'NONE',  ( 12.06949235617739724, 12.14591786802326823, 31.87609039468567929 ) ) ;
#53122=CARTESIAN_POINT ( 'NONE',  ( -0.05219959533937732626, 21.53943276465977519, 37.50109039468568284 ) ) ;
#53123=CARTESIAN_POINT ( 'NONE',  ( -10.72451020669870658, -18.67979575497194134, 89.58442372801901854 ) ) ;
#53124=CARTESIAN_POINT ( 'NONE',  ( -14.29746914071037622, -8.314922557961029526, 79.16775706135234714 ) ) ;
#53125=CARTESIAN_POINT ( 'NONE',  ( -16.51473224551069308, -9.474510206698971260, 76.66557627198103830 ) ) ;
#53126=CARTESIAN_POINT ( 'NONE',  ( 4.379528057220339221, -16.55341960407611168, 77.70724293864770971 ) ) ;
#53127=CARTESIAN_POINT ( 'NONE',  ( 16.53943276465976808, -0.05219959533910856209, 23.74890960531435269 ) ) ;
#53128=CARTESIAN_POINT ( 'NONE',  ( -9.564922557961040184, 16.46253265017147172, 52.91775706135233293 ) ) ;
#53129=CARTESIAN_POINT ( 'NONE',  ( -18.67979575497193778, 10.72451020669871902, 38.33442372801900433 ) ) ;
#53130=CARTESIAN_POINT ( 'NONE',  ( 8.224510206698953496, -14.34966873604960469, 72.91557627198103830 ) ) ;
#53131=CARTESIAN_POINT ( 'NONE',  ( 0.05219959533909260263, 19.03943276465977164, 114.9989096053143669 ) ) ;
#53132=CARTESIAN_POINT ( 'NONE',  ( -4.483927247898782831, 16.52544592524335698, 102.7094237280190185 ) ) ;
#53133=CARTESIAN_POINT ( 'NONE',  ( 15.72974639402176855, 15.80617190586768217, 71.87609039468568994 ) ) ;
#53134=CARTESIAN_POINT ( 'NONE',  ( -12.14591786802326823, 12.06949235617739902, 43.12609039468568284 ) ) ;
#53135=CARTESIAN_POINT ( 'NONE',  ( -21.52544592524334988, -5.823673210054445271, 43.95942372801902565 ) ) ;
#53137=CARTESIAN_POINT ( 'NONE',  ( 0.05219959533907565091, 21.53943276465977519, 114.9989096053143669 ) ) ;
#53138=CARTESIAN_POINT ( 'NONE',  ( 8.224510206698953496, -14.34966873604960469, 97.91557627198103830 ) ) ;
#53140=CARTESIAN_POINT ( 'NONE',  ( -14.34966873604960291, -8.224510206698953496, 51.66557627198102409 ) ) ;
#53141=CARTESIAN_POINT ( 'NONE',  ( -8.314922557961024197, 14.29746914071037800, 92.91775706135236135 ) ) ;
#53142=CARTESIAN_POINT ( 'NONE',  ( 19.03943276465977164, -0.05219959533909143690, 38.74890960531436690 ) ) ;
#53143=CARTESIAN_POINT ( 'NONE',  ( 0.05219959533907565091, 21.53943276465977519, 39.99890960531436690 ) ) ;
#53144=CARTESIAN_POINT ( 'NONE',  ( 4.483927247898545687, 16.52544592524342804, 79.79057627198102409 ) ) ;
#53145=CARTESIAN_POINT ( 'NONE',  ( -18.62759615963270932, 10.81492255796079327, 80.83224293864769550 ) ) ;
#53146=CARTESIAN_POINT ( 'NONE',  ( -19.03943276465977164, 0.05219959533909376836, 91.24890960531436690 ) ) ;
#53147=CARTESIAN_POINT ( 'NONE',  ( 19.05341960407611168, 5.049401038298154454, 33.95724293864769550 ) ) ;
#53148=CARTESIAN_POINT ( 'NONE',  ( -13.97604488694547697, 13.89961937509957934, 88.12609039468563310 ) ) ;
#53149=CARTESIAN_POINT ( 'NONE',  ( -21.52544592524343514, 5.823673210054127303, 31.04057627198102409 ) ) ;
#53150=CARTESIAN_POINT ( 'NONE',  ( -15.80617190586768217, 15.72974639402176855, 58.12609039468568994 ) ) ;
#53151=CARTESIAN_POINT ( 'NONE',  ( -5.719274019375978568, 21.55341960407610458, 60.20724293864768839 ) ) ;
#53152=CARTESIAN_POINT ( 'NONE',  ( 13.89961937509977652, -13.97604488694527269, 58.12390960531436690 ) ) ;
#53153=CARTESIAN_POINT ( 'NONE',  ( -9.564922557960796823, -16.46253265017161027, 82.08224293864768129 ) ) ;
#53155=CARTESIAN_POINT ( 'NONE',  ( -16.53943276465976808, -0.05219959533934237506, 48.75109039468568284 ) ) ;
#53156=CARTESIAN_POINT ( 'NONE',  ( 0.05219959533937995610, -21.53943276465977519, 30.00109039468568284 ) ) ;
#53158=CARTESIAN_POINT ( 'NONE',  ( -0.05219959533937732626, 21.53943276465977519, 72.50109039468568994 ) ) ;
#53159=CARTESIAN_POINT ( 'NONE',  ( 0.05219959533909260263, 19.03943276465977164, 114.9989096053143669 ) ) ;
#53160=CARTESIAN_POINT ( 'NONE',  ( -15.80617190586745835, -15.72974639402198527, 91.87390960531436690 ) ) ;
#53161=CARTESIAN_POINT ( 'NONE',  ( 15.80617190586769283, -15.72974639402175789, 25.62609039468567929 ) ) ;
#53162=CARTESIAN_POINT ( 'NONE',  ( -14.29746914071037622, -8.314922557961029526, 69.16775706135234714 ) ) ;
#53163=CARTESIAN_POINT ( 'NONE',  ( 10.72451020669898902, -18.67979575497178502, 57.91557627198103120 ) ) ;
#53164=CARTESIAN_POINT ( 'NONE',  ( 19.05341960407617918, -5.049401038297876454, 21.04275706135232582 ) ) ;
#53165=CARTESIAN_POINT ( 'NONE',  ( -0.05219959533909027116, -19.03943276465977164, 52.49890960531436690 ) ) ;
#53166=CARTESIAN_POINT ( 'NONE',  ( 9.474510206698971260, -16.51473224551069308, 112.9155762719810383 ) ) ;
#53167=CARTESIAN_POINT ( 'NONE',  ( 19.05341960407611168, 5.049401038298154454, 93.95724293864769550 ) ) ;
#53170=CARTESIAN_POINT ( 'NONE',  ( -16.46253265017146816, -9.564922557961047289, 69.16775706135233293 ) ) ;
#53171=CARTESIAN_POINT ( 'NONE',  ( 5.823673210054125526, 21.52544592524343514, 39.79057627198103830 ) ) ;
#53172=CARTESIAN_POINT ( 'NONE',  ( 8.224510206698953496, -14.34966873604960469, 22.91557627198102765 ) ) ;
#53173=CARTESIAN_POINT ( 'NONE',  ( 13.97604488694548053, -13.89961937509957401, 100.6260903946856615 ) ) ;
#53175=CARTESIAN_POINT ( 'NONE',  ( 18.22780087662125226, -5.499999999999864997, 51.01540105326108687 ) ) ;
#53176=CARTESIAN_POINT ( 'NONE',  ( 5.049401038297881783, 19.05341960407617563, 22.29275706135233648 ) ) ;
#53177=CARTESIAN_POINT ( 'NONE',  ( 19.03943276465977164, 0.05219959533936151252, 96.25109039468567573 ) ) ;
#53178=CARTESIAN_POINT ( 'NONE',  ( -21.52544592524343514, 5.823673210054127303, 91.04057627198103830 ) ) ;
#53179=CARTESIAN_POINT ( 'NONE',  ( 19.02544592524334988, 5.153800228976608722, 51.45942372801900433 ) ) ;
#53181=CARTESIAN_POINT ( 'NONE',  ( 16.51473224551069308, 9.474510206698969483, 59.16557627198102409 ) ) ;
#53182=CARTESIAN_POINT ( 'NONE',  ( 4.483927247898545687, 16.52544592524342804, 69.79057627198102409 ) ) ;
#53184=CARTESIAN_POINT ( 'NONE',  ( -16.51473224551069308, -9.474510206698971260, 46.66557627198102409 ) ) ;
#53185=CARTESIAN_POINT ( 'NONE',  ( -0.05219959533910754901, -16.53943276465976808, 57.49890960531435979 ) ) ;
#53187=CARTESIAN_POINT ( 'NONE',  ( 4.379528057220339221, -16.55341960407611168, 32.70724293864770260 ) ) ;
#53188=CARTESIAN_POINT ( 'NONE',  ( -16.46253265017160317, 9.564922557960807481, 60.83224293864769550 ) ) ;
#53189=CARTESIAN_POINT ( 'NONE',  ( 19.05341960407617918, -5.049401038297876454, 21.04275706135232582 ) ) ;
#53190=CARTESIAN_POINT ( 'NONE',  ( 16.55341960407618274, -4.379528057220086978, 36.04275706135234714 ) ) ;
#53191=CARTESIAN_POINT ( 'NONE',  ( -0.05219959533907301413, -21.53943276465977519, 47.49890960531435979 ) ) ;
#53192=CARTESIAN_POINT ( 'NONE',  ( -0.05219959533937732626, 21.53943276465977519, 107.5010903946856899 ) ) ;
#53194=CARTESIAN_POINT ( 'NONE',  ( -13.97604488694527625, -13.89961937509977652, 61.87390960531435979 ) ) ;
#53196=CARTESIAN_POINT ( 'NONE',  ( 16.51473224551069308, 9.474510206698969483, 94.16557627198103830 ) ) ;
#53198=CARTESIAN_POINT ( 'NONE',  ( 5.719274019375673035, 21.55341960407619339, 27.29275706135234358 ) ) ;
#53199=CARTESIAN_POINT ( 'NONE',  ( 16.52544592524342804, -4.483927247898539470, 93.54057627198103830 ) ) ;
#53200=CARTESIAN_POINT ( 'NONE',  ( 10.81492255796078972, 18.62759615963270932, 89.58224293864768129 ) ) ;
#53201=CARTESIAN_POINT ( 'NONE',  ( -19.05341960407611168, -5.049401038298163336, 66.45724293864769550 ) ) ;
#53202=CARTESIAN_POINT ( 'NONE',  ( -16.51473224551069308, -9.474510206698971260, 86.66557627198102409 ) ) ;
#53203=CARTESIAN_POINT ( 'NONE',  ( 0.05219959533907565091, 21.53943276465977519, 104.9989096053143669 ) ) ;
#53205=CARTESIAN_POINT ( 'NONE',  ( 13.89961937509977652, -13.97604488694527269, 78.12390960531433848 ) ) ;
#53206=CARTESIAN_POINT ( 'NONE',  ( -4.483927247898539470, -16.52544592524342804, 107.2905762719810525 ) ) ;
#53208=CARTESIAN_POINT ( 'NONE',  ( -13.89961937509957401, -13.97604488694547875, 89.37609039468563310 ) ) ;
#53209=CARTESIAN_POINT ( 'NONE',  ( 4.483927247898545687, 16.52544592524342804, 114.7905762719810383 ) ) ;
#53210=CARTESIAN_POINT ( 'NONE',  ( 21.53943276465977519, 0.05219959533937863772, 66.25109039468567573 ) ) ;
#53211=CARTESIAN_POINT ( 'NONE',  ( -19.02544592524342804, 5.153800228976336051, 56.04057627198100988 ) ) ;
#53212=CARTESIAN_POINT ( 'NONE',  ( -21.53943276465977519, -0.05219959533937600094, 28.75109039468567929 ) ) ;
#53213=CARTESIAN_POINT ( 'NONE',  ( 15.80617190586746368, 15.72974639402197994, 104.3739096053143669 ) ) ;
#53215=CARTESIAN_POINT ( 'NONE',  ( -19.03943276465977164, 0.05219959533909376836, 71.24890960531435269 ) ) ;
#53217=CARTESIAN_POINT ( 'NONE',  ( -8.314922557961024197, 14.29746914071037800, 22.91775706135235069 ) ) ;
#53218=CARTESIAN_POINT ( 'NONE',  ( 10.81492255796078972, 18.62759615963270932, 29.58224293864769905 ) ) ;
#53219=CARTESIAN_POINT ( 'NONE',  ( 18.62759615963255655, 10.81492255796105972, 56.66775706135235424 ) ) ;
#53221=CARTESIAN_POINT ( 'NONE',  ( 5.153800228976335163, 19.02544592524342804, 114.7905762719810241 ) ) ;
#53223=CARTESIAN_POINT ( 'NONE',  ( 13.89961937509957401, 13.97604488694547697, 96.87609039468566152 ) ) ;
#53224=CARTESIAN_POINT ( 'NONE',  ( -16.51473224551069308, -9.474510206698971260, 51.66557627198102409 ) ) ;
#53225=CARTESIAN_POINT ( 'NONE',  ( -19.03943276465977164, 0.05219959533909376836, 71.24890960531435269 ) ) ;
#53226=CARTESIAN_POINT ( 'NONE',  ( -8.224510206698948167, 14.34966873604960824, 95.41557627198102409 ) ) ;
#53227=CARTESIAN_POINT ( 'NONE',  ( -9.564922557960796823, -16.46253265017161027, 102.0822429386477097 ) ) ;
#53228=CARTESIAN_POINT ( 'NONE',  ( -16.53943276465976808, 0.05219959533911058130, 96.24890960531435269 ) ) ;
#53229=CARTESIAN_POINT ( 'NONE',  ( 0.05219959533909260263, 19.03943276465977164, 99.99890960531436690 ) ) ;
#53230=CARTESIAN_POINT ( 'NONE',  ( 14.29746914071049879, -8.314922557960816363, 63.33224293864770260 ) ) ;
#53231=CARTESIAN_POINT ( 'NONE',  ( -9.474510206698964154, 16.51473224551069663, 45.41557627198103120 ) ) ;
#53232=CARTESIAN_POINT ( 'NONE',  ( -21.53943276465977519, -0.05219959533937600094, 53.75109039468568994 ) ) ;
#53233=CARTESIAN_POINT ( 'NONE',  ( -19.03943276465977164, -0.05219959533935918106, 93.75109039468566152 ) ) ;
#53234=CARTESIAN_POINT ( 'NONE',  ( -16.55341960407611168, -4.379528057220339221, 46.45724293864769550 ) ) ;
#53235=CARTESIAN_POINT ( 'NONE',  ( 10.72451020669898902, -18.67979575497178502, 107.9155762719810241 ) ) ;
#53236=CARTESIAN_POINT ( 'NONE',  ( 18.67979575497178502, 10.72451020669898547, 49.16557627198102409 ) ) ;
#53237=CARTESIAN_POINT ( 'NONE',  ( 0.05219959533909260263, 19.03943276465977164, 109.9989096053143669 ) ) ;
#53238=CARTESIAN_POINT ( 'NONE',  ( -16.53943276465976808, 0.05219959533911058130, 81.24890960531436690 ) ) ;
#53240=CARTESIAN_POINT ( 'NONE',  ( 0.05219959533909260263, 19.03943276465977164, 54.99890960531435979 ) ) ;
#53241=CARTESIAN_POINT ( 'NONE',  ( -8.314922557960811034, -14.29746914071050412, 22.08224293864769194 ) ) ;
#53242=CARTESIAN_POINT ( 'NONE',  ( 12.14591786802327356, -12.06949235617739191, 95.62609039468568994 ) ) ;
#53243=CARTESIAN_POINT ( 'NONE',  ( -14.29746914071037622, -8.314922557961029526, 79.16775706135234714 ) ) ;
#53244=CARTESIAN_POINT ( 'NONE',  ( -16.46253265017146816, -9.564922557961047289, 44.16775706135232582 ) ) ;
#53246=CARTESIAN_POINT ( 'NONE',  ( -16.46253265017160317, 9.564922557960807481, 90.83224293864769550 ) ) ;
#53247=CARTESIAN_POINT ( 'NONE',  ( 19.05341960407611168, 5.049401038298154454, 38.95724293864767418 ) ) ;
#53248=EDGE_CURVE ( 'NONE', #88472, #179813, #22767, .T. ) ;
#53249=CARTESIAN_POINT ( 'NONE',  ( 0.05219959533910956823, 16.53943276465976808, 64.99890960531435269 ) ) ;
#53250=CARTESIAN_POINT ( 'NONE',  ( -19.02544592524342804, 5.153800228976336051, 106.0405762719810241 ) ) ;
#53251=CARTESIAN_POINT ( 'NONE',  ( 21.55341960407610458, 5.719274019375980345, 38.95724293864768839 ) ) ;
#53252=CARTESIAN_POINT ( 'NONE',  ( -8.224510206698948167, 14.34966873604960824, 80.41557627198103830 ) ) ;
#53253=CARTESIAN_POINT ( 'NONE',  ( -14.29746914071037622, -8.314922557961029526, 44.16775706135234714 ) ) ;
#53254=CARTESIAN_POINT ( 'NONE',  ( 4.483927247898545687, 16.52544592524342804, 74.79057627198105251 ) ) ;
#53256=CARTESIAN_POINT ( 'NONE',  ( 19.03943276465977164, 0.05219959533936151252, 71.25109039468566152 ) ) ;
#53257=CARTESIAN_POINT ( 'NONE',  ( 16.51473224551069308, 9.474510206698969483, 104.1655762719810241 ) ) ;
#53258=CARTESIAN_POINT ( 'NONE',  ( -9.564922557961040184, 16.46253265017147172, 72.91775706135233293 ) ) ;
#53261=CARTESIAN_POINT ( 'NONE',  ( 16.53943276465976808, 0.05219959533934440121, 31.25109039468568639 ) ) ;
#53262=CARTESIAN_POINT ( 'NONE',  ( 12.06949235617739724, 12.14591786802326823, 111.8760903946856615 ) ) ;
#53263=CARTESIAN_POINT ( 'NONE',  ( -19.03943276465977164, -0.05219959533935918106, 68.75109039468566152 ) ) ;
#53264=CARTESIAN_POINT ( 'NONE',  ( -5.823673210054116645, -21.52544592524344225, 32.29057627198102409 ) ) ;
#53265=CARTESIAN_POINT ( 'NONE',  ( 15.80617190586769283, -15.72974639402175789, 70.62609039468567573 ) ) ;
#53266=CARTESIAN_POINT ( 'NONE',  ( 14.29746914071037800, 8.314922557961029526, 26.66775706135235424 ) ) ;
#53267=CARTESIAN_POINT ( 'NONE',  ( 9.564922557960805705, 16.46253265017160317, 29.58224293864769550 ) ) ;
#53268=CARTESIAN_POINT ( 'NONE',  ( 19.02544592524343514, -5.153800228976328945, 93.54057627198102409 ) ) ;
#53270=CARTESIAN_POINT ( 'NONE',  ( -16.52544592524342804, 4.483927247898546575, 86.04057627198102409 ) ) ;
#53271=CARTESIAN_POINT ( 'NONE',  ( 13.97604488694527802, 13.89961937509977652, 94.37390960531436690 ) ) ;
#53272=CARTESIAN_POINT ( 'NONE',  ( 19.02544592524343514, -5.153800228976328945, 93.54057627198102409 ) ) ;
#53274=CARTESIAN_POINT ( 'NONE',  ( 9.474510206698729675, 16.51473224551082808, 97.08442372801900433 ) ) ;
#53275=CARTESIAN_POINT ( 'NONE',  ( 15.72974639402199770, -15.80617190586745480, 83.12390960531436690 ) ) ;
#53276=CARTESIAN_POINT ( 'NONE',  ( -5.153800228976328057, -19.02544592524343514, 32.29057627198102409 ) ) ;
#53277=CARTESIAN_POINT ( 'NONE',  ( 9.564922557961047289, -16.46253265017146816, 70.41775706135233293 ) ) ;
#53278=CARTESIAN_POINT ( 'NONE',  ( -5.719274019375978568, 21.55341960407610458, 110.2072429386477239 ) ) ;
#53279=CARTESIAN_POINT ( 'NONE',  ( 19.02544592524343514, -5.153800228976328945, 73.54057627198103830 ) ) ;
#53280=CARTESIAN_POINT ( 'NONE',  ( -0.05219959533909027116, -19.03943276465977164, 102.4989096053143669 ) ) ;
#53282=CARTESIAN_POINT ( 'NONE',  ( 15.80617190586746368, 15.72974639402197994, 109.3739096053143811 ) ) ;
#53283=CARTESIAN_POINT ( 'NONE',  ( -12.14591786802309592, -12.06949235617757132, 106.8739096053143811 ) ) ;
#53284=CARTESIAN_POINT ( 'NONE',  ( 16.46253265017160672, -9.564922557960803928, 83.33224293864768129 ) ) ;
#53285=CARTESIAN_POINT ( 'NONE',  ( 16.46253265017146816, 9.564922557961045513, 66.66775706135233293 ) ) ;
#53286=CARTESIAN_POINT ( 'NONE',  ( -5.719274019375978568, 21.55341960407610458, 90.20724293864770971 ) ) ;
#53287=CARTESIAN_POINT ( 'NONE',  ( 18.67979575497178502, 10.72451020669898547, 69.16557627198102409 ) ) ;
#53289=CARTESIAN_POINT ( 'NONE',  ( 8.224510206698953496, -14.34966873604960469, 47.91557627198102409 ) ) ;
#53290=CARTESIAN_POINT ( 'NONE',  ( 5.049401038297881783, 19.05341960407617563, 22.29275706135233648 ) ) ;
#53291=CARTESIAN_POINT ( 'NONE',  ( -16.55341960407617563, 4.379528057220093196, 63.54275706135234003 ) ) ;
#53292=CARTESIAN_POINT ( 'NONE',  ( 9.564922557960805705, 16.46253265017160317, 99.58224293864770971 ) ) ;
#53293=CARTESIAN_POINT ( 'NONE',  ( -19.03943276465977164, 0.05219959533909376836, 51.24890960531436690 ) ) ;
#53294=CARTESIAN_POINT ( 'NONE',  ( 0.05219959533937995610, -21.53943276465977519, 55.00109039468568284 ) ) ;
#53295=CARTESIAN_POINT ( 'NONE',  ( 5.823673210054444382, -21.52544592524334988, 60.20942372801902565 ) ) ;
#53296=CARTESIAN_POINT ( 'NONE',  ( -16.46253265017160317, 9.564922557960807481, 60.83224293864769550 ) ) ;
#53297=CARTESIAN_POINT ( 'NONE',  ( 18.62759615963255655, 10.81492255796105972, 41.66775706135235424 ) ) ;
#53298=CARTESIAN_POINT ( 'NONE',  ( 19.02544592524334988, 5.153800228976608722, 76.45942372801897591 ) ) ;
#53299=CARTESIAN_POINT ( 'NONE',  ( 9.564922557961047289, -16.46253265017146816, 75.41775706135234714 ) ) ;
#53300=CARTESIAN_POINT ( 'NONE',  ( -9.564922557960796823, -16.46253265017161027, 42.08224293864769550 ) ) ;
#53301=CARTESIAN_POINT ( 'NONE',  ( 16.52544592524335698, 4.483927247898782831, 81.45942372801900433 ) ) ;
#53302=CARTESIAN_POINT ( 'NONE',  ( 5.049401038298161559, -19.05341960407611168, 47.70724293864770260 ) ) ;
#53304=CARTESIAN_POINT ( 'NONE',  ( -5.049401038298153566, 19.05341960407611168, 95.20724293864770971 ) ) ;
#53305=CARTESIAN_POINT ( 'NONE',  ( 9.564922557960805705, 16.46253265017160317, 44.58224293864769550 ) ) ;
#53307=CARTESIAN_POINT ( 'NONE',  ( -18.62759615963270932, 10.81492255796079327, 90.83224293864769550 ) ) ;
#53308=CARTESIAN_POINT ( 'NONE',  ( -12.06949235617739369, -12.14591786802326823, 54.37609039468568994 ) ) ;
#53309=CARTESIAN_POINT ( 'NONE',  ( 13.97604488694548053, -13.89961937509957401, 20.62609039468567573 ) ) ;
#53310=CARTESIAN_POINT ( 'NONE',  ( 19.02544592524343514, -5.153800228976328945, 53.54057627198102409 ) ) ;
#53311=CARTESIAN_POINT ( 'NONE',  ( 16.55341960407611168, 4.379528057220329451, 48.95724293864770971 ) ) ;
#53312=CARTESIAN_POINT ( 'NONE',  ( -4.483927247898539470, -16.52544592524342804, 82.29057627198103830 ) ) ;
#53313=CARTESIAN_POINT ( 'NONE',  ( -16.51473224551069308, -9.474510206698971260, 76.66557627198103830 ) ) ;
#53314=CARTESIAN_POINT ( 'NONE',  ( 5.823673210054444382, -21.52544592524334988, 35.20942372801901854 ) ) ;
#53315=CARTESIAN_POINT ( 'NONE',  ( -19.02544592524342804, 5.153800228976336051, 91.04057627198100988 ) ) ;
#53316=CARTESIAN_POINT ( 'NONE',  ( 18.62759615963255655, 10.81492255796105972, 101.6677570613523613 ) ) ;
#53317=CARTESIAN_POINT ( 'NONE',  ( -16.52544592524335698, -4.483927247898792601, 68.95942372801901854 ) ) ;
#53318=CARTESIAN_POINT ( 'NONE',  ( 18.67979575497194134, -10.72451020669871369, 30.83442372801902209 ) ) ;
#53319=CARTESIAN_POINT ( 'NONE',  ( -0.05219959533909027116, -19.03943276465977164, 112.4989096053143669 ) ) ;
#53320=CARTESIAN_POINT ( 'NONE',  ( 21.55341960407610458, 5.719274019375980345, 83.95724293864770971 ) ) ;
#53321=CARTESIAN_POINT ( 'NONE',  ( -16.53943276465976808, 0.05219959533911058130, 41.24890960531435269 ) ) ;
#53322=CARTESIAN_POINT ( 'NONE',  ( -5.049401038298153566, 19.05341960407611168, 40.20724293864768839 ) ) ;
#53323=CARTESIAN_POINT ( 'NONE',  ( -16.55341960407611168, -4.379528057220339221, 66.45724293864768129 ) ) ;
#53324=CARTESIAN_POINT ( 'NONE',  ( -5.719274019375978568, 21.55341960407610458, 30.20724293864769550 ) ) ;
#53325=CARTESIAN_POINT ( 'NONE',  ( -13.97604488694547697, 13.89961937509957934, 33.12609039468566863 ) ) ;
#53326=CARTESIAN_POINT ( 'NONE',  ( -4.379528057220328563, 16.55341960407611168, 105.2072429386477097 ) ) ;
#53327=CARTESIAN_POINT ( 'NONE',  ( -13.97604488694527625, -13.89961937509977652, 111.8739096053143243 ) ) ;
#53328=ORIENTED_EDGE ( 'NONE', *, *, #35102, .F. ) ;
#53329=CARTESIAN_POINT ( 'NONE',  ( -16.53943276465976808, -0.05219959533934237506, 58.75109039468568994 ) ) ;
#53330=CARTESIAN_POINT ( 'NONE',  ( -19.05341960407611168, -5.049401038298163336, 51.45724293864770260 ) ) ;
#53332=CARTESIAN_POINT ( 'NONE',  ( -4.483927247898782831, 16.52544592524335698, 87.70942372801901854 ) ) ;
#53333=CARTESIAN_POINT ( 'NONE',  ( -19.05341960407617563, 5.049401038297882671, 113.5427570613523471 ) ) ;
#53334=CARTESIAN_POINT ( 'NONE',  ( 5.823673210054444382, -21.52544592524334988, 75.20942372801901854 ) ) ;
#53335=CARTESIAN_POINT ( 'NONE',  ( 19.03943276465977164, -0.05219959533909143690, 73.74890960531435269 ) ) ;
#53336=CARTESIAN_POINT ( 'NONE',  ( -21.53943276465977519, 0.05219959533907696930, 91.24890960531436690 ) ) ;
#53337=CARTESIAN_POINT ( 'NONE',  ( -8.224510206698735004, -14.34966873604973081, 39.58442372801901143 ) ) ;
#53339=CARTESIAN_POINT ( 'NONE',  ( -14.34966873604960291, -8.224510206698953496, 106.6655762719810383 ) ) ;
#53340=CARTESIAN_POINT ( 'NONE',  ( -8.224510206698735004, -14.34966873604973081, 19.58442372801901143 ) ) ;
#53341=CARTESIAN_POINT ( 'NONE',  ( -5.153800228976607833, 19.02544592524334988, 77.70942372801900433 ) ) ;
#53342=CARTESIAN_POINT ( 'NONE',  ( -21.55341960407610458, -5.719274019375992779, 76.45724293864769550 ) ) ;
#53343=CARTESIAN_POINT ( 'NONE',  ( 5.153800228976615827, -19.02544592524334988, 55.20942372801899722 ) ) ;
#53344=CARTESIAN_POINT ( 'NONE',  ( -19.03943276465977164, 0.05219959533909376836, 111.2489096053143669 ) ) ;
#53345=CARTESIAN_POINT ( 'NONE',  ( -18.62759615963270932, 10.81492255796079327, 85.83224293864768129 ) ) ;
#53346=CARTESIAN_POINT ( 'NONE',  ( 17.50000000000013856, 3.417042746626917538, 27.32619603767528105 ) ) ;
#53347=CARTESIAN_POINT ( 'NONE',  ( 19.05341960407611168, 5.049401038298154454, 63.95724293864769550 ) ) ;
#53350=CARTESIAN_POINT ( 'NONE',  ( 16.46253265017146816, 9.564922557961045513, 111.6677570613523329 ) ) ;
#53352=CARTESIAN_POINT ( 'NONE',  ( 18.67979575497194134, -10.72451020669871369, 55.83442372801901854 ) ) ;
#53353=CARTESIAN_POINT ( 'NONE',  ( 15.80617190586746368, 15.72974639402197994, 109.3739096053143811 ) ) ;
#53354=CARTESIAN_POINT ( 'NONE',  ( 16.55341960407611168, 4.379528057220329451, 58.95724293864770971 ) ) ;
#53355=CARTESIAN_POINT ( 'NONE',  ( 13.97604488694527802, 13.89961937509977652, 69.37390960531436690 ) ) ;
#53357=CARTESIAN_POINT ( 'NONE',  ( -5.823673210054431948, 21.52544592524334988, 67.70942372801901854 ) ) ;
#53358=CARTESIAN_POINT ( 'NONE',  ( -12.06949235617739369, -12.14591786802326823, 19.37609039468568639 ) ) ;
#53359=CARTESIAN_POINT ( 'NONE',  ( 9.564922557961047289, -16.46253265017146816, 25.41775706135234003 ) ) ;
#53360=CARTESIAN_POINT ( 'NONE',  ( -15.72974639402176322, -15.80617190586768395, 44.37609039468567573 ) ) ;
#53361=CARTESIAN_POINT ( 'NONE',  ( 15.72974639402199770, -15.80617190586745480, 108.1239096053143811 ) ) ;
#53362=CARTESIAN_POINT ( 'NONE',  ( -15.72974639402197994, 15.80617190586746368, 60.62390960531437401 ) ) ;
#53363=CARTESIAN_POINT ( 'NONE',  ( -16.51473224551082808, 9.474510206698731452, 98.33442372801900433 ) ) ;
#53364=CARTESIAN_POINT ( 'NONE',  ( -19.02544592524334988, -5.153800228976617603, 63.95942372801899012 ) ) ;
#53365=CARTESIAN_POINT ( 'NONE',  ( -0.05219959533937732626, 21.53943276465977519, 87.50109039468568994 ) ) ;
#53366=CARTESIAN_POINT ( 'NONE',  ( 5.153800228976615827, -19.02544592524334988, 55.20942372801899722 ) ) ;
#53367=CARTESIAN_POINT ( 'NONE',  ( 16.46253265017160672, -9.564922557960803928, 28.33224293864769550 ) ) ;
#53368=CARTESIAN_POINT ( 'NONE',  ( -18.62759615963270932, 10.81492255796079327, 60.83224293864769550 ) ) ;
#53369=CARTESIAN_POINT ( 'NONE',  ( 14.34966873604960469, 8.224510206698951720, 54.16557627198103120 ) ) ;
#53371=CARTESIAN_POINT ( 'NONE',  ( -9.564922557961040184, 16.46253265017147172, 32.91775706135233293 ) ) ;
#53372=CARTESIAN_POINT ( 'NONE',  ( -16.52544592524335698, -4.483927247898792601, 88.95942372801901854 ) ) ;
#53373=CARTESIAN_POINT ( 'NONE',  ( 8.314922557960818139, 14.29746914071049879, 44.58224293864769550 ) ) ;
#53374=CARTESIAN_POINT ( 'NONE',  ( 21.53943276465977519, 0.05219959533937863772, 76.25109039468568994 ) ) ;
#53375=CARTESIAN_POINT ( 'NONE',  ( -15.72974639402176322, -15.80617190586768395, 84.37609039468570415 ) ) ;
#53376=CARTESIAN_POINT ( 'NONE',  ( -15.72974639402197994, 15.80617190586746368, 75.62390960531439532 ) ) ;
#53377=CARTESIAN_POINT ( 'NONE',  ( -19.03943276465977164, 0.05219959533909376836, 36.24890960531436690 ) ) ;
#53378=CARTESIAN_POINT ( 'NONE',  ( 18.67979575497194134, -10.72451020669871369, 50.83442372801901143 ) ) ;
#53379=CARTESIAN_POINT ( 'NONE',  ( -19.03943276465977164, 0.05219959533909376836, 31.24890960531435979 ) ) ;
#53380=VERTEX_POINT ( 'NONE', #180911 ) ;
#53381=CARTESIAN_POINT ( 'NONE',  ( -19.03943276465977164, 0.05219959533909376836, 51.24890960531436690 ) ) ;
#53382=CARTESIAN_POINT ( 'NONE',  ( 0.05219959533910956823, 16.53943276465976808, 99.99890960531436690 ) ) ;
#53383=CARTESIAN_POINT ( 'NONE',  ( 13.89961937509977652, -13.97604488694527269, 103.1239096053143527 ) ) ;
#53384=CARTESIAN_POINT ( 'NONE',  ( 12.06949235617757843, -12.14591786802309237, 38.12390960531436690 ) ) ;
#53385=CARTESIAN_POINT ( 'NONE',  ( 9.474510206698971260, -16.51473224551069308, 22.91557627198102765 ) ) ;
#53386=CARTESIAN_POINT ( 'NONE',  ( 21.53943276465977519, -0.05219959533907433946, 88.74890960531436690 ) ) ;
#53387=CARTESIAN_POINT ( 'NONE',  ( 21.53943276465977519, 0.05219959533937863772, 26.25109039468567573 ) ) ;
#53389=CARTESIAN_POINT ( 'NONE',  ( 4.379528057220092307, 16.55341960407617563, 32.29275706135235424 ) ) ;
#53390=ORIENTED_EDGE ( 'NONE', *, *, #82839, .F. ) ;
#53391=CARTESIAN_POINT ( 'NONE',  ( -15.72974639402197994, 15.80617190586746368, 70.62390960531436690 ) ) ;
#53392=CARTESIAN_POINT ( 'NONE',  ( 15.80617190586769283, -15.72974639402175789, 90.62609039468567573 ) ) ;
#53393=CARTESIAN_POINT ( 'NONE',  ( 0.05219959533909260263, 19.03943276465977164, 94.99890960531436690 ) ) ;
#53394=CARTESIAN_POINT ( 'NONE',  ( 0.05219959533937995610, -21.53943276465977519, 25.00109039468567218 ) ) ;
#53395=CARTESIAN_POINT ( 'NONE',  ( -21.55341960407610458, -5.719274019375992779, 36.45724293864768839 ) ) ;
#53396=CARTESIAN_POINT ( 'NONE',  ( -16.52544592524335698, -4.483927247898792601, 93.95942372801903275 ) ) ;
#53397=CARTESIAN_POINT ( 'NONE',  ( 21.52544592524334988, 5.823673210054432836, 76.45942372801901854 ) ) ;
#53398=CARTESIAN_POINT ( 'NONE',  ( -5.049401038297874678, -19.05341960407617918, 19.79275706135233293 ) ) ;
#53399=CARTESIAN_POINT ( 'NONE',  ( 12.06949235617739724, 12.14591786802326823, 76.87609039468567573 ) ) ;
#53400=CARTESIAN_POINT ( 'NONE',  ( -5.823673210054431948, 21.52544592524334988, 22.70942372801901499 ) ) ;
#53401=CARTESIAN_POINT ( 'NONE',  ( -0.05219959533909027116, -19.03943276465977164, 37.49890960531436690 ) ) ;
#53402=CARTESIAN_POINT ( 'NONE',  ( -21.52544592524334988, -5.823673210054445271, 108.9594237280190185 ) ) ;
#53403=CARTESIAN_POINT ( 'NONE',  ( 5.049401038298161559, -19.05341960407611168, 102.7072429386476955 ) ) ;
#53404=CARTESIAN_POINT ( 'NONE',  ( -10.72451020669898014, 18.67979575497178502, 100.4155762719810241 ) ) ;
#53406=CARTESIAN_POINT ( 'NONE',  ( -5.823673210054116645, -21.52544592524344225, 62.29057627198102409 ) ) ;
#53407=CARTESIAN_POINT ( 'NONE',  ( 4.483927247898790824, -16.52544592524335698, 55.20942372801902565 ) ) ;
#53408=CARTESIAN_POINT ( 'NONE',  ( 14.29746914071049879, -8.314922557960816363, 48.33224293864770260 ) ) ;
#53409=CARTESIAN_POINT ( 'NONE',  ( -17.49999999999999645, -5.500000000000000888, 120.0000000000000142 ) ) ;
#53410=CARTESIAN_POINT ( 'NONE',  ( -9.564922557961040184, 16.46253265017147172, 77.91775706135234714 ) ) ;
#53411=CARTESIAN_POINT ( 'NONE',  ( -16.19135201231367205, 7.376712067591922661, 104.8131914594797252 ) ) ;
#53412=EDGE_CURVE ( 'NONE', #123381, #135811, #44941, .T. ) ;
#53413=CARTESIAN_POINT ( 'NONE',  ( 14.29746914071037800, 8.314922557961029526, 21.66775706135235069 ) ) ;
#53414=CARTESIAN_POINT ( 'NONE',  ( -21.55341960407610458, -5.719274019375992779, 81.45724293864769550 ) ) ;
#53415=CARTESIAN_POINT ( 'NONE',  ( -8.314922557960811034, -14.29746914071050412, 67.08224293864770971 ) ) ;
#53416=CARTESIAN_POINT ( 'NONE',  ( 16.51473224551069308, 9.474510206698969483, 99.16557627198102409 ) ) ;
#53417=CARTESIAN_POINT ( 'NONE',  ( -12.14591786802326823, 12.06949235617739902, 43.12609039468568284 ) ) ;
#53418=CARTESIAN_POINT ( 'NONE',  ( -19.02544592524342804, 5.153800228976336051, 61.04057627198103120 ) ) ;
#53419=CARTESIAN_POINT ( 'NONE',  ( -21.55341960407619339, 5.719274019375674811, 23.54275706135235424 ) ) ;
#53420=CARTESIAN_POINT ( 'NONE',  ( 5.049401038297881783, 19.05341960407617563, 102.2927570613523045 ) ) ;
#53421=CARTESIAN_POINT ( 'NONE',  ( 0.05219959533909260263, 19.03943276465977164, 99.99890960531436690 ) ) ;
#53422=CARTESIAN_POINT ( 'NONE',  ( 16.46253265017160672, -9.564922557960803928, 93.33224293864769550 ) ) ;
#53423=CARTESIAN_POINT ( 'NONE',  ( -10.81492255796078084, -18.62759615963271287, 87.08224293864769550 ) ) ;
#53424=CARTESIAN_POINT ( 'NONE',  ( -19.05341960407611168, -5.049401038298163336, 41.45724293864769550 ) ) ;
#53425=CARTESIAN_POINT ( 'NONE',  ( -16.18388926212241330, -7.379444403734409796, 60.43953151366154941 ) ) ;
#53426=CARTESIAN_POINT ( 'NONE',  ( -16.55341960407611168, -4.379528057220339221, 71.45724293864769550 ) ) ;
#53427=CARTESIAN_POINT ( 'NONE',  ( 19.03943276465977164, -0.05219959533909143690, 108.7489096053143527 ) ) ;
#53429=CARTESIAN_POINT ( 'NONE',  ( -5.049401038297874678, -19.05341960407617918, 74.79275706135231871 ) ) ;
#53431=CARTESIAN_POINT ( 'NONE',  ( 10.81492255796078972, 18.62759615963270932, 84.58224293864769550 ) ) ;
#53432=CARTESIAN_POINT ( 'NONE',  ( 5.153800228976615827, -19.02544592524334988, 55.20942372801899722 ) ) ;
#53433=CARTESIAN_POINT ( 'NONE',  ( -5.049401038298153566, 19.05341960407611168, 100.2072429386476955 ) ) ;
#53434=PRESENTATION_STYLE_ASSIGNMENT (( #5926 ) ) ;
#53435=CARTESIAN_POINT ( 'NONE',  ( -21.53943276465977519, 0.05219959533907696930, 41.24890960531435269 ) ) ;
#53436=CARTESIAN_POINT ( 'NONE',  ( 9.474510206698971260, -16.51473224551069308, 87.91557627198102409 ) ) ;
#53437=CARTESIAN_POINT ( 'NONE',  ( 10.72451020669871369, 18.67979575497193778, 67.08442372801901854 ) ) ;
#53438=CARTESIAN_POINT ( 'NONE',  ( -5.153800228976328057, -19.02544592524343514, 37.29057627198102409 ) ) ;
#53440=CARTESIAN_POINT ( 'NONE',  ( 4.379528057220339221, -16.55341960407611168, 72.70724293864769550 ) ) ;
#53441=CARTESIAN_POINT ( 'NONE',  ( 16.55341960407618274, -4.379528057220086978, 26.04275706135235779 ) ) ;
#53442=CARTESIAN_POINT ( 'NONE',  ( 15.80617190586769283, -15.72974639402175789, 55.62609039468568284 ) ) ;
#53443=VERTEX_POINT ( 'NONE', #94833 ) ;
#53444=CARTESIAN_POINT ( 'NONE',  ( -0.05219959533909027116, -19.03943276465977164, 107.4989096053143527 ) ) ;
#53445=CARTESIAN_POINT ( 'NONE',  ( -13.89961937509957401, -13.97604488694547875, 64.37609039468567573 ) ) ;
#53447=CARTESIAN_POINT ( 'NONE',  ( -15.80617190586768217, 15.72974639402176855, 23.12609039468567573 ) ) ;
#53449=CARTESIAN_POINT ( 'NONE',  ( -5.153800228976607833, 19.02544592524334988, 22.70942372801899012 ) ) ;
#53450=CARTESIAN_POINT ( 'NONE',  ( -16.51473224551069308, -9.474510206698971260, 61.66557627198103120 ) ) ;
#53451=CARTESIAN_POINT ( 'NONE',  ( 15.72974639402176855, 15.80617190586768217, 106.8760903946856899 ) ) ;
#53452=CARTESIAN_POINT ( 'NONE',  ( -16.52544592524335698, -4.483927247898792601, 103.9594237280190185 ) ) ;
#53453=CARTESIAN_POINT ( 'NONE',  ( -9.564922557960796823, -16.46253265017161027, 107.0822429386476955 ) ) ;
#53454=CARTESIAN_POINT ( 'NONE',  ( -5.823673210054431948, 21.52544592524334988, 77.70942372801900433 ) ) ;
#53456=CARTESIAN_POINT ( 'NONE',  ( 19.02544592524343514, -5.153800228976328945, 113.5405762719810241 ) ) ;
#53458=CARTESIAN_POINT ( 'NONE',  ( 12.06949235617739724, 12.14591786802326823, 61.87609039468568284 ) ) ;
#53459=CARTESIAN_POINT ( 'NONE',  ( 21.55341960407619695, -5.719274019375665929, 71.04275706135234714 ) ) ;
#53460=CARTESIAN_POINT ( 'NONE',  ( 10.72451020669871369, 18.67979575497193778, 102.0844237280190185 ) ) ;
#53462=CARTESIAN_POINT ( 'NONE',  ( -9.564922557960796823, -16.46253265017161027, 82.08224293864768129 ) ) ;
#53463=CARTESIAN_POINT ( 'NONE',  ( -19.02544592524342804, 5.153800228976336051, 116.0405762719810383 ) ) ;
#53464=DIRECTION ( 'NONE',  ( 0.000000000000000000, 0.000000000000000000, -1.000000000000000000 ) ) ;
#53465=CARTESIAN_POINT ( 'NONE',  ( 19.03943276465977164, -0.05219959533909143690, 33.74890960531435979 ) ) ;
#53466=CARTESIAN_POINT ( 'NONE',  ( 15.72974639402199770, -15.80617190586745480, 38.12390960531436690 ) ) ;
#53467=CARTESIAN_POINT ( 'NONE',  ( 4.483927247898790824, -16.52544592524335698, 100.2094237280190043 ) ) ;
#53468=CARTESIAN_POINT ( 'NONE',  ( -14.34966873604960291, -8.224510206698953496, 96.66557627198102409 ) ) ;
#53469=CARTESIAN_POINT ( 'NONE',  ( 16.51473224551069308, 9.474510206698969483, 79.16557627198103830 ) ) ;
#53470=CARTESIAN_POINT ( 'NONE',  ( -15.72974639402176322, -15.80617190586768395, 109.3760903946857042 ) ) ;
#53471=CARTESIAN_POINT ( 'NONE',  ( -19.05341960407611168, -5.049401038298163336, 36.45724293864766707 ) ) ;
#53472=CARTESIAN_POINT ( 'NONE',  ( 8.224510206698953496, -14.34966873604960469, 92.91557627198103830 ) ) ;
#53473=CARTESIAN_POINT ( 'NONE',  ( -21.53943276465977519, -0.05219959533937600094, 48.75109039468568284 ) ) ;
#53474=CARTESIAN_POINT ( 'NONE',  ( 21.52544592524344225, -5.823673210054117533, 88.54057627198103830 ) ) ;
#53475=CARTESIAN_POINT ( 'NONE',  ( 19.05341960407617918, -5.049401038297876454, 46.04275706135233293 ) ) ;
#53476=CARTESIAN_POINT ( 'NONE',  ( -13.97604488694527625, -13.89961937509977830, 46.87390960531435979 ) ) ;
#53477=CARTESIAN_POINT ( 'NONE',  ( -19.03943276465977164, 0.05219959533909376836, 91.24890960531436690 ) ) ;
#53478=CARTESIAN_POINT ( 'NONE',  ( -8.314922557960811034, -14.29746914071050412, 57.08224293864769550 ) ) ;
#53479=CARTESIAN_POINT ( 'NONE',  ( -0.05219959533936034679, 19.03943276465977164, 42.50109039468566152 ) ) ;
#53480=CARTESIAN_POINT ( 'NONE',  ( 8.224510206698953496, -14.34966873604960469, 42.91557627198103120 ) ) ;
#53481=CARTESIAN_POINT ( 'NONE',  ( -9.564922557961040184, 16.46253265017147172, 82.91775706135233293 ) ) ;
#53482=CARTESIAN_POINT ( 'NONE',  ( -18.22780087662123805, 5.499999999999981348, 86.01763182126894947 ) ) ;
#53483=CARTESIAN_POINT ( 'NONE',  ( -21.52544592524343514, 5.823673210054127303, 36.04057627198102409 ) ) ;
#53484=ADVANCED_FACE ( 'NONE', ( #110994 ), #124917, .T. ) ;
#53485=CARTESIAN_POINT ( 'NONE',  ( 12.14591786802309770, 12.06949235617756955, 99.37390960531436690 ) ) ;
#53487=CARTESIAN_POINT ( 'NONE',  ( 16.51473224551069308, 9.474510206698969483, 64.16557627198102409 ) ) ;
#53488=CARTESIAN_POINT ( 'NONE',  ( -5.719274019375978568, 21.55341960407610458, 55.20724293864770260 ) ) ;
#53489=CARTESIAN_POINT ( 'NONE',  ( -13.97604488694527625, -13.89961937509977652, 31.87390960531435979 ) ) ;
#53490=CARTESIAN_POINT ( 'NONE',  ( 8.314922557961029526, -14.29746914071037800, 75.41775706135233293 ) ) ;
#53491=CARTESIAN_POINT ( 'NONE',  ( 16.51473224551069308, 9.474510206698969483, 54.16557627198103120 ) ) ;
#53492=CARTESIAN_POINT ( 'NONE',  ( 5.153800228976615827, -19.02544592524334988, 45.20942372801901143 ) ) ;
#53493=CARTESIAN_POINT ( 'NONE',  ( -15.72974639402176322, -15.80617190586768395, 69.37609039468567573 ) ) ;
#53494=CARTESIAN_POINT ( 'NONE',  ( -21.55341960407610458, -5.719274019375992779, 56.45724293864768839 ) ) ;
#53495=CARTESIAN_POINT ( 'NONE',  ( 16.46253265017160672, -9.564922557960803928, 28.33224293864769550 ) ) ;
#53496=CARTESIAN_POINT ( 'NONE',  ( -16.51473224551082808, 9.474510206698731452, 103.3344237280190043 ) ) ;
#53498=CARTESIAN_POINT ( 'NONE',  ( 17.49999999999999645, 4.703611302595025911, 36.84949425462254169 ) ) ;
#53499=CARTESIAN_POINT ( 'NONE',  ( -15.80617190586745835, -15.72974639402198527, 41.87390960531435979 ) ) ;
#53500=CARTESIAN_POINT ( 'NONE',  ( -5.049401038298153566, 19.05341960407611168, 25.20724293864768484 ) ) ;
#53501=CARTESIAN_POINT ( 'NONE',  ( -10.81492255796105439, 18.62759615963255655, 77.91775706135231871 ) ) ;
#53502=CARTESIAN_POINT ( 'NONE',  ( 12.14591786802309770, 12.06949235617756955, 44.37390960531435979 ) ) ;
#53503=CARTESIAN_POINT ( 'NONE',  ( 12.06949235617757843, -12.14591786802309237, 63.12390960531435979 ) ) ;
#53504=CARTESIAN_POINT ( 'NONE',  ( 5.719274019375991003, -21.55341960407610458, 82.70724293864770971 ) ) ;
#53505=CARTESIAN_POINT ( 'NONE',  ( -18.67979575497178146, -10.72451020669898902, 81.66557627198103830 ) ) ;
#53507=CARTESIAN_POINT ( 'NONE',  ( -10.81492255796078084, -18.62759615963271287, 27.08224293864769550 ) ) ;
#53508=CARTESIAN_POINT ( 'NONE',  ( -16.53943276465976808, -0.05219959533934237506, 53.75109039468568994 ) ) ;
#53509=CARTESIAN_POINT ( 'NONE',  ( 4.379528057220339221, -16.55341960407611168, 77.70724293864770971 ) ) ;
#53510=CARTESIAN_POINT ( 'NONE',  ( 5.049401038298161559, -19.05341960407611168, 62.70724293864769550 ) ) ;
#53511=CARTESIAN_POINT ( 'NONE',  ( -19.05341960407611168, -5.049401038298163336, 26.45724293864769550 ) ) ;
#53512=CARTESIAN_POINT ( 'NONE',  ( 17.50000000000000000, -5.500000000000000000, 111.2176903769643559 ) ) ;
#53513=CARTESIAN_POINT ( 'NONE',  ( -12.14591786802326823, 12.06949235617739902, 78.12609039468570415 ) ) ;
#53514=CARTESIAN_POINT ( 'NONE',  ( 15.80617190586769283, -15.72974639402175789, 20.62609039468568639 ) ) ;
#53515=CARTESIAN_POINT ( 'NONE',  ( 9.564922557960805705, 16.46253265017160317, 84.58224293864769550 ) ) ;
#53516=CARTESIAN_POINT ( 'NONE',  ( -21.55341960407619339, 5.719274019375674811, 53.54275706135234714 ) ) ;
#53517=CARTESIAN_POINT ( 'NONE',  ( 5.153800228976335163, 19.02544592524342804, 109.7905762719810099 ) ) ;
#53520=CARTESIAN_POINT ( 'NONE',  ( 0.05219959533937995610, -21.53943276465977519, 45.00109039468568284 ) ) ;
#53521=CARTESIAN_POINT ( 'NONE',  ( 19.03943276465977164, -0.05219959533909143690, 38.74890960531436690 ) ) ;
#53522=CARTESIAN_POINT ( 'NONE',  ( 5.049401038298161559, -19.05341960407611168, 107.7072429386476955 ) ) ;
#53523=CARTESIAN_POINT ( 'NONE',  ( -5.049401038297874678, -19.05341960407617918, 59.79275706135231871 ) ) ;
#53524=CARTESIAN_POINT ( 'NONE',  ( -21.53943276465977519, -0.05219959533937600094, 18.75109039468568639 ) ) ;
#53525=CARTESIAN_POINT ( 'NONE',  ( 16.46253265017146816, 9.564922557961045513, 46.66775706135233293 ) ) ;
#53526=CARTESIAN_POINT ( 'NONE',  ( -16.51473224551069308, -9.474510206698971260, 31.66557627198102054 ) ) ;
#53527=CARTESIAN_POINT ( 'NONE',  ( -12.06949235617739369, -12.14591786802326823, 89.37609039468568994 ) ) ;
#53528=CARTESIAN_POINT ( 'NONE',  ( -5.049401038297874678, -19.05341960407617918, 64.79275706135233293 ) ) ;
#53529=CARTESIAN_POINT ( 'NONE',  ( 4.483927247898790824, -16.52544592524335698, 105.2094237280190328 ) ) ;
#53531=CARTESIAN_POINT ( 'NONE',  ( -5.153800228976328057, -19.02544592524343514, 92.29057627198099567 ) ) ;
#53533=CARTESIAN_POINT ( 'NONE',  ( 21.53943276465977519, 0.05219959533937863772, 91.25109039468568994 ) ) ;
#53534=CARTESIAN_POINT ( 'NONE',  ( -15.80617190586768217, 15.72974639402176855, 113.1260903946856899 ) ) ;
#53536=CARTESIAN_POINT ( 'NONE',  ( 19.02544592524343514, -5.153800228976328945, 103.5405762719809957 ) ) ;
#53537=CARTESIAN_POINT ( 'NONE',  ( 21.52544592524334988, 5.823673210054432836, 76.45942372801901854 ) ) ;
#53538=CARTESIAN_POINT ( 'NONE',  ( 0.05219959533936267826, -19.03943276465977164, 110.0010903946856757 ) ) ;
#53539=CARTESIAN_POINT ( 'NONE',  ( 5.049401038298161559, -19.05341960407611168, 77.70724293864765286 ) ) ;
#53540=CARTESIAN_POINT ( 'NONE',  ( -18.67979575497178146, -10.72451020669898902, 36.66557627198103120 ) ) ;
#53541=CARTESIAN_POINT ( 'NONE',  ( -13.89961937509977652, 13.97604488694528158, 95.62390960531436690 ) ) ;
#53543=CARTESIAN_POINT ( 'NONE',  ( -19.02544592524342804, 5.153800228976336051, 81.04057627198103830 ) ) ;
#53544=CARTESIAN_POINT ( 'NONE',  ( -13.97604488694527625, -13.89961937509977652, 61.87390960531435979 ) ) ;
#53545=CARTESIAN_POINT ( 'NONE',  ( -16.53943276465976808, -0.05219959533934237506, 98.75109039468568994 ) ) ;
#53547=CARTESIAN_POINT ( 'NONE',  ( -13.97604488694547697, 13.89961937509957934, 63.12609039468566152 ) ) ;
#53548=CARTESIAN_POINT ( 'NONE',  ( -9.564922557960796823, -16.46253265017161027, 97.08224293864769550 ) ) ;
#53549=CARTESIAN_POINT ( 'NONE',  ( 0.05219959533910956823, 16.53943276465976808, 79.99890960531435269 ) ) ;
#53550=CARTESIAN_POINT ( 'NONE',  ( 5.719274019375991003, -21.55341960407610458, 32.70724293864770260 ) ) ;
#53551=CARTESIAN_POINT ( 'NONE',  ( 16.46253265017160672, -9.564922557960803928, 113.3322429386476955 ) ) ;
#53552=CARTESIAN_POINT ( 'NONE',  ( -16.53943276465976808, 0.05219959533911058130, 86.24890960531436690 ) ) ;
#53554=CARTESIAN_POINT ( 'NONE',  ( -16.46253265017146816, -9.564922557961047289, 44.16775706135232582 ) ) ;
#53555=CARTESIAN_POINT ( 'NONE',  ( 8.314922557960818139, 14.29746914071049879, 29.58224293864769905 ) ) ;
#53557=CARTESIAN_POINT ( 'NONE',  ( 9.474510206698971260, -16.51473224551069308, 107.9155762719810383 ) ) ;
#53558=CARTESIAN_POINT ( 'NONE',  ( 0.05219959533937995610, -21.53943276465977519, 70.00109039468568994 ) ) ;
#53559=CARTESIAN_POINT ( 'NONE',  ( 21.52544592524344225, -5.823673210054117533, 58.54057627198103120 ) ) ;
#53560=CARTESIAN_POINT ( 'NONE',  ( 10.72451020669871369, 18.67979575497193778, 32.08442372801901854 ) ) ;
#53561=CARTESIAN_POINT ( 'NONE',  ( -10.72451020669898014, 18.67979575497178502, 85.41557627198102409 ) ) ;
#53562=CARTESIAN_POINT ( 'NONE',  ( -21.53943276465977519, -0.05219959533937600094, 38.75109039468567573 ) ) ;
#53563=CARTESIAN_POINT ( 'NONE',  ( 12.06949235617757843, -12.14591786802309237, 108.1239096053143811 ) ) ;
#53564=CARTESIAN_POINT ( 'NONE',  ( -9.564922557961040184, 16.46253265017147172, 67.91775706135233293 ) ) ;
#53565=CARTESIAN_POINT ( 'NONE',  ( -9.564922557960796823, -16.46253265017161027, 47.08224293864769550 ) ) ;
#53566=CARTESIAN_POINT ( 'NONE',  ( 8.314922557960818139, 14.29746914071049879, 94.58224293864769550 ) ) ;
#53567=CARTESIAN_POINT ( 'NONE',  ( -19.05341960407611168, -5.049401038298163336, 96.45724293864769550 ) ) ;
#53568=CARTESIAN_POINT ( 'NONE',  ( -16.51473224551069308, -9.474510206698971260, 96.66557627198102409 ) ) ;
#53569=CARTESIAN_POINT ( 'NONE',  ( -14.29746914071049879, 8.314922557960819915, 110.8322429386476955 ) ) ;
#53571=CARTESIAN_POINT ( 'NONE',  ( -16.55341960407611168, -4.379528057220339221, 41.45724293864769550 ) ) ;
#53572=CARTESIAN_POINT ( 'NONE',  ( 16.52544592524335698, 4.483927247898782831, 106.4594237280190328 ) ) ;
#53573=CARTESIAN_POINT ( 'NONE',  ( 19.02544592524343514, -5.153800228976328945, 58.54057627198102409 ) ) ;
#53574=CARTESIAN_POINT ( 'NONE',  ( -9.564922557960796823, -16.46253265017161027, 22.08224293864768839 ) ) ;
#53575=CARTESIAN_POINT ( 'NONE',  ( 9.474510206698729675, 16.51473224551082808, 27.08442372801900433 ) ) ;
#53576=CARTESIAN_POINT ( 'NONE',  ( 9.564922557960805705, 16.46253265017160317, 109.5822429386476955 ) ) ;
#53577=CARTESIAN_POINT ( 'NONE',  ( 0.05219959533934541429, -16.53943276465976808, 110.0010903946856757 ) ) ;
#53578=CARTESIAN_POINT ( 'NONE',  ( -10.81492255796105439, 18.62759615963255655, 42.91775706135235424 ) ) ;
#53579=CARTESIAN_POINT ( 'NONE',  ( -13.97604488694527625, -13.89961937509977652, 101.8739096053143811 ) ) ;
#53580=CARTESIAN_POINT ( 'NONE',  ( -12.06949235617739369, -12.14591786802326823, 44.37609039468567573 ) ) ;
#53581=CARTESIAN_POINT ( 'NONE',  ( -4.483927247898782831, 16.52544592524335698, 107.7094237280190328 ) ) ;
#53582=CARTESIAN_POINT ( 'NONE',  ( 19.05341960407611168, 5.049401038298154454, 48.95724293864768129 ) ) ;
#53583=CARTESIAN_POINT ( 'NONE',  ( -4.483927247898782831, 16.52544592524335698, 92.70942372801901854 ) ) ;
#53584=CARTESIAN_POINT ( 'NONE',  ( 16.53943276465976808, 0.05219959533934440121, 31.25109039468568639 ) ) ;
#53585=EDGE_CURVE ( 'NONE', #189743, #20330, #163106, .T. ) ;
#53586=CARTESIAN_POINT ( 'NONE',  ( -19.03943276465977164, 0.05219959533909376836, 51.24890960531436690 ) ) ;
#53587=CARTESIAN_POINT ( 'NONE',  ( 14.29746914071049879, -8.314922557960816363, 113.3322429386476955 ) ) ;
#53588=CARTESIAN_POINT ( 'NONE',  ( 10.81492255796106328, -18.62759615963255655, 25.41775706135235779 ) ) ;
#53589=CARTESIAN_POINT ( 'NONE',  ( 16.46253265017160672, -9.564922557960803928, 38.33224293864768839 ) ) ;
#53590=CARTESIAN_POINT ( 'NONE',  ( -13.97604488694527625, -13.89961937509977652, 101.8739096053143811 ) ) ;
#53591=CARTESIAN_POINT ( 'NONE',  ( 16.51473224551069308, 9.474510206698969483, 34.16557627198102409 ) ) ;
#53592=CARTESIAN_POINT ( 'NONE',  ( 19.05341960407611168, 5.049401038298154454, 103.9572429386476671 ) ) ;
#53594=CARTESIAN_POINT ( 'NONE',  ( 19.02544592524343514, -5.153800228976328945, 103.5405762719809957 ) ) ;
#53595=CARTESIAN_POINT ( 'NONE',  ( 18.62759615963255655, 10.81492255796105972, 46.66775706135234714 ) ) ;
#53596=CARTESIAN_POINT ( 'NONE',  ( -0.05219959533910754901, -16.53943276465976808, 102.4989096053143811 ) ) ;
#53597=CARTESIAN_POINT ( 'NONE',  ( 9.474510206698971260, -16.51473224551069308, 112.9155762719810383 ) ) ;
#53598=CARTESIAN_POINT ( 'NONE',  ( 13.97604488694548053, -13.89961937509957401, 70.62609039468567573 ) ) ;
#53599=CARTESIAN_POINT ( 'NONE',  ( -16.55341960407617563, 4.379528057220093196, 58.54275706135235424 ) ) ;
#53600=CARTESIAN_POINT ( 'NONE',  ( 18.67979575497194134, -10.72451020669871369, 95.83442372801903275 ) ) ;
#53601=CARTESIAN_POINT ( 'NONE',  ( 16.53943276465976808, 0.05219959533934440121, 41.25109039468568284 ) ) ;
#53602=CARTESIAN_POINT ( 'NONE',  ( 16.46253265017160672, -9.564922557960803928, 88.33224293864769550 ) ) ;
#53603=CARTESIAN_POINT ( 'NONE',  ( 16.53943276465976808, 0.05219959533934440121, 31.25109039468568639 ) ) ;
#53604=CARTESIAN_POINT ( 'NONE',  ( -5.049401038297874678, -19.05341960407617918, 104.7927570613523471 ) ) ;
#53605=CARTESIAN_POINT ( 'NONE',  ( -12.14591786802326823, 12.06949235617739902, 78.12609039468570415 ) ) ;
#53606=CARTESIAN_POINT ( 'NONE',  ( 13.97604488694548053, -13.89961937509957401, 90.62609039468567573 ) ) ;
#53607=CARTESIAN_POINT ( 'NONE',  ( 16.46253265017160672, -9.564922557960803928, 73.33224293864769550 ) ) ;
#53608=CARTESIAN_POINT ( 'NONE',  ( -5.719274019375978568, 21.55341960407610458, 100.2072429386476955 ) ) ;
#53609=CARTESIAN_POINT ( 'NONE',  ( 8.224510206698953496, -14.34966873604960469, 92.91557627198103830 ) ) ;
#53610=CARTESIAN_POINT ( 'NONE',  ( 19.05341960407617918, -5.049401038297876454, 86.04275706135233293 ) ) ;
#53611=CARTESIAN_POINT ( 'NONE',  ( -14.34966873604972548, 8.224510206698743886, 78.33442372801901854 ) ) ;
#53613=CARTESIAN_POINT ( 'NONE',  ( -9.564922557961040184, 16.46253265017147172, 72.91775706135233293 ) ) ;
#53614=CARTESIAN_POINT ( 'NONE',  ( 8.224510206698953496, -14.34966873604960469, 32.91557627198102409 ) ) ;
#53615=CARTESIAN_POINT ( 'NONE',  ( -4.379528057220328563, 16.55341960407611168, 100.2072429386476955 ) ) ;
#53616=CARTESIAN_POINT ( 'NONE',  ( 5.049401038297881783, 19.05341960407617563, 32.29275706135233293 ) ) ;
#53617=CARTESIAN_POINT ( 'NONE',  ( -13.89961937509957401, -13.97604488694547697, 44.37609039468566863 ) ) ;
#53618=CARTESIAN_POINT ( 'NONE',  ( 5.719274019375673035, 21.55341960407619339, 27.29275706135234358 ) ) ;
#53620=CARTESIAN_POINT ( 'NONE',  ( -9.564922557960796823, -16.46253265017161027, 72.08224293864770971 ) ) ;
#53621=CARTESIAN_POINT ( 'NONE',  ( 5.823673210054444382, -21.52544592524334988, 95.20942372801903275 ) ) ;
#53622=CARTESIAN_POINT ( 'NONE',  ( -16.51473224551069308, -9.474510206698971260, 76.66557627198103830 ) ) ;
#53623=CARTESIAN_POINT ( 'NONE',  ( -10.81492255796078084, -18.62759615963271287, 47.08224293864770260 ) ) ;
#53624=CARTESIAN_POINT ( 'NONE',  ( 16.55341960407611168, 4.379528057220329451, 73.95724293864769550 ) ) ;
#53625=CARTESIAN_POINT ( 'NONE',  ( 5.153800228976335163, 19.02544592524342804, 54.79057627198103120 ) ) ;
#53627=CARTESIAN_POINT ( 'NONE',  ( -14.34966873604960291, -8.224510206698953496, 111.6655762719810525 ) ) ;
#53628=CARTESIAN_POINT ( 'NONE',  ( 21.52544592524334988, 5.823673210054432836, 21.45942372801901499 ) ) ;
#53629=CARTESIAN_POINT ( 'NONE',  ( 21.55341960407619695, -5.719274019375665929, 66.04275706135236135 ) ) ;
#53630=CARTESIAN_POINT ( 'NONE',  ( -9.564922557960796823, -16.46253265017161027, 47.08224293864769550 ) ) ;
#53631=CARTESIAN_POINT ( 'NONE',  ( 16.55341960407618274, -4.379528057220086978, 76.04275706135237556 ) ) ;
#53632=CARTESIAN_POINT ( 'NONE',  ( 5.823673210054125526, 21.52544592524343514, 114.7905762719810383 ) ) ;
#53633=EDGE_LOOP ( 'NONE', ( #58742, #73803 ) ) ;
#53634=CARTESIAN_POINT ( 'NONE',  ( -21.52544592524334988, -5.823673210054445271, 18.95942372801901143 ) ) ;
#53635=CARTESIAN_POINT ( 'NONE',  ( 5.153800228976615827, -19.02544592524334988, 35.20942372801899722 ) ) ;
#53636=CARTESIAN_POINT ( 'NONE',  ( 9.564922557960805705, 16.46253265017160317, 64.58224293864769550 ) ) ;
#53637=CARTESIAN_POINT ( 'NONE',  ( 16.51473224551083163, -9.474510206698727899, 30.83442372801900433 ) ) ;
#53638=CARTESIAN_POINT ( 'NONE',  ( 0.05219959533937995610, -21.53943276465977519, 70.00109039468568994 ) ) ;
#53639=CARTESIAN_POINT ( 'NONE',  ( 15.80617190586746368, 15.72974639402197994, 69.37390960531436690 ) ) ;
#53640=CARTESIAN_POINT ( 'NONE',  ( -4.379528057220328563, 16.55341960407611168, 40.20724293864769550 ) ) ;
#53641=CARTESIAN_POINT ( 'NONE',  ( -21.52544592524334988, -5.823673210054445271, 83.95942372801900433 ) ) ;
#53642=CARTESIAN_POINT ( 'NONE',  ( -19.03943276465977164, -0.05219959533935918106, 28.75109039468566507 ) ) ;
#53643=CARTESIAN_POINT ( 'NONE',  ( 4.483927247898545687, 16.52544592524342804, 64.79057627198103830 ) ) ;
#53644=CARTESIAN_POINT ( 'NONE',  ( -8.224510206698948167, 14.34966873604960824, 110.4155762719810383 ) ) ;
#53645=CARTESIAN_POINT ( 'NONE',  ( 19.05341960407617918, -5.049401038297876454, 61.04275706135232582 ) ) ;
#53646=CARTESIAN_POINT ( 'NONE',  ( -16.55341960407617563, 4.379528057220093196, 108.5427570613523756 ) ) ;
#53647=CARTESIAN_POINT ( 'NONE',  ( 21.52544592524334988, 5.823673210054432836, 66.45942372801903275 ) ) ;
#53648=CARTESIAN_POINT ( 'NONE',  ( -5.049401038298153566, 19.05341960407611168, 75.20724293864769550 ) ) ;
#53649=CARTESIAN_POINT ( 'NONE',  ( 13.89961937509957401, 13.97604488694547697, 41.87609039468566152 ) ) ;
#53650=CARTESIAN_POINT ( 'NONE',  ( -15.80617190586745835, -15.72974639402198527, 51.87390960531437401 ) ) ;
#53651=B_SPLINE_CURVE_WITH_KNOTS ( 'NONE', 3,
 ( #90615, #76441, #93589, #152297, #13781, #185617, #140088, #199799, #171443, #141092, #1580, #122936, #578, #155275 ),
 .UNSPECIFIED., .F., .F.,
 ( 4, 2, 2, 2, 2, 2, 4 ),
 ( 0.000000000000000000, 0.0003275753061460234968, 0.0006551506122920469936, 0.0009827259184380704362, 0.001310301224584093987, 0.001965451836876139138, 0.002620602449168184505 ),
 .UNSPECIFIED. ) ;
#53652=CARTESIAN_POINT ( 'NONE',  ( 18.67979575497194134, -10.72451020669871369, 50.83442372801901143 ) ) ;
#53653=CARTESIAN_POINT ( 'NONE',  ( 10.81492255796078972, 18.62759615963270932, 104.5822429386477097 ) ) ;
#53654=CARTESIAN_POINT ( 'NONE',  ( -5.049401038297874678, -19.05341960407617918, 99.79275706135234714 ) ) ;
#53655=CARTESIAN_POINT ( 'NONE',  ( -16.52544592524335698, -4.483927247898792601, 68.95942372801901854 ) ) ;
#53657=CARTESIAN_POINT ( 'NONE',  ( 5.823673210054125526, 21.52544592524343514, 109.7905762719810383 ) ) ;
#53658=CARTESIAN_POINT ( 'NONE',  ( 12.06949235617757843, -12.14591786802309237, 93.12390960531436690 ) ) ;
#53659=CARTESIAN_POINT ( 'NONE',  ( -17.49999999999999645, -3.565345528327900304, 30.57505513193525815 ) ) ;
#53660=CARTESIAN_POINT ( 'NONE',  ( -16.53943276465976808, -0.05219959533934237506, 28.75109039468567929 ) ) ;
#53661=CARTESIAN_POINT ( 'NONE',  ( 0.05219959533907565091, 21.53943276465977519, 44.99890960531435979 ) ) ;
#53662=CARTESIAN_POINT ( 'NONE',  ( 14.29746914071037800, 8.314922557961029526, 96.66775706135234714 ) ) ;
#53664=CARTESIAN_POINT ( 'NONE',  ( -12.14591786802326823, 12.06949235617739902, 68.12609039468567573 ) ) ;
#53665=CARTESIAN_POINT ( 'NONE',  ( 21.55341960407619695, -5.719274019375665929, 36.04275706135234714 ) ) ;
#53666=CARTESIAN_POINT ( 'NONE',  ( -10.72451020669898014, 18.67979575497178502, 40.41557627198103120 ) ) ;
#53667=CARTESIAN_POINT ( 'NONE',  ( -12.06949235617739369, -12.14591786802326823, 79.37609039468567573 ) ) ;
#53668=CARTESIAN_POINT ( 'NONE',  ( 16.51473224551069308, 9.474510206698969483, 104.1655762719810241 ) ) ;
#53669=CARTESIAN_POINT ( 'NONE',  ( 21.53943276465977519, 0.05219959533937863772, 66.25109039468567573 ) ) ;
#53670=CARTESIAN_POINT ( 'NONE',  ( -10.72451020669898014, 18.67979575497178502, 35.41557627198102409 ) ) ;
#53671=CARTESIAN_POINT ( 'NONE',  ( -18.62759615963270932, 10.81492255796079327, 40.83224293864769550 ) ) ;
#53672=VERTEX_POINT ( 'NONE', #113608 ) ;
#53673=CARTESIAN_POINT ( 'NONE',  ( -0.05219959533936034679, 19.03943276465977164, 52.50109039468566863 ) ) ;
#53674=CARTESIAN_POINT ( 'NONE',  ( -0.05219959533934338120, 16.53943276465976808, 62.50109039468568284 ) ) ;
#53675=CARTESIAN_POINT ( 'NONE',  ( 15.72974639402199770, -15.80617190586745480, 33.12390960531435979 ) ) ;
#53677=EDGE_CURVE ( 'NONE', #10027, #139245, #79305, .T. ) ;
#53678=CARTESIAN_POINT ( 'NONE',  ( -19.03943276465977164, 0.05219959533909376836, 86.24890960531436690 ) ) ;
#53679=CARTESIAN_POINT ( 'NONE',  ( -14.29746914071049879, 8.314922557960819915, 25.83224293864769194 ) ) ;
#53681=CARTESIAN_POINT ( 'NONE',  ( -12.14591786802309592, -12.06949235617757132, 111.8739096053143669 ) ) ;
#53682=CARTESIAN_POINT ( 'NONE',  ( 21.52544592524344225, -5.823673210054117533, 48.54057627198103120 ) ) ;
#53683=CARTESIAN_POINT ( 'NONE',  ( -16.51473224551069308, -9.474510206698971260, 46.66557627198102409 ) ) ;
#53684=CARTESIAN_POINT ( 'NONE',  ( 8.224510206698742110, 14.34966873604972548, 87.08442372801901854 ) ) ;
#53685=CARTESIAN_POINT ( 'NONE',  ( 21.53943276465977519, 0.05219959533937863772, 31.25109039468568639 ) ) ;
#53686=CARTESIAN_POINT ( 'NONE',  ( 5.049401038297881783, 19.05341960407617563, 92.29275706135234714 ) ) ;
#53687=CARTESIAN_POINT ( 'NONE',  ( -8.224510206698948167, 14.34966873604960824, 90.41557627198103830 ) ) ;
#53688=CARTESIAN_POINT ( 'NONE',  ( 19.05341960407611168, 5.049401038298154454, 53.95724293864770260 ) ) ;
#53689=CARTESIAN_POINT ( 'NONE',  ( 19.02544592524343514, -5.153800228976328945, 28.54057627198102409 ) ) ;
#53690=CARTESIAN_POINT ( 'NONE',  ( -21.55341960407619339, 5.719274019375674811, 108.5427570613523756 ) ) ;
#53691=CARTESIAN_POINT ( 'NONE',  ( -9.564922557960796823, -16.46253265017161027, 82.08224293864768129 ) ) ;
#53693=CARTESIAN_POINT ( 'NONE',  ( -8.224510206698735004, -14.34966873604973081, 64.58442372801900433 ) ) ;
#53694=CARTESIAN_POINT ( 'NONE',  ( -5.719274019375665041, -21.55341960407619695, 94.79275706135234714 ) ) ;
#53695=CARTESIAN_POINT ( 'NONE',  ( -18.67979575497178146, -10.72451020669898902, 46.66557627198102409 ) ) ;
#53696=CARTESIAN_POINT ( 'NONE',  ( -12.06949235617739369, -12.14591786802326823, 69.37609039468567573 ) ) ;
#53697=CARTESIAN_POINT ( 'NONE',  ( 19.02544592524334988, 5.153800228976608722, 46.45942372801899012 ) ) ;
#53698=CARTESIAN_POINT ( 'NONE',  ( -13.97604488694547697, 13.89961937509957934, 68.12609039468563310 ) ) ;
#53699=VERTEX_POINT ( 'NONE', #142951 ) ;
#53700=CARTESIAN_POINT ( 'NONE',  ( -21.52544592524334988, -5.823673210054445271, 63.95942372801901854 ) ) ;
#53701=CARTESIAN_POINT ( 'NONE',  ( -19.03943276465977164, 0.05219959533909376836, 66.24890960531436690 ) ) ;
#53702=CARTESIAN_POINT ( 'NONE',  ( -9.474510206698964154, 16.51473224551069663, 30.41557627198102054 ) ) ;
#53703=CARTESIAN_POINT ( 'NONE',  ( 5.153800228976615827, -19.02544592524334988, 55.20942372801899722 ) ) ;
#53704=CARTESIAN_POINT ( 'NONE',  ( 5.049401038298161559, -19.05341960407611168, 107.7072429386476955 ) ) ;
#53705=CARTESIAN_POINT ( 'NONE',  ( -19.03943276465977164, 0.05219959533909376836, 96.24890960531436690 ) ) ;
#53706=CARTESIAN_POINT ( 'NONE',  ( -16.55341960407611168, -4.379528057220339221, 51.45724293864770260 ) ) ;
#53707=CARTESIAN_POINT ( 'NONE',  ( 18.62759615963271287, -10.81492255796078972, 43.33224293864769550 ) ) ;
#53709=CARTESIAN_POINT ( 'NONE',  ( 16.46253265017146816, 9.564922557961045513, 21.66775706135233648 ) ) ;
#53711=CARTESIAN_POINT ( 'NONE',  ( 9.474510206698971260, -16.51473224551069308, 47.91557627198102409 ) ) ;
#53714=CARTESIAN_POINT ( 'NONE',  ( 14.29746914071037800, 8.314922557961029526, 76.66775706135234714 ) ) ;
#53715=CARTESIAN_POINT ( 'NONE',  ( 21.55341960407610458, 5.719274019375980345, 98.95724293864770971 ) ) ;
#53716=CARTESIAN_POINT ( 'NONE',  ( -0.05219959533910754901, -16.53943276465976808, 47.49890960531435979 ) ) ;
#53717=CARTESIAN_POINT ( 'NONE',  ( -13.89961937509977652, 13.97604488694528158, 40.62390960531435979 ) ) ;
#53719=CARTESIAN_POINT ( 'NONE',  ( -15.72974639402176322, -15.80617190586768395, 34.37609039468568284 ) ) ;
#53720=CARTESIAN_POINT ( 'NONE',  ( 5.153800228976615827, -19.02544592524334988, 55.20942372801899722 ) ) ;
#53721=CARTESIAN_POINT ( 'NONE',  ( 5.049401038298161559, -19.05341960407611168, 37.70724293864768839 ) ) ;
#53722=CARTESIAN_POINT ( 'NONE',  ( -18.67979575497193778, 10.72451020669871902, 93.33442372801901854 ) ) ;
#53725=CARTESIAN_POINT ( 'NONE',  ( -12.06949235617756955, 12.14591786802309770, 45.62390960531436690 ) ) ;
#53726=CARTESIAN_POINT ( 'NONE',  ( 18.56101223717332971, 5.499999999999940492, 43.94978406935678095 ) ) ;
#53727=CARTESIAN_POINT ( 'NONE',  ( -18.62759615963270932, 10.81492255796079327, 35.83224293864768839 ) ) ;
#53730=CARTESIAN_POINT ( 'NONE',  ( -13.89961937509977652, 13.97604488694528158, 100.6239096053143669 ) ) ;
#53731=CARTESIAN_POINT ( 'NONE',  ( 16.55341960407611168, 4.379528057220329451, 83.95724293864770971 ) ) ;
#53732=CARTESIAN_POINT ( 'NONE',  ( -0.05219959533934338120, 16.53943276465976808, 27.50109039468567929 ) ) ;
#53733=CARTESIAN_POINT ( 'NONE',  ( 12.14591786802327356, -12.06949235617739191, 110.6260903946857042 ) ) ;
#53734=ORIENTED_EDGE ( 'NONE', *, *, #72299, .F. ) ;
#53735=CARTESIAN_POINT ( 'NONE',  ( 9.474510206698971260, -16.51473224551069308, 92.91557627198103830 ) ) ;
#53737=CARTESIAN_POINT ( 'NONE',  ( 15.72974639402199770, -15.80617190586745480, 98.12390960531436690 ) ) ;
#53738=CARTESIAN_POINT ( 'NONE',  ( 4.483927247898545687, 16.52544592524342804, 29.79057627198102409 ) ) ;
#53739=CARTESIAN_POINT ( 'NONE',  ( -9.564922557960796823, -16.46253265017161027, 97.08224293864769550 ) ) ;
#53740=CARTESIAN_POINT ( 'NONE',  ( 9.564922557961047289, -16.46253265017146816, 75.41775706135234714 ) ) ;
#53741=CARTESIAN_POINT ( 'NONE',  ( 0.05219959533937995610, -21.53943276465977519, 110.0010903946856757 ) ) ;
#53742=CARTESIAN_POINT ( 'NONE',  ( -21.52544592524343514, 5.823673210054127303, 96.04057627198102409 ) ) ;
#53743=CARTESIAN_POINT ( 'NONE',  ( 21.52544592524344225, -5.823673210054117533, 38.54057627198103120 ) ) ;
#53744=CARTESIAN_POINT ( 'NONE',  ( 19.05341960407611168, 5.049401038298154454, 63.95724293864769550 ) ) ;
#53745=CARTESIAN_POINT ( 'NONE',  ( 14.34966873604960469, 8.224510206698951720, 39.16557627198102409 ) ) ;
#53746=CARTESIAN_POINT ( 'NONE',  ( -13.97604488694527625, -13.89961937509977652, 81.87390960531436690 ) ) ;
#53747=ORIENTED_EDGE ( 'NONE', *, *, #12204, .F. ) ;
#53749=CARTESIAN_POINT ( 'NONE',  ( 19.05341960407617918, -5.049401038297876454, 31.04275706135232227 ) ) ;
#53750=CARTESIAN_POINT ( 'NONE',  ( 14.34966873604960469, 8.224510206698951720, 89.16557627198102409 ) ) ;
#53751=CARTESIAN_POINT ( 'NONE',  ( 15.80617190586769283, -15.72974639402175789, 20.62609039468568639 ) ) ;
#53753=CARTESIAN_POINT ( 'NONE',  ( 12.06949235617739724, 12.14591786802326823, 91.87609039468568994 ) ) ;
#53754=CARTESIAN_POINT ( 'NONE',  ( -14.34966873604960291, -8.224510206698953496, 111.6655762719810525 ) ) ;
#53755=CARTESIAN_POINT ( 'NONE',  ( -13.97604488694527625, -13.89961937509977652, 71.87390960531433848 ) ) ;
#53757=CARTESIAN_POINT ( 'NONE',  ( 12.14591786802309770, 12.06949235617756955, 34.37390960531435979 ) ) ;
#53758=CARTESIAN_POINT ( 'NONE',  ( 15.72974639402176855, 15.80617190586768217, 61.87609039468568284 ) ) ;
#53760=CARTESIAN_POINT ( 'NONE',  ( -18.62759615963255300, -10.81492255796106328, 94.16775706135237556 ) ) ;
#53761=CARTESIAN_POINT ( 'NONE',  ( 9.564922557960805705, 16.46253265017160317, 39.58224293864768839 ) ) ;
#53762=CARTESIAN_POINT ( 'NONE',  ( -0.05219959533909027116, -19.03943276465977164, 57.49890960531435979 ) ) ;
#53764=CARTESIAN_POINT ( 'NONE',  ( 0.05219959533937995610, -21.53943276465977519, 95.00109039468568994 ) ) ;
#53765=CARTESIAN_POINT ( 'NONE',  ( 0.05219959533934541429, -16.53943276465976808, 65.00109039468568994 ) ) ;
#53766=CARTESIAN_POINT ( 'NONE',  ( 21.52544592524334988, 5.823673210054432836, 81.45942372801900433 ) ) ;
#53767=CARTESIAN_POINT ( 'NONE',  ( 9.474510206698971260, -16.51473224551069308, 112.9155762719810383 ) ) ;
#53768=CARTESIAN_POINT ( 'NONE',  ( -5.153800228976607833, 19.02544592524334988, 87.70942372801897591 ) ) ;
#53769=CARTESIAN_POINT ( 'NONE',  ( 18.62759615963255655, 10.81492255796105972, 71.66775706135234714 ) ) ;
#53770=CARTESIAN_POINT ( 'NONE',  ( 14.29746914071037800, 8.314922557961029526, 41.66775706135235424 ) ) ;
#53771=CARTESIAN_POINT ( 'NONE',  ( 10.81492255796078972, 18.62759615963270932, 89.58224293864768129 ) ) ;
#53772=CARTESIAN_POINT ( 'NONE',  ( 0.05219959533936267826, -19.03943276465977164, 90.00109039468567573 ) ) ;
#53773=CARTESIAN_POINT ( 'NONE',  ( 19.05341960407611168, 5.049401038298154454, 63.95724293864769550 ) ) ;
#53774=CARTESIAN_POINT ( 'NONE',  ( -9.564922557961040184, 16.46253265017147172, 102.9177570613523329 ) ) ;
#53775=CARTESIAN_POINT ( 'NONE',  ( -9.474510206698720793, -16.51473224551083518, 104.5844237280190043 ) ) ;
#53776=CARTESIAN_POINT ( 'NONE',  ( 14.34966873604960469, 8.224510206698951720, 49.16557627198102409 ) ) ;
#53777=CARTESIAN_POINT ( 'NONE',  ( 13.89961937509957401, 13.97604488694547697, 81.87609039468564731 ) ) ;
#53778=CARTESIAN_POINT ( 'NONE',  ( 14.34966873604972726, -8.224510206698740333, 55.83442372801901854 ) ) ;
#53779=CARTESIAN_POINT ( 'NONE',  ( 13.89961937509977652, -13.97604488694527269, 33.12390960531434558 ) ) ;
#53780=CARTESIAN_POINT ( 'NONE',  ( 13.97604488694527802, 13.89961937509977652, 54.37390960531435979 ) ) ;
#53781=CARTESIAN_POINT ( 'NONE',  ( -8.224510206698735004, -14.34966873604973081, 54.58442372801901143 ) ) ;
#53784=CARTESIAN_POINT ( 'NONE',  ( 5.049401038298161559, -19.05341960407611168, 107.7072429386476955 ) ) ;
#53786=CARTESIAN_POINT ( 'NONE',  ( 19.02544592524343514, -5.153800228976328945, 23.54057627198102054 ) ) ;
#53787=EDGE_LOOP ( 'NONE', ( #181125, #148460 ) ) ;
#53788=CARTESIAN_POINT ( 'NONE',  ( -4.483927247898782831, 16.52544592524335698, 22.70942372801901499 ) ) ;
#53789=CARTESIAN_POINT ( 'NONE',  ( 10.72451020669898902, -18.67979575497178502, 32.91557627198102409 ) ) ;
#53790=CARTESIAN_POINT ( 'NONE',  ( -9.474510206698720793, -16.51473224551083518, 34.58442372801899722 ) ) ;
#53791=CARTESIAN_POINT ( 'NONE',  ( 8.314922557961029526, -14.29746914071037800, 25.41775706135235779 ) ) ;
#53792=CARTESIAN_POINT ( 'NONE',  ( 5.153800228976335163, 19.02544592524342804, 29.79057627198102409 ) ) ;
#53793=CARTESIAN_POINT ( 'NONE',  ( 13.97604488694527802, 13.89961937509977652, 54.37390960531435979 ) ) ;
#53794=CARTESIAN_POINT ( 'NONE',  ( 5.719274019375991003, -21.55341960407610458, 72.70724293864769550 ) ) ;
#53795=CARTESIAN_POINT ( 'NONE',  ( -19.03943276465977164, 0.05219959533909376836, 96.24890960531436690 ) ) ;
#53796=CARTESIAN_POINT ( 'NONE',  ( -5.049401038298153566, 19.05341960407611168, 35.20724293864768839 ) ) ;
#53798=CARTESIAN_POINT ( 'NONE',  ( 9.564922557961047289, -16.46253265017146816, 85.41775706135233293 ) ) ;
#53799=CARTESIAN_POINT ( 'NONE',  ( -14.29746914071049879, 8.314922557960819915, 65.83224293864769550 ) ) ;
#53800=CARTESIAN_POINT ( 'NONE',  ( -15.72974639402197994, 15.80617190586746368, 45.62390960531436690 ) ) ;
#53801=CARTESIAN_POINT ( 'NONE',  ( -10.81492255796105439, 18.62759615963255655, 112.9177570613523329 ) ) ;
#53803=CARTESIAN_POINT ( 'NONE',  ( 5.719274019375991003, -21.55341960407610458, 97.70724293864772392 ) ) ;
#53804=CARTESIAN_POINT ( 'NONE',  ( 18.67979575497194134, -10.72451020669871369, 70.83442372801901854 ) ) ;
#53805=CARTESIAN_POINT ( 'NONE',  ( 18.62759615963255655, 10.81492255796105972, 76.66775706135234714 ) ) ;
#53806=CARTESIAN_POINT ( 'NONE',  ( -13.89961937509977652, 13.97604488694528158, 105.6239096053143527 ) ) ;
#53807=CARTESIAN_POINT ( 'NONE',  ( 12.14591786802327356, -12.06949235617739191, 105.6260903946856899 ) ) ;
#53808=CARTESIAN_POINT ( 'NONE',  ( -21.55341960407619339, 5.719274019375674811, 83.54275706135234714 ) ) ;
#53809=CARTESIAN_POINT ( 'NONE',  ( 5.049401038298161559, -19.05341960407611168, 72.70724293864768129 ) ) ;
#53810=CARTESIAN_POINT ( 'NONE',  ( 19.02544592524334988, 5.153800228976608722, 31.45942372801900433 ) ) ;
#53811=CARTESIAN_POINT ( 'NONE',  ( -10.81492255796105439, 18.62759615963255655, 27.91775706135234358 ) ) ;
#53812=CARTESIAN_POINT ( 'NONE',  ( -9.474510206698964154, 16.51473224551069663, 65.41557627198102409 ) ) ;
#53813=CARTESIAN_POINT ( 'NONE',  ( -0.05219959533910754901, -16.53943276465976808, 87.49890960531436690 ) ) ;
#53814=CARTESIAN_POINT ( 'NONE',  ( -0.05219959533910754901, -16.53943276465976808, 42.49890960531435979 ) ) ;
#53815=CARTESIAN_POINT ( 'NONE',  ( -5.823673210054116645, -21.52544592524344225, 62.29057627198102409 ) ) ;
#53816=CARTESIAN_POINT ( 'NONE',  ( -9.474510206698964154, 16.51473224551069663, 60.41557627198102409 ) ) ;
#53817=CARTESIAN_POINT ( 'NONE',  ( -10.72451020669898014, 18.67979575497178502, 65.41557627198102409 ) ) ;
#53818=CARTESIAN_POINT ( 'NONE',  ( -19.05341960407617563, 5.049401038297882671, 58.54275706135234003 ) ) ;
#53821=CARTESIAN_POINT ( 'NONE',  ( 12.06949235617757843, -12.14591786802309237, 58.12390960531435979 ) ) ;
#53822=CARTESIAN_POINT ( 'NONE',  ( 21.53943276465977519, -0.05219959533907433946, 38.74890960531435979 ) ) ;
#53824=CARTESIAN_POINT ( 'NONE',  ( -17.49999999999999645, 5.499999999999997335, 105.7969038253417153 ) ) ;
#53825=CARTESIAN_POINT ( 'NONE',  ( 8.224510206698742110, 14.34966873604972548, 92.08442372801901854 ) ) ;
#53827=CARTESIAN_POINT ( 'NONE',  ( -5.153800228976607833, 19.02544592524334988, 87.70942372801897591 ) ) ;
#53828=CARTESIAN_POINT ( 'NONE',  ( 0.05219959533910956823, 16.53943276465976808, 69.99890960531435269 ) ) ;
#53829=CARTESIAN_POINT ( 'NONE',  ( -19.19724070472092237, -5.500000000000168754, 61.06193348274385357 ) ) ;
#53830=CARTESIAN_POINT ( 'NONE',  ( -0.05219959533909027116, -19.03943276465977164, 57.49890960531435979 ) ) ;
#53831=CARTESIAN_POINT ( 'NONE',  ( -12.14591786802309592, -12.06949235617757132, 46.87390960531435979 ) ) ;
#53833=CARTESIAN_POINT ( 'NONE',  ( 5.153800228976335163, 19.02544592524342804, 84.79057627198099567 ) ) ;
#53834=CARTESIAN_POINT ( 'NONE',  ( 13.97604488694548053, -13.89961937509957401, 80.62609039468567573 ) ) ;
#53835=CARTESIAN_POINT ( 'NONE',  ( -19.05341960407611168, -5.049401038298163336, 51.45724293864770260 ) ) ;
#53836=CARTESIAN_POINT ( 'NONE',  ( -10.81492255796105439, 18.62759615963255655, 52.91775706135235424 ) ) ;
#53837=CARTESIAN_POINT ( 'NONE',  ( 16.51473224551069308, 9.474510206698969483, 89.16557627198103830 ) ) ;
#53838=CARTESIAN_POINT ( 'NONE',  ( 5.153800228976335163, 19.02544592524342804, 29.79057627198102409 ) ) ;
#53839=CARTESIAN_POINT ( 'NONE',  ( -13.97604488694527625, -13.89961937509977652, 76.87390960531433848 ) ) ;
#53840=CARTESIAN_POINT ( 'NONE',  ( -18.62759615963270932, 10.81492255796079327, 50.83224293864770971 ) ) ;
#53841=CARTESIAN_POINT ( 'NONE',  ( 13.97604488694527802, 13.89961937509977652, 44.37390960531435269 ) ) ;
#53842=CARTESIAN_POINT ( 'NONE',  ( 15.80617190586746368, 15.72974639402197994, 59.37390960531436690 ) ) ;
#53843=CARTESIAN_POINT ( 'NONE',  ( -19.03943276465977164, -0.05219959533935918106, 78.75109039468567573 ) ) ;
#53844=CARTESIAN_POINT ( 'NONE',  ( -14.34966873604972548, 8.224510206698743886, 103.3344237280190043 ) ) ;
#53845=CARTESIAN_POINT ( 'NONE',  ( 13.97604488694548053, -13.89961937509957401, 35.62609039468567573 ) ) ;
#53846=CARTESIAN_POINT ( 'NONE',  ( 8.224510206698742110, 14.34966873604972548, 57.08442372801901854 ) ) ;
#53847=CARTESIAN_POINT ( 'NONE',  ( -8.224510206698735004, -14.34966873604973081, 94.58442372801901854 ) ) ;
#53848=PLANE ( 'NONE',  #101681 ) ;
#53849=CARTESIAN_POINT ( 'NONE',  ( -0.05219959533934338120, 16.53943276465976808, 82.50109039468568994 ) ) ;
#53850=CARTESIAN_POINT ( 'NONE',  ( -18.62759615963270932, 10.81492255796079327, 25.83224293864769194 ) ) ;
#53851=CARTESIAN_POINT ( 'NONE',  ( -13.97604488694527625, -13.89961937509977652, 31.87390960531435979 ) ) ;
#53852=CARTESIAN_POINT ( 'NONE',  ( -8.224510206698735004, -14.34966873604973081, 34.58442372801900433 ) ) ;
#53853=CARTESIAN_POINT ( 'NONE',  ( -9.564922557960796823, -16.46253265017161027, 47.08224293864769550 ) ) ;
#53854=CARTESIAN_POINT ( 'NONE',  ( -15.72974639402176322, -15.80617190586768395, 44.37609039468567573 ) ) ;
#53855=CARTESIAN_POINT ( 'NONE',  ( -14.34966873604972548, 8.224510206698743886, 43.33442372801901143 ) ) ;
#53856=CARTESIAN_POINT ( 'NONE',  ( -14.34966873604972548, 8.224510206698743886, 108.3344237280190185 ) ) ;
#53857=CARTESIAN_POINT ( 'NONE',  ( 9.564922557960805705, 16.46253265017160317, 24.58224293864769194 ) ) ;
#53858=CARTESIAN_POINT ( 'NONE',  ( -5.049401038297874678, -19.05341960407617918, 19.79275706135233293 ) ) ;
#53859=CARTESIAN_POINT ( 'NONE',  ( 5.049401038297881783, 19.05341960407617563, 107.2927570613523187 ) ) ;
#53860=CARTESIAN_POINT ( 'NONE',  ( -19.02544592524334988, -5.153800228976617603, 68.95942372801896170 ) ) ;
#53861=CARTESIAN_POINT ( 'NONE',  ( -16.53943276465976808, 0.05219959533911058130, 66.24890960531436690 ) ) ;
#53862=CARTESIAN_POINT ( 'NONE',  ( 19.05341960407611168, 5.049401038298154454, 33.95724293864769550 ) ) ;
#53863=CARTESIAN_POINT ( 'NONE',  ( 9.564922557961047289, -16.46253265017146816, 75.41775706135234714 ) ) ;
#53864=CARTESIAN_POINT ( 'NONE',  ( 16.18388926212238488, -7.379444403734516378, 92.06046848633846480 ) ) ;
#53865=CARTESIAN_POINT ( 'NONE',  ( 21.53943276465977519, 0.05219959533937863772, 61.25109039468567573 ) ) ;
#53866=CARTESIAN_POINT ( 'NONE',  ( -16.53943276465976808, -0.05219959533934237506, 38.75109039468567573 ) ) ;
#53867=CARTESIAN_POINT ( 'NONE',  ( 18.22780087662123805, -5.499999999999976019, 73.51763182126894947 ) ) ;
#53868=CARTESIAN_POINT ( 'NONE',  ( -21.53943276465977519, 0.05219959533907696930, 41.24890960531435269 ) ) ;
#53869=CARTESIAN_POINT ( 'NONE',  ( -16.53943276465976808, -0.05219959533934237506, 28.75109039468567929 ) ) ;
#53870=CARTESIAN_POINT ( 'NONE',  ( 13.97604488694527802, 13.89961937509977652, 114.3739096053143669 ) ) ;
#53872=CARTESIAN_POINT ( 'NONE',  ( 13.89961937509977652, -13.97604488694527269, 38.12390960531436690 ) ) ;
#53873=CARTESIAN_POINT ( 'NONE',  ( 10.81492255796106328, -18.62759615963255655, 105.4177570613523613 ) ) ;
#53874=CARTESIAN_POINT ( 'NONE',  ( -0.05219959533909027116, -19.03943276465977164, 57.49890960531435979 ) ) ;
#53875=CARTESIAN_POINT ( 'NONE',  ( -21.53943276465977519, -0.05219959533937600094, 63.75109039468568284 ) ) ;
#53876=CARTESIAN_POINT ( 'NONE',  ( 15.80617190586769283, -15.72974639402175789, 100.6260903946857184 ) ) ;
#53877=CARTESIAN_POINT ( 'NONE',  ( 16.52544592524335698, 4.483927247898782831, 111.4594237280190328 ) ) ;
#53878=CARTESIAN_POINT ( 'NONE',  ( 19.02544592524343514, -5.153800228976328945, 28.54057627198102409 ) ) ;
#53879=CARTESIAN_POINT ( 'NONE',  ( 16.46253265017160672, -9.564922557960803928, 88.33224293864769550 ) ) ;
#53880=CARTESIAN_POINT ( 'NONE',  ( 10.81492255796106328, -18.62759615963255655, 55.41775706135234714 ) ) ;
#53881=CARTESIAN_POINT ( 'NONE',  ( 13.89961937509977652, -13.97604488694527269, 33.12390960531434558 ) ) ;
#53882=CARTESIAN_POINT ( 'NONE',  ( -21.52544592524334988, -5.823673210054445271, 58.95942372801902565 ) ) ;
#53883=CARTESIAN_POINT ( 'NONE',  ( 9.474510206698729675, 16.51473224551082808, 97.08442372801900433 ) ) ;
#53884=CARTESIAN_POINT ( 'NONE',  ( -19.02544592524342804, 5.153800228976336051, 101.0405762719810241 ) ) ;
#53885=CARTESIAN_POINT ( 'NONE',  ( 16.46253265017160672, -9.564922557960803928, 23.33224293864769194 ) ) ;
#53886=CARTESIAN_POINT ( 'NONE',  ( -21.53943276465977519, -0.05219959533937600094, 18.75109039468568639 ) ) ;
#53887=CARTESIAN_POINT ( 'NONE',  ( 13.89961937509957401, 13.97604488694547697, 31.87609039468566863 ) ) ;
#53888=CARTESIAN_POINT ( 'NONE',  ( -8.224510206698948167, 14.34966873604960824, 110.4155762719810383 ) ) ;
#53889=CARTESIAN_POINT ( 'NONE',  ( -5.049401038298153566, 19.05341960407611168, 45.20724293864769550 ) ) ;
#53890=CARTESIAN_POINT ( 'NONE',  ( 16.46253265017146816, 9.564922557961045513, 91.66775706135234714 ) ) ;
#53891=CARTESIAN_POINT ( 'NONE',  ( 4.379528057220339221, -16.55341960407611168, 62.70724293864769550 ) ) ;
#53892=CARTESIAN_POINT ( 'NONE',  ( 19.05341960407617918, -5.049401038297876454, 26.04275706135233293 ) ) ;
#53893=CARTESIAN_POINT ( 'NONE',  ( 5.719274019375991003, -21.55341960407610458, 22.70724293864769194 ) ) ;
#53894=CARTESIAN_POINT ( 'NONE',  ( 16.51473224551083163, -9.474510206698727899, 90.83442372801900433 ) ) ;
#53895=CARTESIAN_POINT ( 'NONE',  ( 18.62759615963271287, -10.81492255796078972, 93.33224293864769550 ) ) ;
#53896=CARTESIAN_POINT ( 'NONE',  ( -21.52544592524334988, -5.823673210054445271, 48.95942372801902565 ) ) ;
#53897=CARTESIAN_POINT ( 'NONE',  ( -12.14591786802326823, 12.06949235617739902, 38.12609039468567573 ) ) ;
#53898=CARTESIAN_POINT ( 'NONE',  ( 14.29746914071037800, 8.314922557961029526, 101.6677570613523613 ) ) ;
#53899=CARTESIAN_POINT ( 'NONE',  ( 14.34966873604972726, -8.224510206698740333, 45.83442372801901854 ) ) ;
#53900=CARTESIAN_POINT ( 'NONE',  ( -15.80617190586768217, 15.72974639402176855, 43.12609039468568284 ) ) ;
#53901=CARTESIAN_POINT ( 'NONE',  ( -0.05219959533907301413, -21.53943276465977519, 57.49890960531435979 ) ) ;
#53902=CARTESIAN_POINT ( 'NONE',  ( 13.89961937509977652, -13.97604488694527269, 38.12390960531436690 ) ) ;
#53904=CARTESIAN_POINT ( 'NONE',  ( -14.29746914071037622, -8.314922557961029526, 64.16775706135234714 ) ) ;
#53905=CARTESIAN_POINT ( 'NONE',  ( -5.719274019375978568, 21.55341960407610458, 95.20724293864769550 ) ) ;
#53906=CARTESIAN_POINT ( 'NONE',  ( -16.55341960407611168, -4.379528057220339221, 41.45724293864769550 ) ) ;
#53907=CARTESIAN_POINT ( 'NONE',  ( 4.483927247898790824, -16.52544592524335698, 60.20942372801902565 ) ) ;
#53908=CARTESIAN_POINT ( 'NONE',  ( -9.564922557961040184, 16.46253265017147172, 97.91775706135233293 ) ) ;
#53909=CARTESIAN_POINT ( 'NONE',  ( 21.53943276465977519, -0.05219959533907433946, 93.74890960531436690 ) ) ;
#53910=CARTESIAN_POINT ( 'NONE',  ( -12.06949235617756955, 12.14591786802309770, 30.62390960531436335 ) ) ;
#53912=CARTESIAN_POINT ( 'NONE',  ( 4.379528057220092307, 16.55341960407617563, 82.29275706135234714 ) ) ;
#53914=CARTESIAN_POINT ( 'NONE',  ( 15.80617190586746368, 15.72974639402197994, 69.37390960531436690 ) ) ;
#53916=CARTESIAN_POINT ( 'NONE',  ( -14.34966873604972548, 8.224510206698743886, 108.3344237280190185 ) ) ;
#53917=ORIENTED_EDGE ( 'NONE', *, *, #195432, .T. ) ;
#53918=LINE ( 'NONE', #38752, #33966 ) ;
#53919=CARTESIAN_POINT ( 'NONE',  ( -15.72974639402197994, 15.80617190586746368, 85.62390960531436690 ) ) ;
#53920=CARTESIAN_POINT ( 'NONE',  ( 5.823673210054125526, 21.52544592524343514, 104.7905762719810241 ) ) ;
#53921=CARTESIAN_POINT ( 'NONE',  ( 12.14591786802309770, 12.06949235617756955, 44.37390960531435979 ) ) ;
#53922=CARTESIAN_POINT ( 'NONE',  ( 8.314922557961029526, -14.29746914071037800, 35.41775706135234003 ) ) ;
#53923=CARTESIAN_POINT ( 'NONE',  ( -0.05219959533909027116, -19.03943276465977164, 47.49890960531435979 ) ) ;
#53924=CARTESIAN_POINT ( 'NONE',  ( 16.51473224551069308, 9.474510206698969483, 69.16557627198102409 ) ) ;
#53925=CARTESIAN_POINT ( 'NONE',  ( -18.67979575497178146, -10.72451020669898902, 26.66557627198103475 ) ) ;
#53926=CARTESIAN_POINT ( 'NONE',  ( -13.97604488694527625, -13.89961937509977652, 111.8739096053143243 ) ) ;
#53927=CARTESIAN_POINT ( 'NONE',  ( 19.03943276465977164, 0.05219959533936151252, 106.2510903946856615 ) ) ;
#53928=CARTESIAN_POINT ( 'NONE',  ( 9.564922557961047289, -16.46253265017146816, 45.41775706135232582 ) ) ;
#53929=CARTESIAN_POINT ( 'NONE',  ( -21.55341960407610458, -5.719274019375992779, 91.45724293864769550 ) ) ;
#53930=CARTESIAN_POINT ( 'NONE',  ( -14.34966873604960291, -8.224510206698953496, 26.66557627198103475 ) ) ;
#53931=CARTESIAN_POINT ( 'NONE',  ( 18.67979575497178502, 10.72451020669898547, 44.16557627198103120 ) ) ;
#53932=CARTESIAN_POINT ( 'NONE',  ( -10.81492255796078084, -18.62759615963271287, 87.08224293864769550 ) ) ;
#53933=CARTESIAN_POINT ( 'NONE',  ( 5.049401038297881783, 19.05341960407617563, 112.2927570613523471 ) ) ;
#53934=CARTESIAN_POINT ( 'NONE',  ( 5.049401038298161559, -19.05341960407611168, 102.7072429386476955 ) ) ;
#53935=CARTESIAN_POINT ( 'NONE',  ( 10.81492255796106328, -18.62759615963255655, 75.41775706135233293 ) ) ;
#53936=CARTESIAN_POINT ( 'NONE',  ( -0.05219959533909027116, -19.03943276465977164, 77.49890960531435269 ) ) ;
#53937=CARTESIAN_POINT ( 'NONE',  ( -16.52544592524342804, 4.483927247898546575, 101.0405762719810383 ) ) ;
#53939=CARTESIAN_POINT ( 'NONE',  ( -16.46253265017160317, 9.564922557960807481, 65.83224293864769550 ) ) ;
#53940=CARTESIAN_POINT ( 'NONE',  ( -4.483927247898539470, -16.52544592524342804, 97.29057627198105251 ) ) ;
#53941=ORIENTED_EDGE ( 'NONE', *, *, #100927, .F. ) ;
#53942=CARTESIAN_POINT ( 'NONE',  ( -19.03943276465977164, -0.05219959533935918106, 103.7510903946856757 ) ) ;
#53943=CARTESIAN_POINT ( 'NONE',  ( 16.29526858892876717, -7.335722546920110609, 81.70329402199794799 ) ) ;
#53944=CARTESIAN_POINT ( 'NONE',  ( 19.03943276465977164, -0.05219959533909143690, 63.74890960531435979 ) ) ;
#53945=CARTESIAN_POINT ( 'NONE',  ( -15.72974639402176322, -15.80617190586768395, 84.37609039468570415 ) ) ;
#53946=CARTESIAN_POINT ( 'NONE',  ( -5.049401038298153566, 19.05341960407611168, 95.20724293864770971 ) ) ;
#53947=CARTESIAN_POINT ( 'NONE',  ( -14.29746914071037622, -8.314922557961029526, 74.16775706135231871 ) ) ;
#53948=CARTESIAN_POINT ( 'NONE',  ( -17.50000000000002842, -5.622605283950846911, 76.31207310596114723 ) ) ;
#53949=CARTESIAN_POINT ( 'NONE',  ( -16.46253265017146816, -9.564922557961047289, 59.16775706135233293 ) ) ;
#53950=CARTESIAN_POINT ( 'NONE',  ( -18.62759615963255300, -10.81492255796106328, 104.1677570613523471 ) ) ;
#53953=CARTESIAN_POINT ( 'NONE',  ( -12.14591786802309592, -12.06949235617757132, 21.87390960531436690 ) ) ;
#53954=ADVANCED_FACE ( 'NONE', ( #82262 ), #159750, .F. ) ;
#53955=CARTESIAN_POINT ( 'NONE',  ( -16.46253265017146816, -9.564922557961047289, 74.16775706135234714 ) ) ;
#53956=CARTESIAN_POINT ( 'NONE',  ( 8.224510206698742110, 14.34966873604972548, 97.08442372801904696 ) ) ;
#53958=CARTESIAN_POINT ( 'NONE',  ( 14.29746914071037800, 8.314922557961029526, 71.66775706135234714 ) ) ;
#53959=CARTESIAN_POINT ( 'NONE',  ( 21.52544592524334988, 5.823673210054432836, 81.45942372801900433 ) ) ;
#53960=CARTESIAN_POINT ( 'NONE',  ( 19.05341960407617918, -5.049401038297876454, 86.04275706135233293 ) ) ;
#53961=CARTESIAN_POINT ( 'NONE',  ( -16.51473224551082808, 9.474510206698731452, 43.33442372801900433 ) ) ;
#53962=CARTESIAN_POINT ( 'NONE',  ( -0.05219959533909027116, -19.03943276465977164, 62.49890960531435979 ) ) ;
#53963=CARTESIAN_POINT ( 'NONE',  ( 19.05341960407611168, 5.049401038298154454, 53.95724293864770260 ) ) ;
#53966=CARTESIAN_POINT ( 'NONE',  ( 15.80617190586746368, 15.72974639402197994, 79.37390960531436690 ) ) ;
#53967=CARTESIAN_POINT ( 'NONE',  ( 15.80617190586746368, 15.72974639402197994, 44.37390960531435979 ) ) ;
#53968=CARTESIAN_POINT ( 'NONE',  ( 5.153800228976335163, 19.02544592524342804, 39.79057627198100988 ) ) ;
#53969=CARTESIAN_POINT ( 'NONE',  ( -14.29746914071037622, -8.314922557961029526, 69.16775706135234714 ) ) ;
#53970=UNCERTAINTY_MEASURE_WITH_UNIT (LENGTH_MEASURE( 1.000000000000000082E-05 ), #172890, 'distance_accuracy_value', 'NONE');
#53971=ORIENTED_EDGE ( 'NONE', *, *, #80196, .F. ) ;
#53972=CARTESIAN_POINT ( 'NONE',  ( -10.72451020669870658, -18.67979575497194134, 49.58442372801901143 ) ) ;
#53973=CARTESIAN_POINT ( 'NONE',  ( 8.314922557960818139, 14.29746914071049879, 59.58224293864770260 ) ) ;
#53975=CARTESIAN_POINT ( 'NONE',  ( -16.55341960407617563, 4.379528057220093196, 38.54275706135234714 ) ) ;
#53976=CARTESIAN_POINT ( 'NONE',  ( -19.05341960407617563, 5.049401038297882671, 53.54275706135231871 ) ) ;
#53978=CARTESIAN_POINT ( 'NONE',  ( 8.224510206698953496, -14.34966873604960469, 52.91557627198103830 ) ) ;
#53979=CARTESIAN_POINT ( 'NONE',  ( 0.05219959533937995610, -21.53943276465977519, 30.00109039468568284 ) ) ;
#53980=CARTESIAN_POINT ( 'NONE',  ( -18.22780087662123094, -5.499999999999984901, 71.48459894673891313 ) ) ;
#53981=CARTESIAN_POINT ( 'NONE',  ( -21.52544592524343514, 5.823673210054127303, 86.04057627198102409 ) ) ;
#53982=CARTESIAN_POINT ( 'NONE',  ( -16.51473224551069308, -9.474510206698971260, 106.6655762719810383 ) ) ;
#53983=CARTESIAN_POINT ( 'NONE',  ( -0.05219959533910754901, -16.53943276465976808, 77.49890960531433848 ) ) ;
#53984=CARTESIAN_POINT ( 'NONE',  ( -13.89961937509977652, 13.97604488694528158, 115.6239096053143669 ) ) ;
#53985=CARTESIAN_POINT ( 'NONE',  ( 18.09918380851992481, 5.500000000000035527, 43.98618307335611632 ) ) ;
#53986=CARTESIAN_POINT ( 'NONE',  ( -9.474510206698720793, -16.51473224551083518, 64.58442372801900433 ) ) ;
#53987=CARTESIAN_POINT ( 'NONE',  ( -21.52544592524343514, 5.823673210054127303, 116.0405762719810383 ) ) ;
#53988=CARTESIAN_POINT ( 'NONE',  ( -9.564922557960796823, -16.46253265017161027, 62.08224293864769550 ) ) ;
#53989=CARTESIAN_POINT ( 'NONE',  ( -13.89961937509957401, -13.97604488694547875, 49.37609039468567573 ) ) ;
#53990=CARTESIAN_POINT ( 'NONE',  ( -19.03943276465977164, 0.05219959533909376836, 26.24890960531435624 ) ) ;
#53991=CARTESIAN_POINT ( 'NONE',  ( -0.05219959533937732626, 21.53943276465977519, 67.50109039468568994 ) ) ;
#53992=CARTESIAN_POINT ( 'NONE',  ( -17.26172910966779384, -6.454744622555833367, 69.19353091350774321 ) ) ;
#53993=CARTESIAN_POINT ( 'NONE',  ( -14.34966873604960291, -8.224510206698953496, 56.66557627198103830 ) ) ;
#53994=CARTESIAN_POINT ( 'NONE',  ( 9.564922557960805705, 16.46253265017160317, 64.58224293864769550 ) ) ;
#53995=CARTESIAN_POINT ( 'NONE',  ( -18.62759615963270932, 10.81492255796079327, 90.83224293864769550 ) ) ;
#53996=CARTESIAN_POINT ( 'NONE',  ( -9.564922557960796823, -16.46253265017161027, 52.08224293864768839 ) ) ;
#53998=CARTESIAN_POINT ( 'NONE',  ( 10.72451020669898902, -18.67979575497178502, 82.91557627198103830 ) ) ;
#53999=CARTESIAN_POINT ( 'NONE',  ( -21.52544592524334988, -5.823673210054445271, 103.9594237280190185 ) ) ;
#54000=CARTESIAN_POINT ( 'NONE',  ( 19.02544592524343514, -5.153800228976328945, 28.54057627198102409 ) ) ;
#54001=CARTESIAN_POINT ( 'NONE',  ( -4.483927247898782831, 16.52544592524335698, 92.70942372801901854 ) ) ;
#54002=CARTESIAN_POINT ( 'NONE',  ( 12.06949235617757843, -12.14591786802309237, 88.12390960531436690 ) ) ;
#54003=CARTESIAN_POINT ( 'NONE',  ( -5.049401038297874678, -19.05341960407617918, 94.79275706135230450 ) ) ;
#54005=CARTESIAN_POINT ( 'NONE',  ( 5.823673210054444382, -21.52544592524334988, 20.20942372801900788 ) ) ;
#54006=CARTESIAN_POINT ( 'NONE',  ( -5.049401038297874678, -19.05341960407617918, 44.79275706135232582 ) ) ;
#54007=CARTESIAN_POINT ( 'NONE',  ( -16.52544592524335698, -4.483927247898792601, 98.95942372801903275 ) ) ;
#54008=CARTESIAN_POINT ( 'NONE',  ( 0.05219959533936267826, -19.03943276465977164, 30.00109039468566863 ) ) ;
#54009=CARTESIAN_POINT ( 'NONE',  ( 5.153800228976335163, 19.02544592524342804, 89.79057627198102409 ) ) ;
#54010=CARTESIAN_POINT ( 'NONE',  ( 0.05219959533907565091, 21.53943276465977519, 59.99890960531436690 ) ) ;
#54011=CARTESIAN_POINT ( 'NONE',  ( -19.25663599770058809, 5.499999999999433342, 48.99419308057196787 ) ) ;
#54012=CARTESIAN_POINT ( 'NONE',  ( 12.14591786802309770, 12.06949235617756955, 114.3739096053143527 ) ) ;
#54013=CARTESIAN_POINT ( 'NONE',  ( 21.53943276465977519, 0.05219959533937863772, 106.2510903946856757 ) ) ;
#54014=CARTESIAN_POINT ( 'NONE',  ( -0.05219959533934338120, 16.53943276465976808, 77.50109039468567573 ) ) ;
#54015=CARTESIAN_POINT ( 'NONE',  ( -21.52544592524334988, -5.823673210054445271, 33.95942372801901143 ) ) ;
#54016=CARTESIAN_POINT ( 'NONE',  ( 14.29746914071037800, 8.314922557961029526, 31.66775706135234358 ) ) ;
#54017=CARTESIAN_POINT ( 'NONE',  ( 13.89961937509977652, -13.97604488694527269, 103.1239096053143527 ) ) ;
#54018=CARTESIAN_POINT ( 'NONE',  ( 0.05219959533909260263, 19.03943276465977164, 39.99890960531436690 ) ) ;
#54019=CARTESIAN_POINT ( 'NONE',  ( -16.46253265017160317, 9.564922557960807481, 70.83224293864770971 ) ) ;
#54021=CARTESIAN_POINT ( 'NONE',  ( 4.379528057220092307, 16.55341960407617563, 47.29275706135234003 ) ) ;
#54022=CARTESIAN_POINT ( 'NONE',  ( -12.14591786802309592, -12.06949235617757132, 86.87390960531438111 ) ) ;
#54023=CARTESIAN_POINT ( 'NONE',  ( -4.483927247898782831, 16.52544592524335698, 97.70942372801904696 ) ) ;
#54024=CARTESIAN_POINT ( 'NONE',  ( -5.823673210054431948, 21.52544592524334988, 57.70942372801901143 ) ) ;
#54025=CARTESIAN_POINT ( 'NONE',  ( -13.89961937509977652, 13.97604488694528158, 80.62390960531436690 ) ) ;
#54026=CARTESIAN_POINT ( 'NONE',  ( -19.03943276465977164, 0.05219959533909376836, 61.24890960531436690 ) ) ;
#54027=CARTESIAN_POINT ( 'NONE',  ( 13.97604488694527802, 13.89961937509977652, 99.37390960531436690 ) ) ;
#54028=CARTESIAN_POINT ( 'NONE',  ( -16.52544592524342804, 4.483927247898546575, 41.04057627198103120 ) ) ;
#54029=CARTESIAN_POINT ( 'NONE',  ( -14.29746914071037622, -8.314922557961029526, 99.16775706135234714 ) ) ;
#54031=CARTESIAN_POINT ( 'NONE',  ( -9.474510206698720793, -16.51473224551083518, 44.58442372801900433 ) ) ;
#54033=CARTESIAN_POINT ( 'NONE',  ( 0.05219959533909260263, 19.03943276465977164, 59.99890960531436690 ) ) ;
#54034=CARTESIAN_POINT ( 'NONE',  ( 19.03943276465977164, 0.05219959533936151252, 41.25109039468566152 ) ) ;
#54036=CARTESIAN_POINT ( 'NONE',  ( -16.29526858892878849, -7.335722546920003140, 65.79670597800208043 ) ) ;
#54037=CARTESIAN_POINT ( 'NONE',  ( -14.29746914071037622, -8.314922557961029526, 54.16775706135235424 ) ) ;
#54038=CARTESIAN_POINT ( 'NONE',  ( -9.564922557961040184, 16.46253265017147172, 67.91775706135233293 ) ) ;
#54039=CARTESIAN_POINT ( 'NONE',  ( 12.14591786802327356, -12.06949235617739191, 65.62609039468568994 ) ) ;
#54041=CARTESIAN_POINT ( 'NONE',  ( 16.46253265017160672, -9.564922557960803928, 93.33224293864769550 ) ) ;
#54042=CARTESIAN_POINT ( 'NONE',  ( -15.72974639402176322, -15.80617190586768395, 24.37609039468567573 ) ) ;
#54043=CARTESIAN_POINT ( 'NONE',  ( 0.05219959533936267826, -19.03943276465977164, 75.00109039468566152 ) ) ;
#54044=CARTESIAN_POINT ( 'NONE',  ( 0.05219959533909260263, 19.03943276465977164, 104.9989096053143669 ) ) ;
#54045=CARTESIAN_POINT ( 'NONE',  ( 19.03943276465977164, -0.05219959533909143690, 38.74890960531436690 ) ) ;
#54046=CARTESIAN_POINT ( 'NONE',  ( 19.03943276465977164, -0.05219959533909143690, 93.74890960531435269 ) ) ;
#54047=CARTESIAN_POINT ( 'NONE',  ( -0.05219959533910754901, -16.53943276465976808, 42.49890960531435979 ) ) ;
#54048=CARTESIAN_POINT ( 'NONE',  ( -9.474510206698964154, 16.51473224551069663, 35.41557627198102409 ) ) ;
#54049=CARTESIAN_POINT ( 'NONE',  ( 19.02544592524334988, 5.153800228976608722, 46.45942372801899012 ) ) ;
#54050=CARTESIAN_POINT ( 'NONE',  ( -12.14591786802309592, -12.06949235617757132, 91.87390960531436690 ) ) ;
#54051=CARTESIAN_POINT ( 'NONE',  ( 0.05219959533937995610, -21.53943276465977519, 110.0010903946856757 ) ) ;
#54052=CARTESIAN_POINT ( 'NONE',  ( 9.474510206698971260, -16.51473224551069308, 52.91557627198102409 ) ) ;
#54054=CARTESIAN_POINT ( 'NONE',  ( 10.81492255796078972, 18.62759615963270932, 69.58224293864769550 ) ) ;
#54055=CARTESIAN_POINT ( 'NONE',  ( -4.483927247898539470, -16.52544592524342804, 52.29057627198102409 ) ) ;
#54056=CARTESIAN_POINT ( 'NONE',  ( -5.049401038297874678, -19.05341960407617918, 19.79275706135233293 ) ) ;
#54057=CARTESIAN_POINT ( 'NONE',  ( 9.474510206698971260, -16.51473224551069308, 102.9155762719810241 ) ) ;
#54058=CARTESIAN_POINT ( 'NONE',  ( 0.05219959533909260263, 19.03943276465977164, 109.9989096053143669 ) ) ;
#54059=CARTESIAN_POINT ( 'NONE',  ( 0.05219959533909260263, 19.03943276465977164, 49.99890960531435979 ) ) ;
#54060=CARTESIAN_POINT ( 'NONE',  ( -5.153800228976328057, -19.02544592524343514, 22.29057627198102765 ) ) ;
#54061=CARTESIAN_POINT ( 'NONE',  ( -0.05219959533910754901, -16.53943276465976808, 87.49890960531436690 ) ) ;
#54062=CARTESIAN_POINT ( 'NONE',  ( 5.823673210054125526, 21.52544592524343514, 94.79057627198105251 ) ) ;
#54063=CARTESIAN_POINT ( 'NONE',  ( -16.51473224551069308, -9.474510206698971260, 106.6655762719810383 ) ) ;
#54064=CARTESIAN_POINT ( 'NONE',  ( 18.67979575497178502, 10.72451020669898547, 114.1655762719810383 ) ) ;
#54065=CARTESIAN_POINT ( 'NONE',  ( 16.46253265017160672, -9.564922557960803928, 103.3322429386476955 ) ) ;
#54066=CARTESIAN_POINT ( 'NONE',  ( 12.06949235617757843, -12.14591786802309237, 98.12390960531436690 ) ) ;
#54067=CARTESIAN_POINT ( 'NONE',  ( -10.72451020669870658, -18.67979575497194134, 74.58442372801901854 ) ) ;
#54068=CARTESIAN_POINT ( 'NONE',  ( 21.52544592524344225, -5.823673210054117533, 88.54057627198103830 ) ) ;
#54069=CARTESIAN_POINT ( 'NONE',  ( 16.21995358207305316, -7.366697692864187630, 107.4355100151216078 ) ) ;
#54070=CARTESIAN_POINT ( 'NONE',  ( 9.474510206698971260, -16.51473224551069308, 52.91557627198102409 ) ) ;
#54071=CARTESIAN_POINT ( 'NONE',  ( 19.26498983726238023, -5.499999999999592326, 68.05319577422007171 ) ) ;
#54072=CARTESIAN_POINT ( 'NONE',  ( 14.34966873604972726, -8.224510206698740333, 30.83442372801902209 ) ) ;
#54073=CARTESIAN_POINT ( 'NONE',  ( 8.314922557960818139, 14.29746914071049879, 109.5822429386476955 ) ) ;
#54074=CARTESIAN_POINT ( 'NONE',  ( -17.50000000000000000, -3.805241302050311969, 109.6264752721740905 ) ) ;
#54075=CARTESIAN_POINT ( 'NONE',  ( 19.02544592524343514, -5.153800228976328945, 53.54057627198102409 ) ) ;
#54076=CARTESIAN_POINT ( 'NONE',  ( 16.55341960407611168, 4.379528057220329451, 88.95724293864769550 ) ) ;
#54077=CARTESIAN_POINT ( 'NONE',  ( 21.52544592524344225, -5.823673210054117533, 28.54057627198103120 ) ) ;
#54078=CARTESIAN_POINT ( 'NONE',  ( 8.314922557960818139, 14.29746914071049879, 59.58224293864770260 ) ) ;
#54079=CARTESIAN_POINT ( 'NONE',  ( -5.153800228976607833, 19.02544592524334988, 112.7094237280190043 ) ) ;
#54080=CARTESIAN_POINT ( 'NONE',  ( 18.62759615963255655, 10.81492255796105972, 66.66775706135234714 ) ) ;
#54081=CARTESIAN_POINT ( 'NONE',  ( 17.58332526062528345, 7.635886036038587399, 61.57665040441535353 ) ) ;
#54082=CARTESIAN_POINT ( 'NONE',  ( -16.51473224551069308, -9.474510206698971260, 106.6655762719810383 ) ) ;
#54083=CARTESIAN_POINT ( 'NONE',  ( 12.14591786802327356, -12.06949235617739191, 95.62609039468568994 ) ) ;
#54084=CARTESIAN_POINT ( 'NONE',  ( -5.153800228976328057, -19.02544592524343514, 37.29057627198102409 ) ) ;
#54085=CARTESIAN_POINT ( 'NONE',  ( 16.51473224551069308, 9.474510206698969483, 89.16557627198103830 ) ) ;
#54086=CARTESIAN_POINT ( 'NONE',  ( -15.72974639402197994, 15.80617190586746368, 95.62390960531436690 ) ) ;
#54087=CARTESIAN_POINT ( 'NONE',  ( -4.483927247898782831, 16.52544592524335698, 27.70942372801901854 ) ) ;
#54088=CARTESIAN_POINT ( 'NONE',  ( -12.06949235617756955, 12.14591786802309770, 70.62390960531436690 ) ) ;
#54089=CARTESIAN_POINT ( 'NONE',  ( -21.53943276465977519, -0.05219959533937600094, 68.75109039468568994 ) ) ;
#54090=CARTESIAN_POINT ( 'NONE',  ( -16.53943276465976808, -0.05219959533934237506, 103.7510903946857042 ) ) ;
#54093=CARTESIAN_POINT ( 'NONE',  ( 8.224510206698953496, -14.34966873604960469, 22.91557627198102765 ) ) ;
#54094=CARTESIAN_POINT ( 'NONE',  ( 4.483927247898790824, -16.52544592524335698, 60.20942372801902565 ) ) ;
#54095=CARTESIAN_POINT ( 'NONE',  ( 9.564922557960805705, 16.46253265017160317, 69.58224293864770971 ) ) ;
#54096=CARTESIAN_POINT ( 'NONE',  ( -16.46253265017160317, 9.564922557960807481, 80.83224293864769550 ) ) ;
#54097=CARTESIAN_POINT ( 'NONE',  ( 18.67979575497194134, -10.72451020669871369, 80.83442372801901854 ) ) ;
#54098=CARTESIAN_POINT ( 'NONE',  ( 14.34966873604972726, -8.224510206698740333, 90.83442372801901854 ) ) ;
#54099=CARTESIAN_POINT ( 'NONE',  ( 4.483927247898545687, 16.52544592524342804, 54.79057627198104541 ) ) ;
#54100=CARTESIAN_POINT ( 'NONE',  ( -19.03943276465977164, 0.05219959533909376836, 66.24890960531436690 ) ) ;
#54101=ORIENTED_EDGE ( 'NONE', *, *, #25923, .T. ) ;
#54102=CARTESIAN_POINT ( 'NONE',  ( 9.474510206698729675, 16.51473224551082808, 107.0844237280190043 ) ) ;
#54103=CARTESIAN_POINT ( 'NONE',  ( 4.483927247898545687, 16.52544592524342804, 109.7905762719810383 ) ) ;
#54104=CARTESIAN_POINT ( 'NONE',  ( -13.97604488694527625, -13.89961937509977652, 76.87390960531433848 ) ) ;
#54105=CARTESIAN_POINT ( 'NONE',  ( 16.52544592524335698, 4.483927247898782831, 21.45942372801901499 ) ) ;
#54107=CARTESIAN_POINT ( 'NONE',  ( -21.55341960407619339, 5.719274019375674811, 113.5427570613523756 ) ) ;
#54108=CARTESIAN_POINT ( 'NONE',  ( 16.52544592524335698, 4.483927247898782831, 86.45942372801901854 ) ) ;
#54109=CARTESIAN_POINT ( 'NONE',  ( 13.89961937509957401, 13.97604488694547697, 86.87609039468567573 ) ) ;
#54110=CARTESIAN_POINT ( 'NONE',  ( -9.474510206698964154, 16.51473224551069663, 25.41557627198103120 ) ) ;
#54111=CARTESIAN_POINT ( 'NONE',  ( -12.06949235617739369, -12.14591786802326823, 64.37609039468568994 ) ) ;
#54113=CARTESIAN_POINT ( 'NONE',  ( -0.05219959533936034679, 19.03943276465977164, 57.50109039468566863 ) ) ;
#54114=CARTESIAN_POINT ( 'NONE',  ( 21.52544592524334988, 5.823673210054432836, 101.4594237280190185 ) ) ;
#54115=CARTESIAN_POINT ( 'NONE',  ( 9.564922557960805705, 16.46253265017160317, 39.58224293864768839 ) ) ;
#54116=CARTESIAN_POINT ( 'NONE',  ( -16.51473224551069308, -9.474510206698971260, 76.66557627198103830 ) ) ;
#54117=CARTESIAN_POINT ( 'NONE',  ( 16.52544592524342804, -4.483927247898539470, 68.54057627198103830 ) ) ;
#54119=CARTESIAN_POINT ( 'NONE',  ( 5.719274019375673035, 21.55341960407619339, 87.29275706135236135 ) ) ;
#54120=CARTESIAN_POINT ( 'NONE',  ( -13.97604488694547697, 13.89961937509957934, 53.12609039468565442 ) ) ;
#54121=CARTESIAN_POINT ( 'NONE',  ( 5.049401038297881783, 19.05341960407617563, 42.29275706135234003 ) ) ;
#54122=CARTESIAN_POINT ( 'NONE',  ( -5.823673210054116645, -21.52544592524344225, 42.29057627198103120 ) ) ;
#54123=CARTESIAN_POINT ( 'NONE',  ( -21.53943276465977519, -0.05219959533937600094, 93.75109039468567573 ) ) ;
#54124=CARTESIAN_POINT ( 'NONE',  ( 19.03943276465977164, -0.05219959533909143690, 83.74890960531436690 ) ) ;
#54125=CARTESIAN_POINT ( 'NONE',  ( 0.05219959533937995610, -21.53943276465977519, 110.0010903946856757 ) ) ;
#54126=CARTESIAN_POINT ( 'NONE',  ( -10.72451020669898014, 18.67979575497178502, 55.41557627198102409 ) ) ;
#54127=CARTESIAN_POINT ( 'NONE',  ( 5.049401038298161559, -19.05341960407611168, 102.7072429386476955 ) ) ;
#54128=CARTESIAN_POINT ( 'NONE',  ( -9.564922557961040184, 16.46253265017147172, 77.91775706135234714 ) ) ;
#54129=CARTESIAN_POINT ( 'NONE',  ( 0.05219959533909260263, 19.03943276465977164, 99.99890960531436690 ) ) ;
#54130=CARTESIAN_POINT ( 'NONE',  ( -5.049401038297874678, -19.05341960407617918, 94.79275706135230450 ) ) ;
#54131=CARTESIAN_POINT ( 'NONE',  ( -8.224510206698735004, -14.34966873604973081, 39.58442372801901143 ) ) ;
#54132=CARTESIAN_POINT ( 'NONE',  ( 16.52544592524342804, -4.483927247898539470, 108.5405762719810241 ) ) ;
#54133=CARTESIAN_POINT ( 'NONE',  ( -13.89961937509977652, 13.97604488694528158, 70.62390960531432427 ) ) ;
#54134=CARTESIAN_POINT ( 'NONE',  ( -0.05219959533907301413, -21.53943276465977519, 57.49890960531435979 ) ) ;
#54135=CARTESIAN_POINT ( 'NONE',  ( 14.29746914071037800, 8.314922557961029526, 31.66775706135234358 ) ) ;
#54136=CARTESIAN_POINT ( 'NONE',  ( -15.80617190586768217, 15.72974639402176855, 38.12609039468567573 ) ) ;
#54137=CARTESIAN_POINT ( 'NONE',  ( 0.05219959533937995610, -21.53943276465977519, 85.00109039468568994 ) ) ;
#54138=CARTESIAN_POINT ( 'NONE',  ( -0.05219959533934338120, 16.53943276465976808, 87.50109039468568994 ) ) ;
#54139=CARTESIAN_POINT ( 'NONE',  ( 0.05219959533909260263, 19.03943276465977164, 69.99890960531435269 ) ) ;
#54140=CARTESIAN_POINT ( 'NONE',  ( -14.34966873604960291, -8.224510206698953496, 76.66557627198103830 ) ) ;
#54141=CARTESIAN_POINT ( 'NONE',  ( -12.14591786802309592, -12.06949235617757132, 21.87390960531436690 ) ) ;
#54142=CARTESIAN_POINT ( 'NONE',  ( 19.03943276465977164, 0.05219959533936151252, 51.25109039468567573 ) ) ;
#54144=CARTESIAN_POINT ( 'NONE',  ( 21.53943276465977519, 0.05219959533937863772, 36.25109039468567573 ) ) ;
#54145=CARTESIAN_POINT ( 'NONE',  ( -8.224510206698948167, 14.34966873604960824, 85.41557627198102409 ) ) ;
#54146=CARTESIAN_POINT ( 'NONE',  ( -9.474510206698964154, 16.51473224551069663, 100.4155762719810241 ) ) ;
#54147=CARTESIAN_POINT ( 'NONE',  ( 12.06949235617739724, 12.14591786802326823, 101.8760903946857042 ) ) ;
#54148=CARTESIAN_POINT ( 'NONE',  ( 18.67979575497194134, -10.72451020669871369, 65.83442372801900433 ) ) ;
#54149=CARTESIAN_POINT ( 'NONE',  ( -14.34966873604972548, 8.224510206698743886, 48.33442372801902565 ) ) ;
#54150=CARTESIAN_POINT ( 'NONE',  ( -15.72974639402176322, -15.80617190586768395, 34.37609039468568284 ) ) ;
#54151=CARTESIAN_POINT ( 'NONE',  ( -14.29746914071049879, 8.314922557960819915, 65.83224293864769550 ) ) ;
#54153=CARTESIAN_POINT ( 'NONE',  ( 21.52544592524334988, 5.823673210054432836, 21.45942372801901499 ) ) ;
#54154=CARTESIAN_POINT ( 'NONE',  ( 8.224510206698953496, -14.34966873604960469, 92.91557627198103830 ) ) ;
#54155=CARTESIAN_POINT ( 'NONE',  ( 17.50000000000001066, -3.189878218039098989, 27.37051437428756984 ) ) ;
#54156=CARTESIAN_POINT ( 'NONE',  ( -4.483927247898539470, -16.52544592524342804, 57.29057627198103120 ) ) ;
#54157=CARTESIAN_POINT ( 'NONE',  ( 5.049401038298161559, -19.05341960407611168, 27.70724293864769550 ) ) ;
#54158=CARTESIAN_POINT ( 'NONE',  ( 5.823673210054125526, 21.52544592524343514, 44.79057627198103120 ) ) ;
#54159=CARTESIAN_POINT ( 'NONE',  ( 14.34966873604960469, 8.224510206698951720, 79.16557627198103830 ) ) ;
#54161=CARTESIAN_POINT ( 'NONE',  ( -10.72451020669898014, 18.67979575497178502, 80.41557627198103830 ) ) ;
#54162=CARTESIAN_POINT ( 'NONE',  ( 13.89961937509977652, -13.97604488694527269, 93.12390960531436690 ) ) ;
#54163=CARTESIAN_POINT ( 'NONE',  ( -19.03943276465977164, 0.05219959533909376836, 36.24890960531436690 ) ) ;
#54164=CARTESIAN_POINT ( 'NONE',  ( 9.564922557961047289, -16.46253265017146816, 85.41775706135233293 ) ) ;
#54165=CARTESIAN_POINT ( 'NONE',  ( -5.719274019375665041, -21.55341960407619695, 54.79275706135235424 ) ) ;
#54166=CARTESIAN_POINT ( 'NONE',  ( 5.719274019375991003, -21.55341960407610458, 57.70724293864770260 ) ) ;
#54167=CARTESIAN_POINT ( 'NONE',  ( 9.564922557960805705, 16.46253265017160317, 34.58224293864770260 ) ) ;
#54168=CARTESIAN_POINT ( 'NONE',  ( -9.474510206698964154, 16.51473224551069663, 70.41557627198102409 ) ) ;
#54170=CARTESIAN_POINT ( 'NONE',  ( 16.55341960407618274, -4.379528057220086978, 56.04275706135235424 ) ) ;
#54171=CARTESIAN_POINT ( 'NONE',  ( 15.80617190586769283, -15.72974639402175789, 30.62609039468567929 ) ) ;
#54172=CARTESIAN_POINT ( 'NONE',  ( 10.81492255796106328, -18.62759615963255655, 75.41775706135233293 ) ) ;
#54173=CARTESIAN_POINT ( 'NONE',  ( -9.564922557960796823, -16.46253265017161027, 102.0822429386477097 ) ) ;
#54174=CARTESIAN_POINT ( 'NONE',  ( 0.05219959533907565091, 21.53943276465977519, 84.99890960531436690 ) ) ;
#54175=CARTESIAN_POINT ( 'NONE',  ( -10.72451020669898014, 18.67979575497178502, 115.4155762719810241 ) ) ;
#54176=CARTESIAN_POINT ( 'NONE',  ( -0.05219959533934338120, 16.53943276465976808, 57.50109039468568994 ) ) ;
#54177=CARTESIAN_POINT ( 'NONE',  ( -15.72974639402197994, 15.80617190586746368, 50.62390960531435979 ) ) ;
#54178=CARTESIAN_POINT ( 'NONE',  ( -5.719274019375665041, -21.55341960407619695, 109.7927570613523613 ) ) ;
#54179=CARTESIAN_POINT ( 'NONE',  ( 5.153800228976335163, 19.02544592524342804, 54.79057627198103120 ) ) ;
#54180=CARTESIAN_POINT ( 'NONE',  ( -19.02544592524342804, 5.153800228976336051, 106.0405762719810241 ) ) ;
#54181=CARTESIAN_POINT ( 'NONE',  ( 9.474510206698971260, -16.51473224551069308, 87.91557627198102409 ) ) ;
#54182=CARTESIAN_POINT ( 'NONE',  ( 13.89961937509957579, 13.97604488694547520, 51.87609039468566863 ) ) ;
#54183=CARTESIAN_POINT ( 'NONE',  ( -0.05219959533936034679, 19.03943276465977164, 62.50109039468566863 ) ) ;
#54184=CARTESIAN_POINT ( 'NONE',  ( 21.55341960407610458, 5.719274019375980345, 38.95724293864768839 ) ) ;
#54185=CARTESIAN_POINT ( 'NONE',  ( 4.483927247898545687, 16.52544592524342804, 24.79057627198103120 ) ) ;
#54186=CARTESIAN_POINT ( 'NONE',  ( -5.049401038297874678, -19.05341960407617918, 104.7927570613523471 ) ) ;
#54187=CARTESIAN_POINT ( 'NONE',  ( 19.02544592524343514, -5.153800228976328945, 23.54057627198102054 ) ) ;
#54188=CARTESIAN_POINT ( 'NONE',  ( 13.97604488694548053, -13.89961937509957401, 25.62609039468566507 ) ) ;
#54189=CARTESIAN_POINT ( 'NONE',  ( -5.049401038297874678, -19.05341960407617918, 99.79275706135234714 ) ) ;
#54190=CARTESIAN_POINT ( 'NONE',  ( -21.55341960407610458, -5.719274019375992779, 76.45724293864769550 ) ) ;
#54191=CARTESIAN_POINT ( 'NONE',  ( -9.474510206698720793, -16.51473224551083518, 64.58442372801900433 ) ) ;
#54193=CARTESIAN_POINT ( 'NONE',  ( -9.474510206698964154, 16.51473224551069663, 55.41557627198103120 ) ) ;
#54194=CARTESIAN_POINT ( 'NONE',  ( -0.05219959533910754901, -16.53943276465976808, 67.49890960531436690 ) ) ;
#54195=ADVANCED_FACE ( 'NONE', ( #49969 ), #125808, .T. ) ;
#54196=CARTESIAN_POINT ( 'NONE',  ( -5.049401038298153566, 19.05341960407611168, 40.20724293864768839 ) ) ;
#54197=CARTESIAN_POINT ( 'NONE',  ( -14.29746914071049879, 8.314922557960819915, 45.83224293864769550 ) ) ;
#54199=CARTESIAN_POINT ( 'NONE',  ( -8.224510206698735004, -14.34966873604973081, 104.5844237280190185 ) ) ;
#54200=CARTESIAN_POINT ( 'NONE',  ( 13.89961937509977652, -13.97604488694527269, 68.12390960531436690 ) ) ;
#54201=CARTESIAN_POINT ( 'NONE',  ( 9.564922557961047289, -16.46253265017146816, 30.41775706135232937 ) ) ;
#54202=CARTESIAN_POINT ( 'NONE',  ( -16.53943276465976808, -0.05219959533934237506, 33.75109039468568284 ) ) ;
#54203=CARTESIAN_POINT ( 'NONE',  ( -10.81492255796078084, -18.62759615963271287, 57.08224293864769550 ) ) ;
#54204=CARTESIAN_POINT ( 'NONE',  ( 5.719274019375673035, 21.55341960407619339, 107.2927570613523471 ) ) ;
#54206=CARTESIAN_POINT ( 'NONE',  ( -9.474510206698964154, 16.51473224551069663, 60.41557627198102409 ) ) ;
#54207=FACE_OUTER_BOUND ( 'NONE', #152882, .T. ) ;
#54208=CARTESIAN_POINT ( 'NONE',  ( -13.89961937509977652, 13.97604488694528158, 90.62390960531432427 ) ) ;
#54210=CARTESIAN_POINT ( 'NONE',  ( 18.67979575497194134, -10.72451020669871369, 30.83442372801902209 ) ) ;
#54211=CARTESIAN_POINT ( 'NONE',  ( 4.379528057220339221, -16.55341960407611168, 92.70724293864770971 ) ) ;
#54212=CARTESIAN_POINT ( 'NONE',  ( 18.67979575497178502, 10.72451020669898547, 84.16557627198103830 ) ) ;
#54213=CARTESIAN_POINT ( 'NONE',  ( 19.03943276465977164, -0.05219959533909143690, 63.74890960531435979 ) ) ;
#54214=CARTESIAN_POINT ( 'NONE',  ( 9.474510206698971260, -16.51473224551069308, 67.91557627198102409 ) ) ;
#54215=CARTESIAN_POINT ( 'NONE',  ( 21.55341960407610458, 5.719274019375980345, 103.9572429386476813 ) ) ;
#54216=ORIENTED_EDGE ( 'NONE', *, *, #72299, .T. ) ;
#54217=CARTESIAN_POINT ( 'NONE',  ( 13.97604488694527802, 13.89961937509977652, 79.37390960531435269 ) ) ;
#54218=DIRECTION ( 'NONE',  ( 0.000000000000000000, 0.000000000000000000, -1.000000000000000000 ) ) ;
#54219=CARTESIAN_POINT ( 'NONE',  ( -8.224510206698948167, 14.34966873604960824, 110.4155762719810383 ) ) ;
#54221=CARTESIAN_POINT ( 'NONE',  ( -16.51473224551082808, 9.474510206698731452, 88.33442372801900433 ) ) ;
#54222=CARTESIAN_POINT ( 'NONE',  ( 16.55341960407611168, 4.379528057220329451, 103.9572429386476813 ) ) ;
#54223=CARTESIAN_POINT ( 'NONE',  ( 10.72451020669871369, 18.67979575497193778, 72.08442372801899012 ) ) ;
#54224=CARTESIAN_POINT ( 'NONE',  ( -9.564922557960796823, -16.46253265017161027, 67.08224293864769550 ) ) ;
#54225=CARTESIAN_POINT ( 'NONE',  ( 18.67979575497194134, -10.72451020669871369, 30.83442372801902209 ) ) ;
#54226=CARTESIAN_POINT ( 'NONE',  ( 0.05219959533907565091, 21.53943276465977519, 114.9989096053143669 ) ) ;
#54228=CARTESIAN_POINT ( 'NONE',  ( 5.049401038298161559, -19.05341960407611168, 67.70724293864769550 ) ) ;
#54230=CARTESIAN_POINT ( 'NONE',  ( -12.06949235617739369, -12.14591786802326823, 29.37609039468568284 ) ) ;
#54231=CARTESIAN_POINT ( 'NONE',  ( -5.719274019375978568, 21.55341960407610458, 30.20724293864769550 ) ) ;
#54232=CARTESIAN_POINT ( 'NONE',  ( 21.52544592524334988, 5.823673210054432836, 66.45942372801903275 ) ) ;
#54233=CARTESIAN_POINT ( 'NONE',  ( -16.46253265017160317, 9.564922557960807481, 105.8322429386476955 ) ) ;
#54234=CARTESIAN_POINT ( 'NONE',  ( -5.153800228976607833, 19.02544592524334988, 102.7094237280189759 ) ) ;
#54235=CARTESIAN_POINT ( 'NONE',  ( 13.89961937509977652, -13.97604488694527269, 53.12390960531434558 ) ) ;
#54236=CARTESIAN_POINT ( 'NONE',  ( -13.97604488694527625, -13.89961937509977652, 71.87390960531433848 ) ) ;
#54237=CARTESIAN_POINT ( 'NONE',  ( -12.06949235617756955, 12.14591786802309770, 95.62390960531436690 ) ) ;
#54238=CARTESIAN_POINT ( 'NONE',  ( 5.153800228976335163, 19.02544592524342804, 104.7905762719809957 ) ) ;
#54239=CARTESIAN_POINT ( 'NONE',  ( 8.224510206698953496, -14.34966873604960469, 97.91557627198103830 ) ) ;
#54240=CARTESIAN_POINT ( 'NONE',  ( 13.97604488694527802, 13.89961937509977652, 99.37390960531436690 ) ) ;
#54241=CARTESIAN_POINT ( 'NONE',  ( -14.34966873604960291, -8.224510206698953496, 46.66557627198102409 ) ) ;
#54242=CARTESIAN_POINT ( 'NONE',  ( 13.89961937509977652, -13.97604488694527269, 38.12390960531436690 ) ) ;
#54243=CARTESIAN_POINT ( 'NONE',  ( 21.52544592524334988, 5.823673210054432836, 61.45942372801901854 ) ) ;
#54244=CARTESIAN_POINT ( 'NONE',  ( 16.46253265017146816, 9.564922557961045513, 76.66775706135234714 ) ) ;
#54245=CARTESIAN_POINT ( 'NONE',  ( 16.55341960407611168, 4.379528057220329451, 43.95724293864769550 ) ) ;
#54246=CARTESIAN_POINT ( 'NONE',  ( 21.55341960407610458, 5.719274019375980345, 103.9572429386476813 ) ) ;
#54247=CARTESIAN_POINT ( 'NONE',  ( -0.05219959533907301413, -21.53943276465977519, 42.49890960531435979 ) ) ;
#54248=CARTESIAN_POINT ( 'NONE',  ( -16.46253265017160317, 9.564922557960807481, 115.8322429386477097 ) ) ;
#54249=CARTESIAN_POINT ( 'NONE',  ( -0.05219959533910754901, -16.53943276465976808, 87.49890960531436690 ) ) ;
#54250=CARTESIAN_POINT ( 'NONE',  ( -13.89961937509977652, 13.97604488694528158, 60.62390960531436690 ) ) ;
#54251=CARTESIAN_POINT ( 'NONE',  ( 12.14591786802309770, 12.06949235617756955, 29.37390960531435269 ) ) ;
#54253=CARTESIAN_POINT ( 'NONE',  ( -8.314922557961024197, 14.29746914071037800, 97.91775706135236135 ) ) ;
#54254=CARTESIAN_POINT ( 'NONE',  ( -0.05219959533934338120, 16.53943276465976808, 77.50109039468567573 ) ) ;
#54255=CARTESIAN_POINT ( 'NONE',  ( -13.89961937509957401, -13.97604488694547875, 34.37609039468566863 ) ) ;
#54257=CARTESIAN_POINT ( 'NONE',  ( 19.05341960407611168, 5.049401038298154454, 108.9572429386477097 ) ) ;
#54258=CARTESIAN_POINT ( 'NONE',  ( -19.03943276465977164, 0.05219959533909376836, 81.24890960531436690 ) ) ;
#54259=CARTESIAN_POINT ( 'NONE',  ( -13.89961937509977652, 13.97604488694528158, 40.62390960531435979 ) ) ;
#54260=CARTESIAN_POINT ( 'NONE',  ( 12.06949235617757843, -12.14591786802309237, 48.12390960531436690 ) ) ;
#54261=CARTESIAN_POINT ( 'NONE',  ( 19.02544592524343514, -5.153800228976328945, 103.5405762719809957 ) ) ;
#54262=CARTESIAN_POINT ( 'NONE',  ( -5.823673210054116645, -21.52544592524344225, 42.29057627198103120 ) ) ;
#54263=CARTESIAN_POINT ( 'NONE',  ( -4.483927247898539470, -16.52544592524342804, 82.29057627198103830 ) ) ;
#54264=CARTESIAN_POINT ( 'NONE',  ( -0.05219959533934338120, 16.53943276465976808, 37.50109039468568284 ) ) ;
#54265=CARTESIAN_POINT ( 'NONE',  ( -12.06949235617756955, 12.14591786802309770, 65.62390960531436690 ) ) ;
#54267=CARTESIAN_POINT ( 'NONE',  ( 9.564922557961047289, -16.46253265017146816, 60.41775706135233293 ) ) ;
#54268=CARTESIAN_POINT ( 'NONE',  ( -5.049401038298153566, 19.05341960407611168, 105.2072429386476671 ) ) ;
#54269=CARTESIAN_POINT ( 'NONE',  ( 5.153800228976615827, -19.02544592524334988, 75.20942372801896170 ) ) ;
#54270=CARTESIAN_POINT ( 'NONE',  ( 9.564922557961047289, -16.46253265017146816, 95.41775706135233293 ) ) ;
#54271=CARTESIAN_POINT ( 'NONE',  ( -0.05219959533936034679, 19.03943276465977164, 112.5010903946856757 ) ) ;
#54272=CARTESIAN_POINT ( 'NONE',  ( 8.314922557961029526, -14.29746914071037800, 110.4177570613523756 ) ) ;
#54273=CARTESIAN_POINT ( 'NONE',  ( 9.564922557961047289, -16.46253265017146816, 75.41775706135234714 ) ) ;
#54274=CARTESIAN_POINT ( 'NONE',  ( -21.52544592524343514, 5.823673210054127303, 36.04057627198102409 ) ) ;
#54275=CARTESIAN_POINT ( 'NONE',  ( -5.719274019375665041, -21.55341960407619695, 64.79275706135234714 ) ) ;
#54276=CARTESIAN_POINT ( 'NONE',  ( 19.54388014595539147, 5.500000000000039080, 37.68481143343646522 ) ) ;
#54277=CARTESIAN_POINT ( 'NONE',  ( 9.564922557961047289, -16.46253265017146816, 110.4177570613523471 ) ) ;
#54278=DIRECTION ( 'NONE',  ( 0.000000000000000000, 1.000000000000000000, 0.000000000000000000 ) ) ;
#54279=CARTESIAN_POINT ( 'NONE',  ( -19.03943276465977164, 0.05219959533909376836, 76.24890960531435269 ) ) ;
#54282=CARTESIAN_POINT ( 'NONE',  ( -0.05219959533910754901, -16.53943276465976808, 82.49890960531436690 ) ) ;
#54283=CARTESIAN_POINT ( 'NONE',  ( -19.03943276465977164, 0.05219959533909376836, 71.24890960531435269 ) ) ;
#54284=CARTESIAN_POINT ( 'NONE',  ( -5.153800228976328057, -19.02544592524343514, 92.29057627198099567 ) ) ;
#54285=ORIENTED_EDGE ( 'NONE', *, *, #6630, .T. ) ;
#54286=CARTESIAN_POINT ( 'NONE',  ( -9.474510206698720793, -16.51473224551083518, 94.58442372801900433 ) ) ;
#54287=CARTESIAN_POINT ( 'NONE',  ( -5.719274019375978568, 21.55341960407610458, 75.20724293864769550 ) ) ;
#54288=CARTESIAN_POINT ( 'NONE',  ( -19.03943276465977164, 0.05219959533909376836, 36.24890960531436690 ) ) ;
#54289=CARTESIAN_POINT ( 'NONE',  ( 16.46253265017146816, 9.564922557961045513, 76.66775706135234714 ) ) ;
#54290=CARTESIAN_POINT ( 'NONE',  ( 19.05341960407611168, 5.049401038298154454, 68.95724293864769550 ) ) ;
#54291=CARTESIAN_POINT ( 'NONE',  ( 19.05341960407611168, 5.049401038298154454, 88.95724293864769550 ) ) ;
#54293=CARTESIAN_POINT ( 'NONE',  ( 15.80617190586746368, 15.72974639402197994, 104.3739096053143669 ) ) ;
#54294=CARTESIAN_POINT ( 'NONE',  ( -14.29746914071049879, 8.314922557960819915, 95.83224293864770971 ) ) ;
#54295=CARTESIAN_POINT ( 'NONE',  ( -9.474510206698964154, 16.51473224551069663, 80.41557627198103830 ) ) ;
#54296=CARTESIAN_POINT ( 'NONE',  ( 0.05219959533936267826, -19.03943276465977164, 65.00109039468567573 ) ) ;
#54297=CARTESIAN_POINT ( 'NONE',  ( 18.62759615963271287, -10.81492255796078972, 93.33224293864769550 ) ) ;
#54298=CARTESIAN_POINT ( 'NONE',  ( -10.81492255796078084, -18.62759615963271287, 67.08224293864770971 ) ) ;
#54299=CARTESIAN_POINT ( 'NONE',  ( -4.483927247898539470, -16.52544592524342804, 42.29057627198103120 ) ) ;
#54300=CARTESIAN_POINT ( 'NONE',  ( 0.05219959533937995610, -21.53943276465977519, 105.0010903946856757 ) ) ;
#54301=CARTESIAN_POINT ( 'NONE',  ( 16.55341960407618274, -4.379528057220086978, 66.04275706135236135 ) ) ;
#54302=CARTESIAN_POINT ( 'NONE',  ( 9.564922557960805705, 16.46253265017160317, 89.58224293864769550 ) ) ;
#54303=CARTESIAN_POINT ( 'NONE',  ( 16.51473224551069308, 9.474510206698969483, 34.16557627198102409 ) ) ;
#54304=CARTESIAN_POINT ( 'NONE',  ( 0.05219959533937995610, -21.53943276465977519, 45.00109039468568284 ) ) ;
#54305=CARTESIAN_POINT ( 'NONE',  ( 5.719274019375673035, 21.55341960407619339, 52.29275706135236135 ) ) ;
#54306=CARTESIAN_POINT ( 'NONE',  ( -13.89961937509977652, 13.97604488694528158, 60.62390960531436690 ) ) ;
#54307=CARTESIAN_POINT ( 'NONE',  ( -5.823673210054431948, 21.52544592524334988, 37.70942372801900433 ) ) ;
#54308=CARTESIAN_POINT ( 'NONE',  ( 13.97604488694548053, -13.89961937509957401, 75.62609039468564731 ) ) ;
#54309=CARTESIAN_POINT ( 'NONE',  ( -9.564922557961040184, 16.46253265017147172, 67.91775706135233293 ) ) ;
#54310=CARTESIAN_POINT ( 'NONE',  ( 13.97604488694527802, 13.89961937509977652, 44.37390960531435269 ) ) ;
#54311=CARTESIAN_POINT ( 'NONE',  ( 4.379528057220092307, 16.55341960407617563, 77.29275706135234714 ) ) ;
#54312=CARTESIAN_POINT ( 'NONE',  ( -16.46253265017160317, 9.564922557960807481, 55.83224293864769550 ) ) ;
#54314=CARTESIAN_POINT ( 'NONE',  ( -19.02544592524342804, 5.153800228976336051, 101.0405762719810241 ) ) ;
#54315=CARTESIAN_POINT ( 'NONE',  ( -0.05219959533909027116, -19.03943276465977164, 42.49890960531435269 ) ) ;
#54316=CARTESIAN_POINT ( 'NONE',  ( 10.72451020669898902, -18.67979575497178502, 67.91557627198102409 ) ) ;
#54317=CARTESIAN_POINT ( 'NONE',  ( 16.55341960407618274, -4.379528057220086978, 61.04275706135234714 ) ) ;
#54318=CARTESIAN_POINT ( 'NONE',  ( -13.97604488694547697, 13.89961937509957934, 23.12609039468565442 ) ) ;
#54319=CARTESIAN_POINT ( 'NONE',  ( -5.153800228976328057, -19.02544592524343514, 57.29057627198103120 ) ) ;
#54320=CARTESIAN_POINT ( 'NONE',  ( -8.314922557960811034, -14.29746914071050412, 42.08224293864769550 ) ) ;
#54321=CARTESIAN_POINT ( 'NONE',  ( -12.06949235617756955, 12.14591786802309770, 85.62390960531436690 ) ) ;
#54322=CARTESIAN_POINT ( 'NONE',  ( -9.474510206698964154, 16.51473224551069663, 80.41557627198103830 ) ) ;
#54323=CARTESIAN_POINT ( 'NONE',  ( -10.72451020669870658, -18.67979575497194134, 34.58442372801900433 ) ) ;
#54324=CARTESIAN_POINT ( 'NONE',  ( -16.46253265017160317, 9.564922557960807481, 90.83224293864769550 ) ) ;
#54325=CARTESIAN_POINT ( 'NONE',  ( -15.72974639402176322, -15.80617190586768395, 104.3760903946856899 ) ) ;
#54326=CARTESIAN_POINT ( 'NONE',  ( -12.14591786802326823, 12.06949235617739902, 68.12609039468567573 ) ) ;
#54328=CARTESIAN_POINT ( 'NONE',  ( -13.89961937509977652, 13.97604488694528158, 110.6239096053143243 ) ) ;
#54329=CARTESIAN_POINT ( 'NONE',  ( 18.62759615963271287, -10.81492255796078972, 83.33224293864769550 ) ) ;
#54330=CARTESIAN_POINT ( 'NONE',  ( 4.379528057220339221, -16.55341960407611168, 52.70724293864769550 ) ) ;
#54331=CARTESIAN_POINT ( 'NONE',  ( 13.97604488694527802, 13.89961937509977652, 44.37390960531435269 ) ) ;
#54332=CARTESIAN_POINT ( 'NONE',  ( 8.224510206698953496, -14.34966873604960469, 67.91557627198102409 ) ) ;
#54333=CARTESIAN_POINT ( 'NONE',  ( 10.81492255796078972, 18.62759615963270932, 29.58224293864769905 ) ) ;
#54334=CARTESIAN_POINT ( 'NONE',  ( -21.55341960407610458, -5.719274019375992779, 26.45724293864768839 ) ) ;
#54335=CARTESIAN_POINT ( 'NONE',  ( 13.97604488694548053, -13.89961937509957401, 35.62609039468567573 ) ) ;
#54336=CARTESIAN_POINT ( 'NONE',  ( 8.224510206698953496, -14.34966873604960469, 97.91557627198103830 ) ) ;
#54337=CARTESIAN_POINT ( 'NONE',  ( 9.564922557960805705, 16.46253265017160317, 104.5822429386476955 ) ) ;
#54339=CARTESIAN_POINT ( 'NONE',  ( -8.224510206698735004, -14.34966873604973081, 59.58442372801901854 ) ) ;
#54340=CARTESIAN_POINT ( 'NONE',  ( 19.02544592524343514, -5.153800228976328945, 48.54057627198103120 ) ) ;
#54341=CARTESIAN_POINT ( 'NONE',  ( -17.26608964885399189, -6.138123030024978277, 21.29864325564489747 ) ) ;
#54342=CARTESIAN_POINT ( 'NONE',  ( -19.02544592524334988, -5.153800228976617603, 58.95942372801900433 ) ) ;
#54343=CARTESIAN_POINT ( 'NONE',  ( -14.34966873604972548, 8.224510206698743886, 98.33442372801901854 ) ) ;
#54344=CARTESIAN_POINT ( 'NONE',  ( -16.46253265017146816, -9.564922557961047289, 94.16775706135233293 ) ) ;
#54345=CARTESIAN_POINT ( 'NONE',  ( 15.80617190586769283, -15.72974639402175789, 65.62609039468568994 ) ) ;
#54346=CARTESIAN_POINT ( 'NONE',  ( -16.46253265017160317, 9.564922557960807481, 80.83224293864769550 ) ) ;
#54347=CARTESIAN_POINT ( 'NONE',  ( 18.62759615963271287, -10.81492255796078972, 93.33224293864769550 ) ) ;
#54348=CARTESIAN_POINT ( 'NONE',  ( -13.97604488694527625, -13.89961937509977652, 21.87390960531435979 ) ) ;
#54349=CARTESIAN_POINT ( 'NONE',  ( 19.05341960407617918, -5.049401038297876454, 76.04275706135230450 ) ) ;
#54350=CARTESIAN_POINT ( 'NONE',  ( -5.823673210054116645, -21.52544592524344225, 77.29057627198102409 ) ) ;
#54351=CARTESIAN_POINT ( 'NONE',  ( 16.46253265017146816, 9.564922557961045513, 41.66775706135234003 ) ) ;
#54352=CARTESIAN_POINT ( 'NONE',  ( 19.34837522270365895, 5.499999999999788614, 98.36337684832577111 ) ) ;
#54353=CARTESIAN_POINT ( 'NONE',  ( 15.72974639402199770, -15.80617190586745480, 88.12390960531436690 ) ) ;
#54354=CARTESIAN_POINT ( 'NONE',  ( 17.50000000000002132, 3.345213924137314887, 27.91231376905656347 ) ) ;
#54355=CARTESIAN_POINT ( 'NONE',  ( 9.474510206698971260, -16.51473224551069308, 67.91557627198102409 ) ) ;
#54357=CARTESIAN_POINT ( 'NONE',  ( -5.153800228976607833, 19.02544592524334988, 112.7094237280190043 ) ) ;
#54359=CARTESIAN_POINT ( 'NONE',  ( 16.46253265017160672, -9.564922557960803928, 43.33224293864769550 ) ) ;
#54360=CARTESIAN_POINT ( 'NONE',  ( -21.52544592524343514, 5.823673210054127303, 101.0405762719810383 ) ) ;
#54361=CARTESIAN_POINT ( 'NONE',  ( -14.29746914071049879, 8.314922557960819915, 55.83224293864770260 ) ) ;
#54362=CARTESIAN_POINT ( 'NONE',  ( 13.97604488694527802, 13.89961937509977652, 54.37390960531435979 ) ) ;
#54363=CARTESIAN_POINT ( 'NONE',  ( 15.80617190586769283, -15.72974639402175789, 75.62609039468567573 ) ) ;
#54364=CARTESIAN_POINT ( 'NONE',  ( 16.55341960407618274, -4.379528057220086978, 21.04275706135234714 ) ) ;
#54365=CARTESIAN_POINT ( 'NONE',  ( 9.474510206698729675, 16.51473224551082808, 32.08442372801900433 ) ) ;
#54366=CARTESIAN_POINT ( 'NONE',  ( 0.05219959533910956823, 16.53943276465976808, 24.99890960531435624 ) ) ;
#54367=CARTESIAN_POINT ( 'NONE',  ( 15.72974639402176855, 15.80617190586768217, 41.87609039468568284 ) ) ;
#54368=CARTESIAN_POINT ( 'NONE',  ( -18.62759615963270932, 10.81492255796079327, 115.8322429386477097 ) ) ;
#54369=CARTESIAN_POINT ( 'NONE',  ( -10.81492255796078084, -18.62759615963271287, 57.08224293864769550 ) ) ;
#54370=CARTESIAN_POINT ( 'NONE',  ( -19.05341960407617563, 5.049401038297882671, 98.54275706135233293 ) ) ;
#54371=CARTESIAN_POINT ( 'NONE',  ( 9.474510206698729675, 16.51473224551082808, 72.08442372801900433 ) ) ;
#54372=CARTESIAN_POINT ( 'NONE',  ( 21.52544592524334988, 5.823673210054432836, 71.45942372801901854 ) ) ;
#54373=CARTESIAN_POINT ( 'NONE',  ( 16.46253265017146816, 9.564922557961045513, 56.66775706135233293 ) ) ;
#54374=CARTESIAN_POINT ( 'NONE',  ( -19.02544592524342804, 5.153800228976336051, 26.04057627198103120 ) ) ;
#54375=CARTESIAN_POINT ( 'NONE',  ( -21.52544592524343514, 5.823673210054127303, 46.04057627198103830 ) ) ;
#54376=CARTESIAN_POINT ( 'NONE',  ( -4.483927247898539470, -16.52544592524342804, 52.29057627198102409 ) ) ;
#54377=CARTESIAN_POINT ( 'NONE',  ( -18.22780087662122028, 5.500000000000031086, 93.51540105326107266 ) ) ;
#54378=CARTESIAN_POINT ( 'NONE',  ( -5.719274019375665041, -21.55341960407619695, 109.7927570613523613 ) ) ;
#54379=CARTESIAN_POINT ( 'NONE',  ( 16.52544592524335698, 4.483927247898782831, 91.45942372801901854 ) ) ;
#54380=CARTESIAN_POINT ( 'NONE',  ( -16.55341960407611168, -4.379528057220339221, 41.45724293864769550 ) ) ;
#54381=CARTESIAN_POINT ( 'NONE',  ( -5.823673210054431948, 21.52544592524334988, 72.70942372801901854 ) ) ;
#54382=CARTESIAN_POINT ( 'NONE',  ( -5.719274019375665041, -21.55341960407619695, 74.79275706135234714 ) ) ;
#54383=CARTESIAN_POINT ( 'NONE',  ( 21.53943276465977519, -0.05219959533907433946, 83.74890960531435269 ) ) ;
#54384=CARTESIAN_POINT ( 'NONE',  ( 19.03943276465977164, -0.05219959533909143690, 38.74890960531436690 ) ) ;
#54385=CARTESIAN_POINT ( 'NONE',  ( -5.823673210054431948, 21.52544592524334988, 62.70942372801902565 ) ) ;
#54386=CARTESIAN_POINT ( 'NONE',  ( 5.049401038298161559, -19.05341960407611168, 32.70724293864768129 ) ) ;
#54387=CARTESIAN_POINT ( 'NONE',  ( 19.03943276465977164, -0.05219959533909143690, 58.74890960531435979 ) ) ;
#54388=CARTESIAN_POINT ( 'NONE',  ( 14.34966873604960469, 8.224510206698951720, 99.16557627198100988 ) ) ;
#54389=CARTESIAN_POINT ( 'NONE',  ( -0.05219959533909027116, -19.03943276465977164, 97.49890960531436690 ) ) ;
#54390=CARTESIAN_POINT ( 'NONE',  ( 14.34966873604960469, 8.224510206698951720, 34.16557627198102409 ) ) ;
#54391=CARTESIAN_POINT ( 'NONE',  ( 16.46253265017160672, -9.564922557960803928, 23.33224293864769194 ) ) ;
#54392=CARTESIAN_POINT ( 'NONE',  ( 18.62759615963271287, -10.81492255796078972, 83.33224293864769550 ) ) ;
#54393=CARTESIAN_POINT ( 'NONE',  ( 15.72974639402176855, 15.80617190586768217, 26.87609039468567218 ) ) ;
#54396=CARTESIAN_POINT ( 'NONE',  ( -19.05341960407617563, 5.049401038297882671, 113.5427570613523471 ) ) ;
#54397=CARTESIAN_POINT ( 'NONE',  ( 5.719274019375991003, -21.55341960407610458, 72.70724293864769550 ) ) ;
#54398=CARTESIAN_POINT ( 'NONE',  ( -18.62759615963255300, -10.81492255796106328, 89.16775706135236135 ) ) ;
#54399=CARTESIAN_POINT ( 'NONE',  ( 16.51473224551069308, 9.474510206698969483, 84.16557627198102409 ) ) ;
#54400=CARTESIAN_POINT ( 'NONE',  ( 18.62759615963255655, 10.81492255796105972, 36.66775706135234714 ) ) ;
#54401=CARTESIAN_POINT ( 'NONE',  ( -9.474510206698964154, 16.51473224551069663, 115.4155762719810241 ) ) ;
#54402=CARTESIAN_POINT ( 'NONE',  ( -14.34966873604972548, 8.224510206698743886, 88.33442372801901854 ) ) ;
#54403=CARTESIAN_POINT ( 'NONE',  ( 5.823673210054444382, -21.52544592524334988, 75.20942372801901854 ) ) ;
#54404=CARTESIAN_POINT ( 'NONE',  ( 16.51473224551083163, -9.474510206698727899, 20.83442372801899722 ) ) ;
#54405=CARTESIAN_POINT ( 'NONE',  ( -16.52544592524335698, -4.483927247898792601, 73.95942372801901854 ) ) ;
#54406=CARTESIAN_POINT ( 'NONE',  ( 21.52544592524334988, 5.823673210054432836, 31.45942372801901854 ) ) ;
#54407=CARTESIAN_POINT ( 'NONE',  ( 13.89961937509977652, -13.97604488694527269, 38.12390960531436690 ) ) ;
#54408=CARTESIAN_POINT ( 'NONE',  ( 5.719274019375673035, 21.55341960407619339, 87.29275706135236135 ) ) ;
#54409=CARTESIAN_POINT ( 'NONE',  ( 9.564922557960805705, 16.46253265017160317, 89.58224293864769550 ) ) ;
#54410=CARTESIAN_POINT ( 'NONE',  ( 5.823673210054125526, 21.52544592524343514, 109.7905762719810383 ) ) ;
#54411=CARTESIAN_POINT ( 'NONE',  ( 19.39720447994794483, 5.499999999999967137, 82.16317477297172900 ) ) ;
#54412=CARTESIAN_POINT ( 'NONE',  ( -18.62759615963270932, 10.81492255796079327, 50.83224293864770971 ) ) ;
#54413=CARTESIAN_POINT ( 'NONE',  ( 5.049401038298161559, -19.05341960407611168, 92.70724293864769550 ) ) ;
#54414=CARTESIAN_POINT ( 'NONE',  ( -8.224510206698948167, 14.34966873604960824, 45.41557627198103830 ) ) ;
#54416=CARTESIAN_POINT ( 'NONE',  ( -9.474510206698720793, -16.51473224551083518, 79.58442372801899012 ) ) ;
#54420=CARTESIAN_POINT ( 'NONE',  ( -5.049401038297874678, -19.05341960407617918, 104.7927570613523471 ) ) ;
#54421=CARTESIAN_POINT ( 'NONE',  ( 10.72451020669898902, -18.67979575497178502, 82.91557627198103830 ) ) ;
#54422=CARTESIAN_POINT ( 'NONE',  ( 16.52544592524342804, -4.483927247898539470, 68.54057627198103830 ) ) ;
#54423=CARTESIAN_POINT ( 'NONE',  ( -16.51473224551069308, -9.474510206698971260, 101.6655762719810241 ) ) ;
#54424=CARTESIAN_POINT ( 'NONE',  ( -12.06949235617739369, -12.14591786802326823, 49.37609039468569705 ) ) ;
#54425=CARTESIAN_POINT ( 'NONE',  ( -5.153800228976328057, -19.02544592524343514, 62.29057627198100988 ) ) ;
#54426=CARTESIAN_POINT ( 'NONE',  ( 18.62759615963255655, 10.81492255796105972, 31.66775706135234358 ) ) ;
#54427=CARTESIAN_POINT ( 'NONE',  ( 0.05219959533936267826, -19.03943276465977164, 95.00109039468567573 ) ) ;
#54428=CARTESIAN_POINT ( 'NONE',  ( 13.97604488694527802, 13.89961937509977652, 99.37390960531436690 ) ) ;
#54429=CARTESIAN_POINT ( 'NONE',  ( -19.05341960407611168, -5.049401038298163336, 91.45724293864766707 ) ) ;
#54430=CARTESIAN_POINT ( 'NONE',  ( -21.53943276465977519, 0.05219959533907696930, 86.24890960531436690 ) ) ;
#54431=CARTESIAN_POINT ( 'NONE',  ( -5.049401038298153566, 19.05341960407611168, 40.20724293864768839 ) ) ;
#54433=CARTESIAN_POINT ( 'NONE',  ( 8.224510206698953496, -14.34966873604960469, 67.91557627198102409 ) ) ;
#54434=CARTESIAN_POINT ( 'NONE',  ( -0.05219959533909027116, -19.03943276465977164, 107.4989096053143527 ) ) ;
#54436=CARTESIAN_POINT ( 'NONE',  ( 19.02544592524334988, 5.153800228976608722, 61.45942372801900433 ) ) ;
#54437=CARTESIAN_POINT ( 'NONE',  ( -21.53943276465977519, 0.05219959533907696930, 96.24890960531435269 ) ) ;
#54438=CARTESIAN_POINT ( 'NONE',  ( -5.153800228976607833, 19.02544592524334988, 52.70942372801900433 ) ) ;
#54439=CARTESIAN_POINT ( 'NONE',  ( -19.05341960407611168, -5.049401038298163336, 96.45724293864769550 ) ) ;
#54440=CARTESIAN_POINT ( 'NONE',  ( 5.719274019375991003, -21.55341960407610458, 37.70724293864769550 ) ) ;
#54441=CARTESIAN_POINT ( 'NONE',  ( -19.05341960407611168, -5.049401038298163336, 81.45724293864769550 ) ) ;
#54442=B_SPLINE_CURVE_WITH_KNOTS ( 'NONE', 3,
 ( #71671, #11008, #53498, #41343, #24184, #86835, #69671, #117172, #38337, #162678, #99993, #85834 ),
 .UNSPECIFIED., .F., .F.,
 ( 4, 2, 2, 2, 2, 4 ),
 ( 2.112163857337007370E-17, 0.001213821615218632025, 0.001820732422827935895, 0.002124187826632588372, 0.002275915528534913634, 0.002427643230437238463 ),
 .UNSPECIFIED. ) ;
#54443=CARTESIAN_POINT ( 'NONE',  ( -18.62759615963255300, -10.81492255796106328, 64.16775706135234714 ) ) ;
#54444=CARTESIAN_POINT ( 'NONE',  ( 5.153800228976335163, 19.02544592524342804, 39.79057627198100988 ) ) ;
#54445=CARTESIAN_POINT ( 'NONE',  ( 4.483927247898545687, 16.52544592524342804, 69.79057627198102409 ) ) ;
#54446=CARTESIAN_POINT ( 'NONE',  ( -16.51473224551082808, 9.474510206698731452, 113.3344237280190043 ) ) ;
#54447=CARTESIAN_POINT ( 'NONE',  ( -18.67979575497193778, 10.72451020669871902, 53.33442372801901854 ) ) ;
#54450=CARTESIAN_POINT ( 'NONE',  ( 19.02544592524334988, 5.153800228976608722, 61.45942372801900433 ) ) ;
#54452=CARTESIAN_POINT ( 'NONE',  ( -10.81492255796105439, 18.62759615963255655, 27.91775706135234358 ) ) ;
#54453=CARTESIAN_POINT ( 'NONE',  ( -5.153800228976328057, -19.02544592524343514, 57.29057627198103120 ) ) ;
#54455=CARTESIAN_POINT ( 'NONE',  ( -19.05341960407617563, 5.049401038297882671, 23.54275706135233648 ) ) ;
#54456=CARTESIAN_POINT ( 'NONE',  ( 16.46253265017160672, -9.564922557960803928, 48.33224293864769550 ) ) ;
#54457=CARTESIAN_POINT ( 'NONE',  ( 21.55341960407619695, -5.719274019375665929, 106.0427570613523471 ) ) ;
#54458=CARTESIAN_POINT ( 'NONE',  ( -16.55341960407617563, 4.379528057220093196, 88.54275706135236135 ) ) ;
#54459=CARTESIAN_POINT ( 'NONE',  ( -13.89961937509977652, 13.97604488694528158, 100.6239096053143669 ) ) ;
#54460=CARTESIAN_POINT ( 'NONE',  ( -21.52544592524334988, -5.823673210054445271, 78.95942372801901854 ) ) ;
#54462=CARTESIAN_POINT ( 'NONE',  ( -0.05219959533909027116, -19.03943276465977164, 112.4989096053143669 ) ) ;
#54464=CARTESIAN_POINT ( 'NONE',  ( -16.52544592524335698, -4.483927247898792601, 63.95942372801901854 ) ) ;
#54465=CARTESIAN_POINT ( 'NONE',  ( -10.81492255796105439, 18.62759615963255655, 67.91775706135234714 ) ) ;
#54466=CARTESIAN_POINT ( 'NONE',  ( 5.719274019375673035, 21.55341960407619339, 102.2927570613523613 ) ) ;
#54468=CARTESIAN_POINT ( 'NONE',  ( -13.89961937509977652, 13.97604488694528158, 80.62390960531436690 ) ) ;
#54469=CARTESIAN_POINT ( 'NONE',  ( 13.89961937509977652, -13.97604488694527269, 113.1239096053143527 ) ) ;
#54472=CARTESIAN_POINT ( 'NONE',  ( -9.474510206698964154, 16.51473224551069663, 45.41557627198103120 ) ) ;
#54473=CARTESIAN_POINT ( 'NONE',  ( -0.05219959533907301413, -21.53943276465977519, 37.49890960531436690 ) ) ;
#54474=CARTESIAN_POINT ( 'NONE',  ( -4.379528057220086978, -16.55341960407618274, 99.79275706135234714 ) ) ;
#54475=CARTESIAN_POINT ( 'NONE',  ( 14.29746914071049879, -8.314922557960816363, 88.33224293864769550 ) ) ;
#54476=CARTESIAN_POINT ( 'NONE',  ( -9.474510206698964154, 16.51473224551069663, 80.41557627198103830 ) ) ;
#54477=CARTESIAN_POINT ( 'NONE',  ( 5.823673210054444382, -21.52544592524334988, 105.2094237280190328 ) ) ;
#54478=CARTESIAN_POINT ( 'NONE',  ( -5.049401038298153566, 19.05341960407611168, 40.20724293864768839 ) ) ;
#54479=CARTESIAN_POINT ( 'NONE',  ( 4.483927247898545687, 16.52544592524342804, 84.79057627198102409 ) ) ;
#54480=CARTESIAN_POINT ( 'NONE',  ( -18.67979575497193778, 10.72451020669871902, 38.33442372801900433 ) ) ;
#54481=CARTESIAN_POINT ( 'NONE',  ( -5.719274019375978568, 21.55341960407610458, 90.20724293864770971 ) ) ;
#54482=CARTESIAN_POINT ( 'NONE',  ( -5.049401038297874678, -19.05341960407617918, 44.79275706135232582 ) ) ;
#54484=CARTESIAN_POINT ( 'NONE',  ( 19.05341960407611168, 5.049401038298154454, 93.95724293864769550 ) ) ;
#54485=CARTESIAN_POINT ( 'NONE',  ( -12.14591786802309592, -12.06949235617757132, 56.87390960531436690 ) ) ;
#54486=CARTESIAN_POINT ( 'NONE',  ( 4.379528057220339221, -16.55341960407611168, 52.70724293864769550 ) ) ;
#54487=CARTESIAN_POINT ( 'NONE',  ( -19.05341960407617563, 5.049401038297882671, 83.54275706135233293 ) ) ;
#54488=CARTESIAN_POINT ( 'NONE',  ( -18.87580814761075132, 5.500000000000055067, 85.87172394265761000 ) ) ;
#54489=CARTESIAN_POINT ( 'NONE',  ( 18.67979575497178502, 10.72451020669898547, 29.16557627198103120 ) ) ;
#54490=CARTESIAN_POINT ( 'NONE',  ( 14.34966873604960469, 8.224510206698951720, 89.16557627198102409 ) ) ;
#54492=CARTESIAN_POINT ( 'NONE',  ( 9.474510206698971260, -16.51473224551069308, 47.91557627198102409 ) ) ;
#54493=CARTESIAN_POINT ( 'NONE',  ( 10.81492255796078972, 18.62759615963270932, 49.58224293864769550 ) ) ;
#54494=CARTESIAN_POINT ( 'NONE',  ( -0.05219959533909027116, -19.03943276465977164, 32.49890960531435979 ) ) ;
#54495=CARTESIAN_POINT ( 'NONE',  ( -12.06949235617739369, -12.14591786802326823, 84.37609039468570415 ) ) ;
#54496=CARTESIAN_POINT ( 'NONE',  ( -19.05341960407611168, -5.049401038298163336, 66.45724293864769550 ) ) ;
#54497=CARTESIAN_POINT ( 'NONE',  ( -16.46253265017146816, -9.564922557961047289, 34.16775706135233293 ) ) ;
#54498=CARTESIAN_POINT ( 'NONE',  ( 21.53943276465977519, 0.05219959533937863772, 66.25109039468567573 ) ) ;
#54499=CARTESIAN_POINT ( 'NONE',  ( 21.55341960407610458, 5.719274019375980345, 38.95724293864768839 ) ) ;
#54500=CARTESIAN_POINT ( 'NONE',  ( 16.55341960407611168, 4.379528057220329451, 98.95724293864770971 ) ) ;
#54501=CARTESIAN_POINT ( 'NONE',  ( 9.474510206698729675, 16.51473224551082808, 92.08442372801900433 ) ) ;
#54504=CARTESIAN_POINT ( 'NONE',  ( -21.52544592524343514, 5.823673210054127303, 41.04057627198103120 ) ) ;
#54505=CARTESIAN_POINT ( 'NONE',  ( 17.12812012977026654, -6.668231424566044119, 66.14051240676859322 ) ) ;
#54506=CARTESIAN_POINT ( 'NONE',  ( 15.72974639402176855, 15.80617190586768217, 86.87609039468568994 ) ) ;
#54507=CARTESIAN_POINT ( 'NONE',  ( 16.55341960407611168, 4.379528057220329451, 43.95724293864769550 ) ) ;
#54508=CARTESIAN_POINT ( 'NONE',  ( 4.483927247898790824, -16.52544592524335698, 70.20942372801904696 ) ) ;
#54509=CARTESIAN_POINT ( 'NONE',  ( -8.314922557960811034, -14.29746914071050412, 52.08224293864768839 ) ) ;
#54510=CARTESIAN_POINT ( 'NONE',  ( 5.719274019375991003, -21.55341960407610458, 87.70724293864769550 ) ) ;
#54511=CARTESIAN_POINT ( 'NONE',  ( 18.62759615963271287, -10.81492255796078972, 73.33224293864769550 ) ) ;
#54513=CARTESIAN_POINT ( 'NONE',  ( 5.823673210054125526, 21.52544592524343514, 29.79057627198102409 ) ) ;
#54514=CARTESIAN_POINT ( 'NONE',  ( 0.05219959533934541429, -16.53943276465976808, 55.00109039468568284 ) ) ;
#54515=CARTESIAN_POINT ( 'NONE',  ( -4.379528057220328563, 16.55341960407611168, 75.20724293864769550 ) ) ;
#54516=B_SPLINE_CURVE_WITH_KNOTS ( 'NONE', 3,
 ( #113224, #174914, #115232, #101050, #178925, #69727, #148577, #176923, #100050, #85892, #159729, #37387, #40395, #116231, #161736, #23231, #128388, #146552, #177922, #114211, #131395, #190084, #25251, #36378, #193083, #21225, #144559, #54558, #6045, #67723, #163751, #175916 ),
 .UNSPECIFIED., .F., .F.,
 ( 4, 2, 2, 2, 2, 2, 2, 2, 2, 2, 2, 2, 2, 2, 2, 4 ),
 ( 2.711112516444420852E-17, 0.0003712461730037035289, 0.0007424923460073799527, 0.001113738519011056322, 0.001484984692014732800, 0.002227477038022085756, 0.002598723211025761801, 0.002969969384029437845, 0.003341215557033113889, 0.003712461730036789066, 0.004083707903040465111, 0.004454954076044140288, 0.004826200249047816332, 0.005197446422051492376, 0.005568692595055167553, 0.005939938768058842730 ),
 .UNSPECIFIED. ) ;
#54517=CARTESIAN_POINT ( 'NONE',  ( 19.05341960407611168, 5.049401038298154454, 63.95724293864769550 ) ) ;
#54518=CARTESIAN_POINT ( 'NONE',  ( 19.02544592524343514, -5.153800228976328945, 33.54057627198102409 ) ) ;
#54519=CARTESIAN_POINT ( 'NONE',  ( 17.72662750342723825, 5.500000000000073719, 48.90179492283744622 ) ) ;
#54520=CARTESIAN_POINT ( 'NONE',  ( 14.29746914071037800, 8.314922557961029526, 76.66775706135234714 ) ) ;
#54521=CARTESIAN_POINT ( 'NONE',  ( -0.05219959533937732626, 21.53943276465977519, 22.50109039468567573 ) ) ;
#54522=CARTESIAN_POINT ( 'NONE',  ( -19.02544592524342804, 5.153800228976336051, 71.04057627198099567 ) ) ;
#54523=CARTESIAN_POINT ( 'NONE',  ( 15.72974639402176855, 15.80617190586768217, 51.87609039468568284 ) ) ;
#54524=CARTESIAN_POINT ( 'NONE',  ( 0.05219959533909260263, 19.03943276465977164, 109.9989096053143669 ) ) ;
#54527=CARTESIAN_POINT ( 'NONE',  ( -15.80617190586768217, 15.72974639402176855, 48.12609039468568284 ) ) ;
#54528=CARTESIAN_POINT ( 'NONE',  ( 5.153800228976335163, 19.02544592524342804, 114.7905762719810241 ) ) ;
#54529=CARTESIAN_POINT ( 'NONE',  ( 19.05341960407611168, 5.049401038298154454, 98.95724293864766707 ) ) ;
#54530=CARTESIAN_POINT ( 'NONE',  ( -5.049401038297874678, -19.05341960407617918, 54.79275706135234003 ) ) ;
#54531=CARTESIAN_POINT ( 'NONE',  ( -5.719274019375665041, -21.55341960407619695, 19.79275706135235069 ) ) ;
#54532=CARTESIAN_POINT ( 'NONE',  ( 16.51473224551083163, -9.474510206698727899, 40.83442372801900433 ) ) ;
#54533=CARTESIAN_POINT ( 'NONE',  ( -19.03943276465977164, -0.05219959533935918106, 48.75109039468566863 ) ) ;
#54534=CARTESIAN_POINT ( 'NONE',  ( -12.06949235617739369, -12.14591786802326823, 104.3760903946856899 ) ) ;
#54536=CARTESIAN_POINT ( 'NONE',  ( 0.05219959533909260263, 19.03943276465977164, 89.99890960531436690 ) ) ;
#54537=CARTESIAN_POINT ( 'NONE',  ( 15.80617190586769283, -15.72974639402175789, 90.62609039468567573 ) ) ;
#54538=CARTESIAN_POINT ( 'NONE',  ( -10.72451020669870658, -18.67979575497194134, 89.58442372801901854 ) ) ;
#54540=CARTESIAN_POINT ( 'NONE',  ( 5.049401038298161559, -19.05341960407611168, 107.7072429386476955 ) ) ;
#54541=CARTESIAN_POINT ( 'NONE',  ( -15.72974639402176322, -15.80617190586768395, 74.37609039468568994 ) ) ;
#54542=CARTESIAN_POINT ( 'NONE',  ( -19.05341960407617563, 5.049401038297882671, 108.5427570613523187 ) ) ;
#54543=CARTESIAN_POINT ( 'NONE',  ( 5.153800228976335163, 19.02544592524342804, 74.79057627198103830 ) ) ;
#54544=CARTESIAN_POINT ( 'NONE',  ( -10.72451020669898014, 18.67979575497178502, 25.41557627198103120 ) ) ;
#54545=CARTESIAN_POINT ( 'NONE',  ( 9.474510206698971260, -16.51473224551069308, 92.91557627198103830 ) ) ;
#54546=CARTESIAN_POINT ( 'NONE',  ( 5.049401038297881783, 19.05341960407617918, 87.29275706135234714 ) ) ;
#54547=CARTESIAN_POINT ( 'NONE',  ( 19.02544592524343514, -5.153800228976328945, 73.54057627198103830 ) ) ;
#54548=CARTESIAN_POINT ( 'NONE',  ( 16.51473224551069308, 9.474510206698969483, 69.16557627198102409 ) ) ;
#54549=CARTESIAN_POINT ( 'NONE',  ( 21.53943276465977519, -0.05219959533907433946, 108.7489096053143669 ) ) ;
#54550=CARTESIAN_POINT ( 'NONE',  ( 4.379528057220092307, 16.55341960407617563, 107.2927570613523471 ) ) ;
#54552=CARTESIAN_POINT ( 'NONE',  ( -9.564922557961040184, 16.46253265017147172, 52.91775706135233293 ) ) ;
#54553=CARTESIAN_POINT ( 'NONE',  ( -19.03943276465977164, 0.05219959533909376836, 91.24890960531436690 ) ) ;
#54554=CARTESIAN_POINT ( 'NONE',  ( -14.29746914071049879, 8.314922557960819915, 80.83224293864769550 ) ) ;
#54555=CARTESIAN_POINT ( 'NONE',  ( 18.67979575497178502, 10.72451020669898547, 34.16557627198102409 ) ) ;
#54556=CARTESIAN_POINT ( 'NONE',  ( 21.52544592524344225, -5.823673210054117533, 28.54057627198103120 ) ) ;
#54557=CARTESIAN_POINT ( 'NONE',  ( -0.05219959533910754901, -16.53943276465976808, 97.49890960531436690 ) ) ;
#54558=CARTESIAN_POINT ( 'NONE',  ( -17.40861289039004234, 6.110651285853259118, 53.62767529172569425 ) ) ;
#54559=CARTESIAN_POINT ( 'NONE',  ( -16.46253265017146816, -9.564922557961047289, 49.16775706135233293 ) ) ;
#54560=CARTESIAN_POINT ( 'NONE',  ( -16.53943276465976808, -0.05219959533934237506, 103.7510903946857042 ) ) ;
#54561=CARTESIAN_POINT ( 'NONE',  ( 13.89961937509977652, -13.97604488694527269, 93.12390960531436690 ) ) ;
#54563=CARTESIAN_POINT ( 'NONE',  ( -5.823673210054431948, 21.52544592524334988, 72.70942372801901854 ) ) ;
#54564=CARTESIAN_POINT ( 'NONE',  ( -15.72974639402197994, 15.80617190586746368, 55.62390960531436690 ) ) ;
#54565=CARTESIAN_POINT ( 'NONE',  ( -10.72451020669870658, -18.67979575497194134, 29.58442372801901854 ) ) ;
#54566=CARTESIAN_POINT ( 'NONE',  ( 21.52544592524344225, -5.823673210054117533, 83.54057627198102409 ) ) ;
#54567=CARTESIAN_POINT ( 'NONE',  ( 12.14591786802309770, 12.06949235617756955, 109.3739096053143811 ) ) ;
#54568=CARTESIAN_POINT ( 'NONE',  ( -19.02544592524334988, -5.153800228976617603, 68.95942372801896170 ) ) ;
#54569=CARTESIAN_POINT ( 'NONE',  ( 13.89961937509977652, -13.97604488694527269, 43.12390960531434558 ) ) ;
#54570=CARTESIAN_POINT ( 'NONE',  ( -16.51473224551069308, -9.474510206698971260, 96.66557627198102409 ) ) ;
#54571=CARTESIAN_POINT ( 'NONE',  ( 16.51473224551069308, 9.474510206698969483, 99.16557627198102409 ) ) ;
#54572=CARTESIAN_POINT ( 'NONE',  ( 13.89961937509977652, -13.97604488694527269, 23.12390960531436335 ) ) ;
#54573=CARTESIAN_POINT ( 'NONE',  ( -12.14591786802309592, -12.06949235617757132, 46.87390960531435979 ) ) ;
#54574=CARTESIAN_POINT ( 'NONE',  ( 8.314922557961029526, -14.29746914071037800, 45.41775706135234003 ) ) ;
#54575=CARTESIAN_POINT ( 'NONE',  ( 5.719274019375673035, 21.55341960407619339, 102.2927570613523613 ) ) ;
#54577=CARTESIAN_POINT ( 'NONE',  ( -4.379528057220328563, 16.55341960407611168, 25.20724293864769550 ) ) ;
#54578=CARTESIAN_POINT ( 'NONE',  ( -15.80617190586768217, 15.72974639402176855, 38.12609039468567573 ) ) ;
#54579=CARTESIAN_POINT ( 'NONE',  ( -19.02544592524342804, 5.153800228976336051, 101.0405762719810241 ) ) ;
#54580=CARTESIAN_POINT ( 'NONE',  ( -0.05219959533934338120, 16.53943276465976808, 102.5010903946856899 ) ) ;
#54581=CARTESIAN_POINT ( 'NONE',  ( -14.34966873604972548, 8.224510206698743886, 93.33442372801901854 ) ) ;
#54582=CARTESIAN_POINT ( 'NONE',  ( 4.379528057220092307, 16.55341960407617563, 27.29275706135234358 ) ) ;
#54583=CARTESIAN_POINT ( 'NONE',  ( 9.564922557960805705, 16.46253265017160317, 54.58224293864769550 ) ) ;
#54584=CARTESIAN_POINT ( 'NONE',  ( 16.55341960407611168, 4.379528057220329451, 113.9572429386477239 ) ) ;
#54585=CARTESIAN_POINT ( 'NONE',  ( -10.81492255796105439, 18.62759615963255655, 22.91775706135235069 ) ) ;
#54586=CARTESIAN_POINT ( 'NONE',  ( -9.564922557960796823, -16.46253265017161027, 27.08224293864769550 ) ) ;
#54587=CARTESIAN_POINT ( 'NONE',  ( -9.474510206698964154, 16.51473224551069663, 105.4155762719810383 ) ) ;
#54588=CARTESIAN_POINT ( 'NONE',  ( 19.02544592524343514, -5.153800228976328945, 38.54057627198103120 ) ) ;
#54589=CARTESIAN_POINT ( 'NONE',  ( 5.153800228976335163, 19.02544592524342804, 109.7905762719810099 ) ) ;
#54591=CARTESIAN_POINT ( 'NONE',  ( -16.51473224551069308, -9.474510206698971260, 91.66557627198103830 ) ) ;
#54592=CARTESIAN_POINT ( 'NONE',  ( 15.72974639402176855, 15.80617190586768217, 51.87609039468568284 ) ) ;
#54593=CARTESIAN_POINT ( 'NONE',  ( 4.379528057220339221, -16.55341960407611168, 97.70724293864772392 ) ) ;
#54594=CARTESIAN_POINT ( 'NONE',  ( 19.02544592524343514, -5.153800228976328945, 93.54057627198102409 ) ) ;
#54595=CARTESIAN_POINT ( 'NONE',  ( 17.50000000000000000, -5.499999999999992895, 96.21769037696437010 ) ) ;
#54596=CARTESIAN_POINT ( 'NONE',  ( 8.314922557961029526, -14.29746914071037800, 65.41775706135234714 ) ) ;
#54597=CARTESIAN_POINT ( 'NONE',  ( -5.823673210054431948, 21.52544592524334988, 82.70942372801900433 ) ) ;
#54598=CARTESIAN_POINT ( 'NONE',  ( -8.224510206698735004, -14.34966873604973081, 44.58442372801901854 ) ) ;
#54599=CARTESIAN_POINT ( 'NONE',  ( 19.02544592524343514, -5.153800228976328945, 88.54057627198102409 ) ) ;
#54600=CARTESIAN_POINT ( 'NONE',  ( 9.564922557961047289, -16.46253265017146816, 110.4177570613523471 ) ) ;
#54601=CARTESIAN_POINT ( 'NONE',  ( 8.314922557961029526, -14.29746914071037800, 80.41775706135234714 ) ) ;
#54602=CARTESIAN_POINT ( 'NONE',  ( 5.049401038297881783, 19.05341960407617563, 97.29275706135233293 ) ) ;
#54603=CARTESIAN_POINT ( 'NONE',  ( 9.474510206698971260, -16.51473224551069308, 62.91557627198102409 ) ) ;
#54604=CARTESIAN_POINT ( 'NONE',  ( 21.52544592524344225, -5.823673210054117533, 103.5405762719810383 ) ) ;
#54605=CARTESIAN_POINT ( 'NONE',  ( -14.29746914071049879, 8.314922557960819915, 95.83224293864770971 ) ) ;
#54606=CARTESIAN_POINT ( 'NONE',  ( 19.02544592524334988, 5.153800228976608722, 86.45942372801900433 ) ) ;
#54607=CARTESIAN_POINT ( 'NONE',  ( -16.55341960407617563, 4.379528057220093196, 58.54275706135235424 ) ) ;
#54608=CARTESIAN_POINT ( 'NONE',  ( 17.40805194822033997, -6.112264579159251809, 63.33371272510615313 ) ) ;
#54609=CARTESIAN_POINT ( 'NONE',  ( -0.05219959533936034679, 19.03943276465977164, 57.50109039468566863 ) ) ;
#54610=CARTESIAN_POINT ( 'NONE',  ( -16.55341960407611168, -4.379528057220339221, 31.45724293864769550 ) ) ;
#54611=CARTESIAN_POINT ( 'NONE',  ( 16.53943276465976808, -0.05219959533910856209, 78.74890960531436690 ) ) ;
#54612=CARTESIAN_POINT ( 'NONE',  ( -0.05219959533937732626, 21.53943276465977519, 112.5010903946857042 ) ) ;
#54613=CARTESIAN_POINT ( 'NONE',  ( -21.55341960407619339, 5.719274019375674811, 23.54275706135235424 ) ) ;
#54615=CARTESIAN_POINT ( 'NONE',  ( -13.97604488694527625, -13.89961937509977652, 81.87390960531436690 ) ) ;
#54616=CARTESIAN_POINT ( 'NONE',  ( -10.81492255796105439, 18.62759615963255655, 92.91775706135236135 ) ) ;
#54617=CARTESIAN_POINT ( 'NONE',  ( -9.564922557960796823, -16.46253265017161027, 72.08224293864770971 ) ) ;
#54618=CARTESIAN_POINT ( 'NONE',  ( 21.52544592524344225, -5.823673210054117533, 48.54057627198103120 ) ) ;
#54619=CARTESIAN_POINT ( 'NONE',  ( -4.483927247898539470, -16.52544592524342804, 82.29057627198103830 ) ) ;
#54620=CARTESIAN_POINT ( 'NONE',  ( 19.03943276465977164, -0.05219959533909143690, 53.74890960531436690 ) ) ;
#54621=CARTESIAN_POINT ( 'NONE',  ( -8.224510206698948167, 14.34966873604960824, 105.4155762719810383 ) ) ;
#54622=CARTESIAN_POINT ( 'NONE',  ( 0.05219959533937995610, -21.53943276465977519, 25.00109039468567218 ) ) ;
#54623=CARTESIAN_POINT ( 'NONE',  ( 15.72974639402176855, 15.80617190586768217, 56.87609039468568994 ) ) ;
#54624=CARTESIAN_POINT ( 'NONE',  ( 5.049401038298161559, -19.05341960407611168, 47.70724293864770260 ) ) ;
#54626=CARTESIAN_POINT ( 'NONE',  ( 8.224510206698742110, 14.34966873604972548, 82.08442372801901854 ) ) ;
#54627=CARTESIAN_POINT ( 'NONE',  ( 10.81492255796078972, 18.62759615963270932, 114.5822429386477097 ) ) ;
#54628=CARTESIAN_POINT ( 'NONE',  ( 15.80617190586746368, 15.72974639402197994, 104.3739096053143669 ) ) ;
#54629=CARTESIAN_POINT ( 'NONE',  ( -9.474510206698720793, -16.51473224551083518, 34.58442372801899722 ) ) ;
#54630=CARTESIAN_POINT ( 'NONE',  ( 0.05219959533909260263, 19.03943276465977164, 69.99890960531435269 ) ) ;
#54631=CARTESIAN_POINT ( 'NONE',  ( 19.03943276465977164, 0.05219959533936151252, 36.25109039468567573 ) ) ;
#54632=CARTESIAN_POINT ( 'NONE',  ( -10.81492255796105439, 18.62759615963255655, 67.91775706135234714 ) ) ;
#54633=CARTESIAN_POINT ( 'NONE',  ( -5.719274019375978568, 21.55341960407610458, 50.20724293864769550 ) ) ;
#54634=CARTESIAN_POINT ( 'NONE',  ( 4.379528057220339221, -16.55341960407611168, 42.70724293864770260 ) ) ;
#54635=CARTESIAN_POINT ( 'NONE',  ( 5.823673210054444382, -21.52544592524334988, 85.20942372801901854 ) ) ;
#54636=CARTESIAN_POINT ( 'NONE',  ( -9.474510206698720793, -16.51473224551083518, 19.58442372801899722 ) ) ;
#54637=CARTESIAN_POINT ( 'NONE',  ( 8.314922557960818139, 14.29746914071049879, 54.58224293864769550 ) ) ;
#54638=CARTESIAN_POINT ( 'NONE',  ( 16.55341960407611168, 4.379528057220329451, 108.9572429386476955 ) ) ;
#54639=CARTESIAN_POINT ( 'NONE',  ( 19.02544592524334988, 5.153800228976608722, 61.45942372801900433 ) ) ;
#54640=CARTESIAN_POINT ( 'NONE',  ( -16.55341960407611168, -4.379528057220339221, 21.45724293864769550 ) ) ;
#54641=CARTESIAN_POINT ( 'NONE',  ( -5.823673210054431948, 21.52544592524334988, 62.70942372801902565 ) ) ;
#54642=CARTESIAN_POINT ( 'NONE',  ( -0.05219959533909027116, -19.03943276465977164, 72.49890960531435269 ) ) ;
#54643=CARTESIAN_POINT ( 'NONE',  ( 13.89961937509957401, 13.97604488694547697, 31.87609039468566863 ) ) ;
#54644=CARTESIAN_POINT ( 'NONE',  ( 0.05219959533907565091, 21.53943276465977519, 49.99890960531437401 ) ) ;
#54645=CARTESIAN_POINT ( 'NONE',  ( 5.823673210054444382, -21.52544592524334988, 40.20942372801901854 ) ) ;
#54646=VECTOR ( 'NONE', #176066, 1000.000000000000000 ) ;
#54647=CARTESIAN_POINT ( 'NONE',  ( -5.719274019375978568, 21.55341960407610458, 105.2072429386477097 ) ) ;
#54648=CARTESIAN_POINT ( 'NONE',  ( 19.05341960407617918, -5.049401038297876454, 101.0427570613523045 ) ) ;
#54649=CARTESIAN_POINT ( 'NONE',  ( -16.55341960407617563, 4.379528057220093196, 53.54275706135234714 ) ) ;
#54651=CARTESIAN_POINT ( 'NONE',  ( 10.72451020669898902, -18.67979575497178502, 97.91557627198103830 ) ) ;
#54652=CARTESIAN_POINT ( 'NONE',  ( -8.224510206698948167, 14.34966873604960824, 85.41557627198102409 ) ) ;
#54653=CARTESIAN_POINT ( 'NONE',  ( -16.61371651742600974, -7.165104196376154810, 101.1458493000700827 ) ) ;
#54654=CARTESIAN_POINT ( 'NONE',  ( -16.51473224551082808, 9.474510206698731452, 113.3344237280190043 ) ) ;
#54655=CARTESIAN_POINT ( 'NONE',  ( 18.62759615963271287, -10.81492255796078972, 43.33224293864769550 ) ) ;
#54656=CARTESIAN_POINT ( 'NONE',  ( -4.379528057220086978, -16.55341960407618274, 94.79275706135234714 ) ) ;
#54658=CARTESIAN_POINT ( 'NONE',  ( 16.55341960407618274, -4.379528057220086978, 51.04275706135234714 ) ) ;
#54659=CARTESIAN_POINT ( 'NONE',  ( 5.719274019375673035, 21.55341960407619339, 22.29275706135235069 ) ) ;
#54660=CARTESIAN_POINT ( 'NONE',  ( -10.81492255796078084, -18.62759615963271287, 42.08224293864769550 ) ) ;
#54661=CARTESIAN_POINT ( 'NONE',  ( 4.483927247898790824, -16.52544592524335698, 80.20942372801901854 ) ) ;
#54662=CARTESIAN_POINT ( 'NONE',  ( -19.03943276465977164, 0.05219959533909376836, 96.24890960531436690 ) ) ;
#54663=CARTESIAN_POINT ( 'NONE',  ( -18.62759615963255300, -10.81492255796106328, 64.16775706135234714 ) ) ;
#54664=CARTESIAN_POINT ( 'NONE',  ( 15.80617190586746368, 15.72974639402197994, 39.37390960531436690 ) ) ;
#54665=CARTESIAN_POINT ( 'NONE',  ( -10.72451020669898014, 18.67979575497178502, 25.41557627198103120 ) ) ;
#54667=CARTESIAN_POINT ( 'NONE',  ( 5.153800228976615827, -19.02544592524334988, 55.20942372801899722 ) ) ;
#54668=CARTESIAN_POINT ( 'NONE',  ( 16.52544592524335698, 4.483927247898782831, 71.45942372801901854 ) ) ;
#54669=CARTESIAN_POINT ( 'NONE',  ( -21.53943276465977519, 0.05219959533907696930, 36.24890960531435979 ) ) ;
#54670=ORIENTED_EDGE ( 'NONE', *, *, #93499, .T. ) ;
#54671=CARTESIAN_POINT ( 'NONE',  ( -19.05341960407611168, -5.049401038298163336, 81.45724293864769550 ) ) ;
#54672=CARTESIAN_POINT ( 'NONE',  ( -12.06949235617739369, -12.14591786802326823, 109.3760903946857042 ) ) ;
#54674=CARTESIAN_POINT ( 'NONE',  ( -4.483927247898539470, -16.52544592524342804, 112.2905762719810241 ) ) ;
#54675=CARTESIAN_POINT ( 'NONE',  ( -15.72974639402197994, 15.80617190586746368, 50.62390960531435979 ) ) ;
#54676=CARTESIAN_POINT ( 'NONE',  ( 0.05219959533909260263, 19.03943276465977164, 44.99890960531435979 ) ) ;
#54677=CARTESIAN_POINT ( 'NONE',  ( 16.53943276465976808, 0.05219959533934440121, 81.25109039468568994 ) ) ;
#54678=CARTESIAN_POINT ( 'NONE',  ( -21.53943276465977519, -0.05219959533937600094, 38.75109039468567573 ) ) ;
#54679=CARTESIAN_POINT ( 'NONE',  ( -19.05341960407617563, 5.049401038297882671, 93.54275706135234714 ) ) ;
#54680=CARTESIAN_POINT ( 'NONE',  ( -4.379528057220328563, 16.55341960407611168, 95.20724293864769550 ) ) ;
#54681=CARTESIAN_POINT ( 'NONE',  ( 19.05341960407611168, 5.049401038298154454, 58.95724293864768129 ) ) ;
#54682=CIRCLE ( 'NONE', #193541, 2.500000000000002220 ) ;
#54683=CARTESIAN_POINT ( 'NONE',  ( 5.153800228976335163, 19.02544592524342804, 24.79057627198102765 ) ) ;
#54684=CARTESIAN_POINT ( 'NONE',  ( -15.72974639402176322, -15.80617190586768395, 99.37609039468568994 ) ) ;
#54685=CARTESIAN_POINT ( 'NONE',  ( -13.97604488694527625, -13.89961937509977652, 76.87390960531433848 ) ) ;
#54686=CARTESIAN_POINT ( 'NONE',  ( -8.314922557961024197, 14.29746914071037800, 67.91775706135234714 ) ) ;
#54687=CARTESIAN_POINT ( 'NONE',  ( 18.62759615963255655, 10.81492255796105972, 91.66775706135234714 ) ) ;
#54688=CARTESIAN_POINT ( 'NONE',  ( -18.67979575497178146, -10.72451020669898902, 51.66557627198102409 ) ) ;
#54689=CARTESIAN_POINT ( 'NONE',  ( 12.06949235617739724, 12.14591786802326823, 76.87609039468567573 ) ) ;
#54690=CARTESIAN_POINT ( 'NONE',  ( -0.05219959533936034679, 19.03943276465977164, 52.50109039468566863 ) ) ;
#54691=CARTESIAN_POINT ( 'NONE',  ( 5.153800228976615827, -19.02544592524334988, 60.20942372801899012 ) ) ;
#54693=CARTESIAN_POINT ( 'NONE',  ( -5.719274019375665041, -21.55341960407619695, 64.79275706135234714 ) ) ;
#54694=CARTESIAN_POINT ( 'NONE',  ( -13.97604488694527625, -13.89961937509977652, 66.87390960531436690 ) ) ;
#54695=CARTESIAN_POINT ( 'NONE',  ( 5.153800228976335163, 19.02544592524342804, 24.79057627198102765 ) ) ;
#54696=CARTESIAN_POINT ( 'NONE',  ( 9.564922557961047289, -16.46253265017146816, 60.41775706135233293 ) ) ;
#54697=CARTESIAN_POINT ( 'NONE',  ( -19.03943276465977164, 0.05219959533909376836, 116.2489096053143669 ) ) ;
#54698=CARTESIAN_POINT ( 'NONE',  ( -16.46253265017160317, 9.564922557960807481, 100.8322429386477097 ) ) ;
#54699=CARTESIAN_POINT ( 'NONE',  ( 14.29746914071049879, -8.314922557960816363, 53.33224293864769550 ) ) ;
#54700=CARTESIAN_POINT ( 'NONE',  ( -21.52544592524343514, 5.823673210054127303, 41.04057627198103120 ) ) ;
#54702=CARTESIAN_POINT ( 'NONE',  ( -9.564922557961040184, 16.46253265017147172, 22.91775706135233648 ) ) ;
#54704=CARTESIAN_POINT ( 'NONE',  ( 0.05219959533909260263, 19.03943276465977164, 54.99890960531435979 ) ) ;
#54705=CARTESIAN_POINT ( 'NONE',  ( 9.564922557960805705, 16.46253265017160317, 24.58224293864769194 ) ) ;
#54708=CARTESIAN_POINT ( 'NONE',  ( 8.224510206698742110, 14.34966873604972548, 67.08442372801901854 ) ) ;
#54709=CARTESIAN_POINT ( 'NONE',  ( -10.72451020669898014, 18.67979575497178502, 85.41557627198102409 ) ) ;
#54710=CARTESIAN_POINT ( 'NONE',  ( 16.53943276465976808, -0.05219959533910856209, 48.74890960531435979 ) ) ;
#54711=CARTESIAN_POINT ( 'NONE',  ( -13.97604488694527625, -13.89961937509977652, 36.87390960531436690 ) ) ;
#54713=CARTESIAN_POINT ( 'NONE',  ( 21.52544592524334988, 5.823673210054432836, 46.45942372801901854 ) ) ;
#54714=CARTESIAN_POINT ( 'NONE',  ( -16.46253265017146816, -9.564922557961047289, 49.16775706135233293 ) ) ;
#54715=CARTESIAN_POINT ( 'NONE',  ( -19.05341960407611168, -5.049401038298163336, 31.45724293864769550 ) ) ;
#54716=CARTESIAN_POINT ( 'NONE',  ( -15.72974639402176322, -15.80617190586768395, 84.37609039468570415 ) ) ;
#54717=CARTESIAN_POINT ( 'NONE',  ( 17.50000000000000000, 5.499999999999992895, 96.70309617465829888 ) ) ;
#54718=CARTESIAN_POINT ( 'NONE',  ( -14.29746914071049879, 8.314922557960819915, 35.83224293864768839 ) ) ;
#54719=CARTESIAN_POINT ( 'NONE',  ( 19.20446147854529428, 5.499999999999905853, 41.88999695167679249 ) ) ;
#54720=CARTESIAN_POINT ( 'NONE',  ( 21.55341960407610458, 5.719274019375980345, 38.95724293864768839 ) ) ;
#54722=CARTESIAN_POINT ( 'NONE',  ( -16.46253265017160317, 9.564922557960807481, 90.83224293864769550 ) ) ;
#54723=CARTESIAN_POINT ( 'NONE',  ( 8.314922557960818139, 14.29746914071049879, 84.58224293864769550 ) ) ;
#54724=CARTESIAN_POINT ( 'NONE',  ( -12.14591786802326823, 12.06949235617739902, 28.12609039468568284 ) ) ;
#54725=CARTESIAN_POINT ( 'NONE',  ( 12.06949235617739724, 12.14591786802326823, 111.8760903946856615 ) ) ;
#54727=CARTESIAN_POINT ( 'NONE',  ( 13.97604488694527802, 13.89961937509977652, 29.37390960531435979 ) ) ;
#54729=CARTESIAN_POINT ( 'NONE',  ( -5.049401038298153566, 19.05341960407611168, 80.20724293864769550 ) ) ;
#54730=CARTESIAN_POINT ( 'NONE',  ( -5.823673210054116645, -21.52544592524344225, 92.29057627198103830 ) ) ;
#54731=CARTESIAN_POINT ( 'NONE',  ( 0.05219959533910956823, 16.53943276465976808, 29.99890960531435979 ) ) ;
#54732=CARTESIAN_POINT ( 'NONE',  ( 16.51473224551069308, 9.474510206698969483, 104.1655762719810241 ) ) ;
#54733=CARTESIAN_POINT ( 'NONE',  ( 13.89961937509957401, 13.97604488694547697, 86.87609039468567573 ) ) ;
#54734=CARTESIAN_POINT ( 'NONE',  ( 21.53943276465977519, 0.05219959533937863772, 111.2510903946856899 ) ) ;
#54735=CARTESIAN_POINT ( 'NONE',  ( -10.81492255796078084, -18.62759615963271287, 92.08224293864769550 ) ) ;
#54736=CARTESIAN_POINT ( 'NONE',  ( -0.05219959533907301413, -21.53943276465977519, 32.49890960531435979 ) ) ;
#54737=CARTESIAN_POINT ( 'NONE',  ( 16.51473224551069308, 9.474510206698969483, 64.16557627198102409 ) ) ;
#54738=CARTESIAN_POINT ( 'NONE',  ( -12.14591786802309592, -12.06949235617757132, 26.87390960531435979 ) ) ;
#54739=CARTESIAN_POINT ( 'NONE',  ( 9.474510206698971260, -16.51473224551069308, 82.91557627198103830 ) ) ;
#54742=CARTESIAN_POINT ( 'NONE',  ( -0.05219959533936034679, 19.03943276465977164, 22.50109039468566152 ) ) ;
#54743=CARTESIAN_POINT ( 'NONE',  ( -4.379528057220328563, 16.55341960407611168, 90.20724293864770971 ) ) ;
#54744=CARTESIAN_POINT ( 'NONE',  ( 15.72974639402176855, 15.80617190586768217, 21.87609039468567573 ) ) ;
#54746=CARTESIAN_POINT ( 'NONE',  ( 18.62759615963271287, -10.81492255796078972, 68.33224293864769550 ) ) ;
#54747=CARTESIAN_POINT ( 'NONE',  ( -14.29746914071037622, -8.314922557961029526, 89.16775706135236135 ) ) ;
#54748=CARTESIAN_POINT ( 'NONE',  ( -13.89961937509977652, 13.97604488694528158, 25.62390960531434558 ) ) ;
#54749=CARTESIAN_POINT ( 'NONE',  ( 13.89961937509977652, -13.97604488694527269, 78.12390960531433848 ) ) ;
#54750=CARTESIAN_POINT ( 'NONE',  ( 18.22780087662122384, -5.500000000000022204, 71.01540105326107266 ) ) ;
#54752=CARTESIAN_POINT ( 'NONE',  ( 16.55341960407611168, 4.379528057220329451, 33.95724293864769550 ) ) ;
#54753=CARTESIAN_POINT ( 'NONE',  ( 18.67979575497194134, -10.72451020669871369, 65.83442372801900433 ) ) ;
#54754=CARTESIAN_POINT ( 'NONE',  ( -5.049401038298153566, 19.05341960407611168, 115.2072429386477097 ) ) ;
#54755=CARTESIAN_POINT ( 'NONE',  ( 18.67979575497194134, -10.72451020669871369, 100.8344237280190185 ) ) ;
#54756=CARTESIAN_POINT ( 'NONE',  ( 9.564922557960805705, 16.46253265017160317, 44.58224293864769550 ) ) ;
#54757=CARTESIAN_POINT ( 'NONE',  ( -19.05341960407611168, -5.049401038298163336, 51.45724293864770260 ) ) ;
#54758=ORIENTED_EDGE ( 'NONE', *, *, #82217, .T. ) ;
#54759=CARTESIAN_POINT ( 'NONE',  ( -18.62759615963255300, -10.81492255796106328, 94.16775706135237556 ) ) ;
#54760=CARTESIAN_POINT ( 'NONE',  ( 12.14591786802327356, -12.06949235617739191, 55.62609039468568284 ) ) ;
#54761=CARTESIAN_POINT ( 'NONE',  ( 18.62759615963255655, 10.81492255796105972, 86.66775706135234714 ) ) ;
#54762=CARTESIAN_POINT ( 'NONE',  ( -21.52544592524343514, 5.823673210054127303, 26.04057627198103475 ) ) ;
#54763=CARTESIAN_POINT ( 'NONE',  ( 5.153800228976615827, -19.02544592524334988, 100.2094237280190043 ) ) ;
#54764=CARTESIAN_POINT ( 'NONE',  ( 15.80617190586769283, -15.72974639402175789, 50.62609039468568994 ) ) ;
#54765=CARTESIAN_POINT ( 'NONE',  ( -14.34966873604972548, 8.224510206698743886, 33.33442372801900433 ) ) ;
#54766=CARTESIAN_POINT ( 'NONE',  ( 21.52544592524344225, -5.823673210054117533, 88.54057627198103830 ) ) ;
#54767=CARTESIAN_POINT ( 'NONE',  ( -9.564922557961040184, 16.46253265017147172, 87.91775706135233293 ) ) ;
#54768=CARTESIAN_POINT ( 'NONE',  ( -19.03943276465977164, 0.05219959533909376836, 71.24890960531435269 ) ) ;
#54769=CARTESIAN_POINT ( 'NONE',  ( 5.049401038297881783, 19.05341960407617563, 102.2927570613523045 ) ) ;
#54771=CARTESIAN_POINT ( 'NONE',  ( -16.51473224551082808, 9.474510206698731452, 98.33442372801900433 ) ) ;
#54772=CARTESIAN_POINT ( 'NONE',  ( -12.06949235617756955, 12.14591786802309770, 55.62390960531436690 ) ) ;
#54773=CARTESIAN_POINT ( 'NONE',  ( -9.474510206698720793, -16.51473224551083518, 74.58442372801900433 ) ) ;
#54774=CARTESIAN_POINT ( 'NONE',  ( -14.29746914071037622, -8.314922557961029526, 54.16775706135235424 ) ) ;
#54775=CARTESIAN_POINT ( 'NONE',  ( -19.02544592524334988, -5.153800228976617603, 43.95942372801899012 ) ) ;
#54776=CARTESIAN_POINT ( 'NONE',  ( 13.97604488694527802, 13.89961937509977652, 34.37390960531436690 ) ) ;
#54777=CARTESIAN_POINT ( 'NONE',  ( 13.89961937509977652, -13.97604488694527269, 58.12390960531436690 ) ) ;
#54778=CARTESIAN_POINT ( 'NONE',  ( -16.53943276465976808, -0.05219959533934237506, 53.75109039468568994 ) ) ;
#54781=CARTESIAN_POINT ( 'NONE',  ( -19.03943276465977164, 0.05219959533909376836, 111.2489096053143669 ) ) ;
#54782=CARTESIAN_POINT ( 'NONE',  ( -9.474510206698964154, 16.51473224551069663, 25.41557627198103120 ) ) ;
#54783=CARTESIAN_POINT ( 'NONE',  ( 9.474510206698729675, 16.51473224551082808, 102.0844237280190043 ) ) ;
#54785=CARTESIAN_POINT ( 'NONE',  ( -5.719274019375978568, 21.55341960407610458, 35.20724293864768839 ) ) ;
#54786=CARTESIAN_POINT ( 'NONE',  ( 5.153800228976615827, -19.02544592524334988, 35.20942372801899722 ) ) ;
#54787=CARTESIAN_POINT ( 'NONE',  ( 0.05219959533936267826, -19.03943276465977164, 110.0010903946856757 ) ) ;
#54788=CARTESIAN_POINT ( 'NONE',  ( 16.51473224551069308, 9.474510206698969483, 29.16557627198103475 ) ) ;
#54789=CARTESIAN_POINT ( 'NONE',  ( -19.03943276465977164, 0.05219959533909376836, 46.24890960531435979 ) ) ;
#54790=CARTESIAN_POINT ( 'NONE',  ( 18.67979575497178502, 10.72451020669898547, 69.16557627198102409 ) ) ;
#54791=CARTESIAN_POINT ( 'NONE',  ( 13.97604488694527802, 13.89961937509977652, 99.37390960531436690 ) ) ;
#54792=CARTESIAN_POINT ( 'NONE',  ( 9.474510206698971260, -16.51473224551069308, 32.91557627198102409 ) ) ;
#54794=CARTESIAN_POINT ( 'NONE',  ( 16.51473224551083163, -9.474510206698727899, 80.83442372801899012 ) ) ;
#54795=CARTESIAN_POINT ( 'NONE',  ( 16.52544592524342804, -4.483927247898539470, 58.54057627198103120 ) ) ;
#54796=CARTESIAN_POINT ( 'NONE',  ( 21.52544592524344225, -5.823673210054117533, 38.54057627198103120 ) ) ;
#54797=CARTESIAN_POINT ( 'NONE',  ( 5.823673210054444382, -21.52544592524334988, 110.2094237280190185 ) ) ;
#54798=CARTESIAN_POINT ( 'NONE',  ( -0.05219959533907301413, -21.53943276465977519, 97.49890960531436690 ) ) ;
#54799=CARTESIAN_POINT ( 'NONE',  ( 18.67979575497194134, -10.72451020669871369, 75.83442372801900433 ) ) ;
#54800=CARTESIAN_POINT ( 'NONE',  ( -10.81492255796105439, 18.62759615963255655, 82.91775706135234714 ) ) ;
#54801=CARTESIAN_POINT ( 'NONE',  ( 16.46253265017160672, -9.564922557960803928, 113.3322429386476955 ) ) ;
#54802=CARTESIAN_POINT ( 'NONE',  ( 4.379528057220092307, 16.55341960407617563, 102.2927570613523613 ) ) ;
#54803=CARTESIAN_POINT ( 'NONE',  ( -21.52544592524334988, -5.823673210054445271, 58.95942372801902565 ) ) ;
#54804=CARTESIAN_POINT ( 'NONE',  ( -0.05219959533909027116, -19.03943276465977164, 72.49890960531435269 ) ) ;
#54805=CARTESIAN_POINT ( 'NONE',  ( -5.049401038297874678, -19.05341960407617918, 34.79275706135233293 ) ) ;
#54806=CARTESIAN_POINT ( 'NONE',  ( 21.55341960407619695, -5.719274019375665929, 26.04275706135235779 ) ) ;
#54807=CARTESIAN_POINT ( 'NONE',  ( -0.05219959533909027116, -19.03943276465977164, 67.49890960531436690 ) ) ;
#54808=CARTESIAN_POINT ( 'NONE',  ( -4.483927247898539470, -16.52544592524342804, 82.29057627198103830 ) ) ;
#54809=CARTESIAN_POINT ( 'NONE',  ( -12.06949235617756955, 12.14591786802309770, 50.62390960531435979 ) ) ;
#54810=CARTESIAN_POINT ( 'NONE',  ( -18.67979575497178146, -10.72451020669898902, 51.66557627198102409 ) ) ;
#54811=CARTESIAN_POINT ( 'NONE',  ( -19.03943276465977164, 0.05219959533909376836, 61.24890960531436690 ) ) ;
#54812=CARTESIAN_POINT ( 'NONE',  ( 21.55341960407610458, 5.719274019375980345, 73.95724293864769550 ) ) ;
#54813=CARTESIAN_POINT ( 'NONE',  ( 13.89961937509957401, 13.97604488694547697, 66.87609039468567573 ) ) ;
#54814=CARTESIAN_POINT ( 'NONE',  ( -13.97604488694547520, 13.89961937509957934, 23.12609039468565797 ) ) ;
#54815=CARTESIAN_POINT ( 'NONE',  ( 14.34966873604960469, 8.224510206698951720, 64.16557627198102409 ) ) ;
#54816=CARTESIAN_POINT ( 'NONE',  ( 18.67979575497178502, 10.72451020669898547, 44.16557627198103120 ) ) ;
#54819=CARTESIAN_POINT ( 'NONE',  ( 16.52216118717206683, 7.221426719304504971, 103.5759902104699250 ) ) ;
#54820=CARTESIAN_POINT ( 'NONE',  ( -12.06949235617739369, -12.14591786802326823, 79.37609039468567573 ) ) ;
#54822=CARTESIAN_POINT ( 'NONE',  ( 13.97604488694548053, -13.89961937509957401, 90.62609039468567573 ) ) ;
#54823=EDGE_CURVE ( 'NONE', #101016, #123998, #77077, .T. ) ;
#54824=CARTESIAN_POINT ( 'NONE',  ( -12.14591786802309592, -12.06949235617757132, 51.87390960531437401 ) ) ;
#54826=CARTESIAN_POINT ( 'NONE',  ( -13.97604488694527625, -13.89961937509977652, 46.87390960531435979 ) ) ;
#54827=CARTESIAN_POINT ( 'NONE',  ( 8.314922557960818139, 14.29746914071049879, 39.58224293864769550 ) ) ;
#54828=CARTESIAN_POINT ( 'NONE',  ( 19.02544592524343514, -5.153800228976328945, 93.54057627198102409 ) ) ;
#54829=CARTESIAN_POINT ( 'NONE',  ( -5.153800228976328057, -19.02544592524343514, 47.29057627198102409 ) ) ;
#54830=CARTESIAN_POINT ( 'NONE',  ( -0.05219959533937732626, 21.53943276465977519, 57.50109039468568994 ) ) ;
#54831=CARTESIAN_POINT ( 'NONE',  ( -19.03943276465977164, 0.05219959533909376836, 76.24890960531435269 ) ) ;
#54832=CARTESIAN_POINT ( 'NONE',  ( -9.564922557960796823, -16.46253265017161027, 32.08224293864769550 ) ) ;
#54833=CARTESIAN_POINT ( 'NONE',  ( 9.474510206698971260, -16.51473224551069308, 72.91557627198102409 ) ) ;
#54834=CARTESIAN_POINT ( 'NONE',  ( 0.05219959533907565091, 21.53943276465977519, 49.99890960531437401 ) ) ;
#54835=CARTESIAN_POINT ( 'NONE',  ( 19.03943276465977164, -0.05219959533909143690, 48.74890960531435979 ) ) ;
#54836=CARTESIAN_POINT ( 'NONE',  ( 10.81492255796078972, 18.62759615963270932, 49.58224293864769550 ) ) ;
#54837=CARTESIAN_POINT ( 'NONE',  ( -19.05341960407617563, 5.049401038297882671, 83.54275706135233293 ) ) ;
#54838=CARTESIAN_POINT ( 'NONE',  ( -14.29746914071037622, -8.314922557961029526, 99.16775706135234714 ) ) ;
#54839=CARTESIAN_POINT ( 'NONE',  ( 13.89961937509957401, 13.97604488694547697, 26.87609039468566507 ) ) ;
#54840=CARTESIAN_POINT ( 'NONE',  ( 16.52544592524335698, 4.483927247898782831, 51.45942372801901854 ) ) ;
#54841=CARTESIAN_POINT ( 'NONE',  ( -0.05219959533934338120, 16.53943276465976808, 77.50109039468567573 ) ) ;
#54843=CARTESIAN_POINT ( 'NONE',  ( -16.52544592524335698, -4.483927247898792601, 68.95942372801901854 ) ) ;
#54844=CARTESIAN_POINT ( 'NONE',  ( 10.81492255796078972, 18.62759615963270932, 29.58224293864769905 ) ) ;
#54845=CARTESIAN_POINT ( 'NONE',  ( 16.46253265017160672, -9.564922557960803928, 28.33224293864769550 ) ) ;
#54846=CARTESIAN_POINT ( 'NONE',  ( -16.53943276465976808, -0.05219959533934237506, 38.75109039468567573 ) ) ;
#54847=CARTESIAN_POINT ( 'NONE',  ( -13.89961937509977652, 13.97604488694528158, 45.62390960531433848 ) ) ;
#54848=CARTESIAN_POINT ( 'NONE',  ( -21.55341960407619339, 5.719274019375674811, 38.54275706135234714 ) ) ;
#54849=CARTESIAN_POINT ( 'NONE',  ( 8.224510206698742110, 14.34966873604972548, 42.08442372801901854 ) ) ;
#54850=CARTESIAN_POINT ( 'NONE',  ( 8.314922557961029526, -14.29746914071037800, 100.4177570613523471 ) ) ;
#54852=CARTESIAN_POINT ( 'NONE',  ( 13.97604488694548053, -13.89961937509957401, 20.62609039468567573 ) ) ;
#54853=CARTESIAN_POINT ( 'NONE',  ( 4.483927247898790824, -16.52544592524335698, 20.20942372801900788 ) ) ;
#54854=CARTESIAN_POINT ( 'NONE',  ( -9.564922557961040184, 16.46253265017147172, 72.91775706135233293 ) ) ;
#54855=CARTESIAN_POINT ( 'NONE',  ( -8.224510206698948167, 14.34966873604960824, 70.41557627198102409 ) ) ;
#54856=CARTESIAN_POINT ( 'NONE',  ( 0.05219959533910956823, 16.53943276465976808, 114.9989096053143669 ) ) ;
#54857=CARTESIAN_POINT ( 'NONE',  ( -16.46253265017146816, -9.564922557961047289, 59.16775706135233293 ) ) ;
#54858=CARTESIAN_POINT ( 'NONE',  ( 16.36317988757095421, -7.306389748694852138, 56.59789608363175972 ) ) ;
#54859=CARTESIAN_POINT ( 'NONE',  ( 5.823673210054444382, -21.52544592524334988, 60.20942372801902565 ) ) ;
#54860=CARTESIAN_POINT ( 'NONE',  ( 8.224510206698742110, 14.34966873604972548, 22.08442372801901143 ) ) ;
#54862=CARTESIAN_POINT ( 'NONE',  ( -21.55341960407610458, -5.719274019375992779, 26.45724293864768839 ) ) ;
#54863=CARTESIAN_POINT ( 'NONE',  ( -12.06949235617739369, -12.14591786802326823, 19.37609039468568639 ) ) ;
#54866=CARTESIAN_POINT ( 'NONE',  ( -19.03943276465977164, 0.05219959533909376836, 26.24890960531435624 ) ) ;
#54867=CARTESIAN_POINT ( 'NONE',  ( 21.52544592524334988, 5.823673210054432836, 106.4594237280190328 ) ) ;
#54868=CARTESIAN_POINT ( 'NONE',  ( -16.46253265017160317, 9.564922557960807481, 55.83224293864769550 ) ) ;
#54869=CARTESIAN_POINT ( 'NONE',  ( 21.52544592524334988, 5.823673210054432836, 66.45942372801903275 ) ) ;
#54870=CARTESIAN_POINT ( 'NONE',  ( -0.05219959533937732626, 21.53943276465977519, 102.5010903946856899 ) ) ;
#54871=CARTESIAN_POINT ( 'NONE',  ( -8.314922557960811034, -14.29746914071050412, 27.08224293864769550 ) ) ;
#54872=CARTESIAN_POINT ( 'NONE',  ( 9.564922557960805705, 16.46253265017160317, 34.58224293864770260 ) ) ;
#54873=CARTESIAN_POINT ( 'NONE',  ( -9.564922557960796823, -16.46253265017161027, 77.08224293864769550 ) ) ;
#54874=CARTESIAN_POINT ( 'NONE',  ( 15.80617190586769283, -15.72974639402175789, 55.62609039468568284 ) ) ;
#54875=CARTESIAN_POINT ( 'NONE',  ( -13.97604488694527625, -13.89961937509977652, 36.87390960531436690 ) ) ;
#54876=CARTESIAN_POINT ( 'NONE',  ( 10.81492255796106328, -18.62759615963255655, 55.41775706135234714 ) ) ;
#54877=CARTESIAN_POINT ( 'NONE',  ( -13.97604488694547697, 13.89961937509957934, 78.12609039468567573 ) ) ;
#54878=CARTESIAN_POINT ( 'NONE',  ( -5.153800228976328057, -19.02544592524343514, 112.2905762719810099 ) ) ;
#54879=CARTESIAN_POINT ( 'NONE',  ( 19.02544592524343514, -5.153800228976328945, 28.54057627198102409 ) ) ;
#54880=CARTESIAN_POINT ( 'NONE',  ( -15.72974639402197994, 15.80617190586746368, 105.6239096053143669 ) ) ;
#54881=CARTESIAN_POINT ( 'NONE',  ( -13.89961937509957401, -13.97604488694547875, 39.37609039468566152 ) ) ;
#54882=CARTESIAN_POINT ( 'NONE',  ( -14.34966873604960291, -8.224510206698953496, 91.66557627198103830 ) ) ;
#54883=CARTESIAN_POINT ( 'NONE',  ( 5.153800228976335163, 19.02544592524342804, 44.79057627198103830 ) ) ;
#54884=CARTESIAN_POINT ( 'NONE',  ( -0.05219959533936034679, 19.03943276465977164, 97.50109039468567573 ) ) ;
#54885=CARTESIAN_POINT ( 'NONE',  ( -12.14591786802309592, -12.06949235617757132, 56.87390960531436690 ) ) ;
#54886=CARTESIAN_POINT ( 'NONE',  ( 21.55341960407619695, -5.719274019375665929, 111.0427570613523613 ) ) ;
#54887=CARTESIAN_POINT ( 'NONE',  ( 5.153800228976335163, 19.02544592524342804, 99.79057627198102409 ) ) ;
#54888=CARTESIAN_POINT ( 'NONE',  ( 13.97604488694548053, -13.89961937509957401, 90.62609039468567573 ) ) ;
#54889=CARTESIAN_POINT ( 'NONE',  ( 21.55341960407610458, 5.719274019375980345, 88.95724293864769550 ) ) ;
#54890=CARTESIAN_POINT ( 'NONE',  ( 21.53943276465977519, 0.05219959533937863772, 41.25109039468568284 ) ) ;
#54891=CARTESIAN_POINT ( 'NONE',  ( -14.29746914071037622, -8.314922557961029526, 44.16775706135234714 ) ) ;
#54892=CARTESIAN_POINT ( 'NONE',  ( 8.224510206698742110, 14.34966873604972548, 107.0844237280190043 ) ) ;
#54893=CARTESIAN_POINT ( 'NONE',  ( -16.52544592524335698, -4.483927247898792601, 43.95942372801902565 ) ) ;
#54894=CARTESIAN_POINT ( 'NONE',  ( 10.81492255796106328, -18.62759615963255655, 50.41775706135235424 ) ) ;
#54895=CARTESIAN_POINT ( 'NONE',  ( 18.62759615963271287, -10.81492255796078972, 38.33224293864768839 ) ) ;
#54896=CARTESIAN_POINT ( 'NONE',  ( 0.05219959533909260263, 19.03943276465977164, 29.99890960531435979 ) ) ;
#54898=CARTESIAN_POINT ( 'NONE',  ( 16.53943276465976808, 0.05219959533934440121, 61.25109039468567573 ) ) ;
#54899=CARTESIAN_POINT ( 'NONE',  ( -0.05219959533907301413, -21.53943276465977519, 82.49890960531436690 ) ) ;
#54900=CARTESIAN_POINT ( 'NONE',  ( 0.05219959533910956823, 16.53943276465976808, 39.99890960531436690 ) ) ;
#54901=CARTESIAN_POINT ( 'NONE',  ( -12.06949235617739369, -12.14591786802326823, 64.37609039468568994 ) ) ;
#54902=CARTESIAN_POINT ( 'NONE',  ( 5.049401038298161559, -19.05341960407611168, 62.70724293864769550 ) ) ;
#54904=CARTESIAN_POINT ( 'NONE',  ( -13.89961937509957401, -13.97604488694547875, 94.37609039468566152 ) ) ;
#54905=CARTESIAN_POINT ( 'NONE',  ( 21.52544592524344225, -5.823673210054117533, 83.54057627198102409 ) ) ;
#54906=CARTESIAN_POINT ( 'NONE',  ( 8.224510206698953496, -14.34966873604960469, 32.91557627198102409 ) ) ;
#54909=CARTESIAN_POINT ( 'NONE',  ( 18.62759615963271287, -10.81492255796078972, 68.33224293864769550 ) ) ;
#54911=CARTESIAN_POINT ( 'NONE',  ( -8.224510206698735004, -14.34966873604973081, 109.5844237280190328 ) ) ;
#54914=CARTESIAN_POINT ( 'NONE',  ( 18.67979575497178502, 10.72451020669898547, 94.16557627198103830 ) ) ;
#54915=CARTESIAN_POINT ( 'NONE',  ( 21.55341960407610458, 5.719274019375980345, 103.9572429386476813 ) ) ;
#54916=CARTESIAN_POINT ( 'NONE',  ( -16.52544592524342804, 4.483927247898546575, 26.04057627198103475 ) ) ;
#54917=CARTESIAN_POINT ( 'NONE',  ( -8.224510206698735004, -14.34966873604973081, 39.58442372801901143 ) ) ;
#54918=CARTESIAN_POINT ( 'NONE',  ( 13.97604488694527802, 13.89961937509977652, 29.37390960531435979 ) ) ;
#54919=CARTESIAN_POINT ( 'NONE',  ( -16.46253265017160317, 9.564922557960807481, 65.83224293864769550 ) ) ;
#54921=CARTESIAN_POINT ( 'NONE',  ( 18.62759615963271287, -10.81492255796078972, 23.33224293864769194 ) ) ;
#54923=CARTESIAN_POINT ( 'NONE',  ( 19.02544592524334988, 5.153800228976608722, 101.4594237280189759 ) ) ;
#54924=CARTESIAN_POINT ( 'NONE',  ( -9.474510206698720793, -16.51473224551083518, 34.58442372801899722 ) ) ;
#54925=CARTESIAN_POINT ( 'NONE',  ( -5.719274019375978568, 21.55341960407610458, 95.20724293864769550 ) ) ;
#54926=CARTESIAN_POINT ( 'NONE',  ( -16.55341960407617563, 4.379528057220093196, 113.5427570613523756 ) ) ;
#54927=CARTESIAN_POINT ( 'NONE',  ( -5.719274019375978568, 21.55341960407610458, 45.20724293864769550 ) ) ;
#54928=CARTESIAN_POINT ( 'NONE',  ( -10.81492255796078084, -18.62759615963271287, 82.08224293864768129 ) ) ;
#54929=CARTESIAN_POINT ( 'NONE',  ( 19.02544592524334988, 5.153800228976608722, 111.4594237280190043 ) ) ;
#54930=CARTESIAN_POINT ( 'NONE',  ( 19.02544592524343514, -5.153800228976328945, 98.54057627198100988 ) ) ;
#54931=CARTESIAN_POINT ( 'NONE',  ( 21.55341960407619695, -5.719274019375665929, 76.04275706135237556 ) ) ;
#54932=CARTESIAN_POINT ( 'NONE',  ( -19.03943276465977164, 0.05219959533909376836, 61.24890960531436690 ) ) ;
#54934=CARTESIAN_POINT ( 'NONE',  ( 8.314922557960818139, 14.29746914071049879, 99.58224293864770971 ) ) ;
#54936=CARTESIAN_POINT ( 'NONE',  ( -19.05341960407611168, -5.049401038298163336, 66.45724293864769550 ) ) ;
#54937=CARTESIAN_POINT ( 'NONE',  ( 14.34966873604960469, 8.224510206698951720, 94.16557627198103830 ) ) ;
#54939=CARTESIAN_POINT ( 'NONE',  ( 16.46253265017146816, 9.564922557961045513, 96.66775706135233293 ) ) ;
#54940=CARTESIAN_POINT ( 'NONE',  ( 16.38665767535050577, -7.295008042176161389, 82.76400864214542707 ) ) ;
#54941=CARTESIAN_POINT ( 'NONE',  ( -0.05219959533909027116, -19.03943276465977164, 62.49890960531435979 ) ) ;
#54942=CARTESIAN_POINT ( 'NONE',  ( -21.52544592524334988, -5.823673210054445271, 78.95942372801901854 ) ) ;
#54943=CARTESIAN_POINT ( 'NONE',  ( 19.05341960407611168, 5.049401038298154454, 103.9572429386476671 ) ) ;
#54944=CARTESIAN_POINT ( 'NONE',  ( -8.314922557961024197, 14.29746914071037800, 77.91775706135231871 ) ) ;
#54945=CARTESIAN_POINT ( 'NONE',  ( -17.49999999999999645, -5.499999999999992895, 49.20309617465830598 ) ) ;
#54946=CARTESIAN_POINT ( 'NONE',  ( 13.89961937509957401, 13.97604488694547697, 56.87609039468564731 ) ) ;
#54947=CARTESIAN_POINT ( 'NONE',  ( -10.81492255796105439, 18.62759615963255655, 97.91775706135236135 ) ) ;
#54950=CARTESIAN_POINT ( 'NONE',  ( -16.52544592524335698, -4.483927247898792601, 98.95942372801903275 ) ) ;
#54952=CARTESIAN_POINT ( 'NONE',  ( -14.34966873604972548, 8.224510206698743886, 88.33442372801901854 ) ) ;
#54954=CARTESIAN_POINT ( 'NONE',  ( -14.34966873604972548, 8.224510206698743886, 63.33442372801900433 ) ) ;
#54955=CARTESIAN_POINT ( 'NONE',  ( 18.09805431107246676, -5.500000000000095923, 68.51606229291886052 ) ) ;
#54956=CARTESIAN_POINT ( 'NONE',  ( 18.62759615963255655, 10.81492255796105972, 76.66775706135234714 ) ) ;
#54957=CARTESIAN_POINT ( 'NONE',  ( 19.03943276465977164, 0.05219959533936151252, 91.25109039468566152 ) ) ;
#54958=CARTESIAN_POINT ( 'NONE',  ( -9.474510206698720793, -16.51473224551083518, 39.58442372801899722 ) ) ;
#54959=CARTESIAN_POINT ( 'NONE',  ( -19.02544592524342804, 5.153800228976336051, 71.04057627198099567 ) ) ;
#54960=CARTESIAN_POINT ( 'NONE',  ( -0.05219959533909027116, -19.03943276465977164, 57.49890960531435979 ) ) ;
#54961=CYLINDRICAL_SURFACE ( 'NONE', #120780, 2.000000000000001776 ) ;
#54962=CARTESIAN_POINT ( 'NONE',  ( -21.53943276465977519, 0.05219959533907696930, 86.24890960531436690 ) ) ;
#54964=CARTESIAN_POINT ( 'NONE',  ( -21.52544592524343514, 5.823673210054127303, 36.04057627198102409 ) ) ;
#54965=CARTESIAN_POINT ( 'NONE',  ( 19.03943276465977164, -0.05219959533909143690, 38.74890960531436690 ) ) ;
#54966=CARTESIAN_POINT ( 'NONE',  ( -4.483927247898782831, 16.52544592524335698, 62.70942372801902565 ) ) ;
#54969=CARTESIAN_POINT ( 'NONE',  ( 10.72451020669871369, 18.67979575497193778, 27.08442372801901854 ) ) ;
#54970=CARTESIAN_POINT ( 'NONE',  ( -16.55341960407611168, -4.379528057220339221, 66.45724293864768129 ) ) ;
#54972=CARTESIAN_POINT ( 'NONE',  ( 14.29746914071037800, 8.314922557961029526, 26.66775706135235424 ) ) ;
#54973=CARTESIAN_POINT ( 'NONE',  ( 9.474510206698729675, 16.51473224551082808, 52.08442372801900433 ) ) ;
#54974=CARTESIAN_POINT ( 'NONE',  ( -0.05219959533910754901, -16.53943276465976808, 52.49890960531435979 ) ) ;
#54975=CARTESIAN_POINT ( 'NONE',  ( -10.81492255796105439, 18.62759615963255655, 37.91775706135235424 ) ) ;
#54977=CARTESIAN_POINT ( 'NONE',  ( -15.80617190586745835, -15.72974639402198527, 76.87390960531439532 ) ) ;
#54978=CARTESIAN_POINT ( 'NONE',  ( 5.049401038298161559, -19.05341960407611168, 97.70724293864766707 ) ) ;
#54979=CARTESIAN_POINT ( 'NONE',  ( 16.52544592524342804, -4.483927247898539470, 73.54057627198102409 ) ) ;
#54982=CARTESIAN_POINT ( 'NONE',  ( -13.97604488694547697, 13.89961937509957934, 63.12609039468566152 ) ) ;
#54983=CARTESIAN_POINT ( 'NONE',  ( 10.72451020669898902, -18.67979575497178502, 102.9155762719810383 ) ) ;
#54984=CARTESIAN_POINT ( 'NONE',  ( 9.474510206698971260, -16.51473224551069308, 57.91557627198103120 ) ) ;
#54985=CARTESIAN_POINT ( 'NONE',  ( 19.05341960407617918, -5.049401038297876454, 41.04275706135233293 ) ) ;
#54986=CARTESIAN_POINT ( 'NONE',  ( -19.05341960407611168, -5.049401038298163336, 36.45724293864766707 ) ) ;
#54987=CARTESIAN_POINT ( 'NONE',  ( -10.81492255796105439, 18.62759615963255655, 57.91775706135234714 ) ) ;
#54988=CARTESIAN_POINT ( 'NONE',  ( -16.81555441253552274, -7.025013491695476731, 69.36314554665744936 ) ) ;
#54989=CARTESIAN_POINT ( 'NONE',  ( 16.52544592524342804, -4.483927247898539470, 43.54057627198103830 ) ) ;
#54990=CARTESIAN_POINT ( 'NONE',  ( -5.153800228976328057, -19.02544592524343514, 57.29057627198103120 ) ) ;
#54991=CARTESIAN_POINT ( 'NONE',  ( 18.67979575497178502, 10.72451020669898547, 84.16557627198103830 ) ) ;
#54992=CARTESIAN_POINT ( 'NONE',  ( 13.89961937509977652, -13.97604488694527269, 58.12390960531436690 ) ) ;
#54993=ORIENTED_EDGE ( 'NONE', *, *, #163633, .T. ) ;
#54994=CARTESIAN_POINT ( 'NONE',  ( 10.72451020669898902, -18.67979575497178502, 72.91557627198103830 ) ) ;
#54995=CARTESIAN_POINT ( 'NONE',  ( -15.80617190586768217, 15.72974639402176855, 98.12609039468570415 ) ) ;
#54996=CARTESIAN_POINT ( 'NONE',  ( -13.89961937509977652, 13.97604488694528158, 25.62390960531434558 ) ) ;
#54997=CARTESIAN_POINT ( 'NONE',  ( 12.14591786802327356, -12.06949235617739191, 90.62609039468567573 ) ) ;
#54998=CARTESIAN_POINT ( 'NONE',  ( -12.14591786802309592, -12.06949235617757132, 86.87390960531438111 ) ) ;
#54999=CARTESIAN_POINT ( 'NONE',  ( 13.89961937509957401, 13.97604488694547697, 96.87609039468566152 ) ) ;
#55001=CARTESIAN_POINT ( 'NONE',  ( 13.97604488694548053, -13.89961937509957401, 40.62609039468564731 ) ) ;
#55002=CARTESIAN_POINT ( 'NONE',  ( 14.34966873604972726, -8.224510206698740333, 95.83442372801903275 ) ) ;
#55003=CARTESIAN_POINT ( 'NONE',  ( -9.474510206698720793, -16.51473224551083518, 34.58442372801899722 ) ) ;
#55004=CARTESIAN_POINT ( 'NONE',  ( -5.049401038298153566, 19.05341960407611168, 85.20724293864766707 ) ) ;
#55005=CARTESIAN_POINT ( 'NONE',  ( 15.80617190586746368, 15.72974639402197994, 64.37390960531435269 ) ) ;
#55007=CARTESIAN_POINT ( 'NONE',  ( 8.314922557960818139, 14.29746914071049879, 114.5822429386477097 ) ) ;
#55008=CARTESIAN_POINT ( 'NONE',  ( -21.55341960407619339, 5.719274019375674811, 98.54275706135234714 ) ) ;
#55009=CARTESIAN_POINT ( 'NONE',  ( -8.314922557961024197, 14.29746914071037800, 72.91775706135234714 ) ) ;
#55010=CARTESIAN_POINT ( 'NONE',  ( -15.72974639402176322, -15.80617190586768395, 34.37609039468568284 ) ) ;
#55011=CARTESIAN_POINT ( 'NONE',  ( -8.224510206698735004, -14.34966873604973081, 34.58442372801900433 ) ) ;
#55012=CARTESIAN_POINT ( 'NONE',  ( 19.02544592524343514, -5.153800228976328945, 98.54057627198100988 ) ) ;
#55013=CARTESIAN_POINT ( 'NONE',  ( -9.474510206698964154, 16.51473224551069663, 35.41557627198102409 ) ) ;
#55014=CARTESIAN_POINT ( 'NONE',  ( -16.46253265017160317, 9.564922557960807481, 60.83224293864769550 ) ) ;
#55015=CARTESIAN_POINT ( 'NONE',  ( -16.55341960407617563, 4.379528057220093196, 43.54275706135235424 ) ) ;
#55016=CARTESIAN_POINT ( 'NONE',  ( 14.29746914071049879, -8.314922557960816363, 93.33224293864769550 ) ) ;
#55017=CARTESIAN_POINT ( 'NONE',  ( -12.06949235617739369, -12.14591786802326823, 94.37609039468568994 ) ) ;
#55018=CARTESIAN_POINT ( 'NONE',  ( -21.55341960407619339, 5.719274019375674811, 38.54275706135234714 ) ) ;
#55019=CARTESIAN_POINT ( 'NONE',  ( -5.153800228976328057, -19.02544592524343514, 72.29057627198102409 ) ) ;
#55020=CARTESIAN_POINT ( 'NONE',  ( -13.97604488694527625, -13.89961937509977652, 66.87390960531436690 ) ) ;
#55021=CARTESIAN_POINT ( 'NONE',  ( 5.153800228976335163, 19.02544592524342804, 94.79057627198103830 ) ) ;
#55022=CARTESIAN_POINT ( 'NONE',  ( -4.379528057220328563, 16.55341960407611168, 30.20724293864769550 ) ) ;
#55023=CARTESIAN_POINT ( 'NONE',  ( -16.55341960407617563, 4.379528057220093196, 98.54275706135234714 ) ) ;
#55024=ORIENTED_EDGE ( 'NONE', *, *, #26552, .T. ) ;
#55025=CARTESIAN_POINT ( 'NONE',  ( 13.97604488694548053, -13.89961937509957401, 40.62609039468564731 ) ) ;
#55027=CARTESIAN_POINT ( 'NONE',  ( 19.03943276465977164, -0.05219959533909143690, 58.74890960531435979 ) ) ;
#55028=CARTESIAN_POINT ( 'NONE',  ( 9.474510206698729675, 16.51473224551082808, 42.08442372801900433 ) ) ;
#55030=CARTESIAN_POINT ( 'NONE',  ( 19.52217212775661537, -5.499999999999910294, 72.43993709005259518 ) ) ;
#55031=CARTESIAN_POINT ( 'NONE',  ( 14.34966873604972726, -8.224510206698740333, 45.83442372801901854 ) ) ;
#55032=CARTESIAN_POINT ( 'NONE',  ( 16.46253265017146816, 9.564922557961045513, 76.66775706135234714 ) ) ;
#55033=CARTESIAN_POINT ( 'NONE',  ( 16.52544592524335698, 4.483927247898782831, 61.45942372801901854 ) ) ;
#55035=CARTESIAN_POINT ( 'NONE',  ( 13.89961937509977652, -13.97604488694527269, 93.12390960531436690 ) ) ;
#55036=CARTESIAN_POINT ( 'NONE',  ( -10.81492255796078084, -18.62759615963271287, 107.0822429386476955 ) ) ;
#55037=CARTESIAN_POINT ( 'NONE',  ( -13.97604488694547697, 13.89961937509957934, 73.12609039468568994 ) ) ;
#55038=CARTESIAN_POINT ( 'NONE',  ( -19.02544592524342804, 5.153800228976336051, 101.0405762719810241 ) ) ;
#55039=CARTESIAN_POINT ( 'NONE',  ( 16.46253265017160672, -9.564922557960803928, 28.33224293864769550 ) ) ;
#55040=CARTESIAN_POINT ( 'NONE',  ( -9.564922557960796823, -16.46253265017161027, 72.08224293864770971 ) ) ;
#55041=CARTESIAN_POINT ( 'NONE',  ( 12.14591786802309770, 12.06949235617756955, 54.37390960531435979 ) ) ;
#55042=CARTESIAN_POINT ( 'NONE',  ( -16.51473224551069308, -9.474510206698971260, 36.66557627198102409 ) ) ;
#55043=CARTESIAN_POINT ( 'NONE',  ( -9.564922557961040184, 16.46253265017147172, 57.91775706135233293 ) ) ;
#55044=CARTESIAN_POINT ( 'NONE',  ( -14.29746914071049879, 8.314922557960819915, 85.83224293864768129 ) ) ;
#55045=CARTESIAN_POINT ( 'NONE',  ( 21.52544592524334988, 5.823673210054432836, 106.4594237280190328 ) ) ;
#55046=CARTESIAN_POINT ( 'NONE',  ( 19.02544592524343514, -5.153800228976328945, 53.54057627198102409 ) ) ;
#55047=CARTESIAN_POINT ( 'NONE',  ( -21.52544592524343514, 5.823673210054127303, 56.04057627198102409 ) ) ;
#55048=CARTESIAN_POINT ( 'NONE',  ( 16.52544592524342804, -4.483927247898539470, 53.54057627198103120 ) ) ;
#55049=CARTESIAN_POINT ( 'NONE',  ( 16.46253265017146816, 9.564922557961045513, 21.66775706135233648 ) ) ;
#55050=CARTESIAN_POINT ( 'NONE',  ( 5.153800228976335163, 19.02544592524342804, 109.7905762719810099 ) ) ;
#55051=CARTESIAN_POINT ( 'NONE',  ( 5.049401038298161559, -19.05341960407611168, 102.7072429386476955 ) ) ;
#55052=CARTESIAN_POINT ( 'NONE',  ( 5.049401038298161559, -19.05341960407611168, 37.70724293864768839 ) ) ;
#55053=CARTESIAN_POINT ( 'NONE',  ( 5.049401038298161559, -19.05341960407611168, 27.70724293864769550 ) ) ;
#55054=CARTESIAN_POINT ( 'NONE',  ( 16.53943276465976808, -0.05219959533910856209, 83.74890960531435269 ) ) ;
#55055=CARTESIAN_POINT ( 'NONE',  ( -21.53943276465977519, 0.05219959533907696930, 91.24890960531436690 ) ) ;
#55056=CARTESIAN_POINT ( 'NONE',  ( -9.474510206698964154, 16.51473224551069663, 100.4155762719810241 ) ) ;
#55057=CARTESIAN_POINT ( 'NONE',  ( -18.62759615963270932, 10.81492255796079327, 110.8322429386476955 ) ) ;
#55058=CARTESIAN_POINT ( 'NONE',  ( -19.02544592524342804, 5.153800228976336051, 106.0405762719810241 ) ) ;
#55059=CARTESIAN_POINT ( 'NONE',  ( 8.314922557960818139, 14.29746914071049879, 109.5822429386476955 ) ) ;
#55060=CARTESIAN_POINT ( 'NONE',  ( -13.97604488694527625, -13.89961937509977652, 66.87390960531436690 ) ) ;
#55061=CARTESIAN_POINT ( 'NONE',  ( 5.719274019375991003, -21.55341960407610458, 82.70724293864770971 ) ) ;
#55062=CARTESIAN_POINT ( 'NONE',  ( 16.18388926212238133, -7.379444403734507496, 107.0604684863384790 ) ) ;
#55064=CARTESIAN_POINT ( 'NONE',  ( 15.80617190586746368, 15.72974639402197994, 24.37390960531435979 ) ) ;
#55066=CARTESIAN_POINT ( 'NONE',  ( -4.379528057220086978, -16.55341960407618274, 29.79275706135234358 ) ) ;
#55068=CARTESIAN_POINT ( 'NONE',  ( 0.05219959533910956823, 16.53943276465976808, 99.99890960531436690 ) ) ;
#55069=CARTESIAN_POINT ( 'NONE',  ( -17.49999999999999289, -3.565345528327926505, 110.5750551319352866 ) ) ;
#55070=CARTESIAN_POINT ( 'NONE',  ( -16.51473224551069308, -9.474510206698971260, 61.66557627198103120 ) ) ;
#55071=CARTESIAN_POINT ( 'NONE',  ( 14.29746914071049879, -8.314922557960816363, 83.33224293864769550 ) ) ;
#55072=CARTESIAN_POINT ( 'NONE',  ( -5.823673210054116645, -21.52544592524344225, 37.29057627198102409 ) ) ;
#55073=CARTESIAN_POINT ( 'NONE',  ( -14.29746914071049879, 8.314922557960819915, 70.83224293864770971 ) ) ;
#55074=CARTESIAN_POINT ( 'NONE',  ( 14.29746914071037800, 8.314922557961029526, 21.66775706135235069 ) ) ;
#55075=CARTESIAN_POINT ( 'NONE',  ( -0.05219959533937732626, 21.53943276465977519, 72.50109039468568994 ) ) ;
#55077=CARTESIAN_POINT ( 'NONE',  ( 5.153800228976335163, 19.02544592524342804, 114.7905762719810241 ) ) ;
#55078=CARTESIAN_POINT ( 'NONE',  ( -14.29746914071037622, -8.314922557961029526, 79.16775706135234714 ) ) ;
#55079=CARTESIAN_POINT ( 'NONE',  ( -13.89961937509977652, 13.97604488694528158, 25.62390960531434558 ) ) ;
#55080=CARTESIAN_POINT ( 'NONE',  ( -0.05219959533909027116, -19.03943276465977164, 87.49890960531436690 ) ) ;
#55081=CARTESIAN_POINT ( 'NONE',  ( 18.62759615963271287, -10.81492255796078972, 98.33224293864769550 ) ) ;
#55082=CARTESIAN_POINT ( 'NONE',  ( -16.55341960407617563, 4.379528057220093196, 23.54275706135235424 ) ) ;
#55083=CARTESIAN_POINT ( 'NONE',  ( 16.52544592524342804, -4.483927247898539470, 53.54057627198103120 ) ) ;
#55084=CARTESIAN_POINT ( 'NONE',  ( -15.72974639402176322, -15.80617190586768395, 74.37609039468568994 ) ) ;
#55085=CARTESIAN_POINT ( 'NONE',  ( 16.52544592524335698, 4.483927247898782831, 101.4594237280190185 ) ) ;
#55087=CARTESIAN_POINT ( 'NONE',  ( -16.31925111598456368, 7.325300261831604764, 80.16424538967254421 ) ) ;
#55088=CARTESIAN_POINT ( 'NONE',  ( 16.55341960407618274, -4.379528057220086978, 111.0427570613523613 ) ) ;
#55089=CARTESIAN_POINT ( 'NONE',  ( -12.06949235617739369, -12.14591786802326823, 54.37609039468568994 ) ) ;
#55090=CARTESIAN_POINT ( 'NONE',  ( -0.05219959533909027116, -19.03943276465977164, 67.49890960531436690 ) ) ;
#55091=CARTESIAN_POINT ( 'NONE',  ( -9.564922557960796823, -16.46253265017161027, 92.08224293864769550 ) ) ;
#55092=CARTESIAN_POINT ( 'NONE',  ( -5.719274019375665041, -21.55341960407619695, 69.79275706135234714 ) ) ;
#55094=CARTESIAN_POINT ( 'NONE',  ( 14.34966873604972726, -8.224510206698740333, 80.83442372801901854 ) ) ;
#55095=CARTESIAN_POINT ( 'NONE',  ( 8.314922557960818139, 14.29746914071049879, 64.58224293864769550 ) ) ;
#55096=CARTESIAN_POINT ( 'NONE',  ( 9.564922557960805705, 16.46253265017160317, 49.58224293864770260 ) ) ;
#55098=CARTESIAN_POINT ( 'NONE',  ( -8.224510206698735004, -14.34966873604973081, 19.58442372801901143 ) ) ;
#55099=CARTESIAN_POINT ( 'NONE',  ( 12.06949235617757843, -12.14591786802309237, 113.1239096053143953 ) ) ;
#55100=CARTESIAN_POINT ( 'NONE',  ( -9.564922557960796823, -16.46253265017161027, 77.08224293864769550 ) ) ;
#55101=CARTESIAN_POINT ( 'NONE',  ( -19.05341960407617563, 5.049401038297882671, 98.54275706135233293 ) ) ;
#55103=CARTESIAN_POINT ( 'NONE',  ( -18.67979575497193778, 10.72451020669871902, 108.3344237280190185 ) ) ;
#55104=CARTESIAN_POINT ( 'NONE',  ( 8.314922557961029526, -14.29746914071037800, 75.41775706135233293 ) ) ;
#55105=CARTESIAN_POINT ( 'NONE',  ( -9.564922557961040184, 16.46253265017147172, 92.91775706135233293 ) ) ;
#55106=CARTESIAN_POINT ( 'NONE',  ( -5.823673210054116645, -21.52544592524344225, 57.29057627198103120 ) ) ;
#55107=CARTESIAN_POINT ( 'NONE',  ( -8.314922557961024197, 14.29746914071037800, 67.91775706135234714 ) ) ;
#55109=CARTESIAN_POINT ( 'NONE',  ( 19.03943276465977164, 0.05219959533936151252, 56.25109039468566863 ) ) ;
#55110=CARTESIAN_POINT ( 'NONE',  ( -5.719274019375665041, -21.55341960407619695, 99.79275706135234714 ) ) ;
#55111=CARTESIAN_POINT ( 'NONE',  ( -16.51473224551069308, -9.474510206698971260, 31.66557627198102054 ) ) ;
#55112=CARTESIAN_POINT ( 'NONE',  ( 19.03943276465977164, -0.05219959533909143690, 63.74890960531435979 ) ) ;
#55113=CARTESIAN_POINT ( 'NONE',  ( -14.34966873604960291, -8.224510206698953496, 71.66557627198100988 ) ) ;
#55114=VECTOR ( 'NONE', #28278, 1000.000000000000000 ) ;
#55115=CARTESIAN_POINT ( 'NONE',  ( 21.55341960407619695, -5.719274019375665929, 91.04275706135236135 ) ) ;
#55116=CARTESIAN_POINT ( 'NONE',  ( -13.89961937509957401, -13.97604488694547875, 49.37609039468567573 ) ) ;
#55117=CARTESIAN_POINT ( 'NONE',  ( 19.05341960407617918, -5.049401038297876454, 41.04275706135233293 ) ) ;
#55118=CARTESIAN_POINT ( 'NONE',  ( -21.52544592524343514, 5.823673210054127303, 36.04057627198102409 ) ) ;
#55119=CARTESIAN_POINT ( 'NONE',  ( 10.72451020669871369, 18.67979575497193778, 97.08442372801904696 ) ) ;
#55120=CARTESIAN_POINT ( 'NONE',  ( -19.02544592524342804, 5.153800228976336051, 76.04057627198102409 ) ) ;
#55121=CARTESIAN_POINT ( 'NONE',  ( 18.62759615963255655, 10.81492255796105972, 96.66775706135234714 ) ) ;
#55122=CARTESIAN_POINT ( 'NONE',  ( -21.52544592524343514, 5.823673210054127303, 56.04057627198102409 ) ) ;
#55123=CARTESIAN_POINT ( 'NONE',  ( -0.05219959533909027116, -19.03943276465977164, 87.49890960531436690 ) ) ;
#55124=CARTESIAN_POINT ( 'NONE',  ( 13.89961937509957401, 13.97604488694547697, 76.87609039468566152 ) ) ;
#55125=CARTESIAN_POINT ( 'NONE',  ( 16.51473224551069308, 9.474510206698969483, 94.16557627198103830 ) ) ;
#55126=CARTESIAN_POINT ( 'NONE',  ( -13.89961937509957401, -13.97604488694547875, 99.37609039468567573 ) ) ;
#55127=CARTESIAN_POINT ( 'NONE',  ( -14.29746914071037622, -8.314922557961029526, 49.16775706135234003 ) ) ;
#55128=CARTESIAN_POINT ( 'NONE',  ( -0.05219959533910754901, -16.53943276465976808, 102.4989096053143811 ) ) ;
#55129=CARTESIAN_POINT ( 'NONE',  ( 9.564922557960805705, 16.46253265017160317, 64.58224293864769550 ) ) ;
#55130=CARTESIAN_POINT ( 'NONE',  ( -15.72974639402197994, 15.80617190586746368, 60.62390960531437401 ) ) ;
#55131=CARTESIAN_POINT ( 'NONE',  ( -0.05219959533934338120, 16.53943276465976808, 37.50109039468568284 ) ) ;
#55132=CARTESIAN_POINT ( 'NONE',  ( 10.72451020669871369, 18.67979575497193778, 32.08442372801901854 ) ) ;
#55133=CARTESIAN_POINT ( 'NONE',  ( -10.72451020669870658, -18.67979575497194134, 84.58442372801903275 ) ) ;
#55134=CARTESIAN_POINT ( 'NONE',  ( 8.224510206698742110, 14.34966873604972548, 87.08442372801901854 ) ) ;
#55135=CARTESIAN_POINT ( 'NONE',  ( 5.153800228976335163, 19.02544592524342804, 74.79057627198103830 ) ) ;
#55136=CARTESIAN_POINT ( 'NONE',  ( 8.224510206698953496, -14.34966873604960469, 77.91557627198102409 ) ) ;
#55137=CARTESIAN_POINT ( 'NONE',  ( -16.53943276465976808, -0.05219959533934237506, 108.7510903946857042 ) ) ;
#55138=CARTESIAN_POINT ( 'NONE',  ( -9.474510206698720793, -16.51473224551083518, 59.58442372801900433 ) ) ;
#55139=CARTESIAN_POINT ( 'NONE',  ( 0.05219959533937995610, -21.53943276465977519, 25.00109039468567218 ) ) ;
#55140=CARTESIAN_POINT ( 'NONE',  ( 14.34966873604960469, 8.224510206698951720, 79.16557627198103830 ) ) ;
#55141=CARTESIAN_POINT ( 'NONE',  ( 19.03943276465977164, -0.05219959533909143690, 103.7489096053143669 ) ) ;
#55142=CARTESIAN_POINT ( 'NONE',  ( 14.34966873604972726, -8.224510206698740333, 100.8344237280190185 ) ) ;
#55143=CARTESIAN_POINT ( 'NONE',  ( -21.53943276465977519, -0.05219959533937600094, 78.75109039468568994 ) ) ;
#55144=CARTESIAN_POINT ( 'NONE',  ( -4.379528057220086978, -16.55341960407618274, 39.79275706135235424 ) ) ;
#55145=CARTESIAN_POINT ( 'NONE',  ( -21.53943276465977519, -0.05219959533937600094, 33.75109039468568284 ) ) ;
#55146=CARTESIAN_POINT ( 'NONE',  ( -14.34966873604960291, -8.224510206698953496, 71.66557627198100988 ) ) ;
#55148=CARTESIAN_POINT ( 'NONE',  ( 5.823673210054125526, 21.52544592524343514, 109.7905762719810383 ) ) ;
#55150=CARTESIAN_POINT ( 'NONE',  ( 16.55341960407611168, 4.379528057220329451, 58.95724293864770971 ) ) ;
#55151=CARTESIAN_POINT ( 'NONE',  ( -30.00000000000000000, -5.510910596163089556E-15, 45.00000000000000000 ) ) ;
#55152=CARTESIAN_POINT ( 'NONE',  ( 21.55341960407610458, 5.719274019375980345, 33.95724293864769550 ) ) ;
#55153=CARTESIAN_POINT ( 'NONE',  ( 16.52544592524342804, -4.483927247898539470, 73.54057627198102409 ) ) ;
#55154=CARTESIAN_POINT ( 'NONE',  ( -18.62759615963270932, 10.81492255796079327, 85.83224293864768129 ) ) ;
#55155=CARTESIAN_POINT ( 'NONE',  ( 13.89961937509977652, -13.97604488694527269, 73.12390960531436690 ) ) ;
#55156=CARTESIAN_POINT ( 'NONE',  ( 16.46253265017160672, -9.564922557960803928, 38.33224293864768839 ) ) ;
#55157=CARTESIAN_POINT ( 'NONE',  ( -19.05341960407617563, 5.049401038297882671, 78.54275706135233293 ) ) ;
#55158=CARTESIAN_POINT ( 'NONE',  ( 18.62759615963255655, 10.81492255796105972, 56.66775706135235424 ) ) ;
#55159=CARTESIAN_POINT ( 'NONE',  ( -18.67979575497178146, -10.72451020669898902, 56.66557627198103830 ) ) ;
#55160=CARTESIAN_POINT ( 'NONE',  ( -19.02544592524342804, 5.153800228976336051, 46.04057627198101699 ) ) ;
#55161=CARTESIAN_POINT ( 'NONE',  ( 13.89961937509977652, -13.97604488694527269, 68.12390960531436690 ) ) ;
#55163=CARTESIAN_POINT ( 'NONE',  ( -4.483927247898782831, 16.52544592524335698, 52.70942372801902565 ) ) ;
#55164=CARTESIAN_POINT ( 'NONE',  ( -21.53943276465977519, -0.05219959533937600094, 33.75109039468568284 ) ) ;
#55165=CARTESIAN_POINT ( 'NONE',  ( 0.05219959533937995610, -21.53943276465977519, 60.00109039468568284 ) ) ;
#55166=CARTESIAN_POINT ( 'NONE',  ( -13.89961937509977652, 13.97604488694528158, 110.6239096053143243 ) ) ;
#55167=CARTESIAN_POINT ( 'NONE',  ( 15.80617190586746368, 15.72974639402197994, 84.37390960531438111 ) ) ;
#55168=CARTESIAN_POINT ( 'NONE',  ( 21.55341960407619695, -5.719274019375665929, 21.04275706135234714 ) ) ;
#55169=CARTESIAN_POINT ( 'NONE',  ( 14.34966873604972726, -8.224510206698740333, 50.83442372801901143 ) ) ;
#55171=CARTESIAN_POINT ( 'NONE',  ( 10.81492255796078972, 18.62759615963270932, 44.58224293864769550 ) ) ;
#55172=CARTESIAN_POINT ( 'NONE',  ( 16.51473224551083163, -9.474510206698727899, 20.83442372801899722 ) ) ;
#55173=CARTESIAN_POINT ( 'NONE',  ( -13.97604488694527625, -13.89961937509977652, 51.87390960531436690 ) ) ;
#55174=CARTESIAN_POINT ( 'NONE',  ( -5.049401038298153566, 19.05341960407611168, 115.2072429386477097 ) ) ;
#55175=B_SPLINE_CURVE_WITH_KNOTS ( 'NONE', 3,
 ( #4838, #190873, #128188, #113022, #193883, #58350, #101854, #86681, #136188, #196884, #59330, #43184, #87680, #27038, #165541, #135212, #12858, #120018, #121000, #181703, #88684, #74523, #73539, #104853, #42199, #197863, #57369, #182698, #28040, #44183, #103860, #119042 ),
 .UNSPECIFIED., .F., .F.,
 ( 4, 2, 2, 2, 2, 2, 2, 2, 2, 2, 2, 2, 2, 2, 2, 4 ),
 ( 2.711112516444420852E-17, 0.0003712461730036841758, 0.0007424923460073412466, 0.001113738519010998426, 0.001484984692014655388, 0.002227477038021976469, 0.002598723211025651212, 0.002969969384029325955, 0.003341215557033000699, 0.003712461730036675876, 0.004083707903040349751, 0.004454954076044024928, 0.004826200249047700105, 0.005197446422051375282, 0.005568692595055049592, 0.005939938768058724769 ),
 .UNSPECIFIED. ) ;
#55176=CARTESIAN_POINT ( 'NONE',  ( -0.05219959533909027116, -19.03943276465977164, 87.49890960531436690 ) ) ;
#55177=CARTESIAN_POINT ( 'NONE',  ( 17.50000000000005329, 3.438020150447535173, 102.9915581553581063 ) ) ;
#55178=CARTESIAN_POINT ( 'NONE',  ( -9.474510206698720793, -16.51473224551083518, 74.58442372801900433 ) ) ;
#55179=CARTESIAN_POINT ( 'NONE',  ( -15.72974639402197994, 15.80617190586746368, 45.62390960531436690 ) ) ;
#55180=CARTESIAN_POINT ( 'NONE',  ( -16.53943276465976808, 0.05219959533911058130, 31.24890960531435979 ) ) ;
#55181=CARTESIAN_POINT ( 'NONE',  ( 19.03943276465977164, 0.05219959533936151252, 91.25109039468566152 ) ) ;
#55182=CARTESIAN_POINT ( 'NONE',  ( 5.049401038298161559, -19.05341960407611168, 22.70724293864769194 ) ) ;
#55183=CARTESIAN_POINT ( 'NONE',  ( -0.05219959533937732626, 21.53943276465977519, 112.5010903946857042 ) ) ;
#55184=CARTESIAN_POINT ( 'NONE',  ( -19.03943276465977164, -0.05219959533935918106, 93.75109039468566152 ) ) ;
#55185=CARTESIAN_POINT ( 'NONE',  ( 9.564922557961047289, -16.46253265017146816, 45.41775706135232582 ) ) ;
#55186=CARTESIAN_POINT ( 'NONE',  ( 17.40805194822032220, 6.112264579159320199, 106.6662872748939037 ) ) ;
#55187=CARTESIAN_POINT ( 'NONE',  ( -9.474510206698964154, 16.51473224551069663, 50.41557627198102409 ) ) ;
#55188=CARTESIAN_POINT ( 'NONE',  ( 8.314922557960818139, 14.29746914071049879, 69.58224293864769550 ) ) ;
#55189=CARTESIAN_POINT ( 'NONE',  ( 19.05341960407611168, 5.049401038298154454, 33.95724293864769550 ) ) ;
#55190=CARTESIAN_POINT ( 'NONE',  ( 12.14591786802309770, 12.06949235617756955, 34.37390960531435979 ) ) ;
#55192=CARTESIAN_POINT ( 'NONE',  ( 4.483927247898790824, -16.52544592524335698, 110.2094237280190185 ) ) ;
#55193=CARTESIAN_POINT ( 'NONE',  ( -0.05219959533909027116, -19.03943276465977164, 57.49890960531435979 ) ) ;
#55194=CARTESIAN_POINT ( 'NONE',  ( -9.474510206698720793, -16.51473224551083518, 19.58442372801899722 ) ) ;
#55195=CARTESIAN_POINT ( 'NONE',  ( 8.314922557961029526, -14.29746914071037800, 35.41775706135234003 ) ) ;
#55196=CARTESIAN_POINT ( 'NONE',  ( 10.72451020669898902, -18.67979575497178502, 42.91557627198103120 ) ) ;
#55197=CARTESIAN_POINT ( 'NONE',  ( -0.05219959533937732626, 21.53943276465977519, 102.5010903946856899 ) ) ;
#55198=VERTEX_POINT ( 'NONE', #151944 ) ;
#55199=CARTESIAN_POINT ( 'NONE',  ( -13.97604488694527625, -13.89961937509977652, 66.87390960531436690 ) ) ;
#55200=CARTESIAN_POINT ( 'NONE',  ( 5.049401038298161559, -19.05341960407611168, 102.7072429386476955 ) ) ;
#55201=CARTESIAN_POINT ( 'NONE',  ( 13.97604488694527802, 13.89961937509977652, 94.37390960531436690 ) ) ;
#55203=CARTESIAN_POINT ( 'NONE',  ( 21.52544592524334988, 5.823673210054432836, 31.45942372801901854 ) ) ;
#55204=CARTESIAN_POINT ( 'NONE',  ( -14.29746914071049879, 8.314922557960819915, 90.83224293864769550 ) ) ;
#55205=CARTESIAN_POINT ( 'NONE',  ( -0.05219959533907301413, -21.53943276465977519, 82.49890960531436690 ) ) ;
#55206=CARTESIAN_POINT ( 'NONE',  ( 19.02544592524343514, -5.153800228976328945, 63.54057627198103830 ) ) ;
#55207=CARTESIAN_POINT ( 'NONE',  ( -13.97604488694527625, -13.89961937509977652, 66.87390960531436690 ) ) ;
#55208=CARTESIAN_POINT ( 'NONE',  ( 5.719274019375991003, -21.55341960407610458, 107.7072429386476955 ) ) ;
#55209=ORIENTED_EDGE ( 'NONE', *, *, #149359, .T. ) ;
#55210=CARTESIAN_POINT ( 'NONE',  ( 9.564922557960805705, 16.46253265017160317, 79.58224293864769550 ) ) ;
#55212=CARTESIAN_POINT ( 'NONE',  ( 4.483927247898545687, 16.52544592524342804, 104.7905762719810241 ) ) ;
#55214=CARTESIAN_POINT ( 'NONE',  ( -0.05219959533909027116, -19.03943276465977164, 67.49890960531436690 ) ) ;
#55215=CARTESIAN_POINT ( 'NONE',  ( 19.03943276465977164, 0.05219959533936151252, 91.25109039468566152 ) ) ;
#55216=CARTESIAN_POINT ( 'NONE',  ( 16.55341960407611168, 4.379528057220329451, 93.95724293864770971 ) ) ;
#55217=CARTESIAN_POINT ( 'NONE',  ( -21.55341960407619339, 5.719274019375674811, 78.54275706135236135 ) ) ;
#55218=CARTESIAN_POINT ( 'NONE',  ( -16.51473224551069308, -9.474510206698971260, 46.66557627198102409 ) ) ;
#55219=CARTESIAN_POINT ( 'NONE',  ( -18.62759615963255300, -10.81492255796106328, 24.16775706135235424 ) ) ;
#55220=CARTESIAN_POINT ( 'NONE',  ( -5.823673210054116645, -21.52544592524344225, 112.2905762719810241 ) ) ;
#55222=CARTESIAN_POINT ( 'NONE',  ( -19.05341960407611168, -5.049401038298163336, 66.45724293864769550 ) ) ;
#55223=CARTESIAN_POINT ( 'NONE',  ( 17.50000000000000000, 5.499999999999997335, 111.7030961746582847 ) ) ;
#55224=CARTESIAN_POINT ( 'NONE',  ( -13.97604488694547697, 13.89961937509957934, 103.1260903946856473 ) ) ;
#55225=CARTESIAN_POINT ( 'NONE',  ( 5.823673210054125526, 21.52544592524343514, 29.79057627198102409 ) ) ;
#55226=CARTESIAN_POINT ( 'NONE',  ( 21.52544592524334988, 5.823673210054432836, 61.45942372801901854 ) ) ;
#55227=CARTESIAN_POINT ( 'NONE',  ( -5.049401038298153566, 19.05341960407611168, 100.2072429386476955 ) ) ;
#55228=CARTESIAN_POINT ( 'NONE',  ( -19.02544592524334988, -5.153800228976617603, 83.95942372801901854 ) ) ;
#55229=CARTESIAN_POINT ( 'NONE',  ( -13.89961937509977652, 13.97604488694528158, 45.62390960531433848 ) ) ;
#55230=CARTESIAN_POINT ( 'NONE',  ( -13.97604488694527625, -13.89961937509977652, 66.87390960531436690 ) ) ;
#55231=CARTESIAN_POINT ( 'NONE',  ( 0.05219959533910956823, 16.53943276465976808, 74.99890960531435269 ) ) ;
#55232=CARTESIAN_POINT ( 'NONE',  ( -5.153800228976328057, -19.02544592524343514, 97.29057627198099567 ) ) ;
#55233=CARTESIAN_POINT ( 'NONE',  ( 14.29746914071049879, -8.314922557960816363, 98.33224293864769550 ) ) ;
#55234=CARTESIAN_POINT ( 'NONE',  ( -5.153800228976328057, -19.02544592524343514, 102.2905762719810383 ) ) ;
#55235=CARTESIAN_POINT ( 'NONE',  ( 4.483927247898545687, 16.52544592524342804, 44.79057627198103120 ) ) ;
#55237=CARTESIAN_POINT ( 'NONE',  ( -5.153800228976328057, -19.02544592524343514, 22.29057627198102765 ) ) ;
#55238=ORIENTED_EDGE ( 'NONE', *, *, #112928, .T. ) ;
#55239=CARTESIAN_POINT ( 'NONE',  ( -18.62759615963255300, -10.81492255796106328, 54.16775706135235424 ) ) ;
#55240=CARTESIAN_POINT ( 'NONE',  ( -9.474510206698720793, -16.51473224551083518, 74.58442372801900433 ) ) ;
#55241=CARTESIAN_POINT ( 'NONE',  ( 4.483927247898545687, 16.52544592524342804, 54.79057627198104541 ) ) ;
#55242=CARTESIAN_POINT ( 'NONE',  ( 10.81492255796078972, 18.62759615963270932, 104.5822429386477097 ) ) ;
#55243=CARTESIAN_POINT ( 'NONE',  ( -10.81492255796078084, -18.62759615963271287, 32.08224293864769550 ) ) ;
#55244=CARTESIAN_POINT ( 'NONE',  ( -14.34966873604960291, -8.224510206698953496, 86.66557627198102409 ) ) ;
#55245=CARTESIAN_POINT ( 'NONE',  ( 9.474510206698971260, -16.51473224551069308, 52.91557627198102409 ) ) ;
#55246=CARTESIAN_POINT ( 'NONE',  ( -8.314922557960811034, -14.29746914071050412, 27.08224293864769550 ) ) ;
#55247=CARTESIAN_POINT ( 'NONE',  ( 14.34966873604972726, -8.224510206698740333, 100.8344237280190185 ) ) ;
#55248=CARTESIAN_POINT ( 'NONE',  ( -8.224510206698735004, -14.34966873604973081, 69.58442372801900433 ) ) ;
#55249=CARTESIAN_POINT ( 'NONE',  ( 5.049401038297881783, 19.05341960407617563, 27.29275706135232937 ) ) ;
#55250=CARTESIAN_POINT ( 'NONE',  ( -9.474510206698964154, 16.51473224551069663, 100.4155762719810241 ) ) ;
#55251=CARTESIAN_POINT ( 'NONE',  ( 5.153800228976335163, 19.02544592524342804, 74.79057627198103830 ) ) ;
#55252=CARTESIAN_POINT ( 'NONE',  ( -0.05219959533909027116, -19.03943276465977164, 42.49890960531435269 ) ) ;
#55253=CARTESIAN_POINT ( 'NONE',  ( -8.314922557960811034, -14.29746914071050412, 47.08224293864770260 ) ) ;
#55255=CARTESIAN_POINT ( 'NONE',  ( 9.474510206698971260, -16.51473224551069308, 102.9155762719810241 ) ) ;
#55256=CARTESIAN_POINT ( 'NONE',  ( 10.72451020669898902, -18.67979575497178502, 37.91557627198102409 ) ) ;
#55257=CARTESIAN_POINT ( 'NONE',  ( -16.52544592524342804, 4.483927247898546575, 76.04057627198102409 ) ) ;
#55258=CARTESIAN_POINT ( 'NONE',  ( -4.483927247898782831, 16.52544592524335698, 27.70942372801901854 ) ) ;
#55259=CARTESIAN_POINT ( 'NONE',  ( 12.14591786802309770, 12.06949235617756955, 69.37390960531436690 ) ) ;
#55261=CARTESIAN_POINT ( 'NONE',  ( -16.46253265017146816, -9.564922557961047289, 59.16775706135233293 ) ) ;
#55262=CARTESIAN_POINT ( 'NONE',  ( -9.474510206698964154, 16.51473224551069663, 105.4155762719810383 ) ) ;
#55263=CARTESIAN_POINT ( 'NONE',  ( 5.049401038297881783, 19.05341960407617563, 82.29275706135229029 ) ) ;
#55265=CARTESIAN_POINT ( 'NONE',  ( -9.564922557961040184, 16.46253265017147172, 107.9177570613523471 ) ) ;
#55266=CARTESIAN_POINT ( 'NONE',  ( -12.06949235617739369, -12.14591786802326823, 94.37609039468568994 ) ) ;
#55267=CARTESIAN_POINT ( 'NONE',  ( 13.97604488694527802, 13.89961937509977652, 39.37390960531435269 ) ) ;
#55268=CARTESIAN_POINT ( 'NONE',  ( -21.52544592524343514, 5.823673210054127303, 31.04057627198102409 ) ) ;
#55269=CARTESIAN_POINT ( 'NONE',  ( -15.80617190586768217, 15.72974639402176855, 58.12609039468568994 ) ) ;
#55271=CARTESIAN_POINT ( 'NONE',  ( -0.05219959533934338120, 16.53943276465976808, 22.50109039468567573 ) ) ;
#55272=CARTESIAN_POINT ( 'NONE',  ( 17.50000000000122924, 3.258327458701826718, 22.81645961510181664 ) ) ;
#55273=CARTESIAN_POINT ( 'NONE',  ( 13.97604488694527802, 13.89961937509977652, 69.37390960531436690 ) ) ;
#55274=CARTESIAN_POINT ( 'NONE',  ( -4.483927247898539470, -16.52544592524342804, 82.29057627198103830 ) ) ;
#55275=CARTESIAN_POINT ( 'NONE',  ( -5.049401038298153566, 19.05341960407611168, 70.20724293864769550 ) ) ;
#55276=CARTESIAN_POINT ( 'NONE',  ( 19.02544592524343514, -5.153800228976328945, 83.54057627198100988 ) ) ;
#55277=VERTEX_POINT ( 'NONE', #105439 ) ;
#55278=CARTESIAN_POINT ( 'NONE',  ( 16.51473224551083163, -9.474510206698727899, 85.83442372801900433 ) ) ;
#55279=CARTESIAN_POINT ( 'NONE',  ( -0.05219959533907301413, -21.53943276465977519, 67.49890960531436690 ) ) ;
#55280=CARTESIAN_POINT ( 'NONE',  ( 9.564922557960805705, 16.46253265017160317, 34.58224293864770260 ) ) ;
#55281=CARTESIAN_POINT ( 'NONE',  ( 16.46253265017146816, 9.564922557961045513, 56.66775706135233293 ) ) ;
#55282=CARTESIAN_POINT ( 'NONE',  ( -5.049401038298153566, 19.05341960407611168, 50.20724293864770260 ) ) ;
#55283=CARTESIAN_POINT ( 'NONE',  ( -5.153800228976328057, -19.02544592524343514, 87.29057627198103830 ) ) ;
#55285=CARTESIAN_POINT ( 'NONE',  ( -0.05219959533907301413, -21.53943276465977519, 92.49890960531436690 ) ) ;
#55286=CARTESIAN_POINT ( 'NONE',  ( -0.05219959533910754901, -16.53943276465976808, 97.49890960531436690 ) ) ;
#55287=CARTESIAN_POINT ( 'NONE',  ( -19.05341960407611168, -5.049401038298163336, 86.45724293864769550 ) ) ;
#55288=CARTESIAN_POINT ( 'NONE',  ( 19.05341960407617918, -5.049401038297876454, 66.04275706135233293 ) ) ;
#55289=CARTESIAN_POINT ( 'NONE',  ( -10.72451020669898014, 18.67979575497178502, 90.41557627198103830 ) ) ;
#55290=CARTESIAN_POINT ( 'NONE',  ( 10.72451020669898902, -18.67979575497178502, 77.91557627198102409 ) ) ;
#55291=CARTESIAN_POINT ( 'NONE',  ( 4.483927247898545687, 16.52544592524342804, 29.79057627198102409 ) ) ;
#55292=CARTESIAN_POINT ( 'NONE',  ( -18.67979575497193778, 10.72451020669871902, 108.3344237280190185 ) ) ;
#55293=CARTESIAN_POINT ( 'NONE',  ( -14.34966873604972548, 8.224510206698743886, 53.33442372801901854 ) ) ;
#55294=CARTESIAN_POINT ( 'NONE',  ( -5.049401038298153566, 19.05341960407611168, 75.20724293864769550 ) ) ;
#55295=CARTESIAN_POINT ( 'NONE',  ( -13.97604488694527625, -13.89961937509977652, 36.87390960531436690 ) ) ;
#55296=CARTESIAN_POINT ( 'NONE',  ( -15.80617190586768217, 15.72974639402176855, 33.12609039468569705 ) ) ;
#55297=CARTESIAN_POINT ( 'NONE',  ( -5.823673210054431948, 21.52544592524334988, 57.70942372801901143 ) ) ;
#55298=CARTESIAN_POINT ( 'NONE',  ( -9.474510206698964154, 16.51473224551069663, 45.41557627198103120 ) ) ;
#55299=CARTESIAN_POINT ( 'NONE',  ( -10.81492255796105439, 18.62759615963255655, 22.91775706135235069 ) ) ;
#55300=CARTESIAN_POINT ( 'NONE',  ( 0.05219959533936267826, -19.03943276465977164, 70.00109039468566152 ) ) ;
#55301=CARTESIAN_POINT ( 'NONE',  ( -16.51473224551082808, 9.474510206698731452, 78.33442372801900433 ) ) ;
#55302=CARTESIAN_POINT ( 'NONE',  ( -9.474510206698964154, 16.51473224551069663, 30.41557627198102054 ) ) ;
#55303=CARTESIAN_POINT ( 'NONE',  ( 0.05219959533934541429, -16.53943276465976808, 75.00109039468568994 ) ) ;
#55304=CARTESIAN_POINT ( 'NONE',  ( -13.97604488694527625, -13.89961937509977652, 46.87390960531435979 ) ) ;
#55306=CARTESIAN_POINT ( 'NONE',  ( 19.03943276465977164, -0.05219959533909143690, 93.74890960531435269 ) ) ;
#55307=CARTESIAN_POINT ( 'NONE',  ( -8.224510206698948167, 14.34966873604960824, 115.4155762719810241 ) ) ;
#55308=CARTESIAN_POINT ( 'NONE',  ( -15.80617190586745835, -15.72974639402198527, 66.87390960531436690 ) ) ;
#55309=CARTESIAN_POINT ( 'NONE',  ( 12.14591786802327356, -12.06949235617739191, 55.62609039468568284 ) ) ;
#55310=CARTESIAN_POINT ( 'NONE',  ( -19.03943276465977164, -0.05219959533935918106, 23.75109039468566152 ) ) ;
#55312=CARTESIAN_POINT ( 'NONE',  ( 19.03943276465977164, -0.05219959533909143690, 48.74890960531435979 ) ) ;
#55313=CARTESIAN_POINT ( 'NONE',  ( 12.14591786802309770, 12.06949235617756955, 29.37390960531435269 ) ) ;
#55314=CARTESIAN_POINT ( 'NONE',  ( 0.05219959533910956823, 16.53943276465976808, 69.99890960531435269 ) ) ;
#55315=CARTESIAN_POINT ( 'NONE',  ( -16.46253265017160317, 9.564922557960807481, 75.83224293864769550 ) ) ;
#55316=CARTESIAN_POINT ( 'NONE',  ( 21.53943276465977519, 0.05219959533937863772, 36.25109039468567573 ) ) ;
#55317=CARTESIAN_POINT ( 'NONE',  ( -13.97604488694527625, -13.89961937509977652, 86.87390960531436690 ) ) ;
#55318=CARTESIAN_POINT ( 'NONE',  ( -21.55341960407619339, 5.719274019375674811, 98.54275706135234714 ) ) ;
#55319=CARTESIAN_POINT ( 'NONE',  ( 16.55341960407618274, -4.379528057220086978, 66.04275706135236135 ) ) ;
#55320=CARTESIAN_POINT ( 'NONE',  ( 16.46253265017160672, -9.564922557960803928, 113.3322429386476955 ) ) ;
#55321=CARTESIAN_POINT ( 'NONE',  ( -21.53943276465977519, 0.05219959533907696930, 91.24890960531436690 ) ) ;
#55322=CARTESIAN_POINT ( 'NONE',  ( 0.05219959533910956823, 16.53943276465976808, 44.99890960531435979 ) ) ;
#55323=CARTESIAN_POINT ( 'NONE',  ( 16.51473224551069308, 9.474510206698969483, 29.16557627198103475 ) ) ;
#55324=CARTESIAN_POINT ( 'NONE',  ( -4.483927247898782831, 16.52544592524335698, 52.70942372801902565 ) ) ;
#55325=CARTESIAN_POINT ( 'NONE',  ( -0.05219959533910754901, -16.53943276465976808, 72.49890960531435269 ) ) ;
#55326=CARTESIAN_POINT ( 'NONE',  ( -19.03943276465977164, 0.05219959533909376836, 116.2489096053143669 ) ) ;
#55327=CARTESIAN_POINT ( 'NONE',  ( -15.80617190586745835, -15.72974639402198527, 26.87390960531435979 ) ) ;
#55328=CARTESIAN_POINT ( 'NONE',  ( -9.564922557961040184, 16.46253265017147172, 22.91775706135233648 ) ) ;
#55330=CARTESIAN_POINT ( 'NONE',  ( -4.483927247898539470, -16.52544592524342804, 102.2905762719810383 ) ) ;
#55331=CARTESIAN_POINT ( 'NONE',  ( 19.03943276465977164, -0.05219959533909143690, 103.7489096053143669 ) ) ;
#55332=EDGE_LOOP ( 'NONE', ( #113752, #9608, #102417, #11030 ) ) ;
#55333=CARTESIAN_POINT ( 'NONE',  ( 14.29746914071037800, 8.314922557961029526, 51.66775706135234714 ) ) ;
#55334=CARTESIAN_POINT ( 'NONE',  ( -19.03943276465977164, 0.05219959533909376836, 56.24890960531435979 ) ) ;
#55335=CARTESIAN_POINT ( 'NONE',  ( -16.74176944037747106, -6.099830512274460048, 20.54535278272281573 ) ) ;
#55336=CARTESIAN_POINT ( 'NONE',  ( -5.153800228976607833, 19.02544592524334988, 52.70942372801900433 ) ) ;
#55337=CARTESIAN_POINT ( 'NONE',  ( 8.224510206698742110, 14.34966873604972548, 92.08442372801901854 ) ) ;
#55338=CARTESIAN_POINT ( 'NONE',  ( -16.46253265017146816, -9.564922557961047289, 99.16775706135233293 ) ) ;
#55339=CARTESIAN_POINT ( 'NONE',  ( 21.53943276465977519, 0.05219959533937863772, 61.25109039468567573 ) ) ;
#55340=CARTESIAN_POINT ( 'NONE',  ( -13.89961937509977652, 13.97604488694528158, 70.62390960531432427 ) ) ;
#55341=CARTESIAN_POINT ( 'NONE',  ( -18.62759615963270932, 10.81492255796079327, 90.83224293864769550 ) ) ;
#55342=CARTESIAN_POINT ( 'NONE',  ( -8.314922557960811034, -14.29746914071050412, 107.0822429386476955 ) ) ;
#55343=CARTESIAN_POINT ( 'NONE',  ( 5.153800228976615827, -19.02544592524334988, 85.20942372801900433 ) ) ;
#55344=CARTESIAN_POINT ( 'NONE',  ( 5.719274019375991003, -21.55341960407610458, 72.70724293864769550 ) ) ;
#55345=CARTESIAN_POINT ( 'NONE',  ( -5.153800228976607833, 19.02544592524334988, 37.70942372801899722 ) ) ;
#55346=CARTESIAN_POINT ( 'NONE',  ( -13.89961937509977652, 13.97604488694528158, 115.6239096053143669 ) ) ;
#55347=CARTESIAN_POINT ( 'NONE',  ( -15.72974639402197994, 15.80617190586746368, 85.62390960531436690 ) ) ;
#55348=CARTESIAN_POINT ( 'NONE',  ( -19.49149378614658090, 5.499999999999777067, 54.43757513605361709 ) ) ;
#55349=CARTESIAN_POINT ( 'NONE',  ( 5.153800228976335163, 19.02544592524342804, 69.79057627198103830 ) ) ;
#55351=CARTESIAN_POINT ( 'NONE',  ( -16.53943276465976808, -0.05219959533934237506, 23.75109039468567929 ) ) ;
#55353=CARTESIAN_POINT ( 'NONE',  ( 19.03943276465977164, -0.05219959533909143690, 43.74890960531435979 ) ) ;
#55354=CARTESIAN_POINT ( 'NONE',  ( -21.53943276465977519, 0.05219959533907696930, 21.24890960531436690 ) ) ;
#55355=CARTESIAN_POINT ( 'NONE',  ( 10.72451020669898902, -18.67979575497178502, 107.9155762719810241 ) ) ;
#55356=CARTESIAN_POINT ( 'NONE',  ( -16.53943276465976808, 0.05219959533911058130, 46.24890960531435979 ) ) ;
#55357=CARTESIAN_POINT ( 'NONE',  ( 10.72451020669871369, 18.67979575497193778, 72.08442372801899012 ) ) ;
#55358=CARTESIAN_POINT ( 'NONE',  ( 12.06949235617739724, 12.14591786802326823, 26.87609039468567218 ) ) ;
#55359=CARTESIAN_POINT ( 'NONE',  ( -13.97604488694547697, 13.89961937509957934, 23.12609039468565442 ) ) ;
#55360=CARTESIAN_POINT ( 'NONE',  ( 4.379528057220339221, -16.55341960407611168, 27.70724293864769905 ) ) ;
#55361=CARTESIAN_POINT ( 'NONE',  ( -10.81492255796078084, -18.62759615963271287, 112.0822429386477097 ) ) ;
#55362=CARTESIAN_POINT ( 'NONE',  ( 8.224510206698953496, -14.34966873604960469, 52.91557627198103830 ) ) ;
#55363=CARTESIAN_POINT ( 'NONE',  ( -13.97604488694547697, 13.89961937509957934, 98.12609039468566152 ) ) ;
#55364=CARTESIAN_POINT ( 'NONE',  ( -13.89961937509957401, -13.97604488694547875, 69.37609039468564731 ) ) ;
#55365=CARTESIAN_POINT ( 'NONE',  ( 5.719274019375673035, 21.55341960407619339, 72.29275706135236135 ) ) ;
#55366=CARTESIAN_POINT ( 'NONE',  ( -13.89961937509957401, -13.97604488694547875, 59.37609039468566863 ) ) ;
#55367=CARTESIAN_POINT ( 'NONE',  ( 16.55341960407611168, 4.379528057220329451, 113.9572429386477239 ) ) ;
#55368=CARTESIAN_POINT ( 'NONE',  ( -21.55341960407610458, -5.719274019375992779, 46.45724293864769550 ) ) ;
#55369=CARTESIAN_POINT ( 'NONE',  ( -4.483927247898539470, -16.52544592524342804, 47.29057627198103120 ) ) ;
#55370=CARTESIAN_POINT ( 'NONE',  ( -19.52217212775661181, 5.499999999999920064, 94.93993709005262360 ) ) ;
#55371=CARTESIAN_POINT ( 'NONE',  ( 18.62759615963255655, 10.81492255796105972, 106.6677570613523756 ) ) ;
#55372=CARTESIAN_POINT ( 'NONE',  ( 16.52544592524335698, 4.483927247898782831, 86.45942372801901854 ) ) ;
#55373=CARTESIAN_POINT ( 'NONE',  ( 14.34966873604960469, 8.224510206698951720, 34.16557627198102409 ) ) ;
#55374=CARTESIAN_POINT ( 'NONE',  ( -18.62759615963255300, -10.81492255796106328, 79.16775706135234714 ) ) ;
#55375=CARTESIAN_POINT ( 'NONE',  ( -21.52544592524334988, -5.823673210054445271, 83.95942372801900433 ) ) ;
#55376=CARTESIAN_POINT ( 'NONE',  ( 15.80617190586746368, 15.72974639402197994, 79.37390960531436690 ) ) ;
#55377=CARTESIAN_POINT ( 'NONE',  ( 5.049401038298161559, -19.05341960407611168, 32.70724293864768129 ) ) ;
#55378=CARTESIAN_POINT ( 'NONE',  ( 18.62759615963255655, 10.81492255796105972, 56.66775706135235424 ) ) ;
#55379=CARTESIAN_POINT ( 'NONE',  ( 9.564922557960805705, 16.46253265017160317, 39.58224293864768839 ) ) ;
#55380=CARTESIAN_POINT ( 'NONE',  ( 5.049401038298161559, -19.05341960407611168, 57.70724293864769550 ) ) ;
#55381=CARTESIAN_POINT ( 'NONE',  ( 16.55341960407611168, 4.379528057220329451, 93.95724293864770971 ) ) ;
#55382=CARTESIAN_POINT ( 'NONE',  ( 16.51473224551069308, 9.474510206698969483, 94.16557627198103830 ) ) ;
#55383=CARTESIAN_POINT ( 'NONE',  ( -12.06949235617756955, 12.14591786802309770, 35.62390960531437401 ) ) ;
#55384=CARTESIAN_POINT ( 'NONE',  ( -12.06949235617756955, 12.14591786802309770, 110.6239096053143669 ) ) ;
#55385=CARTESIAN_POINT ( 'NONE',  ( -18.67979575497178146, -10.72451020669898902, 86.66557627198102409 ) ) ;
#55386=CARTESIAN_POINT ( 'NONE',  ( 5.823673210054444382, -21.52544592524334988, 20.20942372801900788 ) ) ;
#55388=CARTESIAN_POINT ( 'NONE',  ( 19.02544592524343514, -5.153800228976328945, 83.54057627198100988 ) ) ;
#55389=CARTESIAN_POINT ( 'NONE',  ( -16.53943276465976808, -0.05219959533934237506, 18.75109039468568639 ) ) ;
#55390=CARTESIAN_POINT ( 'NONE',  ( -18.67979575497178146, -10.72451020669898902, 71.66557627198100988 ) ) ;
#55391=CARTESIAN_POINT ( 'NONE',  ( -15.72974639402176322, -15.80617190586768395, 94.37609039468568994 ) ) ;
#55392=CARTESIAN_POINT ( 'NONE',  ( -13.97604488694527625, -13.89961937509977652, 76.87390960531433848 ) ) ;
#55393=CARTESIAN_POINT ( 'NONE',  ( -21.52544592524334988, -5.823673210054445271, 33.95942372801901143 ) ) ;
#55394=CARTESIAN_POINT ( 'NONE',  ( 13.97604488694527802, 13.89961937509977652, 114.3739096053143669 ) ) ;
#55395=CARTESIAN_POINT ( 'NONE',  ( -16.53943276465976808, -0.05219959533934237506, 88.75109039468567573 ) ) ;
#55396=CARTESIAN_POINT ( 'NONE',  ( 18.67979575497194134, -10.72451020669871369, 70.83442372801901854 ) ) ;
#55397=CARTESIAN_POINT ( 'NONE',  ( 18.62759615963255655, 10.81492255796105972, 101.6677570613523613 ) ) ;
#55398=CARTESIAN_POINT ( 'NONE',  ( 16.53943276465976808, 0.05219959533934440121, 76.25109039468568994 ) ) ;
#55399=CARTESIAN_POINT ( 'NONE',  ( -10.81492255796105439, 18.62759615963255655, 27.91775706135234358 ) ) ;
#55400=CARTESIAN_POINT ( 'NONE',  ( 9.564922557960805705, 16.46253265017160317, 24.58224293864769194 ) ) ;
#55401=CARTESIAN_POINT ( 'NONE',  ( 10.72451020669871369, 18.67979575497193778, 92.08442372801901854 ) ) ;
#55402=CARTESIAN_POINT ( 'NONE',  ( -19.02544592524342804, 5.153800228976336051, 96.04057627198103830 ) ) ;
#55403=CARTESIAN_POINT ( 'NONE',  ( -5.719274019375978568, 21.55341960407610458, 85.20724293864770971 ) ) ;
#55404=CARTESIAN_POINT ( 'NONE',  ( -0.05219959533936034679, 19.03943276465977164, 62.50109039468566863 ) ) ;
#55406=CARTESIAN_POINT ( 'NONE',  ( 5.719274019375991003, -21.55341960407610458, 47.70724293864770260 ) ) ;
#55407=CARTESIAN_POINT ( 'NONE',  ( -13.89961937509977652, 13.97604488694528158, 100.6239096053143669 ) ) ;
#55408=CARTESIAN_POINT ( 'NONE',  ( -4.483927247898539470, -16.52544592524342804, 47.29057627198103120 ) ) ;
#55410=CARTESIAN_POINT ( 'NONE',  ( -16.51473224551082808, 9.474510206698731452, 83.33442372801899012 ) ) ;
#55412=CARTESIAN_POINT ( 'NONE',  ( 9.474510206698729675, 16.51473224551082808, 107.0844237280190043 ) ) ;
#55413=CARTESIAN_POINT ( 'NONE',  ( -15.72974639402197994, 15.80617190586746368, 80.62390960531438111 ) ) ;
#55414=CARTESIAN_POINT ( 'NONE',  ( 16.53943276465976808, -0.05219959533910856209, 68.74890960531435269 ) ) ;
#55415=CARTESIAN_POINT ( 'NONE',  ( -19.05341960407611168, -5.049401038298163336, 106.4572429386476955 ) ) ;
#55416=CARTESIAN_POINT ( 'NONE',  ( 0.05219959533934541429, -16.53943276465976808, 45.00109039468568284 ) ) ;
#55417=CARTESIAN_POINT ( 'NONE',  ( -16.46253265017160317, 9.564922557960807481, 55.83224293864769550 ) ) ;
#55418=CARTESIAN_POINT ( 'NONE',  ( -0.05219959533937732626, 21.53943276465977519, 22.50109039468567573 ) ) ;
#55419=CARTESIAN_POINT ( 'NONE',  ( 19.03943276465977164, 0.05219959533936151252, 81.25109039468567573 ) ) ;
#55420=CARTESIAN_POINT ( 'NONE',  ( 5.049401038298161559, -19.05341960407611168, 92.70724293864769550 ) ) ;
#55421=CARTESIAN_POINT ( 'NONE',  ( -9.474510206698964154, 16.51473224551069663, 80.41557627198103830 ) ) ;
#55422=CARTESIAN_POINT ( 'NONE',  ( 10.72451020669898902, -18.67979575497178502, 72.91557627198103830 ) ) ;
#55423=CARTESIAN_POINT ( 'NONE',  ( 13.97604488694527802, 13.89961937509977652, 49.37390960531434558 ) ) ;
#55425=CARTESIAN_POINT ( 'NONE',  ( 16.53943276465976808, -0.05219959533910856209, 53.74890960531437401 ) ) ;
#55426=CARTESIAN_POINT ( 'NONE',  ( -9.564922557960796823, -16.46253265017161027, 102.0822429386477097 ) ) ;
#55428=CARTESIAN_POINT ( 'NONE',  ( 16.46253265017146816, 9.564922557961045513, 66.66775706135233293 ) ) ;
#55429=CARTESIAN_POINT ( 'NONE',  ( 18.62759615963271287, -10.81492255796078972, 93.33224293864769550 ) ) ;
#55430=CARTESIAN_POINT ( 'NONE',  ( 0.05219959533936267826, -19.03943276465977164, 55.00109039468566863 ) ) ;
#55431=CARTESIAN_POINT ( 'NONE',  ( 9.564922557960805705, 16.46253265017160317, 104.5822429386476955 ) ) ;
#55432=CARTESIAN_POINT ( 'NONE',  ( -17.49999999999999645, -5.499999999999992895, 74.20309617465828467 ) ) ;
#55433=CARTESIAN_POINT ( 'NONE',  ( 15.72974639402199770, -15.80617190586745480, 43.12390960531435269 ) ) ;
#55434=CARTESIAN_POINT ( 'NONE',  ( 13.89961937509977652, -13.97604488694527269, 73.12390960531436690 ) ) ;
#55435=CARTESIAN_POINT ( 'NONE',  ( -21.55341960407619339, 5.719274019375674811, 63.54275706135234003 ) ) ;
#55436=CARTESIAN_POINT ( 'NONE',  ( 13.97604488694527802, 13.89961937509977652, 39.37390960531435269 ) ) ;
#55437=CARTESIAN_POINT ( 'NONE',  ( 8.314922557960818139, 14.29746914071049879, 69.58224293864769550 ) ) ;
#55438=ORIENTED_EDGE ( 'NONE', *, *, #81680, .T. ) ;
#55439=CARTESIAN_POINT ( 'NONE',  ( 8.314922557961029526, -14.29746914071037800, 20.41775706135234714 ) ) ;
#55440=CARTESIAN_POINT ( 'NONE',  ( 10.81492255796106328, -18.62759615963255655, 55.41775706135234714 ) ) ;
#55442=CARTESIAN_POINT ( 'NONE',  ( 5.049401038298161559, -19.05341960407611168, 112.7072429386476813 ) ) ;
#55443=CARTESIAN_POINT ( 'NONE',  ( -5.049401038297874678, -19.05341960407617918, 64.79275706135233293 ) ) ;
#55445=CARTESIAN_POINT ( 'NONE',  ( -10.72451020669870658, -18.67979575497194134, 19.58442372801901143 ) ) ;
#55446=CARTESIAN_POINT ( 'NONE',  ( -9.564922557960796823, -16.46253265017161027, 57.08224293864769550 ) ) ;
#55447=CARTESIAN_POINT ( 'NONE',  ( 16.55341960407618274, -4.379528057220086978, 41.04275706135236135 ) ) ;
#55449=CARTESIAN_POINT ( 'NONE',  ( 10.72451020669871369, 18.67979575497193778, 112.0844237280190185 ) ) ;
#55450=CARTESIAN_POINT ( 'NONE',  ( -13.89961937509977652, 13.97604488694528158, 45.62390960531433848 ) ) ;
#55451=CARTESIAN_POINT ( 'NONE',  ( -18.67979575497193778, 10.72451020669871902, 113.3344237280190328 ) ) ;
#55452=CARTESIAN_POINT ( 'NONE',  ( 14.34966873604972726, -8.224510206698740333, 90.83442372801901854 ) ) ;
#55453=CARTESIAN_POINT ( 'NONE',  ( 19.05341960407611168, 5.049401038298154454, 108.9572429386477097 ) ) ;
#55454=CARTESIAN_POINT ( 'NONE',  ( -10.72451020669870658, -18.67979575497194134, 74.58442372801901854 ) ) ;
#55458=CARTESIAN_POINT ( 'NONE',  ( 16.53943276465976808, 0.05219959533934440121, 51.25109039468568994 ) ) ;
#55459=CARTESIAN_POINT ( 'NONE',  ( 15.72974639402176855, 15.80617190586768217, 76.87609039468567573 ) ) ;
#55460=CARTESIAN_POINT ( 'NONE',  ( -0.05219959533937732626, 21.53943276465977519, 97.50109039468567573 ) ) ;
#55462=CARTESIAN_POINT ( 'NONE',  ( -8.224510206698735004, -14.34966873604973081, 34.58442372801900433 ) ) ;
#55463=CARTESIAN_POINT ( 'NONE',  ( -13.97604488694527625, -13.89961937509977652, 86.87390960531436690 ) ) ;
#55465=CARTESIAN_POINT ( 'NONE',  ( 9.474510206698971260, -16.51473224551069308, 107.9155762719810383 ) ) ;
#55467=CARTESIAN_POINT ( 'NONE',  ( 17.44279575226822132, 5.990770900252482711, 41.66442432485681735 ) ) ;
#55468=CARTESIAN_POINT ( 'NONE',  ( 16.46253265017160672, -9.564922557960803928, 33.33224293864770260 ) ) ;
#55469=CARTESIAN_POINT ( 'NONE',  ( -18.67979575497178146, -10.72451020669898902, 41.66557627198103120 ) ) ;
#55470=CARTESIAN_POINT ( 'NONE',  ( 0.05219959533934541429, -16.53943276465976808, 105.0010903946856757 ) ) ;
#55471=CARTESIAN_POINT ( 'NONE',  ( -12.06949235617756955, 12.14591786802309770, 80.62390960531438111 ) ) ;
#55472=CARTESIAN_POINT ( 'NONE',  ( 9.474510206698971260, -16.51473224551069308, 72.91557627198102409 ) ) ;
#55473=CARTESIAN_POINT ( 'NONE',  ( -10.72451020669870658, -18.67979575497194134, 99.58442372801900433 ) ) ;
#55474=CARTESIAN_POINT ( 'NONE',  ( -8.314922557961024197, 14.29746914071037800, 22.91775706135235069 ) ) ;
#55475=CARTESIAN_POINT ( 'NONE',  ( 12.06949235617757843, -12.14591786802309237, 83.12390960531436690 ) ) ;
#55476=CARTESIAN_POINT ( 'NONE',  ( 18.62759615963255655, 10.81492255796105972, 46.66775706135234714 ) ) ;
#55477=CARTESIAN_POINT ( 'NONE',  ( 21.53943276465977519, -0.05219959533907433946, 68.74890960531435269 ) ) ;
#55478=CARTESIAN_POINT ( 'NONE',  ( 9.474510206698729675, 16.51473224551082808, 52.08442372801900433 ) ) ;
#55480=CARTESIAN_POINT ( 'NONE',  ( -9.474510206698964154, 16.51473224551069663, 100.4155762719810241 ) ) ;
#55481=CARTESIAN_POINT ( 'NONE',  ( -12.14591786802309592, -12.06949235617757132, 66.87390960531436690 ) ) ;
#55482=CARTESIAN_POINT ( 'NONE',  ( 8.224510206698953496, -14.34966873604960469, 52.91557627198103830 ) ) ;
#55483=CARTESIAN_POINT ( 'NONE',  ( -0.05219959533934338120, 16.53943276465976808, 107.5010903946856899 ) ) ;
#55484=CARTESIAN_POINT ( 'NONE',  ( -5.153800228976607833, 19.02544592524334988, 67.70942372801900433 ) ) ;
#55486=CARTESIAN_POINT ( 'NONE',  ( -5.049401038298153566, 19.05341960407611168, 115.2072429386477097 ) ) ;
#55487=CARTESIAN_POINT ( 'NONE',  ( 4.379528057220339221, -16.55341960407611168, 92.70724293864770971 ) ) ;
#55489=CARTESIAN_POINT ( 'NONE',  ( -19.02544592524342804, 5.153800228976336051, 41.04057627198103120 ) ) ;
#55490=CARTESIAN_POINT ( 'NONE',  ( 21.52544592524344225, -5.823673210054117533, 53.54057627198103120 ) ) ;
#55491=CARTESIAN_POINT ( 'NONE',  ( -15.80617190586745835, -15.72974639402198527, 76.87390960531439532 ) ) ;
#55492=CARTESIAN_POINT ( 'NONE',  ( -16.46253265017160317, 9.564922557960807481, 35.83224293864768839 ) ) ;
#55493=CARTESIAN_POINT ( 'NONE',  ( 14.29746914071037800, 8.314922557961029526, 66.66775706135234714 ) ) ;
#55494=CARTESIAN_POINT ( 'NONE',  ( -9.564922557960796823, -16.46253265017161027, 67.08224293864769550 ) ) ;
#55495=CARTESIAN_POINT ( 'NONE',  ( 0.05219959533936267826, -19.03943276465977164, 35.00109039468566863 ) ) ;
#55496=CARTESIAN_POINT ( 'NONE',  ( 21.55341960407619695, -5.719274019375665929, 51.04275706135234714 ) ) ;
#55498=CARTESIAN_POINT ( 'NONE',  ( -0.05219959533907301413, -21.53943276465977519, 37.49890960531436690 ) ) ;
#55499=CARTESIAN_POINT ( 'NONE',  ( 4.379528057220339221, -16.55341960407611168, 107.7072429386476955 ) ) ;
#55500=CARTESIAN_POINT ( 'NONE',  ( 19.02544592524334988, 5.153800228976608722, 86.45942372801900433 ) ) ;
#55503=CARTESIAN_POINT ( 'NONE',  ( 15.72974639402199770, -15.80617190586745480, 53.12390960531436690 ) ) ;
#55504=CARTESIAN_POINT ( 'NONE',  ( 16.81555441253552274, -7.025013491695478507, 68.13685445334259327 ) ) ;
#55505=CARTESIAN_POINT ( 'NONE',  ( 21.55341960407619695, -5.719274019375665929, 86.04275706135236135 ) ) ;
#55506=CARTESIAN_POINT ( 'NONE',  ( 16.53943276465976808, -0.05219959533910856209, 28.74890960531435624 ) ) ;
#55507=CARTESIAN_POINT ( 'NONE',  ( -4.483927247898782831, 16.52544592524335698, 52.70942372801902565 ) ) ;
#55508=CARTESIAN_POINT ( 'NONE',  ( 12.14591786802309770, 12.06949235617756955, 54.37390960531435979 ) ) ;
#55509=CARTESIAN_POINT ( 'NONE',  ( 0.05219959533907565091, 21.53943276465977519, 84.99890960531436690 ) ) ;
#55510=CARTESIAN_POINT ( 'NONE',  ( -18.67979575497178146, -10.72451020669898902, 76.66557627198103830 ) ) ;
#55512=CARTESIAN_POINT ( 'NONE',  ( 9.564922557961047289, -16.46253265017146816, 90.41775706135234714 ) ) ;
#55513=CARTESIAN_POINT ( 'NONE',  ( -10.81492255796078084, -18.62759615963271287, 22.08224293864769194 ) ) ;
#55514=CARTESIAN_POINT ( 'NONE',  ( 16.46253265017160672, -9.564922557960803928, 63.33224293864769550 ) ) ;
#55515=CARTESIAN_POINT ( 'NONE',  ( 16.46253265017160672, -9.564922557960803928, 38.33224293864768839 ) ) ;
#55517=CARTESIAN_POINT ( 'NONE',  ( -12.14591786802326823, 12.06949235617739902, 88.12609039468570415 ) ) ;
#55518=CARTESIAN_POINT ( 'NONE',  ( -10.72451020669870658, -18.67979575497194134, 19.58442372801901143 ) ) ;
#55519=CARTESIAN_POINT ( 'NONE',  ( 9.564922557960805705, 16.46253265017160317, 69.58224293864770971 ) ) ;
#55520=CARTESIAN_POINT ( 'NONE',  ( 0.05219959533937995610, -21.53943276465977519, 55.00109039468568284 ) ) ;
#55521=CARTESIAN_POINT ( 'NONE',  ( -19.02544592524342804, 5.153800228976336051, 101.0405762719810241 ) ) ;
#55524=CARTESIAN_POINT ( 'NONE',  ( 5.719274019375673035, 21.55341960407619339, 42.29275706135235424 ) ) ;
#55525=CARTESIAN_POINT ( 'NONE',  ( -19.02544592524342804, 5.153800228976336051, 26.04057627198103120 ) ) ;
#55526=CARTESIAN_POINT ( 'NONE',  ( 19.03943276465977164, -0.05219959533909143690, 98.74890960531436690 ) ) ;
#55527=CARTESIAN_POINT ( 'NONE',  ( -19.03943276465977164, -0.05219959533935918106, 58.75109039468566863 ) ) ;
#55528=CARTESIAN_POINT ( 'NONE',  ( -18.62759615963270932, 10.81492255796079327, 110.8322429386476955 ) ) ;
#55529=CARTESIAN_POINT ( 'NONE',  ( -0.05219959533936034679, 19.03943276465977164, 47.50109039468566863 ) ) ;
#55530=CARTESIAN_POINT ( 'NONE',  ( 9.564922557961047289, -16.46253265017146816, 45.41775706135232582 ) ) ;
#55531=CARTESIAN_POINT ( 'NONE',  ( -16.52544592524335698, -4.483927247898792601, 103.9594237280190185 ) ) ;
#55532=ORIENTED_EDGE ( 'NONE', *, *, #34066, .F. ) ;
#55535=CARTESIAN_POINT ( 'NONE',  ( -9.564922557960796823, -16.46253265017161027, 72.08224293864770971 ) ) ;
#55536=CARTESIAN_POINT ( 'NONE',  ( 15.80617190586769283, -15.72974639402175789, 75.62609039468567573 ) ) ;
#55537=EDGE_CURVE ( 'NONE', #72076, #135352, #30228, .T. ) ;
#55538=CARTESIAN_POINT ( 'NONE',  ( -15.72974639402176322, -15.80617190586768395, 94.37609039468568994 ) ) ;
#55540=CARTESIAN_POINT ( 'NONE',  ( 19.05341960407611168, 5.049401038298154454, 83.95724293864766707 ) ) ;
#55541=CARTESIAN_POINT ( 'NONE',  ( 21.53943276465977519, 0.05219959533937863772, 76.25109039468568994 ) ) ;
#55542=CARTESIAN_POINT ( 'NONE',  ( 5.153800228976615827, -19.02544592524334988, 110.2094237280189901 ) ) ;
#55543=CARTESIAN_POINT ( 'NONE',  ( 0.05219959533909260263, 19.03943276465977164, 69.99890960531435269 ) ) ;
#55544=CARTESIAN_POINT ( 'NONE',  ( 13.97604488694527802, 13.89961937509977652, 114.3739096053143669 ) ) ;
#55545=CARTESIAN_POINT ( 'NONE',  ( 0.05219959533909260263, 19.03943276465977164, 89.99890960531436690 ) ) ;
#55546=CARTESIAN_POINT ( 'NONE',  ( -13.97604488694527625, -13.89961937509977652, 76.87390960531433848 ) ) ;
#55547=CARTESIAN_POINT ( 'NONE',  ( 5.153800228976335163, 19.02544592524342804, 59.79057627198100988 ) ) ;
#55548=CARTESIAN_POINT ( 'NONE',  ( 10.72451020669898902, -18.67979575497178502, 112.9155762719810383 ) ) ;
#55549=CARTESIAN_POINT ( 'NONE',  ( -0.05219959533934338120, 16.53943276465976808, 97.50109039468567573 ) ) ;
#55551=CARTESIAN_POINT ( 'NONE',  ( 5.153800228976615827, -19.02544592524334988, 60.20942372801899012 ) ) ;
#55552=CARTESIAN_POINT ( 'NONE',  ( 5.049401038298161559, -19.05341960407611168, 92.70724293864769550 ) ) ;
#55553=CARTESIAN_POINT ( 'NONE',  ( 12.14591786802309770, 12.06949235617756955, 89.37390960531435269 ) ) ;
#55554=CARTESIAN_POINT ( 'NONE',  ( 4.483927247898545687, 16.52544592524342804, 109.7905762719810383 ) ) ;
#55555=CARTESIAN_POINT ( 'NONE',  ( -18.67979575497178146, -10.72451020669898902, 36.66557627198103120 ) ) ;
#55556=CARTESIAN_POINT ( 'NONE',  ( 10.72451020669898902, -18.67979575497178502, 22.91557627198102765 ) ) ;
#55557=CARTESIAN_POINT ( 'NONE',  ( -16.53943276465976808, 0.05219959533911058130, 91.24890960531436690 ) ) ;
#55559=CARTESIAN_POINT ( 'NONE',  ( 16.51473224551083163, -9.474510206698727899, 45.83442372801900433 ) ) ;
#55560=CARTESIAN_POINT ( 'NONE',  ( 16.53943276465976808, 0.05219959533934440121, 101.2510903946856757 ) ) ;
#55561=CARTESIAN_POINT ( 'NONE',  ( 19.03943276465977164, -0.05219959533909143690, 93.74890960531435269 ) ) ;
#55562=CARTESIAN_POINT ( 'NONE',  ( -5.823673210054431948, 21.52544592524334988, 67.70942372801901854 ) ) ;
#55563=CARTESIAN_POINT ( 'NONE',  ( -5.823673210054116645, -21.52544592524344225, 42.29057627198103120 ) ) ;
#55564=CARTESIAN_POINT ( 'NONE',  ( -5.823673210054431948, 21.52544592524334988, 27.70942372801901854 ) ) ;
#55565=CARTESIAN_POINT ( 'NONE',  ( -15.72974639402197994, 15.80617190586746368, 85.62390960531436690 ) ) ;
#55566=CARTESIAN_POINT ( 'NONE',  ( -0.05219959533910754901, -16.53943276465976808, 107.4989096053143669 ) ) ;
#55567=CARTESIAN_POINT ( 'NONE',  ( 13.89961937509957401, 13.97604488694547697, 76.87609039468566152 ) ) ;
#55569=CARTESIAN_POINT ( 'NONE',  ( -13.89961937509977652, 13.97604488694528158, 40.62390960531435979 ) ) ;
#55570=CARTESIAN_POINT ( 'NONE',  ( 13.89961937509977652, -13.97604488694527269, 103.1239096053143527 ) ) ;
#55571=CARTESIAN_POINT ( 'NONE',  ( 5.153800228976335163, 19.02544592524342804, 99.79057627198102409 ) ) ;
#55572=CARTESIAN_POINT ( 'NONE',  ( -16.55341960407611168, -4.379528057220339221, 111.4572429386476813 ) ) ;
#55573=CARTESIAN_POINT ( 'NONE',  ( -14.29746914071049879, 8.314922557960819915, 40.83224293864769550 ) ) ;
#55574=CARTESIAN_POINT ( 'NONE',  ( 4.379528057220092307, 16.55341960407617563, 47.29275706135234003 ) ) ;
#55575=CARTESIAN_POINT ( 'NONE',  ( -5.823673210054431948, 21.52544592524334988, 102.7094237280190185 ) ) ;
#55577=CARTESIAN_POINT ( 'NONE',  ( -12.06949235617756955, 12.14591786802309770, 25.62390960531435624 ) ) ;
#55578=CARTESIAN_POINT ( 'NONE',  ( 5.823673210054444382, -21.52544592524334988, 35.20942372801901854 ) ) ;
#55579=CARTESIAN_POINT ( 'NONE',  ( -16.51473224551069308, -9.474510206698971260, 101.6655762719810241 ) ) ;
#55580=CARTESIAN_POINT ( 'NONE',  ( 8.224510206698742110, 14.34966873604972548, 107.0844237280190043 ) ) ;
#55581=CARTESIAN_POINT ( 'NONE',  ( 16.55341960407618274, -4.379528057220086978, 91.04275706135236135 ) ) ;
#55582=CARTESIAN_POINT ( 'NONE',  ( -0.05219959533934338120, 16.53943276465976808, 27.50109039468567929 ) ) ;
#55583=CARTESIAN_POINT ( 'NONE',  ( -19.05341960407611168, -5.049401038298163336, 46.45724293864768129 ) ) ;
#55584=CARTESIAN_POINT ( 'NONE',  ( -8.314922557960811034, -14.29746914071050412, 112.0822429386477097 ) ) ;
#55585=CARTESIAN_POINT ( 'NONE',  ( 15.72974639402176855, 15.80617190586768217, 21.87609039468567573 ) ) ;
#55586=CARTESIAN_POINT ( 'NONE',  ( 19.02544592524343514, -5.153800228976328945, 28.54057627198102409 ) ) ;
#55587=CARTESIAN_POINT ( 'NONE',  ( 9.474510206698971260, -16.51473224551069308, 102.9155762719810241 ) ) ;
#55588=CARTESIAN_POINT ( 'NONE',  ( 18.62759615963255655, 10.81492255796105972, 31.66775706135234358 ) ) ;
#55589=CARTESIAN_POINT ( 'NONE',  ( -19.02544592524342804, 5.153800228976336051, 36.04057627198100988 ) ) ;
#55590=CARTESIAN_POINT ( 'NONE',  ( 16.51473224551069308, 9.474510206698969483, 104.1655762719810241 ) ) ;
#55591=CARTESIAN_POINT ( 'NONE',  ( -17.05116617787824040, -6.768360034955907878, 36.34324446740804859 ) ) ;
#55592=CARTESIAN_POINT ( 'NONE',  ( 5.153800228976335163, 19.02544592524342804, 99.79057627198102409 ) ) ;
#55593=CARTESIAN_POINT ( 'NONE',  ( 5.823673210054444382, -21.52544592524334988, 50.20942372801901854 ) ) ;
#55594=CARTESIAN_POINT ( 'NONE',  ( -14.34966873604960291, -8.224510206698953496, 86.66557627198102409 ) ) ;
#55595=CARTESIAN_POINT ( 'NONE',  ( -16.46253265017160317, 9.564922557960807481, 100.8322429386477097 ) ) ;
#55597=CARTESIAN_POINT ( 'NONE',  ( 16.52544592524335698, 4.483927247898782831, 66.45942372801903275 ) ) ;
#55598=( BOUNDED_SURFACE ( )  B_SPLINE_SURFACE ( 3, 2, ( 
 ( #117250, #133415, #83896, #178942, #162752, #163768, #24261, #118261, #195104, #99067, #38415, #103084, #116248, #177940, #25269, #39407, #148594, #10086, #161757, #23252, #82900, #175938, #179951, #191097, #84895, #41418, #164765, #130396, #144579, #146574, #6065, #67743, #53576, #52572, #115253, #114232, #69745, #131414, #37409, #193102, #152558, #120234, #104081, #29241, #167743, #123206, #14047, #30219, #28264, #89902, #149587, #90874, #11085, #151585, #134432, #199071, #165763, #166762, #91861, #75713, #74741, #44403, #153554, #13074, #183907, #60540, #198082, #42418, #196118, #72762, #61537, #76712, #200069, #136404, #138387, #119258, #59549, #15051, #108037, #121227, #137391, #122216, #184896, #182918, #106057, #57588, #45392, #180942, #107045, #27257, #168717, #88907, #46378, #26260, #87901, #150598, #12096, #73759, #135431, #197102, #58569, #181925, #43406, #105076, #154554, #4827, #20014, #143340, #156548, #81657, #62530, #2858, #35187, #51351, #141371, #80684, #48383, #186912, #142360, #128177, #77708, #111029, #172715, #17042, #33208, #32213, #155548, #188889, #66515, #78696, #158526, #157543, #110040, #18047, #3840, #64536, #34198, #93869, #65519, #16049, #112030, #126202, #140373, #124203, #79700, #1860, #187898, #856, #95860, #185903, #49365, #31216, #139374, #169723, #92867, #63542, #171719, #125216, #50370, #127179, #47388, #94867, #173719, #96841, #19037, #189876, #109043, #170721, #163529, #147359, #54346, #82660, #116017, #101843, #175693, #144344, #194869, #25029, #129165, #177707, #52339, #160521, #192867, #84660, #86673, #37168, #36168, #99838, #98827, #22012, #161522, #148356, #97820, #9852, #191854, #6824, #5832, #117010, #70515, #115014, #146338, #190862, #23014, #159509, #53335, #7826, #85672, #40167, #71511, #133179, #100832, #176708, #69511, #24017, #131177, #39174, #83664, #8847, #21005, #55340, #162515, #145342, #67508, #132183, #68502, #193874, #113995, #178705, #130157, #113011, #174704, #38182, #56342, #118024, #165534, #58343, #27030, #137163, #90656, #41186, #88675, #167521, #183683, #180716, #74515, #45168, #44175, #106824, #152338, #197856, #26027, #59323, #168498, #119033, #87672, #138163, #29996, #72522, #120992, #195885, #103853, #136181, #28032, #91635, #42192, #179714, #43177, #150371, #11867, #104844, #153323, #102849, #14825, #135204, #73532, #149356, #60316, #13824, #120011, #89673, #134197, #166535, #164534, #196876, #151360, #29016, #76486, #10853, #182690, #57359, #105834, #181696, #12849, #75490, #198852, #121992, #122981, #199844, #50136, #188656, #156311, #94632, #63302, #17813, #48149, #61311, #80452, #47152, #46150, #142125, #169488, #18807, #157310, #65289, #109806, #30988, #172480, #79469, #49141, #107804, #64305, #92636, #170489, #124982, #19786, #33968, #158297, #154327, #141138, #2628, #108810, #186679, #62295, #185660, #3610, #173483, #31980, #81427, #184668, #171489, #111795, #15816, #187671, #34956, #125972, #77477, #110799, #95625, #96608, #139147, #32978, #140134, #126948, #624, #123962, #93636, #155321, #16810, #78460, #1626, #163298, #175463, #99607, #177478, #20772, #69276, #38947, #127944, #54115, #131955, #82428, #115789, #22781, #23786, #161287, #116781, #193639, #159276, #36934, #24797, #176473, #37947, #130943, #84429, #146106, #100604, #21781, #98597, #143113, #35942, #7590, #189646, #160290, #192633, #162286, #5596, #85436, #83432, #8614, #147127, #144116, #178472, #145109, #70287, #67276, #128934, #55111, #39939, #101608, #6592, #190635, #4592, #66285, #51121, #112780, #174473, #68271, #129922, #97588, #52110, #113767, #191622, #53101, #114780, #25801, #26794, #152104, #151126, #134969, #104612, #90419, #11632, #43935, #59088, #58116, #102622, #56110, #71287, #121749, #136926, #60081, #73299, #198613, #179486, #119786, #13588, #168259, #181470, #197623, #165301, #103625, #183441, #75255, #44926, #42948, #106582, #150130 ),
 ( #88436, #196646, #9622, #12619, #132952, #166300, #194640, #120755, #87447, #27797, #86445, #74283, #89438, #135953, #148131, #182454, #105596, #167282, #28780, #164308, #117791, #40950, #149132, #10623, #72284, #133961, #195653, #57125, #118799, #180487, #41959, #4099, #143608, #111292, #49629, #144611, #159781, #98083, #189153, #129432, #96118, #66775, #50626, #51608, #128436, #188156, #78958, #48645, #191130, #114266, #14581, #157806, #82933, #140633, #20269, #67775, #173977, #110297, #35445, #5092, #6096, #52604, #65778, #172981, #97097, #2123, #33467, #79963, #29755, #190133, #19297, #80945, #91390, #64797, #112287, #113272, #171979, #158781, #174964, #63805, #36428, #21276, #95125, #153079, #81915, #125478, #187174, #156815, #18307, #141632, #126458, #3122, #127447, #34459, #142620, #9117, #70784, #10118, #54605, #69777, #175970, #68771, #178975, #22279, #131445, #25302, #163800, #38448, #40442, #193132, #41452, #132452, #53609, #11119, #8099, #56619, #115285, #176978, #179984, #194143, #102115, #116279, #100103, #177969, #85940, #148628, #103117, #26293, #55607, #87934, #86944, #130429, #39437, #117281, #37439, #133448, #99099, #160791, #149621, #164798, #71778, #195138, #101097, #118293, #24291, #83930, #72794, #23282, #145611, #134464, #7090, #196149, #57621, #192128, #147629, #161787, #84926, #146606, #162783, #27292, #183935, #88939, #89934, #182950, #139402, #91891, #77736, #150630, #60569, #122245, #166793, #44433, #181956, #105107, #138416, #92896, #28294, #108067, #107073, #59582, #167773, #30248, #90902, #45420, #43438, #153582, #104113, #61564, #75745, #151615, #12126, #29271, #13107, #152588, #73790, #168744, #135462, #106087, #180972, #197131, #119289, #42449, #74772, #121256, #136434, #200096, #15080, #165795, #198115, #76741, #46408, #14079, #137422, #169751, #123233, #31246, #184924, #154582, #58598, #16078, #884, #199102, #120264, #144375, #51381, #78725, #65548, #1889, #110069, #142390, #34227, #36197, #125244, #185931, #49395, #186942, #171749, #111058, #113042, #47416, #97851, #141399, #156580, #32240, #66545, #20043, #64566, #95889, #140401, #172746, #109072, #173747, #157572, #127207, #48413, #35216, #170751, #4860, #19065, #33238, #155576, #80712, #94896, #3869, #93898, #188921, #17071, #50399, #124235, #63570, #62559, #18075, #79730, #126231, #2887, #143368, #96869, #187926, #112059, #158553, #189906, #81686, #128209, #174734, #159540, #21038, #82691, #147390, #175724, #8878, #194898, #68534, #37203, #87699, #56372, #22044, #70546, #145373, #53369, #85704, #177737, #179745, #130189, #129196, #192899, #191885, #115047, #54376, #118055, #190894, #41215, #84690, #99868, #98859, #9881, #163559, #7857, #39206, #83695, #116048, #52370, #146370, #100862, #178734, #133207, #102876, #132214, #164561, #193905, #160554, #69544, #55369, #67538, #25059, #114027, #5862, #26055, #6855, #162544, #24048, #131208, #117039, #40197, #176739, #86702, #38212, #161552, #148387, #23045, #71541, #101877, #14852, #197882, #119061, #122019, #167548, #198878, #57388, #13850, #180743, #120037, #12877, #169515, #183710, #107831, #42219, #90683, #152365, #196903, #74542, #11895, #135231, #168525, #123008, #58370, #138190, #137191, #89701, #59351, #72550, #75517, #134228, #136207, #103880, #45196, #88703, #151387, #76514, #60345, #121019, #29043, #153350, #182717, #106850, #30023, #44202, #165560, #27057, #195913, #184694, #199873, #46178, #105861, #61337, #150399, #91661, #31015, #149384, #10880, #73558, #28060, #166561, #181723, #43205, #104872, #49169, #189676, #156341, #126976, #110828, #111823, #188685, #48179, #139176, #108839, #51148, #174502, #77505, #17841, #143141, #652, #80481, #127973, #33997, #170520, #95653, #3639, #66312, #112809, #126002, #33007, #157341, #62322, #93666, #140164, #92665, #50165, #79499, #141168, #154353, #125012, #172512, #173511, #32009, #18836, #34984, #123992 ),
 ( #185690, #15846, #81455, #155351, #142155, #16841, #1656, #65317, #64334, #47180, #78491, #63334, #2657, #186708, #109835, #187699, #4621, #171518, #94662, #96637, #158325, #19814, #39970, #193671, #37980, #7623, #52140, #22813, #20801, #114811, #146137, #8645, #163331, #86477, #115820, #148162, #23818, #69307, #113797, #5628, #82456, #71319, #9653, #132982, #84459, #194673, #128964, #130973, #101640, #117823, #192664, #147157, #176503, #53132, #56142, #24827, #35969, #54147, #97616, #99637, #70319, #177510, #55142, #131986, #191653, #144144, #175492, #159306, #67305, #190664, #161320, #36965, #98626, #85468, #160320, #38980, #21811, #100636, #116813, #83463, #145140, #162317, #178504, #6623, #68302, #129953, #26826, #199634, #75289, #104645, #42980, #61101, #11664, #135984, #13622, #57155, #105630, #136960, #164338, #90455, #168293, #118834, #152139, #59121, #60115, #197655, #153112, #29789, #195684, #73330, #179516, #12650, #74317, #167319, #120787, #182487, #198649, #58149, #135002, #40984, #72317, #43968, #25833, #196680, #28815, #121783, #41990, #183477, #119817, #44961, #106619, #180517, #14616, #181502, #91425, #103656, #165334, #76273, #137951, #102653, #166332, #88467, #87477, #149164, #10654, #133993, #150164, #27830, #89471, #151162, #187461, #107598, #186466, #30782, #95413, #62089, #63089, #188439, #48929, #171278, #140927, #126736, #47944, #80242, #157098, #49918, #111583, #79255, #19580, #109595, #18594, #2413, #141912, #3403, #78248, #169276, #138935, #81223, #4385, #92429, #32766, #173268, #154115, #110583, #158088, #64093, #415, #125761, #33754, #96401, #142904, #156098, #124768, #172264, #15609, #123752, #170278, #122774, #65078, #94418, #17596, #184464, #155107, #34742, #45943, #185451, #77266, #46941, #108601, #31772, #93420, #16600, #139921, #1410, #146912, #84219, #39727, #116575, #82213, #160078, #86233, #163081, #23573, #36719, #143904, #69066, #5386, #113559, #145898, #37732, #101388, #128728, #189438, #52889, #190424, #175253, #114564, #54901, #50915, #24585, #144900, #21565, #35735, #70076, #85221, #68062, #99394, #67069, #176261, #112573, #6383, #161077, #38741, #193426, #178264, #7382, #147923, #53907, #159068, #129716, #130733, #127736, #8401, #174267, #66070, #97382, #20562, #22572, #192425, #191413, #115582, #177270, #51900, #131744, #98381, #83225, #100399, #162079, #28576, #167074, #75049, #57908, #179273, #182241, #27587, #58882, #117573, #74074, #40737, #180275, #73085, #29551, #43726, #135745, #136715, #90212, #42740, #104402, #105387, #88224, #103409, #9409, #102407, #12412, #55900, #165087, #120548, #197416, #72067, #151895, #26581, #198396, #166084, #87237, #44716, #41745, #13385, #148920, #10409, #59874, #89225, #121540, #149908, #133740, #183235, #150919, #106372, #168054, #91184, #11415, #134756, #132741, #71075, #194429, #196438, #164094, #25593, #195435, #119580, #56910, #118585, #181263, #1167, #63855, #31529, #17354, #94177, #16364, #107355, #60857, #76034, #172028, #48694, #33516, #93182, #110346, #122532, #78012, #125526, #18358, #139680, #32525, #185208, #123515, #95176, #187223, #156863, #62842, #152873, #154867, #79009, #124526, #140683, #2175, #46699, #199393, #169028, #14368, #137709, #30533, #186221, #184223, #92186, #45704, #153870, #15368, #47702, #77024, #138696, #178, #61846, #108361, #170039, #109352, #155856, #171034, #196014, #166660, #57490, #178839, #24157, #71645, #164663, #133312, #43305, #197002, #147494, #195001, #73657, #89803, #86808, #180842, #151485, #150497, #12976, #58468, #103980, #132319, #165659, #74640, #104973, #42319, #136306, #197981, #40307, #56479, #121124, #88804, #59451, #120135, #119159, #27157, #181826, #41318, #118157, #162651, #55474, #11994, #8985, #179847, #135329, #28161, #25166, #182819, #102978, #44301, #85808, #101983, #70653, #26159, #194011, #163664, #148494, #117144, #9985, #87800, #149486 ),
 ( #10982, #72655, #134330, #171617, #170622, #154456, #124098, #109935, #31118, #63436, #78593, #77607, #122117, #75614, #90778, #141265, #156443, #79596, #92766, #17942, #198975, #139278, #33105, #187797, #755, #16939, #184793, #123108, #2755, #94761, #64431, #62426, #126101, #169621, #140266, #185797, #125112, #1758, #61436, #152462, #183806, #105960, #167645, #13948, #15948, #29141, #137293, #93768, #60442, #47285, #45294, #108941, #186810, #106946, #168619, #32111, #46279, #155449, #30119, #91760, #153454, #48280, #14952, #76612, #138290, #199971, #107935, #5726, #83560, #127076, #175591, #145239, #34097, #160420, #38077, #188784, #21909, #129060, #84555, #36068, #111925, #7720, #112908, #69406, #81553, #67405, #6720, #50267, #37067, #68398, #95755, #130050, #99733, #173611, #191750, #190761, #53233, #52236, #22909, #161417, #65415, #143239, #131072, #98726, #176603, #114909, #82560, #144242, #146233, #128073, #4722, #49266, #142254, #113893, #157440, #66411, #110924, #172610, #35081, #18935, #189776, #80580, #3738, #96734, #158423, #51248, #19911, #174602, #97717, #159407, #20902, #118929, #86572, #70415, #195782, #134092, #89569, #180614, #196774, #194767, #56241, #115916, #57255, #177606, #117922, #100731, #165431, #132082, #133077, #58242, #42087, #41084, #10751, #119910, #179611, #150266, #26926, #164435, #8745, #162412, #39074, #27926, #43073, #166431, #102747, #104740, #85568, #25929, #181596, #74410, #87572, #103752, #71413, #9749, #151255, #12745, #192761, #149259, #54244, #72415, #88568, #11760, #73427, #135098, #148256, #23914, #193771, #147254, #55240, #116908, #178601, #40064, #101741, #163429, #24927, #77369, #152233, #139037, #47045, #109698, #171380, #169375, #76376, #517, #120886, #137056, #185551, #44068, #62189, #105728, #106717, #199734, #156199, #108702, #94517, #167415, #123853, #170381, #183574, #61200, #198746, #121881, #155211, #32867, #45059, #124870, #31872, #138053, #184560, #93526, #107696, #16700, #60211, #78350, #182585, #140024, #92530, #168391, #28911, #46041, #29886, #30883, #90551, #1513, #13718, #154219, #63190, #15709, #75384, #197750, #91524, #122872, #153211, #186569, #48042, #14716, #17699, #136076, #59217, #3501, #97479, #6480, #67168, #129812, #113657, #20660, #49028, #82314, #68160, #191511, #176362, #36819, #50020, #95513, #144004, #18693, #126836, #159165, #51010, #52988, #142012, #2514, #66170, #65177, #188542, #127832, #114666, #64194, #37835, #158187, #173372, #110683, #83322, #98485, #81319, #112671, #157199, #189538, #125861, #19677, #174363, #51998, #99495, #161175, #5485, #79356, #128825, #172363, #143002, #190524, #141027, #160178, #187561, #33853, #80340, #111685, #35833, #175351, #4480, #21668, #144999, #34842, #96497, #70176, #69165, #165188, #192523, #41845, #180375, #88323, #71175, #54006, #195536, #40835, #164192, #11519, #150013, #119678, #103512, #193527, #38839, #25690, #162176, #131844, #102508, #194526, #196538, #85322, #145998, #9509, #147014, #55001, #132839, #73189, #7481, #58008, #101491, #116670, #115680, #26683, #134860, #24684, #55998, #100497, #117676, #130832, #163180, #179373, #57010, #181361, #42840, #87335, #104505, #10509, #177368, #86333, #149021, #84319, #22672, #23674, #8499, #178361, #39825, #72171, #133846, #148020, #118683, #14469, #166186, #46800, #13481, #12511, #108459, #135845, #185309, #123614, #31631, #76131, #197514, #138797, #184323, #15471, #74175, #30637, #58982, #136817, #29647, #186319, #278, #124624, #120649, #107456, #169132, #75146, #91279, #28674, #151995, #170136, #139779, #198501, #154965, #153974, #106471, #137809, #77128, #199493, #92290, #90309, #61947, #151020, #93280, #122633, #59972, #182347, #60959, #121639, #45805, #43825, #16461, #105489, #78110, #1267, #62944, #167175, #27687, #183334, #168150, #44816, #47801, #89328, #152970, #18455, #20419, #36578, #33612, #127600, #98233 ),
 ( #2270, #142767, #175110, #191273, #81089, #82069, #188301, #126599, #21423, #159936, #83083, #65927, #6244, #173130, #143762, #189299, #128587, #5243, #64940, #155955, #125622, #67923, #109451, #94277, #34605, #144759, #17452, #97242, #129576, #50776, #187320, #112436, #66923, #171134, #32623, #4247, #49778, #174125, #79108, #110445, #140781, #96264, #172126, #63953, #157950, #48791, #141774, #35596, #190281, #95275, #158930, #51757, #156958, #113418, #80106, #3268, #111443, #19441, #133599, #70936, #26444, #103271, #68926, #146763, #11274, #179131, #180137, #10270, #86093, #147784, #87096, #131600, #8256, #52748, #145759, #55759, #99251, #69936, #102270, #40599, #115438, #117433, #193285, #118445, #9270, #130588, #88086, #85079, #195291, #192283, #53764, #56772, #132604, #163958, #54759, #177129, #25456, #194293, #149772, #148781, #41606, #116433, #178121, #176118, #71929, #37589, #39589, #160938, #164951, #38600, #101248, #72947, #134617, #162937, #114417, #22430, #24444, #84080, #7241, #100256, #161937, #23432, #155480, #95787, #62460, #33137, #16972, #17975, #94795, #154487, #42600, #12275, #157473, #80612, #181126, #124133, #49297, #104264, #186844, #34128, #140301, #73940, #1792, #109968, #172640, #18966, #32143, #139309, #63470, #165946, #197280, #196301, #185832, #58743, #57771, #47319, #119441, #31151, #78626, #156474, #135609, #125145, #79629, #27446, #171647, #187828, #120412, #141297, #48313, #2787, #64466, #89088, #110956, #184827, #92799, #150780, #126133, #46313, #107968, #93800, #169655, #15981, #77640, #788, #108974, #170655, #145271, #188815, #36098, #191783, #130084, #4753, #6752, #159438, #7753, #98757, #19943, #177638, #174633, #22941, #81584, #143270, #146267, #160450, #68431, #97750, #66442, #53265, #83591, #39105, #114942, #69437, #144272, #5759, #65446, #176635, #127108, #67435, #50298, #38110, #128103, #82591, #131105, #99765, #190792, #21941, #192793, #129092, #161450, #84587, #113924, #158454, #111955, #173644, #100761, #54275, #115948, #52266, #162443, #35113, #175624, #23944, #142289, #37098, #3769, #20933, #96765, #189807, #51279, #112940, #147285, #194797, #87601, #56270, #166461, #119940, #70444, #117953, #196803, #12776, #9781, #103781, #74441, #73456, #136108, #181625, #26957, #55269, #88600, #197784, #59250, #182618, #43105, #179644, #101772, #150296, #24957, #133108, #165461, #57284, #120919, #148287, #8775, #72448, #71443, #41113, #134123, #44103, #132110, #105761, #164464, #102777, #116938, #89599, #104773, #149287, #118958, #163459, #195812, #193803, #25958, #180644, #58271, #167447, #85598, #11792, #178631, #135129, #40094, #10781, #27958, #86604, #151287, #42119, #28944, #79394, #17737, #185588, #123890, #92565, #47078, #77403, #90585, #109732, #13751, #45093, #198779, #75419, #64232, #141064, #2550, #15744, #125897, #121916, #62222, #94555, #110721, #551, #140060, #107730, #46076, #187597, #156235, #49066, #108739, #152266, #154253, #63226, #170415, #48076, #124906, #184595, #137093, #106750, #60245, #183609, #168425, #139073, #29920, #91560, #16736, #153248, #31907, #14750, #93560, #1551, #76411, #138087, #155246, #169412, #78384, #199768, #61235, #122907, #186604, #30917, #171416, #32902, #174399, #81354, #53024, #6517, #157236, #143038, #83359, #99531, #96532, #190560, #161213, #160215, #22708, #68196, #113691, #142049, #175386, #84355, #146033, #69201, #129848, #4516, #188579, #36855, #111721, #19712, #52034, #144040, #7516, #34878, #95549, #159201, #158222, #66209, #20696, #130869, #18729, #192559, #51045, #127869, #3536, #176398, #191547, #35869, #5522, #50060, #82352, #80377, #112707, #67202, #145035, #54042, #172403, #98522, #33892, #21705, #65213, #97515, #114705, #126872, #37873, #173407, #189573, #128860, #104536, #72207, #10543, #179406, #133881, #164227, #177404, #162211, #116706, #135875, #58039, #85357, #134892, #73221, #181393 ),
 ( #23710, #57045, #118719, #163217, #40870, #178396, #101526, #196568, #89361, #24719, #166217, #103547, #56032, #25724, #26717, #87370, #180408, #39860, #88356, #100532, #119709, #195572, #86368, #8533, #149055, #148053, #41880, #147050, #165222, #70212, #150049, #42871, #11555, #131879, #117710, #27718, #151050, #12541, #74206, #197546, #115716, #9544, #38875, #193564, #55036, #71210, #132873, #194562, #102544, #32656, #45837, #109486, #152027, #92323, #124658, #140813, #30670, #170172, #137844, #76164, #171169, #186354, #47834, #15504, #155988, #122667, #93315, #77161, #78144, #154999, #14502, #105523, #75178, #17485, #59014, #43858, #184355, #94310, #167209, #46833, #79142, #311, #136850, #61979, #31665, #120681, #182380, #154008, #199525, #123645, #28706, #60006, #90342, #107488, #121673, #13513, #169166, #198535, #91311, #138831, #16495, #183368, #185342, #139812, #44850, #1300, #106506, #168183, #62978, #108493, #29679, #153003, #60993, #52779, #18486, #96293, #160968, #128619, #129607, #159967, #35627, #97272, #36608, #81117, #157980, #2303, #95304, #5276, #48821, #19472, #51788, #190312, #64970, #66958, #142797, #67953, #158960, #80135, #37619, #34634, #83115, #141805, #3298, #6275, #20450, #113448, #4278, #126629, #175141, #143793, #99281, #98265, #191303, #65958, #127629, #125654, #21454, #187351, #189329, #110474, #144792, #188330, #22462, #50806, #112464, #172156, #114448, #176149, #174156, #82101, #49809, #84110, #33642, #63984, #156988, #111474, #173159, #196333, #25485, #57801, #133632, #38631, #9301, #87127, #7271, #103302, #68955, #145789, #119472, #134647, #102299, #40629, #70967, #163988, #194323, #130618, #192314, #146795, #165975, #88118, #115469, #164981, #26476, #11308, #55791, #177158, #118477, #148812, #195324, #53794, #10302, #100288, #116465, #132635, #27477, #180168, #104294, #161966, #71959, #56804, #193316, #117462, #8288, #131632, #149802, #181155, #54790, #42630, #41637, #86124, #179161, #72978, #23462, #85109, #69966, #178154, #39619, #101278, #162968, #24474, #147815, #199286, #59767, #122426, #120441, #153766, #182134, #184118, #93077, #45600, #105282, #150808, #198289, #91080, #121435, #169933, #123410, #73970, #183128, #71, #16259, #13282, #107253, #77910, #76919, #139577, #185103, #30430, #58773, #92077, #1062, #62736, #186112, #46592, #44611, #166970, #15261, #28472, #136609, #168924, #60753, #124417, #151791, #12304, #75928, #74946, #106266, #137603, #47593, #135639, #89120, #109246, #170926, #138590, #61742, #152767, #108253, #31424, #197309, #43618, #90107, #167950, #154761, #29448, #14257, #190081, #98029, #80891, #2069, #5039, #50575, #81865, #140579, #97045, #63748, #3065, #96064, #52547, #66725, #191074, #125422, #173925, #35394, #79906, #157752, #95071, #18253, #51557, #6042, #141577, #21222, #20217, #172927, #142568, #143555, #4047, #158727, #156759, #128385, #17249, #174911, #189102, #64742, #187118, #65724, #126404, #127392, #48590, #113221, #110241, #112235, #36375, #159725, #171922, #94072, #188100, #34406, #49573, #82878, #144556, #78901, #111236, #67720, #129377, #19244, #114208, #32417, #155751, #33412, #10064, #117228, #145554, #178922, #164745, #103063, #72740, #133393, #146549, #192068, #40391, #115228, #23228, #55555, #147577, #149567, #38391, #99041, #162732, #100047, #84871, #24240, #26240, #160731, #11063, #54555, #69724, #7032, #179931, #195084, #177919, #9063, #53550, #85889, #22223, #116228, #70733, #148574, #87879, #134412, #102063, #196098, #163748, #68714, #39387, #25248, #37384, #56565, #83872, #57568, #176920, #131392, #175913, #86889, #130371, #118240, #132400, #194093, #71724, #101046, #193080, #161733, #8044, #41398, #165740, #13054, #168696, #107024, #181904, #183886, #136384, #184874, #75691, #197081, #154530, #151565, #200047, #58548, #120214, #123185, #137371, #45371, #74721, #43382, #122194, #60519, #16027, #30197 ),
 ( #14025, #182896, #199049, #167722, #180922, #27235, #105055, #139353, #61516, #88884, #138366, #76690, #46356, #29220, #150576, #91839, #153533, #15029, #12075, #108014, #73737, #89882, #44380, #833, #169700, #77685, #135410, #31193, #92845, #166738, #106036, #28242, #198061, #119238, #42397, #59527, #104060, #121205, #90853, #152538, #173694, #34174, #127155, #125193, #35162, #47365, #4802, #19013, #186889, #155524, #172689, #33183, #95835, #93845, #188863, #17019, #157519, #66491, #80659, #78672, #124178, #171694, #64511, #94842, #143315, #96817, #109020, #156522, #158502, #189854, #48359, #142335, #51328, #50346, #112988, #19989, #3815, #65493, #112005, #170699, #81632, #32188, #18022, #126178, #82637, #128154, #20980, #140348, #174681, #36146, #110013, #187873, #79675, #141346, #97798, #159487, #2833, #144320, #62507, #49341, #111003, #185880, #1836, #63518, #71244, #181425, #190839, #151082, #165256, #132908, #101562, #118754, #179440, #41915, #39894, #73254, #163253, #103581, #12573, #26750, #24755, #67484, #117746, #10579, #40906, #89394, #42903, #52315, #102579, #119742, #135908, #194595, #88389, #197579, #196601, #59046, #104568, #150083, #175671, #11587, #120712, #182412, #105555, #166251, #164263, #86402, #134924, #148087, #56066, #58072, #180443, #43892, #25758, #129142, #195607, #87404, #149089, #57080, #167241, #113973, #28739, #72240, #133917, #9578, #74239, #27751, #90376, #5809, #168216, #138862, #136883, #30704, #62010, #124691, #79175, #2335, #31697, #64016, #139843, #44883, #15535, #93346, #13546, #109518, #75212, #152061, #125685, #140846, #108525, #46864, #77193, #170204, #342, #198569, #60039, #153036, #172188, #94341, #121707, #171200, #32690, #17517, #123675, #183400, #186388, #184387, #155032, #47865, #29713, #78174, #156020, #106539, #63012, #187383, #91345, #48852, #16527, #110507, #1332, #33673, #14536, #76197, #45868, #137876, #199557, #61026, #122698, #185373, #107521, #169197, #92354, #154040, #95335, #188364, #98298, #141837, #189361, #144823, #83149, #158012, #160000, #112495, #161002, #51821, #173191, #130654, #127661, #176183, #34667, #96325, #99318, #113481, #21488, #50838, #19503, #6307, #36641, #192348, #67985, #22496, #97305, #158991, #18518, #129639, #80165, #20483, #3329, #191335, #81148, #35657, #84143, #52813, #143827, #175175, #145822, #66991, #174189, #114480, #65002, #111505, #126660, #49841, #53830, #7305, #68990, #82133, #115505, #142829, #128650, #177193, #157020, #190345, #37653, #5307, #4309, #65992, #73010, #149835, #25518, #181187, #55825, #41670, #87163, #165013, #103334, #9336, #23496, #131668, #42664, #104326, #85144, #194358, #134679, #146830, #195356, #57833, #10336, #193350, #71992, #118511, #119506, #38666, #148845, #117498, #56836, #8324, #178188, #100321, #102332, #101314, #162000, #133666, #69999, #54826, #71002, #196365, #26507, #116500, #88150, #39653, #163003, #179195, #180201, #24510, #86160, #147850, #132670, #40663, #164022, #11339, #97951, #113141, #19164, #112160, #22143, #65649, #174831, #68634, #6954, #81786, #83793, #36296, #84791, #175829, #96969, #54478, #51479, #99967, #158650, #20141, #23147, #37302, #145473, #159643, #143473, #130290, #160651, #116148, #191984, #146470, #21139, #82794, #142491, #53471, #3969, #144476, #127311, #115148, #4957, #5960, #7962, #176841, #67638, #98961, #69645, #190993, #129297, #38312, #189022, #35315, #50496, #173849, #177839, #131311, #193001, #52469, #39307, #66642, #114128, #100966, #80813, #161651, #128305, #190005, #49093, #94584, #80405, #29951, #63254, #124934, #169443, #185616, #184622, #107759, #141091, #95577, #30946, #79421, #16763, #157263, #47106, #172431, #168454, #109758, #18758, #186631, #138117, #48102, #32929, #142077, #3563, #155274, #62248, #171442, #106779, #122935, #121946, #108766, #46104, #183639, #170443, #45121, #154282, #78411, #156263, #199798, #17765 ) ),
 .UNSPECIFIED., .T., .F., .F. ) 
 B_SPLINE_SURFACE_WITH_KNOTS ( ( 4, 3, 4 ),
 ( 3, 2, 2, 2, 2, 2, 2, 2, 2, 2, 2, 2, 2, 2, 2, 2, 2, 2, 2, 2, 2, 2, 2, 2, 2, 2, 2, 2, 2, 2, 2, 2, 2, 2, 2, 2, 2, 2, 2, 2, 2, 2, 2, 2, 2, 2, 2, 2, 2, 2, 2, 2, 2, 2, 2, 2, 2, 2, 2, 2, 2, 2, 2, 2, 2, 2, 2, 2, 2, 2, 2, 2, 2, 2, 2, 2, 2, 2, 2, 2, 2, 2, 2, 2, 2, 2, 2, 2, 2, 2, 2, 2, 2, 2, 2, 2, 2, 2, 2, 2, 2, 2, 2, 2, 2, 2, 2, 2, 2, 2, 2, 2, 2, 2, 2, 2, 2, 2, 2, 2, 2, 2, 2, 2, 2, 2, 2, 2, 2, 2, 2, 2, 2, 2, 2, 2, 2, 2, 2, 2, 2, 2, 2, 2, 2, 2, 2, 2, 2, 2, 2, 2, 2, 2, 2, 2, 2, 2, 2, 2, 2, 2, 2, 2, 2, 2, 2, 2, 2, 2, 2, 2, 2, 2, 2, 2, 2, 2, 2, 2, 2, 2, 2, 2, 2, 2, 2, 2, 2, 2, 2, 2, 2, 2, 2, 2, 2, 2, 2, 2, 2, 2, 2, 2, 2, 2, 2, 2, 2, 2, 2, 2, 2, 2, 2, 2, 2, 2, 2, 2, 2, 2, 2, 2, 2, 2, 2, 2, 3 ),
 ( 0.000000000000000000, 0.5000000000000000000, 1.000000000000000000 ),
 ( 0.000000000000000000, 0.004385964912280701511, 0.008771929824561403022, 0.01315789473684210453, 0.01754385964912280604, 0.02192982456140350755, 0.02631578947368420907, 0.03070175438596491058, 0.03508771929824561209, 0.03947368421052631360, 0.04385964912280701511, 0.04824561403508771662, 0.05263157894736841813, 0.05701754385964911964, 0.06140350877192982115, 0.06578947368421052266, 0.07017543859649122417, 0.07456140350877192569, 0.07894736842105262720, 0.08333333333333332871, 0.08771929824561403022, 0.09210526315789473173, 0.09649122807017543324, 0.1008771929824561348, 0.1052631578947368363, 0.1096491228070175378, 0.1140350877192982393, 0.1184210526315789408, 0.1228070175438596423, 0.1271929824561403577, 0.1315789473684210453, 0.1359649122807017607, 0.1403508771929824483, 0.1447368421052631637, 0.1491228070175438514, 0.1535087719298245668, 0.1578947368421052544, 0.1622807017543859698, 0.1666666666666666574, 0.1710526315789473728, 0.1754385964912280604, 0.1798245614035087758, 0.1842105263157894635, 0.1885964912280701788, 0.1929824561403508665, 0.1973684210526315819, 0.2017543859649122695, 0.2061403508771929849, 0.2105263157894736725, 0.2149122807017543879, 0.2192982456140350755, 0.2236842105263157909, 0.2280701754385964786, 0.2324561403508771940, 0.2368421052631578816, 0.2412280701754385970, 0.2456140350877192846, 0.2500000000000000000, 0.2543859649122807154, 0.2587719298245614308, 0.2631578947368420907, 0.2675438596491228060, 0.2719298245614035214, 0.2763157894736842368, 0.2807017543859648967, 0.2850877192982456121, 0.2894736842105263275, 0.2938596491228070429, 0.2982456140350877027, 0.3026315789473684181, 0.3070175438596491335, 0.3114035087719298489, 0.3157894736842105088, 0.3201754385964912242, 0.3245614035087719396, 0.3289473684210526550, 0.3333333333333333148, 0.3377192982456140302, 0.3421052631578947456, 0.3464912280701754610, 0.3508771929824561209, 0.3552631578947368363, 0.3596491228070175517, 0.3640350877192982670, 0.3684210526315789269, 0.3728070175438596423, 0.3771929824561403577, 0.3815789473684210731, 0.3859649122807017330, 0.3903508771929824483, 0.3947368421052631637, 0.3991228070175438791, 0.4035087719298245390, 0.4078947368421052544, 0.4122807017543859698, 0.4166666666666666852, 0.4210526315789473450, 0.4254385964912280604, 0.4298245614035087758, 0.4342105263157894912, 0.4385964912280701511, 0.4429824561403508665, 0.4473684210526315819, 0.4517543859649122973, 0.4561403508771929571, 0.4605263157894736725, 0.4649122807017543879, 0.4692982456140351033, 0.4736842105263157632, 0.4780701754385964786, 0.4824561403508771940, 0.4868421052631579093, 0.4912280701754385692, 0.4956140350877192846, 0.5000000000000000000, 0.5043859649122807154, 0.5087719298245614308, 0.5131578947368421462, 0.5175438596491228616, 0.5219298245614034659, 0.5263157894736841813, 0.5307017543859648967, 0.5350877192982456121, 0.5394736842105263275, 0.5438596491228070429, 0.5482456140350877583, 0.5526315789473684736, 0.5570175438596490780, 0.5614035087719297934, 0.5657894736842105088, 0.5701754385964912242, 0.5745614035087719396, 0.5789473684210526550, 0.5833333333333333703, 0.5877192982456140857, 0.5921052631578946901, 0.5964912280701754055, 0.6008771929824561209, 0.6052631578947368363, 0.6096491228070175517, 0.6140350877192982670, 0.6184210526315789824, 0.6228070175438596978, 0.6271929824561403022, 0.6315789473684210176, 0.6359649122807017330, 0.6403508771929824483, 0.6447368421052631637, 0.6491228070175438791, 0.6535087719298245945, 0.6578947368421053099, 0.6622807017543859143, 0.6666666666666666297, 0.6710526315789473450, 0.6754385964912280604, 0.6798245614035087758, 0.6842105263157894912, 0.6885964912280702066, 0.6929824561403509220, 0.6973684210526315264, 0.7017543859649122417, 0.7061403508771929571, 0.7105263157894736725, 0.7149122807017543879, 0.7192982456140351033, 0.7236842105263158187, 0.7280701754385965341, 0.7324561403508771384, 0.7368421052631578538, 0.7412280701754385692, 0.7456140350877192846, 0.7500000000000000000, 0.7543859649122807154, 0.7587719298245614308, 0.7631578947368421462, 0.7675438596491228616, 0.7719298245614034659, 0.7763157894736841813, 0.7807017543859648967, 0.7850877192982456121, 0.7894736842105263275, 0.7938596491228070429, 0.7982456140350877583, 0.8026315789473684736, 0.8070175438596490780, 0.8114035087719297934, 0.8157894736842105088, 0.8201754385964912242, 0.8245614035087719396, 0.8289473684210526550, 0.8333333333333333703, 0.8377192982456140857, 0.8421052631578946901, 0.8464912280701754055, 0.8508771929824561209, 0.8552631578947368363, 0.8596491228070175517, 0.8640350877192982670, 0.8684210526315789824, 0.8728070175438596978, 0.8771929824561403022, 0.8815789473684210176, 0.8859649122807017330, 0.8903508771929824483, 0.8947368421052631637, 0.8991228070175438791, 0.9035087719298245945, 0.9078947368421053099, 0.9122807017543859143, 0.9166666666666666297, 0.9210526315789473450, 0.9254385964912280604, 0.9298245614035087758, 0.9342105263157894912, 0.9385964912280702066, 0.9429824561403509220, 0.9473684210526315264, 0.9517543859649122417, 0.9561403508771929571, 0.9605263157894736725, 0.9649122807017543879, 0.9692982456140351033, 0.9736842105263158187, 0.9780701754385965341, 0.9824561403508771384, 0.9868421052631578538, 0.9912280701754385692, 0.9956140350877192846, 1.000000000000000000 ),
 .UNSPECIFIED. ) 
 GEOMETRIC_REPRESENTATION_ITEM ( )  RATIONAL_B_SPLINE_SURFACE ( (
 ( 1.000000000000000000, 0.9659258262890683122, 1.000000000000000000, 0.9659258262890683122, 1.000000000000000000, 0.9659258262890683122, 1.000000000000000000, 0.9659258262890683122, 1.000000000000000000, 0.9659258262890683122, 1.000000000000000000, 0.9659258262890683122, 1.000000000000000000, 0.9659258262890683122, 1.000000000000000000, 0.9659258262890683122, 1.000000000000000000, 0.9659258262890683122, 1.000000000000000000, 0.9659258262890683122, 1.000000000000000000, 0.9659258262890683122, 1.000000000000000000, 0.9659258262890683122, 1.000000000000000000, 0.9659258262890683122, 1.000000000000000000, 0.9659258262890683122, 1.000000000000000000, 0.9659258262890683122, 1.000000000000000000, 0.9659258262890683122, 1.000000000000000000, 0.9659258262890683122, 1.000000000000000000, 0.9659258262890683122, 1.000000000000000000, 0.9659258262890683122, 1.000000000000000000, 0.9659258262890683122, 1.000000000000000000, 0.9659258262890683122, 1.000000000000000000, 0.9659258262890683122, 1.000000000000000000, 0.9659258262890683122, 1.000000000000000000, 0.9659258262890683122, 1.000000000000000000, 0.9659258262890683122, 1.000000000000000000, 0.9659258262890683122, 1.000000000000000000, 0.9659258262890683122, 1.000000000000000000, 0.9659258262890683122, 1.000000000000000000, 0.9659258262890683122, 1.000000000000000000, 0.9659258262890683122, 1.000000000000000000, 0.9659258262890683122, 1.000000000000000000, 0.9659258262890683122, 1.000000000000000000, 0.9659258262890683122, 1.000000000000000000, 0.9659258262890683122, 1.000000000000000000, 0.9659258262890683122, 1.000000000000000000, 0.9659258262890683122, 1.000000000000000000, 0.9659258262890683122, 1.000000000000000000, 0.9659258262890683122, 1.000000000000000000, 0.9659258262890683122, 1.000000000000000000, 0.9659258262890683122, 1.000000000000000000, 0.9659258262890683122, 1.000000000000000000, 0.9659258262890683122, 1.000000000000000000, 0.9659258262890683122, 1.000000000000000000, 0.9659258262890683122, 1.000000000000000000, 0.9659258262890683122, 1.000000000000000000, 0.9659258262890683122, 1.000000000000000000, 0.9659258262890683122, 1.000000000000000000, 0.9659258262890683122, 1.000000000000000000, 0.9659258262890683122, 1.000000000000000000, 0.9659258262890683122, 1.000000000000000000, 0.9659258262890683122, 1.000000000000000000, 0.9659258262890683122, 1.000000000000000000, 0.9659258262890683122, 1.000000000000000000, 0.9659258262890683122, 1.000000000000000000, 0.9659258262890683122, 1.000000000000000000, 0.9659258262890683122, 1.000000000000000000, 0.9659258262890683122, 1.000000000000000000, 0.9659258262890683122, 1.000000000000000000, 0.9659258262890683122, 1.000000000000000000, 0.9659258262890683122, 1.000000000000000000, 0.9659258262890683122, 1.000000000000000000, 0.9659258262890683122, 1.000000000000000000, 0.9659258262890683122, 1.000000000000000000, 0.9659258262890683122, 1.000000000000000000, 0.9659258262890683122, 1.000000000000000000, 0.9659258262890683122, 1.000000000000000000, 0.9659258262890683122, 1.000000000000000000, 0.9659258262890683122, 1.000000000000000000, 0.9659258262890683122, 1.000000000000000000, 0.9659258262890683122, 1.000000000000000000, 0.9659258262890683122, 1.000000000000000000, 0.9659258262890683122, 1.000000000000000000, 0.9659258262890683122, 1.000000000000000000, 0.9659258262890683122, 1.000000000000000000, 0.9659258262890683122, 1.000000000000000000, 0.9659258262890683122, 1.000000000000000000, 0.9659258262890683122, 1.000000000000000000, 0.9659258262890683122, 1.000000000000000000, 0.9659258262890683122, 1.000000000000000000, 0.9659258262890683122, 1.000000000000000000, 0.9659258262890683122, 1.000000000000000000, 0.9659258262890683122, 1.000000000000000000, 0.9659258262890683122, 1.000000000000000000, 0.9659258262890683122, 1.000000000000000000, 0.9659258262890683122, 1.000000000000000000, 0.9659258262890683122, 1.000000000000000000, 0.9659258262890683122, 1.000000000000000000, 0.9659258262890683122, 1.000000000000000000, 0.9659258262890683122, 1.000000000000000000, 0.9659258262890683122, 1.000000000000000000, 0.9659258262890683122, 1.000000000000000000, 0.9659258262890683122, 1.000000000000000000, 0.9659258262890683122, 1.000000000000000000, 0.9659258262890683122, 1.000000000000000000, 0.9659258262890683122, 1.000000000000000000, 0.9659258262890683122, 1.000000000000000000, 0.9659258262890683122, 1.000000000000000000, 0.9659258262890683122, 1.000000000000000000, 0.9659258262890683122, 1.000000000000000000, 0.9659258262890683122, 1.000000000000000000, 0.9659258262890683122, 1.000000000000000000, 0.9659258262890683122, 1.000000000000000000, 0.9659258262890683122, 1.000000000000000000, 0.9659258262890683122, 1.000000000000000000, 0.9659258262890683122, 1.000000000000000000, 0.9659258262890683122, 1.000000000000000000, 0.9659258262890683122, 1.000000000000000000, 0.9659258262890683122, 1.000000000000000000, 0.9659258262890683122, 1.000000000000000000, 0.9659258262890683122, 1.000000000000000000, 0.9659258262890683122, 1.000000000000000000, 0.9659258262890683122, 1.000000000000000000, 0.9659258262890683122, 1.000000000000000000, 0.9659258262890683122, 1.000000000000000000, 0.9659258262890683122, 1.000000000000000000, 0.9659258262890683122, 1.000000000000000000, 0.9659258262890683122, 1.000000000000000000, 0.9659258262890683122, 1.000000000000000000, 0.9659258262890683122, 1.000000000000000000, 0.9659258262890683122, 1.000000000000000000, 0.9659258262890683122, 1.000000000000000000, 0.9659258262890683122, 1.000000000000000000, 0.9659258262890683122, 1.000000000000000000, 0.9659258262890683122, 1.000000000000000000, 0.9659258262890683122, 1.000000000000000000, 0.9659258262890683122, 1.000000000000000000, 0.9659258262890683122, 1.000000000000000000, 0.9659258262890683122, 1.000000000000000000, 0.9659258262890683122, 1.000000000000000000, 0.9659258262890683122, 1.000000000000000000, 0.9659258262890683122, 1.000000000000000000, 0.9659258262890683122, 1.000000000000000000, 0.9659258262890683122, 1.000000000000000000, 0.9659258262890683122, 1.000000000000000000, 0.9659258262890683122, 1.000000000000000000, 0.9659258262890683122, 1.000000000000000000, 0.9659258262890683122, 1.000000000000000000, 0.9659258262890683122, 1.000000000000000000, 0.9659258262890683122, 1.000000000000000000, 0.9659258262890683122, 1.000000000000000000, 0.9659258262890683122, 1.000000000000000000, 0.9659258262890683122, 1.000000000000000000, 0.9659258262890683122, 1.000000000000000000, 0.9659258262890683122, 1.000000000000000000, 0.9659258262890683122, 1.000000000000000000, 0.9659258262890683122, 1.000000000000000000, 0.9659258262890683122, 1.000000000000000000, 0.9659258262890683122, 1.000000000000000000, 0.9659258262890683122, 1.000000000000000000, 0.9659258262890683122, 1.000000000000000000, 0.9659258262890683122, 1.000000000000000000, 0.9659258262890683122, 1.000000000000000000, 0.9659258262890683122, 1.000000000000000000, 0.9659258262890683122, 1.000000000000000000, 0.9659258262890683122, 1.000000000000000000, 0.9659258262890683122, 1.000000000000000000, 0.9659258262890683122, 1.000000000000000000, 0.9659258262890683122, 1.000000000000000000, 0.9659258262890683122, 1.000000000000000000, 0.9659258262890683122, 1.000000000000000000, 0.9659258262890683122, 1.000000000000000000, 0.9659258262890683122, 1.000000000000000000, 0.9659258262890683122, 1.000000000000000000, 0.9659258262890683122, 1.000000000000000000, 0.9659258262890683122, 1.000000000000000000, 0.9659258262890683122, 1.000000000000000000, 0.9659258262890683122, 1.000000000000000000, 0.9659258262890683122, 1.000000000000000000, 0.9659258262890683122, 1.000000000000000000, 0.9659258262890683122, 1.000000000000000000, 0.9659258262890683122, 1.000000000000000000, 0.9659258262890683122, 1.000000000000000000, 0.9659258262890683122, 1.000000000000000000, 0.9659258262890683122, 1.000000000000000000, 0.9659258262890683122, 1.000000000000000000, 0.9659258262890683122, 1.000000000000000000, 0.9659258262890683122, 1.000000000000000000, 0.9659258262890683122, 1.000000000000000000, 0.9659258262890683122, 1.000000000000000000, 0.9659258262890683122, 1.000000000000000000, 0.9659258262890683122, 1.000000000000000000, 0.9659258262890683122, 1.000000000000000000, 0.9659258262890683122, 1.000000000000000000, 0.9659258262890683122, 1.000000000000000000, 0.9659258262890683122, 1.000000000000000000, 0.9659258262890683122, 1.000000000000000000, 0.9659258262890683122, 1.000000000000000000, 0.9659258262890683122, 1.000000000000000000, 0.9659258262890683122, 1.000000000000000000, 0.9659258262890683122, 1.000000000000000000, 0.9659258262890683122, 1.000000000000000000, 0.9659258262890683122, 1.000000000000000000, 0.9659258262890683122, 1.000000000000000000, 0.9659258262890683122, 1.000000000000000000, 0.9659258262890683122, 1.000000000000000000, 0.9659258262890683122, 1.000000000000000000, 0.9659258262890683122, 1.000000000000000000, 0.9659258262890683122, 1.000000000000000000, 0.9659258262890683122, 1.000000000000000000, 0.9659258262890683122, 1.000000000000000000, 0.9659258262890683122, 1.000000000000000000, 0.9659258262890683122, 1.000000000000000000, 0.9659258262890683122, 1.000000000000000000, 0.9659258262890683122, 1.000000000000000000, 0.9659258262890683122, 1.000000000000000000, 0.9659258262890683122, 1.000000000000000000, 0.9659258262890683122, 1.000000000000000000, 0.9659258262890683122, 1.000000000000000000, 0.9659258262890683122, 1.000000000000000000, 0.9659258262890683122, 1.000000000000000000, 0.9659258262890683122, 1.000000000000000000, 0.9659258262890683122, 1.000000000000000000, 0.9659258262890683122, 1.000000000000000000, 0.9659258262890683122, 1.000000000000000000, 0.9659258262890683122, 1.000000000000000000, 0.9659258262890683122, 1.000000000000000000, 0.9659258262890683122, 1.000000000000000000, 0.9659258262890683122, 1.000000000000000000, 0.9659258262890683122, 1.000000000000000000, 0.9659258262890683122, 1.000000000000000000, 0.9659258262890683122, 1.000000000000000000, 0.9659258262890683122, 1.000000000000000000, 0.9659258262890683122, 1.000000000000000000, 0.9659258262890683122, 1.000000000000000000, 0.9659258262890683122, 1.000000000000000000, 0.9659258262890683122, 1.000000000000000000, 0.9659258262890683122, 1.000000000000000000, 0.9659258262890683122, 1.000000000000000000),
 ( 0.3333333333333333703, 0.3219752754296894559, 0.3333333333333333703, 0.3219752754296894559, 0.3333333333333333703, 0.3219752754296894559, 0.3333333333333333703, 0.3219752754296894559, 0.3333333333333333703, 0.3219752754296894559, 0.3333333333333333703, 0.3219752754296894559, 0.3333333333333333703, 0.3219752754296894559, 0.3333333333333333703, 0.3219752754296894559, 0.3333333333333333703, 0.3219752754296894559, 0.3333333333333333703, 0.3219752754296894559, 0.3333333333333333703, 0.3219752754296894559, 0.3333333333333333703, 0.3219752754296894559, 0.3333333333333333703, 0.3219752754296894559, 0.3333333333333333703, 0.3219752754296894559, 0.3333333333333333703, 0.3219752754296894559, 0.3333333333333333703, 0.3219752754296894559, 0.3333333333333333703, 0.3219752754296894559, 0.3333333333333333703, 0.3219752754296894559, 0.3333333333333333703, 0.3219752754296894559, 0.3333333333333333703, 0.3219752754296894559, 0.3333333333333333703, 0.3219752754296894559, 0.3333333333333333703, 0.3219752754296894559, 0.3333333333333333703, 0.3219752754296894559, 0.3333333333333333703, 0.3219752754296894559, 0.3333333333333333703, 0.3219752754296894559, 0.3333333333333333703, 0.3219752754296894559, 0.3333333333333333703, 0.3219752754296894559, 0.3333333333333333703, 0.3219752754296894559, 0.3333333333333333703, 0.3219752754296894559, 0.3333333333333333703, 0.3219752754296894559, 0.3333333333333333703, 0.3219752754296894559, 0.3333333333333333703, 0.3219752754296894559, 0.3333333333333333703, 0.3219752754296894559, 0.3333333333333333703, 0.3219752754296894559, 0.3333333333333333703, 0.3219752754296894559, 0.3333333333333333703, 0.3219752754296894559, 0.3333333333333333703, 0.3219752754296894559, 0.3333333333333333703, 0.3219752754296894559, 0.3333333333333333703, 0.3219752754296894559, 0.3333333333333333703, 0.3219752754296894559, 0.3333333333333333703, 0.3219752754296894559, 0.3333333333333333703, 0.3219752754296894559, 0.3333333333333333703, 0.3219752754296894559, 0.3333333333333333703, 0.3219752754296894559, 0.3333333333333333703, 0.3219752754296894559, 0.3333333333333333703, 0.3219752754296894559, 0.3333333333333333703, 0.3219752754296894559, 0.3333333333333333703, 0.3219752754296894559, 0.3333333333333333703, 0.3219752754296894559, 0.3333333333333333703, 0.3219752754296894559, 0.3333333333333333703, 0.3219752754296894559, 0.3333333333333333703, 0.3219752754296894559, 0.3333333333333333703, 0.3219752754296894559, 0.3333333333333333703, 0.3219752754296894559, 0.3333333333333333703, 0.3219752754296894559, 0.3333333333333333703, 0.3219752754296894559, 0.3333333333333333703, 0.3219752754296894559, 0.3333333333333333703, 0.3219752754296894559, 0.3333333333333333703, 0.3219752754296894559, 0.3333333333333333703, 0.3219752754296894559, 0.3333333333333333703, 0.3219752754296894559, 0.3333333333333333703, 0.3219752754296894559, 0.3333333333333333703, 0.3219752754296894559, 0.3333333333333333703, 0.3219752754296894559, 0.3333333333333333703, 0.3219752754296894559, 0.3333333333333333703, 0.3219752754296894559, 0.3333333333333333703, 0.3219752754296894559, 0.3333333333333333703, 0.3219752754296894559, 0.3333333333333333703, 0.3219752754296894559, 0.3333333333333333703, 0.3219752754296894559, 0.3333333333333333703, 0.3219752754296894559, 0.3333333333333333703, 0.3219752754296894559, 0.3333333333333333703, 0.3219752754296894559, 0.3333333333333333703, 0.3219752754296894559, 0.3333333333333333703, 0.3219752754296894559, 0.3333333333333333703, 0.3219752754296894559, 0.3333333333333333703, 0.3219752754296894559, 0.3333333333333333703, 0.3219752754296894559, 0.3333333333333333703, 0.3219752754296894559, 0.3333333333333333703, 0.3219752754296894559, 0.3333333333333333703, 0.3219752754296894559, 0.3333333333333333703, 0.3219752754296894559, 0.3333333333333333703, 0.3219752754296894559, 0.3333333333333333703, 0.3219752754296894559, 0.3333333333333333703, 0.3219752754296894559, 0.3333333333333333703, 0.3219752754296894559, 0.3333333333333333703, 0.3219752754296894559, 0.3333333333333333703, 0.3219752754296894559, 0.3333333333333333703, 0.3219752754296894559, 0.3333333333333333703, 0.3219752754296894559, 0.3333333333333333703, 0.3219752754296894559, 0.3333333333333333703, 0.3219752754296894559, 0.3333333333333333703, 0.3219752754296894559, 0.3333333333333333703, 0.3219752754296894559, 0.3333333333333333703, 0.3219752754296894559, 0.3333333333333333703, 0.3219752754296894559, 0.3333333333333333703, 0.3219752754296894559, 0.3333333333333333703, 0.3219752754296894559, 0.3333333333333333703, 0.3219752754296894559, 0.3333333333333333703, 0.3219752754296894559, 0.3333333333333333703, 0.3219752754296894559, 0.3333333333333333703, 0.3219752754296894559, 0.3333333333333333703, 0.3219752754296894559, 0.3333333333333333703, 0.3219752754296894559, 0.3333333333333333703, 0.3219752754296894559, 0.3333333333333333703, 0.3219752754296894559, 0.3333333333333333703, 0.3219752754296894559, 0.3333333333333333703, 0.3219752754296894559, 0.3333333333333333703, 0.3219752754296894559, 0.3333333333333333703, 0.3219752754296894559, 0.3333333333333333703, 0.3219752754296894559, 0.3333333333333333703, 0.3219752754296894559, 0.3333333333333333703, 0.3219752754296894559, 0.3333333333333333703, 0.3219752754296894559, 0.3333333333333333703, 0.3219752754296894559, 0.3333333333333333703, 0.3219752754296894559, 0.3333333333333333703, 0.3219752754296894559, 0.3333333333333333703, 0.3219752754296894559, 0.3333333333333333703, 0.3219752754296894559, 0.3333333333333333703, 0.3219752754296894559, 0.3333333333333333703, 0.3219752754296894559, 0.3333333333333333703, 0.3219752754296894559, 0.3333333333333333703, 0.3219752754296894559, 0.3333333333333333703, 0.3219752754296894559, 0.3333333333333333703, 0.3219752754296894559, 0.3333333333333333703, 0.3219752754296894559, 0.3333333333333333703, 0.3219752754296894559, 0.3333333333333333703, 0.3219752754296894559, 0.3333333333333333703, 0.3219752754296894559, 0.3333333333333333703, 0.3219752754296894559, 0.3333333333333333703, 0.3219752754296894559, 0.3333333333333333703, 0.3219752754296894559, 0.3333333333333333703, 0.3219752754296894559, 0.3333333333333333703, 0.3219752754296894559, 0.3333333333333333703, 0.3219752754296894559, 0.3333333333333333703, 0.3219752754296894559, 0.3333333333333333703, 0.3219752754296894559, 0.3333333333333333703, 0.3219752754296894559, 0.3333333333333333703, 0.3219752754296894559, 0.3333333333333333703, 0.3219752754296894559, 0.3333333333333333703, 0.3219752754296894559, 0.3333333333333333703, 0.3219752754296894559, 0.3333333333333333703, 0.3219752754296894559, 0.3333333333333333703, 0.3219752754296894559, 0.3333333333333333703, 0.3219752754296894559, 0.3333333333333333703, 0.3219752754296894559, 0.3333333333333333703, 0.3219752754296894559, 0.3333333333333333703, 0.3219752754296894559, 0.3333333333333333703, 0.3219752754296894559, 0.3333333333333333703, 0.3219752754296894559, 0.3333333333333333703, 0.3219752754296894559, 0.3333333333333333703, 0.3219752754296894559, 0.3333333333333333703, 0.3219752754296894559, 0.3333333333333333703, 0.3219752754296894559, 0.3333333333333333703, 0.3219752754296894559, 0.3333333333333333703, 0.3219752754296894559, 0.3333333333333333703, 0.3219752754296894559, 0.3333333333333333703, 0.3219752754296894559, 0.3333333333333333703, 0.3219752754296894559, 0.3333333333333333703, 0.3219752754296894559, 0.3333333333333333703, 0.3219752754296894559, 0.3333333333333333703, 0.3219752754296894559, 0.3333333333333333703, 0.3219752754296894559, 0.3333333333333333703, 0.3219752754296894559, 0.3333333333333333703, 0.3219752754296894559, 0.3333333333333333703, 0.3219752754296894559, 0.3333333333333333703, 0.3219752754296894559, 0.3333333333333333703, 0.3219752754296894559, 0.3333333333333333703, 0.3219752754296894559, 0.3333333333333333703, 0.3219752754296894559, 0.3333333333333333703, 0.3219752754296894559, 0.3333333333333333703, 0.3219752754296894559, 0.3333333333333333703, 0.3219752754296894559, 0.3333333333333333703, 0.3219752754296894559, 0.3333333333333333703, 0.3219752754296894559, 0.3333333333333333703, 0.3219752754296894559, 0.3333333333333333703, 0.3219752754296894559, 0.3333333333333333703, 0.3219752754296894559, 0.3333333333333333703, 0.3219752754296894559, 0.3333333333333333703, 0.3219752754296894559, 0.3333333333333333703, 0.3219752754296894559, 0.3333333333333333703, 0.3219752754296894559, 0.3333333333333333703, 0.3219752754296894559, 0.3333333333333333703, 0.3219752754296894559, 0.3333333333333333703, 0.3219752754296894559, 0.3333333333333333703, 0.3219752754296894559, 0.3333333333333333703, 0.3219752754296894559, 0.3333333333333333703, 0.3219752754296894559, 0.3333333333333333703, 0.3219752754296894559, 0.3333333333333333703, 0.3219752754296894559, 0.3333333333333333703, 0.3219752754296894559, 0.3333333333333333703, 0.3219752754296894559, 0.3333333333333333703, 0.3219752754296894559, 0.3333333333333333703, 0.3219752754296894559, 0.3333333333333333703, 0.3219752754296894559, 0.3333333333333333703, 0.3219752754296894559, 0.3333333333333333703, 0.3219752754296894559, 0.3333333333333333703, 0.3219752754296894559, 0.3333333333333333703, 0.3219752754296894559, 0.3333333333333333703, 0.3219752754296894559, 0.3333333333333333703, 0.3219752754296894559, 0.3333333333333333703, 0.3219752754296894559, 0.3333333333333333703, 0.3219752754296894559, 0.3333333333333333703, 0.3219752754296894559, 0.3333333333333333703, 0.3219752754296894559, 0.3333333333333333703, 0.3219752754296894559, 0.3333333333333333703, 0.3219752754296894559, 0.3333333333333333703, 0.3219752754296894559, 0.3333333333333333703, 0.3219752754296894559, 0.3333333333333333703, 0.3219752754296894559, 0.3333333333333333703, 0.3219752754296894559, 0.3333333333333333703, 0.3219752754296894559, 0.3333333333333333703, 0.3219752754296894559, 0.3333333333333333703, 0.3219752754296894559, 0.3333333333333333703, 0.3219752754296894559, 0.3333333333333333703, 0.3219752754296894559, 0.3333333333333333703, 0.3219752754296894559, 0.3333333333333333703, 0.3219752754296894559, 0.3333333333333333703, 0.3219752754296894559, 0.3333333333333333703, 0.3219752754296894559, 0.3333333333333333703, 0.3219752754296894559, 0.3333333333333333703, 0.3219752754296894559, 0.3333333333333333703, 0.3219752754296894559, 0.3333333333333333703, 0.3219752754296894559, 0.3333333333333333703, 0.3219752754296894559, 0.3333333333333333703, 0.3219752754296894559, 0.3333333333333333703, 0.3219752754296894559, 0.3333333333333333703, 0.3219752754296894559, 0.3333333333333333703),
 ( 0.3333333333333333703, 0.3219752754296894559, 0.3333333333333333703, 0.3219752754296894559, 0.3333333333333333703, 0.3219752754296894559, 0.3333333333333333703, 0.3219752754296894559, 0.3333333333333333703, 0.3219752754296894559, 0.3333333333333333703, 0.3219752754296894559, 0.3333333333333333703, 0.3219752754296894559, 0.3333333333333333703, 0.3219752754296894559, 0.3333333333333333703, 0.3219752754296894559, 0.3333333333333333703, 0.3219752754296894559, 0.3333333333333333703, 0.3219752754296894559, 0.3333333333333333703, 0.3219752754296894559, 0.3333333333333333703, 0.3219752754296894559, 0.3333333333333333703, 0.3219752754296894559, 0.3333333333333333703, 0.3219752754296894559, 0.3333333333333333703, 0.3219752754296894559, 0.3333333333333333703, 0.3219752754296894559, 0.3333333333333333703, 0.3219752754296894559, 0.3333333333333333703, 0.3219752754296894559, 0.3333333333333333703, 0.3219752754296894559, 0.3333333333333333703, 0.3219752754296894559, 0.3333333333333333703, 0.3219752754296894559, 0.3333333333333333703, 0.3219752754296894559, 0.3333333333333333703, 0.3219752754296894559, 0.3333333333333333703, 0.3219752754296894559, 0.3333333333333333703, 0.3219752754296894559, 0.3333333333333333703, 0.3219752754296894559, 0.3333333333333333703, 0.3219752754296894559, 0.3333333333333333703, 0.3219752754296894559, 0.3333333333333333703, 0.3219752754296894559, 0.3333333333333333703, 0.3219752754296894559, 0.3333333333333333703, 0.3219752754296894559, 0.3333333333333333703, 0.3219752754296894559, 0.3333333333333333703, 0.3219752754296894559, 0.3333333333333333703, 0.3219752754296894559, 0.3333333333333333703, 0.3219752754296894559, 0.3333333333333333703, 0.3219752754296894559, 0.3333333333333333703, 0.3219752754296894559, 0.3333333333333333703, 0.3219752754296894559, 0.3333333333333333703, 0.3219752754296894559, 0.3333333333333333703, 0.3219752754296894559, 0.3333333333333333703, 0.3219752754296894559, 0.3333333333333333703, 0.3219752754296894559, 0.3333333333333333703, 0.3219752754296894559, 0.3333333333333333703, 0.3219752754296894559, 0.3333333333333333703, 0.3219752754296894559, 0.3333333333333333703, 0.3219752754296894559, 0.3333333333333333703, 0.3219752754296894559, 0.3333333333333333703, 0.3219752754296894559, 0.3333333333333333703, 0.3219752754296894559, 0.3333333333333333703, 0.3219752754296894559, 0.3333333333333333703, 0.3219752754296894559, 0.3333333333333333703, 0.3219752754296894559, 0.3333333333333333703, 0.3219752754296894559, 0.3333333333333333703, 0.3219752754296894559, 0.3333333333333333703, 0.3219752754296894559, 0.3333333333333333703, 0.3219752754296894559, 0.3333333333333333703, 0.3219752754296894559, 0.3333333333333333703, 0.3219752754296894559, 0.3333333333333333703, 0.3219752754296894559, 0.3333333333333333703, 0.3219752754296894559, 0.3333333333333333703, 0.3219752754296894559, 0.3333333333333333703, 0.3219752754296894559, 0.3333333333333333703, 0.3219752754296894559, 0.3333333333333333703, 0.3219752754296894559, 0.3333333333333333703, 0.3219752754296894559, 0.3333333333333333703, 0.3219752754296894559, 0.3333333333333333703, 0.3219752754296894559, 0.3333333333333333703, 0.3219752754296894559, 0.3333333333333333703, 0.3219752754296894559, 0.3333333333333333703, 0.3219752754296894559, 0.3333333333333333703, 0.3219752754296894559, 0.3333333333333333703, 0.3219752754296894559, 0.3333333333333333703, 0.3219752754296894559, 0.3333333333333333703, 0.3219752754296894559, 0.3333333333333333703, 0.3219752754296894559, 0.3333333333333333703, 0.3219752754296894559, 0.3333333333333333703, 0.3219752754296894559, 0.3333333333333333703, 0.3219752754296894559, 0.3333333333333333703, 0.3219752754296894559, 0.3333333333333333703, 0.3219752754296894559, 0.3333333333333333703, 0.3219752754296894559, 0.3333333333333333703, 0.3219752754296894559, 0.3333333333333333703, 0.3219752754296894559, 0.3333333333333333703, 0.3219752754296894559, 0.3333333333333333703, 0.3219752754296894559, 0.3333333333333333703, 0.3219752754296894559, 0.3333333333333333703, 0.3219752754296894559, 0.3333333333333333703, 0.3219752754296894559, 0.3333333333333333703, 0.3219752754296894559, 0.3333333333333333703, 0.3219752754296894559, 0.3333333333333333703, 0.3219752754296894559, 0.3333333333333333703, 0.3219752754296894559, 0.3333333333333333703, 0.3219752754296894559, 0.3333333333333333703, 0.3219752754296894559, 0.3333333333333333703, 0.3219752754296894559, 0.3333333333333333703, 0.3219752754296894559, 0.3333333333333333703, 0.3219752754296894559, 0.3333333333333333703, 0.3219752754296894559, 0.3333333333333333703, 0.3219752754296894559, 0.3333333333333333703, 0.3219752754296894559, 0.3333333333333333703, 0.3219752754296894559, 0.3333333333333333703, 0.3219752754296894559, 0.3333333333333333703, 0.3219752754296894559, 0.3333333333333333703, 0.3219752754296894559, 0.3333333333333333703, 0.3219752754296894559, 0.3333333333333333703, 0.3219752754296894559, 0.3333333333333333703, 0.3219752754296894559, 0.3333333333333333703, 0.3219752754296894559, 0.3333333333333333703, 0.3219752754296894559, 0.3333333333333333703, 0.3219752754296894559, 0.3333333333333333703, 0.3219752754296894559, 0.3333333333333333703, 0.3219752754296894559, 0.3333333333333333703, 0.3219752754296894559, 0.3333333333333333703, 0.3219752754296894559, 0.3333333333333333703, 0.3219752754296894559, 0.3333333333333333703, 0.3219752754296894559, 0.3333333333333333703, 0.3219752754296894559, 0.3333333333333333703, 0.3219752754296894559, 0.3333333333333333703, 0.3219752754296894559, 0.3333333333333333703, 0.3219752754296894559, 0.3333333333333333703, 0.3219752754296894559, 0.3333333333333333703, 0.3219752754296894559, 0.3333333333333333703, 0.3219752754296894559, 0.3333333333333333703, 0.3219752754296894559, 0.3333333333333333703, 0.3219752754296894559, 0.3333333333333333703, 0.3219752754296894559, 0.3333333333333333703, 0.3219752754296894559, 0.3333333333333333703, 0.3219752754296894559, 0.3333333333333333703, 0.3219752754296894559, 0.3333333333333333703, 0.3219752754296894559, 0.3333333333333333703, 0.3219752754296894559, 0.3333333333333333703, 0.3219752754296894559, 0.3333333333333333703, 0.3219752754296894559, 0.3333333333333333703, 0.3219752754296894559, 0.3333333333333333703, 0.3219752754296894559, 0.3333333333333333703, 0.3219752754296894559, 0.3333333333333333703, 0.3219752754296894559, 0.3333333333333333703, 0.3219752754296894559, 0.3333333333333333703, 0.3219752754296894559, 0.3333333333333333703, 0.3219752754296894559, 0.3333333333333333703, 0.3219752754296894559, 0.3333333333333333703, 0.3219752754296894559, 0.3333333333333333703, 0.3219752754296894559, 0.3333333333333333703, 0.3219752754296894559, 0.3333333333333333703, 0.3219752754296894559, 0.3333333333333333703, 0.3219752754296894559, 0.3333333333333333703, 0.3219752754296894559, 0.3333333333333333703, 0.3219752754296894559, 0.3333333333333333703, 0.3219752754296894559, 0.3333333333333333703, 0.3219752754296894559, 0.3333333333333333703, 0.3219752754296894559, 0.3333333333333333703, 0.3219752754296894559, 0.3333333333333333703, 0.3219752754296894559, 0.3333333333333333703, 0.3219752754296894559, 0.3333333333333333703, 0.3219752754296894559, 0.3333333333333333703, 0.3219752754296894559, 0.3333333333333333703, 0.3219752754296894559, 0.3333333333333333703, 0.3219752754296894559, 0.3333333333333333703, 0.3219752754296894559, 0.3333333333333333703, 0.3219752754296894559, 0.3333333333333333703, 0.3219752754296894559, 0.3333333333333333703, 0.3219752754296894559, 0.3333333333333333703, 0.3219752754296894559, 0.3333333333333333703, 0.3219752754296894559, 0.3333333333333333703, 0.3219752754296894559, 0.3333333333333333703, 0.3219752754296894559, 0.3333333333333333703, 0.3219752754296894559, 0.3333333333333333703, 0.3219752754296894559, 0.3333333333333333703, 0.3219752754296894559, 0.3333333333333333703, 0.3219752754296894559, 0.3333333333333333703, 0.3219752754296894559, 0.3333333333333333703, 0.3219752754296894559, 0.3333333333333333703, 0.3219752754296894559, 0.3333333333333333703, 0.3219752754296894559, 0.3333333333333333703, 0.3219752754296894559, 0.3333333333333333703, 0.3219752754296894559, 0.3333333333333333703, 0.3219752754296894559, 0.3333333333333333703, 0.3219752754296894559, 0.3333333333333333703, 0.3219752754296894559, 0.3333333333333333703, 0.3219752754296894559, 0.3333333333333333703, 0.3219752754296894559, 0.3333333333333333703, 0.3219752754296894559, 0.3333333333333333703, 0.3219752754296894559, 0.3333333333333333703, 0.3219752754296894559, 0.3333333333333333703, 0.3219752754296894559, 0.3333333333333333703, 0.3219752754296894559, 0.3333333333333333703, 0.3219752754296894559, 0.3333333333333333703, 0.3219752754296894559, 0.3333333333333333703, 0.3219752754296894559, 0.3333333333333333703, 0.3219752754296894559, 0.3333333333333333703, 0.3219752754296894559, 0.3333333333333333703, 0.3219752754296894559, 0.3333333333333333703, 0.3219752754296894559, 0.3333333333333333703, 0.3219752754296894559, 0.3333333333333333703, 0.3219752754296894559, 0.3333333333333333703, 0.3219752754296894559, 0.3333333333333333703, 0.3219752754296894559, 0.3333333333333333703, 0.3219752754296894559, 0.3333333333333333703, 0.3219752754296894559, 0.3333333333333333703, 0.3219752754296894559, 0.3333333333333333703, 0.3219752754296894559, 0.3333333333333333703, 0.3219752754296894559, 0.3333333333333333703, 0.3219752754296894559, 0.3333333333333333703, 0.3219752754296894559, 0.3333333333333333703, 0.3219752754296894559, 0.3333333333333333703, 0.3219752754296894559, 0.3333333333333333703, 0.3219752754296894559, 0.3333333333333333703, 0.3219752754296894559, 0.3333333333333333703, 0.3219752754296894559, 0.3333333333333333703, 0.3219752754296894559, 0.3333333333333333703, 0.3219752754296894559, 0.3333333333333333703, 0.3219752754296894559, 0.3333333333333333703, 0.3219752754296894559, 0.3333333333333333703, 0.3219752754296894559, 0.3333333333333333703, 0.3219752754296894559, 0.3333333333333333703, 0.3219752754296894559, 0.3333333333333333703, 0.3219752754296894559, 0.3333333333333333703, 0.3219752754296894559, 0.3333333333333333703, 0.3219752754296894559, 0.3333333333333333703, 0.3219752754296894559, 0.3333333333333333703, 0.3219752754296894559, 0.3333333333333333703, 0.3219752754296894559, 0.3333333333333333703, 0.3219752754296894559, 0.3333333333333333703, 0.3219752754296894559, 0.3333333333333333703, 0.3219752754296894559, 0.3333333333333333703, 0.3219752754296894559, 0.3333333333333333703, 0.3219752754296894559, 0.3333333333333333703),
 ( 1.000000000000000000, 0.9659258262890683122, 1.000000000000000000, 0.9659258262890683122, 1.000000000000000000, 0.9659258262890683122, 1.000000000000000000, 0.9659258262890683122, 1.000000000000000000, 0.9659258262890683122, 1.000000000000000000, 0.9659258262890683122, 1.000000000000000000, 0.9659258262890683122, 1.000000000000000000, 0.9659258262890683122, 1.000000000000000000, 0.9659258262890683122, 1.000000000000000000, 0.9659258262890683122, 1.000000000000000000, 0.9659258262890683122, 1.000000000000000000, 0.9659258262890683122, 1.000000000000000000, 0.9659258262890683122, 1.000000000000000000, 0.9659258262890683122, 1.000000000000000000, 0.9659258262890683122, 1.000000000000000000, 0.9659258262890683122, 1.000000000000000000, 0.9659258262890683122, 1.000000000000000000, 0.9659258262890683122, 1.000000000000000000, 0.9659258262890683122, 1.000000000000000000, 0.9659258262890683122, 1.000000000000000000, 0.9659258262890683122, 1.000000000000000000, 0.9659258262890683122, 1.000000000000000000, 0.9659258262890683122, 1.000000000000000000, 0.9659258262890683122, 1.000000000000000000, 0.9659258262890683122, 1.000000000000000000, 0.9659258262890683122, 1.000000000000000000, 0.9659258262890683122, 1.000000000000000000, 0.9659258262890683122, 1.000000000000000000, 0.9659258262890683122, 1.000000000000000000, 0.9659258262890683122, 1.000000000000000000, 0.9659258262890683122, 1.000000000000000000, 0.9659258262890683122, 1.000000000000000000, 0.9659258262890683122, 1.000000000000000000, 0.9659258262890683122, 1.000000000000000000, 0.9659258262890683122, 1.000000000000000000, 0.9659258262890683122, 1.000000000000000000, 0.9659258262890683122, 1.000000000000000000, 0.9659258262890683122, 1.000000000000000000, 0.9659258262890683122, 1.000000000000000000, 0.9659258262890683122, 1.000000000000000000, 0.9659258262890683122, 1.000000000000000000, 0.9659258262890683122, 1.000000000000000000, 0.9659258262890683122, 1.000000000000000000, 0.9659258262890683122, 1.000000000000000000, 0.9659258262890683122, 1.000000000000000000, 0.9659258262890683122, 1.000000000000000000, 0.9659258262890683122, 1.000000000000000000, 0.9659258262890683122, 1.000000000000000000, 0.9659258262890683122, 1.000000000000000000, 0.9659258262890683122, 1.000000000000000000, 0.9659258262890683122, 1.000000000000000000, 0.9659258262890683122, 1.000000000000000000, 0.9659258262890683122, 1.000000000000000000, 0.9659258262890683122, 1.000000000000000000, 0.9659258262890683122, 1.000000000000000000, 0.9659258262890683122, 1.000000000000000000, 0.9659258262890683122, 1.000000000000000000, 0.9659258262890683122, 1.000000000000000000, 0.9659258262890683122, 1.000000000000000000, 0.9659258262890683122, 1.000000000000000000, 0.9659258262890683122, 1.000000000000000000, 0.9659258262890683122, 1.000000000000000000, 0.9659258262890683122, 1.000000000000000000, 0.9659258262890683122, 1.000000000000000000, 0.9659258262890683122, 1.000000000000000000, 0.9659258262890683122, 1.000000000000000000, 0.9659258262890683122, 1.000000000000000000, 0.9659258262890683122, 1.000000000000000000, 0.9659258262890683122, 1.000000000000000000, 0.9659258262890683122, 1.000000000000000000, 0.9659258262890683122, 1.000000000000000000, 0.9659258262890683122, 1.000000000000000000, 0.9659258262890683122, 1.000000000000000000, 0.9659258262890683122, 1.000000000000000000, 0.9659258262890683122, 1.000000000000000000, 0.9659258262890683122, 1.000000000000000000, 0.9659258262890683122, 1.000000000000000000, 0.9659258262890683122, 1.000000000000000000, 0.9659258262890683122, 1.000000000000000000, 0.9659258262890683122, 1.000000000000000000, 0.9659258262890683122, 1.000000000000000000, 0.9659258262890683122, 1.000000000000000000, 0.9659258262890683122, 1.000000000000000000, 0.9659258262890683122, 1.000000000000000000, 0.9659258262890683122, 1.000000000000000000, 0.9659258262890683122, 1.000000000000000000, 0.9659258262890683122, 1.000000000000000000, 0.9659258262890683122, 1.000000000000000000, 0.9659258262890683122, 1.000000000000000000, 0.9659258262890683122, 1.000000000000000000, 0.9659258262890683122, 1.000000000000000000, 0.9659258262890683122, 1.000000000000000000, 0.9659258262890683122, 1.000000000000000000, 0.9659258262890683122, 1.000000000000000000, 0.9659258262890683122, 1.000000000000000000, 0.9659258262890683122, 1.000000000000000000, 0.9659258262890683122, 1.000000000000000000, 0.9659258262890683122, 1.000000000000000000, 0.9659258262890683122, 1.000000000000000000, 0.9659258262890683122, 1.000000000000000000, 0.9659258262890683122, 1.000000000000000000, 0.9659258262890683122, 1.000000000000000000, 0.9659258262890683122, 1.000000000000000000, 0.9659258262890683122, 1.000000000000000000, 0.9659258262890683122, 1.000000000000000000, 0.9659258262890683122, 1.000000000000000000, 0.9659258262890683122, 1.000000000000000000, 0.9659258262890683122, 1.000000000000000000, 0.9659258262890683122, 1.000000000000000000, 0.9659258262890683122, 1.000000000000000000, 0.9659258262890683122, 1.000000000000000000, 0.9659258262890683122, 1.000000000000000000, 0.9659258262890683122, 1.000000000000000000, 0.9659258262890683122, 1.000000000000000000, 0.9659258262890683122, 1.000000000000000000, 0.9659258262890683122, 1.000000000000000000, 0.9659258262890683122, 1.000000000000000000, 0.9659258262890683122, 1.000000000000000000, 0.9659258262890683122, 1.000000000000000000, 0.9659258262890683122, 1.000000000000000000, 0.9659258262890683122, 1.000000000000000000, 0.9659258262890683122, 1.000000000000000000, 0.9659258262890683122, 1.000000000000000000, 0.9659258262890683122, 1.000000000000000000, 0.9659258262890683122, 1.000000000000000000, 0.9659258262890683122, 1.000000000000000000, 0.9659258262890683122, 1.000000000000000000, 0.9659258262890683122, 1.000000000000000000, 0.9659258262890683122, 1.000000000000000000, 0.9659258262890683122, 1.000000000000000000, 0.9659258262890683122, 1.000000000000000000, 0.9659258262890683122, 1.000000000000000000, 0.9659258262890683122, 1.000000000000000000, 0.9659258262890683122, 1.000000000000000000, 0.9659258262890683122, 1.000000000000000000, 0.9659258262890683122, 1.000000000000000000, 0.9659258262890683122, 1.000000000000000000, 0.9659258262890683122, 1.000000000000000000, 0.9659258262890683122, 1.000000000000000000, 0.9659258262890683122, 1.000000000000000000, 0.9659258262890683122, 1.000000000000000000, 0.9659258262890683122, 1.000000000000000000, 0.9659258262890683122, 1.000000000000000000, 0.9659258262890683122, 1.000000000000000000, 0.9659258262890683122, 1.000000000000000000, 0.9659258262890683122, 1.000000000000000000, 0.9659258262890683122, 1.000000000000000000, 0.9659258262890683122, 1.000000000000000000, 0.9659258262890683122, 1.000000000000000000, 0.9659258262890683122, 1.000000000000000000, 0.9659258262890683122, 1.000000000000000000, 0.9659258262890683122, 1.000000000000000000, 0.9659258262890683122, 1.000000000000000000, 0.9659258262890683122, 1.000000000000000000, 0.9659258262890683122, 1.000000000000000000, 0.9659258262890683122, 1.000000000000000000, 0.9659258262890683122, 1.000000000000000000, 0.9659258262890683122, 1.000000000000000000, 0.9659258262890683122, 1.000000000000000000, 0.9659258262890683122, 1.000000000000000000, 0.9659258262890683122, 1.000000000000000000, 0.9659258262890683122, 1.000000000000000000, 0.9659258262890683122, 1.000000000000000000, 0.9659258262890683122, 1.000000000000000000, 0.9659258262890683122, 1.000000000000000000, 0.9659258262890683122, 1.000000000000000000, 0.9659258262890683122, 1.000000000000000000, 0.9659258262890683122, 1.000000000000000000, 0.9659258262890683122, 1.000000000000000000, 0.9659258262890683122, 1.000000000000000000, 0.9659258262890683122, 1.000000000000000000, 0.9659258262890683122, 1.000000000000000000, 0.9659258262890683122, 1.000000000000000000, 0.9659258262890683122, 1.000000000000000000, 0.9659258262890683122, 1.000000000000000000, 0.9659258262890683122, 1.000000000000000000, 0.9659258262890683122, 1.000000000000000000, 0.9659258262890683122, 1.000000000000000000, 0.9659258262890683122, 1.000000000000000000, 0.9659258262890683122, 1.000000000000000000, 0.9659258262890683122, 1.000000000000000000, 0.9659258262890683122, 1.000000000000000000, 0.9659258262890683122, 1.000000000000000000, 0.9659258262890683122, 1.000000000000000000, 0.9659258262890683122, 1.000000000000000000, 0.9659258262890683122, 1.000000000000000000, 0.9659258262890683122, 1.000000000000000000, 0.9659258262890683122, 1.000000000000000000, 0.9659258262890683122, 1.000000000000000000, 0.9659258262890683122, 1.000000000000000000, 0.9659258262890683122, 1.000000000000000000, 0.9659258262890683122, 1.000000000000000000, 0.9659258262890683122, 1.000000000000000000, 0.9659258262890683122, 1.000000000000000000, 0.9659258262890683122, 1.000000000000000000, 0.9659258262890683122, 1.000000000000000000, 0.9659258262890683122, 1.000000000000000000, 0.9659258262890683122, 1.000000000000000000, 0.9659258262890683122, 1.000000000000000000, 0.9659258262890683122, 1.000000000000000000, 0.9659258262890683122, 1.000000000000000000, 0.9659258262890683122, 1.000000000000000000, 0.9659258262890683122, 1.000000000000000000, 0.9659258262890683122, 1.000000000000000000, 0.9659258262890683122, 1.000000000000000000, 0.9659258262890683122, 1.000000000000000000, 0.9659258262890683122, 1.000000000000000000, 0.9659258262890683122, 1.000000000000000000, 0.9659258262890683122, 1.000000000000000000, 0.9659258262890683122, 1.000000000000000000, 0.9659258262890683122, 1.000000000000000000, 0.9659258262890683122, 1.000000000000000000, 0.9659258262890683122, 1.000000000000000000, 0.9659258262890683122, 1.000000000000000000, 0.9659258262890683122, 1.000000000000000000, 0.9659258262890683122, 1.000000000000000000, 0.9659258262890683122, 1.000000000000000000, 0.9659258262890683122, 1.000000000000000000, 0.9659258262890683122, 1.000000000000000000, 0.9659258262890683122, 1.000000000000000000, 0.9659258262890683122, 1.000000000000000000, 0.9659258262890683122, 1.000000000000000000, 0.9659258262890683122, 1.000000000000000000, 0.9659258262890683122, 1.000000000000000000, 0.9659258262890683122, 1.000000000000000000, 0.9659258262890683122, 1.000000000000000000, 0.9659258262890683122, 1.000000000000000000, 0.9659258262890683122, 1.000000000000000000),
 ( 0.3333333333333333703, 0.3219752754296894559, 0.3333333333333333703, 0.3219752754296894559, 0.3333333333333333703, 0.3219752754296894559, 0.3333333333333333703, 0.3219752754296894559, 0.3333333333333333703, 0.3219752754296894559, 0.3333333333333333703, 0.3219752754296894559, 0.3333333333333333703, 0.3219752754296894559, 0.3333333333333333703, 0.3219752754296894559, 0.3333333333333333703, 0.3219752754296894559, 0.3333333333333333703, 0.3219752754296894559, 0.3333333333333333703, 0.3219752754296894559, 0.3333333333333333703, 0.3219752754296894559, 0.3333333333333333703, 0.3219752754296894559, 0.3333333333333333703, 0.3219752754296894559, 0.3333333333333333703, 0.3219752754296894559, 0.3333333333333333703, 0.3219752754296894559, 0.3333333333333333703, 0.3219752754296894559, 0.3333333333333333703, 0.3219752754296894559, 0.3333333333333333703, 0.3219752754296894559, 0.3333333333333333703, 0.3219752754296894559, 0.3333333333333333703, 0.3219752754296894559, 0.3333333333333333703, 0.3219752754296894559, 0.3333333333333333703, 0.3219752754296894559, 0.3333333333333333703, 0.3219752754296894559, 0.3333333333333333703, 0.3219752754296894559, 0.3333333333333333703, 0.3219752754296894559, 0.3333333333333333703, 0.3219752754296894559, 0.3333333333333333703, 0.3219752754296894559, 0.3333333333333333703, 0.3219752754296894559, 0.3333333333333333703, 0.3219752754296894559, 0.3333333333333333703, 0.3219752754296894559, 0.3333333333333333703, 0.3219752754296894559, 0.3333333333333333703, 0.3219752754296894559, 0.3333333333333333703, 0.3219752754296894559, 0.3333333333333333703, 0.3219752754296894559, 0.3333333333333333703, 0.3219752754296894559, 0.3333333333333333703, 0.3219752754296894559, 0.3333333333333333703, 0.3219752754296894559, 0.3333333333333333703, 0.3219752754296894559, 0.3333333333333333703, 0.3219752754296894559, 0.3333333333333333703, 0.3219752754296894559, 0.3333333333333333703, 0.3219752754296894559, 0.3333333333333333703, 0.3219752754296894559, 0.3333333333333333703, 0.3219752754296894559, 0.3333333333333333703, 0.3219752754296894559, 0.3333333333333333703, 0.3219752754296894559, 0.3333333333333333703, 0.3219752754296894559, 0.3333333333333333703, 0.3219752754296894559, 0.3333333333333333703, 0.3219752754296894559, 0.3333333333333333703, 0.3219752754296894559, 0.3333333333333333703, 0.3219752754296894559, 0.3333333333333333703, 0.3219752754296894559, 0.3333333333333333703, 0.3219752754296894559, 0.3333333333333333703, 0.3219752754296894559, 0.3333333333333333703, 0.3219752754296894559, 0.3333333333333333703, 0.3219752754296894559, 0.3333333333333333703, 0.3219752754296894559, 0.3333333333333333703, 0.3219752754296894559, 0.3333333333333333703, 0.3219752754296894559, 0.3333333333333333703, 0.3219752754296894559, 0.3333333333333333703, 0.3219752754296894559, 0.3333333333333333703, 0.3219752754296894559, 0.3333333333333333703, 0.3219752754296894559, 0.3333333333333333703, 0.3219752754296894559, 0.3333333333333333703, 0.3219752754296894559, 0.3333333333333333703, 0.3219752754296894559, 0.3333333333333333703, 0.3219752754296894559, 0.3333333333333333703, 0.3219752754296894559, 0.3333333333333333703, 0.3219752754296894559, 0.3333333333333333703, 0.3219752754296894559, 0.3333333333333333703, 0.3219752754296894559, 0.3333333333333333703, 0.3219752754296894559, 0.3333333333333333703, 0.3219752754296894559, 0.3333333333333333703, 0.3219752754296894559, 0.3333333333333333703, 0.3219752754296894559, 0.3333333333333333703, 0.3219752754296894559, 0.3333333333333333703, 0.3219752754296894559, 0.3333333333333333703, 0.3219752754296894559, 0.3333333333333333703, 0.3219752754296894559, 0.3333333333333333703, 0.3219752754296894559, 0.3333333333333333703, 0.3219752754296894559, 0.3333333333333333703, 0.3219752754296894559, 0.3333333333333333703, 0.3219752754296894559, 0.3333333333333333703, 0.3219752754296894559, 0.3333333333333333703, 0.3219752754296894559, 0.3333333333333333703, 0.3219752754296894559, 0.3333333333333333703, 0.3219752754296894559, 0.3333333333333333703, 0.3219752754296894559, 0.3333333333333333703, 0.3219752754296894559, 0.3333333333333333703, 0.3219752754296894559, 0.3333333333333333703, 0.3219752754296894559, 0.3333333333333333703, 0.3219752754296894559, 0.3333333333333333703, 0.3219752754296894559, 0.3333333333333333703, 0.3219752754296894559, 0.3333333333333333703, 0.3219752754296894559, 0.3333333333333333703, 0.3219752754296894559, 0.3333333333333333703, 0.3219752754296894559, 0.3333333333333333703, 0.3219752754296894559, 0.3333333333333333703, 0.3219752754296894559, 0.3333333333333333703, 0.3219752754296894559, 0.3333333333333333703, 0.3219752754296894559, 0.3333333333333333703, 0.3219752754296894559, 0.3333333333333333703, 0.3219752754296894559, 0.3333333333333333703, 0.3219752754296894559, 0.3333333333333333703, 0.3219752754296894559, 0.3333333333333333703, 0.3219752754296894559, 0.3333333333333333703, 0.3219752754296894559, 0.3333333333333333703, 0.3219752754296894559, 0.3333333333333333703, 0.3219752754296894559, 0.3333333333333333703, 0.3219752754296894559, 0.3333333333333333703, 0.3219752754296894559, 0.3333333333333333703, 0.3219752754296894559, 0.3333333333333333703, 0.3219752754296894559, 0.3333333333333333703, 0.3219752754296894559, 0.3333333333333333703, 0.3219752754296894559, 0.3333333333333333703, 0.3219752754296894559, 0.3333333333333333703, 0.3219752754296894559, 0.3333333333333333703, 0.3219752754296894559, 0.3333333333333333703, 0.3219752754296894559, 0.3333333333333333703, 0.3219752754296894559, 0.3333333333333333703, 0.3219752754296894559, 0.3333333333333333703, 0.3219752754296894559, 0.3333333333333333703, 0.3219752754296894559, 0.3333333333333333703, 0.3219752754296894559, 0.3333333333333333703, 0.3219752754296894559, 0.3333333333333333703, 0.3219752754296894559, 0.3333333333333333703, 0.3219752754296894559, 0.3333333333333333703, 0.3219752754296894559, 0.3333333333333333703, 0.3219752754296894559, 0.3333333333333333703, 0.3219752754296894559, 0.3333333333333333703, 0.3219752754296894559, 0.3333333333333333703, 0.3219752754296894559, 0.3333333333333333703, 0.3219752754296894559, 0.3333333333333333703, 0.3219752754296894559, 0.3333333333333333703, 0.3219752754296894559, 0.3333333333333333703, 0.3219752754296894559, 0.3333333333333333703, 0.3219752754296894559, 0.3333333333333333703, 0.3219752754296894559, 0.3333333333333333703, 0.3219752754296894559, 0.3333333333333333703, 0.3219752754296894559, 0.3333333333333333703, 0.3219752754296894559, 0.3333333333333333703, 0.3219752754296894559, 0.3333333333333333703, 0.3219752754296894559, 0.3333333333333333703, 0.3219752754296894559, 0.3333333333333333703, 0.3219752754296894559, 0.3333333333333333703, 0.3219752754296894559, 0.3333333333333333703, 0.3219752754296894559, 0.3333333333333333703, 0.3219752754296894559, 0.3333333333333333703, 0.3219752754296894559, 0.3333333333333333703, 0.3219752754296894559, 0.3333333333333333703, 0.3219752754296894559, 0.3333333333333333703, 0.3219752754296894559, 0.3333333333333333703, 0.3219752754296894559, 0.3333333333333333703, 0.3219752754296894559, 0.3333333333333333703, 0.3219752754296894559, 0.3333333333333333703, 0.3219752754296894559, 0.3333333333333333703, 0.3219752754296894559, 0.3333333333333333703, 0.3219752754296894559, 0.3333333333333333703, 0.3219752754296894559, 0.3333333333333333703, 0.3219752754296894559, 0.3333333333333333703, 0.3219752754296894559, 0.3333333333333333703, 0.3219752754296894559, 0.3333333333333333703, 0.3219752754296894559, 0.3333333333333333703, 0.3219752754296894559, 0.3333333333333333703, 0.3219752754296894559, 0.3333333333333333703, 0.3219752754296894559, 0.3333333333333333703, 0.3219752754296894559, 0.3333333333333333703, 0.3219752754296894559, 0.3333333333333333703, 0.3219752754296894559, 0.3333333333333333703, 0.3219752754296894559, 0.3333333333333333703, 0.3219752754296894559, 0.3333333333333333703, 0.3219752754296894559, 0.3333333333333333703, 0.3219752754296894559, 0.3333333333333333703, 0.3219752754296894559, 0.3333333333333333703, 0.3219752754296894559, 0.3333333333333333703, 0.3219752754296894559, 0.3333333333333333703, 0.3219752754296894559, 0.3333333333333333703, 0.3219752754296894559, 0.3333333333333333703, 0.3219752754296894559, 0.3333333333333333703, 0.3219752754296894559, 0.3333333333333333703, 0.3219752754296894559, 0.3333333333333333703, 0.3219752754296894559, 0.3333333333333333703, 0.3219752754296894559, 0.3333333333333333703, 0.3219752754296894559, 0.3333333333333333703, 0.3219752754296894559, 0.3333333333333333703, 0.3219752754296894559, 0.3333333333333333703, 0.3219752754296894559, 0.3333333333333333703, 0.3219752754296894559, 0.3333333333333333703, 0.3219752754296894559, 0.3333333333333333703, 0.3219752754296894559, 0.3333333333333333703, 0.3219752754296894559, 0.3333333333333333703, 0.3219752754296894559, 0.3333333333333333703, 0.3219752754296894559, 0.3333333333333333703, 0.3219752754296894559, 0.3333333333333333703, 0.3219752754296894559, 0.3333333333333333703, 0.3219752754296894559, 0.3333333333333333703, 0.3219752754296894559, 0.3333333333333333703, 0.3219752754296894559, 0.3333333333333333703, 0.3219752754296894559, 0.3333333333333333703, 0.3219752754296894559, 0.3333333333333333703, 0.3219752754296894559, 0.3333333333333333703, 0.3219752754296894559, 0.3333333333333333703, 0.3219752754296894559, 0.3333333333333333703, 0.3219752754296894559, 0.3333333333333333703, 0.3219752754296894559, 0.3333333333333333703, 0.3219752754296894559, 0.3333333333333333703, 0.3219752754296894559, 0.3333333333333333703, 0.3219752754296894559, 0.3333333333333333703, 0.3219752754296894559, 0.3333333333333333703, 0.3219752754296894559, 0.3333333333333333703, 0.3219752754296894559, 0.3333333333333333703, 0.3219752754296894559, 0.3333333333333333703, 0.3219752754296894559, 0.3333333333333333703, 0.3219752754296894559, 0.3333333333333333703, 0.3219752754296894559, 0.3333333333333333703, 0.3219752754296894559, 0.3333333333333333703, 0.3219752754296894559, 0.3333333333333333703, 0.3219752754296894559, 0.3333333333333333703, 0.3219752754296894559, 0.3333333333333333703, 0.3219752754296894559, 0.3333333333333333703, 0.3219752754296894559, 0.3333333333333333703, 0.3219752754296894559, 0.3333333333333333703, 0.3219752754296894559, 0.3333333333333333703, 0.3219752754296894559, 0.3333333333333333703, 0.3219752754296894559, 0.3333333333333333703, 0.3219752754296894559, 0.3333333333333333703, 0.3219752754296894559, 0.3333333333333333703, 0.3219752754296894559, 0.3333333333333333703),
 ( 0.3333333333333333703, 0.3219752754296894559, 0.3333333333333333703, 0.3219752754296894559, 0.3333333333333333703, 0.3219752754296894559, 0.3333333333333333703, 0.3219752754296894559, 0.3333333333333333703, 0.3219752754296894559, 0.3333333333333333703, 0.3219752754296894559, 0.3333333333333333703, 0.3219752754296894559, 0.3333333333333333703, 0.3219752754296894559, 0.3333333333333333703, 0.3219752754296894559, 0.3333333333333333703, 0.3219752754296894559, 0.3333333333333333703, 0.3219752754296894559, 0.3333333333333333703, 0.3219752754296894559, 0.3333333333333333703, 0.3219752754296894559, 0.3333333333333333703, 0.3219752754296894559, 0.3333333333333333703, 0.3219752754296894559, 0.3333333333333333703, 0.3219752754296894559, 0.3333333333333333703, 0.3219752754296894559, 0.3333333333333333703, 0.3219752754296894559, 0.3333333333333333703, 0.3219752754296894559, 0.3333333333333333703, 0.3219752754296894559, 0.3333333333333333703, 0.3219752754296894559, 0.3333333333333333703, 0.3219752754296894559, 0.3333333333333333703, 0.3219752754296894559, 0.3333333333333333703, 0.3219752754296894559, 0.3333333333333333703, 0.3219752754296894559, 0.3333333333333333703, 0.3219752754296894559, 0.3333333333333333703, 0.3219752754296894559, 0.3333333333333333703, 0.3219752754296894559, 0.3333333333333333703, 0.3219752754296894559, 0.3333333333333333703, 0.3219752754296894559, 0.3333333333333333703, 0.3219752754296894559, 0.3333333333333333703, 0.3219752754296894559, 0.3333333333333333703, 0.3219752754296894559, 0.3333333333333333703, 0.3219752754296894559, 0.3333333333333333703, 0.3219752754296894559, 0.3333333333333333703, 0.3219752754296894559, 0.3333333333333333703, 0.3219752754296894559, 0.3333333333333333703, 0.3219752754296894559, 0.3333333333333333703, 0.3219752754296894559, 0.3333333333333333703, 0.3219752754296894559, 0.3333333333333333703, 0.3219752754296894559, 0.3333333333333333703, 0.3219752754296894559, 0.3333333333333333703, 0.3219752754296894559, 0.3333333333333333703, 0.3219752754296894559, 0.3333333333333333703, 0.3219752754296894559, 0.3333333333333333703, 0.3219752754296894559, 0.3333333333333333703, 0.3219752754296894559, 0.3333333333333333703, 0.3219752754296894559, 0.3333333333333333703, 0.3219752754296894559, 0.3333333333333333703, 0.3219752754296894559, 0.3333333333333333703, 0.3219752754296894559, 0.3333333333333333703, 0.3219752754296894559, 0.3333333333333333703, 0.3219752754296894559, 0.3333333333333333703, 0.3219752754296894559, 0.3333333333333333703, 0.3219752754296894559, 0.3333333333333333703, 0.3219752754296894559, 0.3333333333333333703, 0.3219752754296894559, 0.3333333333333333703, 0.3219752754296894559, 0.3333333333333333703, 0.3219752754296894559, 0.3333333333333333703, 0.3219752754296894559, 0.3333333333333333703, 0.3219752754296894559, 0.3333333333333333703, 0.3219752754296894559, 0.3333333333333333703, 0.3219752754296894559, 0.3333333333333333703, 0.3219752754296894559, 0.3333333333333333703, 0.3219752754296894559, 0.3333333333333333703, 0.3219752754296894559, 0.3333333333333333703, 0.3219752754296894559, 0.3333333333333333703, 0.3219752754296894559, 0.3333333333333333703, 0.3219752754296894559, 0.3333333333333333703, 0.3219752754296894559, 0.3333333333333333703, 0.3219752754296894559, 0.3333333333333333703, 0.3219752754296894559, 0.3333333333333333703, 0.3219752754296894559, 0.3333333333333333703, 0.3219752754296894559, 0.3333333333333333703, 0.3219752754296894559, 0.3333333333333333703, 0.3219752754296894559, 0.3333333333333333703, 0.3219752754296894559, 0.3333333333333333703, 0.3219752754296894559, 0.3333333333333333703, 0.3219752754296894559, 0.3333333333333333703, 0.3219752754296894559, 0.3333333333333333703, 0.3219752754296894559, 0.3333333333333333703, 0.3219752754296894559, 0.3333333333333333703, 0.3219752754296894559, 0.3333333333333333703, 0.3219752754296894559, 0.3333333333333333703, 0.3219752754296894559, 0.3333333333333333703, 0.3219752754296894559, 0.3333333333333333703, 0.3219752754296894559, 0.3333333333333333703, 0.3219752754296894559, 0.3333333333333333703, 0.3219752754296894559, 0.3333333333333333703, 0.3219752754296894559, 0.3333333333333333703, 0.3219752754296894559, 0.3333333333333333703, 0.3219752754296894559, 0.3333333333333333703, 0.3219752754296894559, 0.3333333333333333703, 0.3219752754296894559, 0.3333333333333333703, 0.3219752754296894559, 0.3333333333333333703, 0.3219752754296894559, 0.3333333333333333703, 0.3219752754296894559, 0.3333333333333333703, 0.3219752754296894559, 0.3333333333333333703, 0.3219752754296894559, 0.3333333333333333703, 0.3219752754296894559, 0.3333333333333333703, 0.3219752754296894559, 0.3333333333333333703, 0.3219752754296894559, 0.3333333333333333703, 0.3219752754296894559, 0.3333333333333333703, 0.3219752754296894559, 0.3333333333333333703, 0.3219752754296894559, 0.3333333333333333703, 0.3219752754296894559, 0.3333333333333333703, 0.3219752754296894559, 0.3333333333333333703, 0.3219752754296894559, 0.3333333333333333703, 0.3219752754296894559, 0.3333333333333333703, 0.3219752754296894559, 0.3333333333333333703, 0.3219752754296894559, 0.3333333333333333703, 0.3219752754296894559, 0.3333333333333333703, 0.3219752754296894559, 0.3333333333333333703, 0.3219752754296894559, 0.3333333333333333703, 0.3219752754296894559, 0.3333333333333333703, 0.3219752754296894559, 0.3333333333333333703, 0.3219752754296894559, 0.3333333333333333703, 0.3219752754296894559, 0.3333333333333333703, 0.3219752754296894559, 0.3333333333333333703, 0.3219752754296894559, 0.3333333333333333703, 0.3219752754296894559, 0.3333333333333333703, 0.3219752754296894559, 0.3333333333333333703, 0.3219752754296894559, 0.3333333333333333703, 0.3219752754296894559, 0.3333333333333333703, 0.3219752754296894559, 0.3333333333333333703, 0.3219752754296894559, 0.3333333333333333703, 0.3219752754296894559, 0.3333333333333333703, 0.3219752754296894559, 0.3333333333333333703, 0.3219752754296894559, 0.3333333333333333703, 0.3219752754296894559, 0.3333333333333333703, 0.3219752754296894559, 0.3333333333333333703, 0.3219752754296894559, 0.3333333333333333703, 0.3219752754296894559, 0.3333333333333333703, 0.3219752754296894559, 0.3333333333333333703, 0.3219752754296894559, 0.3333333333333333703, 0.3219752754296894559, 0.3333333333333333703, 0.3219752754296894559, 0.3333333333333333703, 0.3219752754296894559, 0.3333333333333333703, 0.3219752754296894559, 0.3333333333333333703, 0.3219752754296894559, 0.3333333333333333703, 0.3219752754296894559, 0.3333333333333333703, 0.3219752754296894559, 0.3333333333333333703, 0.3219752754296894559, 0.3333333333333333703, 0.3219752754296894559, 0.3333333333333333703, 0.3219752754296894559, 0.3333333333333333703, 0.3219752754296894559, 0.3333333333333333703, 0.3219752754296894559, 0.3333333333333333703, 0.3219752754296894559, 0.3333333333333333703, 0.3219752754296894559, 0.3333333333333333703, 0.3219752754296894559, 0.3333333333333333703, 0.3219752754296894559, 0.3333333333333333703, 0.3219752754296894559, 0.3333333333333333703, 0.3219752754296894559, 0.3333333333333333703, 0.3219752754296894559, 0.3333333333333333703, 0.3219752754296894559, 0.3333333333333333703, 0.3219752754296894559, 0.3333333333333333703, 0.3219752754296894559, 0.3333333333333333703, 0.3219752754296894559, 0.3333333333333333703, 0.3219752754296894559, 0.3333333333333333703, 0.3219752754296894559, 0.3333333333333333703, 0.3219752754296894559, 0.3333333333333333703, 0.3219752754296894559, 0.3333333333333333703, 0.3219752754296894559, 0.3333333333333333703, 0.3219752754296894559, 0.3333333333333333703, 0.3219752754296894559, 0.3333333333333333703, 0.3219752754296894559, 0.3333333333333333703, 0.3219752754296894559, 0.3333333333333333703, 0.3219752754296894559, 0.3333333333333333703, 0.3219752754296894559, 0.3333333333333333703, 0.3219752754296894559, 0.3333333333333333703, 0.3219752754296894559, 0.3333333333333333703, 0.3219752754296894559, 0.3333333333333333703, 0.3219752754296894559, 0.3333333333333333703, 0.3219752754296894559, 0.3333333333333333703, 0.3219752754296894559, 0.3333333333333333703, 0.3219752754296894559, 0.3333333333333333703, 0.3219752754296894559, 0.3333333333333333703, 0.3219752754296894559, 0.3333333333333333703, 0.3219752754296894559, 0.3333333333333333703, 0.3219752754296894559, 0.3333333333333333703, 0.3219752754296894559, 0.3333333333333333703, 0.3219752754296894559, 0.3333333333333333703, 0.3219752754296894559, 0.3333333333333333703, 0.3219752754296894559, 0.3333333333333333703, 0.3219752754296894559, 0.3333333333333333703, 0.3219752754296894559, 0.3333333333333333703, 0.3219752754296894559, 0.3333333333333333703, 0.3219752754296894559, 0.3333333333333333703, 0.3219752754296894559, 0.3333333333333333703, 0.3219752754296894559, 0.3333333333333333703, 0.3219752754296894559, 0.3333333333333333703, 0.3219752754296894559, 0.3333333333333333703, 0.3219752754296894559, 0.3333333333333333703, 0.3219752754296894559, 0.3333333333333333703, 0.3219752754296894559, 0.3333333333333333703, 0.3219752754296894559, 0.3333333333333333703, 0.3219752754296894559, 0.3333333333333333703, 0.3219752754296894559, 0.3333333333333333703, 0.3219752754296894559, 0.3333333333333333703, 0.3219752754296894559, 0.3333333333333333703, 0.3219752754296894559, 0.3333333333333333703, 0.3219752754296894559, 0.3333333333333333703, 0.3219752754296894559, 0.3333333333333333703, 0.3219752754296894559, 0.3333333333333333703, 0.3219752754296894559, 0.3333333333333333703, 0.3219752754296894559, 0.3333333333333333703, 0.3219752754296894559, 0.3333333333333333703, 0.3219752754296894559, 0.3333333333333333703, 0.3219752754296894559, 0.3333333333333333703, 0.3219752754296894559, 0.3333333333333333703, 0.3219752754296894559, 0.3333333333333333703, 0.3219752754296894559, 0.3333333333333333703, 0.3219752754296894559, 0.3333333333333333703, 0.3219752754296894559, 0.3333333333333333703, 0.3219752754296894559, 0.3333333333333333703, 0.3219752754296894559, 0.3333333333333333703, 0.3219752754296894559, 0.3333333333333333703, 0.3219752754296894559, 0.3333333333333333703, 0.3219752754296894559, 0.3333333333333333703, 0.3219752754296894559, 0.3333333333333333703, 0.3219752754296894559, 0.3333333333333333703, 0.3219752754296894559, 0.3333333333333333703, 0.3219752754296894559, 0.3333333333333333703, 0.3219752754296894559, 0.3333333333333333703, 0.3219752754296894559, 0.3333333333333333703, 0.3219752754296894559, 0.3333333333333333703, 0.3219752754296894559, 0.3333333333333333703, 0.3219752754296894559, 0.3333333333333333703),
 ( 1.000000000000000000, 0.9659258262890683122, 1.000000000000000000, 0.9659258262890683122, 1.000000000000000000, 0.9659258262890683122, 1.000000000000000000, 0.9659258262890683122, 1.000000000000000000, 0.9659258262890683122, 1.000000000000000000, 0.9659258262890683122, 1.000000000000000000, 0.9659258262890683122, 1.000000000000000000, 0.9659258262890683122, 1.000000000000000000, 0.9659258262890683122, 1.000000000000000000, 0.9659258262890683122, 1.000000000000000000, 0.9659258262890683122, 1.000000000000000000, 0.9659258262890683122, 1.000000000000000000, 0.9659258262890683122, 1.000000000000000000, 0.9659258262890683122, 1.000000000000000000, 0.9659258262890683122, 1.000000000000000000, 0.9659258262890683122, 1.000000000000000000, 0.9659258262890683122, 1.000000000000000000, 0.9659258262890683122, 1.000000000000000000, 0.9659258262890683122, 1.000000000000000000, 0.9659258262890683122, 1.000000000000000000, 0.9659258262890683122, 1.000000000000000000, 0.9659258262890683122, 1.000000000000000000, 0.9659258262890683122, 1.000000000000000000, 0.9659258262890683122, 1.000000000000000000, 0.9659258262890683122, 1.000000000000000000, 0.9659258262890683122, 1.000000000000000000, 0.9659258262890683122, 1.000000000000000000, 0.9659258262890683122, 1.000000000000000000, 0.9659258262890683122, 1.000000000000000000, 0.9659258262890683122, 1.000000000000000000, 0.9659258262890683122, 1.000000000000000000, 0.9659258262890683122, 1.000000000000000000, 0.9659258262890683122, 1.000000000000000000, 0.9659258262890683122, 1.000000000000000000, 0.9659258262890683122, 1.000000000000000000, 0.9659258262890683122, 1.000000000000000000, 0.9659258262890683122, 1.000000000000000000, 0.9659258262890683122, 1.000000000000000000, 0.9659258262890683122, 1.000000000000000000, 0.9659258262890683122, 1.000000000000000000, 0.9659258262890683122, 1.000000000000000000, 0.9659258262890683122, 1.000000000000000000, 0.9659258262890683122, 1.000000000000000000, 0.9659258262890683122, 1.000000000000000000, 0.9659258262890683122, 1.000000000000000000, 0.9659258262890683122, 1.000000000000000000, 0.9659258262890683122, 1.000000000000000000, 0.9659258262890683122, 1.000000000000000000, 0.9659258262890683122, 1.000000000000000000, 0.9659258262890683122, 1.000000000000000000, 0.9659258262890683122, 1.000000000000000000, 0.9659258262890683122, 1.000000000000000000, 0.9659258262890683122, 1.000000000000000000, 0.9659258262890683122, 1.000000000000000000, 0.9659258262890683122, 1.000000000000000000, 0.9659258262890683122, 1.000000000000000000, 0.9659258262890683122, 1.000000000000000000, 0.9659258262890683122, 1.000000000000000000, 0.9659258262890683122, 1.000000000000000000, 0.9659258262890683122, 1.000000000000000000, 0.9659258262890683122, 1.000000000000000000, 0.9659258262890683122, 1.000000000000000000, 0.9659258262890683122, 1.000000000000000000, 0.9659258262890683122, 1.000000000000000000, 0.9659258262890683122, 1.000000000000000000, 0.9659258262890683122, 1.000000000000000000, 0.9659258262890683122, 1.000000000000000000, 0.9659258262890683122, 1.000000000000000000, 0.9659258262890683122, 1.000000000000000000, 0.9659258262890683122, 1.000000000000000000, 0.9659258262890683122, 1.000000000000000000, 0.9659258262890683122, 1.000000000000000000, 0.9659258262890683122, 1.000000000000000000, 0.9659258262890683122, 1.000000000000000000, 0.9659258262890683122, 1.000000000000000000, 0.9659258262890683122, 1.000000000000000000, 0.9659258262890683122, 1.000000000000000000, 0.9659258262890683122, 1.000000000000000000, 0.9659258262890683122, 1.000000000000000000, 0.9659258262890683122, 1.000000000000000000, 0.9659258262890683122, 1.000000000000000000, 0.9659258262890683122, 1.000000000000000000, 0.9659258262890683122, 1.000000000000000000, 0.9659258262890683122, 1.000000000000000000, 0.9659258262890683122, 1.000000000000000000, 0.9659258262890683122, 1.000000000000000000, 0.9659258262890683122, 1.000000000000000000, 0.9659258262890683122, 1.000000000000000000, 0.9659258262890683122, 1.000000000000000000, 0.9659258262890683122, 1.000000000000000000, 0.9659258262890683122, 1.000000000000000000, 0.9659258262890683122, 1.000000000000000000, 0.9659258262890683122, 1.000000000000000000, 0.9659258262890683122, 1.000000000000000000, 0.9659258262890683122, 1.000000000000000000, 0.9659258262890683122, 1.000000000000000000, 0.9659258262890683122, 1.000000000000000000, 0.9659258262890683122, 1.000000000000000000, 0.9659258262890683122, 1.000000000000000000, 0.9659258262890683122, 1.000000000000000000, 0.9659258262890683122, 1.000000000000000000, 0.9659258262890683122, 1.000000000000000000, 0.9659258262890683122, 1.000000000000000000, 0.9659258262890683122, 1.000000000000000000, 0.9659258262890683122, 1.000000000000000000, 0.9659258262890683122, 1.000000000000000000, 0.9659258262890683122, 1.000000000000000000, 0.9659258262890683122, 1.000000000000000000, 0.9659258262890683122, 1.000000000000000000, 0.9659258262890683122, 1.000000000000000000, 0.9659258262890683122, 1.000000000000000000, 0.9659258262890683122, 1.000000000000000000, 0.9659258262890683122, 1.000000000000000000, 0.9659258262890683122, 1.000000000000000000, 0.9659258262890683122, 1.000000000000000000, 0.9659258262890683122, 1.000000000000000000, 0.9659258262890683122, 1.000000000000000000, 0.9659258262890683122, 1.000000000000000000, 0.9659258262890683122, 1.000000000000000000, 0.9659258262890683122, 1.000000000000000000, 0.9659258262890683122, 1.000000000000000000, 0.9659258262890683122, 1.000000000000000000, 0.9659258262890683122, 1.000000000000000000, 0.9659258262890683122, 1.000000000000000000, 0.9659258262890683122, 1.000000000000000000, 0.9659258262890683122, 1.000000000000000000, 0.9659258262890683122, 1.000000000000000000, 0.9659258262890683122, 1.000000000000000000, 0.9659258262890683122, 1.000000000000000000, 0.9659258262890683122, 1.000000000000000000, 0.9659258262890683122, 1.000000000000000000, 0.9659258262890683122, 1.000000000000000000, 0.9659258262890683122, 1.000000000000000000, 0.9659258262890683122, 1.000000000000000000, 0.9659258262890683122, 1.000000000000000000, 0.9659258262890683122, 1.000000000000000000, 0.9659258262890683122, 1.000000000000000000, 0.9659258262890683122, 1.000000000000000000, 0.9659258262890683122, 1.000000000000000000, 0.9659258262890683122, 1.000000000000000000, 0.9659258262890683122, 1.000000000000000000, 0.9659258262890683122, 1.000000000000000000, 0.9659258262890683122, 1.000000000000000000, 0.9659258262890683122, 1.000000000000000000, 0.9659258262890683122, 1.000000000000000000, 0.9659258262890683122, 1.000000000000000000, 0.9659258262890683122, 1.000000000000000000, 0.9659258262890683122, 1.000000000000000000, 0.9659258262890683122, 1.000000000000000000, 0.9659258262890683122, 1.000000000000000000, 0.9659258262890683122, 1.000000000000000000, 0.9659258262890683122, 1.000000000000000000, 0.9659258262890683122, 1.000000000000000000, 0.9659258262890683122, 1.000000000000000000, 0.9659258262890683122, 1.000000000000000000, 0.9659258262890683122, 1.000000000000000000, 0.9659258262890683122, 1.000000000000000000, 0.9659258262890683122, 1.000000000000000000, 0.9659258262890683122, 1.000000000000000000, 0.9659258262890683122, 1.000000000000000000, 0.9659258262890683122, 1.000000000000000000, 0.9659258262890683122, 1.000000000000000000, 0.9659258262890683122, 1.000000000000000000, 0.9659258262890683122, 1.000000000000000000, 0.9659258262890683122, 1.000000000000000000, 0.9659258262890683122, 1.000000000000000000, 0.9659258262890683122, 1.000000000000000000, 0.9659258262890683122, 1.000000000000000000, 0.9659258262890683122, 1.000000000000000000, 0.9659258262890683122, 1.000000000000000000, 0.9659258262890683122, 1.000000000000000000, 0.9659258262890683122, 1.000000000000000000, 0.9659258262890683122, 1.000000000000000000, 0.9659258262890683122, 1.000000000000000000, 0.9659258262890683122, 1.000000000000000000, 0.9659258262890683122, 1.000000000000000000, 0.9659258262890683122, 1.000000000000000000, 0.9659258262890683122, 1.000000000000000000, 0.9659258262890683122, 1.000000000000000000, 0.9659258262890683122, 1.000000000000000000, 0.9659258262890683122, 1.000000000000000000, 0.9659258262890683122, 1.000000000000000000, 0.9659258262890683122, 1.000000000000000000, 0.9659258262890683122, 1.000000000000000000, 0.9659258262890683122, 1.000000000000000000, 0.9659258262890683122, 1.000000000000000000, 0.9659258262890683122, 1.000000000000000000, 0.9659258262890683122, 1.000000000000000000, 0.9659258262890683122, 1.000000000000000000, 0.9659258262890683122, 1.000000000000000000, 0.9659258262890683122, 1.000000000000000000, 0.9659258262890683122, 1.000000000000000000, 0.9659258262890683122, 1.000000000000000000, 0.9659258262890683122, 1.000000000000000000, 0.9659258262890683122, 1.000000000000000000, 0.9659258262890683122, 1.000000000000000000, 0.9659258262890683122, 1.000000000000000000, 0.9659258262890683122, 1.000000000000000000, 0.9659258262890683122, 1.000000000000000000, 0.9659258262890683122, 1.000000000000000000, 0.9659258262890683122, 1.000000000000000000, 0.9659258262890683122, 1.000000000000000000, 0.9659258262890683122, 1.000000000000000000, 0.9659258262890683122, 1.000000000000000000, 0.9659258262890683122, 1.000000000000000000, 0.9659258262890683122, 1.000000000000000000, 0.9659258262890683122, 1.000000000000000000, 0.9659258262890683122, 1.000000000000000000, 0.9659258262890683122, 1.000000000000000000, 0.9659258262890683122, 1.000000000000000000, 0.9659258262890683122, 1.000000000000000000, 0.9659258262890683122, 1.000000000000000000, 0.9659258262890683122, 1.000000000000000000, 0.9659258262890683122, 1.000000000000000000, 0.9659258262890683122, 1.000000000000000000, 0.9659258262890683122, 1.000000000000000000, 0.9659258262890683122, 1.000000000000000000, 0.9659258262890683122, 1.000000000000000000, 0.9659258262890683122, 1.000000000000000000, 0.9659258262890683122, 1.000000000000000000, 0.9659258262890683122, 1.000000000000000000, 0.9659258262890683122, 1.000000000000000000, 0.9659258262890683122, 1.000000000000000000, 0.9659258262890683122, 1.000000000000000000, 0.9659258262890683122, 1.000000000000000000, 0.9659258262890683122, 1.000000000000000000, 0.9659258262890683122, 1.000000000000000000, 0.9659258262890683122, 1.000000000000000000) ) ) 
 REPRESENTATION_ITEM ( '' )  SURFACE ( )  );
#55599=CARTESIAN_POINT ( 'NONE',  ( 18.62759615963255655, 10.81492255796105972, 81.66775706135236135 ) ) ;
#55600=CARTESIAN_POINT ( 'NONE',  ( 14.29746914071037800, 8.314922557961029526, 46.66775706135234714 ) ) ;
#55601=CARTESIAN_POINT ( 'NONE',  ( 19.02544592524343514, -5.153800228976328945, 83.54057627198100988 ) ) ;
#55602=CARTESIAN_POINT ( 'NONE',  ( 9.564922557961047289, -16.46253265017146816, 105.4177570613523471 ) ) ;
#55603=CARTESIAN_POINT ( 'NONE',  ( 14.29746914071037800, 8.314922557961029526, 71.66775706135234714 ) ) ;
#55604=CARTESIAN_POINT ( 'NONE',  ( 19.03943276465977164, 0.05219959533936151252, 96.25109039468567573 ) ) ;
#55605=CARTESIAN_POINT ( 'NONE',  ( 19.02544592524343514, -5.153800228976328945, 63.54057627198103830 ) ) ;
#55606=CARTESIAN_POINT ( 'NONE',  ( 21.52544592524344225, -5.823673210054117533, 88.54057627198103830 ) ) ;
#55607=CARTESIAN_POINT ( 'NONE',  ( 8.314922557960818139, 14.29746914071049879, 89.58224293864768129 ) ) ;
#55608=CARTESIAN_POINT ( 'NONE',  ( -5.153800228976607833, 19.02544592524334988, 92.70942372801901854 ) ) ;
#55609=CARTESIAN_POINT ( 'NONE',  ( -12.14591786802326823, 12.06949235617739902, 53.12609039468568284 ) ) ;
#55610=CARTESIAN_POINT ( 'NONE',  ( 17.13100169013303287, -6.664070546373073611, 63.26789835699851494 ) ) ;
#55611=CARTESIAN_POINT ( 'NONE',  ( -16.51473224551082808, 9.474510206698731452, 53.33442372801900433 ) ) ;
#55612=CARTESIAN_POINT ( 'NONE',  ( -4.483927247898539470, -16.52544592524342804, 37.29057627198102409 ) ) ;
#55613=CARTESIAN_POINT ( 'NONE',  ( -16.52544592524342804, 4.483927247898546575, 81.04057627198102409 ) ) ;
#55614=CARTESIAN_POINT ( 'NONE',  ( 5.719274019375673035, 21.55341960407619339, 112.2927570613523471 ) ) ;
#55615=CARTESIAN_POINT ( 'NONE',  ( -17.05587630539706367, 6.762274262136758196, 40.74180309037283365 ) ) ;
#55616=CARTESIAN_POINT ( 'NONE',  ( -0.05219959533937732626, 21.53943276465977519, 22.50109039468567573 ) ) ;
#55617=DIRECTION ( 'NONE',  ( -0.000000000000000000, 1.000000000000000000, 0.000000000000000000 ) ) ;
#55618=CARTESIAN_POINT ( 'NONE',  ( -13.89961937509977652, 13.97604488694528158, 80.62390960531436690 ) ) ;
#55619=CARTESIAN_POINT ( 'NONE',  ( -21.55341960407619339, 5.719274019375674811, 93.54275706135234714 ) ) ;
#55620=CARTESIAN_POINT ( 'NONE',  ( -5.153800228976328057, -19.02544592524343514, 82.29057627198103830 ) ) ;
#55621=CARTESIAN_POINT ( 'NONE',  ( -5.823673210054116645, -21.52544592524344225, 42.29057627198103120 ) ) ;
#55622=CARTESIAN_POINT ( 'NONE',  ( 16.52544592524342804, -4.483927247898539470, 78.54057627198103830 ) ) ;
#55623=CARTESIAN_POINT ( 'NONE',  ( 5.049401038298161559, -19.05341960407611168, 52.70724293864767418 ) ) ;
#55624=CARTESIAN_POINT ( 'NONE',  ( -16.52544592524342804, 4.483927247898546575, 101.0405762719810383 ) ) ;
#55625=CARTESIAN_POINT ( 'NONE',  ( -21.52544592524334988, -5.823673210054445271, 18.95942372801901143 ) ) ;
#55626=CARTESIAN_POINT ( 'NONE',  ( 5.719274019375673035, 21.55341960407619339, 62.29275706135236845 ) ) ;
#55627=CARTESIAN_POINT ( 'NONE',  ( -19.03943276465977164, 0.05219959533909376836, 41.24890960531435269 ) ) ;
#55628=CARTESIAN_POINT ( 'NONE',  ( -12.14591786802326823, 12.06949235617739902, 63.12609039468568994 ) ) ;
#55629=CARTESIAN_POINT ( 'NONE',  ( 10.72451020669898902, -18.67979575497178502, 112.9155762719810383 ) ) ;
#55630=CARTESIAN_POINT ( 'NONE',  ( 10.72451020669898902, -18.67979575497178502, 107.9155762719810241 ) ) ;
#55631=CARTESIAN_POINT ( 'NONE',  ( 16.51473224551083163, -9.474510206698727899, 45.83442372801900433 ) ) ;
#55632=CARTESIAN_POINT ( 'NONE',  ( -13.97604488694527625, -13.89961937509977652, 71.87390960531433848 ) ) ;
#55634=CARTESIAN_POINT ( 'NONE',  ( -18.62759615963255300, -10.81492255796106328, 64.16775706135234714 ) ) ;
#55635=CARTESIAN_POINT ( 'NONE',  ( 10.81492255796078972, 18.62759615963270932, 54.58224293864769550 ) ) ;
#55636=CARTESIAN_POINT ( 'NONE',  ( -16.55341960407611168, -4.379528057220339221, 36.45724293864768839 ) ) ;
#55637=CARTESIAN_POINT ( 'NONE',  ( 21.52544592524334988, 5.823673210054432836, 76.45942372801901854 ) ) ;
#55638=CARTESIAN_POINT ( 'NONE',  ( 10.72451020669871369, 18.67979575497193778, 112.0844237280190185 ) ) ;
#55639=CARTESIAN_POINT ( 'NONE',  ( 12.06949235617757843, -12.14591786802309237, 63.12390960531435979 ) ) ;
#55640=CARTESIAN_POINT ( 'NONE',  ( -16.55341960407611168, -4.379528057220339221, 106.4572429386477097 ) ) ;
#55641=CARTESIAN_POINT ( 'NONE',  ( -5.049401038297874678, -19.05341960407617918, 59.79275706135231871 ) ) ;
#55642=CARTESIAN_POINT ( 'NONE',  ( 14.29746914071037800, 8.314922557961029526, 111.6677570613523613 ) ) ;
#55643=CARTESIAN_POINT ( 'NONE',  ( -21.52544592524334988, -5.823673210054445271, 68.95942372801901854 ) ) ;
#55644=CARTESIAN_POINT ( 'NONE',  ( 0.05219959533909260263, 19.03943276465977164, 54.99890960531435979 ) ) ;
#55645=CARTESIAN_POINT ( 'NONE',  ( -13.97604488694547697, 13.89961937509957934, 38.12609039468566152 ) ) ;
#55646=CARTESIAN_POINT ( 'NONE',  ( -5.823673210054116645, -21.52544592524344225, 37.29057627198102409 ) ) ;
#55647=B_SPLINE_CURVE_WITH_KNOTS ( 'NONE', 3,
 ( #196056, #9025, #71686, #131353, #102023, #176882 ),
 .UNSPECIFIED., .F., .F.,
 ( 4, 2, 4 ),
 ( 0.000000000000000000, 0.0003837532665635129316, 0.0007675065331270258633 ),
 .UNSPECIFIED. ) ;
#55648=CARTESIAN_POINT ( 'NONE',  ( -18.67979575497193778, 10.72451020669871902, 38.33442372801900433 ) ) ;
#55649=CARTESIAN_POINT ( 'NONE',  ( 21.55341960407610458, 5.719274019375980345, 93.95724293864770971 ) ) ;
#55650=CARTESIAN_POINT ( 'NONE',  ( -5.153800228976607833, 19.02544592524334988, 97.70942372801900433 ) ) ;
#55651=CARTESIAN_POINT ( 'NONE',  ( -4.379528057220086978, -16.55341960407618274, 54.79275706135235424 ) ) ;
#55653=CARTESIAN_POINT ( 'NONE',  ( 5.823673210054125526, 21.52544592524343514, 89.79057627198103830 ) ) ;
#55654=CARTESIAN_POINT ( 'NONE',  ( 16.53943276465976808, -0.05219959533910856209, 83.74890960531435269 ) ) ;
#55656=CARTESIAN_POINT ( 'NONE',  ( 4.483927247898790824, -16.52544592524335698, 20.20942372801900788 ) ) ;
#55657=CARTESIAN_POINT ( 'NONE',  ( 21.52544592524344225, -5.823673210054117533, 48.54057627198103120 ) ) ;
#55658=CARTESIAN_POINT ( 'NONE',  ( 4.483927247898790824, -16.52544592524335698, 90.20942372801903275 ) ) ;
#55660=CARTESIAN_POINT ( 'NONE',  ( 12.06949235617739724, 12.14591786802326823, 46.87609039468568994 ) ) ;
#55661=CARTESIAN_POINT ( 'NONE',  ( -5.719274019375665041, -21.55341960407619695, 24.79275706135235779 ) ) ;
#55662=CARTESIAN_POINT ( 'NONE',  ( 15.80617190586746368, 15.72974639402197994, 49.37390960531436690 ) ) ;
#55663=CARTESIAN_POINT ( 'NONE',  ( -12.06949235617739369, -12.14591786802326823, 84.37609039468570415 ) ) ;
#55664=CARTESIAN_POINT ( 'NONE',  ( -9.474510206698964154, 16.51473224551069663, 100.4155762719810241 ) ) ;
#55665=CARTESIAN_POINT ( 'NONE',  ( 21.53943276465977519, 0.05219959533937863772, 56.25109039468568284 ) ) ;
#55666=CARTESIAN_POINT ( 'NONE',  ( 21.53943276465977519, -0.05219959533907433946, 43.74890960531435979 ) ) ;
#55667=CARTESIAN_POINT ( 'NONE',  ( -10.81492255796078084, -18.62759615963271287, 27.08224293864769550 ) ) ;
#55669=CARTESIAN_POINT ( 'NONE',  ( 9.564922557961047289, -16.46253265017146816, 35.41775706135233293 ) ) ;
#55670=CARTESIAN_POINT ( 'NONE',  ( 8.224510206698742110, 14.34966873604972548, 72.08442372801899012 ) ) ;
#55671=CARTESIAN_POINT ( 'NONE',  ( 15.80617190586746368, 15.72974639402197994, 24.37390960531435979 ) ) ;
#55673=CARTESIAN_POINT ( 'NONE',  ( -13.89961937509977652, 13.97604488694528158, 85.62390960531433848 ) ) ;
#55674=CARTESIAN_POINT ( 'NONE',  ( 16.55341960407618274, -4.379528057220086978, 101.0427570613523756 ) ) ;
#55675=CARTESIAN_POINT ( 'NONE',  ( 17.97214573761829826, 5.500000000000077272, 73.96970049038654338 ) ) ;
#55676=CARTESIAN_POINT ( 'NONE',  ( -8.224510206698948167, 14.34966873604960824, 95.41557627198102409 ) ) ;
#55677=CARTESIAN_POINT ( 'NONE',  ( 21.55341960407610458, 5.719274019375980345, 53.95724293864770260 ) ) ;
#55678=CARTESIAN_POINT ( 'NONE',  ( -13.97604488694527625, -13.89961937509977652, 31.87390960531435979 ) ) ;
#55679=CARTESIAN_POINT ( 'NONE',  ( -12.14591786802326823, 12.06949235617739902, 83.12609039468568994 ) ) ;
#55680=CARTESIAN_POINT ( 'NONE',  ( -15.80617190586768217, 15.72974639402176855, 33.12609039468569705 ) ) ;
#55681=CARTESIAN_POINT ( 'NONE',  ( 9.564922557961047289, -16.46253265017146816, 90.41775706135234714 ) ) ;
#55682=CARTESIAN_POINT ( 'NONE',  ( 12.06949235617757843, -12.14591786802309237, 88.12390960531436690 ) ) ;
#55683=CARTESIAN_POINT ( 'NONE',  ( -5.153800228976328057, -19.02544592524343514, 52.29057627198100988 ) ) ;
#55684=CARTESIAN_POINT ( 'NONE',  ( 16.51473224551069308, 9.474510206698969483, 109.1655762719810383 ) ) ;
#55685=CARTESIAN_POINT ( 'NONE',  ( -15.72974639402176322, -15.80617190586768395, 104.3760903946856899 ) ) ;
#55686=CARTESIAN_POINT ( 'NONE',  ( 16.51473224551069308, 9.474510206698969483, 74.16557627198103830 ) ) ;
#55687=CARTESIAN_POINT ( 'NONE',  ( -12.14591786802326823, 12.06949235617739902, 58.12609039468568994 ) ) ;
#55688=CARTESIAN_POINT ( 'NONE',  ( -0.05219959533937732626, 21.53943276465977519, 92.50109039468567573 ) ) ;
#55689=CARTESIAN_POINT ( 'NONE',  ( -8.314922557961024197, 14.29746914071037800, 67.91775706135234714 ) ) ;
#55690=CARTESIAN_POINT ( 'NONE',  ( -19.02544592524334988, -5.153800228976617603, 53.95942372801898301 ) ) ;
#55691=CARTESIAN_POINT ( 'NONE',  ( 5.049401038297881783, 19.05341960407617563, 62.29275706135234003 ) ) ;
#55692=ORIENTED_EDGE ( 'NONE', *, *, #43196, .F. ) ;
#55693=CARTESIAN_POINT ( 'NONE',  ( 5.823673210054444382, -21.52544592524334988, 65.20942372801901854 ) ) ;
#55694=CARTESIAN_POINT ( 'NONE',  ( -19.02544592524342804, 5.153800228976336051, 71.04057627198099567 ) ) ;
#55695=CARTESIAN_POINT ( 'NONE',  ( 9.474510206698971260, -16.51473224551069308, 22.91557627198102765 ) ) ;
#55696=CARTESIAN_POINT ( 'NONE',  ( 16.46253265017146816, 9.564922557961045513, 56.66775706135233293 ) ) ;
#55697=CARTESIAN_POINT ( 'NONE',  ( 13.89961937509977652, -13.97604488694527269, 113.1239096053143527 ) ) ;
#55698=CARTESIAN_POINT ( 'NONE',  ( 16.51473224551069308, 9.474510206698969483, 84.16557627198102409 ) ) ;
#55699=CARTESIAN_POINT ( 'NONE',  ( -12.06949235617756955, 12.14591786802309770, 35.62390960531437401 ) ) ;
#55700=CARTESIAN_POINT ( 'NONE',  ( -21.55341960407610458, -5.719274019375992779, 46.45724293864769550 ) ) ;
#55702=CARTESIAN_POINT ( 'NONE',  ( -10.72451020669870658, -18.67979575497194134, 109.5844237280190328 ) ) ;
#55703=CARTESIAN_POINT ( 'NONE',  ( -17.26172910966779739, -6.454744622555842248, 79.19353091350777163 ) ) ;
#55704=CARTESIAN_POINT ( 'NONE',  ( -19.02544592524342804, 5.153800228976336051, 36.04057627198100988 ) ) ;
#55705=CARTESIAN_POINT ( 'NONE',  ( 5.153800228976335163, 19.02544592524342804, 29.79057627198102409 ) ) ;
#55708=CARTESIAN_POINT ( 'NONE',  ( -21.53943276465977519, -0.05219959533937600094, 63.75109039468568284 ) ) ;
#55710=CARTESIAN_POINT ( 'NONE',  ( -12.14591786802326823, 12.06949235617739902, 63.12609039468568994 ) ) ;
#55711=CARTESIAN_POINT ( 'NONE',  ( 21.52544592524344225, -5.823673210054117533, 88.54057627198103830 ) ) ;
#55712=CARTESIAN_POINT ( 'NONE',  ( 12.06949235617757843, -12.14591786802309237, 53.12390960531436690 ) ) ;
#55713=CARTESIAN_POINT ( 'NONE',  ( 13.97604488694527802, 13.89961937509977652, 29.37390960531435979 ) ) ;
#55715=CARTESIAN_POINT ( 'NONE',  ( 15.72974639402176855, 15.80617190586768217, 46.87609039468568994 ) ) ;
#55716=CARTESIAN_POINT ( 'NONE',  ( -19.03943276465977164, -0.05219959533935918106, 53.75109039468566863 ) ) ;
#55717=CARTESIAN_POINT ( 'NONE',  ( -13.89961937509977652, 13.97604488694528158, 35.62390960531435269 ) ) ;
#55718=CARTESIAN_POINT ( 'NONE',  ( -5.823673210054431948, 21.52544592524334988, 82.70942372801900433 ) ) ;
#55719=CARTESIAN_POINT ( 'NONE',  ( 16.36317988757059538, -7.306389748694917863, 31.59789608363227487 ) ) ;
#55720=CARTESIAN_POINT ( 'NONE',  ( -8.224510206698948167, 14.34966873604960824, 40.41557627198103120 ) ) ;
#55722=CARTESIAN_POINT ( 'NONE',  ( -5.719274019375978568, 21.55341960407610458, 45.20724293864769550 ) ) ;
#55724=CARTESIAN_POINT ( 'NONE',  ( 13.97604488694527802, 13.89961937509977652, 94.37390960531436690 ) ) ;
#55725=CARTESIAN_POINT ( 'NONE',  ( 8.224510206698953496, -14.34966873604960469, 92.91557627198103830 ) ) ;
#55726=CARTESIAN_POINT ( 'NONE',  ( -19.05341960407617563, 5.049401038297882671, 103.5427570613523329 ) ) ;
#55727=CARTESIAN_POINT ( 'NONE',  ( -0.05219959533907301413, -21.53943276465977519, 67.49890960531436690 ) ) ;
#55728=ORIENTED_EDGE ( 'NONE', *, *, #193154, .T. ) ;
#55729=CARTESIAN_POINT ( 'NONE',  ( -5.153800228976328057, -19.02544592524343514, 37.29057627198102409 ) ) ;
#55730=CARTESIAN_POINT ( 'NONE',  ( -19.03943276465977164, 0.05219959533909376836, 86.24890960531436690 ) ) ;
#55731=CARTESIAN_POINT ( 'NONE',  ( 21.52544592524344225, -5.823673210054117533, 88.54057627198103830 ) ) ;
#55732=CARTESIAN_POINT ( 'NONE',  ( -8.224510206698948167, 14.34966873604960824, 30.41557627198101699 ) ) ;
#55733=CARTESIAN_POINT ( 'NONE',  ( 5.153800228976335163, 19.02544592524342804, 104.7905762719809957 ) ) ;
#55734=CARTESIAN_POINT ( 'NONE',  ( 16.51473224551083163, -9.474510206698727899, 85.83442372801900433 ) ) ;
#55735=CARTESIAN_POINT ( 'NONE',  ( -5.719274019375665041, -21.55341960407619695, 89.79275706135236135 ) ) ;
#55736=CARTESIAN_POINT ( 'NONE',  ( -18.67979575497178146, -10.72451020669898902, 81.66557627198103830 ) ) ;
#55737=CARTESIAN_POINT ( 'NONE',  ( 18.62759615963271287, -10.81492255796078972, 33.33224293864769550 ) ) ;
#55738=CARTESIAN_POINT ( 'NONE',  ( 9.474510206698971260, -16.51473224551069308, 52.91557627198102409 ) ) ;
#55739=CARTESIAN_POINT ( 'NONE',  ( -4.483927247898782831, 16.52544592524335698, 112.7094237280190328 ) ) ;
#55740=CARTESIAN_POINT ( 'NONE',  ( -19.03943276465977164, 0.05219959533909376836, 71.24890960531435269 ) ) ;
#55743=CARTESIAN_POINT ( 'NONE',  ( 9.474510206698729675, 16.51473224551082808, 27.08442372801900433 ) ) ;
#55744=CARTESIAN_POINT ( 'NONE',  ( -16.52544592524342804, 4.483927247898546575, 81.04057627198102409 ) ) ;
#55745=CARTESIAN_POINT ( 'NONE',  ( -15.72974639402176322, -15.80617190586768395, 19.37609039468568639 ) ) ;
#55747=CARTESIAN_POINT ( 'NONE',  ( -10.81492255796078084, -18.62759615963271287, 57.08224293864769550 ) ) ;
#55748=CARTESIAN_POINT ( 'NONE',  ( 8.224510206698742110, 14.34966873604972548, 87.08442372801901854 ) ) ;
#55749=CARTESIAN_POINT ( 'NONE',  ( 9.564922557960805705, 16.46253265017160317, 24.58224293864769194 ) ) ;
#55750=CARTESIAN_POINT ( 'NONE',  ( 5.153800228976335163, 19.02544592524342804, 69.79057627198103830 ) ) ;
#55752=CARTESIAN_POINT ( 'NONE',  ( 8.314922557960818139, 14.29746914071049879, 34.58224293864770260 ) ) ;
#55753=CARTESIAN_POINT ( 'NONE',  ( -10.72451020669870658, -18.67979575497194134, 64.58442372801900433 ) ) ;
#55754=CARTESIAN_POINT ( 'NONE',  ( -16.46253265017160317, 9.564922557960807481, 115.8322429386477097 ) ) ;
#55755=CARTESIAN_POINT ( 'NONE',  ( 21.52544592524334988, 5.823673210054432836, 96.45942372801901854 ) ) ;
#55756=CARTESIAN_POINT ( 'NONE',  ( 5.153800228976335163, 19.02544592524342804, 49.79057627198100988 ) ) ;
#55757=CARTESIAN_POINT ( 'NONE',  ( -13.89961937509977652, 13.97604488694528158, 40.62390960531435979 ) ) ;
#55759=CARTESIAN_POINT ( 'NONE',  ( -15.80617190586768217, 15.72974639402176855, 98.12609039468570415 ) ) ;
#55760=CARTESIAN_POINT ( 'NONE',  ( 8.224510206698742110, 14.34966873604972548, 52.08442372801901854 ) ) ;
#55761=CARTESIAN_POINT ( 'NONE',  ( -18.62759615963255300, -10.81492255796106328, 89.16775706135236135 ) ) ;
#55762=CARTESIAN_POINT ( 'NONE',  ( -9.564922557960796823, -16.46253265017161027, 112.0822429386476955 ) ) ;
#55763=CARTESIAN_POINT ( 'NONE',  ( 19.05341960407617918, -5.049401038297876454, 91.04275706135234714 ) ) ;
#55764=CARTESIAN_POINT ( 'NONE',  ( 10.72451020669871369, 18.67979575497193778, 62.08442372801901143 ) ) ;
#55765=CARTESIAN_POINT ( 'NONE',  ( 8.314922557961029526, -14.29746914071037800, 40.41775706135234714 ) ) ;
#55766=CARTESIAN_POINT ( 'NONE',  ( -5.049401038297874678, -19.05341960407617918, 79.79275706135233293 ) ) ;
#55767=CARTESIAN_POINT ( 'NONE',  ( -13.89961937509977652, 13.97604488694528158, 55.62390960531434558 ) ) ;
#55768=CARTESIAN_POINT ( 'NONE',  ( 9.564922557961047289, -16.46253265017146816, 90.41775706135234714 ) ) ;
#55769=CARTESIAN_POINT ( 'NONE',  ( 5.153800228976615827, -19.02544592524334988, 90.20942372801900433 ) ) ;
#55770=CARTESIAN_POINT ( 'NONE',  ( -12.06949235617756955, 12.14591786802309770, 50.62390960531435979 ) ) ;
#55771=CARTESIAN_POINT ( 'NONE',  ( 19.02544592524334988, 5.153800228976608722, 71.45942372801900433 ) ) ;
#55772=CARTESIAN_POINT ( 'NONE',  ( 16.53943276465976808, 0.05219959533934440121, 66.25109039468567573 ) ) ;
#55773=CARTESIAN_POINT ( 'NONE',  ( -13.89961937509957401, -13.97604488694547875, 19.37609039468566507 ) ) ;
#55775=CARTESIAN_POINT ( 'NONE',  ( 19.02544592524343514, -5.153800228976328945, 33.54057627198102409 ) ) ;
#55776=CARTESIAN_POINT ( 'NONE',  ( -5.153800228976328057, -19.02544592524343514, 42.29057627198101699 ) ) ;
#55777=CARTESIAN_POINT ( 'NONE',  ( 8.224510206698742110, 14.34966873604972548, 57.08442372801901854 ) ) ;
#55781=CARTESIAN_POINT ( 'NONE',  ( -5.153800228976328057, -19.02544592524343514, 112.2905762719810099 ) ) ;
#55784=CARTESIAN_POINT ( 'NONE',  ( -0.05219959533936034679, 19.03943276465977164, 92.50109039468566152 ) ) ;
#55786=CARTESIAN_POINT ( 'NONE',  ( 10.81492255796078972, 18.62759615963270932, 39.58224293864769550 ) ) ;
#55787=CARTESIAN_POINT ( 'NONE',  ( 16.51473224551083163, -9.474510206698727899, 30.83442372801900433 ) ) ;
#55788=CARTESIAN_POINT ( 'NONE',  ( 19.05341960407617918, -5.049401038297876454, 111.0427570613523329 ) ) ;
#55789=CARTESIAN_POINT ( 'NONE',  ( 0.05219959533909260263, 19.03943276465977164, 29.99890960531435979 ) ) ;
#55790=CARTESIAN_POINT ( 'NONE',  ( -19.05341960407611168, -5.049401038298163336, 31.45724293864769550 ) ) ;
#55791=CARTESIAN_POINT ( 'NONE',  ( 21.53943276465977519, -0.05219959533907433946, 73.74890960531433848 ) ) ;
#55792=CARTESIAN_POINT ( 'NONE',  ( -9.564922557960796823, -16.46253265017161027, 97.08224293864769550 ) ) ;
#55793=CARTESIAN_POINT ( 'NONE',  ( -0.05219959533909027116, -19.03943276465977164, 42.49890960531435269 ) ) ;
#55795=CARTESIAN_POINT ( 'NONE',  ( -5.049401038297874678, -19.05341960407617918, 84.79275706135233293 ) ) ;
#55796=CARTESIAN_POINT ( 'NONE',  ( 16.55341960407611168, 4.379528057220329451, 48.95724293864770971 ) ) ;
#55797=CARTESIAN_POINT ( 'NONE',  ( -0.05219959533907301413, -21.53943276465977519, 27.49890960531435269 ) ) ;
#55798=CARTESIAN_POINT ( 'NONE',  ( 0.05219959533937995610, -21.53943276465977519, 110.0010903946856757 ) ) ;
#55799=CARTESIAN_POINT ( 'NONE',  ( 10.81492255796078972, 18.62759615963270932, 79.58224293864769550 ) ) ;
#55800=CARTESIAN_POINT ( 'NONE',  ( 10.81492255796106328, -18.62759615963255655, 65.41775706135234714 ) ) ;
#55801=CARTESIAN_POINT ( 'NONE',  ( 15.80617190586769283, -15.72974639402175789, 65.62609039468568994 ) ) ;
#55802=CARTESIAN_POINT ( 'NONE',  ( -9.474510206698964154, 16.51473224551069663, 105.4155762719810383 ) ) ;
#55803=CARTESIAN_POINT ( 'NONE',  ( 14.29746914071037800, 8.314922557961029526, 101.6677570613523613 ) ) ;
#55804=CARTESIAN_POINT ( 'NONE',  ( -15.72974639402176322, -15.80617190586768395, 59.37609039468568284 ) ) ;
#55805=CARTESIAN_POINT ( 'NONE',  ( 9.564922557960805705, 16.46253265017160317, 54.58224293864769550 ) ) ;
#55806=CARTESIAN_POINT ( 'NONE',  ( 16.46253265017146816, 9.564922557961045513, 36.66775706135233293 ) ) ;
#55807=CARTESIAN_POINT ( 'NONE',  ( -21.55341960407619339, 5.719274019375674811, 33.54275706135234714 ) ) ;
#55808=CARTESIAN_POINT ( 'NONE',  ( 16.51473224551069308, 9.474510206698969483, 74.16557627198103830 ) ) ;
#55809=CARTESIAN_POINT ( 'NONE',  ( 0.05219959533910956823, 16.53943276465976808, 79.99890960531435269 ) ) ;
#55810=CARTESIAN_POINT ( 'NONE',  ( 8.314922557960818139, 14.29746914071049879, 49.58224293864769550 ) ) ;
#55811=CARTESIAN_POINT ( 'NONE',  ( 0.05219959533907565091, 21.53943276465977519, 59.99890960531436690 ) ) ;
#55812=CARTESIAN_POINT ( 'NONE',  ( -16.46253265017160317, 9.564922557960807481, 55.83224293864769550 ) ) ;
#55813=CARTESIAN_POINT ( 'NONE',  ( 0.05219959533907565091, 21.53943276465977519, 69.99890960531435269 ) ) ;
#55814=CARTESIAN_POINT ( 'NONE',  ( 5.153800228976615827, -19.02544592524334988, 55.20942372801899722 ) ) ;
#55816=CARTESIAN_POINT ( 'NONE',  ( -8.224510206698948167, 14.34966873604960824, 65.41557627198102409 ) ) ;
#55817=CARTESIAN_POINT ( 'NONE',  ( -5.719274019375978568, 21.55341960407610458, 35.20724293864768839 ) ) ;
#55820=CARTESIAN_POINT ( 'NONE',  ( 14.34966873604972726, -8.224510206698740333, 80.83442372801901854 ) ) ;
#55822=CARTESIAN_POINT ( 'NONE',  ( 5.153800228976615827, -19.02544592524334988, 95.20942372801897591 ) ) ;
#55823=CARTESIAN_POINT ( 'NONE',  ( -0.05219959533910754901, -16.53943276465976808, 57.49890960531435979 ) ) ;
#55825=CARTESIAN_POINT ( 'NONE',  ( 19.03943276465977164, -0.05219959533909143690, 53.74890960531436690 ) ) ;
#55826=CARTESIAN_POINT ( 'NONE',  ( 14.29746914071049879, -8.314922557960816363, 43.33224293864769550 ) ) ;
#55827=CARTESIAN_POINT ( 'NONE',  ( -9.474510206698964154, 16.51473224551069663, 90.41557627198103830 ) ) ;
#55828=CARTESIAN_POINT ( 'NONE',  ( 19.03943276465977164, -0.05219959533909143690, 58.74890960531435979 ) ) ;
#55829=CARTESIAN_POINT ( 'NONE',  ( -18.62759615963255300, -10.81492255796106328, 59.16775706135234714 ) ) ;
#55830=CARTESIAN_POINT ( 'NONE',  ( -5.049401038298153566, 19.05341960407611168, 75.20724293864769550 ) ) ;
#55831=CARTESIAN_POINT ( 'NONE',  ( 19.03943276465977164, -0.05219959533909143690, 23.74890960531435269 ) ) ;
#55832=CARTESIAN_POINT ( 'NONE',  ( -19.03943276465977164, 0.05219959533909376836, 76.24890960531435269 ) ) ;
#55833=CARTESIAN_POINT ( 'NONE',  ( -15.80617190586745835, -15.72974639402198527, 51.87390960531437401 ) ) ;
#55834=CARTESIAN_POINT ( 'NONE',  ( 16.46253265017160672, -9.564922557960803928, 38.33224293864768839 ) ) ;
#55835=CARTESIAN_POINT ( 'NONE',  ( 21.55341960407610458, 5.719274019375980345, 38.95724293864768839 ) ) ;
#55836=CARTESIAN_POINT ( 'NONE',  ( -8.314922557961024197, 14.29746914071037800, 107.9177570613523471 ) ) ;
#55837=CARTESIAN_POINT ( 'NONE',  ( 5.049401038297881783, 19.05341960407617563, 27.29275706135232937 ) ) ;
#55838=CARTESIAN_POINT ( 'NONE',  ( 8.224510206698742110, 14.34966873604972548, 47.08442372801901854 ) ) ;
#55839=CARTESIAN_POINT ( 'NONE',  ( 16.55341960407618274, -4.379528057220086978, 86.04275706135236135 ) ) ;
#55840=CARTESIAN_POINT ( 'NONE',  ( -16.46253265017160317, 9.564922557960807481, 115.8322429386477097 ) ) ;
#55841=CARTESIAN_POINT ( 'NONE',  ( 16.52544592524335698, 4.483927247898782831, 71.45942372801901854 ) ) ;
#55842=CARTESIAN_POINT ( 'NONE',  ( 18.62759615963271287, -10.81492255796078972, 23.33224293864769194 ) ) ;
#55843=CARTESIAN_POINT ( 'NONE',  ( -13.97604488694527625, -13.89961937509977652, 36.87390960531436690 ) ) ;
#55844=CARTESIAN_POINT ( 'NONE',  ( -16.52544592524335698, -4.483927247898792601, 33.95942372801901143 ) ) ;
#55845=CARTESIAN_POINT ( 'NONE',  ( 16.51473224551069308, 9.474510206698969483, 49.16557627198102409 ) ) ;
#55846=CARTESIAN_POINT ( 'NONE',  ( 0.05219959533937995610, -21.53943276465977519, 20.00109039468568639 ) ) ;
#55847=CARTESIAN_POINT ( 'NONE',  ( 12.14591786802327356, -12.06949235617739191, 30.62609039468567929 ) ) ;
#55848=CARTESIAN_POINT ( 'NONE',  ( 16.52544592524335698, 4.483927247898782831, 96.45942372801901854 ) ) ;
#55850=CARTESIAN_POINT ( 'NONE',  ( 5.823673210054444382, -21.52544592524334988, 95.20942372801903275 ) ) ;
#55851=CARTESIAN_POINT ( 'NONE',  ( 16.46253265017146816, 9.564922557961045513, 96.66775706135233293 ) ) ;
#55852=CARTESIAN_POINT ( 'NONE',  ( 16.46253265017146816, 9.564922557961045513, 61.66775706135234003 ) ) ;
#55853=CARTESIAN_POINT ( 'NONE',  ( -14.29746914071049879, 8.314922557960819915, 60.83224293864769550 ) ) ;
#55854=CARTESIAN_POINT ( 'NONE',  ( 8.314922557960818139, 14.29746914071049879, 114.5822429386477097 ) ) ;
#55855=CARTESIAN_POINT ( 'NONE',  ( -5.153800228976607833, 19.02544592524334988, 62.70942372801899722 ) ) ;
#55857=CARTESIAN_POINT ( 'NONE',  ( 18.67979575497194134, -10.72451020669871369, 65.83442372801900433 ) ) ;
#55858=CARTESIAN_POINT ( 'NONE',  ( -4.483927247898782831, 16.52544592524335698, 32.70942372801900433 ) ) ;
#55860=CARTESIAN_POINT ( 'NONE',  ( 18.67979575497178502, 10.72451020669898547, 24.16557627198103120 ) ) ;
#55861=CARTESIAN_POINT ( 'NONE',  ( 16.51473224551083163, -9.474510206698727899, 110.8344237280190043 ) ) ;
#55862=CARTESIAN_POINT ( 'NONE',  ( -9.474510206698964154, 16.51473224551069663, 110.4155762719810383 ) ) ;
#55864=CARTESIAN_POINT ( 'NONE',  ( 0.05219959533909260263, 19.03943276465977164, 29.99890960531435979 ) ) ;
#55865=CARTESIAN_POINT ( 'NONE',  ( 21.53943276465977519, 0.05219959533937863772, 106.2510903946856757 ) ) ;
#55866=CARTESIAN_POINT ( 'NONE',  ( 19.05341960407611168, 5.049401038298154454, 53.95724293864770260 ) ) ;
#55867=CARTESIAN_POINT ( 'NONE',  ( 10.72451020669871369, 18.67979575497193778, 67.08442372801901854 ) ) ;
#55868=CARTESIAN_POINT ( 'NONE',  ( -15.80617190586768217, 15.72974639402176855, 103.1260903946856757 ) ) ;
#55869=CARTESIAN_POINT ( 'NONE',  ( 12.14591786802327356, -12.06949235617739191, 100.6260903946857184 ) ) ;
#55870=CARTESIAN_POINT ( 'NONE',  ( 13.97604488694527802, 13.89961937509977652, 74.37390960531436690 ) ) ;
#55871=CARTESIAN_POINT ( 'NONE',  ( -0.05219959533937732626, 21.53943276465977519, 52.50109039468567573 ) ) ;
#55872=ADVANCED_FACE ( 'NONE', ( #47750 ), #80059, .F. ) ;
#55873=B_SPLINE_CURVE_WITH_KNOTS ( 'NONE', 3,
 ( #170964, #46630, #183166, #135677, #106302, #51591 ),
 .UNSPECIFIED., .F., .F.,
 ( 4, 2, 4 ),
 ( 0.003239945802372288554, 0.003620412082092147252, 0.004000878361812005950 ),
 .UNSPECIFIED. ) ;
#55874=CARTESIAN_POINT ( 'NONE',  ( 5.719274019375673035, 21.55341960407619339, 52.29275706135236135 ) ) ;
#55875=CARTESIAN_POINT ( 'NONE',  ( -0.05219959533936034679, 19.03943276465977164, 82.50109039468567573 ) ) ;
#55876=CARTESIAN_POINT ( 'NONE',  ( 5.153800228976335163, 19.02544592524342804, 104.7905762719809957 ) ) ;
#55877=CARTESIAN_POINT ( 'NONE',  ( 12.06949235617757843, -12.14591786802309237, 113.1239096053143953 ) ) ;
#55878=CARTESIAN_POINT ( 'NONE',  ( -21.53943276465977519, 0.05219959533907696930, 101.2489096053143669 ) ) ;
#55879=CARTESIAN_POINT ( 'NONE',  ( -0.05219959533936034679, 19.03943276465977164, 22.50109039468566152 ) ) ;
#55880=CARTESIAN_POINT ( 'NONE',  ( 4.483927247898545687, 16.52544592524342804, 99.79057627198103830 ) ) ;
#55881=CARTESIAN_POINT ( 'NONE',  ( -13.97604488694527625, -13.89961937509977652, 46.87390960531435979 ) ) ;
#55882=CARTESIAN_POINT ( 'NONE',  ( 13.97604488694548053, -13.89961937509957401, 100.6260903946856615 ) ) ;
#55883=CARTESIAN_POINT ( 'NONE',  ( 4.379528057220339221, -16.55341960407611168, 67.70724293864769550 ) ) ;
#55884=CARTESIAN_POINT ( 'NONE',  ( -21.55341960407619339, 5.719274019375674811, 108.5427570613523756 ) ) ;
#55885=CARTESIAN_POINT ( 'NONE',  ( 0.05219959533909260263, 19.03943276465977164, 109.9989096053143669 ) ) ;
#55886=CARTESIAN_POINT ( 'NONE',  ( 19.05341960407617918, -5.049401038297876454, 81.04275706135231871 ) ) ;
#55887=CARTESIAN_POINT ( 'NONE',  ( -21.52544592524343514, 5.823673210054127303, 76.04057627198102409 ) ) ;
#55888=CARTESIAN_POINT ( 'NONE',  ( -21.55341960407619339, 5.719274019375674811, 48.54275706135234714 ) ) ;
#55889=CARTESIAN_POINT ( 'NONE',  ( -16.52544592524335698, -4.483927247898792601, 38.95942372801901854 ) ) ;
#55890=CARTESIAN_POINT ( 'NONE',  ( 16.52544592524335698, 4.483927247898782831, 86.45942372801901854 ) ) ;
#55891=CARTESIAN_POINT ( 'NONE',  ( 16.52544592524335698, 4.483927247898782831, 36.45942372801901143 ) ) ;
#55892=CARTESIAN_POINT ( 'NONE',  ( -21.55341960407619339, 5.719274019375674811, 33.54275706135234714 ) ) ;
#55893=CARTESIAN_POINT ( 'NONE',  ( 15.72974639402199770, -15.80617190586745480, 38.12390960531436690 ) ) ;
#55894=CARTESIAN_POINT ( 'NONE',  ( 16.51473224551069308, 9.474510206698969483, 29.16557627198103475 ) ) ;
#55896=CARTESIAN_POINT ( 'NONE',  ( -16.55341960407617563, 4.379528057220093196, 63.54275706135234003 ) ) ;
#55898=CARTESIAN_POINT ( 'NONE',  ( -18.62759615963270932, 10.81492255796079327, 90.83224293864769550 ) ) ;
#55899=CARTESIAN_POINT ( 'NONE',  ( 8.314922557960818139, 14.29746914071049879, 44.58224293864769550 ) ) ;
#55900=CARTESIAN_POINT ( 'NONE',  ( 8.314922557961029526, -14.29746914071037800, 50.41775706135235424 ) ) ;
#55901=CARTESIAN_POINT ( 'NONE',  ( -9.564922557960796823, -16.46253265017161027, 62.08224293864769550 ) ) ;
#55902=CARTESIAN_POINT ( 'NONE',  ( -16.46253265017146816, -9.564922557961047289, 84.16775706135233293 ) ) ;
#55903=CARTESIAN_POINT ( 'NONE',  ( -21.55341960407610458, -5.719274019375992779, 86.45724293864770971 ) ) ;
#55904=CARTESIAN_POINT ( 'NONE',  ( 8.224510206698953496, -14.34966873604960469, 37.91557627198102409 ) ) ;
#55907=CARTESIAN_POINT ( 'NONE',  ( -15.80617190586745835, -15.72974639402198527, 66.87390960531436690 ) ) ;
#55908=CARTESIAN_POINT ( 'NONE',  ( 12.14591786802327356, -12.06949235617739191, 110.6260903946857042 ) ) ;
#55909=ORIENTED_EDGE ( 'NONE', *, *, #14853, .F. ) ;
#55910=CARTESIAN_POINT ( 'NONE',  ( 18.22780087662122739, 5.500000000000000888, 86.48236817873107896 ) ) ;
#55911=CARTESIAN_POINT ( 'NONE',  ( -18.67979575497178146, -10.72451020669898902, 86.66557627198102409 ) ) ;
#55912=CARTESIAN_POINT ( 'NONE',  ( 16.53943276465976808, -0.05219959533910856209, 23.74890960531435269 ) ) ;
#55913=CARTESIAN_POINT ( 'NONE',  ( -12.06949235617739369, -12.14591786802326823, 34.37609039468568284 ) ) ;
#55914=CARTESIAN_POINT ( 'NONE',  ( 16.51473224551069308, 9.474510206698969483, 34.16557627198102409 ) ) ;
#55915=CARTESIAN_POINT ( 'NONE',  ( -19.05341960407611168, -5.049401038298163336, 71.45724293864766707 ) ) ;
#55917=CARTESIAN_POINT ( 'NONE',  ( -15.80617190586745835, -15.72974639402198527, 26.87390960531435979 ) ) ;
#55919=CARTESIAN_POINT ( 'NONE',  ( -4.379528057220086978, -16.55341960407618274, 99.79275706135234714 ) ) ;
#55920=CARTESIAN_POINT ( 'NONE',  ( 5.153800228976615827, -19.02544592524334988, 110.2094237280189901 ) ) ;
#55921=CARTESIAN_POINT ( 'NONE',  ( 16.46253265017146816, 9.564922557961045513, 31.66775706135232937 ) ) ;
#55922=CARTESIAN_POINT ( 'NONE',  ( 10.81492255796078972, 18.62759615963270932, 94.58224293864769550 ) ) ;
#55923=CARTESIAN_POINT ( 'NONE',  ( -4.483927247898782831, 16.52544592524335698, 112.7094237280190328 ) ) ;
#55925=CARTESIAN_POINT ( 'NONE',  ( -0.05219959533907301413, -21.53943276465977519, 52.49890960531435979 ) ) ;
#55926=CARTESIAN_POINT ( 'NONE',  ( 0.05219959533936267826, -19.03943276465977164, 110.0010903946856757 ) ) ;
#55927=CARTESIAN_POINT ( 'NONE',  ( -9.564922557960796823, -16.46253265017161027, 107.0822429386476955 ) ) ;
#55928=CARTESIAN_POINT ( 'NONE',  ( 15.80617190586769283, -15.72974639402175789, 60.62609039468567573 ) ) ;
#55929=CARTESIAN_POINT ( 'NONE',  ( 19.03943276465977164, -0.05219959533909143690, 63.74890960531435979 ) ) ;
#55930=CARTESIAN_POINT ( 'NONE',  ( 12.06949235617757843, -12.14591786802309237, 98.12390960531436690 ) ) ;
#55932=CARTESIAN_POINT ( 'NONE',  ( -5.153800228976328057, -19.02544592524343514, 77.29057627198099567 ) ) ;
#55933=CARTESIAN_POINT ( 'NONE',  ( -0.05219959533910754901, -16.53943276465976808, 82.49890960531436690 ) ) ;
#55935=CARTESIAN_POINT ( 'NONE',  ( 9.474510206698729675, 16.51473224551082808, 87.08442372801900433 ) ) ;
#55936=CARTESIAN_POINT ( 'NONE',  ( 19.34837522270366961, 5.499999999999797495, 93.36337684832579953 ) ) ;
#55937=CARTESIAN_POINT ( 'NONE',  ( 13.89961937509977652, -13.97604488694527269, 58.12390960531436690 ) ) ;
#55939=CARTESIAN_POINT ( 'NONE',  ( 15.72974639402176855, 15.80617190586768217, 86.87609039468568994 ) ) ;
#55940=CARTESIAN_POINT ( 'NONE',  ( -16.46253265017160317, 9.564922557960807481, 105.8322429386476955 ) ) ;
#55942=CARTESIAN_POINT ( 'NONE',  ( -4.379528057220086978, -16.55341960407618274, 64.79275706135234714 ) ) ;
#55944=CARTESIAN_POINT ( 'NONE',  ( 5.049401038297881783, 19.05341960407617563, 42.29275706135234003 ) ) ;
#55945=CARTESIAN_POINT ( 'NONE',  ( -0.05219959533937732626, 21.53943276465977519, 102.5010903946856899 ) ) ;
#55948=CARTESIAN_POINT ( 'NONE',  ( 12.06949235617739724, 12.14591786802326823, 101.8760903946857042 ) ) ;
#55950=CARTESIAN_POINT ( 'NONE',  ( -0.05219959533934338120, 16.53943276465976808, 97.50109039468567573 ) ) ;
#55951=CARTESIAN_POINT ( 'NONE',  ( 17.50000000000000000, 5.500000000000011546, 68.78230962303564411 ) ) ;
#55952=CARTESIAN_POINT ( 'NONE',  ( 12.14591786802327356, -12.06949235617739191, 65.62609039468568994 ) ) ;
#55954=CARTESIAN_POINT ( 'NONE',  ( -15.72974639402176322, -15.80617190586768395, 74.37609039468568994 ) ) ;
#55955=CARTESIAN_POINT ( 'NONE',  ( 9.474510206698729675, 16.51473224551082808, 87.08442372801900433 ) ) ;
#55956=CARTESIAN_POINT ( 'NONE',  ( -5.153800228976607833, 19.02544592524334988, 22.70942372801899012 ) ) ;
#55957=CARTESIAN_POINT ( 'NONE',  ( 19.05341960407611168, 5.049401038298154454, 63.95724293864769550 ) ) ;
#55958=CARTESIAN_POINT ( 'NONE',  ( 13.89961937509977652, -13.97604488694527269, 53.12390960531434558 ) ) ;
#55960=CARTESIAN_POINT ( 'NONE',  ( -21.55341960407610458, -5.719274019375992779, 81.45724293864769550 ) ) ;
#55961=CARTESIAN_POINT ( 'NONE',  ( 0.05219959533907565091, 21.53943276465977519, 29.99890960531435979 ) ) ;
#55962=CARTESIAN_POINT ( 'NONE',  ( -0.05219959533909027116, -19.03943276465977164, 37.49890960531436690 ) ) ;
#55963=CARTESIAN_POINT ( 'NONE',  ( -16.52544592524335698, -4.483927247898792601, 63.95942372801901854 ) ) ;
#55966=CARTESIAN_POINT ( 'NONE',  ( 15.72974639402176855, 15.80617190586768217, 36.87609039468568994 ) ) ;
#55967=CARTESIAN_POINT ( 'NONE',  ( 4.483927247898545687, 16.52544592524342804, 64.79057627198103830 ) ) ;
#55969=CARTESIAN_POINT ( 'NONE',  ( 12.14591786802327356, -12.06949235617739191, 20.62609039468568639 ) ) ;
#55970=CARTESIAN_POINT ( 'NONE',  ( 16.46253265017146816, 9.564922557961045513, 51.66775706135233293 ) ) ;
#55971=CARTESIAN_POINT ( 'NONE',  ( -14.34966873604960291, -8.224510206698953496, 56.66557627198103830 ) ) ;
#55972=CARTESIAN_POINT ( 'NONE',  ( -21.53943276465977519, 0.05219959533907696930, 116.2489096053143669 ) ) ;
#55974=CARTESIAN_POINT ( 'NONE',  ( 21.55341960407610458, 5.719274019375980345, 83.95724293864770971 ) ) ;
#55975=CARTESIAN_POINT ( 'NONE',  ( 19.03943276465977164, -0.05219959533909143690, 88.74890960531436690 ) ) ;
#55976=CARTESIAN_POINT ( 'NONE',  ( 16.55341960407611168, 4.379528057220329451, 58.95724293864770971 ) ) ;
#55979=CARTESIAN_POINT ( 'NONE',  ( -9.564922557961040184, 16.46253265017147172, 72.91775706135233293 ) ) ;
#55980=CARTESIAN_POINT ( 'NONE',  ( -18.67979575497178146, -10.72451020669898902, 111.6655762719810525 ) ) ;
#55981=CARTESIAN_POINT ( 'NONE',  ( -19.03943276465977164, 0.05219959533909376836, 51.24890960531436690 ) ) ;
#55982=CARTESIAN_POINT ( 'NONE',  ( 9.564922557961047289, -16.46253265017146816, 40.41775706135234003 ) ) ;
#55983=CARTESIAN_POINT ( 'NONE',  ( -16.46253265017160317, 9.564922557960807481, 35.83224293864768839 ) ) ;
#55985=CARTESIAN_POINT ( 'NONE',  ( -21.52544592524334988, -5.823673210054445271, 63.95942372801901854 ) ) ;
#55986=CARTESIAN_POINT ( 'NONE',  ( -30.00000000000000000, -5.499999999999992895, 102.5000000000000142 ) ) ;
#55987=CARTESIAN_POINT ( 'NONE',  ( -16.53943276465976808, 0.05219959533911058130, 41.24890960531435269 ) ) ;
#55988=CARTESIAN_POINT ( 'NONE',  ( -19.03943276465977164, 0.05219959533909376836, 56.24890960531435979 ) ) ;
#55989=CARTESIAN_POINT ( 'NONE',  ( -10.72451020669898014, 18.67979575497178502, 80.41557627198103830 ) ) ;
#55990=CARTESIAN_POINT ( 'NONE',  ( 19.03943276465977164, -0.05219959533909143690, 58.74890960531435979 ) ) ;
#55991=CARTESIAN_POINT ( 'NONE',  ( -0.05219959533907301413, -21.53943276465977519, 67.49890960531436690 ) ) ;
#55992=CARTESIAN_POINT ( 'NONE',  ( 10.72451020669871369, 18.67979575497193778, 102.0844237280190185 ) ) ;
#55994=CARTESIAN_POINT ( 'NONE',  ( -4.483927247898782831, 16.52544592524335698, 97.70942372801904696 ) ) ;
#55995=CARTESIAN_POINT ( 'NONE',  ( -12.06949235617756955, 12.14591786802309770, 85.62390960531436690 ) ) ;
#55996=CARTESIAN_POINT ( 'NONE',  ( 9.564922557961047289, -16.46253265017146816, 95.41775706135233293 ) ) ;
#55998=CARTESIAN_POINT ( 'NONE',  ( -16.51473224551082808, 9.474510206698731452, 38.33442372801899722 ) ) ;
#55999=CARTESIAN_POINT ( 'NONE',  ( -14.34966873604972548, 8.224510206698743886, 98.33442372801901854 ) ) ;
#56000=CARTESIAN_POINT ( 'NONE',  ( 0.05219959533936267826, -19.03943276465977164, 35.00109039468566863 ) ) ;
#56001=CARTESIAN_POINT ( 'NONE',  ( 5.049401038298161559, -19.05341960407611168, 92.70724293864769550 ) ) ;
#56002=CARTESIAN_POINT ( 'NONE',  ( -21.52544592524343514, 5.823673210054127303, 66.04057627198103830 ) ) ;
#56004=CARTESIAN_POINT ( 'NONE',  ( -9.564922557960796823, -16.46253265017161027, 27.08224293864769550 ) ) ;
#56005=CARTESIAN_POINT ( 'NONE',  ( 15.80617190586769283, -15.72974639402175789, 90.62609039468567573 ) ) ;
#56006=CARTESIAN_POINT ( 'NONE',  ( -14.29746914071037622, -8.314922557961029526, 79.16775706135234714 ) ) ;
#56007=CARTESIAN_POINT ( 'NONE',  ( -0.05219959533937732626, 21.53943276465977519, 27.50109039468567929 ) ) ;
#56008=CARTESIAN_POINT ( 'NONE',  ( 16.55341960407618274, -4.379528057220086978, 26.04275706135235779 ) ) ;
#56009=CARTESIAN_POINT ( 'NONE',  ( 13.97604488694527802, 13.89961937509977652, 109.3739096053143669 ) ) ;
#56010=CARTESIAN_POINT ( 'NONE',  ( 19.05341960407611168, 5.049401038298154454, 33.95724293864769550 ) ) ;
#56011=CARTESIAN_POINT ( 'NONE',  ( 19.03943276465977164, -0.05219959533909143690, 58.74890960531435979 ) ) ;
#56012=CARTESIAN_POINT ( 'NONE',  ( -0.05219959533934338120, 16.53943276465976808, 32.50109039468568284 ) ) ;
#56013=CARTESIAN_POINT ( 'NONE',  ( -4.483927247898539470, -16.52544592524342804, 97.29057627198105251 ) ) ;
#56014=CARTESIAN_POINT ( 'NONE',  ( -8.224510206698735004, -14.34966873604973081, 99.58442372801900433 ) ) ;
#56015=CARTESIAN_POINT ( 'NONE',  ( 10.72451020669871369, 18.67979575497193778, 42.08442372801901854 ) ) ;
#56016=CARTESIAN_POINT ( 'NONE',  ( -5.153800228976328057, -19.02544592524343514, 77.29057627198099567 ) ) ;
#56017=CARTESIAN_POINT ( 'NONE',  ( -9.564922557960796823, -16.46253265017161027, 62.08224293864769550 ) ) ;
#56018=CARTESIAN_POINT ( 'NONE',  ( 5.049401038298161559, -19.05341960407611168, 82.70724293864770971 ) ) ;
#56019=CARTESIAN_POINT ( 'NONE',  ( -12.14591786802309592, -12.06949235617757132, 36.87390960531435979 ) ) ;
#56020=CARTESIAN_POINT ( 'NONE',  ( 4.483927247898790824, -16.52544592524335698, 100.2094237280190043 ) ) ;
#56021=VERTEX_POINT ( 'NONE', #95227 ) ;
#56022=CARTESIAN_POINT ( 'NONE',  ( 13.89961937509957401, 13.97604488694547697, 41.87609039468566152 ) ) ;
#56023=CARTESIAN_POINT ( 'NONE',  ( -16.51473224551069308, -9.474510206698971260, 106.6655762719810383 ) ) ;
#56024=CARTESIAN_POINT ( 'NONE',  ( -19.03943276465977164, 0.05219959533909376836, 56.24890960531435979 ) ) ;
#56025=CARTESIAN_POINT ( 'NONE',  ( -9.474510206698720793, -16.51473224551083518, 34.58442372801899722 ) ) ;
#56027=CARTESIAN_POINT ( 'NONE',  ( -8.224510206698735004, -14.34966873604973081, 39.58442372801901143 ) ) ;
#56028=CARTESIAN_POINT ( 'NONE',  ( -13.97604488694547697, 13.89961937509957934, 73.12609039468568994 ) ) ;
#56029=CARTESIAN_POINT ( 'NONE',  ( 16.55341960407618274, -4.379528057220086978, 51.04275706135234714 ) ) ;
#56031=CARTESIAN_POINT ( 'NONE',  ( 5.049401038298161559, -19.05341960407611168, 92.70724293864769550 ) ) ;
#56032=CARTESIAN_POINT ( 'NONE',  ( 21.53943276465977519, -0.05219959533907433946, 113.7489096053143527 ) ) ;
#56033=CARTESIAN_POINT ( 'NONE',  ( -5.153800228976607833, 19.02544592524334988, 72.70942372801900433 ) ) ;
#56034=CARTESIAN_POINT ( 'NONE',  ( -19.05341960407611168, -5.049401038298163336, 101.4572429386476955 ) ) ;
#56035=CARTESIAN_POINT ( 'NONE',  ( 19.03943276465977164, -0.05219959533909143690, 33.74890960531435979 ) ) ;
#56036=CARTESIAN_POINT ( 'NONE',  ( -13.97604488694527625, -13.89961937509977652, 81.87390960531436690 ) ) ;
#56037=CARTESIAN_POINT ( 'NONE',  ( -8.224510206698948167, 14.34966873604960824, 30.41557627198101699 ) ) ;
#56038=CARTESIAN_POINT ( 'NONE',  ( 19.05341960407611168, 5.049401038298154454, 38.95724293864767418 ) ) ;
#56039=CARTESIAN_POINT ( 'NONE',  ( 9.564922557961047289, -16.46253265017146816, 50.41775706135233293 ) ) ;
#56040=CARTESIAN_POINT ( 'NONE',  ( -12.06949235617756955, 12.14591786802309770, 85.62390960531436690 ) ) ;
#56041=CARTESIAN_POINT ( 'NONE',  ( -0.05219959533936034679, 19.03943276465977164, 22.50109039468566152 ) ) ;
#56042=CARTESIAN_POINT ( 'NONE',  ( -19.05341960407611168, -5.049401038298163336, 46.45724293864768129 ) ) ;
#56043=CARTESIAN_POINT ( 'NONE',  ( -10.72451020669898014, 18.67979575497178502, 50.41557627198103120 ) ) ;
#56044=CARTESIAN_POINT ( 'NONE',  ( -14.34966873604960291, -8.224510206698953496, 51.66557627198102409 ) ) ;
#56045=CARTESIAN_POINT ( 'NONE',  ( 21.53943276465977519, 0.05219959533937863772, 106.2510903946856757 ) ) ;
#56046=CARTESIAN_POINT ( 'NONE',  ( 5.049401038298161559, -19.05341960407611168, 102.7072429386476955 ) ) ;
#56047=CARTESIAN_POINT ( 'NONE',  ( -19.05341960407611168, -5.049401038298163336, 111.4572429386476671 ) ) ;
#56048=CARTESIAN_POINT ( 'NONE',  ( 16.46253265017160672, -9.564922557960803928, 33.33224293864770260 ) ) ;
#56049=CARTESIAN_POINT ( 'NONE',  ( -5.153800228976328057, -19.02544592524343514, 27.29057627198103120 ) ) ;
#56050=CARTESIAN_POINT ( 'NONE',  ( -16.53943276465976808, 0.05219959533911058130, 81.24890960531436690 ) ) ;
#56051=CARTESIAN_POINT ( 'NONE',  ( -15.80617190586745835, -15.72974639402198527, 96.87390960531436690 ) ) ;
#56052=CARTESIAN_POINT ( 'NONE',  ( -19.02544592524342804, 5.153800228976336051, 96.04057627198103830 ) ) ;
#56053=CARTESIAN_POINT ( 'NONE',  ( 18.62759615963271287, -10.81492255796078972, 108.3322429386477097 ) ) ;
#56054=CARTESIAN_POINT ( 'NONE',  ( 16.51473224551069308, 9.474510206698969483, 89.16557627198103830 ) ) ;
#56056=CARTESIAN_POINT ( 'NONE',  ( -4.379528057220328563, 16.55341960407611168, 105.2072429386477097 ) ) ;
#56057=CARTESIAN_POINT ( 'NONE',  ( -19.05341960407611168, -5.049401038298163336, 76.45724293864769550 ) ) ;
#56058=CARTESIAN_POINT ( 'NONE',  ( 10.81492255796078972, 18.62759615963270932, 74.58224293864768129 ) ) ;
#56061=CARTESIAN_POINT ( 'NONE',  ( -18.62759615963270932, 10.81492255796079327, 30.83224293864770260 ) ) ;
#56063=CARTESIAN_POINT ( 'NONE',  ( 0.05219959533934541429, -16.53943276465976808, 40.00109039468567573 ) ) ;
#56064=CARTESIAN_POINT ( 'NONE',  ( 14.34966873604960469, 8.224510206698951720, 89.16557627198102409 ) ) ;
#56065=CARTESIAN_POINT ( 'NONE',  ( -17.49999999999999645, -5.076555817581227537, 111.1795149204977804 ) ) ;
#56066=CARTESIAN_POINT ( 'NONE',  ( -9.474510206698964154, 16.51473224551069663, 85.41557627198102409 ) ) ;
#56067=CARTESIAN_POINT ( 'NONE',  ( -13.97604488694527625, -13.89961937509977652, 51.87390960531436690 ) ) ;
#56068=CARTESIAN_POINT ( 'NONE',  ( -4.483927247898539470, -16.52544592524342804, 77.29057627198102409 ) ) ;
#56070=CARTESIAN_POINT ( 'NONE',  ( -5.719274019375978568, 21.55341960407610458, 35.20724293864768839 ) ) ;
#56071=CARTESIAN_POINT ( 'NONE',  ( -16.53943276465976808, 0.05219959533911058130, 56.24890960531436690 ) ) ;
#56072=CARTESIAN_POINT ( 'NONE',  ( -16.51473224551082808, 9.474510206698731452, 98.33442372801900433 ) ) ;
#56073=CARTESIAN_POINT ( 'NONE',  ( 5.823673210054444382, -21.52544592524334988, 70.20942372801904696 ) ) ;
#56075=CARTESIAN_POINT ( 'NONE',  ( -0.05219959533907301413, -21.53943276465977519, 22.49890960531436335 ) ) ;
#56076=CARTESIAN_POINT ( 'NONE',  ( -12.14591786802326823, 12.06949235617739902, 88.12609039468570415 ) ) ;
#56077=CARTESIAN_POINT ( 'NONE',  ( 13.89961937509977652, -13.97604488694527269, 23.12390960531436335 ) ) ;
#56078=CARTESIAN_POINT ( 'NONE',  ( 5.153800228976335163, 19.02544592524342804, 69.79057627198103830 ) ) ;
#56079=CARTESIAN_POINT ( 'NONE',  ( 10.81492255796078972, 18.62759615963270932, 79.58224293864769550 ) ) ;
#56080=CARTESIAN_POINT ( 'NONE',  ( 14.34966873604972726, -8.224510206698740333, 30.83442372801902209 ) ) ;
#56081=CARTESIAN_POINT ( 'NONE',  ( 0.05219959533910956823, 16.53943276465976808, 54.99890960531435269 ) ) ;
#56082=CARTESIAN_POINT ( 'NONE',  ( -15.80617190586768217, 15.72974639402176855, 68.12609039468567573 ) ) ;
#56083=CARTESIAN_POINT ( 'NONE',  ( 12.06949235617739724, 12.14591786802326823, 91.87609039468568994 ) ) ;
#56084=CARTESIAN_POINT ( 'NONE',  ( 13.89961937509977652, -13.97604488694527269, 113.1239096053143527 ) ) ;
#56087=CARTESIAN_POINT ( 'NONE',  ( -8.314922557961024197, 14.29746914071037800, 102.9177570613523756 ) ) ;
#56088=CARTESIAN_POINT ( 'NONE',  ( 16.55341960407618274, -4.379528057220086978, 61.04275706135234714 ) ) ;
#56089=CARTESIAN_POINT ( 'NONE',  ( -16.46253265017160317, 9.564922557960807481, 65.83224293864769550 ) ) ;
#56090=CARTESIAN_POINT ( 'NONE',  ( -16.46253265017160317, 9.564922557960807481, 85.83224293864769550 ) ) ;
#56091=CARTESIAN_POINT ( 'NONE',  ( 5.719274019375673035, 21.55341960407619339, 67.29275706135234714 ) ) ;
#56092=CARTESIAN_POINT ( 'NONE',  ( 14.29746914071037800, 8.314922557961029526, 76.66775706135234714 ) ) ;
#56093=CARTESIAN_POINT ( 'NONE',  ( -8.314922557960811034, -14.29746914071050412, 47.08224293864770260 ) ) ;
#56094=CARTESIAN_POINT ( 'NONE',  ( 5.153800228976335163, 19.02544592524342804, 49.79057627198100988 ) ) ;
#56095=CARTESIAN_POINT ( 'NONE',  ( 9.474510206698971260, -16.51473224551069308, 47.91557627198102409 ) ) ;
#56097=CARTESIAN_POINT ( 'NONE',  ( -19.05341960407617563, 5.049401038297882671, 98.54275706135233293 ) ) ;
#56098=CARTESIAN_POINT ( 'NONE',  ( -14.29746914071049879, 8.314922557960819915, 110.8322429386476955 ) ) ;
#56099=CARTESIAN_POINT ( 'NONE',  ( 5.153800228976335163, 19.02544592524342804, 69.79057627198103830 ) ) ;
#56100=CARTESIAN_POINT ( 'NONE',  ( -5.049401038297874678, -19.05341960407617918, 94.79275706135230450 ) ) ;
#56102=CARTESIAN_POINT ( 'NONE',  ( 5.823673210054444382, -21.52544592524334988, 100.2094237280190043 ) ) ;
#56103=CARTESIAN_POINT ( 'NONE',  ( 14.29746914071037800, 8.314922557961029526, 66.66775706135234714 ) ) ;
#56104=CARTESIAN_POINT ( 'NONE',  ( -5.049401038297874678, -19.05341960407617918, 89.79275706135230450 ) ) ;
#56105=CARTESIAN_POINT ( 'NONE',  ( 5.719274019375991003, -21.55341960407610458, 57.70724293864770260 ) ) ;
#56106=CARTESIAN_POINT ( 'NONE',  ( -12.14591786802326823, 12.06949235617739902, 48.12609039468568284 ) ) ;
#56108=CARTESIAN_POINT ( 'NONE',  ( 0.05219959533936267826, -19.03943276465977164, 55.00109039468566863 ) ) ;
#56109=CARTESIAN_POINT ( 'NONE',  ( -0.05219959533937732626, 21.53943276465977519, 97.50109039468567573 ) ) ;
#56110=CARTESIAN_POINT ( 'NONE',  ( -9.474510206698964154, 16.51473224551069663, 25.41557627198103120 ) ) ;
#56111=CARTESIAN_POINT ( 'NONE',  ( 16.51473224551069308, 9.474510206698969483, 64.16557627198102409 ) ) ;
#56112=CARTESIAN_POINT ( 'NONE',  ( -16.55341960407611168, -4.379528057220339221, 56.45724293864768839 ) ) ;
#56113=CARTESIAN_POINT ( 'NONE',  ( -10.72451020669870658, -18.67979575497194134, 89.58442372801901854 ) ) ;
#56114=CARTESIAN_POINT ( 'NONE',  ( 5.153800228976615827, -19.02544592524334988, 45.20942372801901143 ) ) ;
#56115=CARTESIAN_POINT ( 'NONE',  ( 16.51473224551083163, -9.474510206698727899, 25.83442372801900078 ) ) ;
#56116=CARTESIAN_POINT ( 'NONE',  ( -10.81492255796078084, -18.62759615963271287, 22.08224293864769194 ) ) ;
#56117=CARTESIAN_POINT ( 'NONE',  ( 5.823673210054444382, -21.52544592524334988, 100.2094237280190043 ) ) ;
#56118=CARTESIAN_POINT ( 'NONE',  ( 19.05341960407611168, 5.049401038298154454, 73.95724293864768129 ) ) ;
#56120=CARTESIAN_POINT ( 'NONE',  ( -21.53943276465977519, -0.05219959533937600094, 93.75109039468567573 ) ) ;
#56121=CARTESIAN_POINT ( 'NONE',  ( -5.823673210054116645, -21.52544592524344225, 52.29057627198102409 ) ) ;
#56122=CARTESIAN_POINT ( 'NONE',  ( -5.153800228976328057, -19.02544592524343514, 77.29057627198099567 ) ) ;
#56123=CARTESIAN_POINT ( 'NONE',  ( 16.46253265017146816, 9.564922557961045513, 71.66775706135233293 ) ) ;
#56124=CARTESIAN_POINT ( 'NONE',  ( -0.05219959533909027116, -19.03943276465977164, 37.49890960531436690 ) ) ;
#56125=CARTESIAN_POINT ( 'NONE',  ( 16.46253265017160672, -9.564922557960803928, 83.33224293864768129 ) ) ;
#56126=CARTESIAN_POINT ( 'NONE',  ( -5.049401038297874678, -19.05341960407617918, 84.79275706135233293 ) ) ;
#56127=CARTESIAN_POINT ( 'NONE',  ( -12.06949235617739369, -12.14591786802326823, 49.37609039468569705 ) ) ;
#56128=CARTESIAN_POINT ( 'NONE',  ( -4.483927247898539470, -16.52544592524342804, 102.2905762719810383 ) ) ;
#56129=CARTESIAN_POINT ( 'NONE',  ( -0.05219959533909027116, -19.03943276465977164, 67.49890960531436690 ) ) ;
#56130=CARTESIAN_POINT ( 'NONE',  ( 18.67979575497178502, 10.72451020669898547, 54.16557627198103120 ) ) ;
#56131=CARTESIAN_POINT ( 'NONE',  ( 4.379528057220092307, 16.55341960407617563, 22.29275706135235069 ) ) ;
#56132=CARTESIAN_POINT ( 'NONE',  ( 0.05219959533937995610, -21.53943276465977519, 30.00109039468568284 ) ) ;
#56133=CARTESIAN_POINT ( 'NONE',  ( -5.719274019375665041, -21.55341960407619695, 84.79275706135234714 ) ) ;
#56134=CARTESIAN_POINT ( 'NONE',  ( -16.55341960407617563, 4.379528057220093196, 88.54275706135236135 ) ) ;
#56136=CARTESIAN_POINT ( 'NONE',  ( 9.474510206698971260, -16.51473224551069308, 72.91557627198102409 ) ) ;
#56137=CARTESIAN_POINT ( 'NONE',  ( 0.05219959533934541429, -16.53943276465976808, 105.0010903946856757 ) ) ;
#56138=CARTESIAN_POINT ( 'NONE',  ( 16.51473224551083163, -9.474510206698727899, 50.83442372801899722 ) ) ;
#56139=CARTESIAN_POINT ( 'NONE',  ( -10.72451020669870658, -18.67979575497194134, 24.58442372801901499 ) ) ;
#56140=CARTESIAN_POINT ( 'NONE',  ( -16.52544592524342804, 4.483927247898546575, 76.04057627198102409 ) ) ;
#56141=CARTESIAN_POINT ( 'NONE',  ( 16.46253265017160672, -9.564922557960803928, 93.33224293864769550 ) ) ;
#56142=CARTESIAN_POINT ( 'NONE',  ( -0.05219959533934338120, 16.53943276465976808, 102.5010903946856899 ) ) ;
#56143=CARTESIAN_POINT ( 'NONE',  ( 5.719274019375673035, 21.55341960407619339, 72.29275706135236135 ) ) ;
#56144=CARTESIAN_POINT ( 'NONE',  ( -16.52544592524335698, -4.483927247898792601, 33.95942372801901143 ) ) ;
#56145=CARTESIAN_POINT ( 'NONE',  ( -10.72451020669870658, -18.67979575497194134, 24.58442372801901499 ) ) ;
#56146=CARTESIAN_POINT ( 'NONE',  ( 4.379528057220339221, -16.55341960407611168, 67.70724293864769550 ) ) ;
#56148=CARTESIAN_POINT ( 'NONE',  ( -21.53943276465977519, 0.05219959533907696930, 101.2489096053143669 ) ) ;
#56149=CARTESIAN_POINT ( 'NONE',  ( 14.29746914071049879, -8.314922557960816363, 58.33224293864768839 ) ) ;
#56150=CARTESIAN_POINT ( 'NONE',  ( -9.564922557960796823, -16.46253265017161027, 32.08224293864769550 ) ) ;
#56151=CARTESIAN_POINT ( 'NONE',  ( 18.67979575497178502, 10.72451020669898547, 29.16557627198103120 ) ) ;
#56152=CARTESIAN_POINT ( 'NONE',  ( -10.72451020669870658, -18.67979575497194134, 44.58442372801901854 ) ) ;
#56153=CARTESIAN_POINT ( 'NONE',  ( 12.14591786802309770, 12.06949235617756955, 59.37390960531436690 ) ) ;
#56155=CARTESIAN_POINT ( 'NONE',  ( -15.80617190586745835, -15.72974639402198527, 61.87390960531436690 ) ) ;
#56156=CARTESIAN_POINT ( 'NONE',  ( 5.153800228976335163, 19.02544592524342804, 69.79057627198103830 ) ) ;
#56157=CARTESIAN_POINT ( 'NONE',  ( 16.51473224551069308, 9.474510206698969483, 24.16557627198102765 ) ) ;
#56158=CARTESIAN_POINT ( 'NONE',  ( -19.03943276465977164, -0.05219959533935918106, 83.75109039468567573 ) ) ;
#56159=CARTESIAN_POINT ( 'NONE',  ( -21.52544592524334988, -5.823673210054445271, 53.95942372801900433 ) ) ;
#56160=CARTESIAN_POINT ( 'NONE',  ( -21.53943276465977519, 0.05219959533907696930, 56.24890960531436690 ) ) ;
#56161=CARTESIAN_POINT ( 'NONE',  ( -5.153800228976328057, -19.02544592524343514, 42.29057627198101699 ) ) ;
#56162=CARTESIAN_POINT ( 'NONE',  ( 16.51473224551069308, 9.474510206698969483, 69.16557627198102409 ) ) ;
#56164=CARTESIAN_POINT ( 'NONE',  ( 8.314922557961029526, -14.29746914071037800, 50.41775706135235424 ) ) ;
#56165=CARTESIAN_POINT ( 'NONE',  ( 15.72974639402176855, 15.80617190586768217, 36.87609039468568994 ) ) ;
#56166=CARTESIAN_POINT ( 'NONE',  ( 15.80617190586769283, -15.72974639402175789, 60.62609039468567573 ) ) ;
#56167=CARTESIAN_POINT ( 'NONE',  ( -13.89961937509977652, 13.97604488694528158, 105.6239096053143527 ) ) ;
#56168=CARTESIAN_POINT ( 'NONE',  ( -21.53943276465977519, 0.05219959533907696930, 86.24890960531436690 ) ) ;
#56169=CARTESIAN_POINT ( 'NONE',  ( -5.823673210054431948, 21.52544592524334988, 27.70942372801901854 ) ) ;
#56170=CARTESIAN_POINT ( 'NONE',  ( 16.53943276465976808, 0.05219959533934440121, 56.25109039468568284 ) ) ;
#56171=CARTESIAN_POINT ( 'NONE',  ( 0.05219959533907565091, 21.53943276465977519, 54.99890960531435269 ) ) ;
#56172=CARTESIAN_POINT ( 'NONE',  ( -10.72451020669870658, -18.67979575497194134, 109.5844237280190328 ) ) ;
#56173=CARTESIAN_POINT ( 'NONE',  ( 19.02544592524343514, -5.153800228976328945, 58.54057627198102409 ) ) ;
#56174=CARTESIAN_POINT ( 'NONE',  ( 5.049401038298161559, -19.05341960407611168, 112.7072429386476813 ) ) ;
#56175=CARTESIAN_POINT ( 'NONE',  ( 19.02544592524343514, -5.153800228976328945, 83.54057627198100988 ) ) ;
#56177=CARTESIAN_POINT ( 'NONE',  ( -13.89961937509957401, -13.97604488694547875, 69.37609039468564731 ) ) ;
#56178=CARTESIAN_POINT ( 'NONE',  ( 15.72974639402199770, -15.80617190586745480, 43.12390960531435269 ) ) ;
#56179=CARTESIAN_POINT ( 'NONE',  ( 4.483927247898545687, 16.52544592524342804, 29.79057627198102409 ) ) ;
#56180=CARTESIAN_POINT ( 'NONE',  ( 19.03943276465977164, 0.05219959533936151252, 86.25109039468567573 ) ) ;
#56181=CARTESIAN_POINT ( 'NONE',  ( -17.40861289039003523, 6.110651285853257342, 58.62767529172568004 ) ) ;
#56182=CARTESIAN_POINT ( 'NONE',  ( -5.719274019375665041, -21.55341960407619695, 109.7927570613523613 ) ) ;
#56183=CARTESIAN_POINT ( 'NONE',  ( 19.03943276465977164, 0.05219959533936151252, 81.25109039468567573 ) ) ;
#56184=CARTESIAN_POINT ( 'NONE',  ( -19.05341960407617563, 5.049401038297882671, 43.54275706135232582 ) ) ;
#56187=CARTESIAN_POINT ( 'NONE',  ( 5.049401038298161559, -19.05341960407611168, 52.70724293864767418 ) ) ;
#56188=CARTESIAN_POINT ( 'NONE',  ( 4.483927247898545687, 16.52544592524342804, 44.79057627198103120 ) ) ;
#56189=CARTESIAN_POINT ( 'NONE',  ( 13.89961937509977652, -13.97604488694527269, 38.12390960531436690 ) ) ;
#56190=CARTESIAN_POINT ( 'NONE',  ( -12.14591786802309592, -12.06949235617757132, 41.87390960531435979 ) ) ;
#56192=CARTESIAN_POINT ( 'NONE',  ( 4.379528057220092307, 16.55341960407617563, 112.2927570613523471 ) ) ;
#56193=CARTESIAN_POINT ( 'NONE',  ( -5.153800228976328057, -19.02544592524343514, 47.29057627198102409 ) ) ;
#56194=CARTESIAN_POINT ( 'NONE',  ( 5.153800228976615827, -19.02544592524334988, 30.20942372801900433 ) ) ;
#56195=CARTESIAN_POINT ( 'NONE',  ( -12.14591786802326823, 12.06949235617739902, 33.12609039468569705 ) ) ;
#56196=CARTESIAN_POINT ( 'NONE',  ( -10.72451020669898014, 18.67979575497178502, 40.41557627198103120 ) ) ;
#56197=CARTESIAN_POINT ( 'NONE',  ( -10.81492255796105439, 18.62759615963255655, 97.91775706135236135 ) ) ;
#56199=CARTESIAN_POINT ( 'NONE',  ( -16.51473224551069308, -9.474510206698971260, 61.66557627198103120 ) ) ;
#56200=CARTESIAN_POINT ( 'NONE',  ( 13.89961937509977652, -13.97604488694527269, 103.1239096053143527 ) ) ;
#56201=CARTESIAN_POINT ( 'NONE',  ( -13.89961937509977652, 13.97604488694528158, 95.62390960531436690 ) ) ;
#56203=CARTESIAN_POINT ( 'NONE',  ( 5.823673210054444382, -21.52544592524334988, 20.20942372801900788 ) ) ;
#56204=CARTESIAN_POINT ( 'NONE',  ( -12.06949235617756955, 12.14591786802309770, 75.62390960531439532 ) ) ;
#56205=CARTESIAN_POINT ( 'NONE',  ( -21.52544592524343514, 5.823673210054127303, 71.04057627198103830 ) ) ;
#56206=CARTESIAN_POINT ( 'NONE',  ( 5.153800228976335163, 19.02544592524342804, 74.79057627198103830 ) ) ;
#56207=CARTESIAN_POINT ( 'NONE',  ( -9.474510206698964154, 16.51473224551069663, 75.41557627198103830 ) ) ;
#56208=CARTESIAN_POINT ( 'NONE',  ( -21.52544592524343514, 5.823673210054127303, 106.0405762719810525 ) ) ;
#56209=EDGE_CURVE ( 'NONE', #11669, #184472, #121901, .T. ) ;
#56210=VERTEX_POINT ( 'NONE', #131296 ) ;
#56211=CARTESIAN_POINT ( 'NONE',  ( 16.51473224551069308, 9.474510206698969483, 79.16557627198103830 ) ) ;
#56213=CARTESIAN_POINT ( 'NONE',  ( -14.29746914071049879, 8.314922557960819915, 100.8322429386477097 ) ) ;
#56214=CARTESIAN_POINT ( 'NONE',  ( -19.05341960407611168, -5.049401038298163336, 21.45724293864768839 ) ) ;
#56215=CARTESIAN_POINT ( 'NONE',  ( 16.51473224551069308, 9.474510206698969483, 59.16557627198102409 ) ) ;
#56216=CARTESIAN_POINT ( 'NONE',  ( 0.05219959533936267826, -19.03943276465977164, 95.00109039468567573 ) ) ;
#56217=CARTESIAN_POINT ( 'NONE',  ( -12.14591786802309592, -12.06949235617757132, 101.8739096053143811 ) ) ;
#56218=CARTESIAN_POINT ( 'NONE',  ( -10.81492255796105439, 18.62759615963255655, 72.91775706135234714 ) ) ;
#56219=CARTESIAN_POINT ( 'NONE',  ( 19.03943276465977164, -0.05219959533909143690, 43.74890960531435979 ) ) ;
#56220=CARTESIAN_POINT ( 'NONE',  ( 0.05219959533907565091, 21.53943276465977519, 114.9989096053143669 ) ) ;
#56221=CARTESIAN_POINT ( 'NONE',  ( -8.224510206698948167, 14.34966873604960824, 105.4155762719810383 ) ) ;
#56223=CARTESIAN_POINT ( 'NONE',  ( -13.97604488694527625, -13.89961937509977652, 76.87390960531433848 ) ) ;
#56224=LINE ( 'NONE', #102730, #124398 ) ;
#56225=CARTESIAN_POINT ( 'NONE',  ( 19.02544592524334988, 5.153800228976608722, 111.4594237280190043 ) ) ;
#56226=CARTESIAN_POINT ( 'NONE',  ( -0.05219959533907301413, -21.53943276465977519, 32.49890960531435979 ) ) ;
#56227=CARTESIAN_POINT ( 'NONE',  ( 10.81492255796106328, -18.62759615963255655, 55.41775706135234714 ) ) ;
#56228=CARTESIAN_POINT ( 'NONE',  ( -5.049401038298153566, 19.05341960407611168, 90.20724293864766707 ) ) ;
#56229=CARTESIAN_POINT ( 'NONE',  ( 9.474510206698729675, 16.51473224551082808, 87.08442372801900433 ) ) ;
#56230=CARTESIAN_POINT ( 'NONE',  ( 19.02544592524343514, -5.153800228976328945, 68.54057627198103830 ) ) ;
#56231=CARTESIAN_POINT ( 'NONE',  ( 14.29746914071049879, -8.314922557960816363, 78.33224293864770971 ) ) ;
#56232=CARTESIAN_POINT ( 'NONE',  ( -19.05341960407611168, -5.049401038298163336, 101.4572429386476955 ) ) ;
#56233=CARTESIAN_POINT ( 'NONE',  ( 12.06949235617757843, -12.14591786802309237, 73.12390960531436690 ) ) ;
#56234=CARTESIAN_POINT ( 'NONE',  ( 5.049401038298161559, -19.05341960407611168, 97.70724293864766707 ) ) ;
#56236=CARTESIAN_POINT ( 'NONE',  ( -19.05341960407611168, -5.049401038298163336, 56.45724293864768129 ) ) ;
#56237=CARTESIAN_POINT ( 'NONE',  ( 0.05219959533910956823, 16.53943276465976808, 49.99890960531437401 ) ) ;
#56238=CARTESIAN_POINT ( 'NONE',  ( 19.05341960407611168, 5.049401038298154454, 33.95724293864769550 ) ) ;
#56240=CARTESIAN_POINT ( 'NONE',  ( -18.67979575497193778, 10.72451020669871902, 63.33442372801900433 ) ) ;
#56241=CARTESIAN_POINT ( 'NONE',  ( -9.474510206698720793, -16.51473224551083518, 84.58442372801900433 ) ) ;
#56242=CARTESIAN_POINT ( 'NONE',  ( 8.224510206698953496, -14.34966873604960469, 52.91557627198103830 ) ) ;
#56243=CARTESIAN_POINT ( 'NONE',  ( 15.72974639402199770, -15.80617190586745480, 98.12390960531436690 ) ) ;
#56244=CARTESIAN_POINT ( 'NONE',  ( -21.55341960407610458, -5.719274019375992779, 36.45724293864768839 ) ) ;
#56245=CARTESIAN_POINT ( 'NONE',  ( -0.05219959533910754901, -16.53943276465976808, 82.49890960531436690 ) ) ;
#56246=CARTESIAN_POINT ( 'NONE',  ( 16.51473224551069308, 9.474510206698969483, 49.16557627198102409 ) ) ;
#56247=CARTESIAN_POINT ( 'NONE',  ( -16.53943276465976808, -0.05219959533934237506, 113.7510903946856757 ) ) ;
#56248=CARTESIAN_POINT ( 'NONE',  ( -8.314922557961024197, 14.29746914071037800, 92.91775706135236135 ) ) ;
#56249=CARTESIAN_POINT ( 'NONE',  ( 16.55341960407618274, -4.379528057220086978, 76.04275706135237556 ) ) ;
#56250=CARTESIAN_POINT ( 'NONE',  ( 16.51473224551083163, -9.474510206698727899, 30.83442372801900433 ) ) ;
#56251=CARTESIAN_POINT ( 'NONE',  ( -16.51473224551069308, -9.474510206698971260, 86.66557627198102409 ) ) ;
#56252=CARTESIAN_POINT ( 'NONE',  ( 19.02544592524343514, -5.153800228976328945, 83.54057627198100988 ) ) ;
#56253=CARTESIAN_POINT ( 'NONE',  ( -8.224510206698735004, -14.34966873604973081, 89.58442372801901854 ) ) ;
#56254=CARTESIAN_POINT ( 'NONE',  ( 13.89961937509977652, -13.97604488694527269, 43.12390960531434558 ) ) ;
#56255=CARTESIAN_POINT ( 'NONE',  ( -16.55341960407611168, -4.379528057220339221, 46.45724293864769550 ) ) ;
#56256=CARTESIAN_POINT ( 'NONE',  ( -9.474510206698964154, 16.51473224551069663, 110.4155762719810383 ) ) ;
#56257=CARTESIAN_POINT ( 'NONE',  ( -5.719274019375978568, 21.55341960407610458, 25.20724293864769550 ) ) ;
#56258=CARTESIAN_POINT ( 'NONE',  ( 16.52544592524342804, -4.483927247898539470, 73.54057627198102409 ) ) ;
#56259=CARTESIAN_POINT ( 'NONE',  ( -16.53943276465976808, 0.05219959533911058130, 71.24890960531435269 ) ) ;
#56260=CARTESIAN_POINT ( 'NONE',  ( 18.10062525802554134, -5.500000000000022204, 86.01383468041923663 ) ) ;
#56262=CARTESIAN_POINT ( 'NONE',  ( -9.564922557961040184, 16.46253265017147172, 57.91775706135233293 ) ) ;
#56263=CARTESIAN_POINT ( 'NONE',  ( 16.46253265017160672, -9.564922557960803928, 98.33224293864769550 ) ) ;
#56264=CARTESIAN_POINT ( 'NONE',  ( -19.02544592524334988, -5.153800228976617603, 78.95942372801900433 ) ) ;
#56266=CARTESIAN_POINT ( 'NONE',  ( 16.51473224551083163, -9.474510206698727899, 105.8344237280190043 ) ) ;
#56267=CARTESIAN_POINT ( 'NONE',  ( 8.224510206698742110, 14.34966873604972548, 92.08442372801901854 ) ) ;
#56268=CARTESIAN_POINT ( 'NONE',  ( 16.51473224551069308, 9.474510206698969483, 34.16557627198102409 ) ) ;
#56269=CARTESIAN_POINT ( 'NONE',  ( -5.719274019375978568, 21.55341960407610458, 40.20724293864769550 ) ) ;
#56270=CARTESIAN_POINT ( 'NONE',  ( 21.55341960407619695, -5.719274019375665929, 61.04275706135234714 ) ) ;
#56271=CARTESIAN_POINT ( 'NONE',  ( -16.51473224551082808, 9.474510206698731452, 113.3344237280190043 ) ) ;
#56272=FACE_OUTER_BOUND ( 'NONE', #20010, .T. ) ;
#56273=CARTESIAN_POINT ( 'NONE',  ( 19.03943276465977164, -0.05219959533909143690, 78.74890960531436690 ) ) ;
#56274=CARTESIAN_POINT ( 'NONE',  ( 9.564922557960805705, 16.46253265017160317, 114.5822429386476955 ) ) ;
#56275=CARTESIAN_POINT ( 'NONE',  ( 14.34966873604960469, 8.224510206698951720, 74.16557627198102409 ) ) ;
#56276=CARTESIAN_POINT ( 'NONE',  ( -19.02544592524342804, 5.153800228976336051, 71.04057627198099567 ) ) ;
#56278=CARTESIAN_POINT ( 'NONE',  ( 19.02544592524343514, -5.153800228976328945, 88.54057627198102409 ) ) ;
#56280=CARTESIAN_POINT ( 'NONE',  ( -13.89961937509957401, -13.97604488694547875, 89.37609039468563310 ) ) ;
#56281=CARTESIAN_POINT ( 'NONE',  ( 21.53943276465977519, -0.05219959533907433946, 63.74890960531435979 ) ) ;
#56282=CARTESIAN_POINT ( 'NONE',  ( -16.51473224551069308, -9.474510206698971260, 31.66557627198102054 ) ) ;
#56283=CARTESIAN_POINT ( 'NONE',  ( 16.46253265017146816, 9.564922557961045513, 61.66775706135234003 ) ) ;
#56284=CARTESIAN_POINT ( 'NONE',  ( 0.05219959533909260263, 19.03943276465977164, 59.99890960531436690 ) ) ;
#56285=CARTESIAN_POINT ( 'NONE',  ( -0.05219959533909027116, -19.03943276465977164, 97.49890960531436690 ) ) ;
#56287=CARTESIAN_POINT ( 'NONE',  ( 15.72974639402199770, -15.80617190586745480, 93.12390960531436690 ) ) ;
#56288=CARTESIAN_POINT ( 'NONE',  ( -16.53943276465976808, 0.05219959533911058130, 96.24890960531435269 ) ) ;
#56289=CARTESIAN_POINT ( 'NONE',  ( -0.05219959533936034679, 19.03943276465977164, 52.50109039468566863 ) ) ;
#56290=CARTESIAN_POINT ( 'NONE',  ( -21.52544592524343514, 5.823673210054127303, 86.04057627198102409 ) ) ;
#56291=CARTESIAN_POINT ( 'NONE',  ( 21.53943276465977519, -0.05219959533907433946, 68.74890960531435269 ) ) ;
#56292=CARTESIAN_POINT ( 'NONE',  ( -14.34966873604960291, -8.224510206698953496, 26.66557627198103475 ) ) ;
#56293=CARTESIAN_POINT ( 'NONE',  ( -15.72974639402176322, -15.80617190586768395, 104.3760903946856899 ) ) ;
#56294=CARTESIAN_POINT ( 'NONE',  ( -14.34966873604972548, 8.224510206698743886, 48.33442372801902565 ) ) ;
#56295=CARTESIAN_POINT ( 'NONE',  ( 13.89961937509977652, -13.97604488694527269, 78.12390960531433848 ) ) ;
#56296=CARTESIAN_POINT ( 'NONE',  ( -16.46253265017160317, 9.564922557960807481, 25.83224293864769194 ) ) ;
#56298=CARTESIAN_POINT ( 'NONE',  ( -15.72974639402176322, -15.80617190586768395, 44.37609039468567573 ) ) ;
#56299=CARTESIAN_POINT ( 'NONE',  ( 21.53943276465977519, 0.05219959533937863772, 56.25109039468568284 ) ) ;
#56300=CARTESIAN_POINT ( 'NONE',  ( -13.97604488694527625, -13.89961937509977652, 41.87390960531435979 ) ) ;
#56301=CARTESIAN_POINT ( 'NONE',  ( -21.52544592524343514, 5.823673210054127303, 116.0405762719810383 ) ) ;
#56302=CARTESIAN_POINT ( 'NONE',  ( 5.049401038297881783, 19.05341960407617563, 67.29275706135234714 ) ) ;
#56303=CARTESIAN_POINT ( 'NONE',  ( -19.03943276465977164, -0.05219959533935918106, 78.75109039468567573 ) ) ;
#56304=CARTESIAN_POINT ( 'NONE',  ( 4.379528057220092307, 16.55341960407617563, 27.29275706135234358 ) ) ;
#56305=CARTESIAN_POINT ( 'NONE',  ( 19.02544592524343514, -5.153800228976328945, 28.54057627198102409 ) ) ;
#56306=CARTESIAN_POINT ( 'NONE',  ( -8.314922557961024197, 14.29746914071037800, 77.91775706135231871 ) ) ;
#56307=CARTESIAN_POINT ( 'NONE',  ( -9.474510206698964154, 16.51473224551069663, 40.41557627198103120 ) ) ;
#56309=CARTESIAN_POINT ( 'NONE',  ( 13.97604488694527802, 13.89961937509977652, 104.3739096053143385 ) ) ;
#56310=CARTESIAN_POINT ( 'NONE',  ( -13.89961937509977652, 13.97604488694528158, 25.62390960531434558 ) ) ;
#56311=CARTESIAN_POINT ( 'NONE',  ( 0.05219959533907565091, 21.53943276465977519, 69.99890960531435269 ) ) ;
#56312=CARTESIAN_POINT ( 'NONE',  ( -16.52544592524335698, -4.483927247898792601, 58.95942372801902565 ) ) ;
#56313=CARTESIAN_POINT ( 'NONE',  ( 13.89961937509957401, 13.97604488694547697, 21.87609039468566152 ) ) ;
#56315=CARTESIAN_POINT ( 'NONE',  ( -19.02544592524342804, 5.153800228976336051, 41.04057627198103120 ) ) ;
#56316=CARTESIAN_POINT ( 'NONE',  ( -4.483927247898539470, -16.52544592524342804, 37.29057627198102409 ) ) ;
#56317=CARTESIAN_POINT ( 'NONE',  ( 16.53943276465976808, -0.05219959533910856209, 63.74890960531435979 ) ) ;
#56318=CARTESIAN_POINT ( 'NONE',  ( 13.97604488694527802, 13.89961937509977652, 69.37390960531436690 ) ) ;
#56319=CARTESIAN_POINT ( 'NONE',  ( -10.81492255796105439, 18.62759615963255655, 32.91775706135234714 ) ) ;
#56320=CARTESIAN_POINT ( 'NONE',  ( -9.474510206698964154, 16.51473224551069663, 75.41557627198103830 ) ) ;
#56321=CARTESIAN_POINT ( 'NONE',  ( 18.62759615963255655, 10.81492255796105972, 81.66775706135236135 ) ) ;
#56322=CARTESIAN_POINT ( 'NONE',  ( 14.29746914071037800, 8.314922557961029526, 71.66775706135234714 ) ) ;
#56323=CARTESIAN_POINT ( 'NONE',  ( 5.049401038298161559, -19.05341960407611168, 112.7072429386476813 ) ) ;
#56325=CARTESIAN_POINT ( 'NONE',  ( -16.55341960407611168, -4.379528057220339221, 31.45724293864769550 ) ) ;
#56326=CARTESIAN_POINT ( 'NONE',  ( 9.474510206698971260, -16.51473224551069308, 32.91557627198102409 ) ) ;
#56327=CARTESIAN_POINT ( 'NONE',  ( 12.14591786802327356, -12.06949235617739191, 55.62609039468568284 ) ) ;
#56328=CARTESIAN_POINT ( 'NONE',  ( -14.34966873604960291, -8.224510206698953496, 51.66557627198102409 ) ) ;
#56329=CARTESIAN_POINT ( 'NONE',  ( -13.97604488694527625, -13.89961937509977652, 106.8739096053143669 ) ) ;
#56330=CARTESIAN_POINT ( 'NONE',  ( 0.05219959533907565091, 21.53943276465977519, 29.99890960531435979 ) ) ;
#56331=CARTESIAN_POINT ( 'NONE',  ( -5.823673210054431948, 21.52544592524334988, 107.7094237280190328 ) ) ;
#56332=CARTESIAN_POINT ( 'NONE',  ( 4.483927247898545687, 16.52544592524342804, 89.79057627198103830 ) ) ;
#56333=CARTESIAN_POINT ( 'NONE',  ( 9.474510206698971260, -16.51473224551069308, 97.91557627198102409 ) ) ;
#56335=CARTESIAN_POINT ( 'NONE',  ( -14.29746914071037622, -8.314922557961029526, 59.16775706135234714 ) ) ;
#56336=CARTESIAN_POINT ( 'NONE',  ( 19.05341960407611168, 5.049401038298154454, 53.95724293864770260 ) ) ;
#56338=CARTESIAN_POINT ( 'NONE',  ( -16.46253265017146816, -9.564922557961047289, 44.16775706135232582 ) ) ;
#56339=CARTESIAN_POINT ( 'NONE',  ( 14.34966873604972726, -8.224510206698740333, 85.83442372801901854 ) ) ;
#56340=CARTESIAN_POINT ( 'NONE',  ( 9.474510206698729675, 16.51473224551082808, 97.08442372801900433 ) ) ;
#56341=CARTESIAN_POINT ( 'NONE',  ( 21.55341960407619695, -5.719274019375665929, 66.04275706135236135 ) ) ;
#56342=CARTESIAN_POINT ( 'NONE',  ( 9.474510206698971260, -16.51473224551069308, 67.91557627198102409 ) ) ;
#56343=CARTESIAN_POINT ( 'NONE',  ( -10.72451020669898014, 18.67979575497178502, 95.41557627198102409 ) ) ;
#56344=CARTESIAN_POINT ( 'NONE',  ( 4.483927247898545687, 16.52544592524342804, 104.7905762719810241 ) ) ;
#56345=CARTESIAN_POINT ( 'NONE',  ( 13.89961937509957401, 13.97604488694547697, 71.87609039468567573 ) ) ;
#56346=CARTESIAN_POINT ( 'NONE',  ( 5.719274019375991003, -21.55341960407610458, 67.70724293864769550 ) ) ;
#56347=CARTESIAN_POINT ( 'NONE',  ( -19.03943276465977164, -0.05219959533935918106, 43.75109039468566863 ) ) ;
#56348=CARTESIAN_POINT ( 'NONE',  ( -9.474510206698964154, 16.51473224551069663, 115.4155762719810241 ) ) ;
#56349=EDGE_CURVE ( 'NONE', #177566, #17000, #143966, .T. ) ;
#56350=CARTESIAN_POINT ( 'NONE',  ( 21.52544592524344225, -5.823673210054117533, 93.54057627198103830 ) ) ;
#56352=CARTESIAN_POINT ( 'NONE',  ( -16.51473224551069308, -9.474510206698971260, 66.66557627198102409 ) ) ;
#56354=CARTESIAN_POINT ( 'NONE',  ( -8.314922557961024197, 14.29746914071037800, 22.91775706135235069 ) ) ;
#56355=CARTESIAN_POINT ( 'NONE',  ( -18.09867054820431065, -5.499999999999968026, 98.98393025253585620 ) ) ;
#56356=CARTESIAN_POINT ( 'NONE',  ( 13.89961937509977652, -13.97604488694527269, 53.12390960531434558 ) ) ;
#56357=CARTESIAN_POINT ( 'NONE',  ( 5.153800228976335163, 19.02544592524342804, 109.7905762719810099 ) ) ;
#56358=CARTESIAN_POINT ( 'NONE',  ( -5.823673210054116645, -21.52544592524344225, 92.29057627198103830 ) ) ;
#56359=CARTESIAN_POINT ( 'NONE',  ( -16.53943276465976808, 0.05219959533911058130, 56.24890960531436690 ) ) ;
#56360=CARTESIAN_POINT ( 'NONE',  ( -21.53943276465977519, -0.05219959533937600094, 73.75109039468567573 ) ) ;
#56361=CARTESIAN_POINT ( 'NONE',  ( -14.29746914071037622, -8.314922557961029526, 24.16775706135235424 ) ) ;
#56362=CARTESIAN_POINT ( 'NONE',  ( -5.153800228976607833, 19.02544592524334988, 22.70942372801899012 ) ) ;
#56363=CARTESIAN_POINT ( 'NONE',  ( -16.53943276465976808, 0.05219959533911058130, 36.24890960531435979 ) ) ;
#56364=CARTESIAN_POINT ( 'NONE',  ( -15.72974639402197994, 15.80617190586746368, 110.6239096053143669 ) ) ;
#56365=CARTESIAN_POINT ( 'NONE',  ( 14.34966873604960469, 8.224510206698951720, 54.16557627198103120 ) ) ;
#56366=CARTESIAN_POINT ( 'NONE',  ( 19.03943276465977164, 0.05219959533936151252, 101.2510903946856757 ) ) ;
#56367=CARTESIAN_POINT ( 'NONE',  ( 16.46253265017146816, 9.564922557961045513, 66.66775706135233293 ) ) ;
#56368=CARTESIAN_POINT ( 'NONE',  ( -5.823673210054431948, 21.52544592524334988, 72.70942372801901854 ) ) ;
#56369=CARTESIAN_POINT ( 'NONE',  ( -0.05219959533936034679, 19.03943276465977164, 52.50109039468566863 ) ) ;
#56370=CARTESIAN_POINT ( 'NONE',  ( 13.97604488694527802, 13.89961937509977652, 29.37390960531435979 ) ) ;
#56371=CARTESIAN_POINT ( 'NONE',  ( 21.53943276465977519, -0.05219959533907433946, 38.74890960531435979 ) ) ;
#56372=CARTESIAN_POINT ( 'NONE',  ( 0.05219959533910956823, 16.53943276465976808, 54.99890960531435269 ) ) ;
#56373=CARTESIAN_POINT ( 'NONE',  ( -17.12812012977026654, -6.668231424566000598, 26.35948759323144941 ) ) ;
#56374=CARTESIAN_POINT ( 'NONE',  ( 0.05219959533937995610, -21.53943276465977519, 110.0010903946856757 ) ) ;
#56375=CARTESIAN_POINT ( 'NONE',  ( -16.55341960407617563, 4.379528057220093196, 88.54275706135236135 ) ) ;
#56376=CARTESIAN_POINT ( 'NONE',  ( -16.55341960407611168, -4.379528057220339221, 46.45724293864769550 ) ) ;
#56377=CARTESIAN_POINT ( 'NONE',  ( 18.67979575497194134, -10.72451020669871369, 75.83442372801900433 ) ) ;
#56378=CARTESIAN_POINT ( 'NONE',  ( 18.67979575497194134, -10.72451020669871369, 65.83442372801900433 ) ) ;
#56379=CARTESIAN_POINT ( 'NONE',  ( -15.80617190586745835, -15.72974639402198527, 76.87390960531439532 ) ) ;
#56381=CARTESIAN_POINT ( 'NONE',  ( 13.97604488694527802, 13.89961937509977652, 44.37390960531435269 ) ) ;
#56382=CARTESIAN_POINT ( 'NONE',  ( -0.05219959533937732626, 21.53943276465977519, 62.50109039468568284 ) ) ;
#56383=CARTESIAN_POINT ( 'NONE',  ( -16.51473224551069308, -9.474510206698971260, 26.66557627198103120 ) ) ;
#56384=CARTESIAN_POINT ( 'NONE',  ( -16.51473224551069308, -9.474510206698971260, 46.66557627198102409 ) ) ;
#56385=CARTESIAN_POINT ( 'NONE',  ( 12.06949235617757843, -12.14591786802309237, 93.12390960531436690 ) ) ;
#56386=CARTESIAN_POINT ( 'NONE',  ( -13.97604488694527625, -13.89961937509977652, 86.87390960531436690 ) ) ;
#56387=CARTESIAN_POINT ( 'NONE',  ( -12.14591786802309592, -12.06949235617757132, 36.87390960531435979 ) ) ;
#56388=CARTESIAN_POINT ( 'NONE',  ( 16.52544592524342804, -4.483927247898539470, 103.5405762719810383 ) ) ;
#56389=CARTESIAN_POINT ( 'NONE',  ( -21.52544592524343514, 5.823673210054127303, 76.04057627198102409 ) ) ;
#56390=CARTESIAN_POINT ( 'NONE',  ( 0.05219959533907565091, 21.53943276465977519, 114.9989096053143669 ) ) ;
#56392=CARTESIAN_POINT ( 'NONE',  ( 16.46253265017160672, -9.564922557960803928, 78.33224293864769550 ) ) ;
#56393=CARTESIAN_POINT ( 'NONE',  ( 4.379528057220092307, 16.55341960407617563, 27.29275706135234358 ) ) ;
#56394=CARTESIAN_POINT ( 'NONE',  ( -5.823673210054116645, -21.52544592524344225, 72.29057627198102409 ) ) ;
#56396=CARTESIAN_POINT ( 'NONE',  ( 5.823673210054444382, -21.52544592524334988, 100.2094237280190043 ) ) ;
#56397=CARTESIAN_POINT ( 'NONE',  ( 16.46253265017160672, -9.564922557960803928, 78.33224293864769550 ) ) ;
#56398=CARTESIAN_POINT ( 'NONE',  ( 15.80617190586746368, 15.72974639402197994, 109.3739096053143811 ) ) ;
#56399=CARTESIAN_POINT ( 'NONE',  ( 19.03943276465977164, -0.05219959533909143690, 113.7489096053143669 ) ) ;
#56400=CARTESIAN_POINT ( 'NONE',  ( 0.05219959533934541429, -16.53943276465976808, 90.00109039468567573 ) ) ;
#56401=CARTESIAN_POINT ( 'NONE',  ( -10.72451020669870658, -18.67979575497194134, 64.58442372801900433 ) ) ;
#56402=CARTESIAN_POINT ( 'NONE',  ( 5.719274019375673035, 21.55341960407619339, 97.29275706135234714 ) ) ;
#56403=CARTESIAN_POINT ( 'NONE',  ( 16.55341960407618274, -4.379528057220086978, 61.04275706135234714 ) ) ;
#56404=CARTESIAN_POINT ( 'NONE',  ( 18.62759615963255655, 10.81492255796105972, 31.66775706135234358 ) ) ;
#56406=CARTESIAN_POINT ( 'NONE',  ( 5.153800228976335163, 19.02544592524342804, 24.79057627198102765 ) ) ;
#56407=CARTESIAN_POINT ( 'NONE',  ( -10.81492255796105439, 18.62759615963255655, 92.91775706135236135 ) ) ;
#56408=CARTESIAN_POINT ( 'NONE',  ( 13.89961937509977652, -13.97604488694527269, 98.12390960531433848 ) ) ;
#56409=CARTESIAN_POINT ( 'NONE',  ( -15.80617190586745835, -15.72974639402198527, 91.87390960531436690 ) ) ;
#56410=CARTESIAN_POINT ( 'NONE',  ( -9.564922557961040184, 16.46253265017147172, 62.91775706135233293 ) ) ;
#56412=CARTESIAN_POINT ( 'NONE',  ( 18.62759615963271287, -10.81492255796078972, 58.33224293864768839 ) ) ;
#56413=CARTESIAN_POINT ( 'NONE',  ( 5.153800228976335163, 19.02544592524342804, 89.79057627198102409 ) ) ;
#56414=CARTESIAN_POINT ( 'NONE',  ( -16.55341960407611168, -4.379528057220339221, 41.45724293864769550 ) ) ;
#56416=CARTESIAN_POINT ( 'NONE',  ( 19.03943276465977164, 0.05219959533936151252, 76.25109039468566152 ) ) ;
#56418=CARTESIAN_POINT ( 'NONE',  ( 5.049401038297881783, 19.05341960407617563, 112.2927570613523471 ) ) ;
#56419=CARTESIAN_POINT ( 'NONE',  ( -18.62759615963270932, 10.81492255796079327, 85.83224293864768129 ) ) ;
#56420=CARTESIAN_POINT ( 'NONE',  ( -8.224510206698948167, 14.34966873604960824, 60.41557627198102409 ) ) ;
#56421=CARTESIAN_POINT ( 'NONE',  ( -12.06949235617739369, -12.14591786802326823, 24.37609039468567573 ) ) ;
#56422=CARTESIAN_POINT ( 'NONE',  ( -9.474510206698964154, 16.51473224551069663, 50.41557627198102409 ) ) ;
#56423=CARTESIAN_POINT ( 'NONE',  ( 21.55341960407619695, -5.719274019375665929, 21.04275706135234714 ) ) ;
#56424=CARTESIAN_POINT ( 'NONE',  ( -16.51473224551082808, 9.474510206698731452, 83.33442372801899012 ) ) ;
#56425=CARTESIAN_POINT ( 'NONE',  ( 19.05341960407611168, 5.049401038298154454, 93.95724293864769550 ) ) ;
#56426=( BOUNDED_CURVE ( )  B_SPLINE_CURVE ( 2, ( #4677, #82515, #144197, #5683, #67359, #190719, #52192, #113850, #94356, #122712, #184402, #106554, #79192 ),
 .UNSPECIFIED., .F., .F. ) 
 B_SPLINE_CURVE_WITH_KNOTS ( ( 3, 2, 2, 2, 2, 2, 3 ),
 ( 0.4235287478280826967, 0.4254385964912280604, 0.4298245614035087758, 0.4342105263157894912, 0.4385964912280701511, 0.4429824561403508665, 0.4449379846255865356 ),
 .UNSPECIFIED. ) 
 CURVE ( )  GEOMETRIC_REPRESENTATION_ITEM ( )  RATIONAL_B_SPLINE_CURVE ( ( 0.9832469066685285419, 0.9851625545550100060, 1.000000000000000000, 0.9659258262890683122, 1.000000000000000000, 0.9659258262890683122, 1.000000000000000000, 0.9659258262890683122, 1.000000000000000000, 0.9659258262890683122, 1.000000000000000000, 0.9848076720550082985, 0.9831626618144002627 ) ) 
 REPRESENTATION_ITEM ( '' )  );
#56427=CARTESIAN_POINT ( 'NONE',  ( 13.97604488694527802, 13.89961937509977652, 69.37390960531436690 ) ) ;
#56428=CARTESIAN_POINT ( 'NONE',  ( -10.72451020669898014, 18.67979575497178502, 70.41557627198102409 ) ) ;
#56429=CARTESIAN_POINT ( 'NONE',  ( 19.02544592524343514, -5.153800228976328945, 48.54057627198103120 ) ) ;
#56431=CARTESIAN_POINT ( 'NONE',  ( 12.14591786802309770, 12.06949235617756955, 49.37390960531436690 ) ) ;
#56432=CARTESIAN_POINT ( 'NONE',  ( -5.153800228976328057, -19.02544592524343514, 102.2905762719810383 ) ) ;
#56434=CARTESIAN_POINT ( 'NONE',  ( 16.51473224551083163, -9.474510206698727899, 70.83442372801900433 ) ) ;
#56435=CARTESIAN_POINT ( 'NONE',  ( -5.823673210054116645, -21.52544592524344225, 82.29057627198103830 ) ) ;
#56436=CARTESIAN_POINT ( 'NONE',  ( 16.46253265017146816, 9.564922557961045513, 31.66775706135232937 ) ) ;
#56437=CARTESIAN_POINT ( 'NONE',  ( -16.46253265017160317, 9.564922557960807481, 100.8322429386477097 ) ) ;
#56439=CARTESIAN_POINT ( 'NONE',  ( 5.823673210054125526, 21.52544592524343514, 39.79057627198103830 ) ) ;
#56441=CARTESIAN_POINT ( 'NONE',  ( -9.564922557960796823, -16.46253265017161027, 67.08224293864769550 ) ) ;
#56442=EDGE_CURVE ( 'NONE', #164406, #148926, #14583, .T. ) ;
#56443=CARTESIAN_POINT ( 'NONE',  ( -10.72451020669870658, -18.67979575497194134, 64.58442372801900433 ) ) ;
#56444=CARTESIAN_POINT ( 'NONE',  ( -9.474510206698964154, 16.51473224551069663, 30.41557627198102054 ) ) ;
#56445=CARTESIAN_POINT ( 'NONE',  ( -10.81492255796078084, -18.62759615963271287, 112.0822429386477097 ) ) ;
#56446=ORIENTED_EDGE ( 'NONE', *, *, #102991, .F. ) ;
#56447=CARTESIAN_POINT ( 'NONE',  ( -15.72974639402176322, -15.80617190586768395, 49.37609039468569705 ) ) ;
#56449=CARTESIAN_POINT ( 'NONE',  ( 5.049401038298161559, -19.05341960407611168, 107.7072429386476955 ) ) ;
#56450=CARTESIAN_POINT ( 'NONE',  ( 16.46253265017146816, 9.564922557961045513, 71.66775706135233293 ) ) ;
#56452=CARTESIAN_POINT ( 'NONE',  ( -21.52544592524343514, 5.823673210054127303, 106.0405762719810525 ) ) ;
#56453=CARTESIAN_POINT ( 'NONE',  ( 9.474510206698971260, -16.51473224551069308, 62.91557627198102409 ) ) ;
#56454=CARTESIAN_POINT ( 'NONE',  ( -14.29746914071037622, -8.314922557961029526, 39.16775706135235424 ) ) ;
#56456=CARTESIAN_POINT ( 'NONE',  ( 5.719274019375673035, 21.55341960407619339, 102.2927570613523613 ) ) ;
#56457=CARTESIAN_POINT ( 'NONE',  ( -5.049401038298153566, 19.05341960407611168, 45.20724293864769550 ) ) ;
#56458=CARTESIAN_POINT ( 'NONE',  ( -9.474510206698720793, -16.51473224551083518, 19.58442372801899722 ) ) ;
#56459=CARTESIAN_POINT ( 'NONE',  ( 13.97604488694527802, 13.89961937509977652, 94.37390960531436690 ) ) ;
#56460=CARTESIAN_POINT ( 'NONE',  ( 21.52544592524334988, 5.823673210054432836, 61.45942372801901854 ) ) ;
#56462=CARTESIAN_POINT ( 'NONE',  ( 13.89961937509977652, -13.97604488694527269, 113.1239096053143527 ) ) ;
#56463=CARTESIAN_POINT ( 'NONE',  ( -17.49999999999999645, 3.565345528327878544, 29.42494486806477738 ) ) ;
#56464=CARTESIAN_POINT ( 'NONE',  ( -12.14591786802326823, 12.06949235617739902, 48.12609039468568284 ) ) ;
#56465=CARTESIAN_POINT ( 'NONE',  ( -10.81492255796105439, 18.62759615963255655, 77.91775706135231871 ) ) ;
#56466=CARTESIAN_POINT ( 'NONE',  ( 21.55341960407619695, -5.719274019375665929, 86.04275706135236135 ) ) ;
#56468=CARTESIAN_POINT ( 'NONE',  ( -12.06949235617739369, -12.14591786802326823, 24.37609039468567573 ) ) ;
#56469=CARTESIAN_POINT ( 'NONE',  ( -9.474510206698964154, 16.51473224551069663, 85.41557627198102409 ) ) ;
#56470=CARTESIAN_POINT ( 'NONE',  ( -9.474510206698964154, 16.51473224551069663, 110.4155762719810383 ) ) ;
#56471=CARTESIAN_POINT ( 'NONE',  ( 17.31728774477272026, 6.344390552232403557, 41.68093348310682700 ) ) ;
#56472=CARTESIAN_POINT ( 'NONE',  ( -19.02544592524342804, 5.153800228976336051, 31.04057627198102409 ) ) ;
#56473=CARTESIAN_POINT ( 'NONE',  ( 21.52544592524344225, -5.823673210054117533, 48.54057627198103120 ) ) ;
#56474=EDGE_CURVE ( 'NONE', #74699, #188324, #76289, .T. ) ;
#56475=CARTESIAN_POINT ( 'NONE',  ( -4.483927247898782831, 16.52544592524335698, 107.7094237280190328 ) ) ;
#56476=CARTESIAN_POINT ( 'NONE',  ( -16.53943276465976808, 0.05219959533911058130, 86.24890960531436690 ) ) ;
#56477=CARTESIAN_POINT ( 'NONE',  ( 19.02544592524343514, -5.153800228976328945, 73.54057627198103830 ) ) ;
#56478=CARTESIAN_POINT ( 'NONE',  ( 15.80617190586769283, -15.72974639402175789, 85.62609039468568994 ) ) ;
#56479=CARTESIAN_POINT ( 'NONE',  ( 4.483927247898790824, -16.52544592524335698, 25.20942372801901854 ) ) ;
#56480=CARTESIAN_POINT ( 'NONE',  ( 8.314922557960818139, 14.29746914071049879, 94.58224293864769550 ) ) ;
#56481=CARTESIAN_POINT ( 'NONE',  ( -10.72451020669870658, -18.67979575497194134, 39.58442372801901143 ) ) ;
#56482=CARTESIAN_POINT ( 'NONE',  ( 10.72451020669898902, -18.67979575497178502, 72.91557627198103830 ) ) ;
#56483=CARTESIAN_POINT ( 'NONE',  ( 19.02544592524334988, 5.153800228976608722, 31.45942372801900433 ) ) ;
#56485=CARTESIAN_POINT ( 'NONE',  ( 9.474510206698971260, -16.51473224551069308, 102.9155762719810241 ) ) ;
#56486=CARTESIAN_POINT ( 'NONE',  ( -14.34966873604960291, -8.224510206698953496, 61.66557627198103120 ) ) ;
#56487=CARTESIAN_POINT ( 'NONE',  ( 0.05219959533910956823, 16.53943276465976808, 54.99890960531435269 ) ) ;
#56488=CARTESIAN_POINT ( 'NONE',  ( 14.34966873604972726, -8.224510206698740333, 110.8344237280190043 ) ) ;
#56489=CARTESIAN_POINT ( 'NONE',  ( 13.89961937509957401, 13.97604488694547697, 71.87609039468567573 ) ) ;
#56490=CARTESIAN_POINT ( 'NONE',  ( 19.19724070472090460, 5.500000000000158096, 53.56193348274384647 ) ) ;
#56491=CARTESIAN_POINT ( 'NONE',  ( -9.564922557960796823, -16.46253265017161027, 112.0822429386476955 ) ) ;
#56492=CARTESIAN_POINT ( 'NONE',  ( -8.314922557960811034, -14.29746914071050412, 82.08224293864768129 ) ) ;
#56494=CARTESIAN_POINT ( 'NONE',  ( 16.46253265017160672, -9.564922557960803928, 43.33224293864769550 ) ) ;
#56495=CARTESIAN_POINT ( 'NONE',  ( -10.81492255796078084, -18.62759615963271287, 52.08224293864768839 ) ) ;
#56496=CARTESIAN_POINT ( 'NONE',  ( 15.72974639402199770, -15.80617190586745480, 78.12390960531436690 ) ) ;
#56497=CARTESIAN_POINT ( 'NONE',  ( 12.14591786802309770, 12.06949235617756955, 109.3739096053143811 ) ) ;
#56498=CARTESIAN_POINT ( 'NONE',  ( 16.52544592524335698, 4.483927247898782831, 61.45942372801901854 ) ) ;
#56499=CARTESIAN_POINT ( 'NONE',  ( 9.474510206698971260, -16.51473224551069308, 47.91557627198102409 ) ) ;
#56500=CARTESIAN_POINT ( 'NONE',  ( -19.03943276465977164, -0.05219959533935918106, 43.75109039468566863 ) ) ;
#56502=CARTESIAN_POINT ( 'NONE',  ( 21.53943276465977519, 0.05219959533937863772, 56.25109039468568284 ) ) ;
#56503=CARTESIAN_POINT ( 'NONE',  ( -8.224510206698948167, 14.34966873604960824, 110.4155762719810383 ) ) ;
#56504=CARTESIAN_POINT ( 'NONE',  ( 19.02544592524334988, 5.153800228976608722, 96.45942372801897591 ) ) ;
#56507=CARTESIAN_POINT ( 'NONE',  ( -18.67979575497178146, -10.72451020669898902, 46.66557627198102409 ) ) ;
#56508=CARTESIAN_POINT ( 'NONE',  ( -5.153800228976328057, -19.02544592524343514, 22.29057627198102765 ) ) ;
#56509=CARTESIAN_POINT ( 'NONE',  ( 10.81492255796106328, -18.62759615963255655, 80.41775706135234714 ) ) ;
#56510=CARTESIAN_POINT ( 'NONE',  ( -4.379528057220328563, 16.55341960407611168, 30.20724293864769550 ) ) ;
#56511=CARTESIAN_POINT ( 'NONE',  ( 8.224510206698742110, 14.34966873604972548, 62.08442372801901143 ) ) ;
#56512=CARTESIAN_POINT ( 'NONE',  ( 4.483927247898545687, 16.52544592524342804, 44.79057627198103120 ) ) ;
#56513=CARTESIAN_POINT ( 'NONE',  ( -18.62759615963270932, 10.81492255796079327, 75.83224293864769550 ) ) ;
#56514=CARTESIAN_POINT ( 'NONE',  ( 18.67979575497178502, 10.72451020669898547, 74.16557627198102409 ) ) ;
#56516=CARTESIAN_POINT ( 'NONE',  ( -19.05341960407617563, 5.049401038297882671, 83.54275706135233293 ) ) ;
#56517=CARTESIAN_POINT ( 'NONE',  ( 15.72974639402199770, -15.80617190586745480, 23.12390960531436335 ) ) ;
#56518=CARTESIAN_POINT ( 'NONE',  ( -16.46253265017160317, 9.564922557960807481, 50.83224293864770260 ) ) ;
#56519=CARTESIAN_POINT ( 'NONE',  ( 19.02544592524343514, -5.153800228976328945, 28.54057627198102409 ) ) ;
#56522=ORIENTED_EDGE ( 'NONE', *, *, #165511, .T. ) ;
#56523=AXIS2_PLACEMENT_3D ( 'NONE', #173770, #132231, #81706 ) ;
#56524=CARTESIAN_POINT ( 'NONE',  ( 8.314922557961029526, -14.29746914071037800, 80.41775706135234714 ) ) ;
#56525=CARTESIAN_POINT ( 'NONE',  ( -21.52544592524343514, 5.823673210054127303, 106.0405762719810525 ) ) ;
#56526=CARTESIAN_POINT ( 'NONE',  ( 9.474510206698971260, -16.51473224551069308, 67.91557627198102409 ) ) ;
#56527=CARTESIAN_POINT ( 'NONE',  ( 18.67979575497194134, -10.72451020669871369, 35.83442372801901143 ) ) ;
#56528=CARTESIAN_POINT ( 'NONE',  ( 9.474510206698971260, -16.51473224551069308, 102.9155762719810241 ) ) ;
#56531=CARTESIAN_POINT ( 'NONE',  ( -15.72974639402176322, -15.80617190586768395, 29.37609039468568284 ) ) ;
#56532=CARTESIAN_POINT ( 'NONE',  ( 5.153800228976335163, 19.02544592524342804, 29.79057627198102409 ) ) ;
#56533=CARTESIAN_POINT ( 'NONE',  ( 16.46253265017160672, -9.564922557960803928, 108.3322429386476955 ) ) ;
#56534=CARTESIAN_POINT ( 'NONE',  ( -16.51473224551082808, 9.474510206698731452, 38.33442372801899722 ) ) ;
#56535=CARTESIAN_POINT ( 'NONE',  ( -5.719274019375978568, 21.55341960407610458, 115.2072429386476955 ) ) ;
#56536=CARTESIAN_POINT ( 'NONE',  ( -16.51473224551082808, 9.474510206698731452, 48.33442372801900433 ) ) ;
#56537=CARTESIAN_POINT ( 'NONE',  ( -5.153800228976607833, 19.02544592524334988, 42.70942372801901143 ) ) ;
#56538=CARTESIAN_POINT ( 'NONE',  ( 12.06949235617739724, 12.14591786802326823, 96.87609039468568994 ) ) ;
#56541=CARTESIAN_POINT ( 'NONE',  ( -9.474510206698964154, 16.51473224551069663, 75.41557627198103830 ) ) ;
#56542=COLOUR_RGB ( '', 0.31764706, 0.68627451, 0.89019608) ;
#56543=CARTESIAN_POINT ( 'NONE',  ( -10.72451020669870658, -18.67979575497194134, 79.58442372801903275 ) ) ;
#56544=CARTESIAN_POINT ( 'NONE',  ( 18.67979575497194134, -10.72451020669871369, 90.83442372801901854 ) ) ;
#56546=CARTESIAN_POINT ( 'NONE',  ( 5.049401038298161559, -19.05341960407611168, 92.70724293864769550 ) ) ;
#56547=CARTESIAN_POINT ( 'NONE',  ( -21.53943276465977519, -0.05219959533937600094, 63.75109039468568284 ) ) ;
#56548=CARTESIAN_POINT ( 'NONE',  ( 9.564922557961047289, -16.46253265017146816, 100.4177570613523329 ) ) ;
#56549=CARTESIAN_POINT ( 'NONE',  ( -9.564922557960796823, -16.46253265017161027, 62.08224293864769550 ) ) ;
#56550=CARTESIAN_POINT ( 'NONE',  ( -5.153800228976328057, -19.02544592524343514, 107.2905762719810383 ) ) ;
#56551=CARTESIAN_POINT ( 'NONE',  ( 19.02544592524343514, -5.153800228976328945, 83.54057627198100988 ) ) ;
#56552=CARTESIAN_POINT ( 'NONE',  ( -17.40805194822030799, -6.112264579159315758, 89.16628727489390371 ) ) ;
#56553=CARTESIAN_POINT ( 'NONE',  ( 13.97604488694527802, 13.89961937509977652, 59.37390960531434558 ) ) ;
#56554=CARTESIAN_POINT ( 'NONE',  ( 5.049401038298161559, -19.05341960407611168, 52.70724293864767418 ) ) ;
#56555=CARTESIAN_POINT ( 'NONE',  ( -15.72974639402197994, 15.80617190586746368, 115.6239096053143669 ) ) ;
#56556=CARTESIAN_POINT ( 'NONE',  ( -12.14591786802326823, 12.06949235617739902, 98.12609039468570415 ) ) ;
#56560=CARTESIAN_POINT ( 'NONE',  ( -19.03943276465977164, -0.05219959533935918106, 63.75109039468566863 ) ) ;
#56561=CARTESIAN_POINT ( 'NONE',  ( -19.03943276465977164, 0.05219959533909376836, 76.24890960531435269 ) ) ;
#56562=CARTESIAN_POINT ( 'NONE',  ( -16.52544592524342804, 4.483927247898546575, 66.04057627198103830 ) ) ;
#56563=CARTESIAN_POINT ( 'NONE',  ( -4.483927247898539470, -16.52544592524342804, 107.2905762719810525 ) ) ;
#56565=CARTESIAN_POINT ( 'NONE',  ( 10.81492255796078972, 18.62759615963270932, 29.58224293864769905 ) ) ;
#56566=CARTESIAN_POINT ( 'NONE',  ( -13.97604488694527625, -13.89961937509977652, 26.87390960531434558 ) ) ;
#56567=CARTESIAN_POINT ( 'NONE',  ( -9.474510206698964154, 16.51473224551069663, 110.4155762719810383 ) ) ;
#56568=CARTESIAN_POINT ( 'NONE',  ( 8.224510206698953496, -14.34966873604960469, 97.91557627198103830 ) ) ;
#56570=CARTESIAN_POINT ( 'NONE',  ( 9.564922557961047289, -16.46253265017146816, 30.41775706135232937 ) ) ;
#56571=CARTESIAN_POINT ( 'NONE',  ( 14.29746914071037800, 8.314922557961029526, 111.6677570613523613 ) ) ;
#56572=CARTESIAN_POINT ( 'NONE',  ( 19.03943276465977164, -0.05219959533909143690, 83.74890960531436690 ) ) ;
#56573=CARTESIAN_POINT ( 'NONE',  ( -15.80617190586768217, 15.72974639402176855, 48.12609039468568284 ) ) ;
#56574=CARTESIAN_POINT ( 'NONE',  ( 15.72974639402199770, -15.80617190586745480, 43.12390960531435269 ) ) ;
#56575=CARTESIAN_POINT ( 'NONE',  ( 18.67979575497194134, -10.72451020669871369, 35.83442372801901143 ) ) ;
#56576=CARTESIAN_POINT ( 'NONE',  ( 21.52544592524344225, -5.823673210054117533, 78.54057627198103830 ) ) ;
#56577=CARTESIAN_POINT ( 'NONE',  ( -14.34966873604960291, -8.224510206698953496, 96.66557627198102409 ) ) ;
#56578=CARTESIAN_POINT ( 'NONE',  ( -9.474510206698720793, -16.51473224551083518, 59.58442372801900433 ) ) ;
#56579=CARTESIAN_POINT ( 'NONE',  ( -16.46253265017160317, 9.564922557960807481, 40.83224293864769550 ) ) ;
#56580=CARTESIAN_POINT ( 'NONE',  ( -5.153800228976328057, -19.02544592524343514, 97.29057627198099567 ) ) ;
#56581=CARTESIAN_POINT ( 'NONE',  ( 9.474510206698971260, -16.51473224551069308, 97.91557627198102409 ) ) ;
#56582=CARTESIAN_POINT ( 'NONE',  ( -19.05341960407611168, -5.049401038298163336, 21.45724293864768839 ) ) ;
#56583=CARTESIAN_POINT ( 'NONE',  ( 12.14591786802309770, 12.06949235617756955, 24.37390960531435979 ) ) ;
#56584=CARTESIAN_POINT ( 'NONE',  ( 14.34966873604972726, -8.224510206698740333, 45.83442372801901854 ) ) ;
#56585=CARTESIAN_POINT ( 'NONE',  ( 10.72451020669871369, 18.67979575497193778, 102.0844237280190185 ) ) ;
#56588=CARTESIAN_POINT ( 'NONE',  ( -14.34966873604960291, -8.224510206698953496, 26.66557627198103475 ) ) ;
#56589=CARTESIAN_POINT ( 'NONE',  ( 15.72974639402176855, 15.80617190586768217, 31.87609039468567929 ) ) ;
#56590=CARTESIAN_POINT ( 'NONE',  ( -9.474510206698964154, 16.51473224551069663, 40.41557627198103120 ) ) ;
#56591=CARTESIAN_POINT ( 'NONE',  ( -14.34966873604972548, 8.224510206698743886, 38.33442372801900433 ) ) ;
#56592=CARTESIAN_POINT ( 'NONE',  ( -4.379528057220086978, -16.55341960407618274, 109.7927570613523613 ) ) ;
#56593=CARTESIAN_POINT ( 'NONE',  ( 8.224510206698742110, 14.34966873604972548, 97.08442372801904696 ) ) ;
#56594=CARTESIAN_POINT ( 'NONE',  ( -0.05219959533934338120, 16.53943276465976808, 22.50109039468567573 ) ) ;
#56595=CARTESIAN_POINT ( 'NONE',  ( -16.46253265017160317, 9.564922557960807481, 40.83224293864769550 ) ) ;
#56596=CARTESIAN_POINT ( 'NONE',  ( -14.34966873604960291, -8.224510206698953496, 106.6655762719810383 ) ) ;
#56597=CARTESIAN_POINT ( 'NONE',  ( -5.823673210054116645, -21.52544592524344225, 112.2905762719810241 ) ) ;
#56598=CARTESIAN_POINT ( 'NONE',  ( 5.049401038298161559, -19.05341960407611168, 32.70724293864768129 ) ) ;
#56599=CARTESIAN_POINT ( 'NONE',  ( 13.97604488694527802, 13.89961937509977652, 104.3739096053143385 ) ) ;
#56600=CARTESIAN_POINT ( 'NONE',  ( -15.80617190586768217, 15.72974639402176855, 33.12609039468569705 ) ) ;
#56601=CARTESIAN_POINT ( 'NONE',  ( 19.03943276465977164, -0.05219959533909143690, 23.74890960531435269 ) ) ;
#56602=CARTESIAN_POINT ( 'NONE',  ( -9.474510206698964154, 16.51473224551069663, 105.4155762719810383 ) ) ;
#56604=CARTESIAN_POINT ( 'NONE',  ( 5.049401038298161559, -19.05341960407611168, 102.7072429386476955 ) ) ;
#56605=CARTESIAN_POINT ( 'NONE',  ( -21.55341960407619339, 5.719274019375674811, 33.54275706135234714 ) ) ;
#56606=CARTESIAN_POINT ( 'NONE',  ( -12.14591786802309592, -12.06949235617757132, 91.87390960531436690 ) ) ;
#56607=CARTESIAN_POINT ( 'NONE',  ( -19.05341960407611168, -5.049401038298163336, 96.45724293864769550 ) ) ;
#56609=CARTESIAN_POINT ( 'NONE',  ( -12.06949235617739369, -12.14591786802326823, 64.37609039468568994 ) ) ;
#56610=CARTESIAN_POINT ( 'NONE',  ( -21.52544592524334988, -5.823673210054445271, 73.95942372801901854 ) ) ;
#56611=CARTESIAN_POINT ( 'NONE',  ( 16.52544592524335698, 4.483927247898782831, 41.45942372801901143 ) ) ;
#56612=CARTESIAN_POINT ( 'NONE',  ( -9.474510206698964154, 16.51473224551069663, 80.41557627198103830 ) ) ;
#56613=CARTESIAN_POINT ( 'NONE',  ( -8.224510206698735004, -14.34966873604973081, 19.58442372801901143 ) ) ;
#56614=CARTESIAN_POINT ( 'NONE',  ( -16.53943276465976808, -0.05219959533934237506, 73.75109039468567573 ) ) ;
#56615=CARTESIAN_POINT ( 'NONE',  ( 21.53943276465977519, 0.05219959533937863772, 111.2510903946856899 ) ) ;
#56616=CARTESIAN_POINT ( 'NONE',  ( 16.46253265017146816, 9.564922557961045513, 96.66775706135233293 ) ) ;
#56617=CARTESIAN_POINT ( 'NONE',  ( -16.51473224551069308, -9.474510206698971260, 66.66557627198102409 ) ) ;
#56618=CARTESIAN_POINT ( 'NONE',  ( 18.67979575497178502, 10.72451020669898547, 79.16557627198103830 ) ) ;
#56619=CARTESIAN_POINT ( 'NONE',  ( -4.483927247898539470, -16.52544592524342804, 92.29057627198103830 ) ) ;
#56620=CARTESIAN_POINT ( 'NONE',  ( 9.564922557961047289, -16.46253265017146816, 90.41775706135234714 ) ) ;
#56621=CARTESIAN_POINT ( 'NONE',  ( -8.224510206698735004, -14.34966873604973081, 59.58442372801901854 ) ) ;
#56623=CARTESIAN_POINT ( 'NONE',  ( -16.51473224551082808, 9.474510206698731452, 58.33442372801900433 ) ) ;
#56624=CARTESIAN_POINT ( 'NONE',  ( 8.224510206698953496, -14.34966873604960469, 27.91557627198103830 ) ) ;
#56625=CARTESIAN_POINT ( 'NONE',  ( 0.05219959533910956823, 16.53943276465976808, 79.99890960531435269 ) ) ;
#56626=CARTESIAN_POINT ( 'NONE',  ( -19.02544592524334988, -5.153800228976617603, 23.95942372801900078 ) ) ;
#56628=CARTESIAN_POINT ( 'NONE',  ( -15.72974639402176322, -15.80617190586768395, 29.37609039468568284 ) ) ;
#56629=CARTESIAN_POINT ( 'NONE',  ( -13.89961937509977652, 13.97604488694528158, 100.6239096053143669 ) ) ;
#56630=CARTESIAN_POINT ( 'NONE',  ( -13.89961937509977652, 13.97604488694528158, 75.62390960531438111 ) ) ;
#56631=CARTESIAN_POINT ( 'NONE',  ( -15.72974639402176322, -15.80617190586768395, 99.37609039468568994 ) ) ;
#56632=CARTESIAN_POINT ( 'NONE',  ( 16.46253265017160672, -9.564922557960803928, 73.33224293864769550 ) ) ;
#56633=CARTESIAN_POINT ( 'NONE',  ( -10.72451020669898014, 18.67979575497178502, 35.41557627198102409 ) ) ;
#56635=CARTESIAN_POINT ( 'NONE',  ( 4.379528057220339221, -16.55341960407611168, 77.70724293864770971 ) ) ;
#56636=CARTESIAN_POINT ( 'NONE',  ( 16.46253265017160672, -9.564922557960803928, 38.33224293864768839 ) ) ;
#56637=CARTESIAN_POINT ( 'NONE',  ( 4.379528057220339221, -16.55341960407611168, 102.7072429386476955 ) ) ;
#56638=CARTESIAN_POINT ( 'NONE',  ( 5.719274019375991003, -21.55341960407610458, 107.7072429386476955 ) ) ;
#56639=CARTESIAN_POINT ( 'NONE',  ( 18.62759615963255655, 10.81492255796105972, 61.66775706135235424 ) ) ;
#56640=CARTESIAN_POINT ( 'NONE',  ( 13.97604488694527802, 13.89961937509977652, 29.37390960531435979 ) ) ;
#56641=CARTESIAN_POINT ( 'NONE',  ( -8.224510206698735004, -14.34966873604973081, 59.58442372801901854 ) ) ;
#56642=CARTESIAN_POINT ( 'NONE',  ( -10.81492255796078084, -18.62759615963271287, 102.0822429386476955 ) ) ;
#56643=CARTESIAN_POINT ( 'NONE',  ( -21.53943276465977519, 0.05219959533907696930, 106.2489096053143811 ) ) ;
#56644=CARTESIAN_POINT ( 'NONE',  ( 19.05341960407617918, -5.049401038297876454, 36.04275706135234003 ) ) ;
#56645=CARTESIAN_POINT ( 'NONE',  ( 19.03943276465977164, -0.05219959533909143690, 58.74890960531435979 ) ) ;
#56647=CARTESIAN_POINT ( 'NONE',  ( -21.52544592524334988, -5.823673210054445271, 68.95942372801901854 ) ) ;
#56648=CARTESIAN_POINT ( 'NONE',  ( -10.81492255796078084, -18.62759615963271287, 62.08224293864769550 ) ) ;
#56649=CARTESIAN_POINT ( 'NONE',  ( -16.55341960407611168, -4.379528057220339221, 41.45724293864769550 ) ) ;
#56650=CARTESIAN_POINT ( 'NONE',  ( -18.62759615963255300, -10.81492255796106328, 74.16775706135231871 ) ) ;
#56651=CARTESIAN_POINT ( 'NONE',  ( -10.72451020669870658, -18.67979575497194134, 109.5844237280190328 ) ) ;
#56652=CARTESIAN_POINT ( 'NONE',  ( -14.34966873604960291, -8.224510206698953496, 61.66557627198103120 ) ) ;
#56653=CARTESIAN_POINT ( 'NONE',  ( -4.379528057220328563, 16.55341960407611168, 110.2072429386477239 ) ) ;
#56654=CARTESIAN_POINT ( 'NONE',  ( -19.03943276465977164, -0.05219959533935918106, 43.75109039468566863 ) ) ;
#56655=CARTESIAN_POINT ( 'NONE',  ( -14.29746914071037622, -8.314922557961029526, 99.16775706135234714 ) ) ;
#56656=CARTESIAN_POINT ( 'NONE',  ( -15.80617190586768217, 15.72974639402176855, 73.12609039468567573 ) ) ;
#56657=CARTESIAN_POINT ( 'NONE',  ( 9.564922557960805705, 16.46253265017160317, 64.58224293864769550 ) ) ;
#56658=CARTESIAN_POINT ( 'NONE',  ( 13.97604488694548053, -13.89961937509957401, 35.62609039468567573 ) ) ;
#56659=CARTESIAN_POINT ( 'NONE',  ( 0.05219959533907565091, 21.53943276465977519, 34.99890960531435979 ) ) ;
#56660=CARTESIAN_POINT ( 'NONE',  ( -10.72451020669870658, -18.67979575497194134, 29.58442372801901854 ) ) ;
#56661=CARTESIAN_POINT ( 'NONE',  ( 18.67979575497178502, 10.72451020669898547, 89.16557627198102409 ) ) ;
#56662=CARTESIAN_POINT ( 'NONE',  ( -9.474510206698720793, -16.51473224551083518, 89.58442372801900433 ) ) ;
#56663=CARTESIAN_POINT ( 'NONE',  ( -0.05219959533934338120, 16.53943276465976808, 52.50109039468567573 ) ) ;
#56665=CARTESIAN_POINT ( 'NONE',  ( 18.62759615963271287, -10.81492255796078972, 93.33224293864769550 ) ) ;
#56666=CARTESIAN_POINT ( 'NONE',  ( 0.05219959533910956823, 16.53943276465976808, 69.99890960531435269 ) ) ;
#56668=CARTESIAN_POINT ( 'NONE',  ( 19.02544592524334988, 5.153800228976608722, 111.4594237280190043 ) ) ;
#56669=CARTESIAN_POINT ( 'NONE',  ( 15.80617190586746368, 15.72974639402197994, 44.37390960531435979 ) ) ;
#56670=CARTESIAN_POINT ( 'NONE',  ( 8.314922557961029526, -14.29746914071037800, 75.41775706135233293 ) ) ;
#56671=LINE ( 'NONE', #86995, #51063 ) ;
#56672=CARTESIAN_POINT ( 'NONE',  ( 14.29746914071037800, 8.314922557961029526, 56.66775706135235424 ) ) ;
#56673=CARTESIAN_POINT ( 'NONE',  ( 10.81492255796106328, -18.62759615963255655, 30.41775706135234358 ) ) ;
#56674=CARTESIAN_POINT ( 'NONE',  ( 18.67979575497178502, 10.72451020669898547, 44.16557627198103120 ) ) ;
#56675=CARTESIAN_POINT ( 'NONE',  ( 0.05219959533934541429, -16.53943276465976808, 75.00109039468568994 ) ) ;
#56676=CARTESIAN_POINT ( 'NONE',  ( 16.46253265017160672, -9.564922557960803928, 103.3322429386476955 ) ) ;
#56677=CARTESIAN_POINT ( 'NONE',  ( -10.81492255796105439, 18.62759615963255655, 57.91775706135234714 ) ) ;
#56678=CARTESIAN_POINT ( 'NONE',  ( -9.474510206698964154, 16.51473224551069663, 25.41557627198103120 ) ) ;
#56679=CARTESIAN_POINT ( 'NONE',  ( -10.72451020669898014, 18.67979575497178502, 40.41557627198103120 ) ) ;
#56680=CARTESIAN_POINT ( 'NONE',  ( 16.51473224551069308, 9.474510206698969483, 114.1655762719810241 ) ) ;
#56682=CARTESIAN_POINT ( 'NONE',  ( -16.51473224551082808, 9.474510206698731452, 33.33442372801899722 ) ) ;
#56683=CARTESIAN_POINT ( 'NONE',  ( 16.52544592524335698, 4.483927247898782831, 56.45942372801902565 ) ) ;
#56684=CARTESIAN_POINT ( 'NONE',  ( 9.564922557960805705, 16.46253265017160317, 109.5822429386476955 ) ) ;
#56686=CARTESIAN_POINT ( 'NONE',  ( 19.02544592524343514, -5.153800228976328945, 88.54057627198102409 ) ) ;
#56687=CARTESIAN_POINT ( 'NONE',  ( 0.05219959533934541429, -16.53943276465976808, 100.0010903946857042 ) ) ;
#56688=CARTESIAN_POINT ( 'NONE',  ( -17.49999999999999289, 5.500000000000036415, 85.79690382534171533 ) ) ;
#56689=CARTESIAN_POINT ( 'NONE',  ( 14.29746914071049879, -8.314922557960816363, 93.33224293864769550 ) ) ;
#56690=CARTESIAN_POINT ( 'NONE',  ( 5.719274019375991003, -21.55341960407610458, 52.70724293864769550 ) ) ;
#56691=CARTESIAN_POINT ( 'NONE',  ( -19.03943276465977164, 0.05219959533909376836, 36.24890960531436690 ) ) ;
#56692=CARTESIAN_POINT ( 'NONE',  ( 16.52544592524335698, 4.483927247898782831, 76.45942372801901854 ) ) ;
#56693=CARTESIAN_POINT ( 'NONE',  ( -21.55341960407619339, 5.719274019375674811, 23.54275706135235424 ) ) ;
#56694=CARTESIAN_POINT ( 'NONE',  ( -19.03943276465977164, -0.05219959533935918106, 93.75109039468566152 ) ) ;
#56695=CARTESIAN_POINT ( 'NONE',  ( 5.049401038298161559, -19.05341960407611168, 42.70724293864767418 ) ) ;
#56697=CARTESIAN_POINT ( 'NONE',  ( -16.51473224551069308, -9.474510206698971260, 106.6655762719810383 ) ) ;
#56698=CARTESIAN_POINT ( 'NONE',  ( -0.05219959533937732626, 21.53943276465977519, 102.5010903946856899 ) ) ;
#56699=CARTESIAN_POINT ( 'NONE',  ( -16.51473224551069308, -9.474510206698971260, 81.66557627198103830 ) ) ;
#56700=CARTESIAN_POINT ( 'NONE',  ( -16.55341960407617563, 4.379528057220093196, 58.54275706135235424 ) ) ;
#56701=CARTESIAN_POINT ( 'NONE',  ( 18.67979575497194134, -10.72451020669871369, 90.83442372801901854 ) ) ;
#56702=CARTESIAN_POINT ( 'NONE',  ( -19.03943276465977164, -0.05219959533935918106, 58.75109039468566863 ) ) ;
#56703=CARTESIAN_POINT ( 'NONE',  ( -0.05219959533936034679, 19.03943276465977164, 72.50109039468566152 ) ) ;
#56705=CARTESIAN_POINT ( 'NONE',  ( 15.80617190586769283, -15.72974639402175789, 60.62609039468567573 ) ) ;
#56707=CARTESIAN_POINT ( 'NONE',  ( 16.51473224551083163, -9.474510206698727899, 60.83442372801900433 ) ) ;
#56708=CARTESIAN_POINT ( 'NONE',  ( -5.049401038298153566, 19.05341960407611168, 105.2072429386476671 ) ) ;
#56709=CARTESIAN_POINT ( 'NONE',  ( 13.97604488694527802, 13.89961937509977652, 79.37390960531435269 ) ) ;
#56710=CARTESIAN_POINT ( 'NONE',  ( -8.224510206698948167, 14.34966873604960824, 40.41557627198103120 ) ) ;
#56711=CARTESIAN_POINT ( 'NONE',  ( -18.67979575497178146, -10.72451020669898902, 31.66557627198102054 ) ) ;
#56714=CARTESIAN_POINT ( 'NONE',  ( 17.50000000000000000, 5.499999999999992895, 56.70309617465829888 ) ) ;
#56715=CARTESIAN_POINT ( 'NONE',  ( -18.67979575497193778, 10.72451020669871902, 113.3344237280190328 ) ) ;
#56717=CARTESIAN_POINT ( 'NONE',  ( 9.474510206698971260, -16.51473224551069308, 32.91557627198102409 ) ) ;
#56718=CARTESIAN_POINT ( 'NONE',  ( 5.153800228976335163, 19.02544592524342804, 24.79057627198102765 ) ) ;
#56721=CARTESIAN_POINT ( 'NONE',  ( -10.81492255796105439, 18.62759615963255655, 67.91775706135234714 ) ) ;
#56723=CARTESIAN_POINT ( 'NONE',  ( -14.29746914071037622, -8.314922557961029526, 69.16775706135234714 ) ) ;
#56724=CARTESIAN_POINT ( 'NONE',  ( 21.52544592524344225, -5.823673210054117533, 83.54057627198102409 ) ) ;
#56726=CARTESIAN_POINT ( 'NONE',  ( -16.53943276465976808, 0.05219959533911058130, 51.24890960531436690 ) ) ;
#56727=CARTESIAN_POINT ( 'NONE',  ( -9.474510206698964154, 16.51473224551069663, 25.41557627198103120 ) ) ;
#56728=CARTESIAN_POINT ( 'NONE',  ( 19.03943276465977164, -0.05219959533909143690, 113.7489096053143669 ) ) ;
#56729=CARTESIAN_POINT ( 'NONE',  ( -21.53943276465977519, -0.05219959533937600094, 28.75109039468567929 ) ) ;
#56730=CARTESIAN_POINT ( 'NONE',  ( 19.02544592524334988, 5.153800228976608722, 31.45942372801900433 ) ) ;
#56731=CARTESIAN_POINT ( 'NONE',  ( -9.474510206698964154, 16.51473224551069663, 40.41557627198103120 ) ) ;
#56732=CARTESIAN_POINT ( 'NONE',  ( -10.72451020669870658, -18.67979575497194134, 84.58442372801903275 ) ) ;
#56734=CARTESIAN_POINT ( 'NONE',  ( 16.52544592524342804, -4.483927247898539470, 23.54057627198102765 ) ) ;
#56736=CARTESIAN_POINT ( 'NONE',  ( 15.72974639402199770, -15.80617190586745480, 43.12390960531435269 ) ) ;
#56737=CARTESIAN_POINT ( 'NONE',  ( 14.34966873604960469, 8.224510206698951720, 99.16557627198100988 ) ) ;
#56739=CARTESIAN_POINT ( 'NONE',  ( -5.049401038298153566, 19.05341960407611168, 95.20724293864770971 ) ) ;
#56740=CARTESIAN_POINT ( 'NONE',  ( 16.55341960407611168, 4.379528057220329451, 93.95724293864770971 ) ) ;
#56741=CARTESIAN_POINT ( 'NONE',  ( -16.46253265017146816, -9.564922557961047289, 104.1677570613523329 ) ) ;
#56742=CARTESIAN_POINT ( 'NONE',  ( 10.81492255796078972, 18.62759615963270932, 59.58224293864770260 ) ) ;
#56743=ORIENTED_EDGE ( 'NONE', *, *, #125362, .T. ) ;
#56744=CARTESIAN_POINT ( 'NONE',  ( -13.97604488694527625, -13.89961937509977652, 26.87390960531434558 ) ) ;
#56745=CARTESIAN_POINT ( 'NONE',  ( -19.03943276465977164, 0.05219959533909376836, 81.24890960531436690 ) ) ;
#56746=CARTESIAN_POINT ( 'NONE',  ( 0.05219959533907565091, 21.53943276465977519, 89.99890960531438111 ) ) ;
#56747=CARTESIAN_POINT ( 'NONE',  ( 12.14591786802327356, -12.06949235617739191, 110.6260903946857042 ) ) ;
#56748=CARTESIAN_POINT ( 'NONE',  ( 16.51473224551069308, 9.474510206698969483, 84.16557627198102409 ) ) ;
#56749=CARTESIAN_POINT ( 'NONE',  ( -0.05219959533936034679, 19.03943276465977164, 77.50109039468566152 ) ) ;
#56750=CARTESIAN_POINT ( 'NONE',  ( -21.53943276465977519, -0.05219959533937600094, 88.75109039468567573 ) ) ;
#56751=CARTESIAN_POINT ( 'NONE',  ( -18.67979575497178146, -10.72451020669898902, 71.66557627198100988 ) ) ;
#56752=CARTESIAN_POINT ( 'NONE',  ( -5.823673210054116645, -21.52544592524344225, 37.29057627198102409 ) ) ;
#56753=CARTESIAN_POINT ( 'NONE',  ( -16.46253265017160317, 9.564922557960807481, 45.83224293864769550 ) ) ;
#56754=CARTESIAN_POINT ( 'NONE',  ( -4.483927247898782831, 16.52544592524335698, 107.7094237280190328 ) ) ;
#56755=CARTESIAN_POINT ( 'NONE',  ( -9.474510206698964154, 16.51473224551069663, 65.41557627198102409 ) ) ;
#56757=CARTESIAN_POINT ( 'NONE',  ( -13.89961937509957401, -13.97604488694547875, 24.37609039468565442 ) ) ;
#56758=CARTESIAN_POINT ( 'NONE',  ( -4.379528057220328563, 16.55341960407611168, 70.20724293864769550 ) ) ;
#56759=CARTESIAN_POINT ( 'NONE',  ( -15.72974639402197994, 15.80617190586746368, 115.6239096053143669 ) ) ;
#56761=CARTESIAN_POINT ( 'NONE',  ( 18.67979575497178502, 10.72451020669898547, 54.16557627198103120 ) ) ;
#56762=CARTESIAN_POINT ( 'NONE',  ( -16.52544592524335698, -4.483927247898792601, 93.95942372801903275 ) ) ;
#56763=CARTESIAN_POINT ( 'NONE',  ( 16.52544592524342804, -4.483927247898539470, 108.5405762719810241 ) ) ;
#56764=CARTESIAN_POINT ( 'NONE',  ( -13.89961937509977652, 13.97604488694528158, 70.62390960531432427 ) ) ;
#56765=CARTESIAN_POINT ( 'NONE',  ( 16.53943276465976808, -0.05219959533910856209, 28.74890960531435624 ) ) ;
#56766=CARTESIAN_POINT ( 'NONE',  ( -15.80617190586768217, 15.72974639402176855, 53.12609039468568284 ) ) ;
#56767=CARTESIAN_POINT ( 'NONE',  ( 19.05341960407611168, 5.049401038298154454, 103.9572429386476671 ) ) ;
#56768=CARTESIAN_POINT ( 'NONE',  ( 5.719274019375673035, 21.55341960407619339, 77.29275706135234714 ) ) ;
#56769=CARTESIAN_POINT ( 'NONE',  ( -19.05341960407611168, -5.049401038298163336, 31.45724293864769550 ) ) ;
#56770=CARTESIAN_POINT ( 'NONE',  ( 19.03943276465977164, -0.05219959533909143690, 33.74890960531435979 ) ) ;
#56772=CARTESIAN_POINT ( 'NONE',  ( -5.719274019375665041, -21.55341960407619695, 94.79275706135234714 ) ) ;
#56773=CARTESIAN_POINT ( 'NONE',  ( -16.53943276465976808, -0.05219959533934237506, 53.75109039468568994 ) ) ;
#56774=CARTESIAN_POINT ( 'NONE',  ( -21.53943276465977519, -0.05219959533937600094, 73.75109039468567573 ) ) ;
#56775=CARTESIAN_POINT ( 'NONE',  ( 5.153800228976335163, 19.02544592524342804, 104.7905762719809957 ) ) ;
#56777=CARTESIAN_POINT ( 'NONE',  ( -13.89961937509957401, -13.97604488694547875, 79.37609039468567573 ) ) ;
#56778=CARTESIAN_POINT ( 'NONE',  ( 21.55341960407619695, -5.719274019375665929, 51.04275706135234714 ) ) ;
#56779=CARTESIAN_POINT ( 'NONE',  ( 14.34966873604972726, -8.224510206698740333, 25.83442372801901499 ) ) ;
#56781=CARTESIAN_POINT ( 'NONE',  ( -16.46253265017146816, -9.564922557961047289, 79.16775706135234714 ) ) ;
#56782=CARTESIAN_POINT ( 'NONE',  ( -5.049401038298153566, 19.05341960407611168, 55.20724293864769550 ) ) ;
#56783=CARTESIAN_POINT ( 'NONE',  ( -16.51473224551082808, 9.474510206698731452, 93.33442372801900433 ) ) ;
#56784=CARTESIAN_POINT ( 'NONE',  ( -4.483927247898782831, 16.52544592524335698, 112.7094237280190328 ) ) ;
#56785=CARTESIAN_POINT ( 'NONE',  ( -19.05341960407617563, 5.049401038297882671, 83.54275706135233293 ) ) ;
#56786=CARTESIAN_POINT ( 'NONE',  ( 4.379528057220339221, -16.55341960407611168, 37.70724293864769550 ) ) ;
#56787=CARTESIAN_POINT ( 'NONE',  ( 19.02544592524334988, 5.153800228976608722, 66.45942372801899012 ) ) ;
#56788=CARTESIAN_POINT ( 'NONE',  ( 4.379528057220092307, 16.55341960407617563, 57.29275706135234714 ) ) ;
#56789=CARTESIAN_POINT ( 'NONE',  ( 19.03943276465977164, 0.05219959533936151252, 21.25109039468565797 ) ) ;
#56790=CARTESIAN_POINT ( 'NONE',  ( 19.03943276465977164, -0.05219959533909143690, 28.74890960531435624 ) ) ;
#56791=CARTESIAN_POINT ( 'NONE',  ( 5.049401038298161559, -19.05341960407611168, 42.70724293864767418 ) ) ;
#56792=CARTESIAN_POINT ( 'NONE',  ( 8.224510206698742110, 14.34966873604972548, 42.08442372801901854 ) ) ;
#56795=CARTESIAN_POINT ( 'NONE',  ( -9.564922557960796823, -16.46253265017161027, 97.08224293864769550 ) ) ;
#56798=CARTESIAN_POINT ( 'NONE',  ( 9.564922557961047289, -16.46253265017146816, 95.41775706135233293 ) ) ;
#56799=CARTESIAN_POINT ( 'NONE',  ( 10.81492255796078972, 18.62759615963270932, 34.58224293864770260 ) ) ;
#56800=CARTESIAN_POINT ( 'NONE',  ( -19.03943276465977164, -0.05219959533935918106, 33.75109039468566863 ) ) ;
#56801=CARTESIAN_POINT ( 'NONE',  ( 16.52544592524335698, 4.483927247898782831, 21.45942372801901499 ) ) ;
#56802=CARTESIAN_POINT ( 'NONE',  ( -16.53943276465976808, 0.05219959533911058130, 106.2489096053143811 ) ) ;
#56803=CARTESIAN_POINT ( 'NONE',  ( 16.46253265017160672, -9.564922557960803928, 38.33224293864768839 ) ) ;
#56804=CARTESIAN_POINT ( 'NONE',  ( -15.72974639402197994, 15.80617190586746368, 70.62390960531436690 ) ) ;
#56805=CARTESIAN_POINT ( 'NONE',  ( -19.05341960407611168, -5.049401038298163336, 31.45724293864769550 ) ) ;
#56807=CARTESIAN_POINT ( 'NONE',  ( -19.03943276465977164, -0.05219959533935918106, 68.75109039468566152 ) ) ;
#56808=CARTESIAN_POINT ( 'NONE',  ( 12.06949235617757843, -12.14591786802309237, 48.12390960531436690 ) ) ;
#56809=CARTESIAN_POINT ( 'NONE',  ( 10.81492255796078972, 18.62759615963270932, 39.58224293864769550 ) ) ;
#56810=CARTESIAN_POINT ( 'NONE',  ( -18.67979575497193778, 10.72451020669871902, 88.33442372801901854 ) ) ;
#56811=CARTESIAN_POINT ( 'NONE',  ( 18.67979575497178502, 10.72451020669898547, 79.16557627198103830 ) ) ;
#56812=CARTESIAN_POINT ( 'NONE',  ( -21.55341960407619339, 5.719274019375674811, 73.54275706135234714 ) ) ;
#56813=CARTESIAN_POINT ( 'NONE',  ( -10.72451020669870658, -18.67979575497194134, 59.58442372801901854 ) ) ;
#56814=CARTESIAN_POINT ( 'NONE',  ( -19.05341960407611168, -5.049401038298163336, 101.4572429386476955 ) ) ;
#56815=CARTESIAN_POINT ( 'NONE',  ( -0.05219959533934338120, 16.53943276465976808, 107.5010903946856899 ) ) ;
#56816=CARTESIAN_POINT ( 'NONE',  ( 5.719274019375673035, 21.55341960407619339, 67.29275706135234714 ) ) ;
#56817=CARTESIAN_POINT ( 'NONE',  ( 9.474510206698971260, -16.51473224551069308, 52.91557627198102409 ) ) ;
#56818=CARTESIAN_POINT ( 'NONE',  ( 15.80617190586769283, -15.72974639402175789, 30.62609039468567929 ) ) ;
#56819=CARTESIAN_POINT ( 'NONE',  ( 13.89961937509977652, -13.97604488694527269, 63.12390960531435979 ) ) ;
#56820=CARTESIAN_POINT ( 'NONE',  ( -16.52544592524342804, 4.483927247898546575, 86.04057627198102409 ) ) ;
#56821=CARTESIAN_POINT ( 'NONE',  ( 4.379528057220339221, -16.55341960407611168, 52.70724293864769550 ) ) ;
#56822=CARTESIAN_POINT ( 'NONE',  ( -18.62759615963270932, 10.81492255796079327, 55.83224293864770260 ) ) ;
#56823=CARTESIAN_POINT ( 'NONE',  ( 13.89961937509977652, -13.97604488694527269, 43.12390960531434558 ) ) ;
#56824=CARTESIAN_POINT ( 'NONE',  ( 21.55341960407610458, 5.719274019375980345, 53.95724293864770260 ) ) ;
#56825=CARTESIAN_POINT ( 'NONE',  ( -0.05219959533936034679, 19.03943276465977164, 57.50109039468566863 ) ) ;
#56826=CARTESIAN_POINT ( 'NONE',  ( -19.05341960407617918, 5.049401038297883559, 23.54275706135233648 ) ) ;
#56827=CARTESIAN_POINT ( 'NONE',  ( -4.483927247898539470, -16.52544592524342804, 62.29057627198102409 ) ) ;
#56828=CARTESIAN_POINT ( 'NONE',  ( 5.823673210054125526, 21.52544592524343514, 39.79057627198103830 ) ) ;
#56831=CARTESIAN_POINT ( 'NONE',  ( 12.06949235617739724, 12.14591786802326823, 86.87609039468568994 ) ) ;
#56833=CARTESIAN_POINT ( 'NONE',  ( 13.97604488694548053, -13.89961937509957401, 85.62609039468568994 ) ) ;
#56834=CARTESIAN_POINT ( 'NONE',  ( -16.55341960407611168, -4.379528057220339221, 56.45724293864768839 ) ) ;
#56835=CARTESIAN_POINT ( 'NONE',  ( -19.49671883438228193, -5.499999999999978684, 59.89279849105680853 ) ) ;
#56836=CARTESIAN_POINT ( 'NONE',  ( 19.03943276465977164, -0.05219959533909143690, 48.74890960531435979 ) ) ;
#56837=CARTESIAN_POINT ( 'NONE',  ( -16.55341960407611168, -4.379528057220339221, 46.45724293864769550 ) ) ;
#56838=CARTESIAN_POINT ( 'NONE',  ( 13.89961937509977652, -13.97604488694527269, 93.12390960531436690 ) ) ;
#56839=CARTESIAN_POINT ( 'NONE',  ( -13.89961937509977652, 13.97604488694528158, 55.62390960531434558 ) ) ;
#56840=CARTESIAN_POINT ( 'NONE',  ( 5.719274019375673035, 21.55341960407619339, 57.29275706135234714 ) ) ;
#56841=CARTESIAN_POINT ( 'NONE',  ( -9.564922557960796823, -16.46253265017161027, 72.08224293864770971 ) ) ;
#56842=CARTESIAN_POINT ( 'NONE',  ( 9.474510206698971260, -16.51473224551069308, 32.91557627198102409 ) ) ;
#56843=CARTESIAN_POINT ( 'NONE',  ( 9.474510206698971260, -16.51473224551069308, 57.91557627198103120 ) ) ;
#56844=CARTESIAN_POINT ( 'NONE',  ( 5.719274019375991003, -21.55341960407610458, 52.70724293864769550 ) ) ;
#56845=CARTESIAN_POINT ( 'NONE',  ( 5.153800228976335163, 19.02544592524342804, 29.79057627198102409 ) ) ;
#56846=CARTESIAN_POINT ( 'NONE',  ( 10.81492255796078972, 18.62759615963270932, 39.58224293864769550 ) ) ;
#56847=CARTESIAN_POINT ( 'NONE',  ( 12.06949235617739724, 12.14591786802326823, 101.8760903946857042 ) ) ;
#56849=CARTESIAN_POINT ( 'NONE',  ( -16.46253265017146816, -9.564922557961047289, 19.16775706135233293 ) ) ;
#56850=CARTESIAN_POINT ( 'NONE',  ( 16.55341960407618274, -4.379528057220086978, 41.04275706135236135 ) ) ;
#56851=CARTESIAN_POINT ( 'NONE',  ( 4.379528057220092307, 16.55341960407617563, 77.29275706135234714 ) ) ;
#56853=CARTESIAN_POINT ( 'NONE',  ( -16.55341960407617563, 4.379528057220093196, 68.54275706135234714 ) ) ;
#56854=CARTESIAN_POINT ( 'NONE',  ( -14.29746914071037622, -8.314922557961029526, 54.16775706135235424 ) ) ;
#56855=CARTESIAN_POINT ( 'NONE',  ( 13.89961937509977652, -13.97604488694527269, 108.1239096053143669 ) ) ;
#56856=CARTESIAN_POINT ( 'NONE',  ( -9.474510206698964154, 16.51473224551069663, 30.41557627198102054 ) ) ;
#56857=CARTESIAN_POINT ( 'NONE',  ( 8.224510206698742110, 14.34966873604972548, 32.08442372801901854 ) ) ;
#56858=CARTESIAN_POINT ( 'NONE',  ( -5.049401038298153566, 19.05341960407611168, 45.20724293864769550 ) ) ;
#56859=CARTESIAN_POINT ( 'NONE',  ( 21.53943276465977519, 0.05219959533937863772, 31.25109039468568639 ) ) ;
#56860=CARTESIAN_POINT ( 'NONE',  ( 16.52544592524335698, 4.483927247898782831, 41.45942372801901143 ) ) ;
#56861=CARTESIAN_POINT ( 'NONE',  ( 16.53943276465976808, 0.05219959533934440121, 101.2510903946856757 ) ) ;
#56863=CARTESIAN_POINT ( 'NONE',  ( -10.81492255796105439, 18.62759615963255655, 102.9177570613523756 ) ) ;
#56864=CARTESIAN_POINT ( 'NONE',  ( -13.97604488694547697, 13.89961937509957934, 103.1260903946856473 ) ) ;
#56865=CARTESIAN_POINT ( 'NONE',  ( 16.52544592524342804, -4.483927247898539470, 53.54057627198103120 ) ) ;
#56866=CARTESIAN_POINT ( 'NONE',  ( -5.153800228976328057, -19.02544592524343514, 27.29057627198103120 ) ) ;
#56867=CARTESIAN_POINT ( 'NONE',  ( -19.03943276465977164, -0.05219959533935918106, 58.75109039468566863 ) ) ;
#56868=CARTESIAN_POINT ( 'NONE',  ( 17.05587630539706012, -6.762274262136750203, 58.24180309037282655 ) ) ;
#56869=CARTESIAN_POINT ( 'NONE',  ( 21.52544592524334988, 5.823673210054432836, 61.45942372801901854 ) ) ;
#56870=CARTESIAN_POINT ( 'NONE',  ( -12.14591786802326823, 12.06949235617739902, 28.12609039468568284 ) ) ;
#56872=CARTESIAN_POINT ( 'NONE',  ( 10.72451020669898902, -18.67979575497178502, 27.91557627198103830 ) ) ;
#56873=CARTESIAN_POINT ( 'NONE',  ( -19.05341960407617563, 5.049401038297882671, 113.5427570613523471 ) ) ;
#56876=CARTESIAN_POINT ( 'NONE',  ( 16.51473224551069308, 9.474510206698969483, 24.16557627198102765 ) ) ;
#56877=CARTESIAN_POINT ( 'NONE',  ( -5.823673210054431948, 21.52544592524334988, 102.7094237280190185 ) ) ;
#56878=CARTESIAN_POINT ( 'NONE',  ( -19.02544592524342804, 5.153800228976336051, 46.04057627198101699 ) ) ;
#56879=AXIS2_PLACEMENT_3D ( 'NONE', #80792, #171828, #34306 ) ;
#56880=CARTESIAN_POINT ( 'NONE',  ( -10.81492255796105439, 18.62759615963255655, 62.91775706135236135 ) ) ;
#56881=CARTESIAN_POINT ( 'NONE',  ( -5.719274019375665041, -21.55341960407619695, 99.79275706135234714 ) ) ;
#56882=CARTESIAN_POINT ( 'NONE',  ( 4.379528057220092307, 16.55341960407617563, 102.2927570613523613 ) ) ;
#56883=CARTESIAN_POINT ( 'NONE',  ( -13.89961937509977652, 13.97604488694528158, 75.62390960531438111 ) ) ;
#56884=CARTESIAN_POINT ( 'NONE',  ( -15.72974639402176322, -15.80617190586768395, 59.37609039468568284 ) ) ;
#56885=CARTESIAN_POINT ( 'NONE',  ( -15.72974639402176322, -15.80617190586768395, 54.37609039468568994 ) ) ;
#56886=CARTESIAN_POINT ( 'NONE',  ( -9.474510206698720793, -16.51473224551083518, 74.58442372801900433 ) ) ;
#56887=CARTESIAN_POINT ( 'NONE',  ( -0.05219959533909027116, -19.03943276465977164, 97.49890960531436690 ) ) ;
#56888=CARTESIAN_POINT ( 'NONE',  ( 9.564922557960805705, 16.46253265017160317, 24.58224293864769194 ) ) ;
#56889=CARTESIAN_POINT ( 'NONE',  ( -21.52544592524343514, 5.823673210054127303, 91.04057627198103830 ) ) ;
#56890=CARTESIAN_POINT ( 'NONE',  ( -5.823673210054431948, 21.52544592524334988, 112.7094237280190328 ) ) ;
#56891=CARTESIAN_POINT ( 'NONE',  ( 8.314922557960818139, 14.29746914071049879, 94.58224293864769550 ) ) ;
#56892=CARTESIAN_POINT ( 'NONE',  ( -19.02544592524342804, 5.153800228976336051, 46.04057627198101699 ) ) ;
#56893=CARTESIAN_POINT ( 'NONE',  ( -19.02544592524334988, -5.153800228976617603, 78.95942372801900433 ) ) ;
#56894=CARTESIAN_POINT ( 'NONE',  ( 14.34966873604960469, 8.224510206698951720, 59.16557627198103120 ) ) ;
#56895=CARTESIAN_POINT ( 'NONE',  ( -18.67979575497193778, 10.72451020669871902, 108.3344237280190185 ) ) ;
#56896=CARTESIAN_POINT ( 'NONE',  ( 19.03943276465977164, -0.05219959533909143690, 108.7489096053143527 ) ) ;
#56897=CARTESIAN_POINT ( 'NONE',  ( 9.474510206698729675, 16.51473224551082808, 77.08442372801900433 ) ) ;
#56898=CARTESIAN_POINT ( 'NONE',  ( 15.72974639402199770, -15.80617190586745480, 73.12390960531436690 ) ) ;
#56899=CARTESIAN_POINT ( 'NONE',  ( 21.52544592524334988, 5.823673210054432836, 26.45942372801901854 ) ) ;
#56900=CARTESIAN_POINT ( 'NONE',  ( -16.55341960407617563, 4.379528057220093196, 23.54275706135235424 ) ) ;
#56901=CARTESIAN_POINT ( 'NONE',  ( -12.06949235617739369, -12.14591786802326823, 99.37609039468568994 ) ) ;
#56902=CARTESIAN_POINT ( 'NONE',  ( 16.52544592524335698, 4.483927247898782831, 41.45942372801901143 ) ) ;
#56903=CARTESIAN_POINT ( 'NONE',  ( 5.823673210054444382, -21.52544592524334988, 35.20942372801901854 ) ) ;
#56904=CARTESIAN_POINT ( 'NONE',  ( 10.81492255796078972, 18.62759615963270932, 44.58224293864769550 ) ) ;
#56905=CARTESIAN_POINT ( 'NONE',  ( -9.564922557960796823, -16.46253265017161027, 37.08224293864768839 ) ) ;
#56907=CARTESIAN_POINT ( 'NONE',  ( -0.05219959533934338120, 16.53943276465976808, 57.50109039468568994 ) ) ;
#56908=CARTESIAN_POINT ( 'NONE',  ( -5.719274019375978568, 21.55341960407610458, 90.20724293864770971 ) ) ;
#56909=CARTESIAN_POINT ( 'NONE',  ( -4.483927247898539470, -16.52544592524342804, 27.29057627198103120 ) ) ;
#56910=CARTESIAN_POINT ( 'NONE',  ( -12.14591786802326823, 12.06949235617739902, 43.12609039468568284 ) ) ;
#56911=CARTESIAN_POINT ( 'NONE',  ( -16.51473224551069308, -9.474510206698971260, 56.66557627198103120 ) ) ;
#56912=CARTESIAN_POINT ( 'NONE',  ( -16.55341960407617563, 4.379528057220093196, 88.54275706135236135 ) ) ;
#56913=CARTESIAN_POINT ( 'NONE',  ( -5.049401038297874678, -19.05341960407617918, 89.79275706135230450 ) ) ;
#56914=CARTESIAN_POINT ( 'NONE',  ( 18.62759615963271287, -10.81492255796078972, 88.33224293864769550 ) ) ;
#56915=CARTESIAN_POINT ( 'NONE',  ( -4.483927247898539470, -16.52544592524342804, 27.29057627198103120 ) ) ;
#56918=CARTESIAN_POINT ( 'NONE',  ( 0.05219959533907565091, 21.53943276465977519, 54.99890960531435269 ) ) ;
#56920=CARTESIAN_POINT ( 'NONE',  ( -4.379528057220086978, -16.55341960407618274, 104.7927570613523898 ) ) ;
#56922=CARTESIAN_POINT ( 'NONE',  ( 18.62759615963271287, -10.81492255796078972, 33.33224293864769550 ) ) ;
#56923=CARTESIAN_POINT ( 'NONE',  ( -15.72974639402197994, 15.80617190586746368, 90.62390960531436690 ) ) ;
#56925=CARTESIAN_POINT ( 'NONE',  ( -14.34966873604960291, -8.224510206698953496, 21.66557627198102409 ) ) ;
#56926=CARTESIAN_POINT ( 'NONE',  ( 12.14591786802327356, -12.06949235617739191, 40.62609039468567573 ) ) ;
#56927=CARTESIAN_POINT ( 'NONE',  ( -13.89961937509977652, 13.97604488694528158, 30.62390960531435269 ) ) ;
#56928=CARTESIAN_POINT ( 'NONE',  ( 8.224510206698742110, 14.34966873604972548, 27.08442372801901854 ) ) ;
#56929=CARTESIAN_POINT ( 'NONE',  ( 19.03943276465977164, -0.05219959533909143690, 58.74890960531435979 ) ) ;
#56930=ADVANCED_FACE ( 'NONE', ( #102962 ), #197964, .F. ) ;
#56932=CARTESIAN_POINT ( 'NONE',  ( 16.46253265017160672, -9.564922557960803928, 108.3322429386476955 ) ) ;
#56933=CARTESIAN_POINT ( 'NONE',  ( 16.46253265017160672, -9.564922557960803928, 113.3322429386476955 ) ) ;
#56934=CARTESIAN_POINT ( 'NONE',  ( 14.29746914071037800, 8.314922557961029526, 96.66775706135234714 ) ) ;
#56935=CARTESIAN_POINT ( 'NONE',  ( 19.02544592524334988, 5.153800228976608722, 96.45942372801897591 ) ) ;
#56936=CARTESIAN_POINT ( 'NONE',  ( -19.02544592524334988, -5.153800228976617603, 43.95942372801899012 ) ) ;
#56937=CARTESIAN_POINT ( 'NONE',  ( 5.719274019375991003, -21.55341960407610458, 77.70724293864770971 ) ) ;
#56938=CARTESIAN_POINT ( 'NONE',  ( -14.34966873604972548, 8.224510206698743886, 98.33442372801901854 ) ) ;
#56939=CARTESIAN_POINT ( 'NONE',  ( -18.67979575497178146, -10.72451020669898902, 26.66557627198103475 ) ) ;
#56940=CARTESIAN_POINT ( 'NONE',  ( 5.049401038297881783, 19.05341960407617563, 102.2927570613523045 ) ) ;
#56941=CARTESIAN_POINT ( 'NONE',  ( 0.05219959533909260263, 19.03943276465977164, 109.9989096053143669 ) ) ;
#56942=CARTESIAN_POINT ( 'NONE',  ( -21.52544592524334988, -5.823673210054445271, 58.95942372801902565 ) ) ;
#56943=CARTESIAN_POINT ( 'NONE',  ( -5.153800228976328057, -19.02544592524343514, 62.29057627198100988 ) ) ;
#56944=CARTESIAN_POINT ( 'NONE',  ( -14.29746914071049879, 8.314922557960819915, 100.8322429386477097 ) ) ;
#56946=CARTESIAN_POINT ( 'NONE',  ( 14.29746914071049879, -8.314922557960816363, 83.33224293864769550 ) ) ;
#56948=CARTESIAN_POINT ( 'NONE',  ( 13.97604488694548053, -13.89961937509957401, 85.62609039468568994 ) ) ;
#56949=CARTESIAN_POINT ( 'NONE',  ( 19.25918095147779496, 5.499999999999526601, 91.95284276293935477 ) ) ;
#56950=CARTESIAN_POINT ( 'NONE',  ( 16.46253265017160672, -9.564922557960803928, 63.33224293864769550 ) ) ;
#56951=CARTESIAN_POINT ( 'NONE',  ( 16.31925111598410183, -7.325300261831686477, 72.66424538967171998 ) ) ;
#56952=CARTESIAN_POINT ( 'NONE',  ( -5.153800228976328057, -19.02544592524343514, 77.29057627198099567 ) ) ;
#56953=CARTESIAN_POINT ( 'NONE',  ( 19.05341960407611168, 5.049401038298154454, 83.95724293864766707 ) ) ;
#56954=CARTESIAN_POINT ( 'NONE',  ( -12.06949235617739369, -12.14591786802326823, 69.37609039468567573 ) ) ;
#56956=CARTESIAN_POINT ( 'NONE',  ( -5.153800228976607833, 19.02544592524334988, 37.70942372801899722 ) ) ;
#56958=CARTESIAN_POINT ( 'NONE',  ( -5.049401038298153566, 19.05341960407611168, 110.2072429386476671 ) ) ;
#56959=CARTESIAN_POINT ( 'NONE',  ( 8.224510206698742110, 14.34966873604972548, 107.0844237280190043 ) ) ;
#56961=CARTESIAN_POINT ( 'NONE',  ( -4.483927247898782831, 16.52544592524335698, 97.70942372801904696 ) ) ;
#56962=CARTESIAN_POINT ( 'NONE',  ( -16.19135201231369692, 7.376712067591784106, 29.81319145947969673 ) ) ;
#56963=CARTESIAN_POINT ( 'NONE',  ( -4.483927247898782831, 16.52544592524335698, 72.70942372801901854 ) ) ;
#56965=CARTESIAN_POINT ( 'NONE',  ( -0.05219959533937732626, 21.53943276465977519, 82.50109039468568994 ) ) ;
#56966=CARTESIAN_POINT ( 'NONE',  ( -13.97604488694547697, 13.89961937509957934, 83.12609039468564731 ) ) ;
#56967=CARTESIAN_POINT ( 'NONE',  ( 5.049401038297881783, 19.05341960407617563, 32.29275706135233293 ) ) ;
#56968=CARTESIAN_POINT ( 'NONE',  ( -13.89961937509977652, 13.97604488694528158, 60.62390960531436690 ) ) ;
#56969=CARTESIAN_POINT ( 'NONE',  ( 13.89961937509977652, -13.97604488694527269, 43.12390960531434558 ) ) ;
#56971=CARTESIAN_POINT ( 'NONE',  ( -18.67979575497178146, -10.72451020669898902, 81.66557627198103830 ) ) ;
#56972=CARTESIAN_POINT ( 'NONE',  ( 15.72974639402199770, -15.80617190586745480, 28.12390960531435979 ) ) ;
#56973=CARTESIAN_POINT ( 'NONE',  ( 19.05341960407611168, 5.049401038298154454, 33.95724293864769550 ) ) ;
#56974=CARTESIAN_POINT ( 'NONE',  ( 8.314922557961029526, -14.29746914071037800, 55.41775706135234714 ) ) ;
#56975=ORIENTED_EDGE ( 'NONE', *, *, #11642, .T. ) ;
#56976=CARTESIAN_POINT ( 'NONE',  ( 21.55341960407619695, -5.719274019375665929, 31.04275706135234714 ) ) ;
#56977=CARTESIAN_POINT ( 'NONE',  ( -16.52544592524342804, 4.483927247898546575, 56.04057627198102409 ) ) ;
#56979=CARTESIAN_POINT ( 'NONE',  ( 0.05219959533934541429, -16.53943276465976808, 30.00109039468568284 ) ) ;
#56980=CARTESIAN_POINT ( 'NONE',  ( -9.564922557961040184, 16.46253265017147172, 42.91775706135234003 ) ) ;
#56981=CARTESIAN_POINT ( 'NONE',  ( 14.34966873604960469, 8.224510206698951720, 54.16557627198103120 ) ) ;
#56982=CARTESIAN_POINT ( 'NONE',  ( 10.81492255796106328, -18.62759615963255655, 20.41775706135234714 ) ) ;
#56984=CARTESIAN_POINT ( 'NONE',  ( -21.55341960407610458, -5.719274019375992779, 76.45724293864769550 ) ) ;
#56985=CARTESIAN_POINT ( 'NONE',  ( 19.05341960407611168, 5.049401038298154454, 88.95724293864769550 ) ) ;
#56986=CARTESIAN_POINT ( 'NONE',  ( -16.52544592524342804, 4.483927247898546575, 61.04057627198103120 ) ) ;
#56987=CARTESIAN_POINT ( 'NONE',  ( -13.89961937509977652, 13.97604488694528158, 110.6239096053143243 ) ) ;
#56989=CARTESIAN_POINT ( 'NONE',  ( 16.51473224551083163, -9.474510206698727899, 70.83442372801900433 ) ) ;
#56990=CARTESIAN_POINT ( 'NONE',  ( 5.719274019375991003, -21.55341960407610458, 112.7072429386476955 ) ) ;
#56991=CARTESIAN_POINT ( 'NONE',  ( -19.03943276465977164, 0.05219959533909376836, 56.24890960531435979 ) ) ;
#56992=CARTESIAN_POINT ( 'NONE',  ( -5.049401038297874678, -19.05341960407617918, 49.79275706135231871 ) ) ;
#56993=CARTESIAN_POINT ( 'NONE',  ( 12.06949235617757843, -12.14591786802309237, 108.1239096053143811 ) ) ;
#56994=CARTESIAN_POINT ( 'NONE',  ( 10.81492255796106328, -18.62759615963255655, 60.41775706135235424 ) ) ;
#56995=CARTESIAN_POINT ( 'NONE',  ( -17.31747979337951548, -6.344076630960985064, 71.37944868065186199 ) ) ;
#56996=CARTESIAN_POINT ( 'NONE',  ( -16.55341960407611168, -4.379528057220339221, 36.45724293864768839 ) ) ;
#56997=CARTESIAN_POINT ( 'NONE',  ( 13.97604488694527802, 13.89961937509977652, 69.37390960531436690 ) ) ;
#56998=CARTESIAN_POINT ( 'NONE',  ( 10.81492255796078972, 18.62759615963270932, 79.58224293864769550 ) ) ;
#57000=CARTESIAN_POINT ( 'NONE',  ( -19.02544592524342804, 5.153800228976336051, 46.04057627198101699 ) ) ;
#57001=ORIENTED_EDGE ( 'NONE', *, *, #105079, .F. ) ;
#57002=CARTESIAN_POINT ( 'NONE',  ( 21.55341960407610458, 5.719274019375980345, 63.95724293864770260 ) ) ;
#57004=CARTESIAN_POINT ( 'NONE',  ( 5.823673210054444382, -21.52544592524334988, 100.2094237280190043 ) ) ;
#57005=CARTESIAN_POINT ( 'NONE',  ( -15.49999999999999822, 5.499999999999998224, 20.00000000000000000 ) ) ;
#57006=CARTESIAN_POINT ( 'NONE',  ( 12.06949235617739724, 12.14591786802326823, 96.87609039468568994 ) ) ;
#57007=CARTESIAN_POINT ( 'NONE',  ( 16.55341960407611168, 4.379528057220329451, 78.95724293864769550 ) ) ;
#57008=CARTESIAN_POINT ( 'NONE',  ( -16.46253265017160317, 9.564922557960807481, 75.83224293864769550 ) ) ;
#57010=CARTESIAN_POINT ( 'NONE',  ( 9.474510206698729675, 16.51473224551082808, 37.08442372801899722 ) ) ;
#57011=CARTESIAN_POINT ( 'NONE',  ( -16.52544592524335698, -4.483927247898792601, 93.95942372801903275 ) ) ;
#57012=CARTESIAN_POINT ( 'NONE',  ( -16.51473224551082808, 9.474510206698731452, 28.33442372801900433 ) ) ;
#57013=CARTESIAN_POINT ( 'NONE',  ( -13.89961937509977652, 13.97604488694528158, 90.62390960531432427 ) ) ;
#57014=CARTESIAN_POINT ( 'NONE',  ( 10.81492255796078972, 18.62759615963270932, 44.58224293864769550 ) ) ;
#57016=CARTESIAN_POINT ( 'NONE',  ( 0.05219959533909260263, 19.03943276465977164, 24.99890960531435269 ) ) ;
#57017=CARTESIAN_POINT ( 'NONE',  ( -15.80617190586768217, 15.72974639402176855, 93.12609039468568994 ) ) ;
#57018=CARTESIAN_POINT ( 'NONE',  ( 12.06949235617739724, 12.14591786802326823, 66.87609039468568994 ) ) ;
#57019=CARTESIAN_POINT ( 'NONE',  ( 5.823673210054125526, 21.52544592524343514, 114.7905762719810383 ) ) ;
#57020=CARTESIAN_POINT ( 'NONE',  ( -16.55341960407617563, 4.379528057220093196, 28.54275706135234358 ) ) ;
#57021=CARTESIAN_POINT ( 'NONE',  ( -13.97604488694527625, -13.89961937509977652, 96.87390960531433848 ) ) ;
#57022=CARTESIAN_POINT ( 'NONE',  ( -16.46253265017160317, 9.564922557960807481, 45.83224293864769550 ) ) ;
#57023=CARTESIAN_POINT ( 'NONE',  ( 13.89961937509977652, -13.97604488694527269, 48.12390960531435979 ) ) ;
#57025=CARTESIAN_POINT ( 'NONE',  ( 16.53943276465976808, 0.05219959533934440121, 31.25109039468568639 ) ) ;
#57026=CARTESIAN_POINT ( 'NONE',  ( 16.52544592524342804, -4.483927247898539470, 98.54057627198105251 ) ) ;
#57027=CARTESIAN_POINT ( 'NONE',  ( 8.314922557961029526, -14.29746914071037800, 105.4177570613523613 ) ) ;
#57028=CARTESIAN_POINT ( 'NONE',  ( 15.72974639402176855, 15.80617190586768217, 46.87609039468568994 ) ) ;
#57029=CARTESIAN_POINT ( 'NONE',  ( 19.05341960407611168, 5.049401038298154454, 78.95724293864769550 ) ) ;
#57030=CARTESIAN_POINT ( 'NONE',  ( 5.049401038298161559, -19.05341960407611168, 52.70724293864767418 ) ) ;
#57031=CARTESIAN_POINT ( 'NONE',  ( 9.474510206698971260, -16.51473224551069308, 87.91557627198102409 ) ) ;
#57032=CARTESIAN_POINT ( 'NONE',  ( 16.52544592524342804, -4.483927247898539470, 38.54057627198103120 ) ) ;
#57033=CARTESIAN_POINT ( 'NONE',  ( -16.52544592524335698, -4.483927247898792601, 103.9594237280190185 ) ) ;
#57035=CARTESIAN_POINT ( 'NONE',  ( -13.97604488694547697, 13.89961937509957934, 38.12609039468566152 ) ) ;
#57036=CARTESIAN_POINT ( 'NONE',  ( -19.05341960407611168, -5.049401038298163336, 111.4572429386476671 ) ) ;
#57037=CARTESIAN_POINT ( 'NONE',  ( 19.05341960407611168, 5.049401038298154454, 43.95724293864769550 ) ) ;
#57038=CARTESIAN_POINT ( 'NONE',  ( 5.049401038297881783, 19.05341960407617563, 22.29275706135233648 ) ) ;
#57040=CARTESIAN_POINT ( 'NONE',  ( -12.06949235617739369, -12.14591786802326823, 44.37609039468567573 ) ) ;
#57041=CARTESIAN_POINT ( 'NONE',  ( -16.46253265017146816, -9.564922557961047289, 69.16775706135233293 ) ) ;
#57042=CARTESIAN_POINT ( 'NONE',  ( 14.34966873604972726, -8.224510206698740333, 60.83442372801901854 ) ) ;
#57044=CARTESIAN_POINT ( 'NONE',  ( 0.05219959533909260263, 19.03943276465977164, 79.99890960531436690 ) ) ;
#57045=CARTESIAN_POINT ( 'NONE',  ( -21.52544592524343514, 5.823673210054127303, 116.0405762719810383 ) ) ;
#57046=CARTESIAN_POINT ( 'NONE',  ( -0.05219959533936034679, 19.03943276465977164, 82.50109039468567573 ) ) ;
#57047=CARTESIAN_POINT ( 'NONE',  ( -9.564922557960796823, -16.46253265017161027, 107.0822429386476955 ) ) ;
#57048=CARTESIAN_POINT ( 'NONE',  ( 13.97604488694527802, 13.89961937509977652, 39.37390960531435269 ) ) ;
#57049=CARTESIAN_POINT ( 'NONE',  ( 13.97604488694527802, 13.89961937509977652, 74.37390960531436690 ) ) ;
#57050=CARTESIAN_POINT ( 'NONE',  ( 14.29746914071049879, -8.314922557960816363, 28.33224293864769550 ) ) ;
#57051=CARTESIAN_POINT ( 'NONE',  ( -16.46253265017160317, 9.564922557960807481, 40.83224293864769550 ) ) ;
#57052=CARTESIAN_POINT ( 'NONE',  ( -0.05219959533936034679, 19.03943276465977164, 47.50109039468566863 ) ) ;
#57053=CARTESIAN_POINT ( 'NONE',  ( 12.06949235617757843, -12.14591786802309237, 73.12390960531436690 ) ) ;
#57054=CARTESIAN_POINT ( 'NONE',  ( -21.55341960407619339, 5.719274019375674811, 113.5427570613523756 ) ) ;
#57055=CARTESIAN_POINT ( 'NONE',  ( 9.564922557960805705, 16.46253265017160317, 54.58224293864769550 ) ) ;
#57056=CARTESIAN_POINT ( 'NONE',  ( -21.52544592524343514, 5.823673210054127303, 46.04057627198103830 ) ) ;
#57057=CARTESIAN_POINT ( 'NONE',  ( -4.379528057220328563, 16.55341960407611168, 60.20724293864768839 ) ) ;
#57058=CARTESIAN_POINT ( 'NONE',  ( 21.55341960407619695, -5.719274019375665929, 101.0427570613523756 ) ) ;
#57059=CARTESIAN_POINT ( 'NONE',  ( -16.51473224551069308, -9.474510206698971260, 91.66557627198103830 ) ) ;
#57060=CARTESIAN_POINT ( 'NONE',  ( -19.03943276465977164, 0.05219959533909376836, 106.2489096053143669 ) ) ;
#57061=CARTESIAN_POINT ( 'NONE',  ( -13.89961937509977652, 13.97604488694528158, 35.62390960531435269 ) ) ;
#57062=CARTESIAN_POINT ( 'NONE',  ( 12.14591786802309770, 12.06949235617756955, 114.3739096053143527 ) ) ;
#57063=CARTESIAN_POINT ( 'NONE',  ( 4.483927247898545687, 16.52544592524342804, 89.79057627198103830 ) ) ;
#57064=CARTESIAN_POINT ( 'NONE',  ( 0.05219959533907565091, 21.53943276465977519, 99.99890960531436690 ) ) ;
#57065=CARTESIAN_POINT ( 'NONE',  ( -19.03943276465977164, 0.05219959533909376836, 91.24890960531436690 ) ) ;
#57066=CARTESIAN_POINT ( 'NONE',  ( -10.72451020669898014, 18.67979575497178502, 110.4155762719810383 ) ) ;
#57067=CARTESIAN_POINT ( 'NONE',  ( 16.46253265017160672, -9.564922557960803928, 88.33224293864769550 ) ) ;
#57069=CARTESIAN_POINT ( 'NONE',  ( 16.55341960407611168, 4.379528057220329451, 98.95724293864770971 ) ) ;
#57071=CARTESIAN_POINT ( 'NONE',  ( -9.564922557960796823, -16.46253265017161027, 77.08224293864769550 ) ) ;
#57072=CARTESIAN_POINT ( 'NONE',  ( -21.52544592524343514, 5.823673210054127303, 76.04057627198102409 ) ) ;
#57073=CARTESIAN_POINT ( 'NONE',  ( -5.049401038298153566, 19.05341960407611168, 115.2072429386477097 ) ) ;
#57075=CARTESIAN_POINT ( 'NONE',  ( 18.62759615963271287, -10.81492255796078972, 23.33224293864769194 ) ) ;
#57077=CARTESIAN_POINT ( 'NONE',  ( -4.379528057220086978, -16.55341960407618274, 39.79275706135235424 ) ) ;
#57078=CARTESIAN_POINT ( 'NONE',  ( 8.314922557960818139, 14.29746914071049879, 94.58224293864769550 ) ) ;
#57079=CARTESIAN_POINT ( 'NONE',  ( -17.13100169013299023, -6.664070546373153547, 94.23210164300155611 ) ) ;
#57080=CARTESIAN_POINT ( 'NONE',  ( 19.02544592524343514, -5.153800228976328945, 83.54057627198100988 ) ) ;
#57081=CARTESIAN_POINT ( 'NONE',  ( 16.51473224551069308, 9.474510206698969483, 44.16557627198103120 ) ) ;
#57082=CARTESIAN_POINT ( 'NONE',  ( -16.53943276465976808, 0.05219959533911058130, 76.24890960531435269 ) ) ;
#57083=CARTESIAN_POINT ( 'NONE',  ( -0.05219959533907301413, -21.53943276465977519, 32.49890960531435979 ) ) ;
#57084=CARTESIAN_POINT ( 'NONE',  ( -8.314922557960811034, -14.29746914071050412, 52.08224293864768839 ) ) ;
#57085=CARTESIAN_POINT ( 'NONE',  ( -16.46253265017146816, -9.564922557961047289, 99.16775706135233293 ) ) ;
#57086=CARTESIAN_POINT ( 'NONE',  ( 5.823673210054444382, -21.52544592524334988, 55.20942372801902565 ) ) ;
#57088=CARTESIAN_POINT ( 'NONE',  ( 13.97604488694527802, 13.89961937509977652, 114.3739096053143669 ) ) ;
#57089=CARTESIAN_POINT ( 'NONE',  ( -4.379528057220086978, -16.55341960407618274, 79.79275706135236135 ) ) ;
#57090=CARTESIAN_POINT ( 'NONE',  ( -16.46253265017160317, 9.564922557960807481, 30.83224293864769550 ) ) ;
#57091=CARTESIAN_POINT ( 'NONE',  ( -19.05341960407611168, -5.049401038298163336, 81.45724293864769550 ) ) ;
#57092=CARTESIAN_POINT ( 'NONE',  ( -21.55341960407610458, -5.719274019375992779, 76.45724293864769550 ) ) ;
#57093=CARTESIAN_POINT ( 'NONE',  ( 12.06949235617739724, 12.14591786802326823, 26.87609039468567218 ) ) ;
#57094=CARTESIAN_POINT ( 'NONE',  ( 4.483927247898545687, 16.52544592524342804, 54.79057627198104541 ) ) ;
#57095=CARTESIAN_POINT ( 'NONE',  ( 5.719274019375673035, 21.55341960407619339, 57.29275706135234714 ) ) ;
#57096=EDGE_CURVE ( 'NONE', #138821, #94779, #114578, .T. ) ;
#57097=CARTESIAN_POINT ( 'NONE',  ( -0.05219959533934338120, 16.53943276465976808, 82.50109039468568994 ) ) ;
#57098=CARTESIAN_POINT ( 'NONE',  ( 10.81492255796078972, 18.62759615963270932, 24.58224293864768839 ) ) ;
#57101=CARTESIAN_POINT ( 'NONE',  ( 4.379528057220092307, 16.55341960407617563, 112.2927570613523471 ) ) ;
#57102=CARTESIAN_POINT ( 'NONE',  ( -4.483927247898782831, 16.52544592524335698, 62.70942372801902565 ) ) ;
#57103=CARTESIAN_POINT ( 'NONE',  ( 19.05341960407611168, 5.049401038298154454, 78.95724293864769550 ) ) ;
#57104=CARTESIAN_POINT ( 'NONE',  ( 13.89961937509977652, -13.97604488694527269, 93.12390960531436690 ) ) ;
#57105=CARTESIAN_POINT ( 'NONE',  ( 0.05219959533937995610, -21.53943276465977519, 70.00109039468568994 ) ) ;
#57106=CARTESIAN_POINT ( 'NONE',  ( -4.483927247898782831, 16.52544592524335698, 77.70942372801900433 ) ) ;
#57107=CARTESIAN_POINT ( 'NONE',  ( 8.314922557960818139, 14.29746914071049879, 49.58224293864769550 ) ) ;
#57108=CARTESIAN_POINT ( 'NONE',  ( 0.05219959533909260263, 19.03943276465977164, 59.99890960531436690 ) ) ;
#57109=CARTESIAN_POINT ( 'NONE',  ( -9.474510206698964154, 16.51473224551069663, 50.41557627198102409 ) ) ;
#57110=CARTESIAN_POINT ( 'NONE',  ( 14.34966873604972726, -8.224510206698740333, 45.83442372801901854 ) ) ;
#57112=CARTESIAN_POINT ( 'NONE',  ( 9.564922557961047289, -16.46253265017146816, 95.41775706135233293 ) ) ;
#57113=CARTESIAN_POINT ( 'NONE',  ( 8.314922557960818139, 14.29746914071049879, 94.58224293864769550 ) ) ;
#57114=CARTESIAN_POINT ( 'NONE',  ( -9.564922557960796823, -16.46253265017161027, 67.08224293864769550 ) ) ;
#57115=CARTESIAN_POINT ( 'NONE',  ( 19.02544592524334988, 5.153800228976608722, 106.4594237280190185 ) ) ;
#57117=CARTESIAN_POINT ( 'NONE',  ( 10.81492255796106328, -18.62759615963255655, 110.4177570613523756 ) ) ;
#57118=CARTESIAN_POINT ( 'NONE',  ( 4.379528057220092307, 16.55341960407617563, 72.29275706135236135 ) ) ;
#57119=CARTESIAN_POINT ( 'NONE',  ( -0.05219959533936034679, 19.03943276465977164, 97.50109039468567573 ) ) ;
#57120=CARTESIAN_POINT ( 'NONE',  ( -10.72451020669898014, 18.67979575497178502, 60.41557627198102409 ) ) ;
#57121=CARTESIAN_POINT ( 'NONE',  ( 16.55341960407618274, -4.379528057220086978, 51.04275706135234714 ) ) ;
#57123=CARTESIAN_POINT ( 'NONE',  ( -19.05341960407617563, 5.049401038297882671, 58.54275706135234003 ) ) ;
#57124=CARTESIAN_POINT ( 'NONE',  ( -16.51473224551069308, -9.474510206698971260, 91.66557627198103830 ) ) ;
#57125=CARTESIAN_POINT ( 'NONE',  ( -12.06949235617756955, 12.14591786802309770, 110.6239096053143669 ) ) ;
#57126=CARTESIAN_POINT ( 'NONE',  ( -16.51473224551069308, -9.474510206698971260, 66.66557627198102409 ) ) ;
#57127=CARTESIAN_POINT ( 'NONE',  ( -0.05219959533910754901, -16.53943276465976808, 57.49890960531435979 ) ) ;
#57128=CARTESIAN_POINT ( 'NONE',  ( 5.823673210054444382, -21.52544592524334988, 80.20942372801901854 ) ) ;
#57129=CARTESIAN_POINT ( 'NONE',  ( -5.153800228976607833, 19.02544592524334988, 52.70942372801900433 ) ) ;
#57130=CARTESIAN_POINT ( 'NONE',  ( -19.02544592524334988, -5.153800228976617603, 28.95942372801900433 ) ) ;
#57131=CARTESIAN_POINT ( 'NONE',  ( -18.67979575497178146, -10.72451020669898902, 21.66557627198102409 ) ) ;
#57132=CARTESIAN_POINT ( 'NONE',  ( -5.823673210054431948, 21.52544592524334988, 97.70942372801904696 ) ) ;
#57133=CARTESIAN_POINT ( 'NONE',  ( 16.46253265017160672, -9.564922557960803928, 63.33224293864769550 ) ) ;
#57134=CARTESIAN_POINT ( 'NONE',  ( 21.53943276465977519, 0.05219959533937863772, 96.25109039468568994 ) ) ;
#57135=CARTESIAN_POINT ( 'NONE',  ( 15.80617190586746368, 15.72974639402197994, 49.37390960531436690 ) ) ;
#57136=CARTESIAN_POINT ( 'NONE',  ( -5.049401038298153566, 19.05341960407611168, 85.20724293864766707 ) ) ;
#57137=CARTESIAN_POINT ( 'NONE',  ( -16.51473224551082808, 9.474510206698731452, 68.33442372801900433 ) ) ;
#57138=CARTESIAN_POINT ( 'NONE',  ( 5.153800228976335163, 19.02544592524342804, 44.79057627198103830 ) ) ;
#57139=CARTESIAN_POINT ( 'NONE',  ( -19.02544592524342804, 5.153800228976336051, 91.04057627198100988 ) ) ;
#57140=CARTESIAN_POINT ( 'NONE',  ( 9.474510206698729675, 16.51473224551082808, 87.08442372801900433 ) ) ;
#57141=CARTESIAN_POINT ( 'NONE',  ( 16.55341960407618274, -4.379528057220086978, 41.04275706135236135 ) ) ;
#57142=CARTESIAN_POINT ( 'NONE',  ( 12.06949235617757843, -12.14591786802309237, 98.12390960531436690 ) ) ;
#57143=CARTESIAN_POINT ( 'NONE',  ( -5.153800228976328057, -19.02544592524343514, 67.29057627198102409 ) ) ;
#57144=CARTESIAN_POINT ( 'NONE',  ( 15.72974639402199770, -15.80617190586745480, 53.12390960531436690 ) ) ;
#57145=CARTESIAN_POINT ( 'NONE',  ( 16.46253265017146816, 9.564922557961045513, 111.6677570613523329 ) ) ;
#57146=CARTESIAN_POINT ( 'NONE',  ( 10.72451020669871369, 18.67979575497193778, 27.08442372801901854 ) ) ;
#57147=CARTESIAN_POINT ( 'NONE',  ( -15.80617190586768217, 15.72974639402176855, 68.12609039468567573 ) ) ;
#57148=CARTESIAN_POINT ( 'NONE',  ( 12.14591786802327356, -12.06949235617739191, 65.62609039468568994 ) ) ;
#57149=CARTESIAN_POINT ( 'NONE',  ( -13.97604488694527625, -13.89961937509977652, 71.87390960531433848 ) ) ;
#57150=CARTESIAN_POINT ( 'NONE',  ( -4.483927247898782831, 16.52544592524335698, 107.7094237280190328 ) ) ;
#57151=CARTESIAN_POINT ( 'NONE',  ( 19.05341960407617918, -5.049401038297876454, 41.04275706135233293 ) ) ;
#57152=CARTESIAN_POINT ( 'NONE',  ( 5.719274019375673035, 21.55341960407619339, 37.29275706135235424 ) ) ;
#57153=CARTESIAN_POINT ( 'NONE',  ( -16.55341960407611168, -4.379528057220339221, 81.45724293864769550 ) ) ;
#57154=CARTESIAN_POINT ( 'NONE',  ( 16.46253265017160672, -9.564922557960803928, 98.33224293864769550 ) ) ;
#57155=CARTESIAN_POINT ( 'NONE',  ( -16.52544592524335698, -4.483927247898792601, 93.95942372801903275 ) ) ;
#57156=CARTESIAN_POINT ( 'NONE',  ( -21.55341960407619339, 5.719274019375674811, 68.54275706135234714 ) ) ;
#57157=CARTESIAN_POINT ( 'NONE',  ( -8.314922557961024197, 14.29746914071037800, 27.91775706135234358 ) ) ;
#57158=CARTESIAN_POINT ( 'NONE',  ( 10.81492255796106328, -18.62759615963255655, 25.41775706135235779 ) ) ;
#57159=CARTESIAN_POINT ( 'NONE',  ( -14.34966873604960291, -8.224510206698953496, 76.66557627198103830 ) ) ;
#57161=CARTESIAN_POINT ( 'NONE',  ( -15.80617190586745835, -15.72974639402198527, 101.8739096053143811 ) ) ;
#57162=CARTESIAN_POINT ( 'NONE',  ( -12.06949235617756955, 12.14591786802309770, 50.62390960531435979 ) ) ;
#57164=CARTESIAN_POINT ( 'NONE',  ( 13.97604488694527802, 13.89961937509977652, 29.37390960531435979 ) ) ;
#57165=CARTESIAN_POINT ( 'NONE',  ( 18.67979575497178502, 10.72451020669898547, 24.16557627198103120 ) ) ;
#57166=CARTESIAN_POINT ( 'NONE',  ( -21.52544592524334988, -5.823673210054445271, 38.95942372801901854 ) ) ;
#57167=CARTESIAN_POINT ( 'NONE',  ( -12.14591786802309592, -12.06949235617757132, 66.87390960531436690 ) ) ;
#57169=CARTESIAN_POINT ( 'NONE',  ( 18.67979575497178502, 10.72451020669898547, 69.16557627198102409 ) ) ;
#57170=CARTESIAN_POINT ( 'NONE',  ( -9.564922557960796823, -16.46253265017161027, 77.08224293864769550 ) ) ;
#57171=CARTESIAN_POINT ( 'NONE',  ( -5.153800228976328057, -19.02544592524343514, 22.29057627198102765 ) ) ;
#57172=CARTESIAN_POINT ( 'NONE',  ( 16.46253265017146816, 9.564922557961045513, 81.66775706135233293 ) ) ;
#57174=CARTESIAN_POINT ( 'NONE',  ( 5.823673210054125526, 21.52544592524343514, 64.79057627198103830 ) ) ;
#57175=CARTESIAN_POINT ( 'NONE',  ( -13.97604488694527625, -13.89961937509977652, 36.87390960531436690 ) ) ;
#57176=CARTESIAN_POINT ( 'NONE',  ( -19.03943276465977164, 0.05219959533909376836, 76.24890960531435269 ) ) ;
#57178=CARTESIAN_POINT ( 'NONE',  ( 12.14591786802327356, -12.06949235617739191, 40.62609039468567573 ) ) ;
#57179=CARTESIAN_POINT ( 'NONE',  ( -18.67979575497193778, 10.72451020669871902, 28.33442372801902209 ) ) ;
#57180=CARTESIAN_POINT ( 'NONE',  ( -18.62759615963255300, -10.81492255796106328, 59.16775706135234714 ) ) ;
#57181=CARTESIAN_POINT ( 'NONE',  ( 5.153800228976335163, 19.02544592524342804, 109.7905762719810099 ) ) ;
#57182=CARTESIAN_POINT ( 'NONE',  ( 15.72974639402199770, -15.80617190586745480, 68.12390960531436690 ) ) ;
#57183=CARTESIAN_POINT ( 'NONE',  ( 18.62759615963271287, -10.81492255796078972, 108.3322429386477097 ) ) ;
#57184=CARTESIAN_POINT ( 'NONE',  ( -4.483927247898782831, 16.52544592524335698, 47.70942372801902565 ) ) ;
#57186=CARTESIAN_POINT ( 'NONE',  ( -18.62759615963270932, 10.81492255796079327, 50.83224293864770971 ) ) ;
#57187=CARTESIAN_POINT ( 'NONE',  ( -15.72974639402176322, -15.80617190586768395, 104.3760903946856899 ) ) ;
#57188=CARTESIAN_POINT ( 'NONE',  ( -19.02544592524342804, 5.153800228976336051, 61.04057627198103120 ) ) ;
#57189=CARTESIAN_POINT ( 'NONE',  ( -5.049401038298153566, 19.05341960407611168, 110.2072429386476671 ) ) ;
#57190=CARTESIAN_POINT ( 'NONE',  ( 16.51473224551069308, 9.474510206698969483, 74.16557627198103830 ) ) ;
#57192=CARTESIAN_POINT ( 'NONE',  ( 17.44279575226788381, -5.990770900253884257, 88.33557567514318976 ) ) ;
#57193=CARTESIAN_POINT ( 'NONE',  ( 5.153800228976615827, -19.02544592524334988, 65.20942372801900433 ) ) ;
#57194=CARTESIAN_POINT ( 'NONE',  ( -10.81492255796105439, 18.62759615963255655, 112.9177570613523329 ) ) ;
#57195=CARTESIAN_POINT ( 'NONE',  ( -10.81492255796078084, -18.62759615963271287, 47.08224293864770260 ) ) ;
#57196=CARTESIAN_POINT ( 'NONE',  ( -8.224510206698735004, -14.34966873604973081, 99.58442372801900433 ) ) ;
#57197=CARTESIAN_POINT ( 'NONE',  ( 19.02544592524334988, 5.153800228976608722, 86.45942372801900433 ) ) ;
#57198=CARTESIAN_POINT ( 'NONE',  ( -17.49999999999999645, -7.500000000000000888, 120.0000000000000142 ) ) ;
#57199=CARTESIAN_POINT ( 'NONE',  ( -13.89961937509957401, -13.97604488694547875, 24.37609039468565442 ) ) ;
#57200=CARTESIAN_POINT ( 'NONE',  ( -19.05341960407617563, 5.049401038297882671, 78.54275706135233293 ) ) ;
#57201=CARTESIAN_POINT ( 'NONE',  ( -5.049401038297874678, -19.05341960407617918, 44.79275706135232582 ) ) ;
#57202=CARTESIAN_POINT ( 'NONE',  ( -16.81555441253551209, -7.025013491695503376, 44.36314554665745646 ) ) ;
#57203=CARTESIAN_POINT ( 'NONE',  ( 16.46253265017160672, -9.564922557960803928, 38.33224293864768839 ) ) ;
#57204=CARTESIAN_POINT ( 'NONE',  ( -4.483927247898539470, -16.52544592524342804, 52.29057627198102409 ) ) ;
#57205=CARTESIAN_POINT ( 'NONE',  ( -13.97604488694527625, -13.89961937509977652, 36.87390960531436690 ) ) ;
#57206=CARTESIAN_POINT ( 'NONE',  ( 14.29746914071049879, -8.314922557960816363, 38.33224293864768839 ) ) ;
#57207=LINE ( 'NONE', #92480, #161445 ) ;
#57208=CARTESIAN_POINT ( 'NONE',  ( -8.224510206698735004, -14.34966873604973081, 109.5844237280190328 ) ) ;
#57209=CARTESIAN_POINT ( 'NONE',  ( 5.153800228976335163, 19.02544592524342804, 44.79057627198103830 ) ) ;
#57210=CARTESIAN_POINT ( 'NONE',  ( 9.564922557961047289, -16.46253265017146816, 25.41775706135234003 ) ) ;
#57211=CARTESIAN_POINT ( 'NONE',  ( 4.483927247898790824, -16.52544592524335698, 30.20942372801902565 ) ) ;
#57212=CARTESIAN_POINT ( 'NONE',  ( 21.52544592524344225, -5.823673210054117533, 38.54057627198103120 ) ) ;
#57213=CARTESIAN_POINT ( 'NONE',  ( -18.62759615963255300, -10.81492255796106328, 94.16775706135237556 ) ) ;
#57215=CARTESIAN_POINT ( 'NONE',  ( 16.46253265017160672, -9.564922557960803928, 108.3322429386476955 ) ) ;
#57216=CARTESIAN_POINT ( 'NONE',  ( 5.049401038298161559, -19.05341960407611168, 77.70724293864765286 ) ) ;
#57218=CARTESIAN_POINT ( 'NONE',  ( 15.72974639402199770, -15.80617190586745480, 113.1239096053143953 ) ) ;
#57220=CARTESIAN_POINT ( 'NONE',  ( -16.53943276465976808, 0.05219959533911058130, 86.24890960531436690 ) ) ;
#57221=CARTESIAN_POINT ( 'NONE',  ( -10.72451020669898014, 18.67979575497178502, 75.41557627198102409 ) ) ;
#57222=CARTESIAN_POINT ( 'NONE',  ( 9.564922557960805705, 16.46253265017160317, 69.58224293864770971 ) ) ;
#57223=CARTESIAN_POINT ( 'NONE',  ( -16.51473224551069308, -9.474510206698971260, 71.66557627198102409 ) ) ;
#57224=CARTESIAN_POINT ( 'NONE',  ( -21.55341960407610458, -5.719274019375992779, 101.4572429386476955 ) ) ;
#57226=CARTESIAN_POINT ( 'NONE',  ( 0.05219959533909260263, 19.03943276465977164, 64.99890960531436690 ) ) ;
#57227=CARTESIAN_POINT ( 'NONE',  ( -0.05219959533910754901, -16.53943276465976808, 102.4989096053143811 ) ) ;
#57228=CARTESIAN_POINT ( 'NONE',  ( 19.03943276465977164, -0.05219959533909143690, 23.74890960531435269 ) ) ;
#57229=CARTESIAN_POINT ( 'NONE',  ( -0.05219959533909027116, -19.03943276465977164, 57.49890960531435979 ) ) ;
#57230=CARTESIAN_POINT ( 'NONE',  ( -13.97604488694547697, 13.89961937509957934, 78.12609039468567573 ) ) ;
#57231=CARTESIAN_POINT ( 'NONE',  ( 8.224510206698953496, -14.34966873604960469, 97.91557627198103830 ) ) ;
#57232=CARTESIAN_POINT ( 'NONE',  ( -15.72974639402176322, -15.80617190586768395, 64.37609039468568994 ) ) ;
#57233=CARTESIAN_POINT ( 'NONE',  ( 5.153800228976335163, 19.02544592524342804, 49.79057627198100988 ) ) ;
#57234=CARTESIAN_POINT ( 'NONE',  ( 5.719274019375991003, -21.55341960407610458, 112.7072429386476955 ) ) ;
#57235=CARTESIAN_POINT ( 'NONE',  ( 0.05219959533910956823, 16.53943276465976808, 94.99890960531436690 ) ) ;
#57237=CARTESIAN_POINT ( 'NONE',  ( -13.97604488694527625, -13.89961937509977652, 71.87390960531433848 ) ) ;
#57238=CARTESIAN_POINT ( 'NONE',  ( 17.48847506799969409, 5.747544572773743532, 111.6730256215672199 ) ) ;
#57239=CARTESIAN_POINT ( 'NONE',  ( 5.153800228976615827, -19.02544592524334988, 110.2094237280189901 ) ) ;
#57240=CARTESIAN_POINT ( 'NONE',  ( -19.05341960407611168, -5.049401038298163336, 106.4572429386476955 ) ) ;
#57241=CARTESIAN_POINT ( 'NONE',  ( -18.62759615963255300, -10.81492255796106328, 49.16775706135234003 ) ) ;
#57242=CARTESIAN_POINT ( 'NONE',  ( -9.474510206698964154, 16.51473224551069663, 100.4155762719810241 ) ) ;
#57243=CARTESIAN_POINT ( 'NONE',  ( 13.97604488694548053, -13.89961937509957401, 80.62609039468567573 ) ) ;
#57244=CARTESIAN_POINT ( 'NONE',  ( -9.474510206698964154, 16.51473224551069663, 65.41557627198102409 ) ) ;
#57245=CARTESIAN_POINT ( 'NONE',  ( -12.14591786802309592, -12.06949235617757132, 76.87390960531439532 ) ) ;
#57246=CARTESIAN_POINT ( 'NONE',  ( -19.03943276465977164, 0.05219959533909376836, 96.24890960531436690 ) ) ;
#57247=CARTESIAN_POINT ( 'NONE',  ( -4.379528057220328563, 16.55341960407611168, 85.20724293864770971 ) ) ;
#57248=CARTESIAN_POINT ( 'NONE',  ( -13.97604488694527625, -13.89961937509977652, 91.87390960531432427 ) ) ;
#57249=CARTESIAN_POINT ( 'NONE',  ( -5.153800228976607833, 19.02544592524334988, 47.70942372801900433 ) ) ;
#57250=CARTESIAN_POINT ( 'NONE',  ( -5.049401038298153566, 19.05341960407611168, 45.20724293864769550 ) ) ;
#57251=CARTESIAN_POINT ( 'NONE',  ( -12.14591786802309592, -12.06949235617757132, 46.87390960531435979 ) ) ;
#57252=CARTESIAN_POINT ( 'NONE',  ( 9.474510206698971260, -16.51473224551069308, 32.91557627198102409 ) ) ;
#57254=CARTESIAN_POINT ( 'NONE',  ( 5.719274019375673035, 21.55341960407619339, 47.29275706135234003 ) ) ;
#57255=CARTESIAN_POINT ( 'NONE',  ( -16.46253265017146816, -9.564922557961047289, 84.16775706135233293 ) ) ;
#57256=CARTESIAN_POINT ( 'NONE',  ( -8.224510206698948167, 14.34966873604960824, 30.41557627198101699 ) ) ;
#57257=CARTESIAN_POINT ( 'NONE',  ( -21.55341960407610458, -5.719274019375992779, 101.4572429386476955 ) ) ;
#57258=CARTESIAN_POINT ( 'NONE',  ( 21.55341960407610458, 5.719274019375980345, 33.95724293864769550 ) ) ;
#57259=CARTESIAN_POINT ( 'NONE',  ( 12.14591786802309770, 12.06949235617756955, 79.37390960531436690 ) ) ;
#57260=CARTESIAN_POINT ( 'NONE',  ( -0.05219959533909027116, -19.03943276465977164, 37.49890960531436690 ) ) ;
#57261=CARTESIAN_POINT ( 'NONE',  ( -12.06949235617739369, -12.14591786802326823, 109.3760903946857042 ) ) ;
#57262=CARTESIAN_POINT ( 'NONE',  ( -8.314922557961024197, 14.29746914071037800, 87.91775706135234714 ) ) ;
#57263=CARTESIAN_POINT ( 'NONE',  ( 16.53943276465976808, 0.05219959533934440121, 71.25109039468568994 ) ) ;
#57264=CARTESIAN_POINT ( 'NONE',  ( -19.05341960407617563, 5.049401038297882671, 28.54275706135232937 ) ) ;
#57265=CARTESIAN_POINT ( 'NONE',  ( -9.564922557960796823, -16.46253265017161027, 87.08224293864769550 ) ) ;
#57266=CARTESIAN_POINT ( 'NONE',  ( 5.153800228976335163, 19.02544592524342804, 79.79057627198102409 ) ) ;
#57267=CARTESIAN_POINT ( 'NONE',  ( -16.53943276465976808, -0.05219959533934237506, 73.75109039468567573 ) ) ;
#57268=CARTESIAN_POINT ( 'NONE',  ( 19.05341960407611168, 5.049401038298154454, 33.95724293864769550 ) ) ;
#57269=CARTESIAN_POINT ( 'NONE',  ( 14.29746914071049879, -8.314922557960816363, 48.33224293864770260 ) ) ;
#57270=CARTESIAN_POINT ( 'NONE',  ( 13.89961937509977652, -13.97604488694527269, 98.12390960531433848 ) ) ;
#57271=CARTESIAN_POINT ( 'NONE',  ( 18.62759615963271287, -10.81492255796078972, 33.33224293864769550 ) ) ;
#57272=CARTESIAN_POINT ( 'NONE',  ( -12.14591786802309592, -12.06949235617757132, 66.87390960531436690 ) ) ;
#57274=CARTESIAN_POINT ( 'NONE',  ( -0.05219959533910754901, -16.53943276465976808, 62.49890960531436690 ) ) ;
#57276=CARTESIAN_POINT ( 'NONE',  ( -9.474510206698720793, -16.51473224551083518, 64.58442372801900433 ) ) ;
#57277=CARTESIAN_POINT ( 'NONE',  ( 19.02544592524343514, -5.153800228976328945, 93.54057627198102409 ) ) ;
#57278=CARTESIAN_POINT ( 'NONE',  ( -16.46253265017146816, -9.564922557961047289, 84.16775706135233293 ) ) ;
#57279=CARTESIAN_POINT ( 'NONE',  ( -5.049401038297874678, -19.05341960407618274, 39.79275706135232582 ) ) ;
#57280=CARTESIAN_POINT ( 'NONE',  ( -19.03943276465977164, -0.05219959533935918106, 113.7510903946856757 ) ) ;
#57281=CARTESIAN_POINT ( 'NONE',  ( 4.379528057220092307, 16.55341960407617563, 97.29275706135234714 ) ) ;
#57282=CARTESIAN_POINT ( 'NONE',  ( -19.02544592524342804, 5.153800228976336051, 46.04057627198101699 ) ) ;
#57283=CARTESIAN_POINT ( 'NONE',  ( 5.719274019375991003, -21.55341960407610458, 27.70724293864769905 ) ) ;
#57284=CARTESIAN_POINT ( 'NONE',  ( 15.80617190586769283, -15.72974639402175789, 55.62609039468568284 ) ) ;
#57285=CARTESIAN_POINT ( 'NONE',  ( -16.53943276465976808, -0.05219959533934237506, 18.75109039468568639 ) ) ;
#57287=CARTESIAN_POINT ( 'NONE',  ( -19.03943276465977164, 0.05219959533909376836, 81.24890960531436690 ) ) ;
#57288=CARTESIAN_POINT ( 'NONE',  ( 9.474510206698971260, -16.51473224551069308, 112.9155762719810383 ) ) ;
#57289=CARTESIAN_POINT ( 'NONE',  ( 14.29746914071049879, -8.314922557960816363, 68.33224293864769550 ) ) ;
#57290=CARTESIAN_POINT ( 'NONE',  ( 19.02544592524343514, -5.153800228976328945, 73.54057627198103830 ) ) ;
#57291=CARTESIAN_POINT ( 'NONE',  ( -13.89961937509977652, 13.97604488694528158, 80.62390960531436690 ) ) ;
#57292=CARTESIAN_POINT ( 'NONE',  ( 13.97604488694548053, -13.89961937509957401, 95.62609039468563310 ) ) ;
#57293=CARTESIAN_POINT ( 'NONE',  ( -21.52544592524343514, 5.823673210054127303, 71.04057627198103830 ) ) ;
#57294=CARTESIAN_POINT ( 'NONE',  ( -16.46253265017160317, 9.564922557960807481, 25.83224293864769194 ) ) ;
#57295=CARTESIAN_POINT ( 'NONE',  ( 5.049401038297881783, 19.05341960407617563, 57.29275706135231871 ) ) ;
#57296=CARTESIAN_POINT ( 'NONE',  ( 5.049401038298161559, -19.05341960407611168, 52.70724293864767418 ) ) ;
#57297=CARTESIAN_POINT ( 'NONE',  ( 5.153800228976335163, 19.02544592524342804, 89.79057627198102409 ) ) ;
#57299=CARTESIAN_POINT ( 'NONE',  ( -10.72451020669898014, 18.67979575497178502, 95.41557627198102409 ) ) ;
#57300=CARTESIAN_POINT ( 'NONE',  ( 4.483927247898545687, 16.52544592524342804, 94.79057627198105251 ) ) ;
#57301=CARTESIAN_POINT ( 'NONE',  ( -9.564922557961040184, 16.46253265017147172, 47.91775706135233293 ) ) ;
#57302=CARTESIAN_POINT ( 'NONE',  ( -10.72451020669898014, 18.67979575497178502, 85.41557627198102409 ) ) ;
#57303=B_SPLINE_CURVE_WITH_KNOTS ( 'NONE', 3,
 ( #162434, #196794, #195803, #42110, #56260, #192783 ),
 .UNSPECIFIED., .F., .F.,
 ( 4, 2, 4 ),
 ( 0.003239945802372255594, 0.003620412082092107353, 0.004000878361811959112 ),
 .UNSPECIFIED. ) ;
#57304=CARTESIAN_POINT ( 'NONE',  ( -18.67979575497178146, -10.72451020669898902, 71.66557627198100988 ) ) ;
#57305=CARTESIAN_POINT ( 'NONE',  ( 14.29746914071049879, -8.314922557960816363, 38.33224293864768839 ) ) ;
#57306=CARTESIAN_POINT ( 'NONE',  ( -18.62759615963255300, -10.81492255796106328, 104.1677570613523471 ) ) ;
#57307=CARTESIAN_POINT ( 'NONE',  ( 5.153800228976335163, 19.02544592524342804, 74.79057627198103830 ) ) ;
#57308=CARTESIAN_POINT ( 'NONE',  ( 9.564922557960805705, 16.46253265017160317, 34.58224293864770260 ) ) ;
#57310=CARTESIAN_POINT ( 'NONE',  ( 15.72974639402176855, 15.80617190586768217, 36.87609039468568994 ) ) ;
#57311=CARTESIAN_POINT ( 'NONE',  ( -18.67979575497193778, 10.72451020669871902, 58.33442372801901143 ) ) ;
#57312=CARTESIAN_POINT ( 'NONE',  ( 19.02544592524343514, -5.153800228976328945, 48.54057627198103120 ) ) ;
#57313=CARTESIAN_POINT ( 'NONE',  ( -5.823673210054431948, 21.52544592524334988, 27.70942372801901854 ) ) ;
#57314=CARTESIAN_POINT ( 'NONE',  ( -9.564922557961040184, 16.46253265017147172, 57.91775706135233293 ) ) ;
#57315=CARTESIAN_POINT ( 'NONE',  ( 16.46253265017160672, -9.564922557960803928, 43.33224293864769550 ) ) ;
#57316=CARTESIAN_POINT ( 'NONE',  ( -4.379528057220086978, -16.55341960407618274, 34.79275706135235424 ) ) ;
#57317=CARTESIAN_POINT ( 'NONE',  ( 13.97604488694527802, 13.89961937509977652, 24.37390960531435624 ) ) ;
#57318=CARTESIAN_POINT ( 'NONE',  ( -14.29746914071037622, -8.314922557961029526, 79.16775706135234714 ) ) ;
#57319=CARTESIAN_POINT ( 'NONE',  ( -5.049401038298153566, 19.05341960407611168, 35.20724293864768839 ) ) ;
#57321=CARTESIAN_POINT ( 'NONE',  ( 16.51473224551069308, 9.474510206698969483, 79.16557627198103830 ) ) ;
#57322=CARTESIAN_POINT ( 'NONE',  ( 16.46253265017160672, -9.564922557960803928, 23.33224293864769194 ) ) ;
#57323=CARTESIAN_POINT ( 'NONE',  ( -5.823673210054116645, -21.52544592524344225, 72.29057627198102409 ) ) ;
#57324=CARTESIAN_POINT ( 'NONE',  ( -8.314922557961024197, 14.29746914071037800, 52.91775706135235424 ) ) ;
#57325=CARTESIAN_POINT ( 'NONE',  ( -13.89961937509957401, -13.97604488694547875, 19.37609039468566507 ) ) ;
#57326=CARTESIAN_POINT ( 'NONE',  ( -19.03943276465977164, 0.05219959533909376836, 36.24890960531436690 ) ) ;
#57327=CARTESIAN_POINT ( 'NONE',  ( 4.483927247898545687, 16.52544592524342804, 34.79057627198103120 ) ) ;
#57328=CARTESIAN_POINT ( 'NONE',  ( -16.53943276465976808, 0.05219959533911058130, 71.24890960531435269 ) ) ;
#57329=CARTESIAN_POINT ( 'NONE',  ( 5.153800228976335163, 19.02544592524342804, 59.79057627198100988 ) ) ;
#57330=CARTESIAN_POINT ( 'NONE',  ( -10.81492255796105439, 18.62759615963255655, 107.9177570613523471 ) ) ;
#57331=CARTESIAN_POINT ( 'NONE',  ( 15.80617190586769283, -15.72974639402175789, 20.62609039468568639 ) ) ;
#57332=CARTESIAN_POINT ( 'NONE',  ( 9.564922557960805705, 16.46253265017160317, 74.58224293864769550 ) ) ;
#57333=CARTESIAN_POINT ( 'NONE',  ( -21.53943276465977519, -0.05219959533937600094, 83.75109039468568994 ) ) ;
#57334=CARTESIAN_POINT ( 'NONE',  ( 14.34966873604972726, -8.224510206698740333, 70.83442372801901854 ) ) ;
#57335=CARTESIAN_POINT ( 'NONE',  ( 16.55341960407618274, -4.379528057220086978, 36.04275706135234714 ) ) ;
#57336=CARTESIAN_POINT ( 'NONE',  ( -14.29746914071049879, 8.314922557960819915, 95.83224293864770971 ) ) ;
#57337=CARTESIAN_POINT ( 'NONE',  ( 5.049401038298161559, -19.05341960407611168, 102.7072429386476955 ) ) ;
#57339=CARTESIAN_POINT ( 'NONE',  ( 16.52544592524342804, -4.483927247898539470, 28.54057627198103120 ) ) ;
#57340=CARTESIAN_POINT ( 'NONE',  ( 9.564922557960805705, 16.46253265017160317, 34.58224293864770260 ) ) ;
#57341=CARTESIAN_POINT ( 'NONE',  ( -16.55341960407617563, 4.379528057220093196, 48.54275706135234714 ) ) ;
#57342=CARTESIAN_POINT ( 'NONE',  ( 8.314922557960818139, 14.29746914071049879, 59.58224293864770260 ) ) ;
#57343=CARTESIAN_POINT ( 'NONE',  ( 16.52544592524335698, 4.483927247898782831, 96.45942372801901854 ) ) ;
#57344=CARTESIAN_POINT ( 'NONE',  ( -5.153800228976328057, -19.02544592524343514, 112.2905762719810099 ) ) ;
#57345=CARTESIAN_POINT ( 'NONE',  ( 21.53943276465977519, -0.05219959533907433946, 28.74890960531435624 ) ) ;
#57346=CARTESIAN_POINT ( 'NONE',  ( 21.53943276465977519, 0.05219959533937863772, 111.2510903946856899 ) ) ;
#57347=CARTESIAN_POINT ( 'NONE',  ( 4.483927247898545687, 16.52544592524342804, 84.79057627198102409 ) ) ;
#57348=CARTESIAN_POINT ( 'NONE',  ( 9.564922557960805705, 16.46253265017160317, 89.58224293864769550 ) ) ;
#57349=ORIENTED_EDGE ( 'NONE', *, *, #158665, .F. ) ;
#57350=CARTESIAN_POINT ( 'NONE',  ( -16.53943276465976808, -0.05219959533934237506, 38.75109039468567573 ) ) ;
#57351=CARTESIAN_POINT ( 'NONE',  ( 5.153800228976335163, 19.02544592524342804, 39.79057627198100988 ) ) ;
#57352=CARTESIAN_POINT ( 'NONE',  ( 4.483927247898790824, -16.52544592524335698, 40.20942372801901854 ) ) ;
#57354=CARTESIAN_POINT ( 'NONE',  ( -16.51473224551082808, 9.474510206698731452, 48.33442372801900433 ) ) ;
#57356=CARTESIAN_POINT ( 'NONE',  ( -19.02544592524342804, 5.153800228976336051, 51.04057627198103120 ) ) ;
#57357=CARTESIAN_POINT ( 'NONE',  ( 14.29746914071037800, 8.314922557961029526, 86.66775706135234714 ) ) ;
#57358=CARTESIAN_POINT ( 'NONE',  ( 13.97604488694548053, -13.89961937509957401, 90.62609039468567573 ) ) ;
#57359=CARTESIAN_POINT ( 'NONE',  ( -19.02544592524342804, 5.153800228976336051, 56.04057627198100988 ) ) ;
#57360=CARTESIAN_POINT ( 'NONE',  ( -0.05219959533907301413, -21.53943276465977519, 92.49890960531436690 ) ) ;
#57361=CARTESIAN_POINT ( 'NONE',  ( 16.53943276465976808, -0.05219959533910856209, 98.74890960531438111 ) ) ;
#57362=VECTOR ( 'NONE', #63388, 1000.000000000000000 ) ;
#57364=CARTESIAN_POINT ( 'NONE',  ( -9.564922557961040184, 16.46253265017147172, 72.91775706135233293 ) ) ;
#57365=CARTESIAN_POINT ( 'NONE',  ( -0.05219959533907301413, -21.53943276465977519, 57.49890960531435979 ) ) ;
#57366=CARTESIAN_POINT ( 'NONE',  ( 19.05341960407617918, -5.049401038297876454, 46.04275706135233293 ) ) ;
#57367=CARTESIAN_POINT ( 'NONE',  ( -5.153800228976328057, -19.02544592524343514, 112.2905762719810099 ) ) ;
#57368=CARTESIAN_POINT ( 'NONE',  ( 10.81492255796078972, 18.62759615963270932, 89.58224293864768129 ) ) ;
#57369=CARTESIAN_POINT ( 'NONE',  ( -17.31747979337949772, 6.344076630960996610, 83.62055131934816643 ) ) ;
#57370=CARTESIAN_POINT ( 'NONE',  ( 19.03943276465977164, 0.05219959533936151252, 101.2510903946856757 ) ) ;
#57371=CARTESIAN_POINT ( 'NONE',  ( -18.87580814761070513, 5.500000000000040856, 60.87172394265760289 ) ) ;
#57372=CARTESIAN_POINT ( 'NONE',  ( 8.224510206698742110, 14.34966873604972548, 27.08442372801901854 ) ) ;
#57373=CARTESIAN_POINT ( 'NONE',  ( 5.049401038298161559, -19.05341960407611168, 47.70724293864770260 ) ) ;
#57374=CARTESIAN_POINT ( 'NONE',  ( -5.049401038298153566, 19.05341960407611168, 110.2072429386476671 ) ) ;
#57375=CARTESIAN_POINT ( 'NONE',  ( 10.72451020669898902, -18.67979575497178502, 92.91557627198103830 ) ) ;
#57376=CARTESIAN_POINT ( 'NONE',  ( -15.80617190586768217, 15.72974639402176855, 63.12609039468568994 ) ) ;
#57377=CARTESIAN_POINT ( 'NONE',  ( 9.564922557961047289, -16.46253265017146816, 105.4177570613523471 ) ) ;
#57378=CARTESIAN_POINT ( 'NONE',  ( 5.153800228976615827, -19.02544592524334988, 25.20942372801900433 ) ) ;
#57379=CARTESIAN_POINT ( 'NONE',  ( -12.06949235617756955, 12.14591786802309770, 30.62390960531436335 ) ) ;
#57380=CARTESIAN_POINT ( 'NONE',  ( -15.72974639402197994, 15.80617190586746368, 100.6239096053143811 ) ) ;
#57381=CARTESIAN_POINT ( 'NONE',  ( -12.06949235617756955, 12.14591786802309770, 50.62390960531435979 ) ) ;
#57382=CARTESIAN_POINT ( 'NONE',  ( 19.03943276465977164, 0.05219959533936151252, 91.25109039468566152 ) ) ;
#57383=CARTESIAN_POINT ( 'NONE',  ( -19.05341960407617563, 5.049401038297882671, 53.54275706135231871 ) ) ;
#57384=CARTESIAN_POINT ( 'NONE',  ( 18.62759615963255655, 10.81492255796105972, 76.66775706135234714 ) ) ;
#57385=CARTESIAN_POINT ( 'NONE',  ( 19.02544592524334988, 5.153800228976608722, 46.45942372801899012 ) ) ;
#57386=CARTESIAN_POINT ( 'NONE',  ( -12.06949235617756955, 12.14591786802309770, 115.6239096053143669 ) ) ;
#57387=CARTESIAN_POINT ( 'NONE',  ( -15.72974639402197994, 15.80617190586746368, 45.62390960531436690 ) ) ;
#57388=CARTESIAN_POINT ( 'NONE',  ( -12.14591786802309592, -12.06949235617757132, 41.87390960531435979 ) ) ;
#57389=CARTESIAN_POINT ( 'NONE',  ( -0.05219959533937732626, 21.53943276465977519, 112.5010903946857042 ) ) ;
#57390=CARTESIAN_POINT ( 'NONE',  ( 4.483927247898790824, -16.52544592524335698, 75.20942372801901854 ) ) ;
#57391=CARTESIAN_POINT ( 'NONE',  ( 14.34966873604960469, 8.224510206698951720, 44.16557627198103120 ) ) ;
#57392=CARTESIAN_POINT ( 'NONE',  ( 15.80617190586769283, -15.72974639402175789, 70.62609039468567573 ) ) ;
#57393=CARTESIAN_POINT ( 'NONE',  ( -15.72974639402176322, -15.80617190586768395, 69.37609039468567573 ) ) ;
#57394=CARTESIAN_POINT ( 'NONE',  ( 21.53943276465977519, -0.05219959533907433946, 63.74890960531435979 ) ) ;
#57396=CARTESIAN_POINT ( 'NONE',  ( -5.153800228976328057, -19.02544592524343514, 37.29057627198102409 ) ) ;
#57397=CARTESIAN_POINT ( 'NONE',  ( -15.80617190586768217, 15.72974639402176855, 38.12609039468567573 ) ) ;
#57398=CARTESIAN_POINT ( 'NONE',  ( 0.05219959533910956823, 16.53943276465976808, 114.9989096053143669 ) ) ;
#57399=CARTESIAN_POINT ( 'NONE',  ( -19.03943276465977164, 0.05219959533909376836, 41.24890960531435269 ) ) ;
#57400=CARTESIAN_POINT ( 'NONE',  ( 14.29746914071049879, -8.314922557960816363, 88.33224293864769550 ) ) ;
#57401=CARTESIAN_POINT ( 'NONE',  ( 5.049401038298161559, -19.05341960407611168, 82.70724293864770971 ) ) ;
#57402=CARTESIAN_POINT ( 'NONE',  ( -4.379528057220328563, 16.55341960407611168, 45.20724293864769550 ) ) ;
#57403=CARTESIAN_POINT ( 'NONE',  ( 8.314922557960818139, 14.29746914071049879, 94.58224293864769550 ) ) ;
#57404=CARTESIAN_POINT ( 'NONE',  ( 18.62759615963271287, -10.81492255796078972, 63.33224293864770260 ) ) ;
#57405=CARTESIAN_POINT ( 'NONE',  ( 18.62759615963271287, -10.81492255796078972, 103.3322429386476955 ) ) ;
#57407=CARTESIAN_POINT ( 'NONE',  ( 5.153800228976335163, 19.02544592524342804, 69.79057627198103830 ) ) ;
#57408=CARTESIAN_POINT ( 'NONE',  ( 0.05219959533934541429, -16.53943276465976808, 25.00109039468567218 ) ) ;
#57409=CARTESIAN_POINT ( 'NONE',  ( 21.52544592524344225, -5.823673210054117533, 63.54057627198103830 ) ) ;
#57410=CARTESIAN_POINT ( 'NONE',  ( -15.80617190586768217, 15.72974639402176855, 93.12609039468568994 ) ) ;
#57411=CARTESIAN_POINT ( 'NONE',  ( 13.97604488694527802, 13.89961937509977652, 74.37390960531436690 ) ) ;
#57412=CARTESIAN_POINT ( 'NONE',  ( 10.81492255796106328, -18.62759615963255655, 20.41775706135234714 ) ) ;
#57413=CARTESIAN_POINT ( 'NONE',  ( 19.02544592524343514, -5.153800228976328945, 108.5405762719810383 ) ) ;
#57414=CARTESIAN_POINT ( 'NONE',  ( -12.06949235617739369, -12.14591786802326823, 89.37609039468568994 ) ) ;
#57415=CARTESIAN_POINT ( 'NONE',  ( -10.72451020669870658, -18.67979575497194134, 74.58442372801901854 ) ) ;
#57416=CARTESIAN_POINT ( 'NONE',  ( -10.81492255796105439, 18.62759615963255655, 97.91775706135236135 ) ) ;
#57417=CARTESIAN_POINT ( 'NONE',  ( -14.29746914071037622, -8.314922557961029526, 59.16775706135234714 ) ) ;
#57418=CARTESIAN_POINT ( 'NONE',  ( -10.72451020669870658, -18.67979575497194134, 34.58442372801900433 ) ) ;
#57419=CARTESIAN_POINT ( 'NONE',  ( 16.46253265017160672, -9.564922557960803928, 23.33224293864769194 ) ) ;
#57420=CARTESIAN_POINT ( 'NONE',  ( 18.67979575497194134, -10.72451020669871369, 85.83442372801901854 ) ) ;
#57421=CARTESIAN_POINT ( 'NONE',  ( -18.67979575497178146, -10.72451020669898902, 91.66557627198103830 ) ) ;
#57422=CARTESIAN_POINT ( 'NONE',  ( 16.51473224551083163, -9.474510206698727899, 50.83442372801899722 ) ) ;
#57423=CARTESIAN_POINT ( 'NONE',  ( -21.52544592524343514, 5.823673210054127303, 51.04057627198103120 ) ) ;
#57424=CARTESIAN_POINT ( 'NONE',  ( -19.03943276465977164, 0.05219959533909376836, 91.24890960531436690 ) ) ;
#57425=CARTESIAN_POINT ( 'NONE',  ( 14.29746914071049879, -8.314922557960816363, 38.33224293864768839 ) ) ;
#57427=CARTESIAN_POINT ( 'NONE',  ( -16.51473224551082808, 9.474510206698731452, 68.33442372801900433 ) ) ;
#57429=CARTESIAN_POINT ( 'NONE',  ( -19.03943276465977164, -0.05219959533935918106, 103.7510903946856757 ) ) ;
#57430=CARTESIAN_POINT ( 'NONE',  ( 21.55341960407610458, 5.719274019375980345, 83.95724293864770971 ) ) ;
#57431=CARTESIAN_POINT ( 'NONE',  ( -12.14591786802309592, -12.06949235617757132, 51.87390960531437401 ) ) ;
#57432=CARTESIAN_POINT ( 'NONE',  ( 12.06949235617739724, 12.14591786802326823, 36.87609039468568994 ) ) ;
#57433=CARTESIAN_POINT ( 'NONE',  ( -16.46253265017160317, 9.564922557960807481, 40.83224293864769550 ) ) ;
#57434=CARTESIAN_POINT ( 'NONE',  ( -0.05219959533907301413, -21.53943276465977519, 112.4989096053143669 ) ) ;
#57435=CARTESIAN_POINT ( 'NONE',  ( 5.049401038297881783, 19.05341960407617563, 87.29275706135234714 ) ) ;
#57436=CARTESIAN_POINT ( 'NONE',  ( 5.153800228976335163, 19.02544592524342804, 89.79057627198102409 ) ) ;
#57437=CARTESIAN_POINT ( 'NONE',  ( -19.03943276465977164, 0.05219959533909376836, 71.24890960531435269 ) ) ;
#57438=CARTESIAN_POINT ( 'NONE',  ( 21.53943276465977519, -0.05219959533907433946, 78.74890960531436690 ) ) ;
#57439=CARTESIAN_POINT ( 'NONE',  ( -13.89961937509977652, 13.97604488694528158, 45.62390960531433848 ) ) ;
#57441=CARTESIAN_POINT ( 'NONE',  ( -12.14591786802309592, -12.06949235617757132, 61.87390960531436690 ) ) ;
#57442=CARTESIAN_POINT ( 'NONE',  ( 16.46253265017160672, -9.564922557960803928, 93.33224293864769550 ) ) ;
#57444=CARTESIAN_POINT ( 'NONE',  ( -5.153800228976607833, 19.02544592524334988, 67.70942372801900433 ) ) ;
#57445=CARTESIAN_POINT ( 'NONE',  ( -10.81492255796078084, -18.62759615963271287, 77.08224293864769550 ) ) ;
#57446=CARTESIAN_POINT ( 'NONE',  ( -13.97604488694547697, 13.89961937509957934, 38.12609039468566152 ) ) ;
#57447=CARTESIAN_POINT ( 'NONE',  ( 13.89961937509977652, -13.97604488694527269, 98.12390960531433848 ) ) ;
#57449=CARTESIAN_POINT ( 'NONE',  ( -21.52544592524343514, 5.823673210054127303, 36.04057627198102409 ) ) ;
#57451=CARTESIAN_POINT ( 'NONE',  ( 19.02544592524343514, -5.153800228976328945, 68.54057627198103830 ) ) ;
#57452=CARTESIAN_POINT ( 'NONE',  ( -15.80617190586768217, 15.72974639402176855, 63.12609039468568994 ) ) ;
#57453=CARTESIAN_POINT ( 'NONE',  ( -0.05219959533909027116, -19.03943276465977164, 22.49890960531436690 ) ) ;
#57454=CARTESIAN_POINT ( 'NONE',  ( 18.62759615963271287, -10.81492255796078972, 108.3322429386477097 ) ) ;
#57456=CARTESIAN_POINT ( 'NONE',  ( -18.62759615963255300, -10.81492255796106328, 54.16775706135235424 ) ) ;
#57458=CARTESIAN_POINT ( 'NONE',  ( -9.474510206698964154, 16.51473224551069663, 105.4155762719810383 ) ) ;
#57460=CARTESIAN_POINT ( 'NONE',  ( 10.72451020669898902, -18.67979575497178502, 102.9155762719810383 ) ) ;
#57461=CARTESIAN_POINT ( 'NONE',  ( -19.05341960407611168, -5.049401038298163336, 66.45724293864769550 ) ) ;
#57462=CARTESIAN_POINT ( 'NONE',  ( -14.34966873604972548, 8.224510206698743886, 38.33442372801900433 ) ) ;
#57463=EDGE_CURVE ( 'NONE', #199515, #106384, #49792, .T. ) ;
#57465=CARTESIAN_POINT ( 'NONE',  ( -21.53943276465977519, -0.05219959533937600094, 103.7510903946857042 ) ) ;
#57466=CARTESIAN_POINT ( 'NONE',  ( 9.474510206698971260, -16.51473224551069308, 42.91557627198103120 ) ) ;
#57467=CARTESIAN_POINT ( 'NONE',  ( -5.719274019375665041, -21.55341960407619695, 99.79275706135234714 ) ) ;
#57468=CARTESIAN_POINT ( 'NONE',  ( 5.049401038298161559, -19.05341960407611168, 82.70724293864770971 ) ) ;
#57469=CARTESIAN_POINT ( 'NONE',  ( 18.62759615963255655, 10.81492255796105972, 61.66775706135235424 ) ) ;
#57471=CARTESIAN_POINT ( 'NONE',  ( 9.474510206698971260, -16.51473224551069308, 107.9155762719810383 ) ) ;
#57472=CARTESIAN_POINT ( 'NONE',  ( -17.50000000000149214, 3.254303733634584805, 30.02395893071415145 ) ) ;
#57473=CARTESIAN_POINT ( 'NONE',  ( 12.06949235617739724, 12.14591786802326823, 46.87609039468568994 ) ) ;
#57474=CARTESIAN_POINT ( 'NONE',  ( 0.05219959533937995610, -21.53943276465977519, 55.00109039468568284 ) ) ;
#57475=CARTESIAN_POINT ( 'NONE',  ( -10.72451020669870658, -18.67979575497194134, 89.58442372801901854 ) ) ;
#57477=CARTESIAN_POINT ( 'NONE',  ( 14.34966873604972726, -8.224510206698740333, 30.83442372801902209 ) ) ;
#57478=CARTESIAN_POINT ( 'NONE',  ( 13.89961937509977652, -13.97604488694527269, 68.12390960531436690 ) ) ;
#57479=CARTESIAN_POINT ( 'NONE',  ( -13.97604488694527625, -13.89961937509977652, 111.8739096053143243 ) ) ;
#57482=CARTESIAN_POINT ( 'NONE',  ( -30.00000000000000000, -5.510910596163089556E-15, 45.00000000000000000 ) ) ;
#57483=CARTESIAN_POINT ( 'NONE',  ( 12.14591786802309770, 12.06949235617756955, 114.3739096053143527 ) ) ;
#57484=CARTESIAN_POINT ( 'NONE',  ( 15.72974639402199770, -15.80617190586745480, 48.12390960531436690 ) ) ;
#57485=CARTESIAN_POINT ( 'NONE',  ( 12.06949235617739724, 12.14591786802326823, 96.87609039468568994 ) ) ;
#57486=CARTESIAN_POINT ( 'NONE',  ( 4.483927247898545687, 16.52544592524342804, 79.79057627198102409 ) ) ;
#57487=CARTESIAN_POINT ( 'NONE',  ( 9.474510206698971260, -16.51473224551069308, 62.91557627198102409 ) ) ;
#57488=CARTESIAN_POINT ( 'NONE',  ( -21.55341960407619339, 5.719274019375674811, 93.54275706135234714 ) ) ;
#57490=CARTESIAN_POINT ( 'NONE',  ( 14.34966873604972726, -8.224510206698740333, 30.83442372801902209 ) ) ;
#57491=CARTESIAN_POINT ( 'NONE',  ( 16.55341960407611168, 4.379528057220329451, 83.95724293864770971 ) ) ;
#57492=CARTESIAN_POINT ( 'NONE',  ( -10.81492255796105439, 18.62759615963255655, 37.91775706135235424 ) ) ;
#57493=CARTESIAN_POINT ( 'NONE',  ( -21.55341960407610458, -5.719274019375992779, 71.45724293864769550 ) ) ;
#57494=CARTESIAN_POINT ( 'NONE',  ( 13.97604488694548053, -13.89961937509957401, 35.62609039468567573 ) ) ;
#57496=CARTESIAN_POINT ( 'NONE',  ( 9.474510206698971260, -16.51473224551069308, 87.91557627198102409 ) ) ;
#57497=CARTESIAN_POINT ( 'NONE',  ( 16.55341960407611168, 4.379528057220329451, 63.95724293864770260 ) ) ;
#57498=CARTESIAN_POINT ( 'NONE',  ( -4.483927247898539470, -16.52544592524342804, 32.29057627198102409 ) ) ;
#57499=CARTESIAN_POINT ( 'NONE',  ( 4.483927247898790824, -16.52544592524335698, 105.2094237280190328 ) ) ;
#57500=CARTESIAN_POINT ( 'NONE',  ( -13.89961937509957401, -13.97604488694547875, 64.37609039468567573 ) ) ;
#57501=CARTESIAN_POINT ( 'NONE',  ( -5.153800228976607833, 19.02544592524335343, 77.70942372801900433 ) ) ;
#57502=CARTESIAN_POINT ( 'NONE',  ( -21.53943276465977519, 0.05219959533907696930, 26.24890960531435624 ) ) ;
#57503=CARTESIAN_POINT ( 'NONE',  ( 8.224510206698953496, -14.34966873604960469, 92.91557627198103830 ) ) ;
#57505=CARTESIAN_POINT ( 'NONE',  ( -13.97604488694527625, -13.89961937509977652, 41.87390960531435979 ) ) ;
#57506=CARTESIAN_POINT ( 'NONE',  ( 10.81492255796078972, 18.62759615963270932, 44.58224293864769550 ) ) ;
#57507=CARTESIAN_POINT ( 'NONE',  ( -21.55341960407610458, -5.719274019375992779, 66.45724293864768129 ) ) ;
#57508=CARTESIAN_POINT ( 'NONE',  ( -14.29746914071049879, 8.314922557960819915, 110.8322429386476955 ) ) ;
#57509=CARTESIAN_POINT ( 'NONE',  ( 16.52544592524335698, 4.483927247898782831, 71.45942372801901854 ) ) ;
#57510=CARTESIAN_POINT ( 'NONE',  ( -16.46253265017160317, 9.564922557960807481, 50.83224293864770260 ) ) ;
#57512=CARTESIAN_POINT ( 'NONE',  ( -10.72451020669870658, -18.67979575497194134, 59.58442372801901854 ) ) ;
#57513=CARTESIAN_POINT ( 'NONE',  ( 16.53943276465976808, -0.05219959533910856209, 108.7489096053143669 ) ) ;
#57514=CARTESIAN_POINT ( 'NONE',  ( -13.89961937509957401, -13.97604488694547875, 89.37609039468563310 ) ) ;
#57517=CARTESIAN_POINT ( 'NONE',  ( 18.67979575497178502, 10.72451020669898547, 39.16557627198102409 ) ) ;
#57518=CARTESIAN_POINT ( 'NONE',  ( 16.46253265017160672, -9.564922557960803928, 28.33224293864769550 ) ) ;
#57519=CARTESIAN_POINT ( 'NONE',  ( 21.53943276465977519, 0.05219959533937863772, 76.25109039468568994 ) ) ;
#57520=CARTESIAN_POINT ( 'NONE',  ( 16.55341960407618274, -4.379528057220086978, 61.04275706135234714 ) ) ;
#57521=CARTESIAN_POINT ( 'NONE',  ( 16.52544592524342804, -4.483927247898539470, 48.54057627198103120 ) ) ;
#57522=CARTESIAN_POINT ( 'NONE',  ( -18.67979575497178146, -10.72451020669898902, 66.66557627198102409 ) ) ;
#57523=CARTESIAN_POINT ( 'NONE',  ( 21.55341960407610458, 5.719274019375980345, 68.95724293864769550 ) ) ;
#57525=CARTESIAN_POINT ( 'NONE',  ( -19.03943276465977164, -0.05219959533935918106, 83.75109039468567573 ) ) ;
#57526=CARTESIAN_POINT ( 'NONE',  ( 18.67979575497178502, 10.72451020669898547, 24.16557627198103120 ) ) ;
#57527=CARTESIAN_POINT ( 'NONE',  ( 19.02544592524343514, -5.153800228976328945, 48.54057627198103120 ) ) ;
#57528=CARTESIAN_POINT ( 'NONE',  ( -16.53943276465976808, 0.05219959533911058130, 111.2489096053143669 ) ) ;
#57529=CARTESIAN_POINT ( 'NONE',  ( -19.05341960407611168, -5.049401038298163336, 111.4572429386476671 ) ) ;
#57531=CARTESIAN_POINT ( 'NONE',  ( -16.52544592524335698, -4.483927247898792601, 78.95942372801901854 ) ) ;
#57532=CARTESIAN_POINT ( 'NONE',  ( -21.55341960407610458, -5.719274019375992779, 101.4572429386476955 ) ) ;
#57533=CARTESIAN_POINT ( 'NONE',  ( 19.02544592524343514, -5.153800228976328945, 73.54057627198103830 ) ) ;
#57534=CARTESIAN_POINT ( 'NONE',  ( 5.823673210054444382, -21.52544592524334988, 35.20942372801901854 ) ) ;
#57535=CARTESIAN_POINT ( 'NONE',  ( 16.46253265017160672, -9.564922557960803928, 98.33224293864769550 ) ) ;
#57538=CARTESIAN_POINT ( 'NONE',  ( 21.55341960407619695, -5.719274019375665929, 26.04275706135235779 ) ) ;
#57539=CARTESIAN_POINT ( 'NONE',  ( 16.51473224551069308, 9.474510206698969483, 29.16557627198103475 ) ) ;
#57540=CARTESIAN_POINT ( 'NONE',  ( -19.03943276465977164, -0.05219959533935918106, 83.75109039468567573 ) ) ;
#57541=CARTESIAN_POINT ( 'NONE',  ( -13.89961937509957401, -13.97604488694547875, 34.37609039468566863 ) ) ;
#57542=CARTESIAN_POINT ( 'NONE',  ( 5.823673210054125526, 21.52544592524343514, 114.7905762719810383 ) ) ;
#57543=CARTESIAN_POINT ( 'NONE',  ( -16.51473224551082808, 9.474510206698731452, 38.33442372801899722 ) ) ;
#57544=CARTESIAN_POINT ( 'NONE',  ( 13.97604488694548053, -13.89961937509957401, 55.62609039468566863 ) ) ;
#57545=CARTESIAN_POINT ( 'NONE',  ( 4.483927247898790824, -16.52544592524335698, 90.20942372801903275 ) ) ;
#57546=CARTESIAN_POINT ( 'NONE',  ( -5.049401038298153566, 19.05341960407611168, 115.2072429386477097 ) ) ;
#57547=CARTESIAN_POINT ( 'NONE',  ( 5.049401038298161559, -19.05341960407611168, 67.70724293864769550 ) ) ;
#57548=CARTESIAN_POINT ( 'NONE',  ( -21.52544592524334988, -5.823673210054445271, 78.95942372801901854 ) ) ;
#57549=CARTESIAN_POINT ( 'NONE',  ( -21.55341960407619339, 5.719274019375674811, 88.54275706135236135 ) ) ;
#57551=CARTESIAN_POINT ( 'NONE',  ( -9.474510206698964154, 16.51473224551069663, 90.41557627198103830 ) ) ;
#57552=CARTESIAN_POINT ( 'NONE',  ( -15.72974639402176322, -15.80617190586768395, 64.37609039468568994 ) ) ;
#57553=CARTESIAN_POINT ( 'NONE',  ( -16.51473224551082808, 9.474510206698731452, 103.3344237280190043 ) ) ;
#57554=CARTESIAN_POINT ( 'NONE',  ( 0.05219959533909260263, 19.03943276465977164, 59.99890960531436690 ) ) ;
#57555=CARTESIAN_POINT ( 'NONE',  ( 16.51473224551069308, 9.474510206698969483, 114.1655762719810241 ) ) ;
#57556=CARTESIAN_POINT ( 'NONE',  ( 19.02544592524343514, -5.153800228976328945, 73.54057627198103830 ) ) ;
#57557=CARTESIAN_POINT ( 'NONE',  ( -17.59860650958991002, -7.585241751807008548, 76.57662985737509587 ) ) ;
#57558=CARTESIAN_POINT ( 'NONE',  ( -13.89961937509977652, 13.97604488694528158, 70.62390960531432427 ) ) ;
#57559=CARTESIAN_POINT ( 'NONE',  ( 13.97604488694527802, 13.89961937509977652, 54.37390960531435979 ) ) ;
#57560=CARTESIAN_POINT ( 'NONE',  ( -21.53943276465977519, 0.05219959533907696930, 111.2489096053143669 ) ) ;
#57561=CARTESIAN_POINT ( 'NONE',  ( 16.53943276465976808, 0.05219959533934440121, 91.25109039468568994 ) ) ;
#57564=CARTESIAN_POINT ( 'NONE',  ( -9.564922557961040184, 16.46253265017147172, 62.91775706135233293 ) ) ;
#57565=CARTESIAN_POINT ( 'NONE',  ( -13.89961937509977652, 13.97604488694528158, 75.62390960531438111 ) ) ;
#57566=CARTESIAN_POINT ( 'NONE',  ( -12.06949235617756955, 12.14591786802309770, 70.62390960531436690 ) ) ;
#57567=CARTESIAN_POINT ( 'NONE',  ( -8.224510206698948167, 14.34966873604960824, 105.4155762719810383 ) ) ;
#57568=CARTESIAN_POINT ( 'NONE',  ( 18.67979575497178502, 10.72451020669898547, 29.16557627198103120 ) ) ;
#57569=CARTESIAN_POINT ( 'NONE',  ( 16.46253265017160672, -9.564922557960803928, 103.3322429386476955 ) ) ;
#57570=CARTESIAN_POINT ( 'NONE',  ( 16.52544592524342804, -4.483927247898539470, 93.54057627198103830 ) ) ;
#57572=CARTESIAN_POINT ( 'NONE',  ( 9.474510206698729675, 16.51473224551082808, 32.08442372801900433 ) ) ;
#57573=CARTESIAN_POINT ( 'NONE',  ( -4.483927247898782831, 16.52544592524335698, 102.7094237280190185 ) ) ;
#57574=CARTESIAN_POINT ( 'NONE',  ( 16.46253265017160672, -9.564922557960803928, 83.33224293864768129 ) ) ;
#57575=CARTESIAN_POINT ( 'NONE',  ( -21.55341960407619339, 5.719274019375674811, 58.54275706135235424 ) ) ;
#57576=CARTESIAN_POINT ( 'NONE',  ( 10.81492255796078972, 18.62759615963270932, 49.58224293864769550 ) ) ;
#57577=CARTESIAN_POINT ( 'NONE',  ( 0.05219959533937995610, -21.53943276465977519, 20.00109039468568639 ) ) ;
#57578=CARTESIAN_POINT ( 'NONE',  ( -10.81492255796078084, -18.62759615963271287, 67.08224293864770971 ) ) ;
#57579=CARTESIAN_POINT ( 'NONE',  ( 16.52544592524342804, -4.483927247898539470, 98.54057627198105251 ) ) ;
#57580=CARTESIAN_POINT ( 'NONE',  ( -16.51473224551082808, 9.474510206698731452, 53.33442372801900433 ) ) ;
#57581=CARTESIAN_POINT ( 'NONE',  ( 19.05341960407611168, 5.049401038298154454, 28.95724293864769550 ) ) ;
#57582=CARTESIAN_POINT ( 'NONE',  ( 16.46253265017160672, -9.564922557960803928, 78.33224293864769550 ) ) ;
#57583=CARTESIAN_POINT ( 'NONE',  ( 13.89961937509977652, -13.97604488694527269, 93.12390960531436690 ) ) ;
#57584=CARTESIAN_POINT ( 'NONE',  ( 16.46253265017160672, -9.564922557960803928, 23.33224293864769194 ) ) ;
#57585=CARTESIAN_POINT ( 'NONE',  ( -12.14591786802309592, -12.06949235617757132, 21.87390960531436690 ) ) ;
#57586=CARTESIAN_POINT ( 'NONE',  ( -8.224510206698735004, -14.34966873604973081, 34.58442372801900433 ) ) ;
#57587=CARTESIAN_POINT ( 'NONE',  ( -21.52544592524334988, -5.823673210054445271, 108.9594237280190185 ) ) ;
#57588=CARTESIAN_POINT ( 'NONE',  ( 19.02544592524343514, -5.153800228976328945, 98.54057627198100988 ) ) ;
#57589=CARTESIAN_POINT ( 'NONE',  ( 10.72451020669871369, 18.67979575497193778, 37.08442372801901143 ) ) ;
#57590=CARTESIAN_POINT ( 'NONE',  ( -16.51473224551069308, -9.474510206698971260, 46.66557627198102409 ) ) ;
#57591=CARTESIAN_POINT ( 'NONE',  ( 8.224510206698742110, 14.34966873604972548, 42.08442372801901854 ) ) ;
#57592=CARTESIAN_POINT ( 'NONE',  ( -14.34966873604972548, 8.224510206698743886, 108.3344237280190185 ) ) ;
#57593=CARTESIAN_POINT ( 'NONE',  ( -14.29746914071037622, -8.314922557961029526, 89.16775706135236135 ) ) ;
#57595=CARTESIAN_POINT ( 'NONE',  ( 16.51473224551083163, -9.474510206698727899, 105.8344237280190043 ) ) ;
#57596=CARTESIAN_POINT ( 'NONE',  ( 19.03943276465977164, -0.05219959533909143690, 28.74890960531435624 ) ) ;
#57597=CARTESIAN_POINT ( 'NONE',  ( -4.379528057220328563, 16.55341960407611168, 90.20724293864770971 ) ) ;
#57598=CARTESIAN_POINT ( 'NONE',  ( -5.719274019375978568, 21.55341960407610458, 105.2072429386477097 ) ) ;
#57599=CARTESIAN_POINT ( 'NONE',  ( 13.97604488694527802, 13.89961937509977652, 29.37390960531435979 ) ) ;
#57600=CARTESIAN_POINT ( 'NONE',  ( 9.564922557960805705, 16.46253265017160317, 104.5822429386476955 ) ) ;
#57601=CARTESIAN_POINT ( 'NONE',  ( -21.55341960407619339, 5.719274019375674811, 28.54275706135234358 ) ) ;
#57602=CARTESIAN_POINT ( 'NONE',  ( -16.51473224551069308, -9.474510206698971260, 21.66557627198102765 ) ) ;
#57603=CARTESIAN_POINT ( 'NONE',  ( 19.05341960407611168, 5.049401038298154454, 108.9572429386477097 ) ) ;
#57605=CARTESIAN_POINT ( 'NONE',  ( 19.02544592524343514, -5.153800228976328945, 78.54057627198099567 ) ) ;
#57606=CARTESIAN_POINT ( 'NONE',  ( -21.53943276465977519, -0.05219959533937600094, 33.75109039468568284 ) ) ;
#57607=CARTESIAN_POINT ( 'NONE',  ( 16.55341960407611168, 4.379528057220329451, 88.95724293864769550 ) ) ;
#57608=CARTESIAN_POINT ( 'NONE',  ( -5.153800228976328057, -19.02544592524343514, 102.2905762719810383 ) ) ;
#57609=CARTESIAN_POINT ( 'NONE',  ( -5.153800228976607833, 19.02544592524334988, 22.70942372801899012 ) ) ;
#57610=CARTESIAN_POINT ( 'NONE',  ( -0.05219959533934338120, 16.53943276465976808, 67.50109039468568994 ) ) ;
#57611=CARTESIAN_POINT ( 'NONE',  ( -18.67979575497193778, 10.72451020669871902, 73.33442372801901854 ) ) ;
#57613=CARTESIAN_POINT ( 'NONE',  ( 16.55341960407618274, -4.379528057220086978, 46.04275706135234714 ) ) ;
#57614=CARTESIAN_POINT ( 'NONE',  ( -16.46253265017160317, 9.564922557960807481, 85.83224293864769550 ) ) ;
#57615=CARTESIAN_POINT ( 'NONE',  ( 13.97604488694548053, -13.89961937509957401, 95.62609039468563310 ) ) ;
#57616=CARTESIAN_POINT ( 'NONE',  ( -4.379528057220086978, -16.55341960407618274, 74.79275706135234714 ) ) ;
#57617=CARTESIAN_POINT ( 'NONE',  ( 5.719274019375673035, 21.55341960407619339, 112.2927570613523471 ) ) ;
#57618=CARTESIAN_POINT ( 'NONE',  ( 0.05219959533936267826, -19.03943276465977164, 85.00109039468567573 ) ) ;
#57619=CARTESIAN_POINT ( 'NONE',  ( 5.153800228976335163, 19.02544592524342804, 69.79057627198103830 ) ) ;
#57620=CARTESIAN_POINT ( 'NONE',  ( -21.52544592524343514, 5.823673210054127303, 86.04057627198102409 ) ) ;
#57621=CARTESIAN_POINT ( 'NONE',  ( 8.314922557960818139, 14.29746914071049879, 84.58224293864769550 ) ) ;
#57622=CARTESIAN_POINT ( 'NONE',  ( -16.51473224551082808, 9.474510206698731452, 93.33442372801900433 ) ) ;
#57623=CARTESIAN_POINT ( 'NONE',  ( 14.29746914071037800, 8.314922557961029526, 56.66775706135235424 ) ) ;
#57624=CARTESIAN_POINT ( 'NONE',  ( 17.50000000000002132, -5.499999999999878320, 63.29690382534172954 ) ) ;
#57625=CARTESIAN_POINT ( 'NONE',  ( -9.564922557961040184, 16.46253265017147172, 57.91775706135233293 ) ) ;
#57627=CARTESIAN_POINT ( 'NONE',  ( -4.379528057220328563, 16.55341960407611168, 25.20724293864769550 ) ) ;
#57628=CARTESIAN_POINT ( 'NONE',  ( -4.483927247898539470, -16.52544592524342804, 77.29057627198102409 ) ) ;
#57629=CARTESIAN_POINT ( 'NONE',  ( -5.153800228976607833, 19.02544592524334988, 22.70942372801899012 ) ) ;
#57630=CARTESIAN_POINT ( 'NONE',  ( -16.52216118717247895, 7.221426719304377073, 38.92400978952973389 ) ) ;
#57631=CARTESIAN_POINT ( 'NONE',  ( -18.62759615963270932, 10.81492255796079327, 115.8322429386477097 ) ) ;
#57633=CARTESIAN_POINT ( 'NONE',  ( 19.03943276465977164, -0.05219959533909143690, 98.74890960531436690 ) ) ;
#57634=CARTESIAN_POINT ( 'NONE',  ( -9.564922557960796823, -16.46253265017161027, 82.08224293864768129 ) ) ;
#57635=CARTESIAN_POINT ( 'NONE',  ( -18.62759615963255300, -10.81492255796106328, 84.16775706135234714 ) ) ;
#57636=CARTESIAN_POINT ( 'NONE',  ( -19.05341960407611168, -5.049401038298163336, 61.45724293864769550 ) ) ;
#57637=CARTESIAN_POINT ( 'NONE',  ( -21.52544592524343514, 5.823673210054127303, 31.04057627198102409 ) ) ;
#57638=CARTESIAN_POINT ( 'NONE',  ( -12.06949235617756955, 12.14591786802309770, 75.62390960531439532 ) ) ;
#57639=CARTESIAN_POINT ( 'NONE',  ( -0.05219959533909027116, -19.03943276465977164, 37.49890960531436690 ) ) ;
#57640=CARTESIAN_POINT ( 'NONE',  ( 8.224510206698953496, -14.34966873604960469, 92.91557627198103830 ) ) ;
#57641=CARTESIAN_POINT ( 'NONE',  ( 15.80617190586746368, 15.72974639402197994, 104.3739096053143669 ) ) ;
#57642=CARTESIAN_POINT ( 'NONE',  ( 5.719274019375673035, 21.55341960407619339, 52.29275706135236135 ) ) ;
#57643=CARTESIAN_POINT ( 'NONE',  ( 13.89961937509977652, -13.97604488694527269, 28.12390960531435624 ) ) ;
#57644=CARTESIAN_POINT ( 'NONE',  ( -12.06949235617739369, -12.14591786802326823, 69.37609039468567573 ) ) ;
#57645=CARTESIAN_POINT ( 'NONE',  ( 10.81492255796078972, 18.62759615963270932, 99.58224293864770971 ) ) ;
#57646=CARTESIAN_POINT ( 'NONE',  ( -10.81492255796078084, -18.62759615963271287, 107.0822429386476955 ) ) ;
#57647=CARTESIAN_POINT ( 'NONE',  ( -0.05219959533936034679, 19.03943276465977164, 37.50109039468567573 ) ) ;
#57648=CARTESIAN_POINT ( 'NONE',  ( 9.474510206698971260, -16.51473224551069308, 57.91557627198103120 ) ) ;
#57650=CARTESIAN_POINT ( 'NONE',  ( 5.823673210054444382, -21.52544592524334988, 55.20942372801902565 ) ) ;
#57651=CARTESIAN_POINT ( 'NONE',  ( 5.823673210054125526, 21.52544592524343514, 54.79057627198104541 ) ) ;
#57652=CARTESIAN_POINT ( 'NONE',  ( -16.55341960407611168, -4.379528057220339221, 31.45724293864769550 ) ) ;
#57653=CARTESIAN_POINT ( 'NONE',  ( 21.55341960407619695, -5.719274019375665929, 76.04275706135237556 ) ) ;
#57654=CARTESIAN_POINT ( 'NONE',  ( -21.55341960407619339, 5.719274019375674811, 113.5427570613523756 ) ) ;
#57655=CARTESIAN_POINT ( 'NONE',  ( -8.314922557960811034, -14.29746914071050412, 62.08224293864769550 ) ) ;
#57656=CARTESIAN_POINT ( 'NONE',  ( -8.314922557960811034, -14.29746914071050412, 102.0822429386476955 ) ) ;
#57657=CARTESIAN_POINT ( 'NONE',  ( -19.05341960407617563, 5.049401038297882671, 43.54275706135232582 ) ) ;
#57658=CARTESIAN_POINT ( 'NONE',  ( -12.06949235617739369, -12.14591786802326823, 99.37609039468568994 ) ) ;
#57659=CARTESIAN_POINT ( 'NONE',  ( -21.53943276465977519, -0.05219959533937600094, 63.75109039468568284 ) ) ;
#57660=CARTESIAN_POINT ( 'NONE',  ( 9.564922557960805705, 16.46253265017160317, 59.58224293864769550 ) ) ;
#57661=CARTESIAN_POINT ( 'NONE',  ( -0.05219959533936034679, 19.03943276465977164, 32.50109039468566863 ) ) ;
#57662=CARTESIAN_POINT ( 'NONE',  ( -21.55341960407610458, -5.719274019375992779, 36.45724293864768839 ) ) ;
#57663=CARTESIAN_POINT ( 'NONE',  ( 15.72974639402176855, 15.80617190586768217, 36.87609039468568994 ) ) ;
#57664=CARTESIAN_POINT ( 'NONE',  ( -5.719274019375978568, 21.55341960407610458, 90.20724293864770971 ) ) ;
#57665=CARTESIAN_POINT ( 'NONE',  ( -16.46253265017146816, -9.564922557961047289, 89.16775706135234714 ) ) ;
#57666=CARTESIAN_POINT ( 'NONE',  ( 16.52544592524335698, 4.483927247898782831, 56.45942372801902565 ) ) ;
#57667=CARTESIAN_POINT ( 'NONE',  ( 17.50000000000001421, -3.190838340304443133, 37.39123124295112177 ) ) ;
#57668=CARTESIAN_POINT ( 'NONE',  ( 10.72451020669898902, -18.67979575497178502, 87.91557627198103830 ) ) ;
#57669=CARTESIAN_POINT ( 'NONE',  ( 4.483927247898790824, -16.52544592524335698, 80.20942372801901854 ) ) ;
#57670=CARTESIAN_POINT ( 'NONE',  ( -8.314922557960811034, -14.29746914071050412, 72.08224293864769550 ) ) ;
#57671=CARTESIAN_POINT ( 'NONE',  ( -17.12812012977026654, -6.668231424565994381, 101.3594875932314636 ) ) ;
#57672=CARTESIAN_POINT ( 'NONE',  ( -12.14591786802326823, 12.06949235617739902, 28.12609039468568284 ) ) ;
#57673=CARTESIAN_POINT ( 'NONE',  ( 15.72974639402199770, -15.80617190586745480, 33.12390960531435979 ) ) ;
#57674=CARTESIAN_POINT ( 'NONE',  ( -8.224510206698735004, -14.34966873604973081, 74.58442372801901854 ) ) ;
#57675=CARTESIAN_POINT ( 'NONE',  ( -13.89961937509977830, 13.97604488694528158, 95.62390960531436690 ) ) ;
#57676=CARTESIAN_POINT ( 'NONE',  ( -4.483927247898782831, 16.52544592524335698, 57.70942372801901143 ) ) ;
#57677=CARTESIAN_POINT ( 'NONE',  ( -21.53943276465977519, -0.05219959533937600094, 28.75109039468567929 ) ) ;
#57678=CARTESIAN_POINT ( 'NONE',  ( -10.72451020669898014, 18.67979575497178502, 45.41557627198103830 ) ) ;
#57679=CARTESIAN_POINT ( 'NONE',  ( 0.05219959533934541429, -16.53943276465976808, 65.00109039468568994 ) ) ;
#57680=CARTESIAN_POINT ( 'NONE',  ( 13.97604488694527802, 13.89961937509977652, 89.37390960531436690 ) ) ;
#57681=CARTESIAN_POINT ( 'NONE',  ( -21.55341960407619339, 5.719274019375674811, 53.54275706135234714 ) ) ;
#57682=CARTESIAN_POINT ( 'NONE',  ( 16.51473224551069308, 9.474510206698969483, 34.16557627198102409 ) ) ;
#57683=CARTESIAN_POINT ( 'NONE',  ( 5.823673210054125526, 21.52544592524343514, 39.79057627198103830 ) ) ;
#57685=CARTESIAN_POINT ( 'NONE',  ( 5.049401038297881783, 19.05341960407617563, 42.29275706135234003 ) ) ;
#57686=CARTESIAN_POINT ( 'NONE',  ( -16.55341960407617563, 4.379528057220093196, 53.54275706135234714 ) ) ;
#57687=CARTESIAN_POINT ( 'NONE',  ( -15.72974639402197994, 15.80617190586746368, 25.62390960531435624 ) ) ;
#57689=CARTESIAN_POINT ( 'NONE',  ( 9.474510206698971260, -16.51473224551069308, 82.91557627198103830 ) ) ;
#57690=CARTESIAN_POINT ( 'NONE',  ( -4.379528057220086978, -16.55341960407618274, 99.79275706135234714 ) ) ;
#57692=CARTESIAN_POINT ( 'NONE',  ( 8.224510206698953496, -14.34966873604960469, 92.91557627198103830 ) ) ;
#57693=CARTESIAN_POINT ( 'NONE',  ( -21.52544592524343514, 5.823673210054127303, 31.04057627198102409 ) ) ;
#57694=CARTESIAN_POINT ( 'NONE',  ( -16.51473224551069308, -9.474510206698971260, 36.66557627198102409 ) ) ;
#57695=CARTESIAN_POINT ( 'NONE',  ( 8.224510206698742110, 14.34966873604972548, 77.08442372801901854 ) ) ;
#57696=CARTESIAN_POINT ( 'NONE',  ( 21.52544592524344225, -5.823673210054117533, 113.5405762719810383 ) ) ;
#57697=CARTESIAN_POINT ( 'NONE',  ( -13.97604488694547697, 13.89961937509957934, 73.12609039468568994 ) ) ;
#57698=CARTESIAN_POINT ( 'NONE',  ( 19.05341960407611168, 5.049401038298154454, 33.95724293864769550 ) ) ;
#57700=CARTESIAN_POINT ( 'NONE',  ( -21.55341960407619339, 5.719274019375674811, 103.5427570613523613 ) ) ;
#57701=CARTESIAN_POINT ( 'NONE',  ( -9.474510206698964154, 16.51473224551069663, 70.41557627198102409 ) ) ;
#57702=CARTESIAN_POINT ( 'NONE',  ( -14.29746914071037622, -8.314922557961029526, 49.16775706135234003 ) ) ;
#57703=CARTESIAN_POINT ( 'NONE',  ( -18.67979575497193778, 10.72451020669871902, 93.33442372801901854 ) ) ;
#57704=CARTESIAN_POINT ( 'NONE',  ( -9.474510206698720793, -16.51473224551083518, 54.58442372801899722 ) ) ;
#57705=CARTESIAN_POINT ( 'NONE',  ( -9.564922557961040184, 16.46253265017147172, 47.91775706135233293 ) ) ;
#57706=ORIENTED_EDGE ( 'NONE', *, *, #82460, .F. ) ;
#57707=CARTESIAN_POINT ( 'NONE',  ( 18.62759615963255655, 10.81492255796105972, 46.66775706135234714 ) ) ;
#57709=CARTESIAN_POINT ( 'NONE',  ( -5.049401038297874678, -19.05341960407617918, 39.79275706135232582 ) ) ;
#57710=CARTESIAN_POINT ( 'NONE',  ( -19.03943276465977164, 0.05219959533909376836, 106.2489096053143669 ) ) ;
#57711=CARTESIAN_POINT ( 'NONE',  ( -13.89961937509977652, 13.97604488694528158, 85.62390960531433848 ) ) ;
#57712=CARTESIAN_POINT ( 'NONE',  ( -14.34966873604960291, -8.224510206698953496, 31.66557627198102054 ) ) ;
#57713=CARTESIAN_POINT ( 'NONE',  ( 10.72451020669898902, -18.67979575497178502, 27.91557627198103830 ) ) ;
#57716=CARTESIAN_POINT ( 'NONE',  ( 9.474510206698729675, 16.51473224551082808, 22.08442372801899722 ) ) ;
#57718=CARTESIAN_POINT ( 'NONE',  ( -5.153800228976328057, -19.02544592524343514, 42.29057627198101699 ) ) ;
#57719=CARTESIAN_POINT ( 'NONE',  ( -5.049401038298153566, 19.05341960407611168, 30.20724293864768839 ) ) ;
#57722=CARTESIAN_POINT ( 'NONE',  ( -16.55341960407617563, 4.379528057220093196, 68.54275706135234714 ) ) ;
#57723=CARTESIAN_POINT ( 'NONE',  ( 10.72451020669898902, -18.67979575497178502, 82.91557627198103830 ) ) ;
#57724=CARTESIAN_POINT ( 'NONE',  ( 12.14591786802309770, 12.06949235617756955, 44.37390960531435979 ) ) ;
#57725=CARTESIAN_POINT ( 'NONE',  ( -13.97604488694527625, -13.89961937509977652, 21.87390960531435979 ) ) ;
#57726=CARTESIAN_POINT ( 'NONE',  ( 16.51473224551069308, 9.474510206698969483, 109.1655762719810383 ) ) ;
#57727=CARTESIAN_POINT ( 'NONE',  ( -5.823673210054431948, 21.52544592524334988, 27.70942372801901854 ) ) ;
#57728=CARTESIAN_POINT ( 'NONE',  ( -19.05341960407617563, 5.049401038297882671, 33.54275706135231871 ) ) ;
#57729=CARTESIAN_POINT ( 'NONE',  ( -19.03943276465977164, 0.05219959533909376836, 36.24890960531436690 ) ) ;
#57730=CARTESIAN_POINT ( 'NONE',  ( 15.80617190586769283, -15.72974639402175789, 80.62609039468567573 ) ) ;
#57731=CARTESIAN_POINT ( 'NONE',  ( 17.50000000000000000, -5.624438216177593652, 33.31670344914648041 ) ) ;
#57732=CARTESIAN_POINT ( 'NONE',  ( 8.314922557960818139, 14.29746914071049879, 29.58224293864769905 ) ) ;
#57734=CARTESIAN_POINT ( 'NONE',  ( -18.62759615963270932, 10.81492255796079327, 30.83224293864770260 ) ) ;
#57735=CARTESIAN_POINT ( 'NONE',  ( -8.224510206698948167, 14.34966873604960824, 100.4155762719810241 ) ) ;
#57737=CARTESIAN_POINT ( 'NONE',  ( 13.97604488694527802, 13.89961937509977652, 84.37390960531433848 ) ) ;
#57738=CARTESIAN_POINT ( 'NONE',  ( -14.29746914071049879, 8.314922557960819915, 80.83224293864769550 ) ) ;
#57739=CARTESIAN_POINT ( 'NONE',  ( 13.89961937509957401, 13.97604488694547697, 106.8760903946856757 ) ) ;
#57740=CARTESIAN_POINT ( 'NONE',  ( 10.72451020669898902, -18.67979575497178502, 67.91557627198102409 ) ) ;
#57741=ORIENTED_EDGE ( 'NONE', *, *, #61248, .F. ) ;
#57742=CARTESIAN_POINT ( 'NONE',  ( -19.03943276465977164, 0.05219959533909376836, 26.24890960531435624 ) ) ;
#57743=CARTESIAN_POINT ( 'NONE',  ( -5.153800228976328057, -19.02544592524343514, 82.29057627198103830 ) ) ;
#57744=CARTESIAN_POINT ( 'NONE',  ( 10.72451020669898902, -18.67979575497178502, 92.91557627198103830 ) ) ;
#57745=CARTESIAN_POINT ( 'NONE',  ( 4.483927247898790824, -16.52544592524335698, 100.2094237280190043 ) ) ;
#57746=CARTESIAN_POINT ( 'NONE',  ( 9.564922557960805705, 16.46253265017160317, 84.58224293864769550 ) ) ;
#57747=CARTESIAN_POINT ( 'NONE',  ( 9.474510206698729675, 16.51473224551082808, 87.08442372801900433 ) ) ;
#57748=CARTESIAN_POINT ( 'NONE',  ( -18.62759615963255300, -10.81492255796106328, 89.16775706135236135 ) ) ;
#57749=CARTESIAN_POINT ( 'NONE',  ( 0.05219959533907565091, 21.53943276465977519, 79.99890960531435269 ) ) ;
#57750=CARTESIAN_POINT ( 'NONE',  ( 21.53943276465977519, -0.05219959533907433946, 33.74890960531436690 ) ) ;
#57751=CARTESIAN_POINT ( 'NONE',  ( 19.05341960407611168, 5.049401038298154454, 48.95724293864768129 ) ) ;
#57752=CARTESIAN_POINT ( 'NONE',  ( 12.06949235617757843, -12.14591786802309237, 23.12390960531436335 ) ) ;
#57753=CARTESIAN_POINT ( 'NONE',  ( 5.153800228976335163, 19.02544592524342804, 59.79057627198100988 ) ) ;
#57755=CARTESIAN_POINT ( 'NONE',  ( 16.51473224551083163, -9.474510206698727899, 30.83442372801900433 ) ) ;
#57756=CARTESIAN_POINT ( 'NONE',  ( -4.483927247898539470, -16.52544592524342804, 77.29057627198102409 ) ) ;
#57757=CARTESIAN_POINT ( 'NONE',  ( 10.72451020669898902, -18.67979575497178502, 112.9155762719810383 ) ) ;
#57758=CARTESIAN_POINT ( 'NONE',  ( -10.81492255796105439, 18.62759615963255655, 22.91775706135235069 ) ) ;
#57760=CARTESIAN_POINT ( 'NONE',  ( -5.719274019375978568, 21.55341960407610458, 60.20724293864768839 ) ) ;
#57761=CARTESIAN_POINT ( 'NONE',  ( 16.55341960407618274, -4.379528057220086978, 91.04275706135236135 ) ) ;
#57762=CARTESIAN_POINT ( 'NONE',  ( -16.53943276465976808, 0.05219959533911058130, 111.2489096053143669 ) ) ;
#57763=CARTESIAN_POINT ( 'NONE',  ( 13.97604488694527802, 13.89961937509977652, 59.37390960531434558 ) ) ;
#57764=CARTESIAN_POINT ( 'NONE',  ( -14.29746914071049879, 8.314922557960819915, 30.83224293864770260 ) ) ;
#57765=CARTESIAN_POINT ( 'NONE',  ( -15.72974639402176322, -15.80617190586768395, 49.37609039468569705 ) ) ;
#57766=CARTESIAN_POINT ( 'NONE',  ( 9.564922557960805705, 16.46253265017160317, 109.5822429386476955 ) ) ;
#57767=CARTESIAN_POINT ( 'NONE',  ( 21.52544592524334988, 5.823673210054432836, 86.45942372801901854 ) ) ;
#57768=CARTESIAN_POINT ( 'NONE',  ( -19.03943276465977164, 0.05219959533909376836, 26.24890960531435624 ) ) ;
#57769=CARTESIAN_POINT ( 'NONE',  ( 5.049401038298161559, -19.05341960407611168, 37.70724293864768839 ) ) ;
#57771=CARTESIAN_POINT ( 'NONE',  ( 18.62759615963255655, 10.81492255796105972, 81.66775706135236135 ) ) ;
#57772=CARTESIAN_POINT ( 'NONE',  ( -12.14591786802326823, 12.06949235617739902, 53.12609039468568284 ) ) ;
#57773=CARTESIAN_POINT ( 'NONE',  ( -5.719274019375665041, -21.55341960407619695, 69.79275706135234714 ) ) ;
#57774=CARTESIAN_POINT ( 'NONE',  ( 5.049401038298161559, -19.05341960407611168, 107.7072429386476955 ) ) ;
#57775=CARTESIAN_POINT ( 'NONE',  ( 16.51473224551083163, -9.474510206698727899, 85.83442372801900433 ) ) ;
#57776=CARTESIAN_POINT ( 'NONE',  ( 5.719274019375673035, 21.55341960407619339, 52.29275706135236135 ) ) ;
#57777=CARTESIAN_POINT ( 'NONE',  ( 14.29746914071037800, 8.314922557961029526, 26.66775706135235424 ) ) ;
#57778=CARTESIAN_POINT ( 'NONE',  ( 5.153800228976615827, -19.02544592524334988, 80.20942372801901854 ) ) ;
#57779=CARTESIAN_POINT ( 'NONE',  ( 0.05219959533909260263, 19.03943276465977164, 49.99890960531435979 ) ) ;
#57780=CARTESIAN_POINT ( 'NONE',  ( 9.474510206698729675, 16.51473224551082808, 82.08442372801899012 ) ) ;
#57781=CARTESIAN_POINT ( 'NONE',  ( -16.52544592524342804, 4.483927247898546575, 31.04057627198102409 ) ) ;
#57782=CARTESIAN_POINT ( 'NONE',  ( 13.97604488694548053, -13.89961937509957401, 90.62609039468567573 ) ) ;
#57783=CARTESIAN_POINT ( 'NONE',  ( -12.06949235617756955, 12.14591786802309770, 35.62390960531437401 ) ) ;
#57784=CARTESIAN_POINT ( 'NONE',  ( 5.049401038297881783, 19.05341960407617563, 62.29275706135234003 ) ) ;
#57785=CARTESIAN_POINT ( 'NONE',  ( -14.29746914071037622, -8.314922557961029526, 44.16775706135234714 ) ) ;
#57786=CARTESIAN_POINT ( 'NONE',  ( -16.51473224551082808, 9.474510206698731452, 23.33442372801900078 ) ) ;
#57787=CARTESIAN_POINT ( 'NONE',  ( 16.55341960407611168, 4.379528057220329451, 113.9572429386477239 ) ) ;
#57788=CARTESIAN_POINT ( 'NONE',  ( -19.05341960407611168, -5.049401038298163336, 36.45724293864766707 ) ) ;
#57789=CARTESIAN_POINT ( 'NONE',  ( 16.53943276465976808, 0.05219959533934440121, 51.25109039468568994 ) ) ;
#57792=CARTESIAN_POINT ( 'NONE',  ( -5.049401038298153566, 19.05341960407611168, 95.20724293864770971 ) ) ;
#57793=LINE ( 'NONE', #87118, #129739 ) ;
#57795=CARTESIAN_POINT ( 'NONE',  ( 16.46253265017146816, 9.564922557961045513, 96.66775706135233293 ) ) ;
#57796=CARTESIAN_POINT ( 'NONE',  ( 15.80617190586746368, 15.72974639402197994, 24.37390960531435979 ) ) ;
#57797=CARTESIAN_POINT ( 'NONE',  ( -0.05219959533937732626, 21.53943276465977519, 112.5010903946857042 ) ) ;
#57798=CARTESIAN_POINT ( 'NONE',  ( 5.049401038297881783, 19.05341960407617563, 112.2927570613523471 ) ) ;
#57799=CARTESIAN_POINT ( 'NONE',  ( -14.34966873604960291, -8.224510206698953496, 106.6655762719810383 ) ) ;
#57800=CARTESIAN_POINT ( 'NONE',  ( 19.05341960407611168, 5.049401038298154454, 43.95724293864769550 ) ) ;
#57801=CARTESIAN_POINT ( 'NONE',  ( 21.55341960407610458, 5.719274019375980345, 78.95724293864769550 ) ) ;
#57802=CARTESIAN_POINT ( 'NONE',  ( 13.89961937509977652, -13.97604488694527269, 33.12390960531434558 ) ) ;
#57803=CARTESIAN_POINT ( 'NONE',  ( -16.51473224551082808, 9.474510206698731452, 48.33442372801900433 ) ) ;
#57804=CARTESIAN_POINT ( 'NONE',  ( 19.03943276465977164, 0.05219959533936151252, 71.25109039468566152 ) ) ;
#57805=CARTESIAN_POINT ( 'NONE',  ( -14.29746914071049879, 8.314922557960819915, 50.83224293864770971 ) ) ;
#57806=CARTESIAN_POINT ( 'NONE',  ( -0.05219959533907301413, -21.53943276465977519, 32.49890960531435979 ) ) ;
#57807=CARTESIAN_POINT ( 'NONE',  ( 5.823673210054444382, -21.52544592524334988, 95.20942372801903275 ) ) ;
#57808=CARTESIAN_POINT ( 'NONE',  ( -21.52544592524343514, 5.823673210054127303, 81.04057627198102409 ) ) ;
#57809=CARTESIAN_POINT ( 'NONE',  ( 21.53943276465977519, 0.05219959533937863772, 71.25109039468568994 ) ) ;
#57810=CARTESIAN_POINT ( 'NONE',  ( 18.67979575497194134, -10.72451020669871369, 65.83442372801900433 ) ) ;
#57811=CARTESIAN_POINT ( 'NONE',  ( -9.474510206698964154, 16.51473224551069663, 90.41557627198103830 ) ) ;
#57812=CARTESIAN_POINT ( 'NONE',  ( 16.53943276465976808, 0.05219959533934440121, 96.25109039468568994 ) ) ;
#57813=CARTESIAN_POINT ( 'NONE',  ( -10.81492255796105439, 18.62759615963255655, 67.91775706135234714 ) ) ;
#57814=CARTESIAN_POINT ( 'NONE',  ( -13.89961937509977652, 13.97604488694528158, 50.62390960531435979 ) ) ;
#57815=CARTESIAN_POINT ( 'NONE',  ( 18.62759615963255655, 10.81492255796105972, 31.66775706135234358 ) ) ;
#57816=CARTESIAN_POINT ( 'NONE',  ( 19.02544592524343514, -5.153800228976328945, 68.54057627198103830 ) ) ;
#57817=CARTESIAN_POINT ( 'NONE',  ( 14.34966873604960469, 8.224510206698951720, 74.16557627198102409 ) ) ;
#57818=CARTESIAN_POINT ( 'NONE',  ( 12.14591786802309770, 12.06949235617756955, 39.37390960531436690 ) ) ;
#57819=CARTESIAN_POINT ( 'NONE',  ( 5.823673210054125526, 21.52544592524343514, 44.79057627198103120 ) ) ;
#57820=CARTESIAN_POINT ( 'NONE',  ( 19.02544592524343514, -5.153800228976328945, 43.54057627198103120 ) ) ;
#57821=CARTESIAN_POINT ( 'NONE',  ( -18.62759615963270932, 10.81492255796079327, 55.83224293864770260 ) ) ;
#57822=CARTESIAN_POINT ( 'NONE',  ( 13.89961937509957401, 13.97604488694547697, 51.87609039468566863 ) ) ;
#57823=CARTESIAN_POINT ( 'NONE',  ( -17.26172910966778318, -6.454744622555875111, 39.19353091350778584 ) ) ;
#57824=CARTESIAN_POINT ( 'NONE',  ( -12.06949235617756955, 12.14591786802309770, 65.62390960531436690 ) ) ;
#57825=CARTESIAN_POINT ( 'NONE',  ( -10.81492255796078084, -18.62759615963271287, 42.08224293864769550 ) ) ;
#57829=CARTESIAN_POINT ( 'NONE',  ( -16.53943276465976808, -0.05219959533934237506, 88.75109039468567573 ) ) ;
#57830=CARTESIAN_POINT ( 'NONE',  ( -16.51473224551082808, 9.474510206698731452, 73.33442372801900433 ) ) ;
#57831=CARTESIAN_POINT ( 'NONE',  ( -16.52544592524342804, 4.483927247898546575, 51.04057627198103120 ) ) ;
#57832=CARTESIAN_POINT ( 'NONE',  ( 17.40805194822033997, -6.112264579159255362, 53.33371272510612471 ) ) ;
#57833=CARTESIAN_POINT ( 'NONE',  ( -13.89961937509977652, 13.97604488694528158, 50.62390960531435979 ) ) ;
#57834=CARTESIAN_POINT ( 'NONE',  ( 4.379528057220339221, -16.55341960407611168, 42.70724293864770260 ) ) ;
#57835=CARTESIAN_POINT ( 'NONE',  ( 16.51473224551069308, 9.474510206698969483, 54.16557627198103120 ) ) ;
#57836=CARTESIAN_POINT ( 'NONE',  ( -5.049401038298153566, 19.05341960407611168, 70.20724293864769550 ) ) ;
#57837=CARTESIAN_POINT ( 'NONE',  ( -9.474510206698964154, 16.51473224551069663, 45.41557627198103120 ) ) ;
#57838=CARTESIAN_POINT ( 'NONE',  ( -21.53943276465977519, -0.05219959533937600094, 43.75109039468568284 ) ) ;
#57839=CARTESIAN_POINT ( 'NONE',  ( -19.03943276465977164, 0.05219959533909376836, 71.24890960531435269 ) ) ;
#57840=CARTESIAN_POINT ( 'NONE',  ( 13.89961937509977652, -13.97604488694527269, 23.12390960531436335 ) ) ;
#57841=CARTESIAN_POINT ( 'NONE',  ( -9.474510206698964154, 16.51473224551069663, 60.41557627198102409 ) ) ;
#57842=CARTESIAN_POINT ( 'NONE',  ( 5.719274019375991003, -21.55341960407610458, 47.70724293864770260 ) ) ;
#57844=CARTESIAN_POINT ( 'NONE',  ( -19.05341960407611168, -5.049401038298163336, 41.45724293864769550 ) ) ;
#57845=CARTESIAN_POINT ( 'NONE',  ( 5.719274019375991003, -21.55341960407610458, 42.70724293864770260 ) ) ;
#57846=CARTESIAN_POINT ( 'NONE',  ( -16.53943276465976808, -0.05219959533934237506, 98.75109039468568994 ) ) ;
#57847=CARTESIAN_POINT ( 'NONE',  ( -5.049401038297874678, -19.05341960407617918, 29.79275706135232227 ) ) ;
#57848=CARTESIAN_POINT ( 'NONE',  ( 0.05219959533934541429, -16.53943276465976808, 40.00109039468567573 ) ) ;
#57849=CARTESIAN_POINT ( 'NONE',  ( -0.05219959533934338120, 16.53943276465976808, 82.50109039468568994 ) ) ;
#57851=CARTESIAN_POINT ( 'NONE',  ( 8.314922557961029526, -14.29746914071037800, 65.41775706135234714 ) ) ;
#57852=CARTESIAN_POINT ( 'NONE',  ( 16.53943276465976808, 0.05219959533934440121, 41.25109039468568284 ) ) ;
#57853=CARTESIAN_POINT ( 'NONE',  ( 19.03943276465977164, -0.05219959533909143690, 108.7489096053143527 ) ) ;
#57854=CARTESIAN_POINT ( 'NONE',  ( -12.06949235617739369, -12.14591786802326823, 39.37609039468567573 ) ) ;
#57855=CARTESIAN_POINT ( 'NONE',  ( -13.89961937509977652, 13.97604488694528158, 30.62390960531435269 ) ) ;
#57856=CARTESIAN_POINT ( 'NONE',  ( 21.53943276465977519, 0.05219959533937863772, 26.25109039468567573 ) ) ;
#57857=CARTESIAN_POINT ( 'NONE',  ( 4.483927247898790824, -16.52544592524335698, 35.20942372801901854 ) ) ;
#57858=CARTESIAN_POINT ( 'NONE',  ( -4.379528057220086978, -16.55341960407618274, 94.79275706135234714 ) ) ;
#57859=CARTESIAN_POINT ( 'NONE',  ( 15.80617190586769283, -15.72974639402175789, 105.6260903946856899 ) ) ;
#57860=CARTESIAN_POINT ( 'NONE',  ( -19.02544592524334988, -5.153800228976617603, 93.95942372801900433 ) ) ;
#57862=CARTESIAN_POINT ( 'NONE',  ( -8.224510206698948167, 14.34966873604960824, 50.41557627198103120 ) ) ;
#57863=CARTESIAN_POINT ( 'NONE',  ( 19.03943276465977164, -0.05219959533909143690, 23.74890960531435269 ) ) ;
#57864=CARTESIAN_POINT ( 'NONE',  ( 9.564922557961047289, -16.46253265017146816, 60.41775706135233293 ) ) ;
#57865=CARTESIAN_POINT ( 'NONE',  ( 16.20579543436677739, 7.371946100355113884, 78.06520834171877254 ) ) ;
#57866=CARTESIAN_POINT ( 'NONE',  ( 15.80617190586769283, -15.72974639402175789, 60.62609039468567573 ) ) ;
#57867=CARTESIAN_POINT ( 'NONE',  ( -0.05219959533934338120, 16.53943276465976808, 32.50109039468568284 ) ) ;
#57869=CARTESIAN_POINT ( 'NONE',  ( 19.05341960407611168, 5.049401038298154454, 113.9572429386477097 ) ) ;
#57870=CARTESIAN_POINT ( 'NONE',  ( 21.52544592524344225, -5.823673210054117533, 68.54057627198103830 ) ) ;
#57871=CARTESIAN_POINT ( 'NONE',  ( 0.05219959533936267826, -19.03943276465977164, 105.0010903946856615 ) ) ;
#57872=CARTESIAN_POINT ( 'NONE',  ( 13.97604488694527802, 13.89961937509977652, 99.37390960531436690 ) ) ;
#57874=CARTESIAN_POINT ( 'NONE',  ( -16.51473224551069308, -9.474510206698971260, 21.66557627198102765 ) ) ;
#57875=CARTESIAN_POINT ( 'NONE',  ( -21.55341960407619339, 5.719274019375674811, 113.5427570613523756 ) ) ;
#57876=CARTESIAN_POINT ( 'NONE',  ( 19.03943276465977164, -0.05219959533909143690, 38.74890960531436690 ) ) ;
#57877=CARTESIAN_POINT ( 'NONE',  ( 21.52544592524334988, 5.823673210054432836, 56.45942372801902565 ) ) ;
#57878=CARTESIAN_POINT ( 'NONE',  ( -5.719274019375665041, -21.55341960407619695, 104.7927570613523898 ) ) ;
#57879=CARTESIAN_POINT ( 'NONE',  ( 16.55341960407618274, -4.379528057220086978, 106.0427570613523471 ) ) ;
#57880=CARTESIAN_POINT ( 'NONE',  ( 9.474510206698971260, -16.51473224551069308, 77.91557627198103830 ) ) ;
#57881=CARTESIAN_POINT ( 'NONE',  ( -5.719274019375665041, -21.55341960407619695, 44.79275706135234714 ) ) ;
#57882=CARTESIAN_POINT ( 'NONE',  ( 0.05219959533937995610, -21.53943276465977519, 55.00109039468568284 ) ) ;
#57883=CARTESIAN_POINT ( 'NONE',  ( -16.46253265017146816, -9.564922557961047289, 79.16775706135234714 ) ) ;
#57884=CARTESIAN_POINT ( 'NONE',  ( 13.89961937509977652, -13.97604488694527269, 88.12390960531438111 ) ) ;
#57885=CARTESIAN_POINT ( 'NONE',  ( 4.379528057220339221, -16.55341960407611168, 97.70724293864772392 ) ) ;
#57886=CARTESIAN_POINT ( 'NONE',  ( -10.72451020669898014, 18.67979575497178502, 95.41557627198102409 ) ) ;
#57887=CARTESIAN_POINT ( 'NONE',  ( -18.67979575497193778, 10.72451020669871902, 113.3344237280190328 ) ) ;
#57888=CARTESIAN_POINT ( 'NONE',  ( -8.314922557960811034, -14.29746914071050412, 92.08224293864769550 ) ) ;
#57889=CARTESIAN_POINT ( 'NONE',  ( -13.89961937509977652, 13.97604488694528158, 45.62390960531433848 ) ) ;
#57890=CARTESIAN_POINT ( 'NONE',  ( -5.049401038297874678, -19.05341960407617918, 84.79275706135233293 ) ) ;
#57891=CARTESIAN_POINT ( 'NONE',  ( -14.29746914071049879, 8.314922557960819915, 45.83224293864769550 ) ) ;
#57892=CARTESIAN_POINT ( 'NONE',  ( 10.72451020669871369, 18.67979575497193778, 102.0844237280190185 ) ) ;
#57893=CARTESIAN_POINT ( 'NONE',  ( 9.474510206698971260, -16.51473224551069308, 102.9155762719810241 ) ) ;
#57894=CARTESIAN_POINT ( 'NONE',  ( -9.564922557961040184, 16.46253265017147172, 72.91775706135233293 ) ) ;
#57895=CARTESIAN_POINT ( 'NONE',  ( -10.81492255796078084, -18.62759615963271287, 72.08224293864769550 ) ) ;
#57896=CARTESIAN_POINT ( 'NONE',  ( 15.80617190586769283, -15.72974639402175789, 35.62609039468568994 ) ) ;
#57897=CARTESIAN_POINT ( 'NONE',  ( 16.53943276465976808, 0.05219959533934440121, 36.25109039468567573 ) ) ;
#57898=CARTESIAN_POINT ( 'NONE',  ( -4.379528057220086978, -16.55341960407618274, 94.79275706135234714 ) ) ;
#57899=CARTESIAN_POINT ( 'NONE',  ( 17.48847506799967988, 5.747544572773808369, 61.67302562156719858 ) ) ;
#57900=CARTESIAN_POINT ( 'NONE',  ( 5.823673210054444382, -21.52544592524334988, 40.20942372801901854 ) ) ;
#57901=CARTESIAN_POINT ( 'NONE',  ( 18.67979575497178502, 10.72451020669898547, 39.16557627198102409 ) ) ;
#57902=CARTESIAN_POINT ( 'NONE',  ( -19.05341960407611168, -5.049401038298163336, 26.45724293864769550 ) ) ;
#57904=CARTESIAN_POINT ( 'NONE',  ( -8.314922557961024197, 14.29746914071037800, 67.91775706135234714 ) ) ;
#57905=CARTESIAN_POINT ( 'NONE',  ( -14.34966873604960291, -8.224510206698953496, 96.66557627198102409 ) ) ;
#57906=CARTESIAN_POINT ( 'NONE',  ( -0.05219959533907301413, -21.53943276465977519, 72.49890960531435269 ) ) ;
#57907=CARTESIAN_POINT ( 'NONE',  ( -16.53943276465976808, 0.05219959533911058130, 31.24890960531435979 ) ) ;
#57908=CARTESIAN_POINT ( 'NONE',  ( 4.483927247898790824, -16.52544592524335698, 55.20942372801902565 ) ) ;
#57909=CARTESIAN_POINT ( 'NONE',  ( -19.02544592524342804, 5.153800228976336051, 61.04057627198103120 ) ) ;
#57910=CARTESIAN_POINT ( 'NONE',  ( -4.483927247898782831, 16.52544592524335698, 97.70942372801904696 ) ) ;
#57911=CARTESIAN_POINT ( 'NONE',  ( 5.049401038297881783, 19.05341960407617563, 82.29275706135229029 ) ) ;
#57912=CARTESIAN_POINT ( 'NONE',  ( -15.72974639402197994, 15.80617190586746368, 90.62390960531436690 ) ) ;
#57913=CARTESIAN_POINT ( 'NONE',  ( 8.224510206698742110, 14.34966873604972548, 112.0844237280190185 ) ) ;
#57915=CARTESIAN_POINT ( 'NONE',  ( 5.153800228976335163, 19.02544592524342804, 114.7905762719810241 ) ) ;
#57916=CARTESIAN_POINT ( 'NONE',  ( -10.81492255796078084, -18.62759615963271287, 57.08224293864769550 ) ) ;
#57918=CARTESIAN_POINT ( 'NONE',  ( 12.14591786802327356, -12.06949235617739191, 90.62609039468567573 ) ) ;
#57920=CARTESIAN_POINT ( 'NONE',  ( 15.80617190586746368, 15.72974639402197994, 34.37390960531435979 ) ) ;
#57921=CARTESIAN_POINT ( 'NONE',  ( 17.50000000000147793, 3.254303733634550166, 107.4760410692860262 ) ) ;
#57922=CARTESIAN_POINT ( 'NONE',  ( 21.53943276465977519, -0.05219959533907433946, 93.74890960531436690 ) ) ;
#57923=CARTESIAN_POINT ( 'NONE',  ( 8.224510206698953496, -14.34966873604960469, 27.91557627198103830 ) ) ;
#57924=CARTESIAN_POINT ( 'NONE',  ( 9.564922557961047289, -16.46253265017146816, 110.4177570613523471 ) ) ;
#57925=CARTESIAN_POINT ( 'NONE',  ( 13.97604488694527802, 13.89961937509977652, 34.37390960531436690 ) ) ;
#57926=CARTESIAN_POINT ( 'NONE',  ( -8.314922557961024197, 14.29746914071037800, 32.91775706135234714 ) ) ;
#57927=CARTESIAN_POINT ( 'NONE',  ( -0.05219959533909027116, -19.03943276465977164, 47.49890960531435979 ) ) ;
#57929=CARTESIAN_POINT ( 'NONE',  ( 13.97604488694527802, 13.89961937509977652, 104.3739096053143385 ) ) ;
#57930=CARTESIAN_POINT ( 'NONE',  ( 5.153800228976335163, 19.02544592524342804, 104.7905762719809957 ) ) ;
#57931=CARTESIAN_POINT ( 'NONE',  ( 16.55341960407618274, -4.379528057220086978, 91.04275706135236135 ) ) ;
#57932=CARTESIAN_POINT ( 'NONE',  ( 9.564922557961047289, -16.46253265017146816, 90.41775706135234714 ) ) ;
#57933=CARTESIAN_POINT ( 'NONE',  ( -13.89961937509957401, -13.97604488694547875, 39.37609039468566152 ) ) ;
#57934=CARTESIAN_POINT ( 'NONE',  ( -18.67979575497178146, -10.72451020669898902, 71.66557627198100988 ) ) ;
#57935=CARTESIAN_POINT ( 'NONE',  ( -12.06949235617739369, -12.14591786802326823, 104.3760903946856899 ) ) ;
#57936=CARTESIAN_POINT ( 'NONE',  ( -5.823673210054116645, -21.52544592524344225, 37.29057627198102409 ) ) ;
#57937=CARTESIAN_POINT ( 'NONE',  ( -0.05219959533936034679, 19.03943276465977164, 87.50109039468567573 ) ) ;
#57938=CARTESIAN_POINT ( 'NONE',  ( -19.05341960407611168, -5.049401038298163336, 56.45724293864768129 ) ) ;
#57939=CARTESIAN_POINT ( 'NONE',  ( -19.02544592524342804, 5.153800228976336051, 106.0405762719810241 ) ) ;
#57940=CARTESIAN_POINT ( 'NONE',  ( 10.81492255796106328, -18.62759615963255655, 65.41775706135234714 ) ) ;
#57941=CARTESIAN_POINT ( 'NONE',  ( -0.05219959533909027116, -19.03943276465977164, 62.49890960531435979 ) ) ;
#57942=CARTESIAN_POINT ( 'NONE',  ( -4.379528057220328563, 16.55341960407611168, 105.2072429386477097 ) ) ;
#57944=CARTESIAN_POINT ( 'NONE',  ( 0.05219959533910956823, 16.53943276465976808, 79.99890960531435269 ) ) ;
#57945=CARTESIAN_POINT ( 'NONE',  ( 21.55341960407610458, 5.719274019375980345, 68.95724293864769550 ) ) ;
#57946=CARTESIAN_POINT ( 'NONE',  ( 5.049401038297881783, 19.05341960407617563, 87.29275706135234714 ) ) ;
#57948=CARTESIAN_POINT ( 'NONE',  ( 16.51473224551069308, 9.474510206698969483, 59.16557627198102409 ) ) ;
#57949=CARTESIAN_POINT ( 'NONE',  ( 16.88567814943194278, -6.947325034625397855, 71.20998877347402356 ) ) ;
#57950=CARTESIAN_POINT ( 'NONE',  ( -16.51473224551069308, -9.474510206698971260, 76.66557627198103830 ) ) ;
#57951=CARTESIAN_POINT ( 'NONE',  ( -19.05341960407611168, -5.049401038298163336, 91.45724293864766707 ) ) ;
#57952=CARTESIAN_POINT ( 'NONE',  ( 16.53943276465976808, 0.05219959533934440121, 71.25109039468568994 ) ) ;
#57953=CARTESIAN_POINT ( 'NONE',  ( -17.40805194822029378, -6.112264579159361055, 49.16628727489391082 ) ) ;
#57954=CARTESIAN_POINT ( 'NONE',  ( -13.97604488694547697, 13.89961937509957934, 48.12609039468566863 ) ) ;
#57955=CARTESIAN_POINT ( 'NONE',  ( 16.74137860779843123, 7.074371978128817240, 21.90872520115863864 ) ) ;
#57956=CARTESIAN_POINT ( 'NONE',  ( 0.05219959533909260263, 19.03943276465977164, 104.9989096053143669 ) ) ;
#57957=CARTESIAN_POINT ( 'NONE',  ( 16.52544592524335698, 4.483927247898782831, 106.4594237280190328 ) ) ;
#57959=CARTESIAN_POINT ( 'NONE',  ( -14.29746914071037622, -8.314922557961029526, 99.16775706135234714 ) ) ;
#57961=CARTESIAN_POINT ( 'NONE',  ( 14.34966873604972726, -8.224510206698740333, 65.83442372801900433 ) ) ;
#57963=CARTESIAN_POINT ( 'NONE',  ( -15.80617190586768217, 15.72974639402176855, 68.12609039468567573 ) ) ;
#57964=CARTESIAN_POINT ( 'NONE',  ( 19.03943276465977164, 0.05219959533936151252, 71.25109039468566152 ) ) ;
#57965=CARTESIAN_POINT ( 'NONE',  ( -19.03943276465977164, -0.05219959533935918106, 23.75109039468566152 ) ) ;
#57966=CARTESIAN_POINT ( 'NONE',  ( 0.05219959533909260263, 19.03943276465977164, 59.99890960531436690 ) ) ;
#57967=CARTESIAN_POINT ( 'NONE',  ( -5.049401038298153566, 19.05341960407611168, 40.20724293864768839 ) ) ;
#57968=CARTESIAN_POINT ( 'NONE',  ( 17.48701582056246551, -5.762792292030415098, 23.32825582371390638 ) ) ;
#57969=CARTESIAN_POINT ( 'NONE',  ( -15.80617190586745835, -15.72974639402198527, 86.87390960531438111 ) ) ;
#57970=CARTESIAN_POINT ( 'NONE',  ( -10.81492255796078084, -18.62759615963271287, 37.08224293864768129 ) ) ;
#57971=CARTESIAN_POINT ( 'NONE',  ( 0.05219959533910956823, 16.53943276465976808, 109.9989096053143527 ) ) ;
#57972=CARTESIAN_POINT ( 'NONE',  ( -8.224510206698735004, -14.34966873604973081, 54.58442372801901143 ) ) ;
#57974=CARTESIAN_POINT ( 'NONE',  ( 21.53943276465977519, 0.05219959533937863772, 31.25109039468568639 ) ) ;
#57975=CARTESIAN_POINT ( 'NONE',  ( 12.06949235617757843, -12.14591786802309237, 58.12390960531435979 ) ) ;
#57977=CARTESIAN_POINT ( 'NONE',  ( 16.53943276465976808, 0.05219959533934440121, 31.25109039468568639 ) ) ;
#57978=CARTESIAN_POINT ( 'NONE',  ( 9.564922557961047289, -16.46253265017146816, 45.41775706135232582 ) ) ;
#57979=CARTESIAN_POINT ( 'NONE',  ( -8.224510206698948167, 14.34966873604960824, 50.41557627198103120 ) ) ;
#57980=CARTESIAN_POINT ( 'NONE',  ( -10.72451020669898014, 18.67979575497178502, 110.4155762719810383 ) ) ;
#57982=CARTESIAN_POINT ( 'NONE',  ( 18.62759615963271287, -10.81492255796078972, 78.33224293864770971 ) ) ;
#57983=CARTESIAN_POINT ( 'NONE',  ( -9.474510206698964154, 16.51473224551069663, 85.41557627198102409 ) ) ;
#57984=CARTESIAN_POINT ( 'NONE',  ( 16.55341960407611168, 4.379528057220329451, 63.95724293864770260 ) ) ;
#57985=CARTESIAN_POINT ( 'NONE',  ( 16.51473224551069308, 9.474510206698969483, 109.1655762719810383 ) ) ;
#57988=CARTESIAN_POINT ( 'NONE',  ( -13.97604488694547697, 13.89961937509957934, 68.12609039468563310 ) ) ;
#57989=CARTESIAN_POINT ( 'NONE',  ( 10.81492255796078972, 18.62759615963270932, 109.5822429386476955 ) ) ;
#57990=CARTESIAN_POINT ( 'NONE',  ( -16.46253265017160317, 9.564922557960807481, 55.83224293864769550 ) ) ;
#57991=CARTESIAN_POINT ( 'NONE',  ( 12.06949235617757843, -12.14591786802309237, 113.1239096053143953 ) ) ;
#57993=CARTESIAN_POINT ( 'NONE',  ( -21.55341960407619339, 5.719274019375674811, 68.54275706135234714 ) ) ;
#57995=CARTESIAN_POINT ( 'NONE',  ( 16.52544592524342804, -4.483927247898539470, 38.54057627198103120 ) ) ;
#57996=CARTESIAN_POINT ( 'NONE',  ( 16.51473224551069308, 9.474510206698969483, 49.16557627198102409 ) ) ;
#57997=CARTESIAN_POINT ( 'NONE',  ( 16.46253265017160672, -9.564922557960803928, 113.3322429386476955 ) ) ;
#57998=CARTESIAN_POINT ( 'NONE',  ( 5.823673210054125526, 21.52544592524343514, 69.79057627198102409 ) ) ;
#58000=CARTESIAN_POINT ( 'NONE',  ( 0.05219959533909260263, 19.03943276465977164, 39.99890960531436690 ) ) ;
#58001=CARTESIAN_POINT ( 'NONE',  ( 5.719274019375991003, -21.55341960407610458, 67.70724293864769550 ) ) ;
#58002=CARTESIAN_POINT ( 'NONE',  ( 15.80617190586769283, -15.72974639402175789, 85.62609039468568994 ) ) ;
#58004=CARTESIAN_POINT ( 'NONE',  ( -4.379528057220086978, -16.55341960407618274, 84.79275706135234714 ) ) ;
#58005=CARTESIAN_POINT ( 'NONE',  ( -16.53943276465976808, 0.05219959533911058130, 86.24890960531436690 ) ) ;
#58006=CARTESIAN_POINT ( 'NONE',  ( -16.51473224551069308, -9.474510206698971260, 71.66557627198102409 ) ) ;
#58008=CARTESIAN_POINT ( 'NONE',  ( -5.049401038297874678, -19.05341960407617918, 39.79275706135232582 ) ) ;
#58009=CARTESIAN_POINT ( 'NONE',  ( 4.379528057220092307, 16.55341960407617563, 92.29275706135236135 ) ) ;
#58010=CARTESIAN_POINT ( 'NONE',  ( -5.049401038297874678, -19.05341960407617918, 19.79275706135233293 ) ) ;
#58011=CARTESIAN_POINT ( 'NONE',  ( 9.474510206698971260, -16.51473224551069308, 92.91557627198103830 ) ) ;
#58012=CARTESIAN_POINT ( 'NONE',  ( 15.72974639402199770, -15.80617190586745480, 43.12390960531435269 ) ) ;
#58013=CARTESIAN_POINT ( 'NONE',  ( 21.53943276465977519, 0.05219959533937863772, 101.2510903946856757 ) ) ;
#58014=CARTESIAN_POINT ( 'NONE',  ( 8.314922557961029526, -14.29746914071037800, 65.41775706135234714 ) ) ;
#58015=CARTESIAN_POINT ( 'NONE',  ( -21.55341960407610458, -5.719274019375992779, 106.4572429386477097 ) ) ;
#58016=CARTESIAN_POINT ( 'NONE',  ( 12.14591786802327356, -12.06949235617739191, 30.62609039468567929 ) ) ;
#58017=CARTESIAN_POINT ( 'NONE',  ( 13.89961937509977652, -13.97604488694527269, 88.12390960531438111 ) ) ;
#58018=CARTESIAN_POINT ( 'NONE',  ( -4.483927247898782831, 16.52544592524335698, 22.70942372801901499 ) ) ;
#58019=CARTESIAN_POINT ( 'NONE',  ( -5.153800228976328057, -19.02544592524343514, 47.29057627198102409 ) ) ;
#58021=CARTESIAN_POINT ( 'NONE',  ( -8.224510206698735004, -14.34966873604973081, 29.58442372801901854 ) ) ;
#58022=CARTESIAN_POINT ( 'NONE',  ( 0.05219959533910956823, 16.53943276465976808, 84.99890960531436690 ) ) ;
#58023=CARTESIAN_POINT ( 'NONE',  ( -16.53943276465976808, -0.05219959533934237506, 93.75109039468567573 ) ) ;
#58024=CARTESIAN_POINT ( 'NONE',  ( 15.80617190586769283, -15.72974639402175789, 40.62609039468567573 ) ) ;
#58025=CARTESIAN_POINT ( 'NONE',  ( 19.02544592524343514, -5.153800228976328945, 68.54057627198103830 ) ) ;
#58026=CARTESIAN_POINT ( 'NONE',  ( -19.02544592524342804, 5.153800228976336051, 76.04057627198102409 ) ) ;
#58027=CARTESIAN_POINT ( 'NONE',  ( -14.29746914071049879, 8.314922557960819915, 30.83224293864770260 ) ) ;
#58028=CARTESIAN_POINT ( 'NONE',  ( 14.34966873604972726, -8.224510206698740333, 80.83442372801901854 ) ) ;
#58030=CARTESIAN_POINT ( 'NONE',  ( 13.89961937509957401, 13.97604488694547697, 26.87609039468566507 ) ) ;
#58031=CARTESIAN_POINT ( 'NONE',  ( 9.564922557960805705, 16.46253265017160317, 99.58224293864770971 ) ) ;
#58032=CARTESIAN_POINT ( 'NONE',  ( 13.89961937509977652, -13.97604488694527269, 43.12390960531434558 ) ) ;
#58034=CARTESIAN_POINT ( 'NONE',  ( 14.34966873604972726, -8.224510206698740333, 40.83442372801901854 ) ) ;
#58035=CARTESIAN_POINT ( 'NONE',  ( 13.89961937509957401, 13.97604488694547697, 71.87609039468567573 ) ) ;
#58036=CARTESIAN_POINT ( 'NONE',  ( -14.29746914071037622, -8.314922557961029526, 59.16775706135234714 ) ) ;
#58037=FACE_OUTER_BOUND ( 'NONE', #10947, .T. ) ;
#58038=CARTESIAN_POINT ( 'NONE',  ( 19.05341960407611168, 5.049401038298154454, 78.95724293864769550 ) ) ;
#58039=CARTESIAN_POINT ( 'NONE',  ( -10.72451020669870658, -18.67979575497194134, 19.58442372801901143 ) ) ;
#58040=CARTESIAN_POINT ( 'NONE',  ( 19.05341960407617918, -5.049401038297876454, 61.04275706135232582 ) ) ;
#58041=CARTESIAN_POINT ( 'NONE',  ( 19.03943276465977164, -0.05219959533909143690, 103.7489096053143669 ) ) ;
#58042=CARTESIAN_POINT ( 'NONE',  ( -5.049401038298153566, 19.05341960407611168, 40.20724293864768839 ) ) ;
#58043=CARTESIAN_POINT ( 'NONE',  ( -5.153800228976328057, -19.02544592524343514, 77.29057627198099567 ) ) ;
#58044=CARTESIAN_POINT ( 'NONE',  ( 12.06949235617757843, -12.14591786802309237, 33.12390960531435979 ) ) ;
#58045=CARTESIAN_POINT ( 'NONE',  ( 5.153800228976335163, 19.02544592524342804, 29.79057627198102409 ) ) ;
#58046=CARTESIAN_POINT ( 'NONE',  ( -0.05219959533936034679, 19.03943276465977164, 32.50109039468566863 ) ) ;
#58047=CARTESIAN_POINT ( 'NONE',  ( -16.52544592524342804, 4.483927247898546575, 71.04057627198103830 ) ) ;
#58048=CARTESIAN_POINT ( 'NONE',  ( -15.72974639402176322, -15.80617190586768395, 109.3760903946857042 ) ) ;
#58049=CARTESIAN_POINT ( 'NONE',  ( -9.564922557960796823, -16.46253265017161027, 57.08224293864769550 ) ) ;
#58050=CARTESIAN_POINT ( 'NONE',  ( -12.06949235617756955, 12.14591786802309770, 40.62390960531435269 ) ) ;
#58051=CARTESIAN_POINT ( 'NONE',  ( -21.55341960407619339, 5.719274019375674811, 103.5427570613523613 ) ) ;
#58052=CARTESIAN_POINT ( 'NONE',  ( 13.97604488694527802, 13.89961937509977652, 99.37390960531436690 ) ) ;
#58053=CARTESIAN_POINT ( 'NONE',  ( 16.51473224551069308, 9.474510206698969483, 114.1655762719810241 ) ) ;
#58054=CARTESIAN_POINT ( 'NONE',  ( 5.049401038298161559, -19.05341960407611168, 42.70724293864767418 ) ) ;
#58055=CARTESIAN_POINT ( 'NONE',  ( 8.314922557960818139, 14.29746914071049879, 104.5822429386477097 ) ) ;
#58056=CARTESIAN_POINT ( 'NONE',  ( -12.06949235617756955, 12.14591786802309770, 90.62390960531436690 ) ) ;
#58057=CARTESIAN_POINT ( 'NONE',  ( -15.80617190586745835, -15.72974639402198527, 101.8739096053143811 ) ) ;
#58058=CARTESIAN_POINT ( 'NONE',  ( -16.46253265017160317, 9.564922557960807481, 90.83224293864769550 ) ) ;
#58059=CARTESIAN_POINT ( 'NONE',  ( 21.53943276465977519, -0.05219959533907433946, 98.74890960531438111 ) ) ;
#58060=CARTESIAN_POINT ( 'NONE',  ( 19.03943276465977164, -0.05219959533909143690, 88.74890960531436690 ) ) ;
#58062=CARTESIAN_POINT ( 'NONE',  ( 16.55341960407611168, 4.379528057220329451, 108.9572429386476955 ) ) ;
#58063=CARTESIAN_POINT ( 'NONE',  ( -19.05341960407611168, -5.049401038298163336, 66.45724293864769550 ) ) ;
#58064=CARTESIAN_POINT ( 'NONE',  ( -18.67979575497178146, -10.72451020669898902, 81.66557627198103830 ) ) ;
#58067=CARTESIAN_POINT ( 'NONE',  ( -10.72451020669898014, 18.67979575497178502, 30.41557627198101699 ) ) ;
#58068=DIRECTION ( 'NONE',  ( -0.000000000000000000, -0.000000000000000000, 1.000000000000000000 ) ) ;
#58069=CARTESIAN_POINT ( 'NONE',  ( -4.483927247898782831, 16.52544592524335698, 27.70942372801901854 ) ) ;
#58070=CARTESIAN_POINT ( 'NONE',  ( 16.52544592524342804, -4.483927247898539470, 98.54057627198105251 ) ) ;
#58072=CARTESIAN_POINT ( 'NONE',  ( -5.049401038298153566, 19.05341960407611168, 85.20724293864766707 ) ) ;
#58073=CARTESIAN_POINT ( 'NONE',  ( -9.564922557960796823, -16.46253265017161027, 47.08224293864769550 ) ) ;
#58074=CARTESIAN_POINT ( 'NONE',  ( -0.05219959533910754901, -16.53943276465976808, 77.49890960531433848 ) ) ;
#58075=CARTESIAN_POINT ( 'NONE',  ( -5.049401038298153566, 19.05341960407611168, 115.2072429386477097 ) ) ;
#58076=CARTESIAN_POINT ( 'NONE',  ( 16.55341960407611168, 4.379528057220329451, 53.95724293864770260 ) ) ;
#58077=CARTESIAN_POINT ( 'NONE',  ( 9.474510206698729675, 16.51473224551082808, 107.0844237280190043 ) ) ;
#58078=CARTESIAN_POINT ( 'NONE',  ( -10.81492255796105439, 18.62759615963255655, 57.91775706135234714 ) ) ;
#58080=CARTESIAN_POINT ( 'NONE',  ( 5.049401038298161559, -19.05341960407611168, 97.70724293864766707 ) ) ;
#58081=CARTESIAN_POINT ( 'NONE',  ( 14.34966873604972726, -8.224510206698740333, 80.83442372801901854 ) ) ;
#58082=CARTESIAN_POINT ( 'NONE',  ( -13.97604488694527625, -13.89961937509977652, 31.87390960531435979 ) ) ;
#58083=CARTESIAN_POINT ( 'NONE',  ( 16.51473224551069308, 9.474510206698969483, 79.16557627198103830 ) ) ;
#58084=CARTESIAN_POINT ( 'NONE',  ( -21.53943276465977519, 0.05219959533907696930, 86.24890960531436690 ) ) ;
#58085=CARTESIAN_POINT ( 'NONE',  ( 5.049401038297881783, 19.05341960407617563, 112.2927570613523471 ) ) ;
#58086=CARTESIAN_POINT ( 'NONE',  ( 12.06949235617757843, -12.14591786802309237, 48.12390960531436690 ) ) ;
#58087=CARTESIAN_POINT ( 'NONE',  ( 21.55341960407619695, -5.719274019375665929, 56.04275706135235424 ) ) ;
#58088=CARTESIAN_POINT ( 'NONE',  ( 8.224510206698742110, 14.34966873604972548, 87.08442372801901854 ) ) ;
#58089=CARTESIAN_POINT ( 'NONE',  ( -15.72974639402197994, 15.80617190586746368, 30.62390960531436335 ) ) ;
#58090=CARTESIAN_POINT ( 'NONE',  ( -13.97604488694527625, -13.89961937509977830, 111.8739096053143527 ) ) ;
#58092=CARTESIAN_POINT ( 'NONE',  ( -14.34966873604972548, 8.224510206698743886, 108.3344237280190185 ) ) ;
#58093=CARTESIAN_POINT ( 'NONE',  ( 8.314922557961029526, -14.29746914071037800, 65.41775706135234714 ) ) ;
#58094=CARTESIAN_POINT ( 'NONE',  ( -19.02544592524342804, 5.153800228976336051, 71.04057627198099567 ) ) ;
#58095=CARTESIAN_POINT ( 'NONE',  ( -5.049401038298153566, 19.05341960407611168, 80.20724293864769550 ) ) ;
#58096=CARTESIAN_POINT ( 'NONE',  ( -15.80617190586768217, 15.72974639402176855, 73.12609039468567573 ) ) ;
#58097=CARTESIAN_POINT ( 'NONE',  ( -0.05219959533934338120, 16.53943276465976808, 77.50109039468567573 ) ) ;
#58098=CARTESIAN_POINT ( 'NONE',  ( -12.14591786802309592, -12.06949235617757132, 41.87390960531435979 ) ) ;
#58099=CARTESIAN_POINT ( 'NONE',  ( -19.02544592524342804, 5.153800228976336051, 56.04057627198100988 ) ) ;
#58100=CARTESIAN_POINT ( 'NONE',  ( 5.049401038298161559, -19.05341960407611168, 47.70724293864770260 ) ) ;
#58101=CARTESIAN_POINT ( 'NONE',  ( -14.34966873604972548, 8.224510206698743886, 43.33442372801901143 ) ) ;
#58102=ORIENTED_EDGE ( 'NONE', *, *, #114142, .F. ) ;
#58103=CARTESIAN_POINT ( 'NONE',  ( 13.89961937509957401, 13.97604488694547697, 101.8760903946856331 ) ) ;
#58104=CARTESIAN_POINT ( 'NONE',  ( -8.314922557960811034, -14.29746914071050412, 97.08224293864770971 ) ) ;
#58105=CARTESIAN_POINT ( 'NONE',  ( 19.02544592524343514, -5.153800228976328945, 68.54057627198103830 ) ) ;
#58106=CARTESIAN_POINT ( 'NONE',  ( 13.89961937509957401, 13.97604488694547697, 101.8760903946856331 ) ) ;
#58108=CARTESIAN_POINT ( 'NONE',  ( 15.72974639402176855, 15.80617190586768217, 101.8760903946857042 ) ) ;
#58109=CARTESIAN_POINT ( 'NONE',  ( 12.14591786802327356, -12.06949235617739191, 65.62609039468568994 ) ) ;
#58111=CARTESIAN_POINT ( 'NONE',  ( 10.81492255796078972, 18.62759615963270932, 64.58224293864769550 ) ) ;
#58112=CARTESIAN_POINT ( 'NONE',  ( -4.483927247898782831, 16.52544592524335698, 52.70942372801902565 ) ) ;
#58114=CARTESIAN_POINT ( 'NONE',  ( -19.02544592524334988, -5.153800228976617603, 48.95942372801900433 ) ) ;
#58115=CARTESIAN_POINT ( 'NONE',  ( 16.51473224551069308, 9.474510206698969483, 84.16557627198102409 ) ) ;
#58116=CARTESIAN_POINT ( 'NONE',  ( -16.46253265017160317, 9.564922557960807481, 25.83224293864769194 ) ) ;
#58117=CARTESIAN_POINT ( 'NONE',  ( 19.05341960407611168, 5.049401038298154454, 68.95724293864769550 ) ) ;
#58118=CARTESIAN_POINT ( 'NONE',  ( -8.224510206698948167, 14.34966873604960824, 60.41557627198102409 ) ) ;
#58119=CARTESIAN_POINT ( 'NONE',  ( 21.53943276465977519, 0.05219959533937863772, 81.25109039468568994 ) ) ;
#58120=CARTESIAN_POINT ( 'NONE',  ( 16.46253265017146816, 9.564922557961045513, 46.66775706135233293 ) ) ;
#58121=CARTESIAN_POINT ( 'NONE',  ( 0.05219959533936267826, -19.03943276465977164, 30.00109039468566863 ) ) ;
#58122=CARTESIAN_POINT ( 'NONE',  ( -5.049401038298153566, 19.05341960407611168, 50.20724293864770260 ) ) ;
#58123=CARTESIAN_POINT ( 'NONE',  ( -5.823673210054116645, -21.52544592524344225, 22.29057627198102765 ) ) ;
#58124=CARTESIAN_POINT ( 'NONE',  ( -10.81492255796105439, 18.62759615963255655, 77.91775706135231871 ) ) ;
#58125=CARTESIAN_POINT ( 'NONE',  ( -13.97604488694527625, -13.89961937509977652, 66.87390960531436690 ) ) ;
#58126=CARTESIAN_POINT ( 'NONE',  ( -15.72974639402176322, -15.80617190586768395, 89.37609039468568994 ) ) ;
#58127=CARTESIAN_POINT ( 'NONE',  ( 10.81492255796078972, 18.62759615963270932, 39.58224293864769550 ) ) ;
#58128=CARTESIAN_POINT ( 'NONE',  ( -5.049401038298153566, 19.05341960407611168, 90.20724293864766707 ) ) ;
#58129=CARTESIAN_POINT ( 'NONE',  ( -0.05219959533937732626, 21.53943276465977519, 32.50109039468568284 ) ) ;
#58130=CARTESIAN_POINT ( 'NONE',  ( -19.05341960407617563, 5.049401038297882671, 58.54275706135234003 ) ) ;
#58131=CARTESIAN_POINT ( 'NONE',  ( 13.89961937509977652, -13.97604488694527269, 43.12390960531434558 ) ) ;
#58132=CARTESIAN_POINT ( 'NONE',  ( 5.153800228976335163, 19.02544592524342804, 94.79057627198103830 ) ) ;
#58133=CARTESIAN_POINT ( 'NONE',  ( -4.483927247898782831, 16.52544592524335698, 27.70942372801901854 ) ) ;
#58134=CARTESIAN_POINT ( 'NONE',  ( -0.05219959533910754901, -16.53943276465976808, 87.49890960531436690 ) ) ;
#58135=CARTESIAN_POINT ( 'NONE',  ( 13.97604488694527802, 13.89961937509977652, 74.37390960531436690 ) ) ;
#58136=CARTESIAN_POINT ( 'NONE',  ( -15.80617190586745835, -15.72974639402198527, 51.87390960531437401 ) ) ;
#58138=CARTESIAN_POINT ( 'NONE',  ( -16.53943276465976808, -0.05219959533934237506, 23.75109039468567929 ) ) ;
#58139=CARTESIAN_POINT ( 'NONE',  ( -0.05219959533907301413, -21.53943276465977519, 112.4989096053143669 ) ) ;
#58140=CARTESIAN_POINT ( 'NONE',  ( 18.67979575497194134, -10.72451020669871369, 75.83442372801900433 ) ) ;
#58141=CARTESIAN_POINT ( 'NONE',  ( 16.52544592524335698, 4.483927247898782831, 71.45942372801901854 ) ) ;
#58142=CARTESIAN_POINT ( 'NONE',  ( -14.29746914071037622, -8.314922557961029526, 74.16775706135231871 ) ) ;
#58143=CARTESIAN_POINT ( 'NONE',  ( -16.46253265017160317, 9.564922557960807481, 55.83224293864769550 ) ) ;
#58144=CARTESIAN_POINT ( 'NONE',  ( 14.29746914071037800, 8.314922557961029526, 106.6677570613523756 ) ) ;
#58145=CARTESIAN_POINT ( 'NONE',  ( -16.51473224551082808, 9.474510206698731452, 48.33442372801900433 ) ) ;
#58146=CARTESIAN_POINT ( 'NONE',  ( 15.72974639402176855, 15.80617190586768217, 26.87609039468567218 ) ) ;
#58147=CARTESIAN_POINT ( 'NONE',  ( 14.29746914071049879, -8.314922557960816363, 63.33224293864770260 ) ) ;
#58148=CARTESIAN_POINT ( 'NONE',  ( 19.05341960407611168, 5.049401038298154454, 103.9572429386476671 ) ) ;
#58149=CARTESIAN_POINT ( 'NONE',  ( -12.06949235617739369, -12.14591786802326823, 89.37609039468568994 ) ) ;
#58150=CARTESIAN_POINT ( 'NONE',  ( 10.81492255796106328, -18.62759615963255655, 55.41775706135234714 ) ) ;
#58151=CARTESIAN_POINT ( 'NONE',  ( 14.34966873604972726, -8.224510206698740333, 25.83442372801901499 ) ) ;
#58152=CARTESIAN_POINT ( 'NONE',  ( -0.05219959533937732626, 21.53943276465977519, 27.50109039468567929 ) ) ;
#58153=CARTESIAN_POINT ( 'NONE',  ( -12.14591786802309592, -12.06949235617757132, 61.87390960531436690 ) ) ;
#58155=CARTESIAN_POINT ( 'NONE',  ( 15.72974639402199770, -15.80617190586745480, 103.1239096053143811 ) ) ;
#58156=CARTESIAN_POINT ( 'NONE',  ( -16.53943276465976808, 0.05219959533911058130, 41.24890960531435269 ) ) ;
#58157=EDGE_LOOP ( 'NONE', ( #158472, #189699 ) ) ;
#58158=CARTESIAN_POINT ( 'NONE',  ( -16.51473224551069308, -9.474510206698971260, 26.66557627198103120 ) ) ;
#58159=CARTESIAN_POINT ( 'NONE',  ( 0.05219959533907565091, 21.53943276465977519, 29.99890960531435979 ) ) ;
#58160=CARTESIAN_POINT ( 'NONE',  ( 15.72974639402176855, 15.80617190586768217, 31.87609039468567929 ) ) ;
#58161=CARTESIAN_POINT ( 'NONE',  ( 0.05219959533910956823, 16.53943276465976808, 64.99890960531435269 ) ) ;
#58163=CARTESIAN_POINT ( 'NONE',  ( -10.72451020669898014, 18.67979575497178502, 60.41557627198102409 ) ) ;
#58164=CARTESIAN_POINT ( 'NONE',  ( 19.02544592524343514, -5.153800228976328945, 78.54057627198099567 ) ) ;
#58165=CARTESIAN_POINT ( 'NONE',  ( 19.02544592524343514, -5.153800228976328945, 23.54057627198102054 ) ) ;
#58166=CARTESIAN_POINT ( 'NONE',  ( -16.51473224551082808, 9.474510206698731452, 83.33442372801899012 ) ) ;
#58167=CARTESIAN_POINT ( 'NONE',  ( 21.53943276465977519, -0.05219959533907433946, 43.74890960531435979 ) ) ;
#58168=CARTESIAN_POINT ( 'NONE',  ( -9.564922557960796823, -16.46253265017161027, 62.08224293864769550 ) ) ;
#58170=CARTESIAN_POINT ( 'NONE',  ( -12.06949235617739369, -12.14591786802326823, 39.37609039468567573 ) ) ;
#58171=CARTESIAN_POINT ( 'NONE',  ( -10.81492255796078084, -18.62759615963271287, 112.0822429386477097 ) ) ;
#58172=CARTESIAN_POINT ( 'NONE',  ( 14.29746914071049879, -8.314922557960816363, 53.33224293864769550 ) ) ;
#58173=CARTESIAN_POINT ( 'NONE',  ( 5.049401038298161559, -19.05341960407611168, 107.7072429386476955 ) ) ;
#58174=CARTESIAN_POINT ( 'NONE',  ( -10.72451020669898014, 18.67979575497178502, 75.41557627198102409 ) ) ;
#58175=CARTESIAN_POINT ( 'NONE',  ( -0.05219959533907301413, -21.53943276465977519, 102.4989096053143811 ) ) ;
#58176=CARTESIAN_POINT ( 'NONE',  ( -12.06949235617739369, -12.14591786802326823, 54.37609039468568994 ) ) ;
#58177=CARTESIAN_POINT ( 'NONE',  ( -15.80617190586745835, -15.72974639402198527, 46.87390960531435979 ) ) ;
#58178=CARTESIAN_POINT ( 'NONE',  ( -5.823673210054431948, 21.52544592524334988, 97.70942372801904696 ) ) ;
#58179=CARTESIAN_POINT ( 'NONE',  ( -16.46253265017160317, 9.564922557960807481, 35.83224293864768839 ) ) ;
#58180=CARTESIAN_POINT ( 'NONE',  ( -0.05219959533909027116, -19.03943276465977164, 102.4989096053143669 ) ) ;
#58181=CARTESIAN_POINT ( 'NONE',  ( 9.474510206698971260, -16.51473224551069308, 72.91557627198102409 ) ) ;
#58183=CARTESIAN_POINT ( 'NONE',  ( -19.02544592524334988, -5.153800228976617603, 58.95942372801900433 ) ) ;
#58184=CARTESIAN_POINT ( 'NONE',  ( 19.03943276465977164, 0.05219959533936151252, 21.25109039468565797 ) ) ;
#58185=CARTESIAN_POINT ( 'NONE',  ( -18.62759615963270932, 10.81492255796079327, 30.83224293864770260 ) ) ;
#58186=CARTESIAN_POINT ( 'NONE',  ( -16.53943276465976808, -0.05219959533934237506, 103.7510903946857042 ) ) ;
#58187=CARTESIAN_POINT ( 'NONE',  ( -19.03943276465977164, -0.05219959533935918106, 83.75109039468567573 ) ) ;
#58189=CARTESIAN_POINT ( 'NONE',  ( 5.049401038297881783, 19.05341960407617563, 82.29275706135229029 ) ) ;
#58190=CARTESIAN_POINT ( 'NONE',  ( -16.51473224551082808, 9.474510206698731452, 48.33442372801900433 ) ) ;
#58191=CARTESIAN_POINT ( 'NONE',  ( -17.05587630539784882, -6.762274262135717251, 44.25819690962688213 ) ) ;
#58192=CARTESIAN_POINT ( 'NONE',  ( 9.564922557960805705, 16.46253265017160317, 44.58224293864769550 ) ) ;
#58193=CARTESIAN_POINT ( 'NONE',  ( 14.34966873604960469, 8.224510206698951720, 54.16557627198103120 ) ) ;
#58194=CARTESIAN_POINT ( 'NONE',  ( 9.564922557960805705, 16.46253265017160317, 29.58224293864769550 ) ) ;
#58195=CARTESIAN_POINT ( 'NONE',  ( 8.314922557960818139, 14.29746914071049879, 39.58224293864769550 ) ) ;
#58197=CARTESIAN_POINT ( 'NONE',  ( 0.05219959533934541429, -16.53943276465976808, 110.0010903946856757 ) ) ;
#58198=CARTESIAN_POINT ( 'NONE',  ( -5.049401038298153566, 19.05341960407611168, 50.20724293864770260 ) ) ;
#58199=CARTESIAN_POINT ( 'NONE',  ( 18.67979575497194134, -10.72451020669871369, 105.8344237280190328 ) ) ;
#58200=CARTESIAN_POINT ( 'NONE',  ( 19.03943276465977164, 0.05219959533936151252, 111.2510903946856757 ) ) ;
#58201=CARTESIAN_POINT ( 'NONE',  ( 5.823673210054125526, 21.52544592524343514, 39.79057627198103830 ) ) ;
#58202=CARTESIAN_POINT ( 'NONE',  ( -10.81492255796105439, 18.62759615963255655, 87.91775706135234714 ) ) ;
#58203=CARTESIAN_POINT ( 'NONE',  ( -19.02544592524342804, 5.153800228976336051, 101.0405762719810241 ) ) ;
#58204=CARTESIAN_POINT ( 'NONE',  ( 16.51473224551069308, 9.474510206698969483, 84.16557627198102409 ) ) ;
#58206=CARTESIAN_POINT ( 'NONE',  ( -5.719274019375978568, 21.55341960407610458, 105.2072429386477097 ) ) ;
#58207=CARTESIAN_POINT ( 'NONE',  ( 14.34966873604960469, 8.224510206698951720, 74.16557627198102409 ) ) ;
#58208=CARTESIAN_POINT ( 'NONE',  ( 21.52544592524344225, -5.823673210054117533, 68.54057627198103830 ) ) ;
#58209=CARTESIAN_POINT ( 'NONE',  ( 13.97604488694527802, 13.89961937509977652, 69.37390960531436690 ) ) ;
#58210=CARTESIAN_POINT ( 'NONE',  ( -15.72974639402197994, 15.80617190586746368, 90.62390960531436690 ) ) ;
#58212=CARTESIAN_POINT ( 'NONE',  ( 13.89961937509977652, -13.97604488694527269, 63.12390960531435979 ) ) ;
#58213=CARTESIAN_POINT ( 'NONE',  ( -12.14591786802309592, -12.06949235617757132, 91.87390960531436690 ) ) ;
#58214=CARTESIAN_POINT ( 'NONE',  ( 17.50000000000000000, -5.499999999999992895, 71.21769037696435589 ) ) ;
#58215=CARTESIAN_POINT ( 'NONE',  ( 19.05341960407611168, 5.049401038298154454, 63.95724293864769550 ) ) ;
#58216=CARTESIAN_POINT ( 'NONE',  ( -16.46253265017146816, -9.564922557961047289, 79.16775706135234714 ) ) ;
#58217=CARTESIAN_POINT ( 'NONE',  ( 8.224510206698953496, -14.34966873604960469, 92.91557627198103830 ) ) ;
#58218=CARTESIAN_POINT ( 'NONE',  ( 21.55341960407619695, -5.719274019375665929, 61.04275706135234714 ) ) ;
#58219=CARTESIAN_POINT ( 'NONE',  ( 9.564922557960805705, 16.46253265017160317, 49.58224293864770260 ) ) ;
#58220=CARTESIAN_POINT ( 'NONE',  ( 21.52544592524334988, 5.823673210054432836, 26.45942372801901854 ) ) ;
#58221=CARTESIAN_POINT ( 'NONE',  ( 4.379528057220339221, -16.55341960407611168, 97.70724293864772392 ) ) ;
#58222=DIRECTION ( 'NONE',  ( 0.000000000000000000, 0.000000000000000000, -1.000000000000000000 ) ) ;
#58223=CARTESIAN_POINT ( 'NONE',  ( -9.564922557960796823, -16.46253265017161027, 62.08224293864769550 ) ) ;
#58225=CARTESIAN_POINT ( 'NONE',  ( 0.05219959533936267826, -19.03943276465977164, 110.0010903946856757 ) ) ;
#58226=CARTESIAN_POINT ( 'NONE',  ( -21.53943276465977519, 0.05219959533907696930, 21.24890960531436690 ) ) ;
#58227=CARTESIAN_POINT ( 'NONE',  ( -15.80617190586768217, 15.72974639402176855, 43.12609039468568284 ) ) ;
#58228=CARTESIAN_POINT ( 'NONE',  ( -13.89961937509977652, 13.97604488694528158, 100.6239096053143669 ) ) ;
#58229=CARTESIAN_POINT ( 'NONE',  ( 19.05341960407617918, -5.049401038297876454, 81.04275706135231871 ) ) ;
#58230=CARTESIAN_POINT ( 'NONE',  ( -13.97604488694527625, -13.89961937509977652, 56.87390960531434558 ) ) ;
#58232=CARTESIAN_POINT ( 'NONE',  ( -14.29746914071049879, 8.314922557960819915, 85.83224293864768129 ) ) ;
#58233=CARTESIAN_POINT ( 'NONE',  ( 19.05341960407611168, 5.049401038298154454, 88.95724293864769550 ) ) ;
#58234=CARTESIAN_POINT ( 'NONE',  ( -8.314922557960811034, -14.29746914071050412, 72.08224293864769550 ) ) ;
#58235=CARTESIAN_POINT ( 'NONE',  ( -5.153800228976328057, -19.02544592524343514, 87.29057627198103830 ) ) ;
#58236=CARTESIAN_POINT ( 'NONE',  ( 19.03943276465977164, 0.05219959533936151252, 31.25109039468566863 ) ) ;
#58237=CARTESIAN_POINT ( 'NONE',  ( 19.03943276465977164, -0.05219959533909143690, 43.74890960531435979 ) ) ;
#58238=CARTESIAN_POINT ( 'NONE',  ( 8.314922557960818139, 14.29746914071049879, 49.58224293864769550 ) ) ;
#58239=CARTESIAN_POINT ( 'NONE',  ( 9.474510206698971260, -16.51473224551069308, 27.91557627198103120 ) ) ;
#58241=CARTESIAN_POINT ( 'NONE',  ( 5.823673210054444382, -21.52544592524334988, 45.20942372801901854 ) ) ;
#58242=CARTESIAN_POINT ( 'NONE',  ( -5.153800228976607833, 19.02544592524334988, 82.70942372801897591 ) ) ;
#58243=CARTESIAN_POINT ( 'NONE',  ( -16.55341960407611168, -4.379528057220339221, 36.45724293864768839 ) ) ;
#58244=CARTESIAN_POINT ( 'NONE',  ( -18.62759615963270932, 10.81492255796079327, 90.83224293864769550 ) ) ;
#58245=CARTESIAN_POINT ( 'NONE',  ( -15.72974639402197994, 15.80617190586746368, 30.62390960531436335 ) ) ;
#58246=CARTESIAN_POINT ( 'NONE',  ( 4.483927247898545687, 16.52544592524342804, 74.79057627198105251 ) ) ;
#58247=CARTESIAN_POINT ( 'NONE',  ( 19.03943276465977164, -0.05219959533909143690, 43.74890960531435979 ) ) ;
#58248=CARTESIAN_POINT ( 'NONE',  ( -8.314922557961024197, 14.29746914071037800, 97.91775706135236135 ) ) ;
#58249=CARTESIAN_POINT ( 'NONE',  ( 4.379528057220092307, 16.55341960407617563, 72.29275706135236135 ) ) ;
#58250=CARTESIAN_POINT ( 'NONE',  ( -16.51473224551082808, 9.474510206698731452, 28.33442372801900433 ) ) ;
#58251=CARTESIAN_POINT ( 'NONE',  ( -19.05341960407611168, -5.049401038298163336, 96.45724293864769550 ) ) ;
#58252=CARTESIAN_POINT ( 'NONE',  ( 16.51473224551069308, 9.474510206698969483, 84.16557627198102409 ) ) ;
#58253=CARTESIAN_POINT ( 'NONE',  ( -8.224510206698735004, -14.34966873604973081, 79.58442372801903275 ) ) ;
#58254=CARTESIAN_POINT ( 'NONE',  ( -13.89961937509977652, 13.97604488694528158, 30.62390960531435269 ) ) ;
#58255=CARTESIAN_POINT ( 'NONE',  ( 8.224510206698953496, -14.34966873604960469, 32.91557627198102409 ) ) ;
#58256=CARTESIAN_POINT ( 'NONE',  ( 9.564922557960805705, 16.46253265017160317, 99.58224293864770971 ) ) ;
#58257=CARTESIAN_POINT ( 'NONE',  ( -13.97604488694527625, -13.89961937509977652, 91.87390960531432427 ) ) ;
#58258=CARTESIAN_POINT ( 'NONE',  ( -5.823673210054116645, -21.52544592524344225, 22.29057627198102765 ) ) ;
#58259=CARTESIAN_POINT ( 'NONE',  ( 12.14591786802309770, 12.06949235617756955, 74.37390960531436690 ) ) ;
#58260=CARTESIAN_POINT ( 'NONE',  ( 0.05219959533910956823, 16.53943276465976808, 69.99890960531435269 ) ) ;
#58261=CARTESIAN_POINT ( 'NONE',  ( -0.05219959533934338120, 16.53943276465976808, 57.50109039468568994 ) ) ;
#58263=CARTESIAN_POINT ( 'NONE',  ( -13.89961937509957401, -13.97604488694547875, 44.37609039468566863 ) ) ;
#58264=CARTESIAN_POINT ( 'NONE',  ( -5.049401038298153566, 19.05341960407611168, 95.20724293864770971 ) ) ;
#58265=CARTESIAN_POINT ( 'NONE',  ( -13.89961937509957401, -13.97604488694547875, 59.37609039468566863 ) ) ;
#58266=CARTESIAN_POINT ( 'NONE',  ( 16.51473224551083163, -9.474510206698727899, 40.83442372801900433 ) ) ;
#58267=CARTESIAN_POINT ( 'NONE',  ( 16.55341960407618274, -4.379528057220086978, 21.04275706135234714 ) ) ;
#58268=CARTESIAN_POINT ( 'NONE',  ( 16.55341960407618274, -4.379528057220086978, 101.0427570613523756 ) ) ;
#58269=CARTESIAN_POINT ( 'NONE',  ( 13.89961937509977652, -13.97604488694527269, 43.12390960531434558 ) ) ;
#58270=CARTESIAN_POINT ( 'NONE',  ( 10.72451020669898902, -18.67979575497178502, 22.91557627198102765 ) ) ;
#58271=CARTESIAN_POINT ( 'NONE',  ( 18.67979575497194134, -10.72451020669871369, 50.83442372801901143 ) ) ;
#58272=CARTESIAN_POINT ( 'NONE',  ( 5.049401038297881783, 19.05341960407617563, 107.2927570613523187 ) ) ;
#58274=CARTESIAN_POINT ( 'NONE',  ( 0.05219959533909260263, 19.03943276465977164, 79.99890960531436690 ) ) ;
#58275=CARTESIAN_POINT ( 'NONE',  ( -19.05341960407611168, -5.049401038298163336, 111.4572429386476671 ) ) ;
#58276=CARTESIAN_POINT ( 'NONE',  ( 12.06949235617757843, -12.14591786802309237, 73.12390960531436690 ) ) ;
#58277=CARTESIAN_POINT ( 'NONE',  ( 19.03943276465977164, -0.05219959533909143690, 73.74890960531435269 ) ) ;
#58278=CARTESIAN_POINT ( 'NONE',  ( 0.05219959533909260263, 19.03943276465977164, 69.99890960531435269 ) ) ;
#58279=CARTESIAN_POINT ( 'NONE',  ( -19.03943276465977164, -0.05219959533935918106, 73.75109039468566152 ) ) ;
#58280=CARTESIAN_POINT ( 'NONE',  ( -18.62759615963270932, 10.81492255796079327, 65.83224293864769550 ) ) ;
#58281=CARTESIAN_POINT ( 'NONE',  ( -19.05341960407611168, -5.049401038298163336, 21.45724293864768839 ) ) ;
#58282=CARTESIAN_POINT ( 'NONE',  ( -9.564922557961040184, 16.46253265017147172, 57.91775706135233293 ) ) ;
#58283=CARTESIAN_POINT ( 'NONE',  ( 19.05341960407611168, 5.049401038298154454, 53.95724293864770260 ) ) ;
#58284=CARTESIAN_POINT ( 'NONE',  ( 13.89961937509977652, -13.97604488694527269, 93.12390960531436690 ) ) ;
#58285=CARTESIAN_POINT ( 'NONE',  ( 21.55341960407610458, 5.719274019375980345, 93.95724293864770971 ) ) ;
#58286=CARTESIAN_POINT ( 'NONE',  ( 4.483927247898545687, 16.52544592524342804, 89.79057627198103830 ) ) ;
#58287=CARTESIAN_POINT ( 'NONE',  ( -0.05219959533936034679, 19.03943276465977164, 42.50109039468566152 ) ) ;
#58288=CARTESIAN_POINT ( 'NONE',  ( 18.67979575497178502, 10.72451020669898547, 79.16557627198103830 ) ) ;
#58289=CARTESIAN_POINT ( 'NONE',  ( 18.67979575497178502, 10.72451020669898547, 54.16557627198103120 ) ) ;
#58290=CARTESIAN_POINT ( 'NONE',  ( 12.06949235617757843, -12.14591786802309237, 28.12390960531435979 ) ) ;
#58291=CARTESIAN_POINT ( 'NONE',  ( -21.55341960407619339, 5.719274019375674811, 108.5427570613523756 ) ) ;
#58292=CARTESIAN_POINT ( 'NONE',  ( -9.564922557960796823, -16.46253265017161027, 77.08224293864769550 ) ) ;
#58293=CARTESIAN_POINT ( 'NONE',  ( 0.05219959533909260263, 19.03943276465977164, 29.99890960531435979 ) ) ;
#58294=CIRCLE ( 'NONE', #80781, 2.000000000000000000 ) ;
#58295=CARTESIAN_POINT ( 'NONE',  ( -21.53943276465977519, -0.05219959533937600094, 43.75109039468568284 ) ) ;
#58296=CARTESIAN_POINT ( 'NONE',  ( 0.05219959533937995610, -21.53943276465977519, 35.00109039468568284 ) ) ;
#58297=CARTESIAN_POINT ( 'NONE',  ( -5.153800228976328057, -19.02544592524343514, 47.29057627198102409 ) ) ;
#58298=CARTESIAN_POINT ( 'NONE',  ( -15.80617190586768217, 15.72974639402176855, 23.12609039468567573 ) ) ;
#58300=CARTESIAN_POINT ( 'NONE',  ( 9.474510206698729675, 16.51473224551082808, 57.08442372801900433 ) ) ;
#58301=CARTESIAN_POINT ( 'NONE',  ( -13.89961937509977652, 13.97604488694528158, 30.62390960531435269 ) ) ;
#58302=CARTESIAN_POINT ( 'NONE',  ( -16.53943276465976808, -0.05219959533934237506, 33.75109039468568284 ) ) ;
#58303=CARTESIAN_POINT ( 'NONE',  ( 5.049401038298161559, -19.05341960407611168, 27.70724293864769550 ) ) ;
#58304=CARTESIAN_POINT ( 'NONE',  ( 16.55341960407618274, -4.379528057220086978, 71.04275706135234714 ) ) ;
#58305=CARTESIAN_POINT ( 'NONE',  ( 19.03943276465977164, -0.05219959533909143690, 33.74890960531435979 ) ) ;
#58306=CARTESIAN_POINT ( 'NONE',  ( 13.97604488694527802, 13.89961937509977652, 89.37390960531436690 ) ) ;
#58307=CARTESIAN_POINT ( 'NONE',  ( -19.02544592524342804, 5.153800228976336051, 31.04057627198102409 ) ) ;
#58308=CARTESIAN_POINT ( 'NONE',  ( 21.55341960407610458, 5.719274019375980345, 68.95724293864769550 ) ) ;
#58309=CARTESIAN_POINT ( 'NONE',  ( -4.379528057220086978, -16.55341960407618274, 44.79275706135234714 ) ) ;
#58310=CARTESIAN_POINT ( 'NONE',  ( 10.81492255796106328, -18.62759615963255655, 95.41775706135234714 ) ) ;
#58311=CARTESIAN_POINT ( 'NONE',  ( -5.049401038298153566, 19.05341960407611168, 40.20724293864768839 ) ) ;
#58312=CARTESIAN_POINT ( 'NONE',  ( -14.34966873604960291, -8.224510206698953496, 26.66557627198103475 ) ) ;
#58313=CARTESIAN_POINT ( 'NONE',  ( -16.52544592524342804, 4.483927247898546575, 71.04057627198103830 ) ) ;
#58314=CARTESIAN_POINT ( 'NONE',  ( -9.564922557960796823, -16.46253265017161027, 62.08224293864769550 ) ) ;
#58315=CARTESIAN_POINT ( 'NONE',  ( -15.80617190586768217, 15.72974639402176855, 103.1260903946856757 ) ) ;
#58316=CARTESIAN_POINT ( 'NONE',  ( -18.62759615963255300, -10.81492255796106328, 29.16775706135234003 ) ) ;
#58317=CARTESIAN_POINT ( 'NONE',  ( -16.51473224551069308, -9.474510206698971260, 81.66557627198103830 ) ) ;
#58318=CARTESIAN_POINT ( 'NONE',  ( 10.72451020669871369, 18.67979575497193778, 87.08442372801901854 ) ) ;
#58319=CARTESIAN_POINT ( 'NONE',  ( -16.52544592524335698, -4.483927247898792601, 58.95942372801902565 ) ) ;
#58320=CARTESIAN_POINT ( 'NONE',  ( -12.14591786802326823, 12.06949235617739902, 33.12609039468569705 ) ) ;
#58321=CARTESIAN_POINT ( 'NONE',  ( 8.314922557960818139, 14.29746914071049879, 89.58224293864768129 ) ) ;
#58322=CARTESIAN_POINT ( 'NONE',  ( 5.823673210054444382, -21.52544592524334988, 105.2094237280190328 ) ) ;
#58323=CARTESIAN_POINT ( 'NONE',  ( -14.29746914071049879, 8.314922557960819915, 35.83224293864768839 ) ) ;
#58324=CARTESIAN_POINT ( 'NONE',  ( -19.03943276465977164, 0.05219959533909376836, 31.24890960531435979 ) ) ;
#58325=CARTESIAN_POINT ( 'NONE',  ( 14.29746914071037800, 8.314922557961029526, 51.66775706135234714 ) ) ;
#58326=CARTESIAN_POINT ( 'NONE',  ( 16.53943276465976808, -0.05219959533910856209, 48.74890960531435979 ) ) ;
#58327=CARTESIAN_POINT ( 'NONE',  ( -16.55341960407617563, 4.379528057220093196, 98.54275706135234714 ) ) ;
#58328=CARTESIAN_POINT ( 'NONE',  ( -21.53943276465977519, 0.05219959533907696930, 21.24890960531436690 ) ) ;
#58329=CARTESIAN_POINT ( 'NONE',  ( -5.823673210054116645, -21.52544592524344225, 32.29057627198102409 ) ) ;
#58330=CARTESIAN_POINT ( 'NONE',  ( -0.05219959533937732626, 21.53943276465977519, 107.5010903946856899 ) ) ;
#58331=CARTESIAN_POINT ( 'NONE',  ( -8.224510206698948167, 14.34966873604960824, 90.41557627198103830 ) ) ;
#58332=CARTESIAN_POINT ( 'NONE',  ( -16.46253265017160317, 9.564922557960807481, 100.8322429386477097 ) ) ;
#58334=CARTESIAN_POINT ( 'NONE',  ( 4.483927247898790824, -16.52544592524335698, 35.20942372801901854 ) ) ;
#58335=CARTESIAN_POINT ( 'NONE',  ( -5.153800228976328057, -19.02544592524343514, 47.29057627198102409 ) ) ;
#58336=CARTESIAN_POINT ( 'NONE',  ( 8.224510206698742110, 14.34966873604972548, 47.08442372801901854 ) ) ;
#58337=CARTESIAN_POINT ( 'NONE',  ( -17.33731399503118453, -5.745198142927167240, 21.23700565386912231 ) ) ;
#58338=CARTESIAN_POINT ( 'NONE',  ( 13.89961937509957401, 13.97604488694547697, 46.87609039468565442 ) ) ;
#58339=CARTESIAN_POINT ( 'NONE',  ( -19.02544592524342804, 5.153800228976336051, 46.04057627198101699 ) ) ;
#58340=CARTESIAN_POINT ( 'NONE',  ( 12.06949235617739724, 12.14591786802326823, 86.87609039468568994 ) ) ;
#58341=CARTESIAN_POINT ( 'NONE',  ( -5.049401038297874678, -19.05341960407617918, 99.79275706135234714 ) ) ;
#58342=CARTESIAN_POINT ( 'NONE',  ( 19.02544592524334988, 5.153800228976608722, 26.45942372801899722 ) ) ;
#58343=CARTESIAN_POINT ( 'NONE',  ( -5.153800228976328057, -19.02544592524343514, 67.29057627198102409 ) ) ;
#58344=CARTESIAN_POINT ( 'NONE',  ( 8.224510206698953496, -14.34966873604960469, 92.91557627198103830 ) ) ;
#58345=CARTESIAN_POINT ( 'NONE',  ( 5.049401038297881783, 19.05341960407617563, 72.29275706135234714 ) ) ;
#58346=CARTESIAN_POINT ( 'NONE',  ( -21.53943276465977519, 0.05219959533907696930, 61.24890960531435979 ) ) ;
#58347=CARTESIAN_POINT ( 'NONE',  ( -5.153800228976607833, 19.02544592524334988, 42.70942372801901143 ) ) ;
#58348=CARTESIAN_POINT ( 'NONE',  ( 19.03943276465977164, -0.05219959533909143690, 103.7489096053143669 ) ) ;
#58349=CARTESIAN_POINT ( 'NONE',  ( -10.81492255796078084, -18.62759615963271287, 77.08224293864769550 ) ) ;
#58350=CARTESIAN_POINT ( 'NONE',  ( -17.31728774477271671, 6.344390552232383129, 85.81906651689314458 ) ) ;
#58352=CARTESIAN_POINT ( 'NONE',  ( 5.049401038297881783, 19.05341960407617563, 107.2927570613523187 ) ) ;
#58353=CARTESIAN_POINT ( 'NONE',  ( 17.58332526062525147, 7.635886036038630920, 96.57665040441536064 ) ) ;
#58354=CARTESIAN_POINT ( 'NONE',  ( 4.379528057220092307, 16.55341960407617563, 22.29275706135235069 ) ) ;
#58355=CARTESIAN_POINT ( 'NONE',  ( -5.153800228976328057, -19.02544592524343514, 42.29057627198101699 ) ) ;
#58356=CARTESIAN_POINT ( 'NONE',  ( 13.97604488694527802, 13.89961937509977652, 109.3739096053143669 ) ) ;
#58357=CARTESIAN_POINT ( 'NONE',  ( 18.67979575497178502, 10.72451020669898547, 89.16557627198102409 ) ) ;
#58358=CARTESIAN_POINT ( 'NONE',  ( 21.55341960407619695, -5.719274019375665929, 56.04275706135235424 ) ) ;
#58359=CARTESIAN_POINT ( 'NONE',  ( 19.05341960407617918, -5.049401038297876454, 106.0427570613523471 ) ) ;
#58360=CARTESIAN_POINT ( 'NONE',  ( 21.53943276465977519, 0.05219959533937863772, 111.2510903946856899 ) ) ;
#58361=CARTESIAN_POINT ( 'NONE',  ( -14.34966873604972548, 8.224510206698743886, 108.3344237280190185 ) ) ;
#58362=CARTESIAN_POINT ( 'NONE',  ( 5.823673210054125526, 21.52544592524343514, 94.79057627198105251 ) ) ;
#58363=CARTESIAN_POINT ( 'NONE',  ( 4.483927247898545687, 16.52544592524342804, 49.79057627198102409 ) ) ;
#58364=CARTESIAN_POINT ( 'NONE',  ( -19.03943276465977164, -0.05219959533935918106, 78.75109039468567573 ) ) ;
#58365=CARTESIAN_POINT ( 'NONE',  ( -13.97604488694547697, 13.89961937509957934, 53.12609039468565442 ) ) ;
#58366=CARTESIAN_POINT ( 'NONE',  ( 10.81492255796106328, -18.62759615963255655, 75.41775706135233293 ) ) ;
#58367=CARTESIAN_POINT ( 'NONE',  ( 13.89961937509957401, 13.97604488694547697, 36.87609039468565442 ) ) ;
#58368=CARTESIAN_POINT ( 'NONE',  ( -12.06949235617756955, 12.14591786802309770, 100.6239096053143811 ) ) ;
#58369=CARTESIAN_POINT ( 'NONE',  ( 10.81492255796078972, 18.62759615963270932, 39.58224293864769550 ) ) ;
#58370=CARTESIAN_POINT ( 'NONE',  ( 14.29746914071049879, -8.314922557960816363, 38.33224293864768839 ) ) ;
#58371=CARTESIAN_POINT ( 'NONE',  ( -16.51473224551082808, 9.474510206698731452, 23.33442372801900078 ) ) ;
#58372=CARTESIAN_POINT ( 'NONE',  ( -14.29746914071037622, -8.314922557961029526, 74.16775706135231871 ) ) ;
#58373=CARTESIAN_POINT ( 'NONE',  ( -16.53943276465976808, 0.05219959533911058130, 31.24890960531435979 ) ) ;
#58374=CARTESIAN_POINT ( 'NONE',  ( 10.72451020669871369, 18.67979575497193778, 62.08442372801901143 ) ) ;
#58375=CARTESIAN_POINT ( 'NONE',  ( -15.80617190586768217, 15.72974639402176855, 68.12609039468567573 ) ) ;
#58376=CARTESIAN_POINT ( 'NONE',  ( -0.05219959533907301413, -21.53943276465977519, 72.49890960531435269 ) ) ;
#58378=CARTESIAN_POINT ( 'NONE',  ( -5.049401038298153566, 19.05341960407611168, 30.20724293864768839 ) ) ;
#58379=CARTESIAN_POINT ( 'NONE',  ( 5.719274019375673035, 21.55341960407619339, 47.29275706135234003 ) ) ;
#58380=CARTESIAN_POINT ( 'NONE',  ( 12.14591786802309770, 12.06949235617756955, 114.3739096053143527 ) ) ;
#58381=CARTESIAN_POINT ( 'NONE',  ( 5.049401038298161559, -19.05341960407611168, 32.70724293864768129 ) ) ;
#58382=CARTESIAN_POINT ( 'NONE',  ( 16.55341960407611168, 4.379528057220329451, 73.95724293864769550 ) ) ;
#58383=CARTESIAN_POINT ( 'NONE',  ( -16.51473224551069308, -9.474510206698971260, 86.66557627198102409 ) ) ;
#58384=CARTESIAN_POINT ( 'NONE',  ( 16.55341960407611168, 4.379528057220329451, 28.95724293864769905 ) ) ;
#58385=CARTESIAN_POINT ( 'NONE',  ( 16.55341960407611168, 4.379528057220329451, 98.95724293864770971 ) ) ;
#58386=CARTESIAN_POINT ( 'NONE',  ( 5.719274019375991003, -21.55341960407610458, 72.70724293864769550 ) ) ;
#58387=CARTESIAN_POINT ( 'NONE',  ( -15.72974639402197994, 15.80617190586746368, 105.6239096053143669 ) ) ;
#58389=CARTESIAN_POINT ( 'NONE',  ( 5.153800228976335163, 19.02544592524342804, 64.79057627198100988 ) ) ;
#58390=CARTESIAN_POINT ( 'NONE',  ( -12.14591786802326823, 12.06949235617739902, 23.12609039468567573 ) ) ;
#58391=CARTESIAN_POINT ( 'NONE',  ( 5.823673210054125526, 21.52544592524343514, 54.79057627198104541 ) ) ;
#58392=CARTESIAN_POINT ( 'NONE',  ( -18.67979575497193778, 10.72451020669871902, 83.33442372801903275 ) ) ;
#58393=CARTESIAN_POINT ( 'NONE',  ( -16.51473224551069308, -9.474510206698971260, 86.66557627198102409 ) ) ;
#58394=EDGE_CURVE ( 'NONE', #166568, #29646, #51233, .T. ) ;
#58395=CARTESIAN_POINT ( 'NONE',  ( -5.049401038298153566, 19.05341960407611168, 110.2072429386476671 ) ) ;
#58396=CARTESIAN_POINT ( 'NONE',  ( 12.06949235617739724, 12.14591786802326823, 76.87609039468567573 ) ) ;
#58397=CARTESIAN_POINT ( 'NONE',  ( -21.52544592524334988, -5.823673210054445271, 58.95942372801902565 ) ) ;
#58398=CARTESIAN_POINT ( 'NONE',  ( 21.52544592524334988, 5.823673210054432836, 106.4594237280190328 ) ) ;
#58399=CARTESIAN_POINT ( 'NONE',  ( -14.29746914071037622, -8.314922557961029526, 64.16775706135234714 ) ) ;
#58400=CARTESIAN_POINT ( 'NONE',  ( -21.52544592524334988, -5.823673210054445271, 18.95942372801901143 ) ) ;
#58401=CARTESIAN_POINT ( 'NONE',  ( 13.97604488694527802, 13.89961937509977652, 24.37390960531435624 ) ) ;
#58402=CARTESIAN_POINT ( 'NONE',  ( 5.719274019375991003, -21.55341960407610458, 92.70724293864770971 ) ) ;
#58403=CARTESIAN_POINT ( 'NONE',  ( -5.153800228976607833, 19.02544592524334988, 47.70942372801900433 ) ) ;
#58404=CARTESIAN_POINT ( 'NONE',  ( 21.55341960407610458, 5.719274019375980345, 53.95724293864770260 ) ) ;
#58405=CARTESIAN_POINT ( 'NONE',  ( 13.89961937509977652, -13.97604488694527269, 98.12390960531433848 ) ) ;
#58406=CARTESIAN_POINT ( 'NONE',  ( -14.34966873604960291, -8.224510206698953496, 31.66557627198102054 ) ) ;
#58408=CARTESIAN_POINT ( 'NONE',  ( -18.22780087662124160, -5.499999999999927169, 78.98236817873106475 ) ) ;
#58409=CARTESIAN_POINT ( 'NONE',  ( -0.05219959533936034679, 19.03943276465977164, 112.5010903946856757 ) ) ;
#58410=CARTESIAN_POINT ( 'NONE',  ( 5.719274019375991003, -21.55341960407610458, 72.70724293864769550 ) ) ;
#58411=CARTESIAN_POINT ( 'NONE',  ( -0.05219959533910754901, -16.53943276465976808, 57.49890960531435979 ) ) ;
#58412=CARTESIAN_POINT ( 'NONE',  ( -16.53943276465976808, -0.05219959533934237506, 33.75109039468568284 ) ) ;
#58413=CARTESIAN_POINT ( 'NONE',  ( 13.89961937509977652, -13.97604488694527269, 48.12390960531435979 ) ) ;
#58414=CARTESIAN_POINT ( 'NONE',  ( 10.81492255796078972, 18.62759615963270932, 114.5822429386477097 ) ) ;
#58415=CARTESIAN_POINT ( 'NONE',  ( 19.05341960407617918, -5.049401038297876454, 81.04275706135231871 ) ) ;
#58416=CARTESIAN_POINT ( 'NONE',  ( 19.02544592524343514, -5.153800228976328945, 78.54057627198099567 ) ) ;
#58417=CARTESIAN_POINT ( 'NONE',  ( 16.51473224551069308, 9.474510206698969483, 69.16557627198102409 ) ) ;
#58418=CARTESIAN_POINT ( 'NONE',  ( 5.823673210054125526, 21.52544592524343514, 74.79057627198105251 ) ) ;
#58419=CARTESIAN_POINT ( 'NONE',  ( -0.05219959533909027116, -19.03943276465977164, 32.49890960531435979 ) ) ;
#58421=CARTESIAN_POINT ( 'NONE',  ( -14.34966873604960291, -8.224510206698953496, 56.66557627198103830 ) ) ;
#58422=CARTESIAN_POINT ( 'NONE',  ( -13.97604488694527625, -13.89961937509977652, 96.87390960531433848 ) ) ;
#58424=CARTESIAN_POINT ( 'NONE',  ( 16.51473224551083163, -9.474510206698727899, 50.83442372801899722 ) ) ;
#58425=CARTESIAN_POINT ( 'NONE',  ( 18.62759615963271287, -10.81492255796078972, 83.33224293864769550 ) ) ;
#58426=CARTESIAN_POINT ( 'NONE',  ( 16.51473224551083163, -9.474510206698727899, 30.83442372801900433 ) ) ;
#58427=CARTESIAN_POINT ( 'NONE',  ( -9.474510206698964154, 16.51473224551069663, 90.41557627198103830 ) ) ;
#58429=CARTESIAN_POINT ( 'NONE',  ( 18.67979575497178502, 10.72451020669898547, 29.16557627198103120 ) ) ;
#58430=CARTESIAN_POINT ( 'NONE',  ( 13.97604488694527802, 13.89961937509977652, 79.37390960531435269 ) ) ;
#58431=CARTESIAN_POINT ( 'NONE',  ( -5.823673210054431948, 21.52544592524334988, 47.70942372801902565 ) ) ;
#58432=CARTESIAN_POINT ( 'NONE',  ( 19.03943276465977164, -0.05219959533909143690, 23.74890960531435269 ) ) ;
#58433=CARTESIAN_POINT ( 'NONE',  ( -0.05219959533907301413, -21.53943276465977519, 112.4989096053143669 ) ) ;
#58435=CARTESIAN_POINT ( 'NONE',  ( -21.53943276465977519, -0.05219959533937600094, 38.75109039468567573 ) ) ;
#58437=CARTESIAN_POINT ( 'NONE',  ( 13.97604488694527802, 13.89961937509977652, 94.37390960531436690 ) ) ;
#58439=CARTESIAN_POINT ( 'NONE',  ( -15.80617190586745835, -15.72974639402198527, 101.8739096053143811 ) ) ;
#58440=CARTESIAN_POINT ( 'NONE',  ( -5.049401038298153566, 19.05341960407611168, 60.20724293864768129 ) ) ;
#58441=CARTESIAN_POINT ( 'NONE',  ( -19.03943276465977164, -0.05219959533935918106, 113.7510903946856757 ) ) ;
#58443=CARTESIAN_POINT ( 'NONE',  ( 5.823673210054444382, -21.52544592524334988, 100.2094237280190043 ) ) ;
#58444=CARTESIAN_POINT ( 'NONE',  ( -13.89961937509977652, 13.97604488694528158, 40.62390960531435979 ) ) ;
#58445=CARTESIAN_POINT ( 'NONE',  ( 5.823673210054444382, -21.52544592524334988, 95.20942372801903275 ) ) ;
#58446=CARTESIAN_POINT ( 'NONE',  ( 5.049401038298161559, -19.05341960407611168, 87.70724293864769550 ) ) ;
#58447=CARTESIAN_POINT ( 'NONE',  ( 5.823673210054444382, -21.52544592524334988, 60.20942372801902565 ) ) ;
#58449=CARTESIAN_POINT ( 'NONE',  ( 9.564922557960805705, 16.46253265017160317, 99.58224293864770971 ) ) ;
#58451=CARTESIAN_POINT ( 'NONE',  ( 12.06949235617739724, 12.14591786802326823, 51.87609039468568284 ) ) ;
#58452=CARTESIAN_POINT ( 'NONE',  ( -16.55341960407617563, 4.379528057220093196, 63.54275706135234003 ) ) ;
#58453=CARTESIAN_POINT ( 'NONE',  ( -18.62759615963255300, -10.81492255796106328, 64.16775706135234714 ) ) ;
#58454=CARTESIAN_POINT ( 'NONE',  ( 21.52544592524334988, 5.823673210054432836, 91.45942372801901854 ) ) ;
#58456=CARTESIAN_POINT ( 'NONE',  ( 12.06949235617739724, 12.14591786802326823, 26.87609039468567218 ) ) ;
#58457=CARTESIAN_POINT ( 'NONE',  ( 19.02544592524343514, -5.153800228976328945, 78.54057627198099567 ) ) ;
#58458=CARTESIAN_POINT ( 'NONE',  ( 5.049401038298161559, -19.05341960407611168, 97.70724293864766707 ) ) ;
#58460=FACE_OUTER_BOUND ( 'NONE', #186, .T. ) ;
#58461=CARTESIAN_POINT ( 'NONE',  ( -19.05341960407611168, -5.049401038298163336, 26.45724293864769550 ) ) ;
#58462=CARTESIAN_POINT ( 'NONE',  ( -5.719274019375978568, 21.55341960407610458, 25.20724293864769550 ) ) ;
#58463=CARTESIAN_POINT ( 'NONE',  ( -14.29746914071037622, -8.314922557961029526, 94.16775706135237556 ) ) ;
#58464=CARTESIAN_POINT ( 'NONE',  ( 4.379528057220339221, -16.55341960407611168, 77.70724293864770971 ) ) ;
#58465=CARTESIAN_POINT ( 'NONE',  ( 13.97604488694527802, 13.89961937509977652, 64.37390960531436690 ) ) ;
#58466=CARTESIAN_POINT ( 'NONE',  ( 18.62759615963255655, 10.81492255796105972, 91.66775706135234714 ) ) ;
#58468=CARTESIAN_POINT ( 'NONE',  ( 4.379528057220092307, 16.55341960407617563, 27.29275706135234358 ) ) ;
#58469=CARTESIAN_POINT ( 'NONE',  ( 12.06949235617757843, -12.14591786802309237, 73.12390960531436690 ) ) ;
#58470=CARTESIAN_POINT ( 'NONE',  ( 21.53943276465977519, 0.05219959533937863772, 36.25109039468567573 ) ) ;
#58471=CARTESIAN_POINT ( 'NONE',  ( 18.62759615963271287, -10.81492255796078972, 68.33224293864769550 ) ) ;
#58472=CARTESIAN_POINT ( 'NONE',  ( -16.51473224551082808, 9.474510206698731452, 43.33442372801900433 ) ) ;
#58474=CARTESIAN_POINT ( 'NONE',  ( 5.049401038298161559, -19.05341960407611168, 82.70724293864770971 ) ) ;
#58475=CARTESIAN_POINT ( 'NONE',  ( 0.05219959533910956823, 16.53943276465976808, 44.99890960531435979 ) ) ;
#58476=CARTESIAN_POINT ( 'NONE',  ( -16.52544592524342804, 4.483927247898546575, 36.04057627198102409 ) ) ;
#58477=CARTESIAN_POINT ( 'NONE',  ( 4.379528057220092307, 16.55341960407617563, 112.2927570613523471 ) ) ;
#58478=CARTESIAN_POINT ( 'NONE',  ( -9.474510206698720793, -16.51473224551083518, 64.58442372801900433 ) ) ;
#58479=CARTESIAN_POINT ( 'NONE',  ( 19.01529144963332030, 5.500000000000157208, 53.73431955728441523 ) ) ;
#58480=CARTESIAN_POINT ( 'NONE',  ( -5.823673210054116645, -21.52544592524344225, 22.29057627198102765 ) ) ;
#58482=CARTESIAN_POINT ( 'NONE',  ( -16.53943276465976808, 0.05219959533911058130, 86.24890960531436690 ) ) ;
#58483=CARTESIAN_POINT ( 'NONE',  ( -18.22780087662122028, 5.500000000000031086, 58.51540105326107977 ) ) ;
#58484=CARTESIAN_POINT ( 'NONE',  ( -9.474510206698964154, 16.51473224551069663, 35.41557627198102409 ) ) ;
#58485=CARTESIAN_POINT ( 'NONE',  ( -5.719274019375978568, 21.55341960407610458, 40.20724293864769550 ) ) ;
#58486=CARTESIAN_POINT ( 'NONE',  ( 10.72451020669898902, -18.67979575497178502, 62.91557627198102409 ) ) ;
#58487=CARTESIAN_POINT ( 'NONE',  ( -16.52544592524342804, 4.483927247898546575, 116.0405762719810383 ) ) ;
#58488=CARTESIAN_POINT ( 'NONE',  ( -4.379528057220086978, -16.55341960407618274, 64.79275706135234714 ) ) ;
#58489=CARTESIAN_POINT ( 'NONE',  ( 19.02544592524343514, -5.153800228976328945, 48.54057627198103120 ) ) ;
#58490=CARTESIAN_POINT ( 'NONE',  ( 15.72974639402176855, 15.80617190586768217, 51.87609039468568284 ) ) ;
#58491=ORIENTED_EDGE ( 'NONE', *, *, #100373, .F. ) ;
#58492=CARTESIAN_POINT ( 'NONE',  ( 12.14591786802309770, 12.06949235617756955, 99.37390960531436690 ) ) ;
#58493=CARTESIAN_POINT ( 'NONE',  ( 5.049401038297881783, 19.05341960407617563, 92.29275706135234714 ) ) ;
#58496=CARTESIAN_POINT ( 'NONE',  ( 5.719274019375991003, -21.55341960407610458, 27.70724293864769905 ) ) ;
#58497=CARTESIAN_POINT ( 'NONE',  ( 17.50000000000000000, -5.499999999999992895, 66.21769037696435589 ) ) ;
#58498=CARTESIAN_POINT ( 'NONE',  ( 0.05219959533937995610, -21.53943276465977519, 65.00109039468568994 ) ) ;
#58499=CARTESIAN_POINT ( 'NONE',  ( 0.05219959533934541429, -16.53943276465976808, 50.00109039468568994 ) ) ;
#58500=CARTESIAN_POINT ( 'NONE',  ( -8.314922557960811034, -14.29746914071050412, 42.08224293864769550 ) ) ;
#58501=CARTESIAN_POINT ( 'NONE',  ( -10.81492255796078084, -18.62759615963271287, 62.08224293864769550 ) ) ;
#58502=CARTESIAN_POINT ( 'NONE',  ( 21.52544592524344225, -5.823673210054117533, 63.54057627198103830 ) ) ;
#58504=CARTESIAN_POINT ( 'NONE',  ( -9.474510206698720793, -16.51473224551083518, 84.58442372801900433 ) ) ;
#58505=CARTESIAN_POINT ( 'NONE',  ( 5.153800228976335163, 19.02544592524342804, 114.7905762719810241 ) ) ;
#58506=CARTESIAN_POINT ( 'NONE',  ( 5.049401038298161559, -19.05341960407611168, 47.70724293864770260 ) ) ;
#58507=CARTESIAN_POINT ( 'NONE',  ( 16.51473224551069308, 9.474510206698969483, 24.16557627198102765 ) ) ;
#58509=CARTESIAN_POINT ( 'NONE',  ( 16.51473224551069308, 9.474510206698969483, 109.1655762719810383 ) ) ;
#58511=CARTESIAN_POINT ( 'NONE',  ( -4.483927247898782831, 16.52544592524335698, 72.70942372801901854 ) ) ;
#58512=CARTESIAN_POINT ( 'NONE',  ( 15.72974639402199770, -15.80617190586745480, 98.12390960531436690 ) ) ;
#58513=CARTESIAN_POINT ( 'NONE',  ( 0.05219959533909260263, 19.03943276465977164, 64.99890960531436690 ) ) ;
#58514=CARTESIAN_POINT ( 'NONE',  ( -5.823673210054431948, 21.52544592524334988, 37.70942372801900433 ) ) ;
#58515=CARTESIAN_POINT ( 'NONE',  ( 5.153800228976335163, 19.02544592524342804, 99.79057627198102409 ) ) ;
#58518=CARTESIAN_POINT ( 'NONE',  ( 15.80617190586769283, -15.72974639402175789, 35.62609039468568994 ) ) ;
#58519=CARTESIAN_POINT ( 'NONE',  ( -5.153800228976328057, -19.02544592524343514, 22.29057627198102765 ) ) ;
#58520=CARTESIAN_POINT ( 'NONE',  ( 19.05341960407617918, -5.049401038297876454, 91.04275706135234714 ) ) ;
#58521=CARTESIAN_POINT ( 'NONE',  ( 13.89961937509957401, 13.97604488694547697, 36.87609039468565442 ) ) ;
#58522=CARTESIAN_POINT ( 'NONE',  ( 18.62759615963271287, -10.81492255796078972, 98.33224293864769550 ) ) ;
#58523=CARTESIAN_POINT ( 'NONE',  ( 9.564922557961047289, -16.46253265017146816, 30.41775706135232937 ) ) ;
#58524=CARTESIAN_POINT ( 'NONE',  ( -0.05219959533936034679, 19.03943276465977164, 52.50109039468566863 ) ) ;
#58525=CARTESIAN_POINT ( 'NONE',  ( -14.34966873604972548, 8.224510206698743886, 88.33442372801901854 ) ) ;
#58528=CARTESIAN_POINT ( 'NONE',  ( -19.05341960407611168, -5.049401038298163336, 71.45724293864766707 ) ) ;
#58529=CARTESIAN_POINT ( 'NONE',  ( 21.53943276465977519, 0.05219959533937863772, 81.25109039468568994 ) ) ;
#58530=CARTESIAN_POINT ( 'NONE',  ( -18.67979575497193778, 10.72451020669871902, 98.33442372801901854 ) ) ;
#58532=CARTESIAN_POINT ( 'NONE',  ( -16.46253265017160317, 9.564922557960807481, 85.83224293864769550 ) ) ;
#58533=CARTESIAN_POINT ( 'NONE',  ( -10.81492255796105439, 18.62759615963255655, 67.91775706135234714 ) ) ;
#58534=CARTESIAN_POINT ( 'NONE',  ( 13.97604488694548053, -13.89961937509957401, 105.6260903946856757 ) ) ;
#58535=CARTESIAN_POINT ( 'NONE',  ( -16.51473224551069308, -9.474510206698971260, 66.66557627198102409 ) ) ;
#58536=CARTESIAN_POINT ( 'NONE',  ( 9.564922557960805705, 16.46253265017160317, 109.5822429386476955 ) ) ;
#58537=CARTESIAN_POINT ( 'NONE',  ( -5.049401038298153566, 19.05341960407611168, 80.20724293864769550 ) ) ;
#58538=CARTESIAN_POINT ( 'NONE',  ( 17.50000000000003553, -3.188534218036753742, 22.34212600958745298 ) ) ;
#58539=CARTESIAN_POINT ( 'NONE',  ( 9.474510206698971260, -16.51473224551069308, 62.91557627198102409 ) ) ;
#58540=CARTESIAN_POINT ( 'NONE',  ( 16.51473224551069308, 9.474510206698969483, 54.16557627198103120 ) ) ;
#58541=CARTESIAN_POINT ( 'NONE',  ( -21.52544592524334988, -5.823673210054445271, 18.95942372801901143 ) ) ;
#58542=CARTESIAN_POINT ( 'NONE',  ( 8.224510206698742110, 14.34966873604972548, 82.08442372801901854 ) ) ;
#58544=CARTESIAN_POINT ( 'NONE',  ( 9.564922557961047289, -16.46253265017146816, 50.41775706135233293 ) ) ;
#58545=CARTESIAN_POINT ( 'NONE',  ( 19.05341960407611168, 5.049401038298154454, 83.95724293864766707 ) ) ;
#58546=CARTESIAN_POINT ( 'NONE',  ( 4.379528057220339221, -16.55341960407611168, 77.70724293864770971 ) ) ;
#58547=CARTESIAN_POINT ( 'NONE',  ( 4.483927247898545687, 16.52544592524342804, 104.7905762719810241 ) ) ;
#58548=CARTESIAN_POINT ( 'NONE',  ( 18.62759615963271287, -10.81492255796078972, 23.33224293864769194 ) ) ;
#58549=CARTESIAN_POINT ( 'NONE',  ( 19.05341960407611168, 5.049401038298154454, 108.9572429386477097 ) ) ;
#58550=CARTESIAN_POINT ( 'NONE',  ( 8.314922557960818139, 14.29746914071049879, 84.58224293864769550 ) ) ;
#58552=CARTESIAN_POINT ( 'NONE',  ( -13.89961937509957401, -13.97604488694547875, 29.37609039468565797 ) ) ;
#58553=CARTESIAN_POINT ( 'NONE',  ( 0.05219959533934541429, -16.53943276465976808, 100.0010903946857042 ) ) ;
#58554=CARTESIAN_POINT ( 'NONE',  ( 13.89961937509977652, -13.97604488694527269, 83.12390960531436690 ) ) ;
#58555=CARTESIAN_POINT ( 'NONE',  ( -10.72451020669870658, -18.67979575497194134, 59.58442372801901854 ) ) ;
#58556=CARTESIAN_POINT ( 'NONE',  ( -18.62759615963270932, 10.81492255796079327, 45.83224293864769550 ) ) ;
#58557=CARTESIAN_POINT ( 'NONE',  ( -10.72451020669898014, 18.67979575497178502, 110.4155762719810383 ) ) ;
#58558=CARTESIAN_POINT ( 'NONE',  ( -21.53943276465977519, 0.05219959533907696930, 76.24890960531435269 ) ) ;
#58559=CARTESIAN_POINT ( 'NONE',  ( 12.14591786802309770, 12.06949235617756955, 94.37390960531436690 ) ) ;
#58560=CARTESIAN_POINT ( 'NONE',  ( 19.05341960407617918, -5.049401038297876454, 61.04275706135232582 ) ) ;
#58561=CARTESIAN_POINT ( 'NONE',  ( 16.51473224551069308, 9.474510206698969483, 29.16557627198103475 ) ) ;
#58562=CARTESIAN_POINT ( 'NONE',  ( 19.05341960407611168, 5.049401038298154454, 88.95724293864769550 ) ) ;
#58563=CARTESIAN_POINT ( 'NONE',  ( -5.153800228976328057, -19.02544592524343514, 77.29057627198099567 ) ) ;
#58564=CARTESIAN_POINT ( 'NONE',  ( 12.06949235617757843, -12.14591786802309237, 98.12390960531436690 ) ) ;
#58565=ORIENTED_EDGE ( 'NONE', *, *, #111802, .T. ) ;
#58566=CARTESIAN_POINT ( 'NONE',  ( 16.55341960407611168, 4.379528057220329451, 33.95724293864769550 ) ) ;
#58567=CARTESIAN_POINT ( 'NONE',  ( 0.05219959533934541429, -16.53943276465976808, 40.00109039468567573 ) ) ;
#58568=CARTESIAN_POINT ( 'NONE',  ( 18.62759615963255655, 10.81492255796105972, 101.6677570613523613 ) ) ;
#58569=CARTESIAN_POINT ( 'NONE',  ( -9.474510206698964154, 16.51473224551069663, 95.41557627198102409 ) ) ;
#58570=CARTESIAN_POINT ( 'NONE',  ( 18.67979575497194134, -10.72451020669871369, 30.83442372801902209 ) ) ;
#58571=CARTESIAN_POINT ( 'NONE',  ( -9.564922557960796823, -16.46253265017161027, 42.08224293864769550 ) ) ;
#58572=CARTESIAN_POINT ( 'NONE',  ( -4.379528057220086978, -16.55341960407618274, 39.79275706135235424 ) ) ;
#58573=CARTESIAN_POINT ( 'NONE',  ( -13.89961937509957401, -13.97604488694547875, 104.3760903946856757 ) ) ;
#58574=CARTESIAN_POINT ( 'NONE',  ( 19.02544592524343514, -5.153800228976328945, 33.54057627198102409 ) ) ;
#58575=CARTESIAN_POINT ( 'NONE',  ( 12.14591786802309770, 12.06949235617756955, 99.37390960531436690 ) ) ;
#58576=CARTESIAN_POINT ( 'NONE',  ( 21.52544592524344225, -5.823673210054117533, 103.5405762719810383 ) ) ;
#58577=CARTESIAN_POINT ( 'NONE',  ( 13.89961937509957401, 13.97604488694547697, 81.87609039468564731 ) ) ;
#58578=CARTESIAN_POINT ( 'NONE',  ( -19.05341960407611168, -5.049401038298163336, 86.45724293864769550 ) ) ;
#58579=CARTESIAN_POINT ( 'NONE',  ( -0.05219959533937732626, 21.53943276465977519, 27.50109039468567929 ) ) ;
#58581=CARTESIAN_POINT ( 'NONE',  ( 0.05219959533909260263, 19.03943276465977164, 94.99890960531436690 ) ) ;
#58583=CARTESIAN_POINT ( 'NONE',  ( 19.02544592524343514, -5.153800228976328945, 83.54057627198100988 ) ) ;
#58584=CARTESIAN_POINT ( 'NONE',  ( 21.53943276465977519, 0.05219959533937863772, 36.25109039468567573 ) ) ;
#58585=CARTESIAN_POINT ( 'NONE',  ( 0.05219959533910956823, 16.53943276465976808, 84.99890960531436690 ) ) ;
#58586=CARTESIAN_POINT ( 'NONE',  ( 0.05219959533909260263, 19.03943276465977164, 99.99890960531436690 ) ) ;
#58587=CARTESIAN_POINT ( 'NONE',  ( 19.05341960407617918, -5.049401038297876454, 31.04275706135232227 ) ) ;
#58588=CARTESIAN_POINT ( 'NONE',  ( 14.29746914071037800, 8.314922557961029526, 46.66775706135234714 ) ) ;
#58589=CARTESIAN_POINT ( 'NONE',  ( -0.05219959533937732626, 21.53943276465977519, 82.50109039468568994 ) ) ;
#58590=CARTESIAN_POINT ( 'NONE',  ( 0.05219959533934541429, -16.53943276465976808, 30.00109039468568284 ) ) ;
#58591=CARTESIAN_POINT ( 'NONE',  ( -13.89961937509977652, 13.97604488694528158, 65.62390960531436690 ) ) ;
#58592=CARTESIAN_POINT ( 'NONE',  ( -5.153800228976607833, 19.02544592524334988, 97.70942372801900433 ) ) ;
#58593=CARTESIAN_POINT ( 'NONE',  ( 14.29746914071037800, 8.314922557961029526, 66.66775706135234714 ) ) ;
#58594=CARTESIAN_POINT ( 'NONE',  ( -9.474510206698720793, -16.51473224551083518, 19.58442372801899722 ) ) ;
#58595=CARTESIAN_POINT ( 'NONE',  ( 5.153800228976615827, -19.02544592524334988, 75.20942372801896170 ) ) ;
#58596=CARTESIAN_POINT ( 'NONE',  ( 19.03943276465977164, -0.05219959533909143690, 58.74890960531435979 ) ) ;
#58597=CARTESIAN_POINT ( 'NONE',  ( -10.72451020669898014, 18.67979575497178502, 85.41557627198102409 ) ) ;
#58598=CARTESIAN_POINT ( 'NONE',  ( -14.29746914071049879, 8.314922557960819915, 70.83224293864770971 ) ) ;
#58599=CARTESIAN_POINT ( 'NONE',  ( -16.46253265017146816, -9.564922557961047289, 74.16775706135234714 ) ) ;
#58600=CARTESIAN_POINT ( 'NONE',  ( -19.35543954521081389, -5.499999999999485745, 69.58901960356449479 ) ) ;
#58601=CARTESIAN_POINT ( 'NONE',  ( 9.564922557961047289, -16.46253265017146816, 55.41775706135234003 ) ) ;
#58602=CARTESIAN_POINT ( 'NONE',  ( 16.52544592524335698, 4.483927247898782831, 111.4594237280190328 ) ) ;
#58603=CARTESIAN_POINT ( 'NONE',  ( -16.53943276465976808, 0.05219959533911058130, 76.24890960531435269 ) ) ;
#58604=CARTESIAN_POINT ( 'NONE',  ( 15.72974639402176855, 15.80617190586768217, 106.8760903946856899 ) ) ;
#58606=CARTESIAN_POINT ( 'NONE',  ( -5.719274019375978568, 21.55341960407610458, 105.2072429386477097 ) ) ;
#58607=CARTESIAN_POINT ( 'NONE',  ( -0.05219959533909027116, -19.03943276465977164, 102.4989096053143669 ) ) ;
#58608=CARTESIAN_POINT ( 'NONE',  ( -19.05341960407611168, -5.049401038298163336, 66.45724293864769550 ) ) ;
#58609=CARTESIAN_POINT ( 'NONE',  ( -5.719274019375665041, -21.55341960407619695, 79.79275706135236135 ) ) ;
#58610=CARTESIAN_POINT ( 'NONE',  ( -9.564922557960796823, -16.46253265017161027, 57.08224293864769550 ) ) ;
#58611=CARTESIAN_POINT ( 'NONE',  ( -13.89961937509977652, 13.97604488694528158, 40.62390960531435979 ) ) ;
#58612=CARTESIAN_POINT ( 'NONE',  ( 5.823673210054125526, 21.52544592524343514, 24.79057627198103120 ) ) ;
#58613=CARTESIAN_POINT ( 'NONE',  ( -4.379528057220328563, 16.55341960407611168, 70.20724293864769550 ) ) ;
#58614=CARTESIAN_POINT ( 'NONE',  ( -19.02544592524342804, 5.153800228976336051, 41.04057627198103120 ) ) ;
#58615=CARTESIAN_POINT ( 'NONE',  ( 16.52544592524342804, -4.483927247898539470, 98.54057627198105251 ) ) ;
#58616=CARTESIAN_POINT ( 'NONE',  ( -15.80617190586745835, -15.72974639402198527, 111.8739096053143669 ) ) ;
#58617=CARTESIAN_POINT ( 'NONE',  ( -5.719274019375665041, -21.55341960407619695, 49.79275706135234714 ) ) ;
#58618=CARTESIAN_POINT ( 'NONE',  ( 13.89961937509977652, -13.97604488694527269, 33.12390960531434558 ) ) ;
#58619=CARTESIAN_POINT ( 'NONE',  ( -16.53943276465976808, -0.05219959533934237506, 58.75109039468568994 ) ) ;
#58620=CARTESIAN_POINT ( 'NONE',  ( -18.67979575497178146, -10.72451020669898902, 96.66557627198102409 ) ) ;
#58621=CARTESIAN_POINT ( 'NONE',  ( 21.53943276465977519, -0.05219959533907433946, 93.74890960531436690 ) ) ;
#58622=CARTESIAN_POINT ( 'NONE',  ( 19.02544592524334988, 5.153800228976608722, 21.45942372801899012 ) ) ;
#58623=CARTESIAN_POINT ( 'NONE',  ( -16.46253265017160317, 9.564922557960807481, 45.83224293864769550 ) ) ;
#58625=CARTESIAN_POINT ( 'NONE',  ( -5.719274019375665041, -21.55341960407619695, 54.79275706135235424 ) ) ;
#58627=CARTESIAN_POINT ( 'NONE',  ( -18.67979575497178146, -10.72451020669898902, 51.66557627198102409 ) ) ;
#58628=CARTESIAN_POINT ( 'NONE',  ( 0.05219959533910956823, 16.53943276465976808, 29.99890960531435979 ) ) ;
#58629=CARTESIAN_POINT ( 'NONE',  ( 18.67979575497194134, -10.72451020669871369, 80.83442372801901854 ) ) ;
#58630=CARTESIAN_POINT ( 'NONE',  ( 19.05341960407617918, -5.049401038297876454, 21.04275706135232582 ) ) ;
#58631=CARTESIAN_POINT ( 'NONE',  ( -9.564922557961040184, 16.46253265017147172, 42.91775706135234003 ) ) ;
#58632=CARTESIAN_POINT ( 'NONE',  ( -8.224510206698735004, -14.34966873604973081, 104.5844237280190185 ) ) ;
#58633=CARTESIAN_POINT ( 'NONE',  ( 5.719274019375673035, 21.55341960407619339, 52.29275706135236135 ) ) ;
#58634=CARTESIAN_POINT ( 'NONE',  ( 16.46253265017160672, -9.564922557960803928, 63.33224293864769550 ) ) ;
#58635=CARTESIAN_POINT ( 'NONE',  ( -19.03943276465977164, -0.05219959533935918106, 38.75109039468566152 ) ) ;
#58636=CARTESIAN_POINT ( 'NONE',  ( 21.52544592524344225, -5.823673210054117533, 43.54057627198103830 ) ) ;
#58637=CARTESIAN_POINT ( 'NONE',  ( 15.72974639402176855, 15.80617190586768217, 31.87609039468567929 ) ) ;
#58638=CARTESIAN_POINT ( 'NONE',  ( -15.80617190586745835, -15.72974639402198527, 91.87390960531436690 ) ) ;
#58639=CARTESIAN_POINT ( 'NONE',  ( 5.049401038297881783, 19.05341960407617563, 82.29275706135229029 ) ) ;
#58640=CARTESIAN_POINT ( 'NONE',  ( -16.55341960407617563, 4.379528057220093196, 48.54275706135234714 ) ) ;
#58642=CARTESIAN_POINT ( 'NONE',  ( 21.53943276465977519, -0.05219959533907433946, 98.74890960531438111 ) ) ;
#58643=CARTESIAN_POINT ( 'NONE',  ( -0.05219959533934338120, 16.53943276465976808, 77.50109039468567573 ) ) ;
#58644=CARTESIAN_POINT ( 'NONE',  ( 4.379528057220339221, -16.55341960407611168, 72.70724293864769550 ) ) ;
#58646=CARTESIAN_POINT ( 'NONE',  ( -16.46253265017146816, -9.564922557961047289, 109.1677570613523471 ) ) ;
#58647=CARTESIAN_POINT ( 'NONE',  ( 10.81492255796078972, 18.62759615963270932, 29.58224293864769905 ) ) ;
#58649=CARTESIAN_POINT ( 'NONE',  ( -16.52544592524335698, -4.483927247898792601, 48.95942372801902565 ) ) ;
#58650=CARTESIAN_POINT ( 'NONE',  ( -5.823673210054431948, 21.52544592524334988, 32.70942372801900433 ) ) ;
#58651=CARTESIAN_POINT ( 'NONE',  ( 10.72451020669898902, -18.67979575497178502, 32.91557627198102409 ) ) ;
#58652=CARTESIAN_POINT ( 'NONE',  ( 16.55341960407618274, -4.379528057220086978, 76.04275706135237556 ) ) ;
#58653=CARTESIAN_POINT ( 'NONE',  ( -5.049401038298153566, 19.05341960407611168, 90.20724293864766707 ) ) ;
#58654=CARTESIAN_POINT ( 'NONE',  ( 15.72974639402176855, 15.80617190586768217, 51.87609039468568284 ) ) ;
#58655=CARTESIAN_POINT ( 'NONE',  ( -0.05219959533909027116, -19.03943276465977164, 32.49890960531435979 ) ) ;
#58656=CARTESIAN_POINT ( 'NONE',  ( -15.80617190586745835, -15.72974639402198527, 26.87390960531435979 ) ) ;
#58657=CARTESIAN_POINT ( 'NONE',  ( 5.049401038297881783, 19.05341960407617563, 37.29275706135232582 ) ) ;
#58658=CARTESIAN_POINT ( 'NONE',  ( 4.483927247898790824, -16.52544592524335698, 55.20942372801902565 ) ) ;
#58659=CARTESIAN_POINT ( 'NONE',  ( -21.55341960407610458, -5.719274019375992779, 21.45724293864769550 ) ) ;
#58660=CARTESIAN_POINT ( 'NONE',  ( 16.46253265017160672, -9.564922557960803928, 78.33224293864769550 ) ) ;
#58661=CARTESIAN_POINT ( 'NONE',  ( -4.483927247898782831, 16.52544592524335698, 97.70942372801904696 ) ) ;
#58663=CARTESIAN_POINT ( 'NONE',  ( -8.224510206698948167, 14.34966873604960824, 100.4155762719810241 ) ) ;
#58664=CARTESIAN_POINT ( 'NONE',  ( -15.72974639402197994, 15.80617190586746368, 40.62390960531435269 ) ) ;
#58665=CARTESIAN_POINT ( 'NONE',  ( 16.51473224551069308, 9.474510206698969483, 34.16557627198102409 ) ) ;
#58666=CARTESIAN_POINT ( 'NONE',  ( 14.29746914071037800, 8.314922557961029526, 71.66775706135234714 ) ) ;
#58667=CARTESIAN_POINT ( 'NONE',  ( 10.72451020669898902, -18.67979575497178502, 112.9155762719810383 ) ) ;
#58668=CARTESIAN_POINT ( 'NONE',  ( 9.564922557961047289, -16.46253265017146816, 70.41775706135233293 ) ) ;
#58669=CARTESIAN_POINT ( 'NONE',  ( 19.02544592524343514, -5.153800228976328945, 43.54057627198103120 ) ) ;
#58670=CARTESIAN_POINT ( 'NONE',  ( -5.719274019375978568, 21.55341960407610458, 75.20724293864769550 ) ) ;
#58672=CARTESIAN_POINT ( 'NONE',  ( -18.62759615963255300, -10.81492255796106328, 94.16775706135237556 ) ) ;
#58673=CARTESIAN_POINT ( 'NONE',  ( -19.02544592524342804, 5.153800228976336051, 71.04057627198099567 ) ) ;
#58674=CARTESIAN_POINT ( 'NONE',  ( -4.379528057220086978, -16.55341960407618274, 49.79275706135234714 ) ) ;
#58675=CARTESIAN_POINT ( 'NONE',  ( 18.67979575497194134, -10.72451020669871369, 80.83442372801901854 ) ) ;
#58676=CARTESIAN_POINT ( 'NONE',  ( -19.05341960407617563, 5.049401038297882671, 38.54275706135233293 ) ) ;
#58677=CARTESIAN_POINT ( 'NONE',  ( -13.89961937509957401, -13.97604488694547875, 59.37609039468566863 ) ) ;
#58679=CARTESIAN_POINT ( 'NONE',  ( -21.52544592524334988, -5.823673210054445271, 53.95942372801900433 ) ) ;
#58680=CARTESIAN_POINT ( 'NONE',  ( -9.474510206698964154, 16.51473224551069663, 55.41557627198103120 ) ) ;
#58681=CARTESIAN_POINT ( 'NONE',  ( -13.89961937509957401, -13.97604488694547875, 49.37609039468567573 ) ) ;
#58682=CARTESIAN_POINT ( 'NONE',  ( 16.51473224551069308, 9.474510206698969483, 99.16557627198102409 ) ) ;
#58683=CARTESIAN_POINT ( 'NONE',  ( 19.02544592524343514, -5.153800228976328945, 78.54057627198099567 ) ) ;
#58684=CARTESIAN_POINT ( 'NONE',  ( 8.224510206698953496, -14.34966873604960469, 37.91557627198102409 ) ) ;
#58685=CARTESIAN_POINT ( 'NONE',  ( -10.72451020669898014, 18.67979575497178502, 40.41557627198103120 ) ) ;
#58688=CARTESIAN_POINT ( 'NONE',  ( -10.81492255796105439, 18.62759615963255655, 92.91775706135236135 ) ) ;
#58690=CARTESIAN_POINT ( 'NONE',  ( 13.97604488694527802, 13.89961937509977652, 34.37390960531436690 ) ) ;
#58692=CARTESIAN_POINT ( 'NONE',  ( 16.52544592524335698, 4.483927247898782831, 56.45942372801902565 ) ) ;
#58693=CARTESIAN_POINT ( 'NONE',  ( 15.80617190586746368, 15.72974639402197994, 79.37390960531436690 ) ) ;
#58694=CARTESIAN_POINT ( 'NONE',  ( -4.379528057220328563, 16.55341960407611168, 35.20724293864768839 ) ) ;
#58695=CARTESIAN_POINT ( 'NONE',  ( -16.46253265017160317, 9.564922557960807481, 30.83224293864769550 ) ) ;
#58696=CARTESIAN_POINT ( 'NONE',  ( 19.05341960407611168, 5.049401038298154454, 108.9572429386477097 ) ) ;
#58697=CARTESIAN_POINT ( 'NONE',  ( -15.80617190586768217, 15.72974639402176855, 33.12609039468569705 ) ) ;
#58698=CARTESIAN_POINT ( 'NONE',  ( -19.02544592524334988, -5.153800228976617603, 33.95942372801897591 ) ) ;
#58699=CARTESIAN_POINT ( 'NONE',  ( 13.97604488694527802, 13.89961937509977652, 24.37390960531435624 ) ) ;
#58700=CARTESIAN_POINT ( 'NONE',  ( 21.55341960407619695, -5.719274019375665929, 86.04275706135236135 ) ) ;
#58701=CARTESIAN_POINT ( 'NONE',  ( 17.44279575226823908, -5.990770900252461395, 33.33557567514318976 ) ) ;
#58702=CARTESIAN_POINT ( 'NONE',  ( 16.53943276465976808, -0.05219959533910856209, 23.74890960531435269 ) ) ;
#58704=CARTESIAN_POINT ( 'NONE',  ( -0.05219959533907301413, -21.53943276465977519, 22.49890960531436335 ) ) ;
#58705=CARTESIAN_POINT ( 'NONE',  ( -16.52544592524342804, 4.483927247898546575, 96.04057627198102409 ) ) ;
#58707=CARTESIAN_POINT ( 'NONE',  ( 19.05341960407611168, 5.049401038298154454, 93.95724293864769550 ) ) ;
#58708=CARTESIAN_POINT ( 'NONE',  ( -14.34966873604960291, -8.224510206698953496, 76.66557627198103830 ) ) ;
#58709=CARTESIAN_POINT ( 'NONE',  ( 5.049401038297881783, 19.05341960407617563, 107.2927570613523187 ) ) ;
#58710=CARTESIAN_POINT ( 'NONE',  ( 15.72974639402199770, -15.80617190586745480, 68.12390960531436690 ) ) ;
#58713=CARTESIAN_POINT ( 'NONE',  ( -19.05341960407611168, -5.049401038298163336, 31.45724293864769550 ) ) ;
#58714=CARTESIAN_POINT ( 'NONE',  ( -9.474510206698964154, 16.51473224551069663, 85.41557627198102409 ) ) ;
#58715=CARTESIAN_POINT ( 'NONE',  ( -21.53943276465977519, 0.05219959533907696930, 76.24890960531435269 ) ) ;
#58716=CARTESIAN_POINT ( 'NONE',  ( -14.34966873604972548, 8.224510206698743886, 108.3344237280190185 ) ) ;
#58717=CARTESIAN_POINT ( 'NONE',  ( -13.89961937509977652, 13.97604488694528158, 85.62390960531433848 ) ) ;
#58718=CARTESIAN_POINT ( 'NONE',  ( 9.474510206698729675, 16.51473224551082808, 62.08442372801899722 ) ) ;
#58719=CARTESIAN_POINT ( 'NONE',  ( -21.52544592524334988, -5.823673210054445271, 98.95942372801903275 ) ) ;
#58720=CARTESIAN_POINT ( 'NONE',  ( -15.80617190586745835, -15.72974639402198527, 76.87390960531439532 ) ) ;
#58721=CARTESIAN_POINT ( 'NONE',  ( 21.53943276465977519, -0.05219959533907433946, 28.74890960531435624 ) ) ;
#58722=CARTESIAN_POINT ( 'NONE',  ( -19.05341960407611168, -5.049401038298163336, 51.45724293864770260 ) ) ;
#58723=CARTESIAN_POINT ( 'NONE',  ( -14.29746914071049879, 8.314922557960819915, 25.83224293864769194 ) ) ;
#58724=CARTESIAN_POINT ( 'NONE',  ( 16.46253265017160672, -9.564922557960803928, 58.33224293864769550 ) ) ;
#58726=CARTESIAN_POINT ( 'NONE',  ( 0.05219959533937995610, -21.53943276465977519, 105.0010903946856757 ) ) ;
#58727=CARTESIAN_POINT ( 'NONE',  ( -16.55341960407611168, -4.379528057220339221, 71.45724293864769550 ) ) ;
#58728=CARTESIAN_POINT ( 'NONE',  ( -21.52544592524343514, 5.823673210054127303, 111.0405762719810525 ) ) ;
#58729=CARTESIAN_POINT ( 'NONE',  ( 15.72974639402199770, -15.80617190586745480, 108.1239096053143811 ) ) ;
#58731=CARTESIAN_POINT ( 'NONE',  ( -10.81492255796078084, -18.62759615963271287, 62.08224293864769550 ) ) ;
#58732=CARTESIAN_POINT ( 'NONE',  ( 0.05219959533934541429, -16.53943276465976808, 80.00109039468568994 ) ) ;
#58733=CARTESIAN_POINT ( 'NONE',  ( 16.52544592524342804, -4.483927247898539470, 98.54057627198105251 ) ) ;
#58734=CARTESIAN_POINT ( 'NONE',  ( 16.51473224551069308, 9.474510206698969483, 54.16557627198103120 ) ) ;
#58735=CARTESIAN_POINT ( 'NONE',  ( 12.14591786802327356, -12.06949235617739191, 105.6260903946856899 ) ) ;
#58737=CARTESIAN_POINT ( 'NONE',  ( 18.62759615963255655, 10.81492255796105972, 46.66775706135234714 ) ) ;
#58738=CARTESIAN_POINT ( 'NONE',  ( 5.049401038298161559, -19.05341960407611168, 112.7072429386476813 ) ) ;
#58739=CARTESIAN_POINT ( 'NONE',  ( -10.72451020669870658, -18.67979575497194134, 84.58442372801903275 ) ) ;
#58740=CARTESIAN_POINT ( 'NONE',  ( 19.03943276465977164, -0.05219959533909143690, 33.74890960531435979 ) ) ;
#58741=CARTESIAN_POINT ( 'NONE',  ( 16.46253265017160672, -9.564922557960803928, 43.33224293864769550 ) ) ;
#58742=ORIENTED_EDGE ( 'NONE', *, *, #101761, .F. ) ;
#58743=CARTESIAN_POINT ( 'NONE',  ( 15.72974639402176855, 15.80617190586768217, 81.87609039468568994 ) ) ;
#58744=CARTESIAN_POINT ( 'NONE',  ( -15.80617190586768217, 15.72974639402176855, 68.12609039468567573 ) ) ;
#58745=CARTESIAN_POINT ( 'NONE',  ( -19.02544592524342804, 5.153800228976336051, 101.0405762719810241 ) ) ;
#58746=CARTESIAN_POINT ( 'NONE',  ( -19.05341960407617563, 5.049401038297882671, 83.54275706135233293 ) ) ;
#58747=CARTESIAN_POINT ( 'NONE',  ( -15.80617190586768217, 15.72974639402176855, 53.12609039468568284 ) ) ;
#58748=CARTESIAN_POINT ( 'NONE',  ( -14.34966873604972548, 8.224510206698743886, 28.33442372801902209 ) ) ;
#58749=CARTESIAN_POINT ( 'NONE',  ( 9.474510206698729675, 16.51473224551082808, 72.08442372801900433 ) ) ;
#58750=CARTESIAN_POINT ( 'NONE',  ( 13.89961937509977652, -13.97604488694527269, 58.12390960531436690 ) ) ;
#58751=CARTESIAN_POINT ( 'NONE',  ( 9.474510206698729675, 16.51473224551082808, 77.08442372801900433 ) ) ;
#58752=CARTESIAN_POINT ( 'NONE',  ( 14.29746914071037800, 8.314922557961029526, 111.6677570613523613 ) ) ;
#58753=CARTESIAN_POINT ( 'NONE',  ( -9.564922557961040184, 16.46253265017147172, 92.91775706135233293 ) ) ;
#58754=CARTESIAN_POINT ( 'NONE',  ( 16.53943276465976808, -0.05219959533910856209, 38.74890960531435979 ) ) ;
#58755=CARTESIAN_POINT ( 'NONE',  ( -19.03943276465977164, -0.05219959533935918106, 58.75109039468566863 ) ) ;
#58756=CARTESIAN_POINT ( 'NONE',  ( 8.314922557961029526, -14.29746914071037800, 50.41775706135235424 ) ) ;
#58757=CARTESIAN_POINT ( 'NONE',  ( -19.02544592524334988, -5.153800228976617603, 23.95942372801900078 ) ) ;
#58758=CARTESIAN_POINT ( 'NONE',  ( -19.02544592524342804, 5.153800228976336051, 36.04057627198100988 ) ) ;
#58759=CARTESIAN_POINT ( 'NONE',  ( -17.44270441346513323, -5.991230190323105553, 66.36335079264229364 ) ) ;
#58760=CARTESIAN_POINT ( 'NONE',  ( -8.224510206698735004, -14.34966873604973081, 39.58442372801901143 ) ) ;
#58764=CARTESIAN_POINT ( 'NONE',  ( -5.153800228976328057, -19.02544592524343514, 97.29057627198099567 ) ) ;
#58767=CARTESIAN_POINT ( 'NONE',  ( -16.51473224551082808, 9.474510206698731452, 103.3344237280190043 ) ) ;
#58768=CARTESIAN_POINT ( 'NONE',  ( -16.46253265017160317, 9.564922557960807481, 115.8322429386477097 ) ) ;
#58769=CARTESIAN_POINT ( 'NONE',  ( -21.52544592524334988, -5.823673210054445271, 108.9594237280190185 ) ) ;
#58770=CARTESIAN_POINT ( 'NONE',  ( -19.02544592524334988, -5.153800228976617603, 98.95942372801900433 ) ) ;
#58771=CARTESIAN_POINT ( 'NONE',  ( -16.52544592524342804, 4.483927247898546575, 116.0405762719810383 ) ) ;
#58772=CARTESIAN_POINT ( 'NONE',  ( 13.89961937509977652, -13.97604488694527269, 43.12390960531434558 ) ) ;
#58773=CARTESIAN_POINT ( 'NONE',  ( -10.72451020669898014, 18.67979575497178502, 60.41557627198102409 ) ) ;
#58774=CARTESIAN_POINT ( 'NONE',  ( -16.53943276465976808, 0.05219959533911058130, 116.2489096053143669 ) ) ;
#58775=CARTESIAN_POINT ( 'NONE',  ( 13.89961937509957579, 13.97604488694547520, 46.87609039468566152 ) ) ;
#58776=CARTESIAN_POINT ( 'NONE',  ( 19.05341960407617918, -5.049401038297876454, 76.04275706135230450 ) ) ;
#58777=CARTESIAN_POINT ( 'NONE',  ( 14.29746914071049879, -8.314922557960816363, 58.33224293864768839 ) ) ;
#58778=CARTESIAN_POINT ( 'NONE',  ( 21.55341960407610458, 5.719274019375980345, 38.95724293864768839 ) ) ;
#58779=CARTESIAN_POINT ( 'NONE',  ( 10.72451020669871369, 18.67979575497193778, 87.08442372801901854 ) ) ;
#58780=CARTESIAN_POINT ( 'NONE',  ( 0.05219959533907565091, 21.53943276465977519, 84.99890960531436690 ) ) ;
#58781=CARTESIAN_POINT ( 'NONE',  ( 10.81492255796106328, -18.62759615963255655, 55.41775706135234714 ) ) ;
#58782=CARTESIAN_POINT ( 'NONE',  ( -18.62759615963255300, -10.81492255796106328, 64.16775706135234714 ) ) ;
#58783=CARTESIAN_POINT ( 'NONE',  ( -5.153800228976328057, -19.02544592524343514, 102.2905762719810383 ) ) ;
#58784=CARTESIAN_POINT ( 'NONE',  ( 14.29746914071037800, 8.314922557961029526, 86.66775706135234714 ) ) ;
#58785=CARTESIAN_POINT ( 'NONE',  ( 5.719274019375673035, 21.55341960407619339, 62.29275706135236845 ) ) ;
#58786=CARTESIAN_POINT ( 'NONE',  ( -19.03943276465977164, 0.05219959533909376836, 51.24890960531436690 ) ) ;
#58787=( BOUNDED_SURFACE ( )  B_SPLINE_SURFACE ( 3, 2, ( 
 ( #172425, #170437, #171436, #158241, #48096, #81373, #95571, #143058, #47099, #51065, #110744, #32923, #189592, #174419, #82374, #157257, #185610, #97535, #2571, #159222, #18752, #20717, #144062, #123911, #5543, #108760, #31928, #93582, #1573, #124927, #186625, #109752, #64252, #94578, #80398, #142070, #156256, #17759, #125919, #3556, #37894, #7537, #23730, #39880, #38895, #36877, #54063, #69222, #98543, #192580, #131900, #162231, #129869, #83379, #161234, #71230, #87390, #191567, #117731, #102564, #163239, #148073, #21726, #9564, #179426, #193584, #160236, #116727, #99552, #52056, #100552, #149075, #25744, #85379, #194582, #53046, #55056, #115737, #145056, #175409, #132893, #40891, #22728, #147072, #114726, #70232, #164249, #130890, #67222, #178416, #8556, #101547, #177424, #24739, #128880, #84376, #86389, #56052, #190580, #113712, #176419, #6537, #68217, #146053, #73240, #182399, #61013, #44870, #76183, #134911, #196588, #169184, #168203, #104555, #30690, #27737, #153023, #107508, #137863, #59033, #57065, #12560, #58058, #150069, #13533, #120700, #152048, #75199, #11574, #151069, #195593, #43877, #92341, #10563, #28726, #199543, #119729, #198555, #197566, #165242, #118740, #14522, #184374, #181412, #105542, #42890, #136870, #72227, #74226, #122685, #60025, #167228, #121692, #135894, #183388, #133902, #166237, #90363, #106526, #29700, #45855, #89380, #91331, #180428, #41901, #103567, #26736, #88375, #188351, #19491, #16514, #78162, #112483, #111493, #47852, #174176, #171187, #96313, #50826, #81136, #2321, #329, #156007, #1319, #93333, #157007, #64003, #95322, #18505, #155018, #94329, #62998, #141824, #139830, #80153, #125673, #3317, #77179, #142817, #140832, #124676, #157999, #4297, #35646, #187371, #15522, #64990, #109505, #65979, #79161, #127648, #126648, #154027, #189348, #138849, #173178, #49829, #61997, #34654, #123663, #185360, #32676, #186373, #110494, #172176, #46851, #108511, #170190, #31684, #17504, #48840, #33661, #69987, #68976, #66978, #84130, #37639, #128638, #22482, #161987, #192335, #159987, #113468, #191322, #101301, #117484, #21474, #147837, #132656, #193337, #178175, #51809, #39640, #9323, #23483, #190332, #146816, #67973, #131655, #162990, #38652, #179182, #145809, #130641, #54811, #175163, #129627, #5295, #53816, #99303, #36629, #158979, #115491, #8311, #83135, #7292, #143813, #100309, #177179, #85132, #70988, #160988, #116486, #24495, #86146, #144811, #98286, #20471, #6294, #194344, #55812, #52800, #97293, #114467, #176169, #82121, #164009, #148832, #75948, #135658, #27497, #198307, #40650, #89139, #151808, #74964, #137622, #29467, #199306, #106283, #91100, #13299, #90124, #42651, #104313, #165996, #150827, #60773, #182152, #167968, #166987, #152788, #105300, #136626, #25505, #11327, #26495, #71978, #12324, #183146, #102319, #72998, #59786, #121454, #44631, #73989, #197330, #58793, #87149, #10322, #120461, #134666, #43637, #14279, #28490, #122445, #149821, #133652, #196352, #57820, #195343, #56823, #118497, #180188, #41658, #103321, #165001, #88137, #119492, #181174, #33432, #79926, #19265, #154780, #172948, #184137, #62757, #30449, #92096, #156780, #108273, #15279, #76939, #1082, #153784, #16277, #61760, #95091, #17269, #188122, #126424, #138608, #169951, #168942, #90, #32438, #110262, #78922, #125442, #186134, #48610, #80911, #77929, #2089, #141599, #47613, #49593, #46611, #140599, #170946, #65745, #31442, #155771, #34426, #18273, #111256, #93096, #139596, #142588, #3086, #124438, #4067, #109267, #96085, #45619, #157774, #94092, #123428, #63769, #187138, #185121, #171943, #64762, #107271, #160753, #143576, #21244, #190102, #83894, #66744, #145577, #129399, #99065, #50595, #100070, #6063, #51577, #176943, #23250, #69743, #191095, #189123, #22245, #36395, #161755, #67741, #84893, #7054, #127413, #131412, #112254, #38413, #53574, #173946, #68736, #130394, #158747 ),
 ( #192091, #146572, #8066, #128405, #98049, #20236, #81884, #175935, #193099, #35413, #115251, #97065, #5059, #113241, #174932, #52570, #159747, #114230, #82898, #144576, #37407, #169614, #126093, #157433, #32104, #156435, #154448, #110917, #187790, #49259, #81548, #48273, #18928, #94754, #188778, #93761, #47278, #31111, #155442, #172603, #64424, #63429, #4717, #170615, #108934, #34089, #17935, #95748, #80573, #16932, #109928, #78585, #142247, #140259, #3732, #79589, #65409, #92759, #35075, #141258, #1751, #50261, #158418, #66406, #2748, #15941, #127070, #125105, #96729, #33098, #19906, #111917, #107928, #143234, #77600, #173605, #128068, #189770, #139271, #747, #62419, #186803, #171610, #124091, #185790, #178595, #55233, #193765, #54239, #21904, #191745, #7715, #23908, #22904, #20897, #38072, #53228, #82555, #176598, #115910, #146228, #113888, #67399, #145233, #116902, #71407, #175586, #101735, #86566, #147248, #132076, #5721, #40058, #163423, #177600, #144237, #100725, #83554, #36063, #84550, #133071, #9743, #69400, #24921, #37062, #39068, #99728, #129055, #159402, #148249, #51243, #6715, #131067, #98721, #162406, #112903, #114904, #174597, #85562, #192756, #8739, #161412, #70408, #97711, #68393, #190756, #52231, #160415, #130045, #57247, #151247, #181587, #76368, #118921, #166423, #45051, #28903, #168383, #119902, #43065, #29878, #136068, #60203, #120877, #121873, #59208, #90543, #179604, #165423, #180606, #25921, #104731, #137046, #198738, #182577, #134084, #27918, #44060, #197742, #105720, #152225, #91516, #26917, #183566, #194761, #73419, #41076, #102740, #167407, #42079, #87565, #149252, #11752, #164428, #88559, #72407, #13710, #89561, #106709, #153202, #10743, #103743, #195774, #150258, #12736, #75376, #14707, #56233, #117915, #74402, #135090, #196766, #58234, #175775, #190939, #9927, #164606, #132260, #160599, #117085, #38257, #52416, #39250, #149428, #26100, #85749, #194944, #191931, #55414, #54422, #22089, #37249, #71586, #41259, #99911, #100906, #53415, #70592, #87743, #69588, #118100, #193951, #162590, #8924, #131255, #178780, #67585, #161596, #147436, #163604, #192943, #133252, #130235, #24095, #116092, #129243, #115092, #40248, #23090, #176784, #84735, #146413, #7904, #114074, #25105, #177780, #98906, #101922, #56420, #83739, #179790, #86749, #145418, #148432, #102921, #6900, #68579, #121064, #152402, #75556, #150440, #151427, #58411, #198916, #135271, #137232, #182758, #13889, #134271, #138230, #197922, #120078, #153395, #61376, #169559, #44242, #72597, #60385, #166602, #122057, #76554, #183749, #45235, #195958, #181766, #196943, #42262, #105899, #14893, #57431, #43247, #106889, #91701, #168562, #12914, #74578, #29080, #119104, #180785, #136246, #104915, #90719, #199912, #30060, #167585, #28102, #123047, #89741, #59390, #184733, #46218, #107871, #31056, #92704, #10924, #11936, #103922, #165602, #27101, #88747, #73599, #189716, #125050, #143181, #154392, #33045, #692, #62364, #127017, #78529, #185732, #47221, #171555, #124033, #186747, #32049, #65356, #187737, #158365, #96677, #108880, #140203, #139217, #170559, #2696, #188724, #19854, #95694, #174541, #141206, #49208, #111863, #93706, #48217, #109871, #1697, #157382, #173553, #15887, #172551, #3678, #63373, #64373, #155388, #18875, #34037, #80521, #128014, #94700, #50209, #126041, #35022, #156377, #16878, #77545, #17882, #142195, #110866, #79536, #51189, #81494, #4661, #66353, #112850, #36008, #133020, #192702, #84497, #55180, #97657, #146175, #8684, #132022, #194710, #86514, #56179, #163368, #148198, #131011, #178540, #101678, #71356, #22850, #7660, #117862, #39017, #24865, #69344, #40006, #159346, #68340, #193711, #9691, #147194, #99675, #161359, #115858, #20842, #67344, #54185, #129990, #177548, #179553, #100672, #162354, #6662, #82500, #191690, #53172, #70355, #116849, #144182, #5668, #129005, #23855, #37005, #85505 ),
 ( #190704, #52177, #114849, #113835, #176543, #175531, #98666, #160360, #21850, #83501, #145178, #38019, #25870, #87514, #89509, #75327, #45000, #182527, #61142, #27868, #74353, #198686, #134030, #11702, #196717, #26866, #44008, #60153, #102689, #59159, #90494, #165372, #151199, #149202, #105670, #120827, #167356, #14655, #181538, #152176, #12687, #121822, #88508, #180555, #164377, #150204, #28854, #197693, #58186, #137993, #103693, #73369, #13660, #10692, #72356, #76315, #136019, #136997, #183517, #41023, #106660, #168333, #29829, #199676, #91466, #122814, #153153, #195723, #57196, #118871, #42029, #135041, #166371, #119854, #43017, #104684, #49962, #110624, #111626, #48970, #18636, #169316, #155150, #170321, #15651, #81262, #46984, #31813, #33795, #107639, #92471, #19620, #79298, #171320, #141954, #184504, #32807, #95455, #80282, #142943, #173311, #4425, #34786, #96441, #17638, #65119, #188482, #158128, #109637, #94459, #66111, #125801, #45984, #172306, #30823, #157140, #3443, #154160, #16643, #93464, #77309, #156140, #126777, #138978, #78290, #456, #62131, #123795, #186510, #47984, #2455, #185493, #108643, #140967, #139964, #64137, #1453, #187503, #63131, #124810, #193467, #36760, #21607, #38783, #85264, #146955, #70116, #131787, #192464, #67110, #114604, #177311, #130772, #100440, #23617, #163123, #98423, #116616, #127777, #6422, #174306, #35775, #162120, #51940, #159108, #20602, #144940, #97422, #160120, #5426, #8443, #161117, #54944, #178305, #82254, #113600, #112614, #143945, #176301, #39768, #101432, #69106, #147965, #37773, #22614, #24626, #128768, #83266, #68103, #175294, #53947, #86274, #189477, #145941, #9452, #129755, #99436, #190467, #115623, #7422, #50955, #191452, #52929, #84259, #57952, #151938, #195478, #10452, #132783, #118628, #12458, #27632, #26624, #56954, #119623, #117618, #74118, #89273, #135789, #44760, #11461, #120594, #181306, #13427, #180319, #72112, #194470, #41787, #197460, #150963, #88267, #168095, #133786, #103454, #182289, #55942, #179316, #106414, #166130, #42784, #28618, #71117, #104447, #43769, #105433, #29593, #59915, #91224, #136758, #121583, #58926, #75091, #198443, #152915, #196482, #167118, #40780, #90255, #183278, #102449, #164137, #25634, #87278, #148963, #165132, #149955, #73132, #134801, #156909, #76075, #185255, #48738, #95223, #63901, #16409, #78056, #32570, #137751, #184267, #139724, #46748, #94223, #141725, #17400, #171079, #123560, #80055, #108407, #170083, #125571, #172074, #33561, #18406, #3215, #79057, #153917, #1213, #187269, #140730, #110392, #64889, #49724, #31575, #126550, #14411, #93226, #60903, #122578, #188250, #138740, #45749, #107401, #154911, #169074, #62891, #92232, #111392, #47746, #173077, #34554, #30580, #222, #199435, #15412, #124571, #96213, #77070, #155904, #61890, #186267, #109399, #2219, #50726, #128534, #113370, #143711, #163637, #118133, #19391, #178812, #9959, #133285, #132293, #127548, #144707, #98181, #189249, #83032, #25139, #55447, #20367, #174076, #51707, #164637, #180815, #82015, #10955, #195990, #56454, #65874, #81040, #102953, #57462, #86781, #112384, #71619, #190229, #142716, #193985, #42294, #119135, #40282, #87775, #5190, #148466, #6192, #35545, #97192, #26132, #134304, #175061, #117118, #66872, #194975, #157902, #159885, #72629, #179821, #101955, #41292, #21374, #149460, #4196, #36527, #158878, #67872, #105933, #107908, #166633, #60418, #90753, #185771, #28135, #183782, #74613, #89775, #151460, #12948, #136279, #62400, #61411, #197955, #124069, #121098, #46254, #728, #169594, #152436, #150471, #167618, #59424, #43278, #106922, #13922, #45268, #168595, #104947, #44275, #182792, #91734, #29114, #30095, #75589, #153430, #27131, #31092, #137268, #198951, #92740, #154428, #103954, #122091, #165633, #14928, #76588, #15922, #138264, #77580, #199947, #88778, #139252, #11966, #123082, #184768, #73631, #135301, #196974 ),
 ( #58441, #120109, #181799, #34071, #4697, #47258, #95729, #158399, #81529, #82537, #36044, #5703, #112885, #97693, #80554, #128050, #51224, #20879, #172584, #157415, #144219, #188758, #174579, #173587, #159384, #111899, #143216, #32085, #17916, #33079, #78566, #18909, #189752, #108915, #79571, #66388, #67380, #96711, #49241, #110899, #65391, #170595, #16913, #142229, #141240, #127052, #129038, #50243, #3714, #156414, #93742, #2729, #64406, #19888, #155423, #140239, #1732, #63410, #35056, #186783, #125085, #48253, #109907, #171591, #94735, #126075, #187771, #179587, #190739, #69379, #37043, #98703, #163405, #114886, #21886, #83536, #7697, #160397, #161394, #68375, #101714, #23890, #194744, #133054, #145215, #176580, #175567, #6697, #39049, #24901, #56216, #132058, #10726, #177582, #85542, #148232, #130027, #22886, #146209, #38054, #193747, #9726, #52213, #8721, #40041, #99710, #100707, #191726, #55215, #70390, #116884, #164411, #131049, #86548, #162387, #71390, #84532, #53208, #113870, #192739, #178576, #147229, #54221, #87548, #115892, #117897, #41059, #102722, #25903, #149235, #72390, #183547, #134065, #46014, #195756, #91497, #45033, #92503, #137028, #198718, #118904, #89543, #181570, #90525, #152207, #61174, #138026, #76349, #60185, #104714, #74384, #13691, #106691, #105702, #103726, #120859, #136049, #165406, #59190, #121855, #28885, #196749, #150239, #27900, #199709, #154192, #58216, #184534, #169347, #29860, #42062, #57230, #122846, #30856, #168364, #26899, #153184, #166404, #180588, #167389, #15682, #88542, #75358, #107670, #119885, #14687, #182559, #11735, #73402, #135073, #43048, #151229, #12718, #197724, #44042, #174334, #79328, #127804, #3472, #110656, #18665, #140998, #141984, #35804, #171350, #95485, #173342, #2486, #81290, #139995, #33825, #64167, #159136, #1484, #157171, #48014, #63162, #124841, #186541, #109670, #97450, #34814, #32839, #77343, #94489, #19649, #139009, #142974, #125832, #123826, #187535, #156171, #16673, #80311, #49000, #65149, #126806, #78322, #17670, #172336, #188514, #49991, #111656, #96469, #158157, #489, #4451, #66141, #189507, #50982, #112642, #62162, #185524, #47016, #108675, #170353, #31845, #93496, #155183, #162147, #100468, #36790, #86303, #117647, #147992, #69135, #67140, #22643, #68132, #160149, #23643, #130802, #85291, #146983, #21640, #161146, #129783, #8470, #144970, #70144, #192493, #131815, #143977, #9481, #7451, #191480, #163151, #71145, #179344, #53976, #82285, #193494, #176333, #132811, #145969, #194497, #54973, #20633, #55970, #5457, #178333, #116643, #40807, #39796, #101460, #128798, #37803, #52958, #177339, #38810, #102477, #24654, #190497, #51970, #114634, #84290, #113629, #175324, #115649, #98456, #83294, #6451, #99466, #89299, #28645, #58953, #26651, #180345, #57978, #168121, #184294, #88294, #14439, #199463, #59942, #72140, #87307, #106440, #60930, #90281, #56980, #13453, #134829, #148990, #135816, #45776, #122604, #182317, #91249, #149982, #151965, #150991, #118654, #133816, #29617, #137777, #196508, #197486, #11488, #167146, #164164, #166158, #76102, #75117, #120621, #105460, #27659, #136785, #25662, #119650, #43797, #121610, #12483, #152940, #73159, #198471, #74144, #10480, #181332, #183305, #42811, #104473, #44787, #103481, #195507, #41813, #165159, #31602, #33585, #17425, #48763, #30607, #34580, #94250, #16434, #49748, #157925, #65899, #79082, #169100, #110418, #62917, #96237, #32597, #19415, #156933, #107428, #81063, #92260, #64913, #18430, #127573, #172099, #95248, #153944, #124597, #154937, #63926, #125595, #142741, #111417, #173103, #80080, #78083, #47772, #187292, #141749, #140755, #77098, #155930, #109425, #138767, #2243, #3239, #126574, #170108, #123587, #1238, #4221, #189274, #93251, #15439, #248, #188275, #61917, #185281, #46773, #108432, #139751, #186292, #171104, #21401, #35569, #22407, #132580, #9245, #68902 ),
 ( #52727, #101223, #177104, #84058, #192259, #114392, #115415, #147759, #144733, #130561, #146736, #176094, #54734, #113396, #7217, #37564, #50750, #175086, #53741, #83059, #36554, #98208, #159912, #6220, #70912, #8232, #116406, #38575, #66898, #178095, #112408, #39565, #99227, #97217, #160914, #67899, #190256, #100231, #145736, #161913, #23407, #129552, #191252, #82041, #85055, #193260, #174100, #69910, #131576, #162912, #24420, #86069, #158903, #20394, #143738, #5217, #128561, #51733, #73915, #121382, #197257, #150755, #103246, #59709, #164928, #88061, #105230, #151738, #13231, #136557, #198238, #58719, #133576, #181102, #43565, #120388, #166918, #90056, #29396, #26421, #183074, #194268, #72924, #40575, #102245, #28419, #118421, #25430, #87071, #11250, #163933, #149748, #71904, #74894, #27418, #44557, #106212, #148756, #180114, #179106, #10245, #42576, #167896, #91026, #135585, #14203, #104239, #89064, #152712, #195266, #134593, #196279, #41582, #182082, #75871, #55735, #12253, #117409, #57748, #165922, #56750, #119418, #155699, #78848, #111180, #77857, #187066, #124362, #18198, #61687, #76865, #199230, #185049, #140526, #94018, #93021, #34351, #13, #46537, #48536, #60695, #45543, #172870, #32365, #186057, #95016, #137547, #47541, #110190, #171868, #96012, #126350, #157697, #3011, #188047, #170874, #79856, #141524, #19187, #62681, #109195, #122371, #2016, #184060, #63695, #107197, #168868, #33357, #30373, #125370, #138535, #139524, #108196, #156704, #123356, #64688, #17194, #49517, #92017, #153710, #15206, #169878, #31371, #154709, #16202, #1007, #142513, #22165, #36319, #7983, #5982, #69666, #130312, #80836, #193021, #3991, #38332, #192008, #39329, #83816, #145496, #65671, #97973, #128330, #37325, #98983, #131333, #84812, #23169, #6976, #51503, #21162, #160673, #53493, #52491, #50520, #67662, #82817, #112183, #129319, #68657, #175853, #143496, #96992, #174853, #146492, #100988, #4981, #54498, #116170, #176863, #189045, #127333, #177860, #162672, #115170, #173871, #99988, #113164, #35340, #114151, #158674, #20164, #161673, #81809, #66667, #190029, #191016, #159666, #144499, #166682, #198003, #195025, #196035, #10007, #27179, #121147, #26180, #74661, #150519, #57512, #165680, #87821, #88826, #182840, #118179, #42341, #120157, #149507, #28183, #86831, #180865, #11004, #105981, #148517, #104002, #56502, #71667, #133334, #179870, #41339, #44322, #181847, #89825, #12017, #40328, #151506, #24179, #12999, #72677, #70674, #134353, #103000, #163686, #73678, #119180, #135351, #58490, #9007, #164686, #197024, #55496, #43327, #136328, #85829, #104994, #59473, #147517, #132341, #194033, #117166, #178862, #102005, #25189, #95522, #138310, #50029, #97488, #173381, #126845, #76632, #35842, #199991, #61458, #81328, #127841, #189547, #112680, #174372, #34851, #106965, #157208, #19686, #96506, #143011, #66179, #5494, #123129, #159174, #167666, #49037, #13970, #75637, #4489, #91782, #198996, #60463, #184814, #137315, #110692, #45315, #51019, #3510, #20669, #82323, #122138, #153476, #152483, #183825, #18702, #144013, #67177, #111694, #190533, #80349, #65186, #128834, #168640, #172372, #33862, #14972, #158196, #52007, #29162, #188551, #90800, #142021, #30139, #160187, #116680, #131853, #55010, #87344, #54015, #163189, #100506, #194536, #37844, #52997, #175360, #161185, #178370, #70185, #69175, #10518, #176371, #22681, #24693, #36828, #21677, #149030, #8507, #162185, #71184, #113666, #23683, #86342, #148029, #72181, #102518, #133855, #179382, #164201, #147023, #56007, #117685, #195545, #38849, #85331, #98494, #39834, #83331, #101500, #145008, #6489, #9518, #68169, #25699, #129821, #40844, #191520, #193536, #114675, #99504, #84328, #132848, #146007, #7490, #130841, #192532, #115689, #177377, #118692, #91287, #41854, #27694, #42847, #88331, #167183, #199501, #180384, #89335, #152978, #137817, #106479, #58990, #120657 ),
 ( #103520, #198509, #12518, #184331, #182355, #45813, #168158, #57019, #169140, #165196, #14477, #29655, #15479, #59980, #121647, #26691, #74182, #104512, #13489, #75154, #107464, #60967, #122641, #183342, #151027, #197522, #136825, #76139, #28682, #150022, #43833, #105497, #11527, #90317, #44824, #152003, #119685, #73197, #135852, #30645, #77136, #181368, #92298, #153982, #138805, #134867, #196545, #58015, #166193, #64948, #93288, #49786, #171142, #185317, #172134, #82076, #158937, #18463, #127607, #124632, #188309, #187328, #154973, #108467, #142775, #174132, #32631, #33620, #186327, #3276, #97249, #2278, #50783, #126607, #95283, #141782, #63961, #111452, #20426, #94285, #80114, #96272, #125630, #4256, #35603, #156966, #48799, #157958, #286, #110453, #173138, #34613, #61955, #189306, #123622, #65935, #112443, #19449, #81097, #46808, #170144, #31639, #16469, #78118, #139787, #1275, #62952, #47809, #109459, #155963, #17460, #79117, #140789, #51764, #145766, #193292, #5250, #129584, #146770, #131607, #161944, #99258, #160945, #192292, #66931, #113425, #22438, #191280, #53771, #116440, #115445, #130595, #67930, #54766, #52755, #114424, #23439, #69943, #8264, #178129, #39596, #38607, #159943, #84087, #85086, #177136, #101255, #162944, #24451, #176126, #86100, #143769, #7248, #175117, #36585, #147791, #37596, #98240, #21430, #68933, #83090, #100263, #144766, #9277, #128594, #190288, #6251, #78774, #110119, #109122, #170800, #172796, #158600, #128254, #65598, #144422, #111107, #157622, #81734, #17122, #94945, #79779, #171797, #127258, #143420, #185982, #142440, #173797, #48462, #34277, #32292, #188971, #3918, #50447, #97897, #64616, #35263, #95936, #4907, #33285, #63620, #47465, #156629, #112106, #80762, #141451, #21085, #186992, #18124, #96918, #93948, #155626, #20090, #2936, #51426, #49444, #113086, #66590, #124285, #36244, #140450, #189952, #174778, #82742, #159588, #5908, #1940, #126278, #187975, #125296, #19112, #21672, #145003, #6484, #130836, #160182, #84323, #191515, #24688, #147018, #117680, #56002, #68164, #99499, #98489, #83326, #162180, #148024, #179377, #55005, #133850, #100501, #8503, #71179, #129816, #146002, #69169, #161180, #116675, #132843, #175355, #131848, #163184, #37839, #23678, #52992, #178365, #193531, #39829, #87339, #54010, #86337, #85326, #194531, #22676, #114670, #36823, #7485, #101495, #70180, #192527, #10513, #176366, #115684, #9513, #177372, #38844, #149025, #40839, #102512, #164196, #113661, #25694, #72176, #195540, #92294, #45809, #15475, #122637, #107460, #90313, #137813, #60963, #30641, #182351, #43829, #153978, #198505, #118687, #183338, #77132, #180379, #91283, #41849, #27691, #42844, #88327, #167179, #199497, #103516, #89332, #152974, #184327, #106475, #58986, #120653, #75150, #165192, #26687, #105493, #151024, #136821, #169136, #59976, #13485, #166190, #138801, #12515, #74179, #121643, #151999, #119682, #73193, #135849, #57014, #150018, #181365, #11523, #134864, #14473, #196542, #58012, #104509, #197518, #44820, #28678, #168154, #29651, #76135, #172130, #82072, #158933, #18459, #19445, #1271, #62948, #187324, #81093, #124628, #139783, #61951, #47805, #141778, #156962, #155959, #97245, #186323, #109455, #49782, #123618, #108463, #35599, #95279, #48795, #157954, #282, #110449, #111447, #34609, #20422, #189302, #185313, #65931, #50779, #33616, #142771, #4252, #174128, #125626, #80110, #46804, #3272, #170140, #126603, #31635, #93284, #96268, #154969, #171138, #32627, #16465, #64944, #127603, #78114, #94281, #112439, #17456, #173134, #2274, #63957, #188305, #79112, #140785, #68929, #114420, #23435, #70939, #146766, #100259, #52751, #9273, #176121, #37592, #54762, #101251, #162940, #86096, #147787, #8259, #83086, #130591, #193288, #69939, #116436, #39592, #179134, #99254, #132607, #143765, #22433, #85082, #25459, #192287, #51760, #175113, #36581, #160941 ),
 ( #24447, #67926, #144762, #5246, #191276, #131603, #161940, #84083, #40602, #6247, #145762, #178124, #66927, #113421, #102273, #38603, #53767, #194296, #128590, #115441, #55762, #117436, #163961, #190284, #98236, #159939, #21426, #177132, #129579, #7244, #60725, #12277, #73942, #122399, #28445, #148784, #13256, #184089, #10273, #121407, #71932, #57774, #72950, #118448, #197282, #29421, #133602, #119444, #183101, #167921, #136582, #89090, #150782, #105256, #195294, #56775, #135611, #181129, #166942, #14229, #90081, #43590, #196304, #152739, #42603, #104267, #198262, #44582, #106239, #91052, #75900, #151763, #26447, #58745, #59738, #74919, #137574, #199258, #45572, #165949, #107225, #87099, #27449, #168896, #180140, #120414, #41609, #103274, #164954, #182105, #88089, #149775, #11277, #134620, #63723, #34381, #172903, #185076, #16233, #15233, #76892, #78876, #64718, #96041, #171899, #53271, #17224, #125398, #188077, #123384, #1037, #186087, #77885, #33387, #49548, #92048, #48565, #79883, #154737, #140555, #138563, #95046, #110218, #141553, #111211, #62710, #2043, #139553, #156735, #130092, #32393, #80867, #18228, #187095, #3042, #94048, #126380, #191790, #124392, #157728, #19217, #155726, #142543, #93050, #6759, #68438, #114949, #47570, #30402, #109222, #170901, #153737, #41, #61716, #46565, #108226, #169906, #31399, #192800, #42125, #73462, #103787, #24964, #22948, #178638, #23951, #115955, #179650, #86610, #117959, #41120, #177644, #116945, #85606, #164470, #100768, #102784, #148293, #25964, #99772, #165467, #163467, #147292, #118966, #26963, #135136, #9787, #38118, #87607, #132117, #88606, #101779, #150302, #149293, #176642, #11798, #161457, #134129, #10787, #196810, #72454, #195818, #84594, #193810, #58277, #57290, #180650, #71449, #146274, #7761, #69444, #8782, #40101, #133114, #131112, #194802, #54283, #56276, #39112, #162450, #70452, #55275, #14756, #182624, #136114, #13757, #123896, #140066, #44109, #170421, #155252, #15750, #27964, #43111, #62228, #16741, #184601, #12782, #169418, #90591, #104779, #91566, #1557, #78390, #75425, #197790, #89605, #105767, #106756, #74448, #151294, #185595, #93566, #168431, #59256, #120925, #47084, #119946, #152273, #153254, #167454, #122913, #181631, #121922, #31913, #46082, #76417, #61241, #183616, #107737, #166467, #137099, #138093, #77409, #45099, #108745, #28950, #199774, #29927, #198785, #60251, #30923, #92571, #154259, #139079, #557, #187603, #21711, #20702, #128866, #143044, #79400, #190566, #160221, #52041, #111727, #109738, #65219, #110728, #2556, #66215, #173413, #4522, #127875, #64238, #3541, #172409, #51051, #49072, #189579, #34884, #112713, #186610, #113697, #50066, #33898, #5528, #175393, #83365, #96539, #124912, #174406, #18736, #36861, #188585, #98528, #35875, #63233, #145041, #48082, #82358, #97521, #171422, #159208, #144046, #32908, #80383, #94562, #67208, #156241, #158228, #17743, #141071, #125904, #95555, #126879, #19718, #157242, #81360, #142055, #193570, #147056, #37879, #131885, #71216, #101532, #69207, #22714, #100538, #10549, #26723, #130875, #57051, #41886, #102550, #114711, #129855, #149061, #103553, #132879, #99537, #56038, #177410, #191553, #178402, #88362, #165228, #162217, #84361, #176404, #192565, #161219, #55042, #8540, #146039, #116712, #194568, #163224, #54048, #7523, #23716, #72213, #6523, #115722, #118726, #68202, #164234, #38881, #53030, #133887, #85364, #117716, #70218, #179412, #39866, #24725, #86374, #148059, #9550, #40877, #25730, #87376, #195578, #180414, #104542, #58045, #92328, #123650, #120687, #121679, #135881, #153009, #46838, #152034, #316, #76170, #183375, #91318, #13519, #14508, #108498, #43864, #168189, #45842, #75184, #154014, #12547, #106512, #136856, #31670, #74213, #29686, #182386, #197552, #59020, #105529, #167215, #170177, #107494, #15509, #137850, #166223, #77166, #150055, #138836, #198541, #196575 ) ),
 .UNSPECIFIED., .T., .F., .F. ) 
 B_SPLINE_SURFACE_WITH_KNOTS ( ( 4, 3, 4 ),
 ( 3, 2, 2, 2, 2, 2, 2, 2, 2, 2, 2, 2, 2, 2, 2, 2, 2, 2, 2, 2, 2, 2, 2, 2, 2, 2, 2, 2, 2, 2, 2, 2, 2, 2, 2, 2, 2, 2, 2, 2, 2, 2, 2, 2, 2, 2, 2, 2, 2, 2, 2, 2, 2, 2, 2, 2, 2, 2, 2, 2, 2, 2, 2, 2, 2, 2, 2, 2, 2, 2, 2, 2, 2, 2, 2, 2, 2, 2, 2, 2, 2, 2, 2, 2, 2, 2, 2, 2, 2, 2, 2, 2, 2, 2, 2, 2, 2, 2, 2, 2, 2, 2, 2, 2, 2, 2, 2, 2, 2, 2, 2, 2, 2, 2, 2, 2, 2, 2, 2, 2, 2, 2, 2, 2, 2, 2, 2, 2, 2, 2, 2, 2, 2, 2, 2, 2, 2, 2, 2, 2, 2, 2, 2, 2, 2, 2, 2, 2, 2, 2, 2, 2, 2, 2, 2, 2, 2, 2, 2, 2, 2, 2, 2, 2, 2, 2, 2, 2, 2, 2, 2, 2, 2, 2, 2, 2, 2, 2, 2, 2, 2, 2, 2, 2, 2, 2, 2, 2, 2, 2, 2, 2, 2, 2, 2, 2, 2, 2, 2, 2, 2, 2, 2, 2, 2, 2, 2, 2, 2, 2, 2, 2, 2, 2, 2, 2, 2, 2, 2, 2, 2, 2, 2, 2, 2, 2, 2, 2, 3 ),
 ( 0.000000000000000000, 0.5000000000000000000, 1.000000000000000000 ),
 ( 0.000000000000000000, 0.004385964912280701511, 0.008771929824561403022, 0.01315789473684210453, 0.01754385964912280604, 0.02192982456140350755, 0.02631578947368420907, 0.03070175438596491058, 0.03508771929824561209, 0.03947368421052631360, 0.04385964912280701511, 0.04824561403508771662, 0.05263157894736841813, 0.05701754385964911964, 0.06140350877192982115, 0.06578947368421052266, 0.07017543859649122417, 0.07456140350877192569, 0.07894736842105262720, 0.08333333333333332871, 0.08771929824561403022, 0.09210526315789473173, 0.09649122807017543324, 0.1008771929824561348, 0.1052631578947368363, 0.1096491228070175378, 0.1140350877192982393, 0.1184210526315789408, 0.1228070175438596423, 0.1271929824561403577, 0.1315789473684210453, 0.1359649122807017607, 0.1403508771929824483, 0.1447368421052631637, 0.1491228070175438514, 0.1535087719298245668, 0.1578947368421052544, 0.1622807017543859698, 0.1666666666666666574, 0.1710526315789473728, 0.1754385964912280604, 0.1798245614035087758, 0.1842105263157894635, 0.1885964912280701788, 0.1929824561403508665, 0.1973684210526315819, 0.2017543859649122695, 0.2061403508771929849, 0.2105263157894736725, 0.2149122807017543879, 0.2192982456140350755, 0.2236842105263157909, 0.2280701754385964786, 0.2324561403508771940, 0.2368421052631578816, 0.2412280701754385970, 0.2456140350877192846, 0.2500000000000000000, 0.2543859649122807154, 0.2587719298245614308, 0.2631578947368420907, 0.2675438596491228060, 0.2719298245614035214, 0.2763157894736842368, 0.2807017543859648967, 0.2850877192982456121, 0.2894736842105263275, 0.2938596491228070429, 0.2982456140350877027, 0.3026315789473684181, 0.3070175438596491335, 0.3114035087719298489, 0.3157894736842105088, 0.3201754385964912242, 0.3245614035087719396, 0.3289473684210526550, 0.3333333333333333148, 0.3377192982456140302, 0.3421052631578947456, 0.3464912280701754610, 0.3508771929824561209, 0.3552631578947368363, 0.3596491228070175517, 0.3640350877192982670, 0.3684210526315789269, 0.3728070175438596423, 0.3771929824561403577, 0.3815789473684210731, 0.3859649122807017330, 0.3903508771929824483, 0.3947368421052631637, 0.3991228070175438791, 0.4035087719298245390, 0.4078947368421052544, 0.4122807017543859698, 0.4166666666666666852, 0.4210526315789473450, 0.4254385964912280604, 0.4298245614035087758, 0.4342105263157894912, 0.4385964912280701511, 0.4429824561403508665, 0.4473684210526315819, 0.4517543859649122973, 0.4561403508771929571, 0.4605263157894736725, 0.4649122807017543879, 0.4692982456140351033, 0.4736842105263157632, 0.4780701754385964786, 0.4824561403508771940, 0.4868421052631579093, 0.4912280701754385692, 0.4956140350877192846, 0.5000000000000000000, 0.5043859649122807154, 0.5087719298245614308, 0.5131578947368421462, 0.5175438596491228616, 0.5219298245614034659, 0.5263157894736841813, 0.5307017543859648967, 0.5350877192982456121, 0.5394736842105263275, 0.5438596491228070429, 0.5482456140350877583, 0.5526315789473684736, 0.5570175438596490780, 0.5614035087719297934, 0.5657894736842105088, 0.5701754385964912242, 0.5745614035087719396, 0.5789473684210526550, 0.5833333333333333703, 0.5877192982456140857, 0.5921052631578946901, 0.5964912280701754055, 0.6008771929824561209, 0.6052631578947368363, 0.6096491228070175517, 0.6140350877192982670, 0.6184210526315789824, 0.6228070175438596978, 0.6271929824561403022, 0.6315789473684210176, 0.6359649122807017330, 0.6403508771929824483, 0.6447368421052631637, 0.6491228070175438791, 0.6535087719298245945, 0.6578947368421053099, 0.6622807017543859143, 0.6666666666666666297, 0.6710526315789473450, 0.6754385964912280604, 0.6798245614035087758, 0.6842105263157894912, 0.6885964912280702066, 0.6929824561403509220, 0.6973684210526315264, 0.7017543859649122417, 0.7061403508771929571, 0.7105263157894736725, 0.7149122807017543879, 0.7192982456140351033, 0.7236842105263158187, 0.7280701754385965341, 0.7324561403508771384, 0.7368421052631578538, 0.7412280701754385692, 0.7456140350877192846, 0.7500000000000000000, 0.7543859649122807154, 0.7587719298245614308, 0.7631578947368421462, 0.7675438596491228616, 0.7719298245614034659, 0.7763157894736841813, 0.7807017543859648967, 0.7850877192982456121, 0.7894736842105263275, 0.7938596491228070429, 0.7982456140350877583, 0.8026315789473684736, 0.8070175438596490780, 0.8114035087719297934, 0.8157894736842105088, 0.8201754385964912242, 0.8245614035087719396, 0.8289473684210526550, 0.8333333333333333703, 0.8377192982456140857, 0.8421052631578946901, 0.8464912280701754055, 0.8508771929824561209, 0.8552631578947368363, 0.8596491228070175517, 0.8640350877192982670, 0.8684210526315789824, 0.8728070175438596978, 0.8771929824561403022, 0.8815789473684210176, 0.8859649122807017330, 0.8903508771929824483, 0.8947368421052631637, 0.8991228070175438791, 0.9035087719298245945, 0.9078947368421053099, 0.9122807017543859143, 0.9166666666666666297, 0.9210526315789473450, 0.9254385964912280604, 0.9298245614035087758, 0.9342105263157894912, 0.9385964912280702066, 0.9429824561403509220, 0.9473684210526315264, 0.9517543859649122417, 0.9561403508771929571, 0.9605263157894736725, 0.9649122807017543879, 0.9692982456140351033, 0.9736842105263158187, 0.9780701754385965341, 0.9824561403508771384, 0.9868421052631578538, 0.9912280701754385692, 0.9956140350877192846, 1.000000000000000000 ),
 .UNSPECIFIED. ) 
 GEOMETRIC_REPRESENTATION_ITEM ( )  RATIONAL_B_SPLINE_SURFACE ( (
 ( 1.000000000000000000, 0.9659258262890683122, 1.000000000000000000, 0.9659258262890683122, 1.000000000000000000, 0.9659258262890683122, 1.000000000000000000, 0.9659258262890683122, 1.000000000000000000, 0.9659258262890683122, 1.000000000000000000, 0.9659258262890683122, 1.000000000000000000, 0.9659258262890683122, 1.000000000000000000, 0.9659258262890683122, 1.000000000000000000, 0.9659258262890683122, 1.000000000000000000, 0.9659258262890683122, 1.000000000000000000, 0.9659258262890683122, 1.000000000000000000, 0.9659258262890683122, 1.000000000000000000, 0.9659258262890683122, 1.000000000000000000, 0.9659258262890683122, 1.000000000000000000, 0.9659258262890683122, 1.000000000000000000, 0.9659258262890683122, 1.000000000000000000, 0.9659258262890683122, 1.000000000000000000, 0.9659258262890683122, 1.000000000000000000, 0.9659258262890683122, 1.000000000000000000, 0.9659258262890683122, 1.000000000000000000, 0.9659258262890683122, 1.000000000000000000, 0.9659258262890683122, 1.000000000000000000, 0.9659258262890683122, 1.000000000000000000, 0.9659258262890683122, 1.000000000000000000, 0.9659258262890683122, 1.000000000000000000, 0.9659258262890683122, 1.000000000000000000, 0.9659258262890683122, 1.000000000000000000, 0.9659258262890683122, 1.000000000000000000, 0.9659258262890683122, 1.000000000000000000, 0.9659258262890683122, 1.000000000000000000, 0.9659258262890683122, 1.000000000000000000, 0.9659258262890683122, 1.000000000000000000, 0.9659258262890683122, 1.000000000000000000, 0.9659258262890683122, 1.000000000000000000, 0.9659258262890683122, 1.000000000000000000, 0.9659258262890683122, 1.000000000000000000, 0.9659258262890683122, 1.000000000000000000, 0.9659258262890683122, 1.000000000000000000, 0.9659258262890683122, 1.000000000000000000, 0.9659258262890683122, 1.000000000000000000, 0.9659258262890683122, 1.000000000000000000, 0.9659258262890683122, 1.000000000000000000, 0.9659258262890683122, 1.000000000000000000, 0.9659258262890683122, 1.000000000000000000, 0.9659258262890683122, 1.000000000000000000, 0.9659258262890683122, 1.000000000000000000, 0.9659258262890683122, 1.000000000000000000, 0.9659258262890683122, 1.000000000000000000, 0.9659258262890683122, 1.000000000000000000, 0.9659258262890683122, 1.000000000000000000, 0.9659258262890683122, 1.000000000000000000, 0.9659258262890683122, 1.000000000000000000, 0.9659258262890683122, 1.000000000000000000, 0.9659258262890683122, 1.000000000000000000, 0.9659258262890683122, 1.000000000000000000, 0.9659258262890683122, 1.000000000000000000, 0.9659258262890683122, 1.000000000000000000, 0.9659258262890683122, 1.000000000000000000, 0.9659258262890683122, 1.000000000000000000, 0.9659258262890683122, 1.000000000000000000, 0.9659258262890683122, 1.000000000000000000, 0.9659258262890683122, 1.000000000000000000, 0.9659258262890683122, 1.000000000000000000, 0.9659258262890683122, 1.000000000000000000, 0.9659258262890683122, 1.000000000000000000, 0.9659258262890683122, 1.000000000000000000, 0.9659258262890683122, 1.000000000000000000, 0.9659258262890683122, 1.000000000000000000, 0.9659258262890683122, 1.000000000000000000, 0.9659258262890683122, 1.000000000000000000, 0.9659258262890683122, 1.000000000000000000, 0.9659258262890683122, 1.000000000000000000, 0.9659258262890683122, 1.000000000000000000, 0.9659258262890683122, 1.000000000000000000, 0.9659258262890683122, 1.000000000000000000, 0.9659258262890683122, 1.000000000000000000, 0.9659258262890683122, 1.000000000000000000, 0.9659258262890683122, 1.000000000000000000, 0.9659258262890683122, 1.000000000000000000, 0.9659258262890683122, 1.000000000000000000, 0.9659258262890683122, 1.000000000000000000, 0.9659258262890683122, 1.000000000000000000, 0.9659258262890683122, 1.000000000000000000, 0.9659258262890683122, 1.000000000000000000, 0.9659258262890683122, 1.000000000000000000, 0.9659258262890683122, 1.000000000000000000, 0.9659258262890683122, 1.000000000000000000, 0.9659258262890683122, 1.000000000000000000, 0.9659258262890683122, 1.000000000000000000, 0.9659258262890683122, 1.000000000000000000, 0.9659258262890683122, 1.000000000000000000, 0.9659258262890683122, 1.000000000000000000, 0.9659258262890683122, 1.000000000000000000, 0.9659258262890683122, 1.000000000000000000, 0.9659258262890683122, 1.000000000000000000, 0.9659258262890683122, 1.000000000000000000, 0.9659258262890683122, 1.000000000000000000, 0.9659258262890683122, 1.000000000000000000, 0.9659258262890683122, 1.000000000000000000, 0.9659258262890683122, 1.000000000000000000, 0.9659258262890683122, 1.000000000000000000, 0.9659258262890683122, 1.000000000000000000, 0.9659258262890683122, 1.000000000000000000, 0.9659258262890683122, 1.000000000000000000, 0.9659258262890683122, 1.000000000000000000, 0.9659258262890683122, 1.000000000000000000, 0.9659258262890683122, 1.000000000000000000, 0.9659258262890683122, 1.000000000000000000, 0.9659258262890683122, 1.000000000000000000, 0.9659258262890683122, 1.000000000000000000, 0.9659258262890683122, 1.000000000000000000, 0.9659258262890683122, 1.000000000000000000, 0.9659258262890683122, 1.000000000000000000, 0.9659258262890683122, 1.000000000000000000, 0.9659258262890683122, 1.000000000000000000, 0.9659258262890683122, 1.000000000000000000, 0.9659258262890683122, 1.000000000000000000, 0.9659258262890683122, 1.000000000000000000, 0.9659258262890683122, 1.000000000000000000, 0.9659258262890683122, 1.000000000000000000, 0.9659258262890683122, 1.000000000000000000, 0.9659258262890683122, 1.000000000000000000, 0.9659258262890683122, 1.000000000000000000, 0.9659258262890683122, 1.000000000000000000, 0.9659258262890683122, 1.000000000000000000, 0.9659258262890683122, 1.000000000000000000, 0.9659258262890683122, 1.000000000000000000, 0.9659258262890683122, 1.000000000000000000, 0.9659258262890683122, 1.000000000000000000, 0.9659258262890683122, 1.000000000000000000, 0.9659258262890683122, 1.000000000000000000, 0.9659258262890683122, 1.000000000000000000, 0.9659258262890683122, 1.000000000000000000, 0.9659258262890683122, 1.000000000000000000, 0.9659258262890683122, 1.000000000000000000, 0.9659258262890683122, 1.000000000000000000, 0.9659258262890683122, 1.000000000000000000, 0.9659258262890683122, 1.000000000000000000, 0.9659258262890683122, 1.000000000000000000, 0.9659258262890683122, 1.000000000000000000, 0.9659258262890683122, 1.000000000000000000, 0.9659258262890683122, 1.000000000000000000, 0.9659258262890683122, 1.000000000000000000, 0.9659258262890683122, 1.000000000000000000, 0.9659258262890683122, 1.000000000000000000, 0.9659258262890683122, 1.000000000000000000, 0.9659258262890683122, 1.000000000000000000, 0.9659258262890683122, 1.000000000000000000, 0.9659258262890683122, 1.000000000000000000, 0.9659258262890683122, 1.000000000000000000, 0.9659258262890683122, 1.000000000000000000, 0.9659258262890683122, 1.000000000000000000, 0.9659258262890683122, 1.000000000000000000, 0.9659258262890683122, 1.000000000000000000, 0.9659258262890683122, 1.000000000000000000, 0.9659258262890683122, 1.000000000000000000, 0.9659258262890683122, 1.000000000000000000, 0.9659258262890683122, 1.000000000000000000, 0.9659258262890683122, 1.000000000000000000, 0.9659258262890683122, 1.000000000000000000, 0.9659258262890683122, 1.000000000000000000, 0.9659258262890683122, 1.000000000000000000, 0.9659258262890683122, 1.000000000000000000, 0.9659258262890683122, 1.000000000000000000, 0.9659258262890683122, 1.000000000000000000, 0.9659258262890683122, 1.000000000000000000, 0.9659258262890683122, 1.000000000000000000, 0.9659258262890683122, 1.000000000000000000, 0.9659258262890683122, 1.000000000000000000, 0.9659258262890683122, 1.000000000000000000, 0.9659258262890683122, 1.000000000000000000, 0.9659258262890683122, 1.000000000000000000, 0.9659258262890683122, 1.000000000000000000, 0.9659258262890683122, 1.000000000000000000, 0.9659258262890683122, 1.000000000000000000, 0.9659258262890683122, 1.000000000000000000, 0.9659258262890683122, 1.000000000000000000, 0.9659258262890683122, 1.000000000000000000, 0.9659258262890683122, 1.000000000000000000, 0.9659258262890683122, 1.000000000000000000, 0.9659258262890683122, 1.000000000000000000, 0.9659258262890683122, 1.000000000000000000, 0.9659258262890683122, 1.000000000000000000, 0.9659258262890683122, 1.000000000000000000, 0.9659258262890683122, 1.000000000000000000, 0.9659258262890683122, 1.000000000000000000, 0.9659258262890683122, 1.000000000000000000, 0.9659258262890683122, 1.000000000000000000, 0.9659258262890683122, 1.000000000000000000, 0.9659258262890683122, 1.000000000000000000, 0.9659258262890683122, 1.000000000000000000, 0.9659258262890683122, 1.000000000000000000, 0.9659258262890683122, 1.000000000000000000, 0.9659258262890683122, 1.000000000000000000, 0.9659258262890683122, 1.000000000000000000, 0.9659258262890683122, 1.000000000000000000, 0.9659258262890683122, 1.000000000000000000, 0.9659258262890683122, 1.000000000000000000, 0.9659258262890683122, 1.000000000000000000, 0.9659258262890683122, 1.000000000000000000, 0.9659258262890683122, 1.000000000000000000, 0.9659258262890683122, 1.000000000000000000, 0.9659258262890683122, 1.000000000000000000, 0.9659258262890683122, 1.000000000000000000, 0.9659258262890683122, 1.000000000000000000, 0.9659258262890683122, 1.000000000000000000, 0.9659258262890683122, 1.000000000000000000, 0.9659258262890683122, 1.000000000000000000, 0.9659258262890683122, 1.000000000000000000, 0.9659258262890683122, 1.000000000000000000, 0.9659258262890683122, 1.000000000000000000, 0.9659258262890683122, 1.000000000000000000, 0.9659258262890683122, 1.000000000000000000, 0.9659258262890683122, 1.000000000000000000, 0.9659258262890683122, 1.000000000000000000, 0.9659258262890683122, 1.000000000000000000, 0.9659258262890683122, 1.000000000000000000, 0.9659258262890683122, 1.000000000000000000, 0.9659258262890683122, 1.000000000000000000, 0.9659258262890683122, 1.000000000000000000, 0.9659258262890683122, 1.000000000000000000, 0.9659258262890683122, 1.000000000000000000, 0.9659258262890683122, 1.000000000000000000, 0.9659258262890683122, 1.000000000000000000, 0.9659258262890683122, 1.000000000000000000, 0.9659258262890683122, 1.000000000000000000, 0.9659258262890683122, 1.000000000000000000, 0.9659258262890683122, 1.000000000000000000),
 ( 0.3333333333333333703, 0.3219752754296894559, 0.3333333333333333703, 0.3219752754296894559, 0.3333333333333333703, 0.3219752754296894559, 0.3333333333333333703, 0.3219752754296894559, 0.3333333333333333703, 0.3219752754296894559, 0.3333333333333333703, 0.3219752754296894559, 0.3333333333333333703, 0.3219752754296894559, 0.3333333333333333703, 0.3219752754296894559, 0.3333333333333333703, 0.3219752754296894559, 0.3333333333333333703, 0.3219752754296894559, 0.3333333333333333703, 0.3219752754296894559, 0.3333333333333333703, 0.3219752754296894559, 0.3333333333333333703, 0.3219752754296894559, 0.3333333333333333703, 0.3219752754296894559, 0.3333333333333333703, 0.3219752754296894559, 0.3333333333333333703, 0.3219752754296894559, 0.3333333333333333703, 0.3219752754296894559, 0.3333333333333333703, 0.3219752754296894559, 0.3333333333333333703, 0.3219752754296894559, 0.3333333333333333703, 0.3219752754296894559, 0.3333333333333333703, 0.3219752754296894559, 0.3333333333333333703, 0.3219752754296894559, 0.3333333333333333703, 0.3219752754296894559, 0.3333333333333333703, 0.3219752754296894559, 0.3333333333333333703, 0.3219752754296894559, 0.3333333333333333703, 0.3219752754296894559, 0.3333333333333333703, 0.3219752754296894559, 0.3333333333333333703, 0.3219752754296894559, 0.3333333333333333703, 0.3219752754296894559, 0.3333333333333333703, 0.3219752754296894559, 0.3333333333333333703, 0.3219752754296894559, 0.3333333333333333703, 0.3219752754296894559, 0.3333333333333333703, 0.3219752754296894559, 0.3333333333333333703, 0.3219752754296894559, 0.3333333333333333703, 0.3219752754296894559, 0.3333333333333333703, 0.3219752754296894559, 0.3333333333333333703, 0.3219752754296894559, 0.3333333333333333703, 0.3219752754296894559, 0.3333333333333333703, 0.3219752754296894559, 0.3333333333333333703, 0.3219752754296894559, 0.3333333333333333703, 0.3219752754296894559, 0.3333333333333333703, 0.3219752754296894559, 0.3333333333333333703, 0.3219752754296894559, 0.3333333333333333703, 0.3219752754296894559, 0.3333333333333333703, 0.3219752754296894559, 0.3333333333333333703, 0.3219752754296894559, 0.3333333333333333703, 0.3219752754296894559, 0.3333333333333333703, 0.3219752754296894559, 0.3333333333333333703, 0.3219752754296894559, 0.3333333333333333703, 0.3219752754296894559, 0.3333333333333333703, 0.3219752754296894559, 0.3333333333333333703, 0.3219752754296894559, 0.3333333333333333703, 0.3219752754296894559, 0.3333333333333333703, 0.3219752754296894559, 0.3333333333333333703, 0.3219752754296894559, 0.3333333333333333703, 0.3219752754296894559, 0.3333333333333333703, 0.3219752754296894559, 0.3333333333333333703, 0.3219752754296894559, 0.3333333333333333703, 0.3219752754296894559, 0.3333333333333333703, 0.3219752754296894559, 0.3333333333333333703, 0.3219752754296894559, 0.3333333333333333703, 0.3219752754296894559, 0.3333333333333333703, 0.3219752754296894559, 0.3333333333333333703, 0.3219752754296894559, 0.3333333333333333703, 0.3219752754296894559, 0.3333333333333333703, 0.3219752754296894559, 0.3333333333333333703, 0.3219752754296894559, 0.3333333333333333703, 0.3219752754296894559, 0.3333333333333333703, 0.3219752754296894559, 0.3333333333333333703, 0.3219752754296894559, 0.3333333333333333703, 0.3219752754296894559, 0.3333333333333333703, 0.3219752754296894559, 0.3333333333333333703, 0.3219752754296894559, 0.3333333333333333703, 0.3219752754296894559, 0.3333333333333333703, 0.3219752754296894559, 0.3333333333333333703, 0.3219752754296894559, 0.3333333333333333703, 0.3219752754296894559, 0.3333333333333333703, 0.3219752754296894559, 0.3333333333333333703, 0.3219752754296894559, 0.3333333333333333703, 0.3219752754296894559, 0.3333333333333333703, 0.3219752754296894559, 0.3333333333333333703, 0.3219752754296894559, 0.3333333333333333703, 0.3219752754296894559, 0.3333333333333333703, 0.3219752754296894559, 0.3333333333333333703, 0.3219752754296894559, 0.3333333333333333703, 0.3219752754296894559, 0.3333333333333333703, 0.3219752754296894559, 0.3333333333333333703, 0.3219752754296894559, 0.3333333333333333703, 0.3219752754296894559, 0.3333333333333333703, 0.3219752754296894559, 0.3333333333333333703, 0.3219752754296894559, 0.3333333333333333703, 0.3219752754296894559, 0.3333333333333333703, 0.3219752754296894559, 0.3333333333333333703, 0.3219752754296894559, 0.3333333333333333703, 0.3219752754296894559, 0.3333333333333333703, 0.3219752754296894559, 0.3333333333333333703, 0.3219752754296894559, 0.3333333333333333703, 0.3219752754296894559, 0.3333333333333333703, 0.3219752754296894559, 0.3333333333333333703, 0.3219752754296894559, 0.3333333333333333703, 0.3219752754296894559, 0.3333333333333333703, 0.3219752754296894559, 0.3333333333333333703, 0.3219752754296894559, 0.3333333333333333703, 0.3219752754296894559, 0.3333333333333333703, 0.3219752754296894559, 0.3333333333333333703, 0.3219752754296894559, 0.3333333333333333703, 0.3219752754296894559, 0.3333333333333333703, 0.3219752754296894559, 0.3333333333333333703, 0.3219752754296894559, 0.3333333333333333703, 0.3219752754296894559, 0.3333333333333333703, 0.3219752754296894559, 0.3333333333333333703, 0.3219752754296894559, 0.3333333333333333703, 0.3219752754296894559, 0.3333333333333333703, 0.3219752754296894559, 0.3333333333333333703, 0.3219752754296894559, 0.3333333333333333703, 0.3219752754296894559, 0.3333333333333333703, 0.3219752754296894559, 0.3333333333333333703, 0.3219752754296894559, 0.3333333333333333703, 0.3219752754296894559, 0.3333333333333333703, 0.3219752754296894559, 0.3333333333333333703, 0.3219752754296894559, 0.3333333333333333703, 0.3219752754296894559, 0.3333333333333333703, 0.3219752754296894559, 0.3333333333333333703, 0.3219752754296894559, 0.3333333333333333703, 0.3219752754296894559, 0.3333333333333333703, 0.3219752754296894559, 0.3333333333333333703, 0.3219752754296894559, 0.3333333333333333703, 0.3219752754296894559, 0.3333333333333333703, 0.3219752754296894559, 0.3333333333333333703, 0.3219752754296894559, 0.3333333333333333703, 0.3219752754296894559, 0.3333333333333333703, 0.3219752754296894559, 0.3333333333333333703, 0.3219752754296894559, 0.3333333333333333703, 0.3219752754296894559, 0.3333333333333333703, 0.3219752754296894559, 0.3333333333333333703, 0.3219752754296894559, 0.3333333333333333703, 0.3219752754296894559, 0.3333333333333333703, 0.3219752754296894559, 0.3333333333333333703, 0.3219752754296894559, 0.3333333333333333703, 0.3219752754296894559, 0.3333333333333333703, 0.3219752754296894559, 0.3333333333333333703, 0.3219752754296894559, 0.3333333333333333703, 0.3219752754296894559, 0.3333333333333333703, 0.3219752754296894559, 0.3333333333333333703, 0.3219752754296894559, 0.3333333333333333703, 0.3219752754296894559, 0.3333333333333333703, 0.3219752754296894559, 0.3333333333333333703, 0.3219752754296894559, 0.3333333333333333703, 0.3219752754296894559, 0.3333333333333333703, 0.3219752754296894559, 0.3333333333333333703, 0.3219752754296894559, 0.3333333333333333703, 0.3219752754296894559, 0.3333333333333333703, 0.3219752754296894559, 0.3333333333333333703, 0.3219752754296894559, 0.3333333333333333703, 0.3219752754296894559, 0.3333333333333333703, 0.3219752754296894559, 0.3333333333333333703, 0.3219752754296894559, 0.3333333333333333703, 0.3219752754296894559, 0.3333333333333333703, 0.3219752754296894559, 0.3333333333333333703, 0.3219752754296894559, 0.3333333333333333703, 0.3219752754296894559, 0.3333333333333333703, 0.3219752754296894559, 0.3333333333333333703, 0.3219752754296894559, 0.3333333333333333703, 0.3219752754296894559, 0.3333333333333333703, 0.3219752754296894559, 0.3333333333333333703, 0.3219752754296894559, 0.3333333333333333703, 0.3219752754296894559, 0.3333333333333333703, 0.3219752754296894559, 0.3333333333333333703, 0.3219752754296894559, 0.3333333333333333703, 0.3219752754296894559, 0.3333333333333333703, 0.3219752754296894559, 0.3333333333333333703, 0.3219752754296894559, 0.3333333333333333703, 0.3219752754296894559, 0.3333333333333333703, 0.3219752754296894559, 0.3333333333333333703, 0.3219752754296894559, 0.3333333333333333703, 0.3219752754296894559, 0.3333333333333333703, 0.3219752754296894559, 0.3333333333333333703, 0.3219752754296894559, 0.3333333333333333703, 0.3219752754296894559, 0.3333333333333333703, 0.3219752754296894559, 0.3333333333333333703, 0.3219752754296894559, 0.3333333333333333703, 0.3219752754296894559, 0.3333333333333333703, 0.3219752754296894559, 0.3333333333333333703, 0.3219752754296894559, 0.3333333333333333703, 0.3219752754296894559, 0.3333333333333333703, 0.3219752754296894559, 0.3333333333333333703, 0.3219752754296894559, 0.3333333333333333703, 0.3219752754296894559, 0.3333333333333333703, 0.3219752754296894559, 0.3333333333333333703, 0.3219752754296894559, 0.3333333333333333703, 0.3219752754296894559, 0.3333333333333333703, 0.3219752754296894559, 0.3333333333333333703, 0.3219752754296894559, 0.3333333333333333703, 0.3219752754296894559, 0.3333333333333333703, 0.3219752754296894559, 0.3333333333333333703, 0.3219752754296894559, 0.3333333333333333703, 0.3219752754296894559, 0.3333333333333333703, 0.3219752754296894559, 0.3333333333333333703, 0.3219752754296894559, 0.3333333333333333703, 0.3219752754296894559, 0.3333333333333333703, 0.3219752754296894559, 0.3333333333333333703, 0.3219752754296894559, 0.3333333333333333703, 0.3219752754296894559, 0.3333333333333333703, 0.3219752754296894559, 0.3333333333333333703, 0.3219752754296894559, 0.3333333333333333703, 0.3219752754296894559, 0.3333333333333333703, 0.3219752754296894559, 0.3333333333333333703, 0.3219752754296894559, 0.3333333333333333703, 0.3219752754296894559, 0.3333333333333333703, 0.3219752754296894559, 0.3333333333333333703, 0.3219752754296894559, 0.3333333333333333703, 0.3219752754296894559, 0.3333333333333333703, 0.3219752754296894559, 0.3333333333333333703, 0.3219752754296894559, 0.3333333333333333703, 0.3219752754296894559, 0.3333333333333333703, 0.3219752754296894559, 0.3333333333333333703, 0.3219752754296894559, 0.3333333333333333703, 0.3219752754296894559, 0.3333333333333333703, 0.3219752754296894559, 0.3333333333333333703, 0.3219752754296894559, 0.3333333333333333703, 0.3219752754296894559, 0.3333333333333333703, 0.3219752754296894559, 0.3333333333333333703, 0.3219752754296894559, 0.3333333333333333703, 0.3219752754296894559, 0.3333333333333333703, 0.3219752754296894559, 0.3333333333333333703, 0.3219752754296894559, 0.3333333333333333703, 0.3219752754296894559, 0.3333333333333333703, 0.3219752754296894559, 0.3333333333333333703),
 ( 0.3333333333333333703, 0.3219752754296894559, 0.3333333333333333703, 0.3219752754296894559, 0.3333333333333333703, 0.3219752754296894559, 0.3333333333333333703, 0.3219752754296894559, 0.3333333333333333703, 0.3219752754296894559, 0.3333333333333333703, 0.3219752754296894559, 0.3333333333333333703, 0.3219752754296894559, 0.3333333333333333703, 0.3219752754296894559, 0.3333333333333333703, 0.3219752754296894559, 0.3333333333333333703, 0.3219752754296894559, 0.3333333333333333703, 0.3219752754296894559, 0.3333333333333333703, 0.3219752754296894559, 0.3333333333333333703, 0.3219752754296894559, 0.3333333333333333703, 0.3219752754296894559, 0.3333333333333333703, 0.3219752754296894559, 0.3333333333333333703, 0.3219752754296894559, 0.3333333333333333703, 0.3219752754296894559, 0.3333333333333333703, 0.3219752754296894559, 0.3333333333333333703, 0.3219752754296894559, 0.3333333333333333703, 0.3219752754296894559, 0.3333333333333333703, 0.3219752754296894559, 0.3333333333333333703, 0.3219752754296894559, 0.3333333333333333703, 0.3219752754296894559, 0.3333333333333333703, 0.3219752754296894559, 0.3333333333333333703, 0.3219752754296894559, 0.3333333333333333703, 0.3219752754296894559, 0.3333333333333333703, 0.3219752754296894559, 0.3333333333333333703, 0.3219752754296894559, 0.3333333333333333703, 0.3219752754296894559, 0.3333333333333333703, 0.3219752754296894559, 0.3333333333333333703, 0.3219752754296894559, 0.3333333333333333703, 0.3219752754296894559, 0.3333333333333333703, 0.3219752754296894559, 0.3333333333333333703, 0.3219752754296894559, 0.3333333333333333703, 0.3219752754296894559, 0.3333333333333333703, 0.3219752754296894559, 0.3333333333333333703, 0.3219752754296894559, 0.3333333333333333703, 0.3219752754296894559, 0.3333333333333333703, 0.3219752754296894559, 0.3333333333333333703, 0.3219752754296894559, 0.3333333333333333703, 0.3219752754296894559, 0.3333333333333333703, 0.3219752754296894559, 0.3333333333333333703, 0.3219752754296894559, 0.3333333333333333703, 0.3219752754296894559, 0.3333333333333333703, 0.3219752754296894559, 0.3333333333333333703, 0.3219752754296894559, 0.3333333333333333703, 0.3219752754296894559, 0.3333333333333333703, 0.3219752754296894559, 0.3333333333333333703, 0.3219752754296894559, 0.3333333333333333703, 0.3219752754296894559, 0.3333333333333333703, 0.3219752754296894559, 0.3333333333333333703, 0.3219752754296894559, 0.3333333333333333703, 0.3219752754296894559, 0.3333333333333333703, 0.3219752754296894559, 0.3333333333333333703, 0.3219752754296894559, 0.3333333333333333703, 0.3219752754296894559, 0.3333333333333333703, 0.3219752754296894559, 0.3333333333333333703, 0.3219752754296894559, 0.3333333333333333703, 0.3219752754296894559, 0.3333333333333333703, 0.3219752754296894559, 0.3333333333333333703, 0.3219752754296894559, 0.3333333333333333703, 0.3219752754296894559, 0.3333333333333333703, 0.3219752754296894559, 0.3333333333333333703, 0.3219752754296894559, 0.3333333333333333703, 0.3219752754296894559, 0.3333333333333333703, 0.3219752754296894559, 0.3333333333333333703, 0.3219752754296894559, 0.3333333333333333703, 0.3219752754296894559, 0.3333333333333333703, 0.3219752754296894559, 0.3333333333333333703, 0.3219752754296894559, 0.3333333333333333703, 0.3219752754296894559, 0.3333333333333333703, 0.3219752754296894559, 0.3333333333333333703, 0.3219752754296894559, 0.3333333333333333703, 0.3219752754296894559, 0.3333333333333333703, 0.3219752754296894559, 0.3333333333333333703, 0.3219752754296894559, 0.3333333333333333703, 0.3219752754296894559, 0.3333333333333333703, 0.3219752754296894559, 0.3333333333333333703, 0.3219752754296894559, 0.3333333333333333703, 0.3219752754296894559, 0.3333333333333333703, 0.3219752754296894559, 0.3333333333333333703, 0.3219752754296894559, 0.3333333333333333703, 0.3219752754296894559, 0.3333333333333333703, 0.3219752754296894559, 0.3333333333333333703, 0.3219752754296894559, 0.3333333333333333703, 0.3219752754296894559, 0.3333333333333333703, 0.3219752754296894559, 0.3333333333333333703, 0.3219752754296894559, 0.3333333333333333703, 0.3219752754296894559, 0.3333333333333333703, 0.3219752754296894559, 0.3333333333333333703, 0.3219752754296894559, 0.3333333333333333703, 0.3219752754296894559, 0.3333333333333333703, 0.3219752754296894559, 0.3333333333333333703, 0.3219752754296894559, 0.3333333333333333703, 0.3219752754296894559, 0.3333333333333333703, 0.3219752754296894559, 0.3333333333333333703, 0.3219752754296894559, 0.3333333333333333703, 0.3219752754296894559, 0.3333333333333333703, 0.3219752754296894559, 0.3333333333333333703, 0.3219752754296894559, 0.3333333333333333703, 0.3219752754296894559, 0.3333333333333333703, 0.3219752754296894559, 0.3333333333333333703, 0.3219752754296894559, 0.3333333333333333703, 0.3219752754296894559, 0.3333333333333333703, 0.3219752754296894559, 0.3333333333333333703, 0.3219752754296894559, 0.3333333333333333703, 0.3219752754296894559, 0.3333333333333333703, 0.3219752754296894559, 0.3333333333333333703, 0.3219752754296894559, 0.3333333333333333703, 0.3219752754296894559, 0.3333333333333333703, 0.3219752754296894559, 0.3333333333333333703, 0.3219752754296894559, 0.3333333333333333703, 0.3219752754296894559, 0.3333333333333333703, 0.3219752754296894559, 0.3333333333333333703, 0.3219752754296894559, 0.3333333333333333703, 0.3219752754296894559, 0.3333333333333333703, 0.3219752754296894559, 0.3333333333333333703, 0.3219752754296894559, 0.3333333333333333703, 0.3219752754296894559, 0.3333333333333333703, 0.3219752754296894559, 0.3333333333333333703, 0.3219752754296894559, 0.3333333333333333703, 0.3219752754296894559, 0.3333333333333333703, 0.3219752754296894559, 0.3333333333333333703, 0.3219752754296894559, 0.3333333333333333703, 0.3219752754296894559, 0.3333333333333333703, 0.3219752754296894559, 0.3333333333333333703, 0.3219752754296894559, 0.3333333333333333703, 0.3219752754296894559, 0.3333333333333333703, 0.3219752754296894559, 0.3333333333333333703, 0.3219752754296894559, 0.3333333333333333703, 0.3219752754296894559, 0.3333333333333333703, 0.3219752754296894559, 0.3333333333333333703, 0.3219752754296894559, 0.3333333333333333703, 0.3219752754296894559, 0.3333333333333333703, 0.3219752754296894559, 0.3333333333333333703, 0.3219752754296894559, 0.3333333333333333703, 0.3219752754296894559, 0.3333333333333333703, 0.3219752754296894559, 0.3333333333333333703, 0.3219752754296894559, 0.3333333333333333703, 0.3219752754296894559, 0.3333333333333333703, 0.3219752754296894559, 0.3333333333333333703, 0.3219752754296894559, 0.3333333333333333703, 0.3219752754296894559, 0.3333333333333333703, 0.3219752754296894559, 0.3333333333333333703, 0.3219752754296894559, 0.3333333333333333703, 0.3219752754296894559, 0.3333333333333333703, 0.3219752754296894559, 0.3333333333333333703, 0.3219752754296894559, 0.3333333333333333703, 0.3219752754296894559, 0.3333333333333333703, 0.3219752754296894559, 0.3333333333333333703, 0.3219752754296894559, 0.3333333333333333703, 0.3219752754296894559, 0.3333333333333333703, 0.3219752754296894559, 0.3333333333333333703, 0.3219752754296894559, 0.3333333333333333703, 0.3219752754296894559, 0.3333333333333333703, 0.3219752754296894559, 0.3333333333333333703, 0.3219752754296894559, 0.3333333333333333703, 0.3219752754296894559, 0.3333333333333333703, 0.3219752754296894559, 0.3333333333333333703, 0.3219752754296894559, 0.3333333333333333703, 0.3219752754296894559, 0.3333333333333333703, 0.3219752754296894559, 0.3333333333333333703, 0.3219752754296894559, 0.3333333333333333703, 0.3219752754296894559, 0.3333333333333333703, 0.3219752754296894559, 0.3333333333333333703, 0.3219752754296894559, 0.3333333333333333703, 0.3219752754296894559, 0.3333333333333333703, 0.3219752754296894559, 0.3333333333333333703, 0.3219752754296894559, 0.3333333333333333703, 0.3219752754296894559, 0.3333333333333333703, 0.3219752754296894559, 0.3333333333333333703, 0.3219752754296894559, 0.3333333333333333703, 0.3219752754296894559, 0.3333333333333333703, 0.3219752754296894559, 0.3333333333333333703, 0.3219752754296894559, 0.3333333333333333703, 0.3219752754296894559, 0.3333333333333333703, 0.3219752754296894559, 0.3333333333333333703, 0.3219752754296894559, 0.3333333333333333703, 0.3219752754296894559, 0.3333333333333333703, 0.3219752754296894559, 0.3333333333333333703, 0.3219752754296894559, 0.3333333333333333703, 0.3219752754296894559, 0.3333333333333333703, 0.3219752754296894559, 0.3333333333333333703, 0.3219752754296894559, 0.3333333333333333703, 0.3219752754296894559, 0.3333333333333333703, 0.3219752754296894559, 0.3333333333333333703, 0.3219752754296894559, 0.3333333333333333703, 0.3219752754296894559, 0.3333333333333333703, 0.3219752754296894559, 0.3333333333333333703, 0.3219752754296894559, 0.3333333333333333703, 0.3219752754296894559, 0.3333333333333333703, 0.3219752754296894559, 0.3333333333333333703, 0.3219752754296894559, 0.3333333333333333703, 0.3219752754296894559, 0.3333333333333333703, 0.3219752754296894559, 0.3333333333333333703, 0.3219752754296894559, 0.3333333333333333703, 0.3219752754296894559, 0.3333333333333333703, 0.3219752754296894559, 0.3333333333333333703, 0.3219752754296894559, 0.3333333333333333703, 0.3219752754296894559, 0.3333333333333333703, 0.3219752754296894559, 0.3333333333333333703, 0.3219752754296894559, 0.3333333333333333703, 0.3219752754296894559, 0.3333333333333333703, 0.3219752754296894559, 0.3333333333333333703, 0.3219752754296894559, 0.3333333333333333703, 0.3219752754296894559, 0.3333333333333333703, 0.3219752754296894559, 0.3333333333333333703, 0.3219752754296894559, 0.3333333333333333703, 0.3219752754296894559, 0.3333333333333333703, 0.3219752754296894559, 0.3333333333333333703, 0.3219752754296894559, 0.3333333333333333703, 0.3219752754296894559, 0.3333333333333333703, 0.3219752754296894559, 0.3333333333333333703, 0.3219752754296894559, 0.3333333333333333703, 0.3219752754296894559, 0.3333333333333333703, 0.3219752754296894559, 0.3333333333333333703, 0.3219752754296894559, 0.3333333333333333703, 0.3219752754296894559, 0.3333333333333333703, 0.3219752754296894559, 0.3333333333333333703, 0.3219752754296894559, 0.3333333333333333703, 0.3219752754296894559, 0.3333333333333333703, 0.3219752754296894559, 0.3333333333333333703, 0.3219752754296894559, 0.3333333333333333703, 0.3219752754296894559, 0.3333333333333333703, 0.3219752754296894559, 0.3333333333333333703, 0.3219752754296894559, 0.3333333333333333703, 0.3219752754296894559, 0.3333333333333333703, 0.3219752754296894559, 0.3333333333333333703),
 ( 1.000000000000000000, 0.9659258262890683122, 1.000000000000000000, 0.9659258262890683122, 1.000000000000000000, 0.9659258262890683122, 1.000000000000000000, 0.9659258262890683122, 1.000000000000000000, 0.9659258262890683122, 1.000000000000000000, 0.9659258262890683122, 1.000000000000000000, 0.9659258262890683122, 1.000000000000000000, 0.9659258262890683122, 1.000000000000000000, 0.9659258262890683122, 1.000000000000000000, 0.9659258262890683122, 1.000000000000000000, 0.9659258262890683122, 1.000000000000000000, 0.9659258262890683122, 1.000000000000000000, 0.9659258262890683122, 1.000000000000000000, 0.9659258262890683122, 1.000000000000000000, 0.9659258262890683122, 1.000000000000000000, 0.9659258262890683122, 1.000000000000000000, 0.9659258262890683122, 1.000000000000000000, 0.9659258262890683122, 1.000000000000000000, 0.9659258262890683122, 1.000000000000000000, 0.9659258262890683122, 1.000000000000000000, 0.9659258262890683122, 1.000000000000000000, 0.9659258262890683122, 1.000000000000000000, 0.9659258262890683122, 1.000000000000000000, 0.9659258262890683122, 1.000000000000000000, 0.9659258262890683122, 1.000000000000000000, 0.9659258262890683122, 1.000000000000000000, 0.9659258262890683122, 1.000000000000000000, 0.9659258262890683122, 1.000000000000000000, 0.9659258262890683122, 1.000000000000000000, 0.9659258262890683122, 1.000000000000000000, 0.9659258262890683122, 1.000000000000000000, 0.9659258262890683122, 1.000000000000000000, 0.9659258262890683122, 1.000000000000000000, 0.9659258262890683122, 1.000000000000000000, 0.9659258262890683122, 1.000000000000000000, 0.9659258262890683122, 1.000000000000000000, 0.9659258262890683122, 1.000000000000000000, 0.9659258262890683122, 1.000000000000000000, 0.9659258262890683122, 1.000000000000000000, 0.9659258262890683122, 1.000000000000000000, 0.9659258262890683122, 1.000000000000000000, 0.9659258262890683122, 1.000000000000000000, 0.9659258262890683122, 1.000000000000000000, 0.9659258262890683122, 1.000000000000000000, 0.9659258262890683122, 1.000000000000000000, 0.9659258262890683122, 1.000000000000000000, 0.9659258262890683122, 1.000000000000000000, 0.9659258262890683122, 1.000000000000000000, 0.9659258262890683122, 1.000000000000000000, 0.9659258262890683122, 1.000000000000000000, 0.9659258262890683122, 1.000000000000000000, 0.9659258262890683122, 1.000000000000000000, 0.9659258262890683122, 1.000000000000000000, 0.9659258262890683122, 1.000000000000000000, 0.9659258262890683122, 1.000000000000000000, 0.9659258262890683122, 1.000000000000000000, 0.9659258262890683122, 1.000000000000000000, 0.9659258262890683122, 1.000000000000000000, 0.9659258262890683122, 1.000000000000000000, 0.9659258262890683122, 1.000000000000000000, 0.9659258262890683122, 1.000000000000000000, 0.9659258262890683122, 1.000000000000000000, 0.9659258262890683122, 1.000000000000000000, 0.9659258262890683122, 1.000000000000000000, 0.9659258262890683122, 1.000000000000000000, 0.9659258262890683122, 1.000000000000000000, 0.9659258262890683122, 1.000000000000000000, 0.9659258262890683122, 1.000000000000000000, 0.9659258262890683122, 1.000000000000000000, 0.9659258262890683122, 1.000000000000000000, 0.9659258262890683122, 1.000000000000000000, 0.9659258262890683122, 1.000000000000000000, 0.9659258262890683122, 1.000000000000000000, 0.9659258262890683122, 1.000000000000000000, 0.9659258262890683122, 1.000000000000000000, 0.9659258262890683122, 1.000000000000000000, 0.9659258262890683122, 1.000000000000000000, 0.9659258262890683122, 1.000000000000000000, 0.9659258262890683122, 1.000000000000000000, 0.9659258262890683122, 1.000000000000000000, 0.9659258262890683122, 1.000000000000000000, 0.9659258262890683122, 1.000000000000000000, 0.9659258262890683122, 1.000000000000000000, 0.9659258262890683122, 1.000000000000000000, 0.9659258262890683122, 1.000000000000000000, 0.9659258262890683122, 1.000000000000000000, 0.9659258262890683122, 1.000000000000000000, 0.9659258262890683122, 1.000000000000000000, 0.9659258262890683122, 1.000000000000000000, 0.9659258262890683122, 1.000000000000000000, 0.9659258262890683122, 1.000000000000000000, 0.9659258262890683122, 1.000000000000000000, 0.9659258262890683122, 1.000000000000000000, 0.9659258262890683122, 1.000000000000000000, 0.9659258262890683122, 1.000000000000000000, 0.9659258262890683122, 1.000000000000000000, 0.9659258262890683122, 1.000000000000000000, 0.9659258262890683122, 1.000000000000000000, 0.9659258262890683122, 1.000000000000000000, 0.9659258262890683122, 1.000000000000000000, 0.9659258262890683122, 1.000000000000000000, 0.9659258262890683122, 1.000000000000000000, 0.9659258262890683122, 1.000000000000000000, 0.9659258262890683122, 1.000000000000000000, 0.9659258262890683122, 1.000000000000000000, 0.9659258262890683122, 1.000000000000000000, 0.9659258262890683122, 1.000000000000000000, 0.9659258262890683122, 1.000000000000000000, 0.9659258262890683122, 1.000000000000000000, 0.9659258262890683122, 1.000000000000000000, 0.9659258262890683122, 1.000000000000000000, 0.9659258262890683122, 1.000000000000000000, 0.9659258262890683122, 1.000000000000000000, 0.9659258262890683122, 1.000000000000000000, 0.9659258262890683122, 1.000000000000000000, 0.9659258262890683122, 1.000000000000000000, 0.9659258262890683122, 1.000000000000000000, 0.9659258262890683122, 1.000000000000000000, 0.9659258262890683122, 1.000000000000000000, 0.9659258262890683122, 1.000000000000000000, 0.9659258262890683122, 1.000000000000000000, 0.9659258262890683122, 1.000000000000000000, 0.9659258262890683122, 1.000000000000000000, 0.9659258262890683122, 1.000000000000000000, 0.9659258262890683122, 1.000000000000000000, 0.9659258262890683122, 1.000000000000000000, 0.9659258262890683122, 1.000000000000000000, 0.9659258262890683122, 1.000000000000000000, 0.9659258262890683122, 1.000000000000000000, 0.9659258262890683122, 1.000000000000000000, 0.9659258262890683122, 1.000000000000000000, 0.9659258262890683122, 1.000000000000000000, 0.9659258262890683122, 1.000000000000000000, 0.9659258262890683122, 1.000000000000000000, 0.9659258262890683122, 1.000000000000000000, 0.9659258262890683122, 1.000000000000000000, 0.9659258262890683122, 1.000000000000000000, 0.9659258262890683122, 1.000000000000000000, 0.9659258262890683122, 1.000000000000000000, 0.9659258262890683122, 1.000000000000000000, 0.9659258262890683122, 1.000000000000000000, 0.9659258262890683122, 1.000000000000000000, 0.9659258262890683122, 1.000000000000000000, 0.9659258262890683122, 1.000000000000000000, 0.9659258262890683122, 1.000000000000000000, 0.9659258262890683122, 1.000000000000000000, 0.9659258262890683122, 1.000000000000000000, 0.9659258262890683122, 1.000000000000000000, 0.9659258262890683122, 1.000000000000000000, 0.9659258262890683122, 1.000000000000000000, 0.9659258262890683122, 1.000000000000000000, 0.9659258262890683122, 1.000000000000000000, 0.9659258262890683122, 1.000000000000000000, 0.9659258262890683122, 1.000000000000000000, 0.9659258262890683122, 1.000000000000000000, 0.9659258262890683122, 1.000000000000000000, 0.9659258262890683122, 1.000000000000000000, 0.9659258262890683122, 1.000000000000000000, 0.9659258262890683122, 1.000000000000000000, 0.9659258262890683122, 1.000000000000000000, 0.9659258262890683122, 1.000000000000000000, 0.9659258262890683122, 1.000000000000000000, 0.9659258262890683122, 1.000000000000000000, 0.9659258262890683122, 1.000000000000000000, 0.9659258262890683122, 1.000000000000000000, 0.9659258262890683122, 1.000000000000000000, 0.9659258262890683122, 1.000000000000000000, 0.9659258262890683122, 1.000000000000000000, 0.9659258262890683122, 1.000000000000000000, 0.9659258262890683122, 1.000000000000000000, 0.9659258262890683122, 1.000000000000000000, 0.9659258262890683122, 1.000000000000000000, 0.9659258262890683122, 1.000000000000000000, 0.9659258262890683122, 1.000000000000000000, 0.9659258262890683122, 1.000000000000000000, 0.9659258262890683122, 1.000000000000000000, 0.9659258262890683122, 1.000000000000000000, 0.9659258262890683122, 1.000000000000000000, 0.9659258262890683122, 1.000000000000000000, 0.9659258262890683122, 1.000000000000000000, 0.9659258262890683122, 1.000000000000000000, 0.9659258262890683122, 1.000000000000000000, 0.9659258262890683122, 1.000000000000000000, 0.9659258262890683122, 1.000000000000000000, 0.9659258262890683122, 1.000000000000000000, 0.9659258262890683122, 1.000000000000000000, 0.9659258262890683122, 1.000000000000000000, 0.9659258262890683122, 1.000000000000000000, 0.9659258262890683122, 1.000000000000000000, 0.9659258262890683122, 1.000000000000000000, 0.9659258262890683122, 1.000000000000000000, 0.9659258262890683122, 1.000000000000000000, 0.9659258262890683122, 1.000000000000000000, 0.9659258262890683122, 1.000000000000000000, 0.9659258262890683122, 1.000000000000000000, 0.9659258262890683122, 1.000000000000000000, 0.9659258262890683122, 1.000000000000000000, 0.9659258262890683122, 1.000000000000000000, 0.9659258262890683122, 1.000000000000000000, 0.9659258262890683122, 1.000000000000000000, 0.9659258262890683122, 1.000000000000000000, 0.9659258262890683122, 1.000000000000000000, 0.9659258262890683122, 1.000000000000000000, 0.9659258262890683122, 1.000000000000000000, 0.9659258262890683122, 1.000000000000000000, 0.9659258262890683122, 1.000000000000000000, 0.9659258262890683122, 1.000000000000000000, 0.9659258262890683122, 1.000000000000000000, 0.9659258262890683122, 1.000000000000000000, 0.9659258262890683122, 1.000000000000000000, 0.9659258262890683122, 1.000000000000000000, 0.9659258262890683122, 1.000000000000000000, 0.9659258262890683122, 1.000000000000000000, 0.9659258262890683122, 1.000000000000000000, 0.9659258262890683122, 1.000000000000000000, 0.9659258262890683122, 1.000000000000000000, 0.9659258262890683122, 1.000000000000000000, 0.9659258262890683122, 1.000000000000000000, 0.9659258262890683122, 1.000000000000000000, 0.9659258262890683122, 1.000000000000000000, 0.9659258262890683122, 1.000000000000000000, 0.9659258262890683122, 1.000000000000000000, 0.9659258262890683122, 1.000000000000000000, 0.9659258262890683122, 1.000000000000000000, 0.9659258262890683122, 1.000000000000000000, 0.9659258262890683122, 1.000000000000000000, 0.9659258262890683122, 1.000000000000000000, 0.9659258262890683122, 1.000000000000000000),
 ( 0.3333333333333333703, 0.3219752754296894559, 0.3333333333333333703, 0.3219752754296894559, 0.3333333333333333703, 0.3219752754296894559, 0.3333333333333333703, 0.3219752754296894559, 0.3333333333333333703, 0.3219752754296894559, 0.3333333333333333703, 0.3219752754296894559, 0.3333333333333333703, 0.3219752754296894559, 0.3333333333333333703, 0.3219752754296894559, 0.3333333333333333703, 0.3219752754296894559, 0.3333333333333333703, 0.3219752754296894559, 0.3333333333333333703, 0.3219752754296894559, 0.3333333333333333703, 0.3219752754296894559, 0.3333333333333333703, 0.3219752754296894559, 0.3333333333333333703, 0.3219752754296894559, 0.3333333333333333703, 0.3219752754296894559, 0.3333333333333333703, 0.3219752754296894559, 0.3333333333333333703, 0.3219752754296894559, 0.3333333333333333703, 0.3219752754296894559, 0.3333333333333333703, 0.3219752754296894559, 0.3333333333333333703, 0.3219752754296894559, 0.3333333333333333703, 0.3219752754296894559, 0.3333333333333333703, 0.3219752754296894559, 0.3333333333333333703, 0.3219752754296894559, 0.3333333333333333703, 0.3219752754296894559, 0.3333333333333333703, 0.3219752754296894559, 0.3333333333333333703, 0.3219752754296894559, 0.3333333333333333703, 0.3219752754296894559, 0.3333333333333333703, 0.3219752754296894559, 0.3333333333333333703, 0.3219752754296894559, 0.3333333333333333703, 0.3219752754296894559, 0.3333333333333333703, 0.3219752754296894559, 0.3333333333333333703, 0.3219752754296894559, 0.3333333333333333703, 0.3219752754296894559, 0.3333333333333333703, 0.3219752754296894559, 0.3333333333333333703, 0.3219752754296894559, 0.3333333333333333703, 0.3219752754296894559, 0.3333333333333333703, 0.3219752754296894559, 0.3333333333333333703, 0.3219752754296894559, 0.3333333333333333703, 0.3219752754296894559, 0.3333333333333333703, 0.3219752754296894559, 0.3333333333333333703, 0.3219752754296894559, 0.3333333333333333703, 0.3219752754296894559, 0.3333333333333333703, 0.3219752754296894559, 0.3333333333333333703, 0.3219752754296894559, 0.3333333333333333703, 0.3219752754296894559, 0.3333333333333333703, 0.3219752754296894559, 0.3333333333333333703, 0.3219752754296894559, 0.3333333333333333703, 0.3219752754296894559, 0.3333333333333333703, 0.3219752754296894559, 0.3333333333333333703, 0.3219752754296894559, 0.3333333333333333703, 0.3219752754296894559, 0.3333333333333333703, 0.3219752754296894559, 0.3333333333333333703, 0.3219752754296894559, 0.3333333333333333703, 0.3219752754296894559, 0.3333333333333333703, 0.3219752754296894559, 0.3333333333333333703, 0.3219752754296894559, 0.3333333333333333703, 0.3219752754296894559, 0.3333333333333333703, 0.3219752754296894559, 0.3333333333333333703, 0.3219752754296894559, 0.3333333333333333703, 0.3219752754296894559, 0.3333333333333333703, 0.3219752754296894559, 0.3333333333333333703, 0.3219752754296894559, 0.3333333333333333703, 0.3219752754296894559, 0.3333333333333333703, 0.3219752754296894559, 0.3333333333333333703, 0.3219752754296894559, 0.3333333333333333703, 0.3219752754296894559, 0.3333333333333333703, 0.3219752754296894559, 0.3333333333333333703, 0.3219752754296894559, 0.3333333333333333703, 0.3219752754296894559, 0.3333333333333333703, 0.3219752754296894559, 0.3333333333333333703, 0.3219752754296894559, 0.3333333333333333703, 0.3219752754296894559, 0.3333333333333333703, 0.3219752754296894559, 0.3333333333333333703, 0.3219752754296894559, 0.3333333333333333703, 0.3219752754296894559, 0.3333333333333333703, 0.3219752754296894559, 0.3333333333333333703, 0.3219752754296894559, 0.3333333333333333703, 0.3219752754296894559, 0.3333333333333333703, 0.3219752754296894559, 0.3333333333333333703, 0.3219752754296894559, 0.3333333333333333703, 0.3219752754296894559, 0.3333333333333333703, 0.3219752754296894559, 0.3333333333333333703, 0.3219752754296894559, 0.3333333333333333703, 0.3219752754296894559, 0.3333333333333333703, 0.3219752754296894559, 0.3333333333333333703, 0.3219752754296894559, 0.3333333333333333703, 0.3219752754296894559, 0.3333333333333333703, 0.3219752754296894559, 0.3333333333333333703, 0.3219752754296894559, 0.3333333333333333703, 0.3219752754296894559, 0.3333333333333333703, 0.3219752754296894559, 0.3333333333333333703, 0.3219752754296894559, 0.3333333333333333703, 0.3219752754296894559, 0.3333333333333333703, 0.3219752754296894559, 0.3333333333333333703, 0.3219752754296894559, 0.3333333333333333703, 0.3219752754296894559, 0.3333333333333333703, 0.3219752754296894559, 0.3333333333333333703, 0.3219752754296894559, 0.3333333333333333703, 0.3219752754296894559, 0.3333333333333333703, 0.3219752754296894559, 0.3333333333333333703, 0.3219752754296894559, 0.3333333333333333703, 0.3219752754296894559, 0.3333333333333333703, 0.3219752754296894559, 0.3333333333333333703, 0.3219752754296894559, 0.3333333333333333703, 0.3219752754296894559, 0.3333333333333333703, 0.3219752754296894559, 0.3333333333333333703, 0.3219752754296894559, 0.3333333333333333703, 0.3219752754296894559, 0.3333333333333333703, 0.3219752754296894559, 0.3333333333333333703, 0.3219752754296894559, 0.3333333333333333703, 0.3219752754296894559, 0.3333333333333333703, 0.3219752754296894559, 0.3333333333333333703, 0.3219752754296894559, 0.3333333333333333703, 0.3219752754296894559, 0.3333333333333333703, 0.3219752754296894559, 0.3333333333333333703, 0.3219752754296894559, 0.3333333333333333703, 0.3219752754296894559, 0.3333333333333333703, 0.3219752754296894559, 0.3333333333333333703, 0.3219752754296894559, 0.3333333333333333703, 0.3219752754296894559, 0.3333333333333333703, 0.3219752754296894559, 0.3333333333333333703, 0.3219752754296894559, 0.3333333333333333703, 0.3219752754296894559, 0.3333333333333333703, 0.3219752754296894559, 0.3333333333333333703, 0.3219752754296894559, 0.3333333333333333703, 0.3219752754296894559, 0.3333333333333333703, 0.3219752754296894559, 0.3333333333333333703, 0.3219752754296894559, 0.3333333333333333703, 0.3219752754296894559, 0.3333333333333333703, 0.3219752754296894559, 0.3333333333333333703, 0.3219752754296894559, 0.3333333333333333703, 0.3219752754296894559, 0.3333333333333333703, 0.3219752754296894559, 0.3333333333333333703, 0.3219752754296894559, 0.3333333333333333703, 0.3219752754296894559, 0.3333333333333333703, 0.3219752754296894559, 0.3333333333333333703, 0.3219752754296894559, 0.3333333333333333703, 0.3219752754296894559, 0.3333333333333333703, 0.3219752754296894559, 0.3333333333333333703, 0.3219752754296894559, 0.3333333333333333703, 0.3219752754296894559, 0.3333333333333333703, 0.3219752754296894559, 0.3333333333333333703, 0.3219752754296894559, 0.3333333333333333703, 0.3219752754296894559, 0.3333333333333333703, 0.3219752754296894559, 0.3333333333333333703, 0.3219752754296894559, 0.3333333333333333703, 0.3219752754296894559, 0.3333333333333333703, 0.3219752754296894559, 0.3333333333333333703, 0.3219752754296894559, 0.3333333333333333703, 0.3219752754296894559, 0.3333333333333333703, 0.3219752754296894559, 0.3333333333333333703, 0.3219752754296894559, 0.3333333333333333703, 0.3219752754296894559, 0.3333333333333333703, 0.3219752754296894559, 0.3333333333333333703, 0.3219752754296894559, 0.3333333333333333703, 0.3219752754296894559, 0.3333333333333333703, 0.3219752754296894559, 0.3333333333333333703, 0.3219752754296894559, 0.3333333333333333703, 0.3219752754296894559, 0.3333333333333333703, 0.3219752754296894559, 0.3333333333333333703, 0.3219752754296894559, 0.3333333333333333703, 0.3219752754296894559, 0.3333333333333333703, 0.3219752754296894559, 0.3333333333333333703, 0.3219752754296894559, 0.3333333333333333703, 0.3219752754296894559, 0.3333333333333333703, 0.3219752754296894559, 0.3333333333333333703, 0.3219752754296894559, 0.3333333333333333703, 0.3219752754296894559, 0.3333333333333333703, 0.3219752754296894559, 0.3333333333333333703, 0.3219752754296894559, 0.3333333333333333703, 0.3219752754296894559, 0.3333333333333333703, 0.3219752754296894559, 0.3333333333333333703, 0.3219752754296894559, 0.3333333333333333703, 0.3219752754296894559, 0.3333333333333333703, 0.3219752754296894559, 0.3333333333333333703, 0.3219752754296894559, 0.3333333333333333703, 0.3219752754296894559, 0.3333333333333333703, 0.3219752754296894559, 0.3333333333333333703, 0.3219752754296894559, 0.3333333333333333703, 0.3219752754296894559, 0.3333333333333333703, 0.3219752754296894559, 0.3333333333333333703, 0.3219752754296894559, 0.3333333333333333703, 0.3219752754296894559, 0.3333333333333333703, 0.3219752754296894559, 0.3333333333333333703, 0.3219752754296894559, 0.3333333333333333703, 0.3219752754296894559, 0.3333333333333333703, 0.3219752754296894559, 0.3333333333333333703, 0.3219752754296894559, 0.3333333333333333703, 0.3219752754296894559, 0.3333333333333333703, 0.3219752754296894559, 0.3333333333333333703, 0.3219752754296894559, 0.3333333333333333703, 0.3219752754296894559, 0.3333333333333333703, 0.3219752754296894559, 0.3333333333333333703, 0.3219752754296894559, 0.3333333333333333703, 0.3219752754296894559, 0.3333333333333333703, 0.3219752754296894559, 0.3333333333333333703, 0.3219752754296894559, 0.3333333333333333703, 0.3219752754296894559, 0.3333333333333333703, 0.3219752754296894559, 0.3333333333333333703, 0.3219752754296894559, 0.3333333333333333703, 0.3219752754296894559, 0.3333333333333333703, 0.3219752754296894559, 0.3333333333333333703, 0.3219752754296894559, 0.3333333333333333703, 0.3219752754296894559, 0.3333333333333333703, 0.3219752754296894559, 0.3333333333333333703, 0.3219752754296894559, 0.3333333333333333703, 0.3219752754296894559, 0.3333333333333333703, 0.3219752754296894559, 0.3333333333333333703, 0.3219752754296894559, 0.3333333333333333703, 0.3219752754296894559, 0.3333333333333333703, 0.3219752754296894559, 0.3333333333333333703, 0.3219752754296894559, 0.3333333333333333703, 0.3219752754296894559, 0.3333333333333333703, 0.3219752754296894559, 0.3333333333333333703, 0.3219752754296894559, 0.3333333333333333703, 0.3219752754296894559, 0.3333333333333333703, 0.3219752754296894559, 0.3333333333333333703, 0.3219752754296894559, 0.3333333333333333703, 0.3219752754296894559, 0.3333333333333333703, 0.3219752754296894559, 0.3333333333333333703, 0.3219752754296894559, 0.3333333333333333703, 0.3219752754296894559, 0.3333333333333333703, 0.3219752754296894559, 0.3333333333333333703, 0.3219752754296894559, 0.3333333333333333703, 0.3219752754296894559, 0.3333333333333333703, 0.3219752754296894559, 0.3333333333333333703, 0.3219752754296894559, 0.3333333333333333703, 0.3219752754296894559, 0.3333333333333333703),
 ( 0.3333333333333333703, 0.3219752754296894559, 0.3333333333333333703, 0.3219752754296894559, 0.3333333333333333703, 0.3219752754296894559, 0.3333333333333333703, 0.3219752754296894559, 0.3333333333333333703, 0.3219752754296894559, 0.3333333333333333703, 0.3219752754296894559, 0.3333333333333333703, 0.3219752754296894559, 0.3333333333333333703, 0.3219752754296894559, 0.3333333333333333703, 0.3219752754296894559, 0.3333333333333333703, 0.3219752754296894559, 0.3333333333333333703, 0.3219752754296894559, 0.3333333333333333703, 0.3219752754296894559, 0.3333333333333333703, 0.3219752754296894559, 0.3333333333333333703, 0.3219752754296894559, 0.3333333333333333703, 0.3219752754296894559, 0.3333333333333333703, 0.3219752754296894559, 0.3333333333333333703, 0.3219752754296894559, 0.3333333333333333703, 0.3219752754296894559, 0.3333333333333333703, 0.3219752754296894559, 0.3333333333333333703, 0.3219752754296894559, 0.3333333333333333703, 0.3219752754296894559, 0.3333333333333333703, 0.3219752754296894559, 0.3333333333333333703, 0.3219752754296894559, 0.3333333333333333703, 0.3219752754296894559, 0.3333333333333333703, 0.3219752754296894559, 0.3333333333333333703, 0.3219752754296894559, 0.3333333333333333703, 0.3219752754296894559, 0.3333333333333333703, 0.3219752754296894559, 0.3333333333333333703, 0.3219752754296894559, 0.3333333333333333703, 0.3219752754296894559, 0.3333333333333333703, 0.3219752754296894559, 0.3333333333333333703, 0.3219752754296894559, 0.3333333333333333703, 0.3219752754296894559, 0.3333333333333333703, 0.3219752754296894559, 0.3333333333333333703, 0.3219752754296894559, 0.3333333333333333703, 0.3219752754296894559, 0.3333333333333333703, 0.3219752754296894559, 0.3333333333333333703, 0.3219752754296894559, 0.3333333333333333703, 0.3219752754296894559, 0.3333333333333333703, 0.3219752754296894559, 0.3333333333333333703, 0.3219752754296894559, 0.3333333333333333703, 0.3219752754296894559, 0.3333333333333333703, 0.3219752754296894559, 0.3333333333333333703, 0.3219752754296894559, 0.3333333333333333703, 0.3219752754296894559, 0.3333333333333333703, 0.3219752754296894559, 0.3333333333333333703, 0.3219752754296894559, 0.3333333333333333703, 0.3219752754296894559, 0.3333333333333333703, 0.3219752754296894559, 0.3333333333333333703, 0.3219752754296894559, 0.3333333333333333703, 0.3219752754296894559, 0.3333333333333333703, 0.3219752754296894559, 0.3333333333333333703, 0.3219752754296894559, 0.3333333333333333703, 0.3219752754296894559, 0.3333333333333333703, 0.3219752754296894559, 0.3333333333333333703, 0.3219752754296894559, 0.3333333333333333703, 0.3219752754296894559, 0.3333333333333333703, 0.3219752754296894559, 0.3333333333333333703, 0.3219752754296894559, 0.3333333333333333703, 0.3219752754296894559, 0.3333333333333333703, 0.3219752754296894559, 0.3333333333333333703, 0.3219752754296894559, 0.3333333333333333703, 0.3219752754296894559, 0.3333333333333333703, 0.3219752754296894559, 0.3333333333333333703, 0.3219752754296894559, 0.3333333333333333703, 0.3219752754296894559, 0.3333333333333333703, 0.3219752754296894559, 0.3333333333333333703, 0.3219752754296894559, 0.3333333333333333703, 0.3219752754296894559, 0.3333333333333333703, 0.3219752754296894559, 0.3333333333333333703, 0.3219752754296894559, 0.3333333333333333703, 0.3219752754296894559, 0.3333333333333333703, 0.3219752754296894559, 0.3333333333333333703, 0.3219752754296894559, 0.3333333333333333703, 0.3219752754296894559, 0.3333333333333333703, 0.3219752754296894559, 0.3333333333333333703, 0.3219752754296894559, 0.3333333333333333703, 0.3219752754296894559, 0.3333333333333333703, 0.3219752754296894559, 0.3333333333333333703, 0.3219752754296894559, 0.3333333333333333703, 0.3219752754296894559, 0.3333333333333333703, 0.3219752754296894559, 0.3333333333333333703, 0.3219752754296894559, 0.3333333333333333703, 0.3219752754296894559, 0.3333333333333333703, 0.3219752754296894559, 0.3333333333333333703, 0.3219752754296894559, 0.3333333333333333703, 0.3219752754296894559, 0.3333333333333333703, 0.3219752754296894559, 0.3333333333333333703, 0.3219752754296894559, 0.3333333333333333703, 0.3219752754296894559, 0.3333333333333333703, 0.3219752754296894559, 0.3333333333333333703, 0.3219752754296894559, 0.3333333333333333703, 0.3219752754296894559, 0.3333333333333333703, 0.3219752754296894559, 0.3333333333333333703, 0.3219752754296894559, 0.3333333333333333703, 0.3219752754296894559, 0.3333333333333333703, 0.3219752754296894559, 0.3333333333333333703, 0.3219752754296894559, 0.3333333333333333703, 0.3219752754296894559, 0.3333333333333333703, 0.3219752754296894559, 0.3333333333333333703, 0.3219752754296894559, 0.3333333333333333703, 0.3219752754296894559, 0.3333333333333333703, 0.3219752754296894559, 0.3333333333333333703, 0.3219752754296894559, 0.3333333333333333703, 0.3219752754296894559, 0.3333333333333333703, 0.3219752754296894559, 0.3333333333333333703, 0.3219752754296894559, 0.3333333333333333703, 0.3219752754296894559, 0.3333333333333333703, 0.3219752754296894559, 0.3333333333333333703, 0.3219752754296894559, 0.3333333333333333703, 0.3219752754296894559, 0.3333333333333333703, 0.3219752754296894559, 0.3333333333333333703, 0.3219752754296894559, 0.3333333333333333703, 0.3219752754296894559, 0.3333333333333333703, 0.3219752754296894559, 0.3333333333333333703, 0.3219752754296894559, 0.3333333333333333703, 0.3219752754296894559, 0.3333333333333333703, 0.3219752754296894559, 0.3333333333333333703, 0.3219752754296894559, 0.3333333333333333703, 0.3219752754296894559, 0.3333333333333333703, 0.3219752754296894559, 0.3333333333333333703, 0.3219752754296894559, 0.3333333333333333703, 0.3219752754296894559, 0.3333333333333333703, 0.3219752754296894559, 0.3333333333333333703, 0.3219752754296894559, 0.3333333333333333703, 0.3219752754296894559, 0.3333333333333333703, 0.3219752754296894559, 0.3333333333333333703, 0.3219752754296894559, 0.3333333333333333703, 0.3219752754296894559, 0.3333333333333333703, 0.3219752754296894559, 0.3333333333333333703, 0.3219752754296894559, 0.3333333333333333703, 0.3219752754296894559, 0.3333333333333333703, 0.3219752754296894559, 0.3333333333333333703, 0.3219752754296894559, 0.3333333333333333703, 0.3219752754296894559, 0.3333333333333333703, 0.3219752754296894559, 0.3333333333333333703, 0.3219752754296894559, 0.3333333333333333703, 0.3219752754296894559, 0.3333333333333333703, 0.3219752754296894559, 0.3333333333333333703, 0.3219752754296894559, 0.3333333333333333703, 0.3219752754296894559, 0.3333333333333333703, 0.3219752754296894559, 0.3333333333333333703, 0.3219752754296894559, 0.3333333333333333703, 0.3219752754296894559, 0.3333333333333333703, 0.3219752754296894559, 0.3333333333333333703, 0.3219752754296894559, 0.3333333333333333703, 0.3219752754296894559, 0.3333333333333333703, 0.3219752754296894559, 0.3333333333333333703, 0.3219752754296894559, 0.3333333333333333703, 0.3219752754296894559, 0.3333333333333333703, 0.3219752754296894559, 0.3333333333333333703, 0.3219752754296894559, 0.3333333333333333703, 0.3219752754296894559, 0.3333333333333333703, 0.3219752754296894559, 0.3333333333333333703, 0.3219752754296894559, 0.3333333333333333703, 0.3219752754296894559, 0.3333333333333333703, 0.3219752754296894559, 0.3333333333333333703, 0.3219752754296894559, 0.3333333333333333703, 0.3219752754296894559, 0.3333333333333333703, 0.3219752754296894559, 0.3333333333333333703, 0.3219752754296894559, 0.3333333333333333703, 0.3219752754296894559, 0.3333333333333333703, 0.3219752754296894559, 0.3333333333333333703, 0.3219752754296894559, 0.3333333333333333703, 0.3219752754296894559, 0.3333333333333333703, 0.3219752754296894559, 0.3333333333333333703, 0.3219752754296894559, 0.3333333333333333703, 0.3219752754296894559, 0.3333333333333333703, 0.3219752754296894559, 0.3333333333333333703, 0.3219752754296894559, 0.3333333333333333703, 0.3219752754296894559, 0.3333333333333333703, 0.3219752754296894559, 0.3333333333333333703, 0.3219752754296894559, 0.3333333333333333703, 0.3219752754296894559, 0.3333333333333333703, 0.3219752754296894559, 0.3333333333333333703, 0.3219752754296894559, 0.3333333333333333703, 0.3219752754296894559, 0.3333333333333333703, 0.3219752754296894559, 0.3333333333333333703, 0.3219752754296894559, 0.3333333333333333703, 0.3219752754296894559, 0.3333333333333333703, 0.3219752754296894559, 0.3333333333333333703, 0.3219752754296894559, 0.3333333333333333703, 0.3219752754296894559, 0.3333333333333333703, 0.3219752754296894559, 0.3333333333333333703, 0.3219752754296894559, 0.3333333333333333703, 0.3219752754296894559, 0.3333333333333333703, 0.3219752754296894559, 0.3333333333333333703, 0.3219752754296894559, 0.3333333333333333703, 0.3219752754296894559, 0.3333333333333333703, 0.3219752754296894559, 0.3333333333333333703, 0.3219752754296894559, 0.3333333333333333703, 0.3219752754296894559, 0.3333333333333333703, 0.3219752754296894559, 0.3333333333333333703, 0.3219752754296894559, 0.3333333333333333703, 0.3219752754296894559, 0.3333333333333333703, 0.3219752754296894559, 0.3333333333333333703, 0.3219752754296894559, 0.3333333333333333703, 0.3219752754296894559, 0.3333333333333333703, 0.3219752754296894559, 0.3333333333333333703, 0.3219752754296894559, 0.3333333333333333703, 0.3219752754296894559, 0.3333333333333333703, 0.3219752754296894559, 0.3333333333333333703, 0.3219752754296894559, 0.3333333333333333703, 0.3219752754296894559, 0.3333333333333333703, 0.3219752754296894559, 0.3333333333333333703, 0.3219752754296894559, 0.3333333333333333703, 0.3219752754296894559, 0.3333333333333333703, 0.3219752754296894559, 0.3333333333333333703, 0.3219752754296894559, 0.3333333333333333703, 0.3219752754296894559, 0.3333333333333333703, 0.3219752754296894559, 0.3333333333333333703, 0.3219752754296894559, 0.3333333333333333703, 0.3219752754296894559, 0.3333333333333333703, 0.3219752754296894559, 0.3333333333333333703, 0.3219752754296894559, 0.3333333333333333703, 0.3219752754296894559, 0.3333333333333333703, 0.3219752754296894559, 0.3333333333333333703, 0.3219752754296894559, 0.3333333333333333703, 0.3219752754296894559, 0.3333333333333333703, 0.3219752754296894559, 0.3333333333333333703, 0.3219752754296894559, 0.3333333333333333703, 0.3219752754296894559, 0.3333333333333333703, 0.3219752754296894559, 0.3333333333333333703, 0.3219752754296894559, 0.3333333333333333703, 0.3219752754296894559, 0.3333333333333333703, 0.3219752754296894559, 0.3333333333333333703, 0.3219752754296894559, 0.3333333333333333703, 0.3219752754296894559, 0.3333333333333333703),
 ( 1.000000000000000000, 0.9659258262890683122, 1.000000000000000000, 0.9659258262890683122, 1.000000000000000000, 0.9659258262890683122, 1.000000000000000000, 0.9659258262890683122, 1.000000000000000000, 0.9659258262890683122, 1.000000000000000000, 0.9659258262890683122, 1.000000000000000000, 0.9659258262890683122, 1.000000000000000000, 0.9659258262890683122, 1.000000000000000000, 0.9659258262890683122, 1.000000000000000000, 0.9659258262890683122, 1.000000000000000000, 0.9659258262890683122, 1.000000000000000000, 0.9659258262890683122, 1.000000000000000000, 0.9659258262890683122, 1.000000000000000000, 0.9659258262890683122, 1.000000000000000000, 0.9659258262890683122, 1.000000000000000000, 0.9659258262890683122, 1.000000000000000000, 0.9659258262890683122, 1.000000000000000000, 0.9659258262890683122, 1.000000000000000000, 0.9659258262890683122, 1.000000000000000000, 0.9659258262890683122, 1.000000000000000000, 0.9659258262890683122, 1.000000000000000000, 0.9659258262890683122, 1.000000000000000000, 0.9659258262890683122, 1.000000000000000000, 0.9659258262890683122, 1.000000000000000000, 0.9659258262890683122, 1.000000000000000000, 0.9659258262890683122, 1.000000000000000000, 0.9659258262890683122, 1.000000000000000000, 0.9659258262890683122, 1.000000000000000000, 0.9659258262890683122, 1.000000000000000000, 0.9659258262890683122, 1.000000000000000000, 0.9659258262890683122, 1.000000000000000000, 0.9659258262890683122, 1.000000000000000000, 0.9659258262890683122, 1.000000000000000000, 0.9659258262890683122, 1.000000000000000000, 0.9659258262890683122, 1.000000000000000000, 0.9659258262890683122, 1.000000000000000000, 0.9659258262890683122, 1.000000000000000000, 0.9659258262890683122, 1.000000000000000000, 0.9659258262890683122, 1.000000000000000000, 0.9659258262890683122, 1.000000000000000000, 0.9659258262890683122, 1.000000000000000000, 0.9659258262890683122, 1.000000000000000000, 0.9659258262890683122, 1.000000000000000000, 0.9659258262890683122, 1.000000000000000000, 0.9659258262890683122, 1.000000000000000000, 0.9659258262890683122, 1.000000000000000000, 0.9659258262890683122, 1.000000000000000000, 0.9659258262890683122, 1.000000000000000000, 0.9659258262890683122, 1.000000000000000000, 0.9659258262890683122, 1.000000000000000000, 0.9659258262890683122, 1.000000000000000000, 0.9659258262890683122, 1.000000000000000000, 0.9659258262890683122, 1.000000000000000000, 0.9659258262890683122, 1.000000000000000000, 0.9659258262890683122, 1.000000000000000000, 0.9659258262890683122, 1.000000000000000000, 0.9659258262890683122, 1.000000000000000000, 0.9659258262890683122, 1.000000000000000000, 0.9659258262890683122, 1.000000000000000000, 0.9659258262890683122, 1.000000000000000000, 0.9659258262890683122, 1.000000000000000000, 0.9659258262890683122, 1.000000000000000000, 0.9659258262890683122, 1.000000000000000000, 0.9659258262890683122, 1.000000000000000000, 0.9659258262890683122, 1.000000000000000000, 0.9659258262890683122, 1.000000000000000000, 0.9659258262890683122, 1.000000000000000000, 0.9659258262890683122, 1.000000000000000000, 0.9659258262890683122, 1.000000000000000000, 0.9659258262890683122, 1.000000000000000000, 0.9659258262890683122, 1.000000000000000000, 0.9659258262890683122, 1.000000000000000000, 0.9659258262890683122, 1.000000000000000000, 0.9659258262890683122, 1.000000000000000000, 0.9659258262890683122, 1.000000000000000000, 0.9659258262890683122, 1.000000000000000000, 0.9659258262890683122, 1.000000000000000000, 0.9659258262890683122, 1.000000000000000000, 0.9659258262890683122, 1.000000000000000000, 0.9659258262890683122, 1.000000000000000000, 0.9659258262890683122, 1.000000000000000000, 0.9659258262890683122, 1.000000000000000000, 0.9659258262890683122, 1.000000000000000000, 0.9659258262890683122, 1.000000000000000000, 0.9659258262890683122, 1.000000000000000000, 0.9659258262890683122, 1.000000000000000000, 0.9659258262890683122, 1.000000000000000000, 0.9659258262890683122, 1.000000000000000000, 0.9659258262890683122, 1.000000000000000000, 0.9659258262890683122, 1.000000000000000000, 0.9659258262890683122, 1.000000000000000000, 0.9659258262890683122, 1.000000000000000000, 0.9659258262890683122, 1.000000000000000000, 0.9659258262890683122, 1.000000000000000000, 0.9659258262890683122, 1.000000000000000000, 0.9659258262890683122, 1.000000000000000000, 0.9659258262890683122, 1.000000000000000000, 0.9659258262890683122, 1.000000000000000000, 0.9659258262890683122, 1.000000000000000000, 0.9659258262890683122, 1.000000000000000000, 0.9659258262890683122, 1.000000000000000000, 0.9659258262890683122, 1.000000000000000000, 0.9659258262890683122, 1.000000000000000000, 0.9659258262890683122, 1.000000000000000000, 0.9659258262890683122, 1.000000000000000000, 0.9659258262890683122, 1.000000000000000000, 0.9659258262890683122, 1.000000000000000000, 0.9659258262890683122, 1.000000000000000000, 0.9659258262890683122, 1.000000000000000000, 0.9659258262890683122, 1.000000000000000000, 0.9659258262890683122, 1.000000000000000000, 0.9659258262890683122, 1.000000000000000000, 0.9659258262890683122, 1.000000000000000000, 0.9659258262890683122, 1.000000000000000000, 0.9659258262890683122, 1.000000000000000000, 0.9659258262890683122, 1.000000000000000000, 0.9659258262890683122, 1.000000000000000000, 0.9659258262890683122, 1.000000000000000000, 0.9659258262890683122, 1.000000000000000000, 0.9659258262890683122, 1.000000000000000000, 0.9659258262890683122, 1.000000000000000000, 0.9659258262890683122, 1.000000000000000000, 0.9659258262890683122, 1.000000000000000000, 0.9659258262890683122, 1.000000000000000000, 0.9659258262890683122, 1.000000000000000000, 0.9659258262890683122, 1.000000000000000000, 0.9659258262890683122, 1.000000000000000000, 0.9659258262890683122, 1.000000000000000000, 0.9659258262890683122, 1.000000000000000000, 0.9659258262890683122, 1.000000000000000000, 0.9659258262890683122, 1.000000000000000000, 0.9659258262890683122, 1.000000000000000000, 0.9659258262890683122, 1.000000000000000000, 0.9659258262890683122, 1.000000000000000000, 0.9659258262890683122, 1.000000000000000000, 0.9659258262890683122, 1.000000000000000000, 0.9659258262890683122, 1.000000000000000000, 0.9659258262890683122, 1.000000000000000000, 0.9659258262890683122, 1.000000000000000000, 0.9659258262890683122, 1.000000000000000000, 0.9659258262890683122, 1.000000000000000000, 0.9659258262890683122, 1.000000000000000000, 0.9659258262890683122, 1.000000000000000000, 0.9659258262890683122, 1.000000000000000000, 0.9659258262890683122, 1.000000000000000000, 0.9659258262890683122, 1.000000000000000000, 0.9659258262890683122, 1.000000000000000000, 0.9659258262890683122, 1.000000000000000000, 0.9659258262890683122, 1.000000000000000000, 0.9659258262890683122, 1.000000000000000000, 0.9659258262890683122, 1.000000000000000000, 0.9659258262890683122, 1.000000000000000000, 0.9659258262890683122, 1.000000000000000000, 0.9659258262890683122, 1.000000000000000000, 0.9659258262890683122, 1.000000000000000000, 0.9659258262890683122, 1.000000000000000000, 0.9659258262890683122, 1.000000000000000000, 0.9659258262890683122, 1.000000000000000000, 0.9659258262890683122, 1.000000000000000000, 0.9659258262890683122, 1.000000000000000000, 0.9659258262890683122, 1.000000000000000000, 0.9659258262890683122, 1.000000000000000000, 0.9659258262890683122, 1.000000000000000000, 0.9659258262890683122, 1.000000000000000000, 0.9659258262890683122, 1.000000000000000000, 0.9659258262890683122, 1.000000000000000000, 0.9659258262890683122, 1.000000000000000000, 0.9659258262890683122, 1.000000000000000000, 0.9659258262890683122, 1.000000000000000000, 0.9659258262890683122, 1.000000000000000000, 0.9659258262890683122, 1.000000000000000000, 0.9659258262890683122, 1.000000000000000000, 0.9659258262890683122, 1.000000000000000000, 0.9659258262890683122, 1.000000000000000000, 0.9659258262890683122, 1.000000000000000000, 0.9659258262890683122, 1.000000000000000000, 0.9659258262890683122, 1.000000000000000000, 0.9659258262890683122, 1.000000000000000000, 0.9659258262890683122, 1.000000000000000000, 0.9659258262890683122, 1.000000000000000000, 0.9659258262890683122, 1.000000000000000000, 0.9659258262890683122, 1.000000000000000000, 0.9659258262890683122, 1.000000000000000000, 0.9659258262890683122, 1.000000000000000000, 0.9659258262890683122, 1.000000000000000000, 0.9659258262890683122, 1.000000000000000000, 0.9659258262890683122, 1.000000000000000000, 0.9659258262890683122, 1.000000000000000000, 0.9659258262890683122, 1.000000000000000000, 0.9659258262890683122, 1.000000000000000000, 0.9659258262890683122, 1.000000000000000000, 0.9659258262890683122, 1.000000000000000000, 0.9659258262890683122, 1.000000000000000000, 0.9659258262890683122, 1.000000000000000000, 0.9659258262890683122, 1.000000000000000000, 0.9659258262890683122, 1.000000000000000000, 0.9659258262890683122, 1.000000000000000000, 0.9659258262890683122, 1.000000000000000000, 0.9659258262890683122, 1.000000000000000000, 0.9659258262890683122, 1.000000000000000000, 0.9659258262890683122, 1.000000000000000000, 0.9659258262890683122, 1.000000000000000000, 0.9659258262890683122, 1.000000000000000000, 0.9659258262890683122, 1.000000000000000000, 0.9659258262890683122, 1.000000000000000000, 0.9659258262890683122, 1.000000000000000000, 0.9659258262890683122, 1.000000000000000000, 0.9659258262890683122, 1.000000000000000000, 0.9659258262890683122, 1.000000000000000000, 0.9659258262890683122, 1.000000000000000000, 0.9659258262890683122, 1.000000000000000000, 0.9659258262890683122, 1.000000000000000000, 0.9659258262890683122, 1.000000000000000000, 0.9659258262890683122, 1.000000000000000000, 0.9659258262890683122, 1.000000000000000000, 0.9659258262890683122, 1.000000000000000000, 0.9659258262890683122, 1.000000000000000000, 0.9659258262890683122, 1.000000000000000000, 0.9659258262890683122, 1.000000000000000000, 0.9659258262890683122, 1.000000000000000000, 0.9659258262890683122, 1.000000000000000000, 0.9659258262890683122, 1.000000000000000000, 0.9659258262890683122, 1.000000000000000000, 0.9659258262890683122, 1.000000000000000000, 0.9659258262890683122, 1.000000000000000000, 0.9659258262890683122, 1.000000000000000000, 0.9659258262890683122, 1.000000000000000000, 0.9659258262890683122, 1.000000000000000000) ) ) 
 REPRESENTATION_ITEM ( '' )  SURFACE ( )  );
#58788=CARTESIAN_POINT ( 'NONE',  ( 19.02544592524343514, -5.153800228976328945, 23.54057627198102054 ) ) ;
#58789=CARTESIAN_POINT ( 'NONE',  ( 5.049401038298161559, -19.05341960407611168, 57.70724293864769550 ) ) ;
#58790=CARTESIAN_POINT ( 'NONE',  ( -14.34966873604960291, -8.224510206698953496, 66.66557627198102409 ) ) ;
#58791=CARTESIAN_POINT ( 'NONE',  ( 14.34966873604960469, 8.224510206698951720, 34.16557627198102409 ) ) ;
#58792=CARTESIAN_POINT ( 'NONE',  ( -10.72451020669898014, 18.67979575497178502, 50.41557627198103120 ) ) ;
#58793=CARTESIAN_POINT ( 'NONE',  ( -19.02544592524342804, 5.153800228976336051, 46.04057627198101699 ) ) ;
#58794=CARTESIAN_POINT ( 'NONE',  ( -0.05219959533907301413, -21.53943276465977519, 62.49890960531436690 ) ) ;
#58795=CARTESIAN_POINT ( 'NONE',  ( 19.03943276465977164, 0.05219959533936151252, 46.25109039468566863 ) ) ;
#58797=CARTESIAN_POINT ( 'NONE',  ( -16.53943276465976808, 0.05219959533911058130, 46.24890960531435979 ) ) ;
#58798=CARTESIAN_POINT ( 'NONE',  ( -21.53943276465977519, 0.05219959533907696930, 26.24890960531435624 ) ) ;
#58800=ORIENTED_EDGE ( 'NONE', *, *, #15818, .F. ) ;
#58802=CARTESIAN_POINT ( 'NONE',  ( 8.314922557961029526, -14.29746914071037800, 75.41775706135233293 ) ) ;
#58803=CARTESIAN_POINT ( 'NONE',  ( 19.05341960407617918, -5.049401038297876454, 76.04275706135230450 ) ) ;
#58804=CARTESIAN_POINT ( 'NONE',  ( 8.224510206698953496, -14.34966873604960469, 52.91557627198103830 ) ) ;
#58806=CARTESIAN_POINT ( 'NONE',  ( 14.34966873604960469, 8.224510206698951720, 24.16557627198103120 ) ) ;
#58807=CARTESIAN_POINT ( 'NONE',  ( -19.05341960407611168, -5.049401038298163336, 51.45724293864770260 ) ) ;
#58808=CARTESIAN_POINT ( 'NONE',  ( 13.97604488694527802, 13.89961937509977652, 69.37390960531436690 ) ) ;
#58809=CARTESIAN_POINT ( 'NONE',  ( 13.97604488694527802, 13.89961937509977652, 34.37390960531436690 ) ) ;
#58810=CARTESIAN_POINT ( 'NONE',  ( 21.52544592524334988, 5.823673210054432836, 51.45942372801901854 ) ) ;
#58811=CARTESIAN_POINT ( 'NONE',  ( -19.02544592524342804, 5.153800228976336051, 76.04057627198102409 ) ) ;
#58813=CARTESIAN_POINT ( 'NONE',  ( 13.89961937509977652, -13.97604488694527269, 58.12390960531436690 ) ) ;
#58815=CARTESIAN_POINT ( 'NONE',  ( 5.719274019375991003, -21.55341960407610458, 37.70724293864769550 ) ) ;
#58816=CARTESIAN_POINT ( 'NONE',  ( 13.89961937509977652, -13.97604488694527269, 33.12390960531434558 ) ) ;
#58817=CARTESIAN_POINT ( 'NONE',  ( 15.80617190586746368, 15.72974639402197994, 44.37390960531435979 ) ) ;
#58818=CARTESIAN_POINT ( 'NONE',  ( -8.314922557961024197, 14.29746914071037800, 92.91775706135236135 ) ) ;
#58819=CARTESIAN_POINT ( 'NONE',  ( 5.153800228976615827, -19.02544592524334988, 25.20942372801900433 ) ) ;
#58820=CARTESIAN_POINT ( 'NONE',  ( -8.224510206698735004, -14.34966873604973081, 44.58442372801901854 ) ) ;
#58821=CARTESIAN_POINT ( 'NONE',  ( 12.14591786802327356, -12.06949235617739191, 85.62609039468568994 ) ) ;
#58822=CARTESIAN_POINT ( 'NONE',  ( 16.46253265017160672, -9.564922557960803928, 103.3322429386476955 ) ) ;
#58823=EDGE_CURVE ( 'NONE', #141307, #91492, #56224, .T. ) ;
#58824=CARTESIAN_POINT ( 'NONE',  ( -8.314922557961024197, 14.29746914071037800, 67.91775706135234714 ) ) ;
#58825=CARTESIAN_POINT ( 'NONE',  ( 14.34966873604972726, -8.224510206698740333, 35.83442372801901143 ) ) ;
#58826=CARTESIAN_POINT ( 'NONE',  ( -5.153800228976328057, -19.02544592524343514, 112.2905762719810099 ) ) ;
#58827=CARTESIAN_POINT ( 'NONE',  ( -12.06949235617739369, -12.14591786802326823, 19.37609039468568639 ) ) ;
#58828=CARTESIAN_POINT ( 'NONE',  ( 19.02544592524343514, -5.153800228976328945, 38.54057627198103120 ) ) ;
#58829=CARTESIAN_POINT ( 'NONE',  ( -18.62759615963255300, -10.81492255796106328, 24.16775706135235424 ) ) ;
#58830=CARTESIAN_POINT ( 'NONE',  ( -13.97604488694547697, 13.89961937509957934, 113.1260903946856757 ) ) ;
#58831=CARTESIAN_POINT ( 'NONE',  ( 12.14591786802327356, -12.06949235617739191, 105.6260903946856899 ) ) ;
#58833=CARTESIAN_POINT ( 'NONE',  ( 5.719274019375673035, 21.55341960407619339, 97.29275706135234714 ) ) ;
#58834=CARTESIAN_POINT ( 'NONE',  ( -16.46253265017146816, -9.564922557961047289, 94.16775706135233293 ) ) ;
#58835=CARTESIAN_POINT ( 'NONE',  ( -8.224510206698948167, 14.34966873604960824, 60.41557627198102409 ) ) ;
#58836=CARTESIAN_POINT ( 'NONE',  ( 19.02544592524343514, -5.153800228976328945, 23.54057627198102054 ) ) ;
#58837=CARTESIAN_POINT ( 'NONE',  ( 0.05219959533936267826, -19.03943276465977164, 65.00109039468567573 ) ) ;
#58838=CARTESIAN_POINT ( 'NONE',  ( 17.26172910966717211, -6.454744622556960465, 58.30646908649209337 ) ) ;
#58839=CARTESIAN_POINT ( 'NONE',  ( 10.81492255796106328, -18.62759615963255655, 55.41775706135234714 ) ) ;
#58840=CARTESIAN_POINT ( 'NONE',  ( 8.224510206698742110, 14.34966873604972548, 32.08442372801901854 ) ) ;
#58842=CARTESIAN_POINT ( 'NONE',  ( 5.049401038298161559, -19.05341960407611168, 112.7072429386476813 ) ) ;
#58843=CARTESIAN_POINT ( 'NONE',  ( 21.53943276465977519, -0.05219959533907433946, 78.74890960531436690 ) ) ;
#58844=CARTESIAN_POINT ( 'NONE',  ( -19.05341960407617563, 5.049401038297882671, 108.5427570613523187 ) ) ;
#58845=CARTESIAN_POINT ( 'NONE',  ( -0.05219959533909027116, -19.03943276465977164, 97.49890960531436690 ) ) ;
#58847=CARTESIAN_POINT ( 'NONE',  ( -13.97604488694527625, -13.89961937509977652, 31.87390960531435979 ) ) ;
#58848=CARTESIAN_POINT ( 'NONE',  ( 10.72451020669871369, 18.67979575497193778, 92.08442372801901854 ) ) ;
#58849=CARTESIAN_POINT ( 'NONE',  ( -13.89961937509977652, 13.97604488694528158, 40.62390960531435979 ) ) ;
#58850=CARTESIAN_POINT ( 'NONE',  ( 5.719274019375673035, 21.55341960407619339, 47.29275706135234003 ) ) ;
#58851=CARTESIAN_POINT ( 'NONE',  ( 5.719274019375673035, 21.55341960407619339, 92.29275706135236135 ) ) ;
#58852=CARTESIAN_POINT ( 'NONE',  ( 0.05219959533934541429, -16.53943276465976808, 100.0010903946857042 ) ) ;
#58853=CARTESIAN_POINT ( 'NONE',  ( 16.51473224551069308, 9.474510206698969483, 84.16557627198102409 ) ) ;
#58854=CARTESIAN_POINT ( 'NONE',  ( -21.55341960407619339, 5.719274019375674811, 38.54275706135234714 ) ) ;
#58855=CARTESIAN_POINT ( 'NONE',  ( 21.52544592524334988, 5.823673210054432836, 41.45942372801901143 ) ) ;
#58856=CARTESIAN_POINT ( 'NONE',  ( 0.05219959533936267826, -19.03943276465977164, 80.00109039468567573 ) ) ;
#58857=CARTESIAN_POINT ( 'NONE',  ( -0.05219959533909027116, -19.03943276465977164, 87.49890960531436690 ) ) ;
#58858=CARTESIAN_POINT ( 'NONE',  ( -14.29746914071049879, 8.314922557960819915, 105.8322429386476955 ) ) ;
#58860=CARTESIAN_POINT ( 'NONE',  ( -21.55341960407610458, -5.719274019375992779, 101.4572429386476955 ) ) ;
#58861=CARTESIAN_POINT ( 'NONE',  ( 16.53943276465976808, -0.05219959533910856209, 83.74890960531435269 ) ) ;
#58862=CARTESIAN_POINT ( 'NONE',  ( -19.05341960407617563, 5.049401038297882671, 23.54275706135233648 ) ) ;
#58863=CARTESIAN_POINT ( 'NONE',  ( -4.379528057220328563, 16.55341960407611168, 95.20724293864769550 ) ) ;
#58864=CARTESIAN_POINT ( 'NONE',  ( 5.153800228976335163, 19.02544592524342804, 39.79057627198100988 ) ) ;
#58865=CARTESIAN_POINT ( 'NONE',  ( -5.153800228976607833, 19.02544592524334988, 87.70942372801897591 ) ) ;
#58866=CARTESIAN_POINT ( 'NONE',  ( -14.34966873604960291, -8.224510206698953496, 46.66557627198102409 ) ) ;
#58867=CARTESIAN_POINT ( 'NONE',  ( -21.55341960407619339, 5.719274019375674811, 88.54275706135236135 ) ) ;
#58868=CARTESIAN_POINT ( 'NONE',  ( -19.03943276465977164, 0.05219959533909376836, 111.2489096053143669 ) ) ;
#58869=CARTESIAN_POINT ( 'NONE',  ( -5.153800228976607833, 19.02544592524334988, 72.70942372801900433 ) ) ;
#58870=CARTESIAN_POINT ( 'NONE',  ( 18.67979575497178502, 10.72451020669898547, 74.16557627198102409 ) ) ;
#58871=CARTESIAN_POINT ( 'NONE',  ( 10.81492255796106328, -18.62759615963255655, 25.41775706135235779 ) ) ;
#58872=CARTESIAN_POINT ( 'NONE',  ( -16.53943276465976808, -0.05219959533934237506, 28.75109039468567929 ) ) ;
#58873=CARTESIAN_POINT ( 'NONE',  ( -12.06949235617739369, -12.14591786802326823, 94.37609039468568994 ) ) ;
#58874=CARTESIAN_POINT ( 'NONE',  ( -16.46253265017160317, 9.564922557960807481, 25.83224293864769194 ) ) ;
#58875=CARTESIAN_POINT ( 'NONE',  ( 21.55341960407619695, -5.719274019375665929, 41.04275706135236135 ) ) ;
#58876=CARTESIAN_POINT ( 'NONE',  ( -4.379528057220328563, 16.55341960407611168, 115.2072429386476955 ) ) ;
#58878=CARTESIAN_POINT ( 'NONE',  ( -14.34966873604972548, 8.224510206698743886, 48.33442372801902565 ) ) ;
#58879=CARTESIAN_POINT ( 'NONE',  ( -14.34966873604960291, -8.224510206698953496, 81.66557627198103830 ) ) ;
#58880=CARTESIAN_POINT ( 'NONE',  ( -15.80617190586745835, -15.72974639402198527, 71.87390960531438111 ) ) ;
#58881=CARTESIAN_POINT ( 'NONE',  ( -14.34966873604960291, -8.224510206698953496, 21.66557627198102409 ) ) ;
#58882=CARTESIAN_POINT ( 'NONE',  ( -12.06949235617739369, -12.14591786802326823, 54.37609039468568994 ) ) ;
#58883=CARTESIAN_POINT ( 'NONE',  ( -5.049401038298153566, 19.05341960407611168, 50.20724293864770260 ) ) ;
#58884=CARTESIAN_POINT ( 'NONE',  ( 16.55341960407618274, -4.379528057220086978, 96.04275706135236135 ) ) ;
#58885=CARTESIAN_POINT ( 'NONE',  ( 9.474510206698729675, 16.51473224551082808, 92.08442372801900433 ) ) ;
#58886=CARTESIAN_POINT ( 'NONE',  ( -21.52544592524343514, 5.823673210054127303, 91.04057627198103830 ) ) ;
#58887=CARTESIAN_POINT ( 'NONE',  ( 12.14591786802327356, -12.06949235617739191, 110.6260903946857042 ) ) ;
#58888=ORIENTED_EDGE ( 'NONE', *, *, #29212, .T. ) ;
#58890=CARTESIAN_POINT ( 'NONE',  ( 10.81492255796078972, 18.62759615963270932, 64.58224293864769550 ) ) ;
#58892=CARTESIAN_POINT ( 'NONE',  ( 16.52544592524335698, 4.483927247898782831, 86.45942372801901854 ) ) ;
#58893=ORIENTED_EDGE ( 'NONE', *, *, #20020, .T. ) ;
#58894=CARTESIAN_POINT ( 'NONE',  ( -18.67979575497178146, -10.72451020669898902, 36.66557627198103120 ) ) ;
#58895=CARTESIAN_POINT ( 'NONE',  ( 17.50000000000000000, 5.499999999999995559, 108.7823096230356867 ) ) ;
#58896=CARTESIAN_POINT ( 'NONE',  ( 21.55341960407610458, 5.719274019375980345, 73.95724293864769550 ) ) ;
#58897=CARTESIAN_POINT ( 'NONE',  ( -12.14591786802309592, -12.06949235617757132, 21.87390960531436690 ) ) ;
#58898=CARTESIAN_POINT ( 'NONE',  ( -8.314922557961024197, 14.29746914071037800, 27.91775706135234358 ) ) ;
#58899=CARTESIAN_POINT ( 'NONE',  ( -5.153800228976328057, -19.02544592524343514, 37.29057627198102409 ) ) ;
#58900=CARTESIAN_POINT ( 'NONE',  ( 4.483927247898790824, -16.52544592524335698, 35.20942372801901854 ) ) ;
#58901=CARTESIAN_POINT ( 'NONE',  ( -19.02544592524342804, 5.153800228976336051, 56.04057627198100988 ) ) ;
#58903=CARTESIAN_POINT ( 'NONE',  ( 19.03943276465977164, -0.05219959533909143690, 103.7489096053143669 ) ) ;
#58904=CARTESIAN_POINT ( 'NONE',  ( -19.02544592524342804, 5.153800228976336051, 101.0405762719810241 ) ) ;
#58905=CARTESIAN_POINT ( 'NONE',  ( -4.379528057220086978, -16.55341960407618274, 84.79275706135234714 ) ) ;
#58906=CARTESIAN_POINT ( 'NONE',  ( -9.564922557961040184, 16.46253265017147172, 92.91775706135233293 ) ) ;
#58907=CARTESIAN_POINT ( 'NONE',  ( 16.51473224551083163, -9.474510206698727899, 40.83442372801900433 ) ) ;
#58908=CARTESIAN_POINT ( 'NONE',  ( 5.823673210054125526, 21.52544592524343514, 79.79057627198102409 ) ) ;
#58909=CARTESIAN_POINT ( 'NONE',  ( 8.314922557961029526, -14.29746914071037800, 95.41775706135234714 ) ) ;
#58910=CARTESIAN_POINT ( 'NONE',  ( 21.53943276465977519, -0.05219959533907433946, 28.74890960531435624 ) ) ;
#58911=CARTESIAN_POINT ( 'NONE',  ( 16.51473224551083163, -9.474510206698727899, 95.83442372801900433 ) ) ;
#58912=CARTESIAN_POINT ( 'NONE',  ( 5.153800228976335163, 19.02544592524342804, 44.79057627198103830 ) ) ;
#58913=CARTESIAN_POINT ( 'NONE',  ( -16.51473224551069308, -9.474510206698971260, 91.66557627198103830 ) ) ;
#58914=CARTESIAN_POINT ( 'NONE',  ( -10.72451020669870658, -18.67979575497194134, 59.58442372801901854 ) ) ;
#58915=CARTESIAN_POINT ( 'NONE',  ( -16.46253265017160317, 9.564922557960807481, 55.83224293864769550 ) ) ;
#58916=CARTESIAN_POINT ( 'NONE',  ( -14.34966873604960291, -8.224510206698953496, 81.66557627198103830 ) ) ;
#58917=CARTESIAN_POINT ( 'NONE',  ( -16.21995358207302118, -7.366697692864224933, 85.06448998487842061 ) ) ;
#58918=CARTESIAN_POINT ( 'NONE',  ( 12.06949235617757843, -12.14591786802309237, 83.12390960531436690 ) ) ;
#58919=CARTESIAN_POINT ( 'NONE',  ( 18.67979575497178502, 10.72451020669898547, 74.16557627198102409 ) ) ;
#58920=CARTESIAN_POINT ( 'NONE',  ( 9.564922557961047289, -16.46253265017146816, 95.41775706135233293 ) ) ;
#58922=CARTESIAN_POINT ( 'NONE',  ( -13.97604488694547697, 13.89961937509957934, 38.12609039468566152 ) ) ;
#58923=CARTESIAN_POINT ( 'NONE',  ( 16.29526858892906915, -7.335722546920036002, 71.70329402199735114 ) ) ;
#58924=CARTESIAN_POINT ( 'NONE',  ( -16.46253265017160317, 9.564922557960807481, 75.83224293864769550 ) ) ;
#58925=CARTESIAN_POINT ( 'NONE',  ( 19.02544592524343514, -5.153800228976328945, 93.54057627198102409 ) ) ;
#58926=CARTESIAN_POINT ( 'NONE',  ( 14.29746914071037800, 8.314922557961029526, 61.66775706135235424 ) ) ;
#58928=CARTESIAN_POINT ( 'NONE',  ( -13.97604488694547697, 13.89961937509957934, 38.12609039468566152 ) ) ;
#58929=CARTESIAN_POINT ( 'NONE',  ( 17.06703543724471217, 6.729882984710979343, 21.75716082082560021 ) ) ;
#58930=CARTESIAN_POINT ( 'NONE',  ( 9.564922557960805705, 16.46253265017160317, 109.5822429386476955 ) ) ;
#58931=CARTESIAN_POINT ( 'NONE',  ( 12.06949235617739724, 12.14591786802326823, 106.8760903946856899 ) ) ;
#58933=CARTESIAN_POINT ( 'NONE',  ( 14.34966873604972726, -8.224510206698740333, 75.83442372801900433 ) ) ;
#58935=CARTESIAN_POINT ( 'NONE',  ( -12.06949235617739369, -12.14591786802326823, 59.37609039468568284 ) ) ;
#58936=CARTESIAN_POINT ( 'NONE',  ( 5.153800228976335163, 19.02544592524342804, 74.79057627198103830 ) ) ;
#58937=CARTESIAN_POINT ( 'NONE',  ( -18.67979575497193778, 10.72451020669871902, 73.33442372801901854 ) ) ;
#58938=CARTESIAN_POINT ( 'NONE',  ( 0.05219959533936267826, -19.03943276465977164, 70.00109039468566152 ) ) ;
#58939=CARTESIAN_POINT ( 'NONE',  ( 19.03943276465977164, 0.05219959533936151252, 21.25109039468565797 ) ) ;
#58940=CARTESIAN_POINT ( 'NONE',  ( -13.97604488694527625, -13.89961937509977652, 51.87390960531436690 ) ) ;
#58941=CARTESIAN_POINT ( 'NONE',  ( -13.89961937509977652, 13.97604488694528158, 45.62390960531433848 ) ) ;
#58943=CARTESIAN_POINT ( 'NONE',  ( 15.80617190586746368, 15.72974639402197994, 74.37390960531436690 ) ) ;
#58944=EDGE_CURVE ( 'NONE', #188641, #13916, #66610, .T. ) ;
#58945=CARTESIAN_POINT ( 'NONE',  ( 5.719274019375991003, -21.55341960407610458, 32.70724293864770260 ) ) ;
#58946=CARTESIAN_POINT ( 'NONE',  ( 14.34966873604960469, 8.224510206698951720, 114.1655762719810383 ) ) ;
#58947=CARTESIAN_POINT ( 'NONE',  ( -16.52544592524335698, -4.483927247898792601, 53.95942372801900433 ) ) ;
#58949=CARTESIAN_POINT ( 'NONE',  ( 5.719274019375673035, 21.55341960407619339, 37.29275706135235424 ) ) ;
#58950=CARTESIAN_POINT ( 'NONE',  ( 8.224510206698953496, -14.34966873604960469, 47.91557627198102409 ) ) ;
#58952=CARTESIAN_POINT ( 'NONE',  ( 16.55341960407618274, -4.379528057220086978, 26.04275706135235779 ) ) ;
#58953=CARTESIAN_POINT ( 'NONE',  ( 19.05341960407617918, -5.049401038297876454, 46.04275706135233293 ) ) ;
#58954=CARTESIAN_POINT ( 'NONE',  ( 4.379528057220339221, -16.55341960407611168, 47.70724293864770260 ) ) ;
#58955=CARTESIAN_POINT ( 'NONE',  ( -18.62759615963255300, -10.81492255796106328, 24.16775706135235424 ) ) ;
#58956=CARTESIAN_POINT ( 'NONE',  ( 9.564922557960805705, 16.46253265017160317, 99.58224293864770971 ) ) ;
#58957=CARTESIAN_POINT ( 'NONE',  ( 18.67979575497178502, 10.72451020669898547, 79.16557627198103830 ) ) ;
#58958=CARTESIAN_POINT ( 'NONE',  ( 5.153800228976335163, 19.02544592524342804, 89.79057627198102409 ) ) ;
#58959=CARTESIAN_POINT ( 'NONE',  ( 12.06949235617757843, -12.14591786802309237, 63.12390960531435979 ) ) ;
#58960=CARTESIAN_POINT ( 'NONE',  ( -16.46253265017160317, 9.564922557960807481, 105.8322429386476955 ) ) ;
#58962=CARTESIAN_POINT ( 'NONE',  ( 5.049401038297881783, 19.05341960407617563, 52.29275706135234003 ) ) ;
#58963=CARTESIAN_POINT ( 'NONE',  ( -15.80617190586745835, -15.72974639402198527, 111.8739096053143669 ) ) ;
#58964=CARTESIAN_POINT ( 'NONE',  ( 19.03943276465977164, -0.05219959533909143690, 48.74890960531435979 ) ) ;
#58965=CARTESIAN_POINT ( 'NONE',  ( -14.34966873604960291, -8.224510206698953496, 106.6655762719810383 ) ) ;
#58966=CARTESIAN_POINT ( 'NONE',  ( 21.55341960407619695, -5.719274019375665929, 51.04275706135234714 ) ) ;
#58968=CARTESIAN_POINT ( 'NONE',  ( 4.483927247898545687, 16.52544592524342804, 34.79057627198103120 ) ) ;
#58969=CARTESIAN_POINT ( 'NONE',  ( 13.89961937509977652, -13.97604488694527269, 43.12390960531434558 ) ) ;
#58970=CARTESIAN_POINT ( 'NONE',  ( 9.564922557960805705, 16.46253265017160317, 104.5822429386476955 ) ) ;
#58971=CARTESIAN_POINT ( 'NONE',  ( 15.80617190586746368, 15.72974639402197994, 79.37390960531436690 ) ) ;
#58973=CARTESIAN_POINT ( 'NONE',  ( -13.97604488694527625, -13.89961937509977652, 46.87390960531435979 ) ) ;
#58974=CARTESIAN_POINT ( 'NONE',  ( -21.52544592524343514, 5.823673210054127303, 71.04057627198103830 ) ) ;
#58975=ADVANCED_FACE ( 'NONE', ( #14696 ), #167397, .F. ) ;
#58976=CARTESIAN_POINT ( 'NONE',  ( 15.80617190586769283, -15.72974639402175789, 90.62609039468567573 ) ) ;
#58978=CARTESIAN_POINT ( 'NONE',  ( -8.224510206698735004, -14.34966873604973081, 79.58442372801903275 ) ) ;
#58979=CARTESIAN_POINT ( 'NONE',  ( 0.05219959533910956823, 16.53943276465976808, 69.99890960531435269 ) ) ;
#58980=CARTESIAN_POINT ( 'NONE',  ( 5.049401038298161559, -19.05341960407611168, 72.70724293864768129 ) ) ;
#58982=CARTESIAN_POINT ( 'NONE',  ( -9.474510206698720793, -16.51473224551083518, 29.58442372801900433 ) ) ;
#58983=CARTESIAN_POINT ( 'NONE',  ( -16.53943276465976808, -0.05219959533934237506, 93.75109039468567573 ) ) ;
#58984=CARTESIAN_POINT ( 'NONE',  ( 10.72451020669871369, 18.67979575497193778, 112.0844237280190185 ) ) ;
#58985=CARTESIAN_POINT ( 'NONE',  ( -9.564922557960796823, -16.46253265017161027, 72.08224293864770971 ) ) ;
#58986=CARTESIAN_POINT ( 'NONE',  ( 21.53943276465977519, -0.05219959533907433946, 48.74890960531435979 ) ) ;
#58987=CARTESIAN_POINT ( 'NONE',  ( 14.29746914071037800, 8.314922557961029526, 26.66775706135235424 ) ) ;
#58988=CARTESIAN_POINT ( 'NONE',  ( 5.823673210054444382, -21.52544592524334988, 90.20942372801903275 ) ) ;
#58989=CARTESIAN_POINT ( 'NONE',  ( 16.53943276465976808, 0.05219959533934440121, 56.25109039468568284 ) ) ;
#58990=CARTESIAN_POINT ( 'NONE',  ( -21.52544592524334988, -5.823673210054445271, 18.95942372801901143 ) ) ;
#58991=CARTESIAN_POINT ( 'NONE',  ( -16.55341960407617563, 4.379528057220093196, 23.54275706135235424 ) ) ;
#58992=CARTESIAN_POINT ( 'NONE',  ( -0.05219959533909027116, -19.03943276465977164, 87.49890960531436690 ) ) ;
#58994=CARTESIAN_POINT ( 'NONE',  ( 16.53943276465976808, 0.05219959533934440121, 31.25109039468568639 ) ) ;
#58995=CARTESIAN_POINT ( 'NONE',  ( 0.05219959533909260263, 19.03943276465977164, 54.99890960531435979 ) ) ;
#58996=CARTESIAN_POINT ( 'NONE',  ( 8.224510206698742110, 14.34966873604972548, 32.08442372801901854 ) ) ;
#58997=CARTESIAN_POINT ( 'NONE',  ( 4.379528057220339221, -16.55341960407611168, 77.70724293864770971 ) ) ;
#58998=CARTESIAN_POINT ( 'NONE',  ( -4.483927247898782831, 16.52544592524335698, 82.70942372801900433 ) ) ;
#58999=CARTESIAN_POINT ( 'NONE',  ( 21.52544592524334988, 5.823673210054432836, 46.45942372801901854 ) ) ;
#59000=CARTESIAN_POINT ( 'NONE',  ( 19.03943276465977164, -0.05219959533909143690, 58.74890960531435979 ) ) ;
#59001=CARTESIAN_POINT ( 'NONE',  ( 13.89961937509977652, -13.97604488694527269, 83.12390960531436690 ) ) ;
#59002=CARTESIAN_POINT ( 'NONE',  ( 4.379528057220092307, 16.55341960407617563, 82.29275706135234714 ) ) ;
#59005=CARTESIAN_POINT ( 'NONE',  ( 16.51473224551083163, -9.474510206698727899, 35.83442372801899722 ) ) ;
#59006=CARTESIAN_POINT ( 'NONE',  ( 19.03943276465977164, -0.05219959533909143690, 93.74890960531435269 ) ) ;
#59007=CARTESIAN_POINT ( 'NONE',  ( -16.46253265017160317, 9.564922557960807481, 55.83224293864769550 ) ) ;
#59009=CARTESIAN_POINT ( 'NONE',  ( -12.06949235617739369, -12.14591786802326823, 49.37609039468569705 ) ) ;
#59010=CARTESIAN_POINT ( 'NONE',  ( -9.474510206698720793, -16.51473224551083518, 64.58442372801900433 ) ) ;
#59011=CARTESIAN_POINT ( 'NONE',  ( -0.05219959533934338120, 16.53943276465976808, 57.50109039468568994 ) ) ;
#59013=CARTESIAN_POINT ( 'NONE',  ( 5.049401038298161559, -19.05341960407611168, 77.70724293864765286 ) ) ;
#59014=CARTESIAN_POINT ( 'NONE',  ( -18.62759615963270932, 10.81492255796079327, 100.8322429386477097 ) ) ;
#59015=CARTESIAN_POINT ( 'NONE',  ( 16.51473224551083163, -9.474510206698727899, 60.83442372801900433 ) ) ;
#59016=CARTESIAN_POINT ( 'NONE',  ( 16.46253265017160672, -9.564922557960803928, 88.33224293864769550 ) ) ;
#59017=CARTESIAN_POINT ( 'NONE',  ( -9.474510206698964154, 16.51473224551069663, 25.41557627198103120 ) ) ;
#59018=CARTESIAN_POINT ( 'NONE',  ( -16.51473224551069308, -9.474510206698971260, 81.66557627198103830 ) ) ;
#59019=CARTESIAN_POINT ( 'NONE',  ( 8.224510206698953496, -14.34966873604960469, 37.91557627198102409 ) ) ;
#59020=CARTESIAN_POINT ( 'NONE',  ( 19.03943276465977164, -0.05219959533909143690, 23.74890960531435269 ) ) ;
#59021=CARTESIAN_POINT ( 'NONE',  ( -19.02544592524334988, -5.153800228976617603, 43.95942372801899012 ) ) ;
#59022=CARTESIAN_POINT ( 'NONE',  ( 16.55341960407611168, 4.379528057220329451, 68.95724293864769550 ) ) ;
#59023=CARTESIAN_POINT ( 'NONE',  ( -21.53943276465977519, -0.05219959533937600094, 103.7510903946857042 ) ) ;
#59024=CARTESIAN_POINT ( 'NONE',  ( -19.02544592524342804, 5.153800228976336051, 46.04057627198101699 ) ) ;
#59025=CARTESIAN_POINT ( 'NONE',  ( 0.05219959533910956823, 16.53943276465976808, 34.99890960531435979 ) ) ;
#59026=CARTESIAN_POINT ( 'NONE',  ( -18.67979575497193778, 10.72451020669871902, 98.33442372801901854 ) ) ;
#59027=CARTESIAN_POINT ( 'NONE',  ( -5.049401038298153566, 19.05341960407611168, 95.20724293864770971 ) ) ;
#59028=CARTESIAN_POINT ( 'NONE',  ( 19.02544592524343514, -5.153800228976328945, 93.54057627198102409 ) ) ;
#59029=CARTESIAN_POINT ( 'NONE',  ( 9.474510206698971260, -16.51473224551069308, 37.91557627198102409 ) ) ;
#59030=CARTESIAN_POINT ( 'NONE',  ( -12.14591786802309592, -12.06949235617757132, 101.8739096053143811 ) ) ;
#59031=CARTESIAN_POINT ( 'NONE',  ( 0.05219959533910956823, 16.53943276465976808, 69.99890960531435269 ) ) ;
#59032=CARTESIAN_POINT ( 'NONE',  ( 21.55341960407610458, 5.719274019375980345, 88.95724293864769550 ) ) ;
#59033=CARTESIAN_POINT ( 'NONE',  ( -19.05341960407611168, -5.049401038298163336, 91.45724293864766707 ) ) ;
#59034=CARTESIAN_POINT ( 'NONE',  ( -10.81492255796078084, -18.62759615963271287, 92.08224293864769550 ) ) ;
#59035=CARTESIAN_POINT ( 'NONE',  ( -9.474510206698964154, 16.51473224551069663, 90.41557627198103830 ) ) ;
#59036=LINE ( 'NONE', #63002, #168771 ) ;
#59037=CARTESIAN_POINT ( 'NONE',  ( 16.52544592524342804, -4.483927247898539470, 88.54057627198103830 ) ) ;
#59038=CARTESIAN_POINT ( 'NONE',  ( -19.02544592524342804, 5.153800228976336051, 66.04057627198103830 ) ) ;
#59039=CARTESIAN_POINT ( 'NONE',  ( 21.55341960407610458, 5.719274019375980345, 78.95724293864769550 ) ) ;
#59041=CARTESIAN_POINT ( 'NONE',  ( -21.52544592524343514, 5.823673210054127303, 31.04057627198102409 ) ) ;
#59043=CARTESIAN_POINT ( 'NONE',  ( -16.46253265017146816, -9.564922557961047289, 109.1677570613523471 ) ) ;
#59044=CARTESIAN_POINT ( 'NONE',  ( -4.483927247898539470, -16.52544592524342804, 97.29057627198105251 ) ) ;
#59045=CARTESIAN_POINT ( 'NONE',  ( -17.26058549869092218, -6.457015423128487974, 96.37745837476067834 ) ) ;
#59046=CARTESIAN_POINT ( 'NONE',  ( 13.89961937509977652, -13.97604488694527269, 88.12390960531438111 ) ) ;
#59047=CARTESIAN_POINT ( 'NONE',  ( 9.474510206698971260, -16.51473224551069308, 42.91557627198103120 ) ) ;
#59048=CARTESIAN_POINT ( 'NONE',  ( -14.34966873604960291, -8.224510206698953496, 76.66557627198103830 ) ) ;
#59049=CARTESIAN_POINT ( 'NONE',  ( -5.049401038298153566, 19.05341960407611168, 110.2072429386476671 ) ) ;
#59050=CARTESIAN_POINT ( 'NONE',  ( 0.05219959533910956823, 16.53943276465976808, 54.99890960531435269 ) ) ;
#59051=CARTESIAN_POINT ( 'NONE',  ( 16.46253265017146816, 9.564922557961045513, 106.6677570613523471 ) ) ;
#59052=CARTESIAN_POINT ( 'NONE',  ( -21.52544592524334988, -5.823673210054445271, 53.95942372801900433 ) ) ;
#59053=CARTESIAN_POINT ( 'NONE',  ( 16.51473224551069308, 9.474510206698969483, 104.1655762719810241 ) ) ;
#59054=CARTESIAN_POINT ( 'NONE',  ( -5.823673210054116645, -21.52544592524344225, 87.29057627198103830 ) ) ;
#59055=CARTESIAN_POINT ( 'NONE',  ( 12.06949235617739724, 12.14591786802326823, 81.87609039468568994 ) ) ;
#59056=CARTESIAN_POINT ( 'NONE',  ( -19.02544592524342804, 5.153800228976336051, 31.04057627198102409 ) ) ;
#59057=CARTESIAN_POINT ( 'NONE',  ( -13.89961937509977652, 13.97604488694528158, 70.62390960531432427 ) ) ;
#59058=CARTESIAN_POINT ( 'NONE',  ( -10.72451020669898014, 18.67979575497178502, 80.41557627198103830 ) ) ;
#59059=CARTESIAN_POINT ( 'NONE',  ( 19.03943276465977164, 0.05219959533936151252, 111.2510903946856757 ) ) ;
#59060=CARTESIAN_POINT ( 'NONE',  ( 14.29746914071049879, -8.314922557960816363, 53.33224293864769550 ) ) ;
#59061=CARTESIAN_POINT ( 'NONE',  ( 5.719274019375673035, 21.55341960407619339, 62.29275706135236845 ) ) ;
#59062=CARTESIAN_POINT ( 'NONE',  ( 0.05219959533934541429, -16.53943276465976808, 80.00109039468568994 ) ) ;
#59063=CARTESIAN_POINT ( 'NONE',  ( -21.53943276465977519, 0.05219959533907696930, 26.24890960531435624 ) ) ;
#59064=CARTESIAN_POINT ( 'NONE',  ( 19.05341960407611168, 5.049401038298154454, 108.9572429386476955 ) ) ;
#59066=CARTESIAN_POINT ( 'NONE',  ( -16.53943276465976808, -0.05219959533934237506, 103.7510903946857042 ) ) ;
#59067=CARTESIAN_POINT ( 'NONE',  ( -16.53943276465976808, -0.05219959533934237506, 43.75109039468568284 ) ) ;
#59068=CARTESIAN_POINT ( 'NONE',  ( -13.89961937509977652, 13.97604488694528158, 60.62390960531436690 ) ) ;
#59069=CARTESIAN_POINT ( 'NONE',  ( -9.474510206698964154, 16.51473224551069663, 80.41557627198103830 ) ) ;
#59070=CARTESIAN_POINT ( 'NONE',  ( -16.52544592524335698, -4.483927247898792601, 73.95942372801901854 ) ) ;
#59071=CARTESIAN_POINT ( 'NONE',  ( 4.483927247898545687, 16.52544592524342804, 49.79057627198102409 ) ) ;
#59072=CARTESIAN_POINT ( 'NONE',  ( -16.51473224551069308, -9.474510206698971260, 56.66557627198103120 ) ) ;
#59073=CARTESIAN_POINT ( 'NONE',  ( -0.05219959533909027116, -19.03943276465977164, 47.49890960531435979 ) ) ;
#59074=CARTESIAN_POINT ( 'NONE',  ( 12.14591786802327356, -12.06949235617739191, 45.62609039468567573 ) ) ;
#59075=CARTESIAN_POINT ( 'NONE',  ( 0.05219959533936267826, -19.03943276465977164, 95.00109039468567573 ) ) ;
#59076=CARTESIAN_POINT ( 'NONE',  ( 4.379528057220339221, -16.55341960407611168, 97.70724293864772392 ) ) ;
#59077=CARTESIAN_POINT ( 'NONE',  ( -5.153800228976328057, -19.02544592524343514, 67.29057627198102409 ) ) ;
#59078=CARTESIAN_POINT ( 'NONE',  ( 0.05219959533936267826, -19.03943276465977164, 105.0010903946856615 ) ) ;
#59080=CARTESIAN_POINT ( 'NONE',  ( -21.55341960407619339, 5.719274019375674811, 88.54275706135236135 ) ) ;
#59081=CARTESIAN_POINT ( 'NONE',  ( -14.29746914071037622, -8.314922557961029526, 69.16775706135234714 ) ) ;
#59083=CARTESIAN_POINT ( 'NONE',  ( 15.80617190586746368, 15.72974639402197994, 64.37390960531435269 ) ) ;
#59084=CARTESIAN_POINT ( 'NONE',  ( 16.52544592524335698, 4.483927247898782831, 56.45942372801902565 ) ) ;
#59085=CARTESIAN_POINT ( 'NONE',  ( -13.89961937509977830, 13.97604488694528158, 35.62390960531435979 ) ) ;
#59086=CARTESIAN_POINT ( 'NONE',  ( -19.05341960407617563, 5.049401038297882671, 48.54275706135233293 ) ) ;
#59087=CARTESIAN_POINT ( 'NONE',  ( 5.153800228976335163, 19.02544592524342804, 89.79057627198102409 ) ) ;
#59088=CARTESIAN_POINT ( 'NONE',  ( -19.02544592524342804, 5.153800228976336051, 26.04057627198103120 ) ) ;
#59089=CARTESIAN_POINT ( 'NONE',  ( 9.564922557960805705, 16.46253265017160317, 59.58224293864769550 ) ) ;
#59090=B_SPLINE_CURVE_WITH_KNOTS ( 'NONE', 3,
 ( #73684, #139052, #532, #79374, #123868, #47060 ),
 .UNSPECIFIED., .F., .F.,
 ( 4, 2, 4 ),
 ( 0.000000000000000000, 0.0003837532665635213884, 0.0007675065331270427768 ),
 .UNSPECIFIED. ) ;
#59091=CARTESIAN_POINT ( 'NONE',  ( -15.80617190586768217, 15.72974639402176855, 78.12609039468570415 ) ) ;
#59092=CARTESIAN_POINT ( 'NONE',  ( -5.153800228976607833, 19.02544592524334988, 37.70942372801899722 ) ) ;
#59093=CARTESIAN_POINT ( 'NONE',  ( -19.05341960407617563, 5.049401038297882671, 23.54275706135233648 ) ) ;
#59094=CARTESIAN_POINT ( 'NONE',  ( 0.05219959533909260263, 19.03943276465977164, 59.99890960531436690 ) ) ;
#59095=CARTESIAN_POINT ( 'NONE',  ( 21.53943276465977519, -0.05219959533907433946, 28.74890960531435624 ) ) ;
#59096=CARTESIAN_POINT ( 'NONE',  ( 18.62759615963255655, 10.81492255796105972, 81.66775706135236135 ) ) ;
#59097=CARTESIAN_POINT ( 'NONE',  ( 13.89961937509977652, -13.97604488694527269, 58.12390960531436690 ) ) ;
#59099=CARTESIAN_POINT ( 'NONE',  ( 21.52544592524334988, 5.823673210054432836, 76.45942372801901854 ) ) ;
#59100=CARTESIAN_POINT ( 'NONE',  ( -21.52544592524343514, 5.823673210054127303, 41.04057627198103120 ) ) ;
#59101=CARTESIAN_POINT ( 'NONE',  ( 9.564922557960805705, 16.46253265017160317, 84.58224293864769550 ) ) ;
#59102=CARTESIAN_POINT ( 'NONE',  ( 21.53943276465977519, 0.05219959533937863772, 36.25109039468567573 ) ) ;
#59103=CARTESIAN_POINT ( 'NONE',  ( 9.564922557961047289, -16.46253265017146816, 55.41775706135234003 ) ) ;
#59104=CARTESIAN_POINT ( 'NONE',  ( -13.89961937509977652, 13.97604488694528158, 35.62390960531435269 ) ) ;
#59105=CARTESIAN_POINT ( 'NONE',  ( 0.05219959533909260263, 19.03943276465977164, 84.99890960531436690 ) ) ;
#59106=CARTESIAN_POINT ( 'NONE',  ( -8.314922557961024197, 14.29746914071037800, 22.91775706135235069 ) ) ;
#59107=CARTESIAN_POINT ( 'NONE',  ( -8.314922557960811034, -14.29746914071050412, 92.08224293864769550 ) ) ;
#59108=CARTESIAN_POINT ( 'NONE',  ( -19.03943276465977164, 0.05219959533909376836, 61.24890960531436690 ) ) ;
#59109=CARTESIAN_POINT ( 'NONE',  ( 18.62759615963271287, -10.81492255796078972, 48.33224293864770260 ) ) ;
#59110=CARTESIAN_POINT ( 'NONE',  ( -4.483927247898782831, 16.52544592524335698, 22.70942372801901499 ) ) ;
#59111=CARTESIAN_POINT ( 'NONE',  ( -0.05219959533937732626, 21.53943276465977519, 22.50109039468567573 ) ) ;
#59112=CARTESIAN_POINT ( 'NONE',  ( 15.72974639402176855, 15.80617190586768217, 76.87609039468567573 ) ) ;
#59113=CARTESIAN_POINT ( 'NONE',  ( -14.34966873604972548, 8.224510206698743886, 63.33442372801900433 ) ) ;
#59114=CARTESIAN_POINT ( 'NONE',  ( 12.06949235617739724, 12.14591786802326823, 61.87609039468568284 ) ) ;
#59115=CARTESIAN_POINT ( 'NONE',  ( 9.564922557960805705, 16.46253265017160317, 59.58224293864769550 ) ) ;
#59116=CARTESIAN_POINT ( 'NONE',  ( 14.29746914071037800, 8.314922557961029526, 96.66775706135234714 ) ) ;
#59117=CARTESIAN_POINT ( 'NONE',  ( 16.51473224551083163, -9.474510206698727899, 45.83442372801900433 ) ) ;
#59118=CARTESIAN_POINT ( 'NONE',  ( 5.823673210054125526, 21.52544592524343514, 114.7905762719810383 ) ) ;
#59119=CARTESIAN_POINT ( 'NONE',  ( -12.14591786802309592, -12.06949235617757132, 66.87390960531436690 ) ) ;
#59120=CARTESIAN_POINT ( 'NONE',  ( -9.474510206698964154, 16.51473224551069663, 90.41557627198103830 ) ) ;
#59121=CARTESIAN_POINT ( 'NONE',  ( 4.379528057220092307, 16.55341960407617563, 92.29275706135236135 ) ) ;
#59122=CARTESIAN_POINT ( 'NONE',  ( -18.67979575497193778, 10.72451020669871902, 53.33442372801901854 ) ) ;
#59123=CARTESIAN_POINT ( 'NONE',  ( -12.14591786802326823, 12.06949235617739902, 33.12609039468569705 ) ) ;
#59124=CARTESIAN_POINT ( 'NONE',  ( 18.62759615963255655, 10.81492255796105972, 26.66775706135235424 ) ) ;
#59125=CARTESIAN_POINT ( 'NONE',  ( -14.29746914071049879, 8.314922557960819915, 55.83224293864770260 ) ) ;
#59126=ORIENTED_EDGE ( 'NONE', *, *, #179989, .F. ) ;
#59127=CARTESIAN_POINT ( 'NONE',  ( 5.823673210054125526, 21.52544592524343514, 104.7905762719810241 ) ) ;
#59128=CARTESIAN_POINT ( 'NONE',  ( 14.34966873604960469, 8.224510206698951720, 39.16557627198102409 ) ) ;
#59131=CARTESIAN_POINT ( 'NONE',  ( 21.52544592524344225, -5.823673210054117533, 28.54057627198103120 ) ) ;
#59132=CARTESIAN_POINT ( 'NONE',  ( -10.72451020669870658, -18.67979575497194134, 34.58442372801900433 ) ) ;
#59133=CARTESIAN_POINT ( 'NONE',  ( -8.224510206698948167, 14.34966873604960824, 60.41557627198102409 ) ) ;
#59134=CARTESIAN_POINT ( 'NONE',  ( 19.05341960407611168, 5.049401038298154454, 68.95724293864769550 ) ) ;
#59135=CARTESIAN_POINT ( 'NONE',  ( -9.564922557960796823, -16.46253265017161027, 22.08224293864768839 ) ) ;
#59136=CARTESIAN_POINT ( 'NONE',  ( -13.97604488694547697, 13.89961937509957934, 68.12609039468563310 ) ) ;
#59137=CARTESIAN_POINT ( 'NONE',  ( -21.52544592524343514, 5.823673210054127303, 46.04057627198103830 ) ) ;
#59138=CARTESIAN_POINT ( 'NONE',  ( -19.02544592524342804, 5.153800228976336051, 56.04057627198100988 ) ) ;
#59139=CARTESIAN_POINT ( 'NONE',  ( 0.05219959533934541429, -16.53943276465976808, 35.00109039468568284 ) ) ;
#59140=CARTESIAN_POINT ( 'NONE',  ( -15.72974639402197994, 15.80617190586746368, 115.6239096053143669 ) ) ;
#59141=CARTESIAN_POINT ( 'NONE',  ( 4.483927247898545687, 16.52544592524342804, 44.79057627198103120 ) ) ;
#59143=CARTESIAN_POINT ( 'NONE',  ( 16.46253265017160672, -9.564922557960803928, 93.33224293864769550 ) ) ;
#59144=CARTESIAN_POINT ( 'NONE',  ( -5.823673210054116645, -21.52544592524344225, 72.29057627198102409 ) ) ;
#59145=CARTESIAN_POINT ( 'NONE',  ( -15.80617190586745835, -15.72974639402198527, 111.8739096053143669 ) ) ;
#59146=CARTESIAN_POINT ( 'NONE',  ( -16.52544592524335698, -4.483927247898792601, 33.95942372801901143 ) ) ;
#59147=CARTESIAN_POINT ( 'NONE',  ( -10.72451020669898014, 18.67979575497178502, 40.41557627198103120 ) ) ;
#59148=CARTESIAN_POINT ( 'NONE',  ( 15.80617190586769283, -15.72974639402175789, 95.62609039468568994 ) ) ;
#59149=CARTESIAN_POINT ( 'NONE',  ( 5.153800228976335163, 19.02544592524342804, 94.79057627198103830 ) ) ;
#59150=CARTESIAN_POINT ( 'NONE',  ( 16.46253265017160672, -9.564922557960803928, 43.33224293864769550 ) ) ;
#59151=CARTESIAN_POINT ( 'NONE',  ( -13.97604488694527625, -13.89961937509977652, 96.87390960531433848 ) ) ;
#59152=CARTESIAN_POINT ( 'NONE',  ( 13.89961937509977652, -13.97604488694527269, 78.12390960531433848 ) ) ;
#59155=CARTESIAN_POINT ( 'NONE',  ( 16.46253265017146816, 9.564922557961045513, 61.66775706135234003 ) ) ;
#59156=CARTESIAN_POINT ( 'NONE',  ( 10.81492255796106328, -18.62759615963255655, 110.4177570613523756 ) ) ;
#59157=CARTESIAN_POINT ( 'NONE',  ( -10.81492255796078084, -18.62759615963271287, 37.08224293864768129 ) ) ;
#59159=CARTESIAN_POINT ( 'NONE',  ( -4.483927247898782831, 16.52544592524335698, 107.7094237280190328 ) ) ;
#59160=CARTESIAN_POINT ( 'NONE',  ( 9.564922557961047289, -16.46253265017146816, 85.41775706135233293 ) ) ;
#59161=CARTESIAN_POINT ( 'NONE',  ( -16.38665767535054840, 7.295008042176026386, 60.26400864214547681 ) ) ;
#59162=CARTESIAN_POINT ( 'NONE',  ( -5.049401038297874678, -19.05341960407617918, 84.79275706135233293 ) ) ;
#59163=CARTESIAN_POINT ( 'NONE',  ( -16.51473224551082808, 9.474510206698731452, 43.33442372801900433 ) ) ;
#59164=CARTESIAN_POINT ( 'NONE',  ( 16.61371651742600264, 7.165104196376156587, 108.6458493000700543 ) ) ;
#59165=CARTESIAN_POINT ( 'NONE',  ( -9.474510206698964154, 16.51473224551069663, 40.41557627198103120 ) ) ;
#59166=CARTESIAN_POINT ( 'NONE',  ( -14.34966873604960291, -8.224510206698953496, 46.66557627198102409 ) ) ;
#59167=CARTESIAN_POINT ( 'NONE',  ( -16.61371651742600264, -7.165104196376159251, 111.1458493000700116 ) ) ;
#59168=CARTESIAN_POINT ( 'NONE',  ( -14.34966873604972548, 8.224510206698743886, 113.3344237280190328 ) ) ;
#59170=CARTESIAN_POINT ( 'NONE',  ( -4.379528057220086978, -16.55341960407618274, 89.79275706135236135 ) ) ;
#59171=CARTESIAN_POINT ( 'NONE',  ( -9.564922557960796823, -16.46253265017161027, 47.08224293864769550 ) ) ;
#59172=CARTESIAN_POINT ( 'NONE',  ( 5.823673210054444382, -21.52544592524334988, 110.2094237280190185 ) ) ;
#59173=CARTESIAN_POINT ( 'NONE',  ( -16.51473224551082808, 9.474510206698731452, 113.3344237280190043 ) ) ;
#59174=CARTESIAN_POINT ( 'NONE',  ( 21.53943276465977519, -0.05219959533907433946, 33.74890960531436690 ) ) ;
#59175=CARTESIAN_POINT ( 'NONE',  ( 10.72451020669871369, 18.67979575497193778, 92.08442372801901854 ) ) ;
#59176=CARTESIAN_POINT ( 'NONE',  ( 13.89961937509977652, -13.97604488694527269, 108.1239096053143669 ) ) ;
#59177=CARTESIAN_POINT ( 'NONE',  ( -5.049401038298153566, 19.05341960407611168, 85.20724293864766707 ) ) ;
#59179=CARTESIAN_POINT ( 'NONE',  ( 10.81492255796078972, 18.62759615963270932, 114.5822429386477097 ) ) ;
#59180=CARTESIAN_POINT ( 'NONE',  ( 4.379528057220339221, -16.55341960407611168, 77.70724293864770971 ) ) ;
#59181=CARTESIAN_POINT ( 'NONE',  ( -18.62759615963270932, 10.81492255796079327, 75.83224293864769550 ) ) ;
#59182=CARTESIAN_POINT ( 'NONE',  ( 19.02544592524343514, -5.153800228976328945, 58.54057627198102409 ) ) ;
#59183=CARTESIAN_POINT ( 'NONE',  ( -10.81492255796078084, -18.62759615963271287, 102.0822429386476955 ) ) ;
#59184=CARTESIAN_POINT ( 'NONE',  ( 16.53943276465976808, 0.05219959533934440121, 91.25109039468568994 ) ) ;
#59186=CARTESIAN_POINT ( 'NONE',  ( -0.05219959533909027116, -19.03943276465977164, 57.49890960531435979 ) ) ;
#59187=CARTESIAN_POINT ( 'NONE',  ( 16.53943276465976808, -0.05219959533910856209, 98.74890960531438111 ) ) ;
#59189=CARTESIAN_POINT ( 'NONE',  ( 16.46253265017160672, -9.564922557960803928, 63.33224293864769550 ) ) ;
#59190=CARTESIAN_POINT ( 'NONE',  ( 16.51473224551083163, -9.474510206698727899, 80.83442372801899012 ) ) ;
#59191=CARTESIAN_POINT ( 'NONE',  ( -0.05219959533910754901, -16.53943276465976808, 87.49890960531436690 ) ) ;
#59192=CARTESIAN_POINT ( 'NONE',  ( -21.52544592524334988, -5.823673210054445271, 63.95942372801901854 ) ) ;
#59193=CARTESIAN_POINT ( 'NONE',  ( 16.46253265017160672, -9.564922557960803928, 48.33224293864769550 ) ) ;
#59194=CARTESIAN_POINT ( 'NONE',  ( 18.67979575497194134, -10.72451020669871369, 25.83442372801901499 ) ) ;
#59195=CARTESIAN_POINT ( 'NONE',  ( 0.05219959533910956823, 16.53943276465976808, 104.9989096053143669 ) ) ;
#59197=CARTESIAN_POINT ( 'NONE',  ( 0.05219959533909260263, 19.03943276465977164, 54.99890960531435979 ) ) ;
#59199=CARTESIAN_POINT ( 'NONE',  ( 16.46253265017146816, 9.564922557961045513, 106.6677570613523471 ) ) ;
#59200=CARTESIAN_POINT ( 'NONE',  ( -5.823673210054116645, -21.52544592524344225, 22.29057627198102765 ) ) ;
#59201=CARTESIAN_POINT ( 'NONE',  ( -21.53943276465977519, -0.05219959533937600094, 48.75109039468568284 ) ) ;
#59202=CARTESIAN_POINT ( 'NONE',  ( -5.153800228976328057, -19.02544592524343514, 102.2905762719810383 ) ) ;
#59203=CARTESIAN_POINT ( 'NONE',  ( 9.474510206698729675, 16.51473224551082808, 82.08442372801899012 ) ) ;
#59204=CARTESIAN_POINT ( 'NONE',  ( -9.474510206698964154, 16.51473224551069663, 55.41557627198103120 ) ) ;
#59205=CARTESIAN_POINT ( 'NONE',  ( -12.06949235617756955, 12.14591786802309770, 70.62390960531436690 ) ) ;
#59206=CARTESIAN_POINT ( 'NONE',  ( -4.379528057220328563, 16.55341960407611168, 80.20724293864769550 ) ) ;
#59207=CARTESIAN_POINT ( 'NONE',  ( -5.049401038298153566, 19.05341960407611168, 85.20724293864766707 ) ) ;
#59208=CARTESIAN_POINT ( 'NONE',  ( -12.14591786802309592, -12.06949235617757132, 81.87390960531435269 ) ) ;
#59209=CARTESIAN_POINT ( 'NONE',  ( -19.02544592524342804, 5.153800228976336051, 86.04057627198103830 ) ) ;
#59211=CARTESIAN_POINT ( 'NONE',  ( 16.51473224551083163, -9.474510206698727899, 30.83442372801900433 ) ) ;
#59212=CARTESIAN_POINT ( 'NONE',  ( -16.46253265017160317, 9.564922557960807481, 45.83224293864769550 ) ) ;
#59213=CARTESIAN_POINT ( 'NONE',  ( -12.14591786802309592, -12.06949235617757132, 31.87390960531435979 ) ) ;
#59214=CARTESIAN_POINT ( 'NONE',  ( 16.46253265017160672, -9.564922557960803928, 33.33224293864770260 ) ) ;
#59216=CARTESIAN_POINT ( 'NONE',  ( -5.719274019375665041, -21.55341960407619695, 44.79275706135234714 ) ) ;
#59217=CARTESIAN_POINT ( 'NONE',  ( 0.05219959533936267826, -19.03943276465977164, 60.00109039468566863 ) ) ;
#59218=CARTESIAN_POINT ( 'NONE',  ( 14.29746914071049879, -8.314922557960816363, 33.33224293864769550 ) ) ;
#59219=CARTESIAN_POINT ( 'NONE',  ( -21.53943276465977519, 0.05219959533907696930, 86.24890960531436690 ) ) ;
#59220=CARTESIAN_POINT ( 'NONE',  ( -5.719274019375978568, 21.55341960407610458, 30.20724293864769550 ) ) ;
#59221=CARTESIAN_POINT ( 'NONE',  ( 16.55341960407611168, 4.379528057220329451, 73.95724293864769550 ) ) ;
#59222=CARTESIAN_POINT ( 'NONE',  ( 13.97604488694527802, 13.89961937509977652, 39.37390960531435269 ) ) ;
#59223=CARTESIAN_POINT ( 'NONE',  ( 16.53943276465976808, 0.05219959533934440121, 101.2510903946856757 ) ) ;
#59224=CARTESIAN_POINT ( 'NONE',  ( 16.55341960407618274, -4.379528057220086978, 51.04275706135234714 ) ) ;
#59225=CARTESIAN_POINT ( 'NONE',  ( -5.823673210054116645, -21.52544592524344225, 42.29057627198103120 ) ) ;
#59226=CARTESIAN_POINT ( 'NONE',  ( 0.05219959533937995610, -21.53943276465977519, 110.0010903946856757 ) ) ;
#59227=CARTESIAN_POINT ( 'NONE',  ( 5.049401038298161559, -19.05341960407611168, 87.70724293864769550 ) ) ;
#59228=CARTESIAN_POINT ( 'NONE',  ( -4.483927247898782831, 16.52544592524335698, 72.70942372801901854 ) ) ;
#59229=CARTESIAN_POINT ( 'NONE',  ( 4.483927247898545687, 16.52544592524342804, 114.7905762719810383 ) ) ;
#59230=CARTESIAN_POINT ( 'NONE',  ( -4.483927247898539470, -16.52544592524342804, 37.29057627198102409 ) ) ;
#59231=CARTESIAN_POINT ( 'NONE',  ( 13.97604488694527802, 13.89961937509977652, 109.3739096053143669 ) ) ;
#59232=CARTESIAN_POINT ( 'NONE',  ( -9.474510206698964154, 16.51473224551069663, 85.41557627198102409 ) ) ;
#59233=CARTESIAN_POINT ( 'NONE',  ( -19.03943276465977164, 0.05219959533909376836, 116.2489096053143669 ) ) ;
#59234=CARTESIAN_POINT ( 'NONE',  ( 14.29746914071049879, -8.314922557960816363, 68.33224293864769550 ) ) ;
#59236=CARTESIAN_POINT ( 'NONE',  ( -16.55341960407611168, -4.379528057220339221, 51.45724293864770260 ) ) ;
#59238=CARTESIAN_POINT ( 'NONE',  ( -16.52544592524335698, -4.483927247898792601, 53.95942372801900433 ) ) ;
#59240=CARTESIAN_POINT ( 'NONE',  ( 16.46253265017146816, 9.564922557961045513, 51.66775706135233293 ) ) ;
#59241=CARTESIAN_POINT ( 'NONE',  ( 19.05341960407611168, 5.049401038298154454, 83.95724293864766707 ) ) ;
#59242=CARTESIAN_POINT ( 'NONE',  ( -19.02544592524334988, -5.153800228976617603, 68.95942372801896170 ) ) ;
#59244=CARTESIAN_POINT ( 'NONE',  ( 9.564922557961047289, -16.46253265017146816, 55.41775706135234003 ) ) ;
#59245=CARTESIAN_POINT ( 'NONE',  ( 16.46253265017146816, 9.564922557961045513, 101.6677570613523329 ) ) ;
#59246=CARTESIAN_POINT ( 'NONE',  ( 8.314922557961029526, -14.29746914071037800, 100.4177570613523471 ) ) ;
#59248=CARTESIAN_POINT ( 'NONE',  ( 13.97604488694527802, 13.89961937509977652, 44.37390960531435269 ) ) ;
#59249=CARTESIAN_POINT ( 'NONE',  ( 5.049401038298161559, -19.05341960407611168, 112.7072429386476813 ) ) ;
#59250=CARTESIAN_POINT ( 'NONE',  ( -0.05219959533937732626, 21.53943276465977519, 57.50109039468568994 ) ) ;
#59251=CARTESIAN_POINT ( 'NONE',  ( -0.05219959533936034679, 19.03943276465977164, 97.50109039468567573 ) ) ;
#59252=DIRECTION ( 'NONE',  ( -1.000000000000000000, -0.000000000000000000, -0.000000000000000000 ) ) ;
#59253=CARTESIAN_POINT ( 'NONE',  ( -13.97604488694527625, -13.89961937509977652, 66.87390960531436690 ) ) ;
#59255=CARTESIAN_POINT ( 'NONE',  ( 8.314922557960818139, 14.29746914071049879, 79.58224293864769550 ) ) ;
#59256=CARTESIAN_POINT ( 'NONE',  ( 16.46253265017160672, -9.564922557960803928, 63.33224293864769550 ) ) ;
#59257=CARTESIAN_POINT ( 'NONE',  ( -16.51473224551069308, -9.474510206698971260, 71.66557627198102409 ) ) ;
#59258=CARTESIAN_POINT ( 'NONE',  ( 16.46253265017146816, 9.564922557961045513, 71.66775706135233293 ) ) ;
#59259=CARTESIAN_POINT ( 'NONE',  ( 0.05219959533907565091, 21.53943276465977519, 69.99890960531435269 ) ) ;
#59260=CARTESIAN_POINT ( 'NONE',  ( -9.564922557960796823, -16.46253265017161027, 22.08224293864768839 ) ) ;
#59261=CARTESIAN_POINT ( 'NONE',  ( 9.474510206698729675, 16.51473224551082808, 52.08442372801900433 ) ) ;
#59262=CARTESIAN_POINT ( 'NONE',  ( 5.153800228976335163, 19.02544592524342804, 59.79057627198100988 ) ) ;
#59263=CARTESIAN_POINT ( 'NONE',  ( 0.05219959533909260263, 19.03943276465977164, 79.99890960531436690 ) ) ;
#59264=CARTESIAN_POINT ( 'NONE',  ( -21.53943276465977519, 0.05219959533907696930, 91.24890960531436690 ) ) ;
#59265=CARTESIAN_POINT ( 'NONE',  ( 12.14591786802309770, 12.06949235617756955, 79.37390960531436690 ) ) ;
#59266=CARTESIAN_POINT ( 'NONE',  ( 0.05219959533936267826, -19.03943276465977164, 45.00109039468566863 ) ) ;
#59267=CARTESIAN_POINT ( 'NONE',  ( -18.67979575497178146, -10.72451020669898902, 81.66557627198103830 ) ) ;
#59268=CARTESIAN_POINT ( 'NONE',  ( 5.823673210054125526, 21.52544592524343514, 64.79057627198103830 ) ) ;
#59269=CARTESIAN_POINT ( 'NONE',  ( 16.55341960407611168, 4.379528057220329451, 33.95724293864769550 ) ) ;
#59270=CARTESIAN_POINT ( 'NONE',  ( 0.05219959533937995610, -21.53943276465977519, 90.00109039468567573 ) ) ;
#59271=CARTESIAN_POINT ( 'NONE',  ( -19.02544592524342804, 5.153800228976336051, 81.04057627198103830 ) ) ;
#59272=CARTESIAN_POINT ( 'NONE',  ( -13.89961937509977652, 13.97604488694528158, 25.62390960531434558 ) ) ;
#59273=CARTESIAN_POINT ( 'NONE',  ( -5.719274019375665041, -21.55341960407619695, 24.79275706135235779 ) ) ;
#59274=CARTESIAN_POINT ( 'NONE',  ( 5.823673210054444382, -21.52544592524334988, 40.20942372801901854 ) ) ;
#59275=CARTESIAN_POINT ( 'NONE',  ( 9.474510206698971260, -16.51473224551069308, 47.91557627198102409 ) ) ;
#59276=CARTESIAN_POINT ( 'NONE',  ( 10.81492255796106328, -18.62759615963255655, 25.41775706135235779 ) ) ;
#59277=CARTESIAN_POINT ( 'NONE',  ( 9.564922557961047289, -16.46253265017146816, 60.41775706135233293 ) ) ;
#59278=CARTESIAN_POINT ( 'NONE',  ( -19.05341960407611168, -5.049401038298163336, 41.45724293864769550 ) ) ;
#59279=CARTESIAN_POINT ( 'NONE',  ( -16.53943276465976808, -0.05219959533934237506, 28.75109039468567929 ) ) ;
#59280=CARTESIAN_POINT ( 'NONE',  ( 16.46253265017160672, -9.564922557960803928, 28.33224293864769550 ) ) ;
#59281=CARTESIAN_POINT ( 'NONE',  ( 14.34966873604972726, -8.224510206698740333, 65.83442372801900433 ) ) ;
#59282=CARTESIAN_POINT ( 'NONE',  ( -19.05341960407611168, -5.049401038298163336, 36.45724293864766707 ) ) ;
#59285=CARTESIAN_POINT ( 'NONE',  ( -9.474510206698964154, 16.51473224551069663, 90.41557627198103830 ) ) ;
#59286=CARTESIAN_POINT ( 'NONE',  ( -4.379528057220328563, 16.55341960407611168, 115.2072429386476955 ) ) ;
#59287=CARTESIAN_POINT ( 'NONE',  ( -15.72974639402197994, 15.80617190586746368, 60.62390960531437401 ) ) ;
#59288=CARTESIAN_POINT ( 'NONE',  ( -4.483927247898782831, 16.52544592524335698, 52.70942372801902565 ) ) ;
#59289=CARTESIAN_POINT ( 'NONE',  ( -15.72974639402176322, -15.80617190586768395, 94.37609039468568994 ) ) ;
#59290=CARTESIAN_POINT ( 'NONE',  ( 16.51473224551069308, 9.474510206698969483, 34.16557627198102409 ) ) ;
#59291=CARTESIAN_POINT ( 'NONE',  ( 14.29746914071049879, -8.314922557960816363, 33.33224293864769550 ) ) ;
#59292=CARTESIAN_POINT ( 'NONE',  ( 14.29746914071049879, -8.314922557960816363, 63.33224293864770260 ) ) ;
#59293=CARTESIAN_POINT ( 'NONE',  ( 0.05219959533909260263, 19.03943276465977164, 69.99890960531435269 ) ) ;
#59294=CARTESIAN_POINT ( 'NONE',  ( 15.72974639402176855, 15.80617190586768217, 111.8760903946856615 ) ) ;
#59295=CARTESIAN_POINT ( 'NONE',  ( -15.72974639402176322, -15.80617190586768395, 29.37609039468568284 ) ) ;
#59296=CIRCLE ( 'NONE', #17293, 2.000000000000000000 ) ;
#59297=CARTESIAN_POINT ( 'NONE',  ( 21.52544592524334988, 5.823673210054432836, 91.45942372801901854 ) ) ;
#59298=CARTESIAN_POINT ( 'NONE',  ( 14.34966873604972726, -8.224510206698740333, 55.83442372801901854 ) ) ;
#59299=CARTESIAN_POINT ( 'NONE',  ( 8.314922557961029526, -14.29746914071037800, 30.41775706135234358 ) ) ;
#59300=CARTESIAN_POINT ( 'NONE',  ( 0.05219959533910956823, 16.53943276465976808, 89.99890960531438111 ) ) ;
#59301=CARTESIAN_POINT ( 'NONE',  ( 21.53943276465977519, 0.05219959533937863772, 96.25109039468568994 ) ) ;
#59302=CARTESIAN_POINT ( 'NONE',  ( 8.314922557960818139, 14.29746914071049879, 39.58224293864769550 ) ) ;
#59303=CARTESIAN_POINT ( 'NONE',  ( 19.03943276465977164, -0.05219959533909143690, 23.74890960531435269 ) ) ;
#59304=CARTESIAN_POINT ( 'NONE',  ( -12.06949235617739369, -12.14591786802326823, 59.37609039468568284 ) ) ;
#59305=CARTESIAN_POINT ( 'NONE',  ( -12.14591786802309592, -12.06949235617757132, 56.87390960531436690 ) ) ;
#59306=CARTESIAN_POINT ( 'NONE',  ( 14.29746914071037800, 8.314922557961029526, 106.6677570613523756 ) ) ;
#59307=CARTESIAN_POINT ( 'NONE',  ( 10.72451020669898902, -18.67979575497178502, 22.91557627198102765 ) ) ;
#59308=CARTESIAN_POINT ( 'NONE',  ( -9.474510206698964154, 16.51473224551069663, 115.4155762719810241 ) ) ;
#59309=CARTESIAN_POINT ( 'NONE',  ( 13.97604488694548053, -13.89961937509957401, 20.62609039468567573 ) ) ;
#59310=CARTESIAN_POINT ( 'NONE',  ( -14.29746914071049879, 8.314922557960819915, 85.83224293864768129 ) ) ;
#59311=CARTESIAN_POINT ( 'NONE',  ( -9.474510206698964154, 16.51473224551069663, 95.41557627198102409 ) ) ;
#59313=CARTESIAN_POINT ( 'NONE',  ( 16.53943276465976808, 0.05219959533934440121, 41.25109039468568284 ) ) ;
#59314=CARTESIAN_POINT ( 'NONE',  ( -9.474510206698964154, 16.51473224551069663, 45.41557627198103120 ) ) ;
#59315=CARTESIAN_POINT ( 'NONE',  ( -5.153800228976328057, -19.02544592524343514, 107.2905762719810383 ) ) ;
#59316=CARTESIAN_POINT ( 'NONE',  ( -14.34966873604972548, 8.224510206698743886, 48.33442372801902565 ) ) ;
#59317=CARTESIAN_POINT ( 'NONE',  ( 15.50000000000000355, 5.499999999999998224, 22.00000000000000711 ) ) ;
#59318=CARTESIAN_POINT ( 'NONE',  ( 19.03943276465977164, 0.05219959533936151252, 51.25109039468567573 ) ) ;
#59319=CARTESIAN_POINT ( 'NONE',  ( -9.564922557960796823, -16.46253265017161027, 42.08224293864769550 ) ) ;
#59320=CARTESIAN_POINT ( 'NONE',  ( -12.14591786802326823, 12.06949235617739902, 78.12609039468570415 ) ) ;
#59321=CARTESIAN_POINT ( 'NONE',  ( 19.03943276465977164, 0.05219959533936151252, 76.25109039468566152 ) ) ;
#59322=CARTESIAN_POINT ( 'NONE',  ( 13.97604488694548053, -13.89961937509957401, 25.62609039468566507 ) ) ;
#59323=CARTESIAN_POINT ( 'NONE',  ( 19.05341960407611168, 5.049401038298154454, 63.95724293864769550 ) ) ;
#59324=CARTESIAN_POINT ( 'NONE',  ( 4.379528057220339221, -16.55341960407611168, 102.7072429386476955 ) ) ;
#59325=CARTESIAN_POINT ( 'NONE',  ( 16.46253265017146816, 9.564922557961045513, 61.66775706135234003 ) ) ;
#59326=CARTESIAN_POINT ( 'NONE',  ( -21.55341960407610458, -5.719274019375992779, 61.45724293864770260 ) ) ;
#59327=CARTESIAN_POINT ( 'NONE',  ( -19.05341960407617563, 5.049401038297882671, 28.54275706135232937 ) ) ;
#59328=CARTESIAN_POINT ( 'NONE',  ( 13.89961937509977652, -13.97604488694527269, 98.12390960531433848 ) ) ;
#59329=CARTESIAN_POINT ( 'NONE',  ( 21.53943276465977519, -0.05219959533907433946, 78.74890960531436690 ) ) ;
#59330=CARTESIAN_POINT ( 'NONE',  ( -16.62475595723700650, 7.163666690055240593, 85.52713351810471920 ) ) ;
#59331=CARTESIAN_POINT ( 'NONE',  ( 5.049401038297881783, 19.05341960407617563, 97.29275706135233293 ) ) ;
#59333=CARTESIAN_POINT ( 'NONE',  ( -8.314922557961024197, 14.29746914071037800, 32.91775706135234714 ) ) ;
#59334=CARTESIAN_POINT ( 'NONE',  ( -5.049401038298153566, 19.05341960407611168, 40.20724293864768839 ) ) ;
#59335=CARTESIAN_POINT ( 'NONE',  ( -9.564922557960796823, -16.46253265017161027, 107.0822429386476955 ) ) ;
#59336=CARTESIAN_POINT ( 'NONE',  ( -18.67979575497178146, -10.72451020669898902, 96.66557627198102409 ) ) ;
#59337=CARTESIAN_POINT ( 'NONE',  ( -15.72974639402176322, -15.80617190586768395, 54.37609039468568994 ) ) ;
#59338=CARTESIAN_POINT ( 'NONE',  ( 9.474510206698729675, 16.51473224551082808, 107.0844237280190043 ) ) ;
#59339=CARTESIAN_POINT ( 'NONE',  ( -18.62759615963255300, -10.81492255796106328, 109.1677570613523613 ) ) ;
#59340=CARTESIAN_POINT ( 'NONE',  ( -14.34966873604972548, 8.224510206698743886, 113.3344237280190328 ) ) ;
#59341=EDGE_CURVE ( 'NONE', #158898, #74699, #122128, .T. ) ;
#59342=CARTESIAN_POINT ( 'NONE',  ( 18.67979575497178502, 10.72451020669898547, 104.1655762719810241 ) ) ;
#59343=CARTESIAN_POINT ( 'NONE',  ( 16.53943276465976808, -0.05219959533910856209, 48.74890960531435979 ) ) ;
#59344=CARTESIAN_POINT ( 'NONE',  ( -5.153800228976607833, 19.02544592524334988, 82.70942372801897591 ) ) ;
#59346=CARTESIAN_POINT ( 'NONE',  ( 5.049401038297881783, 19.05341960407617563, 52.29275706135234003 ) ) ;
#59347=CARTESIAN_POINT ( 'NONE',  ( -10.81492255796105439, 18.62759615963255655, 52.91775706135235424 ) ) ;
#59348=CARTESIAN_POINT ( 'NONE',  ( -0.05219959533936034679, 19.03943276465977164, 37.50109039468567573 ) ) ;
#59349=CARTESIAN_POINT ( 'NONE',  ( -16.55341960407611168, -4.379528057220339221, 106.4572429386477097 ) ) ;
#59350=CARTESIAN_POINT ( 'NONE',  ( -18.62759615963270932, 10.81492255796079327, 25.83224293864769194 ) ) ;
#59351=CARTESIAN_POINT ( 'NONE',  ( -0.05219959533910754901, -16.53943276465976808, 37.49890960531436690 ) ) ;
#59352=CARTESIAN_POINT ( 'NONE',  ( -21.55341960407619339, 5.719274019375674811, 103.5427570613523613 ) ) ;
#59353=CARTESIAN_POINT ( 'NONE',  ( -8.314922557961024197, 14.29746914071037800, 77.91775706135231871 ) ) ;
#59354=CARTESIAN_POINT ( 'NONE',  ( -14.29746914071049879, 8.314922557960819915, 30.83224293864770260 ) ) ;
#59355=CARTESIAN_POINT ( 'NONE',  ( 0.05219959533937995610, -21.53943276465977519, 65.00109039468568994 ) ) ;
#59356=CARTESIAN_POINT ( 'NONE',  ( -10.81492255796105439, 18.62759615963255655, 67.91775706135234714 ) ) ;
#59357=CARTESIAN_POINT ( 'NONE',  ( 18.67979575497178502, 10.72451020669898547, 74.16557627198102409 ) ) ;
#59358=ORIENTED_EDGE ( 'NONE', *, *, #100927, .T. ) ;
#59359=CARTESIAN_POINT ( 'NONE',  ( 18.22780087662123805, -5.499999999999989342, 63.51763182126896368 ) ) ;
#59360=CARTESIAN_POINT ( 'NONE',  ( -18.67979575497193778, 10.72451020669871902, 48.33442372801902565 ) ) ;
#59361=CARTESIAN_POINT ( 'NONE',  ( -14.34966873604960291, -8.224510206698953496, 111.6655762719810525 ) ) ;
#59362=CARTESIAN_POINT ( 'NONE',  ( 13.89961937509977652, -13.97604488694527269, 43.12390960531434558 ) ) ;
#59363=CARTESIAN_POINT ( 'NONE',  ( 16.52544592524342804, -4.483927247898539470, 78.54057627198103830 ) ) ;
#59364=CARTESIAN_POINT ( 'NONE',  ( -19.05341960407611168, -5.049401038298163336, 86.45724293864769550 ) ) ;
#59365=CARTESIAN_POINT ( 'NONE',  ( -12.14591786802309592, -12.06949235617757132, 21.87390960531436690 ) ) ;
#59366=CARTESIAN_POINT ( 'NONE',  ( 0.05219959533910956823, 16.53943276465976808, 104.9989096053143669 ) ) ;
#59367=CARTESIAN_POINT ( 'NONE',  ( -0.05219959533907301413, -21.53943276465977519, 67.49890960531436690 ) ) ;
#59368=CARTESIAN_POINT ( 'NONE',  ( -5.719274019375978568, 21.55341960407610458, 100.2072429386476955 ) ) ;
#59370=CARTESIAN_POINT ( 'NONE',  ( -5.049401038298153566, 19.05341960407611168, 65.20724293864765286 ) ) ;
#59371=CARTESIAN_POINT ( 'NONE',  ( 9.474510206698729675, 16.51473224551082808, 102.0844237280190043 ) ) ;
#59372=CARTESIAN_POINT ( 'NONE',  ( -0.05219959533907301413, -21.53943276465977519, 57.49890960531435979 ) ) ;
#59373=CARTESIAN_POINT ( 'NONE',  ( 15.80617190586769283, -15.72974639402175789, 85.62609039468568994 ) ) ;
#59374=CARTESIAN_POINT ( 'NONE',  ( -19.05341960407611168, -5.049401038298163336, 61.45724293864769550 ) ) ;
#59376=CARTESIAN_POINT ( 'NONE',  ( 0.05219959533909260263, 19.03943276465977164, 94.99890960531436690 ) ) ;
#59377=CARTESIAN_POINT ( 'NONE',  ( 16.52544592524335698, 4.483927247898782831, 71.45942372801901854 ) ) ;
#59378=CARTESIAN_POINT ( 'NONE',  ( -0.05219959533937732626, 21.53943276465977519, 52.50109039468567573 ) ) ;
#59379=CARTESIAN_POINT ( 'NONE',  ( 21.52544592524334988, 5.823673210054432836, 101.4594237280190185 ) ) ;
#59380=CARTESIAN_POINT ( 'NONE',  ( 18.62759615963255655, 10.81492255796105972, 21.66775706135235069 ) ) ;
#59381=CARTESIAN_POINT ( 'NONE',  ( -21.53943276465977519, 0.05219959533907696930, 76.24890960531435269 ) ) ;
#59382=CARTESIAN_POINT ( 'NONE',  ( -13.89961937509957401, -13.97604488694547875, 44.37609039468566863 ) ) ;
#59383=CARTESIAN_POINT ( 'NONE',  ( -18.62759615963270932, 10.81492255796079327, 40.83224293864769550 ) ) ;
#59384=CARTESIAN_POINT ( 'NONE',  ( -5.049401038298153566, 19.05341960407611168, 85.20724293864766707 ) ) ;
#59385=CARTESIAN_POINT ( 'NONE',  ( -4.379528057220328563, 16.55341960407611168, 35.20724293864768839 ) ) ;
#59386=CARTESIAN_POINT ( 'NONE',  ( -16.81555441253553340, 7.025013491695480283, 65.63685445334260748 ) ) ;
#59387=CARTESIAN_POINT ( 'NONE',  ( -19.39720447994794483, -5.500000000000082601, 79.66317477297182847 ) ) ;
#59388=CARTESIAN_POINT ( 'NONE',  ( -13.97604488694547697, 13.89961937509957934, 93.12609039468566152 ) ) ;
#59389=CARTESIAN_POINT ( 'NONE',  ( -10.72451020669898014, 18.67979575497178502, 65.41557627198102409 ) ) ;
#59390=CARTESIAN_POINT ( 'NONE',  ( 8.224510206698953496, -14.34966873604960469, 47.91557627198102409 ) ) ;
#59391=CARTESIAN_POINT ( 'NONE',  ( 12.06949235617739724, 12.14591786802326823, 26.87609039468567218 ) ) ;
#59392=CARTESIAN_POINT ( 'NONE',  ( -19.02544592524342804, 5.153800228976336051, 46.04057627198101699 ) ) ;
#59393=CARTESIAN_POINT ( 'NONE',  ( 5.823673210054444382, -21.52544592524334988, 20.20942372801900788 ) ) ;
#59394=CARTESIAN_POINT ( 'NONE',  ( -16.46253265017146816, -9.564922557961047289, 89.16775706135234714 ) ) ;
#59395=CARTESIAN_POINT ( 'NONE',  ( -9.474510206698964154, 16.51473224551069663, 80.41557627198103830 ) ) ;
#59396=CARTESIAN_POINT ( 'NONE',  ( -14.29746914071049879, 8.314922557960819915, 85.83224293864768129 ) ) ;
#59397=CARTESIAN_POINT ( 'NONE',  ( 13.97604488694527802, 13.89961937509977652, 74.37390960531436690 ) ) ;
#59398=CARTESIAN_POINT ( 'NONE',  ( 15.72974639402199770, -15.80617190586745480, 73.12390960531436690 ) ) ;
#59399=CARTESIAN_POINT ( 'NONE',  ( 5.153800228976335163, 19.02544592524342804, 29.79057627198102409 ) ) ;
#59401=CARTESIAN_POINT ( 'NONE',  ( -0.05219959533910754901, -16.53943276465976808, 52.49890960531435979 ) ) ;
#59402=CARTESIAN_POINT ( 'NONE',  ( 13.97604488694527802, 13.89961937509977652, 94.37390960531436690 ) ) ;
#59404=CARTESIAN_POINT ( 'NONE',  ( 5.049401038297881783, 19.05341960407617563, 47.29275706135231161 ) ) ;
#59405=CARTESIAN_POINT ( 'NONE',  ( -4.483927247898782831, 16.52544592524335698, 62.70942372801902565 ) ) ;
#59406=CARTESIAN_POINT ( 'NONE',  ( 5.719274019375991003, -21.55341960407610458, 82.70724293864770971 ) ) ;
#59407=CARTESIAN_POINT ( 'NONE',  ( -5.153800228976607833, 19.02544592524334988, 42.70942372801901143 ) ) ;
#59408=CARTESIAN_POINT ( 'NONE',  ( 13.89961937509977652, -13.97604488694527269, 83.12390960531436690 ) ) ;
#59410=CARTESIAN_POINT ( 'NONE',  ( -10.72451020669898014, 18.67979575497178502, 30.41557627198101699 ) ) ;
#59411=CARTESIAN_POINT ( 'NONE',  ( -16.46253265017160317, 9.564922557960807481, 70.83224293864770971 ) ) ;
#59412=CARTESIAN_POINT ( 'NONE',  ( 0.05219959533937995610, -21.53943276465977519, 50.00109039468568994 ) ) ;
#59413=CARTESIAN_POINT ( 'NONE',  ( 13.97604488694527802, 13.89961937509977652, 29.37390960531435979 ) ) ;
#59415=CARTESIAN_POINT ( 'NONE',  ( -5.719274019375978568, 21.55341960407610458, 110.2072429386477239 ) ) ;
#59416=CARTESIAN_POINT ( 'NONE',  ( -19.03943276465977164, 0.05219959533909376836, 91.24890960531436690 ) ) ;
#59418=CARTESIAN_POINT ( 'NONE',  ( 10.81492255796106328, -18.62759615963255655, 45.41775706135234003 ) ) ;
#59420=CARTESIAN_POINT ( 'NONE',  ( -16.51473224551069308, -9.474510206698971260, 106.6655762719810383 ) ) ;
#59422=CARTESIAN_POINT ( 'NONE',  ( -18.62759615963270932, 10.81492255796079327, 110.8322429386476955 ) ) ;
#59423=CARTESIAN_POINT ( 'NONE',  ( 19.02544592524343514, -5.153800228976328945, 48.54057627198103120 ) ) ;
#59424=CARTESIAN_POINT ( 'NONE',  ( 16.53943276465976808, 0.05219959533934440121, 26.25109039468567573 ) ) ;
#59426=CARTESIAN_POINT ( 'NONE',  ( 5.823673210054444382, -21.52544592524334988, 105.2094237280190328 ) ) ;
#59427=CARTESIAN_POINT ( 'NONE',  ( 16.51473224551069308, 9.474510206698969483, 24.16557627198102765 ) ) ;
#59428=CARTESIAN_POINT ( 'NONE',  ( 5.719274019375673035, 21.55341960407619339, 92.29275706135236135 ) ) ;
#59430=CARTESIAN_POINT ( 'NONE',  ( -5.153800228976328057, -19.02544592524343514, 92.29057627198099567 ) ) ;
#59431=CARTESIAN_POINT ( 'NONE',  ( -21.53943276465977519, -0.05219959533937600094, 63.75109039468568284 ) ) ;
#59433=CARTESIAN_POINT ( 'NONE',  ( 13.97604488694527802, 13.89961937509977652, 99.37390960531436690 ) ) ;
#59434=DIRECTION ( 'NONE',  ( 0.000000000000000000, 0.000000000000000000, -1.000000000000000000 ) ) ;
#59435=CARTESIAN_POINT ( 'NONE',  ( 14.34966873604972726, -8.224510206698740333, 50.83442372801901143 ) ) ;
#59436=CARTESIAN_POINT ( 'NONE',  ( 4.379528057220092307, 16.55341960407617563, 62.29275706135236845 ) ) ;
#59437=CARTESIAN_POINT ( 'NONE',  ( 15.72974639402176855, 15.80617190586768217, 51.87609039468568284 ) ) ;
#59438=CARTESIAN_POINT ( 'NONE',  ( -5.823673210054431948, 21.52544592524334988, 87.70942372801901854 ) ) ;
#59440=CARTESIAN_POINT ( 'NONE',  ( -8.224510206698735004, -14.34966873604973081, 24.58442372801901499 ) ) ;
#59441=CARTESIAN_POINT ( 'NONE',  ( -19.03943276465977164, 0.05219959533909376836, 71.24890960531435269 ) ) ;
#59442=CARTESIAN_POINT ( 'NONE',  ( -9.474510206698964154, 16.51473224551069663, 95.41557627198102409 ) ) ;
#59443=CARTESIAN_POINT ( 'NONE',  ( 18.09867054820431775, 5.499999999999960032, 91.48393025253585620 ) ) ;
#59444=CARTESIAN_POINT ( 'NONE',  ( 9.564922557960805705, 16.46253265017160317, 29.58224293864769550 ) ) ;
#59445=CARTESIAN_POINT ( 'NONE',  ( -15.72974639402197994, 15.80617190586746368, 30.62390960531436335 ) ) ;
#59446=CARTESIAN_POINT ( 'NONE',  ( 16.53943276465976808, 0.05219959533934440121, 91.25109039468568994 ) ) ;
#59447=CARTESIAN_POINT ( 'NONE',  ( 14.34966873604960469, 8.224510206698951720, 74.16557627198102409 ) ) ;
#59448=CARTESIAN_POINT ( 'NONE',  ( -5.153800228976328057, -19.02544592524343514, 72.29057627198102409 ) ) ;
#59449=CARTESIAN_POINT ( 'NONE',  ( -15.72974639402176322, -15.80617190586768395, 94.37609039468568994 ) ) ;
#59450=CARTESIAN_POINT ( 'NONE',  ( -19.02544592524342804, 5.153800228976336051, 116.0405762719810383 ) ) ;
#59451=CARTESIAN_POINT ( 'NONE',  ( -8.224510206698735004, -14.34966873604973081, 24.58442372801901499 ) ) ;
#59452=CARTESIAN_POINT ( 'NONE',  ( -14.29746914071049879, 8.314922557960819915, 80.83224293864769550 ) ) ;
#59453=CARTESIAN_POINT ( 'NONE',  ( -21.52544592524334988, -5.823673210054445271, 33.95942372801901143 ) ) ;
#59454=CARTESIAN_POINT ( 'NONE',  ( -15.72974639402197994, 15.80617190586746368, 70.62390960531436690 ) ) ;
#59455=CARTESIAN_POINT ( 'NONE',  ( -9.474510206698720793, -16.51473224551083518, 39.58442372801899722 ) ) ;
#59457=CARTESIAN_POINT ( 'NONE',  ( 9.564922557960805705, 16.46253265017160317, 84.58224293864769550 ) ) ;
#59458=CARTESIAN_POINT ( 'NONE',  ( 16.53943276465976808, -0.05219959533910856209, 43.74890960531435979 ) ) ;
#59460=CARTESIAN_POINT ( 'NONE',  ( -16.53943276465976808, 0.05219959533911058130, 41.24890960531435269 ) ) ;
#59461=CARTESIAN_POINT ( 'NONE',  ( 8.314922557961029526, -14.29746914071037800, 105.4177570613523613 ) ) ;
#59462=CARTESIAN_POINT ( 'NONE',  ( 5.153800228976615827, -19.02544592524334988, 60.20942372801899012 ) ) ;
#59463=CARTESIAN_POINT ( 'NONE',  ( 18.22780087662121673, 5.500000000000056843, 53.98459894673893444 ) ) ;
#59464=CARTESIAN_POINT ( 'NONE',  ( -16.46253265017160317, 9.564922557960807481, 100.8322429386477097 ) ) ;
#59465=CARTESIAN_POINT ( 'NONE',  ( 14.29746914071049879, -8.314922557960816363, 78.33224293864770971 ) ) ;
#59467=CARTESIAN_POINT ( 'NONE',  ( -13.97604488694527625, -13.89961937509977652, 26.87390960531434558 ) ) ;
#59468=CARTESIAN_POINT ( 'NONE',  ( 5.823673210054125526, 21.52544592524343514, 39.79057627198103830 ) ) ;
#59469=CARTESIAN_POINT ( 'NONE',  ( -5.719274019375978568, 21.55341960407610458, 70.20724293864769550 ) ) ;
#59470=CARTESIAN_POINT ( 'NONE',  ( -14.29746914071049879, 8.314922557960819915, 115.8322429386477097 ) ) ;
#59471=CARTESIAN_POINT ( 'NONE',  ( -12.14591786802326823, 12.06949235617739902, 63.12609039468568994 ) ) ;
#59472=CARTESIAN_POINT ( 'NONE',  ( 19.05341960407611168, 5.049401038298154454, 48.95724293864768129 ) ) ;
#59473=CARTESIAN_POINT ( 'NONE',  ( 0.05219959533937995610, -21.53943276465977519, 50.00109039468568994 ) ) ;
#59474=CARTESIAN_POINT ( 'NONE',  ( 12.14591786802309770, 12.06949235617756955, 94.37390960531436690 ) ) ;
#59475=CARTESIAN_POINT ( 'NONE',  ( 17.26172910966779739, -6.454744622555848466, 38.30646908649224969 ) ) ;
#59477=CARTESIAN_POINT ( 'NONE',  ( -5.719274019375978568, 21.55341960407610458, 35.20724293864768839 ) ) ;
#59479=CARTESIAN_POINT ( 'NONE',  ( 10.81492255796106328, -18.62759615963255655, 65.41775706135234714 ) ) ;
#59481=CARTESIAN_POINT ( 'NONE',  ( 12.06949235617739724, 12.14591786802326823, 61.87609039468568284 ) ) ;
#59482=CARTESIAN_POINT ( 'NONE',  ( -12.06949235617756955, 12.14591786802309770, 45.62390960531436690 ) ) ;
#59483=CARTESIAN_POINT ( 'NONE',  ( -21.53943276465977519, 0.05219959533907696930, 71.24890960531435269 ) ) ;
#59484=CARTESIAN_POINT ( 'NONE',  ( -5.823673210054116645, -21.52544592524344225, 57.29057627198103120 ) ) ;
#59485=FACE_OUTER_BOUND ( 'NONE', #8953, .T. ) ;
#59486=CARTESIAN_POINT ( 'NONE',  ( 16.46253265017146816, 9.564922557961045513, 86.66775706135233293 ) ) ;
#59487=CARTESIAN_POINT ( 'NONE',  ( 21.53943276465977519, -0.05219959533907433946, 23.74890960531435269 ) ) ;
#59488=CARTESIAN_POINT ( 'NONE',  ( 9.564922557960805705, 16.46253265017160317, 49.58224293864770260 ) ) ;
#59489=CARTESIAN_POINT ( 'NONE',  ( 14.29746914071049879, -8.314922557960816363, 113.3322429386476955 ) ) ;
#59490=FACE_BOUND ( 'NONE', #5824, .T. ) ;
#59491=ORIENTED_EDGE ( 'NONE', *, *, #134324, .F. ) ;
#59492=CARTESIAN_POINT ( 'NONE',  ( -16.55341960407617563, 4.379528057220093196, 63.54275706135234003 ) ) ;
#59493=CARTESIAN_POINT ( 'NONE',  ( -15.72974639402197994, 15.80617190586746368, 110.6239096053143669 ) ) ;
#59494=CARTESIAN_POINT ( 'NONE',  ( 5.049401038298161559, -19.05341960407611168, 52.70724293864767418 ) ) ;
#59495=CARTESIAN_POINT ( 'NONE',  ( 21.55341960407619695, -5.719274019375665929, 36.04275706135234714 ) ) ;
#59496=CARTESIAN_POINT ( 'NONE',  ( 13.97604488694527802, 13.89961937509977652, 94.37390960531436690 ) ) ;
#59499=CARTESIAN_POINT ( 'NONE',  ( 10.81492255796106328, -18.62759615963255655, 30.41775706135234358 ) ) ;
#59500=CARTESIAN_POINT ( 'NONE',  ( -19.02544592524342804, 5.153800228976336051, 101.0405762719810241 ) ) ;
#59501=CARTESIAN_POINT ( 'NONE',  ( -13.89961937509957401, -13.97604488694547875, 94.37609039468566152 ) ) ;
#59502=CARTESIAN_POINT ( 'NONE',  ( 5.153800228976615827, -19.02544592524334988, 40.20942372801898301 ) ) ;
#59503=CARTESIAN_POINT ( 'NONE',  ( -21.52544592524343514, 5.823673210054127303, 101.0405762719810383 ) ) ;
#59504=CARTESIAN_POINT ( 'NONE',  ( 13.89961937509957401, 13.97604488694547697, 31.87609039468566863 ) ) ;
#59505=CARTESIAN_POINT ( 'NONE',  ( 13.97604488694548053, -13.89961937509957401, 30.62609039468566863 ) ) ;
#59506=CARTESIAN_POINT ( 'NONE',  ( -8.314922557961024197, 14.29746914071037800, 87.91775706135234714 ) ) ;
#59507=CARTESIAN_POINT ( 'NONE',  ( 16.46253265017160672, -9.564922557960803928, 113.3322429386476955 ) ) ;
#59508=CARTESIAN_POINT ( 'NONE',  ( 16.46253265017160672, -9.564922557960803928, 78.33224293864769550 ) ) ;
#59509=CARTESIAN_POINT ( 'NONE',  ( -21.55341960407619339, 5.719274019375674811, 73.54275706135234714 ) ) ;
#59510=CARTESIAN_POINT ( 'NONE',  ( -10.72451020669870658, -18.67979575497194134, 74.58442372801901854 ) ) ;
#59511=CARTESIAN_POINT ( 'NONE',  ( -19.05341960407611168, -5.049401038298163336, 91.45724293864766707 ) ) ;
#59512=CARTESIAN_POINT ( 'NONE',  ( -10.81492255796105439, 18.62759615963255655, 62.91775706135236135 ) ) ;
#59513=CARTESIAN_POINT ( 'NONE',  ( 9.564922557961047289, -16.46253265017146816, 105.4177570613523471 ) ) ;
#59514=CARTESIAN_POINT ( 'NONE',  ( 5.049401038298161559, -19.05341960407611168, 62.70724293864769550 ) ) ;
#59515=CARTESIAN_POINT ( 'NONE',  ( -5.153800228976328057, -19.02544592524343514, 112.2905762719810099 ) ) ;
#59516=CARTESIAN_POINT ( 'NONE',  ( -13.89961937509977652, 13.97604488694528158, 75.62390960531438111 ) ) ;
#59518=CARTESIAN_POINT ( 'NONE',  ( -0.05219959533909027116, -19.03943276465977164, 62.49890960531435979 ) ) ;
#59519=CARTESIAN_POINT ( 'NONE',  ( 13.97604488694527802, 13.89961937509977652, 49.37390960531434558 ) ) ;
#59520=CARTESIAN_POINT ( 'NONE',  ( 10.72451020669898902, -18.67979575497178502, 97.91557627198103830 ) ) ;
#59521=CARTESIAN_POINT ( 'NONE',  ( -8.314922557961024197, 14.29746914071037800, 82.91775706135234714 ) ) ;
#59523=CARTESIAN_POINT ( 'NONE',  ( 5.049401038297881783, 19.05341960407617563, 47.29275706135231161 ) ) ;
#59524=CARTESIAN_POINT ( 'NONE',  ( -9.474510206698964154, 16.51473224551069663, 75.41557627198103830 ) ) ;
#59525=CARTESIAN_POINT ( 'NONE',  ( 12.06949235617757843, -12.14591786802309237, 68.12390960531436690 ) ) ;
#59526=CARTESIAN_POINT ( 'NONE',  ( -12.14591786802309592, -12.06949235617757132, 111.8739096053143669 ) ) ;
#59527=CARTESIAN_POINT ( 'NONE',  ( 19.05341960407611168, 5.049401038298154454, 108.9572429386477097 ) ) ;
#59528=CARTESIAN_POINT ( 'NONE',  ( 13.89961937509977652, -13.97604488694527269, 103.1239096053143527 ) ) ;
#59529=CARTESIAN_POINT ( 'NONE',  ( 14.34966873604960469, 8.224510206698951720, 79.16557627198103830 ) ) ;
#59531=CARTESIAN_POINT ( 'NONE',  ( 9.564922557961047289, -16.46253265017146816, 25.41775706135234003 ) ) ;
#59532=CARTESIAN_POINT ( 'NONE',  ( -16.55341960407617563, 4.379528057220093196, 98.54275706135234714 ) ) ;
#59533=CARTESIAN_POINT ( 'NONE',  ( -5.153800228976328057, -19.02544592524343514, 72.29057627198102409 ) ) ;
#59534=CARTESIAN_POINT ( 'NONE',  ( 10.81492255796106328, -18.62759615963255655, 50.41775706135235424 ) ) ;
#59535=CARTESIAN_POINT ( 'NONE',  ( 18.67979575497178502, 10.72451020669898547, 39.16557627198102409 ) ) ;
#59536=CARTESIAN_POINT ( 'NONE',  ( 21.53943276465977519, 0.05219959533937863772, 21.25109039468567218 ) ) ;
#59537=CARTESIAN_POINT ( 'NONE',  ( -10.72451020669898014, 18.67979575497178502, 70.41557627198102409 ) ) ;
#59538=CARTESIAN_POINT ( 'NONE',  ( 12.14591786802309770, 12.06949235617756955, 99.37390960531436690 ) ) ;
#59539=CARTESIAN_POINT ( 'NONE',  ( 16.46253265017146816, 9.564922557961045513, 56.66775706135233293 ) ) ;
#59541=CARTESIAN_POINT ( 'NONE',  ( -19.05341960407611168, -5.049401038298163336, 36.45724293864766707 ) ) ;
#59542=CARTESIAN_POINT ( 'NONE',  ( -19.03943276465977164, 0.05219959533909376836, 81.24890960531436690 ) ) ;
#59543=CARTESIAN_POINT ( 'NONE',  ( 9.474510206698971260, -16.51473224551069308, 82.91557627198103830 ) ) ;
#59544=CARTESIAN_POINT ( 'NONE',  ( -16.52544592524342804, 4.483927247898546575, 101.0405762719810383 ) ) ;
#59545=ORIENTED_EDGE ( 'NONE', *, *, #79441, .T. ) ;
#59546=CARTESIAN_POINT ( 'NONE',  ( -16.52544592524342804, 4.483927247898546575, 26.04057627198103475 ) ) ;
#59547=CARTESIAN_POINT ( 'NONE',  ( 12.06949235617739724, 12.14591786802326823, 26.87609039468567218 ) ) ;
#59548=CARTESIAN_POINT ( 'NONE',  ( -21.55341960407619339, 5.719274019375674811, 93.54275706135234714 ) ) ;
#59549=CARTESIAN_POINT ( 'NONE',  ( -9.474510206698964154, 16.51473224551069663, 100.4155762719810241 ) ) ;
#59550=CARTESIAN_POINT ( 'NONE',  ( -15.72974639402176322, -15.80617190586768395, 24.37609039468567573 ) ) ;
#59551=CARTESIAN_POINT ( 'NONE',  ( -13.97604488694527625, -13.89961937509977652, 46.87390960531435979 ) ) ;
#59552=CARTESIAN_POINT ( 'NONE',  ( -16.52544592524335698, -4.483927247898792601, 38.95942372801901854 ) ) ;
#59553=CARTESIAN_POINT ( 'NONE',  ( 13.97604488694548053, -13.89961937509957401, 110.6260903946856615 ) ) ;
#59554=CARTESIAN_POINT ( 'NONE',  ( 5.049401038298161559, -19.05341960407611168, 37.70724293864768839 ) ) ;
#59555=CARTESIAN_POINT ( 'NONE',  ( -16.55341960407611168, -4.379528057220339221, 96.45724293864770971 ) ) ;
#59556=CARTESIAN_POINT ( 'NONE',  ( 18.62759615963271287, -10.81492255796078972, 103.3322429386476955 ) ) ;
#59557=CARTESIAN_POINT ( 'NONE',  ( -19.02544592524334988, -5.153800228976617603, 63.95942372801899012 ) ) ;
#59559=CARTESIAN_POINT ( 'NONE',  ( -13.89961937509977652, 13.97604488694528158, 95.62390960531436690 ) ) ;
#59560=CARTESIAN_POINT ( 'NONE',  ( -5.719274019375665041, -21.55341960407619695, 24.79275706135235779 ) ) ;
#59562=CARTESIAN_POINT ( 'NONE',  ( -16.46253265017160317, 9.564922557960807481, 85.83224293864769550 ) ) ;
#59564=CARTESIAN_POINT ( 'NONE',  ( 17.26058549869091507, -6.457015423128544818, 111.1225416252393643 ) ) ;
#59565=CARTESIAN_POINT ( 'NONE',  ( -19.03943276465977164, 0.05219959533909376836, 86.24890960531436690 ) ) ;
#59566=CARTESIAN_POINT ( 'NONE',  ( -15.80617190586768217, 15.72974639402176855, 33.12609039468569705 ) ) ;
#59567=CARTESIAN_POINT ( 'NONE',  ( 16.55341960407611168, 4.379528057220329451, 83.95724293864770971 ) ) ;
#59568=CARTESIAN_POINT ( 'NONE',  ( -9.474510206698964154, 16.51473224551069663, 85.41557627198102409 ) ) ;
#59569=CARTESIAN_POINT ( 'NONE',  ( -19.03943276465977164, -0.05219959533935918106, 23.75109039468566152 ) ) ;
#59570=CARTESIAN_POINT ( 'NONE',  ( -4.379528057220086978, -16.55341960407618274, 44.79275706135234714 ) ) ;
#59571=CARTESIAN_POINT ( 'NONE',  ( -0.05219959533936034679, 19.03943276465977164, 57.50109039468566863 ) ) ;
#59572=CARTESIAN_POINT ( 'NONE',  ( 21.55341960407619695, -5.719274019375665929, 66.04275706135236135 ) ) ;
#59573=CARTESIAN_POINT ( 'NONE',  ( 8.224510206698742110, 14.34966873604972548, 27.08442372801901854 ) ) ;
#59574=CARTESIAN_POINT ( 'NONE',  ( 19.02544592524343514, -5.153800228976328945, 63.54057627198103830 ) ) ;
#59576=CARTESIAN_POINT ( 'NONE',  ( -19.03943276465977164, -0.05219959533935918106, 98.75109039468567573 ) ) ;
#59577=CARTESIAN_POINT ( 'NONE',  ( 16.55341960407618274, -4.379528057220086978, 76.04275706135237556 ) ) ;
#59578=CARTESIAN_POINT ( 'NONE',  ( 13.89961937509957401, 13.97604488694547697, 21.87609039468566152 ) ) ;
#59579=CARTESIAN_POINT ( 'NONE',  ( -19.05341960407617563, 5.049401038297882671, 73.54275706135233293 ) ) ;
#59580=CARTESIAN_POINT ( 'NONE',  ( 13.97604488694527802, 13.89961937509977652, 54.37390960531435979 ) ) ;
#59581=CARTESIAN_POINT ( 'NONE',  ( -5.823673210054116645, -21.52544592524344225, 82.29057627198103830 ) ) ;
#59582=CARTESIAN_POINT ( 'NONE',  ( 16.55341960407611168, 4.379528057220329451, 78.95724293864769550 ) ) ;
#59583=CARTESIAN_POINT ( 'NONE',  ( -13.89961937509957401, -13.97604488694547875, 74.37609039468566152 ) ) ;
#59585=CARTESIAN_POINT ( 'NONE',  ( -5.049401038297874678, -19.05341960407617918, 39.79275706135232582 ) ) ;
#59586=CARTESIAN_POINT ( 'NONE',  ( 8.314922557961029526, -14.29746914071037800, 105.4177570613523613 ) ) ;
#59587=CARTESIAN_POINT ( 'NONE',  ( 12.06949235617757843, -12.14591786802309237, 63.12390960531435979 ) ) ;
#59588=CARTESIAN_POINT ( 'NONE',  ( -21.52544592524334988, -5.823673210054445271, 103.9594237280190185 ) ) ;
#59590=CARTESIAN_POINT ( 'NONE',  ( 5.823673210054125526, 21.52544592524343514, 109.7905762719810383 ) ) ;
#59591=CARTESIAN_POINT ( 'NONE',  ( -13.89961937509977652, 13.97604488694528158, 65.62390960531436690 ) ) ;
#59592=CARTESIAN_POINT ( 'NONE',  ( -5.719274019375665041, -21.55341960407619695, 84.79275706135234714 ) ) ;
#59593=CARTESIAN_POINT ( 'NONE',  ( -5.153800228976328057, -19.02544592524343514, 62.29057627198100988 ) ) ;
#59595=CARTESIAN_POINT ( 'NONE',  ( 16.55341960407611168, 4.379528057220329451, 113.9572429386477239 ) ) ;
#59596=CARTESIAN_POINT ( 'NONE',  ( 21.52544592524344225, -5.823673210054117533, 23.54057627198102765 ) ) ;
#59597=CARTESIAN_POINT ( 'NONE',  ( 16.52544592524342804, -4.483927247898539470, 63.54057627198103830 ) ) ;
#59598=CARTESIAN_POINT ( 'NONE',  ( 16.51473224551069308, 9.474510206698969483, 49.16557627198102409 ) ) ;
#59599=CARTESIAN_POINT ( 'NONE',  ( -4.483927247898539470, -16.52544592524342804, 97.29057627198105251 ) ) ;
#59601=CARTESIAN_POINT ( 'NONE',  ( 21.55341960407610458, 5.719274019375980345, 113.9572429386477239 ) ) ;
#59602=CARTESIAN_POINT ( 'NONE',  ( -10.81492255796105439, 18.62759615963255655, 42.91775706135235424 ) ) ;
#59603=CARTESIAN_POINT ( 'NONE',  ( 16.46253265017160672, -9.564922557960803928, 33.33224293864770260 ) ) ;
#59604=CARTESIAN_POINT ( 'NONE',  ( -12.06949235617739369, -12.14591786802326823, 64.37609039468568994 ) ) ;
#59606=CARTESIAN_POINT ( 'NONE',  ( 18.62759615963271287, -10.81492255796078972, 103.3322429386476955 ) ) ;
#59607=CARTESIAN_POINT ( 'NONE',  ( 21.52544592524344225, -5.823673210054117533, 103.5405762719810383 ) ) ;
#59608=CARTESIAN_POINT ( 'NONE',  ( 13.97604488694548053, -13.89961937509957401, 20.62609039468567573 ) ) ;
#59609=CARTESIAN_POINT ( 'NONE',  ( 16.46253265017160672, -9.564922557960803928, 58.33224293864769550 ) ) ;
#59610=CARTESIAN_POINT ( 'NONE',  ( 16.46253265017160672, -9.564922557960803928, 103.3322429386476955 ) ) ;
#59611=CARTESIAN_POINT ( 'NONE',  ( -10.81492255796105439, 18.62759615963255655, 52.91775706135235424 ) ) ;
#59612=CARTESIAN_POINT ( 'NONE',  ( 15.80617190586746368, 15.72974639402197994, 49.37390960531436690 ) ) ;
#59613=CARTESIAN_POINT ( 'NONE',  ( -16.55341960407617563, 4.379528057220093196, 113.5427570613523756 ) ) ;
#59614=CARTESIAN_POINT ( 'NONE',  ( -21.55341960407619339, 5.719274019375674811, 83.54275706135234714 ) ) ;
#59615=CARTESIAN_POINT ( 'NONE',  ( 15.72974639402176855, 15.80617190586768217, 96.87609039468568994 ) ) ;
#59616=CARTESIAN_POINT ( 'NONE',  ( -9.564922557961040184, 16.46253265017147172, 47.91775706135233293 ) ) ;
#59617=CARTESIAN_POINT ( 'NONE',  ( 4.483927247898790824, -16.52544592524335698, 95.20942372801903275 ) ) ;
#59618=CARTESIAN_POINT ( 'NONE',  ( 10.72451020669871369, 18.67979575497193778, 52.08442372801901854 ) ) ;
#59619=CARTESIAN_POINT ( 'NONE',  ( 13.97604488694527802, 13.89961937509977652, 64.37390960531436690 ) ) ;
#59620=CARTESIAN_POINT ( 'NONE',  ( 19.03943276465977164, 0.05219959533936151252, 21.25109039468565797 ) ) ;
#59621=CARTESIAN_POINT ( 'NONE',  ( 21.53943276465977519, -0.05219959533907433946, 33.74890960531436690 ) ) ;
#59622=CARTESIAN_POINT ( 'NONE',  ( 21.52544592524334988, 5.823673210054432836, 26.45942372801901854 ) ) ;
#59623=CARTESIAN_POINT ( 'NONE',  ( -21.52544592524343514, 5.823673210054127303, 91.04057627198103830 ) ) ;
#59624=CARTESIAN_POINT ( 'NONE',  ( -13.89961937509957401, -13.97604488694547875, 84.37609039468567573 ) ) ;
#59625=CARTESIAN_POINT ( 'NONE',  ( 14.29746914071037800, 8.314922557961029526, 36.66775706135234714 ) ) ;
#59627=CARTESIAN_POINT ( 'NONE',  ( 0.05219959533907565091, 21.53943276465977519, 84.99890960531436690 ) ) ;
#59628=CARTESIAN_POINT ( 'NONE',  ( -14.29746914071037622, -8.314922557961029526, 59.16775706135234714 ) ) ;
#59629=CARTESIAN_POINT ( 'NONE',  ( 8.224510206698953496, -14.34966873604960469, 82.91557627198103830 ) ) ;
#59631=CARTESIAN_POINT ( 'NONE',  ( -0.05219959533936034679, 19.03943276465977164, 107.5010903946856615 ) ) ;
#59632=CARTESIAN_POINT ( 'NONE',  ( -15.72974639402197994, 15.80617190586746368, 40.62390960531435269 ) ) ;
#59633=CARTESIAN_POINT ( 'NONE',  ( 5.153800228976335163, 19.02544592524342804, 94.79057627198103830 ) ) ;
#59634=CARTESIAN_POINT ( 'NONE',  ( 14.34966873604972726, -8.224510206698740333, 40.83442372801901854 ) ) ;
#59635=CARTESIAN_POINT ( 'NONE',  ( 18.67979575497178502, 10.72451020669898547, 114.1655762719810383 ) ) ;
#59636=CARTESIAN_POINT ( 'NONE',  ( -0.05219959533907301413, -21.53943276465977519, 27.49890960531435269 ) ) ;
#59637=CARTESIAN_POINT ( 'NONE',  ( 14.34966873604972726, -8.224510206698740333, 65.83442372801900433 ) ) ;
#59638=CARTESIAN_POINT ( 'NONE',  ( 16.46253265017160672, -9.564922557960803928, 88.33224293864769550 ) ) ;
#59639=CARTESIAN_POINT ( 'NONE',  ( 15.72974639402176855, 15.80617190586768217, 56.87609039468568994 ) ) ;
#59640=CARTESIAN_POINT ( 'NONE',  ( 16.51473224551069308, 9.474510206698969483, 29.16557627198103475 ) ) ;
#59641=CARTESIAN_POINT ( 'NONE',  ( -21.53943276465977519, 0.05219959533907696930, 21.24890960531436690 ) ) ;
#59643=CARTESIAN_POINT ( 'NONE',  ( 13.97604488694548053, -13.89961937509957401, 45.62609039468566863 ) ) ;
#59644=CARTESIAN_POINT ( 'NONE',  ( -8.224510206698735004, -14.34966873604973081, 54.58442372801901143 ) ) ;
#59645=CARTESIAN_POINT ( 'NONE',  ( -9.474510206698964154, 16.51473224551069663, 110.4155762719810383 ) ) ;
#59646=CARTESIAN_POINT ( 'NONE',  ( -19.03943276465977164, 0.05219959533909376836, 76.24890960531435269 ) ) ;
#59647=CARTESIAN_POINT ( 'NONE',  ( 0.05219959533934541429, -16.53943276465976808, 95.00109039468568994 ) ) ;
#59649=CARTESIAN_POINT ( 'NONE',  ( 16.55341960407611168, 4.379528057220329451, 93.95724293864770971 ) ) ;
#59650=CARTESIAN_POINT ( 'NONE',  ( 21.53943276465977519, -0.05219959533907433946, 28.74890960531435624 ) ) ;
#59651=CARTESIAN_POINT ( 'NONE',  ( 9.474510206698971260, -16.51473224551069308, 32.91557627198102409 ) ) ;
#59652=CARTESIAN_POINT ( 'NONE',  ( -8.314922557961024197, 14.29746914071037800, 62.91775706135236135 ) ) ;
#59653=CARTESIAN_POINT ( 'NONE',  ( 15.72974639402176855, 15.80617190586768217, 21.87609039468567573 ) ) ;
#59654=CARTESIAN_POINT ( 'NONE',  ( -9.564922557961040184, 16.46253265017147172, 77.91775706135234714 ) ) ;
#59655=CARTESIAN_POINT ( 'NONE',  ( 19.05341960407611168, 5.049401038298154454, 38.95724293864767418 ) ) ;
#59656=CARTESIAN_POINT ( 'NONE',  ( -15.80617190586745835, -15.72974639402198527, 71.87390960531438111 ) ) ;
#59657=CARTESIAN_POINT ( 'NONE',  ( -19.02544592524342804, 5.153800228976336051, 116.0405762719810383 ) ) ;
#59658=CARTESIAN_POINT ( 'NONE',  ( -10.81492255796105439, 18.62759615963255655, 97.91775706135236135 ) ) ;
#59659=CARTESIAN_POINT ( 'NONE',  ( 16.46253265017160672, -9.564922557960803928, 68.33224293864770971 ) ) ;
#59661=CARTESIAN_POINT ( 'NONE',  ( 14.29746914071037800, 8.314922557961029526, 46.66775706135234714 ) ) ;
#59662=CARTESIAN_POINT ( 'NONE',  ( -19.03943276465977164, 0.05219959533909376836, 76.24890960531435269 ) ) ;
#59663=CARTESIAN_POINT ( 'NONE',  ( -5.823673210054431948, 21.52544592524334988, 82.70942372801900433 ) ) ;
#59664=CARTESIAN_POINT ( 'NONE',  ( -9.474510206698720793, -16.51473224551083518, 34.58442372801899722 ) ) ;
#59665=CARTESIAN_POINT ( 'NONE',  ( -13.89961937509957401, -13.97604488694547875, 49.37609039468567573 ) ) ;
#59667=CARTESIAN_POINT ( 'NONE',  ( 15.80617190586769283, -15.72974639402175789, 50.62609039468568994 ) ) ;
#59669=CARTESIAN_POINT ( 'NONE',  ( 0.05219959533936267826, -19.03943276465977164, 45.00109039468566863 ) ) ;
#59670=CARTESIAN_POINT ( 'NONE',  ( -0.05219959533909027116, -19.03943276465977164, 102.4989096053143669 ) ) ;
#59671=CARTESIAN_POINT ( 'NONE',  ( -5.153800228976328057, -19.02544592524343514, 87.29057627198103830 ) ) ;
#59672=CARTESIAN_POINT ( 'NONE',  ( -0.05219959533910754901, -16.53943276465976808, 37.49890960531436690 ) ) ;
#59673=CARTESIAN_POINT ( 'NONE',  ( -15.72974639402197994, 15.80617190586746368, 35.62390960531437401 ) ) ;
#59674=CARTESIAN_POINT ( 'NONE',  ( -21.53943276465977519, -0.05219959533937600094, 98.75109039468568994 ) ) ;
#59677=CARTESIAN_POINT ( 'NONE',  ( -21.55341960407619339, 5.719274019375674811, 93.54275706135234714 ) ) ;
#59679=CARTESIAN_POINT ( 'NONE',  ( -5.153800228976328057, -19.02544592524343514, 32.29057627198102409 ) ) ;
#59680=CARTESIAN_POINT ( 'NONE',  ( 16.51473224551069308, 9.474510206698969483, 109.1655762719810383 ) ) ;
#59683=CARTESIAN_POINT ( 'NONE',  ( 12.06949235617739724, 12.14591786802326823, 51.87609039468568284 ) ) ;
#59684=CARTESIAN_POINT ( 'NONE',  ( -21.53943276465977519, 0.05219959533907696930, 71.24890960531435269 ) ) ;
#59685=CARTESIAN_POINT ( 'NONE',  ( 16.55341960407611168, 4.379528057220329451, 38.95724293864768839 ) ) ;
#59686=CARTESIAN_POINT ( 'NONE',  ( -16.51473224551069308, -9.474510206698971260, 31.66557627198102054 ) ) ;
#59687=CARTESIAN_POINT ( 'NONE',  ( 19.02544592524343514, -5.153800228976328945, 103.5405762719809957 ) ) ;
#59688=CARTESIAN_POINT ( 'NONE',  ( -5.719274019375665041, -21.55341960407619695, 24.79275706135235779 ) ) ;
#59689=CARTESIAN_POINT ( 'NONE',  ( -16.51473224551082808, 9.474510206698731452, 33.33442372801899722 ) ) ;
#59690=CARTESIAN_POINT ( 'NONE',  ( -4.379528057220328563, 16.55341960407611168, 110.2072429386477239 ) ) ;
#59691=CARTESIAN_POINT ( 'NONE',  ( -15.80617190586768217, 15.72974639402176855, 73.12609039468567573 ) ) ;
#59692=CARTESIAN_POINT ( 'NONE',  ( 17.48853670773246449, 5.747243402303094939, 98.83328700250008580 ) ) ;
#59693=CARTESIAN_POINT ( 'NONE',  ( -16.53943276465976808, 0.05219959533911058130, 26.24890960531435624 ) ) ;
#59694=CARTESIAN_POINT ( 'NONE',  ( 17.49999999999998934, 4.640572885337552300, 111.8621183545115798 ) ) ;
#59695=CARTESIAN_POINT ( 'NONE',  ( 18.62759615963271287, -10.81492255796078972, 28.33224293864769550 ) ) ;
#59696=CARTESIAN_POINT ( 'NONE',  ( -14.34966873604960291, -8.224510206698953496, 86.66557627198102409 ) ) ;
#59697=CARTESIAN_POINT ( 'NONE',  ( 18.22780087662121673, 5.500000000000056843, 53.98459894673893444 ) ) ;
#59698=CARTESIAN_POINT ( 'NONE',  ( -16.51473224551069308, -9.474510206698971260, 76.66557627198103830 ) ) ;
#59699=CARTESIAN_POINT ( 'NONE',  ( 14.34966873604960469, 8.224510206698951720, 74.16557627198102409 ) ) ;
#59700=CARTESIAN_POINT ( 'NONE',  ( -9.474510206698720793, -16.51473224551083518, 109.5844237280190043 ) ) ;
#59701=CARTESIAN_POINT ( 'NONE',  ( 5.823673210054125526, 21.52544592524343514, 59.79057627198103120 ) ) ;
#59703=CARTESIAN_POINT ( 'NONE',  ( 14.29746914071049879, -8.314922557960816363, 108.3322429386477097 ) ) ;
#59704=CARTESIAN_POINT ( 'NONE',  ( 19.05341960407611168, 5.049401038298154454, 68.95724293864769550 ) ) ;
#59705=CARTESIAN_POINT ( 'NONE',  ( -0.05219959533907301413, -21.53943276465977519, 72.49890960531435269 ) ) ;
#59706=CARTESIAN_POINT ( 'NONE',  ( -0.05219959533934338120, 16.53943276465976808, 107.5010903946856899 ) ) ;
#59707=CARTESIAN_POINT ( 'NONE',  ( -19.02544592524342804, 5.153800228976336051, 86.04057627198103830 ) ) ;
#59708=CARTESIAN_POINT ( 'NONE',  ( 19.05341960407617918, -5.049401038297876454, 61.04275706135232582 ) ) ;
#59709=CARTESIAN_POINT ( 'NONE',  ( 15.80617190586769283, -15.72974639402175789, 100.6260903946857184 ) ) ;
#59710=CARTESIAN_POINT ( 'NONE',  ( 18.62759615963271287, -10.81492255796078972, 73.33224293864769550 ) ) ;
#59711=CARTESIAN_POINT ( 'NONE',  ( 21.55341960407610458, 5.719274019375980345, 28.95724293864769905 ) ) ;
#59713=CARTESIAN_POINT ( 'NONE',  ( -13.97604488694527625, -13.89961937509977652, 46.87390960531435979 ) ) ;
#59714=CARTESIAN_POINT ( 'NONE',  ( -8.224510206698735004, -14.34966873604973081, 94.58442372801901854 ) ) ;
#59715=CARTESIAN_POINT ( 'NONE',  ( -19.02544592524342804, 5.153800228976336051, 66.04057627198103830 ) ) ;
#59716=CARTESIAN_POINT ( 'NONE',  ( 4.483927247898790824, -16.52544592524335698, 20.20942372801900788 ) ) ;
#59717=CARTESIAN_POINT ( 'NONE',  ( 17.13100169013299023, 6.664070546373166870, 51.73210164300153480 ) ) ;
#59718=CARTESIAN_POINT ( 'NONE',  ( 0.05219959533937995610, -21.53943276465977519, 110.0010903946856757 ) ) ;
#59720=CARTESIAN_POINT ( 'NONE',  ( 4.483927247898545687, 16.52544592524342804, 79.79057627198102409 ) ) ;
#59722=CARTESIAN_POINT ( 'NONE',  ( 5.823673210054125526, 21.52544592524343514, 104.7905762719810241 ) ) ;
#59723=CARTESIAN_POINT ( 'NONE',  ( -21.53943276465977519, 0.05219959533907696930, 106.2489096053143811 ) ) ;
#59725=CARTESIAN_POINT ( 'NONE',  ( 21.55341960407610458, 5.719274019375980345, 58.95724293864770971 ) ) ;
#59726=CARTESIAN_POINT ( 'NONE',  ( -4.379528057220086978, -16.55341960407618274, 84.79275706135234714 ) ) ;
#59727=CARTESIAN_POINT ( 'NONE',  ( 8.224510206698953496, -14.34966873604960469, 107.9155762719810241 ) ) ;
#59728=CARTESIAN_POINT ( 'NONE',  ( 5.153800228976335163, 19.02544592524342804, 64.79057627198100988 ) ) ;
#59730=CARTESIAN_POINT ( 'NONE',  ( -4.379528057220086978, -16.55341960407618274, 109.7927570613523613 ) ) ;
#59731=CARTESIAN_POINT ( 'NONE',  ( -18.67979575497193778, 10.72451020669871902, 43.33442372801901143 ) ) ;
#59732=CARTESIAN_POINT ( 'NONE',  ( 5.049401038298161559, -19.05341960407611168, 97.70724293864766707 ) ) ;
#59733=CARTESIAN_POINT ( 'NONE',  ( -15.72974639402176322, -15.80617190586768395, 84.37609039468570415 ) ) ;
#59734=CARTESIAN_POINT ( 'NONE',  ( -19.03943276465977164, 0.05219959533909376836, 31.24890960531435979 ) ) ;
#59735=CARTESIAN_POINT ( 'NONE',  ( -5.153800228976328057, -19.02544592524343514, 42.29057627198101699 ) ) ;
#59736=EDGE_LOOP ( 'NONE', ( #50919, #61911, #60411, #198314, #132362, #8021, #90479, #66270 ) ) ;
#59737=CARTESIAN_POINT ( 'NONE',  ( 21.52544592524334988, 5.823673210054432836, 76.45942372801901854 ) ) ;
#59738=CARTESIAN_POINT ( 'NONE',  ( -16.46253265017160317, 9.564922557960807481, 100.8322429386477097 ) ) ;
#59739=CARTESIAN_POINT ( 'NONE',  ( 19.05341960407617918, -5.049401038297876454, 81.04275706135231871 ) ) ;
#59740=CARTESIAN_POINT ( 'NONE',  ( -18.62759615963255300, -10.81492255796106328, 39.16775706135235424 ) ) ;
#59741=CARTESIAN_POINT ( 'NONE',  ( -16.52544592524335698, -4.483927247898792601, 28.95942372801902209 ) ) ;
#59742=CARTESIAN_POINT ( 'NONE',  ( -0.05219959533936034679, 19.03943276465977164, 67.50109039468566152 ) ) ;
#59743=CARTESIAN_POINT ( 'NONE',  ( 9.474510206698971260, -16.51473224551069308, 57.91557627198103120 ) ) ;
#59744=CARTESIAN_POINT ( 'NONE',  ( 16.51473224551083163, -9.474510206698727899, 80.83442372801899012 ) ) ;
#59746=CARTESIAN_POINT ( 'NONE',  ( -16.52544592524342804, 4.483927247898546575, 26.04057627198103475 ) ) ;
#59747=CARTESIAN_POINT ( 'NONE',  ( 0.05219959533936267826, -19.03943276465977164, 85.00109039468567573 ) ) ;
#59748=CARTESIAN_POINT ( 'NONE',  ( -0.05219959533910754901, -16.53943276465976808, 37.49890960531436690 ) ) ;
#59749=CARTESIAN_POINT ( 'NONE',  ( -5.153800228976607833, 19.02544592524334988, 57.70942372801899012 ) ) ;
#59750=CARTESIAN_POINT ( 'NONE',  ( -8.224510206698735004, -14.34966873604973081, 44.58442372801901854 ) ) ;
#59751=CARTESIAN_POINT ( 'NONE',  ( -19.02544592524334988, -5.153800228976617603, 18.95942372801899722 ) ) ;
#59752=CARTESIAN_POINT ( 'NONE',  ( 9.564922557960805705, 16.46253265017160317, 24.58224293864769194 ) ) ;
#59753=CARTESIAN_POINT ( 'NONE',  ( -17.26172910966778318, -6.454744622555873335, 64.19353091350780005 ) ) ;
#59754=CARTESIAN_POINT ( 'NONE',  ( -8.224510206698735004, -14.34966873604973081, 44.58442372801901854 ) ) ;
#59756=EDGE_CURVE ( 'NONE', #145773, #163091, #98104, .T. ) ;
#59758=CARTESIAN_POINT ( 'NONE',  ( 9.564922557960805705, 16.46253265017160317, 94.58224293864769550 ) ) ;
#59759=CARTESIAN_POINT ( 'NONE',  ( -17.72560187377287022, -5.499999999999974243, 69.07814504131316369 ) ) ;
#59761=CARTESIAN_POINT ( 'NONE',  ( 19.05341960407617918, -5.049401038297876454, 91.04275706135234714 ) ) ;
#59762=CARTESIAN_POINT ( 'NONE',  ( 15.72974639402199770, -15.80617190586745480, 28.12390960531435979 ) ) ;
#59763=CARTESIAN_POINT ( 'NONE',  ( 5.049401038297881783, 19.05341960407617563, 22.29275706135233648 ) ) ;
#59764=CARTESIAN_POINT ( 'NONE',  ( 19.02544592524334988, 5.153800228976608722, 96.45942372801897591 ) ) ;
#59765=CARTESIAN_POINT ( 'NONE',  ( -5.153800228976328057, -19.02544592524343514, 22.29057627198102765 ) ) ;
#59766=CARTESIAN_POINT ( 'NONE',  ( 19.02544592524343514, -5.153800228976328945, 43.54057627198103120 ) ) ;
#59767=CARTESIAN_POINT ( 'NONE',  ( -18.62759615963270932, 10.81492255796079327, 65.83224293864769550 ) ) ;
#59768=CARTESIAN_POINT ( 'NONE',  ( 16.51473224551069308, 9.474510206698969483, 24.16557627198102765 ) ) ;
#59770=CARTESIAN_POINT ( 'NONE',  ( 5.049401038297881783, 19.05341960407617563, 67.29275706135234714 ) ) ;
#59771=CARTESIAN_POINT ( 'NONE',  ( -14.29746914071049879, 8.314922557960819915, 40.83224293864769550 ) ) ;
#59772=CARTESIAN_POINT ( 'NONE',  ( 5.823673210054125526, 21.52544592524343514, 24.79057627198103120 ) ) ;
#59773=CARTESIAN_POINT ( 'NONE',  ( 10.81492255796106328, -18.62759615963255655, 95.41775706135234714 ) ) ;
#59774=CARTESIAN_POINT ( 'NONE',  ( 18.67979575497178502, 10.72451020669898547, 84.16557627198103830 ) ) ;
#59775=CARTESIAN_POINT ( 'NONE',  ( 10.72451020669871369, 18.67979575497193778, 62.08442372801901143 ) ) ;
#59776=CARTESIAN_POINT ( 'NONE',  ( -5.823673210054431948, 21.52544592524334988, 62.70942372801902565 ) ) ;
#59777=CARTESIAN_POINT ( 'NONE',  ( -5.049401038298153566, 19.05341960407611168, 100.2072429386476955 ) ) ;
#59778=CARTESIAN_POINT ( 'NONE',  ( 14.34966873604972726, -8.224510206698740333, 95.83442372801903275 ) ) ;
#59779=CARTESIAN_POINT ( 'NONE',  ( -18.62759615963255300, -10.81492255796106328, 54.16775706135235424 ) ) ;
#59780=CARTESIAN_POINT ( 'NONE',  ( -13.97604488694527625, -13.89961937509977652, 21.87390960531435979 ) ) ;
#59781=VECTOR ( 'NONE', #18603, 1000.000000000000000 ) ;
#59782=CARTESIAN_POINT ( 'NONE',  ( -16.52544592524342804, 4.483927247898546575, 61.04057627198103120 ) ) ;
#59783=CARTESIAN_POINT ( 'NONE',  ( -12.06949235617756955, 12.14591786802309770, 30.62390960531436335 ) ) ;
#59784=CARTESIAN_POINT ( 'NONE',  ( -5.823673210054116645, -21.52544592524344225, 42.29057627198103120 ) ) ;
#59785=CARTESIAN_POINT ( 'NONE',  ( -16.51473224551069308, -9.474510206698971260, 61.66557627198103120 ) ) ;
#59786=CARTESIAN_POINT ( 'NONE',  ( -9.564922557960796823, -16.46253265017161027, 47.08224293864769550 ) ) ;
#59787=CARTESIAN_POINT ( 'NONE',  ( -10.81492255796078084, -18.62759615963271287, 57.08224293864769550 ) ) ;
#59788=CARTESIAN_POINT ( 'NONE',  ( -9.474510206698720793, -16.51473224551083518, 49.58442372801899722 ) ) ;
#59790=CARTESIAN_POINT ( 'NONE',  ( 16.53943276465976808, -0.05219959533910856209, 43.74890960531435979 ) ) ;
#59791=CARTESIAN_POINT ( 'NONE',  ( -19.03943276465977164, 0.05219959533909376836, 116.2489096053143669 ) ) ;
#59793=VERTEX_POINT ( 'NONE', #88302 ) ;
#59794=CARTESIAN_POINT ( 'NONE',  ( -4.379528057220086978, -16.55341960407618274, 74.79275706135234714 ) ) ;
#59795=CARTESIAN_POINT ( 'NONE',  ( -19.03943276465977164, -0.05219959533935918106, 73.75109039468566152 ) ) ;
#59796=CARTESIAN_POINT ( 'NONE',  ( -12.14591786802309592, -12.06949235617757132, 46.87390960531435979 ) ) ;
#59797=DIRECTION ( 'NONE',  ( -1.000000000000000000, -0.000000000000000000, -0.000000000000000000 ) ) ;
#59798=CARTESIAN_POINT ( 'NONE',  ( -12.14591786802309592, -12.06949235617757132, 21.87390960531436690 ) ) ;
#59799=CARTESIAN_POINT ( 'NONE',  ( 19.05341960407611168, 5.049401038298154454, 48.95724293864768129 ) ) ;
#59800=CARTESIAN_POINT ( 'NONE',  ( -16.46253265017160317, 9.564922557960807481, 75.83224293864769550 ) ) ;
#59801=CARTESIAN_POINT ( 'NONE',  ( -16.46253265017160317, 9.564922557960807481, 35.83224293864768839 ) ) ;
#59802=CARTESIAN_POINT ( 'NONE',  ( -18.62759615963255300, -10.81492255796106328, 49.16775706135234003 ) ) ;
#59803=CARTESIAN_POINT ( 'NONE',  ( 13.89961937509977652, -13.97604488694527269, 53.12390960531434558 ) ) ;
#59804=CARTESIAN_POINT ( 'NONE',  ( 30.00000000000000000, 5.499999999999992895, 37.50000000000000000 ) ) ;
#59805=CARTESIAN_POINT ( 'NONE',  ( -9.564922557960796823, -16.46253265017161027, 57.08224293864769550 ) ) ;
#59806=CARTESIAN_POINT ( 'NONE',  ( 0.05219959533907565091, 21.53943276465977519, 39.99890960531436690 ) ) ;
#59807=CARTESIAN_POINT ( 'NONE',  ( 13.97604488694527802, 13.89961937509977652, 39.37390960531435269 ) ) ;
#59808=CARTESIAN_POINT ( 'NONE',  ( 21.55341960407610458, 5.719274019375980345, 43.95724293864769550 ) ) ;
#59809=CARTESIAN_POINT ( 'NONE',  ( 14.29746914071037800, 8.314922557961029526, 86.66775706135234714 ) ) ;
#59810=CARTESIAN_POINT ( 'NONE',  ( -0.05219959533937732626, 21.53943276465977519, 107.5010903946856899 ) ) ;
#59811=CARTESIAN_POINT ( 'NONE',  ( 8.224510206698742110, 14.34966873604972548, 62.08442372801901143 ) ) ;
#59812=CARTESIAN_POINT ( 'NONE',  ( 19.05341960407611168, 5.049401038298154454, 108.9572429386477097 ) ) ;
#59813=CARTESIAN_POINT ( 'NONE',  ( -8.314922557961024197, 14.29746914071037800, 52.91775706135235424 ) ) ;
#59814=CARTESIAN_POINT ( 'NONE',  ( -8.224510206698735004, -14.34966873604973081, 34.58442372801900433 ) ) ;
#59815=CARTESIAN_POINT ( 'NONE',  ( -5.049401038298153566, 19.05341960407611168, 110.2072429386476671 ) ) ;
#59816=CARTESIAN_POINT ( 'NONE',  ( 16.55341960407618274, -4.379528057220086978, 21.04275706135234714 ) ) ;
#59817=CARTESIAN_POINT ( 'NONE',  ( 13.89961937509977652, -13.97604488694527269, 38.12390960531436690 ) ) ;
#59818=CARTESIAN_POINT ( 'NONE',  ( 18.62759615963255655, 10.81492255796105972, 26.66775706135235424 ) ) ;
#59819=CARTESIAN_POINT ( 'NONE',  ( -8.224510206698735004, -14.34966873604973081, 19.58442372801901143 ) ) ;
#59820=CARTESIAN_POINT ( 'NONE',  ( 16.53943276465976808, 0.05219959533934440121, 81.25109039468568994 ) ) ;
#59822=CARTESIAN_POINT ( 'NONE',  ( 21.55341960407619695, -5.719274019375665929, 86.04275706135236135 ) ) ;
#59823=CARTESIAN_POINT ( 'NONE',  ( 13.89961937509957401, 13.97604488694547697, 96.87609039468566152 ) ) ;
#59824=CARTESIAN_POINT ( 'NONE',  ( -16.52544592524342804, 4.483927247898546575, 51.04057627198103120 ) ) ;
#59825=CARTESIAN_POINT ( 'NONE',  ( 14.29746914071049879, -8.314922557960816363, 113.3322429386476955 ) ) ;
#59826=CARTESIAN_POINT ( 'NONE',  ( -16.46253265017146816, -9.564922557961047289, 44.16775706135232582 ) ) ;
#59828=CARTESIAN_POINT ( 'NONE',  ( 10.81492255796106328, -18.62759615963255655, 45.41775706135234003 ) ) ;
#59829=CARTESIAN_POINT ( 'NONE',  ( -13.89961937509957401, -13.97604488694547875, 104.3760903946856757 ) ) ;
#59830=CARTESIAN_POINT ( 'NONE',  ( 16.38665767535056261, 7.295008042176082341, 82.23599135785454450 ) ) ;
#59831=CARTESIAN_POINT ( 'NONE',  ( -19.05341960407611168, -5.049401038298163336, 111.4572429386476671 ) ) ;
#59832=CARTESIAN_POINT ( 'NONE',  ( -21.55341960407610458, -5.719274019375992779, 66.45724293864768129 ) ) ;
#59833=CARTESIAN_POINT ( 'NONE',  ( 19.03943276465977164, 0.05219959533936151252, 91.25109039468566152 ) ) ;
#59834=EDGE_CURVE ( 'NONE', #4577, #98417, #70153, .T. ) ;
#59835=CARTESIAN_POINT ( 'NONE',  ( 19.03943276465977164, -0.05219959533909143690, 103.7489096053143669 ) ) ;
#59837=CARTESIAN_POINT ( 'NONE',  ( -4.483927247898539470, -16.52544592524342804, 102.2905762719810383 ) ) ;
#59838=CARTESIAN_POINT ( 'NONE',  ( 18.67979575497194134, -10.72451020669871369, 90.83442372801901854 ) ) ;
#59839=CARTESIAN_POINT ( 'NONE',  ( -5.153800228976328057, -19.02544592524343514, 47.29057627198102409 ) ) ;
#59841=CARTESIAN_POINT ( 'NONE',  ( -21.52544592524334988, -5.823673210054445271, 48.95942372801902565 ) ) ;
#59842=CARTESIAN_POINT ( 'NONE',  ( 5.823673210054444382, -21.52544592524334988, 95.20942372801903275 ) ) ;
#59843=CARTESIAN_POINT ( 'NONE',  ( -4.483927247898782831, 16.52544592524335698, 107.7094237280190328 ) ) ;
#59845=CARTESIAN_POINT ( 'NONE',  ( -5.049401038298153566, 19.05341960407611168, 65.20724293864765286 ) ) ;
#59846=CARTESIAN_POINT ( 'NONE',  ( 18.67979575497194134, -10.72451020669871369, 40.83442372801901854 ) ) ;
#59847=CARTESIAN_POINT ( 'NONE',  ( 10.81492255796106328, -18.62759615963255655, 45.41775706135234003 ) ) ;
#59848=CARTESIAN_POINT ( 'NONE',  ( 5.153800228976615827, -19.02544592524334988, 70.20942372801899012 ) ) ;
#59849=CARTESIAN_POINT ( 'NONE',  ( 19.03943276465977164, -0.05219959533909143690, 98.74890960531436690 ) ) ;
#59850=CARTESIAN_POINT ( 'NONE',  ( -4.379528057220328563, 16.55341960407611168, 105.2072429386477097 ) ) ;
#59851=CARTESIAN_POINT ( 'NONE',  ( -15.72974639402197994, 15.80617190586746368, 90.62390960531436690 ) ) ;
#59852=CARTESIAN_POINT ( 'NONE',  ( 14.34966873604960469, 8.224510206698951720, 64.16557627198102409 ) ) ;
#59853=CARTESIAN_POINT ( 'NONE',  ( -16.46253265017146816, -9.564922557961047289, 19.16775706135233293 ) ) ;
#59854=CARTESIAN_POINT ( 'NONE',  ( -0.05219959533910754901, -16.53943276465976808, 87.49890960531436690 ) ) ;
#59855=CARTESIAN_POINT ( 'NONE',  ( -9.474510206698964154, 16.51473224551069663, 30.41557627198102054 ) ) ;
#59856=CARTESIAN_POINT ( 'NONE',  ( -16.46253265017146816, -9.564922557961047289, 89.16775706135234714 ) ) ;
#59857=CARTESIAN_POINT ( 'NONE',  ( -12.14591786802309592, -12.06949235617757132, 46.87390960531435979 ) ) ;
#59858=CARTESIAN_POINT ( 'NONE',  ( 15.72974639402176855, 15.80617190586768217, 91.87609039468568994 ) ) ;
#59859=CARTESIAN_POINT ( 'NONE',  ( 19.02544592524343514, -5.153800228976328945, 88.54057627198102409 ) ) ;
#59860=CARTESIAN_POINT ( 'NONE',  ( 16.51473224551083163, -9.474510206698727899, 70.83442372801900433 ) ) ;
#59861=CARTESIAN_POINT ( 'NONE',  ( 18.62759615963271287, -10.81492255796078972, 78.33224293864770971 ) ) ;
#59862=CARTESIAN_POINT ( 'NONE',  ( 5.823673210054444382, -21.52544592524334988, 25.20942372801901854 ) ) ;
#59863=CARTESIAN_POINT ( 'NONE',  ( 8.224510206698742110, 14.34966873604972548, 27.08442372801901854 ) ) ;
#59864=CARTESIAN_POINT ( 'NONE',  ( 16.55341960407618274, -4.379528057220086978, 91.04275706135236135 ) ) ;
#59865=CARTESIAN_POINT ( 'NONE',  ( 9.564922557960805705, 16.46253265017160317, 24.58224293864769194 ) ) ;
#59866=CARTESIAN_POINT ( 'NONE',  ( 10.81492255796106328, -18.62759615963255655, 40.41775706135234714 ) ) ;
#59867=CARTESIAN_POINT ( 'NONE',  ( 16.51473224551069308, 9.474510206698969483, 24.16557627198102765 ) ) ;
#59869=CARTESIAN_POINT ( 'NONE',  ( 4.483927247898790824, -16.52544592524335698, 55.20942372801902565 ) ) ;
#59870=CARTESIAN_POINT ( 'NONE',  ( 12.14591786802309770, 12.06949235617756955, 74.37390960531436690 ) ) ;
#59871=CARTESIAN_POINT ( 'NONE',  ( -5.719274019375978568, 21.55341960407610458, 70.20724293864769550 ) ) ;
#59873=CARTESIAN_POINT ( 'NONE',  ( 4.379528057220339221, -16.55341960407611168, 22.70724293864769194 ) ) ;
#59874=CARTESIAN_POINT ( 'NONE',  ( 4.379528057220092307, 16.55341960407617563, 47.29275706135234003 ) ) ;
#59875=CARTESIAN_POINT ( 'NONE',  ( -16.46253265017160317, 9.564922557960807481, 50.83224293864770260 ) ) ;
#59876=CARTESIAN_POINT ( 'NONE',  ( 16.52544592524335698, 4.483927247898782831, 76.45942372801901854 ) ) ;
#59877=CARTESIAN_POINT ( 'NONE',  ( 9.564922557961047289, -16.46253265017146816, 80.41775706135234714 ) ) ;
#59878=CARTESIAN_POINT ( 'NONE',  ( 10.72451020669898902, -18.67979575497178502, 72.91557627198103830 ) ) ;
#59879=CARTESIAN_POINT ( 'NONE',  ( 4.483927247898545687, 16.52544592524342804, 24.79057627198103120 ) ) ;
#59880=ORIENTED_EDGE ( 'NONE', *, *, #56209, .T. ) ;
#59881=CARTESIAN_POINT ( 'NONE',  ( -9.474510206698964154, 16.51473224551069663, 115.4155762719810241 ) ) ;
#59882=CARTESIAN_POINT ( 'NONE',  ( 21.55341960407610458, 5.719274019375980345, 63.95724293864770260 ) ) ;
#59884=CARTESIAN_POINT ( 'NONE',  ( -4.483927247898782831, 16.52544592524335698, 92.70942372801901854 ) ) ;
#59885=VERTEX_POINT ( 'NONE', #72148 ) ;
#59886=CARTESIAN_POINT ( 'NONE',  ( 18.62759615963271287, -10.81492255796078972, 23.33224293864769194 ) ) ;
#59887=CARTESIAN_POINT ( 'NONE',  ( 17.49999999999998934, 3.512728167236884413, 107.2719000481888258 ) ) ;
#59888=CARTESIAN_POINT ( 'NONE',  ( -5.719274019375978568, 21.55341960407610458, 75.20724293864769550 ) ) ;
#59889=CARTESIAN_POINT ( 'NONE',  ( -16.55341960407617563, 4.379528057220093196, 108.5427570613523756 ) ) ;
#59890=CARTESIAN_POINT ( 'NONE',  ( 12.14591786802327356, -12.06949235617739191, 25.62609039468567929 ) ) ;
#59891=CARTESIAN_POINT ( 'NONE',  ( -13.97604488694527625, -13.89961937509977652, 26.87390960531434558 ) ) ;
#59892=CARTESIAN_POINT ( 'NONE',  ( -4.483927247898782831, 16.52544592524335698, 27.70942372801901854 ) ) ;
#59893=CARTESIAN_POINT ( 'NONE',  ( -13.89961937509977652, 13.97604488694528158, 50.62390960531435979 ) ) ;
#59895=CARTESIAN_POINT ( 'NONE',  ( 19.05341960407611168, 5.049401038298154454, 98.95724293864766707 ) ) ;
#59896=CARTESIAN_POINT ( 'NONE',  ( 8.314922557961029526, -14.29746914071037800, 90.41775706135236135 ) ) ;
#59897=CARTESIAN_POINT ( 'NONE',  ( 5.153800228976615827, -19.02544592524334988, 90.20942372801900433 ) ) ;
#59898=CARTESIAN_POINT ( 'NONE',  ( -19.05341960407617563, 5.049401038297882671, 28.54275706135232937 ) ) ;
#59899=CARTESIAN_POINT ( 'NONE',  ( -15.80617190586745835, -15.72974639402198527, 76.87390960531439532 ) ) ;
#59900=CARTESIAN_POINT ( 'NONE',  ( -14.29746914071037622, -8.314922557961029526, 104.1677570613523471 ) ) ;
#59901=CARTESIAN_POINT ( 'NONE',  ( -5.153800228976607833, 19.02544592524334988, 87.70942372801897591 ) ) ;
#59902=CARTESIAN_POINT ( 'NONE',  ( -19.02544592524342804, 5.153800228976336051, 51.04057627198103120 ) ) ;
#59903=CARTESIAN_POINT ( 'NONE',  ( -13.97604488694527625, -13.89961937509977652, 96.87390960531433848 ) ) ;
#59904=CARTESIAN_POINT ( 'NONE',  ( -10.81492255796105439, 18.62759615963255655, 67.91775706135234714 ) ) ;
#59905=CARTESIAN_POINT ( 'NONE',  ( -13.97604488694527625, -13.89961937509977652, 46.87390960531435979 ) ) ;
#59906=CARTESIAN_POINT ( 'NONE',  ( -16.52216118717210236, -7.221426719304506747, 86.07599021046992505 ) ) ;
#59907=CARTESIAN_POINT ( 'NONE',  ( -4.483927247898539470, -16.52544592524342804, 82.29057627198103830 ) ) ;
#59908=CARTESIAN_POINT ( 'NONE',  ( 5.823673210054125526, 21.52544592524343514, 74.79057627198105251 ) ) ;
#59911=CARTESIAN_POINT ( 'NONE',  ( -13.97604488694547697, 13.89961937509957934, 43.12609039468566152 ) ) ;
#59912=CARTESIAN_POINT ( 'NONE',  ( 16.62475595723613253, -7.163666690055873865, 73.02713351810406550 ) ) ;
#59913=CARTESIAN_POINT ( 'NONE',  ( 9.474510206698971260, -16.51473224551069308, 72.91557627198102409 ) ) ;
#59914=CARTESIAN_POINT ( 'NONE',  ( -13.97604488694527625, -13.89961937509977652, 91.87390960531432427 ) ) ;
#59915=CARTESIAN_POINT ( 'NONE',  ( -0.05219959533934338120, 16.53943276465976808, 62.50109039468568284 ) ) ;
#59917=CARTESIAN_POINT ( 'NONE',  ( -9.564922557961040184, 16.46253265017147172, 27.91775706135232582 ) ) ;
#59919=CARTESIAN_POINT ( 'NONE',  ( -19.05341960407611168, -5.049401038298163336, 106.4572429386476955 ) ) ;
#59920=CARTESIAN_POINT ( 'NONE',  ( -16.53943276465976808, -0.05219959533934237506, 88.75109039468567573 ) ) ;
#59922=CARTESIAN_POINT ( 'NONE',  ( 4.379528057220092307, 16.55341960407617563, 77.29275706135234714 ) ) ;
#59924=CARTESIAN_POINT ( 'NONE',  ( -0.05219959533934338120, 16.53943276465976808, 57.50109039468568994 ) ) ;
#59925=CARTESIAN_POINT ( 'NONE',  ( -18.09867054820433907, -5.499999999999827693, 58.98393025253588462 ) ) ;
#59926=CARTESIAN_POINT ( 'NONE',  ( 15.72974639402176855, 15.80617190586768217, 71.87609039468568994 ) ) ;
#59927=CARTESIAN_POINT ( 'NONE',  ( 19.05341960407617918, -5.049401038297876454, 81.04275706135231871 ) ) ;
#59928=CARTESIAN_POINT ( 'NONE',  ( 19.03943276465977164, 0.05219959533936151252, 26.25109039468566507 ) ) ;
#59930=CARTESIAN_POINT ( 'NONE',  ( -9.564922557960796823, -16.46253265017161027, 47.08224293864769550 ) ) ;
#59931=CARTESIAN_POINT ( 'NONE',  ( -16.46253265017160317, 9.564922557960807481, 45.83224293864769550 ) ) ;
#59932=CARTESIAN_POINT ( 'NONE',  ( 16.73155767950884965, -7.079819277068864380, 23.08152769347067945 ) ) ;
#59933=CARTESIAN_POINT ( 'NONE',  ( -21.55341960407610458, -5.719274019375992779, 61.45724293864770260 ) ) ;
#59934=CARTESIAN_POINT ( 'NONE',  ( -0.05219959533907301413, -21.53943276465977519, 27.49890960531435269 ) ) ;
#59935=CARTESIAN_POINT ( 'NONE',  ( 4.483927247898545687, 16.52544592524342804, 109.7905762719810383 ) ) ;
#59936=CARTESIAN_POINT ( 'NONE',  ( 4.379528057220092307, 16.55341960407617563, 52.29275706135236135 ) ) ;
#59938=CARTESIAN_POINT ( 'NONE',  ( -18.62759615963270932, 10.81492255796079327, 115.8322429386477097 ) ) ;
#59939=CARTESIAN_POINT ( 'NONE',  ( 4.379528057220339221, -16.55341960407611168, 47.70724293864770260 ) ) ;
#59941=CARTESIAN_POINT ( 'NONE',  ( -16.46253265017146816, -9.564922557961047289, 109.1677570613523471 ) ) ;
#59942=CARTESIAN_POINT ( 'NONE',  ( -16.46253265017146816, -9.564922557961047289, 44.16775706135232582 ) ) ;
#59943=CARTESIAN_POINT ( 'NONE',  ( -4.483927247898539470, -16.52544592524342804, 47.29057627198103120 ) ) ;
#59944=CARTESIAN_POINT ( 'NONE',  ( 15.80617190586746368, 15.72974639402197994, 114.3739096053143527 ) ) ;
#59946=CARTESIAN_POINT ( 'NONE',  ( 16.36317988757057762, 7.306389748694947173, 33.40210391636777132 ) ) ;
#59947=CARTESIAN_POINT ( 'NONE',  ( 18.62759615963271287, -10.81492255796078972, 68.33224293864769550 ) ) ;
#59948=CARTESIAN_POINT ( 'NONE',  ( -13.89961937509977652, 13.97604488694528158, 85.62390960531433848 ) ) ;
#59949=CARTESIAN_POINT ( 'NONE',  ( -16.53943276465976808, 0.05219959533911058130, 61.24890960531435979 ) ) ;
#59950=CARTESIAN_POINT ( 'NONE',  ( 9.564922557960805705, 16.46253265017160317, 104.5822429386476955 ) ) ;
#59952=CARTESIAN_POINT ( 'NONE',  ( -9.564922557961040184, 16.46253265017147172, 52.91775706135233293 ) ) ;
#59953=CARTESIAN_POINT ( 'NONE',  ( -0.05219959533907301413, -21.53943276465977519, 87.49890960531436690 ) ) ;
#59954=CARTESIAN_POINT ( 'NONE',  ( 16.46253265017160672, -9.564922557960803928, 43.33224293864769550 ) ) ;
#59955=CARTESIAN_POINT ( 'NONE',  ( 16.55341960407611168, 4.379528057220329451, 113.9572429386477239 ) ) ;
#59956=CARTESIAN_POINT ( 'NONE',  ( 5.719274019375673035, 21.55341960407619339, 52.29275706135236135 ) ) ;
#59959=CARTESIAN_POINT ( 'NONE',  ( -4.483927247898539470, -16.52544592524342804, 32.29057627198102409 ) ) ;
#59960=CARTESIAN_POINT ( 'NONE',  ( -9.474510206698964154, 16.51473224551069663, 55.41557627198103120 ) ) ;
#59961=CARTESIAN_POINT ( 'NONE',  ( 19.02544592524343514, -5.153800228976328945, 93.54057627198102409 ) ) ;
#59962=CARTESIAN_POINT ( 'NONE',  ( 15.72974639402199770, -15.80617190586745480, 73.12390960531436690 ) ) ;
#59964=CARTESIAN_POINT ( 'NONE',  ( -16.46253265017160317, 9.564922557960807481, 45.83224293864769550 ) ) ;
#59965=CARTESIAN_POINT ( 'NONE',  ( 18.67979575497178502, 10.72451020669898547, 59.16557627198103120 ) ) ;
#59966=CARTESIAN_POINT ( 'NONE',  ( -18.62759615963255300, -10.81492255796106328, 89.16775706135236135 ) ) ;
#59968=CARTESIAN_POINT ( 'NONE',  ( 12.06949235617739724, 12.14591786802326823, 76.87609039468567573 ) ) ;
#59969=CARTESIAN_POINT ( 'NONE',  ( 16.53943276465976808, -0.05219959533910856209, 63.74890960531435979 ) ) ;
#59970=CARTESIAN_POINT ( 'NONE',  ( -0.05219959533909027116, -19.03943276465977164, 72.49890960531435269 ) ) ;
#59972=CARTESIAN_POINT ( 'NONE',  ( -19.03943276465977164, -0.05219959533935918106, 23.75109039468566152 ) ) ;
#59973=CARTESIAN_POINT ( 'NONE',  ( -8.224510206698735004, -14.34966873604973081, 94.58442372801901854 ) ) ;
#59974=CARTESIAN_POINT ( 'NONE',  ( 0.05219959533937995610, -21.53943276465977519, 110.0010903946856757 ) ) ;
#59975=CARTESIAN_POINT ( 'NONE',  ( 13.97604488694527802, 13.89961937509977652, 79.37390960531435269 ) ) ;
#59976=CARTESIAN_POINT ( 'NONE',  ( -15.80617190586745835, -15.72974639402198527, 46.87390960531435979 ) ) ;
#59977=CARTESIAN_POINT ( 'NONE',  ( 8.314922557961029526, -14.29746914071037800, 25.41775706135235779 ) ) ;
#59978=CARTESIAN_POINT ( 'NONE',  ( -21.55341960407619339, 5.719274019375674811, 78.54275706135236135 ) ) ;
#59979=CARTESIAN_POINT ( 'NONE',  ( 16.53943276465976808, 0.05219959533934440121, 61.25109039468567573 ) ) ;
#59980=CARTESIAN_POINT ( 'NONE',  ( 21.52544592524344225, -5.823673210054117533, 113.5405762719810383 ) ) ;
#59981=CARTESIAN_POINT ( 'NONE',  ( 14.34966873604972726, -8.224510206698740333, 20.83442372801901143 ) ) ;
#59982=CARTESIAN_POINT ( 'NONE',  ( -5.153800228976328057, -19.02544592524343514, 97.29057627198099567 ) ) ;
#59983=CARTESIAN_POINT ( 'NONE',  ( 12.14591786802327356, -12.06949235617739191, 30.62609039468567929 ) ) ;
#59984=CARTESIAN_POINT ( 'NONE',  ( -9.564922557960796823, -16.46253265017161027, 42.08224293864769550 ) ) ;
#59985=CARTESIAN_POINT ( 'NONE',  ( -14.34966873604972548, 8.224510206698743886, 38.33442372801900433 ) ) ;
#59986=CARTESIAN_POINT ( 'NONE',  ( -14.34966873604960291, -8.224510206698953496, 81.66557627198103830 ) ) ;
#59987=CARTESIAN_POINT ( 'NONE',  ( 12.14591786802327356, -12.06949235617739191, 90.62609039468567573 ) ) ;
#59988=CARTESIAN_POINT ( 'NONE',  ( 0.05219959533937995610, -21.53943276465977519, 35.00109039468568284 ) ) ;
#59989=CARTESIAN_POINT ( 'NONE',  ( 19.05341960407611168, 5.049401038298154454, 63.95724293864769550 ) ) ;
#59990=CARTESIAN_POINT ( 'NONE',  ( 19.05341960407611168, 5.049401038298154454, 88.95724293864769550 ) ) ;
#59991=CARTESIAN_POINT ( 'NONE',  ( 0.05219959533934541429, -16.53943276465976808, 85.00109039468568994 ) ) ;
#59992=EDGE_CURVE ( 'NONE', #27205, #174275, #121618, .T. ) ;
#59996=CARTESIAN_POINT ( 'NONE',  ( 16.46253265017146816, 9.564922557961045513, 31.66775706135232937 ) ) ;
#59997=CARTESIAN_POINT ( 'NONE',  ( -5.049401038298153566, 19.05341960407611168, 105.2072429386476671 ) ) ;
#59998=CARTESIAN_POINT ( 'NONE',  ( 16.46253265017160672, -9.564922557960803928, 53.33224293864768839 ) ) ;
#59999=CARTESIAN_POINT ( 'NONE',  ( 19.03943276465977164, -0.05219959533909143690, 113.7489096053143669 ) ) ;
#60000=ORIENTED_EDGE ( 'NONE', *, *, #32834, .T. ) ;
#60001=CARTESIAN_POINT ( 'NONE',  ( 4.483927247898790824, -16.52544592524335698, 30.20942372801902565 ) ) ;
#60002=CARTESIAN_POINT ( 'NONE',  ( 19.03943276465977164, 0.05219959533936151252, 56.25109039468566863 ) ) ;
#60003=CARTESIAN_POINT ( 'NONE',  ( 4.379528057220092307, 16.55341960407617563, 37.29275706135235424 ) ) ;
#60004=CARTESIAN_POINT ( 'NONE',  ( -9.564922557960796823, -16.46253265017161027, 107.0822429386476955 ) ) ;
#60005=CARTESIAN_POINT ( 'NONE',  ( -16.51473224551069308, -9.474510206698971260, 76.66557627198103830 ) ) ;
#60006=CARTESIAN_POINT ( 'NONE',  ( -5.823673210054116645, -21.52544592524344225, 97.29057627198105251 ) ) ;
#60007=CARTESIAN_POINT ( 'NONE',  ( 5.153800228976615827, -19.02544592524334988, 65.20942372801900433 ) ) ;
#60008=CARTESIAN_POINT ( 'NONE',  ( -9.564922557960796823, -16.46253265017161027, 92.08224293864769550 ) ) ;
#60009=CARTESIAN_POINT ( 'NONE',  ( 17.50000000000114042, -3.530325368900714356, 21.94660113358420617 ) ) ;
#60010=CARTESIAN_POINT ( 'NONE',  ( -13.97604488694527625, -13.89961937509977652, 66.87390960531436690 ) ) ;
#60011=CARTESIAN_POINT ( 'NONE',  ( 8.314922557960818139, 14.29746914071049879, 39.58224293864769550 ) ) ;
#60013=CARTESIAN_POINT ( 'NONE',  ( -19.05341960407617563, 5.049401038297882671, 38.54275706135233293 ) ) ;
#60014=CARTESIAN_POINT ( 'NONE',  ( -8.224510206698948167, 14.34966873604960824, 75.41557627198102409 ) ) ;
#60015=CARTESIAN_POINT ( 'NONE',  ( -15.72974639402176322, -15.80617190586768395, 94.37609039468568994 ) ) ;
#60016=CARTESIAN_POINT ( 'NONE',  ( -16.46253265017160317, 9.564922557960807481, 40.83224293864769550 ) ) ;
#60017=CARTESIAN_POINT ( 'NONE',  ( 8.224510206698742110, 14.34966873604972548, 52.08442372801901854 ) ) ;
#60018=CARTESIAN_POINT ( 'NONE',  ( 8.224510206698953496, -14.34966873604960469, 37.91557627198102409 ) ) ;
#60019=CARTESIAN_POINT ( 'NONE',  ( 15.72974639402176855, 15.80617190586768217, 106.8760903946856899 ) ) ;
#60020=CARTESIAN_POINT ( 'NONE',  ( -5.153800228976328057, -19.02544592524343514, 92.29057627198099567 ) ) ;
#60021=CARTESIAN_POINT ( 'NONE',  ( -19.03943276465977164, 0.05219959533909376836, 96.24890960531436690 ) ) ;
#60022=CARTESIAN_POINT ( 'NONE',  ( -0.05219959533910754901, -16.53943276465976808, 102.4989096053143811 ) ) ;
#60023=CARTESIAN_POINT ( 'NONE',  ( -12.14591786802309592, -12.06949235617757132, 76.87390960531439532 ) ) ;
#60024=CARTESIAN_POINT ( 'NONE',  ( -21.53943276465977519, 0.05219959533907696930, 81.24890960531436690 ) ) ;
#60025=CARTESIAN_POINT ( 'NONE',  ( 0.05219959533909260263, 19.03943276465977164, 84.99890960531436690 ) ) ;
#60026=CARTESIAN_POINT ( 'NONE',  ( 15.72974639402199770, -15.80617190586745480, 103.1239096053143811 ) ) ;
#60027=CARTESIAN_POINT ( 'NONE',  ( -16.46253265017160317, 9.564922557960807481, 90.83224293864769550 ) ) ;
#60029=CARTESIAN_POINT ( 'NONE',  ( -17.58332526062528345, -7.635886036038592728, 64.07665040441534643 ) ) ;
#60030=CARTESIAN_POINT ( 'NONE',  ( -16.55341960407611168, -4.379528057220339221, 96.45724293864770971 ) ) ;
#60031=CARTESIAN_POINT ( 'NONE',  ( 9.474510206698971260, -16.51473224551069308, 57.91557627198103120 ) ) ;
#60032=CARTESIAN_POINT ( 'NONE',  ( 15.80617190586746368, 15.72974639402197994, 64.37390960531435269 ) ) ;
#60034=CARTESIAN_POINT ( 'NONE',  ( 14.29746914071037800, 8.314922557961029526, 106.6677570613523756 ) ) ;
#60036=CARTESIAN_POINT ( 'NONE',  ( 16.52544592524335698, 4.483927247898782831, 26.45942372801901854 ) ) ;
#60037=CARTESIAN_POINT ( 'NONE',  ( -12.06949235617756955, 12.14591786802309770, 85.62390960531436690 ) ) ;
#60039=CARTESIAN_POINT ( 'NONE',  ( -16.46253265017160317, 9.564922557960807481, 75.83224293864769550 ) ) ;
#60040=CARTESIAN_POINT ( 'NONE',  ( -19.02544592524342804, 5.153800228976336051, 41.04057627198103120 ) ) ;
#60041=CARTESIAN_POINT ( 'NONE',  ( 14.34966873604960469, 8.224510206698951720, 64.16557627198102409 ) ) ;
#60042=CARTESIAN_POINT ( 'NONE',  ( -21.55341960407610458, -5.719274019375992779, 21.45724293864769550 ) ) ;
#60043=CARTESIAN_POINT ( 'NONE',  ( 5.153800228976615827, -19.02544592524334988, 105.2094237280190185 ) ) ;
#60044=CARTESIAN_POINT ( 'NONE',  ( 15.72974639402176855, 15.80617190586768217, 56.87609039468568994 ) ) ;
#60045=CARTESIAN_POINT ( 'NONE',  ( 9.474510206698971260, -16.51473224551069308, 92.91557627198103830 ) ) ;
#60046=CARTESIAN_POINT ( 'NONE',  ( -18.62759615963270932, 10.81492255796079327, 75.83224293864769550 ) ) ;
#60047=CARTESIAN_POINT ( 'NONE',  ( -14.34966873604972548, 8.224510206698743886, 73.33442372801901854 ) ) ;
#60048=CARTESIAN_POINT ( 'NONE',  ( 5.049401038297881783, 19.05341960407617918, 107.2927570613523187 ) ) ;
#60049=CARTESIAN_POINT ( 'NONE',  ( 13.97604488694527802, 13.89961937509977652, 69.37390960531436690 ) ) ;
#60050=CARTESIAN_POINT ( 'NONE',  ( 5.719274019375991003, -21.55341960407610458, 82.70724293864770971 ) ) ;
#60051=CARTESIAN_POINT ( 'NONE',  ( -0.05219959533936034679, 19.03943276465977164, 107.5010903946856615 ) ) ;
#60052=CARTESIAN_POINT ( 'NONE',  ( -16.52544592524342804, 4.483927247898546575, 36.04057627198102409 ) ) ;
#60053=CARTESIAN_POINT ( 'NONE',  ( -15.72974639402176322, -15.80617190586768395, 59.37609039468568284 ) ) ;
#60054=CARTESIAN_POINT ( 'NONE',  ( 14.34966873604972726, -8.224510206698740333, 85.83442372801901854 ) ) ;
#60055=CARTESIAN_POINT ( 'NONE',  ( -19.05341960407611168, -5.049401038298163336, 101.4572429386476955 ) ) ;
#60056=CARTESIAN_POINT ( 'NONE',  ( -9.474510206698964154, 16.51473224551069663, 105.4155762719810383 ) ) ;
#60058=CARTESIAN_POINT ( 'NONE',  ( 4.483927247898790824, -16.52544592524335698, 90.20942372801903275 ) ) ;
#60059=CARTESIAN_POINT ( 'NONE',  ( 16.52544592524335698, 4.483927247898782831, 41.45942372801901143 ) ) ;
#60060=CARTESIAN_POINT ( 'NONE',  ( 9.474510206698971260, -16.51473224551069308, 62.91557627198102409 ) ) ;
#60061=CARTESIAN_POINT ( 'NONE',  ( -19.02544592524342804, 5.153800228976336051, 71.04057627198099567 ) ) ;
#60062=CARTESIAN_POINT ( 'NONE',  ( 18.67979575497194134, -10.72451020669871369, 70.83442372801901854 ) ) ;
#60063=CARTESIAN_POINT ( 'NONE',  ( -16.55341960407617563, 4.379528057220093196, 63.54275706135234003 ) ) ;
#60064=CARTESIAN_POINT ( 'NONE',  ( 16.52544592524342804, -4.483927247898539470, 48.54057627198103120 ) ) ;
#60065=CARTESIAN_POINT ( 'NONE',  ( -13.89961937509977652, 13.97604488694528158, 45.62390960531433848 ) ) ;
#60066=CARTESIAN_POINT ( 'NONE',  ( 16.51473224551069308, 9.474510206698969483, 49.16557627198102409 ) ) ;
#60067=CARTESIAN_POINT ( 'NONE',  ( -0.05219959533934338120, 16.53943276465976808, 37.50109039468568284 ) ) ;
#60068=CARTESIAN_POINT ( 'NONE',  ( -13.89961937509957401, -13.97604488694547875, 89.37609039468563310 ) ) ;
#60069=CARTESIAN_POINT ( 'NONE',  ( 8.224510206698953496, -14.34966873604960469, 102.9155762719810383 ) ) ;
#60070=CARTESIAN_POINT ( 'NONE',  ( -13.89961937509977652, 13.97604488694528158, 65.62390960531436690 ) ) ;
#60071=CARTESIAN_POINT ( 'NONE',  ( 19.05341960407617918, -5.049401038297876454, 91.04275706135234714 ) ) ;
#60073=CARTESIAN_POINT ( 'NONE',  ( 0.05219959533937995610, -21.53943276465977519, 95.00109039468568994 ) ) ;
#60074=CARTESIAN_POINT ( 'NONE',  ( 12.06949235617739724, 12.14591786802326823, 71.87609039468568994 ) ) ;
#60076=CARTESIAN_POINT ( 'NONE',  ( 0.05219959533907565091, 21.53943276465977519, 49.99890960531437401 ) ) ;
#60077=CARTESIAN_POINT ( 'NONE',  ( 16.53943276465976808, 0.05219959533934440121, 36.25109039468567573 ) ) ;
#60078=CARTESIAN_POINT ( 'NONE',  ( -19.05341960407611168, -5.049401038298164224, 36.45724293864768129 ) ) ;
#60079=CARTESIAN_POINT ( 'NONE',  ( -9.474510206698720793, -16.51473224551083518, 39.58442372801899722 ) ) ;
#60080=CARTESIAN_POINT ( 'NONE',  ( -9.474510206698964154, 16.51473224551069663, 90.41557627198103830 ) ) ;
#60081=CARTESIAN_POINT ( 'NONE',  ( 9.564922557960805705, 16.46253265017160317, 24.58224293864769194 ) ) ;
#60082=CARTESIAN_POINT ( 'NONE',  ( -16.46253265017160317, 9.564922557960807481, 50.83224293864770260 ) ) ;
#60084=CARTESIAN_POINT ( 'NONE',  ( -0.05219959533937732626, 21.53943276465977519, 77.50109039468567573 ) ) ;
#60086=CARTESIAN_POINT ( 'NONE',  ( 5.153800228976615827, -19.02544592524334988, 35.20942372801899722 ) ) ;
#60087=CARTESIAN_POINT ( 'NONE',  ( 19.02544592524334988, 5.153800228976608722, 26.45942372801899722 ) ) ;
#60088=CARTESIAN_POINT ( 'NONE',  ( -4.379528057220328563, 16.55341960407611168, 55.20724293864770260 ) ) ;
#60089=CARTESIAN_POINT ( 'NONE',  ( -19.05341960407611168, -5.049401038298163336, 61.45724293864769550 ) ) ;
#60090=CARTESIAN_POINT ( 'NONE',  ( 10.72451020669898902, -18.67979575497178502, 27.91557627198103830 ) ) ;
#60091=CARTESIAN_POINT ( 'NONE',  ( 10.72451020669871369, 18.67979575497193778, 77.08442372801901854 ) ) ;
#60092=CARTESIAN_POINT ( 'NONE',  ( 19.02544592524343514, -5.153800228976328945, 68.54057627198103830 ) ) ;
#60093=CARTESIAN_POINT ( 'NONE',  ( 18.62759615963255655, 10.81492255796105972, 76.66775706135234714 ) ) ;
#60094=CARTESIAN_POINT ( 'NONE',  ( -5.719274019375978568, 21.55341960407610458, 35.20724293864768839 ) ) ;
#60095=CARTESIAN_POINT ( 'NONE',  ( 18.67979575497194134, -10.72451020669871369, 35.83442372801901143 ) ) ;
#60096=CARTESIAN_POINT ( 'NONE',  ( 19.03943276465977164, 0.05219959533936151252, 61.25109039468566863 ) ) ;
#60097=CARTESIAN_POINT ( 'NONE',  ( -9.474510206698964154, 16.51473224551069663, 35.41557627198102409 ) ) ;
#60098=CARTESIAN_POINT ( 'NONE',  ( 19.05341960407611168, 5.049401038298154454, 73.95724293864768129 ) ) ;
#60099=CARTESIAN_POINT ( 'NONE',  ( -14.34966873604972548, 8.224510206698743886, 33.33442372801900433 ) ) ;
#60100=CARTESIAN_POINT ( 'NONE',  ( -8.314922557960811034, -14.29746914071050412, 87.08224293864769550 ) ) ;
#60101=CARTESIAN_POINT ( 'NONE',  ( 16.51473224551069308, 9.474510206698969483, 59.16557627198102409 ) ) ;
#60102=CARTESIAN_POINT ( 'NONE',  ( -15.72974639402197994, 15.80617190586746368, 40.62390960531435269 ) ) ;
#60103=CARTESIAN_POINT ( 'NONE',  ( 9.474510206698729675, 16.51473224551082808, 112.0844237280190043 ) ) ;
#60104=CARTESIAN_POINT ( 'NONE',  ( 10.81492255796106328, -18.62759615963255655, 20.41775706135234714 ) ) ;
#60105=CARTESIAN_POINT ( 'NONE',  ( 15.72974639402176855, 15.80617190586768217, 71.87609039468568994 ) ) ;
#60106=CARTESIAN_POINT ( 'NONE',  ( 4.483927247898790824, -16.52544592524335698, 70.20942372801904696 ) ) ;
#60107=CARTESIAN_POINT ( 'NONE',  ( -14.34966873604972548, 8.224510206698743886, 73.33442372801901854 ) ) ;
#60109=CARTESIAN_POINT ( 'NONE',  ( -19.03943276465977164, 0.05219959533909376836, 56.24890960531435979 ) ) ;
#60110=CARTESIAN_POINT ( 'NONE',  ( 14.29746914071037800, 8.314922557961029526, 86.66775706135234714 ) ) ;
#60111=CARTESIAN_POINT ( 'NONE',  ( 13.97604488694548053, -13.89961937509957401, 45.62609039468566863 ) ) ;
#60112=CARTESIAN_POINT ( 'NONE',  ( 5.719274019375673035, 21.55341960407619339, 22.29275706135235069 ) ) ;
#60113=CARTESIAN_POINT ( 'NONE',  ( -4.483927247898539470, -16.52544592524342804, 67.29057627198103830 ) ) ;
#60114=CARTESIAN_POINT ( 'NONE',  ( -19.02544592524342804, 5.153800228976336051, 81.04057627198103830 ) ) ;
#60115=CARTESIAN_POINT ( 'NONE',  ( 8.224510206698742110, 14.34966873604972548, 92.08442372801901854 ) ) ;
#60116=CARTESIAN_POINT ( 'NONE',  ( 21.53943276465977519, 0.05219959533937863772, 56.25109039468568284 ) ) ;
#60117=CARTESIAN_POINT ( 'NONE',  ( -8.314922557961024197, 14.29746914071037800, 37.91775706135235424 ) ) ;
#60118=CARTESIAN_POINT ( 'NONE',  ( 10.81492255796078972, 18.62759615963270932, 114.5822429386477097 ) ) ;
#60119=CARTESIAN_POINT ( 'NONE',  ( -14.34966873604960291, -8.224510206698953496, 61.66557627198103120 ) ) ;
#60120=EDGE_CURVE ( 'NONE', #29984, #192686, #139760, .T. ) ;
#60122=CARTESIAN_POINT ( 'NONE',  ( 10.81492255796078972, 18.62759615963270932, 104.5822429386477097 ) ) ;
#60123=CARTESIAN_POINT ( 'NONE',  ( -8.314922557960811034, -14.29746914071050412, 42.08224293864769550 ) ) ;
#60124=ORIENTED_EDGE ( 'NONE', *, *, #120600, .T. ) ;
#60126=CARTESIAN_POINT ( 'NONE',  ( 5.049401038298161559, -19.05341960407611168, 107.7072429386476955 ) ) ;
#60127=CARTESIAN_POINT ( 'NONE',  ( 10.81492255796106328, -18.62759615963255655, 35.41775706135234003 ) ) ;
#60128=CARTESIAN_POINT ( 'NONE',  ( -16.53943276465976808, 0.05219959533911058130, 46.24890960531435979 ) ) ;
#60129=CARTESIAN_POINT ( 'NONE',  ( -13.89961937509977652, 13.97604488694528158, 60.62390960531436690 ) ) ;
#60130=CARTESIAN_POINT ( 'NONE',  ( 19.03943276465977164, 0.05219959533936151252, 61.25109039468566863 ) ) ;
#60131=CARTESIAN_POINT ( 'NONE',  ( -9.474510206698964154, 16.51473224551069663, 95.41557627198102409 ) ) ;
#60132=CARTESIAN_POINT ( 'NONE',  ( -5.719274019375978568, 21.55341960407610458, 50.20724293864769550 ) ) ;
#60134=CARTESIAN_POINT ( 'NONE',  ( 19.03943276465977164, -0.05219959533909143690, 58.74890960531435979 ) ) ;
#60135=CARTESIAN_POINT ( 'NONE',  ( 14.34966873604972726, -8.224510206698740333, 30.83442372801902209 ) ) ;
#60136=CARTESIAN_POINT ( 'NONE',  ( 18.67979575497178502, 10.72451020669898547, 109.1655762719810383 ) ) ;
#60137=CARTESIAN_POINT ( 'NONE',  ( 4.483927247898545687, 16.52544592524342804, 49.79057627198102409 ) ) ;
#60139=CARTESIAN_POINT ( 'NONE',  ( -13.89961937509977652, 13.97604488694528158, 90.62390960531432427 ) ) ;
#60140=CARTESIAN_POINT ( 'NONE',  ( -5.823673210054116645, -21.52544592524344225, 67.29057627198103830 ) ) ;
#60141=CARTESIAN_POINT ( 'NONE',  ( -15.72974639402197994, 15.80617190586746368, 105.6239096053143669 ) ) ;
#60142=CARTESIAN_POINT ( 'NONE',  ( -14.34966873604972548, 8.224510206698743886, 38.33442372801900433 ) ) ;
#60143=CARTESIAN_POINT ( 'NONE',  ( -18.67979575497178146, -10.72451020669898902, 31.66557627198102054 ) ) ;
#60144=CARTESIAN_POINT ( 'NONE',  ( 18.62759615963255655, 10.81492255796105972, 101.6677570613523613 ) ) ;
#60145=CARTESIAN_POINT ( 'NONE',  ( -19.02544592524342804, 5.153800228976336051, 106.0405762719810241 ) ) ;
#60146=CARTESIAN_POINT ( 'NONE',  ( 16.51473224551069308, 9.474510206698969483, 39.16557627198103120 ) ) ;
#60147=CARTESIAN_POINT ( 'NONE',  ( -9.474510206698964154, 16.51473224551069663, 100.4155762719810241 ) ) ;
#60148=CARTESIAN_POINT ( 'NONE',  ( -13.97604488694527625, -13.89961937509977652, 81.87390960531436690 ) ) ;
#60150=CARTESIAN_POINT ( 'NONE',  ( 19.05341960407617918, -5.049401038297876454, 61.04275706135232582 ) ) ;
#60151=CARTESIAN_POINT ( 'NONE',  ( 19.02544592524334988, 5.153800228976608722, 21.45942372801899012 ) ) ;
#60152=CARTESIAN_POINT ( 'NONE',  ( -18.67979575497178146, -10.72451020669898902, 36.66557627198103120 ) ) ;
#60153=CARTESIAN_POINT ( 'NONE',  ( -12.14591786802326823, 12.06949235617739902, 108.1260903946856757 ) ) ;
#60154=CARTESIAN_POINT ( 'NONE',  ( -19.02544592524334988, -5.153800228976617603, 78.95942372801900433 ) ) ;
#60155=CARTESIAN_POINT ( 'NONE',  ( -16.52216118717209170, 7.221426719304504083, 58.92400978953009627 ) ) ;
#60156=CARTESIAN_POINT ( 'NONE',  ( -9.474510206698720793, -16.51473224551083518, 79.58442372801899012 ) ) ;
#60157=CARTESIAN_POINT ( 'NONE',  ( 19.03943276465977164, 0.05219959533936151252, 36.25109039468567573 ) ) ;
#60159=CARTESIAN_POINT ( 'NONE',  ( 5.049401038298161559, -19.05341960407611168, 37.70724293864768839 ) ) ;
#60160=CARTESIAN_POINT ( 'NONE',  ( 14.34966873604960469, 8.224510206698951720, 49.16557627198102409 ) ) ;
#60161=CARTESIAN_POINT ( 'NONE',  ( -17.13100169013300444, -6.664070546373134007, 109.2321016430015135 ) ) ;
#60162=CARTESIAN_POINT ( 'NONE',  ( 8.224510206698953496, -14.34966873604960469, 32.91557627198102409 ) ) ;
#60163=CARTESIAN_POINT ( 'NONE',  ( -17.49999999999999645, -5.500000000000000888, 22.00000000000000711 ) ) ;
#60164=CARTESIAN_POINT ( 'NONE',  ( 8.314922557961029526, -14.29746914071037800, 100.4177570613523471 ) ) ;
#60165=CARTESIAN_POINT ( 'NONE',  ( 16.46253265017160672, -9.564922557960803928, 48.33224293864769550 ) ) ;
#60166=CARTESIAN_POINT ( 'NONE',  ( 21.55341960407619695, -5.719274019375665929, 111.0427570613523613 ) ) ;
#60167=CARTESIAN_POINT ( 'NONE',  ( -5.049401038297874678, -19.05341960407617918, 109.7927570613523187 ) ) ;
#60168=CARTESIAN_POINT ( 'NONE',  ( -18.67979575497193778, 10.72451020669871902, 98.33442372801901854 ) ) ;
#60169=CARTESIAN_POINT ( 'NONE',  ( -9.564922557961040184, 16.46253265017147172, 67.91775706135233293 ) ) ;
#60170=CARTESIAN_POINT ( 'NONE',  ( 5.153800228976335163, 19.02544592524342804, 94.79057627198103830 ) ) ;
#60171=CARTESIAN_POINT ( 'NONE',  ( 13.97604488694527802, 13.89961937509977652, 89.37390960531436690 ) ) ;
#60173=CARTESIAN_POINT ( 'NONE',  ( 21.52544592524344225, -5.823673210054117533, 113.5405762719810383 ) ) ;
#60175=CARTESIAN_POINT ( 'NONE',  ( -14.29746914071049879, 8.314922557960819915, 85.83224293864768129 ) ) ;
#60176=CARTESIAN_POINT ( 'NONE',  ( 18.67979575497178502, 10.72451020669898547, 59.16557627198103120 ) ) ;
#60177=CARTESIAN_POINT ( 'NONE',  ( 5.153800228976335163, 19.02544592524342804, 59.79057627198100988 ) ) ;
#60178=CARTESIAN_POINT ( 'NONE',  ( 21.52544592524344225, -5.823673210054117533, 98.54057627198105251 ) ) ;
#60179=CARTESIAN_POINT ( 'NONE',  ( -8.314922557961024197, 14.29746914071037800, 92.91775706135236135 ) ) ;
#60181=CARTESIAN_POINT ( 'NONE',  ( 19.03943276465977164, -0.05219959533909143690, 58.74890960531435979 ) ) ;
#60182=CARTESIAN_POINT ( 'NONE',  ( -8.314922557960811034, -14.29746914071050412, 97.08224293864770971 ) ) ;
#60184=CARTESIAN_POINT ( 'NONE',  ( 0.05219959533909260263, 19.03943276465977164, 44.99890960531435979 ) ) ;
#60185=CARTESIAN_POINT ( 'NONE',  ( -9.564922557961040184, 16.46253265017147172, 82.91775706135233293 ) ) ;
#60186=CARTESIAN_POINT ( 'NONE',  ( -16.55341960407611168, -4.379528057220339221, 81.45724293864769550 ) ) ;
#60187=CARTESIAN_POINT ( 'NONE',  ( -21.53943276465977519, -0.05219959533937600094, 63.75109039468568284 ) ) ;
#60188=CARTESIAN_POINT ( 'NONE',  ( -19.05341960407611168, -5.049401038298163336, 36.45724293864766707 ) ) ;
#60189=CARTESIAN_POINT ( 'NONE',  ( 18.67979575497178502, 10.72451020669898547, 109.1655762719810383 ) ) ;
#60190=CARTESIAN_POINT ( 'NONE',  ( -14.29746914071049879, 8.314922557960819915, 105.8322429386476955 ) ) ;
#60192=CARTESIAN_POINT ( 'NONE',  ( -13.89961937509977652, 13.97604488694528158, 60.62390960531436690 ) ) ;
#60193=CARTESIAN_POINT ( 'NONE',  ( 19.34837522270365540, 5.499999999999731770, 48.36337684832581374 ) ) ;
#60194=CARTESIAN_POINT ( 'NONE',  ( 9.474510206698729675, 16.51473224551082808, 97.08442372801900433 ) ) ;
#60195=CARTESIAN_POINT ( 'NONE',  ( -9.474510206698964154, 16.51473224551069663, 110.4155762719810383 ) ) ;
#60196=CARTESIAN_POINT ( 'NONE',  ( 5.719274019375673035, 21.55341960407619339, 47.29275706135234003 ) ) ;
#60197=CARTESIAN_POINT ( 'NONE',  ( 9.564922557960805705, 16.46253265017160317, 84.58224293864769550 ) ) ;
#60198=CARTESIAN_POINT ( 'NONE',  ( -19.03943276465977164, -0.05219959533935918106, 73.75109039468566152 ) ) ;
#60199=CARTESIAN_POINT ( 'NONE',  ( -9.564922557960796823, -16.46253265017161027, 62.08224293864769550 ) ) ;
#60200=CARTESIAN_POINT ( 'NONE',  ( -0.05219959533910754901, -16.53943276465976808, 72.49890960531435269 ) ) ;
#60201=CARTESIAN_POINT ( 'NONE',  ( 14.34966873604960469, 8.224510206698951720, 69.16557627198102409 ) ) ;
#60202=CARTESIAN_POINT ( 'NONE',  ( 16.51473224551069308, 9.474510206698969483, 89.16557627198103830 ) ) ;
#60203=CARTESIAN_POINT ( 'NONE',  ( -0.05219959533910754901, -16.53943276465976808, 82.49890960531436690 ) ) ;
#60204=CARTESIAN_POINT ( 'NONE',  ( -13.97604488694527625, -13.89961937509977652, 86.87390960531436690 ) ) ;
#60205=CARTESIAN_POINT ( 'NONE',  ( 5.049401038297881783, 19.05341960407617563, 27.29275706135232937 ) ) ;
#60206=CARTESIAN_POINT ( 'NONE',  ( 19.05341960407611168, 5.049401038298154454, 48.95724293864768129 ) ) ;
#60207=CARTESIAN_POINT ( 'NONE',  ( 16.55341960407611168, 4.379528057220329451, 33.95724293864769550 ) ) ;
#60208=CARTESIAN_POINT ( 'NONE',  ( 16.52544592524342804, -4.483927247898539470, 108.5405762719810241 ) ) ;
#60210=CARTESIAN_POINT ( 'NONE',  ( -21.53943276465977519, -0.05219959533937600094, 38.75109039468567573 ) ) ;
#60211=CARTESIAN_POINT ( 'NONE',  ( 9.564922557961047289, -16.46253265017146816, 65.41775706135233293 ) ) ;
#60212=CARTESIAN_POINT ( 'NONE',  ( 16.52544592524342804, -4.483927247898539470, 38.54057627198103120 ) ) ;
#60213=CARTESIAN_POINT ( 'NONE',  ( 10.72451020669898902, -18.67979575497178502, 87.91557627198103830 ) ) ;
#60214=CARTESIAN_POINT ( 'NONE',  ( -10.72451020669898014, 18.67979575497178502, 25.41557627198103120 ) ) ;
#60215=CARTESIAN_POINT ( 'NONE',  ( 16.52544592524342804, -4.483927247898539470, 63.54057627198103830 ) ) ;
#60216=CARTESIAN_POINT ( 'NONE',  ( 9.474510206698971260, -16.51473224551069308, 47.91557627198102409 ) ) ;
#60217=CARTESIAN_POINT ( 'NONE',  ( -16.46253265017146816, -9.564922557961047289, 44.16775706135232582 ) ) ;
#60218=CARTESIAN_POINT ( 'NONE',  ( -14.29746914071037622, -8.314922557961029526, 99.16775706135234714 ) ) ;
#60219=CARTESIAN_POINT ( 'NONE',  ( -14.34966873604972548, 8.224510206698743886, 63.33442372801900433 ) ) ;
#60220=CARTESIAN_POINT ( 'NONE',  ( -18.67979575497178146, -10.72451020669898902, 31.66557627198102054 ) ) ;
#60221=CARTESIAN_POINT ( 'NONE',  ( 15.72974639402176855, 15.80617190586768217, 101.8760903946857042 ) ) ;
#60222=CARTESIAN_POINT ( 'NONE',  ( 19.03943276465977164, -0.05219959533909143690, 88.74890960531436690 ) ) ;
#60224=CARTESIAN_POINT ( 'NONE',  ( 0.05219959533934541429, -16.53943276465976808, 70.00109039468568994 ) ) ;
#60225=CARTESIAN_POINT ( 'NONE',  ( -0.05219959533909027116, -19.03943276465977164, 22.49890960531436690 ) ) ;
#60226=CARTESIAN_POINT ( 'NONE',  ( -0.05219959533910754901, -16.53943276465976808, 32.49890960531435979 ) ) ;
#60227=CARTESIAN_POINT ( 'NONE',  ( 16.51473224551069308, 9.474510206698969483, 104.1655762719810241 ) ) ;
#60228=CARTESIAN_POINT ( 'NONE',  ( -0.05219959533909027116, -19.03943276465977164, 97.49890960531436690 ) ) ;
#60229=CARTESIAN_POINT ( 'NONE',  ( 21.53943276465977519, -0.05219959533907433946, 33.74890960531436690 ) ) ;
#60230=CARTESIAN_POINT ( 'NONE',  ( -4.379528057220328563, 16.55341960407611168, 65.20724293864768129 ) ) ;
#60231=CARTESIAN_POINT ( 'NONE',  ( 8.224510206698953496, -14.34966873604960469, 32.91557627198102409 ) ) ;
#60232=CARTESIAN_POINT ( 'NONE',  ( -16.53943276465976808, 0.05219959533911058130, 46.24890960531435979 ) ) ;
#60233=CARTESIAN_POINT ( 'NONE',  ( 12.06949235617739724, 12.14591786802326823, 51.87609039468568284 ) ) ;
#60234=CARTESIAN_POINT ( 'NONE',  ( -9.474510206698720793, -16.51473224551083518, 59.58442372801900433 ) ) ;
#60235=CARTESIAN_POINT ( 'NONE',  ( 5.049401038297881783, 19.05341960407617563, 52.29275706135234003 ) ) ;
#60236=CARTESIAN_POINT ( 'NONE',  ( 9.564922557960805705, 16.46253265017160317, 89.58224293864769550 ) ) ;
#60237=CARTESIAN_POINT ( 'NONE',  ( -19.05341960407617563, 5.049401038297882671, 68.54275706135230450 ) ) ;
#60239=CARTESIAN_POINT ( 'NONE',  ( 5.049401038297881783, 19.05341960407617563, 62.29275706135234003 ) ) ;
#60240=CARTESIAN_POINT ( 'NONE',  ( -19.03943276465977164, -0.05219959533935918106, 93.75109039468566152 ) ) ;
#60241=CARTESIAN_POINT ( 'NONE',  ( -16.52544592524335698, -4.483927247898792601, 83.95942372801900433 ) ) ;
#60243=CARTESIAN_POINT ( 'NONE',  ( -9.564922557960796823, -16.46253265017161027, 32.08224293864769550 ) ) ;
#60244=CARTESIAN_POINT ( 'NONE',  ( -21.53943276465977519, 0.05219959533907696930, 26.24890960531435624 ) ) ;
#60245=CARTESIAN_POINT ( 'NONE',  ( 0.05219959533937995610, -21.53943276465977519, 40.00109039468567573 ) ) ;
#60246=CARTESIAN_POINT ( 'NONE',  ( -13.97604488694547697, 13.89961937509957934, 103.1260903946856473 ) ) ;
#60247=CARTESIAN_POINT ( 'NONE',  ( 17.50000000000000000, -3.345213924137362849, 107.0876862309434614 ) ) ;
#60248=CARTESIAN_POINT ( 'NONE',  ( -5.153800228976328057, -19.02544592524343514, 57.29057627198103120 ) ) ;
#60249=CARTESIAN_POINT ( 'NONE',  ( -16.51473224551069308, -9.474510206698971260, 106.6655762719810383 ) ) ;
#60250=CARTESIAN_POINT ( 'NONE',  ( -8.314922557960811034, -14.29746914071050412, 72.08224293864769550 ) ) ;
#60251=CARTESIAN_POINT ( 'NONE',  ( 9.474510206698971260, -16.51473224551069308, 57.91557627198103120 ) ) ;
#60252=CARTESIAN_POINT ( 'NONE',  ( -5.049401038298153566, 19.05341960407611168, 70.20724293864769550 ) ) ;
#60253=CARTESIAN_POINT ( 'NONE',  ( -13.89961937509957401, -13.97604488694547875, 79.37609039468567573 ) ) ;
#60254=CARTESIAN_POINT ( 'NONE',  ( 5.823673210054125526, 21.52544592524343514, 49.79057627198102409 ) ) ;
#60255=CARTESIAN_POINT ( 'NONE',  ( 4.483927247898545687, 16.52544592524342804, 114.7905762719810383 ) ) ;
#60256=CARTESIAN_POINT ( 'NONE',  ( -16.46253265017146816, -9.564922557961047289, 39.16775706135234003 ) ) ;
#60257=CARTESIAN_POINT ( 'NONE',  ( -9.564922557960796823, -16.46253265017161027, 82.08224293864768129 ) ) ;
#60258=CARTESIAN_POINT ( 'NONE',  ( -5.719274019375978568, 21.55341960407610458, 80.20724293864769550 ) ) ;
#60259=CARTESIAN_POINT ( 'NONE',  ( -0.05219959533910754901, -16.53943276465976808, 77.49890960531433848 ) ) ;
#60260=CARTESIAN_POINT ( 'NONE',  ( 5.049401038297881783, 19.05341960407617563, 52.29275706135234003 ) ) ;
#60261=CARTESIAN_POINT ( 'NONE',  ( 10.72451020669898902, -18.67979575497178502, 72.91557627198103830 ) ) ;
#60262=CARTESIAN_POINT ( 'NONE',  ( 21.52544592524344225, -5.823673210054117533, 63.54057627198103830 ) ) ;
#60263=CARTESIAN_POINT ( 'NONE',  ( -0.05219959533907301413, -21.53943276465977519, 37.49890960531436690 ) ) ;
#60264=CARTESIAN_POINT ( 'NONE',  ( 5.719274019375673035, 21.55341960407619339, 87.29275706135236135 ) ) ;
#60265=CARTESIAN_POINT ( 'NONE',  ( 16.51473224551069308, 9.474510206698969483, 64.16557627198102409 ) ) ;
#60266=CARTESIAN_POINT ( 'NONE',  ( 16.53943276465976808, -0.05219959533910856209, 113.7489096053143527 ) ) ;
#60267=CARTESIAN_POINT ( 'NONE',  ( 21.53943276465977519, 0.05219959533937863772, 31.25109039468568639 ) ) ;
#60268=CARTESIAN_POINT ( 'NONE',  ( 5.823673210054444382, -21.52544592524334988, 35.20942372801901854 ) ) ;
#60269=CARTESIAN_POINT ( 'NONE',  ( 19.03943276465977164, -0.05219959533909143690, 28.74890960531435624 ) ) ;
#60270=CARTESIAN_POINT ( 'NONE',  ( -5.823673210054116645, -21.52544592524344225, 102.2905762719810383 ) ) ;
#60271=CARTESIAN_POINT ( 'NONE',  ( 9.474510206698729675, 16.51473224551082808, 42.08442372801900433 ) ) ;
#60272=CARTESIAN_POINT ( 'NONE',  ( 16.51473224551069308, 9.474510206698969483, 34.16557627198102409 ) ) ;
#60273=CARTESIAN_POINT ( 'NONE',  ( 16.52544592524335698, 4.483927247898782831, 26.45942372801901854 ) ) ;
#60275=CARTESIAN_POINT ( 'NONE',  ( -16.53943276465976808, -0.05219959533934237506, 63.75109039468568284 ) ) ;
#60276=CARTESIAN_POINT ( 'NONE',  ( 13.89961937509977652, -13.97604488694527269, 33.12390960531434558 ) ) ;
#60278=CARTESIAN_POINT ( 'NONE',  ( 9.474510206698971260, -16.51473224551069308, 82.91557627198103830 ) ) ;
#60279=CARTESIAN_POINT ( 'NONE',  ( 12.06949235617757843, -12.14591786802309237, 103.1239096053143811 ) ) ;
#60280=CARTESIAN_POINT ( 'NONE',  ( 5.823673210054125526, 21.52544592524343514, 54.79057627198104541 ) ) ;
#60281=CARTESIAN_POINT ( 'NONE',  ( 4.379528057220092307, 16.55341960407617563, 42.29275706135235424 ) ) ;
#60282=CARTESIAN_POINT ( 'NONE',  ( 21.55341960407619695, -5.719274019375665929, 101.0427570613523756 ) ) ;
#60283=CARTESIAN_POINT ( 'NONE',  ( 9.564922557960805705, 16.46253265017160317, 44.58224293864769550 ) ) ;
#60284=CARTESIAN_POINT ( 'NONE',  ( -4.379528057220086978, -16.55341960407618274, 104.7927570613523898 ) ) ;
#60285=CARTESIAN_POINT ( 'NONE',  ( -12.14591786802309592, -12.06949235617757132, 56.87390960531436690 ) ) ;
#60286=CARTESIAN_POINT ( 'NONE',  ( 19.05341960407611168, 5.049401038298154454, 63.95724293864769550 ) ) ;
#60287=CARTESIAN_POINT ( 'NONE',  ( -5.719274019375665041, -21.55341960407619695, 104.7927570613523898 ) ) ;
#60288=CARTESIAN_POINT ( 'NONE',  ( -15.72974639402197994, 15.80617190586746368, 115.6239096053143669 ) ) ;
#60289=CARTESIAN_POINT ( 'NONE',  ( 15.72974639402176855, 15.80617190586768217, 71.87609039468568994 ) ) ;
#60290=CARTESIAN_POINT ( 'NONE',  ( -0.05219959533934338120, 16.53943276465976808, 52.50109039468567573 ) ) ;
#60291=CARTESIAN_POINT ( 'NONE',  ( 16.52544592524335698, 4.483927247898782831, 26.45942372801901854 ) ) ;
#60292=CARTESIAN_POINT ( 'NONE',  ( 8.314922557960818139, 14.29746914071049879, 79.58224293864769550 ) ) ;
#60293=CARTESIAN_POINT ( 'NONE',  ( -18.62759615963255300, -10.81492255796106328, 94.16775706135237556 ) ) ;
#60294=CARTESIAN_POINT ( 'NONE',  ( 0.05219959533910956823, 16.53943276465976808, 39.99890960531436690 ) ) ;
#60295=CARTESIAN_POINT ( 'NONE',  ( -17.44279575226824974, 5.990770900252412545, 115.8355756751432182 ) ) ;
#60296=CARTESIAN_POINT ( 'NONE',  ( -16.52544592524335698, -4.483927247898792601, 38.95942372801901854 ) ) ;
#60297=CARTESIAN_POINT ( 'NONE',  ( 0.05219959533910956823, 16.53943276465976808, 59.99890960531436690 ) ) ;
#60298=CARTESIAN_POINT ( 'NONE',  ( -4.483927247898782831, 16.52544592524335698, 87.70942372801901854 ) ) ;
#60299=CARTESIAN_POINT ( 'NONE',  ( 19.02544592524343514, -5.153800228976328945, 93.54057627198102409 ) ) ;
#60300=CARTESIAN_POINT ( 'NONE',  ( -13.97604488694527625, -13.89961937509977652, 111.8739096053143243 ) ) ;
#60301=CARTESIAN_POINT ( 'NONE',  ( -10.81492255796105439, 18.62759615963255655, 97.91775706135236135 ) ) ;
#60302=CARTESIAN_POINT ( 'NONE',  ( -4.483927247898782831, 16.52544592524335698, 107.7094237280190328 ) ) ;
#60303=CARTESIAN_POINT ( 'NONE',  ( 16.53943276465976808, -0.05219959533910856209, 83.74890960531435269 ) ) ;
#60304=CARTESIAN_POINT ( 'NONE',  ( -16.46253265017160317, 9.564922557960807481, 95.83224293864769550 ) ) ;
#60306=CARTESIAN_POINT ( 'NONE',  ( -4.379528057220086978, -16.55341960407618274, 44.79275706135234714 ) ) ;
#60307=CARTESIAN_POINT ( 'NONE',  ( -9.564922557960796823, -16.46253265017161027, 42.08224293864769550 ) ) ;
#60308=CARTESIAN_POINT ( 'NONE',  ( 9.474510206698971260, -16.51473224551069308, 102.9155762719810241 ) ) ;
#60309=CARTESIAN_POINT ( 'NONE',  ( -4.379528057220086978, -16.55341960407618274, 49.79275706135234714 ) ) ;
#60311=CARTESIAN_POINT ( 'NONE',  ( -0.05219959533936034679, 19.03943276465977164, 32.50109039468566863 ) ) ;
#60312=CARTESIAN_POINT ( 'NONE',  ( -16.46253265017160317, 9.564922557960807481, 40.83224293864769550 ) ) ;
#60313=CARTESIAN_POINT ( 'NONE',  ( 16.52544592524335698, 4.483927247898782831, 81.45942372801900433 ) ) ;
#60314=CARTESIAN_POINT ( 'NONE',  ( 5.049401038297881783, 19.05341960407617563, 87.29275706135234714 ) ) ;
#60315=CARTESIAN_POINT ( 'NONE',  ( -16.51473224551082808, 9.474510206698731452, 23.33442372801900078 ) ) ;
#60316=CARTESIAN_POINT ( 'NONE',  ( 19.03943276465977164, -0.05219959533909143690, 58.74890960531435979 ) ) ;
#60317=CARTESIAN_POINT ( 'NONE',  ( -8.314922557960811034, -14.29746914071050412, 97.08224293864770971 ) ) ;
#60320=CARTESIAN_POINT ( 'NONE',  ( -19.05341960407617563, 5.049401038297882671, 63.54275706135234003 ) ) ;
#60321=CARTESIAN_POINT ( 'NONE',  ( -15.80617190586745835, -15.72974639402198527, 61.87390960531436690 ) ) ;
#60322=CARTESIAN_POINT ( 'NONE',  ( -9.474510206698720793, -16.51473224551083518, 29.58442372801900433 ) ) ;
#60323=CARTESIAN_POINT ( 'NONE',  ( 5.153800228976335163, 19.02544592524342804, 104.7905762719809957 ) ) ;
#60324=CARTESIAN_POINT ( 'NONE',  ( -18.67979575497178146, -10.72451020669898902, 71.66557627198100988 ) ) ;
#60325=CARTESIAN_POINT ( 'NONE',  ( -13.89961937509977652, 13.97604488694528158, 105.6239096053143527 ) ) ;
#60327=CARTESIAN_POINT ( 'NONE',  ( -19.03943276465977164, -0.05219959533935918106, 98.75109039468567573 ) ) ;
#60328=CARTESIAN_POINT ( 'NONE',  ( -5.153800228976328057, -19.02544592524343514, 112.2905762719810099 ) ) ;
#60329=CARTESIAN_POINT ( 'NONE',  ( 0.05219959533934541429, -16.53943276465976808, 25.00109039468567218 ) ) ;
#60330=CARTESIAN_POINT ( 'NONE',  ( 19.03943276465977164, -0.05219959533909143690, 28.74890960531435624 ) ) ;
#60331=CARTESIAN_POINT ( 'NONE',  ( 9.474510206698971260, -16.51473224551069308, 92.91557627198103830 ) ) ;
#60332=CARTESIAN_POINT ( 'NONE',  ( -21.52544592524343514, 5.823673210054127303, 86.04057627198102409 ) ) ;
#60333=CARTESIAN_POINT ( 'NONE',  ( 21.55341960407619695, -5.719274019375665929, 66.04275706135236135 ) ) ;
#60334=CARTESIAN_POINT ( 'NONE',  ( -13.97604488694547697, 13.89961937509957934, 108.1260903946856331 ) ) ;
#60335=CARTESIAN_POINT ( 'NONE',  ( -21.55341960407619339, 5.719274019375674811, 108.5427570613523756 ) ) ;
#60336=CARTESIAN_POINT ( 'NONE',  ( 0.05219959533934541429, -16.53943276465976808, 110.0010903946856757 ) ) ;
#60337=CARTESIAN_POINT ( 'NONE',  ( -10.81492255796078084, -18.62759615963271287, 107.0822429386476955 ) ) ;
#60338=CARTESIAN_POINT ( 'NONE',  ( -14.29746914071049879, 8.314922557960819915, 30.83224293864770260 ) ) ;
#60339=CARTESIAN_POINT ( 'NONE',  ( 13.97604488694548053, -13.89961937509957401, 80.62609039468567573 ) ) ;
#60340=CARTESIAN_POINT ( 'NONE',  ( -16.51473224551082808, 9.474510206698731452, 58.33442372801900433 ) ) ;
#60341=CARTESIAN_POINT ( 'NONE',  ( -18.62759615963255300, -10.81492255796106328, 59.16775706135234714 ) ) ;
#60342=CARTESIAN_POINT ( 'NONE',  ( -9.474510206698720793, -16.51473224551083518, 39.58442372801899722 ) ) ;
#60343=CARTESIAN_POINT ( 'NONE',  ( 8.314922557960818139, 14.29746914071049879, 109.5822429386476955 ) ) ;
#60344=CARTESIAN_POINT ( 'NONE',  ( 15.80617190586746368, 15.72974639402197994, 29.37390960531435269 ) ) ;
#60345=CARTESIAN_POINT ( 'NONE',  ( -8.224510206698948167, 14.34966873604960824, 35.41557627198102409 ) ) ;
#60346=CARTESIAN_POINT ( 'NONE',  ( 21.53943276465977519, 0.05219959533937863772, 96.25109039468568994 ) ) ;
#60347=CARTESIAN_POINT ( 'NONE',  ( 14.29746914071037800, 8.314922557961029526, 71.66775706135234714 ) ) ;
#60348=CARTESIAN_POINT ( 'NONE',  ( 16.52544592524342804, -4.483927247898539470, 23.54057627198102765 ) ) ;
#60349=CARTESIAN_POINT ( 'NONE',  ( 21.53943276465977519, 0.05219959533937863772, 61.25109039468567573 ) ) ;
#60350=CARTESIAN_POINT ( 'NONE',  ( 21.52544592524334988, 5.823673210054432836, 71.45942372801901854 ) ) ;
#60351=CARTESIAN_POINT ( 'NONE',  ( 0.05219959533907565091, 21.53943276465977519, 64.99890960531435269 ) ) ;
#60354=CARTESIAN_POINT ( 'NONE',  ( -5.153800228976328057, -19.02544592524343514, 62.29057627198102409 ) ) ;
#60355=CARTESIAN_POINT ( 'NONE',  ( 21.55341960407619695, -5.719274019375665929, 41.04275706135236135 ) ) ;
#60356=CARTESIAN_POINT ( 'NONE',  ( -16.51473224551069308, -9.474510206698971260, 21.66557627198102765 ) ) ;
#60357=CARTESIAN_POINT ( 'NONE',  ( 9.474510206698971260, -16.51473224551069308, 42.91557627198103120 ) ) ;
#60358=CARTESIAN_POINT ( 'NONE',  ( 8.224510206698953496, -14.34966873604960469, 77.91557627198102409 ) ) ;
#60359=CARTESIAN_POINT ( 'NONE',  ( -9.474510206698964154, 16.51473224551069663, 80.41557627198103830 ) ) ;
#60360=CARTESIAN_POINT ( 'NONE',  ( -8.314922557960811034, -14.29746914071050412, 27.08224293864769550 ) ) ;
#60361=CARTESIAN_POINT ( 'NONE',  ( 21.53943276465977519, -0.05219959533907433946, 68.74890960531435269 ) ) ;
#60363=CARTESIAN_POINT ( 'NONE',  ( -21.55341960407610458, -5.719274019375992779, 106.4572429386477097 ) ) ;
#60364=CARTESIAN_POINT ( 'NONE',  ( 5.153800228976335163, 19.02544592524342804, 104.7905762719809957 ) ) ;
#60365=CARTESIAN_POINT ( 'NONE',  ( 16.51473224551069308, 9.474510206698969483, 69.16557627198102409 ) ) ;
#60366=CARTESIAN_POINT ( 'NONE',  ( -19.03943276465977164, -0.05219959533935918106, 103.7510903946856757 ) ) ;
#60367=CARTESIAN_POINT ( 'NONE',  ( 10.72451020669898902, -18.67979575497178502, 62.91557627198102409 ) ) ;
#60368=CARTESIAN_POINT ( 'NONE',  ( 21.52544592524334988, 5.823673210054432836, 86.45942372801901854 ) ) ;
#60369=CARTESIAN_POINT ( 'NONE',  ( -9.474510206698964154, 16.51473224551069663, 65.41557627198102409 ) ) ;
#60370=CARTESIAN_POINT ( 'NONE',  ( -19.03943276465977164, 0.05219959533909376836, 101.2489096053143669 ) ) ;
#60371=CARTESIAN_POINT ( 'NONE',  ( 16.53943276465976808, 0.05219959533934440121, 71.25109039468568994 ) ) ;
#60372=CARTESIAN_POINT ( 'NONE',  ( 21.55341960407619695, -5.719274019375665929, 51.04275706135234714 ) ) ;
#60373=CARTESIAN_POINT ( 'NONE',  ( 5.719274019375673035, 21.55341960407619339, 82.29275706135234714 ) ) ;
#60374=CARTESIAN_POINT ( 'NONE',  ( 21.52544592524334988, 5.823673210054432836, 21.45942372801901499 ) ) ;
#60375=CARTESIAN_POINT ( 'NONE',  ( -21.55341960407610458, -5.719274019375992779, 71.45724293864769550 ) ) ;
#60376=CARTESIAN_POINT ( 'NONE',  ( 19.02544592524334988, 5.153800228976608722, 51.45942372801900433 ) ) ;
#60377=CARTESIAN_POINT ( 'NONE',  ( -15.80617190586745835, -15.72974639402198527, 46.87390960531435979 ) ) ;
#60378=CARTESIAN_POINT ( 'NONE',  ( 19.05341960407611168, 5.049401038298154454, 78.95724293864769550 ) ) ;
#60379=CARTESIAN_POINT ( 'NONE',  ( -4.379528057220328563, 16.55341960407611168, 30.20724293864769550 ) ) ;
#60380=CARTESIAN_POINT ( 'NONE',  ( -16.88567814943165857, 6.947325034625572826, 63.70998877347415146 ) ) ;
#60381=CARTESIAN_POINT ( 'NONE',  ( 9.564922557960805705, 16.46253265017160317, 114.5822429386476955 ) ) ;
#60383=CARTESIAN_POINT ( 'NONE',  ( 0.05219959533936267826, -19.03943276465977164, 90.00109039468567573 ) ) ;
#60384=CARTESIAN_POINT ( 'NONE',  ( -18.62759615963270932, 10.81492255796079327, 75.83224293864769550 ) ) ;
#60385=CARTESIAN_POINT ( 'NONE',  ( 12.14591786802309770, 12.06949235617756955, 54.37390960531435979 ) ) ;
#60386=CARTESIAN_POINT ( 'NONE',  ( 12.14591786802327356, -12.06949235617739191, 25.62609039468567929 ) ) ;
#60387=CARTESIAN_POINT ( 'NONE',  ( -19.03943276465977164, 0.05219959533909376836, 46.24890960531435979 ) ) ;
#60388=CARTESIAN_POINT ( 'NONE',  ( -15.72974639402197994, 15.80617190586746368, 105.6239096053143669 ) ) ;
#60389=CARTESIAN_POINT ( 'NONE',  ( -0.05219959533936034679, 19.03943276465977164, 67.50109039468566152 ) ) ;
#60390=CARTESIAN_POINT ( 'NONE',  ( -9.474510206698964154, 16.51473224551069663, 85.41557627198102409 ) ) ;
#60391=CARTESIAN_POINT ( 'NONE',  ( 12.14591786802309770, 12.06949235617756955, 89.37390960531435269 ) ) ;
#60392=CARTESIAN_POINT ( 'NONE',  ( 19.05341960407611168, 5.049401038298154454, 63.95724293864769550 ) ) ;
#60393=CARTESIAN_POINT ( 'NONE',  ( 14.29746914071049879, -8.314922557960816363, 73.33224293864769550 ) ) ;
#60394=CARTESIAN_POINT ( 'NONE',  ( 19.02544592524343514, -5.153800228976328945, 38.54057627198103120 ) ) ;
#60396=CARTESIAN_POINT ( 'NONE',  ( -0.05219959533910754901, -16.53943276465976808, 42.49890960531435979 ) ) ;
#60397=CARTESIAN_POINT ( 'NONE',  ( -5.049401038298153566, 19.05341960407611168, 85.20724293864766707 ) ) ;
#60399=CARTESIAN_POINT ( 'NONE',  ( 13.97604488694548053, -13.89961937509957401, 50.62609039468566152 ) ) ;
#60400=CARTESIAN_POINT ( 'NONE',  ( 16.52544592524335698, 4.483927247898782831, 56.45942372801902565 ) ) ;
#60401=CARTESIAN_POINT ( 'NONE',  ( -10.81492255796078084, -18.62759615963271287, 82.08224293864768129 ) ) ;
#60402=CARTESIAN_POINT ( 'NONE',  ( 16.51473224551083163, -9.474510206698727899, 35.83442372801899722 ) ) ;
#60403=CARTESIAN_POINT ( 'NONE',  ( -13.97604488694527625, -13.89961937509977652, 86.87390960531436690 ) ) ;
#60405=CARTESIAN_POINT ( 'NONE',  ( -10.81492255796078084, -18.62759615963271287, 22.08224293864769194 ) ) ;
#60406=CARTESIAN_POINT ( 'NONE',  ( 13.89961937509977652, -13.97604488694527269, 58.12390960531436690 ) ) ;
#60407=CARTESIAN_POINT ( 'NONE',  ( -10.72451020669870658, -18.67979575497194134, 49.58442372801901143 ) ) ;
#60408=CARTESIAN_POINT ( 'NONE',  ( -13.89961937509977652, 13.97604488694528158, 30.62390960531435269 ) ) ;
#60409=CARTESIAN_POINT ( 'NONE',  ( -10.72451020669898014, 18.67979575497178502, 110.4155762719810383 ) ) ;
#60410=CARTESIAN_POINT ( 'NONE',  ( 0.05219959533909260263, 19.03943276465977164, 99.99890960531436690 ) ) ;
#60411=ORIENTED_EDGE ( 'NONE', *, *, #143390, .T. ) ;
#60412=CARTESIAN_POINT ( 'NONE',  ( -21.52544592524334988, -5.823673210054445271, 38.95942372801901854 ) ) ;
#60413=ORIENTED_EDGE ( 'NONE', *, *, #160688, .F. ) ;
#60414=CARTESIAN_POINT ( 'NONE',  ( -5.049401038298153566, 19.05341960407611168, 100.2072429386476955 ) ) ;
#60416=CARTESIAN_POINT ( 'NONE',  ( -15.80617190586745835, -15.72974639402198527, 111.8739096053143669 ) ) ;
#60417=CARTESIAN_POINT ( 'NONE',  ( 16.46253265017160672, -9.564922557960803928, 53.33224293864768839 ) ) ;
#60418=CARTESIAN_POINT ( 'NONE',  ( 12.14591786802327356, -12.06949235617739191, 30.62609039468567929 ) ) ;
#60420=CARTESIAN_POINT ( 'NONE',  ( 5.049401038298161559, -19.05341960407611168, 27.70724293864769550 ) ) ;
#60421=CARTESIAN_POINT ( 'NONE',  ( -0.05219959533937732626, 21.53943276465977519, 97.50109039468567573 ) ) ;
#60422=CARTESIAN_POINT ( 'NONE',  ( -9.564922557960796823, -16.46253265017161027, 82.08224293864768129 ) ) ;
#60423=CARTESIAN_POINT ( 'NONE',  ( -15.72974639402176322, -15.80617190586768395, 54.37609039468568994 ) ) ;
#60425=CARTESIAN_POINT ( 'NONE',  ( -19.02544592524342804, 5.153800228976336051, 101.0405762719810241 ) ) ;
#60427=CARTESIAN_POINT ( 'NONE',  ( -8.224510206698735004, -14.34966873604973081, 44.58442372801901854 ) ) ;
#60428=CARTESIAN_POINT ( 'NONE',  ( 8.224510206698742110, 14.34966873604972548, 72.08442372801899012 ) ) ;
#60429=CARTESIAN_POINT ( 'NONE',  ( -10.81492255796105439, 18.62759615963255655, 62.91775706135236135 ) ) ;
#60430=CARTESIAN_POINT ( 'NONE',  ( 5.823673210054444382, -21.52544592524334988, 85.20942372801901854 ) ) ;
#60432=CARTESIAN_POINT ( 'NONE',  ( 13.89961937509957401, 13.97604488694547697, 106.8760903946856757 ) ) ;
#60433=CARTESIAN_POINT ( 'NONE',  ( 9.564922557960805705, 16.46253265017160317, 79.58224293864769550 ) ) ;
#60434=CARTESIAN_POINT ( 'NONE',  ( -16.46253265017160317, 9.564922557960807481, 95.83224293864769550 ) ) ;
#60435=CARTESIAN_POINT ( 'NONE',  ( 16.46253265017160672, -9.564922557960803928, 23.33224293864769194 ) ) ;
#60436=CARTESIAN_POINT ( 'NONE',  ( 18.62759615963271287, -10.81492255796078972, 33.33224293864769550 ) ) ;
#60437=CARTESIAN_POINT ( 'NONE',  ( -8.314922557961024197, 14.29746914071037800, 97.91775706135236135 ) ) ;
#60438=CARTESIAN_POINT ( 'NONE',  ( -4.483927247898539470, -16.52544592524342804, 72.29057627198102409 ) ) ;
#60439=CARTESIAN_POINT ( 'NONE',  ( -19.03943276465977164, 0.05219959533909376836, 61.24890960531436690 ) ) ;
#60440=CARTESIAN_POINT ( 'NONE',  ( -18.62759615963255300, -10.81492255796106328, 94.16775706135237556 ) ) ;
#60442=CARTESIAN_POINT ( 'NONE',  ( -19.03943276465977164, -0.05219959533935918106, 103.7510903946856757 ) ) ;
#60443=CARTESIAN_POINT ( 'NONE',  ( -8.314922557960811034, -14.29746914071050412, 77.08224293864769550 ) ) ;
#60444=CARTESIAN_POINT ( 'NONE',  ( 10.72451020669871369, 18.67979575497193778, 27.08442372801901854 ) ) ;
#60445=CARTESIAN_POINT ( 'NONE',  ( -0.05219959533907301413, -21.53943276465977519, 62.49890960531436690 ) ) ;
#60446=CARTESIAN_POINT ( 'NONE',  ( -16.51473224551082808, 9.474510206698731452, 38.33442372801899722 ) ) ;
#60448=CARTESIAN_POINT ( 'NONE',  ( -13.97604488694527625, -13.89961937509977652, 81.87390960531436690 ) ) ;
#60449=CARTESIAN_POINT ( 'NONE',  ( -12.06949235617756955, 12.14591786802309770, 50.62390960531435979 ) ) ;
#60450=VECTOR ( 'NONE', #54278, 1000.000000000000000 ) ;
#60451=CARTESIAN_POINT ( 'NONE',  ( 8.314922557960818139, 14.29746914071049879, 39.58224293864769550 ) ) ;
#60452=CARTESIAN_POINT ( 'NONE',  ( 8.314922557961029526, -14.29746914071037800, 100.4177570613523471 ) ) ;
#60453=CARTESIAN_POINT ( 'NONE',  ( -9.474510206698720793, -16.51473224551083518, 54.58442372801899722 ) ) ;
#60454=CARTESIAN_POINT ( 'NONE',  ( -13.97604488694547520, 13.89961937509957934, 78.12609039468566152 ) ) ;
#60455=CARTESIAN_POINT ( 'NONE',  ( 19.02544592524343514, -5.153800228976328945, 103.5405762719809957 ) ) ;
#60456=CARTESIAN_POINT ( 'NONE',  ( 16.52544592524342804, -4.483927247898539470, 73.54057627198102409 ) ) ;
#60457=CARTESIAN_POINT ( 'NONE',  ( 5.153800228976615827, -19.02544592524334988, 50.20942372801897591 ) ) ;
#60458=CARTESIAN_POINT ( 'NONE',  ( -19.02544592524342804, 5.153800228976336051, 36.04057627198100988 ) ) ;
#60459=CARTESIAN_POINT ( 'NONE',  ( -18.62759615963270932, 10.81492255796079327, 40.83224293864769550 ) ) ;
#60460=CARTESIAN_POINT ( 'NONE',  ( -10.72451020669898014, 18.67979575497178502, 70.41557627198102409 ) ) ;
#60461=CARTESIAN_POINT ( 'NONE',  ( 0.05219959533910956823, 16.53943276465976808, 109.9989096053143527 ) ) ;
#60462=CARTESIAN_POINT ( 'NONE',  ( 4.483927247898790824, -16.52544592524335698, 55.20942372801902565 ) ) ;
#60463=CARTESIAN_POINT ( 'NONE',  ( 18.62759615963255655, 10.81492255796105972, 41.66775706135235424 ) ) ;
#60464=CARTESIAN_POINT ( 'NONE',  ( 0.05219959533910956823, 16.53943276465976808, 94.99890960531436690 ) ) ;
#60465=CARTESIAN_POINT ( 'NONE',  ( 16.52216118717207749, -7.221426719304488984, 36.42400978953008206 ) ) ;
#60467=CARTESIAN_POINT ( 'NONE',  ( -10.72451020669898014, 18.67979575497178502, 40.41557627198103120 ) ) ;
#60468=CARTESIAN_POINT ( 'NONE',  ( 17.31747979337950483, -6.344076630960995722, 66.12055131934813801 ) ) ;
#60469=CARTESIAN_POINT ( 'NONE',  ( -12.06949235617739369, -12.14591786802326823, 44.37609039468567573 ) ) ;
#60470=CARTESIAN_POINT ( 'NONE',  ( -16.52544592524342804, 4.483927247898546575, 41.04057627198103120 ) ) ;
#60471=CARTESIAN_POINT ( 'NONE',  ( -5.719274019375978568, 21.55341960407610458, 70.20724293864769550 ) ) ;
#60472=CARTESIAN_POINT ( 'NONE',  ( -19.03943276465977164, -0.05219959533935918106, 83.75109039468567573 ) ) ;
#60473=CARTESIAN_POINT ( 'NONE',  ( 18.62759615963271287, -10.81492255796078972, 68.33224293864769550 ) ) ;
#60475=CARTESIAN_POINT ( 'NONE',  ( -19.03943276465977164, 0.05219959533909376836, 41.24890960531435269 ) ) ;
#60476=CARTESIAN_POINT ( 'NONE',  ( -5.153800228976328057, -19.02544592524343514, 107.2905762719810383 ) ) ;
#60477=EDGE_CURVE ( 'NONE', #147765, #189743, #154946, .T. ) ;
#60478=CARTESIAN_POINT ( 'NONE',  ( 16.51473224551069308, 9.474510206698969483, 44.16557627198103120 ) ) ;
#60479=CARTESIAN_POINT ( 'NONE',  ( -14.29746914071049879, 8.314922557960819915, 115.8322429386477097 ) ) ;
#60481=CARTESIAN_POINT ( 'NONE',  ( 5.153800228976335163, 19.02544592524342804, 114.7905762719810241 ) ) ;
#60482=VERTEX_POINT ( 'NONE', #108440 ) ;
#60483=CARTESIAN_POINT ( 'NONE',  ( -4.483927247898782831, 16.52544592524335698, 67.70942372801901854 ) ) ;
#60484=CARTESIAN_POINT ( 'NONE',  ( 21.52544592524344225, -5.823673210054117533, 98.54057627198105251 ) ) ;
#60485=CARTESIAN_POINT ( 'NONE',  ( 5.153800228976335163, 19.02544592524342804, 59.79057627198100988 ) ) ;
#60486=CARTESIAN_POINT ( 'NONE',  ( 21.55341960407619695, -5.719274019375665929, 46.04275706135234714 ) ) ;
#60487=CARTESIAN_POINT ( 'NONE',  ( 13.97604488694527802, 13.89961937509977652, 84.37390960531433848 ) ) ;
#60490=CARTESIAN_POINT ( 'NONE',  ( -21.52544592524334988, -5.823673210054445271, 38.95942372801901854 ) ) ;
#60491=CARTESIAN_POINT ( 'NONE',  ( 5.153800228976335163, 19.02544592524342804, 104.7905762719809957 ) ) ;
#60492=CARTESIAN_POINT ( 'NONE',  ( 9.564922557961047289, -16.46253265017146816, 85.41775706135233293 ) ) ;
#60493=CARTESIAN_POINT ( 'NONE',  ( 19.05341960407617918, -5.049401038297876454, 41.04275706135233293 ) ) ;
#60494=CARTESIAN_POINT ( 'NONE',  ( -21.53943276465977519, 0.05219959533907696930, 101.2489096053143669 ) ) ;
#60495=CARTESIAN_POINT ( 'NONE',  ( 19.05341960407617918, -5.049401038297876454, 36.04275706135234003 ) ) ;
#60496=CARTESIAN_POINT ( 'NONE',  ( 19.03943276465977164, 0.05219959533936151252, 36.25109039468567573 ) ) ;
#60497=CARTESIAN_POINT ( 'NONE',  ( -14.29746914071037622, -8.314922557961029526, 89.16775706135236135 ) ) ;
#60498=CARTESIAN_POINT ( 'NONE',  ( -0.05219959533909027116, -19.03943276465977164, 107.4989096053143527 ) ) ;
#60499=CARTESIAN_POINT ( 'NONE',  ( -19.02544592524342804, 5.153800228976336051, 61.04057627198103120 ) ) ;
#60501=CARTESIAN_POINT ( 'NONE',  ( -10.81492255796105439, 18.62759615963255655, 62.91775706135236135 ) ) ;
#60502=CARTESIAN_POINT ( 'NONE',  ( 18.62759615963255655, 10.81492255796105972, 76.66775706135234714 ) ) ;
#60503=CARTESIAN_POINT ( 'NONE',  ( -13.89961937509977652, 13.97604488694528158, 115.6239096053143669 ) ) ;
#60504=CARTESIAN_POINT ( 'NONE',  ( -16.46253265017160317, 9.564922557960807481, 75.83224293864769550 ) ) ;
#60505=CARTESIAN_POINT ( 'NONE',  ( -21.55341960407619339, 5.719274019375674811, 53.54275706135234714 ) ) ;
#60506=CARTESIAN_POINT ( 'NONE',  ( -9.474510206698720793, -16.51473224551083518, 104.5844237280190043 ) ) ;
#60507=CARTESIAN_POINT ( 'NONE',  ( -5.153800228976328057, -19.02544592524343514, 57.29057627198103120 ) ) ;
#60508=CARTESIAN_POINT ( 'NONE',  ( -9.474510206698964154, 16.51473224551069663, 100.4155762719810241 ) ) ;
#60509=CARTESIAN_POINT ( 'NONE',  ( -13.89961937509977652, 13.97604488694528158, 80.62390960531436690 ) ) ;
#60510=CARTESIAN_POINT ( 'NONE',  ( -16.51473224551069308, -9.474510206698971260, 76.66557627198103830 ) ) ;
#60511=CARTESIAN_POINT ( 'NONE',  ( 0.05219959533909260263, 19.03943276465977164, 59.99890960531436690 ) ) ;
#60512=CARTESIAN_POINT ( 'NONE',  ( -10.72451020669898014, 18.67979575497178502, 95.41557627198102409 ) ) ;
#60513=CARTESIAN_POINT ( 'NONE',  ( -14.34966873604972548, 8.224510206698743886, 83.33442372801903275 ) ) ;
#60515=CARTESIAN_POINT ( 'NONE',  ( -19.03943276465977164, -0.05219959533935918106, 48.75109039468566863 ) ) ;
#60516=CARTESIAN_POINT ( 'NONE',  ( 16.51473224551069308, 9.474510206698969483, 74.16557627198103830 ) ) ;
#60517=CARTESIAN_POINT ( 'NONE',  ( 8.314922557960818139, 14.29746914071049879, 74.58224293864768129 ) ) ;
#60518=CARTESIAN_POINT ( 'NONE',  ( -12.14591786802309592, -12.06949235617757132, 96.87390960531436690 ) ) ;
#60519=CARTESIAN_POINT ( 'NONE',  ( -18.67979575497178146, -10.72451020669898902, 21.66557627198102409 ) ) ;
#60521=CARTESIAN_POINT ( 'NONE',  ( 5.049401038298161559, -19.05341960407611168, 102.7072429386476955 ) ) ;
#60522=CARTESIAN_POINT ( 'NONE',  ( 5.153800228976615827, -19.02544592524334988, 30.20942372801900433 ) ) ;
#60523=CARTESIAN_POINT ( 'NONE',  ( 14.34966873604972726, -8.224510206698740333, 95.83442372801903275 ) ) ;
#60524=CARTESIAN_POINT ( 'NONE',  ( -16.51473224551069308, -9.474510206698971260, 76.66557627198103830 ) ) ;
#60525=CARTESIAN_POINT ( 'NONE',  ( 21.53943276465977519, 0.05219959533937863772, 51.25109039468568994 ) ) ;
#60526=CARTESIAN_POINT ( 'NONE',  ( 18.62759615963271287, -10.81492255796078972, 28.33224293864769550 ) ) ;
#60527=CARTESIAN_POINT ( 'NONE',  ( 15.72974639402176855, 15.80617190586768217, 21.87609039468567573 ) ) ;
#60528=CARTESIAN_POINT ( 'NONE',  ( 5.719274019375991003, -21.55341960407610458, 67.70724293864769550 ) ) ;
#60529=CARTESIAN_POINT ( 'NONE',  ( 0.05219959533910956823, 16.53943276465976808, 99.99890960531436690 ) ) ;
#60530=CARTESIAN_POINT ( 'NONE',  ( 16.51473224551083163, -9.474510206698727899, 50.83442372801899722 ) ) ;
#60531=CARTESIAN_POINT ( 'NONE',  ( 16.51473224551069308, 9.474510206698969483, 34.16557627198102409 ) ) ;
#60532=CARTESIAN_POINT ( 'NONE',  ( 0.05219959533909260263, 19.03943276465977164, 89.99890960531436690 ) ) ;
#60533=CARTESIAN_POINT ( 'NONE',  ( -13.89961937509977652, 13.97604488694528158, 85.62390960531433848 ) ) ;
#60535=CARTESIAN_POINT ( 'NONE',  ( 14.34966873604960469, 8.224510206698951720, 99.16557627198100988 ) ) ;
#60537=CARTESIAN_POINT ( 'NONE',  ( 4.379528057220339221, -16.55341960407611168, 27.70724293864769905 ) ) ;
#60538=CARTESIAN_POINT ( 'NONE',  ( -12.06949235617739369, -12.14591786802326823, 24.37609039468567573 ) ) ;
#60539=CARTESIAN_POINT ( 'NONE',  ( -21.55341960407619339, 5.719274019375674811, 98.54275706135234714 ) ) ;
#60540=CARTESIAN_POINT ( 'NONE',  ( 5.049401038298161559, -19.05341960407611168, 102.7072429386476955 ) ) ;
#60541=CARTESIAN_POINT ( 'NONE',  ( -5.823673210054116645, -21.52544592524344225, 112.2905762719810241 ) ) ;
#60542=CARTESIAN_POINT ( 'NONE',  ( -19.02544592524342804, 5.153800228976336051, 46.04057627198101699 ) ) ;
#60544=CARTESIAN_POINT ( 'NONE',  ( 16.53943276465976808, 0.05219959533934440121, 46.25109039468567573 ) ) ;
#60545=CARTESIAN_POINT ( 'NONE',  ( 19.05341960407617918, -5.049401038297876454, 111.0427570613523329 ) ) ;
#60546=CARTESIAN_POINT ( 'NONE',  ( -8.224510206698948167, 14.34966873604960824, 95.41557627198102409 ) ) ;
#60547=CARTESIAN_POINT ( 'NONE',  ( -21.52544592524343514, 5.823673210054127303, 106.0405762719810525 ) ) ;
#60548=CARTESIAN_POINT ( 'NONE',  ( -0.05219959533936034679, 19.03943276465977164, 62.50109039468566863 ) ) ;
#60550=CARTESIAN_POINT ( 'NONE',  ( 18.62759615963271287, -10.81492255796078972, 113.3322429386476955 ) ) ;
#60552=CARTESIAN_POINT ( 'NONE',  ( -5.049401038298153566, 19.05341960407611168, 85.20724293864766707 ) ) ;
#60553=CARTESIAN_POINT ( 'NONE',  ( 16.61371651742598132, -7.165104196376176127, 111.3541506999299742 ) ) ;
#60554=CARTESIAN_POINT ( 'NONE',  ( 5.049401038298161559, -19.05341960407611168, 87.70724293864769550 ) ) ;
#60555=CARTESIAN_POINT ( 'NONE',  ( 10.72451020669871369, 18.67979575497193778, 32.08442372801901854 ) ) ;
#60556=CARTESIAN_POINT ( 'NONE',  ( -4.483927247898539470, -16.52544592524342804, 72.29057627198102409 ) ) ;
#60557=CARTESIAN_POINT ( 'NONE',  ( -5.153800228976328057, -19.02544592524343514, 82.29057627198103830 ) ) ;
#60558=CARTESIAN_POINT ( 'NONE',  ( 16.55341960407618274, -4.379528057220086978, 56.04275706135235424 ) ) ;
#60559=CARTESIAN_POINT ( 'NONE',  ( -19.05341960407617563, 5.049401038297882671, 58.54275706135234003 ) ) ;
#60560=CARTESIAN_POINT ( 'NONE',  ( -10.72451020669870658, -18.67979575497194134, 59.58442372801901854 ) ) ;
#60561=CARTESIAN_POINT ( 'NONE',  ( 8.224510206698742110, 14.34966873604972548, 32.08442372801901854 ) ) ;
#60562=CARTESIAN_POINT ( 'NONE',  ( -5.049401038298153566, 19.05341960407611168, 65.20724293864765286 ) ) ;
#60563=CARTESIAN_POINT ( 'NONE',  ( -9.474510206698720793, -16.51473224551083518, 94.58442372801900433 ) ) ;
#60564=CARTESIAN_POINT ( 'NONE',  ( -0.05219959533934338120, 16.53943276465976808, 62.50109039468568284 ) ) ;
#60565=CARTESIAN_POINT ( 'NONE',  ( 21.55341960407619695, -5.719274019375665929, 101.0427570613523756 ) ) ;
#60566=CARTESIAN_POINT ( 'NONE',  ( 5.153800228976615827, -19.02544592524334988, 80.20942372801901854 ) ) ;
#60567=CARTESIAN_POINT ( 'NONE',  ( -9.474510206698964154, 16.51473224551069663, 55.41557627198103120 ) ) ;
#60568=CARTESIAN_POINT ( 'NONE',  ( -15.80617190586745835, -15.72974639402198527, 71.87390960531438111 ) ) ;
#60569=CARTESIAN_POINT ( 'NONE',  ( -16.53943276465976808, 0.05219959533911058130, 81.24890960531436690 ) ) ;
#60570=CARTESIAN_POINT ( 'NONE',  ( -9.474510206698720793, -16.51473224551083518, 79.58442372801899012 ) ) ;
#60571=CARTESIAN_POINT ( 'NONE',  ( 17.26058549869092218, -6.457015423128527942, 61.12254162523935719 ) ) ;
#60572=CARTESIAN_POINT ( 'NONE',  ( 5.049401038297881783, 19.05341960407617563, 42.29275706135234003 ) ) ;
#60573=CARTESIAN_POINT ( 'NONE',  ( 16.52544592524342804, -4.483927247898539470, 23.54057627198102765 ) ) ;
#60574=CARTESIAN_POINT ( 'NONE',  ( 16.55341960407611168, 4.379528057220329451, 68.95724293864769550 ) ) ;
#60575=CARTESIAN_POINT ( 'NONE',  ( 21.53943276465977519, 0.05219959533937863772, 96.25109039468568994 ) ) ;
#60577=CARTESIAN_POINT ( 'NONE',  ( 0.05219959533907565091, 21.53943276465977519, 109.9989096053143527 ) ) ;
#60578=CARTESIAN_POINT ( 'NONE',  ( 5.153800228976335163, 19.02544592524342804, 64.79057627198100988 ) ) ;
#60579=CARTESIAN_POINT ( 'NONE',  ( -21.52544592524334988, -5.823673210054445271, 83.95942372801900433 ) ) ;
#60580=CARTESIAN_POINT ( 'NONE',  ( -16.46253265017160317, 9.564922557960807481, 65.83224293864769550 ) ) ;
#60582=CARTESIAN_POINT ( 'NONE',  ( 0.05219959533909260263, 19.03943276465977164, 24.99890960531435269 ) ) ;
#60583=CARTESIAN_POINT ( 'NONE',  ( 21.52544592524344225, -5.823673210054117533, 28.54057627198103120 ) ) ;
#60584=CARTESIAN_POINT ( 'NONE',  ( -12.06949235617756955, 12.14591786802309770, 70.62390960531436690 ) ) ;
#60585=CARTESIAN_POINT ( 'NONE',  ( -0.05219959533909027116, -19.03943276465977164, 42.49890960531435269 ) ) ;
#60586=CARTESIAN_POINT ( 'NONE',  ( 14.29746914071049879, -8.314922557960816363, 88.33224293864769550 ) ) ;
#60588=CARTESIAN_POINT ( 'NONE',  ( 10.81492255796078972, 18.62759615963270932, 114.5822429386477097 ) ) ;
#60589=CARTESIAN_POINT ( 'NONE',  ( 5.823673210054444382, -21.52544592524334988, 55.20942372801902565 ) ) ;
#60590=CARTESIAN_POINT ( 'NONE',  ( -9.474510206698964154, 16.51473224551069663, 25.41557627198103120 ) ) ;
#60591=CARTESIAN_POINT ( 'NONE',  ( 16.55341960407618274, -4.379528057220086978, 56.04275706135235424 ) ) ;
#60592=CARTESIAN_POINT ( 'NONE',  ( -5.823673210054116645, -21.52544592524344225, 97.29057627198105251 ) ) ;
#60593=CARTESIAN_POINT ( 'NONE',  ( 5.719274019375991003, -21.55341960407610458, 92.70724293864770971 ) ) ;
#60594=CARTESIAN_POINT ( 'NONE',  ( 16.51473224551083163, -9.474510206698727899, 25.83442372801900078 ) ) ;
#60595=CARTESIAN_POINT ( 'NONE',  ( -9.474510206698964154, 16.51473224551069663, 55.41557627198103120 ) ) ;
#60596=CARTESIAN_POINT ( 'NONE',  ( 13.97604488694527802, 13.89961937509977652, 104.3739096053143385 ) ) ;
#60597=CARTESIAN_POINT ( 'NONE',  ( 10.72451020669871369, 18.67979575497193778, 62.08442372801901143 ) ) ;
#60598=CARTESIAN_POINT ( 'NONE',  ( 10.81492255796078972, 18.62759615963270932, 44.58224293864769550 ) ) ;
#60599=CARTESIAN_POINT ( 'NONE',  ( 8.314922557961029526, -14.29746914071037800, 110.4177570613523756 ) ) ;
#60600=CARTESIAN_POINT ( 'NONE',  ( -21.55341960407619339, 5.719274019375674811, 58.54275706135235424 ) ) ;
#60601=CARTESIAN_POINT ( 'NONE',  ( 15.72974639402176855, 15.80617190586768217, 101.8760903946857042 ) ) ;
#60602=CARTESIAN_POINT ( 'NONE',  ( 19.05341960407617918, -5.049401038297876454, 46.04275706135233293 ) ) ;
#60603=CARTESIAN_POINT ( 'NONE',  ( -12.14591786802326823, 12.06949235617739902, 103.1260903946856757 ) ) ;
#60604=CARTESIAN_POINT ( 'NONE',  ( 18.62759615963255655, 10.81492255796105972, 56.66775706135235424 ) ) ;
#60605=CARTESIAN_POINT ( 'NONE',  ( 16.51473224551069308, 9.474510206698969483, 44.16557627198103120 ) ) ;
#60606=CARTESIAN_POINT ( 'NONE',  ( 5.049401038297881783, 19.05341960407617563, 22.29275706135233648 ) ) ;
#60607=CARTESIAN_POINT ( 'NONE',  ( -5.049401038298153566, 19.05341960407611168, 115.2072429386477097 ) ) ;
#60608=CARTESIAN_POINT ( 'NONE',  ( -18.62759615963270932, 10.81492255796079327, 110.8322429386476955 ) ) ;
#60609=CARTESIAN_POINT ( 'NONE',  ( -18.67979575497178146, -10.72451020669898902, 71.66557627198100988 ) ) ;
#60610=CARTESIAN_POINT ( 'NONE',  ( 4.483927247898790824, -16.52544592524335698, 40.20942372801901854 ) ) ;
#60611=CARTESIAN_POINT ( 'NONE',  ( 17.49999999999997868, -3.232540337672884956, 37.21909520004585659 ) ) ;
#60612=CARTESIAN_POINT ( 'NONE',  ( 21.53943276465977519, -0.05219959533907433946, 78.74890960531436690 ) ) ;
#60613=CARTESIAN_POINT ( 'NONE',  ( 16.55341960407618274, -4.379528057220086978, 66.04275706135236135 ) ) ;
#60614=CARTESIAN_POINT ( 'NONE',  ( 8.224510206698953496, -14.34966873604960469, 77.91557627198102409 ) ) ;
#60616=CARTESIAN_POINT ( 'NONE',  ( 13.89961937509957401, 13.97604488694547697, 106.8760903946856757 ) ) ;
#60617=CARTESIAN_POINT ( 'NONE',  ( -5.719274019375978568, 21.55341960407610458, 40.20724293864769550 ) ) ;
#60620=CARTESIAN_POINT ( 'NONE',  ( -16.53943276465976808, -0.05219959533934237506, 33.75109039468568284 ) ) ;
#60621=CARTESIAN_POINT ( 'NONE',  ( 10.72451020669898902, -18.67979575497178502, 112.9155762719810383 ) ) ;
#60622=CARTESIAN_POINT ( 'NONE',  ( -21.55341960407610458, -5.719274019375992779, 36.45724293864768839 ) ) ;
#60623=CARTESIAN_POINT ( 'NONE',  ( -0.05219959533934338120, 16.53943276465976808, 72.50109039468568994 ) ) ;
#60624=CARTESIAN_POINT ( 'NONE',  ( -5.049401038298153566, 19.05341960407611168, 80.20724293864769550 ) ) ;
#60625=CARTESIAN_POINT ( 'NONE',  ( 21.52544592524334988, 5.823673210054432836, 46.45942372801901854 ) ) ;
#60626=CARTESIAN_POINT ( 'NONE',  ( 9.564922557960805705, 16.46253265017160317, 34.58224293864770260 ) ) ;
#60627=CARTESIAN_POINT ( 'NONE',  ( 21.52544592524344225, -5.823673210054117533, 23.54057627198102765 ) ) ;
#60629=CARTESIAN_POINT ( 'NONE',  ( -13.89961937509957401, -13.97604488694547875, 24.37609039468565442 ) ) ;
#60630=CARTESIAN_POINT ( 'NONE',  ( 14.34966873604972726, -8.224510206698740333, 50.83442372801901143 ) ) ;
#60631=CARTESIAN_POINT ( 'NONE',  ( 13.89961937509977652, -13.97604488694527269, 98.12390960531433848 ) ) ;
#60632=CARTESIAN_POINT ( 'NONE',  ( -21.53943276465977519, 0.05219959533907696930, 106.2489096053143811 ) ) ;
#60633=CARTESIAN_POINT ( 'NONE',  ( -19.03943276465977164, 0.05219959533909376836, 66.24890960531436690 ) ) ;
#60634=CARTESIAN_POINT ( 'NONE',  ( -16.79531203550650886, 7.028104445595467098, 23.74755011779560121 ) ) ;
#60636=CARTESIAN_POINT ( 'NONE',  ( 16.52544592524342804, -4.483927247898539470, 78.54057627198103830 ) ) ;
#60637=CARTESIAN_POINT ( 'NONE',  ( -15.80617190586745835, -15.72974639402198527, 36.87390960531435979 ) ) ;
#60639=CARTESIAN_POINT ( 'NONE',  ( -4.483927247898782831, 16.52544592524335698, 67.70942372801901854 ) ) ;
#60640=CARTESIAN_POINT ( 'NONE',  ( -21.52544592524334988, -5.823673210054445271, 18.95942372801901143 ) ) ;
#60641=CARTESIAN_POINT ( 'NONE',  ( 16.46253265017146816, 9.564922557961045513, 81.66775706135233293 ) ) ;
#60642=CARTESIAN_POINT ( 'NONE',  ( 0.05219959533909260263, 19.03943276465977164, 44.99890960531435979 ) ) ;
#60643=CARTESIAN_POINT ( 'NONE',  ( 18.62759615963271287, -10.81492255796078972, 63.33224293864770260 ) ) ;
#60644=CARTESIAN_POINT ( 'NONE',  ( 13.97604488694527802, 13.89961937509977652, 104.3739096053143385 ) ) ;
#60645=CARTESIAN_POINT ( 'NONE',  ( -15.72974639402176322, -15.80617190586768395, 94.37609039468568994 ) ) ;
#60646=CARTESIAN_POINT ( 'NONE',  ( 19.02544592524343514, -5.153800228976328945, 68.54057627198103830 ) ) ;
#60647=CARTESIAN_POINT ( 'NONE',  ( -4.379528057220086978, -16.55341960407618274, 54.79275706135235424 ) ) ;
#60648=B_SPLINE_CURVE_WITH_KNOTS ( 'NONE', 3,
 ( #3096, #61771, #123439, #125453, #172958, #62768, #77939, #188133, #171955, #46623, #49604, #185132, #170957, #48622, #32451, #139606, #169961, #33443, #94104, #168953 ),
 .UNSPECIFIED., .F., .F.,
 ( 4, 2, 2, 2, 2, 2, 2, 2, 2, 4 ),
 ( 3.469446951953614189E-18, 0.0004987090165372718353, 0.0009974180330745402012, 0.001246772541343170535, 0.001496127049611800869, 0.001994836066149057417, 0.002493545082686314182, 0.002742899590954942998, 0.002992254099223570947, 0.003989672132298160805 ),
 .UNSPECIFIED. ) ;
#60649=CARTESIAN_POINT ( 'NONE',  ( -5.153800228976328057, -19.02544592524343514, 57.29057627198103120 ) ) ;
#60650=CARTESIAN_POINT ( 'NONE',  ( 10.81492255796106328, -18.62759615963255655, 85.41775706135236135 ) ) ;
#60652=CARTESIAN_POINT ( 'NONE',  ( -9.564922557961040184, 16.46253265017147172, 37.91775706135233293 ) ) ;
#60653=CARTESIAN_POINT ( 'NONE',  ( 13.89961937509957401, 13.97604488694547697, 46.87609039468565442 ) ) ;
#60654=CARTESIAN_POINT ( 'NONE',  ( 15.72974639402176855, 15.80617190586768217, 51.87609039468568284 ) ) ;
#60656=CARTESIAN_POINT ( 'NONE',  ( 9.474510206698729675, 16.51473224551082808, 42.08442372801900433 ) ) ;
#60657=CARTESIAN_POINT ( 'NONE',  ( -13.97604488694527625, -13.89961937509977652, 96.87390960531433848 ) ) ;
#60658=CARTESIAN_POINT ( 'NONE',  ( 9.474510206698971260, -16.51473224551069308, 67.91557627198102409 ) ) ;
#60659=CARTESIAN_POINT ( 'NONE',  ( 4.483927247898545687, 16.52544592524342804, 24.79057627198103120 ) ) ;
#60660=CARTESIAN_POINT ( 'NONE',  ( -5.719274019375978568, 21.55341960407610458, 40.20724293864769550 ) ) ;
#60661=CARTESIAN_POINT ( 'NONE',  ( -18.67979575497193778, 10.72451020669871902, 98.33442372801901854 ) ) ;
#60662=B_SPLINE_CURVE_WITH_KNOTS ( 'NONE', 3,
 ( #121574, #91215, #197451, #26614, #42775, #15403, #167107, #75082, #27623, #169065, #198433, #88257, #44749, #58917, #149944, #153908, #43760, #77060, #46737, #59906, #184258, #61881, #152906, #183269, #120585, #199427, #28608, #119614, #73122, #123551, #138732, #182279 ),
 .UNSPECIFIED., .F., .F.,
 ( 4, 2, 2, 2, 2, 2, 2, 2, 2, 2, 2, 2, 2, 2, 2, 4 ),
 ( 5.204170427930421283E-18, 0.0003712461730036837964, 0.0007424923460073623886, 0.001113738519011040927, 0.001484984692014719573, 0.002227477038022076649, 0.002598723211025754862, 0.002969969384029433074, 0.003341215557033111287, 0.003712461730036788633, 0.004083707903040466845, 0.004454954076044144624, 0.004826200249047822403, 0.005197446422051501050, 0.005568692595055177962, 0.005939938768058855741 ),
 .UNSPECIFIED. ) ;
#60664=CARTESIAN_POINT ( 'NONE',  ( 16.52216118717208104, 7.221426719304524511, 58.57599021046992505 ) ) ;
#60665=CARTESIAN_POINT ( 'NONE',  ( -15.72974639402176322, -15.80617190586768395, 99.37609039468568994 ) ) ;
#60667=CARTESIAN_POINT ( 'NONE',  ( 19.02544592524343514, -5.153800228976328945, 28.54057627198102409 ) ) ;
#60668=CARTESIAN_POINT ( 'NONE',  ( 13.89961937509977652, -13.97604488694527269, 108.1239096053143669 ) ) ;
#60670=CARTESIAN_POINT ( 'NONE',  ( -12.14591786802326823, 12.06949235617739902, 48.12609039468568284 ) ) ;
#60671=CARTESIAN_POINT ( 'NONE',  ( 18.62759615963271287, -10.81492255796078972, 68.33224293864769550 ) ) ;
#60672=CARTESIAN_POINT ( 'NONE',  ( -14.29746914071049879, 8.314922557960819915, 40.83224293864769550 ) ) ;
#60673=CARTESIAN_POINT ( 'NONE',  ( 8.224510206698953496, -14.34966873604960469, 107.9155762719810241 ) ) ;
#60674=CARTESIAN_POINT ( 'NONE',  ( 13.97604488694527802, 13.89961937509977652, 104.3739096053143385 ) ) ;
#60675=CARTESIAN_POINT ( 'NONE',  ( 13.97604488694548053, -13.89961937509957401, 35.62609039468567573 ) ) ;
#60676=CARTESIAN_POINT ( 'NONE',  ( 16.51473224551069308, 9.474510206698969483, 24.16557627198102765 ) ) ;
#60677=CARTESIAN_POINT ( 'NONE',  ( -0.05219959533937732626, 21.53943276465977519, 67.50109039468568994 ) ) ;
#60678=CARTESIAN_POINT ( 'NONE',  ( 5.049401038298161559, -19.05341960407611168, 112.7072429386476813 ) ) ;
#60679=CARTESIAN_POINT ( 'NONE',  ( -4.483927247898539470, -16.52544592524342804, 32.29057627198102409 ) ) ;
#60680=CARTESIAN_POINT ( 'NONE',  ( -16.51473224551082808, 9.474510206698731452, 68.33442372801900433 ) ) ;
#60681=CARTESIAN_POINT ( 'NONE',  ( -10.72451020669898014, 18.67979575497178502, 25.41557627198103120 ) ) ;
#60682=CARTESIAN_POINT ( 'NONE',  ( -14.34966873604960291, -8.224510206698953496, 91.66557627198103830 ) ) ;
#60683=CARTESIAN_POINT ( 'NONE',  ( -19.02544592524334988, -5.153800228976617603, 63.95942372801899012 ) ) ;
#60684=CARTESIAN_POINT ( 'NONE',  ( -5.153800228976328057, -19.02544592524343514, 77.29057627198099567 ) ) ;
#60685=CARTESIAN_POINT ( 'NONE',  ( -12.14591786802309592, -12.06949235617757132, 81.87390960531435269 ) ) ;
#60686=CARTESIAN_POINT ( 'NONE',  ( 16.51473224551083163, -9.474510206698727899, 90.83442372801900433 ) ) ;
#60687=CARTESIAN_POINT ( 'NONE',  ( 10.81492255796078972, 18.62759615963270932, 44.58224293864769550 ) ) ;
#60689=CARTESIAN_POINT ( 'NONE',  ( 19.03943276465977164, -0.05219959533909143690, 23.74890960531435269 ) ) ;
#60690=CARTESIAN_POINT ( 'NONE',  ( -0.05219959533909027116, -19.03943276465977164, 77.49890960531435269 ) ) ;
#60691=CARTESIAN_POINT ( 'NONE',  ( 21.55341960407610458, 5.719274019375980345, 78.95724293864769550 ) ) ;
#60692=CARTESIAN_POINT ( 'NONE',  ( -4.379528057220086978, -16.55341960407618274, 104.7927570613523898 ) ) ;
#60693=CARTESIAN_POINT ( 'NONE',  ( -5.153800228976328057, -19.02544592524343514, 92.29057627198099567 ) ) ;
#60694=CARTESIAN_POINT ( 'NONE',  ( -19.02544592524334988, -5.153800228976617603, 63.95942372801899012 ) ) ;
#60695=CARTESIAN_POINT ( 'NONE',  ( -10.72451020669870658, -18.67979575497194134, 84.58442372801903275 ) ) ;
#60696=CARTESIAN_POINT ( 'NONE',  ( 0.05219959533907565091, 21.53943276465977519, 59.99890960531436690 ) ) ;
#60697=CARTESIAN_POINT ( 'NONE',  ( -18.62759615963270932, 10.81492255796079327, 25.83224293864769194 ) ) ;
#60698=CARTESIAN_POINT ( 'NONE',  ( 9.474510206698971260, -16.51473224551069308, 42.91557627198103120 ) ) ;
#60699=CARTESIAN_POINT ( 'NONE',  ( 8.314922557961029526, -14.29746914071037800, 95.41775706135234714 ) ) ;
#60700=CARTESIAN_POINT ( 'NONE',  ( -0.05219959533909027116, -19.03943276465977164, 57.49890960531435979 ) ) ;
#60701=CARTESIAN_POINT ( 'NONE',  ( -0.05219959533936034679, 19.03943276465977164, 112.5010903946856757 ) ) ;
#60702=CARTESIAN_POINT ( 'NONE',  ( -18.22780087662122028, 5.500000000000031086, 83.51540105326107266 ) ) ;
#60703=CARTESIAN_POINT ( 'NONE',  ( -0.05219959533937732626, 21.53943276465977519, 112.5010903946857042 ) ) ;
#60704=CARTESIAN_POINT ( 'NONE',  ( -12.14591786802309592, -12.06949235617757132, 71.87390960531438111 ) ) ;
#60705=CARTESIAN_POINT ( 'NONE',  ( 21.55341960407610458, 5.719274019375980345, 113.9572429386477239 ) ) ;
#60706=CARTESIAN_POINT ( 'NONE',  ( -18.67979575497178146, -10.72451020669898902, 106.6655762719810383 ) ) ;
#60709=CARTESIAN_POINT ( 'NONE',  ( 21.53943276465977519, -0.05219959533907433946, 48.74890960531435979 ) ) ;
#60711=CARTESIAN_POINT ( 'NONE',  ( 14.34966873604972726, -8.224510206698740333, 85.83442372801901854 ) ) ;
#60712=CARTESIAN_POINT ( 'NONE',  ( 14.29746914071049879, -8.314922557960816363, 98.33224293864769550 ) ) ;
#60713=CARTESIAN_POINT ( 'NONE',  ( -19.05341960407611168, -5.049401038298163336, 56.45724293864768129 ) ) ;
#60714=SURFACE_STYLE_FILL_AREA ( #17211 ) ;
#60716=CARTESIAN_POINT ( 'NONE',  ( -4.483927247898782831, 16.52544592524335698, 112.7094237280190328 ) ) ;
#60717=CARTESIAN_POINT ( 'NONE',  ( -0.05219959533937732626, 21.53943276465977519, 52.50109039468567573 ) ) ;
#60718=CARTESIAN_POINT ( 'NONE',  ( 9.474510206698971260, -16.51473224551069308, 92.91557627198103830 ) ) ;
#60719=CARTESIAN_POINT ( 'NONE',  ( 21.52544592524334988, 5.823673210054432836, 76.45942372801901854 ) ) ;
#60721=CARTESIAN_POINT ( 'NONE',  ( -13.89961937509977652, 13.97604488694528158, 30.62390960531435269 ) ) ;
#60723=CARTESIAN_POINT ( 'NONE',  ( -21.55341960407619339, 5.719274019375674811, 68.54275706135234714 ) ) ;
#60724=CARTESIAN_POINT ( 'NONE',  ( -9.564922557960796823, -16.46253265017161027, 52.08224293864768839 ) ) ;
#60725=CARTESIAN_POINT ( 'NONE',  ( 0.05219959533909260263, 19.03943276465977164, 109.9989096053143669 ) ) ;
#60726=CARTESIAN_POINT ( 'NONE',  ( -19.05341960407617563, 5.049401038297882671, 78.54275706135233293 ) ) ;
#60727=CARTESIAN_POINT ( 'NONE',  ( -5.719274019375665041, -21.55341960407619695, 39.79275706135235424 ) ) ;
#60728=CARTESIAN_POINT ( 'NONE',  ( 5.049401038297881783, 19.05341960407617563, 102.2927570613523045 ) ) ;
#60729=CARTESIAN_POINT ( 'NONE',  ( -19.03943276465977164, -0.05219959533935918106, 78.75109039468567573 ) ) ;
#60730=CARTESIAN_POINT ( 'NONE',  ( 13.97604488694527802, 13.89961937509977652, 34.37390960531436690 ) ) ;
#60731=CARTESIAN_POINT ( 'NONE',  ( 0.05219959533936267826, -19.03943276465977164, 80.00109039468567573 ) ) ;
#60733=CARTESIAN_POINT ( 'NONE',  ( 14.34966873604972726, -8.224510206698740333, 100.8344237280190185 ) ) ;
#60734=CARTESIAN_POINT ( 'NONE',  ( -13.97604488694547697, 13.89961937509957934, 78.12609039468567573 ) ) ;
#60735=CARTESIAN_POINT ( 'NONE',  ( -16.52544592524342804, 4.483927247898546575, 41.04057627198103120 ) ) ;
#60736=CARTESIAN_POINT ( 'NONE',  ( 19.03943276465977164, 0.05219959533936151252, 61.25109039468566863 ) ) ;
#60737=CARTESIAN_POINT ( 'NONE',  ( -5.823673210054431948, 21.52544592524334988, 107.7094237280190328 ) ) ;
#60738=CARTESIAN_POINT ( 'NONE',  ( 13.89961937509957401, 13.97604488694547697, 26.87609039468566507 ) ) ;
#60739=CARTESIAN_POINT ( 'NONE',  ( 16.51473224551069308, 9.474510206698969483, 29.16557627198103475 ) ) ;
#60741=CARTESIAN_POINT ( 'NONE',  ( -0.05219959533934338120, 16.53943276465976808, 52.50109039468567573 ) ) ;
#60744=CARTESIAN_POINT ( 'NONE',  ( 9.474510206698971260, -16.51473224551069308, 97.91557627198102409 ) ) ;
#60745=CARTESIAN_POINT ( 'NONE',  ( -17.48847506799948448, 5.747544572775424854, 100.8269743784329222 ) ) ;
#60746=VERTEX_POINT ( 'NONE', #199471 ) ;
#60747=CARTESIAN_POINT ( 'NONE',  ( 5.049401038297881783, 19.05341960407617563, 82.29275706135229029 ) ) ;
#60748=CARTESIAN_POINT ( 'NONE',  ( 5.823673210054125526, 21.52544592524343514, 29.79057627198102409 ) ) ;
#60749=CARTESIAN_POINT ( 'NONE',  ( -5.049401038297874678, -19.05341960407617918, 19.79275706135233293 ) ) ;
#60750=CARTESIAN_POINT ( 'NONE',  ( 0.05219959533936267826, -19.03943276465977164, 100.0010903946856757 ) ) ;
#60751=CARTESIAN_POINT ( 'NONE',  ( -8.314922557960811034, -14.29746914071050412, 112.0822429386477097 ) ) ;
#60752=CARTESIAN_POINT ( 'NONE',  ( 5.049401038298161559, -19.05341960407611168, 27.70724293864769550 ) ) ;
#60753=CARTESIAN_POINT ( 'NONE',  ( 10.72451020669898902, -18.67979575497178502, 57.91557627198103120 ) ) ;
#60754=CARTESIAN_POINT ( 'NONE',  ( -15.72974639402197994, 15.80617190586746368, 45.62390960531436690 ) ) ;
#60755=CARTESIAN_POINT ( 'NONE',  ( -5.153800228976328057, -19.02544592524343514, 27.29057627198103120 ) ) ;
#60757=CARTESIAN_POINT ( 'NONE',  ( 13.97604488694548053, -13.89961937509957401, 65.62609039468567573 ) ) ;
#60758=CARTESIAN_POINT ( 'NONE',  ( 16.55341960407611168, 4.379528057220329451, 33.95724293864769550 ) ) ;
#60760=CARTESIAN_POINT ( 'NONE',  ( 19.03943276465977164, -0.05219959533909143690, 113.7489096053143669 ) ) ;
#60761=CARTESIAN_POINT ( 'NONE',  ( -21.52544592524334988, -5.823673210054445271, 98.95942372801903275 ) ) ;
#60762=CARTESIAN_POINT ( 'NONE',  ( -21.52544592524343514, 5.823673210054127303, 66.04057627198103830 ) ) ;
#60763=CARTESIAN_POINT ( 'NONE',  ( 21.52544592524334988, 5.823673210054432836, 61.45942372801901854 ) ) ;
#60764=CARTESIAN_POINT ( 'NONE',  ( -18.67979575497193778, 10.72451020669871902, 53.33442372801901854 ) ) ;
#60765=CARTESIAN_POINT ( 'NONE',  ( 0.05219959533909260263, 19.03943276465977164, 94.99890960531436690 ) ) ;
#60766=CARTESIAN_POINT ( 'NONE',  ( 12.06949235617739724, 12.14591786802326823, 91.87609039468568994 ) ) ;
#60767=CARTESIAN_POINT ( 'NONE',  ( -10.81492255796105439, 18.62759615963255655, 47.91775706135234714 ) ) ;
#60768=CARTESIAN_POINT ( 'NONE',  ( -9.564922557960796823, -16.46253265017161027, 27.08224293864769550 ) ) ;
#60770=CARTESIAN_POINT ( 'NONE',  ( -4.379528057220328563, 16.55341960407611168, 70.20724293864769550 ) ) ;
#60771=CARTESIAN_POINT ( 'NONE',  ( -0.05219959533910754901, -16.53943276465976808, 32.49890960531435979 ) ) ;
#60772=CARTESIAN_POINT ( 'NONE',  ( 19.03943276465977164, -0.05219959533909143690, 63.74890960531435979 ) ) ;
#60773=CARTESIAN_POINT ( 'NONE',  ( -5.049401038298153566, 19.05341960407611168, 50.20724293864770260 ) ) ;
#60774=CARTESIAN_POINT ( 'NONE',  ( -21.52544592524343514, 5.823673210054127303, 61.04057627198103120 ) ) ;
#60775=CARTESIAN_POINT ( 'NONE',  ( -16.51473224551082808, 9.474510206698731452, 38.33442372801899722 ) ) ;
#60777=CARTESIAN_POINT ( 'NONE',  ( -8.224510206698948167, 14.34966873604960824, 45.41557627198103830 ) ) ;
#60778=CARTESIAN_POINT ( 'NONE',  ( -21.52544592524343514, 5.823673210054127303, 31.04057627198102409 ) ) ;
#60781=CARTESIAN_POINT ( 'NONE',  ( -4.483927247898782831, 16.52544592524335698, 67.70942372801901854 ) ) ;
#60783=CARTESIAN_POINT ( 'NONE',  ( 19.03943276465977164, 0.05219959533936151252, 81.25109039468567573 ) ) ;
#60784=CARTESIAN_POINT ( 'NONE',  ( 4.379528057220339221, -16.55341960407611168, 42.70724293864770260 ) ) ;
#60785=CARTESIAN_POINT ( 'NONE',  ( 17.31728774477277355, -6.344390552232304969, 53.31906651689320142 ) ) ;
#60786=CARTESIAN_POINT ( 'NONE',  ( -4.379528057220328563, 16.55341960407611168, 30.20724293864769550 ) ) ;
#60787=CARTESIAN_POINT ( 'NONE',  ( 5.049401038298161559, -19.05341960407611168, 52.70724293864767418 ) ) ;
#60788=CARTESIAN_POINT ( 'NONE',  ( -13.89961937509977652, 13.97604488694528158, 80.62390960531436690 ) ) ;
#60789=CARTESIAN_POINT ( 'NONE',  ( 9.564922557960805705, 16.46253265017160317, 44.58224293864769550 ) ) ;
#60790=CARTESIAN_POINT ( 'NONE',  ( 21.53943276465977519, 0.05219959533937863772, 46.25109039468567573 ) ) ;
#60791=CARTESIAN_POINT ( 'NONE',  ( 13.97604488694527802, 13.89961937509977652, 54.37390960531435979 ) ) ;
#60793=CARTESIAN_POINT ( 'NONE',  ( 9.474510206698971260, -16.51473224551069308, 52.91557627198102409 ) ) ;
#60794=CARTESIAN_POINT ( 'NONE',  ( -21.55341960407610458, -5.719274019375992779, 36.45724293864768839 ) ) ;
#60795=CARTESIAN_POINT ( 'NONE',  ( -19.02544592524342804, 5.153800228976336051, 26.04057627198103120 ) ) ;
#60796=CARTESIAN_POINT ( 'NONE',  ( -18.67979575497178146, -10.72451020669898902, 26.66557627198103475 ) ) ;
#60797=CARTESIAN_POINT ( 'NONE',  ( -4.379528057220086978, -16.55341960407618274, 84.79275706135234714 ) ) ;
#60798=CARTESIAN_POINT ( 'NONE',  ( 18.62759615963255655, 10.81492255796105972, 106.6677570613523756 ) ) ;
#60799=CARTESIAN_POINT ( 'NONE',  ( -12.14591786802326823, 12.06949235617739902, 73.12609039468567573 ) ) ;
#60800=CARTESIAN_POINT ( 'NONE',  ( -19.03943276465977164, 0.05219959533909376836, 106.2489096053143669 ) ) ;
#60801=CARTESIAN_POINT ( 'NONE',  ( -12.14591786802326823, 12.06949235617739902, 58.12609039468568994 ) ) ;
#60802=CARTESIAN_POINT ( 'NONE',  ( -16.55341960407617563, 4.379528057220093196, 38.54275706135234714 ) ) ;
#60803=CARTESIAN_POINT ( 'NONE',  ( -12.06949235617739369, -12.14591786802326823, 94.37609039468568994 ) ) ;
#60804=CARTESIAN_POINT ( 'NONE',  ( 8.224510206698742110, 14.34966873604972548, 22.08442372801901143 ) ) ;
#60805=CARTESIAN_POINT ( 'NONE',  ( -5.153800228976328057, -19.02544592524343514, 37.29057627198102409 ) ) ;
#60806=CARTESIAN_POINT ( 'NONE',  ( -10.72451020669898014, 18.67979575497178502, 105.4155762719810383 ) ) ;
#60807=CARTESIAN_POINT ( 'NONE',  ( -16.55341960407617563, 4.379528057220093196, 28.54275706135234358 ) ) ;
#60808=CARTESIAN_POINT ( 'NONE',  ( 4.483927247898790824, -16.52544592524335698, 90.20942372801903275 ) ) ;
#60810=CARTESIAN_POINT ( 'NONE',  ( -21.53943276465977519, -0.05219959533937600094, 83.75109039468568994 ) ) ;
#60811=CARTESIAN_POINT ( 'NONE',  ( -16.46253265017146816, -9.564922557961047289, 79.16775706135234714 ) ) ;
#60812=CARTESIAN_POINT ( 'NONE',  ( -12.06949235617756955, 12.14591786802309770, 45.62390960531436690 ) ) ;
#60813=CARTESIAN_POINT ( 'NONE',  ( -4.483927247898539470, -16.52544592524342804, 102.2905762719810383 ) ) ;
#60814=CARTESIAN_POINT ( 'NONE',  ( -13.97604488694547697, 13.89961937509957934, 43.12609039468566152 ) ) ;
#60815=CARTESIAN_POINT ( 'NONE',  ( 17.31747979337962207, -6.344076630960735486, 56.12055131934818775 ) ) ;
#60816=CARTESIAN_POINT ( 'NONE',  ( 18.62759615963255655, 10.81492255796105972, 46.66775706135234714 ) ) ;
#60817=CARTESIAN_POINT ( 'NONE',  ( 19.02544592524334988, 5.153800228976608722, 111.4594237280190043 ) ) ;
#60818=CARTESIAN_POINT ( 'NONE',  ( 17.05116617787824396, 6.768360034955831495, 83.84324446740799885 ) ) ;
#60819=CARTESIAN_POINT ( 'NONE',  ( -9.474510206698964154, 16.51473224551069663, 110.4155762719810383 ) ) ;
#60820=CARTESIAN_POINT ( 'NONE',  ( -18.67979575497178146, -10.72451020669898902, 71.66557627198100988 ) ) ;
#60821=CARTESIAN_POINT ( 'NONE',  ( 9.474510206698729675, 16.51473224551082808, 92.08442372801900433 ) ) ;
#60822=CARTESIAN_POINT ( 'NONE',  ( -16.51473224551069308, -9.474510206698971260, 101.6655762719810241 ) ) ;
#60824=CARTESIAN_POINT ( 'NONE',  ( -0.05219959533910754901, -16.53943276465976808, 107.4989096053143669 ) ) ;
#60825=CARTESIAN_POINT ( 'NONE',  ( 10.81492255796106328, -18.62759615963255655, 100.4177570613523471 ) ) ;
#60826=CARTESIAN_POINT ( 'NONE',  ( -5.049401038298153566, 19.05341960407611168, 40.20724293864768839 ) ) ;
#60827=CARTESIAN_POINT ( 'NONE',  ( -15.72974639402176322, -15.80617190586768395, 49.37609039468569705 ) ) ;
#60828=CARTESIAN_POINT ( 'NONE',  ( -5.823673210054431948, 21.52544592524334988, 92.70942372801901854 ) ) ;
#60829=CARTESIAN_POINT ( 'NONE',  ( 12.14591786802327356, -12.06949235617739191, 95.62609039468568994 ) ) ;
#60830=CARTESIAN_POINT ( 'NONE',  ( 10.81492255796106328, -18.62759615963255655, 45.41775706135234003 ) ) ;
#60831=CARTESIAN_POINT ( 'NONE',  ( -18.62759615963255300, -10.81492255796106328, 44.16775706135234714 ) ) ;
#60832=CARTESIAN_POINT ( 'NONE',  ( -13.89961937509957401, -13.97604488694547875, 69.37609039468564731 ) ) ;
#60833=CARTESIAN_POINT ( 'NONE',  ( 9.474510206698971260, -16.51473224551069308, 97.91557627198102409 ) ) ;
#60834=CARTESIAN_POINT ( 'NONE',  ( -8.314922557960811034, -14.29746914071050412, 102.0822429386476955 ) ) ;
#60835=CARTESIAN_POINT ( 'NONE',  ( 21.55341960407610458, 5.719274019375980345, 88.95724293864769550 ) ) ;
#60836=CARTESIAN_POINT ( 'NONE',  ( -12.14591786802309592, -12.06949235617757132, 66.87390960531436690 ) ) ;
#60837=CARTESIAN_POINT ( 'NONE',  ( -0.05219959533937732626, 21.53943276465977519, 102.5010903946856899 ) ) ;
#60838=CARTESIAN_POINT ( 'NONE',  ( 4.379528057220339221, -16.55341960407611168, 82.70724293864770971 ) ) ;
#60839=CARTESIAN_POINT ( 'NONE',  ( 9.474510206698971260, -16.51473224551069308, 37.91557627198102409 ) ) ;
#60840=CARTESIAN_POINT ( 'NONE',  ( -19.05341960407617563, 5.049401038297882671, 83.54275706135233293 ) ) ;
#60841=CARTESIAN_POINT ( 'NONE',  ( 16.52544592524342804, -4.483927247898539470, 48.54057627198103120 ) ) ;
#60842=CARTESIAN_POINT ( 'NONE',  ( 21.52544592524334988, 5.823673210054432836, 91.45942372801901854 ) ) ;
#60843=CARTESIAN_POINT ( 'NONE',  ( -0.05219959533909027116, -19.03943276465977164, 97.49890960531436690 ) ) ;
#60844=CARTESIAN_POINT ( 'NONE',  ( 9.474510206698729675, 16.51473224551082808, 67.08442372801900433 ) ) ;
#60845=CARTESIAN_POINT ( 'NONE',  ( 15.80617190586746368, 15.72974639402197994, 59.37390960531436690 ) ) ;
#60846=CARTESIAN_POINT ( 'NONE',  ( 10.81492255796106328, -18.62759615963255655, 35.41775706135234003 ) ) ;
#60847=CARTESIAN_POINT ( 'NONE',  ( 12.14591786802327356, -12.06949235617739191, 25.62609039468567929 ) ) ;
#60848=CARTESIAN_POINT ( 'NONE',  ( 14.34966873604972726, -8.224510206698740333, 85.83442372801901854 ) ) ;
#60849=CARTESIAN_POINT ( 'NONE',  ( -16.51473224551069308, -9.474510206698971260, 21.66557627198102765 ) ) ;
#60850=CARTESIAN_POINT ( 'NONE',  ( 21.55341960407610458, 5.719274019375980345, 113.9572429386477239 ) ) ;
#60851=CARTESIAN_POINT ( 'NONE',  ( -16.52544592524342804, 4.483927247898546575, 111.0405762719810525 ) ) ;
#60853=CARTESIAN_POINT ( 'NONE',  ( -16.53943276465976808, -0.05219959533934237506, 48.75109039468568284 ) ) ;
#60854=CARTESIAN_POINT ( 'NONE',  ( 12.14591786802309770, 12.06949235617756955, 84.37390960531438111 ) ) ;
#60855=CARTESIAN_POINT ( 'NONE',  ( -18.62759615963270932, 10.81492255796079327, 80.83224293864769550 ) ) ;
#60856=CARTESIAN_POINT ( 'NONE',  ( -8.224510206698948167, 14.34966873604960824, 30.41557627198101699 ) ) ;
#60857=CARTESIAN_POINT ( 'NONE',  ( 16.55341960407618274, -4.379528057220086978, 41.04275706135236135 ) ) ;
#60858=CARTESIAN_POINT ( 'NONE',  ( -5.049401038298153566, 19.05341960407611168, 40.20724293864768839 ) ) ;
#60859=CARTESIAN_POINT ( 'NONE',  ( 16.53943276465976808, 0.05219959533934440121, 76.25109039468568994 ) ) ;
#60860=CARTESIAN_POINT ( 'NONE',  ( -19.05341960407617563, 5.049401038297882671, 68.54275706135230450 ) ) ;
#60861=CARTESIAN_POINT ( 'NONE',  ( 21.53943276465977519, -0.05219959533907433946, 73.74890960531433848 ) ) ;
#60862=CARTESIAN_POINT ( 'NONE',  ( 12.06949235617757843, -12.14591786802309237, 23.12390960531436335 ) ) ;
#60865=CARTESIAN_POINT ( 'NONE',  ( -21.53943276465977519, 0.05219959533907696930, 51.24890960531436690 ) ) ;
#60866=VERTEX_POINT ( 'NONE', #155937 ) ;
#60867=CARTESIAN_POINT ( 'NONE',  ( 0.05219959533934541429, -16.53943276465976808, 95.00109039468568994 ) ) ;
#60869=CARTESIAN_POINT ( 'NONE',  ( 16.46253265017160672, -9.564922557960803928, 108.3322429386476955 ) ) ;
#60871=CARTESIAN_POINT ( 'NONE',  ( -0.05219959533909027116, -19.03943276465977164, 42.49890960531435269 ) ) ;
#60872=CARTESIAN_POINT ( 'NONE',  ( 5.719274019375991003, -21.55341960407610458, 72.70724293864769550 ) ) ;
#60873=CARTESIAN_POINT ( 'NONE',  ( 14.29746914071037800, 8.314922557961029526, 101.6677570613523613 ) ) ;
#60874=CARTESIAN_POINT ( 'NONE',  ( 15.72974639402176855, 15.80617190586768217, 61.87609039468568284 ) ) ;
#60875=CARTESIAN_POINT ( 'NONE',  ( 14.29746914071037800, 8.314922557961029526, 21.66775706135235069 ) ) ;
#60876=CARTESIAN_POINT ( 'NONE',  ( -4.379528057220328563, 16.55341960407611168, 110.2072429386477239 ) ) ;
#60877=CARTESIAN_POINT ( 'NONE',  ( -4.483927247898782831, 16.52544592524335698, 22.70942372801901499 ) ) ;
#60878=CARTESIAN_POINT ( 'NONE',  ( -16.46253265017160317, 9.564922557960807481, 55.83224293864769550 ) ) ;
#60880=CARTESIAN_POINT ( 'NONE',  ( -13.97604488694527625, -13.89961937509977652, 106.8739096053143669 ) ) ;
#60881=CARTESIAN_POINT ( 'NONE',  ( 12.06949235617739724, 12.14591786802326823, 86.87609039468568994 ) ) ;
#60882=CARTESIAN_POINT ( 'NONE',  ( -13.97604488694547697, 13.89961937509957934, 88.12609039468563310 ) ) ;
#60883=CARTESIAN_POINT ( 'NONE',  ( 16.51473224551083163, -9.474510206698727899, 25.83442372801900078 ) ) ;
#60884=CARTESIAN_POINT ( 'NONE',  ( 21.53943276465977519, -0.05219959533907433946, 68.74890960531435269 ) ) ;
#60886=CARTESIAN_POINT ( 'NONE',  ( -0.05219959533934338120, 16.53943276465976808, 102.5010903946856899 ) ) ;
#60887=CARTESIAN_POINT ( 'NONE',  ( 5.153800228976615827, -19.02544592524334988, 95.20942372801897591 ) ) ;
#60888=CARTESIAN_POINT ( 'NONE',  ( -19.05341960407611168, -5.049401038298163336, 46.45724293864768129 ) ) ;
#60889=CARTESIAN_POINT ( 'NONE',  ( -16.46253265017160317, 9.564922557960807481, 90.83224293864769550 ) ) ;
#60890=CARTESIAN_POINT ( 'NONE',  ( 5.719274019375673035, 21.55341960407619339, 52.29275706135236135 ) ) ;
#60891=CARTESIAN_POINT ( 'NONE',  ( 16.51473224551069308, 9.474510206698969483, 44.16557627198103120 ) ) ;
#60893=CARTESIAN_POINT ( 'NONE',  ( 5.049401038298161559, -19.05341960407611168, 112.7072429386476813 ) ) ;
#60894=CARTESIAN_POINT ( 'NONE',  ( -12.14591786802309592, -12.06949235617757132, 61.87390960531436690 ) ) ;
#60895=CARTESIAN_POINT ( 'NONE',  ( 18.67979575497178502, 10.72451020669898547, 79.16557627198103830 ) ) ;
#60896=CARTESIAN_POINT ( 'NONE',  ( -18.22780087662124160, -5.499999999999927169, 73.98236817873106475 ) ) ;
#60897=( BOUNDED_SURFACE ( )  B_SPLINE_SURFACE ( 3, 2, ( 
 ( #54697, #113362, #67864, #86034, #22371, #130525, #177069, #52693, #51699, #194231, #162875, #68866, #38540, #145700, #24383, #55697, #10207, #87034, #147721, #40536, #175054, #117370, #9208, #36518, #179067, #159875, #163896, #25392, #7182, #83024, #115381, #6184, #144698, #129519, #114357, #192222, #176062, #37529, #99192, #160880, #84022, #53704, #100196, #161878, #23372, #8195, #165882, #197220, #57710, #164889, #28380, #14163, #13194, #56708, #11209, #29357, #27379, #73878, #120349, #196241, #195227, #137509, #74857, #12215, #182044, #89025, #59670, #75831, #153670, #30335, #106174, #184022, #118381, #199190, #152674, #180075, #183035, #91976, #121342, #136519, #150716, #90987, #58682, #149710, #103207, #15167, #45504, #135548, #198200, #26383, #41544, #107159, #76826, #60657, #43527, #72884, #167857, #122330, #88022, #134553, #44518, #119380, #168830, #181063, #105192, #90018, #42538, #104201, #166879, #151701, #20872, #5696, #174571, #46494, #160390, #200179, #108155, #36037, #130019, #61648, #37035, #6690, #31331, #38047, #92982, #78810, #114879, #191718, #124321, #99703, #190732, #98696, #145207, #128043, #161387, #155661, #51217, #22878, #97686, #16163, #140489, #21879, #53202, #123316, #77817, #159376, #1977, #32328, #112878, #113863, #138497, #83529, #185009, #47501, #169837, #189744, #175559, #63657, #52205, #67372, #68368, #176573, #154667, #139486, #109157, #968, #62644, #186019, #170836, #93981, #17157, #82530, #144212, #129031, #116876, #149228, #165399, #178567, #72382, #43041, #87541, #26892, #177575, #195749, #100699, #194737, #41051, #163396, #102715, #164404, #10719, #40032, #84525, #162380, #135066, #86541, #56207, #147222, #88535, #117890, #146202, #25896, #101706, #7688, #73395, #24893, #11727, #166397, #179580, #42055, #148225, #134057, #23882, #85534, #57223, #118896, #180581, #9719, #71383, #8713, #103719, #133047, #150232, #196742, #70382, #58209, #119878, #104707, #181563, #69372, #131042, #192732, #54214, #115885, #39042, #132050, #193739, #55207, #186532, #136042, #170344, #76341, #75350, #197717, #138017, #123817, #16664, #167380, #61166, #169338, #63153, #12711, #182551, #120851, #124832, #31836, #153176, #137020, #91489, #185515, #479, #184526, #13683, #199700, #78312, #183539, #30847, #48005, #139985, #44033, #92494, #60177, #122837, #198710, #14679, #121846, #93487, #59182, #62153, #155173, #47007, #1474, #46006, #109661, #154183, #107661, #27893, #168356, #89535, #105694, #28877, #15673, #45024, #77333, #151222, #74377, #90517, #139000, #106683, #108666, #29852, #152199, #157163, #175315, #140989, #143968, #36782, #190490, #21630, #66132, #129775, #97443, #127797, #171341, #111647, #160141, #64158, #110646, #35796, #80303, #2477, #113621, #52950, #94480, #98447, #172327, #18657, #83286, #4444, #3464, #159128, #51961, #65141, #20626, #191471, #174327, #144960, #125823, #82275, #187526, #81282, #189498, #49983, #50974, #112634, #5448, #126798, #32829, #48991, #6442, #173333, #142965, #33816, #68123, #67131, #156161, #128789, #188504, #17659, #79319, #34806, #95476, #141976, #96461, #158149, #19640, #40800, #53968, #115642, #102470, #164157, #148983, #54965, #193487, #177331, #194490, #8463, #178325, #55962, #100459, #41806, #26643, #73151, #25655, #116636, #87300, #132803, #70137, #117639, #24647, #161137, #38803, #114625, #134822, #22634, #56973, #163144, #162139, #84280, #86296, #10472, #103474, #23635, #147985, #179337, #149975, #99457, #69127, #7442, #11480, #118647, #39788, #85284, #101453, #72133, #133808, #71138, #146975, #9474, #165152, #196501, #145961, #180338, #195499, #131808, #130793, #88286, #176325, #37794, #192486, #91242, #199454, #93243, #42804, #12476, #150983, #154928, #61907, #183298, #167138, #121602, #15431, #30599, #14431, #43789, #168114, #46765, #13446, #60922, #16426, #108424, #74137, #122596, #90274, #152932, #105453, #44779 ),
 ( #170100, #135809, #197479, #184285, #28637, #89291, #240, #139741, #181325, #123578, #58946, #151958, #31594, #76094, #75110, #45767, #138758, #136778, #107419, #78073, #169092, #185273, #120614, #92252, #182310, #29610, #137769, #198464, #153936, #77089, #57971, #59935, #119643, #106432, #104466, #166150, #27652, #63918, #5208, #34572, #1230, #81056, #95239, #62909, #190247, #80072, #128550, #83050, #96229, #158895, #18422, #127565, #140747, #2235, #189266, #50741, #35561, #141741, #3231, #125587, #142733, #156925, #64905, #4212, #187284, #51724, #113387, #159903, #112400, #126566, #174092, #19407, #188265, #65890, #111409, #47764, #48755, #124589, #97209, #49740, #173094, #157917, #20385, #82032, #21391, #36543, #143729, #175077, #186284, #66889, #98199, #109417, #171096, #32588, #94241, #155921, #17416, #79074, #110408, #172090, #33577, #103235, #133565, #38566, #86059, #176085, #144724, #56740, #26411, #10234, #177094, #160905, #55725, #163923, #164917, #6210, #147748, #191243, #132569, #41572, #115406, #39554, #118411, #9235, #87061, #25419, #24410, #70902, #178085, #52717, #148746, #67890, #114381, #101212, #195255, #129543, #40565, #71894, #37555, #99217, #22398, #85044, #180104, #84048, #130552, #145727, #194258, #102235, #7208, #131566, #68892, #161903, #54723, #192249, #162901, #53731, #146725, #100222, #23397, #8222, #69899, #117397, #193250, #116396, #179096, #60685, #108185, #184049, #134583, #197247, #57738, #136546, #122360, #13221, #137537, #14191, #92005, #153699, #72913, #196269, #119408, #107186, #167886, #45532, #106202, #165910, #181091, #89054, #198227, #74884, #58708, #90046, #150744, #42566, #121371, #168857, #29385, #149738, #104229, #30362, #120378, #166908, #59699, #12243, #88050, #15194, #27408, #151728, #76853, #2, #11239, #73905, #91016, #28407, #182071, #183064, #138524, #169866, #61676, #135575, #43554, #105220, #44547, #123345, #152702, #199219, #75861, #185038, #46525, #16191, #77846, #139513, #50507, #111168, #189033, #49505, #109184, #996, #32354, #141513, #18187, #2005, #33346, #94007, #62670, #64676, #112171, #172858, #93010, #47529, #65659, #63684, #110179, #156693, #155688, #31360, #173859, #34339, #48525, #79844, #125358, #96000, #35326, #190016, #66654, #142501, #20151, #154696, #96979, #158660, #124351, #19175, #128316, #157684, #80823, #187055, #127321, #95005, #186046, #170863, #51490, #81796, #171858, #3979, #17183, #78837, #143483, #113151, #4968, #2999, #140515, #126338, #188035, #133320, #56487, #116157, #21150, #162659, #71653, #145484, #69653, #86816, #177847, #117152, #55482, #54486, #39315, #7970, #82805, #194019, #36306, #144487, #131320, #163672, #97961, #70661, #40314, #67650, #195010, #129307, #115158, #148503, #25174, #160662, #174841, #24165, #132328, #178848, #161660, #159653, #191994, #84800, #5970, #193009, #101991, #191003, #85816, #52479, #100975, #147503, #68644, #8993, #38321, #114138, #175839, #37313, #9993, #130300, #98971, #22153, #83804, #6964, #53480, #176851, #99976, #23157, #146479, #137302, #76620, #199979, #59460, #164672, #105968, #14960, #88813, #12985, #30127, #121133, #60451, #198983, #197989, #182827, #151493, #26167, #122125, #179856, #87808, #74648, #106954, #41326, #13956, #183813, #10991, #138298, #72663, #58476, #91769, #168627, #103988, #118165, #167653, #75623, #45303, #104981, #102986, #135337, #28170, #149494, #136314, #196023, #120143, #153463, #134339, #57498, #119167, #44309, #181834, #12004, #89812, #90786, #180851, #42327, #165667, #27166, #150506, #166668, #152470, #43314, #29149, #73665, #197011, #127084, #46287, #107944, #169630, #80588, #141274, #18943, #79604, #139286, #31126, #62434, #171625, #48288, #32119, #63445, #124107, #92775, #94769, #142263, #2763, #123116, #77616, #95763, #93776, #140275, #186818, #185807, #61445, #3746, #64439, #78601, #109944, #155457, #126110, #65423, #19919 ),
 ( #154464, #170630, #15956, #33113, #34106, #156452, #110932, #187805, #188793, #50275, #763, #47293, #108950, #111933, #49274, #173620, #172619, #16947, #1767, #125121, #17951, #157449, #35089, #96742, #158432, #81561, #143247, #184801, #22918, #66420, #20911, #39082, #175599, #83569, #130060, #5736, #4731, #147262, #84564, #21918, #191759, #98735, #69414, #85576, #163437, #40071, #115924, #193778, #128081, #23921, #162419, #189785, #192769, #101749, #131080, #146242, #160428, #100738, #68407, #159415, #112916, #24934, #55247, #145248, #7728, #36076, #51256, #116915, #86580, #70423, #37076, #82569, #177614, #8752, #174611, #97725, #54253, #144250, #132089, #67413, #6729, #99742, #178608, #129068, #190769, #52244, #113901, #53242, #38087, #114919, #176612, #161426, #194774, #29644, #92286, #9756, #184320, #30633, #117930, #138793, #56248, #195790, #15467, #153970, #25936, #274, #199490, #45801, #169128, #180621, #61943, #134100, #106468, #148263, #91276, #164442, #44813, #77124, #71420, #179619, #87579, #152967, #133084, #41091, #57262, #122630, #107453, #102755, #72422, #118936, #168147, #149266, #10758, #14466, #76128, #137806, #60956, #104160, #85227, #114569, #38746, #120309, #84224, #72841, #166838, #182002, #83230, #134511, #161082, #162085, #176266, #53912, #37738, #135508, #98386, #165841, #197178, #150674, #43485, #23579, #89978, #57669, #146918, #128733, #69071, #105152, #21570, #68067, #196197, #99399, #160084, #73837, #13153, #51905, #58643, #129721, #22577, #28339, #8407, #145903, #119336, #12172, #7387, #181022, #151659, #42496, #190429, #144905, #27338, #6388, #100404, #88984, #130738, #113564, #175258, #36724, #192430, #191418, #52894, #115587, #177275, #184966, #137467, #78766, #108110, #74816, #154626, #168788, #136478, #63612, #153627, #1933, #156622, #169794, #32285, #91935, #926, #14122, #75789, #62600, #124278, #109114, #15123, #76785, #199147, #16120, #30290, #138456, #77776, #60613, #125287, #186984, #33278, #185974, #200137, #47458, #92938, #61606, #139444, #46450, #121302, #122288, #198158, #94937, #182994, #17115, #123275, #183977, #44477, #93940, #170793, #155619, #140443, #152632, #106132, #45463, #31287, #48455, #107117, #110112, #171790, #167816, #59628, #29315, #90945, #79772, #34270, #52409, #188964, #96910, #143412, #19105, #18117, #160592, #97889, #35256, #4900, #112099, #82734, #98898, #176777, #53407, #129236, #6893, #141442, #37242, #175766, #2929, #5901, #115085, #144415, #36237, #173789, #114068, #81727, #172789, #126271, #38249, #68571, #158593, #159581, #49438, #64608, #130228, #99904, #83732, #50440, #95929, #190932, #22081, #187968, #111099, #21078, #157614, #67578, #80755, #20082, #113079, #191923, #145411, #142432, #3911, #65591, #127251, #51419, #66582, #128247, #189944, #174771, #67138, #21638, #20631, #3470, #99464, #82283, #4449, #159134, #52956, #68130, #51968, #81288, #5455, #84288, #50980, #36788, #130801, #145967, #49989, #98454, #127802, #128796, #142972, #143975, #66139, #161144, #65147, #129781, #22641, #114632, #7449, #190495, #53975, #83292, #113627, #95483, #35802, #69133, #188512, #34812, #160147, #189505, #126804, #37801, #177338, #18663, #192492, #157169, #111654, #191478, #112640, #174332, #175322, #96467, #80309, #115648, #144968, #97448, #6449, #176331, #141982, #173340, #158155, #19647, #149981, #27658, #38809, #57977, #196507, #162146, #26650, #135815, #165158, #56979, #132810, #73158, #102476, #193493, #146982, #197485, #89298, #194496, #180344, #70143, #100467, #150990, #120620, #104472, #71144, #54972, #11487, #119649, #58952, #23642, #41812, #85290, #88293, #8469, #9480, #133815, #12482, #103480, #181331, #42810, #118653, #134828, #72139, #131814, #166157, #116642, #178332, #74143, #39795, #101459, #163150, #24653, #86302, #147991, #55969, #179343, #117646, #40806, #164163, #25661, #87306, #148989, #10479, #195506 ),
 ( #76101, #92259, #154936, #2242, #78082, #28644, #91248, #151964, #30606, #16433, #107427, #31601, #108431, #186291, #47771, #167145, #90280, #13452, #1237, #61916, #139750, #247, #59941, #75116, #183304, #153943, #169099, #152939, #184293, #44786, #136784, #15438, #62916, #123586, #109424, #198470, #121609, #106439, #124596, #185280, #171103, #46772, #168120, #29616, #14438, #77097, #138766, #137776, #45775, #199462, #60929, #170107, #32596, #93250, #43796, #122603, #94249, #155929, #17424, #79081, #140754, #182316, #63925, #105459, #142740, #50749, #19414, #190255, #6219, #84057, #160913, #36553, #114391, #125594, #144732, #83058, #48762, #113395, #22406, #51732, #143737, #81062, #159911, #189273, #80079, #33584, #145735, #176093, #4220, #66897, #156932, #187291, #37563, #7216, #191251, #157924, #141748, #98207, #67898, #110417, #172098, #128560, #95247, #175085, #18429, #96236, #20393, #99226, #21400, #129551, #52726, #5216, #3238, #158902, #64912, #126573, #188274, #49747, #111416, #173102, #34579, #65898, #127572, #112407, #174099, #35568, #97216, #82040, #57747, #54733, #27417, #118420, #26420, #72923, #55734, #89063, #86068, #179105, #165921, #163932, #146735, #70911, #88060, #181101, #192258, #8231, #87070, #9244, #162911, #40574, #41581, #150754, #164927, #115414, #178094, #38574, #117408, #103245, #194267, #180113, #195265, #134592, #102244, #116405, #25429, #39564, #196278, #100230, #149747, #119417, #11249, #42575, #148755, #68901, #56749, #10244, #130560, #132579, #104238, #161912, #69909, #133575, #101222, #23406, #53740, #177103, #85054, #131575, #193259, #24419, #147758, #71903, #44556, #76864, #93020, #106211, #12, #170873, #15205, #154708, #105229, #123355, #28418, #122370, #168867, #91025, #30372, #92016, #138534, #167895, #12252, #90055, #62680, #14202, #184059, #74893, #16201, #45542, #73914, #153709, #29395, #135584, #1006, #152711, #139523, #94017, #107196, #169877, #75870, #61686, #151737, #13230, #185048, #46536, #108195, #137546, #199229, #136556, #31370, #60694, #77856, #124361, #198237, #186056, #47540, #32364, #109194, #197256, #58718, #120387, #182081, #43564, #166917, #59708, #121381, #183073, #114150, #63694, #97972, #3990, #3010, #125369, #65670, #51502, #144498, #95015, #189044, #96991, #191014, #127332, #81808, #80835, #187065, #159664, #142512, #64687, #19186, #113162, #128329, #112182, #141523, #50519, #5981, #111179, #158673, #52490, #67661, #110189, #20163, #188046, #175851, #129318, #49516, #143495, #48535, #155698, #37324, #17193, #21161, #172869, #171867, #66666, #174852, #78847, #140525, #4980, #2015, #190028, #33356, #126349, #173870, #156703, #36318, #82816, #18197, #35338, #79854, #34350, #96011, #157695, #160672, #68655, #105734, #178861, #40327, #10006, #167421, #192006, #198752, #53492, #39328, #75390, #90557, #84811, #60217, #148516, #56500, #28917, #85828, #121887, #116169, #9006, #183580, #194032, #176862, #100987, #118178, #13724, #22164, #38331, #117165, #162671, #193020, #70673, #71666, #98982, #195024, #145495, #7981, #130311, #147516, #133333, #24177, #182591, #25188, #152239, #137062, #83815, #6975, #115169, #44075, #102003, #99987, #163685, #161672, #23168, #146490, #132340, #55495, #69665, #86830, #131332, #54497, #177859, #64201, #63197, #106723, #61206, #79363, #15715, #123859, #170387, #46047, #45065, #187568, #124877, #62195, #31878, #139043, #109705, #125868, #3508, #80347, #156206, #33860, #168397, #49035, #2521, #29892, #32874, #142019, #171387, #186576, #523, #141034, #108708, #199740, #153217, #91530, #110690, #172370, #14722, #94524, #65184, #17706, #48049, #185557, #95520, #93532, #122878, #76382, #126843, #157206, #47051, #18700, #138059, #184566, #107702, #169381, #30889, #77375, #92536, #154225, #155217, #16706, #78356, #140030, #1519, #176369, #85329, #159172, #83329, #100504, #191518, #130839, #69173, #68167 ),
 ( #81326, #128832, #162183, #177375, #174370, #147021, #37842, #146005, #192530, #175358, #8505, #5492, #98492, #70183, #145006, #66177, #190531, #7488, #23681, #111692, #127839, #6487, #52005, #82321, #160185, #161183, #188549, #84326, #34849, #97486, #158194, #36826, #22679, #113664, #99502, #114673, #54013, #115687, #173379, #96504, #50027, #35840, #19684, #21675, #20667, #52995, #38847, #144011, #143009, #4487, #189545, #51017, #112678, #67175, #129819, #41852, #88329, #10516, #150020, #11525, #58013, #164199, #131851, #9516, #182353, #133853, #103518, #194534, #135850, #165194, #193534, #73195, #25697, #55008, #120655, #72179, #43831, #116678, #151025, #89333, #178368, #119683, #28680, #181366, #134865, #87342, #166191, #195543, #86340, #39832, #90315, #105495, #149028, #196543, #163187, #101498, #167181, #13487, #197520, #57017, #148027, #42845, #12516, #152001, #24691, #104510, #71182, #27692, #132846, #102516, #26689, #56005, #74180, #58988, #117683, #179380, #40842, #118690, #180382, #94283, #136823, #44822, #79114, #154971, #16467, #186325, #140787, #168156, #172132, #29653, #15477, #48797, #63959, #60965, #33618, #124630, #32629, #2276, #61953, #95281, #92296, #185315, #156964, #170142, #152976, #77134, #155961, #187326, #198507, #14475, #93286, #138803, #169138, #46806, #47807, #75152, #171140, #121645, #184329, #106477, #123620, #109457, #284, #17458, #1273, #125628, #108465, #30643, #110451, #59978, #183340, #78116, #91285, #139785, #76137, #137815, #199499, #31637, #62950, #45811, #122639, #107462, #153980, #51762, #37594, #36583, #80112, #34611, #52753, #189304, #97247, #143767, #19447, #18461, #160943, #98238, #35601, #5248, #112441, #83088, #99256, #177134, #53769, #129582, #159941, #21428, #191278, #84085, #111449, #115443, #173136, #158935, #192289, #7246, #4254, #38605, #67928, #176123, #22436, #66929, #100261, #20424, #128592, #141780, #113423, #96270, #82074, #145764, #130593, #3274, #157956, #144764, #190286, #174130, #175115, #114422, #64946, #68931, #126605, #127605, #188307, #6249, #49784, #81095, #142773, #65933, #50781, #102275, #55764, #12279, #120416, #181131, #41611, #119446, #180142, #39594, #69941, #162942, #71934, #148786, #132609, #163963, #24449, #131605, #195297, #42605, #103276, #23437, #178127, #196306, #194298, #40604, #87101, #86098, #161942, #104269, #164956, #179136, #10275, #117438, #26449, #165951, #182107, #197284, #72952, #150784, #85084, #27451, #89092, #146768, #149777, #58747, #88091, #11279, #25461, #57776, #133604, #116438, #193290, #43592, #73944, #56778, #134622, #54764, #8261, #135613, #101253, #147789, #118451, #9275, #70941, #124394, #63725, #187097, #46567, #151765, #93052, #2045, #75902, #43, #17226, #108228, #47572, #186089, #185078, #169908, #138565, #13258, #109224, #166944, #74921, #170903, #184091, #30404, #106241, #105258, #32395, #31401, #122401, #92050, #199260, #154739, #94050, #125400, #140557, #16235, #155728, #28447, #78878, #62712, #90083, #77887, #136584, #139555, #123386, #60727, #1039, #168898, #59740, #198264, #121409, #183103, #45574, #44584, #167923, #29423, #91054, #152741, #14231, #137576, #107227, #153739, #15235, #76894, #61718, #190057, #95048, #36351, #145528, #19219, #143527, #160706, #51533, #191048, #129353, #128361, #113196, #81839, #156737, #67695, #110220, #18230, #52521, #174885, #98004, #159698, #114182, #141555, #7007, #3044, #189079, #22197, #37357, #34383, #68689, #21195, #6016, #175886, #35371, #130344, #65701, #158704, #48567, #5015, #126382, #50552, #99015, #83846, #171901, #188079, #66697, #112212, #142545, #20193, #82851, #33389, #144530, #79885, #157730, #64720, #97023, #49550, #173902, #111213, #172905, #96043, #80869, #4023, #127367, #150549, #11035, #71699, #149540, #10039, #69698, #100020, #193054, #102037, #178894, #162706, #194067, #54531, #161707, #25222, #72711, #133366, #53524 ),
 ( #134383, #115202, #23203, #196069, #195057, #56535, #103036, #57542, #84846, #88856, #146524, #132374, #165713, #180896, #177893, #12048, #41370, #119211, #42371, #40362, #73712, #9037, #163720, #192043, #86864, #131365, #55528, #104034, #27210, #176894, #116204, #118213, #117202, #85860, #148548, #164718, #38365, #87852, #8015, #101021, #39363, #179904, #26213, #24211, #147549, #70706, #139331, #75668, #29195, #185855, #93822, #154508, #15005, #92822, #153508, #13028, #43357, #136359, #45347, #122170, #106012, #137345, #198035, #105028, #168672, #16004, #76665, #197054, #151539, #169676, #167698, #14001, #60494, #59503, #135384, #77662, #138344, #152513, #183860, #90829, #200024, #810, #155502, #170677, #46334, #124155, #58522, #62483, #47341, #120188, #123162, #32165, #61492, #184850, #199025, #31172, #106999, #89856, #166712, #16995, #108996, #30173, #107990, #28216, #181878, #74694, #121178, #182872, #91816, #44353, #189830, #97773, #37121, #160474, #19966, #125168, #66466, #175646, #49320, #80635, #141321, #48336, #111978, #159460, #96789, #140324, #94819, #112963, #110980, #157496, #3792, #79652, #78649, #20956, #158478, #95810, #65469, #172665, #143292, #82613, #98780, #113947, #51302, #67458, #1814, #144294, #36121, #63493, #128128, #186867, #4778, #81608, #34151, #174656, #142312, #33160, #109991, #171671, #129116, #18989, #5784, #156497, #17999, #190815, #2810, #52290, #127132, #64488, #126155, #187851, #188838, #50323, #173670, #35137, #9801, #118980, #192816, #116962, #134143, #24978, #164484, #102798, #101793, #86624, #55290, #130110, #41134, #83616, #191806, #25978, #163481, #148307, #133128, #87621, #114966, #180663, #176659, #162465, #195832, #10801, #7778, #42139, #71463, #179664, #149307, #8797, #103800, #39127, #132133, #21965, #178653, #99789, #23966, #72470, #57304, #145294, #161475, #40115, #85621, #115970, #193825, #194819, #6777, #117973, #68456, #131128, #53287, #70467, #56291, #147308, #38136, #22964, #84612, #146291, #177658, #69461, #54298, #100782, #45110, #122923, #183628, #43123, #73476, #166479, #75436, #152284, #106767, #59268, #26976, #154269, #44120, #92581, #47093, #60262, #184611, #182637, #91577, #104791, #27978, #153266, #14767, #199785, #105779, #167466, #89617, #168442, #120937, #28961, #29938, #151306, #15760, #77419, #123905, #76428, #90602, #138104, #61253, #13768, #46092, #137110, #11812, #12795, #165480, #185604, #135149, #107747, #198796, #74460, #196822, #121933, #169428, #139091, #136126, #30933, #566, #62237, #88619, #150316, #58289, #119958, #181644, #197802, #17752, #172419, #68962, #84116, #65228, #94572, #18745, #100294, #64246, #50075, #146801, #161972, #63241, #111736, #141079, #142064, #156250, #33907, #79408, #115476, #78399, #145795, #177164, #130624, #23468, #3550, #69972, #37625, #126888, #108754, #49081, #85117, #1566, #48090, #173423, #2564, #140075, #53800, #80392, #124921, #38637, #170430, #125913, #8294, #188594, #187611, #99288, #192320, #110738, #160974, #131639, #22468, #193322, #186618, #7278, #109746, #31922, #93576, #95564, #155261, #16751, #171430, #157251, #32917, #132641, #105287, #56809, #164986, #117469, #58778, #88123, #54796, #134652, #26481, #101285, #179167, #116471, #13287, #162975, #197314, #103307, #102304, #24480, #149807, #150813, #43623, #194329, #11313, #196338, #90112, #72983, #181160, #180174, #86130, #120446, #41642, #163993, #118483, #12310, #27482, #57806, #40635, #119477, #166975, #10307, #42636, #151796, #28478, #9307, #104299, #87132, #165981, #25490, #89125, #148817, #182140, #147822, #73975, #74951, #135644, #136614, #178160, #39625, #70973, #55797, #71964, #195329, #133638, #91086, #137609, #62743, #107259, #29454, #140585, #169939, #152773, #2075, #59772, #45606, #110247, #31430, #30436, #124423, #78908, #92083, #186119, #156765, #1068, #63754, #14265, #109253, #75934, #108259, #154767, #76926 ),
 ( #77916, #153772, #121440, #187124, #138596, #125428, #79912, #93084, #155757, #15267, #47599, #199292, #60760, #170932, #32423, #94078, #78, #61748, #122432, #139583, #123416, #185109, #17255, #184124, #48596, #171929, #18259, #33418, #46599, #95077, #16265, #198295, #183133, #44617, #106270, #167955, #168930, #38397, #112241, #36381, #53557, #144562, #83878, #22229, #21228, #6048, #174917, #49579, #160737, #3072, #111242, #145560, #82884, #67726, #52553, #7038, #34412, #100053, #96070, #81871, #115235, #130377, #127399, #161739, #191080, #99047, #68720, #128391, #23234, #158733, #51563, #141584, #98035, #19250, #143562, #192075, #176926, #64748, #80897, #159732, #5045, #35400, #113227, #114214, #126410, #37390, #188106, #50581, #172933, #190088, #175919, #66731, #157760, #129384, #142574, #4053, #97051, #65730, #189108, #173932, #20223, #42403, #103069, #162738, #193086, #85895, #195089, #71730, #55561, #86896, #147583, #54561, #118246, #104066, #164751, #146555, #101053, #119244, #117235, #163754, #10070, #9069, #84878, #27241, #26246, #102069, #133400, #178928, #149573, #165747, #43389, #120220, #196104, #73744, #8051, #88890, #150582, #69730, #72747, #181910, #11069, #87885, #40398, #180928, #148580, #39393, #116234, #105061, #135416, #25254, #134418, #177925, #131398, #197087, #166745, #12081, #56572, #24246, #57574, #58554, #179937, #70739, #41404, #132406, #194099, #139358, #122199, #137376, #124184, #170704, #154535, #138372, #16032, #76695, #182902, #74726, #106041, #30203, #168701, #14031, #183891, #167727, #136390, #153538, #77690, #200052, #89888, #121211, #31199, #75696, #60524, #107029, #29225, #28248, #839, #61521, #45376, #91844, #15035, #46361, #62512, #93851, #32193, #92850, #185885, #151571, #47370, #109025, #198067, #169705, #13060, #59533, #44386, #123190, #90858, #108019, #184879, #199054, #152543, #197723, #102721, #150238, #40040, #8720, #120858, #90524, #74383, #41058, #24900, #119884, #27899, #167388, #70389, #11734, #55214, #196748, #105701, #179586, #103725, #182558, #73401, #151228, #89542, #88541, #135072, #42061, #116883, #12717, #132057, #178575, #136048, #58215, #181569, #43047, #59189, #101713, #28884, #163404, #149234, #44041, #193746, #194743, #86547, #104713, #166403, #148231, #195755, #9725, #25902, #118903, #71389, #165405, #133053, #10725, #56215, #117896, #164410, #87547, #26898, #72389, #134064, #180587, #57229, #172334, #48012, #198717, #61173, #121854, #91496, #16671, #122845, #183546, #94487, #123824, #106690, #156169, #13690, #199708, #64165, #185522, #184533, #78320, #32837, #46013, #139993, #110654, #155181, #17668, #45032, #63160, #168363, #62160, #108673, #30854, #170351, #31843, #1482, #107668, #152206, #29859, #2484, #154190, #47014, #14686, #79326, #93494, #75357, #124839, #169345, #137027, #140996, #92501, #125830, #33823, #186539, #109668, #15680, #171348, #153183, #76348, #187533, #48998, #60184, #77341, #139007, #138025, #487, #125148, #45329, #13983, #126136, #95790, #79632, #46316, #30153, #186847, #33140, #172643, #75649, #155483, #60475, #1795, #110959, #184830, #108977, #187831, #16975, #156477, #94798, #93803, #78629, #47322, #122151, #17978, #137327, #183840, #141300, #140304, #63473, #48316, #2790, #106979, #34131, #168653, #154490, #49300, #64469, #200006, #199008, #109971, #171650, #91796, #791, #153490, #31154, #124136, #14986, #170658, #76646, #15984, #138324, #61472, #123143, #107971, #32146, #77643, #169658, #185835, #92802, #139312, #62463, #3772, #66445, #127111, #5762, #130087, #53267, #65449, #128106, #188818, #67438, #191786, #82593, #6755, #83594, #161453, #97753, #51282, #7756, #115951, #176638, #37101, #114945, #175627, #35116, #50301, #158457, #129095, #144275, #189810, #159441, #19946, #111958, #190795, #38113, #98760, #18969, #173647, #99768, #112943, #36101, #52269, #81587, #157476, #22944, #160453, #174636 ) ),
 .UNSPECIFIED., .T., .F., .F. ) 
 B_SPLINE_SURFACE_WITH_KNOTS ( ( 4, 3, 4 ),
 ( 3, 2, 2, 2, 2, 2, 2, 2, 2, 2, 2, 2, 2, 2, 2, 2, 2, 2, 2, 2, 2, 2, 2, 2, 2, 2, 2, 2, 2, 2, 2, 2, 2, 2, 2, 2, 2, 2, 2, 2, 2, 2, 2, 2, 2, 2, 2, 2, 2, 2, 2, 2, 2, 2, 2, 2, 2, 2, 2, 2, 2, 2, 2, 2, 2, 2, 2, 2, 2, 2, 2, 2, 2, 2, 2, 2, 2, 2, 2, 2, 2, 2, 2, 2, 2, 2, 2, 2, 2, 2, 2, 2, 2, 2, 2, 2, 2, 2, 2, 2, 2, 2, 2, 2, 2, 2, 2, 2, 2, 2, 2, 2, 2, 2, 2, 2, 2, 2, 2, 2, 2, 2, 2, 2, 2, 2, 2, 2, 2, 2, 2, 2, 2, 2, 2, 2, 2, 2, 2, 2, 2, 2, 2, 2, 2, 2, 2, 2, 2, 2, 2, 2, 2, 2, 2, 2, 2, 2, 2, 2, 2, 2, 2, 2, 2, 2, 2, 2, 2, 2, 2, 2, 2, 2, 2, 2, 2, 2, 2, 2, 2, 2, 2, 2, 2, 2, 2, 2, 2, 2, 2, 2, 2, 2, 2, 2, 2, 2, 2, 2, 2, 2, 2, 2, 2, 2, 2, 2, 2, 2, 2, 2, 2, 2, 2, 2, 2, 2, 2, 2, 2, 2, 2, 2, 2, 2, 2, 2, 3 ),
 ( 0.000000000000000000, 0.5000000000000000000, 1.000000000000000000 ),
 ( 0.000000000000000000, 0.004385964912280701511, 0.008771929824561403022, 0.01315789473684210453, 0.01754385964912280604, 0.02192982456140350755, 0.02631578947368420907, 0.03070175438596491058, 0.03508771929824561209, 0.03947368421052631360, 0.04385964912280701511, 0.04824561403508771662, 0.05263157894736841813, 0.05701754385964911964, 0.06140350877192982115, 0.06578947368421052266, 0.07017543859649122417, 0.07456140350877192569, 0.07894736842105262720, 0.08333333333333332871, 0.08771929824561403022, 0.09210526315789473173, 0.09649122807017543324, 0.1008771929824561348, 0.1052631578947368363, 0.1096491228070175378, 0.1140350877192982393, 0.1184210526315789408, 0.1228070175438596423, 0.1271929824561403577, 0.1315789473684210453, 0.1359649122807017607, 0.1403508771929824483, 0.1447368421052631637, 0.1491228070175438514, 0.1535087719298245668, 0.1578947368421052544, 0.1622807017543859698, 0.1666666666666666574, 0.1710526315789473728, 0.1754385964912280604, 0.1798245614035087758, 0.1842105263157894635, 0.1885964912280701788, 0.1929824561403508665, 0.1973684210526315819, 0.2017543859649122695, 0.2061403508771929849, 0.2105263157894736725, 0.2149122807017543879, 0.2192982456140350755, 0.2236842105263157909, 0.2280701754385964786, 0.2324561403508771940, 0.2368421052631578816, 0.2412280701754385970, 0.2456140350877192846, 0.2500000000000000000, 0.2543859649122807154, 0.2587719298245614308, 0.2631578947368420907, 0.2675438596491228060, 0.2719298245614035214, 0.2763157894736842368, 0.2807017543859648967, 0.2850877192982456121, 0.2894736842105263275, 0.2938596491228070429, 0.2982456140350877027, 0.3026315789473684181, 0.3070175438596491335, 0.3114035087719298489, 0.3157894736842105088, 0.3201754385964912242, 0.3245614035087719396, 0.3289473684210526550, 0.3333333333333333148, 0.3377192982456140302, 0.3421052631578947456, 0.3464912280701754610, 0.3508771929824561209, 0.3552631578947368363, 0.3596491228070175517, 0.3640350877192982670, 0.3684210526315789269, 0.3728070175438596423, 0.3771929824561403577, 0.3815789473684210731, 0.3859649122807017330, 0.3903508771929824483, 0.3947368421052631637, 0.3991228070175438791, 0.4035087719298245390, 0.4078947368421052544, 0.4122807017543859698, 0.4166666666666666852, 0.4210526315789473450, 0.4254385964912280604, 0.4298245614035087758, 0.4342105263157894912, 0.4385964912280701511, 0.4429824561403508665, 0.4473684210526315819, 0.4517543859649122973, 0.4561403508771929571, 0.4605263157894736725, 0.4649122807017543879, 0.4692982456140351033, 0.4736842105263157632, 0.4780701754385964786, 0.4824561403508771940, 0.4868421052631579093, 0.4912280701754385692, 0.4956140350877192846, 0.5000000000000000000, 0.5043859649122807154, 0.5087719298245614308, 0.5131578947368421462, 0.5175438596491228616, 0.5219298245614034659, 0.5263157894736841813, 0.5307017543859648967, 0.5350877192982456121, 0.5394736842105263275, 0.5438596491228070429, 0.5482456140350877583, 0.5526315789473684736, 0.5570175438596490780, 0.5614035087719297934, 0.5657894736842105088, 0.5701754385964912242, 0.5745614035087719396, 0.5789473684210526550, 0.5833333333333333703, 0.5877192982456140857, 0.5921052631578946901, 0.5964912280701754055, 0.6008771929824561209, 0.6052631578947368363, 0.6096491228070175517, 0.6140350877192982670, 0.6184210526315789824, 0.6228070175438596978, 0.6271929824561403022, 0.6315789473684210176, 0.6359649122807017330, 0.6403508771929824483, 0.6447368421052631637, 0.6491228070175438791, 0.6535087719298245945, 0.6578947368421053099, 0.6622807017543859143, 0.6666666666666666297, 0.6710526315789473450, 0.6754385964912280604, 0.6798245614035087758, 0.6842105263157894912, 0.6885964912280702066, 0.6929824561403509220, 0.6973684210526315264, 0.7017543859649122417, 0.7061403508771929571, 0.7105263157894736725, 0.7149122807017543879, 0.7192982456140351033, 0.7236842105263158187, 0.7280701754385965341, 0.7324561403508771384, 0.7368421052631578538, 0.7412280701754385692, 0.7456140350877192846, 0.7500000000000000000, 0.7543859649122807154, 0.7587719298245614308, 0.7631578947368421462, 0.7675438596491228616, 0.7719298245614034659, 0.7763157894736841813, 0.7807017543859648967, 0.7850877192982456121, 0.7894736842105263275, 0.7938596491228070429, 0.7982456140350877583, 0.8026315789473684736, 0.8070175438596490780, 0.8114035087719297934, 0.8157894736842105088, 0.8201754385964912242, 0.8245614035087719396, 0.8289473684210526550, 0.8333333333333333703, 0.8377192982456140857, 0.8421052631578946901, 0.8464912280701754055, 0.8508771929824561209, 0.8552631578947368363, 0.8596491228070175517, 0.8640350877192982670, 0.8684210526315789824, 0.8728070175438596978, 0.8771929824561403022, 0.8815789473684210176, 0.8859649122807017330, 0.8903508771929824483, 0.8947368421052631637, 0.8991228070175438791, 0.9035087719298245945, 0.9078947368421053099, 0.9122807017543859143, 0.9166666666666666297, 0.9210526315789473450, 0.9254385964912280604, 0.9298245614035087758, 0.9342105263157894912, 0.9385964912280702066, 0.9429824561403509220, 0.9473684210526315264, 0.9517543859649122417, 0.9561403508771929571, 0.9605263157894736725, 0.9649122807017543879, 0.9692982456140351033, 0.9736842105263158187, 0.9780701754385965341, 0.9824561403508771384, 0.9868421052631578538, 0.9912280701754385692, 0.9956140350877192846, 1.000000000000000000 ),
 .UNSPECIFIED. ) 
 GEOMETRIC_REPRESENTATION_ITEM ( )  RATIONAL_B_SPLINE_SURFACE ( (
 ( 1.000000000000000000, 0.9659258262890683122, 1.000000000000000000, 0.9659258262890683122, 1.000000000000000000, 0.9659258262890683122, 1.000000000000000000, 0.9659258262890683122, 1.000000000000000000, 0.9659258262890683122, 1.000000000000000000, 0.9659258262890683122, 1.000000000000000000, 0.9659258262890683122, 1.000000000000000000, 0.9659258262890683122, 1.000000000000000000, 0.9659258262890683122, 1.000000000000000000, 0.9659258262890683122, 1.000000000000000000, 0.9659258262890683122, 1.000000000000000000, 0.9659258262890683122, 1.000000000000000000, 0.9659258262890683122, 1.000000000000000000, 0.9659258262890683122, 1.000000000000000000, 0.9659258262890683122, 1.000000000000000000, 0.9659258262890683122, 1.000000000000000000, 0.9659258262890683122, 1.000000000000000000, 0.9659258262890683122, 1.000000000000000000, 0.9659258262890683122, 1.000000000000000000, 0.9659258262890683122, 1.000000000000000000, 0.9659258262890683122, 1.000000000000000000, 0.9659258262890683122, 1.000000000000000000, 0.9659258262890683122, 1.000000000000000000, 0.9659258262890683122, 1.000000000000000000, 0.9659258262890683122, 1.000000000000000000, 0.9659258262890683122, 1.000000000000000000, 0.9659258262890683122, 1.000000000000000000, 0.9659258262890683122, 1.000000000000000000, 0.9659258262890683122, 1.000000000000000000, 0.9659258262890683122, 1.000000000000000000, 0.9659258262890683122, 1.000000000000000000, 0.9659258262890683122, 1.000000000000000000, 0.9659258262890683122, 1.000000000000000000, 0.9659258262890683122, 1.000000000000000000, 0.9659258262890683122, 1.000000000000000000, 0.9659258262890683122, 1.000000000000000000, 0.9659258262890683122, 1.000000000000000000, 0.9659258262890683122, 1.000000000000000000, 0.9659258262890683122, 1.000000000000000000, 0.9659258262890683122, 1.000000000000000000, 0.9659258262890683122, 1.000000000000000000, 0.9659258262890683122, 1.000000000000000000, 0.9659258262890683122, 1.000000000000000000, 0.9659258262890683122, 1.000000000000000000, 0.9659258262890683122, 1.000000000000000000, 0.9659258262890683122, 1.000000000000000000, 0.9659258262890683122, 1.000000000000000000, 0.9659258262890683122, 1.000000000000000000, 0.9659258262890683122, 1.000000000000000000, 0.9659258262890683122, 1.000000000000000000, 0.9659258262890683122, 1.000000000000000000, 0.9659258262890683122, 1.000000000000000000, 0.9659258262890683122, 1.000000000000000000, 0.9659258262890683122, 1.000000000000000000, 0.9659258262890683122, 1.000000000000000000, 0.9659258262890683122, 1.000000000000000000, 0.9659258262890683122, 1.000000000000000000, 0.9659258262890683122, 1.000000000000000000, 0.9659258262890683122, 1.000000000000000000, 0.9659258262890683122, 1.000000000000000000, 0.9659258262890683122, 1.000000000000000000, 0.9659258262890683122, 1.000000000000000000, 0.9659258262890683122, 1.000000000000000000, 0.9659258262890683122, 1.000000000000000000, 0.9659258262890683122, 1.000000000000000000, 0.9659258262890683122, 1.000000000000000000, 0.9659258262890683122, 1.000000000000000000, 0.9659258262890683122, 1.000000000000000000, 0.9659258262890683122, 1.000000000000000000, 0.9659258262890683122, 1.000000000000000000, 0.9659258262890683122, 1.000000000000000000, 0.9659258262890683122, 1.000000000000000000, 0.9659258262890683122, 1.000000000000000000, 0.9659258262890683122, 1.000000000000000000, 0.9659258262890683122, 1.000000000000000000, 0.9659258262890683122, 1.000000000000000000, 0.9659258262890683122, 1.000000000000000000, 0.9659258262890683122, 1.000000000000000000, 0.9659258262890683122, 1.000000000000000000, 0.9659258262890683122, 1.000000000000000000, 0.9659258262890683122, 1.000000000000000000, 0.9659258262890683122, 1.000000000000000000, 0.9659258262890683122, 1.000000000000000000, 0.9659258262890683122, 1.000000000000000000, 0.9659258262890683122, 1.000000000000000000, 0.9659258262890683122, 1.000000000000000000, 0.9659258262890683122, 1.000000000000000000, 0.9659258262890683122, 1.000000000000000000, 0.9659258262890683122, 1.000000000000000000, 0.9659258262890683122, 1.000000000000000000, 0.9659258262890683122, 1.000000000000000000, 0.9659258262890683122, 1.000000000000000000, 0.9659258262890683122, 1.000000000000000000, 0.9659258262890683122, 1.000000000000000000, 0.9659258262890683122, 1.000000000000000000, 0.9659258262890683122, 1.000000000000000000, 0.9659258262890683122, 1.000000000000000000, 0.9659258262890683122, 1.000000000000000000, 0.9659258262890683122, 1.000000000000000000, 0.9659258262890683122, 1.000000000000000000, 0.9659258262890683122, 1.000000000000000000, 0.9659258262890683122, 1.000000000000000000, 0.9659258262890683122, 1.000000000000000000, 0.9659258262890683122, 1.000000000000000000, 0.9659258262890683122, 1.000000000000000000, 0.9659258262890683122, 1.000000000000000000, 0.9659258262890683122, 1.000000000000000000, 0.9659258262890683122, 1.000000000000000000, 0.9659258262890683122, 1.000000000000000000, 0.9659258262890683122, 1.000000000000000000, 0.9659258262890683122, 1.000000000000000000, 0.9659258262890683122, 1.000000000000000000, 0.9659258262890683122, 1.000000000000000000, 0.9659258262890683122, 1.000000000000000000, 0.9659258262890683122, 1.000000000000000000, 0.9659258262890683122, 1.000000000000000000, 0.9659258262890683122, 1.000000000000000000, 0.9659258262890683122, 1.000000000000000000, 0.9659258262890683122, 1.000000000000000000, 0.9659258262890683122, 1.000000000000000000, 0.9659258262890683122, 1.000000000000000000, 0.9659258262890683122, 1.000000000000000000, 0.9659258262890683122, 1.000000000000000000, 0.9659258262890683122, 1.000000000000000000, 0.9659258262890683122, 1.000000000000000000, 0.9659258262890683122, 1.000000000000000000, 0.9659258262890683122, 1.000000000000000000, 0.9659258262890683122, 1.000000000000000000, 0.9659258262890683122, 1.000000000000000000, 0.9659258262890683122, 1.000000000000000000, 0.9659258262890683122, 1.000000000000000000, 0.9659258262890683122, 1.000000000000000000, 0.9659258262890683122, 1.000000000000000000, 0.9659258262890683122, 1.000000000000000000, 0.9659258262890683122, 1.000000000000000000, 0.9659258262890683122, 1.000000000000000000, 0.9659258262890683122, 1.000000000000000000, 0.9659258262890683122, 1.000000000000000000, 0.9659258262890683122, 1.000000000000000000, 0.9659258262890683122, 1.000000000000000000, 0.9659258262890683122, 1.000000000000000000, 0.9659258262890683122, 1.000000000000000000, 0.9659258262890683122, 1.000000000000000000, 0.9659258262890683122, 1.000000000000000000, 0.9659258262890683122, 1.000000000000000000, 0.9659258262890683122, 1.000000000000000000, 0.9659258262890683122, 1.000000000000000000, 0.9659258262890683122, 1.000000000000000000, 0.9659258262890683122, 1.000000000000000000, 0.9659258262890683122, 1.000000000000000000, 0.9659258262890683122, 1.000000000000000000, 0.9659258262890683122, 1.000000000000000000, 0.9659258262890683122, 1.000000000000000000, 0.9659258262890683122, 1.000000000000000000, 0.9659258262890683122, 1.000000000000000000, 0.9659258262890683122, 1.000000000000000000, 0.9659258262890683122, 1.000000000000000000, 0.9659258262890683122, 1.000000000000000000, 0.9659258262890683122, 1.000000000000000000, 0.9659258262890683122, 1.000000000000000000, 0.9659258262890683122, 1.000000000000000000, 0.9659258262890683122, 1.000000000000000000, 0.9659258262890683122, 1.000000000000000000, 0.9659258262890683122, 1.000000000000000000, 0.9659258262890683122, 1.000000000000000000, 0.9659258262890683122, 1.000000000000000000, 0.9659258262890683122, 1.000000000000000000, 0.9659258262890683122, 1.000000000000000000, 0.9659258262890683122, 1.000000000000000000, 0.9659258262890683122, 1.000000000000000000, 0.9659258262890683122, 1.000000000000000000, 0.9659258262890683122, 1.000000000000000000, 0.9659258262890683122, 1.000000000000000000, 0.9659258262890683122, 1.000000000000000000, 0.9659258262890683122, 1.000000000000000000, 0.9659258262890683122, 1.000000000000000000, 0.9659258262890683122, 1.000000000000000000, 0.9659258262890683122, 1.000000000000000000, 0.9659258262890683122, 1.000000000000000000, 0.9659258262890683122, 1.000000000000000000, 0.9659258262890683122, 1.000000000000000000, 0.9659258262890683122, 1.000000000000000000, 0.9659258262890683122, 1.000000000000000000, 0.9659258262890683122, 1.000000000000000000, 0.9659258262890683122, 1.000000000000000000, 0.9659258262890683122, 1.000000000000000000, 0.9659258262890683122, 1.000000000000000000, 0.9659258262890683122, 1.000000000000000000, 0.9659258262890683122, 1.000000000000000000, 0.9659258262890683122, 1.000000000000000000, 0.9659258262890683122, 1.000000000000000000, 0.9659258262890683122, 1.000000000000000000, 0.9659258262890683122, 1.000000000000000000, 0.9659258262890683122, 1.000000000000000000, 0.9659258262890683122, 1.000000000000000000, 0.9659258262890683122, 1.000000000000000000, 0.9659258262890683122, 1.000000000000000000, 0.9659258262890683122, 1.000000000000000000, 0.9659258262890683122, 1.000000000000000000, 0.9659258262890683122, 1.000000000000000000, 0.9659258262890683122, 1.000000000000000000, 0.9659258262890683122, 1.000000000000000000, 0.9659258262890683122, 1.000000000000000000, 0.9659258262890683122, 1.000000000000000000, 0.9659258262890683122, 1.000000000000000000, 0.9659258262890683122, 1.000000000000000000, 0.9659258262890683122, 1.000000000000000000, 0.9659258262890683122, 1.000000000000000000, 0.9659258262890683122, 1.000000000000000000, 0.9659258262890683122, 1.000000000000000000, 0.9659258262890683122, 1.000000000000000000, 0.9659258262890683122, 1.000000000000000000, 0.9659258262890683122, 1.000000000000000000, 0.9659258262890683122, 1.000000000000000000, 0.9659258262890683122, 1.000000000000000000, 0.9659258262890683122, 1.000000000000000000, 0.9659258262890683122, 1.000000000000000000, 0.9659258262890683122, 1.000000000000000000, 0.9659258262890683122, 1.000000000000000000, 0.9659258262890683122, 1.000000000000000000, 0.9659258262890683122, 1.000000000000000000, 0.9659258262890683122, 1.000000000000000000, 0.9659258262890683122, 1.000000000000000000, 0.9659258262890683122, 1.000000000000000000, 0.9659258262890683122, 1.000000000000000000, 0.9659258262890683122, 1.000000000000000000, 0.9659258262890683122, 1.000000000000000000, 0.9659258262890683122, 1.000000000000000000),
 ( 0.3333333333333333703, 0.3219752754296894559, 0.3333333333333333703, 0.3219752754296894559, 0.3333333333333333703, 0.3219752754296894559, 0.3333333333333333703, 0.3219752754296894559, 0.3333333333333333703, 0.3219752754296894559, 0.3333333333333333703, 0.3219752754296894559, 0.3333333333333333703, 0.3219752754296894559, 0.3333333333333333703, 0.3219752754296894559, 0.3333333333333333703, 0.3219752754296894559, 0.3333333333333333703, 0.3219752754296894559, 0.3333333333333333703, 0.3219752754296894559, 0.3333333333333333703, 0.3219752754296894559, 0.3333333333333333703, 0.3219752754296894559, 0.3333333333333333703, 0.3219752754296894559, 0.3333333333333333703, 0.3219752754296894559, 0.3333333333333333703, 0.3219752754296894559, 0.3333333333333333703, 0.3219752754296894559, 0.3333333333333333703, 0.3219752754296894559, 0.3333333333333333703, 0.3219752754296894559, 0.3333333333333333703, 0.3219752754296894559, 0.3333333333333333703, 0.3219752754296894559, 0.3333333333333333703, 0.3219752754296894559, 0.3333333333333333703, 0.3219752754296894559, 0.3333333333333333703, 0.3219752754296894559, 0.3333333333333333703, 0.3219752754296894559, 0.3333333333333333703, 0.3219752754296894559, 0.3333333333333333703, 0.3219752754296894559, 0.3333333333333333703, 0.3219752754296894559, 0.3333333333333333703, 0.3219752754296894559, 0.3333333333333333703, 0.3219752754296894559, 0.3333333333333333703, 0.3219752754296894559, 0.3333333333333333703, 0.3219752754296894559, 0.3333333333333333703, 0.3219752754296894559, 0.3333333333333333703, 0.3219752754296894559, 0.3333333333333333703, 0.3219752754296894559, 0.3333333333333333703, 0.3219752754296894559, 0.3333333333333333703, 0.3219752754296894559, 0.3333333333333333703, 0.3219752754296894559, 0.3333333333333333703, 0.3219752754296894559, 0.3333333333333333703, 0.3219752754296894559, 0.3333333333333333703, 0.3219752754296894559, 0.3333333333333333703, 0.3219752754296894559, 0.3333333333333333703, 0.3219752754296894559, 0.3333333333333333703, 0.3219752754296894559, 0.3333333333333333703, 0.3219752754296894559, 0.3333333333333333703, 0.3219752754296894559, 0.3333333333333333703, 0.3219752754296894559, 0.3333333333333333703, 0.3219752754296894559, 0.3333333333333333703, 0.3219752754296894559, 0.3333333333333333703, 0.3219752754296894559, 0.3333333333333333703, 0.3219752754296894559, 0.3333333333333333703, 0.3219752754296894559, 0.3333333333333333703, 0.3219752754296894559, 0.3333333333333333703, 0.3219752754296894559, 0.3333333333333333703, 0.3219752754296894559, 0.3333333333333333703, 0.3219752754296894559, 0.3333333333333333703, 0.3219752754296894559, 0.3333333333333333703, 0.3219752754296894559, 0.3333333333333333703, 0.3219752754296894559, 0.3333333333333333703, 0.3219752754296894559, 0.3333333333333333703, 0.3219752754296894559, 0.3333333333333333703, 0.3219752754296894559, 0.3333333333333333703, 0.3219752754296894559, 0.3333333333333333703, 0.3219752754296894559, 0.3333333333333333703, 0.3219752754296894559, 0.3333333333333333703, 0.3219752754296894559, 0.3333333333333333703, 0.3219752754296894559, 0.3333333333333333703, 0.3219752754296894559, 0.3333333333333333703, 0.3219752754296894559, 0.3333333333333333703, 0.3219752754296894559, 0.3333333333333333703, 0.3219752754296894559, 0.3333333333333333703, 0.3219752754296894559, 0.3333333333333333703, 0.3219752754296894559, 0.3333333333333333703, 0.3219752754296894559, 0.3333333333333333703, 0.3219752754296894559, 0.3333333333333333703, 0.3219752754296894559, 0.3333333333333333703, 0.3219752754296894559, 0.3333333333333333703, 0.3219752754296894559, 0.3333333333333333703, 0.3219752754296894559, 0.3333333333333333703, 0.3219752754296894559, 0.3333333333333333703, 0.3219752754296894559, 0.3333333333333333703, 0.3219752754296894559, 0.3333333333333333703, 0.3219752754296894559, 0.3333333333333333703, 0.3219752754296894559, 0.3333333333333333703, 0.3219752754296894559, 0.3333333333333333703, 0.3219752754296894559, 0.3333333333333333703, 0.3219752754296894559, 0.3333333333333333703, 0.3219752754296894559, 0.3333333333333333703, 0.3219752754296894559, 0.3333333333333333703, 0.3219752754296894559, 0.3333333333333333703, 0.3219752754296894559, 0.3333333333333333703, 0.3219752754296894559, 0.3333333333333333703, 0.3219752754296894559, 0.3333333333333333703, 0.3219752754296894559, 0.3333333333333333703, 0.3219752754296894559, 0.3333333333333333703, 0.3219752754296894559, 0.3333333333333333703, 0.3219752754296894559, 0.3333333333333333703, 0.3219752754296894559, 0.3333333333333333703, 0.3219752754296894559, 0.3333333333333333703, 0.3219752754296894559, 0.3333333333333333703, 0.3219752754296894559, 0.3333333333333333703, 0.3219752754296894559, 0.3333333333333333703, 0.3219752754296894559, 0.3333333333333333703, 0.3219752754296894559, 0.3333333333333333703, 0.3219752754296894559, 0.3333333333333333703, 0.3219752754296894559, 0.3333333333333333703, 0.3219752754296894559, 0.3333333333333333703, 0.3219752754296894559, 0.3333333333333333703, 0.3219752754296894559, 0.3333333333333333703, 0.3219752754296894559, 0.3333333333333333703, 0.3219752754296894559, 0.3333333333333333703, 0.3219752754296894559, 0.3333333333333333703, 0.3219752754296894559, 0.3333333333333333703, 0.3219752754296894559, 0.3333333333333333703, 0.3219752754296894559, 0.3333333333333333703, 0.3219752754296894559, 0.3333333333333333703, 0.3219752754296894559, 0.3333333333333333703, 0.3219752754296894559, 0.3333333333333333703, 0.3219752754296894559, 0.3333333333333333703, 0.3219752754296894559, 0.3333333333333333703, 0.3219752754296894559, 0.3333333333333333703, 0.3219752754296894559, 0.3333333333333333703, 0.3219752754296894559, 0.3333333333333333703, 0.3219752754296894559, 0.3333333333333333703, 0.3219752754296894559, 0.3333333333333333703, 0.3219752754296894559, 0.3333333333333333703, 0.3219752754296894559, 0.3333333333333333703, 0.3219752754296894559, 0.3333333333333333703, 0.3219752754296894559, 0.3333333333333333703, 0.3219752754296894559, 0.3333333333333333703, 0.3219752754296894559, 0.3333333333333333703, 0.3219752754296894559, 0.3333333333333333703, 0.3219752754296894559, 0.3333333333333333703, 0.3219752754296894559, 0.3333333333333333703, 0.3219752754296894559, 0.3333333333333333703, 0.3219752754296894559, 0.3333333333333333703, 0.3219752754296894559, 0.3333333333333333703, 0.3219752754296894559, 0.3333333333333333703, 0.3219752754296894559, 0.3333333333333333703, 0.3219752754296894559, 0.3333333333333333703, 0.3219752754296894559, 0.3333333333333333703, 0.3219752754296894559, 0.3333333333333333703, 0.3219752754296894559, 0.3333333333333333703, 0.3219752754296894559, 0.3333333333333333703, 0.3219752754296894559, 0.3333333333333333703, 0.3219752754296894559, 0.3333333333333333703, 0.3219752754296894559, 0.3333333333333333703, 0.3219752754296894559, 0.3333333333333333703, 0.3219752754296894559, 0.3333333333333333703, 0.3219752754296894559, 0.3333333333333333703, 0.3219752754296894559, 0.3333333333333333703, 0.3219752754296894559, 0.3333333333333333703, 0.3219752754296894559, 0.3333333333333333703, 0.3219752754296894559, 0.3333333333333333703, 0.3219752754296894559, 0.3333333333333333703, 0.3219752754296894559, 0.3333333333333333703, 0.3219752754296894559, 0.3333333333333333703, 0.3219752754296894559, 0.3333333333333333703, 0.3219752754296894559, 0.3333333333333333703, 0.3219752754296894559, 0.3333333333333333703, 0.3219752754296894559, 0.3333333333333333703, 0.3219752754296894559, 0.3333333333333333703, 0.3219752754296894559, 0.3333333333333333703, 0.3219752754296894559, 0.3333333333333333703, 0.3219752754296894559, 0.3333333333333333703, 0.3219752754296894559, 0.3333333333333333703, 0.3219752754296894559, 0.3333333333333333703, 0.3219752754296894559, 0.3333333333333333703, 0.3219752754296894559, 0.3333333333333333703, 0.3219752754296894559, 0.3333333333333333703, 0.3219752754296894559, 0.3333333333333333703, 0.3219752754296894559, 0.3333333333333333703, 0.3219752754296894559, 0.3333333333333333703, 0.3219752754296894559, 0.3333333333333333703, 0.3219752754296894559, 0.3333333333333333703, 0.3219752754296894559, 0.3333333333333333703, 0.3219752754296894559, 0.3333333333333333703, 0.3219752754296894559, 0.3333333333333333703, 0.3219752754296894559, 0.3333333333333333703, 0.3219752754296894559, 0.3333333333333333703, 0.3219752754296894559, 0.3333333333333333703, 0.3219752754296894559, 0.3333333333333333703, 0.3219752754296894559, 0.3333333333333333703, 0.3219752754296894559, 0.3333333333333333703, 0.3219752754296894559, 0.3333333333333333703, 0.3219752754296894559, 0.3333333333333333703, 0.3219752754296894559, 0.3333333333333333703, 0.3219752754296894559, 0.3333333333333333703, 0.3219752754296894559, 0.3333333333333333703, 0.3219752754296894559, 0.3333333333333333703, 0.3219752754296894559, 0.3333333333333333703, 0.3219752754296894559, 0.3333333333333333703, 0.3219752754296894559, 0.3333333333333333703, 0.3219752754296894559, 0.3333333333333333703, 0.3219752754296894559, 0.3333333333333333703, 0.3219752754296894559, 0.3333333333333333703, 0.3219752754296894559, 0.3333333333333333703, 0.3219752754296894559, 0.3333333333333333703, 0.3219752754296894559, 0.3333333333333333703, 0.3219752754296894559, 0.3333333333333333703, 0.3219752754296894559, 0.3333333333333333703, 0.3219752754296894559, 0.3333333333333333703, 0.3219752754296894559, 0.3333333333333333703, 0.3219752754296894559, 0.3333333333333333703, 0.3219752754296894559, 0.3333333333333333703, 0.3219752754296894559, 0.3333333333333333703, 0.3219752754296894559, 0.3333333333333333703, 0.3219752754296894559, 0.3333333333333333703, 0.3219752754296894559, 0.3333333333333333703, 0.3219752754296894559, 0.3333333333333333703, 0.3219752754296894559, 0.3333333333333333703, 0.3219752754296894559, 0.3333333333333333703, 0.3219752754296894559, 0.3333333333333333703, 0.3219752754296894559, 0.3333333333333333703, 0.3219752754296894559, 0.3333333333333333703, 0.3219752754296894559, 0.3333333333333333703, 0.3219752754296894559, 0.3333333333333333703, 0.3219752754296894559, 0.3333333333333333703, 0.3219752754296894559, 0.3333333333333333703, 0.3219752754296894559, 0.3333333333333333703, 0.3219752754296894559, 0.3333333333333333703, 0.3219752754296894559, 0.3333333333333333703, 0.3219752754296894559, 0.3333333333333333703, 0.3219752754296894559, 0.3333333333333333703, 0.3219752754296894559, 0.3333333333333333703, 0.3219752754296894559, 0.3333333333333333703, 0.3219752754296894559, 0.3333333333333333703, 0.3219752754296894559, 0.3333333333333333703),
 ( 0.3333333333333333703, 0.3219752754296894559, 0.3333333333333333703, 0.3219752754296894559, 0.3333333333333333703, 0.3219752754296894559, 0.3333333333333333703, 0.3219752754296894559, 0.3333333333333333703, 0.3219752754296894559, 0.3333333333333333703, 0.3219752754296894559, 0.3333333333333333703, 0.3219752754296894559, 0.3333333333333333703, 0.3219752754296894559, 0.3333333333333333703, 0.3219752754296894559, 0.3333333333333333703, 0.3219752754296894559, 0.3333333333333333703, 0.3219752754296894559, 0.3333333333333333703, 0.3219752754296894559, 0.3333333333333333703, 0.3219752754296894559, 0.3333333333333333703, 0.3219752754296894559, 0.3333333333333333703, 0.3219752754296894559, 0.3333333333333333703, 0.3219752754296894559, 0.3333333333333333703, 0.3219752754296894559, 0.3333333333333333703, 0.3219752754296894559, 0.3333333333333333703, 0.3219752754296894559, 0.3333333333333333703, 0.3219752754296894559, 0.3333333333333333703, 0.3219752754296894559, 0.3333333333333333703, 0.3219752754296894559, 0.3333333333333333703, 0.3219752754296894559, 0.3333333333333333703, 0.3219752754296894559, 0.3333333333333333703, 0.3219752754296894559, 0.3333333333333333703, 0.3219752754296894559, 0.3333333333333333703, 0.3219752754296894559, 0.3333333333333333703, 0.3219752754296894559, 0.3333333333333333703, 0.3219752754296894559, 0.3333333333333333703, 0.3219752754296894559, 0.3333333333333333703, 0.3219752754296894559, 0.3333333333333333703, 0.3219752754296894559, 0.3333333333333333703, 0.3219752754296894559, 0.3333333333333333703, 0.3219752754296894559, 0.3333333333333333703, 0.3219752754296894559, 0.3333333333333333703, 0.3219752754296894559, 0.3333333333333333703, 0.3219752754296894559, 0.3333333333333333703, 0.3219752754296894559, 0.3333333333333333703, 0.3219752754296894559, 0.3333333333333333703, 0.3219752754296894559, 0.3333333333333333703, 0.3219752754296894559, 0.3333333333333333703, 0.3219752754296894559, 0.3333333333333333703, 0.3219752754296894559, 0.3333333333333333703, 0.3219752754296894559, 0.3333333333333333703, 0.3219752754296894559, 0.3333333333333333703, 0.3219752754296894559, 0.3333333333333333703, 0.3219752754296894559, 0.3333333333333333703, 0.3219752754296894559, 0.3333333333333333703, 0.3219752754296894559, 0.3333333333333333703, 0.3219752754296894559, 0.3333333333333333703, 0.3219752754296894559, 0.3333333333333333703, 0.3219752754296894559, 0.3333333333333333703, 0.3219752754296894559, 0.3333333333333333703, 0.3219752754296894559, 0.3333333333333333703, 0.3219752754296894559, 0.3333333333333333703, 0.3219752754296894559, 0.3333333333333333703, 0.3219752754296894559, 0.3333333333333333703, 0.3219752754296894559, 0.3333333333333333703, 0.3219752754296894559, 0.3333333333333333703, 0.3219752754296894559, 0.3333333333333333703, 0.3219752754296894559, 0.3333333333333333703, 0.3219752754296894559, 0.3333333333333333703, 0.3219752754296894559, 0.3333333333333333703, 0.3219752754296894559, 0.3333333333333333703, 0.3219752754296894559, 0.3333333333333333703, 0.3219752754296894559, 0.3333333333333333703, 0.3219752754296894559, 0.3333333333333333703, 0.3219752754296894559, 0.3333333333333333703, 0.3219752754296894559, 0.3333333333333333703, 0.3219752754296894559, 0.3333333333333333703, 0.3219752754296894559, 0.3333333333333333703, 0.3219752754296894559, 0.3333333333333333703, 0.3219752754296894559, 0.3333333333333333703, 0.3219752754296894559, 0.3333333333333333703, 0.3219752754296894559, 0.3333333333333333703, 0.3219752754296894559, 0.3333333333333333703, 0.3219752754296894559, 0.3333333333333333703, 0.3219752754296894559, 0.3333333333333333703, 0.3219752754296894559, 0.3333333333333333703, 0.3219752754296894559, 0.3333333333333333703, 0.3219752754296894559, 0.3333333333333333703, 0.3219752754296894559, 0.3333333333333333703, 0.3219752754296894559, 0.3333333333333333703, 0.3219752754296894559, 0.3333333333333333703, 0.3219752754296894559, 0.3333333333333333703, 0.3219752754296894559, 0.3333333333333333703, 0.3219752754296894559, 0.3333333333333333703, 0.3219752754296894559, 0.3333333333333333703, 0.3219752754296894559, 0.3333333333333333703, 0.3219752754296894559, 0.3333333333333333703, 0.3219752754296894559, 0.3333333333333333703, 0.3219752754296894559, 0.3333333333333333703, 0.3219752754296894559, 0.3333333333333333703, 0.3219752754296894559, 0.3333333333333333703, 0.3219752754296894559, 0.3333333333333333703, 0.3219752754296894559, 0.3333333333333333703, 0.3219752754296894559, 0.3333333333333333703, 0.3219752754296894559, 0.3333333333333333703, 0.3219752754296894559, 0.3333333333333333703, 0.3219752754296894559, 0.3333333333333333703, 0.3219752754296894559, 0.3333333333333333703, 0.3219752754296894559, 0.3333333333333333703, 0.3219752754296894559, 0.3333333333333333703, 0.3219752754296894559, 0.3333333333333333703, 0.3219752754296894559, 0.3333333333333333703, 0.3219752754296894559, 0.3333333333333333703, 0.3219752754296894559, 0.3333333333333333703, 0.3219752754296894559, 0.3333333333333333703, 0.3219752754296894559, 0.3333333333333333703, 0.3219752754296894559, 0.3333333333333333703, 0.3219752754296894559, 0.3333333333333333703, 0.3219752754296894559, 0.3333333333333333703, 0.3219752754296894559, 0.3333333333333333703, 0.3219752754296894559, 0.3333333333333333703, 0.3219752754296894559, 0.3333333333333333703, 0.3219752754296894559, 0.3333333333333333703, 0.3219752754296894559, 0.3333333333333333703, 0.3219752754296894559, 0.3333333333333333703, 0.3219752754296894559, 0.3333333333333333703, 0.3219752754296894559, 0.3333333333333333703, 0.3219752754296894559, 0.3333333333333333703, 0.3219752754296894559, 0.3333333333333333703, 0.3219752754296894559, 0.3333333333333333703, 0.3219752754296894559, 0.3333333333333333703, 0.3219752754296894559, 0.3333333333333333703, 0.3219752754296894559, 0.3333333333333333703, 0.3219752754296894559, 0.3333333333333333703, 0.3219752754296894559, 0.3333333333333333703, 0.3219752754296894559, 0.3333333333333333703, 0.3219752754296894559, 0.3333333333333333703, 0.3219752754296894559, 0.3333333333333333703, 0.3219752754296894559, 0.3333333333333333703, 0.3219752754296894559, 0.3333333333333333703, 0.3219752754296894559, 0.3333333333333333703, 0.3219752754296894559, 0.3333333333333333703, 0.3219752754296894559, 0.3333333333333333703, 0.3219752754296894559, 0.3333333333333333703, 0.3219752754296894559, 0.3333333333333333703, 0.3219752754296894559, 0.3333333333333333703, 0.3219752754296894559, 0.3333333333333333703, 0.3219752754296894559, 0.3333333333333333703, 0.3219752754296894559, 0.3333333333333333703, 0.3219752754296894559, 0.3333333333333333703, 0.3219752754296894559, 0.3333333333333333703, 0.3219752754296894559, 0.3333333333333333703, 0.3219752754296894559, 0.3333333333333333703, 0.3219752754296894559, 0.3333333333333333703, 0.3219752754296894559, 0.3333333333333333703, 0.3219752754296894559, 0.3333333333333333703, 0.3219752754296894559, 0.3333333333333333703, 0.3219752754296894559, 0.3333333333333333703, 0.3219752754296894559, 0.3333333333333333703, 0.3219752754296894559, 0.3333333333333333703, 0.3219752754296894559, 0.3333333333333333703, 0.3219752754296894559, 0.3333333333333333703, 0.3219752754296894559, 0.3333333333333333703, 0.3219752754296894559, 0.3333333333333333703, 0.3219752754296894559, 0.3333333333333333703, 0.3219752754296894559, 0.3333333333333333703, 0.3219752754296894559, 0.3333333333333333703, 0.3219752754296894559, 0.3333333333333333703, 0.3219752754296894559, 0.3333333333333333703, 0.3219752754296894559, 0.3333333333333333703, 0.3219752754296894559, 0.3333333333333333703, 0.3219752754296894559, 0.3333333333333333703, 0.3219752754296894559, 0.3333333333333333703, 0.3219752754296894559, 0.3333333333333333703, 0.3219752754296894559, 0.3333333333333333703, 0.3219752754296894559, 0.3333333333333333703, 0.3219752754296894559, 0.3333333333333333703, 0.3219752754296894559, 0.3333333333333333703, 0.3219752754296894559, 0.3333333333333333703, 0.3219752754296894559, 0.3333333333333333703, 0.3219752754296894559, 0.3333333333333333703, 0.3219752754296894559, 0.3333333333333333703, 0.3219752754296894559, 0.3333333333333333703, 0.3219752754296894559, 0.3333333333333333703, 0.3219752754296894559, 0.3333333333333333703, 0.3219752754296894559, 0.3333333333333333703, 0.3219752754296894559, 0.3333333333333333703, 0.3219752754296894559, 0.3333333333333333703, 0.3219752754296894559, 0.3333333333333333703, 0.3219752754296894559, 0.3333333333333333703, 0.3219752754296894559, 0.3333333333333333703, 0.3219752754296894559, 0.3333333333333333703, 0.3219752754296894559, 0.3333333333333333703, 0.3219752754296894559, 0.3333333333333333703, 0.3219752754296894559, 0.3333333333333333703, 0.3219752754296894559, 0.3333333333333333703, 0.3219752754296894559, 0.3333333333333333703, 0.3219752754296894559, 0.3333333333333333703, 0.3219752754296894559, 0.3333333333333333703, 0.3219752754296894559, 0.3333333333333333703, 0.3219752754296894559, 0.3333333333333333703, 0.3219752754296894559, 0.3333333333333333703, 0.3219752754296894559, 0.3333333333333333703, 0.3219752754296894559, 0.3333333333333333703, 0.3219752754296894559, 0.3333333333333333703, 0.3219752754296894559, 0.3333333333333333703, 0.3219752754296894559, 0.3333333333333333703, 0.3219752754296894559, 0.3333333333333333703, 0.3219752754296894559, 0.3333333333333333703, 0.3219752754296894559, 0.3333333333333333703, 0.3219752754296894559, 0.3333333333333333703, 0.3219752754296894559, 0.3333333333333333703, 0.3219752754296894559, 0.3333333333333333703, 0.3219752754296894559, 0.3333333333333333703, 0.3219752754296894559, 0.3333333333333333703, 0.3219752754296894559, 0.3333333333333333703, 0.3219752754296894559, 0.3333333333333333703, 0.3219752754296894559, 0.3333333333333333703, 0.3219752754296894559, 0.3333333333333333703, 0.3219752754296894559, 0.3333333333333333703, 0.3219752754296894559, 0.3333333333333333703, 0.3219752754296894559, 0.3333333333333333703, 0.3219752754296894559, 0.3333333333333333703, 0.3219752754296894559, 0.3333333333333333703, 0.3219752754296894559, 0.3333333333333333703, 0.3219752754296894559, 0.3333333333333333703, 0.3219752754296894559, 0.3333333333333333703, 0.3219752754296894559, 0.3333333333333333703, 0.3219752754296894559, 0.3333333333333333703, 0.3219752754296894559, 0.3333333333333333703, 0.3219752754296894559, 0.3333333333333333703, 0.3219752754296894559, 0.3333333333333333703, 0.3219752754296894559, 0.3333333333333333703, 0.3219752754296894559, 0.3333333333333333703, 0.3219752754296894559, 0.3333333333333333703),
 ( 1.000000000000000000, 0.9659258262890683122, 1.000000000000000000, 0.9659258262890683122, 1.000000000000000000, 0.9659258262890683122, 1.000000000000000000, 0.9659258262890683122, 1.000000000000000000, 0.9659258262890683122, 1.000000000000000000, 0.9659258262890683122, 1.000000000000000000, 0.9659258262890683122, 1.000000000000000000, 0.9659258262890683122, 1.000000000000000000, 0.9659258262890683122, 1.000000000000000000, 0.9659258262890683122, 1.000000000000000000, 0.9659258262890683122, 1.000000000000000000, 0.9659258262890683122, 1.000000000000000000, 0.9659258262890683122, 1.000000000000000000, 0.9659258262890683122, 1.000000000000000000, 0.9659258262890683122, 1.000000000000000000, 0.9659258262890683122, 1.000000000000000000, 0.9659258262890683122, 1.000000000000000000, 0.9659258262890683122, 1.000000000000000000, 0.9659258262890683122, 1.000000000000000000, 0.9659258262890683122, 1.000000000000000000, 0.9659258262890683122, 1.000000000000000000, 0.9659258262890683122, 1.000000000000000000, 0.9659258262890683122, 1.000000000000000000, 0.9659258262890683122, 1.000000000000000000, 0.9659258262890683122, 1.000000000000000000, 0.9659258262890683122, 1.000000000000000000, 0.9659258262890683122, 1.000000000000000000, 0.9659258262890683122, 1.000000000000000000, 0.9659258262890683122, 1.000000000000000000, 0.9659258262890683122, 1.000000000000000000, 0.9659258262890683122, 1.000000000000000000, 0.9659258262890683122, 1.000000000000000000, 0.9659258262890683122, 1.000000000000000000, 0.9659258262890683122, 1.000000000000000000, 0.9659258262890683122, 1.000000000000000000, 0.9659258262890683122, 1.000000000000000000, 0.9659258262890683122, 1.000000000000000000, 0.9659258262890683122, 1.000000000000000000, 0.9659258262890683122, 1.000000000000000000, 0.9659258262890683122, 1.000000000000000000, 0.9659258262890683122, 1.000000000000000000, 0.9659258262890683122, 1.000000000000000000, 0.9659258262890683122, 1.000000000000000000, 0.9659258262890683122, 1.000000000000000000, 0.9659258262890683122, 1.000000000000000000, 0.9659258262890683122, 1.000000000000000000, 0.9659258262890683122, 1.000000000000000000, 0.9659258262890683122, 1.000000000000000000, 0.9659258262890683122, 1.000000000000000000, 0.9659258262890683122, 1.000000000000000000, 0.9659258262890683122, 1.000000000000000000, 0.9659258262890683122, 1.000000000000000000, 0.9659258262890683122, 1.000000000000000000, 0.9659258262890683122, 1.000000000000000000, 0.9659258262890683122, 1.000000000000000000, 0.9659258262890683122, 1.000000000000000000, 0.9659258262890683122, 1.000000000000000000, 0.9659258262890683122, 1.000000000000000000, 0.9659258262890683122, 1.000000000000000000, 0.9659258262890683122, 1.000000000000000000, 0.9659258262890683122, 1.000000000000000000, 0.9659258262890683122, 1.000000000000000000, 0.9659258262890683122, 1.000000000000000000, 0.9659258262890683122, 1.000000000000000000, 0.9659258262890683122, 1.000000000000000000, 0.9659258262890683122, 1.000000000000000000, 0.9659258262890683122, 1.000000000000000000, 0.9659258262890683122, 1.000000000000000000, 0.9659258262890683122, 1.000000000000000000, 0.9659258262890683122, 1.000000000000000000, 0.9659258262890683122, 1.000000000000000000, 0.9659258262890683122, 1.000000000000000000, 0.9659258262890683122, 1.000000000000000000, 0.9659258262890683122, 1.000000000000000000, 0.9659258262890683122, 1.000000000000000000, 0.9659258262890683122, 1.000000000000000000, 0.9659258262890683122, 1.000000000000000000, 0.9659258262890683122, 1.000000000000000000, 0.9659258262890683122, 1.000000000000000000, 0.9659258262890683122, 1.000000000000000000, 0.9659258262890683122, 1.000000000000000000, 0.9659258262890683122, 1.000000000000000000, 0.9659258262890683122, 1.000000000000000000, 0.9659258262890683122, 1.000000000000000000, 0.9659258262890683122, 1.000000000000000000, 0.9659258262890683122, 1.000000000000000000, 0.9659258262890683122, 1.000000000000000000, 0.9659258262890683122, 1.000000000000000000, 0.9659258262890683122, 1.000000000000000000, 0.9659258262890683122, 1.000000000000000000, 0.9659258262890683122, 1.000000000000000000, 0.9659258262890683122, 1.000000000000000000, 0.9659258262890683122, 1.000000000000000000, 0.9659258262890683122, 1.000000000000000000, 0.9659258262890683122, 1.000000000000000000, 0.9659258262890683122, 1.000000000000000000, 0.9659258262890683122, 1.000000000000000000, 0.9659258262890683122, 1.000000000000000000, 0.9659258262890683122, 1.000000000000000000, 0.9659258262890683122, 1.000000000000000000, 0.9659258262890683122, 1.000000000000000000, 0.9659258262890683122, 1.000000000000000000, 0.9659258262890683122, 1.000000000000000000, 0.9659258262890683122, 1.000000000000000000, 0.9659258262890683122, 1.000000000000000000, 0.9659258262890683122, 1.000000000000000000, 0.9659258262890683122, 1.000000000000000000, 0.9659258262890683122, 1.000000000000000000, 0.9659258262890683122, 1.000000000000000000, 0.9659258262890683122, 1.000000000000000000, 0.9659258262890683122, 1.000000000000000000, 0.9659258262890683122, 1.000000000000000000, 0.9659258262890683122, 1.000000000000000000, 0.9659258262890683122, 1.000000000000000000, 0.9659258262890683122, 1.000000000000000000, 0.9659258262890683122, 1.000000000000000000, 0.9659258262890683122, 1.000000000000000000, 0.9659258262890683122, 1.000000000000000000, 0.9659258262890683122, 1.000000000000000000, 0.9659258262890683122, 1.000000000000000000, 0.9659258262890683122, 1.000000000000000000, 0.9659258262890683122, 1.000000000000000000, 0.9659258262890683122, 1.000000000000000000, 0.9659258262890683122, 1.000000000000000000, 0.9659258262890683122, 1.000000000000000000, 0.9659258262890683122, 1.000000000000000000, 0.9659258262890683122, 1.000000000000000000, 0.9659258262890683122, 1.000000000000000000, 0.9659258262890683122, 1.000000000000000000, 0.9659258262890683122, 1.000000000000000000, 0.9659258262890683122, 1.000000000000000000, 0.9659258262890683122, 1.000000000000000000, 0.9659258262890683122, 1.000000000000000000, 0.9659258262890683122, 1.000000000000000000, 0.9659258262890683122, 1.000000000000000000, 0.9659258262890683122, 1.000000000000000000, 0.9659258262890683122, 1.000000000000000000, 0.9659258262890683122, 1.000000000000000000, 0.9659258262890683122, 1.000000000000000000, 0.9659258262890683122, 1.000000000000000000, 0.9659258262890683122, 1.000000000000000000, 0.9659258262890683122, 1.000000000000000000, 0.9659258262890683122, 1.000000000000000000, 0.9659258262890683122, 1.000000000000000000, 0.9659258262890683122, 1.000000000000000000, 0.9659258262890683122, 1.000000000000000000, 0.9659258262890683122, 1.000000000000000000, 0.9659258262890683122, 1.000000000000000000, 0.9659258262890683122, 1.000000000000000000, 0.9659258262890683122, 1.000000000000000000, 0.9659258262890683122, 1.000000000000000000, 0.9659258262890683122, 1.000000000000000000, 0.9659258262890683122, 1.000000000000000000, 0.9659258262890683122, 1.000000000000000000, 0.9659258262890683122, 1.000000000000000000, 0.9659258262890683122, 1.000000000000000000, 0.9659258262890683122, 1.000000000000000000, 0.9659258262890683122, 1.000000000000000000, 0.9659258262890683122, 1.000000000000000000, 0.9659258262890683122, 1.000000000000000000, 0.9659258262890683122, 1.000000000000000000, 0.9659258262890683122, 1.000000000000000000, 0.9659258262890683122, 1.000000000000000000, 0.9659258262890683122, 1.000000000000000000, 0.9659258262890683122, 1.000000000000000000, 0.9659258262890683122, 1.000000000000000000, 0.9659258262890683122, 1.000000000000000000, 0.9659258262890683122, 1.000000000000000000, 0.9659258262890683122, 1.000000000000000000, 0.9659258262890683122, 1.000000000000000000, 0.9659258262890683122, 1.000000000000000000, 0.9659258262890683122, 1.000000000000000000, 0.9659258262890683122, 1.000000000000000000, 0.9659258262890683122, 1.000000000000000000, 0.9659258262890683122, 1.000000000000000000, 0.9659258262890683122, 1.000000000000000000, 0.9659258262890683122, 1.000000000000000000, 0.9659258262890683122, 1.000000000000000000, 0.9659258262890683122, 1.000000000000000000, 0.9659258262890683122, 1.000000000000000000, 0.9659258262890683122, 1.000000000000000000, 0.9659258262890683122, 1.000000000000000000, 0.9659258262890683122, 1.000000000000000000, 0.9659258262890683122, 1.000000000000000000, 0.9659258262890683122, 1.000000000000000000, 0.9659258262890683122, 1.000000000000000000, 0.9659258262890683122, 1.000000000000000000, 0.9659258262890683122, 1.000000000000000000, 0.9659258262890683122, 1.000000000000000000, 0.9659258262890683122, 1.000000000000000000, 0.9659258262890683122, 1.000000000000000000, 0.9659258262890683122, 1.000000000000000000, 0.9659258262890683122, 1.000000000000000000, 0.9659258262890683122, 1.000000000000000000, 0.9659258262890683122, 1.000000000000000000, 0.9659258262890683122, 1.000000000000000000, 0.9659258262890683122, 1.000000000000000000, 0.9659258262890683122, 1.000000000000000000, 0.9659258262890683122, 1.000000000000000000, 0.9659258262890683122, 1.000000000000000000, 0.9659258262890683122, 1.000000000000000000, 0.9659258262890683122, 1.000000000000000000, 0.9659258262890683122, 1.000000000000000000, 0.9659258262890683122, 1.000000000000000000, 0.9659258262890683122, 1.000000000000000000, 0.9659258262890683122, 1.000000000000000000, 0.9659258262890683122, 1.000000000000000000, 0.9659258262890683122, 1.000000000000000000, 0.9659258262890683122, 1.000000000000000000, 0.9659258262890683122, 1.000000000000000000, 0.9659258262890683122, 1.000000000000000000, 0.9659258262890683122, 1.000000000000000000, 0.9659258262890683122, 1.000000000000000000, 0.9659258262890683122, 1.000000000000000000, 0.9659258262890683122, 1.000000000000000000, 0.9659258262890683122, 1.000000000000000000, 0.9659258262890683122, 1.000000000000000000, 0.9659258262890683122, 1.000000000000000000, 0.9659258262890683122, 1.000000000000000000, 0.9659258262890683122, 1.000000000000000000, 0.9659258262890683122, 1.000000000000000000, 0.9659258262890683122, 1.000000000000000000, 0.9659258262890683122, 1.000000000000000000, 0.9659258262890683122, 1.000000000000000000, 0.9659258262890683122, 1.000000000000000000, 0.9659258262890683122, 1.000000000000000000, 0.9659258262890683122, 1.000000000000000000, 0.9659258262890683122, 1.000000000000000000),
 ( 0.3333333333333333703, 0.3219752754296894559, 0.3333333333333333703, 0.3219752754296894559, 0.3333333333333333703, 0.3219752754296894559, 0.3333333333333333703, 0.3219752754296894559, 0.3333333333333333703, 0.3219752754296894559, 0.3333333333333333703, 0.3219752754296894559, 0.3333333333333333703, 0.3219752754296894559, 0.3333333333333333703, 0.3219752754296894559, 0.3333333333333333703, 0.3219752754296894559, 0.3333333333333333703, 0.3219752754296894559, 0.3333333333333333703, 0.3219752754296894559, 0.3333333333333333703, 0.3219752754296894559, 0.3333333333333333703, 0.3219752754296894559, 0.3333333333333333703, 0.3219752754296894559, 0.3333333333333333703, 0.3219752754296894559, 0.3333333333333333703, 0.3219752754296894559, 0.3333333333333333703, 0.3219752754296894559, 0.3333333333333333703, 0.3219752754296894559, 0.3333333333333333703, 0.3219752754296894559, 0.3333333333333333703, 0.3219752754296894559, 0.3333333333333333703, 0.3219752754296894559, 0.3333333333333333703, 0.3219752754296894559, 0.3333333333333333703, 0.3219752754296894559, 0.3333333333333333703, 0.3219752754296894559, 0.3333333333333333703, 0.3219752754296894559, 0.3333333333333333703, 0.3219752754296894559, 0.3333333333333333703, 0.3219752754296894559, 0.3333333333333333703, 0.3219752754296894559, 0.3333333333333333703, 0.3219752754296894559, 0.3333333333333333703, 0.3219752754296894559, 0.3333333333333333703, 0.3219752754296894559, 0.3333333333333333703, 0.3219752754296894559, 0.3333333333333333703, 0.3219752754296894559, 0.3333333333333333703, 0.3219752754296894559, 0.3333333333333333703, 0.3219752754296894559, 0.3333333333333333703, 0.3219752754296894559, 0.3333333333333333703, 0.3219752754296894559, 0.3333333333333333703, 0.3219752754296894559, 0.3333333333333333703, 0.3219752754296894559, 0.3333333333333333703, 0.3219752754296894559, 0.3333333333333333703, 0.3219752754296894559, 0.3333333333333333703, 0.3219752754296894559, 0.3333333333333333703, 0.3219752754296894559, 0.3333333333333333703, 0.3219752754296894559, 0.3333333333333333703, 0.3219752754296894559, 0.3333333333333333703, 0.3219752754296894559, 0.3333333333333333703, 0.3219752754296894559, 0.3333333333333333703, 0.3219752754296894559, 0.3333333333333333703, 0.3219752754296894559, 0.3333333333333333703, 0.3219752754296894559, 0.3333333333333333703, 0.3219752754296894559, 0.3333333333333333703, 0.3219752754296894559, 0.3333333333333333703, 0.3219752754296894559, 0.3333333333333333703, 0.3219752754296894559, 0.3333333333333333703, 0.3219752754296894559, 0.3333333333333333703, 0.3219752754296894559, 0.3333333333333333703, 0.3219752754296894559, 0.3333333333333333703, 0.3219752754296894559, 0.3333333333333333703, 0.3219752754296894559, 0.3333333333333333703, 0.3219752754296894559, 0.3333333333333333703, 0.3219752754296894559, 0.3333333333333333703, 0.3219752754296894559, 0.3333333333333333703, 0.3219752754296894559, 0.3333333333333333703, 0.3219752754296894559, 0.3333333333333333703, 0.3219752754296894559, 0.3333333333333333703, 0.3219752754296894559, 0.3333333333333333703, 0.3219752754296894559, 0.3333333333333333703, 0.3219752754296894559, 0.3333333333333333703, 0.3219752754296894559, 0.3333333333333333703, 0.3219752754296894559, 0.3333333333333333703, 0.3219752754296894559, 0.3333333333333333703, 0.3219752754296894559, 0.3333333333333333703, 0.3219752754296894559, 0.3333333333333333703, 0.3219752754296894559, 0.3333333333333333703, 0.3219752754296894559, 0.3333333333333333703, 0.3219752754296894559, 0.3333333333333333703, 0.3219752754296894559, 0.3333333333333333703, 0.3219752754296894559, 0.3333333333333333703, 0.3219752754296894559, 0.3333333333333333703, 0.3219752754296894559, 0.3333333333333333703, 0.3219752754296894559, 0.3333333333333333703, 0.3219752754296894559, 0.3333333333333333703, 0.3219752754296894559, 0.3333333333333333703, 0.3219752754296894559, 0.3333333333333333703, 0.3219752754296894559, 0.3333333333333333703, 0.3219752754296894559, 0.3333333333333333703, 0.3219752754296894559, 0.3333333333333333703, 0.3219752754296894559, 0.3333333333333333703, 0.3219752754296894559, 0.3333333333333333703, 0.3219752754296894559, 0.3333333333333333703, 0.3219752754296894559, 0.3333333333333333703, 0.3219752754296894559, 0.3333333333333333703, 0.3219752754296894559, 0.3333333333333333703, 0.3219752754296894559, 0.3333333333333333703, 0.3219752754296894559, 0.3333333333333333703, 0.3219752754296894559, 0.3333333333333333703, 0.3219752754296894559, 0.3333333333333333703, 0.3219752754296894559, 0.3333333333333333703, 0.3219752754296894559, 0.3333333333333333703, 0.3219752754296894559, 0.3333333333333333703, 0.3219752754296894559, 0.3333333333333333703, 0.3219752754296894559, 0.3333333333333333703, 0.3219752754296894559, 0.3333333333333333703, 0.3219752754296894559, 0.3333333333333333703, 0.3219752754296894559, 0.3333333333333333703, 0.3219752754296894559, 0.3333333333333333703, 0.3219752754296894559, 0.3333333333333333703, 0.3219752754296894559, 0.3333333333333333703, 0.3219752754296894559, 0.3333333333333333703, 0.3219752754296894559, 0.3333333333333333703, 0.3219752754296894559, 0.3333333333333333703, 0.3219752754296894559, 0.3333333333333333703, 0.3219752754296894559, 0.3333333333333333703, 0.3219752754296894559, 0.3333333333333333703, 0.3219752754296894559, 0.3333333333333333703, 0.3219752754296894559, 0.3333333333333333703, 0.3219752754296894559, 0.3333333333333333703, 0.3219752754296894559, 0.3333333333333333703, 0.3219752754296894559, 0.3333333333333333703, 0.3219752754296894559, 0.3333333333333333703, 0.3219752754296894559, 0.3333333333333333703, 0.3219752754296894559, 0.3333333333333333703, 0.3219752754296894559, 0.3333333333333333703, 0.3219752754296894559, 0.3333333333333333703, 0.3219752754296894559, 0.3333333333333333703, 0.3219752754296894559, 0.3333333333333333703, 0.3219752754296894559, 0.3333333333333333703, 0.3219752754296894559, 0.3333333333333333703, 0.3219752754296894559, 0.3333333333333333703, 0.3219752754296894559, 0.3333333333333333703, 0.3219752754296894559, 0.3333333333333333703, 0.3219752754296894559, 0.3333333333333333703, 0.3219752754296894559, 0.3333333333333333703, 0.3219752754296894559, 0.3333333333333333703, 0.3219752754296894559, 0.3333333333333333703, 0.3219752754296894559, 0.3333333333333333703, 0.3219752754296894559, 0.3333333333333333703, 0.3219752754296894559, 0.3333333333333333703, 0.3219752754296894559, 0.3333333333333333703, 0.3219752754296894559, 0.3333333333333333703, 0.3219752754296894559, 0.3333333333333333703, 0.3219752754296894559, 0.3333333333333333703, 0.3219752754296894559, 0.3333333333333333703, 0.3219752754296894559, 0.3333333333333333703, 0.3219752754296894559, 0.3333333333333333703, 0.3219752754296894559, 0.3333333333333333703, 0.3219752754296894559, 0.3333333333333333703, 0.3219752754296894559, 0.3333333333333333703, 0.3219752754296894559, 0.3333333333333333703, 0.3219752754296894559, 0.3333333333333333703, 0.3219752754296894559, 0.3333333333333333703, 0.3219752754296894559, 0.3333333333333333703, 0.3219752754296894559, 0.3333333333333333703, 0.3219752754296894559, 0.3333333333333333703, 0.3219752754296894559, 0.3333333333333333703, 0.3219752754296894559, 0.3333333333333333703, 0.3219752754296894559, 0.3333333333333333703, 0.3219752754296894559, 0.3333333333333333703, 0.3219752754296894559, 0.3333333333333333703, 0.3219752754296894559, 0.3333333333333333703, 0.3219752754296894559, 0.3333333333333333703, 0.3219752754296894559, 0.3333333333333333703, 0.3219752754296894559, 0.3333333333333333703, 0.3219752754296894559, 0.3333333333333333703, 0.3219752754296894559, 0.3333333333333333703, 0.3219752754296894559, 0.3333333333333333703, 0.3219752754296894559, 0.3333333333333333703, 0.3219752754296894559, 0.3333333333333333703, 0.3219752754296894559, 0.3333333333333333703, 0.3219752754296894559, 0.3333333333333333703, 0.3219752754296894559, 0.3333333333333333703, 0.3219752754296894559, 0.3333333333333333703, 0.3219752754296894559, 0.3333333333333333703, 0.3219752754296894559, 0.3333333333333333703, 0.3219752754296894559, 0.3333333333333333703, 0.3219752754296894559, 0.3333333333333333703, 0.3219752754296894559, 0.3333333333333333703, 0.3219752754296894559, 0.3333333333333333703, 0.3219752754296894559, 0.3333333333333333703, 0.3219752754296894559, 0.3333333333333333703, 0.3219752754296894559, 0.3333333333333333703, 0.3219752754296894559, 0.3333333333333333703, 0.3219752754296894559, 0.3333333333333333703, 0.3219752754296894559, 0.3333333333333333703, 0.3219752754296894559, 0.3333333333333333703, 0.3219752754296894559, 0.3333333333333333703, 0.3219752754296894559, 0.3333333333333333703, 0.3219752754296894559, 0.3333333333333333703, 0.3219752754296894559, 0.3333333333333333703, 0.3219752754296894559, 0.3333333333333333703, 0.3219752754296894559, 0.3333333333333333703, 0.3219752754296894559, 0.3333333333333333703, 0.3219752754296894559, 0.3333333333333333703, 0.3219752754296894559, 0.3333333333333333703, 0.3219752754296894559, 0.3333333333333333703, 0.3219752754296894559, 0.3333333333333333703, 0.3219752754296894559, 0.3333333333333333703, 0.3219752754296894559, 0.3333333333333333703, 0.3219752754296894559, 0.3333333333333333703, 0.3219752754296894559, 0.3333333333333333703, 0.3219752754296894559, 0.3333333333333333703, 0.3219752754296894559, 0.3333333333333333703, 0.3219752754296894559, 0.3333333333333333703, 0.3219752754296894559, 0.3333333333333333703, 0.3219752754296894559, 0.3333333333333333703, 0.3219752754296894559, 0.3333333333333333703, 0.3219752754296894559, 0.3333333333333333703, 0.3219752754296894559, 0.3333333333333333703, 0.3219752754296894559, 0.3333333333333333703, 0.3219752754296894559, 0.3333333333333333703, 0.3219752754296894559, 0.3333333333333333703, 0.3219752754296894559, 0.3333333333333333703, 0.3219752754296894559, 0.3333333333333333703, 0.3219752754296894559, 0.3333333333333333703, 0.3219752754296894559, 0.3333333333333333703, 0.3219752754296894559, 0.3333333333333333703, 0.3219752754296894559, 0.3333333333333333703, 0.3219752754296894559, 0.3333333333333333703, 0.3219752754296894559, 0.3333333333333333703, 0.3219752754296894559, 0.3333333333333333703, 0.3219752754296894559, 0.3333333333333333703, 0.3219752754296894559, 0.3333333333333333703, 0.3219752754296894559, 0.3333333333333333703, 0.3219752754296894559, 0.3333333333333333703, 0.3219752754296894559, 0.3333333333333333703, 0.3219752754296894559, 0.3333333333333333703, 0.3219752754296894559, 0.3333333333333333703, 0.3219752754296894559, 0.3333333333333333703),
 ( 0.3333333333333333703, 0.3219752754296894559, 0.3333333333333333703, 0.3219752754296894559, 0.3333333333333333703, 0.3219752754296894559, 0.3333333333333333703, 0.3219752754296894559, 0.3333333333333333703, 0.3219752754296894559, 0.3333333333333333703, 0.3219752754296894559, 0.3333333333333333703, 0.3219752754296894559, 0.3333333333333333703, 0.3219752754296894559, 0.3333333333333333703, 0.3219752754296894559, 0.3333333333333333703, 0.3219752754296894559, 0.3333333333333333703, 0.3219752754296894559, 0.3333333333333333703, 0.3219752754296894559, 0.3333333333333333703, 0.3219752754296894559, 0.3333333333333333703, 0.3219752754296894559, 0.3333333333333333703, 0.3219752754296894559, 0.3333333333333333703, 0.3219752754296894559, 0.3333333333333333703, 0.3219752754296894559, 0.3333333333333333703, 0.3219752754296894559, 0.3333333333333333703, 0.3219752754296894559, 0.3333333333333333703, 0.3219752754296894559, 0.3333333333333333703, 0.3219752754296894559, 0.3333333333333333703, 0.3219752754296894559, 0.3333333333333333703, 0.3219752754296894559, 0.3333333333333333703, 0.3219752754296894559, 0.3333333333333333703, 0.3219752754296894559, 0.3333333333333333703, 0.3219752754296894559, 0.3333333333333333703, 0.3219752754296894559, 0.3333333333333333703, 0.3219752754296894559, 0.3333333333333333703, 0.3219752754296894559, 0.3333333333333333703, 0.3219752754296894559, 0.3333333333333333703, 0.3219752754296894559, 0.3333333333333333703, 0.3219752754296894559, 0.3333333333333333703, 0.3219752754296894559, 0.3333333333333333703, 0.3219752754296894559, 0.3333333333333333703, 0.3219752754296894559, 0.3333333333333333703, 0.3219752754296894559, 0.3333333333333333703, 0.3219752754296894559, 0.3333333333333333703, 0.3219752754296894559, 0.3333333333333333703, 0.3219752754296894559, 0.3333333333333333703, 0.3219752754296894559, 0.3333333333333333703, 0.3219752754296894559, 0.3333333333333333703, 0.3219752754296894559, 0.3333333333333333703, 0.3219752754296894559, 0.3333333333333333703, 0.3219752754296894559, 0.3333333333333333703, 0.3219752754296894559, 0.3333333333333333703, 0.3219752754296894559, 0.3333333333333333703, 0.3219752754296894559, 0.3333333333333333703, 0.3219752754296894559, 0.3333333333333333703, 0.3219752754296894559, 0.3333333333333333703, 0.3219752754296894559, 0.3333333333333333703, 0.3219752754296894559, 0.3333333333333333703, 0.3219752754296894559, 0.3333333333333333703, 0.3219752754296894559, 0.3333333333333333703, 0.3219752754296894559, 0.3333333333333333703, 0.3219752754296894559, 0.3333333333333333703, 0.3219752754296894559, 0.3333333333333333703, 0.3219752754296894559, 0.3333333333333333703, 0.3219752754296894559, 0.3333333333333333703, 0.3219752754296894559, 0.3333333333333333703, 0.3219752754296894559, 0.3333333333333333703, 0.3219752754296894559, 0.3333333333333333703, 0.3219752754296894559, 0.3333333333333333703, 0.3219752754296894559, 0.3333333333333333703, 0.3219752754296894559, 0.3333333333333333703, 0.3219752754296894559, 0.3333333333333333703, 0.3219752754296894559, 0.3333333333333333703, 0.3219752754296894559, 0.3333333333333333703, 0.3219752754296894559, 0.3333333333333333703, 0.3219752754296894559, 0.3333333333333333703, 0.3219752754296894559, 0.3333333333333333703, 0.3219752754296894559, 0.3333333333333333703, 0.3219752754296894559, 0.3333333333333333703, 0.3219752754296894559, 0.3333333333333333703, 0.3219752754296894559, 0.3333333333333333703, 0.3219752754296894559, 0.3333333333333333703, 0.3219752754296894559, 0.3333333333333333703, 0.3219752754296894559, 0.3333333333333333703, 0.3219752754296894559, 0.3333333333333333703, 0.3219752754296894559, 0.3333333333333333703, 0.3219752754296894559, 0.3333333333333333703, 0.3219752754296894559, 0.3333333333333333703, 0.3219752754296894559, 0.3333333333333333703, 0.3219752754296894559, 0.3333333333333333703, 0.3219752754296894559, 0.3333333333333333703, 0.3219752754296894559, 0.3333333333333333703, 0.3219752754296894559, 0.3333333333333333703, 0.3219752754296894559, 0.3333333333333333703, 0.3219752754296894559, 0.3333333333333333703, 0.3219752754296894559, 0.3333333333333333703, 0.3219752754296894559, 0.3333333333333333703, 0.3219752754296894559, 0.3333333333333333703, 0.3219752754296894559, 0.3333333333333333703, 0.3219752754296894559, 0.3333333333333333703, 0.3219752754296894559, 0.3333333333333333703, 0.3219752754296894559, 0.3333333333333333703, 0.3219752754296894559, 0.3333333333333333703, 0.3219752754296894559, 0.3333333333333333703, 0.3219752754296894559, 0.3333333333333333703, 0.3219752754296894559, 0.3333333333333333703, 0.3219752754296894559, 0.3333333333333333703, 0.3219752754296894559, 0.3333333333333333703, 0.3219752754296894559, 0.3333333333333333703, 0.3219752754296894559, 0.3333333333333333703, 0.3219752754296894559, 0.3333333333333333703, 0.3219752754296894559, 0.3333333333333333703, 0.3219752754296894559, 0.3333333333333333703, 0.3219752754296894559, 0.3333333333333333703, 0.3219752754296894559, 0.3333333333333333703, 0.3219752754296894559, 0.3333333333333333703, 0.3219752754296894559, 0.3333333333333333703, 0.3219752754296894559, 0.3333333333333333703, 0.3219752754296894559, 0.3333333333333333703, 0.3219752754296894559, 0.3333333333333333703, 0.3219752754296894559, 0.3333333333333333703, 0.3219752754296894559, 0.3333333333333333703, 0.3219752754296894559, 0.3333333333333333703, 0.3219752754296894559, 0.3333333333333333703, 0.3219752754296894559, 0.3333333333333333703, 0.3219752754296894559, 0.3333333333333333703, 0.3219752754296894559, 0.3333333333333333703, 0.3219752754296894559, 0.3333333333333333703, 0.3219752754296894559, 0.3333333333333333703, 0.3219752754296894559, 0.3333333333333333703, 0.3219752754296894559, 0.3333333333333333703, 0.3219752754296894559, 0.3333333333333333703, 0.3219752754296894559, 0.3333333333333333703, 0.3219752754296894559, 0.3333333333333333703, 0.3219752754296894559, 0.3333333333333333703, 0.3219752754296894559, 0.3333333333333333703, 0.3219752754296894559, 0.3333333333333333703, 0.3219752754296894559, 0.3333333333333333703, 0.3219752754296894559, 0.3333333333333333703, 0.3219752754296894559, 0.3333333333333333703, 0.3219752754296894559, 0.3333333333333333703, 0.3219752754296894559, 0.3333333333333333703, 0.3219752754296894559, 0.3333333333333333703, 0.3219752754296894559, 0.3333333333333333703, 0.3219752754296894559, 0.3333333333333333703, 0.3219752754296894559, 0.3333333333333333703, 0.3219752754296894559, 0.3333333333333333703, 0.3219752754296894559, 0.3333333333333333703, 0.3219752754296894559, 0.3333333333333333703, 0.3219752754296894559, 0.3333333333333333703, 0.3219752754296894559, 0.3333333333333333703, 0.3219752754296894559, 0.3333333333333333703, 0.3219752754296894559, 0.3333333333333333703, 0.3219752754296894559, 0.3333333333333333703, 0.3219752754296894559, 0.3333333333333333703, 0.3219752754296894559, 0.3333333333333333703, 0.3219752754296894559, 0.3333333333333333703, 0.3219752754296894559, 0.3333333333333333703, 0.3219752754296894559, 0.3333333333333333703, 0.3219752754296894559, 0.3333333333333333703, 0.3219752754296894559, 0.3333333333333333703, 0.3219752754296894559, 0.3333333333333333703, 0.3219752754296894559, 0.3333333333333333703, 0.3219752754296894559, 0.3333333333333333703, 0.3219752754296894559, 0.3333333333333333703, 0.3219752754296894559, 0.3333333333333333703, 0.3219752754296894559, 0.3333333333333333703, 0.3219752754296894559, 0.3333333333333333703, 0.3219752754296894559, 0.3333333333333333703, 0.3219752754296894559, 0.3333333333333333703, 0.3219752754296894559, 0.3333333333333333703, 0.3219752754296894559, 0.3333333333333333703, 0.3219752754296894559, 0.3333333333333333703, 0.3219752754296894559, 0.3333333333333333703, 0.3219752754296894559, 0.3333333333333333703, 0.3219752754296894559, 0.3333333333333333703, 0.3219752754296894559, 0.3333333333333333703, 0.3219752754296894559, 0.3333333333333333703, 0.3219752754296894559, 0.3333333333333333703, 0.3219752754296894559, 0.3333333333333333703, 0.3219752754296894559, 0.3333333333333333703, 0.3219752754296894559, 0.3333333333333333703, 0.3219752754296894559, 0.3333333333333333703, 0.3219752754296894559, 0.3333333333333333703, 0.3219752754296894559, 0.3333333333333333703, 0.3219752754296894559, 0.3333333333333333703, 0.3219752754296894559, 0.3333333333333333703, 0.3219752754296894559, 0.3333333333333333703, 0.3219752754296894559, 0.3333333333333333703, 0.3219752754296894559, 0.3333333333333333703, 0.3219752754296894559, 0.3333333333333333703, 0.3219752754296894559, 0.3333333333333333703, 0.3219752754296894559, 0.3333333333333333703, 0.3219752754296894559, 0.3333333333333333703, 0.3219752754296894559, 0.3333333333333333703, 0.3219752754296894559, 0.3333333333333333703, 0.3219752754296894559, 0.3333333333333333703, 0.3219752754296894559, 0.3333333333333333703, 0.3219752754296894559, 0.3333333333333333703, 0.3219752754296894559, 0.3333333333333333703, 0.3219752754296894559, 0.3333333333333333703, 0.3219752754296894559, 0.3333333333333333703, 0.3219752754296894559, 0.3333333333333333703, 0.3219752754296894559, 0.3333333333333333703, 0.3219752754296894559, 0.3333333333333333703, 0.3219752754296894559, 0.3333333333333333703, 0.3219752754296894559, 0.3333333333333333703, 0.3219752754296894559, 0.3333333333333333703, 0.3219752754296894559, 0.3333333333333333703, 0.3219752754296894559, 0.3333333333333333703, 0.3219752754296894559, 0.3333333333333333703, 0.3219752754296894559, 0.3333333333333333703, 0.3219752754296894559, 0.3333333333333333703, 0.3219752754296894559, 0.3333333333333333703, 0.3219752754296894559, 0.3333333333333333703, 0.3219752754296894559, 0.3333333333333333703, 0.3219752754296894559, 0.3333333333333333703, 0.3219752754296894559, 0.3333333333333333703, 0.3219752754296894559, 0.3333333333333333703, 0.3219752754296894559, 0.3333333333333333703, 0.3219752754296894559, 0.3333333333333333703, 0.3219752754296894559, 0.3333333333333333703, 0.3219752754296894559, 0.3333333333333333703, 0.3219752754296894559, 0.3333333333333333703, 0.3219752754296894559, 0.3333333333333333703, 0.3219752754296894559, 0.3333333333333333703, 0.3219752754296894559, 0.3333333333333333703, 0.3219752754296894559, 0.3333333333333333703, 0.3219752754296894559, 0.3333333333333333703, 0.3219752754296894559, 0.3333333333333333703, 0.3219752754296894559, 0.3333333333333333703, 0.3219752754296894559, 0.3333333333333333703, 0.3219752754296894559, 0.3333333333333333703, 0.3219752754296894559, 0.3333333333333333703, 0.3219752754296894559, 0.3333333333333333703),
 ( 1.000000000000000000, 0.9659258262890683122, 1.000000000000000000, 0.9659258262890683122, 1.000000000000000000, 0.9659258262890683122, 1.000000000000000000, 0.9659258262890683122, 1.000000000000000000, 0.9659258262890683122, 1.000000000000000000, 0.9659258262890683122, 1.000000000000000000, 0.9659258262890683122, 1.000000000000000000, 0.9659258262890683122, 1.000000000000000000, 0.9659258262890683122, 1.000000000000000000, 0.9659258262890683122, 1.000000000000000000, 0.9659258262890683122, 1.000000000000000000, 0.9659258262890683122, 1.000000000000000000, 0.9659258262890683122, 1.000000000000000000, 0.9659258262890683122, 1.000000000000000000, 0.9659258262890683122, 1.000000000000000000, 0.9659258262890683122, 1.000000000000000000, 0.9659258262890683122, 1.000000000000000000, 0.9659258262890683122, 1.000000000000000000, 0.9659258262890683122, 1.000000000000000000, 0.9659258262890683122, 1.000000000000000000, 0.9659258262890683122, 1.000000000000000000, 0.9659258262890683122, 1.000000000000000000, 0.9659258262890683122, 1.000000000000000000, 0.9659258262890683122, 1.000000000000000000, 0.9659258262890683122, 1.000000000000000000, 0.9659258262890683122, 1.000000000000000000, 0.9659258262890683122, 1.000000000000000000, 0.9659258262890683122, 1.000000000000000000, 0.9659258262890683122, 1.000000000000000000, 0.9659258262890683122, 1.000000000000000000, 0.9659258262890683122, 1.000000000000000000, 0.9659258262890683122, 1.000000000000000000, 0.9659258262890683122, 1.000000000000000000, 0.9659258262890683122, 1.000000000000000000, 0.9659258262890683122, 1.000000000000000000, 0.9659258262890683122, 1.000000000000000000, 0.9659258262890683122, 1.000000000000000000, 0.9659258262890683122, 1.000000000000000000, 0.9659258262890683122, 1.000000000000000000, 0.9659258262890683122, 1.000000000000000000, 0.9659258262890683122, 1.000000000000000000, 0.9659258262890683122, 1.000000000000000000, 0.9659258262890683122, 1.000000000000000000, 0.9659258262890683122, 1.000000000000000000, 0.9659258262890683122, 1.000000000000000000, 0.9659258262890683122, 1.000000000000000000, 0.9659258262890683122, 1.000000000000000000, 0.9659258262890683122, 1.000000000000000000, 0.9659258262890683122, 1.000000000000000000, 0.9659258262890683122, 1.000000000000000000, 0.9659258262890683122, 1.000000000000000000, 0.9659258262890683122, 1.000000000000000000, 0.9659258262890683122, 1.000000000000000000, 0.9659258262890683122, 1.000000000000000000, 0.9659258262890683122, 1.000000000000000000, 0.9659258262890683122, 1.000000000000000000, 0.9659258262890683122, 1.000000000000000000, 0.9659258262890683122, 1.000000000000000000, 0.9659258262890683122, 1.000000000000000000, 0.9659258262890683122, 1.000000000000000000, 0.9659258262890683122, 1.000000000000000000, 0.9659258262890683122, 1.000000000000000000, 0.9659258262890683122, 1.000000000000000000, 0.9659258262890683122, 1.000000000000000000, 0.9659258262890683122, 1.000000000000000000, 0.9659258262890683122, 1.000000000000000000, 0.9659258262890683122, 1.000000000000000000, 0.9659258262890683122, 1.000000000000000000, 0.9659258262890683122, 1.000000000000000000, 0.9659258262890683122, 1.000000000000000000, 0.9659258262890683122, 1.000000000000000000, 0.9659258262890683122, 1.000000000000000000, 0.9659258262890683122, 1.000000000000000000, 0.9659258262890683122, 1.000000000000000000, 0.9659258262890683122, 1.000000000000000000, 0.9659258262890683122, 1.000000000000000000, 0.9659258262890683122, 1.000000000000000000, 0.9659258262890683122, 1.000000000000000000, 0.9659258262890683122, 1.000000000000000000, 0.9659258262890683122, 1.000000000000000000, 0.9659258262890683122, 1.000000000000000000, 0.9659258262890683122, 1.000000000000000000, 0.9659258262890683122, 1.000000000000000000, 0.9659258262890683122, 1.000000000000000000, 0.9659258262890683122, 1.000000000000000000, 0.9659258262890683122, 1.000000000000000000, 0.9659258262890683122, 1.000000000000000000, 0.9659258262890683122, 1.000000000000000000, 0.9659258262890683122, 1.000000000000000000, 0.9659258262890683122, 1.000000000000000000, 0.9659258262890683122, 1.000000000000000000, 0.9659258262890683122, 1.000000000000000000, 0.9659258262890683122, 1.000000000000000000, 0.9659258262890683122, 1.000000000000000000, 0.9659258262890683122, 1.000000000000000000, 0.9659258262890683122, 1.000000000000000000, 0.9659258262890683122, 1.000000000000000000, 0.9659258262890683122, 1.000000000000000000, 0.9659258262890683122, 1.000000000000000000, 0.9659258262890683122, 1.000000000000000000, 0.9659258262890683122, 1.000000000000000000, 0.9659258262890683122, 1.000000000000000000, 0.9659258262890683122, 1.000000000000000000, 0.9659258262890683122, 1.000000000000000000, 0.9659258262890683122, 1.000000000000000000, 0.9659258262890683122, 1.000000000000000000, 0.9659258262890683122, 1.000000000000000000, 0.9659258262890683122, 1.000000000000000000, 0.9659258262890683122, 1.000000000000000000, 0.9659258262890683122, 1.000000000000000000, 0.9659258262890683122, 1.000000000000000000, 0.9659258262890683122, 1.000000000000000000, 0.9659258262890683122, 1.000000000000000000, 0.9659258262890683122, 1.000000000000000000, 0.9659258262890683122, 1.000000000000000000, 0.9659258262890683122, 1.000000000000000000, 0.9659258262890683122, 1.000000000000000000, 0.9659258262890683122, 1.000000000000000000, 0.9659258262890683122, 1.000000000000000000, 0.9659258262890683122, 1.000000000000000000, 0.9659258262890683122, 1.000000000000000000, 0.9659258262890683122, 1.000000000000000000, 0.9659258262890683122, 1.000000000000000000, 0.9659258262890683122, 1.000000000000000000, 0.9659258262890683122, 1.000000000000000000, 0.9659258262890683122, 1.000000000000000000, 0.9659258262890683122, 1.000000000000000000, 0.9659258262890683122, 1.000000000000000000, 0.9659258262890683122, 1.000000000000000000, 0.9659258262890683122, 1.000000000000000000, 0.9659258262890683122, 1.000000000000000000, 0.9659258262890683122, 1.000000000000000000, 0.9659258262890683122, 1.000000000000000000, 0.9659258262890683122, 1.000000000000000000, 0.9659258262890683122, 1.000000000000000000, 0.9659258262890683122, 1.000000000000000000, 0.9659258262890683122, 1.000000000000000000, 0.9659258262890683122, 1.000000000000000000, 0.9659258262890683122, 1.000000000000000000, 0.9659258262890683122, 1.000000000000000000, 0.9659258262890683122, 1.000000000000000000, 0.9659258262890683122, 1.000000000000000000, 0.9659258262890683122, 1.000000000000000000, 0.9659258262890683122, 1.000000000000000000, 0.9659258262890683122, 1.000000000000000000, 0.9659258262890683122, 1.000000000000000000, 0.9659258262890683122, 1.000000000000000000, 0.9659258262890683122, 1.000000000000000000, 0.9659258262890683122, 1.000000000000000000, 0.9659258262890683122, 1.000000000000000000, 0.9659258262890683122, 1.000000000000000000, 0.9659258262890683122, 1.000000000000000000, 0.9659258262890683122, 1.000000000000000000, 0.9659258262890683122, 1.000000000000000000, 0.9659258262890683122, 1.000000000000000000, 0.9659258262890683122, 1.000000000000000000, 0.9659258262890683122, 1.000000000000000000, 0.9659258262890683122, 1.000000000000000000, 0.9659258262890683122, 1.000000000000000000, 0.9659258262890683122, 1.000000000000000000, 0.9659258262890683122, 1.000000000000000000, 0.9659258262890683122, 1.000000000000000000, 0.9659258262890683122, 1.000000000000000000, 0.9659258262890683122, 1.000000000000000000, 0.9659258262890683122, 1.000000000000000000, 0.9659258262890683122, 1.000000000000000000, 0.9659258262890683122, 1.000000000000000000, 0.9659258262890683122, 1.000000000000000000, 0.9659258262890683122, 1.000000000000000000, 0.9659258262890683122, 1.000000000000000000, 0.9659258262890683122, 1.000000000000000000, 0.9659258262890683122, 1.000000000000000000, 0.9659258262890683122, 1.000000000000000000, 0.9659258262890683122, 1.000000000000000000, 0.9659258262890683122, 1.000000000000000000, 0.9659258262890683122, 1.000000000000000000, 0.9659258262890683122, 1.000000000000000000, 0.9659258262890683122, 1.000000000000000000, 0.9659258262890683122, 1.000000000000000000, 0.9659258262890683122, 1.000000000000000000, 0.9659258262890683122, 1.000000000000000000, 0.9659258262890683122, 1.000000000000000000, 0.9659258262890683122, 1.000000000000000000, 0.9659258262890683122, 1.000000000000000000, 0.9659258262890683122, 1.000000000000000000, 0.9659258262890683122, 1.000000000000000000, 0.9659258262890683122, 1.000000000000000000, 0.9659258262890683122, 1.000000000000000000, 0.9659258262890683122, 1.000000000000000000, 0.9659258262890683122, 1.000000000000000000, 0.9659258262890683122, 1.000000000000000000, 0.9659258262890683122, 1.000000000000000000, 0.9659258262890683122, 1.000000000000000000, 0.9659258262890683122, 1.000000000000000000, 0.9659258262890683122, 1.000000000000000000, 0.9659258262890683122, 1.000000000000000000, 0.9659258262890683122, 1.000000000000000000, 0.9659258262890683122, 1.000000000000000000, 0.9659258262890683122, 1.000000000000000000, 0.9659258262890683122, 1.000000000000000000, 0.9659258262890683122, 1.000000000000000000, 0.9659258262890683122, 1.000000000000000000, 0.9659258262890683122, 1.000000000000000000, 0.9659258262890683122, 1.000000000000000000, 0.9659258262890683122, 1.000000000000000000, 0.9659258262890683122, 1.000000000000000000, 0.9659258262890683122, 1.000000000000000000, 0.9659258262890683122, 1.000000000000000000, 0.9659258262890683122, 1.000000000000000000, 0.9659258262890683122, 1.000000000000000000, 0.9659258262890683122, 1.000000000000000000, 0.9659258262890683122, 1.000000000000000000, 0.9659258262890683122, 1.000000000000000000, 0.9659258262890683122, 1.000000000000000000, 0.9659258262890683122, 1.000000000000000000, 0.9659258262890683122, 1.000000000000000000, 0.9659258262890683122, 1.000000000000000000, 0.9659258262890683122, 1.000000000000000000, 0.9659258262890683122, 1.000000000000000000, 0.9659258262890683122, 1.000000000000000000, 0.9659258262890683122, 1.000000000000000000, 0.9659258262890683122, 1.000000000000000000, 0.9659258262890683122, 1.000000000000000000, 0.9659258262890683122, 1.000000000000000000, 0.9659258262890683122, 1.000000000000000000, 0.9659258262890683122, 1.000000000000000000, 0.9659258262890683122, 1.000000000000000000, 0.9659258262890683122, 1.000000000000000000) ) ) 
 REPRESENTATION_ITEM ( '' )  SURFACE ( )  );
#60898=CARTESIAN_POINT ( 'NONE',  ( 5.153800228976615827, -19.02544592524334988, 45.20942372801901143 ) ) ;
#60899=CARTESIAN_POINT ( 'NONE',  ( 16.38665767534995510, -7.295008042176407415, 72.76400864214468811 ) ) ;
#60901=CARTESIAN_POINT ( 'NONE',  ( -5.153800228976328057, -19.02544592524343514, 62.29057627198100988 ) ) ;
#60902=CARTESIAN_POINT ( 'NONE',  ( 5.153800228976335163, 19.02544592524342804, 84.79057627198099567 ) ) ;
#60903=CARTESIAN_POINT ( 'NONE',  ( 0.05219959533934541429, -16.53943276465976808, 50.00109039468568994 ) ) ;
#60905=CARTESIAN_POINT ( 'NONE',  ( -19.02544592524334988, -5.153800228976617603, 23.95942372801900078 ) ) ;
#60907=CARTESIAN_POINT ( 'NONE',  ( 16.55341960407618274, -4.379528057220086978, 91.04275706135236135 ) ) ;
#60909=CARTESIAN_POINT ( 'NONE',  ( 16.53943276465976808, 0.05219959533934440121, 81.25109039468568994 ) ) ;
#60910=CARTESIAN_POINT ( 'NONE',  ( -16.55341960407617563, 4.379528057220093196, 58.54275706135235424 ) ) ;
#60911=CARTESIAN_POINT ( 'NONE',  ( -16.46253265017160317, 9.564922557960807481, 50.83224293864770260 ) ) ;
#60913=CARTESIAN_POINT ( 'NONE',  ( 10.81492255796106328, -18.62759615963255655, 70.41775706135236135 ) ) ;
#60914=CARTESIAN_POINT ( 'NONE',  ( -13.97604488694547697, 13.89961937509957934, 73.12609039468568994 ) ) ;
#60915=CARTESIAN_POINT ( 'NONE',  ( 18.67979575497194134, -10.72451020669871369, 110.8344237280190043 ) ) ;
#60916=CARTESIAN_POINT ( 'NONE',  ( 9.474510206698971260, -16.51473224551069308, 47.91557627198102409 ) ) ;
#60917=CARTESIAN_POINT ( 'NONE',  ( 16.51473224551069308, 9.474510206698969483, 49.16557627198102409 ) ) ;
#60919=CARTESIAN_POINT ( 'NONE',  ( 5.823673210054125526, 21.52544592524343514, 69.79057627198102409 ) ) ;
#60920=EDGE_CURVE ( 'NONE', #194071, #30776, #123707, .T. ) ;
#60921=CARTESIAN_POINT ( 'NONE',  ( -5.049401038298153566, 19.05341960407611168, 110.2072429386476671 ) ) ;
#60922=CARTESIAN_POINT ( 'NONE',  ( 9.474510206698971260, -16.51473224551069308, 22.91557627198102765 ) ) ;
#60923=CARTESIAN_POINT ( 'NONE',  ( 4.379528057220092307, 16.55341960407617563, 57.29275706135234714 ) ) ;
#60924=CARTESIAN_POINT ( 'NONE',  ( -8.224510206698948167, 14.34966873604960824, 30.41557627198101699 ) ) ;
#60926=CARTESIAN_POINT ( 'NONE',  ( 0.05219959533907565091, 21.53943276465977519, 114.9989096053143669 ) ) ;
#60927=CARTESIAN_POINT ( 'NONE',  ( -0.05219959533910754901, -16.53943276465976808, 52.49890960531435979 ) ) ;
#60929=CARTESIAN_POINT ( 'NONE',  ( -16.51473224551082808, 9.474510206698731452, 103.3344237280190043 ) ) ;
#60930=CARTESIAN_POINT ( 'NONE',  ( -16.51473224551082808, 9.474510206698731452, 43.33442372801900433 ) ) ;
#60931=CARTESIAN_POINT ( 'NONE',  ( 0.05219959533910956823, 16.53943276465976808, 44.99890960531435979 ) ) ;
#60932=CARTESIAN_POINT ( 'NONE',  ( 5.823673210054125526, 21.52544592524343514, 104.7905762719810241 ) ) ;
#60933=CARTESIAN_POINT ( 'NONE',  ( 16.18388926212241330, 7.379444403734403579, 32.93953151366154231 ) ) ;
#60934=CARTESIAN_POINT ( 'NONE',  ( 5.823673210054125526, 21.52544592524343514, 69.79057627198102409 ) ) ;
#60935=CARTESIAN_POINT ( 'NONE',  ( 9.564922557960805705, 16.46253265017160317, 74.58224293864769550 ) ) ;
#60936=CARTESIAN_POINT ( 'NONE',  ( -0.05219959533910754901, -16.53943276465976808, 47.49890960531435979 ) ) ;
#60937=CARTESIAN_POINT ( 'NONE',  ( 13.89961937509977652, -13.97604488694527269, 108.1239096053143669 ) ) ;
#60939=CARTESIAN_POINT ( 'NONE',  ( 0.05219959533936267826, -19.03943276465977164, 55.00109039468566863 ) ) ;
#60940=CARTESIAN_POINT ( 'NONE',  ( -10.72451020669898014, 18.67979575497178502, 90.41557627198103830 ) ) ;
#60941=CARTESIAN_POINT ( 'NONE',  ( 5.153800228976335163, 19.02544592524342804, 49.79057627198100988 ) ) ;
#60942=CARTESIAN_POINT ( 'NONE',  ( 16.52544592524342804, -4.483927247898539470, 113.5405762719810383 ) ) ;
#60943=CARTESIAN_POINT ( 'NONE',  ( -18.67979575497193778, 10.72451020669871902, 48.33442372801902565 ) ) ;
#60945=CARTESIAN_POINT ( 'NONE',  ( -16.55341960407611168, -4.379528057220339221, 21.45724293864769550 ) ) ;
#60946=CARTESIAN_POINT ( 'NONE',  ( -19.05341960407611168, -5.049401038298163336, 51.45724293864770260 ) ) ;
#60947=CARTESIAN_POINT ( 'NONE',  ( 16.46253265017160672, -9.564922557960803928, 103.3322429386476955 ) ) ;
#60948=CARTESIAN_POINT ( 'NONE',  ( -18.67979575497178146, -10.72451020669898902, 66.66557627198102409 ) ) ;
#60950=CARTESIAN_POINT ( 'NONE',  ( -9.474510206698964154, 16.51473224551069663, 45.41557627198103120 ) ) ;
#60951=CARTESIAN_POINT ( 'NONE',  ( 18.67979575497178502, 10.72451020669898547, 54.16557627198103120 ) ) ;
#60953=CARTESIAN_POINT ( 'NONE',  ( -18.67979575497193778, 10.72451020669871902, 93.33442372801901854 ) ) ;
#60955=CARTESIAN_POINT ( 'NONE',  ( -12.06949235617739369, -12.14591786802326823, 79.37609039468567573 ) ) ;
#60956=CARTESIAN_POINT ( 'NONE',  ( 8.314922557961029526, -14.29746914071037800, 85.41775706135236135 ) ) ;
#60957=CARTESIAN_POINT ( 'NONE',  ( 16.46253265017160672, -9.564922557960803928, 68.33224293864770971 ) ) ;
#60958=ORIENTED_EDGE ( 'NONE', *, *, #68626, .F. ) ;
#60959=CARTESIAN_POINT ( 'NONE',  ( -16.51473224551082808, 9.474510206698731452, 23.33442372801900078 ) ) ;
#60960=CARTESIAN_POINT ( 'NONE',  ( 12.14591786802327356, -12.06949235617739191, 85.62609039468568994 ) ) ;
#60961=CARTESIAN_POINT ( 'NONE',  ( -19.02544592524334988, -5.153800228976617603, 18.95942372801899722 ) ) ;
#60962=CARTESIAN_POINT ( 'NONE',  ( -16.46253265017160317, 9.564922557960807481, 80.83224293864769550 ) ) ;
#60963=CARTESIAN_POINT ( 'NONE',  ( 18.62759615963271287, -10.81492255796078972, 53.33224293864769550 ) ) ;
#60964=CARTESIAN_POINT ( 'NONE',  ( -12.06949235617739369, -12.14591786802326823, 24.37609039468567573 ) ) ;
#60965=CARTESIAN_POINT ( 'NONE',  ( 21.55341960407619695, -5.719274019375665929, 86.04275706135236135 ) ) ;
#60966=CARTESIAN_POINT ( 'NONE',  ( -14.34966873604972548, 8.224510206698743886, 68.33442372801900433 ) ) ;
#60967=CARTESIAN_POINT ( 'NONE',  ( -15.80617190586745835, -15.72974639402198527, 111.8739096053143669 ) ) ;
#60968=CARTESIAN_POINT ( 'NONE',  ( -5.153800228976607833, 19.02544592524334988, 112.7094237280190043 ) ) ;
#60969=CARTESIAN_POINT ( 'NONE',  ( 13.97604488694527802, 13.89961937509977652, 94.37390960531436690 ) ) ;
#60970=CARTESIAN_POINT ( 'NONE',  ( -12.06949235617739369, -12.14591786802326823, 34.37609039468568284 ) ) ;
#60971=CARTESIAN_POINT ( 'NONE',  ( 19.02544592524343514, -5.153800228976328945, 38.54057627198103120 ) ) ;
#60972=CARTESIAN_POINT ( 'NONE',  ( -4.379528057220086978, -16.55341960407618274, 19.79275706135235069 ) ) ;
#60973=CARTESIAN_POINT ( 'NONE',  ( -4.379528057220328563, 16.55341960407611168, 80.20724293864769550 ) ) ;
#60974=CARTESIAN_POINT ( 'NONE',  ( 4.379528057220092307, 16.55341960407617563, 92.29275706135236135 ) ) ;
#60975=CARTESIAN_POINT ( 'NONE',  ( -15.80617190586768217, 15.72974639402176855, 33.12609039468569705 ) ) ;
#60976=CARTESIAN_POINT ( 'NONE',  ( -0.05219959533909027116, -19.03943276465977164, 62.49890960531435979 ) ) ;
#60977=CARTESIAN_POINT ( 'NONE',  ( 5.049401038298161559, -19.05341960407611168, 72.70724293864768129 ) ) ;
#60979=CARTESIAN_POINT ( 'NONE',  ( 12.14591786802327356, -12.06949235617739191, 80.62609039468567573 ) ) ;
#60983=CARTESIAN_POINT ( 'NONE',  ( -5.153800228976607833, 19.02544592524334988, 27.70942372801899722 ) ) ;
#60984=CARTESIAN_POINT ( 'NONE',  ( 16.46253265017160672, -9.564922557960803928, 33.33224293864770260 ) ) ;
#60987=CARTESIAN_POINT ( 'NONE',  ( -4.379528057220086978, -16.55341960407618274, 24.79275706135235779 ) ) ;
#60989=CARTESIAN_POINT ( 'NONE',  ( 0.05219959533936267826, -19.03943276465977164, 60.00109039468566863 ) ) ;
#60990=CARTESIAN_POINT ( 'NONE',  ( -14.34966873604972548, 8.224510206698743886, 48.33442372801902565 ) ) ;
#60991=CARTESIAN_POINT ( 'NONE',  ( 9.564922557960805705, 16.46253265017160317, 99.58224293864770971 ) ) ;
#60992=CARTESIAN_POINT ( 'NONE',  ( 13.97604488694527802, 13.89961937509977652, 79.37390960531435269 ) ) ;
#60993=CARTESIAN_POINT ( 'NONE',  ( 10.72451020669898902, -18.67979575497178502, 92.91557627198103830 ) ) ;
#60994=CARTESIAN_POINT ( 'NONE',  ( -16.51473224551082808, 9.474510206698731452, 68.33442372801900433 ) ) ;
#60995=CARTESIAN_POINT ( 'NONE',  ( 16.46253265017160672, -9.564922557960803928, 93.33224293864769550 ) ) ;
#60996=CARTESIAN_POINT ( 'NONE',  ( -0.05219959533909027116, -19.03943276465977164, 22.49890960531436690 ) ) ;
#60998=CARTESIAN_POINT ( 'NONE',  ( -9.564922557960796823, -16.46253265017161027, 57.08224293864769550 ) ) ;
#60999=CARTESIAN_POINT ( 'NONE',  ( -16.55341960407611168, -4.379528057220339221, 26.45724293864768839 ) ) ;
#61000=CARTESIAN_POINT ( 'NONE',  ( -17.58332526062529411, 7.635886036038502134, 70.92334959558468199 ) ) ;
#61001=CARTESIAN_POINT ( 'NONE',  ( 13.97604488694548053, -13.89961937509957401, 35.62609039468567573 ) ) ;
#61002=CARTESIAN_POINT ( 'NONE',  ( 8.314922557960818139, 14.29746914071049879, 69.58224293864769550 ) ) ;
#61003=CARTESIAN_POINT ( 'NONE',  ( -18.62759615963255300, -10.81492255796106328, 94.16775706135237556 ) ) ;
#61004=CARTESIAN_POINT ( 'NONE',  ( 5.049401038298161559, -19.05341960407611168, 42.70724293864767418 ) ) ;
#61005=CARTESIAN_POINT ( 'NONE',  ( -14.29746914071037622, -8.314922557961029526, 54.16775706135235424 ) ) ;
#61006=CARTESIAN_POINT ( 'NONE',  ( 16.52544592524342804, -4.483927247898539470, 38.54057627198103120 ) ) ;
#61007=CARTESIAN_POINT ( 'NONE',  ( 5.719274019375673035, 21.55341960407619339, 87.29275706135236135 ) ) ;
#61008=CARTESIAN_POINT ( 'NONE',  ( 19.05341960407611168, 5.049401038298154454, 98.95724293864766707 ) ) ;
#61009=CARTESIAN_POINT ( 'NONE',  ( 19.03943276465977164, -0.05219959533909143690, 93.74890960531435269 ) ) ;
#61010=CARTESIAN_POINT ( 'NONE',  ( 0.05219959533910956823, 16.53943276465976808, 104.9989096053143669 ) ) ;
#61011=CARTESIAN_POINT ( 'NONE',  ( 4.379528057220339221, -16.55341960407611168, 67.70724293864769550 ) ) ;
#61012=CARTESIAN_POINT ( 'NONE',  ( -15.72974639402197994, 15.80617190586746368, 80.62390960531438111 ) ) ;
#61013=CARTESIAN_POINT ( 'NONE',  ( 16.51473224551069308, 9.474510206698969483, 94.16557627198103830 ) ) ;
#61014=CARTESIAN_POINT ( 'NONE',  ( -10.72451020669898014, 18.67979575497178502, 95.41557627198102409 ) ) ;
#61015=CARTESIAN_POINT ( 'NONE',  ( 16.46253265017146816, 9.564922557961045513, 81.66775706135233293 ) ) ;
#61016=CARTESIAN_POINT ( 'NONE',  ( -19.39720447994792707, -5.500000000000080824, 89.66317477297177163 ) ) ;
#61017=CARTESIAN_POINT ( 'NONE',  ( 0.05219959533910956823, 16.53943276465976808, 94.99890960531436690 ) ) ;
#61018=CARTESIAN_POINT ( 'NONE',  ( 9.474510206698971260, -16.51473224551069308, 52.91557627198102409 ) ) ;
#61019=CARTESIAN_POINT ( 'NONE',  ( 5.719274019375991003, -21.55341960407610458, 67.70724293864769550 ) ) ;
#61020=CARTESIAN_POINT ( 'NONE',  ( 17.26172910966779739, -6.454744622555848466, 28.30646908649225324 ) ) ;
#61021=CARTESIAN_POINT ( 'NONE',  ( -16.53943276465976808, 0.05219959533911058130, 21.24890960531436690 ) ) ;
#61022=CARTESIAN_POINT ( 'NONE',  ( -17.49999999999999645, 5.499999999999992895, 58.71769037696435589 ) ) ;
#61023=CARTESIAN_POINT ( 'NONE',  ( -14.29746914071037622, -8.314922557961029526, 19.16775706135234714 ) ) ;
#61024=CARTESIAN_POINT ( 'NONE',  ( -14.29746914071049879, 8.314922557960819915, 85.83224293864768129 ) ) ;
#61025=CARTESIAN_POINT ( 'NONE',  ( -16.18388926212238133, -7.379444403734540359, 95.43953151366154941 ) ) ;
#61026=CARTESIAN_POINT ( 'NONE',  ( 13.97604488694527802, 13.89961937509977652, 69.37390960531436690 ) ) ;
#61027=CARTESIAN_POINT ( 'NONE',  ( -19.05341960407611168, -5.049401038298163336, 31.45724293864769550 ) ) ;
#61028=CARTESIAN_POINT ( 'NONE',  ( 8.314922557960818139, 14.29746914071049879, 69.58224293864769550 ) ) ;
#61029=CARTESIAN_POINT ( 'NONE',  ( -18.67979575497178146, -10.72451020669898902, 21.66557627198102409 ) ) ;
#61030=CARTESIAN_POINT ( 'NONE',  ( 0.05219959533936267826, -19.03943276465977164, 85.00109039468567573 ) ) ;
#61031=CARTESIAN_POINT ( 'NONE',  ( -19.02544592524342804, 5.153800228976336051, 101.0405762719810241 ) ) ;
#61032=CARTESIAN_POINT ( 'NONE',  ( -18.67979575497178146, -10.72451020669898902, 76.66557627198103830 ) ) ;
#61033=CARTESIAN_POINT ( 'NONE',  ( -16.53943276465976808, -0.05219959533934237506, 73.75109039468567573 ) ) ;
#61034=CARTESIAN_POINT ( 'NONE',  ( -13.97604488694547520, 13.89961937509957934, 108.1260903946856473 ) ) ;
#61035=CARTESIAN_POINT ( 'NONE',  ( -16.51473224551069308, -9.474510206698971260, 66.66557627198102409 ) ) ;
#61036=CARTESIAN_POINT ( 'NONE',  ( 10.81492255796078972, 18.62759615963270932, 74.58224293864768129 ) ) ;
#61037=CARTESIAN_POINT ( 'NONE',  ( 5.049401038297881783, 19.05341960407617563, 102.2927570613523045 ) ) ;
#61038=CARTESIAN_POINT ( 'NONE',  ( -4.483927247898539470, -16.52544592524342804, 37.29057627198102409 ) ) ;
#61039=CARTESIAN_POINT ( 'NONE',  ( 18.67979575497194134, -10.72451020669871369, 65.83442372801900433 ) ) ;
#61041=CARTESIAN_POINT ( 'NONE',  ( 14.29746914071037800, 8.314922557961029526, 71.66775706135234714 ) ) ;
#61042=CARTESIAN_POINT ( 'NONE',  ( -5.049401038298153566, 19.05341960407611168, 100.2072429386476955 ) ) ;
#61044=LINE ( 'NONE', #155051, #64767 ) ;
#61045=CARTESIAN_POINT ( 'NONE',  ( 4.379528057220092307, 16.55341960407617563, 97.29275706135234714 ) ) ;
#61046=CARTESIAN_POINT ( 'NONE',  ( -14.34966873604972548, 8.224510206698743886, 48.33442372801902565 ) ) ;
#61047=CARTESIAN_POINT ( 'NONE',  ( 0.05219959533909260263, 19.03943276465977164, 54.99890960531435979 ) ) ;
#61048=CARTESIAN_POINT ( 'NONE',  ( 16.46253265017160672, -9.564922557960803928, 73.33224293864769550 ) ) ;
#61049=CARTESIAN_POINT ( 'NONE',  ( -0.05219959533937732626, 21.53943276465977519, 72.50109039468568994 ) ) ;
#61050=CARTESIAN_POINT ( 'NONE',  ( -8.314922557961024197, 14.29746914071037800, 62.91775706135236135 ) ) ;
#61051=CARTESIAN_POINT ( 'NONE',  ( 4.483927247898545687, 16.52544592524342804, 34.79057627198103120 ) ) ;
#61052=CARTESIAN_POINT ( 'NONE',  ( 9.474510206698971260, -16.51473224551069308, 37.91557627198102409 ) ) ;
#61053=CARTESIAN_POINT ( 'NONE',  ( 5.153800228976335163, 19.02544592524342804, 34.79057627198102409 ) ) ;
#61054=CARTESIAN_POINT ( 'NONE',  ( -4.379528057220086978, -16.55341960407618274, 29.79275706135234358 ) ) ;
#61055=CARTESIAN_POINT ( 'NONE',  ( -19.02544592524334988, -5.153800228976617603, 78.95942372801900433 ) ) ;
#61056=CARTESIAN_POINT ( 'NONE',  ( 16.55341960407611168, 4.379528057220329451, 93.95724293864770971 ) ) ;
#61057=CARTESIAN_POINT ( 'NONE',  ( 9.474510206698971260, -16.51473224551069308, 57.91557627198103120 ) ) ;
#61058=CARTESIAN_POINT ( 'NONE',  ( -5.153800228976607833, 19.02544592524334988, 82.70942372801897591 ) ) ;
#61060=CARTESIAN_POINT ( 'NONE',  ( 21.55341960407619695, -5.719274019375665929, 86.04275706135236135 ) ) ;
#61061=CARTESIAN_POINT ( 'NONE',  ( 12.06949235617739724, 12.14591786802326823, 56.87609039468568994 ) ) ;
#61063=CARTESIAN_POINT ( 'NONE',  ( 18.62759615963271287, -10.81492255796078972, 43.33224293864769550 ) ) ;
#61064=CARTESIAN_POINT ( 'NONE',  ( -12.06949235617739369, -12.14591786802326823, 34.37609039468568284 ) ) ;
#61065=CARTESIAN_POINT ( 'NONE',  ( -16.46253265017160317, 9.564922557960807481, 35.83224293864768839 ) ) ;
#61066=CARTESIAN_POINT ( 'NONE',  ( -9.564922557961040184, 16.46253265017147172, 47.91775706135233293 ) ) ;
#61067=CARTESIAN_POINT ( 'NONE',  ( 13.89961937509977652, -13.97604488694527269, 88.12390960531438111 ) ) ;
#61068=CARTESIAN_POINT ( 'NONE',  ( -5.153800228976328057, -19.02544592524343514, 52.29057627198100988 ) ) ;
#61070=CARTESIAN_POINT ( 'NONE',  ( -18.67979575497193778, 10.72451020669871902, 73.33442372801901854 ) ) ;
#61072=CARTESIAN_POINT ( 'NONE',  ( -19.02544592524334988, -5.153800228976617603, 38.95942372801900433 ) ) ;
#61073=CARTESIAN_POINT ( 'NONE',  ( 21.52544592524334988, 5.823673210054432836, 106.4594237280190328 ) ) ;
#61074=CARTESIAN_POINT ( 'NONE',  ( -8.314922557960811034, -14.29746914071050412, 47.08224293864770260 ) ) ;
#61075=CARTESIAN_POINT ( 'NONE',  ( 9.474510206698971260, -16.51473224551069308, 52.91557627198102409 ) ) ;
#61076=CARTESIAN_POINT ( 'NONE',  ( 16.46253265017160672, -9.564922557960803928, 108.3322429386476955 ) ) ;
#61077=CARTESIAN_POINT ( 'NONE',  ( -21.55341960407619339, 5.719274019375674811, 88.54275706135236135 ) ) ;
#61078=CARTESIAN_POINT ( 'NONE',  ( -9.474510206698964154, 16.51473224551069663, 70.41557627198102409 ) ) ;
#61079=CARTESIAN_POINT ( 'NONE',  ( 0.05219959533937995610, -21.53943276465977519, 85.00109039468568994 ) ) ;
#61080=CARTESIAN_POINT ( 'NONE',  ( -5.823673210054116645, -21.52544592524344225, 37.29057627198102409 ) ) ;
#61081=CARTESIAN_POINT ( 'NONE',  ( -18.67979575497193778, 10.72451020669871902, 28.33442372801902209 ) ) ;
#61082=CARTESIAN_POINT ( 'NONE',  ( -19.05341960407617563, 5.049401038297882671, 53.54275706135231871 ) ) ;
#61083=CARTESIAN_POINT ( 'NONE',  ( -19.02544592524342804, 5.153800228976336051, 31.04057627198102409 ) ) ;
#61084=CARTESIAN_POINT ( 'NONE',  ( -16.51473224551069308, -9.474510206698971260, 76.66557627198103830 ) ) ;
#61085=EDGE_CURVE ( 'NONE', #162452, #94244, #32981, .T. ) ;
#61086=CARTESIAN_POINT ( 'NONE',  ( -16.55341960407617563, 4.379528057220093196, 33.54275706135234714 ) ) ;
#61087=CARTESIAN_POINT ( 'NONE',  ( -16.53943276465976808, 0.05219959533911058130, 91.24890960531436690 ) ) ;
#61088=CARTESIAN_POINT ( 'NONE',  ( 5.153800228976335163, 19.02544592524342804, 54.79057627198103120 ) ) ;
#61089=CARTESIAN_POINT ( 'NONE',  ( 21.52544592524344225, -5.823673210054117533, 33.54057627198102409 ) ) ;
#61090=CARTESIAN_POINT ( 'NONE',  ( -5.153800228976607833, 19.02544592524334988, 107.7094237280189759 ) ) ;
#61091=CARTESIAN_POINT ( 'NONE',  ( 21.53943276465977519, 0.05219959533937863772, 21.25109039468567218 ) ) ;
#61092=CARTESIAN_POINT ( 'NONE',  ( -15.80617190586768217, 15.72974639402176855, 73.12609039468567573 ) ) ;
#61093=CARTESIAN_POINT ( 'NONE',  ( -16.53943276465976808, -0.05219959533934237506, 68.75109039468568994 ) ) ;
#61094=CARTESIAN_POINT ( 'NONE',  ( 12.06949235617739724, 12.14591786802326823, 71.87609039468568994 ) ) ;
#61095=CARTESIAN_POINT ( 'NONE',  ( -16.46253265017160317, 9.564922557960807481, 60.83224293864769550 ) ) ;
#61096=CARTESIAN_POINT ( 'NONE',  ( -4.483927247898782831, 16.52544592524335698, 92.70942372801901854 ) ) ;
#61097=CARTESIAN_POINT ( 'NONE',  ( 16.51473224551083163, -9.474510206698727899, 35.83442372801899722 ) ) ;
#61098=CARTESIAN_POINT ( 'NONE',  ( 5.823673210054444382, -21.52544592524334988, 20.20942372801900788 ) ) ;
#61099=CARTESIAN_POINT ( 'NONE',  ( -16.53943276465976808, 0.05219959533911058130, 66.24890960531436690 ) ) ;
#61100=CARTESIAN_POINT ( 'NONE',  ( 9.474510206698971260, -16.51473224551069308, 87.91557627198102409 ) ) ;
#61101=CARTESIAN_POINT ( 'NONE',  ( -4.379528057220086978, -16.55341960407618274, 94.79275706135234714 ) ) ;
#61102=CARTESIAN_POINT ( 'NONE',  ( -5.823673210054431948, 21.52544592524334988, 62.70942372801902565 ) ) ;
#61103=CARTESIAN_POINT ( 'NONE',  ( 8.314922557961029526, -14.29746914071037800, 20.41775706135234714 ) ) ;
#61104=CARTESIAN_POINT ( 'NONE',  ( -18.67979575497178146, -10.72451020669898902, 106.6655762719810383 ) ) ;
#61105=CARTESIAN_POINT ( 'NONE',  ( 14.29746914071049879, -8.314922557960816363, 58.33224293864768839 ) ) ;
#61107=CARTESIAN_POINT ( 'NONE',  ( -15.72974639402197994, 15.80617190586746368, 90.62390960531436690 ) ) ;
#61108=CARTESIAN_POINT ( 'NONE',  ( -8.224510206698948167, 14.34966873604960824, 45.41557627198103830 ) ) ;
#61111=CARTESIAN_POINT ( 'NONE',  ( -10.81492255796105439, 18.62759615963255655, 22.91775706135235069 ) ) ;
#61112=CARTESIAN_POINT ( 'NONE',  ( -18.67979575497178146, -10.72451020669898902, 21.66557627198102409 ) ) ;
#61113=CARTESIAN_POINT ( 'NONE',  ( 21.52544592524334988, 5.823673210054432836, 31.45942372801901854 ) ) ;
#61114=CARTESIAN_POINT ( 'NONE',  ( -4.483927247898539470, -16.52544592524342804, 47.29057627198103120 ) ) ;
#61115=CARTESIAN_POINT ( 'NONE',  ( 5.049401038298161559, -19.05341960407611168, 62.70724293864769550 ) ) ;
#61116=CARTESIAN_POINT ( 'NONE',  ( 13.97604488694548053, -13.89961937509957401, 65.62609039468567573 ) ) ;
#61117=CARTESIAN_POINT ( 'NONE',  ( -5.049401038298153566, 19.05341960407611168, 100.2072429386476955 ) ) ;
#61118=CARTESIAN_POINT ( 'NONE',  ( 21.52544592524344225, -5.823673210054117533, 43.54057627198103830 ) ) ;
#61120=CARTESIAN_POINT ( 'NONE',  ( -13.89961937509977652, 13.97604488694528158, 55.62390960531434558 ) ) ;
#61121=CARTESIAN_POINT ( 'NONE',  ( -16.53943276465976808, -0.05219959533934237506, 38.75109039468567573 ) ) ;
#61122=CARTESIAN_POINT ( 'NONE',  ( 5.049401038297881783, 19.05341960407617563, 62.29275706135234003 ) ) ;
#61123=CARTESIAN_POINT ( 'NONE',  ( -18.62759615963255300, -10.81492255796106328, 19.16775706135234714 ) ) ;
#61125=CARTESIAN_POINT ( 'NONE',  ( -0.05219959533910754901, -16.53943276465976808, 47.49890960531435979 ) ) ;
#61126=CARTESIAN_POINT ( 'NONE',  ( 5.153800228976335163, 19.02544592524342804, 84.79057627198099567 ) ) ;
#61127=CARTESIAN_POINT ( 'NONE',  ( 18.67979575497178502, 10.72451020669898547, 79.16557627198103830 ) ) ;
#61128=CARTESIAN_POINT ( 'NONE',  ( 18.62759615963271287, -10.81492255796078972, 103.3322429386476955 ) ) ;
#61129=CARTESIAN_POINT ( 'NONE',  ( -14.34966873604972548, 8.224510206698743886, 33.33442372801900433 ) ) ;
#61130=CARTESIAN_POINT ( 'NONE',  ( 10.81492255796078972, 18.62759615963270932, 39.58224293864769550 ) ) ;
#61131=CARTESIAN_POINT ( 'NONE',  ( 5.719274019375673035, 21.55341960407619339, 97.29275706135234714 ) ) ;
#61132=CARTESIAN_POINT ( 'NONE',  ( 19.02544592524343514, -5.153800228976328945, 93.54057627198102409 ) ) ;
#61134=CARTESIAN_POINT ( 'NONE',  ( 9.474510206698971260, -16.51473224551069308, 47.91557627198102409 ) ) ;
#61135=CARTESIAN_POINT ( 'NONE',  ( -5.153800228976328057, -19.02544592524343514, 97.29057627198099567 ) ) ;
#61136=CARTESIAN_POINT ( 'NONE',  ( -9.564922557960796823, -16.46253265017161027, 72.08224293864770971 ) ) ;
#61137=CARTESIAN_POINT ( 'NONE',  ( -14.29746914071037622, -8.314922557961029526, 29.16775706135234003 ) ) ;
#61138=CARTESIAN_POINT ( 'NONE',  ( 17.50000000000015987, 3.292511757969722286, 32.43479729789459753 ) ) ;
#61139=CARTESIAN_POINT ( 'NONE',  ( -5.153800228976607833, 19.02544592524334988, 52.70942372801900433 ) ) ;
#61140=CARTESIAN_POINT ( 'NONE',  ( 5.719274019375673035, 21.55341960407619339, 107.2927570613523471 ) ) ;
#61141=CARTESIAN_POINT ( 'NONE',  ( 18.62759615963271287, -10.81492255796078972, 38.33224293864768839 ) ) ;
#61142=CARTESIAN_POINT ( 'NONE',  ( 0.05219959533934541429, -16.53943276465976808, 110.0010903946856757 ) ) ;
#61144=CARTESIAN_POINT ( 'NONE',  ( 13.89961937509957401, 13.97604488694547697, 66.87609039468567573 ) ) ;
#61145=CARTESIAN_POINT ( 'NONE',  ( 5.153800228976615827, -19.02544592524334988, 25.20942372801900433 ) ) ;
#61147=CARTESIAN_POINT ( 'NONE',  ( -13.89961937509977652, 13.97604488694528158, 40.62390960531435979 ) ) ;
#61148=CARTESIAN_POINT ( 'NONE',  ( -16.55341960407611168, -4.379528057220339221, 31.45724293864769550 ) ) ;
#61149=CARTESIAN_POINT ( 'NONE',  ( -5.153800228976328057, -19.02544592524343514, 27.29057627198103120 ) ) ;
#61150=CARTESIAN_POINT ( 'NONE',  ( -14.34966873604960291, -8.224510206698953496, 31.66557627198102054 ) ) ;
#61152=CARTESIAN_POINT ( 'NONE',  ( 14.34966873604972726, -8.224510206698740333, 95.83442372801903275 ) ) ;
#61153=CARTESIAN_POINT ( 'NONE',  ( -9.474510206698964154, 16.51473224551069663, 35.41557627198102409 ) ) ;
#61154=CARTESIAN_POINT ( 'NONE',  ( -5.719274019375665041, -21.55341960407619695, 104.7927570613523898 ) ) ;
#61155=CARTESIAN_POINT ( 'NONE',  ( -14.29746914071037622, -8.314922557961029526, 24.16775706135235424 ) ) ;
#61156=CARTESIAN_POINT ( 'NONE',  ( -18.67979575497193778, 10.72451020669871902, 73.33442372801901854 ) ) ;
#61158=CARTESIAN_POINT ( 'NONE',  ( -13.89961937509957401, -13.97604488694547875, 49.37609039468567573 ) ) ;
#61159=CARTESIAN_POINT ( 'NONE',  ( -19.05341960407611168, -5.049401038298163336, 96.45724293864769550 ) ) ;
#61160=CARTESIAN_POINT ( 'NONE',  ( 13.97604488694527802, 13.89961937509977652, 84.37390960531433848 ) ) ;
#61162=CARTESIAN_POINT ( 'NONE',  ( -21.55341960407610458, -5.719274019375992779, 106.4572429386477097 ) ) ;
#61164=CARTESIAN_POINT ( 'NONE',  ( -16.55341960407611168, -4.379528057220339221, 71.45724293864769550 ) ) ;
#61165=CARTESIAN_POINT ( 'NONE',  ( -21.55341960407610458, -5.719274019375992779, 56.45724293864768839 ) ) ;
#61166=CARTESIAN_POINT ( 'NONE',  ( 9.564922557960805705, 16.46253265017160317, 64.58224293864769550 ) ) ;
#61167=CARTESIAN_POINT ( 'NONE',  ( -5.823673210054116645, -21.52544592524344225, 97.29057627198105251 ) ) ;
#61168=CARTESIAN_POINT ( 'NONE',  ( 16.55341960407618274, -4.379528057220086978, 91.04275706135236135 ) ) ;
#61169=ORIENTED_EDGE ( 'NONE', *, *, #65499, .T. ) ;
#61170=CARTESIAN_POINT ( 'NONE',  ( -9.564922557960796823, -16.46253265017161027, 67.08224293864769550 ) ) ;
#61171=CARTESIAN_POINT ( 'NONE',  ( 12.14591786802309770, 12.06949235617756955, 89.37390960531435269 ) ) ;
#61173=CARTESIAN_POINT ( 'NONE',  ( -16.51473224551069308, -9.474510206698971260, 56.66557627198103120 ) ) ;
#61174=CARTESIAN_POINT ( 'NONE',  ( -19.05341960407617563, 5.049401038297882671, 83.54275706135233293 ) ) ;
#61175=CARTESIAN_POINT ( 'NONE',  ( 8.224510206698953496, -14.34966873604960469, 77.91557627198102409 ) ) ;
#61176=CARTESIAN_POINT ( 'NONE',  ( 0.05219959533937995610, -21.53943276465977519, 55.00109039468568284 ) ) ;
#61177=CARTESIAN_POINT ( 'NONE',  ( 9.564922557960805705, 16.46253265017160317, 29.58224293864769550 ) ) ;
#61178=CARTESIAN_POINT ( 'NONE',  ( 10.72451020669898902, -18.67979575497178502, 102.9155762719810383 ) ) ;
#61179=CARTESIAN_POINT ( 'NONE',  ( -12.06949235617756955, 12.14591786802309770, 85.62390960531436690 ) ) ;
#61181=CARTESIAN_POINT ( 'NONE',  ( -16.51473224551069308, -9.474510206698971260, 56.66557627198103120 ) ) ;
#61183=CARTESIAN_POINT ( 'NONE',  ( 19.03943276465977164, 0.05219959533936151252, 91.25109039468566152 ) ) ;
#61184=CARTESIAN_POINT ( 'NONE',  ( -16.51473224551069308, -9.474510206698971260, 106.6655762719810383 ) ) ;
#61185=CARTESIAN_POINT ( 'NONE',  ( -21.55341960407619339, 5.719274019375674811, 38.54275706135234714 ) ) ;
#61186=CARTESIAN_POINT ( 'NONE',  ( -9.474510206698964154, 16.51473224551069663, 85.41557627198102409 ) ) ;
#61187=CARTESIAN_POINT ( 'NONE',  ( -9.474510206698720793, -16.51473224551083518, 64.58442372801900433 ) ) ;
#61188=CARTESIAN_POINT ( 'NONE',  ( -5.153800228976328057, -19.02544592524343514, 57.29057627198103120 ) ) ;
#61189=CARTESIAN_POINT ( 'NONE',  ( 8.314922557960818139, 14.29746914071049879, 79.58224293864769550 ) ) ;
#61190=CARTESIAN_POINT ( 'NONE',  ( 12.06949235617757843, -12.14591786802309237, 63.12390960531435979 ) ) ;
#61191=CARTESIAN_POINT ( 'NONE',  ( 9.474510206698971260, -16.51473224551069308, 87.91557627198102409 ) ) ;
#61192=CARTESIAN_POINT ( 'NONE',  ( 21.53943276465977519, -0.05219959533907433946, 98.74890960531438111 ) ) ;
#61193=CARTESIAN_POINT ( 'NONE',  ( 19.03943276465977164, -0.05219959533909143690, 88.74890960531436690 ) ) ;
#61194=CARTESIAN_POINT ( 'NONE',  ( 13.89961937509957401, 13.97604488694547697, 31.87609039468566863 ) ) ;
#61195=CARTESIAN_POINT ( 'NONE',  ( 9.474510206698971260, -16.51473224551069308, 42.91557627198103120 ) ) ;
#61196=CARTESIAN_POINT ( 'NONE',  ( -8.314922557960811034, -14.29746914071050412, 27.08224293864769550 ) ) ;
#61197=CARTESIAN_POINT ( 'NONE',  ( -16.52544592524342804, 4.483927247898546575, 116.0405762719810383 ) ) ;
#61199=CARTESIAN_POINT ( 'NONE',  ( 5.823673210054444382, -21.52544592524334988, 50.20942372801901854 ) ) ;
#61200=CARTESIAN_POINT ( 'NONE',  ( -13.97604488694547697, 13.89961937509957934, 68.12609039468563310 ) ) ;
#61201=CARTESIAN_POINT ( 'NONE',  ( 16.53943276465976808, -0.05219959533910856209, 33.74890960531436690 ) ) ;
#61202=CARTESIAN_POINT ( 'NONE',  ( -18.67979575497178146, -10.72451020669898902, 86.66557627198102409 ) ) ;
#61203=CARTESIAN_POINT ( 'NONE',  ( 0.05219959533909260263, 19.03943276465977164, 109.9989096053143669 ) ) ;
#61204=CARTESIAN_POINT ( 'NONE',  ( -12.06949235617756955, 12.14591786802309770, 75.62390960531439532 ) ) ;
#61205=CARTESIAN_POINT ( 'NONE',  ( -16.51473224551069308, -9.474510206698971260, 31.66557627198102054 ) ) ;
#61206=CARTESIAN_POINT ( 'NONE',  ( -13.97604488694547697, 13.89961937509957934, 33.12609039468566863 ) ) ;
#61207=CARTESIAN_POINT ( 'NONE',  ( -8.314922557961024197, 14.29746914071037800, 107.9177570613523471 ) ) ;
#61208=CARTESIAN_POINT ( 'NONE',  ( -16.53943276465976808, -0.05219959533934237506, 53.75109039468568994 ) ) ;
#61209=CARTESIAN_POINT ( 'NONE',  ( -15.72974639402197994, 15.80617190586746368, 30.62390960531436335 ) ) ;
#61210=CARTESIAN_POINT ( 'NONE',  ( 0.05219959533937995610, -21.53943276465977519, 105.0010903946856757 ) ) ;
#61211=CARTESIAN_POINT ( 'NONE',  ( 0.05219959533909260263, 19.03943276465977164, 74.99890960531435269 ) ) ;
#61212=CARTESIAN_POINT ( 'NONE',  ( -4.379528057220086978, -16.55341960407618274, 74.79275706135234714 ) ) ;
#61213=CARTESIAN_POINT ( 'NONE',  ( -19.05341960407611168, -5.049401038298163336, 21.45724293864768839 ) ) ;
#61214=CARTESIAN_POINT ( 'NONE',  ( 12.06949235617757843, -12.14591786802309237, 28.12390960531435979 ) ) ;
#61215=CARTESIAN_POINT ( 'NONE',  ( -0.05219959533909027116, -19.03943276465977164, 102.4989096053143669 ) ) ;
#61216=CARTESIAN_POINT ( 'NONE',  ( -19.03943276465977164, 0.05219959533909376836, 91.24890960531436690 ) ) ;
#61217=CARTESIAN_POINT ( 'NONE',  ( -5.153800228976328057, -19.02544592524343514, 107.2905762719810383 ) ) ;
#61219=CARTESIAN_POINT ( 'NONE',  ( 12.06949235617757843, -12.14591786802309237, 63.12390960531435979 ) ) ;
#61220=CARTESIAN_POINT ( 'NONE',  ( -14.29746914071049879, 8.314922557960819915, 30.83224293864770260 ) ) ;
#61222=CARTESIAN_POINT ( 'NONE',  ( 16.52544592524342804, -4.483927247898539470, 48.54057627198103120 ) ) ;
#61223=CARTESIAN_POINT ( 'NONE',  ( -8.314922557961024197, 14.29746914071037800, 42.91775706135235424 ) ) ;
#61225=CARTESIAN_POINT ( 'NONE',  ( 0.05219959533936267826, -19.03943276465977164, 50.00109039468566863 ) ) ;
#61226=CARTESIAN_POINT ( 'NONE',  ( -5.153800228976328057, -19.02544592524343514, 87.29057627198103830 ) ) ;
#61227=CARTESIAN_POINT ( 'NONE',  ( -9.474510206698720793, -16.51473224551083518, 69.58442372801901854 ) ) ;
#61229=CARTESIAN_POINT ( 'NONE',  ( -5.153800228976607833, 19.02544592524334988, 57.70942372801899012 ) ) ;
#61230=CARTESIAN_POINT ( 'NONE',  ( 13.89961937509957401, 13.97604488694547697, 91.87609039468567573 ) ) ;
#61231=CARTESIAN_POINT ( 'NONE',  ( -8.314922557961024197, 14.29746914071037800, 87.91775706135234714 ) ) ;
#61233=CARTESIAN_POINT ( 'NONE',  ( 9.564922557960805705, 16.46253265017160317, 29.58224293864769550 ) ) ;
#61234=CARTESIAN_POINT ( 'NONE',  ( -18.62759615963270932, 10.81492255796079327, 25.83224293864769194 ) ) ;
#61235=CARTESIAN_POINT ( 'NONE',  ( 21.53943276465977519, 0.05219959533937863772, 36.25109039468567573 ) ) ;
#61236=CARTESIAN_POINT ( 'NONE',  ( -13.89961937509957401, -13.97604488694547875, 104.3760903946856757 ) ) ;
#61237=CARTESIAN_POINT ( 'NONE',  ( 17.50000000000000000, 5.499999999999997335, 23.78230962303566542 ) ) ;
#61238=CARTESIAN_POINT ( 'NONE',  ( -9.474510206698964154, 16.51473224551069663, 65.41557627198102409 ) ) ;
#61239=CARTESIAN_POINT ( 'NONE',  ( 16.46253265017160672, -9.564922557960803928, 98.33224293864769550 ) ) ;
#61240=CARTESIAN_POINT ( 'NONE',  ( 0.05219959533910956823, 16.53943276465976808, 54.99890960531435269 ) ) ;
#61241=CARTESIAN_POINT ( 'NONE',  ( -13.89961937509977652, 13.97604488694528158, 60.62390960531436690 ) ) ;
#61242=CARTESIAN_POINT ( 'NONE',  ( 16.51473224551069308, 9.474510206698969483, 69.16557627198102409 ) ) ;
#61243=CARTESIAN_POINT ( 'NONE',  ( 19.05341960407617918, -5.049401038297876454, 76.04275706135230450 ) ) ;
#61244=CARTESIAN_POINT ( 'NONE',  ( -0.05219959533907301413, -21.53943276465977519, 57.49890960531435979 ) ) ;
#61245=CARTESIAN_POINT ( 'NONE',  ( -4.379528057220328563, 16.55341960407611168, 115.2072429386476955 ) ) ;
#61246=CARTESIAN_POINT ( 'NONE',  ( 16.46253265017146816, 9.564922557961045513, 41.66775706135234003 ) ) ;
#61247=CARTESIAN_POINT ( 'NONE',  ( -5.049401038298153566, 19.05341960407611168, 80.20724293864769550 ) ) ;
#61248=EDGE_CURVE ( 'NONE', #83484, #91305, #49415, .T. ) ;
#61249=CARTESIAN_POINT ( 'NONE',  ( -15.72974639402197994, 15.80617190586746368, 70.62390960531436690 ) ) ;
#61250=CARTESIAN_POINT ( 'NONE',  ( -16.53943276465976808, 0.05219959533911058130, 81.24890960531436690 ) ) ;
#61251=CARTESIAN_POINT ( 'NONE',  ( -13.89961937509957401, -13.97604488694547875, 29.37609039468565797 ) ) ;
#61252=CARTESIAN_POINT ( 'NONE',  ( -18.67979575497178146, -10.72451020669898902, 76.66557627198103830 ) ) ;
#61253=CARTESIAN_POINT ( 'NONE',  ( 21.53943276465977519, -0.05219959533907433946, 58.74890960531436690 ) ) ;
#61254=CARTESIAN_POINT ( 'NONE',  ( -5.823673210054116645, -21.52544592524344225, 37.29057627198102409 ) ) ;
#61255=CARTESIAN_POINT ( 'NONE',  ( 15.80617190586769283, -15.72974639402175789, 95.62609039468568994 ) ) ;
#61256=CARTESIAN_POINT ( 'NONE',  ( -19.05341960407611168, -5.049401038298163336, 61.45724293864769550 ) ) ;
#61257=CARTESIAN_POINT ( 'NONE',  ( 0.05219959533909260263, 19.03943276465977164, 24.99890960531435269 ) ) ;
#61258=CARTESIAN_POINT ( 'NONE',  ( 18.62759615963255655, 10.81492255796105972, 26.66775706135235424 ) ) ;
#61259=CARTESIAN_POINT ( 'NONE',  ( -17.49999999999999645, -5.499999999999992895, 49.20309617465830598 ) ) ;
#61260=CARTESIAN_POINT ( 'NONE',  ( -10.72451020669870658, -18.67979575497194134, 44.58442372801901854 ) ) ;
#61261=CARTESIAN_POINT ( 'NONE',  ( 19.03943276465977164, -0.05219959533909143690, 33.74890960531435979 ) ) ;
#61262=CARTESIAN_POINT ( 'NONE',  ( 10.81492255796078972, 18.62759615963270932, 104.5822429386477097 ) ) ;
#61263=CARTESIAN_POINT ( 'NONE',  ( 13.89961937509957401, 13.97604488694547697, 41.87609039468566152 ) ) ;
#61264=CARTESIAN_POINT ( 'NONE',  ( -13.97604488694527625, -13.89961937509977652, 36.87390960531436690 ) ) ;
#61267=CARTESIAN_POINT ( 'NONE',  ( 0.05219959533934541429, -16.53943276465976808, 55.00109039468568284 ) ) ;
#61268=CARTESIAN_POINT ( 'NONE',  ( 16.51473224551069308, 9.474510206698969483, 24.16557627198102765 ) ) ;
#61270=CARTESIAN_POINT ( 'NONE',  ( -9.564922557960796823, -16.46253265017161027, 87.08224293864769550 ) ) ;
#61271=CARTESIAN_POINT ( 'NONE',  ( -16.55341960407611168, -4.379528057220339221, 101.4572429386476955 ) ) ;
#61272=CARTESIAN_POINT ( 'NONE',  ( 10.72451020669898902, -18.67979575497178502, 57.91557627198103120 ) ) ;
#61273=CARTESIAN_POINT ( 'NONE',  ( -0.05219959533934338120, 16.53943276465976808, 47.50109039468568994 ) ) ;
#61274=CARTESIAN_POINT ( 'NONE',  ( -15.80617190586768217, 15.72974639402176855, 103.1260903946856757 ) ) ;
#61275=CARTESIAN_POINT ( 'NONE',  ( 9.564922557960805705, 16.46253265017160317, 24.58224293864769194 ) ) ;
#61276=CARTESIAN_POINT ( 'NONE',  ( -0.05219959533910754901, -16.53943276465976808, 22.49890960531436335 ) ) ;
#61277=CARTESIAN_POINT ( 'NONE',  ( -0.05219959533910754901, -16.53943276465976808, 57.49890960531435979 ) ) ;
#61279=CARTESIAN_POINT ( 'NONE',  ( 13.89961937509977652, -13.97604488694527269, 53.12390960531434558 ) ) ;
#61280=CARTESIAN_POINT ( 'NONE',  ( 10.81492255796106328, -18.62759615963255655, 90.41775706135236135 ) ) ;
#61281=CARTESIAN_POINT ( 'NONE',  ( 15.80617190586769283, -15.72974639402175789, 25.62609039468567929 ) ) ;
#61282=CARTESIAN_POINT ( 'NONE',  ( -5.719274019375665041, -21.55341960407619695, 69.79275706135234714 ) ) ;
#61283=CARTESIAN_POINT ( 'NONE',  ( 4.483927247898790824, -16.52544592524335698, 55.20942372801902565 ) ) ;
#61284=CARTESIAN_POINT ( 'NONE',  ( -4.483927247898782831, 16.52544592524335698, 27.70942372801901854 ) ) ;
#61285=CARTESIAN_POINT ( 'NONE',  ( 16.53943276465976808, -0.05219959533910856209, 83.74890960531435269 ) ) ;
#61286=CARTESIAN_POINT ( 'NONE',  ( -10.81492255796105439, 18.62759615963255655, 102.9177570613523756 ) ) ;
#61287=CARTESIAN_POINT ( 'NONE',  ( -0.05219959533910754901, -16.53943276465976808, 22.49890960531436335 ) ) ;
#61289=CARTESIAN_POINT ( 'NONE',  ( 8.314922557961029526, -14.29746914071037800, 45.41775706135234003 ) ) ;
#61290=CARTESIAN_POINT ( 'NONE',  ( -16.53943276465976808, 0.05219959533911058130, 46.24890960531435979 ) ) ;
#61291=CARTESIAN_POINT ( 'NONE',  ( -16.52544592524335698, -4.483927247898792601, 83.95942372801900433 ) ) ;
#61292=CARTESIAN_POINT ( 'NONE',  ( 19.02544592524343514, -5.153800228976328945, 103.5405762719809957 ) ) ;
#61293=CARTESIAN_POINT ( 'NONE',  ( -13.89961937509977652, 13.97604488694528158, 110.6239096053143243 ) ) ;
#61294=CARTESIAN_POINT ( 'NONE',  ( -18.62759615963255300, -10.81492255796106328, 94.16775706135237556 ) ) ;
#61295=CARTESIAN_POINT ( 'NONE',  ( 8.224510206698742110, 14.34966873604972548, 102.0844237280190185 ) ) ;
#61296=CARTESIAN_POINT ( 'NONE',  ( 16.52544592524342804, -4.483927247898539470, 78.54057627198103830 ) ) ;
#61297=CARTESIAN_POINT ( 'NONE',  ( -0.05219959533909027116, -19.03943276465977164, 82.49890960531436690 ) ) ;
#61298=ORIENTED_EDGE ( 'NONE', *, *, #1307, .T. ) ;
#61299=CARTESIAN_POINT ( 'NONE',  ( 16.53943276465976808, 0.05219959533934440121, 36.25109039468567573 ) ) ;
#61300=CARTESIAN_POINT ( 'NONE',  ( 9.564922557960805705, 16.46253265017160317, 39.58224293864768839 ) ) ;
#61301=CARTESIAN_POINT ( 'NONE',  ( 13.89961937509977652, -13.97604488694527269, 93.12390960531436690 ) ) ;
#61302=CARTESIAN_POINT ( 'NONE',  ( -4.379528057220086978, -16.55341960407618274, 34.79275706135235424 ) ) ;
#61304=CARTESIAN_POINT ( 'NONE',  ( 13.97604488694548053, -13.89961937509957401, 35.62609039468567573 ) ) ;
#61305=CARTESIAN_POINT ( 'NONE',  ( -12.14591786802326823, 12.06949235617739902, 93.12609039468568994 ) ) ;
#61306=CARTESIAN_POINT ( 'NONE',  ( 13.97604488694527802, 13.89961937509977652, 34.37390960531436690 ) ) ;
#61307=CARTESIAN_POINT ( 'NONE',  ( -12.06949235617739369, -12.14591786802326823, 84.37609039468570415 ) ) ;
#61308=CARTESIAN_POINT ( 'NONE',  ( 12.14591786802327356, -12.06949235617739191, 70.62609039468567573 ) ) ;
#61309=CARTESIAN_POINT ( 'NONE',  ( -9.564922557961040184, 16.46253265017147172, 82.91775706135233293 ) ) ;
#61310=CARTESIAN_POINT ( 'NONE',  ( -16.51473224551082808, 9.474510206698731452, 28.33442372801900433 ) ) ;
#61311=CARTESIAN_POINT ( 'NONE',  ( 5.049401038298161559, -19.05341960407611168, 52.70724293864767418 ) ) ;
#61312=CARTESIAN_POINT ( 'NONE',  ( 4.483927247898545687, 16.52544592524342804, 89.79057627198103830 ) ) ;
#61313=CARTESIAN_POINT ( 'NONE',  ( -19.05341960407617563, 5.049401038297882671, 58.54275706135234003 ) ) ;
#61314=CARTESIAN_POINT ( 'NONE',  ( 10.81492255796078972, 18.62759615963270932, 49.58224293864769550 ) ) ;
#61315=CARTESIAN_POINT ( 'NONE',  ( 9.564922557961047289, -16.46253265017146816, 25.41775706135234003 ) ) ;
#61316=CARTESIAN_POINT ( 'NONE',  ( 9.564922557960805705, 16.46253265017160317, 104.5822429386476955 ) ) ;
#61317=CARTESIAN_POINT ( 'NONE',  ( -5.823673210054116645, -21.52544592524344225, 77.29057627198102409 ) ) ;
#61318=CARTESIAN_POINT ( 'NONE',  ( 13.89961937509977652, -13.97604488694527269, 108.1239096053143669 ) ) ;
#61319=CARTESIAN_POINT ( 'NONE',  ( 5.153800228976615827, -19.02544592524334988, 95.20942372801897591 ) ) ;
#61321=CARTESIAN_POINT ( 'NONE',  ( 19.05341960407617918, -5.049401038297876454, 111.0427570613523329 ) ) ;
#61322=CARTESIAN_POINT ( 'NONE',  ( 13.97604488694527802, 13.89961937509977652, 39.37390960531435269 ) ) ;
#61323=CARTESIAN_POINT ( 'NONE',  ( 9.564922557960805705, 16.46253265017160317, 99.58224293864770971 ) ) ;
#61324=CARTESIAN_POINT ( 'NONE',  ( 18.62759615963271287, -10.81492255796078972, 78.33224293864770971 ) ) ;
#61325=CARTESIAN_POINT ( 'NONE',  ( 8.314922557961029526, -14.29746914071037800, 55.41775706135234714 ) ) ;
#61326=CARTESIAN_POINT ( 'NONE',  ( 0.05219959533937995610, -21.53943276465977519, 60.00109039468568284 ) ) ;
#61327=CARTESIAN_POINT ( 'NONE',  ( 5.153800228976615827, -19.02544592524334988, 110.2094237280189901 ) ) ;
#61328=CARTESIAN_POINT ( 'NONE',  ( -16.46253265017146816, -9.564922557961047289, 19.16775706135233293 ) ) ;
#61329=CARTESIAN_POINT ( 'NONE',  ( -14.29746914071037622, -8.314922557961029526, 109.1677570613523613 ) ) ;
#61330=CARTESIAN_POINT ( 'NONE',  ( -21.53943276465977519, 0.05219959533907696930, 106.2489096053143811 ) ) ;
#61331=CARTESIAN_POINT ( 'NONE',  ( -12.14591786802309592, -12.06949235617757132, 41.87390960531435979 ) ) ;
#61332=CARTESIAN_POINT ( 'NONE',  ( -16.46253265017146816, -9.564922557961047289, 79.16775706135234714 ) ) ;
#61333=CARTESIAN_POINT ( 'NONE',  ( -0.05219959533937732626, 21.53943276465977519, 62.50109039468568284 ) ) ;
#61334=CARTESIAN_POINT ( 'NONE',  ( -16.46253265017146816, -9.564922557961047289, 39.16775706135234003 ) ) ;
#61335=CARTESIAN_POINT ( 'NONE',  ( 8.224510206698953496, -14.34966873604960469, 107.9155762719810241 ) ) ;
#61336=CARTESIAN_POINT ( 'NONE',  ( 0.05219959533907565091, 21.53943276465977519, 34.99890960531435979 ) ) ;
#61337=CARTESIAN_POINT ( 'NONE',  ( -4.483927247898539470, -16.52544592524342804, 32.29057627198102409 ) ) ;
#61338=CARTESIAN_POINT ( 'NONE',  ( -0.05219959533937732626, 21.53943276465977519, 97.50109039468567573 ) ) ;
#61339=CARTESIAN_POINT ( 'NONE',  ( 12.14591786802327356, -12.06949235617739191, 65.62609039468568994 ) ) ;
#61340=CARTESIAN_POINT ( 'NONE',  ( 14.29746914071049879, -8.314922557960816363, 23.33224293864769194 ) ) ;
#61341=CARTESIAN_POINT ( 'NONE',  ( -21.55341960407619339, 5.719274019375674811, 58.54275706135235424 ) ) ;
#61342=CARTESIAN_POINT ( 'NONE',  ( 21.52544592524334988, 5.823673210054432836, 51.45942372801901854 ) ) ;
#61343=ORIENTED_EDGE ( 'NONE', *, *, #46412, .F. ) ;
#61344=CARTESIAN_POINT ( 'NONE',  ( 19.02544592524343514, -5.153800228976328945, 28.54057627198102409 ) ) ;
#61345=CARTESIAN_POINT ( 'NONE',  ( -5.823673210054431948, 21.52544592524334988, 42.70942372801901854 ) ) ;
#61346=CARTESIAN_POINT ( 'NONE',  ( 8.224510206698953496, -14.34966873604960469, 107.9155762719810241 ) ) ;
#61347=CARTESIAN_POINT ( 'NONE',  ( -16.46253265017160317, 9.564922557960807481, 35.83224293864768839 ) ) ;
#61348=CARTESIAN_POINT ( 'NONE',  ( -4.379528057220328563, 16.55341960407611168, 80.20724293864769550 ) ) ;
#61349=CARTESIAN_POINT ( 'NONE',  ( 19.03943276465977164, -0.05219959533909143690, 73.74890960531435269 ) ) ;
#61350=CARTESIAN_POINT ( 'NONE',  ( 8.314922557960818139, 14.29746914071049879, 24.58224293864768839 ) ) ;
#61351=CARTESIAN_POINT ( 'NONE',  ( 21.53943276465977519, -0.05219959533907433946, 58.74890960531436690 ) ) ;
#61352=CARTESIAN_POINT ( 'NONE',  ( 4.379528057220339221, -16.55341960407611168, 92.70724293864770971 ) ) ;
#61353=CARTESIAN_POINT ( 'NONE',  ( 5.719274019375991003, -21.55341960407610458, 112.7072429386476955 ) ) ;
#61354=CARTESIAN_POINT ( 'NONE',  ( -19.02544592524342804, 5.153800228976336051, 101.0405762719810241 ) ) ;
#61355=CARTESIAN_POINT ( 'NONE',  ( -0.05219959533909027116, -19.03943276465977164, 67.49890960531436690 ) ) ;
#61356=CARTESIAN_POINT ( 'NONE',  ( -0.05219959533936034679, 19.03943276465977164, 107.5010903946856615 ) ) ;
#61357=CARTESIAN_POINT ( 'NONE',  ( 0.05219959533907565091, 21.53943276465977519, 59.99890960531436690 ) ) ;
#61358=CARTESIAN_POINT ( 'NONE',  ( -21.53943276465977519, -0.05219959533937600094, 78.75109039468568994 ) ) ;
#61359=CARTESIAN_POINT ( 'NONE',  ( -16.46253265017160317, 9.564922557960807481, 65.83224293864769550 ) ) ;
#61360=CARTESIAN_POINT ( 'NONE',  ( -19.05341960407611168, -5.049401038298163336, 101.4572429386476955 ) ) ;
#61361=CARTESIAN_POINT ( 'NONE',  ( 12.14591786802327356, -12.06949235617739191, 75.62609039468567573 ) ) ;
#61362=CARTESIAN_POINT ( 'NONE',  ( -21.55341960407619339, 5.719274019375674811, 58.54275706135235424 ) ) ;
#61363=CARTESIAN_POINT ( 'NONE',  ( 10.72451020669871369, 18.67979575497193778, 87.08442372801901854 ) ) ;
#61364=CARTESIAN_POINT ( 'NONE',  ( -15.80617190586745835, -15.72974639402198527, 106.8739096053143811 ) ) ;
#61365=CARTESIAN_POINT ( 'NONE',  ( -16.52544592524335698, -4.483927247898792601, 83.95942372801900433 ) ) ;
#61366=CARTESIAN_POINT ( 'NONE',  ( -21.53943276465977519, 0.05219959533907696930, 81.24890960531436690 ) ) ;
#61367=CARTESIAN_POINT ( 'NONE',  ( 9.564922557961047289, -16.46253265017146816, 45.41775706135232582 ) ) ;
#61368=CARTESIAN_POINT ( 'NONE',  ( 18.62759615963271287, -10.81492255796078972, 43.33224293864769550 ) ) ;
#61369=CARTESIAN_POINT ( 'NONE',  ( -13.97604488694527625, -13.89961937509977652, 86.87390960531436690 ) ) ;
#61370=CARTESIAN_POINT ( 'NONE',  ( 12.06949235617757843, -12.14591786802309237, 28.12390960531435979 ) ) ;
#61371=CARTESIAN_POINT ( 'NONE',  ( -17.05587630539787369, 6.762274262135695935, 65.74180309037313918 ) ) ;
#61372=CARTESIAN_POINT ( 'NONE',  ( -5.153800228976328057, -19.02544592524343514, 112.2905762719810099 ) ) ;
#61373=CARTESIAN_POINT ( 'NONE',  ( -18.39639308325438805, -5.499999999999988454, 81.48252246182198633 ) ) ;
#61374=CARTESIAN_POINT ( 'NONE',  ( -19.03943276465977164, -0.05219959533935918106, 88.75109039468567573 ) ) ;
#61375=CARTESIAN_POINT ( 'NONE',  ( -18.67979575497178146, -10.72451020669898902, 71.66557627198100988 ) ) ;
#61376=CARTESIAN_POINT ( 'NONE',  ( -4.379528057220328563, 16.55341960407611168, 55.20724293864770260 ) ) ;
#61377=CARTESIAN_POINT ( 'NONE',  ( 12.06949235617739724, 12.14591786802326823, 21.87609039468567573 ) ) ;
#61378=CARTESIAN_POINT ( 'NONE',  ( -13.89961937509977652, 13.97604488694528158, 35.62390960531435269 ) ) ;
#61379=CARTESIAN_POINT ( 'NONE',  ( -9.564922557961040184, 16.46253265017147172, 107.9177570613523471 ) ) ;
#61380=CARTESIAN_POINT ( 'NONE',  ( -10.81492255796078084, -18.62759615963271287, 102.0822429386476955 ) ) ;
#61381=CARTESIAN_POINT ( 'NONE',  ( 5.049401038297881783, 19.05341960407617563, 67.29275706135234714 ) ) ;
#61382=CARTESIAN_POINT ( 'NONE',  ( 13.89961937509977652, -13.97604488694527269, 83.12390960531436690 ) ) ;
#61383=CARTESIAN_POINT ( 'NONE',  ( 4.483927247898545687, 16.52544592524342804, 79.79057627198102409 ) ) ;
#61384=CARTESIAN_POINT ( 'NONE',  ( -5.153800228976328057, -19.02544592524343514, 62.29057627198100988 ) ) ;
#61385=CARTESIAN_POINT ( 'NONE',  ( -12.14591786802309592, -12.06949235617757132, 71.87390960531438111 ) ) ;
#61386=CARTESIAN_POINT ( 'NONE',  ( -9.564922557960796823, -16.46253265017161027, 32.08224293864769550 ) ) ;
#61388=CARTESIAN_POINT ( 'NONE',  ( -12.06949235617756955, 12.14591786802309770, 40.62390960531435269 ) ) ;
#61389=CARTESIAN_POINT ( 'NONE',  ( 19.02544592524343514, -5.153800228976328945, 93.54057627198102409 ) ) ;
#61391=CARTESIAN_POINT ( 'NONE',  ( -13.89961937509957401, -13.97604488694547875, 54.37609039468565442 ) ) ;
#61392=CARTESIAN_POINT ( 'NONE',  ( -8.314922557961024197, 14.29746914071037800, 57.91775706135234714 ) ) ;
#61393=CARTESIAN_POINT ( 'NONE',  ( 10.81492255796078972, 18.62759615963270932, 59.58224293864770260 ) ) ;
#61394=CARTESIAN_POINT ( 'NONE',  ( -5.049401038297874678, -19.05341960407617918, 19.79275706135233293 ) ) ;
#61395=CARTESIAN_POINT ( 'NONE',  ( -9.564922557960796823, -16.46253265017161027, 92.08224293864769550 ) ) ;
#61397=CARTESIAN_POINT ( 'NONE',  ( -5.719274019375978568, 21.55341960407610458, 30.20724293864769550 ) ) ;
#61398=CARTESIAN_POINT ( 'NONE',  ( 9.474510206698971260, -16.51473224551069308, 62.91557627198102409 ) ) ;
#61399=CARTESIAN_POINT ( 'NONE',  ( -10.81492255796105439, 18.62759615963255655, 52.91775706135235424 ) ) ;
#61400=PRODUCT_DEFINITION_SHAPE ( 'NONE', 'NONE',  #48691 ) ;
#61401=CARTESIAN_POINT ( 'NONE',  ( 16.55341960407611168, 4.379528057220329451, 103.9572429386476813 ) ) ;
#61402=CARTESIAN_POINT ( 'NONE',  ( 21.53943276465977519, -0.05219959533907433946, 103.7489096053143669 ) ) ;
#61403=CARTESIAN_POINT ( 'NONE',  ( -19.05341960407611168, -5.049401038298163336, 101.4572429386476955 ) ) ;
#61405=CARTESIAN_POINT ( 'NONE',  ( -5.719274019375665041, -21.55341960407619695, 39.79275706135235424 ) ) ;
#61407=CARTESIAN_POINT ( 'NONE',  ( -9.564922557960796823, -16.46253265017161027, 107.0822429386476955 ) ) ;
#61409=CARTESIAN_POINT ( 'NONE',  ( 10.72451020669898902, -18.67979575497178502, 97.91557627198103830 ) ) ;
#61410=CARTESIAN_POINT ( 'NONE',  ( 19.02544592524343514, -5.153800228976328945, 43.54057627198103120 ) ) ;
#61411=CARTESIAN_POINT ( 'NONE',  ( -14.34966873604972548, 8.224510206698743886, 28.33442372801902209 ) ) ;
#61413=CARTESIAN_POINT ( 'NONE',  ( 9.564922557960805705, 16.46253265017160317, 29.58224293864769550 ) ) ;
#61414=CARTESIAN_POINT ( 'NONE',  ( 21.53943276465977519, 0.05219959533937863772, 101.2510903946856757 ) ) ;
#61415=CARTESIAN_POINT ( 'NONE',  ( 9.564922557960805705, 16.46253265017160317, 74.58224293864769550 ) ) ;
#61416=CARTESIAN_POINT ( 'NONE',  ( 5.823673210054444382, -21.52544592524334988, 40.20942372801901854 ) ) ;
#61419=CARTESIAN_POINT ( 'NONE',  ( -5.049401038298153566, 19.05341960407611168, 100.2072429386476955 ) ) ;
#61420=CARTESIAN_POINT ( 'NONE',  ( 18.22780087662126647, 5.499999999999818812, 61.48236817873107185 ) ) ;
#61421=CARTESIAN_POINT ( 'NONE',  ( -12.06949235617739369, -12.14591786802326823, 34.37609039468568284 ) ) ;
#61422=CARTESIAN_POINT ( 'NONE',  ( -16.55341960407617563, 4.379528057220093196, 73.54275706135234714 ) ) ;
#61423=CARTESIAN_POINT ( 'NONE',  ( -5.719274019375665041, -21.55341960407619695, 59.79275706135234714 ) ) ;
#61424=CARTESIAN_POINT ( 'NONE',  ( -10.72451020669870658, -18.67979575497194134, 79.58442372801903275 ) ) ;
#61426=CARTESIAN_POINT ( 'NONE',  ( -13.97604488694547697, 13.89961937509957934, 108.1260903946856331 ) ) ;
#61427=CARTESIAN_POINT ( 'NONE',  ( 19.02544592524343514, -5.153800228976328945, 73.54057627198103830 ) ) ;
#61428=CARTESIAN_POINT ( 'NONE',  ( 19.02544592524343514, -5.153800228976328945, 103.5405762719809957 ) ) ;
#61429=CARTESIAN_POINT ( 'NONE',  ( -4.379528057220328563, 16.55341960407611168, 110.2072429386477239 ) ) ;
#61430=CARTESIAN_POINT ( 'NONE',  ( -21.55341960407610458, -5.719274019375992779, 26.45724293864768839 ) ) ;
#61431=CARTESIAN_POINT ( 'NONE',  ( 16.55341960407618274, -4.379528057220086978, 96.04275706135236135 ) ) ;
#61432=CARTESIAN_POINT ( 'NONE',  ( 12.14591786802309770, 12.06949235617756955, 74.37390960531436690 ) ) ;
#61433=CARTESIAN_POINT ( 'NONE',  ( -19.03943276465977164, 0.05219959533909376836, 51.24890960531436690 ) ) ;
#61434=CARTESIAN_POINT ( 'NONE',  ( -15.72974639402176322, -15.80617190586768395, 74.37609039468568994 ) ) ;
#61435=CARTESIAN_POINT ( 'NONE',  ( 17.50000000000000355, 4.403995465277920296, 21.93328991121576621 ) ) ;
#61436=CARTESIAN_POINT ( 'NONE',  ( 16.51473224551083163, -9.474510206698727899, 105.8344237280190043 ) ) ;
#61437=CARTESIAN_POINT ( 'NONE',  ( 0.05219959533910956823, 16.53943276465976808, 79.99890960531435269 ) ) ;
#61438=CARTESIAN_POINT ( 'NONE',  ( 21.55341960407619695, -5.719274019375665929, 26.04275706135235779 ) ) ;
#61439=CARTESIAN_POINT ( 'NONE',  ( -5.719274019375978568, 21.55341960407610458, 55.20724293864770260 ) ) ;
#61440=CARTESIAN_POINT ( 'NONE',  ( -17.31728774477274158, -6.344390552232370695, 104.1809334831068838 ) ) ;
#61442=CARTESIAN_POINT ( 'NONE',  ( 5.049401038298161559, -19.05341960407611168, 87.70724293864769550 ) ) ;
#61443=CARTESIAN_POINT ( 'NONE',  ( 4.483927247898545687, 16.52544592524342804, 54.79057627198104541 ) ) ;
#61445=CARTESIAN_POINT ( 'NONE',  ( 8.224510206698953496, -14.34966873604960469, 22.91557627198102765 ) ) ;
#61446=CARTESIAN_POINT ( 'NONE',  ( 12.06949235617739724, 12.14591786802326823, 96.87609039468568994 ) ) ;
#61447=CARTESIAN_POINT ( 'NONE',  ( -13.89961937509957401, -13.97604488694547875, 54.37609039468565442 ) ) ;
#61450=CARTESIAN_POINT ( 'NONE',  ( -9.564922557960796823, -16.46253265017161027, 107.0822429386476955 ) ) ;
#61451=CARTESIAN_POINT ( 'NONE',  ( -8.314922557960811034, -14.29746914071050412, 77.08224293864769550 ) ) ;
#61452=CARTESIAN_POINT ( 'NONE',  ( -5.153800228976607833, 19.02544592524334988, 47.70942372801900433 ) ) ;
#61453=CARTESIAN_POINT ( 'NONE',  ( 19.03943276465977164, -0.05219959533909143690, 33.74890960531435979 ) ) ;
#61454=CARTESIAN_POINT ( 'NONE',  ( -15.72974639402197994, 15.80617190586746368, 40.62390960531435269 ) ) ;
#61455=CARTESIAN_POINT ( 'NONE',  ( 21.53943276465977519, -0.05219959533907433946, 73.74890960531433848 ) ) ;
#61456=CARTESIAN_POINT ( 'NONE',  ( 4.483927247898545687, 16.52544592524342804, 94.79057627198105251 ) ) ;
#61457=CARTESIAN_POINT ( 'NONE',  ( -12.06949235617739369, -12.14591786802326823, 54.37609039468568994 ) ) ;
#61458=CARTESIAN_POINT ( 'NONE',  ( 21.52544592524334988, 5.823673210054432836, 46.45942372801901854 ) ) ;
#61459=CARTESIAN_POINT ( 'NONE',  ( -16.55341960407611168, -4.379528057220339221, 91.45724293864769550 ) ) ;
#61461=CARTESIAN_POINT ( 'NONE',  ( -16.19135201231370047, 7.376712067591785882, 49.81319145947971094 ) ) ;
#61462=CARTESIAN_POINT ( 'NONE',  ( 5.719274019375991003, -21.55341960407610458, 32.70724293864770260 ) ) ;
#61465=CARTESIAN_POINT ( 'NONE',  ( -0.05219959533934338120, 16.53943276465976808, 47.50109039468568994 ) ) ;
#61466=CARTESIAN_POINT ( 'NONE',  ( 0.05219959533910956823, 16.53943276465976808, 29.99890960531435979 ) ) ;
#61467=CARTESIAN_POINT ( 'NONE',  ( -18.62759615963270932, 10.81492255796079327, 70.83224293864770971 ) ) ;
#61468=CARTESIAN_POINT ( 'NONE',  ( 13.89961937509957401, 13.97604488694547697, 81.87609039468564731 ) ) ;
#61469=CARTESIAN_POINT ( 'NONE',  ( -18.62759615963270932, 10.81492255796079327, 60.83224293864769550 ) ) ;
#61471=CARTESIAN_POINT ( 'NONE',  ( 12.14591786802327356, -12.06949235617739191, 50.62609039468568994 ) ) ;
#61472=CARTESIAN_POINT ( 'NONE',  ( 5.049401038298161559, -19.05341960407611168, 32.70724293864768129 ) ) ;
#61473=CARTESIAN_POINT ( 'NONE',  ( -5.049401038298153566, 19.05341960407611168, 95.20724293864770971 ) ) ;
#61474=CARTESIAN_POINT ( 'NONE',  ( 19.02544592524343514, -5.153800228976328945, 38.54057627198103120 ) ) ;
#61475=CARTESIAN_POINT ( 'NONE',  ( 16.55341960407611168, 4.379528057220329451, 113.9572429386477239 ) ) ;
#61477=CARTESIAN_POINT ( 'NONE',  ( 5.153800228976335163, 19.02544592524342804, 109.7905762719810099 ) ) ;
#61478=ORIENTED_EDGE ( 'NONE', *, *, #69172, .F. ) ;
#61479=CARTESIAN_POINT ( 'NONE',  ( 16.53943276465976808, 0.05219959533934440121, 66.25109039468567573 ) ) ;
#61480=CARTESIAN_POINT ( 'NONE',  ( 21.53943276465977519, -0.05219959533907433946, 88.74890960531436690 ) ) ;
#61481=CARTESIAN_POINT ( 'NONE',  ( 5.049401038298161559, -19.05341960407611168, 57.70724293864769550 ) ) ;
#61482=CARTESIAN_POINT ( 'NONE',  ( 21.53943276465977519, 0.05219959533937863772, 31.25109039468568639 ) ) ;
#61483=CARTESIAN_POINT ( 'NONE',  ( -13.89961937509977652, 13.97604488694528158, 80.62390960531436690 ) ) ;
#61484=CARTESIAN_POINT ( 'NONE',  ( 9.474510206698971260, -16.51473224551069308, 112.9155762719810383 ) ) ;
#61486=VERTEX_POINT ( 'NONE', #147766 ) ;
#61487=CARTESIAN_POINT ( 'NONE',  ( 15.72974639402176855, 15.80617190586768217, 21.87609039468567573 ) ) ;
#61488=CARTESIAN_POINT ( 'NONE',  ( -4.379528057220328563, 16.55341960407611168, 115.2072429386476955 ) ) ;
#61489=CARTESIAN_POINT ( 'NONE',  ( -13.89961937509977652, 13.97604488694528158, 110.6239096053143243 ) ) ;
#61490=CARTESIAN_POINT ( 'NONE',  ( -9.474510206698720793, -16.51473224551083518, 89.58442372801900433 ) ) ;
#61491=CARTESIAN_POINT ( 'NONE',  ( 16.51473224551083163, -9.474510206698727899, 25.83442372801900078 ) ) ;
#61492=CARTESIAN_POINT ( 'NONE',  ( -10.81492255796078084, -18.62759615963271287, 97.08224293864770971 ) ) ;
#61493=CARTESIAN_POINT ( 'NONE',  ( 13.89961937509957401, 13.97604488694547697, 41.87609039468566152 ) ) ;
#61494=CARTESIAN_POINT ( 'NONE',  ( 4.483927247898790824, -16.52544592524335698, 85.20942372801901854 ) ) ;
#61496=CARTESIAN_POINT ( 'NONE',  ( 16.51473224551069308, 9.474510206698969483, 109.1655762719810383 ) ) ;
#61497=CARTESIAN_POINT ( 'NONE',  ( 16.51473224551069308, 9.474510206698969483, 64.16557627198102409 ) ) ;
#61498=CARTESIAN_POINT ( 'NONE',  ( 21.53943276465977519, 0.05219959533937863772, 61.25109039468567573 ) ) ;
#61499=CARTESIAN_POINT ( 'NONE',  ( -21.53943276465977519, -0.05219959533937600094, 83.75109039468568994 ) ) ;
#61500=CARTESIAN_POINT ( 'NONE',  ( 16.46253265017160672, -9.564922557960803928, 113.3322429386476955 ) ) ;
#61501=CARTESIAN_POINT ( 'NONE',  ( -13.97604488694527625, -13.89961937509977652, 71.87390960531433848 ) ) ;
#61502=CARTESIAN_POINT ( 'NONE',  ( -10.81492255796105439, 18.62759615963255655, 47.91775706135234714 ) ) ;
#61503=CARTESIAN_POINT ( 'NONE',  ( 9.474510206698729675, 16.51473224551082808, 92.08442372801900433 ) ) ;
#61504=CARTESIAN_POINT ( 'NONE',  ( -16.46253265017160317, 9.564922557960807481, 50.83224293864770260 ) ) ;
#61505=CARTESIAN_POINT ( 'NONE',  ( 13.89961937509977652, -13.97604488694527269, 93.12390960531436690 ) ) ;
#61506=CARTESIAN_POINT ( 'NONE',  ( -16.46253265017160317, 9.564922557960807481, 60.83224293864769550 ) ) ;
#61508=CARTESIAN_POINT ( 'NONE',  ( 9.564922557960805705, 16.46253265017160317, 49.58224293864770260 ) ) ;
#61509=CARTESIAN_POINT ( 'NONE',  ( -21.52544592524343514, 5.823673210054127303, 106.0405762719810525 ) ) ;
#61510=CARTESIAN_POINT ( 'NONE',  ( 0.05219959533934541429, -16.53943276465976808, 90.00109039468567573 ) ) ;
#61512=CARTESIAN_POINT ( 'NONE',  ( -0.05219959533936034679, 19.03943276465977164, 42.50109039468566152 ) ) ;
#61513=CARTESIAN_POINT ( 'NONE',  ( -0.05219959533909027116, -19.03943276465977164, 67.49890960531436690 ) ) ;
#61514=CARTESIAN_POINT ( 'NONE',  ( 0.05219959533910956823, 16.53943276465976808, 54.99890960531435269 ) ) ;
#61515=CARTESIAN_POINT ( 'NONE',  ( -14.34966873604960291, -8.224510206698953496, 91.66557627198103830 ) ) ;
#61516=CARTESIAN_POINT ( 'NONE',  ( 9.564922557960805705, 16.46253265017160317, 114.5822429386476955 ) ) ;
#61517=CARTESIAN_POINT ( 'NONE',  ( 19.02544592524343514, -5.153800228976328945, 98.54057627198100988 ) ) ;
#61518=CARTESIAN_POINT ( 'NONE',  ( -13.89961937509977652, 13.97604488694528158, 110.6239096053143243 ) ) ;
#61519=CARTESIAN_POINT ( 'NONE',  ( -13.97604488694547697, 13.89961937509957934, 23.12609039468565442 ) ) ;
#61520=CARTESIAN_POINT ( 'NONE',  ( 16.52544592524335698, 4.483927247898782831, 96.45942372801901854 ) ) ;
#61521=CARTESIAN_POINT ( 'NONE',  ( -13.89961937509977652, 13.97604488694528158, 75.62390960531438111 ) ) ;
#61522=CARTESIAN_POINT ( 'NONE',  ( -21.55341960407619339, 5.719274019375674811, 38.54275706135234714 ) ) ;
#61523=CARTESIAN_POINT ( 'NONE',  ( -10.72451020669898014, 18.67979575497178502, 35.41557627198102409 ) ) ;
#61524=CARTESIAN_POINT ( 'NONE',  ( -21.53943276465977519, -0.05219959533937600094, 18.75109039468568639 ) ) ;
#61525=CARTESIAN_POINT ( 'NONE',  ( -15.72974639402197994, 15.80617190586746368, 70.62390960531436690 ) ) ;
#61526=CARTESIAN_POINT ( 'NONE',  ( -16.52544592524342804, 4.483927247898546575, 86.04057627198102409 ) ) ;
#61527=CARTESIAN_POINT ( 'NONE',  ( -5.153800228976607833, 19.02544592524334988, 37.70942372801899722 ) ) ;
#61528=CARTESIAN_POINT ( 'NONE',  ( -4.483927247898539470, -16.52544592524342804, 112.2905762719810241 ) ) ;
#61529=CARTESIAN_POINT ( 'NONE',  ( -5.153800228976328057, -19.02544592524343514, 77.29057627198099567 ) ) ;
#61530=CARTESIAN_POINT ( 'NONE',  ( -9.564922557960796823, -16.46253265017161027, 87.08224293864769550 ) ) ;
#61532=CARTESIAN_POINT ( 'NONE',  ( -8.224510206698948167, 14.34966873604960824, 95.41557627198102409 ) ) ;
#61533=VERTEX_POINT ( 'NONE', #40582 ) ;
#61534=CARTESIAN_POINT ( 'NONE',  ( -0.05219959533934338120, 16.53943276465976808, 102.5010903946856899 ) ) ;
#61535=CARTESIAN_POINT ( 'NONE',  ( -8.224510206698735004, -14.34966873604973081, 29.58442372801901854 ) ) ;
#61536=CARTESIAN_POINT ( 'NONE',  ( -21.52544592524334988, -5.823673210054445271, 98.95942372801903275 ) ) ;
#61537=CARTESIAN_POINT ( 'NONE',  ( -16.51473224551069308, -9.474510206698971260, 101.6655762719810241 ) ) ;
#61538=CARTESIAN_POINT ( 'NONE',  ( 5.719274019375673035, 21.55341960407619339, 22.29275706135235069 ) ) ;
#61539=CARTESIAN_POINT ( 'NONE',  ( -16.46253265017160317, 9.564922557960807481, 25.83224293864769194 ) ) ;
#61540=CARTESIAN_POINT ( 'NONE',  ( 14.34966873604972726, -8.224510206698740333, 30.83442372801902209 ) ) ;
#61541=CARTESIAN_POINT ( 'NONE',  ( 13.89961937509957401, 13.97604488694547697, 91.87609039468567573 ) ) ;
#61542=CARTESIAN_POINT ( 'NONE',  ( -5.719274019375978568, 21.55341960407610458, 100.2072429386476955 ) ) ;
#61543=CARTESIAN_POINT ( 'NONE',  ( 19.03943276465977164, 0.05219959533936151252, 71.25109039468566152 ) ) ;
#61544=CARTESIAN_POINT ( 'NONE',  ( -9.564922557960796823, -16.46253265017161027, 22.08224293864768839 ) ) ;
#61545=CARTESIAN_POINT ( 'NONE',  ( -18.62759615963270932, 10.81492255796079327, 110.8322429386476955 ) ) ;
#61547=CARTESIAN_POINT ( 'NONE',  ( -13.97604488694527625, -13.89961937509977652, 91.87390960531432427 ) ) ;
#61549=CARTESIAN_POINT ( 'NONE',  ( 9.474510206698971260, -16.51473224551069308, 87.91557627198102409 ) ) ;
#61550=CARTESIAN_POINT ( 'NONE',  ( -15.72974639402176322, -15.80617190586768395, 24.37609039468567573 ) ) ;
#61551=CARTESIAN_POINT ( 'NONE',  ( -12.06949235617756955, 12.14591786802309770, 80.62390960531438111 ) ) ;
#61552=CARTESIAN_POINT ( 'NONE',  ( 13.97604488694527802, 13.89961937509977652, 79.37390960531435269 ) ) ;
#61553=CARTESIAN_POINT ( 'NONE',  ( 4.379528057220092307, 16.55341960407617563, 57.29275706135234714 ) ) ;
#61554=CARTESIAN_POINT ( 'NONE',  ( -16.51473224551082808, 9.474510206698731452, 58.33442372801900433 ) ) ;
#61555=CARTESIAN_POINT ( 'NONE',  ( -21.55341960407619339, 5.719274019375674811, 63.54275706135234003 ) ) ;
#61556=CARTESIAN_POINT ( 'NONE',  ( -0.05219959533934338120, 16.53943276465976808, 22.50109039468567573 ) ) ;
#61557=CARTESIAN_POINT ( 'NONE',  ( -5.153800228976328057, -19.02544592524343514, 62.29057627198100988 ) ) ;
#61558=CARTESIAN_POINT ( 'NONE',  ( 16.46253265017146816, 9.564922557961045513, 91.66775706135234714 ) ) ;
#61559=CARTESIAN_POINT ( 'NONE',  ( 4.483927247898790824, -16.52544592524335698, 50.20942372801901854 ) ) ;
#61560=CARTESIAN_POINT ( 'NONE',  ( 15.72974639402176855, 15.80617190586768217, 91.87609039468568994 ) ) ;
#61561=CARTESIAN_POINT ( 'NONE',  ( 19.05341960407617918, -5.049401038297876454, 76.04275706135230450 ) ) ;
#61562=CARTESIAN_POINT ( 'NONE',  ( 16.46253265017160672, -9.564922557960803928, 48.33224293864769550 ) ) ;
#61563=CARTESIAN_POINT ( 'NONE',  ( 21.52544592524344225, -5.823673210054117533, 68.54057627198103830 ) ) ;
#61564=CARTESIAN_POINT ( 'NONE',  ( -4.483927247898539470, -16.52544592524342804, 77.29057627198102409 ) ) ;
#61565=CARTESIAN_POINT ( 'NONE',  ( -5.049401038297874678, -19.05341960407617918, 79.79275706135233293 ) ) ;
#61567=CARTESIAN_POINT ( 'NONE',  ( 19.05341960407617918, -5.049401038297876454, 46.04275706135233293 ) ) ;
#61568=CARTESIAN_POINT ( 'NONE',  ( 4.483927247898790824, -16.52544592524335698, 110.2094237280190185 ) ) ;
#61569=CARTESIAN_POINT ( 'NONE',  ( -16.52544592524342804, 4.483927247898546575, 71.04057627198103830 ) ) ;
#61570=CARTESIAN_POINT ( 'NONE',  ( 18.67979575497194134, -10.72451020669871369, 105.8344237280190328 ) ) ;
#61572=CARTESIAN_POINT ( 'NONE',  ( 10.72451020669898902, -18.67979575497178502, 107.9155762719810241 ) ) ;
#61573=CARTESIAN_POINT ( 'NONE',  ( 16.51473224551069308, 9.474510206698969483, 69.16557627198102409 ) ) ;
#61574=CARTESIAN_POINT ( 'NONE',  ( 21.53943276465977519, 0.05219959533937863772, 81.25109039468568994 ) ) ;
#61575=CARTESIAN_POINT ( 'NONE',  ( 5.049401038298161559, -19.05341960407611168, 62.70724293864769550 ) ) ;
#61577=CARTESIAN_POINT ( 'NONE',  ( -16.46253265017160317, 9.564922557960807481, 25.83224293864769194 ) ) ;
#61578=CARTESIAN_POINT ( 'NONE',  ( 16.46253265017160672, -9.564922557960803928, 113.3322429386476955 ) ) ;
#61579=CARTESIAN_POINT ( 'NONE',  ( 16.55341960407611168, 4.379528057220329451, 68.95724293864769550 ) ) ;
#61580=CARTESIAN_POINT ( 'NONE',  ( 9.474510206698971260, -16.51473224551069308, 32.91557627198102409 ) ) ;
#61581=CARTESIAN_POINT ( 'NONE',  ( -12.06949235617756955, 12.14591786802309770, 80.62390960531438111 ) ) ;
#61582=CARTESIAN_POINT ( 'NONE',  ( -15.72974639402197994, 15.80617190586746368, 100.6239096053143811 ) ) ;
#61583=B_SPLINE_CURVE_WITH_KNOTS ( 'NONE', 3,
 ( #139467, #109137, #91958, #45486, #15146, #33300, #107141, #14146, #170816, #156643, #153651, #172809, #75813, #31309, #141466, #1956, #138479, #90969, #154648, #110133, #32308, #2950, #152656, #17137, #16143, #126291, #137491, #61630, #63635, #125311, #123298, #199171 ),
 .UNSPECIFIED., .F., .F.,
 ( 4, 2, 2, 2, 2, 2, 2, 2, 2, 2, 2, 2, 2, 2, 2, 4 ),
 ( 1.262897753262583006E-17, 0.0003712461730036916568, 0.0007424923460073706285, 0.001113738519011049600, 0.001484984692014728680, 0.002227477038022086624, 0.002598723211025759199, 0.002969969384029431773, 0.003341215557033103915, 0.003712461730036776056, 0.004083707903040449498, 0.004454954076044122073, 0.004826200249047793780, 0.005197446422051466355, 0.005568692595055138930, 0.005939938768058811505 ),
 .UNSPECIFIED. ) ;
#61584=CARTESIAN_POINT ( 'NONE',  ( 21.55341960407619695, -5.719274019375665929, 51.04275706135234714 ) ) ;
#61586=CARTESIAN_POINT ( 'NONE',  ( -12.14591786802326823, 12.06949235617739902, 48.12609039468568284 ) ) ;
#61587=CARTESIAN_POINT ( 'NONE',  ( 10.81492255796078972, 18.62759615963270932, 94.58224293864769550 ) ) ;
#61588=CARTESIAN_POINT ( 'NONE',  ( 13.97604488694548053, -13.89961937509957401, 30.62609039468566863 ) ) ;
#61589=CARTESIAN_POINT ( 'NONE',  ( -19.02544592524342804, 5.153800228976336051, 101.0405762719810241 ) ) ;
#61590=CARTESIAN_POINT ( 'NONE',  ( 0.05219959533937995610, -21.53943276465977519, 45.00109039468568284 ) ) ;
#61591=CARTESIAN_POINT ( 'NONE',  ( 21.52544592524344225, -5.823673210054117533, 38.54057627198103120 ) ) ;
#61592=CARTESIAN_POINT ( 'NONE',  ( -16.53943276465976808, 0.05219959533911058130, 21.24890960531436690 ) ) ;
#61593=CARTESIAN_POINT ( 'NONE',  ( 21.52544592524334988, 5.823673210054432836, 66.45942372801903275 ) ) ;
#61594=CARTESIAN_POINT ( 'NONE',  ( 18.62759615963255655, 10.81492255796105972, 91.66775706135234714 ) ) ;
#61595=CARTESIAN_POINT ( 'NONE',  ( 19.02544592524334988, 5.153800228976608722, 36.45942372801900433 ) ) ;
#61596=CARTESIAN_POINT ( 'NONE',  ( -4.379528057220086978, -16.55341960407618274, 94.79275706135234714 ) ) ;
#61597=CARTESIAN_POINT ( 'NONE',  ( -21.55341960407619339, 5.719274019375674811, 58.54275706135235424 ) ) ;
#61598=CARTESIAN_POINT ( 'NONE',  ( 9.474510206698971260, -16.51473224551069308, 47.91557627198102409 ) ) ;
#61599=CARTESIAN_POINT ( 'NONE',  ( -16.46253265017146816, -9.564922557961047289, 19.16775706135233293 ) ) ;
#61600=CARTESIAN_POINT ( 'NONE',  ( -18.62759615963270932, 10.81492255796079327, 30.83224293864770260 ) ) ;
#61601=CARTESIAN_POINT ( 'NONE',  ( -15.80617190586768217, 15.72974639402176855, 23.12609039468567573 ) ) ;
#61602=CARTESIAN_POINT ( 'NONE',  ( 18.67979575497178502, 10.72451020669898547, 74.16557627198102409 ) ) ;
#61603=CARTESIAN_POINT ( 'NONE',  ( -16.53943276465976808, -0.05219959533934237506, 38.75109039468567573 ) ) ;
#61604=LINE ( 'NONE', #18115, #135536 ) ;
#61605=CARTESIAN_POINT ( 'NONE',  ( -18.67979575497178146, -10.72451020669898902, 76.66557627198103830 ) ) ;
#61606=CARTESIAN_POINT ( 'NONE',  ( -12.06949235617739369, -12.14591786802326823, 64.37609039468568994 ) ) ;
#61607=CARTESIAN_POINT ( 'NONE',  ( 12.06949235617757843, -12.14591786802309237, 58.12390960531435979 ) ) ;
#61609=CARTESIAN_POINT ( 'NONE',  ( 5.049401038297881783, 19.05341960407617563, 107.2927570613523187 ) ) ;
#61610=EDGE_CURVE ( 'NONE', #68126, #133003, #155778, .T. ) ;
#61611=CARTESIAN_POINT ( 'NONE',  ( -10.72451020669898014, 18.67979575497178502, 35.41557627198102409 ) ) ;
#61613=CARTESIAN_POINT ( 'NONE',  ( 8.314922557961029526, -14.29746914071037800, 45.41775706135234003 ) ) ;
#61614=CARTESIAN_POINT ( 'NONE',  ( 0.05219959533907565091, 21.53943276465977519, 114.9989096053143669 ) ) ;
#61615=CARTESIAN_POINT ( 'NONE',  ( 18.62759615963271287, -10.81492255796078972, 28.33224293864769550 ) ) ;
#61616=CARTESIAN_POINT ( 'NONE',  ( -14.29746914071037622, -8.314922557961029526, 64.16775706135234714 ) ) ;
#61617=CARTESIAN_POINT ( 'NONE',  ( -19.03943276465977164, 0.05219959533909376836, 91.24890960531436690 ) ) ;
#61618=CARTESIAN_POINT ( 'NONE',  ( 15.72974639402176855, 15.80617190586768217, 36.87609039468568994 ) ) ;
#61619=CARTESIAN_POINT ( 'NONE',  ( -9.564922557961040184, 16.46253265017147172, 112.9177570613523329 ) ) ;
#61620=CARTESIAN_POINT ( 'NONE',  ( -10.81492255796078084, -18.62759615963271287, 27.08224293864769550 ) ) ;
#61622=CARTESIAN_POINT ( 'NONE',  ( -16.46253265017146816, -9.564922557961047289, 24.16775706135233648 ) ) ;
#61623=CARTESIAN_POINT ( 'NONE',  ( 0.05219959533934541429, -16.53943276465976808, 40.00109039468567573 ) ) ;
#61624=CARTESIAN_POINT ( 'NONE',  ( 16.46253265017160672, -9.564922557960803928, 103.3322429386476955 ) ) ;
#61625=CARTESIAN_POINT ( 'NONE',  ( 15.72974639402199770, -15.80617190586745480, 103.1239096053143811 ) ) ;
#61626=CARTESIAN_POINT ( 'NONE',  ( 5.049401038298161559, -19.05341960407611168, 67.70724293864769550 ) ) ;
#61628=CARTESIAN_POINT ( 'NONE',  ( -14.29746914071049879, 8.314922557960819915, 80.83224293864769550 ) ) ;
#61629=CARTESIAN_POINT ( 'NONE',  ( -5.823673210054116645, -21.52544592524344225, 37.29057627198102409 ) ) ;
#61630=CARTESIAN_POINT ( 'NONE',  ( -17.40861289039003523, 6.110651285853256454, 33.62767529172568004 ) ) ;
#61631=CARTESIAN_POINT ( 'NONE',  ( -14.34966873604972548, 8.224510206698743886, 63.33442372801900433 ) ) ;
#61632=CARTESIAN_POINT ( 'NONE',  ( 21.55341960407610458, 5.719274019375980345, 98.95724293864770971 ) ) ;
#61633=CARTESIAN_POINT ( 'NONE',  ( 19.05341960407617918, -5.049401038297876454, 76.04275706135230450 ) ) ;
#61634=CARTESIAN_POINT ( 'NONE',  ( 16.51473224551069308, 9.474510206698969483, 24.16557627198102765 ) ) ;
#61635=CARTESIAN_POINT ( 'NONE',  ( -5.823673210054116645, -21.52544592524344225, 62.29057627198102409 ) ) ;
#61636=CARTESIAN_POINT ( 'NONE',  ( 0.05219959533909260263, 19.03943276465977164, 94.99890960531436690 ) ) ;
#61637=CARTESIAN_POINT ( 'NONE',  ( 21.53943276465977519, 0.05219959533937863772, 96.25109039468568994 ) ) ;
#61638=CARTESIAN_POINT ( 'NONE',  ( 19.02544592524343514, -5.153800228976328945, 63.54057627198103830 ) ) ;
#61639=CARTESIAN_POINT ( 'NONE',  ( -12.06949235617739369, -12.14591786802326823, 49.37609039468569705 ) ) ;
#61640=CARTESIAN_POINT ( 'NONE',  ( 5.049401038298161559, -19.05341960407611168, 57.70724293864769550 ) ) ;
#61641=CARTESIAN_POINT ( 'NONE',  ( -21.52544592524334988, -5.823673210054445271, 78.95942372801901854 ) ) ;
#61643=CARTESIAN_POINT ( 'NONE',  ( 19.03943276465977164, 0.05219959533936151252, 36.25109039468567573 ) ) ;
#61644=CARTESIAN_POINT ( 'NONE',  ( -16.51473224551082808, 9.474510206698731452, 53.33442372801900433 ) ) ;
#61645=CARTESIAN_POINT ( 'NONE',  ( -10.81492255796105439, 18.62759615963255655, 52.91775706135235424 ) ) ;
#61647=CARTESIAN_POINT ( 'NONE',  ( 16.51473224551083163, -9.474510206698727899, 40.83442372801900433 ) ) ;
#61648=CARTESIAN_POINT ( 'NONE',  ( -19.05341960407611168, -5.049401038298163336, 91.45724293864766707 ) ) ;
#61649=CARTESIAN_POINT ( 'NONE',  ( 9.564922557960805705, 16.46253265017160317, 64.58224293864769550 ) ) ;
#61650=CARTESIAN_POINT ( 'NONE',  ( -12.06949235617756955, 12.14591786802309770, 25.62390960531435624 ) ) ;
#61651=CARTESIAN_POINT ( 'NONE',  ( -19.02544592524342804, 5.153800228976336051, 116.0405762719810383 ) ) ;
#61652=CARTESIAN_POINT ( 'NONE',  ( -15.80617190586768217, 15.72974639402176855, 93.12609039468568994 ) ) ;
#61654=CARTESIAN_POINT ( 'NONE',  ( 16.20579543436682002, 7.371946100354976217, 58.06520834171880097 ) ) ;
#61655=CARTESIAN_POINT ( 'NONE',  ( 18.67979575497194134, -10.72451020669871369, 95.83442372801903275 ) ) ;
#61657=CARTESIAN_POINT ( 'NONE',  ( 16.52544592524342804, -4.483927247898539470, 113.5405762719810383 ) ) ;
#61658=CARTESIAN_POINT ( 'NONE',  ( -9.564922557960796823, -16.46253265017161027, 112.0822429386476955 ) ) ;
#61660=CARTESIAN_POINT ( 'NONE',  ( 4.379528057220092307, 16.55341960407617563, 47.29275706135234003 ) ) ;
#61661=CARTESIAN_POINT ( 'NONE',  ( 5.719274019375991003, -21.55341960407610458, 67.70724293864769550 ) ) ;
#61662=CARTESIAN_POINT ( 'NONE',  ( 4.379528057220339221, -16.55341960407611168, 37.70724293864769550 ) ) ;
#61663=CARTESIAN_POINT ( 'NONE',  ( 4.483927247898545687, 16.52544592524342804, 104.7905762719810241 ) ) ;
#61664=CARTESIAN_POINT ( 'NONE',  ( -16.51473224551069308, -9.474510206698971260, 91.66557627198103830 ) ) ;
#61665=CARTESIAN_POINT ( 'NONE',  ( 21.52544592524334988, 5.823673210054432836, 111.4594237280190328 ) ) ;
#61666=CARTESIAN_POINT ( 'NONE',  ( 8.314922557960818139, 14.29746914071049879, 114.5822429386477097 ) ) ;
#61667=CARTESIAN_POINT ( 'NONE',  ( -15.72974639402176322, -15.80617190586768395, 69.37609039468567573 ) ) ;
#61668=CARTESIAN_POINT ( 'NONE',  ( 5.153800228976335163, 19.02544592524342804, 114.7905762719810241 ) ) ;
#61669=CARTESIAN_POINT ( 'NONE',  ( 12.06949235617739724, 12.14591786802326823, 101.8760903946857042 ) ) ;
#61670=CARTESIAN_POINT ( 'NONE',  ( -19.03943276465977164, -0.05219959533935918106, 68.75109039468566152 ) ) ;
#61672=CARTESIAN_POINT ( 'NONE',  ( 21.53943276465977519, -0.05219959533907433946, 23.74890960531435269 ) ) ;
#61673=CARTESIAN_POINT ( 'NONE',  ( -14.29746914071049879, 8.314922557960819915, 90.83224293864769550 ) ) ;
#61674=CARTESIAN_POINT ( 'NONE',  ( 16.51473224551083163, -9.474510206698727899, 60.83442372801900433 ) ) ;
#61675=CARTESIAN_POINT ( 'NONE',  ( -16.51473224551069308, -9.474510206698971260, 81.66557627198103830 ) ) ;
#61676=CARTESIAN_POINT ( 'NONE',  ( -14.29746914071049879, 8.314922557960819915, 70.83224293864770971 ) ) ;
#61677=CARTESIAN_POINT ( 'NONE',  ( -13.89961937509957401, -13.97604488694547875, 94.37609039468566152 ) ) ;
#61678=CARTESIAN_POINT ( 'NONE',  ( -15.72974639402197994, 15.80617190586746368, 55.62390960531436690 ) ) ;
#61680=CARTESIAN_POINT ( 'NONE',  ( -14.29746914071049879, 8.314922557960819915, 115.8322429386477097 ) ) ;
#61682=CARTESIAN_POINT ( 'NONE',  ( -16.46253265017160317, 9.564922557960807481, 75.83224293864769550 ) ) ;
#61683=CARTESIAN_POINT ( 'NONE',  ( 15.80617190586746368, 15.72974639402197994, 79.37390960531436690 ) ) ;
#61684=CARTESIAN_POINT ( 'NONE',  ( -14.29746914071037622, -8.314922557961029526, 94.16775706135237556 ) ) ;
#61685=CARTESIAN_POINT ( 'NONE',  ( 13.97604488694527802, 13.89961937509977652, 74.37390960531436690 ) ) ;
#61686=CARTESIAN_POINT ( 'NONE',  ( 19.05341960407617918, -5.049401038297876454, 66.04275706135233293 ) ) ;
#61687=CARTESIAN_POINT ( 'NONE',  ( 15.72974639402176855, 15.80617190586768217, 86.87609039468568994 ) ) ;
#61688=CARTESIAN_POINT ( 'NONE',  ( -18.67979575497178146, -10.72451020669898902, 56.66557627198103830 ) ) ;
#61689=CARTESIAN_POINT ( 'NONE',  ( 5.719274019375991003, -21.55341960407610458, 22.70724293864769194 ) ) ;
#61690=CARTESIAN_POINT ( 'NONE',  ( -19.05341960407611168, -5.049401038298163336, 41.45724293864769550 ) ) ;
#61691=CARTESIAN_POINT ( 'NONE',  ( 12.06949235617739724, 12.14591786802326823, 106.8760903946856899 ) ) ;
#61692=CARTESIAN_POINT ( 'NONE',  ( -19.03943276465977164, 0.05219959533909376836, 56.24890960531435979 ) ) ;
#61693=CARTESIAN_POINT ( 'NONE',  ( 16.46253265017146816, 9.564922557961045513, 111.6677570613523329 ) ) ;
#61694=CARTESIAN_POINT ( 'NONE',  ( 13.89961937509957579, 13.97604488694547520, 81.87609039468566152 ) ) ;
#61695=CARTESIAN_POINT ( 'NONE',  ( 5.719274019375673035, 21.55341960407619339, 112.2927570613523471 ) ) ;
#61696=CARTESIAN_POINT ( 'NONE',  ( -8.314922557960811034, -14.29746914071050412, 62.08224293864769550 ) ) ;
#61697=CARTESIAN_POINT ( 'NONE',  ( 21.53943276465977519, -0.05219959533907433946, 113.7489096053143527 ) ) ;
#61698=CARTESIAN_POINT ( 'NONE',  ( -21.53943276465977519, 0.05219959533907696930, 96.24890960531435269 ) ) ;
#61700=CARTESIAN_POINT ( 'NONE',  ( 0.05219959533907565091, 21.53943276465977519, 49.99890960531437401 ) ) ;
#61701=CARTESIAN_POINT ( 'NONE',  ( -8.314922557961024197, 14.29746914071037800, 82.91775706135234714 ) ) ;
#61702=CARTESIAN_POINT ( 'NONE',  ( 16.52544592524342804, -4.483927247898539470, 93.54057627198103830 ) ) ;
#61703=CARTESIAN_POINT ( 'NONE',  ( 13.97604488694527802, 13.89961937509977652, 64.37390960531436690 ) ) ;
#61704=CARTESIAN_POINT ( 'NONE',  ( -15.49999999999999822, 5.499999999999997335, 22.00000000000000711 ) ) ;
#61705=CARTESIAN_POINT ( 'NONE',  ( 16.52544592524335698, 4.483927247898782831, 106.4594237280190328 ) ) ;
#61706=CARTESIAN_POINT ( 'NONE',  ( 10.81492255796106328, -18.62759615963255655, 35.41775706135234003 ) ) ;
#61707=CARTESIAN_POINT ( 'NONE',  ( 9.564922557960805705, 16.46253265017160317, 99.58224293864770971 ) ) ;
#61708=CARTESIAN_POINT ( 'NONE',  ( -5.719274019375665041, -21.55341960407619695, 69.79275706135234714 ) ) ;
#61709=CARTESIAN_POINT ( 'NONE',  ( -9.564922557960796823, -16.46253265017161027, 22.08224293864768839 ) ) ;
#61710=CARTESIAN_POINT ( 'NONE',  ( 16.46253265017160672, -9.564922557960803928, 28.33224293864769550 ) ) ;
#61712=( BOUNDED_SURFACE ( )  B_SPLINE_SURFACE ( 3, 2, ( 
 ( #52934, #12462, #133791, #89277, #196486, #195483, #121587, #179321, #105437, #120598, #183282, #44764, #42788, #75095, #119627, #149959, #181310, #40785, #148968, #102454, #164142, #166134, #26628, #104451, #74122, #167122, #150967, #13431, #73136, #56958, #28622, #27636, #58930, #135793, #103458, #118632, #134806, #136762, #25639, #88271, #87283, #10457, #198447, #72118, #165136, #182293, #43773, #59919, #180323, #41791, #90259, #11465, #197464, #151942, #57956, #41435, #101083, #159767, #21262, #116265, #85926, #53594, #37424, #162768, #24277, #56604, #147615, #69762, #82918, #68756, #23268, #9102, #144595, #178960, #71763, #192112, #177955, #70769, #129417, #55592, #161773, #163785, #22264, #40429, #146591, #133433, #6081, #39423, #130413, #8085, #132438, #25286, #102100, #38433, #86929, #67760, #191115, #131431, #52589, #194129, #114249, #175955, #117267, #148612, #115270, #99084, #10103, #195122, #118278, #179969, #193117, #160775, #176963, #84912, #83914, #145596, #7075, #100089, #54591, #121240, #106070, #72779, #199086, #105092, #107058, #165780, #183920, #89918, #15064, #184908, #182934, #73774, #88923, #27275, #150615, #12111, #61549, #60554, #168729, #44417, #119274, #30233, #134449, #91875, #59565, #166778, #28279, #135447, #42434, #167757, #200081, #197116, #151600, #29255, #181940, #103102, #74757, #58583, #120249, #136419, #43423, #90887, #180957, #123218, #26277, #13091, #76725, #198099, #152573, #164783, #87919, #149606, #14063, #104097, #75730, #137406, #122229, #11104, #196134, #45405, #153567, #57605, #138400, #195598, #163244, #12565, #88380, #178421, #57071, #148078, #40897, #56057, #117736, #102569, #179431, #24745, #196593, #118745, #164254, #86394, #74231, #131905, #70237, #193589, #133907, #119734, #89386, #26741, #105548, #72232, #180433, #42895, #39885, #25749, #9569, #71235, #147077, #104560, #101552, #87395, #132898, #194587, #8562, #181417, #135899, #197571, #43883, #149080, #10568, #166242, #27743, #41906, #103572, #165247, #150074, #11579, #73246, #55060, #134916, #58063, #151074, #59038, #120705, #182404, #167233, #85384, #116732, #90368, #64008, #139835, #113235, #46857, #140838, #14528, #44875, #15527, #77184, #1324, #63004, #128399, #121698, #123668, #185365, #108517, #62002, #109510, #32681, #2327, #154033, #138854, #190096, #170196, #152053, #155023, #51571, #13538, #31689, #93338, #28731, #75204, #60031, #334, #171192, #136875, #198561, #124682, #186379, #183393, #94334, #30696, #16519, #106531, #156012, #168208, #78167, #47857, #17509, #79167, #29705, #91336, #153028, #76189, #137869, #199548, #61018, #122690, #169189, #184379, #45860, #107513, #92347, #174926, #177933, #24253, #70746, #10079, #160745, #84886, #52562, #102076, #39400, #67734, #146565, #37398, #130386, #145568, #7046, #192083, #68728, #114222, #85903, #8060, #53565, #175927, #163761, #21237, #159740, #82892, #23242, #9076, #178935, #116241, #195097, #161747, #69737, #131405, #99057, #191088, #193093, #144570, #115243, #54569, #147591, #25261, #86904, #101060, #148587, #132414, #162745, #36389, #71737, #194106, #56579, #55569, #133408, #22237, #83886, #117242, #40405, #98043, #6056, #129392, #176935, #38405, #100062, #74733, #151578, #199062, #122207, #91853, #43398, #105068, #153545, #59541, #179944, #44394, #15042, #41411, #136397, #182909, #200060, #103076, #149580, #28256, #60531, #164758, #26253, #14038, #90865, #87894, #183898, #120227, #13067, #76703, #45383, #11078, #121219, #198074, #166753, #106048, #75704, #72754, #134425, #107036, #167734, #89895, #118253, #196111, #58561, #57581, #29232, #152550, #137383, #119251, #168708, #30210, #138379, #180935, #104073, #42410, #165755, #27249, #88898, #150589, #12088, #73751, #135423, #197094, #181917, #78685, #32203, #139366, #172704, #94856, #155537, #62520, #50360, #108028, #46369, #169714, #110030, #95849, #65508, #2847, #81646, #48373, #156537 ),
 ( #80673, #17031, #171708, #127169, #63531, #18036, #20003, #188879, #123197, #64525, #79690, #186902, #126192, #19027, #184887, #31207, #3829, #187888, #33198, #61528, #16040, #1849, #92858, #49355, #34188, #141360, #154545, #111018, #157533, #142349, #96831, #47378, #112019, #847, #173708, #35176, #77699, #158515, #124193, #140362, #93859, #125206, #143330, #185893, #109033, #170712, #38173, #98818, #5822, #193864, #51341, #189867, #113001, #53326, #39164, #8837, #146328, #25019, #191845, #99829, #162505, #97811, #175684, #82651, #144334, #66505, #100822, #55330, #117000, #163520, #67498, #190852, #24006, #85662, #160512, #115005, #176699, #129155, #20996, #161513, #174695, #83655, #23005, #177697, #132173, #178695, #84651, #40157, #54336, #192857, #128167, #101833, #116007, #86662, #7817, #4817, #52329, #113986, #69501, #131167, #147349, #70505, #36159, #159500, #37159, #22003, #145333, #6815, #68493, #130148, #121978, #73520, #135191, #183669, #89662, #9842, #74503, #45154, #71501, #104833, #12837, #29982, #133169, #179703, #58331, #90643, #194859, #56332, #44162, #120979, #118014, #29003, #27018, #152325, #41175, #102838, #196865, #148346, #151348, #164524, #26017, #166523, #136169, #42181, #87661, #197844, #59310, #106810, #182677, #119999, #149346, #57347, #11855, #105821, #10843, #167508, #60303, #180705, #28020, #13811, #72512, #75477, #150358, #137150, #134187, #198839, #181685, #168484, #195874, #119022, #103841, #165522, #88663, #43166, #15801, #50118, #49124, #157293, #171472, #107788, #18790, #61296, #80435, #48132, #93619, #155305, #139132, #30974, #94615, #188639, #185645, #140118, #109789, #170474, #91621, #63285, #47137, #609, #124965, #31964, #32961, #169473, #111778, #14810, #16794, #3593, #1609, #17795, #173466, #153309, #76471, #156294, #92621, #79451, #78444, #154312, #138148, #199829, #110782, #2611, #122966, #141121, #62279, #142108, #64288, #108795, #186662, #184653, #46135, #77462, #123947, #125955, #187653, #172463, #33950, #95608, #65271, #126931, #67259, #66268, #7574, #160273, #99590, #129905, #97571, #51103, #128917, #38931, #55095, #159259, #85420, #70271, #130926, #193623, #19769, #145092, #83415, #22764, #100588, #175446, #176456, #112763, #116765, #158280, #113750, #147111, #6575, #161270, #34939, #96591, #81410, #84413, #174456, #114762, #21764, #35925, #143096, #4575, #192617, #146090, #127927, #37929, #144099, #162270, #69260, #190618, #68254, #131939, #189629, #20755, #82410, #191605, #5579, #36916, #53084, #54099, #115773, #177462, #52093, #98579, #23770, #8597, #42930, #73281, #40933, #194622, #72267, #182437, #198596, #102605, #28764, #13571, #74265, #136909, #163280, #88418, #26776, #166281, #43917, #59071, #57107, #105579, #24781, #86428, #165283, #60064, #119768, #178456, #39923, #134951, #104594, #133944, #56093, #181452, #27778, #75238, #89420, #150112, #101592, #87430, #41941, #151109, #148114, #197605, #90401, #10606, #196629, #12601, #9605, #135935, #180469, #167265, #164291, #120738, #11613, #152086, #71270, #58098, #149115, #132935, #117774, #103607, #179468, #25784, #195634, #118781, #47891, #157048, #183424, #78200, #186414, #3355, #106565, #153062, #31723, #64043, #44908, #168242, #17543, #94367, #91371, #187412, #123702, #16553, #80192, #125713, #29738, #156046, #110535, #33700, #141864, #61051, #107547, #140873, #2362, #77218, #170230, #93371, #122723, #137901, #108551, #14564, #367, #155058, #79204, #48880, #172216, #1359, #95363, #171226, #109544, #76222, #18545, #32715, #121732, #139870, #199583, #169223, #184413, #63038, #124716, #45894, #30732, #92379, #154065, #15560, #138887, #62038, #185400, #46891, #99343, #115530, #190374, #51849, #100347, #6332, #126686, #191360, #162026, #188390, #21514, #129664, #146856, #49867, #96351, #175203, #7329, #111533, #173218, #161026, #37678, #34694, #130679, #67018, #160027, #23522, #69013 ),
 ( #52838, #142856, #144849, #113508, #4335, #85168, #65030, #22520, #176209, #158038, #68012, #174216, #192373, #114507, #20511, #36668, #19529, #81174, #66019, #127687, #98327, #189387, #5334, #83175, #84167, #145847, #53856, #97332, #50864, #177218, #38691, #112522, #35684, #159018, #82159, #143855, #128677, #28525, #132693, #58831, #43674, #104350, #167024, #193374, #118536, #73034, #86184, #88175, #133690, #147874, #90161, #8349, #166034, #119530, #70024, #11364, #117522, #135694, #134706, #164045, #56861, #105336, #116524, #131693, #54850, #180225, #194381, #148869, #165038, #181213, #41695, #89175, #40686, #39676, #42689, #195383, #196389, #103360, #71025, #24533, #102356, #12361, #178212, #55848, #120498, #101338, #27534, #163027, #9360, #26531, #149859, #57858, #74024, #150867, #87188, #197366, #179220, #25544, #182189, #10360, #72017, #151844, #13334, #108307, #77963, #45654, #29501, #154815, #93130, #48647, #139630, #61795, #74999, #60808, #15315, #16313, #136664, #170982, #63807, #184172, #169987, #1118, #121490, #47652, #153820, #155807, #14318, #32475, #138645, #125480, #33469, #187176, #78960, #107305, #110299, #75983, #137656, #171981, #109303, #17305, #31478, #168005, #140635, #183184, #2125, #62792, #76974, #126, #199343, #91134, #124473, #198346, #168977, #123465, #186170, #30482, #59820, #185157, #92133, #122481, #46647, #94128, #44666, #152824, #106319, #18309, #173979, #7092, #143610, #21278, #53611, #156817, #176980, #79965, #141634, #5094, #129434, #99101, #36430, #115287, #81917, #128438, #52606, #188158, #65780, #172983, #34461, #3124, #191132, #83932, #68773, #95127, #96120, #80947, #114268, #175972, #50628, #66777, #190135, #157808, #111294, #51610, #64799, #35447, #113274, #67777, #22281, #145613, #174966, #130431, #144613, #82935, #126460, #192130, #6098, #49631, #98085, #19299, #142622, #4101, #159783, #37441, #160793, #127449, #189155, #112289, #97099, #158783, #20271, #10120, #117283, #72796, #91649, #163802, #25304, #76502, #179986, #100105, #164800, #138178, #161789, #195140, #103119, #122996, #23284, #69779, #148630, #180974, #84928, #146608, #134466, #11121, #8101, #106838, #40444, #133450, #199860, #45184, #131447, #41454, #56621, #86946, #26295, #196151, #193134, #54607, #168513, #87936, #71780, #38450, #116281, #178977, #177971, #149623, #57623, #118295, #39439, #119291, #30011, #153338, #61325, #24293, #14839, #101099, #162785, #85942, #147631, #9119, #70786, #194145, #132454, #55609, #102117, #155338, #62309, #95641, #17829, #78478, #185677, #173500, #31002, #184682, #139162, #125000, #92651, #125989, #157329, #156329, #46165, #187687, #33985, #80469, #19802, #170505, #94649, #123979, #111812, #49157, #77492, #79487, #47167, #140151, #16827, #1643, #63321, #186695, #108826, #18824, #141156, #48166, #31996, #34973, #154340, #169503, #15833, #32995, #142142, #188673, #110815, #4609, #171506, #2645, #3626, #639, #109823, #93653, #64322, #107819, #65305, #96626, #158314, #143129, #172498, #126964, #50153, #81443, #66301, #176492, #37968, #67294, #144133, #114799, #112798, #6612, #99626, #100624, #55131, #178493, #7611, #39959, #177499, #115809, #189664, #163320, #38968, #9643, #146126, #101630, #113786, #5615, #161308, #22802, #162306, #23806, #24817, #20790, #84448, #69296, #130962, #192652, #68291, #85457, #86466, #53121, #54135, #148151, #147146, #51137, #8634, #127961, #174491, #70306, #131975, #35958, #97605, #159293, #193660, #116801, #82445, #128953, #190653, #52129, #175481, #36953, #129942, #98615, #160309, #21799, #83451, #145129, #191641, #196669, #135973, #28803, #194662, #117813, #13610, #197644, #119806, #150152, #105619, #121771, #58138, #181491, #106606, #12639, #132972, #59110, #168281, #56131, #27818, #120775, #153101, #179506, #102643, #42969, #75278, #40974, #164328, #167307, #43957, #25822, #136948, #73319, #166321, #29778, #198637 ),
 ( #11653, #87467, #74306, #182476, #104632, #71309, #90443, #152128, #60103, #91414, #57145, #89460, #149154, #183464, #44950, #10644, #151148, #133983, #26816, #41980, #103646, #88456, #165324, #72305, #195674, #118822, #134990, #180507, #3392, #61090, #199623, #122763, #63079, #48918, #18583, #156087, #34731, #1399, #47930, #172253, #107587, #185441, #92418, #154104, #76261, #110572, #65067, #126724, #173256, #15598, #405, #33741, #95401, #170267, #124758, #186454, #77256, #30771, #109584, #184452, #93410, #171267, #187450, #141901, #188428, #94406, #49906, #64080, #2402, #137939, #111572, #125750, #96389, #32755, #14605, #62077, #138925, #17584, #79244, #157087, #80230, #45932, #169265, #140915, #123742, #46931, #108590, #31761, #155096, #16590, #78238, #139909, #130719, #85208, #8388, #37719, #70063, #7368, #145885, #19567, #193413, #69053, #39712, #176248, #131731, #143892, #174255, #144888, #6370, #192412, #53894, #54888, #50902, #52877, #114549, #99381, #129704, #36706, #115569, #116562, #83213, #68050, #178251, #161064, #81211, #84205, #158076, #142892, #22559, #177256, #4374, #66058, #189427, #191400, #100386, #127725, #112560, #38728, #162064, #35723, #23560, #160066, #146897, #97370, #159056, #20550, #82200, #5373, #67057, #128715, #190412, #51888, #113547, #175241, #98368, #21553, #101375, #55886, #41731, #9396, #42726, #12399, #73070, #163065, #104388, #150905, #197403, #136702, #87224, #11401, #179259, #28562, #166071, #194416, #134742, #164081, #56897, #72053, #133727, #118571, #195419, #40724, #74061, #196424, #180261, #102393, #90199, #147910, #86220, #71062, #149894, #135732, #105374, #27573, #121527, #88210, #57894, #58869, #117559, #103395, #25580, #148906, #24571, #120535, #151882, #13372, #59860, #10396, #165073, #182228, #43713, #26567, #119566, #181249, #89212, #167061, #75036, #132728, #198383, #183222, #126496, #62830, #156851, #30520, #60844, #31516, #93169, #155844, #78997, #80001, #137695, #139667, #1155, #124513, #16352, #123502, #140671, #95163, #170026, #154854, #141670, #186209, #106357, #171022, #3161, #168041, #47690, #109340, #44703, #29538, #76020, #78000, #187211, #91171, #152860, #2163, #17341, #14355, #110334, #46686, #32513, #64834, #48682, #199380, #94165, #63842, #125514, #172015, #33504, #122519, #184209, #18346, #45691, #107342, #169015, #92171, #185195, #153857, #15355, #77011, #138683, #164, #61832, #108346, #83969, #23320, #174016, #98125, #65818, #115327, #191170, #80985, #159822, #50666, #143648, #158820, #20308, #5131, #81956, #127487, #99141, #21317, #66814, #189192, #177018, #34499, #173020, #96157, #36468, #22318, #192169, #129471, #8140, #175004, #82975, #145649, #142660, #128476, #112326, #35487, #49666, #7130, #38487, #100144, #146646, #97137, #190172, #68813, #130472, #51648, #144651, #6133, #113312, #4139, #67816, #157846, #52644, #114308, #160830, #161825, #84964, #176010, #69817, #37479, #188194, #53649, #111330, #19338, #149661, #134503, #101135, #27330, #133485, #135499, #194181, #12164, #118331, #43476, #13145, #105144, #58635, #86982, #166830, #55645, #117318, #89970, #88976, #197170, #11159, #147669, #120301, #162821, #181994, #87973, #195177, #56658, #179014, #70823, #196189, #28331, #25341, #180024, #72833, #10157, #131484, #103156, #148669, #40482, #164837, #71817, #57661, #9157, #151650, #54643, #41492, #193171, #26333, #119328, #116318, #178007, #39474, #181014, #132492, #42488, #104151, #102154, #24330, #85980, #150666, #165833, #163840, #73829, #183969, #1926, #139437, #30283, #123268, #171784, #182986, #33272, #136470, #184959, #199139, #15116, #31280, #47451, #46443, #155612, #107110, #106124, #109107, #200130, #919, #169787, #137460, #90938, #168780, #78759, #94931, #60606, #125281, #110105, #170786, #156616, #59620, #108103, #92931, #62593, #140436, #17107, #153620, #63605, #121293, #44470, #61599, #74808, #16112 ),
 ( #138449, #122281, #91928, #45456, #76777, #154618, #77770, #32276, #124271, #186978, #185967, #167808, #93933, #48448, #198150, #29308, #152625, #14115, #75782, #22076, #38244, #142426, #68566, #53402, #114063, #176772, #2923, #128242, #66577, #5896, #83727, #98893, #96904, #145406, #64601, #126265, #4895, #99899, #159576, #18111, #79765, #174766, #144410, #112094, #95923, #21073, #82729, #115080, #67572, #189939, #141436, #127245, #81721, #129230, #187962, #37237, #130223, #50435, #36232, #190927, #49432, #175761, #20077, #6888, #80748, #160587, #51414, #191919, #111093, #172783, #34264, #173784, #157608, #3905, #65585, #19099, #188958, #35251, #97884, #158588, #143407, #113074, #52404, #148419, #117071, #178767, #24081, #177768, #194931, #103911, #70578, #101909, #9914, #193938, #161584, #86734, #132246, #85736, #71573, #40233, #56407, #39237, #165592, #84723, #55401, #180775, #163591, #179778, #27090, #23078, #146401, #41247, #162577, #118088, #25092, #147423, #7891, #69576, #195946, #10912, #131242, #164593, #133239, #192930, #149416, #102909, #26087, #54408, #87731, #116080, #8910, #72585, #100893, #134259, #57420, #119093, #42250, #36881, #100556, #146057, #3559, #145060, #98547, #67226, #6541, #99556, #65237, #188603, #84380, #68221, #190584, #142073, #96557, #82378, #50084, #83383, #53050, #113716, #126897, #129873, #191571, #37898, #177428, #127893, #52060, #19735, #69226, #114730, #34902, #175413, #4539, #144066, #130894, #160241, #23735, #112730, #81376, #176424, #21730, #35892, #143061, #192584, #111744, #173432, #158244, #161238, #22732, #7541, #54067, #162235, #128884, #115741, #38899, #66233, #174423, #189596, #51069, #97539, #159226, #20721, #5547, #192393, #40706, #83195, #21535, #23541, #118554, #178231, #36688, #98348, #193393, #163047, #130698, #114528, #39695, #101357, #133709, #24554, #146877, #160047, #145866, #100366, #86203, #144869, #55867, #148888, #69033, #54869, #147893, #6352, #132711, #38709, #102376, #99362, #117541, #85187, #10379, #68032, #72036, #164064, #53875, #195402, #161045, #22539, #56880, #194399, #25563, #116543, #52857, #87207, #129683, #191381, #9379, #162045, #8369, #84186, #176229, #37699, #179240, #71044, #70044, #7348, #115549, #177237, #131712, #121509, #91154, #151863, #180244, #183204, #29520, #76003, #15337, #166053, #90180, #57877, #107325, #44685, #73053, #13354, #42708, #120517, #168998, #75018, #61815, #150887, #119549, #152843, #136683, #74043, #181232, #30502, #26549, #165056, #88193, #28544, #14337, #184192, #106338, #146, #167043, #198365, #137677, #134725, #12381, #104369, #27554, #41713, #199363, #60827, #89194, #59841, #168024, #135714, #122501, #45674, #197385, #92153, #153840, #58850, #196407, #76994, #149877, #182209, #138665, #103378, #11383, #43694, #105356, #35465, #173000, #111311, #185177, #158799, #34479, #5111, #141651, #97116, #109323, #139650, #110316, #171998, #96137, #157826, #20288, #16334, #18327, #79983, #3141, #95144, #2146, #19316, #173996, #48664, #33486, #81935, #64816, #46668, #49648, #143626, #108328, #126477, #188175, #123485, #170008, #154835, #156833, #65797, #31499, #93151, #80964, #142640, #77983, #189172, #125496, #4118, #1138, #127466, #62812, #50645, #112306, #124496, #186191, #47672, #171003, #32495, #187193, #94148, #155827, #17324, #78979, #140654, #63824, #115304, #23300, #145629, #66793, #38466, #22298, #114287, #100122, #7109, #8118, #144630, #25320, #190152, #68791, #178994, #176996, #193150, #86962, #128456, #148647, #131464, #6113, #146626, #192147, #67795, #51627, #113292, #24310, #177987, #174983, #69796, #175989, #194161, #54622, #83949, #161805, #163819, #36447, #21295, #98103, #102134, #116297, #130449, #84944, #39454, #101115, #147648, #99119, #159800, #162801, #53628, #85959, #9136, #129451, #82953, #160810, #70802, #191150, #52624, #117298, #37458, #132470, #55625, #40461 ),
 ( #149641, #26312, #197150, #195157, #88958, #120283, #182968, #137441, #60588, #89952, #122263, #59601, #198132, #71797, #45438, #121274, #91910, #28313, #183952, #196168, #87952, #58616, #181975, #44452, #106105, #107091, #103135, #105126, #166812, #151632, #43457, #150648, #167790, #168762, #135481, #13126, #30265, #74789, #133466, #136451, #10136, #56638, #41471, #118311, #29289, #12146, #90920, #152606, #14096, #75764, #42469, #164816, #199120, #180004, #11139, #72813, #134482, #57641, #104131, #119307, #180991, #165813, #27311, #73809, #49414, #112078, #138433, #63589, #1910, #169770, #186962, #902, #109091, #157592, #200114, #61582, #140420, #35234, #94914, #153603, #15099, #110088, #79749, #47434, #31264, #156600, #18094, #50419, #141419, #125264, #76759, #62576, #17090, #2906, #123251, #172767, #65567, #185950, #171767, #64584, #184942, #111077, #155595, #19083, #16096, #34247, #48432, #127227, #46427, #188942, #80731, #170770, #173768, #77754, #139420, #108086, #95907, #142410, #33256, #92915, #3888, #154600, #124255, #126249, #78743, #187945, #32259, #93917, #99884, #193922, #190910, #145389, #53386, #175742, #96888, #68550, #52387, #144393, #130206, #37220, #38229, #174750, #55385, #20060, #98875, #8894, #6871, #23062, #117055, #158571, #178750, #161569, #36214, #176756, #22060, #97867, #81704, #143387, #54392, #7874, #4879, #84707, #5878, #24065, #146386, #114044, #191901, #66561, #128226, #51398, #100878, #69560, #189923, #83711, #115064, #116065, #113058, #67555, #159557, #21055, #82710, #131225, #192915, #129212, #177753, #39222, #160571, #162560, #85720, #147406, #70562, #132229, #179761, #56389, #27074, #25075, #119076, #150415, #12893, #167564, #90697, #120053, #152380, #89718, #28077, #101893, #75532, #151403, #122034, #58386, #13865, #26071, #118071, #88720, #11910, #74556, #136223, #137207, #133223, #135247, #196919, #181740, #73574, #180758, #197898, #198893, #165575, #43221, #60361, #104889, #163575, #166577, #40214, #86718, #59367, #121036, #148403, #9897, #71558, #182734, #44218, #194914, #41231, #105877, #29057, #102892, #164577, #42234, #87714, #149400, #10895, #72568, #134243, #195928, #57404, #103895, #141180, #106864, #30036, #126016, #109846, #32023, #183724, #138205, #124006, #91674, #125025, #94674, #155364, #45210, #186721, #33019, #79510, #18849, #169529, #93681, #61351, #110841, #48192, #76528, #16853, #46192, #185704, #172525, #78504, #65330, #154367, #123022, #156353, #140177, #77519, #184707, #34010, #153365, #168538, #14867, #1670, #17854, #47193, #95667, #63348, #199887, #15861, #107845, #2670, #171531, #139191, #31029, #157354, #92679, #666, #62336, #64347, #187711, #49183, #80494, #3652, #170533, #142168, #108853, #19826, #97628, #4634, #66324, #188697, #161330, #22823, #112821, #83474, #114822, #174514, #146147, #7634, #82468, #175503, #36977, #127985, #143153, #113808, #111835, #5639, #98637, #99647, #54158, #177520, #6635, #38990, #176514, #37991, #50178, #162327, #84469, #8655, #145151, #100646, #35981, #189688, #160332, #21822, #69318, #130984, #23828, #81467, #68313, #129964, #191664, #53143, #67316, #192675, #85478, #52151, #115831, #147167, #126990, #173524, #34995, #96649, #158337, #51161, #159317, #20812, #144154, #128976, #190675, #12660, #131996, #193682, #166343, #42991, #39979, #135994, #72327, #165344, #28825, #74327, #55152, #73340, #26837, #195694, #135013, #27840, #116822, #178513, #197665, #196690, #118844, #70329, #24836, #10664, #101649, #11674, #181512, #42000, #163341, #58159, #119827, #89481, #105640, #56151, #180527, #148171, #59131, #104656, #86486, #103666, #132991, #182499, #120798, #25843, #43978, #194682, #117833, #90465, #151172, #167329, #150174, #9662, #152149, #71329, #179526, #88477, #134003, #57165, #40995, #102663, #164348, #87487, #149175, #62101, #170290, #92441, #13632, #185463, #169287, #61112, #46954, #154127 ),
 ( #93433, #138947, #153123, #172276, #75299, #171290, #124780, #33765, #16613, #122785, #140938, #78260, #30793, #123764, #110594, #121793, #168303, #44971, #48941, #63102, #15621, #31784, #186478, #108613, #94429, #45954, #106629, #47955, #427, #139933, #155119, #76284, #29800, #107609, #17607, #95425, #137963, #64105, #136970, #109606, #198660, #60126, #1422, #32777, #91436, #156110, #184475, #77278, #79267, #183487, #14627, #2425, #199646, #125772, #187472, #157109, #116336, #85999, #53668, #34753, #162840, #101153, #56676, #147688, #69835, #80253, #68832, #23338, #24348, #18605, #179034, #71835, #192187, #178025, #9175, #126748, #55664, #161844, #163860, #22337, #40500, #146664, #133504, #41512, #141923, #3414, #188450, #131502, #102172, #65089, #49930, #117338, #132510, #111595, #25359, #84982, #54662, #118349, #87000, #173280, #70842, #39493, #8159, #194199, #148687, #96412, #160848, #10175, #180043, #83988, #145667, #195196, #7148, #130491, #193189, #115346, #177036, #38506, #100162, #14132, #61617, #106144, #12183, #30302, #167826, #58653, #151669, #200147, #11177, #57680, #134522, #138466, #152642, #43496, #59638, #75799, #74827, #183988, #135518, #196208, #137477, #28350, #29326, #198168, #165852, #119348, #197189, #107127, #123285, #27348, #153638, #184976, #199157, #103175, #87991, #13163, #136488, #181032, #121312, #150685, #120319, #168798, #149679, #72852, #89988, #164855, #44488, #26351, #42506, #183004, #90955, #182013, #104170, #60624, #122298, #88994, #45473, #91945, #73847, #105162, #166848, #15133, #76795, #65601, #158603, #78777, #64619, #49447, #16130, #142443, #48465, #50450, #109125, #127261, #33288, #20093, #128257, #81737, #173800, #1943, #143423, #170803, #32295, #4910, #3921, #112109, #126281, #62609, #35266, #77785, #96921, #2939, #66593, #154635, #935, #139454, #46461, #95939, #186995, #187978, #19115, #18127, #188974, #140453, #124288, #80765, #171800, #111110, #141454, #93951, #185985, #63623, #108121, #169804, #155629, #31297, #92949, #47468, #17125, #125299, #156632, #94948, #110122, #79782, #172799, #34280, #157625, #36247, #174781, #176787, #71589, #131258, #189955, #51429, #146416, #116095, #83742, #67588, #192946, #54425, #86752, #177783, #99914, #113089, #98909, #53418, #39253, #97900, #8927, #101925, #22092, #7907, #100909, #159591, #85752, #191934, #193954, #52419, #70595, #38260, #163607, #21088, #25108, #117088, #145421, #148435, #114077, #175778, #9930, #147439, #55417, #69591, #5911, #178783, #82745, #40251, #162593, #115095, #161599, #37252, #129246, #24098, #144425, #6903, #23093, #132263, #68582, #190942, #84738, #130238, #160602, #166604, #73601, #74580, #10926, #91703, #56422, #11938, #122059, #182760, #72599, #153397, #194946, #14895, #197924, #134273, #12916, #58413, #195960, #133255, #118102, #90721, #44244, #179792, #136248, #42264, #60387, #59392, #88749, #181768, #135273, #28104, #41261, #137234, #102923, #121066, #89743, #120080, #105901, #152404, #164608, #196945, #13891, #43249, #167587, #26102, #87745, #104917, #149430, #29082, #75558, #151429, #57433, #198918, #183751, #45237, #168564, #119106, #106891, #180787, #30062, #103924, #165604, #27103, #150442, #16880, #3680, #171557, #158367, #47223, #154394, #187739, #109873, #170561, #77547, #65358, #123049, #61378, #184735, #125052, #110868, #80523, #17884, #96679, #63375, #33047, #34039, #169561, #108882, #15889, #139219, #138232, #172553, #95696, #62366, #94702, #64375, #124035, #157384, #18877, #32051, #186749, #48219, #694, #92706, #156379, #46220, #155390, #79538, #49210, #127019, #188726, #141208, #50211, #126043, #142197, #199914, #111865, #173555, #76556, #2698, #35024, #185734, #93708, #107873, #31058, #78531, #140205, #1699, #112852, #114851, #176545, #38021, #191692, #98668, #54187, #70357, #145180, #6664, #55182, #161361, #81496, #146177, #116851, #143183, #99677, #84499 ) ),
 .UNSPECIFIED., .T., .F., .F. ) 
 B_SPLINE_SURFACE_WITH_KNOTS ( ( 4, 3, 4 ),
 ( 3, 2, 2, 2, 2, 2, 2, 2, 2, 2, 2, 2, 2, 2, 2, 2, 2, 2, 2, 2, 2, 2, 2, 2, 2, 2, 2, 2, 2, 2, 2, 2, 2, 2, 2, 2, 2, 2, 2, 2, 2, 2, 2, 2, 2, 2, 2, 2, 2, 2, 2, 2, 2, 2, 2, 2, 2, 2, 2, 2, 2, 2, 2, 2, 2, 2, 2, 2, 2, 2, 2, 2, 2, 2, 2, 2, 2, 2, 2, 2, 2, 2, 2, 2, 2, 2, 2, 2, 2, 2, 2, 2, 2, 2, 2, 2, 2, 2, 2, 2, 2, 2, 2, 2, 2, 2, 2, 2, 2, 2, 2, 2, 2, 2, 2, 2, 2, 2, 2, 2, 2, 2, 2, 2, 2, 2, 2, 2, 2, 2, 2, 2, 2, 2, 2, 2, 2, 2, 2, 2, 2, 2, 2, 2, 2, 2, 2, 2, 2, 2, 2, 2, 2, 2, 2, 2, 2, 2, 2, 2, 2, 2, 2, 2, 2, 2, 2, 2, 2, 2, 2, 2, 2, 2, 2, 2, 2, 2, 2, 2, 2, 2, 2, 2, 2, 2, 2, 2, 2, 2, 2, 2, 2, 2, 2, 2, 2, 2, 2, 2, 2, 2, 2, 2, 2, 2, 2, 2, 2, 2, 2, 2, 2, 2, 2, 2, 2, 2, 2, 2, 2, 2, 2, 2, 2, 2, 2, 2, 3 ),
 ( 0.000000000000000000, 0.5000000000000000000, 1.000000000000000000 ),
 ( 0.000000000000000000, 0.004385964912280701511, 0.008771929824561403022, 0.01315789473684210453, 0.01754385964912280604, 0.02192982456140350755, 0.02631578947368420907, 0.03070175438596491058, 0.03508771929824561209, 0.03947368421052631360, 0.04385964912280701511, 0.04824561403508771662, 0.05263157894736841813, 0.05701754385964911964, 0.06140350877192982115, 0.06578947368421052266, 0.07017543859649122417, 0.07456140350877192569, 0.07894736842105262720, 0.08333333333333332871, 0.08771929824561403022, 0.09210526315789473173, 0.09649122807017543324, 0.1008771929824561348, 0.1052631578947368363, 0.1096491228070175378, 0.1140350877192982393, 0.1184210526315789408, 0.1228070175438596423, 0.1271929824561403577, 0.1315789473684210453, 0.1359649122807017607, 0.1403508771929824483, 0.1447368421052631637, 0.1491228070175438514, 0.1535087719298245668, 0.1578947368421052544, 0.1622807017543859698, 0.1666666666666666574, 0.1710526315789473728, 0.1754385964912280604, 0.1798245614035087758, 0.1842105263157894635, 0.1885964912280701788, 0.1929824561403508665, 0.1973684210526315819, 0.2017543859649122695, 0.2061403508771929849, 0.2105263157894736725, 0.2149122807017543879, 0.2192982456140350755, 0.2236842105263157909, 0.2280701754385964786, 0.2324561403508771940, 0.2368421052631578816, 0.2412280701754385970, 0.2456140350877192846, 0.2500000000000000000, 0.2543859649122807154, 0.2587719298245614308, 0.2631578947368420907, 0.2675438596491228060, 0.2719298245614035214, 0.2763157894736842368, 0.2807017543859648967, 0.2850877192982456121, 0.2894736842105263275, 0.2938596491228070429, 0.2982456140350877027, 0.3026315789473684181, 0.3070175438596491335, 0.3114035087719298489, 0.3157894736842105088, 0.3201754385964912242, 0.3245614035087719396, 0.3289473684210526550, 0.3333333333333333148, 0.3377192982456140302, 0.3421052631578947456, 0.3464912280701754610, 0.3508771929824561209, 0.3552631578947368363, 0.3596491228070175517, 0.3640350877192982670, 0.3684210526315789269, 0.3728070175438596423, 0.3771929824561403577, 0.3815789473684210731, 0.3859649122807017330, 0.3903508771929824483, 0.3947368421052631637, 0.3991228070175438791, 0.4035087719298245390, 0.4078947368421052544, 0.4122807017543859698, 0.4166666666666666852, 0.4210526315789473450, 0.4254385964912280604, 0.4298245614035087758, 0.4342105263157894912, 0.4385964912280701511, 0.4429824561403508665, 0.4473684210526315819, 0.4517543859649122973, 0.4561403508771929571, 0.4605263157894736725, 0.4649122807017543879, 0.4692982456140351033, 0.4736842105263157632, 0.4780701754385964786, 0.4824561403508771940, 0.4868421052631579093, 0.4912280701754385692, 0.4956140350877192846, 0.5000000000000000000, 0.5043859649122807154, 0.5087719298245614308, 0.5131578947368421462, 0.5175438596491228616, 0.5219298245614034659, 0.5263157894736841813, 0.5307017543859648967, 0.5350877192982456121, 0.5394736842105263275, 0.5438596491228070429, 0.5482456140350877583, 0.5526315789473684736, 0.5570175438596490780, 0.5614035087719297934, 0.5657894736842105088, 0.5701754385964912242, 0.5745614035087719396, 0.5789473684210526550, 0.5833333333333333703, 0.5877192982456140857, 0.5921052631578946901, 0.5964912280701754055, 0.6008771929824561209, 0.6052631578947368363, 0.6096491228070175517, 0.6140350877192982670, 0.6184210526315789824, 0.6228070175438596978, 0.6271929824561403022, 0.6315789473684210176, 0.6359649122807017330, 0.6403508771929824483, 0.6447368421052631637, 0.6491228070175438791, 0.6535087719298245945, 0.6578947368421053099, 0.6622807017543859143, 0.6666666666666666297, 0.6710526315789473450, 0.6754385964912280604, 0.6798245614035087758, 0.6842105263157894912, 0.6885964912280702066, 0.6929824561403509220, 0.6973684210526315264, 0.7017543859649122417, 0.7061403508771929571, 0.7105263157894736725, 0.7149122807017543879, 0.7192982456140351033, 0.7236842105263158187, 0.7280701754385965341, 0.7324561403508771384, 0.7368421052631578538, 0.7412280701754385692, 0.7456140350877192846, 0.7500000000000000000, 0.7543859649122807154, 0.7587719298245614308, 0.7631578947368421462, 0.7675438596491228616, 0.7719298245614034659, 0.7763157894736841813, 0.7807017543859648967, 0.7850877192982456121, 0.7894736842105263275, 0.7938596491228070429, 0.7982456140350877583, 0.8026315789473684736, 0.8070175438596490780, 0.8114035087719297934, 0.8157894736842105088, 0.8201754385964912242, 0.8245614035087719396, 0.8289473684210526550, 0.8333333333333333703, 0.8377192982456140857, 0.8421052631578946901, 0.8464912280701754055, 0.8508771929824561209, 0.8552631578947368363, 0.8596491228070175517, 0.8640350877192982670, 0.8684210526315789824, 0.8728070175438596978, 0.8771929824561403022, 0.8815789473684210176, 0.8859649122807017330, 0.8903508771929824483, 0.8947368421052631637, 0.8991228070175438791, 0.9035087719298245945, 0.9078947368421053099, 0.9122807017543859143, 0.9166666666666666297, 0.9210526315789473450, 0.9254385964912280604, 0.9298245614035087758, 0.9342105263157894912, 0.9385964912280702066, 0.9429824561403509220, 0.9473684210526315264, 0.9517543859649122417, 0.9561403508771929571, 0.9605263157894736725, 0.9649122807017543879, 0.9692982456140351033, 0.9736842105263158187, 0.9780701754385965341, 0.9824561403508771384, 0.9868421052631578538, 0.9912280701754385692, 0.9956140350877192846, 1.000000000000000000 ),
 .UNSPECIFIED. ) 
 GEOMETRIC_REPRESENTATION_ITEM ( )  RATIONAL_B_SPLINE_SURFACE ( (
 ( 1.000000000000000000, 0.9659258262890683122, 1.000000000000000000, 0.9659258262890683122, 1.000000000000000000, 0.9659258262890683122, 1.000000000000000000, 0.9659258262890683122, 1.000000000000000000, 0.9659258262890683122, 1.000000000000000000, 0.9659258262890683122, 1.000000000000000000, 0.9659258262890683122, 1.000000000000000000, 0.9659258262890683122, 1.000000000000000000, 0.9659258262890683122, 1.000000000000000000, 0.9659258262890683122, 1.000000000000000000, 0.9659258262890683122, 1.000000000000000000, 0.9659258262890683122, 1.000000000000000000, 0.9659258262890683122, 1.000000000000000000, 0.9659258262890683122, 1.000000000000000000, 0.9659258262890683122, 1.000000000000000000, 0.9659258262890683122, 1.000000000000000000, 0.9659258262890683122, 1.000000000000000000, 0.9659258262890683122, 1.000000000000000000, 0.9659258262890683122, 1.000000000000000000, 0.9659258262890683122, 1.000000000000000000, 0.9659258262890683122, 1.000000000000000000, 0.9659258262890683122, 1.000000000000000000, 0.9659258262890683122, 1.000000000000000000, 0.9659258262890683122, 1.000000000000000000, 0.9659258262890683122, 1.000000000000000000, 0.9659258262890683122, 1.000000000000000000, 0.9659258262890683122, 1.000000000000000000, 0.9659258262890683122, 1.000000000000000000, 0.9659258262890683122, 1.000000000000000000, 0.9659258262890683122, 1.000000000000000000, 0.9659258262890683122, 1.000000000000000000, 0.9659258262890683122, 1.000000000000000000, 0.9659258262890683122, 1.000000000000000000, 0.9659258262890683122, 1.000000000000000000, 0.9659258262890683122, 1.000000000000000000, 0.9659258262890683122, 1.000000000000000000, 0.9659258262890683122, 1.000000000000000000, 0.9659258262890683122, 1.000000000000000000, 0.9659258262890683122, 1.000000000000000000, 0.9659258262890683122, 1.000000000000000000, 0.9659258262890683122, 1.000000000000000000, 0.9659258262890683122, 1.000000000000000000, 0.9659258262890683122, 1.000000000000000000, 0.9659258262890683122, 1.000000000000000000, 0.9659258262890683122, 1.000000000000000000, 0.9659258262890683122, 1.000000000000000000, 0.9659258262890683122, 1.000000000000000000, 0.9659258262890683122, 1.000000000000000000, 0.9659258262890683122, 1.000000000000000000, 0.9659258262890683122, 1.000000000000000000, 0.9659258262890683122, 1.000000000000000000, 0.9659258262890683122, 1.000000000000000000, 0.9659258262890683122, 1.000000000000000000, 0.9659258262890683122, 1.000000000000000000, 0.9659258262890683122, 1.000000000000000000, 0.9659258262890683122, 1.000000000000000000, 0.9659258262890683122, 1.000000000000000000, 0.9659258262890683122, 1.000000000000000000, 0.9659258262890683122, 1.000000000000000000, 0.9659258262890683122, 1.000000000000000000, 0.9659258262890683122, 1.000000000000000000, 0.9659258262890683122, 1.000000000000000000, 0.9659258262890683122, 1.000000000000000000, 0.9659258262890683122, 1.000000000000000000, 0.9659258262890683122, 1.000000000000000000, 0.9659258262890683122, 1.000000000000000000, 0.9659258262890683122, 1.000000000000000000, 0.9659258262890683122, 1.000000000000000000, 0.9659258262890683122, 1.000000000000000000, 0.9659258262890683122, 1.000000000000000000, 0.9659258262890683122, 1.000000000000000000, 0.9659258262890683122, 1.000000000000000000, 0.9659258262890683122, 1.000000000000000000, 0.9659258262890683122, 1.000000000000000000, 0.9659258262890683122, 1.000000000000000000, 0.9659258262890683122, 1.000000000000000000, 0.9659258262890683122, 1.000000000000000000, 0.9659258262890683122, 1.000000000000000000, 0.9659258262890683122, 1.000000000000000000, 0.9659258262890683122, 1.000000000000000000, 0.9659258262890683122, 1.000000000000000000, 0.9659258262890683122, 1.000000000000000000, 0.9659258262890683122, 1.000000000000000000, 0.9659258262890683122, 1.000000000000000000, 0.9659258262890683122, 1.000000000000000000, 0.9659258262890683122, 1.000000000000000000, 0.9659258262890683122, 1.000000000000000000, 0.9659258262890683122, 1.000000000000000000, 0.9659258262890683122, 1.000000000000000000, 0.9659258262890683122, 1.000000000000000000, 0.9659258262890683122, 1.000000000000000000, 0.9659258262890683122, 1.000000000000000000, 0.9659258262890683122, 1.000000000000000000, 0.9659258262890683122, 1.000000000000000000, 0.9659258262890683122, 1.000000000000000000, 0.9659258262890683122, 1.000000000000000000, 0.9659258262890683122, 1.000000000000000000, 0.9659258262890683122, 1.000000000000000000, 0.9659258262890683122, 1.000000000000000000, 0.9659258262890683122, 1.000000000000000000, 0.9659258262890683122, 1.000000000000000000, 0.9659258262890683122, 1.000000000000000000, 0.9659258262890683122, 1.000000000000000000, 0.9659258262890683122, 1.000000000000000000, 0.9659258262890683122, 1.000000000000000000, 0.9659258262890683122, 1.000000000000000000, 0.9659258262890683122, 1.000000000000000000, 0.9659258262890683122, 1.000000000000000000, 0.9659258262890683122, 1.000000000000000000, 0.9659258262890683122, 1.000000000000000000, 0.9659258262890683122, 1.000000000000000000, 0.9659258262890683122, 1.000000000000000000, 0.9659258262890683122, 1.000000000000000000, 0.9659258262890683122, 1.000000000000000000, 0.9659258262890683122, 1.000000000000000000, 0.9659258262890683122, 1.000000000000000000, 0.9659258262890683122, 1.000000000000000000, 0.9659258262890683122, 1.000000000000000000, 0.9659258262890683122, 1.000000000000000000, 0.9659258262890683122, 1.000000000000000000, 0.9659258262890683122, 1.000000000000000000, 0.9659258262890683122, 1.000000000000000000, 0.9659258262890683122, 1.000000000000000000, 0.9659258262890683122, 1.000000000000000000, 0.9659258262890683122, 1.000000000000000000, 0.9659258262890683122, 1.000000000000000000, 0.9659258262890683122, 1.000000000000000000, 0.9659258262890683122, 1.000000000000000000, 0.9659258262890683122, 1.000000000000000000, 0.9659258262890683122, 1.000000000000000000, 0.9659258262890683122, 1.000000000000000000, 0.9659258262890683122, 1.000000000000000000, 0.9659258262890683122, 1.000000000000000000, 0.9659258262890683122, 1.000000000000000000, 0.9659258262890683122, 1.000000000000000000, 0.9659258262890683122, 1.000000000000000000, 0.9659258262890683122, 1.000000000000000000, 0.9659258262890683122, 1.000000000000000000, 0.9659258262890683122, 1.000000000000000000, 0.9659258262890683122, 1.000000000000000000, 0.9659258262890683122, 1.000000000000000000, 0.9659258262890683122, 1.000000000000000000, 0.9659258262890683122, 1.000000000000000000, 0.9659258262890683122, 1.000000000000000000, 0.9659258262890683122, 1.000000000000000000, 0.9659258262890683122, 1.000000000000000000, 0.9659258262890683122, 1.000000000000000000, 0.9659258262890683122, 1.000000000000000000, 0.9659258262890683122, 1.000000000000000000, 0.9659258262890683122, 1.000000000000000000, 0.9659258262890683122, 1.000000000000000000, 0.9659258262890683122, 1.000000000000000000, 0.9659258262890683122, 1.000000000000000000, 0.9659258262890683122, 1.000000000000000000, 0.9659258262890683122, 1.000000000000000000, 0.9659258262890683122, 1.000000000000000000, 0.9659258262890683122, 1.000000000000000000, 0.9659258262890683122, 1.000000000000000000, 0.9659258262890683122, 1.000000000000000000, 0.9659258262890683122, 1.000000000000000000, 0.9659258262890683122, 1.000000000000000000, 0.9659258262890683122, 1.000000000000000000, 0.9659258262890683122, 1.000000000000000000, 0.9659258262890683122, 1.000000000000000000, 0.9659258262890683122, 1.000000000000000000, 0.9659258262890683122, 1.000000000000000000, 0.9659258262890683122, 1.000000000000000000, 0.9659258262890683122, 1.000000000000000000, 0.9659258262890683122, 1.000000000000000000, 0.9659258262890683122, 1.000000000000000000, 0.9659258262890683122, 1.000000000000000000, 0.9659258262890683122, 1.000000000000000000, 0.9659258262890683122, 1.000000000000000000, 0.9659258262890683122, 1.000000000000000000, 0.9659258262890683122, 1.000000000000000000, 0.9659258262890683122, 1.000000000000000000, 0.9659258262890683122, 1.000000000000000000, 0.9659258262890683122, 1.000000000000000000, 0.9659258262890683122, 1.000000000000000000, 0.9659258262890683122, 1.000000000000000000, 0.9659258262890683122, 1.000000000000000000, 0.9659258262890683122, 1.000000000000000000, 0.9659258262890683122, 1.000000000000000000, 0.9659258262890683122, 1.000000000000000000, 0.9659258262890683122, 1.000000000000000000, 0.9659258262890683122, 1.000000000000000000, 0.9659258262890683122, 1.000000000000000000, 0.9659258262890683122, 1.000000000000000000, 0.9659258262890683122, 1.000000000000000000, 0.9659258262890683122, 1.000000000000000000, 0.9659258262890683122, 1.000000000000000000, 0.9659258262890683122, 1.000000000000000000, 0.9659258262890683122, 1.000000000000000000, 0.9659258262890683122, 1.000000000000000000, 0.9659258262890683122, 1.000000000000000000, 0.9659258262890683122, 1.000000000000000000, 0.9659258262890683122, 1.000000000000000000, 0.9659258262890683122, 1.000000000000000000, 0.9659258262890683122, 1.000000000000000000, 0.9659258262890683122, 1.000000000000000000, 0.9659258262890683122, 1.000000000000000000, 0.9659258262890683122, 1.000000000000000000, 0.9659258262890683122, 1.000000000000000000, 0.9659258262890683122, 1.000000000000000000, 0.9659258262890683122, 1.000000000000000000, 0.9659258262890683122, 1.000000000000000000, 0.9659258262890683122, 1.000000000000000000, 0.9659258262890683122, 1.000000000000000000, 0.9659258262890683122, 1.000000000000000000, 0.9659258262890683122, 1.000000000000000000, 0.9659258262890683122, 1.000000000000000000, 0.9659258262890683122, 1.000000000000000000, 0.9659258262890683122, 1.000000000000000000, 0.9659258262890683122, 1.000000000000000000, 0.9659258262890683122, 1.000000000000000000, 0.9659258262890683122, 1.000000000000000000, 0.9659258262890683122, 1.000000000000000000, 0.9659258262890683122, 1.000000000000000000, 0.9659258262890683122, 1.000000000000000000, 0.9659258262890683122, 1.000000000000000000, 0.9659258262890683122, 1.000000000000000000, 0.9659258262890683122, 1.000000000000000000, 0.9659258262890683122, 1.000000000000000000, 0.9659258262890683122, 1.000000000000000000, 0.9659258262890683122, 1.000000000000000000, 0.9659258262890683122, 1.000000000000000000, 0.9659258262890683122, 1.000000000000000000, 0.9659258262890683122, 1.000000000000000000),
 ( 0.3333333333333333703, 0.3219752754296894559, 0.3333333333333333703, 0.3219752754296894559, 0.3333333333333333703, 0.3219752754296894559, 0.3333333333333333703, 0.3219752754296894559, 0.3333333333333333703, 0.3219752754296894559, 0.3333333333333333703, 0.3219752754296894559, 0.3333333333333333703, 0.3219752754296894559, 0.3333333333333333703, 0.3219752754296894559, 0.3333333333333333703, 0.3219752754296894559, 0.3333333333333333703, 0.3219752754296894559, 0.3333333333333333703, 0.3219752754296894559, 0.3333333333333333703, 0.3219752754296894559, 0.3333333333333333703, 0.3219752754296894559, 0.3333333333333333703, 0.3219752754296894559, 0.3333333333333333703, 0.3219752754296894559, 0.3333333333333333703, 0.3219752754296894559, 0.3333333333333333703, 0.3219752754296894559, 0.3333333333333333703, 0.3219752754296894559, 0.3333333333333333703, 0.3219752754296894559, 0.3333333333333333703, 0.3219752754296894559, 0.3333333333333333703, 0.3219752754296894559, 0.3333333333333333703, 0.3219752754296894559, 0.3333333333333333703, 0.3219752754296894559, 0.3333333333333333703, 0.3219752754296894559, 0.3333333333333333703, 0.3219752754296894559, 0.3333333333333333703, 0.3219752754296894559, 0.3333333333333333703, 0.3219752754296894559, 0.3333333333333333703, 0.3219752754296894559, 0.3333333333333333703, 0.3219752754296894559, 0.3333333333333333703, 0.3219752754296894559, 0.3333333333333333703, 0.3219752754296894559, 0.3333333333333333703, 0.3219752754296894559, 0.3333333333333333703, 0.3219752754296894559, 0.3333333333333333703, 0.3219752754296894559, 0.3333333333333333703, 0.3219752754296894559, 0.3333333333333333703, 0.3219752754296894559, 0.3333333333333333703, 0.3219752754296894559, 0.3333333333333333703, 0.3219752754296894559, 0.3333333333333333703, 0.3219752754296894559, 0.3333333333333333703, 0.3219752754296894559, 0.3333333333333333703, 0.3219752754296894559, 0.3333333333333333703, 0.3219752754296894559, 0.3333333333333333703, 0.3219752754296894559, 0.3333333333333333703, 0.3219752754296894559, 0.3333333333333333703, 0.3219752754296894559, 0.3333333333333333703, 0.3219752754296894559, 0.3333333333333333703, 0.3219752754296894559, 0.3333333333333333703, 0.3219752754296894559, 0.3333333333333333703, 0.3219752754296894559, 0.3333333333333333703, 0.3219752754296894559, 0.3333333333333333703, 0.3219752754296894559, 0.3333333333333333703, 0.3219752754296894559, 0.3333333333333333703, 0.3219752754296894559, 0.3333333333333333703, 0.3219752754296894559, 0.3333333333333333703, 0.3219752754296894559, 0.3333333333333333703, 0.3219752754296894559, 0.3333333333333333703, 0.3219752754296894559, 0.3333333333333333703, 0.3219752754296894559, 0.3333333333333333703, 0.3219752754296894559, 0.3333333333333333703, 0.3219752754296894559, 0.3333333333333333703, 0.3219752754296894559, 0.3333333333333333703, 0.3219752754296894559, 0.3333333333333333703, 0.3219752754296894559, 0.3333333333333333703, 0.3219752754296894559, 0.3333333333333333703, 0.3219752754296894559, 0.3333333333333333703, 0.3219752754296894559, 0.3333333333333333703, 0.3219752754296894559, 0.3333333333333333703, 0.3219752754296894559, 0.3333333333333333703, 0.3219752754296894559, 0.3333333333333333703, 0.3219752754296894559, 0.3333333333333333703, 0.3219752754296894559, 0.3333333333333333703, 0.3219752754296894559, 0.3333333333333333703, 0.3219752754296894559, 0.3333333333333333703, 0.3219752754296894559, 0.3333333333333333703, 0.3219752754296894559, 0.3333333333333333703, 0.3219752754296894559, 0.3333333333333333703, 0.3219752754296894559, 0.3333333333333333703, 0.3219752754296894559, 0.3333333333333333703, 0.3219752754296894559, 0.3333333333333333703, 0.3219752754296894559, 0.3333333333333333703, 0.3219752754296894559, 0.3333333333333333703, 0.3219752754296894559, 0.3333333333333333703, 0.3219752754296894559, 0.3333333333333333703, 0.3219752754296894559, 0.3333333333333333703, 0.3219752754296894559, 0.3333333333333333703, 0.3219752754296894559, 0.3333333333333333703, 0.3219752754296894559, 0.3333333333333333703, 0.3219752754296894559, 0.3333333333333333703, 0.3219752754296894559, 0.3333333333333333703, 0.3219752754296894559, 0.3333333333333333703, 0.3219752754296894559, 0.3333333333333333703, 0.3219752754296894559, 0.3333333333333333703, 0.3219752754296894559, 0.3333333333333333703, 0.3219752754296894559, 0.3333333333333333703, 0.3219752754296894559, 0.3333333333333333703, 0.3219752754296894559, 0.3333333333333333703, 0.3219752754296894559, 0.3333333333333333703, 0.3219752754296894559, 0.3333333333333333703, 0.3219752754296894559, 0.3333333333333333703, 0.3219752754296894559, 0.3333333333333333703, 0.3219752754296894559, 0.3333333333333333703, 0.3219752754296894559, 0.3333333333333333703, 0.3219752754296894559, 0.3333333333333333703, 0.3219752754296894559, 0.3333333333333333703, 0.3219752754296894559, 0.3333333333333333703, 0.3219752754296894559, 0.3333333333333333703, 0.3219752754296894559, 0.3333333333333333703, 0.3219752754296894559, 0.3333333333333333703, 0.3219752754296894559, 0.3333333333333333703, 0.3219752754296894559, 0.3333333333333333703, 0.3219752754296894559, 0.3333333333333333703, 0.3219752754296894559, 0.3333333333333333703, 0.3219752754296894559, 0.3333333333333333703, 0.3219752754296894559, 0.3333333333333333703, 0.3219752754296894559, 0.3333333333333333703, 0.3219752754296894559, 0.3333333333333333703, 0.3219752754296894559, 0.3333333333333333703, 0.3219752754296894559, 0.3333333333333333703, 0.3219752754296894559, 0.3333333333333333703, 0.3219752754296894559, 0.3333333333333333703, 0.3219752754296894559, 0.3333333333333333703, 0.3219752754296894559, 0.3333333333333333703, 0.3219752754296894559, 0.3333333333333333703, 0.3219752754296894559, 0.3333333333333333703, 0.3219752754296894559, 0.3333333333333333703, 0.3219752754296894559, 0.3333333333333333703, 0.3219752754296894559, 0.3333333333333333703, 0.3219752754296894559, 0.3333333333333333703, 0.3219752754296894559, 0.3333333333333333703, 0.3219752754296894559, 0.3333333333333333703, 0.3219752754296894559, 0.3333333333333333703, 0.3219752754296894559, 0.3333333333333333703, 0.3219752754296894559, 0.3333333333333333703, 0.3219752754296894559, 0.3333333333333333703, 0.3219752754296894559, 0.3333333333333333703, 0.3219752754296894559, 0.3333333333333333703, 0.3219752754296894559, 0.3333333333333333703, 0.3219752754296894559, 0.3333333333333333703, 0.3219752754296894559, 0.3333333333333333703, 0.3219752754296894559, 0.3333333333333333703, 0.3219752754296894559, 0.3333333333333333703, 0.3219752754296894559, 0.3333333333333333703, 0.3219752754296894559, 0.3333333333333333703, 0.3219752754296894559, 0.3333333333333333703, 0.3219752754296894559, 0.3333333333333333703, 0.3219752754296894559, 0.3333333333333333703, 0.3219752754296894559, 0.3333333333333333703, 0.3219752754296894559, 0.3333333333333333703, 0.3219752754296894559, 0.3333333333333333703, 0.3219752754296894559, 0.3333333333333333703, 0.3219752754296894559, 0.3333333333333333703, 0.3219752754296894559, 0.3333333333333333703, 0.3219752754296894559, 0.3333333333333333703, 0.3219752754296894559, 0.3333333333333333703, 0.3219752754296894559, 0.3333333333333333703, 0.3219752754296894559, 0.3333333333333333703, 0.3219752754296894559, 0.3333333333333333703, 0.3219752754296894559, 0.3333333333333333703, 0.3219752754296894559, 0.3333333333333333703, 0.3219752754296894559, 0.3333333333333333703, 0.3219752754296894559, 0.3333333333333333703, 0.3219752754296894559, 0.3333333333333333703, 0.3219752754296894559, 0.3333333333333333703, 0.3219752754296894559, 0.3333333333333333703, 0.3219752754296894559, 0.3333333333333333703, 0.3219752754296894559, 0.3333333333333333703, 0.3219752754296894559, 0.3333333333333333703, 0.3219752754296894559, 0.3333333333333333703, 0.3219752754296894559, 0.3333333333333333703, 0.3219752754296894559, 0.3333333333333333703, 0.3219752754296894559, 0.3333333333333333703, 0.3219752754296894559, 0.3333333333333333703, 0.3219752754296894559, 0.3333333333333333703, 0.3219752754296894559, 0.3333333333333333703, 0.3219752754296894559, 0.3333333333333333703, 0.3219752754296894559, 0.3333333333333333703, 0.3219752754296894559, 0.3333333333333333703, 0.3219752754296894559, 0.3333333333333333703, 0.3219752754296894559, 0.3333333333333333703, 0.3219752754296894559, 0.3333333333333333703, 0.3219752754296894559, 0.3333333333333333703, 0.3219752754296894559, 0.3333333333333333703, 0.3219752754296894559, 0.3333333333333333703, 0.3219752754296894559, 0.3333333333333333703, 0.3219752754296894559, 0.3333333333333333703, 0.3219752754296894559, 0.3333333333333333703, 0.3219752754296894559, 0.3333333333333333703, 0.3219752754296894559, 0.3333333333333333703, 0.3219752754296894559, 0.3333333333333333703, 0.3219752754296894559, 0.3333333333333333703, 0.3219752754296894559, 0.3333333333333333703, 0.3219752754296894559, 0.3333333333333333703, 0.3219752754296894559, 0.3333333333333333703, 0.3219752754296894559, 0.3333333333333333703, 0.3219752754296894559, 0.3333333333333333703, 0.3219752754296894559, 0.3333333333333333703, 0.3219752754296894559, 0.3333333333333333703, 0.3219752754296894559, 0.3333333333333333703, 0.3219752754296894559, 0.3333333333333333703, 0.3219752754296894559, 0.3333333333333333703, 0.3219752754296894559, 0.3333333333333333703, 0.3219752754296894559, 0.3333333333333333703, 0.3219752754296894559, 0.3333333333333333703, 0.3219752754296894559, 0.3333333333333333703, 0.3219752754296894559, 0.3333333333333333703, 0.3219752754296894559, 0.3333333333333333703, 0.3219752754296894559, 0.3333333333333333703, 0.3219752754296894559, 0.3333333333333333703, 0.3219752754296894559, 0.3333333333333333703, 0.3219752754296894559, 0.3333333333333333703, 0.3219752754296894559, 0.3333333333333333703, 0.3219752754296894559, 0.3333333333333333703, 0.3219752754296894559, 0.3333333333333333703, 0.3219752754296894559, 0.3333333333333333703, 0.3219752754296894559, 0.3333333333333333703, 0.3219752754296894559, 0.3333333333333333703, 0.3219752754296894559, 0.3333333333333333703, 0.3219752754296894559, 0.3333333333333333703, 0.3219752754296894559, 0.3333333333333333703, 0.3219752754296894559, 0.3333333333333333703, 0.3219752754296894559, 0.3333333333333333703, 0.3219752754296894559, 0.3333333333333333703, 0.3219752754296894559, 0.3333333333333333703, 0.3219752754296894559, 0.3333333333333333703, 0.3219752754296894559, 0.3333333333333333703, 0.3219752754296894559, 0.3333333333333333703, 0.3219752754296894559, 0.3333333333333333703, 0.3219752754296894559, 0.3333333333333333703),
 ( 0.3333333333333333703, 0.3219752754296894559, 0.3333333333333333703, 0.3219752754296894559, 0.3333333333333333703, 0.3219752754296894559, 0.3333333333333333703, 0.3219752754296894559, 0.3333333333333333703, 0.3219752754296894559, 0.3333333333333333703, 0.3219752754296894559, 0.3333333333333333703, 0.3219752754296894559, 0.3333333333333333703, 0.3219752754296894559, 0.3333333333333333703, 0.3219752754296894559, 0.3333333333333333703, 0.3219752754296894559, 0.3333333333333333703, 0.3219752754296894559, 0.3333333333333333703, 0.3219752754296894559, 0.3333333333333333703, 0.3219752754296894559, 0.3333333333333333703, 0.3219752754296894559, 0.3333333333333333703, 0.3219752754296894559, 0.3333333333333333703, 0.3219752754296894559, 0.3333333333333333703, 0.3219752754296894559, 0.3333333333333333703, 0.3219752754296894559, 0.3333333333333333703, 0.3219752754296894559, 0.3333333333333333703, 0.3219752754296894559, 0.3333333333333333703, 0.3219752754296894559, 0.3333333333333333703, 0.3219752754296894559, 0.3333333333333333703, 0.3219752754296894559, 0.3333333333333333703, 0.3219752754296894559, 0.3333333333333333703, 0.3219752754296894559, 0.3333333333333333703, 0.3219752754296894559, 0.3333333333333333703, 0.3219752754296894559, 0.3333333333333333703, 0.3219752754296894559, 0.3333333333333333703, 0.3219752754296894559, 0.3333333333333333703, 0.3219752754296894559, 0.3333333333333333703, 0.3219752754296894559, 0.3333333333333333703, 0.3219752754296894559, 0.3333333333333333703, 0.3219752754296894559, 0.3333333333333333703, 0.3219752754296894559, 0.3333333333333333703, 0.3219752754296894559, 0.3333333333333333703, 0.3219752754296894559, 0.3333333333333333703, 0.3219752754296894559, 0.3333333333333333703, 0.3219752754296894559, 0.3333333333333333703, 0.3219752754296894559, 0.3333333333333333703, 0.3219752754296894559, 0.3333333333333333703, 0.3219752754296894559, 0.3333333333333333703, 0.3219752754296894559, 0.3333333333333333703, 0.3219752754296894559, 0.3333333333333333703, 0.3219752754296894559, 0.3333333333333333703, 0.3219752754296894559, 0.3333333333333333703, 0.3219752754296894559, 0.3333333333333333703, 0.3219752754296894559, 0.3333333333333333703, 0.3219752754296894559, 0.3333333333333333703, 0.3219752754296894559, 0.3333333333333333703, 0.3219752754296894559, 0.3333333333333333703, 0.3219752754296894559, 0.3333333333333333703, 0.3219752754296894559, 0.3333333333333333703, 0.3219752754296894559, 0.3333333333333333703, 0.3219752754296894559, 0.3333333333333333703, 0.3219752754296894559, 0.3333333333333333703, 0.3219752754296894559, 0.3333333333333333703, 0.3219752754296894559, 0.3333333333333333703, 0.3219752754296894559, 0.3333333333333333703, 0.3219752754296894559, 0.3333333333333333703, 0.3219752754296894559, 0.3333333333333333703, 0.3219752754296894559, 0.3333333333333333703, 0.3219752754296894559, 0.3333333333333333703, 0.3219752754296894559, 0.3333333333333333703, 0.3219752754296894559, 0.3333333333333333703, 0.3219752754296894559, 0.3333333333333333703, 0.3219752754296894559, 0.3333333333333333703, 0.3219752754296894559, 0.3333333333333333703, 0.3219752754296894559, 0.3333333333333333703, 0.3219752754296894559, 0.3333333333333333703, 0.3219752754296894559, 0.3333333333333333703, 0.3219752754296894559, 0.3333333333333333703, 0.3219752754296894559, 0.3333333333333333703, 0.3219752754296894559, 0.3333333333333333703, 0.3219752754296894559, 0.3333333333333333703, 0.3219752754296894559, 0.3333333333333333703, 0.3219752754296894559, 0.3333333333333333703, 0.3219752754296894559, 0.3333333333333333703, 0.3219752754296894559, 0.3333333333333333703, 0.3219752754296894559, 0.3333333333333333703, 0.3219752754296894559, 0.3333333333333333703, 0.3219752754296894559, 0.3333333333333333703, 0.3219752754296894559, 0.3333333333333333703, 0.3219752754296894559, 0.3333333333333333703, 0.3219752754296894559, 0.3333333333333333703, 0.3219752754296894559, 0.3333333333333333703, 0.3219752754296894559, 0.3333333333333333703, 0.3219752754296894559, 0.3333333333333333703, 0.3219752754296894559, 0.3333333333333333703, 0.3219752754296894559, 0.3333333333333333703, 0.3219752754296894559, 0.3333333333333333703, 0.3219752754296894559, 0.3333333333333333703, 0.3219752754296894559, 0.3333333333333333703, 0.3219752754296894559, 0.3333333333333333703, 0.3219752754296894559, 0.3333333333333333703, 0.3219752754296894559, 0.3333333333333333703, 0.3219752754296894559, 0.3333333333333333703, 0.3219752754296894559, 0.3333333333333333703, 0.3219752754296894559, 0.3333333333333333703, 0.3219752754296894559, 0.3333333333333333703, 0.3219752754296894559, 0.3333333333333333703, 0.3219752754296894559, 0.3333333333333333703, 0.3219752754296894559, 0.3333333333333333703, 0.3219752754296894559, 0.3333333333333333703, 0.3219752754296894559, 0.3333333333333333703, 0.3219752754296894559, 0.3333333333333333703, 0.3219752754296894559, 0.3333333333333333703, 0.3219752754296894559, 0.3333333333333333703, 0.3219752754296894559, 0.3333333333333333703, 0.3219752754296894559, 0.3333333333333333703, 0.3219752754296894559, 0.3333333333333333703, 0.3219752754296894559, 0.3333333333333333703, 0.3219752754296894559, 0.3333333333333333703, 0.3219752754296894559, 0.3333333333333333703, 0.3219752754296894559, 0.3333333333333333703, 0.3219752754296894559, 0.3333333333333333703, 0.3219752754296894559, 0.3333333333333333703, 0.3219752754296894559, 0.3333333333333333703, 0.3219752754296894559, 0.3333333333333333703, 0.3219752754296894559, 0.3333333333333333703, 0.3219752754296894559, 0.3333333333333333703, 0.3219752754296894559, 0.3333333333333333703, 0.3219752754296894559, 0.3333333333333333703, 0.3219752754296894559, 0.3333333333333333703, 0.3219752754296894559, 0.3333333333333333703, 0.3219752754296894559, 0.3333333333333333703, 0.3219752754296894559, 0.3333333333333333703, 0.3219752754296894559, 0.3333333333333333703, 0.3219752754296894559, 0.3333333333333333703, 0.3219752754296894559, 0.3333333333333333703, 0.3219752754296894559, 0.3333333333333333703, 0.3219752754296894559, 0.3333333333333333703, 0.3219752754296894559, 0.3333333333333333703, 0.3219752754296894559, 0.3333333333333333703, 0.3219752754296894559, 0.3333333333333333703, 0.3219752754296894559, 0.3333333333333333703, 0.3219752754296894559, 0.3333333333333333703, 0.3219752754296894559, 0.3333333333333333703, 0.3219752754296894559, 0.3333333333333333703, 0.3219752754296894559, 0.3333333333333333703, 0.3219752754296894559, 0.3333333333333333703, 0.3219752754296894559, 0.3333333333333333703, 0.3219752754296894559, 0.3333333333333333703, 0.3219752754296894559, 0.3333333333333333703, 0.3219752754296894559, 0.3333333333333333703, 0.3219752754296894559, 0.3333333333333333703, 0.3219752754296894559, 0.3333333333333333703, 0.3219752754296894559, 0.3333333333333333703, 0.3219752754296894559, 0.3333333333333333703, 0.3219752754296894559, 0.3333333333333333703, 0.3219752754296894559, 0.3333333333333333703, 0.3219752754296894559, 0.3333333333333333703, 0.3219752754296894559, 0.3333333333333333703, 0.3219752754296894559, 0.3333333333333333703, 0.3219752754296894559, 0.3333333333333333703, 0.3219752754296894559, 0.3333333333333333703, 0.3219752754296894559, 0.3333333333333333703, 0.3219752754296894559, 0.3333333333333333703, 0.3219752754296894559, 0.3333333333333333703, 0.3219752754296894559, 0.3333333333333333703, 0.3219752754296894559, 0.3333333333333333703, 0.3219752754296894559, 0.3333333333333333703, 0.3219752754296894559, 0.3333333333333333703, 0.3219752754296894559, 0.3333333333333333703, 0.3219752754296894559, 0.3333333333333333703, 0.3219752754296894559, 0.3333333333333333703, 0.3219752754296894559, 0.3333333333333333703, 0.3219752754296894559, 0.3333333333333333703, 0.3219752754296894559, 0.3333333333333333703, 0.3219752754296894559, 0.3333333333333333703, 0.3219752754296894559, 0.3333333333333333703, 0.3219752754296894559, 0.3333333333333333703, 0.3219752754296894559, 0.3333333333333333703, 0.3219752754296894559, 0.3333333333333333703, 0.3219752754296894559, 0.3333333333333333703, 0.3219752754296894559, 0.3333333333333333703, 0.3219752754296894559, 0.3333333333333333703, 0.3219752754296894559, 0.3333333333333333703, 0.3219752754296894559, 0.3333333333333333703, 0.3219752754296894559, 0.3333333333333333703, 0.3219752754296894559, 0.3333333333333333703, 0.3219752754296894559, 0.3333333333333333703, 0.3219752754296894559, 0.3333333333333333703, 0.3219752754296894559, 0.3333333333333333703, 0.3219752754296894559, 0.3333333333333333703, 0.3219752754296894559, 0.3333333333333333703, 0.3219752754296894559, 0.3333333333333333703, 0.3219752754296894559, 0.3333333333333333703, 0.3219752754296894559, 0.3333333333333333703, 0.3219752754296894559, 0.3333333333333333703, 0.3219752754296894559, 0.3333333333333333703, 0.3219752754296894559, 0.3333333333333333703, 0.3219752754296894559, 0.3333333333333333703, 0.3219752754296894559, 0.3333333333333333703, 0.3219752754296894559, 0.3333333333333333703, 0.3219752754296894559, 0.3333333333333333703, 0.3219752754296894559, 0.3333333333333333703, 0.3219752754296894559, 0.3333333333333333703, 0.3219752754296894559, 0.3333333333333333703, 0.3219752754296894559, 0.3333333333333333703, 0.3219752754296894559, 0.3333333333333333703, 0.3219752754296894559, 0.3333333333333333703, 0.3219752754296894559, 0.3333333333333333703, 0.3219752754296894559, 0.3333333333333333703, 0.3219752754296894559, 0.3333333333333333703, 0.3219752754296894559, 0.3333333333333333703, 0.3219752754296894559, 0.3333333333333333703, 0.3219752754296894559, 0.3333333333333333703, 0.3219752754296894559, 0.3333333333333333703, 0.3219752754296894559, 0.3333333333333333703, 0.3219752754296894559, 0.3333333333333333703, 0.3219752754296894559, 0.3333333333333333703, 0.3219752754296894559, 0.3333333333333333703, 0.3219752754296894559, 0.3333333333333333703, 0.3219752754296894559, 0.3333333333333333703, 0.3219752754296894559, 0.3333333333333333703, 0.3219752754296894559, 0.3333333333333333703, 0.3219752754296894559, 0.3333333333333333703, 0.3219752754296894559, 0.3333333333333333703, 0.3219752754296894559, 0.3333333333333333703, 0.3219752754296894559, 0.3333333333333333703, 0.3219752754296894559, 0.3333333333333333703, 0.3219752754296894559, 0.3333333333333333703, 0.3219752754296894559, 0.3333333333333333703, 0.3219752754296894559, 0.3333333333333333703, 0.3219752754296894559, 0.3333333333333333703, 0.3219752754296894559, 0.3333333333333333703, 0.3219752754296894559, 0.3333333333333333703, 0.3219752754296894559, 0.3333333333333333703),
 ( 1.000000000000000000, 0.9659258262890683122, 1.000000000000000000, 0.9659258262890683122, 1.000000000000000000, 0.9659258262890683122, 1.000000000000000000, 0.9659258262890683122, 1.000000000000000000, 0.9659258262890683122, 1.000000000000000000, 0.9659258262890683122, 1.000000000000000000, 0.9659258262890683122, 1.000000000000000000, 0.9659258262890683122, 1.000000000000000000, 0.9659258262890683122, 1.000000000000000000, 0.9659258262890683122, 1.000000000000000000, 0.9659258262890683122, 1.000000000000000000, 0.9659258262890683122, 1.000000000000000000, 0.9659258262890683122, 1.000000000000000000, 0.9659258262890683122, 1.000000000000000000, 0.9659258262890683122, 1.000000000000000000, 0.9659258262890683122, 1.000000000000000000, 0.9659258262890683122, 1.000000000000000000, 0.9659258262890683122, 1.000000000000000000, 0.9659258262890683122, 1.000000000000000000, 0.9659258262890683122, 1.000000000000000000, 0.9659258262890683122, 1.000000000000000000, 0.9659258262890683122, 1.000000000000000000, 0.9659258262890683122, 1.000000000000000000, 0.9659258262890683122, 1.000000000000000000, 0.9659258262890683122, 1.000000000000000000, 0.9659258262890683122, 1.000000000000000000, 0.9659258262890683122, 1.000000000000000000, 0.9659258262890683122, 1.000000000000000000, 0.9659258262890683122, 1.000000000000000000, 0.9659258262890683122, 1.000000000000000000, 0.9659258262890683122, 1.000000000000000000, 0.9659258262890683122, 1.000000000000000000, 0.9659258262890683122, 1.000000000000000000, 0.9659258262890683122, 1.000000000000000000, 0.9659258262890683122, 1.000000000000000000, 0.9659258262890683122, 1.000000000000000000, 0.9659258262890683122, 1.000000000000000000, 0.9659258262890683122, 1.000000000000000000, 0.9659258262890683122, 1.000000000000000000, 0.9659258262890683122, 1.000000000000000000, 0.9659258262890683122, 1.000000000000000000, 0.9659258262890683122, 1.000000000000000000, 0.9659258262890683122, 1.000000000000000000, 0.9659258262890683122, 1.000000000000000000, 0.9659258262890683122, 1.000000000000000000, 0.9659258262890683122, 1.000000000000000000, 0.9659258262890683122, 1.000000000000000000, 0.9659258262890683122, 1.000000000000000000, 0.9659258262890683122, 1.000000000000000000, 0.9659258262890683122, 1.000000000000000000, 0.9659258262890683122, 1.000000000000000000, 0.9659258262890683122, 1.000000000000000000, 0.9659258262890683122, 1.000000000000000000, 0.9659258262890683122, 1.000000000000000000, 0.9659258262890683122, 1.000000000000000000, 0.9659258262890683122, 1.000000000000000000, 0.9659258262890683122, 1.000000000000000000, 0.9659258262890683122, 1.000000000000000000, 0.9659258262890683122, 1.000000000000000000, 0.9659258262890683122, 1.000000000000000000, 0.9659258262890683122, 1.000000000000000000, 0.9659258262890683122, 1.000000000000000000, 0.9659258262890683122, 1.000000000000000000, 0.9659258262890683122, 1.000000000000000000, 0.9659258262890683122, 1.000000000000000000, 0.9659258262890683122, 1.000000000000000000, 0.9659258262890683122, 1.000000000000000000, 0.9659258262890683122, 1.000000000000000000, 0.9659258262890683122, 1.000000000000000000, 0.9659258262890683122, 1.000000000000000000, 0.9659258262890683122, 1.000000000000000000, 0.9659258262890683122, 1.000000000000000000, 0.9659258262890683122, 1.000000000000000000, 0.9659258262890683122, 1.000000000000000000, 0.9659258262890683122, 1.000000000000000000, 0.9659258262890683122, 1.000000000000000000, 0.9659258262890683122, 1.000000000000000000, 0.9659258262890683122, 1.000000000000000000, 0.9659258262890683122, 1.000000000000000000, 0.9659258262890683122, 1.000000000000000000, 0.9659258262890683122, 1.000000000000000000, 0.9659258262890683122, 1.000000000000000000, 0.9659258262890683122, 1.000000000000000000, 0.9659258262890683122, 1.000000000000000000, 0.9659258262890683122, 1.000000000000000000, 0.9659258262890683122, 1.000000000000000000, 0.9659258262890683122, 1.000000000000000000, 0.9659258262890683122, 1.000000000000000000, 0.9659258262890683122, 1.000000000000000000, 0.9659258262890683122, 1.000000000000000000, 0.9659258262890683122, 1.000000000000000000, 0.9659258262890683122, 1.000000000000000000, 0.9659258262890683122, 1.000000000000000000, 0.9659258262890683122, 1.000000000000000000, 0.9659258262890683122, 1.000000000000000000, 0.9659258262890683122, 1.000000000000000000, 0.9659258262890683122, 1.000000000000000000, 0.9659258262890683122, 1.000000000000000000, 0.9659258262890683122, 1.000000000000000000, 0.9659258262890683122, 1.000000000000000000, 0.9659258262890683122, 1.000000000000000000, 0.9659258262890683122, 1.000000000000000000, 0.9659258262890683122, 1.000000000000000000, 0.9659258262890683122, 1.000000000000000000, 0.9659258262890683122, 1.000000000000000000, 0.9659258262890683122, 1.000000000000000000, 0.9659258262890683122, 1.000000000000000000, 0.9659258262890683122, 1.000000000000000000, 0.9659258262890683122, 1.000000000000000000, 0.9659258262890683122, 1.000000000000000000, 0.9659258262890683122, 1.000000000000000000, 0.9659258262890683122, 1.000000000000000000, 0.9659258262890683122, 1.000000000000000000, 0.9659258262890683122, 1.000000000000000000, 0.9659258262890683122, 1.000000000000000000, 0.9659258262890683122, 1.000000000000000000, 0.9659258262890683122, 1.000000000000000000, 0.9659258262890683122, 1.000000000000000000, 0.9659258262890683122, 1.000000000000000000, 0.9659258262890683122, 1.000000000000000000, 0.9659258262890683122, 1.000000000000000000, 0.9659258262890683122, 1.000000000000000000, 0.9659258262890683122, 1.000000000000000000, 0.9659258262890683122, 1.000000000000000000, 0.9659258262890683122, 1.000000000000000000, 0.9659258262890683122, 1.000000000000000000, 0.9659258262890683122, 1.000000000000000000, 0.9659258262890683122, 1.000000000000000000, 0.9659258262890683122, 1.000000000000000000, 0.9659258262890683122, 1.000000000000000000, 0.9659258262890683122, 1.000000000000000000, 0.9659258262890683122, 1.000000000000000000, 0.9659258262890683122, 1.000000000000000000, 0.9659258262890683122, 1.000000000000000000, 0.9659258262890683122, 1.000000000000000000, 0.9659258262890683122, 1.000000000000000000, 0.9659258262890683122, 1.000000000000000000, 0.9659258262890683122, 1.000000000000000000, 0.9659258262890683122, 1.000000000000000000, 0.9659258262890683122, 1.000000000000000000, 0.9659258262890683122, 1.000000000000000000, 0.9659258262890683122, 1.000000000000000000, 0.9659258262890683122, 1.000000000000000000, 0.9659258262890683122, 1.000000000000000000, 0.9659258262890683122, 1.000000000000000000, 0.9659258262890683122, 1.000000000000000000, 0.9659258262890683122, 1.000000000000000000, 0.9659258262890683122, 1.000000000000000000, 0.9659258262890683122, 1.000000000000000000, 0.9659258262890683122, 1.000000000000000000, 0.9659258262890683122, 1.000000000000000000, 0.9659258262890683122, 1.000000000000000000, 0.9659258262890683122, 1.000000000000000000, 0.9659258262890683122, 1.000000000000000000, 0.9659258262890683122, 1.000000000000000000, 0.9659258262890683122, 1.000000000000000000, 0.9659258262890683122, 1.000000000000000000, 0.9659258262890683122, 1.000000000000000000, 0.9659258262890683122, 1.000000000000000000, 0.9659258262890683122, 1.000000000000000000, 0.9659258262890683122, 1.000000000000000000, 0.9659258262890683122, 1.000000000000000000, 0.9659258262890683122, 1.000000000000000000, 0.9659258262890683122, 1.000000000000000000, 0.9659258262890683122, 1.000000000000000000, 0.9659258262890683122, 1.000000000000000000, 0.9659258262890683122, 1.000000000000000000, 0.9659258262890683122, 1.000000000000000000, 0.9659258262890683122, 1.000000000000000000, 0.9659258262890683122, 1.000000000000000000, 0.9659258262890683122, 1.000000000000000000, 0.9659258262890683122, 1.000000000000000000, 0.9659258262890683122, 1.000000000000000000, 0.9659258262890683122, 1.000000000000000000, 0.9659258262890683122, 1.000000000000000000, 0.9659258262890683122, 1.000000000000000000, 0.9659258262890683122, 1.000000000000000000, 0.9659258262890683122, 1.000000000000000000, 0.9659258262890683122, 1.000000000000000000, 0.9659258262890683122, 1.000000000000000000, 0.9659258262890683122, 1.000000000000000000, 0.9659258262890683122, 1.000000000000000000, 0.9659258262890683122, 1.000000000000000000, 0.9659258262890683122, 1.000000000000000000, 0.9659258262890683122, 1.000000000000000000, 0.9659258262890683122, 1.000000000000000000, 0.9659258262890683122, 1.000000000000000000, 0.9659258262890683122, 1.000000000000000000, 0.9659258262890683122, 1.000000000000000000, 0.9659258262890683122, 1.000000000000000000, 0.9659258262890683122, 1.000000000000000000, 0.9659258262890683122, 1.000000000000000000, 0.9659258262890683122, 1.000000000000000000, 0.9659258262890683122, 1.000000000000000000, 0.9659258262890683122, 1.000000000000000000, 0.9659258262890683122, 1.000000000000000000, 0.9659258262890683122, 1.000000000000000000, 0.9659258262890683122, 1.000000000000000000, 0.9659258262890683122, 1.000000000000000000, 0.9659258262890683122, 1.000000000000000000, 0.9659258262890683122, 1.000000000000000000, 0.9659258262890683122, 1.000000000000000000, 0.9659258262890683122, 1.000000000000000000, 0.9659258262890683122, 1.000000000000000000, 0.9659258262890683122, 1.000000000000000000, 0.9659258262890683122, 1.000000000000000000, 0.9659258262890683122, 1.000000000000000000, 0.9659258262890683122, 1.000000000000000000, 0.9659258262890683122, 1.000000000000000000, 0.9659258262890683122, 1.000000000000000000, 0.9659258262890683122, 1.000000000000000000, 0.9659258262890683122, 1.000000000000000000, 0.9659258262890683122, 1.000000000000000000, 0.9659258262890683122, 1.000000000000000000, 0.9659258262890683122, 1.000000000000000000, 0.9659258262890683122, 1.000000000000000000, 0.9659258262890683122, 1.000000000000000000, 0.9659258262890683122, 1.000000000000000000, 0.9659258262890683122, 1.000000000000000000, 0.9659258262890683122, 1.000000000000000000, 0.9659258262890683122, 1.000000000000000000, 0.9659258262890683122, 1.000000000000000000, 0.9659258262890683122, 1.000000000000000000, 0.9659258262890683122, 1.000000000000000000, 0.9659258262890683122, 1.000000000000000000, 0.9659258262890683122, 1.000000000000000000, 0.9659258262890683122, 1.000000000000000000, 0.9659258262890683122, 1.000000000000000000),
 ( 0.3333333333333333703, 0.3219752754296894559, 0.3333333333333333703, 0.3219752754296894559, 0.3333333333333333703, 0.3219752754296894559, 0.3333333333333333703, 0.3219752754296894559, 0.3333333333333333703, 0.3219752754296894559, 0.3333333333333333703, 0.3219752754296894559, 0.3333333333333333703, 0.3219752754296894559, 0.3333333333333333703, 0.3219752754296894559, 0.3333333333333333703, 0.3219752754296894559, 0.3333333333333333703, 0.3219752754296894559, 0.3333333333333333703, 0.3219752754296894559, 0.3333333333333333703, 0.3219752754296894559, 0.3333333333333333703, 0.3219752754296894559, 0.3333333333333333703, 0.3219752754296894559, 0.3333333333333333703, 0.3219752754296894559, 0.3333333333333333703, 0.3219752754296894559, 0.3333333333333333703, 0.3219752754296894559, 0.3333333333333333703, 0.3219752754296894559, 0.3333333333333333703, 0.3219752754296894559, 0.3333333333333333703, 0.3219752754296894559, 0.3333333333333333703, 0.3219752754296894559, 0.3333333333333333703, 0.3219752754296894559, 0.3333333333333333703, 0.3219752754296894559, 0.3333333333333333703, 0.3219752754296894559, 0.3333333333333333703, 0.3219752754296894559, 0.3333333333333333703, 0.3219752754296894559, 0.3333333333333333703, 0.3219752754296894559, 0.3333333333333333703, 0.3219752754296894559, 0.3333333333333333703, 0.3219752754296894559, 0.3333333333333333703, 0.3219752754296894559, 0.3333333333333333703, 0.3219752754296894559, 0.3333333333333333703, 0.3219752754296894559, 0.3333333333333333703, 0.3219752754296894559, 0.3333333333333333703, 0.3219752754296894559, 0.3333333333333333703, 0.3219752754296894559, 0.3333333333333333703, 0.3219752754296894559, 0.3333333333333333703, 0.3219752754296894559, 0.3333333333333333703, 0.3219752754296894559, 0.3333333333333333703, 0.3219752754296894559, 0.3333333333333333703, 0.3219752754296894559, 0.3333333333333333703, 0.3219752754296894559, 0.3333333333333333703, 0.3219752754296894559, 0.3333333333333333703, 0.3219752754296894559, 0.3333333333333333703, 0.3219752754296894559, 0.3333333333333333703, 0.3219752754296894559, 0.3333333333333333703, 0.3219752754296894559, 0.3333333333333333703, 0.3219752754296894559, 0.3333333333333333703, 0.3219752754296894559, 0.3333333333333333703, 0.3219752754296894559, 0.3333333333333333703, 0.3219752754296894559, 0.3333333333333333703, 0.3219752754296894559, 0.3333333333333333703, 0.3219752754296894559, 0.3333333333333333703, 0.3219752754296894559, 0.3333333333333333703, 0.3219752754296894559, 0.3333333333333333703, 0.3219752754296894559, 0.3333333333333333703, 0.3219752754296894559, 0.3333333333333333703, 0.3219752754296894559, 0.3333333333333333703, 0.3219752754296894559, 0.3333333333333333703, 0.3219752754296894559, 0.3333333333333333703, 0.3219752754296894559, 0.3333333333333333703, 0.3219752754296894559, 0.3333333333333333703, 0.3219752754296894559, 0.3333333333333333703, 0.3219752754296894559, 0.3333333333333333703, 0.3219752754296894559, 0.3333333333333333703, 0.3219752754296894559, 0.3333333333333333703, 0.3219752754296894559, 0.3333333333333333703, 0.3219752754296894559, 0.3333333333333333703, 0.3219752754296894559, 0.3333333333333333703, 0.3219752754296894559, 0.3333333333333333703, 0.3219752754296894559, 0.3333333333333333703, 0.3219752754296894559, 0.3333333333333333703, 0.3219752754296894559, 0.3333333333333333703, 0.3219752754296894559, 0.3333333333333333703, 0.3219752754296894559, 0.3333333333333333703, 0.3219752754296894559, 0.3333333333333333703, 0.3219752754296894559, 0.3333333333333333703, 0.3219752754296894559, 0.3333333333333333703, 0.3219752754296894559, 0.3333333333333333703, 0.3219752754296894559, 0.3333333333333333703, 0.3219752754296894559, 0.3333333333333333703, 0.3219752754296894559, 0.3333333333333333703, 0.3219752754296894559, 0.3333333333333333703, 0.3219752754296894559, 0.3333333333333333703, 0.3219752754296894559, 0.3333333333333333703, 0.3219752754296894559, 0.3333333333333333703, 0.3219752754296894559, 0.3333333333333333703, 0.3219752754296894559, 0.3333333333333333703, 0.3219752754296894559, 0.3333333333333333703, 0.3219752754296894559, 0.3333333333333333703, 0.3219752754296894559, 0.3333333333333333703, 0.3219752754296894559, 0.3333333333333333703, 0.3219752754296894559, 0.3333333333333333703, 0.3219752754296894559, 0.3333333333333333703, 0.3219752754296894559, 0.3333333333333333703, 0.3219752754296894559, 0.3333333333333333703, 0.3219752754296894559, 0.3333333333333333703, 0.3219752754296894559, 0.3333333333333333703, 0.3219752754296894559, 0.3333333333333333703, 0.3219752754296894559, 0.3333333333333333703, 0.3219752754296894559, 0.3333333333333333703, 0.3219752754296894559, 0.3333333333333333703, 0.3219752754296894559, 0.3333333333333333703, 0.3219752754296894559, 0.3333333333333333703, 0.3219752754296894559, 0.3333333333333333703, 0.3219752754296894559, 0.3333333333333333703, 0.3219752754296894559, 0.3333333333333333703, 0.3219752754296894559, 0.3333333333333333703, 0.3219752754296894559, 0.3333333333333333703, 0.3219752754296894559, 0.3333333333333333703, 0.3219752754296894559, 0.3333333333333333703, 0.3219752754296894559, 0.3333333333333333703, 0.3219752754296894559, 0.3333333333333333703, 0.3219752754296894559, 0.3333333333333333703, 0.3219752754296894559, 0.3333333333333333703, 0.3219752754296894559, 0.3333333333333333703, 0.3219752754296894559, 0.3333333333333333703, 0.3219752754296894559, 0.3333333333333333703, 0.3219752754296894559, 0.3333333333333333703, 0.3219752754296894559, 0.3333333333333333703, 0.3219752754296894559, 0.3333333333333333703, 0.3219752754296894559, 0.3333333333333333703, 0.3219752754296894559, 0.3333333333333333703, 0.3219752754296894559, 0.3333333333333333703, 0.3219752754296894559, 0.3333333333333333703, 0.3219752754296894559, 0.3333333333333333703, 0.3219752754296894559, 0.3333333333333333703, 0.3219752754296894559, 0.3333333333333333703, 0.3219752754296894559, 0.3333333333333333703, 0.3219752754296894559, 0.3333333333333333703, 0.3219752754296894559, 0.3333333333333333703, 0.3219752754296894559, 0.3333333333333333703, 0.3219752754296894559, 0.3333333333333333703, 0.3219752754296894559, 0.3333333333333333703, 0.3219752754296894559, 0.3333333333333333703, 0.3219752754296894559, 0.3333333333333333703, 0.3219752754296894559, 0.3333333333333333703, 0.3219752754296894559, 0.3333333333333333703, 0.3219752754296894559, 0.3333333333333333703, 0.3219752754296894559, 0.3333333333333333703, 0.3219752754296894559, 0.3333333333333333703, 0.3219752754296894559, 0.3333333333333333703, 0.3219752754296894559, 0.3333333333333333703, 0.3219752754296894559, 0.3333333333333333703, 0.3219752754296894559, 0.3333333333333333703, 0.3219752754296894559, 0.3333333333333333703, 0.3219752754296894559, 0.3333333333333333703, 0.3219752754296894559, 0.3333333333333333703, 0.3219752754296894559, 0.3333333333333333703, 0.3219752754296894559, 0.3333333333333333703, 0.3219752754296894559, 0.3333333333333333703, 0.3219752754296894559, 0.3333333333333333703, 0.3219752754296894559, 0.3333333333333333703, 0.3219752754296894559, 0.3333333333333333703, 0.3219752754296894559, 0.3333333333333333703, 0.3219752754296894559, 0.3333333333333333703, 0.3219752754296894559, 0.3333333333333333703, 0.3219752754296894559, 0.3333333333333333703, 0.3219752754296894559, 0.3333333333333333703, 0.3219752754296894559, 0.3333333333333333703, 0.3219752754296894559, 0.3333333333333333703, 0.3219752754296894559, 0.3333333333333333703, 0.3219752754296894559, 0.3333333333333333703, 0.3219752754296894559, 0.3333333333333333703, 0.3219752754296894559, 0.3333333333333333703, 0.3219752754296894559, 0.3333333333333333703, 0.3219752754296894559, 0.3333333333333333703, 0.3219752754296894559, 0.3333333333333333703, 0.3219752754296894559, 0.3333333333333333703, 0.3219752754296894559, 0.3333333333333333703, 0.3219752754296894559, 0.3333333333333333703, 0.3219752754296894559, 0.3333333333333333703, 0.3219752754296894559, 0.3333333333333333703, 0.3219752754296894559, 0.3333333333333333703, 0.3219752754296894559, 0.3333333333333333703, 0.3219752754296894559, 0.3333333333333333703, 0.3219752754296894559, 0.3333333333333333703, 0.3219752754296894559, 0.3333333333333333703, 0.3219752754296894559, 0.3333333333333333703, 0.3219752754296894559, 0.3333333333333333703, 0.3219752754296894559, 0.3333333333333333703, 0.3219752754296894559, 0.3333333333333333703, 0.3219752754296894559, 0.3333333333333333703, 0.3219752754296894559, 0.3333333333333333703, 0.3219752754296894559, 0.3333333333333333703, 0.3219752754296894559, 0.3333333333333333703, 0.3219752754296894559, 0.3333333333333333703, 0.3219752754296894559, 0.3333333333333333703, 0.3219752754296894559, 0.3333333333333333703, 0.3219752754296894559, 0.3333333333333333703, 0.3219752754296894559, 0.3333333333333333703, 0.3219752754296894559, 0.3333333333333333703, 0.3219752754296894559, 0.3333333333333333703, 0.3219752754296894559, 0.3333333333333333703, 0.3219752754296894559, 0.3333333333333333703, 0.3219752754296894559, 0.3333333333333333703, 0.3219752754296894559, 0.3333333333333333703, 0.3219752754296894559, 0.3333333333333333703, 0.3219752754296894559, 0.3333333333333333703, 0.3219752754296894559, 0.3333333333333333703, 0.3219752754296894559, 0.3333333333333333703, 0.3219752754296894559, 0.3333333333333333703, 0.3219752754296894559, 0.3333333333333333703, 0.3219752754296894559, 0.3333333333333333703, 0.3219752754296894559, 0.3333333333333333703, 0.3219752754296894559, 0.3333333333333333703, 0.3219752754296894559, 0.3333333333333333703, 0.3219752754296894559, 0.3333333333333333703, 0.3219752754296894559, 0.3333333333333333703, 0.3219752754296894559, 0.3333333333333333703, 0.3219752754296894559, 0.3333333333333333703, 0.3219752754296894559, 0.3333333333333333703, 0.3219752754296894559, 0.3333333333333333703, 0.3219752754296894559, 0.3333333333333333703, 0.3219752754296894559, 0.3333333333333333703, 0.3219752754296894559, 0.3333333333333333703, 0.3219752754296894559, 0.3333333333333333703, 0.3219752754296894559, 0.3333333333333333703, 0.3219752754296894559, 0.3333333333333333703, 0.3219752754296894559, 0.3333333333333333703, 0.3219752754296894559, 0.3333333333333333703, 0.3219752754296894559, 0.3333333333333333703, 0.3219752754296894559, 0.3333333333333333703, 0.3219752754296894559, 0.3333333333333333703, 0.3219752754296894559, 0.3333333333333333703, 0.3219752754296894559, 0.3333333333333333703, 0.3219752754296894559, 0.3333333333333333703, 0.3219752754296894559, 0.3333333333333333703, 0.3219752754296894559, 0.3333333333333333703),
 ( 0.3333333333333333703, 0.3219752754296894559, 0.3333333333333333703, 0.3219752754296894559, 0.3333333333333333703, 0.3219752754296894559, 0.3333333333333333703, 0.3219752754296894559, 0.3333333333333333703, 0.3219752754296894559, 0.3333333333333333703, 0.3219752754296894559, 0.3333333333333333703, 0.3219752754296894559, 0.3333333333333333703, 0.3219752754296894559, 0.3333333333333333703, 0.3219752754296894559, 0.3333333333333333703, 0.3219752754296894559, 0.3333333333333333703, 0.3219752754296894559, 0.3333333333333333703, 0.3219752754296894559, 0.3333333333333333703, 0.3219752754296894559, 0.3333333333333333703, 0.3219752754296894559, 0.3333333333333333703, 0.3219752754296894559, 0.3333333333333333703, 0.3219752754296894559, 0.3333333333333333703, 0.3219752754296894559, 0.3333333333333333703, 0.3219752754296894559, 0.3333333333333333703, 0.3219752754296894559, 0.3333333333333333703, 0.3219752754296894559, 0.3333333333333333703, 0.3219752754296894559, 0.3333333333333333703, 0.3219752754296894559, 0.3333333333333333703, 0.3219752754296894559, 0.3333333333333333703, 0.3219752754296894559, 0.3333333333333333703, 0.3219752754296894559, 0.3333333333333333703, 0.3219752754296894559, 0.3333333333333333703, 0.3219752754296894559, 0.3333333333333333703, 0.3219752754296894559, 0.3333333333333333703, 0.3219752754296894559, 0.3333333333333333703, 0.3219752754296894559, 0.3333333333333333703, 0.3219752754296894559, 0.3333333333333333703, 0.3219752754296894559, 0.3333333333333333703, 0.3219752754296894559, 0.3333333333333333703, 0.3219752754296894559, 0.3333333333333333703, 0.3219752754296894559, 0.3333333333333333703, 0.3219752754296894559, 0.3333333333333333703, 0.3219752754296894559, 0.3333333333333333703, 0.3219752754296894559, 0.3333333333333333703, 0.3219752754296894559, 0.3333333333333333703, 0.3219752754296894559, 0.3333333333333333703, 0.3219752754296894559, 0.3333333333333333703, 0.3219752754296894559, 0.3333333333333333703, 0.3219752754296894559, 0.3333333333333333703, 0.3219752754296894559, 0.3333333333333333703, 0.3219752754296894559, 0.3333333333333333703, 0.3219752754296894559, 0.3333333333333333703, 0.3219752754296894559, 0.3333333333333333703, 0.3219752754296894559, 0.3333333333333333703, 0.3219752754296894559, 0.3333333333333333703, 0.3219752754296894559, 0.3333333333333333703, 0.3219752754296894559, 0.3333333333333333703, 0.3219752754296894559, 0.3333333333333333703, 0.3219752754296894559, 0.3333333333333333703, 0.3219752754296894559, 0.3333333333333333703, 0.3219752754296894559, 0.3333333333333333703, 0.3219752754296894559, 0.3333333333333333703, 0.3219752754296894559, 0.3333333333333333703, 0.3219752754296894559, 0.3333333333333333703, 0.3219752754296894559, 0.3333333333333333703, 0.3219752754296894559, 0.3333333333333333703, 0.3219752754296894559, 0.3333333333333333703, 0.3219752754296894559, 0.3333333333333333703, 0.3219752754296894559, 0.3333333333333333703, 0.3219752754296894559, 0.3333333333333333703, 0.3219752754296894559, 0.3333333333333333703, 0.3219752754296894559, 0.3333333333333333703, 0.3219752754296894559, 0.3333333333333333703, 0.3219752754296894559, 0.3333333333333333703, 0.3219752754296894559, 0.3333333333333333703, 0.3219752754296894559, 0.3333333333333333703, 0.3219752754296894559, 0.3333333333333333703, 0.3219752754296894559, 0.3333333333333333703, 0.3219752754296894559, 0.3333333333333333703, 0.3219752754296894559, 0.3333333333333333703, 0.3219752754296894559, 0.3333333333333333703, 0.3219752754296894559, 0.3333333333333333703, 0.3219752754296894559, 0.3333333333333333703, 0.3219752754296894559, 0.3333333333333333703, 0.3219752754296894559, 0.3333333333333333703, 0.3219752754296894559, 0.3333333333333333703, 0.3219752754296894559, 0.3333333333333333703, 0.3219752754296894559, 0.3333333333333333703, 0.3219752754296894559, 0.3333333333333333703, 0.3219752754296894559, 0.3333333333333333703, 0.3219752754296894559, 0.3333333333333333703, 0.3219752754296894559, 0.3333333333333333703, 0.3219752754296894559, 0.3333333333333333703, 0.3219752754296894559, 0.3333333333333333703, 0.3219752754296894559, 0.3333333333333333703, 0.3219752754296894559, 0.3333333333333333703, 0.3219752754296894559, 0.3333333333333333703, 0.3219752754296894559, 0.3333333333333333703, 0.3219752754296894559, 0.3333333333333333703, 0.3219752754296894559, 0.3333333333333333703, 0.3219752754296894559, 0.3333333333333333703, 0.3219752754296894559, 0.3333333333333333703, 0.3219752754296894559, 0.3333333333333333703, 0.3219752754296894559, 0.3333333333333333703, 0.3219752754296894559, 0.3333333333333333703, 0.3219752754296894559, 0.3333333333333333703, 0.3219752754296894559, 0.3333333333333333703, 0.3219752754296894559, 0.3333333333333333703, 0.3219752754296894559, 0.3333333333333333703, 0.3219752754296894559, 0.3333333333333333703, 0.3219752754296894559, 0.3333333333333333703, 0.3219752754296894559, 0.3333333333333333703, 0.3219752754296894559, 0.3333333333333333703, 0.3219752754296894559, 0.3333333333333333703, 0.3219752754296894559, 0.3333333333333333703, 0.3219752754296894559, 0.3333333333333333703, 0.3219752754296894559, 0.3333333333333333703, 0.3219752754296894559, 0.3333333333333333703, 0.3219752754296894559, 0.3333333333333333703, 0.3219752754296894559, 0.3333333333333333703, 0.3219752754296894559, 0.3333333333333333703, 0.3219752754296894559, 0.3333333333333333703, 0.3219752754296894559, 0.3333333333333333703, 0.3219752754296894559, 0.3333333333333333703, 0.3219752754296894559, 0.3333333333333333703, 0.3219752754296894559, 0.3333333333333333703, 0.3219752754296894559, 0.3333333333333333703, 0.3219752754296894559, 0.3333333333333333703, 0.3219752754296894559, 0.3333333333333333703, 0.3219752754296894559, 0.3333333333333333703, 0.3219752754296894559, 0.3333333333333333703, 0.3219752754296894559, 0.3333333333333333703, 0.3219752754296894559, 0.3333333333333333703, 0.3219752754296894559, 0.3333333333333333703, 0.3219752754296894559, 0.3333333333333333703, 0.3219752754296894559, 0.3333333333333333703, 0.3219752754296894559, 0.3333333333333333703, 0.3219752754296894559, 0.3333333333333333703, 0.3219752754296894559, 0.3333333333333333703, 0.3219752754296894559, 0.3333333333333333703, 0.3219752754296894559, 0.3333333333333333703, 0.3219752754296894559, 0.3333333333333333703, 0.3219752754296894559, 0.3333333333333333703, 0.3219752754296894559, 0.3333333333333333703, 0.3219752754296894559, 0.3333333333333333703, 0.3219752754296894559, 0.3333333333333333703, 0.3219752754296894559, 0.3333333333333333703, 0.3219752754296894559, 0.3333333333333333703, 0.3219752754296894559, 0.3333333333333333703, 0.3219752754296894559, 0.3333333333333333703, 0.3219752754296894559, 0.3333333333333333703, 0.3219752754296894559, 0.3333333333333333703, 0.3219752754296894559, 0.3333333333333333703, 0.3219752754296894559, 0.3333333333333333703, 0.3219752754296894559, 0.3333333333333333703, 0.3219752754296894559, 0.3333333333333333703, 0.3219752754296894559, 0.3333333333333333703, 0.3219752754296894559, 0.3333333333333333703, 0.3219752754296894559, 0.3333333333333333703, 0.3219752754296894559, 0.3333333333333333703, 0.3219752754296894559, 0.3333333333333333703, 0.3219752754296894559, 0.3333333333333333703, 0.3219752754296894559, 0.3333333333333333703, 0.3219752754296894559, 0.3333333333333333703, 0.3219752754296894559, 0.3333333333333333703, 0.3219752754296894559, 0.3333333333333333703, 0.3219752754296894559, 0.3333333333333333703, 0.3219752754296894559, 0.3333333333333333703, 0.3219752754296894559, 0.3333333333333333703, 0.3219752754296894559, 0.3333333333333333703, 0.3219752754296894559, 0.3333333333333333703, 0.3219752754296894559, 0.3333333333333333703, 0.3219752754296894559, 0.3333333333333333703, 0.3219752754296894559, 0.3333333333333333703, 0.3219752754296894559, 0.3333333333333333703, 0.3219752754296894559, 0.3333333333333333703, 0.3219752754296894559, 0.3333333333333333703, 0.3219752754296894559, 0.3333333333333333703, 0.3219752754296894559, 0.3333333333333333703, 0.3219752754296894559, 0.3333333333333333703, 0.3219752754296894559, 0.3333333333333333703, 0.3219752754296894559, 0.3333333333333333703, 0.3219752754296894559, 0.3333333333333333703, 0.3219752754296894559, 0.3333333333333333703, 0.3219752754296894559, 0.3333333333333333703, 0.3219752754296894559, 0.3333333333333333703, 0.3219752754296894559, 0.3333333333333333703, 0.3219752754296894559, 0.3333333333333333703, 0.3219752754296894559, 0.3333333333333333703, 0.3219752754296894559, 0.3333333333333333703, 0.3219752754296894559, 0.3333333333333333703, 0.3219752754296894559, 0.3333333333333333703, 0.3219752754296894559, 0.3333333333333333703, 0.3219752754296894559, 0.3333333333333333703, 0.3219752754296894559, 0.3333333333333333703, 0.3219752754296894559, 0.3333333333333333703, 0.3219752754296894559, 0.3333333333333333703, 0.3219752754296894559, 0.3333333333333333703, 0.3219752754296894559, 0.3333333333333333703, 0.3219752754296894559, 0.3333333333333333703, 0.3219752754296894559, 0.3333333333333333703, 0.3219752754296894559, 0.3333333333333333703, 0.3219752754296894559, 0.3333333333333333703, 0.3219752754296894559, 0.3333333333333333703, 0.3219752754296894559, 0.3333333333333333703, 0.3219752754296894559, 0.3333333333333333703, 0.3219752754296894559, 0.3333333333333333703, 0.3219752754296894559, 0.3333333333333333703, 0.3219752754296894559, 0.3333333333333333703, 0.3219752754296894559, 0.3333333333333333703, 0.3219752754296894559, 0.3333333333333333703, 0.3219752754296894559, 0.3333333333333333703, 0.3219752754296894559, 0.3333333333333333703, 0.3219752754296894559, 0.3333333333333333703, 0.3219752754296894559, 0.3333333333333333703, 0.3219752754296894559, 0.3333333333333333703, 0.3219752754296894559, 0.3333333333333333703, 0.3219752754296894559, 0.3333333333333333703, 0.3219752754296894559, 0.3333333333333333703, 0.3219752754296894559, 0.3333333333333333703, 0.3219752754296894559, 0.3333333333333333703, 0.3219752754296894559, 0.3333333333333333703, 0.3219752754296894559, 0.3333333333333333703, 0.3219752754296894559, 0.3333333333333333703, 0.3219752754296894559, 0.3333333333333333703, 0.3219752754296894559, 0.3333333333333333703, 0.3219752754296894559, 0.3333333333333333703, 0.3219752754296894559, 0.3333333333333333703, 0.3219752754296894559, 0.3333333333333333703, 0.3219752754296894559, 0.3333333333333333703, 0.3219752754296894559, 0.3333333333333333703, 0.3219752754296894559, 0.3333333333333333703, 0.3219752754296894559, 0.3333333333333333703, 0.3219752754296894559, 0.3333333333333333703),
 ( 1.000000000000000000, 0.9659258262890683122, 1.000000000000000000, 0.9659258262890683122, 1.000000000000000000, 0.9659258262890683122, 1.000000000000000000, 0.9659258262890683122, 1.000000000000000000, 0.9659258262890683122, 1.000000000000000000, 0.9659258262890683122, 1.000000000000000000, 0.9659258262890683122, 1.000000000000000000, 0.9659258262890683122, 1.000000000000000000, 0.9659258262890683122, 1.000000000000000000, 0.9659258262890683122, 1.000000000000000000, 0.9659258262890683122, 1.000000000000000000, 0.9659258262890683122, 1.000000000000000000, 0.9659258262890683122, 1.000000000000000000, 0.9659258262890683122, 1.000000000000000000, 0.9659258262890683122, 1.000000000000000000, 0.9659258262890683122, 1.000000000000000000, 0.9659258262890683122, 1.000000000000000000, 0.9659258262890683122, 1.000000000000000000, 0.9659258262890683122, 1.000000000000000000, 0.9659258262890683122, 1.000000000000000000, 0.9659258262890683122, 1.000000000000000000, 0.9659258262890683122, 1.000000000000000000, 0.9659258262890683122, 1.000000000000000000, 0.9659258262890683122, 1.000000000000000000, 0.9659258262890683122, 1.000000000000000000, 0.9659258262890683122, 1.000000000000000000, 0.9659258262890683122, 1.000000000000000000, 0.9659258262890683122, 1.000000000000000000, 0.9659258262890683122, 1.000000000000000000, 0.9659258262890683122, 1.000000000000000000, 0.9659258262890683122, 1.000000000000000000, 0.9659258262890683122, 1.000000000000000000, 0.9659258262890683122, 1.000000000000000000, 0.9659258262890683122, 1.000000000000000000, 0.9659258262890683122, 1.000000000000000000, 0.9659258262890683122, 1.000000000000000000, 0.9659258262890683122, 1.000000000000000000, 0.9659258262890683122, 1.000000000000000000, 0.9659258262890683122, 1.000000000000000000, 0.9659258262890683122, 1.000000000000000000, 0.9659258262890683122, 1.000000000000000000, 0.9659258262890683122, 1.000000000000000000, 0.9659258262890683122, 1.000000000000000000, 0.9659258262890683122, 1.000000000000000000, 0.9659258262890683122, 1.000000000000000000, 0.9659258262890683122, 1.000000000000000000, 0.9659258262890683122, 1.000000000000000000, 0.9659258262890683122, 1.000000000000000000, 0.9659258262890683122, 1.000000000000000000, 0.9659258262890683122, 1.000000000000000000, 0.9659258262890683122, 1.000000000000000000, 0.9659258262890683122, 1.000000000000000000, 0.9659258262890683122, 1.000000000000000000, 0.9659258262890683122, 1.000000000000000000, 0.9659258262890683122, 1.000000000000000000, 0.9659258262890683122, 1.000000000000000000, 0.9659258262890683122, 1.000000000000000000, 0.9659258262890683122, 1.000000000000000000, 0.9659258262890683122, 1.000000000000000000, 0.9659258262890683122, 1.000000000000000000, 0.9659258262890683122, 1.000000000000000000, 0.9659258262890683122, 1.000000000000000000, 0.9659258262890683122, 1.000000000000000000, 0.9659258262890683122, 1.000000000000000000, 0.9659258262890683122, 1.000000000000000000, 0.9659258262890683122, 1.000000000000000000, 0.9659258262890683122, 1.000000000000000000, 0.9659258262890683122, 1.000000000000000000, 0.9659258262890683122, 1.000000000000000000, 0.9659258262890683122, 1.000000000000000000, 0.9659258262890683122, 1.000000000000000000, 0.9659258262890683122, 1.000000000000000000, 0.9659258262890683122, 1.000000000000000000, 0.9659258262890683122, 1.000000000000000000, 0.9659258262890683122, 1.000000000000000000, 0.9659258262890683122, 1.000000000000000000, 0.9659258262890683122, 1.000000000000000000, 0.9659258262890683122, 1.000000000000000000, 0.9659258262890683122, 1.000000000000000000, 0.9659258262890683122, 1.000000000000000000, 0.9659258262890683122, 1.000000000000000000, 0.9659258262890683122, 1.000000000000000000, 0.9659258262890683122, 1.000000000000000000, 0.9659258262890683122, 1.000000000000000000, 0.9659258262890683122, 1.000000000000000000, 0.9659258262890683122, 1.000000000000000000, 0.9659258262890683122, 1.000000000000000000, 0.9659258262890683122, 1.000000000000000000, 0.9659258262890683122, 1.000000000000000000, 0.9659258262890683122, 1.000000000000000000, 0.9659258262890683122, 1.000000000000000000, 0.9659258262890683122, 1.000000000000000000, 0.9659258262890683122, 1.000000000000000000, 0.9659258262890683122, 1.000000000000000000, 0.9659258262890683122, 1.000000000000000000, 0.9659258262890683122, 1.000000000000000000, 0.9659258262890683122, 1.000000000000000000, 0.9659258262890683122, 1.000000000000000000, 0.9659258262890683122, 1.000000000000000000, 0.9659258262890683122, 1.000000000000000000, 0.9659258262890683122, 1.000000000000000000, 0.9659258262890683122, 1.000000000000000000, 0.9659258262890683122, 1.000000000000000000, 0.9659258262890683122, 1.000000000000000000, 0.9659258262890683122, 1.000000000000000000, 0.9659258262890683122, 1.000000000000000000, 0.9659258262890683122, 1.000000000000000000, 0.9659258262890683122, 1.000000000000000000, 0.9659258262890683122, 1.000000000000000000, 0.9659258262890683122, 1.000000000000000000, 0.9659258262890683122, 1.000000000000000000, 0.9659258262890683122, 1.000000000000000000, 0.9659258262890683122, 1.000000000000000000, 0.9659258262890683122, 1.000000000000000000, 0.9659258262890683122, 1.000000000000000000, 0.9659258262890683122, 1.000000000000000000, 0.9659258262890683122, 1.000000000000000000, 0.9659258262890683122, 1.000000000000000000, 0.9659258262890683122, 1.000000000000000000, 0.9659258262890683122, 1.000000000000000000, 0.9659258262890683122, 1.000000000000000000, 0.9659258262890683122, 1.000000000000000000, 0.9659258262890683122, 1.000000000000000000, 0.9659258262890683122, 1.000000000000000000, 0.9659258262890683122, 1.000000000000000000, 0.9659258262890683122, 1.000000000000000000, 0.9659258262890683122, 1.000000000000000000, 0.9659258262890683122, 1.000000000000000000, 0.9659258262890683122, 1.000000000000000000, 0.9659258262890683122, 1.000000000000000000, 0.9659258262890683122, 1.000000000000000000, 0.9659258262890683122, 1.000000000000000000, 0.9659258262890683122, 1.000000000000000000, 0.9659258262890683122, 1.000000000000000000, 0.9659258262890683122, 1.000000000000000000, 0.9659258262890683122, 1.000000000000000000, 0.9659258262890683122, 1.000000000000000000, 0.9659258262890683122, 1.000000000000000000, 0.9659258262890683122, 1.000000000000000000, 0.9659258262890683122, 1.000000000000000000, 0.9659258262890683122, 1.000000000000000000, 0.9659258262890683122, 1.000000000000000000, 0.9659258262890683122, 1.000000000000000000, 0.9659258262890683122, 1.000000000000000000, 0.9659258262890683122, 1.000000000000000000, 0.9659258262890683122, 1.000000000000000000, 0.9659258262890683122, 1.000000000000000000, 0.9659258262890683122, 1.000000000000000000, 0.9659258262890683122, 1.000000000000000000, 0.9659258262890683122, 1.000000000000000000, 0.9659258262890683122, 1.000000000000000000, 0.9659258262890683122, 1.000000000000000000, 0.9659258262890683122, 1.000000000000000000, 0.9659258262890683122, 1.000000000000000000, 0.9659258262890683122, 1.000000000000000000, 0.9659258262890683122, 1.000000000000000000, 0.9659258262890683122, 1.000000000000000000, 0.9659258262890683122, 1.000000000000000000, 0.9659258262890683122, 1.000000000000000000, 0.9659258262890683122, 1.000000000000000000, 0.9659258262890683122, 1.000000000000000000, 0.9659258262890683122, 1.000000000000000000, 0.9659258262890683122, 1.000000000000000000, 0.9659258262890683122, 1.000000000000000000, 0.9659258262890683122, 1.000000000000000000, 0.9659258262890683122, 1.000000000000000000, 0.9659258262890683122, 1.000000000000000000, 0.9659258262890683122, 1.000000000000000000, 0.9659258262890683122, 1.000000000000000000, 0.9659258262890683122, 1.000000000000000000, 0.9659258262890683122, 1.000000000000000000, 0.9659258262890683122, 1.000000000000000000, 0.9659258262890683122, 1.000000000000000000, 0.9659258262890683122, 1.000000000000000000, 0.9659258262890683122, 1.000000000000000000, 0.9659258262890683122, 1.000000000000000000, 0.9659258262890683122, 1.000000000000000000, 0.9659258262890683122, 1.000000000000000000, 0.9659258262890683122, 1.000000000000000000, 0.9659258262890683122, 1.000000000000000000, 0.9659258262890683122, 1.000000000000000000, 0.9659258262890683122, 1.000000000000000000, 0.9659258262890683122, 1.000000000000000000, 0.9659258262890683122, 1.000000000000000000, 0.9659258262890683122, 1.000000000000000000, 0.9659258262890683122, 1.000000000000000000, 0.9659258262890683122, 1.000000000000000000, 0.9659258262890683122, 1.000000000000000000, 0.9659258262890683122, 1.000000000000000000, 0.9659258262890683122, 1.000000000000000000, 0.9659258262890683122, 1.000000000000000000, 0.9659258262890683122, 1.000000000000000000, 0.9659258262890683122, 1.000000000000000000, 0.9659258262890683122, 1.000000000000000000, 0.9659258262890683122, 1.000000000000000000, 0.9659258262890683122, 1.000000000000000000, 0.9659258262890683122, 1.000000000000000000, 0.9659258262890683122, 1.000000000000000000, 0.9659258262890683122, 1.000000000000000000, 0.9659258262890683122, 1.000000000000000000, 0.9659258262890683122, 1.000000000000000000, 0.9659258262890683122, 1.000000000000000000, 0.9659258262890683122, 1.000000000000000000, 0.9659258262890683122, 1.000000000000000000, 0.9659258262890683122, 1.000000000000000000, 0.9659258262890683122, 1.000000000000000000, 0.9659258262890683122, 1.000000000000000000, 0.9659258262890683122, 1.000000000000000000, 0.9659258262890683122, 1.000000000000000000, 0.9659258262890683122, 1.000000000000000000, 0.9659258262890683122, 1.000000000000000000, 0.9659258262890683122, 1.000000000000000000, 0.9659258262890683122, 1.000000000000000000, 0.9659258262890683122, 1.000000000000000000, 0.9659258262890683122, 1.000000000000000000, 0.9659258262890683122, 1.000000000000000000, 0.9659258262890683122, 1.000000000000000000, 0.9659258262890683122, 1.000000000000000000, 0.9659258262890683122, 1.000000000000000000, 0.9659258262890683122, 1.000000000000000000, 0.9659258262890683122, 1.000000000000000000, 0.9659258262890683122, 1.000000000000000000, 0.9659258262890683122, 1.000000000000000000, 0.9659258262890683122, 1.000000000000000000, 0.9659258262890683122, 1.000000000000000000, 0.9659258262890683122, 1.000000000000000000, 0.9659258262890683122, 1.000000000000000000, 0.9659258262890683122, 1.000000000000000000) ) ) 
 REPRESENTATION_ITEM ( '' )  SURFACE ( )  );
#61714=CARTESIAN_POINT ( 'NONE',  ( -10.72451020669870658, -18.67979575497194134, 54.58442372801901143 ) ) ;
#61715=CARTESIAN_POINT ( 'NONE',  ( 19.05341960407611168, 5.049401038298154454, 48.95724293864768129 ) ) ;
#61716=CARTESIAN_POINT ( 'NONE',  ( 13.97604488694527802, 13.89961937509977652, 84.37390960531433848 ) ) ;
#61717=CARTESIAN_POINT ( 'NONE',  ( -16.51473224551082808, 9.474510206698731452, 63.33442372801900433 ) ) ;
#61718=CARTESIAN_POINT ( 'NONE',  ( 18.67979575497194134, -10.72451020669871369, 35.83442372801901143 ) ) ;
#61719=CARTESIAN_POINT ( 'NONE',  ( 19.02544592524334988, 5.153800228976608722, 101.4594237280189759 ) ) ;
#61720=CARTESIAN_POINT ( 'NONE',  ( -5.049401038297874678, -19.05341960407617918, 74.79275706135231871 ) ) ;
#61721=CARTESIAN_POINT ( 'NONE',  ( -19.05341960407611168, -5.049401038298163336, 41.45724293864769550 ) ) ;
#61722=CARTESIAN_POINT ( 'NONE',  ( -0.05219959533936034679, 19.03943276465977164, 87.50109039468567573 ) ) ;
#61723=CARTESIAN_POINT ( 'NONE',  ( 16.53943276465976808, 0.05219959533934440121, 111.2510903946856899 ) ) ;
#61724=CARTESIAN_POINT ( 'NONE',  ( 5.153800228976615827, -19.02544592524334988, 80.20942372801901854 ) ) ;
#61725=CARTESIAN_POINT ( 'NONE',  ( 8.314922557960818139, 14.29746914071049879, 29.58224293864769905 ) ) ;
#61726=CARTESIAN_POINT ( 'NONE',  ( -9.474510206698720793, -16.51473224551083518, 54.58442372801899722 ) ) ;
#61727=CARTESIAN_POINT ( 'NONE',  ( 10.81492255796106328, -18.62759615963255655, 100.4177570613523471 ) ) ;
#61728=CARTESIAN_POINT ( 'NONE',  ( 0.05219959533936267826, -19.03943276465977164, 30.00109039468566863 ) ) ;
#61729=CARTESIAN_POINT ( 'NONE',  ( 16.51473224551069308, 9.474510206698969483, 24.16557627198102765 ) ) ;
#61730=CARTESIAN_POINT ( 'NONE',  ( -15.80617190586768217, 15.72974639402176855, 83.12609039468568994 ) ) ;
#61731=CARTESIAN_POINT ( 'NONE',  ( 4.379528057220092307, 16.55341960407617563, 32.29275706135235424 ) ) ;
#61732=CARTESIAN_POINT ( 'NONE',  ( 5.153800228976335163, 19.02544592524342804, 89.79057627198102409 ) ) ;
#61734=CARTESIAN_POINT ( 'NONE',  ( -19.05341960407611168, -5.049401038298163336, 76.45724293864769550 ) ) ;
#61736=CARTESIAN_POINT ( 'NONE',  ( 9.474510206698729675, 16.51473224551082808, 82.08442372801899012 ) ) ;
#61737=CARTESIAN_POINT ( 'NONE',  ( 5.153800228976335163, 19.02544592524342804, 114.7905762719810241 ) ) ;
#61738=CARTESIAN_POINT ( 'NONE',  ( -15.72974639402176322, -15.80617190586768395, 109.3760903946857042 ) ) ;
#61739=CARTESIAN_POINT ( 'NONE',  ( 13.89961937509957401, 13.97604488694547697, 101.8760903946856331 ) ) ;
#61740=CARTESIAN_POINT ( 'NONE',  ( -16.52544592524342804, 4.483927247898546575, 96.04057627198102409 ) ) ;
#61741=CARTESIAN_POINT ( 'NONE',  ( -16.51473224551069308, -9.474510206698971260, 21.66557627198102765 ) ) ;
#61742=CARTESIAN_POINT ( 'NONE',  ( 0.05219959533907565091, 21.53943276465977519, 54.99890960531435269 ) ) ;
#61743=CARTESIAN_POINT ( 'NONE',  ( -5.823673210054116645, -21.52544592524344225, 47.29057627198103120 ) ) ;
#61744=CARTESIAN_POINT ( 'NONE',  ( 4.483927247898545687, 16.52544592524342804, 114.7905762719810383 ) ) ;
#61746=CARTESIAN_POINT ( 'NONE',  ( 13.89961937509957401, 13.97604488694547697, 56.87609039468564731 ) ) ;
#61747=CARTESIAN_POINT ( 'NONE',  ( 8.314922557960818139, 14.29746914071049879, 34.58224293864770260 ) ) ;
#61748=CARTESIAN_POINT ( 'NONE',  ( 5.049401038298161559, -19.05341960407611168, 112.7072429386476813 ) ) ;
#61749=CARTESIAN_POINT ( 'NONE',  ( 15.80617190586769283, -15.72974639402175789, 75.62609039468567573 ) ) ;
#61750=CARTESIAN_POINT ( 'NONE',  ( -5.719274019375978568, 21.55341960407610458, 65.20724293864768129 ) ) ;
#61751=CARTESIAN_POINT ( 'NONE',  ( 15.72974639402176855, 15.80617190586768217, 61.87609039468568284 ) ) ;
#61752=CARTESIAN_POINT ( 'NONE',  ( 10.81492255796106328, -18.62759615963255655, 45.41775706135234003 ) ) ;
#61753=CARTESIAN_POINT ( 'NONE',  ( 5.049401038298161559, -19.05341960407611168, 77.70724293864765286 ) ) ;
#61754=CARTESIAN_POINT ( 'NONE',  ( -4.379528057220086978, -16.55341960407618274, 89.79275706135236135 ) ) ;
#61755=CARTESIAN_POINT ( 'NONE',  ( -9.474510206698964154, 16.51473224551069663, 25.41557627198103120 ) ) ;
#61757=CARTESIAN_POINT ( 'NONE',  ( -14.29746914071049879, 8.314922557960819915, 65.83224293864769550 ) ) ;
#61758=CARTESIAN_POINT ( 'NONE',  ( -12.14591786802309592, -12.06949235617757132, 36.87390960531435979 ) ) ;
#61759=CARTESIAN_POINT ( 'NONE',  ( -19.02544592524342804, 5.153800228976336051, 61.04057627198103120 ) ) ;
#61760=CARTESIAN_POINT ( 'NONE',  ( 9.474510206698971260, -16.51473224551069308, 37.91557627198102409 ) ) ;
#61761=CARTESIAN_POINT ( 'NONE',  ( -0.05219959533907301413, -21.53943276465977519, 42.49890960531435979 ) ) ;
#61762=CARTESIAN_POINT ( 'NONE',  ( -5.049401038297874678, -19.05341960407617918, 34.79275706135233293 ) ) ;
#61763=CARTESIAN_POINT ( 'NONE',  ( 30.00000000000000000, -5.499999999999992895, 37.50000000000000000 ) ) ;
#61764=CARTESIAN_POINT ( 'NONE',  ( -4.379528057220328563, 16.55341960407611168, 55.20724293864770260 ) ) ;
#61765=CARTESIAN_POINT ( 'NONE',  ( -21.55341960407610458, -5.719274019375992779, 26.45724293864768839 ) ) ;
#61767=CARTESIAN_POINT ( 'NONE',  ( 14.29746914071037800, 8.314922557961029526, 71.66775706135234714 ) ) ;
#61768=CARTESIAN_POINT ( 'NONE',  ( 5.153800228976615827, -19.02544592524334988, 75.20942372801896170 ) ) ;
#61769=CARTESIAN_POINT ( 'NONE',  ( -0.05219959533910754901, -16.53943276465976808, 47.49890960531435979 ) ) ;
#61770=VERTEX_POINT ( 'NONE', #8239 ) ;
#61771=CARTESIAN_POINT ( 'NONE',  ( -18.39639308325438094, -5.499999999999986677, 76.48252246182195790 ) ) ;
#61772=CARTESIAN_POINT ( 'NONE',  ( -4.379528057220328563, 16.55341960407611168, 25.20724293864769550 ) ) ;
#61773=CARTESIAN_POINT ( 'NONE',  ( -13.97604488694527625, -13.89961937509977652, 56.87390960531434558 ) ) ;
#61774=CARTESIAN_POINT ( 'NONE',  ( -5.153800228976328057, -19.02544592524343514, 72.29057627198102409 ) ) ;
#61775=CARTESIAN_POINT ( 'NONE',  ( 0.05219959533909260263, 19.03943276465977164, 44.99890960531435979 ) ) ;
#61776=CARTESIAN_POINT ( 'NONE',  ( 18.67979575497194134, -10.72451020669871369, 40.83442372801901854 ) ) ;
#61777=CARTESIAN_POINT ( 'NONE',  ( 13.89961937509977652, -13.97604488694527269, 63.12390960531435979 ) ) ;
#61779=CARTESIAN_POINT ( 'NONE',  ( -19.02544592524342804, 5.153800228976336051, 46.04057627198101699 ) ) ;
#61780=CARTESIAN_POINT ( 'NONE',  ( 10.81492255796078972, 18.62759615963270932, 34.58224293864770260 ) ) ;
#61781=CARTESIAN_POINT ( 'NONE',  ( 15.72974639402176855, 15.80617190586768217, 66.87609039468568994 ) ) ;
#61782=CARTESIAN_POINT ( 'NONE',  ( -16.51473224551069308, -9.474510206698971260, 26.66557627198103120 ) ) ;
#61783=CARTESIAN_POINT ( 'NONE',  ( 18.67979575497178502, 10.72451020669898547, 29.16557627198103120 ) ) ;
#61784=CARTESIAN_POINT ( 'NONE',  ( -12.14591786802326823, 12.06949235617739902, 88.12609039468570415 ) ) ;
#61785=CARTESIAN_POINT ( 'NONE',  ( 18.62759615963255655, 10.81492255796105972, 101.6677570613523613 ) ) ;
#61786=CARTESIAN_POINT ( 'NONE',  ( 14.29746914071037800, 8.314922557961029526, 61.66775706135235424 ) ) ;
#61787=CARTESIAN_POINT ( 'NONE',  ( 9.474510206698971260, -16.51473224551069308, 112.9155762719810383 ) ) ;
#61788=CARTESIAN_POINT ( 'NONE',  ( 16.52544592524335698, 4.483927247898782831, 51.45942372801901854 ) ) ;
#61789=CARTESIAN_POINT ( 'NONE',  ( 4.379528057220092307, 16.55341960407617563, 42.29275706135235424 ) ) ;
#61790=CARTESIAN_POINT ( 'NONE',  ( -12.14591786802326823, 12.06949235617739902, 93.12609039468568994 ) ) ;
#61791=CARTESIAN_POINT ( 'NONE',  ( -21.53943276465977519, -0.05219959533937600094, 48.75109039468568284 ) ) ;
#61792=CARTESIAN_POINT ( 'NONE',  ( -4.379528057220086978, -16.55341960407618274, 19.79275706135235069 ) ) ;
#61793=CARTESIAN_POINT ( 'NONE',  ( -21.52544592524343514, 5.823673210054127303, 116.0405762719810383 ) ) ;
#61794=CARTESIAN_POINT ( 'NONE',  ( -0.05219959533934338120, 16.53943276465976808, 22.50109039468567573 ) ) ;
#61795=CARTESIAN_POINT ( 'NONE',  ( 12.14591786802327356, -12.06949235617739191, 90.62609039468567573 ) ) ;
#61797=CARTESIAN_POINT ( 'NONE',  ( 10.72451020669871369, 18.67979575497193778, 82.08442372801901854 ) ) ;
#61798=CARTESIAN_POINT ( 'NONE',  ( -16.46253265017146816, -9.564922557961047289, 89.16775706135234714 ) ) ;
#61799=CARTESIAN_POINT ( 'NONE',  ( -14.29746914071049879, 8.314922557960819915, 55.83224293864770260 ) ) ;
#61800=CARTESIAN_POINT ( 'NONE',  ( 16.55341960407611168, 4.379528057220329451, 38.95724293864768839 ) ) ;
#61801=CARTESIAN_POINT ( 'NONE',  ( 16.52544592524342804, -4.483927247898539470, 103.5405762719810383 ) ) ;
#61802=CARTESIAN_POINT ( 'NONE',  ( -0.05219959533936034679, 19.03943276465977164, 47.50109039468566863 ) ) ;
#61803=CARTESIAN_POINT ( 'NONE',  ( 17.72517630440436065, -5.499999999999998224, 53.42175719257213728 ) ) ;
#61804=CARTESIAN_POINT ( 'NONE',  ( -5.719274019375665041, -21.55341960407619695, 44.79275706135234714 ) ) ;
#61805=CARTESIAN_POINT ( 'NONE',  ( -19.03943276465977164, -0.05219959533935918106, 113.7510903946856757 ) ) ;
#61807=CARTESIAN_POINT ( 'NONE',  ( -5.049401038298153566, 19.05341960407611168, 105.2072429386476671 ) ) ;
#61808=CARTESIAN_POINT ( 'NONE',  ( -5.823673210054116645, -21.52544592524344225, 77.29057627198102409 ) ) ;
#61809=CARTESIAN_POINT ( 'NONE',  ( -19.05341960407617563, 5.049401038297882671, 98.54275706135233293 ) ) ;
#61810=CARTESIAN_POINT ( 'NONE',  ( 19.02544592524343514, -5.153800228976328945, 103.5405762719809957 ) ) ;
#61811=CARTESIAN_POINT ( 'NONE',  ( 13.97604488694548053, -13.89961937509957401, 50.62609039468566152 ) ) ;
#61812=CARTESIAN_POINT ( 'NONE',  ( -14.29746914071049879, 8.314922557960819915, 110.8322429386476955 ) ) ;
#61813=CARTESIAN_POINT ( 'NONE',  ( -18.67979575497193778, 10.72451020669871902, 98.33442372801901854 ) ) ;
#61814=CARTESIAN_POINT ( 'NONE',  ( 19.05341960407611168, 5.049401038298154454, 28.95724293864769550 ) ) ;
#61815=CARTESIAN_POINT ( 'NONE',  ( -10.72451020669870658, -18.67979575497194134, 54.58442372801901143 ) ) ;
#61816=CARTESIAN_POINT ( 'NONE',  ( 21.53943276465977519, 0.05219959533937863772, 91.25109039468568994 ) ) ;
#61817=CARTESIAN_POINT ( 'NONE',  ( 16.53943276465976808, 0.05219959533934440121, 86.25109039468568994 ) ) ;
#61818=CARTESIAN_POINT ( 'NONE',  ( 15.72974639402176855, 15.80617190586768217, 36.87609039468568994 ) ) ;
#61819=CARTESIAN_POINT ( 'NONE',  ( 5.823673210054444382, -21.52544592524334988, 35.20942372801901854 ) ) ;
#61820=CARTESIAN_POINT ( 'NONE',  ( 19.03943276465977164, 0.05219959533936151252, 66.25109039468567573 ) ) ;
#61821=CARTESIAN_POINT ( 'NONE',  ( 5.153800228976335163, 19.02544592524342804, 79.79057627198102409 ) ) ;
#61822=CARTESIAN_POINT ( 'NONE',  ( 8.224510206698953496, -14.34966873604960469, 102.9155762719810383 ) ) ;
#61823=CARTESIAN_POINT ( 'NONE',  ( 5.719274019375991003, -21.55341960407610458, 77.70724293864770971 ) ) ;
#61824=CARTESIAN_POINT ( 'NONE',  ( 12.06949235617757843, -12.14591786802309237, 63.12390960531435979 ) ) ;
#61825=CARTESIAN_POINT ( 'NONE',  ( 5.823673210054444382, -21.52544592524334988, 110.2094237280190185 ) ) ;
#61826=CARTESIAN_POINT ( 'NONE',  ( 4.379528057220339221, -16.55341960407611168, 87.70724293864769550 ) ) ;
#61827=CARTESIAN_POINT ( 'NONE',  ( 9.564922557960805705, 16.46253265017160317, 39.58224293864768839 ) ) ;
#61828=CARTESIAN_POINT ( 'NONE',  ( 16.51473224551083163, -9.474510206698727899, 65.83442372801900433 ) ) ;
#61829=CARTESIAN_POINT ( 'NONE',  ( 0.05219959533910956823, 16.53943276465976808, 49.99890960531437401 ) ) ;
#61830=CARTESIAN_POINT ( 'NONE',  ( 10.81492255796106328, -18.62759615963255655, 90.41775706135236135 ) ) ;
#61831=CARTESIAN_POINT ( 'NONE',  ( -9.564922557960796823, -16.46253265017161027, 87.08224293864769550 ) ) ;
#61832=CARTESIAN_POINT ( 'NONE',  ( 0.05219959533936267826, -19.03943276465977164, 55.00109039468566863 ) ) ;
#61833=CARTESIAN_POINT ( 'NONE',  ( 21.52544592524344225, -5.823673210054117533, 58.54057627198103120 ) ) ;
#61834=CARTESIAN_POINT ( 'NONE',  ( 21.55341960407610458, 5.719274019375980345, 108.9572429386476955 ) ) ;
#61835=CARTESIAN_POINT ( 'NONE',  ( -16.53943276465976808, -0.05219959533934237506, 18.75109039468568639 ) ) ;
#61836=CARTESIAN_POINT ( 'NONE',  ( -0.05219959533934338120, 16.53943276465976808, 77.50109039468567573 ) ) ;
#61837=CARTESIAN_POINT ( 'NONE',  ( 18.22780087662126647, 5.499999999999818812, 56.48236817873107185 ) ) ;
#61838=CARTESIAN_POINT ( 'NONE',  ( 15.72974639402176855, 15.80617190586768217, 26.87609039468567218 ) ) ;
#61839=CARTESIAN_POINT ( 'NONE',  ( 19.02544592524343514, -5.153800228976328945, 23.54057627198102054 ) ) ;
#61841=CARTESIAN_POINT ( 'NONE',  ( -12.06949235617739369, -12.14591786802326823, 44.37609039468567573 ) ) ;
#61843=CARTESIAN_POINT ( 'NONE',  ( -4.483927247898539470, -16.52544592524342804, 82.29057627198103830 ) ) ;
#61844=CARTESIAN_POINT ( 'NONE',  ( 18.67979575497178502, 10.72451020669898547, 79.16557627198103830 ) ) ;
#61845=CARTESIAN_POINT ( 'NONE',  ( 4.379528057220092307, 16.55341960407617563, 102.2927570613523613 ) ) ;
#61846=CARTESIAN_POINT ( 'NONE',  ( -0.05219959533934338120, 16.53943276465976808, 32.50109039468568284 ) ) ;
#61847=CARTESIAN_POINT ( 'NONE',  ( 13.97604488694527802, 13.89961937509977652, 49.37390960531434558 ) ) ;
#61848=CARTESIAN_POINT ( 'NONE',  ( 12.14591786802327356, -12.06949235617739191, 80.62609039468567573 ) ) ;
#61849=CARTESIAN_POINT ( 'NONE',  ( -19.05341960407617563, 5.049401038297882671, 78.54275706135233293 ) ) ;
#61850=CARTESIAN_POINT ( 'NONE',  ( -15.72974639402197994, 15.80617190586746368, 70.62390960531436690 ) ) ;
#61851=CARTESIAN_POINT ( 'NONE',  ( 12.06949235617739724, 12.14591786802326823, 101.8760903946857042 ) ) ;
#61852=CARTESIAN_POINT ( 'NONE',  ( 0.05219959533937995610, -21.53943276465977519, 85.00109039468568994 ) ) ;
#61853=CARTESIAN_POINT ( 'NONE',  ( 10.81492255796078972, 18.62759615963270932, 64.58224293864769550 ) ) ;
#61854=CARTESIAN_POINT ( 'NONE',  ( -0.05219959533907301413, -21.53943276465977519, 42.49890960531435979 ) ) ;
#61856=CARTESIAN_POINT ( 'NONE',  ( 4.379528057220092307, 16.55341960407617563, 72.29275706135236135 ) ) ;
#61857=CARTESIAN_POINT ( 'NONE',  ( -15.72974639402197994, 15.80617190586746368, 50.62390960531435979 ) ) ;
#61859=CARTESIAN_POINT ( 'NONE',  ( 10.72451020669898902, -18.67979575497178502, 22.91557627198102765 ) ) ;
#61860=CARTESIAN_POINT ( 'NONE',  ( -19.26498983726237313, 5.499999999999801048, 75.55319577422001487 ) ) ;
#61861=CARTESIAN_POINT ( 'NONE',  ( -0.05219959533909027116, -19.03943276465977164, 27.49890960531435624 ) ) ;
#61862=CARTESIAN_POINT ( 'NONE',  ( -21.53943276465977519, 0.05219959533907696930, 76.24890960531435269 ) ) ;
#61863=CARTESIAN_POINT ( 'NONE',  ( 12.14591786802327356, -12.06949235617739191, 100.6260903946857184 ) ) ;
#61864=CARTESIAN_POINT ( 'NONE',  ( -15.80617190586768217, 15.72974639402176855, 63.12609039468568994 ) ) ;
#61865=CARTESIAN_POINT ( 'NONE',  ( 14.29746914071037800, 8.314922557961029526, 26.66775706135235424 ) ) ;
#61866=CARTESIAN_POINT ( 'NONE',  ( -0.05219959533910754901, -16.53943276465976808, 112.4989096053143669 ) ) ;
#61867=CARTESIAN_POINT ( 'NONE',  ( -13.97604488694547697, 13.89961937509957934, 113.1260903946856757 ) ) ;
#61868=CARTESIAN_POINT ( 'NONE',  ( 0.05219959533909260263, 19.03943276465977164, 34.99890960531435979 ) ) ;
#61870=CARTESIAN_POINT ( 'NONE',  ( 13.89961937509977652, -13.97604488694527269, 103.1239096053143527 ) ) ;
#61871=CARTESIAN_POINT ( 'NONE',  ( -16.53943276465976808, -0.05219959533934237506, 83.75109039468568994 ) ) ;
#61872=CARTESIAN_POINT ( 'NONE',  ( 19.03943276465977164, 0.05219959533936151252, 81.25109039468567573 ) ) ;
#61873=CARTESIAN_POINT ( 'NONE',  ( -19.02544592524334988, -5.153800228976617603, 23.95942372801900078 ) ) ;
#61874=CARTESIAN_POINT ( 'NONE',  ( 0.05219959533907565091, 21.53943276465977519, 64.99890960531435269 ) ) ;
#61875=CARTESIAN_POINT ( 'NONE',  ( 0.05219959533934541429, -16.53943276465976808, 90.00109039468567573 ) ) ;
#61876=CARTESIAN_POINT ( 'NONE',  ( -19.05341960407617563, 5.049401038297882671, 88.54275706135230450 ) ) ;
#61877=CARTESIAN_POINT ( 'NONE',  ( 19.05341960407611168, 5.049401038298154454, 48.95724293864768129 ) ) ;
#61878=CARTESIAN_POINT ( 'NONE',  ( 0.05219959533909260263, 19.03943276465977164, 89.99890960531436690 ) ) ;
#61879=CARTESIAN_POINT ( 'NONE',  ( 10.72451020669871369, 18.67979575497193778, 47.08442372801901854 ) ) ;
#61880=CARTESIAN_POINT ( 'NONE',  ( -9.474510206698964154, 16.51473224551069663, 50.41557627198102409 ) ) ;
#61881=CARTESIAN_POINT ( 'NONE',  ( -16.79531203550649110, -7.028104445595613647, 86.25244988220445919 ) ) ;
#61882=CARTESIAN_POINT ( 'NONE',  ( -5.049401038298153566, 19.05341960407611168, 105.2072429386476671 ) ) ;
#61883=CARTESIAN_POINT ( 'NONE',  ( -8.314922557960811034, -14.29746914071050412, 62.08224293864769550 ) ) ;
#61884=CARTESIAN_POINT ( 'NONE',  ( 21.55341960407610458, 5.719274019375980345, 58.95724293864770971 ) ) ;
#61886=CARTESIAN_POINT ( 'NONE',  ( 5.049401038297881783, 19.05341960407617563, 47.29275706135231161 ) ) ;
#61888=CARTESIAN_POINT ( 'NONE',  ( -9.474510206698964154, 16.51473224551069663, 70.41557627198102409 ) ) ;
#61889=CARTESIAN_POINT ( 'NONE',  ( -16.51473224551069308, -9.474510206698971260, 76.66557627198103830 ) ) ;
#61890=CARTESIAN_POINT ( 'NONE',  ( 8.314922557961029526, -14.29746914071037800, 45.41775706135234003 ) ) ;
#61892=CARTESIAN_POINT ( 'NONE',  ( 13.89961937509957401, 13.97604488694547697, 31.87609039468566863 ) ) ;
#61894=CARTESIAN_POINT ( 'NONE',  ( -16.52544592524335698, -4.483927247898792601, 88.95942372801901854 ) ) ;
#61896=CARTESIAN_POINT ( 'NONE',  ( 16.55341960407618274, -4.379528057220086978, 81.04275706135236135 ) ) ;
#61897=CARTESIAN_POINT ( 'NONE',  ( -14.29746914071037622, -8.314922557961029526, 54.16775706135235424 ) ) ;
#61898=CARTESIAN_POINT ( 'NONE',  ( 0.05219959533936267826, -19.03943276465977164, 25.00109039468566152 ) ) ;
#61899=CARTESIAN_POINT ( 'NONE',  ( 0.05219959533909260263, 19.03943276465977164, 49.99890960531435979 ) ) ;
#61900=CARTESIAN_POINT ( 'NONE',  ( 10.81492255796106328, -18.62759615963255655, 50.41775706135235424 ) ) ;
#61901=CARTESIAN_POINT ( 'NONE',  ( -16.51473224551082808, 9.474510206698731452, 73.33442372801900433 ) ) ;
#61902=CARTESIAN_POINT ( 'NONE',  ( 15.72974639402176855, 15.80617190586768217, 106.8760903946856899 ) ) ;
#61903=CARTESIAN_POINT ( 'NONE',  ( 19.02544592524343514, -5.153800228976328945, 33.54057627198102409 ) ) ;
#61905=CARTESIAN_POINT ( 'NONE',  ( 15.80617190586746368, 15.72974639402197994, 64.37390960531435269 ) ) ;
#61906=CARTESIAN_POINT ( 'NONE',  ( 5.719274019375991003, -21.55341960407610458, 22.70724293864769194 ) ) ;
#61907=CARTESIAN_POINT ( 'NONE',  ( -5.049401038298153566, 19.05341960407611168, 25.20724293864768484 ) ) ;
#61908=CARTESIAN_POINT ( 'NONE',  ( -12.14591786802326823, 12.06949235617739902, 33.12609039468569705 ) ) ;
#61910=CARTESIAN_POINT ( 'NONE',  ( -0.05219959533910754901, -16.53943276465976808, 32.49890960531435979 ) ) ;
#61911=ORIENTED_EDGE ( 'NONE', *, *, #154616, .T. ) ;
#61912=CARTESIAN_POINT ( 'NONE',  ( -10.81492255796105439, 18.62759615963255655, 22.91775706135235069 ) ) ;
#61913=CARTESIAN_POINT ( 'NONE',  ( -14.29746914071049879, 8.314922557960819915, 45.83224293864769550 ) ) ;
#61916=CARTESIAN_POINT ( 'NONE',  ( -5.049401038297874678, -19.05341960407617918, 109.7927570613523187 ) ) ;
#61917=CARTESIAN_POINT ( 'NONE',  ( 19.03943276465977164, 0.05219959533936151252, 21.25109039468565797 ) ) ;
#61918=CARTESIAN_POINT ( 'NONE',  ( 4.379528057220339221, -16.55341960407611168, 42.70724293864770260 ) ) ;
#61919=CARTESIAN_POINT ( 'NONE',  ( 18.62759615963271287, -10.81492255796078972, 98.33224293864769550 ) ) ;
#61921=CARTESIAN_POINT ( 'NONE',  ( 21.52544592524344225, -5.823673210054117533, 58.54057627198103120 ) ) ;
#61922=CARTESIAN_POINT ( 'NONE',  ( -13.97604488694527625, -13.89961937509977652, 76.87390960531433848 ) ) ;
#61923=CARTESIAN_POINT ( 'NONE',  ( 4.483927247898545687, 16.52544592524342804, 49.79057627198102409 ) ) ;
#61924=CARTESIAN_POINT ( 'NONE',  ( 16.46253265017160672, -9.564922557960803928, 93.33224293864769550 ) ) ;
#61926=CARTESIAN_POINT ( 'NONE',  ( -17.49999999999999645, -7.500000000000000888, 118.0000000000000142 ) ) ;
#61927=CARTESIAN_POINT ( 'NONE',  ( -5.049401038297874678, -19.05341960407617918, 54.79275706135234003 ) ) ;
#61928=CARTESIAN_POINT ( 'NONE',  ( -21.55341960407610458, -5.719274019375992779, 91.45724293864769550 ) ) ;
#61929=CARTESIAN_POINT ( 'NONE',  ( -16.53943276465976808, 0.05219959533911058130, 101.2489096053143669 ) ) ;
#61930=CARTESIAN_POINT ( 'NONE',  ( 15.80617190586769283, -15.72974639402175789, 55.62609039468568284 ) ) ;
#61932=CARTESIAN_POINT ( 'NONE',  ( 4.379528057220339221, -16.55341960407611168, 32.70724293864770260 ) ) ;
#61933=CARTESIAN_POINT ( 'NONE',  ( 9.564922557960805705, 16.46253265017160317, 39.58224293864768839 ) ) ;
#61934=CARTESIAN_POINT ( 'NONE',  ( 19.05341960407611168, 5.049401038298154454, 103.9572429386476671 ) ) ;
#61935=CARTESIAN_POINT ( 'NONE',  ( -10.72451020669898014, 18.67979575497178502, 55.41557627198102409 ) ) ;
#61937=CARTESIAN_POINT ( 'NONE',  ( -9.564922557960796823, -16.46253265017161027, 37.08224293864768839 ) ) ;
#61938=CARTESIAN_POINT ( 'NONE',  ( 10.81492255796078972, 18.62759615963270932, 59.58224293864770260 ) ) ;
#61940=CARTESIAN_POINT ( 'NONE',  ( -0.05219959533937732626, 21.53943276465977519, 87.50109039468568994 ) ) ;
#61942=CARTESIAN_POINT ( 'NONE',  ( 16.55341960407618274, -4.379528057220086978, 81.04275706135236135 ) ) ;
#61943=CARTESIAN_POINT ( 'NONE',  ( 14.34966873604972726, -8.224510206698740333, 90.83442372801901854 ) ) ;
#61944=CARTESIAN_POINT ( 'NONE',  ( 0.05219959533909260263, 19.03943276465977164, 59.99890960531436690 ) ) ;
#61945=CARTESIAN_POINT ( 'NONE',  ( 9.564922557960805705, 16.46253265017160317, 64.58224293864769550 ) ) ;
#61947=CARTESIAN_POINT ( 'NONE',  ( -9.474510206698720793, -16.51473224551083518, 24.58442372801900078 ) ) ;
#61948=CARTESIAN_POINT ( 'NONE',  ( -0.05219959533934338120, 16.53943276465976808, 77.50109039468567573 ) ) ;
#61949=CARTESIAN_POINT ( 'NONE',  ( 19.02544592524334988, 5.153800228976608722, 21.45942372801899012 ) ) ;
#61950=CARTESIAN_POINT ( 'NONE',  ( -16.51473224551069308, -9.474510206698971260, 76.66557627198103830 ) ) ;
#61951=CARTESIAN_POINT ( 'NONE',  ( 18.67979575497178502, 10.72451020669898547, 39.16557627198102409 ) ) ;
#61952=CARTESIAN_POINT ( 'NONE',  ( 8.224510206698742110, 14.34966873604972548, 27.08442372801901854 ) ) ;
#61953=CARTESIAN_POINT ( 'NONE',  ( 0.05219959533937995610, -21.53943276465977519, 85.00109039468568994 ) ) ;
#61954=CARTESIAN_POINT ( 'NONE',  ( -14.29746914071037622, -8.314922557961029526, 49.16775706135234003 ) ) ;
#61955=CARTESIAN_POINT ( 'NONE',  ( -10.81492255796078084, -18.62759615963271287, 97.08224293864770971 ) ) ;
#61956=CARTESIAN_POINT ( 'NONE',  ( 4.379528057220092307, 16.55341960407617563, 22.29275706135235069 ) ) ;
#61957=CARTESIAN_POINT ( 'NONE',  ( 16.46253265017160672, -9.564922557960803928, 73.33224293864769550 ) ) ;
#61958=CARTESIAN_POINT ( 'NONE',  ( -14.29746914071037622, -8.314922557961029526, 29.16775706135234003 ) ) ;
#61959=CARTESIAN_POINT ( 'NONE',  ( 9.564922557960805705, 16.46253265017160317, 44.58224293864769550 ) ) ;
#61960=CARTESIAN_POINT ( 'NONE',  ( 19.02544592524334988, 5.153800228976608722, 111.4594237280190043 ) ) ;
#61961=CARTESIAN_POINT ( 'NONE',  ( 16.53943276465976808, -0.05219959533910856209, 73.74890960531433848 ) ) ;
#61962=CARTESIAN_POINT ( 'NONE',  ( -8.314922557961024197, 14.29746914071037800, 82.91775706135234714 ) ) ;
#61963=CARTESIAN_POINT ( 'NONE',  ( -10.72451020669870658, -18.67979575497194134, 29.58442372801901854 ) ) ;
#61964=CARTESIAN_POINT ( 'NONE',  ( 5.153800228976335163, 19.02544592524342804, 49.79057627198100988 ) ) ;
#61965=CARTESIAN_POINT ( 'NONE',  ( 5.153800228976335163, 19.02544592524342804, 69.79057627198103830 ) ) ;
#61966=CARTESIAN_POINT ( 'NONE',  ( -4.379528057220086978, -16.55341960407618274, 89.79275706135236135 ) ) ;
#61967=CARTESIAN_POINT ( 'NONE',  ( -17.72662750342728089, -5.500000000000019540, 81.40179492283745333 ) ) ;
#61970=CARTESIAN_POINT ( 'NONE',  ( -19.03943276465977164, -0.05219959533935918106, 28.75109039468566507 ) ) ;
#61971=CARTESIAN_POINT ( 'NONE',  ( -5.049401038298153566, 19.05341960407611168, 30.20724293864768839 ) ) ;
#61972=CARTESIAN_POINT ( 'NONE',  ( 9.564922557960805705, 16.46253265017160317, 109.5822429386476955 ) ) ;
#61974=CARTESIAN_POINT ( 'NONE',  ( 14.34966873604972726, -8.224510206698740333, 35.83442372801901143 ) ) ;
#61975=CARTESIAN_POINT ( 'NONE',  ( 13.89961937509957401, 13.97604488694547697, 51.87609039468566863 ) ) ;
#61976=CARTESIAN_POINT ( 'NONE',  ( -0.05219959533934338120, 16.53943276465976808, 47.50109039468568994 ) ) ;
#61977=CARTESIAN_POINT ( 'NONE',  ( 19.05341960407611168, 5.049401038298154454, 108.9572429386477097 ) ) ;
#61978=CARTESIAN_POINT ( 'NONE',  ( 0.05219959533909260263, 19.03943276465977164, 64.99890960531436690 ) ) ;
#61979=CARTESIAN_POINT ( 'NONE',  ( 21.55341960407610458, 5.719274019375980345, 98.95724293864770971 ) ) ;
#61980=CARTESIAN_POINT ( 'NONE',  ( -13.89961937509977652, 13.97604488694528158, 90.62390960531432427 ) ) ;
#61981=DIRECTION ( 'NONE',  ( 0.000000000000000000, 0.000000000000000000, -1.000000000000000000 ) ) ;
#61982=CARTESIAN_POINT ( 'NONE',  ( -16.46253265017160317, 9.564922557960807481, 65.83224293864769550 ) ) ;
#61983=CARTESIAN_POINT ( 'NONE',  ( 16.53943276465976808, -0.05219959533910856209, 23.74890960531435269 ) ) ;
#61984=CARTESIAN_POINT ( 'NONE',  ( 13.97604488694527802, 13.89961937509977830, 69.37390960531436690 ) ) ;
#61985=CARTESIAN_POINT ( 'NONE',  ( -19.05341960407617563, 5.049401038297882671, 43.54275706135232582 ) ) ;
#61986=CARTESIAN_POINT ( 'NONE',  ( 8.314922557960818139, 14.29746914071049879, 64.58224293864769550 ) ) ;
#61987=CARTESIAN_POINT ( 'NONE',  ( -0.05219959533937732626, 21.53943276465977519, 97.50109039468567573 ) ) ;
#61988=CARTESIAN_POINT ( 'NONE',  ( 0.05219959533909260263, 19.03943276465977164, 39.99890960531436690 ) ) ;
#61989=CARTESIAN_POINT ( 'NONE',  ( -4.483927247898782831, 16.52544592524335698, 52.70942372801902565 ) ) ;
#61990=CARTESIAN_POINT ( 'NONE',  ( 16.53943276465976808, -0.05219959533910856209, 38.74890960531435979 ) ) ;
#61991=CARTESIAN_POINT ( 'NONE',  ( 15.80617190586769283, -15.72974639402175789, 85.62609039468568994 ) ) ;
#61992=CARTESIAN_POINT ( 'NONE',  ( 9.474510206698971260, -16.51473224551069308, 82.91557627198103830 ) ) ;
#61993=CARTESIAN_POINT ( 'NONE',  ( -16.46253265017160317, 9.564922557960807481, 90.83224293864769550 ) ) ;
#61994=CARTESIAN_POINT ( 'NONE',  ( -12.14591786802309592, -12.06949235617757132, 111.8739096053143669 ) ) ;
#61995=CARTESIAN_POINT ( 'NONE',  ( -4.379528057220328563, 16.55341960407611168, 80.20724293864769550 ) ) ;
#61996=CARTESIAN_POINT ( 'NONE',  ( 18.67979575497178502, 10.72451020669898547, 84.16557627198103830 ) ) ;
#61997=CARTESIAN_POINT ( 'NONE',  ( -19.02544592524342804, 5.153800228976336051, 71.04057627198099567 ) ) ;
#61998=CARTESIAN_POINT ( 'NONE',  ( 5.719274019375991003, -21.55341960407610458, 102.7072429386476955 ) ) ;
#61999=CARTESIAN_POINT ( 'NONE',  ( -13.97604488694547697, 13.89961937509957934, 78.12609039468567573 ) ) ;
#62000=CARTESIAN_POINT ( 'NONE',  ( 18.87075004821571866, -5.499999999999894307, 46.17408112101048090 ) ) ;
#62001=CARTESIAN_POINT ( 'NONE',  ( 12.06949235617757843, -12.14591786802309237, 88.12390960531436690 ) ) ;
#62002=CARTESIAN_POINT ( 'NONE',  ( -19.03943276465977164, 0.05219959533909376836, 61.24890960531436690 ) ) ;
#62003=CARTESIAN_POINT ( 'NONE',  ( -15.80617190586745835, -15.72974639402198527, 66.87390960531436690 ) ) ;
#62004=CARTESIAN_POINT ( 'NONE',  ( -17.97058386085788229, -5.499999999999975131, 84.00390968646217971 ) ) ;
#62005=CARTESIAN_POINT ( 'NONE',  ( -12.06949235617756955, 12.14591786802309770, 25.62390960531435624 ) ) ;
#62007=CARTESIAN_POINT ( 'NONE',  ( -19.02544592524334988, -5.153800228976617603, 108.9594237280189759 ) ) ;
#62008=CARTESIAN_POINT ( 'NONE',  ( 8.224510206698953496, -14.34966873604960469, 87.91557627198103830 ) ) ;
#62009=CARTESIAN_POINT ( 'NONE',  ( -19.49671883438227127, -5.500000000000027534, 94.89279849105682274 ) ) ;
#62010=CARTESIAN_POINT ( 'NONE',  ( -9.474510206698964154, 16.51473224551069663, 80.41557627198103830 ) ) ;
#62011=CARTESIAN_POINT ( 'NONE',  ( -5.049401038298153566, 19.05341960407611168, 30.20724293864768839 ) ) ;
#62012=CARTESIAN_POINT ( 'NONE',  ( 16.53943276465976808, -0.05219959533910856209, 73.74890960531433848 ) ) ;
#62013=ADVANCED_FACE ( 'NONE', ( #31378 ), #151744, .F. ) ;
#62014=CARTESIAN_POINT ( 'NONE',  ( 10.81492255796078972, 18.62759615963270932, 24.58224293864768839 ) ) ;
#62015=CARTESIAN_POINT ( 'NONE',  ( -16.46253265017146816, -9.564922557961047289, 94.16775706135233293 ) ) ;
#62016=CARTESIAN_POINT ( 'NONE',  ( -16.51473224551069308, -9.474510206698971260, 76.66557627198103830 ) ) ;
#62017=CARTESIAN_POINT ( 'NONE',  ( 9.564922557960805705, 16.46253265017160317, 84.58224293864769550 ) ) ;
#62018=CARTESIAN_POINT ( 'NONE',  ( -5.719274019375978568, 21.55341960407610458, 70.20724293864769550 ) ) ;
#62019=CARTESIAN_POINT ( 'NONE',  ( -0.05219959533934338120, 16.53943276465976808, 72.50109039468568994 ) ) ;
#62021=CARTESIAN_POINT ( 'NONE',  ( -9.474510206698964154, 16.51473224551069663, 60.41557627198102409 ) ) ;
#62022=CARTESIAN_POINT ( 'NONE',  ( 18.62759615963271287, -10.81492255796078972, 68.33224293864769550 ) ) ;
#62023=CARTESIAN_POINT ( 'NONE',  ( 16.46253265017146816, 9.564922557961045513, 111.6677570613523329 ) ) ;
#62024=CARTESIAN_POINT ( 'NONE',  ( 4.483927247898545687, 16.52544592524342804, 34.79057627198103120 ) ) ;
#62025=CARTESIAN_POINT ( 'NONE',  ( -21.55341960407619339, 5.719274019375674811, 48.54275706135234714 ) ) ;
#62027=CARTESIAN_POINT ( 'NONE',  ( -4.379528057220086978, -16.55341960407618274, 79.79275706135236135 ) ) ;
#62028=CARTESIAN_POINT ( 'NONE',  ( -19.03943276465977164, 0.05219959533909376836, 101.2489096053143669 ) ) ;
#62032=CARTESIAN_POINT ( 'NONE',  ( -16.53943276465976808, -0.05219959533934237506, 93.75109039468567573 ) ) ;
#62033=CARTESIAN_POINT ( 'NONE',  ( -4.483927247898782831, 16.52544592524335698, 52.70942372801902565 ) ) ;
#62034=CARTESIAN_POINT ( 'NONE',  ( 19.05341960407611168, 5.049401038298154454, 58.95724293864768129 ) ) ;
#62035=CARTESIAN_POINT ( 'NONE',  ( 9.564922557960805705, 16.46253265017160317, 69.58224293864770971 ) ) ;
#62036=CARTESIAN_POINT ( 'NONE',  ( -15.72974639402176322, -15.80617190586768395, 59.37609039468568284 ) ) ;
#62037=CARTESIAN_POINT ( 'NONE',  ( -16.52544592524335698, -4.483927247898792601, 68.95942372801901854 ) ) ;
#62038=CARTESIAN_POINT ( 'NONE',  ( -4.483927247898539470, -16.52544592524342804, 27.29057627198103120 ) ) ;
#62039=CARTESIAN_POINT ( 'NONE',  ( -19.02544592524342804, 5.153800228976336051, 36.04057627198100988 ) ) ;
#62040=CARTESIAN_POINT ( 'NONE',  ( -9.474510206698964154, 16.51473224551069663, 35.41557627198102409 ) ) ;
#62041=CARTESIAN_POINT ( 'NONE',  ( -16.55341960407617563, 4.379528057220093196, 23.54275706135235424 ) ) ;
#62042=ORIENTED_EDGE ( 'NONE', *, *, #82839, .T. ) ;
#62043=CARTESIAN_POINT ( 'NONE',  ( 16.51473224551083163, -9.474510206698727899, 75.83442372801900433 ) ) ;
#62044=CARTESIAN_POINT ( 'NONE',  ( -8.314922557960811034, -14.29746914071050412, 77.08224293864769550 ) ) ;
#62045=CARTESIAN_POINT ( 'NONE',  ( -16.46253265017160317, 9.564922557960807481, 45.83224293864769550 ) ) ;
#62046=CARTESIAN_POINT ( 'NONE',  ( 16.51473224551083163, -9.474510206698727899, 80.83442372801899012 ) ) ;
#62048=CARTESIAN_POINT ( 'NONE',  ( -18.62759615963255300, -10.81492255796106328, 94.16775706135237556 ) ) ;
#62049=CARTESIAN_POINT ( 'NONE',  ( -12.14591786802326823, 12.06949235617739902, 48.12609039468568284 ) ) ;
#62051=CARTESIAN_POINT ( 'NONE',  ( -21.53943276465977519, 0.05219959533907696930, 46.24890960531435979 ) ) ;
#62052=CARTESIAN_POINT ( 'NONE',  ( -14.34966873604972548, 8.224510206698743886, 33.33442372801900433 ) ) ;
#62053=CARTESIAN_POINT ( 'NONE',  ( 19.02544592524343514, -5.153800228976328945, 33.54057627198102409 ) ) ;
#62054=CARTESIAN_POINT ( 'NONE',  ( -5.049401038297874678, -19.05341960407617918, 44.79275706135232582 ) ) ;
#62055=CARTESIAN_POINT ( 'NONE',  ( -0.05219959533909027116, -19.03943276465977164, 77.49890960531435269 ) ) ;
#62056=CARTESIAN_POINT ( 'NONE',  ( -19.03943276465977164, 0.05219959533909376836, 46.24890960531435979 ) ) ;
#62058=CARTESIAN_POINT ( 'NONE',  ( 5.049401038298161559, -19.05341960407611168, 72.70724293864768129 ) ) ;
#62060=CARTESIAN_POINT ( 'NONE',  ( -13.97604488694547697, 13.89961937509957934, 33.12609039468566863 ) ) ;
#62061=CARTESIAN_POINT ( 'NONE',  ( 10.81492255796106328, -18.62759615963255655, 105.4177570613523613 ) ) ;
#62062=CARTESIAN_POINT ( 'NONE',  ( -4.379528057220328563, 16.55341960407611168, 40.20724293864769550 ) ) ;
#62063=CARTESIAN_POINT ( 'NONE',  ( 9.474510206698971260, -16.51473224551069308, 37.91557627198102409 ) ) ;
#62064=CARTESIAN_POINT ( 'NONE',  ( -19.05341960407611168, -5.049401038298163336, 106.4572429386476955 ) ) ;
#62065=CARTESIAN_POINT ( 'NONE',  ( 10.81492255796106328, -18.62759615963255655, 85.41775706135236135 ) ) ;
#62066=CARTESIAN_POINT ( 'NONE',  ( 5.153800228976335163, 19.02544592524342804, 54.79057627198103120 ) ) ;
#62067=CARTESIAN_POINT ( 'NONE',  ( 21.55341960407619695, -5.719274019375665929, 86.04275706135236135 ) ) ;
#62068=CARTESIAN_POINT ( 'NONE',  ( 21.53943276465977519, -0.05219959533907433946, 43.74890960531435979 ) ) ;
#62069=CARTESIAN_POINT ( 'NONE',  ( 18.62759615963255655, 10.81492255796105972, 21.66775706135235069 ) ) ;
#62070=CARTESIAN_POINT ( 'NONE',  ( 16.51473224551083163, -9.474510206698727899, 50.83442372801899722 ) ) ;
#62071=CARTESIAN_POINT ( 'NONE',  ( -5.153800228976328057, -19.02544592524343514, 22.29057627198102765 ) ) ;
#62072=CARTESIAN_POINT ( 'NONE',  ( -0.05219959533909027116, -19.03943276465977164, 77.49890960531435269 ) ) ;
#62073=CARTESIAN_POINT ( 'NONE',  ( 12.14591786802327356, -12.06949235617739191, 35.62609039468568994 ) ) ;
#62074=CARTESIAN_POINT ( 'NONE',  ( 16.53943276465976808, -0.05219959533910856209, 93.74890960531436690 ) ) ;
#62075=CARTESIAN_POINT ( 'NONE',  ( -13.89961937509977652, 13.97604488694528158, 60.62390960531436690 ) ) ;
#62076=CARTESIAN_POINT ( 'NONE',  ( -21.52544592524343514, 5.823673210054127303, 41.04057627198103120 ) ) ;
#62077=CARTESIAN_POINT ( 'NONE',  ( -13.97604488694547697, 13.89961937509957934, 98.12609039468566152 ) ) ;
#62078=CARTESIAN_POINT ( 'NONE',  ( -21.52544592524343514, 5.823673210054127303, 101.0405762719810383 ) ) ;
#62079=CARTESIAN_POINT ( 'NONE',  ( 15.80617190586769283, -15.72974639402175789, 55.62609039468568284 ) ) ;
#62080=CARTESIAN_POINT ( 'NONE',  ( 16.52544592524335698, 4.483927247898782831, 61.45942372801901854 ) ) ;
#62081=CARTESIAN_POINT ( 'NONE',  ( -12.14591786802326823, 12.06949235617739902, 73.12609039468567573 ) ) ;
#62083=CARTESIAN_POINT ( 'NONE',  ( 13.89961937509977652, -13.97604488694527269, 58.12390960531436690 ) ) ;
#62084=CARTESIAN_POINT ( 'NONE',  ( 16.53943276465976808, 0.05219959533934440121, 91.25109039468568994 ) ) ;
#62086=CARTESIAN_POINT ( 'NONE',  ( 15.72974639402176855, 15.80617190586768217, 21.87609039468567573 ) ) ;
#62087=CARTESIAN_POINT ( 'NONE',  ( -16.52544592524342804, 4.483927247898546575, 66.04057627198103830 ) ) ;
#62088=CARTESIAN_POINT ( 'NONE',  ( -5.153800228976328057, -19.02544592524343514, 87.29057627198103830 ) ) ;
#62089=CARTESIAN_POINT ( 'NONE',  ( 16.52544592524335698, 4.483927247898782831, 81.45942372801900433 ) ) ;
#62090=CARTESIAN_POINT ( 'NONE',  ( -21.52544592524334988, -5.823673210054445271, 58.95942372801902565 ) ) ;
#62091=CARTESIAN_POINT ( 'NONE',  ( -5.049401038297874678, -19.05341960407617918, 109.7927570613523187 ) ) ;
#62092=CARTESIAN_POINT ( 'NONE',  ( -18.62759615963270932, 10.81492255796079327, 115.8322429386477097 ) ) ;
#62093=CARTESIAN_POINT ( 'NONE',  ( 4.379528057220339221, -16.55341960407611168, 52.70724293864769550 ) ) ;
#62095=CARTESIAN_POINT ( 'NONE',  ( 18.87075004821568314, -5.499999999999984013, 91.17408112101047379 ) ) ;
#62096=CARTESIAN_POINT ( 'NONE',  ( 18.62759615963271287, -10.81492255796078972, 83.33224293864769550 ) ) ;
#62097=CARTESIAN_POINT ( 'NONE',  ( 14.34966873604960469, 8.224510206698951720, 34.16557627198102409 ) ) ;
#62100=CARTESIAN_POINT ( 'NONE',  ( 21.55341960407610458, 5.719274019375980345, 113.9572429386477239 ) ) ;
#62101=CARTESIAN_POINT ( 'NONE',  ( 10.72451020669898902, -18.67979575497178502, 22.91557627198102765 ) ) ;
#62102=CARTESIAN_POINT ( 'NONE',  ( -5.823673210054431948, 21.52544592524334988, 27.70942372801901854 ) ) ;
#62103=CARTESIAN_POINT ( 'NONE',  ( -12.06949235617756955, 12.14591786802309770, 55.62390960531436690 ) ) ;
#62104=CARTESIAN_POINT ( 'NONE',  ( 8.224510206698742110, 14.34966873604972548, 62.08442372801901143 ) ) ;
#62105=CARTESIAN_POINT ( 'NONE',  ( -16.46253265017160317, 9.564922557960807481, 65.83224293864769550 ) ) ;
#62106=CARTESIAN_POINT ( 'NONE',  ( 9.474510206698729675, 16.51473224551082808, 72.08442372801900433 ) ) ;
#62107=CARTESIAN_POINT ( 'NONE',  ( -13.89961937509977652, 13.97604488694528158, 75.62390960531438111 ) ) ;
#62108=EDGE_CURVE ( 'NONE', #199703, #123077, #193433, .T. ) ;
#62109=CARTESIAN_POINT ( 'NONE',  ( 5.823673210054125526, 21.52544592524343514, 49.79057627198102409 ) ) ;
#62111=CARTESIAN_POINT ( 'NONE',  ( -19.03943276465977164, 0.05219959533909376836, 56.24890960531435979 ) ) ;
#62112=CARTESIAN_POINT ( 'NONE',  ( -12.06949235617739369, -12.14591786802326823, 29.37609039468568284 ) ) ;
#62113=CARTESIAN_POINT ( 'NONE',  ( 9.474510206698729675, 16.51473224551082808, 67.08442372801900433 ) ) ;
#62114=CARTESIAN_POINT ( 'NONE',  ( -21.52544592524343514, 5.823673210054127303, 111.0405762719810525 ) ) ;
#62115=CARTESIAN_POINT ( 'NONE',  ( -14.34966873604960291, -8.224510206698953496, 51.66557627198102409 ) ) ;
#62116=CARTESIAN_POINT ( 'NONE',  ( -0.05219959533909027116, -19.03943276465977164, 92.49890960531436690 ) ) ;
#62117=CARTESIAN_POINT ( 'NONE',  ( 18.62759615963271287, -10.81492255796078972, 58.33224293864768839 ) ) ;
#62118=CARTESIAN_POINT ( 'NONE',  ( -21.55341960407610458, -5.719274019375992779, 101.4572429386476955 ) ) ;
#62119=CARTESIAN_POINT ( 'NONE',  ( 14.34966873604972726, -8.224510206698740333, 40.83442372801901854 ) ) ;
#62120=CARTESIAN_POINT ( 'NONE',  ( -0.05219959533907301413, -21.53943276465977519, 37.49890960531436690 ) ) ;
#62121=CARTESIAN_POINT ( 'NONE',  ( -15.80617190586768217, 15.72974639402176855, 88.12609039468570415 ) ) ;
#62122=CARTESIAN_POINT ( 'NONE',  ( 13.97604488694527802, 13.89961937509977652, 89.37390960531436690 ) ) ;
#62123=CARTESIAN_POINT ( 'NONE',  ( -13.89961937509977652, 13.97604488694528158, 45.62390960531433848 ) ) ;
#62124=CARTESIAN_POINT ( 'NONE',  ( -19.05341960407611168, -5.049401038298163336, 91.45724293864766707 ) ) ;
#62125=CARTESIAN_POINT ( 'NONE',  ( -8.314922557960811034, -14.29746914071050412, 102.0822429386476955 ) ) ;
#62126=CARTESIAN_POINT ( 'NONE',  ( 16.51473224551069308, 9.474510206698969483, 59.16557627198102409 ) ) ;
#62127=CARTESIAN_POINT ( 'NONE',  ( -14.29746914071037622, -8.314922557961029526, 19.16775706135234714 ) ) ;
#62128=CARTESIAN_POINT ( 'NONE',  ( 17.49999999999999645, 5.068104630630414498, 31.77181594659973030 ) ) ;
#62129=CARTESIAN_POINT ( 'NONE',  ( -15.80617190586768217, 15.72974639402176855, 93.12609039468568994 ) ) ;
#62130=CARTESIAN_POINT ( 'NONE',  ( 10.72451020669898902, -18.67979575497178502, 37.91557627198102409 ) ) ;
#62131=CARTESIAN_POINT ( 'NONE',  ( -0.05219959533934338120, 16.53943276465976808, 87.50109039468568994 ) ) ;
#62133=CARTESIAN_POINT ( 'NONE',  ( 5.153800228976615827, -19.02544592524334988, 75.20942372801896170 ) ) ;
#62134=CARTESIAN_POINT ( 'NONE',  ( -19.03943276465977164, -0.05219959533935918106, 33.75109039468566863 ) ) ;
#62135=DIRECTION ( 'NONE',  ( -1.000000000000000000, 0.000000000000000000, 0.000000000000000000 ) ) ;
#62136=CARTESIAN_POINT ( 'NONE',  ( -16.46253265017160317, 9.564922557960807481, 25.83224293864769194 ) ) ;
#62137=CARTESIAN_POINT ( 'NONE',  ( -14.34966873604960291, -8.224510206698953496, 36.66557627198103120 ) ) ;
#62138=CARTESIAN_POINT ( 'NONE',  ( 16.51473224551069308, 9.474510206698969483, 24.16557627198102765 ) ) ;
#62139=CARTESIAN_POINT ( 'NONE',  ( -14.34966873604960291, -8.224510206698953496, 21.66557627198102409 ) ) ;
#62140=CARTESIAN_POINT ( 'NONE',  ( -18.89770734986045753, -5.500000000000000888, 84.10214472496637939 ) ) ;
#62141=CARTESIAN_POINT ( 'NONE',  ( 14.29746914071037800, 8.314922557961029526, 91.66775706135234714 ) ) ;
#62142=CARTESIAN_POINT ( 'NONE',  ( -13.89961937509977652, 13.97604488694528158, 30.62390960531435269 ) ) ;
#62143=CARTESIAN_POINT ( 'NONE',  ( 5.719274019375673035, 21.55341960407619339, 112.2927570613523471 ) ) ;
#62144=CARTESIAN_POINT ( 'NONE',  ( -4.379528057220086978, -16.55341960407618274, 19.79275706135235069 ) ) ;
#62145=CARTESIAN_POINT ( 'NONE',  ( -5.823673210054431948, 21.52544592524334988, 72.70942372801901854 ) ) ;
#62146=CARTESIAN_POINT ( 'NONE',  ( 13.89961937509957401, 13.97604488694547697, 51.87609039468566863 ) ) ;
#62147=CARTESIAN_POINT ( 'NONE',  ( -5.049401038298153566, 19.05341960407611168, 95.20724293864770971 ) ) ;
#62148=CARTESIAN_POINT ( 'NONE',  ( 0.05219959533909260263, 19.03943276465977164, 69.99890960531435269 ) ) ;
#62149=CARTESIAN_POINT ( 'NONE',  ( -19.49149378614658090, 5.499999999999783284, 39.43757513605363840 ) ) ;
#62150=CARTESIAN_POINT ( 'NONE',  ( -10.72451020669898014, 18.67979575497178502, 100.4155762719810241 ) ) ;
#62151=CARTESIAN_POINT ( 'NONE',  ( -14.29746914071049879, 8.314922557960819915, 60.83224293864769550 ) ) ;
#62152=CARTESIAN_POINT ( 'NONE',  ( 5.823673210054125526, 21.52544592524343514, 54.79057627198104541 ) ) ;
#62153=CARTESIAN_POINT ( 'NONE',  ( 16.46253265017160672, -9.564922557960803928, 58.33224293864769550 ) ) ;
#62154=CARTESIAN_POINT ( 'NONE',  ( 21.55341960407610458, 5.719274019375980345, 88.95724293864769550 ) ) ;
#62155=CARTESIAN_POINT ( 'NONE',  ( 8.314922557961029526, -14.29746914071037800, 75.41775706135233293 ) ) ;
#62157=CARTESIAN_POINT ( 'NONE',  ( 5.049401038298161559, -19.05341960407611168, 42.70724293864767418 ) ) ;
#62158=CARTESIAN_POINT ( 'NONE',  ( -14.34966873604960291, -8.224510206698953496, 96.66557627198102409 ) ) ;
#62160=CARTESIAN_POINT ( 'NONE',  ( -19.05341960407611168, -5.049401038298163336, 51.45724293864770260 ) ) ;
#62161=CARTESIAN_POINT ( 'NONE',  ( -5.049401038298153566, 19.05341960407611168, 25.20724293864768484 ) ) ;
#62162=CARTESIAN_POINT ( 'NONE',  ( 19.02544592524334988, 5.153800228976608722, 61.45942372801900433 ) ) ;
#62163=CARTESIAN_POINT ( 'NONE',  ( -16.55341960407611168, -4.379528057220339221, 86.45724293864770971 ) ) ;
#62164=CARTESIAN_POINT ( 'NONE',  ( 0.05219959533937995610, -21.53943276465977519, 45.00109039468568284 ) ) ;
#62165=CARTESIAN_POINT ( 'NONE',  ( 13.97604488694527802, 13.89961937509977652, 39.37390960531435269 ) ) ;
#62166=CARTESIAN_POINT ( 'NONE',  ( -0.05219959533907301413, -21.53943276465977519, 107.4989096053143669 ) ) ;
#62167=CARTESIAN_POINT ( 'NONE',  ( -16.53943276465976808, 0.05219959533911058130, 91.24890960531436690 ) ) ;
#62169=CARTESIAN_POINT ( 'NONE',  ( 5.153800228976335163, 19.02544592524342804, 64.79057627198100988 ) ) ;
#62171=CARTESIAN_POINT ( 'NONE',  ( 16.51473224551083163, -9.474510206698727899, 95.83442372801900433 ) ) ;
#62172=CARTESIAN_POINT ( 'NONE',  ( -19.03943276465977164, 0.05219959533909376836, 101.2489096053143669 ) ) ;
#62173=CARTESIAN_POINT ( 'NONE',  ( 21.52544592524334988, 5.823673210054432836, 36.45942372801901143 ) ) ;
#62174=CARTESIAN_POINT ( 'NONE',  ( 9.564922557960805705, 16.46253265017160317, 79.58224293864769550 ) ) ;
#62175=CARTESIAN_POINT ( 'NONE',  ( -9.564922557961040184, 16.46253265017147172, 72.91775706135233293 ) ) ;
#62176=CARTESIAN_POINT ( 'NONE',  ( 9.474510206698971260, -16.51473224551069308, 52.91557627198102409 ) ) ;
#62177=CARTESIAN_POINT ( 'NONE',  ( -16.52544592524342804, 4.483927247898546575, 76.04057627198102409 ) ) ;
#62178=CARTESIAN_POINT ( 'NONE',  ( -8.224510206698948167, 14.34966873604960824, 65.41557627198102409 ) ) ;
#62179=CARTESIAN_POINT ( 'NONE',  ( 9.564922557960805705, 16.46253265017160317, 89.58224293864769550 ) ) ;
#62180=CARTESIAN_POINT ( 'NONE',  ( -21.55341960407610458, -5.719274019375992779, 106.4572429386477097 ) ) ;
#62181=CARTESIAN_POINT ( 'NONE',  ( -16.46253265017160317, 9.564922557960807481, 80.83224293864769550 ) ) ;
#62182=CARTESIAN_POINT ( 'NONE',  ( 9.474510206698729675, 16.51473224551082808, 27.08442372801900433 ) ) ;
#62183=CARTESIAN_POINT ( 'NONE',  ( 9.564922557960805705, 16.46253265017160317, 34.58224293864770260 ) ) ;
#62184=CARTESIAN_POINT ( 'NONE',  ( 14.29746914071049879, -8.314922557960816363, 28.33224293864769550 ) ) ;
#62185=CARTESIAN_POINT ( 'NONE',  ( 16.53943276465976808, -0.05219959533910856209, 103.7489096053143669 ) ) ;
#62186=CARTESIAN_POINT ( 'NONE',  ( -16.46253265017146816, -9.564922557961047289, 99.16775706135233293 ) ) ;
#62187=EDGE_LOOP ( 'NONE', ( #71840, #180312, #45826, #113191, #148805, #131599, #73755, #119356 ) ) ;
#62188=CARTESIAN_POINT ( 'NONE',  ( -21.52544592524334988, -5.823673210054445271, 28.95942372801902209 ) ) ;
#62189=CARTESIAN_POINT ( 'NONE',  ( 9.564922557961047289, -16.46253265017146816, 70.41775706135233293 ) ) ;
#62190=CARTESIAN_POINT ( 'NONE',  ( -14.29746914071049879, 8.314922557960819915, 25.83224293864769194 ) ) ;
#62191=CARTESIAN_POINT ( 'NONE',  ( 5.719274019375991003, -21.55341960407610458, 82.70724293864770971 ) ) ;
#62192=CARTESIAN_POINT ( 'NONE',  ( 21.53943276465977519, -0.05219959533907433946, 23.74890960531435269 ) ) ;
#62193=CARTESIAN_POINT ( 'NONE',  ( -16.52544592524342804, 4.483927247898546575, 76.04057627198102409 ) ) ;
#62194=CARTESIAN_POINT ( 'NONE',  ( 19.03943276465977164, -0.05219959533909143690, 23.74890960531435269 ) ) ;
#62195=CARTESIAN_POINT ( 'NONE',  ( 19.03943276465977164, 0.05219959533936151252, 31.25109039468566863 ) ) ;
#62196=CARTESIAN_POINT ( 'NONE',  ( 8.224510206698742110, 14.34966873604972548, 92.08442372801901854 ) ) ;
#62197=CARTESIAN_POINT ( 'NONE',  ( -16.55341960407617563, 4.379528057220093196, 63.54275706135234003 ) ) ;
#62198=CARTESIAN_POINT ( 'NONE',  ( 19.05341960407611168, 5.049401038298154454, 113.9572429386477097 ) ) ;
#62199=CARTESIAN_POINT ( 'NONE',  ( 21.53943276465977519, 0.05219959533937863772, 111.2510903946856899 ) ) ;
#62200=CARTESIAN_POINT ( 'NONE',  ( 9.474510206698971260, -16.51473224551069308, 77.91557627198103830 ) ) ;
#62201=CARTESIAN_POINT ( 'NONE',  ( -4.379528057220086978, -16.55341960407618274, 59.79275706135234714 ) ) ;
#62202=CARTESIAN_POINT ( 'NONE',  ( -5.049401038298153566, 19.05341960407611168, 25.20724293864768484 ) ) ;
#62203=CARTESIAN_POINT ( 'NONE',  ( 12.14591786802309770, 12.06949235617756955, 29.37390960531435269 ) ) ;
#62205=CARTESIAN_POINT ( 'NONE',  ( 19.02544592524343514, -5.153800228976328945, 103.5405762719809957 ) ) ;
#62206=CARTESIAN_POINT ( 'NONE',  ( -16.51473224551069308, -9.474510206698971260, 81.66557627198103830 ) ) ;
#62207=CARTESIAN_POINT ( 'NONE',  ( -19.02544592524342804, 5.153800228976336051, 111.0405762719810099 ) ) ;
#62208=CARTESIAN_POINT ( 'NONE',  ( -12.14591786802309592, -12.06949235617757132, 56.87390960531436690 ) ) ;
#62209=CARTESIAN_POINT ( 'NONE',  ( 14.34966873604960469, 8.224510206698951720, 34.16557627198102409 ) ) ;
#62210=CARTESIAN_POINT ( 'NONE',  ( 16.52544592524342804, -4.483927247898539470, 53.54057627198103120 ) ) ;
#62211=CARTESIAN_POINT ( 'NONE',  ( -12.06949235617739369, -12.14591786802326823, 44.37609039468567573 ) ) ;
#62212=CARTESIAN_POINT ( 'NONE',  ( 19.03943276465977164, 0.05219959533936151252, 46.25109039468566863 ) ) ;
#62213=CARTESIAN_POINT ( 'NONE',  ( -19.05341960407611168, -5.049401038298163336, 76.45724293864769550 ) ) ;
#62214=CARTESIAN_POINT ( 'NONE',  ( 13.97604488694548053, -13.89961937509957401, 50.62609039468566152 ) ) ;
#62216=CARTESIAN_POINT ( 'NONE',  ( 5.049401038297881783, 19.05341960407617563, 57.29275706135231871 ) ) ;
#62217=CARTESIAN_POINT ( 'NONE',  ( -16.51473224551082808, 9.474510206698731452, 98.33442372801900433 ) ) ;
#62218=CARTESIAN_POINT ( 'NONE',  ( 16.52544592524335698, 4.483927247898782831, 81.45942372801900433 ) ) ;
#62220=CARTESIAN_POINT ( 'NONE',  ( -9.564922557960796823, -16.46253265017161027, 27.08224293864769550 ) ) ;
#62221=CARTESIAN_POINT ( 'NONE',  ( 5.049401038298161559, -19.05341960407611168, 97.70724293864766707 ) ) ;
#62222=CARTESIAN_POINT ( 'NONE',  ( -18.62759615963255300, -10.81492255796106328, 44.16775706135234714 ) ) ;
#62223=CARTESIAN_POINT ( 'NONE',  ( -19.03943276465977164, -0.05219959533935918106, 98.75109039468567573 ) ) ;
#62225=CARTESIAN_POINT ( 'NONE',  ( 19.05341960407611168, 5.049401038298154454, 63.95724293864769550 ) ) ;
#62226=CARTESIAN_POINT ( 'NONE',  ( 13.97604488694527802, 13.89961937509977652, 104.3739096053143385 ) ) ;
#62227=CARTESIAN_POINT ( 'NONE',  ( 8.314922557960818139, 14.29746914071049879, 64.58224293864769550 ) ) ;
#62228=CARTESIAN_POINT ( 'NONE',  ( -0.05219959533909027116, -19.03943276465977164, 67.49890960531436690 ) ) ;
#62229=CARTESIAN_POINT ( 'NONE',  ( 9.474510206698971260, -16.51473224551069308, 57.91557627198103120 ) ) ;
#62230=CARTESIAN_POINT ( 'NONE',  ( -19.05341960407617563, 5.049401038297882671, 83.54275706135233293 ) ) ;
#62231=CARTESIAN_POINT ( 'NONE',  ( -5.719274019375978568, 21.55341960407610458, 45.20724293864769550 ) ) ;
#62232=CARTESIAN_POINT ( 'NONE',  ( -9.564922557961040184, 16.46253265017147172, 47.91775706135233293 ) ) ;
#62233=CARTESIAN_POINT ( 'NONE',  ( -19.02544592524342804, 5.153800228976336051, 76.04057627198102409 ) ) ;
#62234=CARTESIAN_POINT ( 'NONE',  ( 18.62759615963271287, -10.81492255796078972, 83.33224293864769550 ) ) ;
#62235=CARTESIAN_POINT ( 'NONE',  ( -0.05219959533910754901, -16.53943276465976808, 82.49890960531436690 ) ) ;
#62236=CARTESIAN_POINT ( 'NONE',  ( 16.46253265017146816, 9.564922557961045513, 36.66775706135233293 ) ) ;
#62237=CARTESIAN_POINT ( 'NONE',  ( 5.823673210054125526, 21.52544592524343514, 54.79057627198104541 ) ) ;
#62238=CARTESIAN_POINT ( 'NONE',  ( 18.67979575497178502, 10.72451020669898547, 44.16557627198103120 ) ) ;
#62239=CARTESIAN_POINT ( 'NONE',  ( -19.02544592524342804, 5.153800228976336051, 66.04057627198103830 ) ) ;
#62240=CARTESIAN_POINT ( 'NONE',  ( 16.52544592524342804, -4.483927247898539470, 108.5405762719810241 ) ) ;
#62241=CARTESIAN_POINT ( 'NONE',  ( -5.823673210054431948, 21.52544592524334988, 27.70942372801901854 ) ) ;
#62243=CARTESIAN_POINT ( 'NONE',  ( 0.05219959533937995610, -21.53943276465977519, 45.00109039468568284 ) ) ;
#62244=CARTESIAN_POINT ( 'NONE',  ( 13.89961937509977652, -13.97604488694527269, 38.12390960531436690 ) ) ;
#62245=CARTESIAN_POINT ( 'NONE',  ( -18.62759615963270932, 10.81492255796079327, 100.8322429386477097 ) ) ;
#62246=CARTESIAN_POINT ( 'NONE',  ( -19.05341960407617563, 5.049401038297882671, 53.54275706135231871 ) ) ;
#62247=CARTESIAN_POINT ( 'NONE',  ( 5.049401038298161559, -19.05341960407611168, 27.70724293864769550 ) ) ;
#62248=CARTESIAN_POINT ( 'NONE',  ( 16.51473224551069308, 9.474510206698969483, 24.16557627198102765 ) ) ;
#62250=CARTESIAN_POINT ( 'NONE',  ( 4.483927247898790824, -16.52544592524335698, 60.20942372801902565 ) ) ;
#62251=CARTESIAN_POINT ( 'NONE',  ( -19.05341960407611168, -5.049401038298163336, 21.45724293864768839 ) ) ;
#62253=CARTESIAN_POINT ( 'NONE',  ( 16.51473224551069308, 9.474510206698969483, 69.16557627198102409 ) ) ;
#62254=CARTESIAN_POINT ( 'NONE',  ( -4.483927247898539470, -16.52544592524342804, 102.2905762719810383 ) ) ;
#62257=CARTESIAN_POINT ( 'NONE',  ( -5.719274019375978568, 21.55341960407610458, 65.20724293864768129 ) ) ;
#62258=CARTESIAN_POINT ( 'NONE',  ( 0.05219959533934541429, -16.53943276465976808, 35.00109039468568284 ) ) ;
#62259=CARTESIAN_POINT ( 'NONE',  ( 15.80617190586769283, -15.72974639402175789, 105.6260903946856899 ) ) ;
#62260=CARTESIAN_POINT ( 'NONE',  ( -9.474510206698964154, 16.51473224551069663, 25.41557627198103120 ) ) ;
#62261=CARTESIAN_POINT ( 'NONE',  ( 16.52544592524342804, -4.483927247898539470, 23.54057627198102765 ) ) ;
#62262=CARTESIAN_POINT ( 'NONE',  ( 16.52544592524342804, -4.483927247898539470, 48.54057627198103120 ) ) ;
#62263=CARTESIAN_POINT ( 'NONE',  ( 5.153800228976335163, 19.02544592524342804, 49.79057627198100988 ) ) ;
#62264=CARTESIAN_POINT ( 'NONE',  ( 18.67979575497194134, -10.72451020669871369, 95.83442372801903275 ) ) ;
#62265=CARTESIAN_POINT ( 'NONE',  ( 10.72451020669898902, -18.67979575497178502, 112.9155762719810383 ) ) ;
#62266=CARTESIAN_POINT ( 'NONE',  ( 15.72974639402176855, 15.80617190586768217, 76.87609039468567573 ) ) ;
#62267=CARTESIAN_POINT ( 'NONE',  ( -16.55341960407617563, 4.379528057220093196, 53.54275706135234714 ) ) ;
#62268=CARTESIAN_POINT ( 'NONE',  ( -0.05219959533910754901, -16.53943276465976808, 82.49890960531436690 ) ) ;
#62269=CARTESIAN_POINT ( 'NONE',  ( 10.72451020669871369, 18.67979575497193778, 102.0844237280190185 ) ) ;
#62270=CARTESIAN_POINT ( 'NONE',  ( 16.55341960407618274, -4.379528057220086978, 111.0427570613523613 ) ) ;
#62271=CARTESIAN_POINT ( 'NONE',  ( -16.62475595723700295, 7.163666690055284114, 115.5271335181047760 ) ) ;
#62272=CARTESIAN_POINT ( 'NONE',  ( -14.34966873604972548, 8.224510206698743886, 33.33442372801900433 ) ) ;
#62273=CARTESIAN_POINT ( 'NONE',  ( 4.379528057220339221, -16.55341960407611168, 37.70724293864769550 ) ) ;
#62274=CARTESIAN_POINT ( 'NONE',  ( 14.34966873604972726, -8.224510206698740333, 80.83442372801901854 ) ) ;
#62275=CARTESIAN_POINT ( 'NONE',  ( 16.51473224551069308, 9.474510206698969483, 94.16557627198103830 ) ) ;
#62276=CARTESIAN_POINT ( 'NONE',  ( 13.97604488694527802, 13.89961937509977652, 109.3739096053143669 ) ) ;
#62277=CARTESIAN_POINT ( 'NONE',  ( -15.80617190586768217, 15.72974639402176855, 93.12609039468568994 ) ) ;
#62278=CARTESIAN_POINT ( 'NONE',  ( -4.379528057220086978, -16.55341960407618274, 104.7927570613523898 ) ) ;
#62279=CARTESIAN_POINT ( 'NONE',  ( 0.05219959533910956823, 16.53943276465976808, 69.99890960531435269 ) ) ;
#62280=CARTESIAN_POINT ( 'NONE',  ( -9.564922557960796823, -16.46253265017161027, 77.08224293864769550 ) ) ;
#62281=VERTEX_POINT ( 'NONE', #123363 ) ;
#62282=CARTESIAN_POINT ( 'NONE',  ( 16.55341960407618274, -4.379528057220086978, 31.04275706135234714 ) ) ;
#62283=CARTESIAN_POINT ( 'NONE',  ( -13.89961937509977652, 13.97604488694528158, 25.62390960531434558 ) ) ;
#62284=CARTESIAN_POINT ( 'NONE',  ( 5.049401038298161559, -19.05341960407611168, 87.70724293864769550 ) ) ;
#62285=CARTESIAN_POINT ( 'NONE',  ( -4.483927247898782831, 16.52544592524335698, 37.70942372801900433 ) ) ;
#62287=CARTESIAN_POINT ( 'NONE',  ( 16.46253265017146816, 9.564922557961045513, 36.66775706135233293 ) ) ;
#62288=CARTESIAN_POINT ( 'NONE',  ( -16.55341960407617563, 4.379528057220093196, 88.54275706135236135 ) ) ;
#62289=CARTESIAN_POINT ( 'NONE',  ( -19.02544592524342804, 5.153800228976336051, 31.04057627198102409 ) ) ;
#62291=CARTESIAN_POINT ( 'NONE',  ( -16.52544592524335698, -4.483927247898792601, 73.95942372801901854 ) ) ;
#62292=CARTESIAN_POINT ( 'NONE',  ( 12.06949235617739724, 12.14591786802326823, 66.87609039468568994 ) ) ;
#62293=CARTESIAN_POINT ( 'NONE',  ( -13.97604488694547697, 13.89961937509957934, 83.12609039468564731 ) ) ;
#62294=CARTESIAN_POINT ( 'NONE',  ( 9.474510206698729675, 16.51473224551082808, 32.08442372801900433 ) ) ;
#62295=CARTESIAN_POINT ( 'NONE',  ( -9.564922557960796823, -16.46253265017161027, 47.08224293864769550 ) ) ;
#62296=CARTESIAN_POINT ( 'NONE',  ( 0.05219959533910956823, 16.53943276465976808, 84.99890960531436690 ) ) ;
#62297=CARTESIAN_POINT ( 'NONE',  ( 16.51473224551083163, -9.474510206698727899, 55.83442372801899722 ) ) ;
#62298=CARTESIAN_POINT ( 'NONE',  ( -10.72451020669898014, 18.67979575497178502, 45.41557627198103830 ) ) ;
#62299=CARTESIAN_POINT ( 'NONE',  ( -5.153800228976607833, 19.02544592524334988, 32.70942372801899722 ) ) ;
#62300=CARTESIAN_POINT ( 'NONE',  ( -16.51473224551069308, -9.474510206698971260, 101.6655762719810241 ) ) ;
#62301=CARTESIAN_POINT ( 'NONE',  ( -5.719274019375978568, 21.55341960407610458, 75.20724293864769550 ) ) ;
#62302=CARTESIAN_POINT ( 'NONE',  ( 19.03943276465977164, -0.05219959533909143690, 113.7489096053143669 ) ) ;
#62303=CARTESIAN_POINT ( 'NONE',  ( 16.51473224551083163, -9.474510206698727899, 90.83442372801900433 ) ) ;
#62304=CARTESIAN_POINT ( 'NONE',  ( 9.564922557960805705, 16.46253265017160317, 114.5822429386476955 ) ) ;
#62305=CARTESIAN_POINT ( 'NONE',  ( 5.153800228976615827, -19.02544592524334988, 110.2094237280189901 ) ) ;
#62306=CARTESIAN_POINT ( 'NONE',  ( 0.05219959533909260263, 19.03943276465977164, 34.99890960531435979 ) ) ;
#62307=CARTESIAN_POINT ( 'NONE',  ( -13.97604488694527625, -13.89961937509977652, 91.87390960531432427 ) ) ;
#62308=CARTESIAN_POINT ( 'NONE',  ( -21.55341960407610458, -5.719274019375992779, 71.45724293864769550 ) ) ;
#62309=CARTESIAN_POINT ( 'NONE',  ( -0.05219959533934338120, 16.53943276465976808, 52.50109039468567573 ) ) ;
#62310=CARTESIAN_POINT ( 'NONE',  ( 15.72974639402176855, 15.80617190586768217, 41.87609039468568284 ) ) ;
#62311=CARTESIAN_POINT ( 'NONE',  ( -5.153800228976607833, 19.02544592524334988, 87.70942372801897591 ) ) ;
#62312=CARTESIAN_POINT ( 'NONE',  ( 0.05219959533937995610, -21.53943276465977519, 95.00109039468568994 ) ) ;
#62313=CARTESIAN_POINT ( 'NONE',  ( 14.34966873604972726, -8.224510206698740333, 105.8344237280190328 ) ) ;
#62314=CARTESIAN_POINT ( 'NONE',  ( 19.03943276465977164, -0.05219959533909143690, 103.7489096053143669 ) ) ;
#62315=CARTESIAN_POINT ( 'NONE',  ( 12.14591786802309770, 12.06949235617756955, 94.37390960531436690 ) ) ;
#62316=CARTESIAN_POINT ( 'NONE',  ( 14.29746914071049879, -8.314922557960816363, 38.33224293864768839 ) ) ;
#62317=CARTESIAN_POINT ( 'NONE',  ( 5.049401038297881783, 19.05341960407617563, 82.29275706135229029 ) ) ;
#62318=CARTESIAN_POINT ( 'NONE',  ( 18.62759615963255655, 10.81492255796105972, 61.66775706135235424 ) ) ;
#62319=CARTESIAN_POINT ( 'NONE',  ( -5.153800228976607833, 19.02544592524334988, 32.70942372801899722 ) ) ;
#62320=CARTESIAN_POINT ( 'NONE',  ( -12.06949235617756955, 12.14591786802309770, 105.6239096053143669 ) ) ;
#62321=CARTESIAN_POINT ( 'NONE',  ( 18.67979575497178502, 10.72451020669898547, 34.16557627198102409 ) ) ;
#62322=CARTESIAN_POINT ( 'NONE',  ( 14.34966873604960469, 8.224510206698951720, 24.16557627198103120 ) ) ;
#62323=CARTESIAN_POINT ( 'NONE',  ( -18.62759615963255300, -10.81492255796106328, 99.16775706135234714 ) ) ;
#62324=CARTESIAN_POINT ( 'NONE',  ( 12.06949235617739724, 12.14591786802326823, 61.87609039468568284 ) ) ;
#62325=CARTESIAN_POINT ( 'NONE',  ( -12.14591786802309592, -12.06949235617757132, 26.87390960531435979 ) ) ;
#62326=CARTESIAN_POINT ( 'NONE',  ( 5.719274019375673035, 21.55341960407619339, 67.29275706135234714 ) ) ;
#62327=CARTESIAN_POINT ( 'NONE',  ( -15.72974639402176322, -15.80617190586768395, 49.37609039468569705 ) ) ;
#62329=CARTESIAN_POINT ( 'NONE',  ( -18.22780087662121673, -5.500000000000062172, 61.48459894673894155 ) ) ;
#62330=CARTESIAN_POINT ( 'NONE',  ( 15.80617190586769283, -15.72974639402175789, 25.62609039468567929 ) ) ;
#62331=CARTESIAN_POINT ( 'NONE',  ( -16.55341960407611168, -4.379528057220339221, 101.4572429386476955 ) ) ;
#62332=CARTESIAN_POINT ( 'NONE',  ( 0.05219959533909260263, 19.03943276465977164, 29.99890960531435979 ) ) ;
#62333=CARTESIAN_POINT ( 'NONE',  ( -16.55341960407611168, -4.379528057220339221, 81.45724293864769550 ) ) ;
#62334=CARTESIAN_POINT ( 'NONE',  ( 5.049401038298161559, -19.05341960407611168, 67.70724293864769550 ) ) ;
#62335=CARTESIAN_POINT ( 'NONE',  ( -16.52544592524342804, 4.483927247898546575, 26.04057627198103475 ) ) ;
#62336=CARTESIAN_POINT ( 'NONE',  ( -21.55341960407610458, -5.719274019375992779, 51.45724293864770260 ) ) ;
#62337=CARTESIAN_POINT ( 'NONE',  ( -14.29746914071049879, 8.314922557960819915, 95.83224293864770971 ) ) ;
#62338=CARTESIAN_POINT ( 'NONE',  ( -18.62759615963270932, 10.81492255796079327, 90.83224293864769550 ) ) ;
#62339=CARTESIAN_POINT ( 'NONE',  ( -16.51473224551069308, -9.474510206698971260, 106.6655762719810383 ) ) ;
#62340=CARTESIAN_POINT ( 'NONE',  ( -19.02544592524342804, 5.153800228976336051, 56.04057627198100988 ) ) ;
#62341=CARTESIAN_POINT ( 'NONE',  ( 13.89961937509957401, 13.97604488694547697, 101.8760903946856331 ) ) ;
#62342=EDGE_CURVE ( 'NONE', #50977, #122302, #88100, .T. ) ;
#62343=CARTESIAN_POINT ( 'NONE',  ( -18.67979575497178146, -10.72451020669898902, 46.66557627198102409 ) ) ;
#62344=CARTESIAN_POINT ( 'NONE',  ( 21.53943276465977519, 0.05219959533937863772, 81.25109039468568994 ) ) ;
#62345=CARTESIAN_POINT ( 'NONE',  ( 19.03943276465977164, -0.05219959533909143690, 63.74890960531435979 ) ) ;
#62346=CARTESIAN_POINT ( 'NONE',  ( -0.05219959533909027116, -19.03943276465977164, 97.49890960531436690 ) ) ;
#62347=CARTESIAN_POINT ( 'NONE',  ( 16.53943276465976808, 0.05219959533934440121, 76.25109039468568994 ) ) ;
#62348=CARTESIAN_POINT ( 'NONE',  ( -15.80617190586768217, 15.72974639402176855, 58.12609039468568994 ) ) ;
#62349=CARTESIAN_POINT ( 'NONE',  ( -15.80617190586768217, 15.72974639402176855, 93.12609039468568994 ) ) ;
#62350=CARTESIAN_POINT ( 'NONE',  ( -21.52544592524343514, 5.823673210054127303, 106.0405762719810525 ) ) ;
#62351=CARTESIAN_POINT ( 'NONE',  ( 15.80617190586769283, -15.72974639402175789, 40.62609039468567573 ) ) ;
#62352=CARTESIAN_POINT ( 'NONE',  ( 16.53943276465976808, 0.05219959533934440121, 76.25109039468568994 ) ) ;
#62353=CARTESIAN_POINT ( 'NONE',  ( -15.72974639402197994, 15.80617190586746368, 75.62390960531439532 ) ) ;
#62354=CARTESIAN_POINT ( 'NONE',  ( 0.05219959533936267826, -19.03943276465977164, 30.00109039468566863 ) ) ;
#62355=CARTESIAN_POINT ( 'NONE',  ( 18.67979575497178502, 10.72451020669898547, 39.16557627198102409 ) ) ;
#62356=CARTESIAN_POINT ( 'NONE',  ( -5.153800228976328057, -19.02544592524343514, 87.29057627198103830 ) ) ;
#62357=CARTESIAN_POINT ( 'NONE',  ( -4.483927247898539470, -16.52544592524342804, 22.29057627198102765 ) ) ;
#62358=CARTESIAN_POINT ( 'NONE',  ( -16.21995358207306737, 7.366697692864093483, 64.93551001512160781 ) ) ;
#62359=CARTESIAN_POINT ( 'NONE',  ( 13.89961937509977652, -13.97604488694527269, 108.1239096053143669 ) ) ;
#62361=CARTESIAN_POINT ( 'NONE',  ( 17.97058386085786097, 5.500000000000042633, 81.50390968646220813 ) ) ;
#62362=CARTESIAN_POINT ( 'NONE',  ( 19.05341960407617918, -5.049401038297876454, 101.0427570613523045 ) ) ;
#62363=CARTESIAN_POINT ( 'NONE',  ( 21.55341960407610458, 5.719274019375980345, 73.95724293864769550 ) ) ;
#62364=CARTESIAN_POINT ( 'NONE',  ( 16.55341960407611168, 4.379528057220329451, 43.95724293864769550 ) ) ;
#62365=CARTESIAN_POINT ( 'NONE',  ( -0.05219959533934338120, 16.53943276465976808, 22.50109039468567573 ) ) ;
#62366=CARTESIAN_POINT ( 'NONE',  ( -9.564922557960796823, -16.46253265017161027, 32.08224293864769550 ) ) ;
#62367=CARTESIAN_POINT ( 'NONE',  ( -14.29746914071037622, -8.314922557961029526, 19.16775706135234714 ) ) ;
#62368=CARTESIAN_POINT ( 'NONE',  ( -21.55341960407610458, -5.719274019375992779, 96.45724293864770971 ) ) ;
#62369=CARTESIAN_POINT ( 'NONE',  ( -19.05341960407617563, 5.049401038297882671, 68.54275706135230450 ) ) ;
#62370=CARTESIAN_POINT ( 'NONE',  ( -16.53943276465976808, -0.05219959533934237506, 73.75109039468567573 ) ) ;
#62371=CARTESIAN_POINT ( 'NONE',  ( -16.51473224551069308, -9.474510206698971260, 66.66557627198102409 ) ) ;
#62372=CARTESIAN_POINT ( 'NONE',  ( 16.52544592524342804, -4.483927247898539470, 73.54057627198102409 ) ) ;
#62373=CARTESIAN_POINT ( 'NONE',  ( -16.51473224551069308, -9.474510206698971260, 61.66557627198103120 ) ) ;
#62374=CARTESIAN_POINT ( 'NONE',  ( 16.53943276465976808, -0.05219959533910856209, 68.74890960531435269 ) ) ;
#62375=CARTESIAN_POINT ( 'NONE',  ( -0.05219959533909027116, -19.03943276465977164, 37.49890960531436690 ) ) ;
#62377=CARTESIAN_POINT ( 'NONE',  ( 8.224510206698953496, -14.34966873604960469, 42.91557627198103120 ) ) ;
#62378=CARTESIAN_POINT ( 'NONE',  ( 9.474510206698971260, -16.51473224551069308, 72.91557627198102409 ) ) ;
#62380=CARTESIAN_POINT ( 'NONE',  ( -19.03943276465977164, -0.05219959533935918106, 53.75109039468566863 ) ) ;
#62381=CARTESIAN_POINT ( 'NONE',  ( -8.224510206698735004, -14.34966873604973081, 59.58442372801901854 ) ) ;
#62382=CARTESIAN_POINT ( 'NONE',  ( 15.80617190586746368, 15.72974639402197994, 64.37390960531435269 ) ) ;
#62383=CARTESIAN_POINT ( 'NONE',  ( -0.05219959533936034679, 19.03943276465977164, 22.50109039468566152 ) ) ;
#62384=CARTESIAN_POINT ( 'NONE',  ( 5.049401038298161559, -19.05341960407611168, 87.70724293864769550 ) ) ;
#62386=CARTESIAN_POINT ( 'NONE',  ( 21.53943276465977519, -0.05219959533907433946, 23.74890960531435269 ) ) ;
#62387=CARTESIAN_POINT ( 'NONE',  ( -9.564922557960796823, -16.46253265017161027, 62.08224293864769550 ) ) ;
#62388=CARTESIAN_POINT ( 'NONE',  ( -15.80617190586768217, 15.72974639402176855, 53.12609039468568284 ) ) ;
#62389=CARTESIAN_POINT ( 'NONE',  ( -12.06949235617756955, 12.14591786802309770, 105.6239096053143669 ) ) ;
#62390=CARTESIAN_POINT ( 'NONE',  ( -21.53943276465977519, 0.05219959533907696930, 106.2489096053143811 ) ) ;
#62391=CARTESIAN_POINT ( 'NONE',  ( 0.05219959533909260263, 19.03943276465977164, 94.99890960531436690 ) ) ;
#62392=ORIENTED_EDGE ( 'NONE', *, *, #157116, .F. ) ;
#62393=CARTESIAN_POINT ( 'NONE',  ( -10.72451020669870658, -18.67979575497194134, 39.58442372801901143 ) ) ;
#62394=ORIENTED_EDGE ( 'NONE', *, *, #188637, .T. ) ;
#62395=CARTESIAN_POINT ( 'NONE',  ( -0.05219959533909027116, -19.03943276465977164, 87.49890960531436690 ) ) ;
#62397=CARTESIAN_POINT ( 'NONE',  ( 19.02130022317636460, -5.499999999999792166, 83.28188669246573284 ) ) ;
#62398=CARTESIAN_POINT ( 'NONE',  ( 10.72451020669898902, -18.67979575497178502, 87.91557627198103830 ) ) ;
#62399=CARTESIAN_POINT ( 'NONE',  ( -16.46253265017160317, 9.564922557960807481, 50.83224293864770260 ) ) ;
#62400=CARTESIAN_POINT ( 'NONE',  ( -16.55341960407617563, 4.379528057220093196, 28.54275706135234358 ) ) ;
#62402=CARTESIAN_POINT ( 'NONE',  ( -16.46253265017160317, 9.564922557960807481, 25.83224293864769194 ) ) ;
#62403=CARTESIAN_POINT ( 'NONE',  ( -18.67979575497193778, 10.72451020669871902, 83.33442372801903275 ) ) ;
#62404=CARTESIAN_POINT ( 'NONE',  ( -5.049401038298153566, 19.05341960407611168, 75.20724293864769550 ) ) ;
#62405=CARTESIAN_POINT ( 'NONE',  ( 15.72974639402176855, 15.80617190586768217, 46.87609039468568994 ) ) ;
#62406=CARTESIAN_POINT ( 'NONE',  ( 0.05219959533937995610, -21.53943276465977519, 30.00109039468568284 ) ) ;
#62408=CARTESIAN_POINT ( 'NONE',  ( -13.89961937509977652, 13.97604488694528158, 100.6239096053143669 ) ) ;
#62410=CARTESIAN_POINT ( 'NONE',  ( -8.314922557961024197, 14.29746914071037800, 37.91775706135235424 ) ) ;
#62411=CARTESIAN_POINT ( 'NONE',  ( -4.379528057220086978, -16.55341960407618274, 64.79275706135234714 ) ) ;
#62412=CARTESIAN_POINT ( 'NONE',  ( -15.80617190586768217, 15.72974639402176855, 48.12609039468568284 ) ) ;
#62413=CARTESIAN_POINT ( 'NONE',  ( 21.52544592524334988, 5.823673210054432836, 76.45942372801901854 ) ) ;
#62415=CARTESIAN_POINT ( 'NONE',  ( 16.55341960407618274, -4.379528057220086978, 21.04275706135234714 ) ) ;
#62416=CARTESIAN_POINT ( 'NONE',  ( 13.97604488694527802, 13.89961937509977652, 64.37390960531436690 ) ) ;
#62417=CARTESIAN_POINT ( 'NONE',  ( 9.474510206698971260, -16.51473224551069308, 97.91557627198102409 ) ) ;
#62418=CARTESIAN_POINT ( 'NONE',  ( -8.314922557960811034, -14.29746914071050412, 112.0822429386477097 ) ) ;
#62419=CARTESIAN_POINT ( 'NONE',  ( 8.314922557960818139, 14.29746914071049879, 99.58224293864770971 ) ) ;
#62420=CARTESIAN_POINT ( 'NONE',  ( 5.823673210054125526, 21.52544592524343514, 29.79057627198102409 ) ) ;
#62421=CARTESIAN_POINT ( 'NONE',  ( 4.379528057220092307, 16.55341960407617563, 82.29275706135234714 ) ) ;
#62422=CARTESIAN_POINT ( 'NONE',  ( -14.34966873604960291, -8.224510206698953496, 71.66557627198100988 ) ) ;
#62423=CARTESIAN_POINT ( 'NONE',  ( -16.51473224551069308, -9.474510206698971260, 51.66557627198102409 ) ) ;
#62424=CARTESIAN_POINT ( 'NONE',  ( 21.55341960407619695, -5.719274019375665929, 71.04275706135234714 ) ) ;
#62425=CARTESIAN_POINT ( 'NONE',  ( 5.823673210054444382, -21.52544592524334988, 70.20942372801904696 ) ) ;
#62426=CARTESIAN_POINT ( 'NONE',  ( 5.049401038297881783, 19.05341960407617563, 107.2927570613523187 ) ) ;
#62427=CARTESIAN_POINT ( 'NONE',  ( 4.483927247898545687, 16.52544592524342804, 79.79057627198102409 ) ) ;
#62428=CARTESIAN_POINT ( 'NONE',  ( 5.719274019375673035, 21.55341960407619339, 32.29275706135235424 ) ) ;
#62429=CARTESIAN_POINT ( 'NONE',  ( -18.62759615963270932, 10.81492255796079327, 55.83224293864770260 ) ) ;
#62430=CARTESIAN_POINT ( 'NONE',  ( -17.48853670773244318, -5.747243402303109150, 106.3332870025001284 ) ) ;
#62432=CARTESIAN_POINT ( 'NONE',  ( 13.97604488694527802, 13.89961937509977652, 69.37390960531436690 ) ) ;
#62433=CARTESIAN_POINT ( 'NONE',  ( 12.14591786802309770, 12.06949235617756955, 49.37390960531436690 ) ) ;
#62434=CARTESIAN_POINT ( 'NONE',  ( -16.55341960407611168, -4.379528057220339221, 26.45724293864768839 ) ) ;
#62435=CARTESIAN_POINT ( 'NONE',  ( 14.29746914071037800, 8.314922557961029526, 101.6677570613523613 ) ) ;
#62436=CARTESIAN_POINT ( 'NONE',  ( -0.05219959533936034679, 19.03943276465977164, 52.50109039468566863 ) ) ;
#62437=CARTESIAN_POINT ( 'NONE',  ( 0.05219959533909260263, 19.03943276465977164, 104.9989096053143669 ) ) ;
#62438=CARTESIAN_POINT ( 'NONE',  ( -4.483927247898539470, -16.52544592524342804, 72.29057627198102409 ) ) ;
#62439=CARTESIAN_POINT ( 'NONE',  ( -13.97604488694547697, 13.89961937509957934, 43.12609039468566152 ) ) ;
#62440=CARTESIAN_POINT ( 'NONE',  ( 16.46253265017160672, -9.564922557960803928, 38.33224293864768839 ) ) ;
#62441=CARTESIAN_POINT ( 'NONE',  ( 5.823673210054125526, 21.52544592524343514, 34.79057627198103120 ) ) ;
#62442=CARTESIAN_POINT ( 'NONE',  ( 21.53943276465977519, -0.05219959533907433946, 53.74890960531437401 ) ) ;
#62444=CARTESIAN_POINT ( 'NONE',  ( 0.05219959533910956823, 16.53943276465976808, 104.9989096053143669 ) ) ;
#62445=CARTESIAN_POINT ( 'NONE',  ( -4.379528057220086978, -16.55341960407618274, 54.79275706135235424 ) ) ;
#62446=CARTESIAN_POINT ( 'NONE',  ( -14.29746914071049879, 8.314922557960819915, 90.83224293864769550 ) ) ;
#62447=EDGE_CURVE ( 'NONE', #30776, #61770, #182308, .T. ) ;
#62450=CARTESIAN_POINT ( 'NONE',  ( 18.62759615963271287, -10.81492255796078972, 23.33224293864769194 ) ) ;
#62454=CARTESIAN_POINT ( 'NONE',  ( -12.06949235617739369, -12.14591786802326823, 39.37609039468567573 ) ) ;
#62455=CARTESIAN_POINT ( 'NONE',  ( 12.14591786802309770, 12.06949235617756955, 24.37390960531435979 ) ) ;
#62456=CARTESIAN_POINT ( 'NONE',  ( -21.53943276465977519, 0.05219959533907696930, 56.24890960531436690 ) ) ;
#62458=CARTESIAN_POINT ( 'NONE',  ( -16.51473224551082808, 9.474510206698731452, 78.33442372801900433 ) ) ;
#62459=CARTESIAN_POINT ( 'NONE',  ( 5.823673210054125526, 21.52544592524343514, 64.79057627198103830 ) ) ;
#62460=CARTESIAN_POINT ( 'NONE',  ( -10.81492255796105439, 18.62759615963255655, 87.91775706135234714 ) ) ;
#62462=CARTESIAN_POINT ( 'NONE',  ( -8.314922557961024197, 14.29746914071037800, 47.91775706135234714 ) ) ;
#62463=CARTESIAN_POINT ( 'NONE',  ( -16.46253265017160317, 9.564922557960807481, 30.83224293864769550 ) ) ;
#62464=CARTESIAN_POINT ( 'NONE',  ( 9.564922557960805705, 16.46253265017160317, 99.58224293864770971 ) ) ;
#62465=CARTESIAN_POINT ( 'NONE',  ( 19.03943276465977164, -0.05219959533909143690, 38.74890960531436690 ) ) ;
#62466=CARTESIAN_POINT ( 'NONE',  ( 4.379528057220339221, -16.55341960407611168, 107.7072429386476955 ) ) ;
#62469=CARTESIAN_POINT ( 'NONE',  ( 13.97604488694527802, 13.89961937509977652, 99.37390960531436690 ) ) ;
#62471=CARTESIAN_POINT ( 'NONE',  ( 0.05219959533934541429, -16.53943276465976808, 70.00109039468568994 ) ) ;
#62472=CARTESIAN_POINT ( 'NONE',  ( -5.823673210054116645, -21.52544592524344225, 92.29057627198103830 ) ) ;
#62473=CARTESIAN_POINT ( 'NONE',  ( 13.89961937509977652, -13.97604488694527269, 53.12390960531434558 ) ) ;
#62474=CARTESIAN_POINT ( 'NONE',  ( 10.72451020669871369, 18.67979575497193778, 22.08442372801901143 ) ) ;
#62475=CARTESIAN_POINT ( 'NONE',  ( -9.474510206698964154, 16.51473224551069663, 85.41557627198102409 ) ) ;
#62477=ORIENTED_EDGE ( 'NONE', *, *, #129099, .F. ) ;
#62478=CARTESIAN_POINT ( 'NONE',  ( 21.55341960407610458, 5.719274019375980345, 113.9572429386477239 ) ) ;
#62479=CARTESIAN_POINT ( 'NONE',  ( -19.03943276465977164, 0.05219959533909376836, 26.24890960531435624 ) ) ;
#62480=CARTESIAN_POINT ( 'NONE',  ( 19.03943276465977164, -0.05219959533909143690, 103.7489096053143669 ) ) ;
#62481=CARTESIAN_POINT ( 'NONE',  ( 16.51473224551083163, -9.474510206698727899, 70.83442372801900433 ) ) ;
#62482=CARTESIAN_POINT ( 'NONE',  ( -5.153800228976607833, 19.02544592524334988, 27.70942372801899722 ) ) ;
#62483=CARTESIAN_POINT ( 'NONE',  ( 15.72974639402199770, -15.80617190586745480, 98.12390960531436690 ) ) ;
#62484=CARTESIAN_POINT ( 'NONE',  ( 19.05341960407617918, -5.049401038297876454, 41.04275706135233293 ) ) ;
#62485=CARTESIAN_POINT ( 'NONE',  ( 4.483927247898790824, -16.52544592524335698, 75.20942372801901854 ) ) ;
#62486=CARTESIAN_POINT ( 'NONE',  ( 16.51473224551069308, 9.474510206698969483, 104.1655762719810241 ) ) ;
#62488=CARTESIAN_POINT ( 'NONE',  ( 13.89961937509977652, -13.97604488694527269, 63.12390960531435979 ) ) ;
#62489=CARTESIAN_POINT ( 'NONE',  ( -10.72451020669870658, -18.67979575497194134, 59.58442372801901854 ) ) ;
#62490=CARTESIAN_POINT ( 'NONE',  ( 10.81492255796106328, -18.62759615963255655, 80.41775706135234714 ) ) ;
#62491=CARTESIAN_POINT ( 'NONE',  ( 5.049401038298161559, -19.05341960407611168, 77.70724293864765286 ) ) ;
#62492=CARTESIAN_POINT ( 'NONE',  ( -0.05219959533937732626, 21.53943276465977519, 42.50109039468567573 ) ) ;
#62493=CARTESIAN_POINT ( 'NONE',  ( -0.05219959533936034679, 19.03943276465977164, 92.50109039468566152 ) ) ;
#62494=CARTESIAN_POINT ( 'NONE',  ( -13.97604488694527625, -13.89961937509977652, 46.87390960531435979 ) ) ;
#62495=CARTESIAN_POINT ( 'NONE',  ( 5.153800228976335163, 19.02544592524342804, 99.79057627198102409 ) ) ;
#62496=CARTESIAN_POINT ( 'NONE',  ( -19.02544592524342804, 5.153800228976336051, 66.04057627198103830 ) ) ;
#62497=CARTESIAN_POINT ( 'NONE',  ( -19.03943276465977164, 0.05219959533909376836, 111.2489096053143669 ) ) ;
#62498=CARTESIAN_POINT ( 'NONE',  ( -5.049401038298153566, 19.05341960407611168, 50.20724293864770260 ) ) ;
#62500=CARTESIAN_POINT ( 'NONE',  ( 10.72451020669898902, -18.67979575497178502, 102.9155762719810383 ) ) ;
#62501=CARTESIAN_POINT ( 'NONE',  ( 12.14591786802327356, -12.06949235617739191, 80.62609039468567573 ) ) ;
#62503=CARTESIAN_POINT ( 'NONE',  ( -13.97604488694547697, 13.89961937509957934, 38.12609039468566152 ) ) ;
#62504=CARTESIAN_POINT ( 'NONE',  ( 16.51473224551069308, 9.474510206698969483, 64.16557627198102409 ) ) ;
#62505=CARTESIAN_POINT ( 'NONE',  ( 12.06949235617757843, -12.14591786802309237, 58.12390960531435979 ) ) ;
#62506=CARTESIAN_POINT ( 'NONE',  ( 12.06949235617757843, -12.14591786802309237, 98.12390960531436690 ) ) ;
#62507=CARTESIAN_POINT ( 'NONE',  ( -16.46253265017160317, 9.564922557960807481, 95.83224293864769550 ) ) ;
#62508=CARTESIAN_POINT ( 'NONE',  ( -19.03943276465977164, 0.05219959533909376836, 86.24890960531436690 ) ) ;
#62509=CARTESIAN_POINT ( 'NONE',  ( 13.97604488694527802, 13.89961937509977652, 104.3739096053143385 ) ) ;
#62510=CARTESIAN_POINT ( 'NONE',  ( -0.05219959533937732626, 21.53943276465977519, 107.5010903946856899 ) ) ;
#62511=CARTESIAN_POINT ( 'NONE',  ( -16.53943276465976808, -0.05219959533934237506, 93.75109039468567573 ) ) ;
#62512=CARTESIAN_POINT ( 'NONE',  ( 9.564922557960805705, 16.46253265017160317, 74.58224293864769550 ) ) ;
#62513=CARTESIAN_POINT ( 'NONE',  ( -18.67979575497193778, 10.72451020669871902, 33.33442372801900433 ) ) ;
#62514=CARTESIAN_POINT ( 'NONE',  ( -21.53943276465977519, 0.05219959533907696930, 36.24890960531435979 ) ) ;
#62515=CARTESIAN_POINT ( 'NONE',  ( -10.81492255796078084, -18.62759615963271287, 102.0822429386476955 ) ) ;
#62516=CARTESIAN_POINT ( 'NONE',  ( 14.34966873604960469, 8.224510206698951720, 59.16557627198103120 ) ) ;
#62517=CARTESIAN_POINT ( 'NONE',  ( 19.03943276465977164, -0.05219959533909143690, 48.74890960531435979 ) ) ;
#62518=CARTESIAN_POINT ( 'NONE',  ( 8.314922557960818139, 14.29746914071049879, 84.58224293864769550 ) ) ;
#62519=CARTESIAN_POINT ( 'NONE',  ( -5.049401038297874678, -19.05341960407617918, 44.79275706135232582 ) ) ;
#62520=CARTESIAN_POINT ( 'NONE',  ( 19.02544592524343514, -5.153800228976328945, 23.54057627198102054 ) ) ;
#62521=CARTESIAN_POINT ( 'NONE',  ( -4.379528057220086978, -16.55341960407618274, 69.79275706135234714 ) ) ;
#62522=CARTESIAN_POINT ( 'NONE',  ( -5.153800228976328057, -19.02544592524343514, 87.29057627198103830 ) ) ;
#62524=CARTESIAN_POINT ( 'NONE',  ( 8.314922557960818139, 14.29746914071049879, 104.5822429386477097 ) ) ;
#62525=CARTESIAN_POINT ( 'NONE',  ( 5.823673210054125526, 21.52544592524343514, 39.79057627198103830 ) ) ;
#62526=EDGE_LOOP ( 'NONE', ( #85864, #50307, #158845, #194292, #76344, #136549, #199692, #6762 ) ) ;
#62527=CARTESIAN_POINT ( 'NONE',  ( 16.52544592524335698, 4.483927247898782831, 106.4594237280190328 ) ) ;
#62528=CARTESIAN_POINT ( 'NONE',  ( 8.224510206698742110, 14.34966873604972548, 32.08442372801901854 ) ) ;
#62529=CARTESIAN_POINT ( 'NONE',  ( -18.67979575497193778, 10.72451020669871902, 88.33442372801901854 ) ) ;
#62530=CARTESIAN_POINT ( 'NONE',  ( 16.46253265017160672, -9.564922557960803928, 93.33224293864769550 ) ) ;
#62531=CARTESIAN_POINT ( 'NONE',  ( -18.62759615963270932, 10.81492255796079327, 115.8322429386477097 ) ) ;
#62532=CARTESIAN_POINT ( 'NONE',  ( 9.564922557960805705, 16.46253265017160317, 24.58224293864769194 ) ) ;
#62533=CARTESIAN_POINT ( 'NONE',  ( 0.05219959533934541429, -16.53943276465976808, 30.00109039468568284 ) ) ;
#62534=CARTESIAN_POINT ( 'NONE',  ( 19.03943276465977164, 0.05219959533936151252, 91.25109039468566152 ) ) ;
#62536=CARTESIAN_POINT ( 'NONE',  ( -21.52544592524343514, 5.823673210054127303, 86.04057627198102409 ) ) ;
#62537=CARTESIAN_POINT ( 'NONE',  ( -9.564922557961040184, 16.46253265017147172, 67.91775706135233293 ) ) ;
#62538=CARTESIAN_POINT ( 'NONE',  ( -5.153800228976328057, -19.02544592524343514, 22.29057627198102765 ) ) ;
#62539=CARTESIAN_POINT ( 'NONE',  ( 15.72974639402176855, 15.80617190586768217, 21.87609039468567573 ) ) ;
#62540=CARTESIAN_POINT ( 'NONE',  ( -9.564922557960796823, -16.46253265017161027, 72.08224293864770971 ) ) ;
#62541=CARTESIAN_POINT ( 'NONE',  ( -19.03943276465977164, 0.05219959533909376836, 96.24890960531436690 ) ) ;
#62542=CARTESIAN_POINT ( 'NONE',  ( 4.379528057220092307, 16.55341960407617563, 27.29275706135234358 ) ) ;
#62544=CARTESIAN_POINT ( 'NONE',  ( -13.89961937509957401, -13.97604488694547875, 59.37609039468566863 ) ) ;
#62545=CARTESIAN_POINT ( 'NONE',  ( -21.53943276465977519, -0.05219959533937600094, 18.75109039468568639 ) ) ;
#62546=CARTESIAN_POINT ( 'NONE',  ( 14.34966873604960469, 8.224510206698951720, 79.16557627198103830 ) ) ;
#62547=CARTESIAN_POINT ( 'NONE',  ( 19.02544592524343514, -5.153800228976328945, 88.54057627198102409 ) ) ;
#62548=CARTESIAN_POINT ( 'NONE',  ( 14.34966873604972726, -8.224510206698740333, 50.83442372801901143 ) ) ;
#62549=CARTESIAN_POINT ( 'NONE',  ( -5.049401038297874678, -19.05341960407617918, 54.79275706135234003 ) ) ;
#62550=CARTESIAN_POINT ( 'NONE',  ( -10.72451020669870658, -18.67979575497194134, 69.58442372801900433 ) ) ;
#62551=CARTESIAN_POINT ( 'NONE',  ( 16.53943276465976808, 0.05219959533934440121, 31.25109039468568639 ) ) ;
#62552=CARTESIAN_POINT ( 'NONE',  ( 19.03943276465977164, -0.05219959533909143690, 73.74890960531435269 ) ) ;
#62553=CARTESIAN_POINT ( 'NONE',  ( 13.89961937509957401, 13.97604488694547697, 81.87609039468564731 ) ) ;
#62554=CARTESIAN_POINT ( 'NONE',  ( 14.34966873604972726, -8.224510206698740333, 55.83442372801901854 ) ) ;
#62555=CARTESIAN_POINT ( 'NONE',  ( 18.62759615963255655, 10.81492255796105972, 91.66775706135234714 ) ) ;
#62556=CARTESIAN_POINT ( 'NONE',  ( 9.474510206698729675, 16.51473224551082808, 67.08442372801900433 ) ) ;
#62557=CARTESIAN_POINT ( 'NONE',  ( -5.049401038298153566, 19.05341960407611168, 50.20724293864770260 ) ) ;
#62558=CARTESIAN_POINT ( 'NONE',  ( -18.62759615963270932, 10.81492255796079327, 70.83224293864770971 ) ) ;
#62559=CARTESIAN_POINT ( 'NONE',  ( 0.05219959533910956823, 16.53943276465976808, 59.99890960531436690 ) ) ;
#62560=CARTESIAN_POINT ( 'NONE',  ( 16.51473224551083163, -9.474510206698727899, 80.83442372801899012 ) ) ;
#62561=CARTESIAN_POINT ( 'NONE',  ( 16.20579543436675962, -7.371946100355160958, 61.93479165828127009 ) ) ;
#62562=CARTESIAN_POINT ( 'NONE',  ( -13.97604488694547697, 13.89961937509957934, 43.12609039468566152 ) ) ;
#62563=CARTESIAN_POINT ( 'NONE',  ( -12.06949235617739369, -12.14591786802326823, 104.3760903946856899 ) ) ;
#62564=CARTESIAN_POINT ( 'NONE',  ( -16.52544592524342804, 4.483927247898546575, 66.04057627198103830 ) ) ;
#62565=CARTESIAN_POINT ( 'NONE',  ( -18.62759615963255300, -10.81492255796106328, 99.16775706135234714 ) ) ;
#62567=CARTESIAN_POINT ( 'NONE',  ( 15.80617190586746368, 15.72974639402197994, 99.37390960531436690 ) ) ;
#62568=CARTESIAN_POINT ( 'NONE',  ( 13.97604488694527802, 13.89961937509977652, 59.37390960531434558 ) ) ;
#62569=CARTESIAN_POINT ( 'NONE',  ( 21.52544592524334988, 5.823673210054432836, 76.45942372801901854 ) ) ;
#62570=CARTESIAN_POINT ( 'NONE',  ( 13.89961937509977652, -13.97604488694527269, 48.12390960531435979 ) ) ;
#62571=CARTESIAN_POINT ( 'NONE',  ( -13.97604488694527625, -13.89961937509977652, 26.87390960531434558 ) ) ;
#62572=CARTESIAN_POINT ( 'NONE',  ( -19.05341960407611168, -5.049401038298163336, 111.4572429386476671 ) ) ;
#62573=CARTESIAN_POINT ( 'NONE',  ( -16.53943276465976808, 0.05219959533911058130, 66.24890960531436690 ) ) ;
#62574=CARTESIAN_POINT ( 'NONE',  ( 19.03943276465977164, -0.05219959533909143690, 23.74890960531435269 ) ) ;
#62575=CARTESIAN_POINT ( 'NONE',  ( -4.379528057220328563, 16.55341960407611168, 85.20724293864770971 ) ) ;
#62576=CARTESIAN_POINT ( 'NONE',  ( -5.823673210054116645, -21.52544592524344225, 97.29057627198105251 ) ) ;
#62578=CARTESIAN_POINT ( 'NONE',  ( 18.62759615963255655, 10.81492255796105972, 36.66775706135234714 ) ) ;
#62580=CARTESIAN_POINT ( 'NONE',  ( -16.53943276465976808, -0.05219959533934237506, 53.75109039468568994 ) ) ;
#62581=CARTESIAN_POINT ( 'NONE',  ( -21.52544592524343514, 5.823673210054127303, 81.04057627198102409 ) ) ;
#62582=CARTESIAN_POINT ( 'NONE',  ( -13.97604488694547697, 13.89961937509957934, 28.12609039468565797 ) ) ;
#62583=CARTESIAN_POINT ( 'NONE',  ( 16.46253265017160672, -9.564922557960803928, 108.3322429386476955 ) ) ;
#62584=CARTESIAN_POINT ( 'NONE',  ( -5.823673210054431948, 21.52544592524334988, 42.70942372801901854 ) ) ;
#62585=CARTESIAN_POINT ( 'NONE',  ( -21.53943276465977519, 0.05219959533907696930, 46.24890960531435979 ) ) ;
#62586=CARTESIAN_POINT ( 'NONE',  ( 8.224510206698953496, -14.34966873604960469, 22.91557627198102765 ) ) ;
#62587=CARTESIAN_POINT ( 'NONE',  ( 21.55341960407619695, -5.719274019375665929, 66.04275706135236135 ) ) ;
#62588=CARTESIAN_POINT ( 'NONE',  ( 21.55341960407619695, -5.719274019375665929, 96.04275706135236135 ) ) ;
#62589=CARTESIAN_POINT ( 'NONE',  ( -13.97604488694547697, 13.89961937509957934, 33.12609039468566863 ) ) ;
#62590=CARTESIAN_POINT ( 'NONE',  ( 4.379528057220092307, 16.55341960407617563, 92.29275706135236135 ) ) ;
#62591=CARTESIAN_POINT ( 'NONE',  ( -15.72974639402176322, -15.80617190586768395, 54.37609039468568994 ) ) ;
#62592=CARTESIAN_POINT ( 'NONE',  ( -16.51473224551069308, -9.474510206698971260, 51.66557627198102409 ) ) ;
#62593=CARTESIAN_POINT ( 'NONE',  ( 13.97604488694548053, -13.89961937509957401, 20.62609039468567573 ) ) ;
#62594=CARTESIAN_POINT ( 'NONE',  ( -10.81492255796078084, -18.62759615963271287, 27.08224293864769550 ) ) ;
#62595=CARTESIAN_POINT ( 'NONE',  ( -21.55341960407619339, 5.719274019375674811, 23.54275706135235424 ) ) ;
#62596=CARTESIAN_POINT ( 'NONE',  ( -5.719274019375978568, 21.55341960407610458, 75.20724293864769550 ) ) ;
#62597=CARTESIAN_POINT ( 'NONE',  ( -14.34966873604972548, 8.224510206698743886, 38.33442372801900433 ) ) ;
#62599=CARTESIAN_POINT ( 'NONE',  ( 21.55341960407610458, 5.719274019375980345, 73.95724293864769550 ) ) ;
#62600=CARTESIAN_POINT ( 'NONE',  ( -12.14591786802326823, 12.06949235617739902, 68.12609039468567573 ) ) ;
#62601=CARTESIAN_POINT ( 'NONE',  ( -16.52544592524342804, 4.483927247898546575, 66.04057627198103830 ) ) ;
#62603=CARTESIAN_POINT ( 'NONE',  ( -19.03943276465977164, -0.05219959533935918106, 98.75109039468567573 ) ) ;
#62605=CARTESIAN_POINT ( 'NONE',  ( -8.224510206698735004, -14.34966873604973081, 39.58442372801901143 ) ) ;
#62606=CARTESIAN_POINT ( 'NONE',  ( -15.72974639402197994, 15.80617190586746368, 105.6239096053143669 ) ) ;
#62607=CARTESIAN_POINT ( 'NONE',  ( -21.55341960407610458, -5.719274019375992779, 26.45724293864768839 ) ) ;
#62608=CARTESIAN_POINT ( 'NONE',  ( 0.05219959533934541429, -16.53943276465976808, 60.00109039468568284 ) ) ;
#62609=CARTESIAN_POINT ( 'NONE',  ( 13.89961937509977652, -13.97604488694527269, 73.12390960531436690 ) ) ;
#62610=CARTESIAN_POINT ( 'NONE',  ( 18.67979575497194134, -10.72451020669871369, 40.83442372801901854 ) ) ;
#62611=CARTESIAN_POINT ( 'NONE',  ( -0.05219959533934338120, 16.53943276465976808, 22.50109039468567573 ) ) ;
#62613=CARTESIAN_POINT ( 'NONE',  ( -21.52544592524343514, 5.823673210054127303, 31.04057627198102409 ) ) ;
#62614=CARTESIAN_POINT ( 'NONE',  ( -16.51473224551082808, 9.474510206698731452, 23.33442372801900078 ) ) ;
#62615=CARTESIAN_POINT ( 'NONE',  ( 14.29746914071037800, 8.314922557961029526, 41.66775706135235424 ) ) ;
#62616=CARTESIAN_POINT ( 'NONE',  ( -13.97604488694527625, -13.89961937509977652, 106.8739096053143669 ) ) ;
#62617=CARTESIAN_POINT ( 'NONE',  ( -18.67979575497178146, -10.72451020669898902, 96.66557627198102409 ) ) ;
#62618=CARTESIAN_POINT ( 'NONE',  ( 13.97604488694527802, 13.89961937509977652, 69.37390960531436690 ) ) ;
#62619=CARTESIAN_POINT ( 'NONE',  ( -17.44279575226823198, 5.990770900252464060, 25.83557567514319686 ) ) ;
#62620=CARTESIAN_POINT ( 'NONE',  ( 8.314922557960818139, 14.29746914071049879, 84.58224293864769550 ) ) ;
#62621=CARTESIAN_POINT ( 'NONE',  ( -9.564922557960796823, -16.46253265017161027, 112.0822429386476955 ) ) ;
#62623=CARTESIAN_POINT ( 'NONE',  ( -12.14591786802326823, 12.06949235617739902, 68.12609039468567573 ) ) ;
#62624=CARTESIAN_POINT ( 'NONE',  ( 15.80617190586746368, 15.72974639402197994, 109.3739096053143811 ) ) ;
#62625=CARTESIAN_POINT ( 'NONE',  ( -13.97604488694547697, 13.89961937509957934, 68.12609039468563310 ) ) ;
#62626=CARTESIAN_POINT ( 'NONE',  ( -5.823673210054116645, -21.52544592524344225, 27.29057627198103120 ) ) ;
#62628=CARTESIAN_POINT ( 'NONE',  ( 9.564922557960805705, 16.46253265017160317, 24.58224293864769194 ) ) ;
#62629=CARTESIAN_POINT ( 'NONE',  ( 21.55341960407610458, 5.719274019375980345, 73.95724293864769550 ) ) ;
#62630=VECTOR ( 'NONE', #92032, 1000.000000000000000 ) ;
#62631=CARTESIAN_POINT ( 'NONE',  ( -0.05219959533909027116, -19.03943276465977164, 102.4989096053143669 ) ) ;
#62632=CARTESIAN_POINT ( 'NONE',  ( 5.823673210054444382, -21.52544592524334988, 90.20942372801903275 ) ) ;
#62633=CARTESIAN_POINT ( 'NONE',  ( 19.02544592524343514, -5.153800228976328945, 48.54057627198103120 ) ) ;
#62634=CARTESIAN_POINT ( 'NONE',  ( 16.55341960407611168, 4.379528057220329451, 88.95724293864769550 ) ) ;
#62635=CARTESIAN_POINT ( 'NONE',  ( -16.53943276465976808, -0.05219959533934237506, 38.75109039468567573 ) ) ;
#62636=CARTESIAN_POINT ( 'NONE',  ( 19.05341960407611168, 5.049401038298154454, 58.95724293864768129 ) ) ;
#62637=CARTESIAN_POINT ( 'NONE',  ( -18.62759615963255300, -10.81492255796106328, 74.16775706135231871 ) ) ;
#62639=CARTESIAN_POINT ( 'NONE',  ( 0.05219959533936267826, -19.03943276465977164, 45.00109039468566863 ) ) ;
#62640=CARTESIAN_POINT ( 'NONE',  ( 19.05341960407617918, -5.049401038297876454, 41.04275706135233293 ) ) ;
#62641=CARTESIAN_POINT ( 'NONE',  ( -5.823673210054431948, 21.52544592524334988, 42.70942372801901854 ) ) ;
#62643=CARTESIAN_POINT ( 'NONE',  ( 19.03943276465977164, 0.05219959533936151252, 26.25109039468566507 ) ) ;
#62644=CARTESIAN_POINT ( 'NONE',  ( -16.51473224551069308, -9.474510206698971260, 81.66557627198103830 ) ) ;
#62645=CARTESIAN_POINT ( 'NONE',  ( 5.049401038298161559, -19.05341960407611168, 72.70724293864768129 ) ) ;
#62646=CARTESIAN_POINT ( 'NONE',  ( -14.29746914071049879, 8.314922557960819915, 25.83224293864769194 ) ) ;
#62647=CARTESIAN_POINT ( 'NONE',  ( -15.80617190586745835, -15.72974639402198527, 26.87390960531435979 ) ) ;
#62648=CARTESIAN_POINT ( 'NONE',  ( 10.72451020669871369, 18.67979575497193778, 82.08442372801901854 ) ) ;
#62651=CARTESIAN_POINT ( 'NONE',  ( 18.67979575497194134, -10.72451020669871369, 100.8344237280190185 ) ) ;
#62653=CARTESIAN_POINT ( 'NONE',  ( 16.51473224551069308, 9.474510206698969483, 114.1655762719810241 ) ) ;
#62655=CARTESIAN_POINT ( 'NONE',  ( -8.224510206698735004, -14.34966873604973081, 49.58442372801901143 ) ) ;
#62656=CARTESIAN_POINT ( 'NONE',  ( -21.53943276465977519, 0.05219959533907696930, 76.24890960531435269 ) ) ;
#62657=CARTESIAN_POINT ( 'NONE',  ( 8.224510206698953496, -14.34966873604960469, 27.91557627198103830 ) ) ;
#62658=CARTESIAN_POINT ( 'NONE',  ( -16.51473224551069308, -9.474510206698971260, 21.66557627198102765 ) ) ;
#62659=CARTESIAN_POINT ( 'NONE',  ( 9.474510206698971260, -16.51473224551069308, 97.91557627198102409 ) ) ;
#62660=CARTESIAN_POINT ( 'NONE',  ( -13.89961937509957401, -13.97604488694547875, 19.37609039468566507 ) ) ;
#62661=CARTESIAN_POINT ( 'NONE',  ( -5.153800228976328057, -19.02544592524343514, 22.29057627198102765 ) ) ;
#62662=CARTESIAN_POINT ( 'NONE',  ( -15.72974639402176322, -15.80617190586768395, 64.37609039468568994 ) ) ;
#62663=CARTESIAN_POINT ( 'NONE',  ( 16.53943276465976808, 0.05219959533934440121, 111.2510903946856899 ) ) ;
#62664=CARTESIAN_POINT ( 'NONE',  ( 5.153800228976615827, -19.02544592524334988, 65.20942372801900433 ) ) ;
#62666=CARTESIAN_POINT ( 'NONE',  ( -16.51473224551069308, -9.474510206698971260, 106.6655762719810383 ) ) ;
#62667=CARTESIAN_POINT ( 'NONE',  ( 8.314922557960818139, 14.29746914071049879, 89.58224293864768129 ) ) ;
#62668=CARTESIAN_POINT ( 'NONE',  ( -19.05341960407617563, 5.049401038297882671, 58.54275706135234003 ) ) ;
#62669=CARTESIAN_POINT ( 'NONE',  ( -16.46253265017160317, 9.564922557960807481, 75.83224293864769550 ) ) ;
#62670=CARTESIAN_POINT ( 'NONE',  ( -8.224510206698948167, 14.34966873604960824, 65.41557627198102409 ) ) ;
#62671=CARTESIAN_POINT ( 'NONE',  ( -5.049401038297874678, -19.05341960407617918, 94.79275706135230450 ) ) ;
#62672=CARTESIAN_POINT ( 'NONE',  ( 5.823673210054125526, 21.52544592524343514, 54.79057627198104541 ) ) ;
#62673=ORIENTED_EDGE ( 'NONE', *, *, #85633, .F. ) ;
#62674=CARTESIAN_POINT ( 'NONE',  ( -16.53943276465976808, 0.05219959533911058130, 116.2489096053143669 ) ) ;
#62675=CARTESIAN_POINT ( 'NONE',  ( -17.48847506799968343, -5.747544572773811034, 29.17302562156720924 ) ) ;
#62676=CARTESIAN_POINT ( 'NONE',  ( -0.05219959533909027116, -19.03943276465977164, 72.49890960531435269 ) ) ;
#62677=CARTESIAN_POINT ( 'NONE',  ( -10.72451020669898014, 18.67979575497178502, 80.41557627198103830 ) ) ;
#62678=CARTESIAN_POINT ( 'NONE',  ( 8.224510206698742110, 14.34966873604972548, 97.08442372801904696 ) ) ;
#62679=CARTESIAN_POINT ( 'NONE',  ( 9.474510206698971260, -16.51473224551069308, 77.91557627198103830 ) ) ;
#62680=CARTESIAN_POINT ( 'NONE',  ( -9.474510206698720793, -16.51473224551083518, 69.58442372801901854 ) ) ;
#62681=CARTESIAN_POINT ( 'NONE',  ( 15.80617190586769283, -15.72974639402175789, 80.62609039468567573 ) ) ;
#62682=CARTESIAN_POINT ( 'NONE',  ( -21.53943276465977519, 0.05219959533907696930, 61.24890960531435979 ) ) ;
#62683=CARTESIAN_POINT ( 'NONE',  ( -15.72974639402197994, 15.80617190586746368, 30.62390960531436335 ) ) ;
#62684=CARTESIAN_POINT ( 'NONE',  ( -16.51473224551069308, -9.474510206698971260, 41.66557627198103120 ) ) ;
#62685=CARTESIAN_POINT ( 'NONE',  ( 8.224510206698742110, 14.34966873604972548, 107.0844237280190043 ) ) ;
#62686=CARTESIAN_POINT ( 'NONE',  ( -16.51473224551069308, -9.474510206698971260, 51.66557627198102409 ) ) ;
#62687=CARTESIAN_POINT ( 'NONE',  ( 8.314922557961029526, -14.29746914071037800, 20.41775706135234714 ) ) ;
#62688=DIRECTION ( 'NONE',  ( -1.000000000000000000, -0.000000000000000000, -0.000000000000000000 ) ) ;
#62689=CARTESIAN_POINT ( 'NONE',  ( -21.53943276465977519, -0.05219959533937600094, 108.7510903946857042 ) ) ;
#62690=CARTESIAN_POINT ( 'NONE',  ( -4.379528057220328563, 16.55341960407611168, 55.20724293864770260 ) ) ;
#62691=CARTESIAN_POINT ( 'NONE',  ( 18.67979575497178502, 10.72451020669898547, 99.16557627198100988 ) ) ;
#62692=CARTESIAN_POINT ( 'NONE',  ( -18.62759615963270932, 10.81492255796079327, 105.8322429386476955 ) ) ;
#62694=CARTESIAN_POINT ( 'NONE',  ( 0.05219959533907565091, 21.53943276465977519, 44.99890960531435979 ) ) ;
#62695=CARTESIAN_POINT ( 'NONE',  ( 16.55341960407618274, -4.379528057220086978, 86.04275706135236135 ) ) ;
#62696=CARTESIAN_POINT ( 'NONE',  ( -14.29746914071049879, 8.314922557960819915, 90.83224293864769550 ) ) ;
#62697=CARTESIAN_POINT ( 'NONE',  ( -16.46253265017160317, 9.564922557960807481, 45.83224293864769550 ) ) ;
#62699=CARTESIAN_POINT ( 'NONE',  ( -14.34966873604972548, 8.224510206698743886, 103.3344237280190043 ) ) ;
#62700=CARTESIAN_POINT ( 'NONE',  ( 0.05219959533937995610, -21.53943276465977519, 35.00109039468568284 ) ) ;
#62701=CARTESIAN_POINT ( 'NONE',  ( -19.03943276465977164, 0.05219959533909376836, 96.24890960531436690 ) ) ;
#62702=CARTESIAN_POINT ( 'NONE',  ( 10.72451020669871369, 18.67979575497193778, 72.08442372801899012 ) ) ;
#62704=CARTESIAN_POINT ( 'NONE',  ( 13.89961937509977652, -13.97604488694527269, 28.12390960531435624 ) ) ;
#62706=ORIENTED_EDGE ( 'NONE', *, *, #81519, .T. ) ;
#62707=CARTESIAN_POINT ( 'NONE',  ( 18.62759615963255655, 10.81492255796105972, 61.66775706135235424 ) ) ;
#62708=CARTESIAN_POINT ( 'NONE',  ( 9.564922557960805705, 16.46253265017160317, 54.58224293864769550 ) ) ;
#62709=CARTESIAN_POINT ( 'NONE',  ( 9.564922557960805705, 16.46253265017160317, 114.5822429386476955 ) ) ;
#62710=CARTESIAN_POINT ( 'NONE',  ( -5.049401038298153566, 19.05341960407611168, 90.20724293864766707 ) ) ;
#62711=CARTESIAN_POINT ( 'NONE',  ( 19.03943276465977164, 0.05219959533936151252, 71.25109039468566152 ) ) ;
#62712=CARTESIAN_POINT ( 'NONE',  ( 21.55341960407619695, -5.719274019375665929, 41.04275706135236135 ) ) ;
#62713=CARTESIAN_POINT ( 'NONE',  ( -13.89961937509957401, -13.97604488694547875, 104.3760903946856757 ) ) ;
#62714=CARTESIAN_POINT ( 'NONE',  ( -16.51473224551082808, 9.474510206698731452, 58.33442372801900433 ) ) ;
#62715=CARTESIAN_POINT ( 'NONE',  ( 19.03943276465977164, -0.05219959533909143690, 38.74890960531436690 ) ) ;
#62716=CARTESIAN_POINT ( 'NONE',  ( -16.55341960407617563, 4.379528057220093196, 103.5427570613523613 ) ) ;
#62717=CARTESIAN_POINT ( 'NONE',  ( 19.02544592524334988, 5.153800228976608722, 71.45942372801900433 ) ) ;
#62718=CARTESIAN_POINT ( 'NONE',  ( -4.379528057220328563, 16.55341960407611168, 30.20724293864769550 ) ) ;
#62719=CARTESIAN_POINT ( 'NONE',  ( -16.51473224551082808, 9.474510206698731452, 53.33442372801900433 ) ) ;
#62720=CARTESIAN_POINT ( 'NONE',  ( -18.67979575497193778, 10.72451020669871902, 108.3344237280190185 ) ) ;
#62721=CARTESIAN_POINT ( 'NONE',  ( -13.89961937509957401, -13.97604488694547875, 24.37609039468565442 ) ) ;
#62722=CARTESIAN_POINT ( 'NONE',  ( -16.46253265017160317, 9.564922557960807481, 25.83224293864769194 ) ) ;
#62723=CARTESIAN_POINT ( 'NONE',  ( -21.55341960407619339, 5.719274019375674811, 88.54275706135236135 ) ) ;
#62724=CARTESIAN_POINT ( 'NONE',  ( 0.05219959533934541429, -16.53943276465976808, 35.00109039468568284 ) ) ;
#62726=CARTESIAN_POINT ( 'NONE',  ( 9.474510206698971260, -16.51473224551069308, 92.91557627198103830 ) ) ;
#62728=CARTESIAN_POINT ( 'NONE',  ( 9.564922557960805705, 16.46253265017160317, 79.58224293864769550 ) ) ;
#62729=CARTESIAN_POINT ( 'NONE',  ( -16.81555441253467009, 7.025013491696203261, 100.6368544533421101 ) ) ;
#62730=AXIS2_PLACEMENT_3D ( 'NONE', #168455, #124935, #186632 ) ;
#62731=CARTESIAN_POINT ( 'NONE',  ( -19.03943276465977164, -0.05219959533935918106, 78.75109039468567573 ) ) ;
#62732=CARTESIAN_POINT ( 'NONE',  ( 5.049401038298161559, -19.05341960407611168, 107.7072429386476955 ) ) ;
#62733=CARTESIAN_POINT ( 'NONE',  ( 5.823673210054444382, -21.52544592524334988, 100.2094237280190043 ) ) ;
#62734=CARTESIAN_POINT ( 'NONE',  ( -16.55341960407611168, -4.379528057220339221, 101.4572429386476955 ) ) ;
#62735=CARTESIAN_POINT ( 'NONE',  ( 19.05341960407611168, 5.049401038298154454, 28.95724293864769550 ) ) ;
#62736=CARTESIAN_POINT ( 'NONE',  ( 5.823673210054125526, 21.52544592524343514, 59.79057627198103120 ) ) ;
#62738=CARTESIAN_POINT ( 'NONE',  ( -10.72451020669898014, 18.67979575497178502, 40.41557627198103120 ) ) ;
#62739=CARTESIAN_POINT ( 'NONE',  ( 16.46253265017160672, -9.564922557960803928, 23.33224293864769194 ) ) ;
#62741=CARTESIAN_POINT ( 'NONE',  ( -19.05341960407617563, 5.049401038297882671, 58.54275706135234003 ) ) ;
#62742=CARTESIAN_POINT ( 'NONE',  ( -8.224510206698948167, 14.34966873604960824, 40.41557627198103120 ) ) ;
#62743=CARTESIAN_POINT ( 'NONE',  ( -21.53943276465977519, 0.05219959533907696930, 26.24890960531435624 ) ) ;
#62744=CARTESIAN_POINT ( 'NONE',  ( -10.81492255796105439, 18.62759615963255655, 82.91775706135234714 ) ) ;
#62745=CARTESIAN_POINT ( 'NONE',  ( -21.52544592524343514, 5.823673210054127303, 71.04057627198103830 ) ) ;
#62746=CARTESIAN_POINT ( 'NONE',  ( -15.80617190586768217, 15.72974639402176855, 63.12609039468568994 ) ) ;
#62747=CARTESIAN_POINT ( 'NONE',  ( -15.72974639402197994, 15.80617190586746368, 95.62390960531436690 ) ) ;
#62748=CARTESIAN_POINT ( 'NONE',  ( 15.80617190586769283, -15.72974639402175789, 55.62609039468568284 ) ) ;
#62749=CARTESIAN_POINT ( 'NONE',  ( -9.564922557960796823, -16.46253265017161027, 22.08224293864768839 ) ) ;
#62750=CARTESIAN_POINT ( 'NONE',  ( -9.564922557960796823, -16.46253265017161027, 87.08224293864769550 ) ) ;
#62751=CARTESIAN_POINT ( 'NONE',  ( 8.314922557961029526, -14.29746914071037800, 80.41775706135234714 ) ) ;
#62752=CARTESIAN_POINT ( 'NONE',  ( 16.52544592524342804, -4.483927247898539470, 108.5405762719810241 ) ) ;
#62754=CARTESIAN_POINT ( 'NONE',  ( 0.05219959533910956823, 16.53943276465976808, 54.99890960531435269 ) ) ;
#62755=CARTESIAN_POINT ( 'NONE',  ( -0.05219959533934338120, 16.53943276465976808, 107.5010903946856899 ) ) ;
#62756=CARTESIAN_POINT ( 'NONE',  ( -13.89961937509977652, 13.97604488694528158, 70.62390960531432427 ) ) ;
#62757=CARTESIAN_POINT ( 'NONE',  ( 0.05219959533909260263, 19.03943276465977164, 39.99890960531436690 ) ) ;
#62758=CARTESIAN_POINT ( 'NONE',  ( 21.52544592524344225, -5.823673210054117533, 43.54057627198103830 ) ) ;
#62759=CARTESIAN_POINT ( 'NONE',  ( -16.46253265017146816, -9.564922557961047289, 44.16775706135232582 ) ) ;
#62762=CARTESIAN_POINT ( 'NONE',  ( -8.314922557960811034, -14.29746914071050412, 47.08224293864770260 ) ) ;
#62763=CARTESIAN_POINT ( 'NONE',  ( 5.719274019375991003, -21.55341960407610458, 32.70724293864770260 ) ) ;
#62765=CARTESIAN_POINT ( 'NONE',  ( 4.379528057220092307, 16.55341960407617563, 67.29275706135234714 ) ) ;
#62766=CARTESIAN_POINT ( 'NONE',  ( -19.05341960407617563, 5.049401038297882671, 58.54275706135234003 ) ) ;
#62767=CARTESIAN_POINT ( 'NONE',  ( -4.483927247898539470, -16.52544592524342804, 42.29057627198103120 ) ) ;
#62768=CARTESIAN_POINT ( 'NONE',  ( -19.19724070472092592, -5.500000000000081712, 76.06193348274379673 ) ) ;
#62769=CARTESIAN_POINT ( 'NONE',  ( -12.14591786802309592, -12.06949235617757132, 26.87390960531435979 ) ) ;
#62770=CARTESIAN_POINT ( 'NONE',  ( -16.51473224551069308, -9.474510206698971260, 41.66557627198103120 ) ) ;
#62771=CARTESIAN_POINT ( 'NONE',  ( -0.05219959533909027116, -19.03943276465977164, 62.49890960531435979 ) ) ;
#62772=CARTESIAN_POINT ( 'NONE',  ( -13.97604488694527625, -13.89961937509977652, 26.87390960531434558 ) ) ;
#62773=CARTESIAN_POINT ( 'NONE',  ( 18.62759615963255655, 10.81492255796105972, 36.66775706135234714 ) ) ;
#62774=CARTESIAN_POINT ( 'NONE',  ( 13.89961937509977652, -13.97604488694527269, 58.12390960531436690 ) ) ;
#62776=CARTESIAN_POINT ( 'NONE',  ( -13.89961937509977652, 13.97604488694528158, 50.62390960531435979 ) ) ;
#62777=CARTESIAN_POINT ( 'NONE',  ( -0.05219959533907301413, -21.53943276465977519, 42.49890960531435979 ) ) ;
#62778=CARTESIAN_POINT ( 'NONE',  ( -0.05219959533937732626, 21.53943276465977519, 57.50109039468568994 ) ) ;
#62779=CARTESIAN_POINT ( 'NONE',  ( 19.05341960407611168, 5.049401038298154454, 28.95724293864769550 ) ) ;
#62780=CARTESIAN_POINT ( 'NONE',  ( 21.53943276465977519, -0.05219959533907433946, 23.74890960531435269 ) ) ;
#62781=CARTESIAN_POINT ( 'NONE',  ( 16.52544592524335698, 4.483927247898782831, 91.45942372801901854 ) ) ;
#62782=CARTESIAN_POINT ( 'NONE',  ( 21.52544592524334988, 5.823673210054432836, 106.4594237280190328 ) ) ;
#62783=CARTESIAN_POINT ( 'NONE',  ( 8.314922557961029526, -14.29746914071037800, 65.41775706135234714 ) ) ;
#62784=CARTESIAN_POINT ( 'NONE',  ( 9.474510206698971260, -16.51473224551069308, 107.9155762719810383 ) ) ;
#62785=CARTESIAN_POINT ( 'NONE',  ( 0.05219959533934541429, -16.53943276465976808, 50.00109039468568994 ) ) ;
#62786=CARTESIAN_POINT ( 'NONE',  ( 14.29746914071037800, 8.314922557961029526, 31.66775706135234358 ) ) ;
#62787=CARTESIAN_POINT ( 'NONE',  ( 8.314922557961029526, -14.29746914071037800, 90.41775706135236135 ) ) ;
#62788=CARTESIAN_POINT ( 'NONE',  ( 18.62759615963255655, 10.81492255796105972, 56.66775706135235424 ) ) ;
#62789=CARTESIAN_POINT ( 'NONE',  ( 16.53943276465976808, 0.05219959533934440121, 26.25109039468567573 ) ) ;
#62790=CARTESIAN_POINT ( 'NONE',  ( 5.823673210054125526, 21.52544592524343514, 104.7905762719810241 ) ) ;
#62791=CARTESIAN_POINT ( 'NONE',  ( 8.314922557961029526, -14.29746914071037800, 20.41775706135234714 ) ) ;
#62792=CARTESIAN_POINT ( 'NONE',  ( -16.55341960407617563, 4.379528057220093196, 83.54275706135234714 ) ) ;
#62794=CARTESIAN_POINT ( 'NONE',  ( -15.72974639402176322, -15.80617190586768395, 89.37609039468568994 ) ) ;
#62795=CARTESIAN_POINT ( 'NONE',  ( 13.89961937509957401, 13.97604488694547697, 86.87609039468567573 ) ) ;
#62796=CARTESIAN_POINT ( 'NONE',  ( 4.379528057220339221, -16.55341960407611168, 42.70724293864770260 ) ) ;
#62797=CARTESIAN_POINT ( 'NONE',  ( -8.314922557960811034, -14.29746914071050412, 37.08224293864768129 ) ) ;
#62798=CARTESIAN_POINT ( 'NONE',  ( 16.55341960407611168, 4.379528057220329451, 103.9572429386476813 ) ) ;
#62799=CARTESIAN_POINT ( 'NONE',  ( -19.02544592524334988, -5.153800228976617603, 48.95942372801900433 ) ) ;
#62800=CARTESIAN_POINT ( 'NONE',  ( 17.50000000000000000, -5.499999999999992895, 56.21769037696436300 ) ) ;
#62801=CARTESIAN_POINT ( 'NONE',  ( -21.52544592524334988, -5.823673210054445271, 53.95942372801900433 ) ) ;
#62802=CARTESIAN_POINT ( 'NONE',  ( 5.049401038297881783, 19.05341960407617563, 112.2927570613523471 ) ) ;
#62804=CARTESIAN_POINT ( 'NONE',  ( -5.049401038298153566, 19.05341960407611168, 100.2072429386476955 ) ) ;
#62805=CARTESIAN_POINT ( 'NONE',  ( -21.53943276465977519, 0.05219959533907696930, 56.24890960531436690 ) ) ;
#62806=CARTESIAN_POINT ( 'NONE',  ( 19.02544592524334988, 5.153800228976608722, 96.45942372801897591 ) ) ;
#62807=CARTESIAN_POINT ( 'NONE',  ( 19.02544592524343514, -5.153800228976328945, 88.54057627198102409 ) ) ;
#62808=CARTESIAN_POINT ( 'NONE',  ( -0.05219959533907301413, -21.53943276465977519, 62.49890960531436690 ) ) ;
#62809=CARTESIAN_POINT ( 'NONE',  ( 0.05219959533910956823, 16.53943276465976808, 109.9989096053143527 ) ) ;
#62810=CARTESIAN_POINT ( 'NONE',  ( -19.03943276465977164, 0.05219959533909376836, 71.24890960531435269 ) ) ;
#62811=CARTESIAN_POINT ( 'NONE',  ( 16.46253265017160672, -9.564922557960803928, 28.33224293864769550 ) ) ;
#62812=CARTESIAN_POINT ( 'NONE',  ( 0.05219959533937995610, -21.53943276465977519, 35.00109039468568284 ) ) ;
#62813=CARTESIAN_POINT ( 'NONE',  ( -21.53943276465977519, -0.05219959533937600094, 83.75109039468568994 ) ) ;
#62814=CARTESIAN_POINT ( 'NONE',  ( 16.55341960407618274, -4.379528057220086978, 91.04275706135236135 ) ) ;
#62815=CARTESIAN_POINT ( 'NONE',  ( 21.52544592524334988, 5.823673210054432836, 36.45942372801901143 ) ) ;
#62816=CARTESIAN_POINT ( 'NONE',  ( -21.52544592524334988, -5.823673210054445271, 43.95942372801902565 ) ) ;
#62817=CARTESIAN_POINT ( 'NONE',  ( -19.03943276465977164, -0.05219959533935918106, 68.75109039468566152 ) ) ;
#62818=CARTESIAN_POINT ( 'NONE',  ( 13.89961937509977652, -13.97604488694527269, 73.12390960531436690 ) ) ;
#62819=CARTESIAN_POINT ( 'NONE',  ( -18.62759615963255300, -10.81492255796106328, 89.16775706135236135 ) ) ;
#62821=CARTESIAN_POINT ( 'NONE',  ( 5.719274019375991003, -21.55341960407610458, 82.70724293864770971 ) ) ;
#62822=CARTESIAN_POINT ( 'NONE',  ( 12.14591786802309770, 12.06949235617756955, 59.37390960531436690 ) ) ;
#62823=CARTESIAN_POINT ( 'NONE',  ( -15.72974639402176322, -15.80617190586768395, 104.3760903946856899 ) ) ;
#62824=CARTESIAN_POINT ( 'NONE',  ( 12.14591786802309770, 12.06949235617756955, 84.37390960531438111 ) ) ;
#62825=CARTESIAN_POINT ( 'NONE',  ( -5.153800228976328057, -19.02544592524343514, 42.29057627198101699 ) ) ;
#62826=CARTESIAN_POINT ( 'NONE',  ( -5.049401038297874678, -19.05341960407617918, 64.79275706135233293 ) ) ;
#62827=CARTESIAN_POINT ( 'NONE',  ( 0.05219959533910956823, 16.53943276465976808, 29.99890960531435979 ) ) ;
#62828=CARTESIAN_POINT ( 'NONE',  ( -21.55341960407619339, 5.719274019375674811, 98.54275706135234714 ) ) ;
#62829=CARTESIAN_POINT ( 'NONE',  ( 9.474510206698971260, -16.51473224551069308, 87.91557627198102409 ) ) ;
#62830=CARTESIAN_POINT ( 'NONE',  ( -5.153800228976607833, 19.02544592524334988, 67.70942372801900433 ) ) ;
#62831=CARTESIAN_POINT ( 'NONE',  ( -10.81492255796078084, -18.62759615963271287, 67.08224293864770971 ) ) ;
#62832=CARTESIAN_POINT ( 'NONE',  ( -15.72974639402176322, -15.80617190586768395, 19.37609039468568639 ) ) ;
#62833=CARTESIAN_POINT ( 'NONE',  ( 16.51473224551083163, -9.474510206698727899, 105.8344237280190043 ) ) ;
#62834=CARTESIAN_POINT ( 'NONE',  ( 4.483927247898790824, -16.52544592524335698, 85.20942372801901854 ) ) ;
#62835=LINE ( 'NONE', #124519, #116020 ) ;
#62836=CARTESIAN_POINT ( 'NONE',  ( -15.72974639402176322, -15.80617190586768395, 24.37609039468567573 ) ) ;
#62837=CARTESIAN_POINT ( 'NONE',  ( 4.483927247898545687, 16.52544592524342804, 99.79057627198103830 ) ) ;
#62839=CARTESIAN_POINT ( 'NONE',  ( -4.379528057220086978, -16.55341960407618274, 54.79275706135235424 ) ) ;
#62840=CARTESIAN_POINT ( 'NONE',  ( -21.55341960407610458, -5.719274019375992779, 61.45724293864770260 ) ) ;
#62841=CARTESIAN_POINT ( 'NONE',  ( -4.483927247898782831, 16.52544592524335698, 107.7094237280190328 ) ) ;
#62842=CARTESIAN_POINT ( 'NONE',  ( 4.379528057220092307, 16.55341960407617563, 37.29275706135235424 ) ) ;
#62843=CARTESIAN_POINT ( 'NONE',  ( -16.46253265017160317, 9.564922557960807481, 25.83224293864769194 ) ) ;
#62844=CARTESIAN_POINT ( 'NONE',  ( -12.06949235617739369, -12.14591786802326823, 79.37609039468567573 ) ) ;
#62845=CARTESIAN_POINT ( 'NONE',  ( 9.564922557961047289, -16.46253265017146816, 70.41775706135233293 ) ) ;
#62846=CARTESIAN_POINT ( 'NONE',  ( 0.05219959533907565091, 21.53943276465977519, 74.99890960531435269 ) ) ;
#62847=CARTESIAN_POINT ( 'NONE',  ( 8.224510206698742110, 14.34966873604972548, 102.0844237280190185 ) ) ;
#62848=CARTESIAN_POINT ( 'NONE',  ( -5.719274019375665041, -21.55341960407619695, 79.79275706135236135 ) ) ;
#62851=CARTESIAN_POINT ( 'NONE',  ( 18.67979575497178502, 10.72451020669898547, 64.16557627198102409 ) ) ;
#62852=CARTESIAN_POINT ( 'NONE',  ( -15.72974639402197994, 15.80617190586746368, 50.62390960531435979 ) ) ;
#62853=ORIENTED_EDGE ( 'NONE', *, *, #38977, .T. ) ;
#62854=CARTESIAN_POINT ( 'NONE',  ( 8.314922557961029526, -14.29746914071037800, 80.41775706135234714 ) ) ;
#62855=CARTESIAN_POINT ( 'NONE',  ( 21.55341960407610458, 5.719274019375980345, 43.95724293864769550 ) ) ;
#62857=CARTESIAN_POINT ( 'NONE',  ( 5.719274019375991003, -21.55341960407610458, 22.70724293864769194 ) ) ;
#62859=CARTESIAN_POINT ( 'NONE',  ( 13.89961937509977652, -13.97604488694527269, 28.12390960531435624 ) ) ;
#62860=CARTESIAN_POINT ( 'NONE',  ( -15.80617190586745835, -15.72974639402198527, 71.87390960531438111 ) ) ;
#62861=CARTESIAN_POINT ( 'NONE',  ( 16.53943276465976808, 0.05219959533934440121, 101.2510903946856757 ) ) ;
#62862=CARTESIAN_POINT ( 'NONE',  ( -18.62759615963255300, -10.81492255796106328, 49.16775706135234003 ) ) ;
#62863=CARTESIAN_POINT ( 'NONE',  ( -16.46253265017146816, -9.564922557961047289, 104.1677570613523329 ) ) ;
#62864=CARTESIAN_POINT ( 'NONE',  ( -8.314922557960811034, -14.29746914071050412, 112.0822429386477097 ) ) ;
#62865=CARTESIAN_POINT ( 'NONE',  ( -19.02544592524334988, -5.153800228976617603, 108.9594237280189759 ) ) ;
#62866=CARTESIAN_POINT ( 'NONE',  ( 13.97604488694527802, 13.89961937509977652, 44.37390960531435269 ) ) ;
#62868=CARTESIAN_POINT ( 'NONE',  ( 5.049401038298161559, -19.05341960407611168, 92.70724293864769550 ) ) ;
#62870=CARTESIAN_POINT ( 'NONE',  ( -8.224510206698735004, -14.34966873604973081, 69.58442372801900433 ) ) ;
#62871=CARTESIAN_POINT ( 'NONE',  ( 5.049401038297881783, 19.05341960407617563, 82.29275706135229029 ) ) ;
#62872=CARTESIAN_POINT ( 'NONE',  ( -5.049401038297874678, -19.05341960407617918, 29.79275706135232227 ) ) ;
#62873=CARTESIAN_POINT ( 'NONE',  ( 21.52544592524344225, -5.823673210054117533, 58.54057627198103120 ) ) ;
#62874=CARTESIAN_POINT ( 'NONE',  ( 12.06949235617739724, 12.14591786802326823, 86.87609039468568994 ) ) ;
#62875=CARTESIAN_POINT ( 'NONE',  ( 19.03943276465977164, 0.05219959533936151252, 81.25109039468567573 ) ) ;
#62876=CARTESIAN_POINT ( 'NONE',  ( -5.049401038298153566, 19.05341960407611168, 35.20724293864768839 ) ) ;
#62877=CARTESIAN_POINT ( 'NONE',  ( 16.51473224551069308, 9.474510206698969483, 84.16557627198102409 ) ) ;
#62879=CARTESIAN_POINT ( 'NONE',  ( -18.62759615963255300, -10.81492255796106328, 49.16775706135234003 ) ) ;
#62880=CARTESIAN_POINT ( 'NONE',  ( 19.03943276465977164, -0.05219959533909143690, 53.74890960531436690 ) ) ;
#62882=CARTESIAN_POINT ( 'NONE',  ( -16.51473224551069308, -9.474510206698971260, 111.6655762719810383 ) ) ;
#62883=CARTESIAN_POINT ( 'NONE',  ( -4.483927247898539470, -16.52544592524342804, 67.29057627198103830 ) ) ;
#62884=CARTESIAN_POINT ( 'NONE',  ( 5.823673210054125526, 21.52544592524343514, 54.79057627198104541 ) ) ;
#62885=CARTESIAN_POINT ( 'NONE',  ( 18.22780087662122739, 5.500000000000000888, 81.48236817873103632 ) ) ;
#62887=CARTESIAN_POINT ( 'NONE',  ( -9.564922557961040184, 16.46253265017147172, 47.91775706135233293 ) ) ;
#62889=CARTESIAN_POINT ( 'NONE',  ( 13.89961937509977652, -13.97604488694527269, 58.12390960531436690 ) ) ;
#62890=CARTESIAN_POINT ( 'NONE',  ( -19.03943276465977164, 0.05219959533909376836, 71.24890960531435269 ) ) ;
#62891=CARTESIAN_POINT ( 'NONE',  ( -14.34966873604972548, 8.224510206698743886, 48.33442372801902565 ) ) ;
#62893=CARTESIAN_POINT ( 'NONE',  ( -16.55341960407617563, 4.379528057220093196, 83.54275706135234714 ) ) ;
#62895=CARTESIAN_POINT ( 'NONE',  ( 0.05219959533934541429, -16.53943276465976808, 80.00109039468568994 ) ) ;
#62897=CARTESIAN_POINT ( 'NONE',  ( 4.483927247898790824, -16.52544592524335698, 50.20942372801901854 ) ) ;
#62898=CARTESIAN_POINT ( 'NONE',  ( 0.05219959533936267826, -19.03943276465977164, 30.00109039468566863 ) ) ;
#62899=CARTESIAN_POINT ( 'NONE',  ( 19.05341960407611168, 5.049401038298154454, 58.95724293864768129 ) ) ;
#62901=CARTESIAN_POINT ( 'NONE',  ( 21.52544592524334988, 5.823673210054432836, 51.45942372801901854 ) ) ;
#62902=CARTESIAN_POINT ( 'NONE',  ( 5.049401038297881783, 19.05341960407617563, 62.29275706135234003 ) ) ;
#62903=CARTESIAN_POINT ( 'NONE',  ( -10.72451020669870658, -18.67979575497194134, 104.5844237280190185 ) ) ;
#62904=CARTESIAN_POINT ( 'NONE',  ( 9.564922557960805705, 16.46253265017160317, 34.58224293864770260 ) ) ;
#62906=CARTESIAN_POINT ( 'NONE',  ( -21.53943276465977519, 0.05219959533907696930, 71.24890960531435269 ) ) ;
#62908=CARTESIAN_POINT ( 'NONE',  ( -0.05219959533907301413, -21.53943276465977519, 22.49890960531436335 ) ) ;
#62909=CARTESIAN_POINT ( 'NONE',  ( -4.483927247898539470, -16.52544592524342804, 107.2905762719810525 ) ) ;
#62910=CARTESIAN_POINT ( 'NONE',  ( 0.05219959533934541429, -16.53943276465976808, 35.00109039468568284 ) ) ;
#62911=CARTESIAN_POINT ( 'NONE',  ( -16.52544592524342804, 4.483927247898546575, 36.04057627198102409 ) ) ;
#62913=CARTESIAN_POINT ( 'NONE',  ( 21.53943276465977519, 0.05219959533937863772, 21.25109039468567218 ) ) ;
#62914=CARTESIAN_POINT ( 'NONE',  ( 14.29746914071049879, -8.314922557960816363, 38.33224293864768839 ) ) ;
#62916=CARTESIAN_POINT ( 'NONE',  ( 9.474510206698729675, 16.51473224551082808, 107.0844237280190043 ) ) ;
#62917=CARTESIAN_POINT ( 'NONE',  ( 5.153800228976615827, -19.02544592524334988, 30.20942372801900433 ) ) ;
#62918=CARTESIAN_POINT ( 'NONE',  ( 12.14591786802309770, 12.06949235617756955, 29.37390960531435269 ) ) ;
#62919=CARTESIAN_POINT ( 'NONE',  ( -18.67979575497178146, -10.72451020669898902, 96.66557627198102409 ) ) ;
#62920=CARTESIAN_POINT ( 'NONE',  ( 17.31728774477272381, 6.344390552232406222, 31.68093348310680568 ) ) ;
#62921=CARTESIAN_POINT ( 'NONE',  ( -15.80617190586745835, -15.72974639402198527, 61.87390960531436690 ) ) ;
#62922=CARTESIAN_POINT ( 'NONE',  ( -16.51473224551069308, -9.474510206698971260, 71.66557627198102409 ) ) ;
#62923=CARTESIAN_POINT ( 'NONE',  ( -12.14591786802309592, -12.06949235617757132, 46.87390960531435979 ) ) ;
#62924=CARTESIAN_POINT ( 'NONE',  ( 9.564922557960805705, 16.46253265017160317, 89.58224293864769550 ) ) ;
#62926=CARTESIAN_POINT ( 'NONE',  ( 9.474510206698729675, 16.51473224551082808, 57.08442372801900433 ) ) ;
#62927=CARTESIAN_POINT ( 'NONE',  ( 5.823673210054125526, 21.52544592524343514, 94.79057627198105251 ) ) ;
#62928=CARTESIAN_POINT ( 'NONE',  ( -16.52544592524342804, 4.483927247898546575, 96.04057627198102409 ) ) ;
#62929=CARTESIAN_POINT ( 'NONE',  ( 18.67979575497194134, -10.72451020669871369, 40.83442372801901854 ) ) ;
#62931=CARTESIAN_POINT ( 'NONE',  ( -0.05219959533910754901, -16.53943276465976808, 27.49890960531435269 ) ) ;
#62932=CARTESIAN_POINT ( 'NONE',  ( 19.03943276465977164, -0.05219959533909143690, 38.74890960531436690 ) ) ;
#62933=CARTESIAN_POINT ( 'NONE',  ( -19.02544592524342804, 5.153800228976336051, 96.04057627198103830 ) ) ;
#62934=CARTESIAN_POINT ( 'NONE',  ( -21.52544592524343514, 5.823673210054127303, 66.04057627198103830 ) ) ;
#62935=CARTESIAN_POINT ( 'NONE',  ( -18.87580814761071935, 5.500000000000041744, 45.87172394265761710 ) ) ;
#62936=CARTESIAN_POINT ( 'NONE',  ( 9.474510206698971260, -16.51473224551069308, 27.91557627198103120 ) ) ;
#62937=CARTESIAN_POINT ( 'NONE',  ( -18.62759615963270932, 10.81492255796079327, 55.83224293864770260 ) ) ;
#62938=CARTESIAN_POINT ( 'NONE',  ( 0.05219959533937995610, -21.53943276465977519, 70.00109039468568994 ) ) ;
#62940=CARTESIAN_POINT ( 'NONE',  ( 14.29746914071037800, 8.314922557961029526, 71.66775706135234714 ) ) ;
#62941=CARTESIAN_POINT ( 'NONE',  ( -0.05219959533909027116, -19.03943276465977164, 62.49890960531435979 ) ) ;
#62942=CARTESIAN_POINT ( 'NONE',  ( 16.51473224551069308, 9.474510206698969483, 59.16557627198102409 ) ) ;
#62944=CARTESIAN_POINT ( 'NONE',  ( 16.46253265017146816, 9.564922557961045513, 21.66775706135233648 ) ) ;
#62945=CARTESIAN_POINT ( 'NONE',  ( -12.14591786802326823, 12.06949235617739902, 78.12609039468570415 ) ) ;
#62946=CARTESIAN_POINT ( 'NONE',  ( -21.52544592524334988, -5.823673210054445271, 93.95942372801903275 ) ) ;
#62947=CARTESIAN_POINT ( 'NONE',  ( -16.51473224551069308, -9.474510206698971260, 71.66557627198102409 ) ) ;
#62948=CARTESIAN_POINT ( 'NONE',  ( -5.719274019375978568, 21.55341960407610458, 40.20724293864769550 ) ) ;
#62949=CARTESIAN_POINT ( 'NONE',  ( 19.03943276465977164, 0.05219959533936151252, 106.2510903946856615 ) ) ;
#62950=CARTESIAN_POINT ( 'NONE',  ( 18.62759615963255655, 10.81492255796105972, 76.66775706135234714 ) ) ;
#62951=CARTESIAN_POINT ( 'NONE',  ( -16.53943276465976808, -0.05219959533934237506, 53.75109039468568994 ) ) ;
#62952=CARTESIAN_POINT ( 'NONE',  ( 18.67979575497178502, 10.72451020669898547, 94.16557627198103830 ) ) ;
#62953=CARTESIAN_POINT ( 'NONE',  ( 13.89961937509957401, 13.97604488694547697, 111.8760903946856757 ) ) ;
#62954=CARTESIAN_POINT ( 'NONE',  ( 19.03943276465977164, -0.05219959533909143690, 78.74890960531436690 ) ) ;
#62955=CARTESIAN_POINT ( 'NONE',  ( 8.314922557961029526, -14.29746914071037800, 20.41775706135234714 ) ) ;
#62956=CARTESIAN_POINT ( 'NONE',  ( -19.05341960407611168, -5.049401038298163336, 41.45724293864769550 ) ) ;
#62957=CARTESIAN_POINT ( 'NONE',  ( -13.89961937509957401, -13.97604488694547875, 109.3760903946856331 ) ) ;
#62958=CARTESIAN_POINT ( 'NONE',  ( 14.34966873604960469, 8.224510206698951720, 69.16557627198102409 ) ) ;
#62959=CARTESIAN_POINT ( 'NONE',  ( 14.34966873604972726, -8.224510206698740333, 70.83442372801901854 ) ) ;
#62960=CARTESIAN_POINT ( 'NONE',  ( 15.72974639402176855, 15.80617190586768217, 26.87609039468567218 ) ) ;
#62961=CARTESIAN_POINT ( 'NONE',  ( -19.02544592524342804, 5.153800228976336051, 56.04057627198100988 ) ) ;
#62962=CARTESIAN_POINT ( 'NONE',  ( -5.049401038298153566, 19.05341960407611168, 65.20724293864765286 ) ) ;
#62963=CARTESIAN_POINT ( 'NONE',  ( -14.34966873604972548, 8.224510206698743886, 73.33442372801901854 ) ) ;
#62965=CARTESIAN_POINT ( 'NONE',  ( -18.22780087662123094, -5.499999999999984901, 81.48459894673892734 ) ) ;
#62968=CARTESIAN_POINT ( 'NONE',  ( 13.97604488694548053, -13.89961937509957401, 20.62609039468567573 ) ) ;
#62969=CARTESIAN_POINT ( 'NONE',  ( 9.564922557960805705, 16.46253265017160317, 39.58224293864768839 ) ) ;
#62970=FACE_OUTER_BOUND ( 'NONE', #21958, .T. ) ;
#62972=CARTESIAN_POINT ( 'NONE',  ( -12.06949235617739369, -12.14591786802326823, 29.37609039468568284 ) ) ;
#62973=CARTESIAN_POINT ( 'NONE',  ( -9.474510206698720793, -16.51473224551083518, 54.58442372801899722 ) ) ;
#62974=CARTESIAN_POINT ( 'NONE',  ( 4.379528057220092307, 16.55341960407617563, 42.29275706135235424 ) ) ;
#62975=CARTESIAN_POINT ( 'NONE',  ( 16.46253265017160672, -9.564922557960803928, 43.33224293864769550 ) ) ;
#62976=CARTESIAN_POINT ( 'NONE',  ( -19.03943276465977164, 0.05219959533909376836, 106.2489096053143669 ) ) ;
#62977=CARTESIAN_POINT ( 'NONE',  ( 19.05341960407611168, 5.049401038298154454, 58.95724293864768129 ) ) ;
#62978=CARTESIAN_POINT ( 'NONE',  ( 21.53943276465977519, -0.05219959533907433946, 93.74890960531436690 ) ) ;
#62979=CARTESIAN_POINT ( 'NONE',  ( -9.474510206698964154, 16.51473224551069663, 95.41557627198102409 ) ) ;
#62980=CARTESIAN_POINT ( 'NONE',  ( -5.049401038298153566, 19.05341960407611168, 25.20724293864768484 ) ) ;
#62981=EDGE_CURVE ( 'NONE', #68796, #89992, #73811, .T. ) ;
#62982=CARTESIAN_POINT ( 'NONE',  ( -0.05219959533909027116, -19.03943276465977164, 62.49890960531435979 ) ) ;
#62983=CARTESIAN_POINT ( 'NONE',  ( -4.483927247898782831, 16.52544592524335698, 112.7094237280190328 ) ) ;
#62985=CARTESIAN_POINT ( 'NONE',  ( 19.05341960407617918, -5.049401038297876454, 96.04275706135231871 ) ) ;
#62986=CARTESIAN_POINT ( 'NONE',  ( 19.03943276465977164, 0.05219959533936151252, 26.25109039468566507 ) ) ;
#62988=CARTESIAN_POINT ( 'NONE',  ( -8.224510206698948167, 14.34966873604960824, 55.41557627198102409 ) ) ;
#62989=CARTESIAN_POINT ( 'NONE',  ( 5.823673210054444382, -21.52544592524334988, 95.20942372801903275 ) ) ;
#62990=CARTESIAN_POINT ( 'NONE',  ( -16.46253265017160317, 9.564922557960807481, 45.83224293864769550 ) ) ;
#62991=CARTESIAN_POINT ( 'NONE',  ( 4.379528057220339221, -16.55341960407611168, 22.70724293864769194 ) ) ;
#62992=CARTESIAN_POINT ( 'NONE',  ( -18.62759615963255300, -10.81492255796106328, 84.16775706135234714 ) ) ;
#62993=CARTESIAN_POINT ( 'NONE',  ( 16.46253265017160672, -9.564922557960803928, 83.33224293864768129 ) ) ;
#62994=CARTESIAN_POINT ( 'NONE',  ( -0.05219959533909027116, -19.03943276465977164, 92.49890960531436690 ) ) ;
#62995=CARTESIAN_POINT ( 'NONE',  ( 12.14591786802309770, 12.06949235617756955, 89.37390960531435269 ) ) ;
#62996=CARTESIAN_POINT ( 'NONE',  ( -16.55341960407611168, -4.379528057220339221, 71.45724293864769550 ) ) ;
#62997=CARTESIAN_POINT ( 'NONE',  ( 0.05219959533907565091, 21.53943276465977519, 79.99890960531435269 ) ) ;
#62998=CARTESIAN_POINT ( 'NONE',  ( -19.05341960407611168, -5.049401038298163336, 76.45724293864769550 ) ) ;
#62999=CARTESIAN_POINT ( 'NONE',  ( 21.55341960407610458, 5.719274019375980345, 78.95724293864769550 ) ) ;
#63001=CARTESIAN_POINT ( 'NONE',  ( -16.46253265017146816, -9.564922557961047289, 84.16775706135233293 ) ) ;
#63002=CARTESIAN_POINT ( 'NONE',  ( -17.49999999999999645, -5.500000000000000888, 120.0000000000000142 ) ) ;
#63003=CARTESIAN_POINT ( 'NONE',  ( -16.52544592524342804, 4.483927247898546575, 96.04057627198102409 ) ) ;
#63004=CARTESIAN_POINT ( 'NONE',  ( -0.05219959533909027116, -19.03943276465977164, 62.49890960531435979 ) ) ;
#63005=CARTESIAN_POINT ( 'NONE',  ( -10.81492255796078084, -18.62759615963271287, 62.08224293864769550 ) ) ;
#63007=CARTESIAN_POINT ( 'NONE',  ( 16.53943276465976808, 0.05219959533934440121, 111.2510903946856899 ) ) ;
#63009=CARTESIAN_POINT ( 'NONE',  ( 5.153800228976615827, -19.02544592524334988, 110.2094237280189901 ) ) ;
#63010=CARTESIAN_POINT ( 'NONE',  ( -16.55341960407611168, -4.379528057220339221, 86.45724293864770971 ) ) ;
#63012=CARTESIAN_POINT ( 'NONE',  ( -9.564922557960796823, -16.46253265017161027, 72.08224293864770971 ) ) ;
#63013=CARTESIAN_POINT ( 'NONE',  ( 0.05219959533909260263, 19.03943276465977164, 34.99890960531435979 ) ) ;
#63014=CARTESIAN_POINT ( 'NONE',  ( -16.53943276465976808, 0.05219959533911058130, 71.24890960531435269 ) ) ;
#63015=CARTESIAN_POINT ( 'NONE',  ( -13.89961937509977652, 13.97604488694528158, 100.6239096053143669 ) ) ;
#63016=CARTESIAN_POINT ( 'NONE',  ( -5.049401038297874678, -19.05341960407617918, 94.79275706135230450 ) ) ;
#63017=CARTESIAN_POINT ( 'NONE',  ( 5.153800228976335163, 19.02544592524342804, 79.79057627198102409 ) ) ;
#63018=CARTESIAN_POINT ( 'NONE',  ( 16.51473224551069308, 9.474510206698969483, 89.16557627198103830 ) ) ;
#63019=CARTESIAN_POINT ( 'NONE',  ( -5.719274019375978568, 21.55341960407610458, 75.20724293864769550 ) ) ;
#63020=CARTESIAN_POINT ( 'NONE',  ( -16.53943276465976808, -0.05219959533934237506, 68.75109039468568994 ) ) ;
#63022=CARTESIAN_POINT ( 'NONE',  ( -16.31925111598408051, 7.325300261831769078, 95.16424538967171998 ) ) ;
#63023=CARTESIAN_POINT ( 'NONE',  ( -13.97604488694527625, -13.89961937509977652, 61.87390960531435979 ) ) ;
#63024=CARTESIAN_POINT ( 'NONE',  ( 5.823673210054125526, 21.52544592524343514, 69.79057627198102409 ) ) ;
#63025=CARTESIAN_POINT ( 'NONE',  ( 13.97604488694548053, -13.89961937509957401, 100.6260903946856615 ) ) ;
#63026=CARTESIAN_POINT ( 'NONE',  ( -12.14591786802309592, -12.06949235617757132, 31.87390960531435979 ) ) ;
#63027=CARTESIAN_POINT ( 'NONE',  ( -10.81492255796105439, 18.62759615963255655, 42.91775706135235424 ) ) ;
#63029=CARTESIAN_POINT ( 'NONE',  ( 8.314922557961029526, -14.29746914071037800, 70.41775706135236135 ) ) ;
#63030=CARTESIAN_POINT ( 'NONE',  ( -9.474510206698964154, 16.51473224551069663, 100.4155762719810241 ) ) ;
#63031=CARTESIAN_POINT ( 'NONE',  ( 19.02544592524343514, -5.153800228976328945, 108.5405762719810383 ) ) ;
#63032=CARTESIAN_POINT ( 'NONE',  ( 12.14591786802327356, -12.06949235617739191, 90.62609039468567573 ) ) ;
#63033=CARTESIAN_POINT ( 'NONE',  ( -4.379528057220086978, -16.55341960407618274, 44.79275706135234714 ) ) ;
#63034=CARTESIAN_POINT ( 'NONE',  ( 9.564922557960805705, 16.46253265017160317, 59.58224293864769550 ) ) ;
#63035=CARTESIAN_POINT ( 'NONE',  ( 0.05219959533909260263, 19.03943276465977164, 64.99890960531436690 ) ) ;
#63036=CARTESIAN_POINT ( 'NONE',  ( 21.52544592524334988, 5.823673210054432836, 51.45942372801901854 ) ) ;
#63037=CARTESIAN_POINT ( 'NONE',  ( 4.379528057220092307, 16.55341960407617563, 67.29275706135234714 ) ) ;
#63038=CARTESIAN_POINT ( 'NONE',  ( 16.55341960407611168, 4.379528057220329451, 28.95724293864769905 ) ) ;
#63039=CARTESIAN_POINT ( 'NONE',  ( -5.049401038298153566, 19.05341960407611168, 35.20724293864768839 ) ) ;
#63040=CARTESIAN_POINT ( 'NONE',  ( 16.46253265017160672, -9.564922557960803928, 28.33224293864769550 ) ) ;
#63041=CARTESIAN_POINT ( 'NONE',  ( 12.06949235617739724, 12.14591786802326823, 21.87609039468567573 ) ) ;
#63042=CARTESIAN_POINT ( 'NONE',  ( 9.474510206698729675, 16.51473224551082808, 87.08442372801900433 ) ) ;
#63043=CARTESIAN_POINT ( 'NONE',  ( -14.29746914071049879, 8.314922557960819915, 80.83224293864769550 ) ) ;
#63044=CARTESIAN_POINT ( 'NONE',  ( -5.153800228976328057, -19.02544592524343514, 52.29057627198100988 ) ) ;
#63045=CARTESIAN_POINT ( 'NONE',  ( -19.05341960407617563, 5.049401038297882671, 88.54275706135230450 ) ) ;
#63047=CARTESIAN_POINT ( 'NONE',  ( 0.05219959533937995610, -21.53943276465977519, 90.00109039468567573 ) ) ;
#63048=CARTESIAN_POINT ( 'NONE',  ( 14.29746914071037800, 8.314922557961029526, 51.66775706135234714 ) ) ;
#63050=CARTESIAN_POINT ( 'NONE',  ( -18.67979575497178146, -10.72451020669898902, 46.66557627198102409 ) ) ;
#63051=CARTESIAN_POINT ( 'NONE',  ( -12.06949235617739369, -12.14591786802326823, 44.37609039468567573 ) ) ;
#63052=CARTESIAN_POINT ( 'NONE',  ( 9.474510206698971260, -16.51473224551069308, 37.91557627198102409 ) ) ;
#63053=CARTESIAN_POINT ( 'NONE',  ( 13.89961937509957401, 13.97604488694547697, 31.87609039468566863 ) ) ;
#63054=CARTESIAN_POINT ( 'NONE',  ( -0.05219959533909027116, -19.03943276465977164, 72.49890960531435269 ) ) ;
#63056=CARTESIAN_POINT ( 'NONE',  ( -5.049401038298153566, 19.05341960407611168, 55.20724293864769550 ) ) ;
#63057=CARTESIAN_POINT ( 'NONE',  ( -17.49999999999999645, 5.499999999999997335, 120.0000000000000142 ) ) ;
#63058=CARTESIAN_POINT ( 'NONE',  ( 13.97604488694527802, 13.89961937509977652, 69.37390960531436690 ) ) ;
#63059=CARTESIAN_POINT ( 'NONE',  ( -18.89770734986051082, -5.499999999999912959, 54.10214472496640070 ) ) ;
#63061=EDGE_CURVE ( 'NONE', #3830, #179309, #134724, .T. ) ;
#63062=CARTESIAN_POINT ( 'NONE',  ( 9.474510206698729675, 16.51473224551082808, 37.08442372801899722 ) ) ;
#63063=CARTESIAN_POINT ( 'NONE',  ( -5.719274019375665041, -21.55341960407619695, 104.7927570613523898 ) ) ;
#63064=CARTESIAN_POINT ( 'NONE',  ( 14.29746914071049879, -8.314922557960816363, 38.33224293864768839 ) ) ;
#63065=CARTESIAN_POINT ( 'NONE',  ( -16.51473224551069308, -9.474510206698971260, 46.66557627198102409 ) ) ;
#63066=CARTESIAN_POINT ( 'NONE',  ( 5.153800228976335163, 19.02544592524342804, 104.7905762719809957 ) ) ;
#63067=CARTESIAN_POINT ( 'NONE',  ( 5.823673210054444382, -21.52544592524334988, 75.20942372801901854 ) ) ;
#63068=CARTESIAN_POINT ( 'NONE',  ( -13.89961937509977652, 13.97604488694528158, 50.62390960531435979 ) ) ;
#63069=CARTESIAN_POINT ( 'NONE',  ( 5.823673210054444382, -21.52544592524334988, 85.20942372801901854 ) ) ;
#63070=CARTESIAN_POINT ( 'NONE',  ( 0.05219959533907565091, 21.53943276465977519, 29.99890960531435979 ) ) ;
#63071=CARTESIAN_POINT ( 'NONE',  ( 16.46253265017160672, -9.564922557960803928, 33.33224293864770260 ) ) ;
#63072=CARTESIAN_POINT ( 'NONE',  ( -21.52544592524334988, -5.823673210054445271, 28.95942372801902209 ) ) ;
#63073=CARTESIAN_POINT ( 'NONE',  ( -9.474510206698720793, -16.51473224551083518, 54.58442372801899722 ) ) ;
#63074=CARTESIAN_POINT ( 'NONE',  ( 19.03943276465977164, -0.05219959533909143690, 28.74890960531435624 ) ) ;
#63075=CARTESIAN_POINT ( 'NONE',  ( -13.89961937509977652, 13.97604488694528158, 75.62390960531438111 ) ) ;
#63076=CARTESIAN_POINT ( 'NONE',  ( -16.46253265017146816, -9.564922557961047289, 109.1677570613523471 ) ) ;
#63077=CARTESIAN_POINT ( 'NONE',  ( 4.483927247898545687, 16.52544592524342804, 74.79057627198105251 ) ) ;
#63078=CARTESIAN_POINT ( 'NONE',  ( -5.719274019375978568, 21.55341960407610458, 40.20724293864769550 ) ) ;
#63079=CARTESIAN_POINT ( 'NONE',  ( 9.474510206698729675, 16.51473224551082808, 107.0844237280190043 ) ) ;
#63080=CARTESIAN_POINT ( 'NONE',  ( 15.80617190586746368, 15.72974639402197994, 99.37390960531436690 ) ) ;
#63081=CARTESIAN_POINT ( 'NONE',  ( -21.52544592524334988, -5.823673210054445271, 63.95942372801901854 ) ) ;
#63082=CARTESIAN_POINT ( 'NONE',  ( 12.06949235617739724, 12.14591786802326823, 51.87609039468568284 ) ) ;
#63083=CARTESIAN_POINT ( 'NONE',  ( -4.379528057220086978, -16.55341960407618274, 54.79275706135235424 ) ) ;
#63084=CARTESIAN_POINT ( 'NONE',  ( 9.564922557960805705, 16.46253265017160317, 54.58224293864769550 ) ) ;
#63085=CARTESIAN_POINT ( 'NONE',  ( -14.34966873604972548, 8.224510206698743886, 83.33442372801903275 ) ) ;
#63086=CARTESIAN_POINT ( 'NONE',  ( -15.72974639402197994, 15.80617190586746368, 110.6239096053143669 ) ) ;
#63087=CARTESIAN_POINT ( 'NONE',  ( -16.55341960407611168, -4.379528057220339221, 56.45724293864768839 ) ) ;
#63088=CARTESIAN_POINT ( 'NONE',  ( 16.51473224551069308, 9.474510206698969483, 84.16557627198102409 ) ) ;
#63089=CARTESIAN_POINT ( 'NONE',  ( 16.53943276465976808, 0.05219959533934440121, 81.25109039468568994 ) ) ;
#63090=CARTESIAN_POINT ( 'NONE',  ( 18.67979575497194134, -10.72451020669871369, 45.83442372801901854 ) ) ;
#63091=CARTESIAN_POINT ( 'NONE',  ( 5.049401038297881783, 19.05341960407617563, 107.2927570613523187 ) ) ;
#63092=CARTESIAN_POINT ( 'NONE',  ( 15.80617190586746368, 15.72974639402197994, 109.3739096053143811 ) ) ;
#63093=CARTESIAN_POINT ( 'NONE',  ( 16.55341960407611168, 4.379528057220329451, 48.95724293864770971 ) ) ;
#63094=ORIENTED_EDGE ( 'NONE', *, *, #90349, .F. ) ;
#63095=CARTESIAN_POINT ( 'NONE',  ( -16.52216118717208815, 7.221426719304501418, 68.92400978953010338 ) ) ;
#63096=CARTESIAN_POINT ( 'NONE',  ( 21.55341960407610458, 5.719274019375980345, 93.95724293864770971 ) ) ;
#63097=CARTESIAN_POINT ( 'NONE',  ( -0.05219959533934338120, 16.53943276465976808, 112.5010903946857042 ) ) ;
#63099=CARTESIAN_POINT ( 'NONE',  ( -17.44270441346512968, -5.991230190323104665, 56.36335079264227943 ) ) ;
#63100=CARTESIAN_POINT ( 'NONE',  ( 10.72451020669871369, 18.67979575497193778, 22.08442372801901143 ) ) ;
#63102=CARTESIAN_POINT ( 'NONE',  ( -5.153800228976328057, -19.02544592524343514, 112.2905762719810099 ) ) ;
#63103=CARTESIAN_POINT ( 'NONE',  ( -0.05219959533937732626, 21.53943276465977519, 22.50109039468567573 ) ) ;
#63104=CARTESIAN_POINT ( 'NONE',  ( -4.379528057220328563, 16.55341960407611168, 55.20724293864770260 ) ) ;
#63105=CARTESIAN_POINT ( 'NONE',  ( -8.224510206698735004, -14.34966873604973081, 64.58442372801900433 ) ) ;
#63106=CARTESIAN_POINT ( 'NONE',  ( -5.153800228976328057, -19.02544592524343514, 67.29057627198102409 ) ) ;
#63107=CARTESIAN_POINT ( 'NONE',  ( 9.564922557961047289, -16.46253265017146816, 65.41775706135233293 ) ) ;
#63108=CARTESIAN_POINT ( 'NONE',  ( 16.51473224551069308, 9.474510206698969483, 74.16557627198103830 ) ) ;
#63109=CARTESIAN_POINT ( 'NONE',  ( -5.719274019375978568, 21.55341960407610458, 30.20724293864769550 ) ) ;
#63111=CARTESIAN_POINT ( 'NONE',  ( 19.02544592524343514, -5.153800228976328945, 48.54057627198103120 ) ) ;
#63112=CARTESIAN_POINT ( 'NONE',  ( 16.55341960407618274, -4.379528057220086978, 21.04275706135234714 ) ) ;
#63113=CARTESIAN_POINT ( 'NONE',  ( -16.46253265017146816, -9.564922557961047289, 59.16775706135233293 ) ) ;
#63114=CARTESIAN_POINT ( 'NONE',  ( 5.719274019375991003, -21.55341960407610458, 102.7072429386476955 ) ) ;
#63115=CARTESIAN_POINT ( 'NONE',  ( 4.483927247898545687, 16.52544592524342804, 34.79057627198103120 ) ) ;
#63116=CARTESIAN_POINT ( 'NONE',  ( -5.049401038298153566, 19.05341960407611168, 95.20724293864770971 ) ) ;
#63117=CARTESIAN_POINT ( 'NONE',  ( -21.52544592524343514, 5.823673210054127303, 61.04057627198103120 ) ) ;
#63118=CARTESIAN_POINT ( 'NONE',  ( 21.55341960407610458, 5.719274019375980345, 88.95724293864769550 ) ) ;
#63119=CARTESIAN_POINT ( 'NONE',  ( 8.314922557961029526, -14.29746914071037800, 20.41775706135234714 ) ) ;
#63120=CARTESIAN_POINT ( 'NONE',  ( -15.72974639402197994, 15.80617190586746368, 30.62390960531436335 ) ) ;
#63121=CARTESIAN_POINT ( 'NONE',  ( 21.53943276465977519, 0.05219959533937863772, 91.25109039468568994 ) ) ;
#63122=CARTESIAN_POINT ( 'NONE',  ( 0.05219959533909260263, 19.03943276465977164, 89.99890960531436690 ) ) ;
#63123=CARTESIAN_POINT ( 'NONE',  ( -9.474510206698964154, 16.51473224551069663, 25.41557627198103120 ) ) ;
#63124=CARTESIAN_POINT ( 'NONE',  ( 16.46253265017160672, -9.564922557960803928, 83.33224293864768129 ) ) ;
#63125=CARTESIAN_POINT ( 'NONE',  ( 16.53943276465976808, -0.05219959533910856209, 103.7489096053143669 ) ) ;
#63126=CARTESIAN_POINT ( 'NONE',  ( -5.153800228976328057, -19.02544592524343514, 62.29057627198100988 ) ) ;
#63127=CARTESIAN_POINT ( 'NONE',  ( 8.224510206698742110, 14.34966873604972548, 22.08442372801901143 ) ) ;
#63128=CARTESIAN_POINT ( 'NONE',  ( 17.26058549869104652, -6.457015423128285470, 86.12254162523935008 ) ) ;
#63129=CARTESIAN_POINT ( 'NONE',  ( 21.55341960407619695, -5.719274019375665929, 96.04275706135236135 ) ) ;
#63130=CARTESIAN_POINT ( 'NONE',  ( 13.89961937509977652, -13.97604488694527269, 108.1239096053143669 ) ) ;
#63131=CARTESIAN_POINT ( 'NONE',  ( 0.05219959533934541429, -16.53943276465976808, 85.00109039468568994 ) ) ;
#63133=CARTESIAN_POINT ( 'NONE',  ( 13.97604488694548053, -13.89961937509957401, 70.62609039468567573 ) ) ;
#63134=CARTESIAN_POINT ( 'NONE',  ( 9.474510206698729675, 16.51473224551082808, 27.08442372801900433 ) ) ;
#63136=CARTESIAN_POINT ( 'NONE',  ( 16.51473224551069308, 9.474510206698969483, 29.16557627198103475 ) ) ;
#63137=CARTESIAN_POINT ( 'NONE',  ( 12.06949235617757843, -12.14591786802309237, 33.12390960531435979 ) ) ;
#63138=CARTESIAN_POINT ( 'NONE',  ( -17.31747979337946575, -6.344076630961068552, 111.3794486806518194 ) ) ;
#63139=CARTESIAN_POINT ( 'NONE',  ( 8.224510206698953496, -14.34966873604960469, 27.91557627198103830 ) ) ;
#63141=CARTESIAN_POINT ( 'NONE',  ( 16.55341960407618274, -4.379528057220086978, 101.0427570613523756 ) ) ;
#63142=CARTESIAN_POINT ( 'NONE',  ( 0.05219959533909260263, 19.03943276465977164, 39.99890960531436690 ) ) ;
#63143=CARTESIAN_POINT ( 'NONE',  ( 10.81492255796106328, -18.62759615963255655, 90.41775706135236135 ) ) ;
#63144=CARTESIAN_POINT ( 'NONE',  ( -16.51473224551082808, 9.474510206698731452, 98.33442372801900433 ) ) ;
#63145=CARTESIAN_POINT ( 'NONE',  ( -18.62759615963255300, -10.81492255796106328, 84.16775706135234714 ) ) ;
#63146=CARTESIAN_POINT ( 'NONE',  ( 9.564922557961047289, -16.46253265017146816, 50.41775706135233293 ) ) ;
#63147=CARTESIAN_POINT ( 'NONE',  ( 16.46253265017160672, -9.564922557960803928, 98.33224293864769550 ) ) ;
#63148=CARTESIAN_POINT ( 'NONE',  ( -0.05219959533909027116, -19.03943276465977164, 67.49890960531436690 ) ) ;
#63149=CARTESIAN_POINT ( 'NONE',  ( 17.49999999999999645, 5.500000000000007994, 73.78230962303568674 ) ) ;
#63150=AXIS2_PLACEMENT_3D ( 'NONE', #4034, #189090, #50563 ) ;
#63151=CARTESIAN_POINT ( 'NONE',  ( 4.379528057220339221, -16.55341960407611168, 72.70724293864769550 ) ) ;
#63152=CARTESIAN_POINT ( 'NONE',  ( 10.81492255796078972, 18.62759615963270932, 64.58224293864769550 ) ) ;
#63153=CARTESIAN_POINT ( 'NONE',  ( 16.51473224551069308, 9.474510206698969483, 64.16557627198102409 ) ) ;
#63154=CARTESIAN_POINT ( 'NONE',  ( -18.67979575497178146, -10.72451020669898902, 86.66557627198102409 ) ) ;
#63155=CARTESIAN_POINT ( 'NONE',  ( -14.34966873604972548, 8.224510206698743886, 73.33442372801901854 ) ) ;
#63157=CARTESIAN_POINT ( 'NONE',  ( 5.153800228976335163, 19.02544592524342804, 49.79057627198100988 ) ) ;
#63158=CARTESIAN_POINT ( 'NONE',  ( -12.06949235617756955, 12.14591786802309770, 85.62390960531436690 ) ) ;
#63160=CARTESIAN_POINT ( 'NONE',  ( -13.97604488694527625, -13.89961937509977652, 51.87390960531436690 ) ) ;
#63161=CARTESIAN_POINT ( 'NONE',  ( -14.29746914071049879, 8.314922557960819915, 115.8322429386477097 ) ) ;
#63162=CARTESIAN_POINT ( 'NONE',  ( -19.03943276465977164, -0.05219959533935918106, 68.75109039468566152 ) ) ;
#63163=CARTESIAN_POINT ( 'NONE',  ( 8.314922557960818139, 14.29746914071049879, 79.58224293864769550 ) ) ;
#63164=CARTESIAN_POINT ( 'NONE',  ( 0.05219959533937995610, -21.53943276465977519, 40.00109039468567573 ) ) ;
#63165=CARTESIAN_POINT ( 'NONE',  ( 9.564922557960805705, 16.46253265017160317, 34.58224293864770260 ) ) ;
#63166=CARTESIAN_POINT ( 'NONE',  ( 21.53943276465977519, -0.05219959533907433946, 103.7489096053143669 ) ) ;
#63167=CARTESIAN_POINT ( 'NONE',  ( -9.474510206698964154, 16.51473224551069663, 110.4155762719810383 ) ) ;
#63168=CARTESIAN_POINT ( 'NONE',  ( 0.05219959533910956823, 16.53943276465976808, 84.99890960531436690 ) ) ;
#63170=CARTESIAN_POINT ( 'NONE',  ( -9.474510206698964154, 16.51473224551069663, 45.41557627198103120 ) ) ;
#63171=DIRECTION ( 'NONE',  ( 1.000000000000000000, -0.000000000000000000, -0.000000000000000000 ) ) ;
#63172=CARTESIAN_POINT ( 'NONE',  ( 19.02544592524334988, 5.153800228976608722, 91.45942372801900433 ) ) ;
#63173=CARTESIAN_POINT ( 'NONE',  ( -0.05219959533909027116, -19.03943276465977164, 92.49890960531436690 ) ) ;
#63174=CARTESIAN_POINT ( 'NONE',  ( -5.719274019375665041, -21.55341960407619695, 34.79275706135235424 ) ) ;
#63175=CARTESIAN_POINT ( 'NONE',  ( 13.89961937509977652, -13.97604488694527269, 78.12390960531433848 ) ) ;
#63176=CARTESIAN_POINT ( 'NONE',  ( 13.97604488694548053, -13.89961937509957401, 75.62609039468564731 ) ) ;
#63177=CARTESIAN_POINT ( 'NONE',  ( 9.474510206698971260, -16.51473224551069308, 42.91557627198103120 ) ) ;
#63178=CARTESIAN_POINT ( 'NONE',  ( -4.379528057220328563, 16.55341960407611168, 70.20724293864769550 ) ) ;
#63179=CARTESIAN_POINT ( 'NONE',  ( 12.06949235617757843, -12.14591786802309237, 68.12390960531436690 ) ) ;
#63180=CARTESIAN_POINT ( 'NONE',  ( -19.05341960407611168, -5.049401038298163336, 76.45724293864769550 ) ) ;
#63181=CARTESIAN_POINT ( 'NONE',  ( -5.719274019375978568, 21.55341960407610458, 100.2072429386476955 ) ) ;
#63182=CARTESIAN_POINT ( 'NONE',  ( 9.564922557960805705, 16.46253265017160317, 74.58224293864769550 ) ) ;
#63183=CARTESIAN_POINT ( 'NONE',  ( 9.474510206698729675, 16.51473224551082808, 22.08442372801899722 ) ) ;
#63184=CARTESIAN_POINT ( 'NONE',  ( 13.89961937509977652, -13.97604488694527269, 38.12390960531436690 ) ) ;
#63185=CARTESIAN_POINT ( 'NONE',  ( -12.14591786802309592, -12.06949235617757132, 26.87390960531435979 ) ) ;
#63186=CARTESIAN_POINT ( 'NONE',  ( -16.55341960407611168, -4.379528057220339221, 106.4572429386477097 ) ) ;
#63187=CARTESIAN_POINT ( 'NONE',  ( 0.05219959533936267826, -19.03943276465977164, 100.0010903946856757 ) ) ;
#63189=CARTESIAN_POINT ( 'NONE',  ( 15.80617190586769283, -15.72974639402175789, 25.62609039468567929 ) ) ;
#63190=CARTESIAN_POINT ( 'NONE',  ( -0.05219959533936034679, 19.03943276465977164, 62.50109039468566863 ) ) ;
#63191=CARTESIAN_POINT ( 'NONE',  ( 4.379528057220092307, 16.55341960407617563, 112.2927570613523471 ) ) ;
#63192=CARTESIAN_POINT ( 'NONE',  ( 10.72451020669898902, -18.67979575497178502, 67.91557627198102409 ) ) ;
#63193=CARTESIAN_POINT ( 'NONE',  ( 9.564922557960805705, 16.46253265017160317, 109.5822429386476955 ) ) ;
#63194=CARTESIAN_POINT ( 'NONE',  ( -12.14591786802309592, -12.06949235617757132, 61.87390960531436690 ) ) ;
#63195=CARTESIAN_POINT ( 'NONE',  ( 16.51473224551069308, 9.474510206698969483, 29.16557627198103475 ) ) ;
#63196=CARTESIAN_POINT ( 'NONE',  ( 5.153800228976335163, 19.02544592524342804, 44.79057627198103830 ) ) ;
#63197=CARTESIAN_POINT ( 'NONE',  ( -19.05341960407617563, 5.049401038297882671, 33.54275706135231871 ) ) ;
#63198=CARTESIAN_POINT ( 'NONE',  ( -8.224510206698735004, -14.34966873604973081, 94.58442372801901854 ) ) ;
#63199=CARTESIAN_POINT ( 'NONE',  ( -4.483927247898782831, 16.52544592524335698, 62.70942372801902565 ) ) ;
#63200=CARTESIAN_POINT ( 'NONE',  ( -21.52544592524343514, 5.823673210054127303, 26.04057627198103475 ) ) ;
#63201=CARTESIAN_POINT ( 'NONE',  ( 10.72451020669871369, 18.67979575497193778, 107.0844237280190043 ) ) ;
#63202=CARTESIAN_POINT ( 'NONE',  ( 19.03943276465977164, -0.05219959533909143690, 78.74890960531436690 ) ) ;
#63204=CARTESIAN_POINT ( 'NONE',  ( -12.14591786802326823, 12.06949235617739902, 63.12609039468568994 ) ) ;
#63205=CARTESIAN_POINT ( 'NONE',  ( 12.06949235617757843, -12.14591786802309237, 108.1239096053143811 ) ) ;
#63206=CARTESIAN_POINT ( 'NONE',  ( -12.14591786802326823, 12.06949235617739902, 113.1260903946856899 ) ) ;
#63208=CARTESIAN_POINT ( 'NONE',  ( 18.62759615963255655, 10.81492255796105972, 71.66775706135234714 ) ) ;
#63209=CARTESIAN_POINT ( 'NONE',  ( -0.05219959533909027116, -19.03943276465977164, 87.49890960531436690 ) ) ;
#63210=CARTESIAN_POINT ( 'NONE',  ( -13.89961937509977652, 13.97604488694528158, 75.62390960531438111 ) ) ;
#63211=CARTESIAN_POINT ( 'NONE',  ( -16.51473224551069308, -9.474510206698971260, 106.6655762719810383 ) ) ;
#63212=CARTESIAN_POINT ( 'NONE',  ( 8.314922557960818139, 14.29746914071049879, 59.58224293864770260 ) ) ;
#63213=CARTESIAN_POINT ( 'NONE',  ( 12.14591786802309770, 12.06949235617756955, 24.37390960531435979 ) ) ;
#63214=CARTESIAN_POINT ( 'NONE',  ( -0.05219959533910754901, -16.53943276465976808, 47.49890960531435979 ) ) ;
#63215=CARTESIAN_POINT ( 'NONE',  ( -16.55341960407617563, 4.379528057220093196, 38.54275706135234714 ) ) ;
#63216=CARTESIAN_POINT ( 'NONE',  ( -18.22780087662121673, -5.500000000000063061, 66.48459894673892734 ) ) ;
#63217=CARTESIAN_POINT ( 'NONE',  ( -5.153800228976607833, 19.02544592524334988, 37.70942372801899722 ) ) ;
#63218=CARTESIAN_POINT ( 'NONE',  ( -13.97604488694527625, -13.89961937509977652, 76.87390960531433848 ) ) ;
#63219=CARTESIAN_POINT ( 'NONE',  ( -0.05219959533936034679, 19.03943276465977164, 47.50109039468566863 ) ) ;
#63220=CARTESIAN_POINT ( 'NONE',  ( -0.05219959533936034679, 19.03943276465977164, 57.50109039468566863 ) ) ;
#63221=CARTESIAN_POINT ( 'NONE',  ( 0.05219959533936267826, -19.03943276465977164, 100.0010903946856757 ) ) ;
#63222=CARTESIAN_POINT ( 'NONE',  ( 12.14591786802327356, -12.06949235617739191, 80.62609039468567573 ) ) ;
#63224=CARTESIAN_POINT ( 'NONE',  ( -16.46253265017160317, 9.564922557960807481, 30.83224293864769550 ) ) ;
#63225=CARTESIAN_POINT ( 'NONE',  ( 5.153800228976335163, 19.02544592524342804, 109.7905762719810099 ) ) ;
#63226=CARTESIAN_POINT ( 'NONE',  ( 21.52544592524334988, 5.823673210054432836, 41.45942372801901143 ) ) ;
#63227=CARTESIAN_POINT ( 'NONE',  ( -5.153800228976607833, 19.02544592524334988, 92.70942372801901854 ) ) ;
#63229=CARTESIAN_POINT ( 'NONE',  ( 19.03943276465977164, -0.05219959533909143690, 63.74890960531435979 ) ) ;
#63230=EDGE_CURVE ( 'NONE', #109664, #165524, #54442, .T. ) ;
#63231=CARTESIAN_POINT ( 'NONE',  ( 19.03943276465977164, -0.05219959533909143690, 98.74890960531436690 ) ) ;
#63232=CARTESIAN_POINT ( 'NONE',  ( 4.483927247898545687, 16.52544592524342804, 54.79057627198104541 ) ) ;
#63233=CARTESIAN_POINT ( 'NONE',  ( 13.89961937509977652, -13.97604488694527269, 48.12390960531435979 ) ) ;
#63234=CARTESIAN_POINT ( 'NONE',  ( -5.153800228976328057, -19.02544592524343514, 67.29057627198102409 ) ) ;
#63235=CARTESIAN_POINT ( 'NONE',  ( -19.03943276465977164, -0.05219959533935918106, 58.75109039468566863 ) ) ;
#63236=CARTESIAN_POINT ( 'NONE',  ( 9.564922557961047289, -16.46253265017146816, 40.41775706135234003 ) ) ;
#63237=CARTESIAN_POINT ( 'NONE',  ( 13.97604488694527802, 13.89961937509977652, 84.37390960531433848 ) ) ;
#63238=CARTESIAN_POINT ( 'NONE',  ( -21.55341960407610458, -5.719274019375992779, 81.45724293864769550 ) ) ;
#63239=CARTESIAN_POINT ( 'NONE',  ( -16.55341960407611168, -4.379528057220339221, 81.45724293864769550 ) ) ;
#63240=CARTESIAN_POINT ( 'NONE',  ( 19.03943276465977164, 0.05219959533936151252, 41.25109039468566152 ) ) ;
#63241=CARTESIAN_POINT ( 'NONE',  ( -18.62759615963270932, 10.81492255796079327, 50.83224293864770971 ) ) ;
#63243=CARTESIAN_POINT ( 'NONE',  ( 21.55341960407610458, 5.719274019375980345, 33.95724293864769550 ) ) ;
#63244=CARTESIAN_POINT ( 'NONE',  ( 9.564922557960805705, 16.46253265017160317, 64.58224293864769550 ) ) ;
#63245=CARTESIAN_POINT ( 'NONE',  ( 13.89961937509977652, -13.97604488694527269, 58.12390960531436690 ) ) ;
#63246=CARTESIAN_POINT ( 'NONE',  ( -16.53943276465976808, 0.05219959533911058130, 111.2489096053143669 ) ) ;
#63247=CARTESIAN_POINT ( 'NONE',  ( 18.67979575497194134, -10.72451020669871369, 20.83442372801901143 ) ) ;
#63249=CARTESIAN_POINT ( 'NONE',  ( 21.52544592524334988, 5.823673210054432836, 31.45942372801901854 ) ) ;
#63250=CARTESIAN_POINT ( 'NONE',  ( 13.97604488694527802, 13.89961937509977652, 29.37390960531435979 ) ) ;
#63251=CARTESIAN_POINT ( 'NONE',  ( -10.81492255796078084, -18.62759615963271287, 102.0822429386476955 ) ) ;
#63252=CARTESIAN_POINT ( 'NONE',  ( 5.049401038297881783, 19.05341960407617563, 42.29275706135234003 ) ) ;
#63254=CARTESIAN_POINT ( 'NONE',  ( 16.51473224551069308, 9.474510206698969483, 29.16557627198103475 ) ) ;
#63256=CARTESIAN_POINT ( 'NONE',  ( 14.29746914071037800, 8.314922557961029526, 61.66775706135235424 ) ) ;
#63257=CARTESIAN_POINT ( 'NONE',  ( -16.53943276465976808, 0.05219959533911058130, 116.2489096053143669 ) ) ;
#63259=CARTESIAN_POINT ( 'NONE',  ( -16.51473224551069308, -9.474510206698971260, 66.66557627198102409 ) ) ;
#63260=CARTESIAN_POINT ( 'NONE',  ( 16.53943276465976808, -0.05219959533910856209, 108.7489096053143669 ) ) ;
#63261=CARTESIAN_POINT ( 'NONE',  ( 0.05219959533907565091, 21.53943276465977519, 59.99890960531436690 ) ) ;
#63262=CARTESIAN_POINT ( 'NONE',  ( 0.05219959533910956823, 16.53943276465976808, 74.99890960531435269 ) ) ;
#63263=CARTESIAN_POINT ( 'NONE',  ( -16.55341960407617563, 4.379528057220093196, 28.54275706135234358 ) ) ;
#63264=CARTESIAN_POINT ( 'NONE',  ( 21.53943276465977519, 0.05219959533937863772, 86.25109039468568994 ) ) ;
#63265=CARTESIAN_POINT ( 'NONE',  ( -19.02544592524342804, 5.153800228976336051, 26.04057627198103120 ) ) ;
#63266=CARTESIAN_POINT ( 'NONE',  ( 16.53943276465976808, -0.05219959533910856209, 23.74890960531435269 ) ) ;
#63267=CARTESIAN_POINT ( 'NONE',  ( 16.52544592524342804, -4.483927247898539470, 58.54057627198103120 ) ) ;
#63268=CARTESIAN_POINT ( 'NONE',  ( -19.02544592524342804, 5.153800228976336051, 51.04057627198103120 ) ) ;
#63269=CARTESIAN_POINT ( 'NONE',  ( 15.80617190586769283, -15.72974639402175789, 100.6260903946857184 ) ) ;
#63270=CARTESIAN_POINT ( 'NONE',  ( -5.823673210054116645, -21.52544592524344225, 107.2905762719810525 ) ) ;
#63271=( BOUNDED_SURFACE ( )  B_SPLINE_SURFACE ( 3, 2, ( 
 ( #191487, #148998, #71152, #53984, #6458, #132818, #190504, #23650, #194504, #68139, #39802, #87314, #128805, #192500, #52965, #129790, #37812, #176340, #101467, #69142, #99473, #161153, #22650, #84297, #100475, #115657, #146990, #56987, #105467, #167153, #106447, #150998, #120628, #75124, #57985, #165166, #104481, #28652, #151972, #60937, #134836, #136792, #89306, #137785, #91256, #14446, #153951, #12490, #41820, #152947, #58960, #74151, #90288, #198478, #166165, #149989, #59950, #13460, #169107, #121617, #76109, #135823, #197493, #195514, #183312, #118661, #182325, #180352, #43804, #44794, #11495, #103488, #168128, #26659, #29624, #199470, #122611, #184301, #88301, #45783, #73166, #196515, #119657, #107435, #30614, #92267, #72147, #133823, #181339, #42818, #27666, #97223, #187298, #126580, #94256, #32603, #48770, #156939, #109432, #81069, #112414, #79088, #49755, #172105, #33591, #47779, #15447, #95254, #2249, #50756, #61924, #123594, #140761, #65906, #185288, #3245, #174106, #18436, #31609, #80086, #188281, #189280, #35575, #110424, #155936, #141755, #255, #16441, #62924, #142747, #77105, #63932, #111423, #64919, #173109, #171112, #138774, #34586, #125601, #46780, #108439, #170115, #96243, #127579, #93259, #157931, #154944, #19421, #78090, #4227, #139758, #1245, #124604, #186299, #17431, #23412, #143744, #159917, #6225, #179112, #54739, #84063, #66904, #116411, #20400, #53746, #193265, #36559, #85060, #178100, #39570, #22412, #83064, #190262, #67904, #82049, #146742, #99232, #132585, #9250, #175091, #52732, #130567, #40580, #129557, #5223, #192264, #115420, #101228, #37569, #7222, #161918, #144738, #51739, #191257, #177109, #38580, #147764, #21406, #8237, #176099, #24425, #162917, #86074, #158909, #160919, #128567, #70917, #145741, #68907, #100236, #69915, #114398, #98214, #131581, #194273, #55740, #117414, #113401, #104244, #165927, #25435, #166923, #87076, #27424, #10250, #150760, #91031, #164933, #26426, #195271, #41587, #28424, #151743, #71909, #105235, #90061, #180119, #44562, #133581, #121387, #59715, #167901, #12258, #56755, #74899, #120393, #13236, #118426, #136562, #103251, #72929, #89069, #122376, #198243, #102250, #135590, #88066, #183079, #149753, #73920, #163938, #11256, #148761, #106217, #134598, #152717, #184065, #29401, #14208, #196284, #57753, #119423, #75876, #197262, #181107, #42581, #137552, #58724, #199235, #43570, #182087, #60700, #37081, #190774, #168873, #52249, #18, #61692, #51261, #185054, #93026, #47546, #108202, #1012, #169883, #35095, #98740, #31376, #113906, #96747, #160433, #30378, #83574, #159420, #145253, #5742, #158437, #124368, #82574, #62686, #123361, #19924, #92023, #186063, #81566, #20916, #175604, #21923, #128086, #6734, #36081, #138540, #111938, #189790, #107203, #67418, #153715, #143252, #68412, #154714, #16207, #46542, #77862, #112921, #97730, #15211, #174616, #144255, #139529, #130065, #76870, #129073, #45548, #173625, #4736, #66425, #164448, #9762, #41097, #99748, #56254, #161432, #162425, #55252, #11775, #25942, #191764, #73439, #23926, #133090, #39088, #116920, #54259, #87585, #163442, #117936, #102761, #84570, #165443, #22924, #53247, #149272, #24939, #179625, #115930, #10764, #176618, #134106, #148270, #177620, #146248, #101754, #85581, #114925, #132094, #7734, #72428, #178613, #193783, #71426, #195796, #147267, #69420, #194780, #57268, #88580, #118942, #180627, #40076, #86586, #38093, #42099, #131086, #103764, #192775, #100744, #8757, #70428, #150278, #26938, #58254, #152246, #91537, #46054, #92544, #181608, #153224, #151267, #104753, #119922, #170394, #185564, #108716, #121894, #47058, #27939, #168404, #530, #16713, #106730, #107709, #13731, #75397, #29899, #76390, #28924, #62202, #31885, #198759, #169388, #14729, #138066, #167428, #135110, #199747, #183587, #93539, #43086, #166443, #60225, #155224, #89581, #122885, #196786, #61213, #12757 ),
 ( #74422, #184573, #136088, #123866, #197762, #15722, #30896, #59229, #44083, #120898, #154232, #45072, #182598, #105741, #90564, #137069, #77382, #139050, #48056, #19692, #67183, #20675, #1526, #82330, #32882, #94532, #81334, #17714, #125876, #80356, #141043, #33870, #2529, #65193, #128840, #64209, #144020, #126852, #190539, #63205, #113672, #189553, #175366, #140037, #109712, #78363, #127848, #124885, #52013, #98500, #159180, #112686, #186583, #187576, #171395, #143017, #188558, #156214, #79372, #5501, #142028, #97494, #4495, #49044, #66186, #36834, #160194, #110699, #172379, #95529, #157216, #51025, #18709, #3517, #50037, #111701, #173387, #34857, #96512, #158202, #174378, #35848, #70192, #10524, #145014, #57026, #132854, #118699, #179388, #131859, #100512, #56013, #38855, #176377, #8514, #6495, #162191, #193543, #194542, #149036, #72187, #101506, #133861, #9524, #114682, #85337, #163196, #83337, #40851, #68175, #55016, #195552, #84334, #146013, #37851, #161191, #86349, #71190, #129827, #24700, #117691, #99510, #164207, #191526, #102525, #25705, #87350, #116686, #53003, #180390, #39840, #41861, #22687, #148035, #7496, #192539, #147030, #103527, #21684, #69181, #130847, #54022, #115695, #177384, #178376, #23689, #137824, #136832, #29661, #14483, #58022, #138812, #134874, #46814, #76145, #198515, #91293, #27700, #199507, #150028, #107470, #121654, #89342, #119691, #75160, #135858, #59986, #196551, #152984, #181375, #152009, #13495, #42853, #60973, #183348, #122648, #73203, #184337, #104518, #197528, #28688, #185324, #45819, #165202, #26697, #58997, #106486, #12524, #90324, #151034, #169147, #44830, #30651, #92305, #166199, #292, #74189, #88337, #153988, #168164, #15485, #120663, #77142, #11534, #61961, #123628, #182361, #43839, #105504, #167190, #141787, #139793, #173143, #1282, #95288, #170152, #78124, #108473, #157963, #154980, #97254, #128599, #189311, #142780, #93294, #17467, #62958, #34618, #18469, #124639, #16475, #35609, #110458, #127612, #49791, #186334, #111457, #158942, #50789, #31645, #112448, #47816, #109465, #96277, #171149, #155969, #172139, #32637, #63967, #94291, #156972, #20431, #79123, #174137, #80119, #82082, #140796, #143774, #19455, #5255, #65941, #3282, #187334, #4261, #125637, #2285, #64953, #48804, #33625, #126612, #81102, #66937, #190293, #188314, #102281, #39601, #144771, #115451, #193297, #113430, #9282, #175122, #100268, #40611, #114430, #176131, #6256, #191285, #116446, #101260, #159948, #54772, #162950, #129589, #194304, #21435, #70947, #132617, #117444, #85091, #146776, #86105, #130601, #161949, #178134, #37601, #67936, #84093, #8269, #131613, #163969, #99264, #24456, #68938, #179143, #55770, #25467, #133611, #192297, #83096, #87107, #38612, #53776, #69948, #147797, #145771, #52760, #148793, #10283, #71941, #51770, #36590, #177141, #23444, #98246, #160950, #22443, #7253, #103283, #195305, #104276, #180150, #92058, #106248, #118458, #12287, #151772, #167930, #152748, #41618, #13265, #11287, #164963, #26456, #30411, #45581, #168905, #182114, #107234, #88098, #28454, #60735, #76901, #166951, #29430, #73952, #135620, #90090, #136591, #89100, #122408, #153747, #58754, #91061, #74928, #198271, #27459, #56786, #59748, #43600, #15242, #149784, #72960, #120423, #134629, #196314, #183110, #57783, #121418, #119453, #44592, #14238, #181138, #42612, #75910, #197291, #137584, #165958, #150791, #105265, #199267, #184098, #63730, #46574, #96048, #50, #33394, #172910, #16241, #64725, #34388, #157735, #2051, #62718, #169915, #47577, #61725, #126387, #78883, #112217, #189084, #154745, #32400, #110225, #158709, #186095, #123393, #111218, #138572, #20198, #170908, #79890, #109229, #125405, #1045, #19224, #171906, #3049, #188084, #31407, #173907, #108235, #185085, #49555, #95053, #80874, #124401, #142550, #93058, #4028, #156742, #94055, #77893, #48572, #155733, #18236, #139561 ),
 ( #17231, #140562, #65706, #141560, #187102, #127372, #50557, #35376, #97028, #23208, #51538, #84851, #70709, #24214, #5020, #85863, #36356, #98008, #146528, #21200, #129358, #83851, #144535, #37362, #6021, #68694, #132377, #67700, #147552, #130349, #194070, #66702, #117205, #193057, #178897, #39366, #192048, #160711, #116207, #99020, #159703, #53529, #128366, #22202, #115207, #54534, #9040, #55531, #161712, #40365, #69701, #174890, #145533, #8019, #143532, #101024, #190062, #176899, #102040, #191053, #52526, #82856, #114187, #131368, #177896, #113201, #162709, #163723, #175891, #81844, #7012, #38370, #100025, #90832, #73715, #195060, #198038, #43360, #74697, #133369, #89859, #56538, #196072, #88859, #45350, #10042, #134386, #118216, #151542, #135387, #179907, #41373, #152516, #27213, #44356, #166715, #103039, #28219, #14004, #167701, #148551, #29198, #164721, #26216, #13031, #87855, #72714, #150552, #149543, #180899, #11038, #12051, #75671, #57545, #137348, #197057, #199028, #71702, #60497, #136362, #122173, #182875, #58525, #104037, #59506, #42374, #119214, #120191, #165716, #181881, #105031, #121181, #183863, #107002, #106015, #25225, #86867, #61494, #32167, #109993, #30175, #126157, #91818, #16997, #157499, #31174, #92824, #123164, #107992, #33162, #18001, #76667, #171673, #156499, #46336, #110982, #138346, #187853, #49322, #34153, #78651, #200026, #141323, #186869, #79654, #184852, #94821, #169678, #139333, #93824, #188841, #2812, #168675, #50326, #812, #64490, #16006, #155504, #154510, #172667, #140326, #95813, #18992, #77664, #142315, #62485, #153510, #80638, #1816, #3795, #124157, #65472, #15007, #127135, #125170, #185857, #47343, #63495, #108998, #48338, #170679, #176662, #143295, #98783, #173673, #81611, #111981, #161478, #158481, #100785, #132136, #192819, #146294, #145297, #7781, #190818, #160477, #114969, #97776, #4781, #144297, #68459, #191809, #162468, #174659, #38139, #129119, #177661, #131131, #54301, #193828, #52293, #66469, #115973, #21968, #113950, #130113, #99792, #5787, #189833, #22967, #53291, #8800, #84615, #39130, #175649, #37124, #35140, #69465, #96792, #83619, #19969, #128131, #20959, #51305, #70470, #23969, #112966, #6780, #85625, #147311, #36124, #159463, #82616, #67461, #163484, #178656, #77171, #154019, #138841, #136861, #15514, #24981, #183380, #169176, #123655, #121684, #137855, #90354, #28717, #44862, #29692, #102801, #30681, #321, #75189, #61005, #106517, #168195, #164487, #55293, #91323, #198547, #61989, #101797, #86627, #60017, #116965, #148310, #199535, #40118, #184366, #152039, #45847, #92333, #9804, #71466, #122677, #153014, #133131, #179667, #14514, #76175, #194822, #56294, #107500, #13524, #117977, #41137, #55574, #27255, #180940, #131411, #117248, #177938, #11083, #56584, #39405, #54574, #88905, #164763, #120232, #197100, #162750, #40410, #118259, #166760, #194111, #193098, #179949, #8065, #178940, #148592, #102082, #150596, #42416, #116246, #163766, #101065, #72759, #41416, #24258, #73757, #134430, #58567, #104079, #87899, #85909, #149585, #135429, #12094, #69742, #181923, #147596, #9081, #196116, #70751, #25266, #10084, #132419, #86909, #71742, #133413, #43404, #195102, #105074, #103082, #28262, #26258, #146571, #57586, #119256, #165761, #138385, #168715, #124201, #107043, #44401, #76710, #74739, #30217, #200067, #62528, #17040, #140371, #169721, #1858, #77706, #182916, #153552, #31214, #151583, #47386, #13072, #61535, #78694, #152556, #14045, #106055, #29239, #154552, #139372, #198080, #92865, #854, #167741, #32211, #59547, #109041, #170719, #155546, #123204, #121225, #185901, #108035, #93867, #90872, #16047, #75711, #60538, #15049, #110038, #63540, #89900, #171717, #122214, #125214, #137389, #184894, #199069, #186910, #46376, #48381, #136402, #183905, #45390, #91859, #115012, #144342, #4825, #97818, #95858, #5830, #18045, #175691, #189874, #157541 ),
 ( #66513, #53333, #80682, #79698, #128175, #51349, #67506, #112028, #81655, #36166, #19035, #126200, #65517, #113009, #174702, #22010, #142358, #159507, #50368, #98825, #52337, #37166, #33206, #173717, #2856, #113993, #20012, #35185, #21003, #82658, #127177, #111027, #129163, #190860, #130155, #160519, #83662, #96839, #158524, #156546, #145340, #141369, #143338, #64534, #94865, #3838, #187896, #191852, #6822, #49363, #68500, #172713, #34196, #188887, #23012, #133177, #192865, #146336, #161520, #11865, #27028, #150369, #163527, #88673, #69509, #9850, #42191, #58341, #148354, #87670, #55338, #193872, #71509, #118022, #70513, #103851, #73530, #40165, #10852, #194867, #56340, #8845, #176706, #179712, #25027, #135202, #84658, #7824, #101841, #196874, #131175, #164532, #38180, #41184, #54344, #102847, #149355, #99836, #116015, #26025, #117008, #72521, #177705, #39172, #24015, #100830, #134196, #86671, #195884, #162513, #132181, #57358, #119032, #85670, #180715, #165532, #147357, #178703, #44173, #151358, #92634, #199842, #622, #138161, #93634, #170487, #153321, #60314, #184666, #104842, #120990, #167519, #140132, #15814, #45166, #183681, #1623, #152336, #76484, #154325, #197854, #46148, #77475, #139145, #106822, #105832, #12847, #62293, #61309, #123960, #122979, #155319, #31978, #136179, #13822, #91633, #120009, #29014, #166533, #14823, #107802, #185658, #198850, #168496, #169486, #90654, #74513, #75488, #30986, #47150, #108808, #182688, #16808, #137161, #78458, #181694, #43175, #28030, #121990, #89671, #59321, #29994, #65287, #19784, #189644, #157308, #141136, #66283, #4590, #160288, #51119, #67274, #126946, #188654, #186677, #127942, #48147, #50133, #171487, #63300, #172478, #109804, #21779, #174471, #32976, #80450, #81425, #35940, #20770, #94630, #143111, #79467, #156309, #17810, #98594, #113765, #36932, #111793, #175461, #2626, #96606, #128932, #145107, #34954, #97586, #142123, #3608, #158295, #112778, #18805, #190633, #83430, #173481, #159274, #82425, #144114, #95623, #124980, #5594, #52108, #64303, #125970, #187669, #49139, #110797, #33965, #194638, #41957, #148129, #22779, #9620, #117789, #180485, #103623, #132950, #102620, #40948, #70285, #130940, #37945, #179483, #86443, #87445, #24795, #165299, #57123, #84427, #100602, #178470, #26792, #54113, #191620, #39937, #101606, #164306, #85434, #55109, #71285, #192631, #99605, #38945, #163295, #56108, #195650, #69274, #25799, #23784, #72282, #149130, #10621, #88434, #147125, #176471, #133959, #193637, #8612, #118797, #6590, #162284, #146104, #68269, #129920, #53099, #114777, #161285, #131953, #116779, #7588, #115787, #177476, #13586, #58114, #150128, #59086, #134967, #46907, #61066, #73297, #167280, #106580, #122738, #107562, #196644, #168257, #166298, #119784, #181468, #185416, #382, #123719, #136924, #62054, #42946, #183439, #15575, #31739, #121747, #184429, #28778, #90417, #44924, #91388, #43932, #77233, #108567, #75253, #45909, #29753, #153077, #182452, #11629, #14579, #198611, #170245, #104610, #27794, #60079, #89436, #151124, #137916, #12617, #76237, #74281, #199599, #169240, #135951, #197621, #30746, #152102, #92394, #120753, #105594, #154081, #138902, #189402, #18560, #157063, #113524, #125728, #49883, #127702, #171241, #78215, #190389, #4350, #16568, #110550, #111548, #66035, #50879, #139885, #173233, #109560, #63053, #1374, #128692, #143870, #67033, #80208, #5349, #186430, #126701, #159033, #175218, #65045, #112537, #172231, #33716, #188405, #34709, #187427, #20526, #51864, #141879, #174231, #96366, #158054, #48895, #93387, #19544, #3370, #155073, #124732, #47906, #81189, #32730, #94382, #142871, #156061, #35700, #17559, #97347, #82174, #79219, #140888, #2378, #95378, #64058, #21529, #37693, #86940, #59578, #135458, #164794, #103113, #121252, #71774, #196145, #73786, #114523, #165791, #197127, #58594, #26289, #163796, #68027, #12122 ),
 ( #120260, #118289, #87930, #42445, #25298, #129678, #133444, #57617, #119285, #28290, #102111, #104109, #56615, #105103, #181952, #43434, #36683, #179980, #6347, #166789, #149617, #41448, #180968, #27288, #195134, #176224, #88934, #150626, #136430, #89930, #151611, #11115, #72790, #160042, #13103, #83190, #134460, #144864, #98343, #148624, #74768, #198111, #191376, #52852, #10114, #46404, #124231, #44429, #140397, #106083, #31242, #171745, #45416, #107069, #75741, #122241, #47412, #32236, #90898, #185927, #170747, #60565, #125240, #152584, #1885, #63566, #48409, #92892, #14074, #155572, #880, #93894, #137418, #109068, #199098, #153578, #108063, #2883, #17067, #182946, #64562, #15076, #78721, #30244, #169747, #168740, #186938, #154578, #110065, #33234, #183931, #156576, #91887, #167769, #94892, #16074, #18071, #76736, #79726, #29267, #141395, #139398, #138412, #200092, #77732, #61560, #62555, #123229, #184920, #157568, #113038, #187922, #95885, #126227, #49391, #35212, #128205, #96865, #6851, #160550, #111054, #158549, #19061, #190890, #36193, #80708, #53365, #114023, #176735, #22040, #67534, #142386, #129192, #115043, #68530, #172742, #130185, #3865, #65544, #52366, #127203, #173743, #189902, #188917, #81682, #50395, #174730, #38208, #112055, #191881, #97847, #99864, #34223, #161548, #37199, #23041, #83691, #159536, #4856, #145369, #143364, #20039, #21034, #66541, #51377, #82687, #98855, #84686, #144371, #146366, #7853, #5858, #175720, #100858, #134224, #179741, #162540, #196899, #57384, #120033, #103876, #10876, #39202, #72546, #58366, #11891, #192895, #73554, #24044, #85700, #195909, #8874, #117035, #71537, #132210, #25055, #193901, #56368, #181719, #55365, #135227, #118051, #43201, #54372, #104868, #180739, #166557, #27053, #41211, #148383, #165556, #86698, #147386, #102872, #116044, #9877, #164557, #42215, #28056, #89697, #149380, #151383, #119057, #70542, #133203, #88699, #131204, #150395, #177733, #26051, #69540, #178730, #40192, #101873, #163555, #194894, #87695, #121015, #15842, #648, #90679, #155347, #182713, #32005, #170516, #78487, #61333, #44198, #185686, #31011, #62318, #105857, #77501, #167544, #183706, #76510, #33003, #47176, #12873, #94657, #45192, #154349, #60341, #138186, #75513, #108835, #184690, #139171, #123988, #29039, #186704, #152361, #74538, #93662, #46174, #16836, #137187, #140160, #197878, #1652, #169511, #198874, #13846, #123004, #106846, #107827, #122015, #63330, #168521, #199869, #136203, #30019, #59347, #91657, #153346, #14848, #92661, #125008, #48175, #109831, #171514, #49165, #129950, #125998, #37977, #67302, #127969, #20798, #18832, #128961, #141164, #98623, #112806, #80477, #110824, #66309, #126973, #189673, #187695, #82453, #172506, #143138, #17837, #33993, #156337, #79495, #65313, #158322, #188681, #36962, #190661, #2653, #50161, #95649, #144141, #51145, #157337, #83459, #5624, #6620, #52137, #97613, #142151, #159303, #145137, #160317, #64330, #21808, #3635, #111820, #113794, #173508, #34981, #19811, #96634, #81452, #4617, #174499, #68299, #35966, #191650, #175489, #53129, #114808, #176500, #10651, #196677, #57152, #148159, #178501, #133990, #116809, #54144, #86474, #84456, #39967, #9650, #72313, #26823, #150160, #179513, #11661, #87474, #192661, #163328, #40981, #161316, #118831, #22810, #71316, #88464, #162314, #23815, #115817, #38976, #164335, #149161, #7620, #102650, #195681, #177507, #41987, #69304, #180514, #103653, #165331, #132979, #130970, #73327, #117820, #134999, #100633, #25830, #85465, #70316, #24824, #119814, #58146, #99634, #181499, #131983, #146134, #147154, #194669, #8642, #193668, #55139, #101637, #56139, #90452, #44958, #105627, #45940, #75286, #199631, #122771, #31769, #167316, #107595, #60112, #108598, #62086, #185448, #124765, #183474, #12647, #123749, #29786, #106616, #61098, #169273, #136957, #120784, #30779, #184461, #139918, #92426 ),
 ( #166329, #121780, #154112, #15606, #412, #89468, #77263, #59118, #74314, #27826, #78245, #93417, #16597, #91422, #155104, #135981, #76270, #170275, #42977, #14613, #138932, #168290, #153109, #137948, #46938, #198646, #1407, #63086, #104642, #151159, #197652, #182484, #43965, #28812, #152136, #13619, #21563, #32763, #94415, #49915, #36717, #156095, #174265, #83223, #127734, #2410, #189436, #97380, #160076, #144898, #19577, #126733, #50913, #171275, #187458, #33751, #6381, #82211, #111580, #173265, #68060, #18591, #142901, #20560, #64090, #112571, #143902, #5384, #34739, #110580, #17593, #159066, #66068, #67067, #4383, #186463, #98379, #125758, #80239, #158085, #47941, #95410, #157095, #96398, #48926, #128726, #81220, #35733, #190422, #79252, #109592, #140924, #172261, #51898, #113557, #175251, #141909, #3400, #65075, #188436, #86231, #53905, #22570, #39725, #100397, #163079, #161075, #194427, #84217, #116573, #191411, #99392, #129714, #52887, #38739, #131742, #162077, #10407, #164092, #114562, #23571, #145896, #55898, #101386, #7380, #56908, #117571, #180273, #25591, #71073, #69064, #132739, #118583, #72065, #176259, #133738, #130731, #192423, #179271, #115580, #177268, #9407, #24583, #103407, #85219, #178262, #41743, #146910, #195433, #147921, #165085, #37730, #26579, #40735, #88222, #87235, #102405, #8399, #148918, #70074, #193424, #149906, #54899, #11413, #183233, #45702, #176, #123513, #152871, #185206, #60855, #166082, #136713, #14366, #134754, #30531, #196436, #121538, #61844, #135743, #197414, #27585, #12410, #137707, #122530, #181261, #76031, #184221, #150917, #15366, #42738, #92184, #153868, #138694, #44714, #104400, #107353, #91182, #169026, #89223, #199391, #74072, #43724, #198394, #93180, #77022, #73083, #154865, #105385, #46697, #57906, #108358, #29549, #58880, #120546, #106370, #167072, #168052, #182239, #170037, #28574, #59871, #119578, #90210, #151893, #13383, #75047, #31527, #125524, #97148, #50679, #1165, #187221, #47700, #80995, #126506, #109350, #143660, #4149, #66825, #112337, #157857, #186219, #19347, #5143, #158831, #139678, #20319, #171032, #32523, #142670, #155854, #63853, #96167, #188204, #190184, #79007, #3171, #128489, #140681, #81968, #64844, #51659, #62840, #113323, #127497, #175015, #174027, #49676, #95174, #35498, #33514, #94175, #111340, #124524, #156861, #173031, #189202, #36480, #98136, #65828, #16362, #78010, #17352, #80011, #2173, #48692, #110344, #172026, #34509, #18356, #141680, #22330, #52656, #99152, #24341, #9168, #67827, #162832, #147680, #37490, #102165, #129483, #179025, #117331, #25352, #8151, #191181, #132503, #178018, #70835, #114319, #85991, #176021, #130483, #23331, #180035, #194192, #159834, #41504, #192180, #101146, #7141, #84975, #83981, #55657, #131495, #40493, #163851, #160841, #133497, #145660, #21328, #86993, #193182, #148680, #68824, #10168, #146657, #161837, #116329, #71828, #53661, #115339, #195189, #56669, #118342, #82986, #144662, #69828, #54655, #6146, #177029, #38499, #39486, #100155, #103168, #12176, #87984, #200141, #14126, #26344, #120313, #59632, #75793, #60617, #149672, #121306, #119340, #72846, #11170, #138460, #153632, #76789, #89982, #15127, #196201, #136482, #168792, #184970, #74820, #137471, #182007, #43489, #198162, #44481, #197182, #30295, #61611, #166842, #199151, #182998, #106137, #135512, #164848, #167820, #151663, #123279, #134515, #57673, #28344, #181026, #42500, #90949, #104164, #29319, #165846, #152636, #122292, #27342, #88988, #183982, #105156, #45467, #150679, #73841, #58647, #13157, #107121, #91939, #112836, #69332, #81481, #5654, #83489, #127003, #175517, #145166, #6650, #174528, #173540, #80508, #21836, #128992, #129978, #67330, #22838, #99662, #65343, #143168, #20828, #130998, #96664, #31291, #82484, #144168, #68328, #128001, #4648, #46455, #142181, #52165, #66339, #190690, #113822, #38007, #111850 ),
 ( #84485, #160347, #146162, #191678, #97642, #189703, #53159, #51176, #3665, #35995, #92942, #159331, #36992, #114837, #176531, #161347, #98653, #7648, #108114, #188711, #169798, #157368, #18862, #50194, #35009, #158351, #19840, #55166, #116837, #85493, #132010, #57181, #42015, #100660, #195709, #180541, #70343, #135028, #162342, #11689, #150191, #58173, #41010, #23843, #165359, #10678, #103680, #147181, #118858, #8670, #163356, #56167, #12673, #26853, #192690, #74340, #24852, #134017, #39994, #117848, #178527, #88494, #164362, #73355, #196703, #193697, #166357, #101666, #54173, #119840, #25857, #181525, #86501, #43004, #177535, #104671, #149189, #148185, #9679, #102677, #71344, #87501, #133007, #27855, #194698, #179541, #115846, #72343, #39005, #89495, #151185, #137978, #44985, #16628, #170305, #120813, #106645, #167342, #441, #45968, #28839, #63116, #123779, #186493, #31798, #77292, #105654, #138963, #124795, #78275, #59143, #139948, #90480, #152162, #62116, #75312, #183502, #15635, #107622, #109621, #198672, #122799, #47969, #60139, #169300, #108627, #171305, #32791, #185478, #94444, #46968, #13645, #199660, #93447, #197678, #155134, #182513, #184489, #156124, #121806, #168317, #136983, #29814, #1438, #17623, #43992, #136006, #91450, #153138, #14640, #76300, #61126, #30806, #92455, #154143, #187488, #159092, #127761, #97405, #125786, #174289, #48954, #65103, #34769, #83249, #20586, #79282, #144924, #188464, #112597, #3427, #96426, #18619, #82238, #4409, #35759, #143928, #172290, #160103, #110607, #140952, #5410, #66094, #67093, #80266, #128752, #33779, #51924, #189461, #126761, #95439, #50939, #49946, #190449, #157123, #113584, #141936, #142928, #64121, #111610, #2439, #158112, #175278, #36743, #98407, #173295, #19604, #21590, #81246, #91099, #124437, #169950, #152787, #187137, #47612, #110261, #94091, #1081, #29466, #62756, #48609, #2088, #183145, #63768, #14278, #75947, #186133, #199305, #107270, #139595, #31441, #33431, #122444, #46610, #171942, #184136, #125441, #108272, #95090, #44630, #156779, #170945, #18272, #17268, #93095, #138607, #155770, #76938, #137621, #154779, #106282, #89, #60772, #16276, #30448, #77928, #45618, #109266, #168941, #32437, #121453, #92095, #59785, #167967, #153783, #61759, #15278, #140598, #78921, #123427, #185120, #79925, #141598, #113240, #34425, #130393, #191094, #53573, #37406, #144575, #172947, #6062, #192090, #145576, #126423, #7053, #157773, #19264, #67740, #142587, #50594, #82897, #174931, #176942, #65744, #190101, #115250, #127412, #68735, #51576, #38412, #188121, #100069, #114229, #161754, #160752, #36394, #81883, #99064, #20235, #80910, #98048, #49592, #143575, #159746, #175934, #23249, #84892, #129398, #3085, #52569, #96084, #66743, #22244, #64761, #83893, #111255, #21243, #4066, #189122, #112253, #173945, #35412, #97064, #158746, #5058, #128404, #57282, #163457, #116936, #132108, #182616, #197782, #120917, #134121, #59248, #40092, #180642, #12774, #28942, #118956, #58269, #25956, #164462, #42117, #88598, #41111, #74439, #44101, #10779, #181623, #103779, #165458, #179641, #147283, #26955, #195810, #105759, #193800, #55267, #72446, #167445, #178629, #135127, #8773, #150294, #24955, #11790, #119938, #70442, #136106, #101770, #73454, #86602, #196801, #148285, #43103, #104771, #9779, #166459, #71441, #27956, #133106, #194795, #56268, #117951, #102775, #89597, #151284, #87599, #149285, #109730, #77401, #32900, #60243, #171414, #48074, #156233, #139071, #121914, #63224, #108736, #140058, #198777, #155244, #183607, #61233, #154251, #110719, #124904, #90583, #172401, #122904, #31905, #138085, #15742, #153246, #186602, #62220, #16734, #1549, #45091, #64230, #106748, #152264, #94552, #123888, #78382, #14748, #17735, #75417, #79392, #47076, #76409, #168423, #549, #184593, #185586, #29918, #141062, #91558, #170413, #13749, #199766, #137090, #46074, #107728 ) ),
 .UNSPECIFIED., .T., .F., .T. ) 
 B_SPLINE_SURFACE_WITH_KNOTS ( ( 4, 3, 4 ),
 ( 3, 2, 2, 2, 2, 2, 2, 2, 2, 2, 2, 2, 2, 2, 2, 2, 2, 2, 2, 2, 2, 2, 2, 2, 2, 2, 2, 2, 2, 2, 2, 2, 2, 2, 2, 2, 2, 2, 2, 2, 2, 2, 2, 2, 2, 2, 2, 2, 2, 2, 2, 2, 2, 2, 2, 2, 2, 2, 2, 2, 2, 2, 2, 2, 2, 2, 2, 2, 2, 2, 2, 2, 2, 2, 2, 2, 2, 2, 2, 2, 2, 2, 2, 2, 2, 2, 2, 2, 2, 2, 2, 2, 2, 2, 2, 2, 2, 2, 2, 2, 2, 2, 2, 2, 2, 2, 2, 2, 2, 2, 2, 2, 2, 2, 2, 2, 2, 2, 2, 2, 2, 2, 2, 2, 2, 2, 2, 2, 2, 2, 2, 2, 2, 2, 2, 2, 2, 2, 2, 2, 2, 2, 2, 2, 2, 2, 2, 2, 2, 2, 2, 2, 2, 2, 2, 2, 2, 2, 2, 2, 2, 2, 2, 2, 2, 2, 2, 2, 2, 2, 2, 2, 2, 2, 2, 2, 2, 2, 2, 2, 2, 2, 2, 2, 2, 2, 2, 2, 2, 2, 2, 2, 2, 2, 2, 2, 2, 2, 2, 2, 2, 2, 2, 2, 2, 2, 2, 2, 2, 2, 2, 2, 2, 2, 2, 2, 2, 2, 2, 2, 2, 2, 2, 2, 2, 2, 2, 2, 3 ),
 ( 0.000000000000000000, 0.5000000000000000000, 1.000000000000000000 ),
 ( 0.000000000000000000, 0.004385964912280701511, 0.008771929824561403022, 0.01315789473684210453, 0.01754385964912280604, 0.02192982456140350755, 0.02631578947368420907, 0.03070175438596491058, 0.03508771929824561209, 0.03947368421052631360, 0.04385964912280701511, 0.04824561403508771662, 0.05263157894736841813, 0.05701754385964911964, 0.06140350877192982115, 0.06578947368421052266, 0.07017543859649122417, 0.07456140350877192569, 0.07894736842105262720, 0.08333333333333332871, 0.08771929824561403022, 0.09210526315789473173, 0.09649122807017543324, 0.1008771929824561348, 0.1052631578947368363, 0.1096491228070175378, 0.1140350877192982393, 0.1184210526315789408, 0.1228070175438596423, 0.1271929824561403577, 0.1315789473684210453, 0.1359649122807017607, 0.1403508771929824483, 0.1447368421052631637, 0.1491228070175438514, 0.1535087719298245668, 0.1578947368421052544, 0.1622807017543859698, 0.1666666666666666574, 0.1710526315789473728, 0.1754385964912280604, 0.1798245614035087758, 0.1842105263157894635, 0.1885964912280701788, 0.1929824561403508665, 0.1973684210526315819, 0.2017543859649122695, 0.2061403508771929849, 0.2105263157894736725, 0.2149122807017543879, 0.2192982456140350755, 0.2236842105263157909, 0.2280701754385964786, 0.2324561403508771940, 0.2368421052631578816, 0.2412280701754385970, 0.2456140350877192846, 0.2500000000000000000, 0.2543859649122807154, 0.2587719298245614308, 0.2631578947368420907, 0.2675438596491228060, 0.2719298245614035214, 0.2763157894736842368, 0.2807017543859648967, 0.2850877192982456121, 0.2894736842105263275, 0.2938596491228070429, 0.2982456140350877027, 0.3026315789473684181, 0.3070175438596491335, 0.3114035087719298489, 0.3157894736842105088, 0.3201754385964912242, 0.3245614035087719396, 0.3289473684210526550, 0.3333333333333333148, 0.3377192982456140302, 0.3421052631578947456, 0.3464912280701754610, 0.3508771929824561209, 0.3552631578947368363, 0.3596491228070175517, 0.3640350877192982670, 0.3684210526315789269, 0.3728070175438596423, 0.3771929824561403577, 0.3815789473684210731, 0.3859649122807017330, 0.3903508771929824483, 0.3947368421052631637, 0.3991228070175438791, 0.4035087719298245390, 0.4078947368421052544, 0.4122807017543859698, 0.4166666666666666852, 0.4210526315789473450, 0.4254385964912280604, 0.4298245614035087758, 0.4342105263157894912, 0.4385964912280701511, 0.4429824561403508665, 0.4473684210526315819, 0.4517543859649122973, 0.4561403508771929571, 0.4605263157894736725, 0.4649122807017543879, 0.4692982456140351033, 0.4736842105263157632, 0.4780701754385964786, 0.4824561403508771940, 0.4868421052631579093, 0.4912280701754385692, 0.4956140350877192846, 0.5000000000000000000, 0.5043859649122807154, 0.5087719298245614308, 0.5131578947368421462, 0.5175438596491228616, 0.5219298245614034659, 0.5263157894736841813, 0.5307017543859648967, 0.5350877192982456121, 0.5394736842105263275, 0.5438596491228070429, 0.5482456140350877583, 0.5526315789473684736, 0.5570175438596490780, 0.5614035087719297934, 0.5657894736842105088, 0.5701754385964912242, 0.5745614035087719396, 0.5789473684210526550, 0.5833333333333333703, 0.5877192982456140857, 0.5921052631578946901, 0.5964912280701754055, 0.6008771929824561209, 0.6052631578947368363, 0.6096491228070175517, 0.6140350877192982670, 0.6184210526315789824, 0.6228070175438596978, 0.6271929824561403022, 0.6315789473684210176, 0.6359649122807017330, 0.6403508771929824483, 0.6447368421052631637, 0.6491228070175438791, 0.6535087719298245945, 0.6578947368421053099, 0.6622807017543859143, 0.6666666666666666297, 0.6710526315789473450, 0.6754385964912280604, 0.6798245614035087758, 0.6842105263157894912, 0.6885964912280702066, 0.6929824561403509220, 0.6973684210526315264, 0.7017543859649122417, 0.7061403508771929571, 0.7105263157894736725, 0.7149122807017543879, 0.7192982456140351033, 0.7236842105263158187, 0.7280701754385965341, 0.7324561403508771384, 0.7368421052631578538, 0.7412280701754385692, 0.7456140350877192846, 0.7500000000000000000, 0.7543859649122807154, 0.7587719298245614308, 0.7631578947368421462, 0.7675438596491228616, 0.7719298245614034659, 0.7763157894736841813, 0.7807017543859648967, 0.7850877192982456121, 0.7894736842105263275, 0.7938596491228070429, 0.7982456140350877583, 0.8026315789473684736, 0.8070175438596490780, 0.8114035087719297934, 0.8157894736842105088, 0.8201754385964912242, 0.8245614035087719396, 0.8289473684210526550, 0.8333333333333333703, 0.8377192982456140857, 0.8421052631578946901, 0.8464912280701754055, 0.8508771929824561209, 0.8552631578947368363, 0.8596491228070175517, 0.8640350877192982670, 0.8684210526315789824, 0.8728070175438596978, 0.8771929824561403022, 0.8815789473684210176, 0.8859649122807017330, 0.8903508771929824483, 0.8947368421052631637, 0.8991228070175438791, 0.9035087719298245945, 0.9078947368421053099, 0.9122807017543859143, 0.9166666666666666297, 0.9210526315789473450, 0.9254385964912280604, 0.9298245614035087758, 0.9342105263157894912, 0.9385964912280702066, 0.9429824561403509220, 0.9473684210526315264, 0.9517543859649122417, 0.9561403508771929571, 0.9605263157894736725, 0.9649122807017543879, 0.9692982456140351033, 0.9736842105263158187, 0.9780701754385965341, 0.9824561403508771384, 0.9868421052631578538, 0.9912280701754385692, 0.9956140350877192846, 1.000000000000000000 ),
 .UNSPECIFIED. ) 
 GEOMETRIC_REPRESENTATION_ITEM ( )  RATIONAL_B_SPLINE_SURFACE ( (
 ( 1.000000000000000000, 0.9659258262890683122, 1.000000000000000000, 0.9659258262890683122, 1.000000000000000000, 0.9659258262890683122, 1.000000000000000000, 0.9659258262890683122, 1.000000000000000000, 0.9659258262890683122, 1.000000000000000000, 0.9659258262890683122, 1.000000000000000000, 0.9659258262890683122, 1.000000000000000000, 0.9659258262890683122, 1.000000000000000000, 0.9659258262890683122, 1.000000000000000000, 0.9659258262890683122, 1.000000000000000000, 0.9659258262890683122, 1.000000000000000000, 0.9659258262890683122, 1.000000000000000000, 0.9659258262890683122, 1.000000000000000000, 0.9659258262890683122, 1.000000000000000000, 0.9659258262890683122, 1.000000000000000000, 0.9659258262890683122, 1.000000000000000000, 0.9659258262890683122, 1.000000000000000000, 0.9659258262890683122, 1.000000000000000000, 0.9659258262890683122, 1.000000000000000000, 0.9659258262890683122, 1.000000000000000000, 0.9659258262890683122, 1.000000000000000000, 0.9659258262890683122, 1.000000000000000000, 0.9659258262890683122, 1.000000000000000000, 0.9659258262890683122, 1.000000000000000000, 0.9659258262890683122, 1.000000000000000000, 0.9659258262890683122, 1.000000000000000000, 0.9659258262890683122, 1.000000000000000000, 0.9659258262890683122, 1.000000000000000000, 0.9659258262890683122, 1.000000000000000000, 0.9659258262890683122, 1.000000000000000000, 0.9659258262890683122, 1.000000000000000000, 0.9659258262890683122, 1.000000000000000000, 0.9659258262890683122, 1.000000000000000000, 0.9659258262890683122, 1.000000000000000000, 0.9659258262890683122, 1.000000000000000000, 0.9659258262890683122, 1.000000000000000000, 0.9659258262890683122, 1.000000000000000000, 0.9659258262890683122, 1.000000000000000000, 0.9659258262890683122, 1.000000000000000000, 0.9659258262890683122, 1.000000000000000000, 0.9659258262890683122, 1.000000000000000000, 0.9659258262890683122, 1.000000000000000000, 0.9659258262890683122, 1.000000000000000000, 0.9659258262890683122, 1.000000000000000000, 0.9659258262890683122, 1.000000000000000000, 0.9659258262890683122, 1.000000000000000000, 0.9659258262890683122, 1.000000000000000000, 0.9659258262890683122, 1.000000000000000000, 0.9659258262890683122, 1.000000000000000000, 0.9659258262890683122, 1.000000000000000000, 0.9659258262890683122, 1.000000000000000000, 0.9659258262890683122, 1.000000000000000000, 0.9659258262890683122, 1.000000000000000000, 0.9659258262890683122, 1.000000000000000000, 0.9659258262890683122, 1.000000000000000000, 0.9659258262890683122, 1.000000000000000000, 0.9659258262890683122, 1.000000000000000000, 0.9659258262890683122, 1.000000000000000000, 0.9659258262890683122, 1.000000000000000000, 0.9659258262890683122, 1.000000000000000000, 0.9659258262890683122, 1.000000000000000000, 0.9659258262890683122, 1.000000000000000000, 0.9659258262890683122, 1.000000000000000000, 0.9659258262890683122, 1.000000000000000000, 0.9659258262890683122, 1.000000000000000000, 0.9659258262890683122, 1.000000000000000000, 0.9659258262890683122, 1.000000000000000000, 0.9659258262890683122, 1.000000000000000000, 0.9659258262890683122, 1.000000000000000000, 0.9659258262890683122, 1.000000000000000000, 0.9659258262890683122, 1.000000000000000000, 0.9659258262890683122, 1.000000000000000000, 0.9659258262890683122, 1.000000000000000000, 0.9659258262890683122, 1.000000000000000000, 0.9659258262890683122, 1.000000000000000000, 0.9659258262890683122, 1.000000000000000000, 0.9659258262890683122, 1.000000000000000000, 0.9659258262890683122, 1.000000000000000000, 0.9659258262890683122, 1.000000000000000000, 0.9659258262890683122, 1.000000000000000000, 0.9659258262890683122, 1.000000000000000000, 0.9659258262890683122, 1.000000000000000000, 0.9659258262890683122, 1.000000000000000000, 0.9659258262890683122, 1.000000000000000000, 0.9659258262890683122, 1.000000000000000000, 0.9659258262890683122, 1.000000000000000000, 0.9659258262890683122, 1.000000000000000000, 0.9659258262890683122, 1.000000000000000000, 0.9659258262890683122, 1.000000000000000000, 0.9659258262890683122, 1.000000000000000000, 0.9659258262890683122, 1.000000000000000000, 0.9659258262890683122, 1.000000000000000000, 0.9659258262890683122, 1.000000000000000000, 0.9659258262890683122, 1.000000000000000000, 0.9659258262890683122, 1.000000000000000000, 0.9659258262890683122, 1.000000000000000000, 0.9659258262890683122, 1.000000000000000000, 0.9659258262890683122, 1.000000000000000000, 0.9659258262890683122, 1.000000000000000000, 0.9659258262890683122, 1.000000000000000000, 0.9659258262890683122, 1.000000000000000000, 0.9659258262890683122, 1.000000000000000000, 0.9659258262890683122, 1.000000000000000000, 0.9659258262890683122, 1.000000000000000000, 0.9659258262890683122, 1.000000000000000000, 0.9659258262890683122, 1.000000000000000000, 0.9659258262890683122, 1.000000000000000000, 0.9659258262890683122, 1.000000000000000000, 0.9659258262890683122, 1.000000000000000000, 0.9659258262890683122, 1.000000000000000000, 0.9659258262890683122, 1.000000000000000000, 0.9659258262890683122, 1.000000000000000000, 0.9659258262890683122, 1.000000000000000000, 0.9659258262890683122, 1.000000000000000000, 0.9659258262890683122, 1.000000000000000000, 0.9659258262890683122, 1.000000000000000000, 0.9659258262890683122, 1.000000000000000000, 0.9659258262890683122, 1.000000000000000000, 0.9659258262890683122, 1.000000000000000000, 0.9659258262890683122, 1.000000000000000000, 0.9659258262890683122, 1.000000000000000000, 0.9659258262890683122, 1.000000000000000000, 0.9659258262890683122, 1.000000000000000000, 0.9659258262890683122, 1.000000000000000000, 0.9659258262890683122, 1.000000000000000000, 0.9659258262890683122, 1.000000000000000000, 0.9659258262890683122, 1.000000000000000000, 0.9659258262890683122, 1.000000000000000000, 0.9659258262890683122, 1.000000000000000000, 0.9659258262890683122, 1.000000000000000000, 0.9659258262890683122, 1.000000000000000000, 0.9659258262890683122, 1.000000000000000000, 0.9659258262890683122, 1.000000000000000000, 0.9659258262890683122, 1.000000000000000000, 0.9659258262890683122, 1.000000000000000000, 0.9659258262890683122, 1.000000000000000000, 0.9659258262890683122, 1.000000000000000000, 0.9659258262890683122, 1.000000000000000000, 0.9659258262890683122, 1.000000000000000000, 0.9659258262890683122, 1.000000000000000000, 0.9659258262890683122, 1.000000000000000000, 0.9659258262890683122, 1.000000000000000000, 0.9659258262890683122, 1.000000000000000000, 0.9659258262890683122, 1.000000000000000000, 0.9659258262890683122, 1.000000000000000000, 0.9659258262890683122, 1.000000000000000000, 0.9659258262890683122, 1.000000000000000000, 0.9659258262890683122, 1.000000000000000000, 0.9659258262890683122, 1.000000000000000000, 0.9659258262890683122, 1.000000000000000000, 0.9659258262890683122, 1.000000000000000000, 0.9659258262890683122, 1.000000000000000000, 0.9659258262890683122, 1.000000000000000000, 0.9659258262890683122, 1.000000000000000000, 0.9659258262890683122, 1.000000000000000000, 0.9659258262890683122, 1.000000000000000000, 0.9659258262890683122, 1.000000000000000000, 0.9659258262890683122, 1.000000000000000000, 0.9659258262890683122, 1.000000000000000000, 0.9659258262890683122, 1.000000000000000000, 0.9659258262890683122, 1.000000000000000000, 0.9659258262890683122, 1.000000000000000000, 0.9659258262890683122, 1.000000000000000000, 0.9659258262890683122, 1.000000000000000000, 0.9659258262890683122, 1.000000000000000000, 0.9659258262890683122, 1.000000000000000000, 0.9659258262890683122, 1.000000000000000000, 0.9659258262890683122, 1.000000000000000000, 0.9659258262890683122, 1.000000000000000000, 0.9659258262890683122, 1.000000000000000000, 0.9659258262890683122, 1.000000000000000000, 0.9659258262890683122, 1.000000000000000000, 0.9659258262890683122, 1.000000000000000000, 0.9659258262890683122, 1.000000000000000000, 0.9659258262890683122, 1.000000000000000000, 0.9659258262890683122, 1.000000000000000000, 0.9659258262890683122, 1.000000000000000000, 0.9659258262890683122, 1.000000000000000000, 0.9659258262890683122, 1.000000000000000000, 0.9659258262890683122, 1.000000000000000000, 0.9659258262890683122, 1.000000000000000000, 0.9659258262890683122, 1.000000000000000000, 0.9659258262890683122, 1.000000000000000000, 0.9659258262890683122, 1.000000000000000000, 0.9659258262890683122, 1.000000000000000000, 0.9659258262890683122, 1.000000000000000000, 0.9659258262890683122, 1.000000000000000000, 0.9659258262890683122, 1.000000000000000000, 0.9659258262890683122, 1.000000000000000000, 0.9659258262890683122, 1.000000000000000000, 0.9659258262890683122, 1.000000000000000000, 0.9659258262890683122, 1.000000000000000000, 0.9659258262890683122, 1.000000000000000000, 0.9659258262890683122, 1.000000000000000000, 0.9659258262890683122, 1.000000000000000000, 0.9659258262890683122, 1.000000000000000000, 0.9659258262890683122, 1.000000000000000000, 0.9659258262890683122, 1.000000000000000000, 0.9659258262890683122, 1.000000000000000000, 0.9659258262890683122, 1.000000000000000000, 0.9659258262890683122, 1.000000000000000000, 0.9659258262890683122, 1.000000000000000000, 0.9659258262890683122, 1.000000000000000000, 0.9659258262890683122, 1.000000000000000000, 0.9659258262890683122, 1.000000000000000000, 0.9659258262890683122, 1.000000000000000000, 0.9659258262890683122, 1.000000000000000000, 0.9659258262890683122, 1.000000000000000000, 0.9659258262890683122, 1.000000000000000000, 0.9659258262890683122, 1.000000000000000000, 0.9659258262890683122, 1.000000000000000000, 0.9659258262890683122, 1.000000000000000000, 0.9659258262890683122, 1.000000000000000000, 0.9659258262890683122, 1.000000000000000000, 0.9659258262890683122, 1.000000000000000000, 0.9659258262890683122, 1.000000000000000000, 0.9659258262890683122, 1.000000000000000000, 0.9659258262890683122, 1.000000000000000000, 0.9659258262890683122, 1.000000000000000000, 0.9659258262890683122, 1.000000000000000000, 0.9659258262890683122, 1.000000000000000000, 0.9659258262890683122, 1.000000000000000000, 0.9659258262890683122, 1.000000000000000000, 0.9659258262890683122, 1.000000000000000000, 0.9659258262890683122, 1.000000000000000000, 0.9659258262890683122, 1.000000000000000000, 0.9659258262890683122, 1.000000000000000000, 0.9659258262890683122, 1.000000000000000000),
 ( 0.3333333333333333703, 0.3219752754296894559, 0.3333333333333333703, 0.3219752754296894559, 0.3333333333333333703, 0.3219752754296894559, 0.3333333333333333703, 0.3219752754296894559, 0.3333333333333333703, 0.3219752754296894559, 0.3333333333333333703, 0.3219752754296894559, 0.3333333333333333703, 0.3219752754296894559, 0.3333333333333333703, 0.3219752754296894559, 0.3333333333333333703, 0.3219752754296894559, 0.3333333333333333703, 0.3219752754296894559, 0.3333333333333333703, 0.3219752754296894559, 0.3333333333333333703, 0.3219752754296894559, 0.3333333333333333703, 0.3219752754296894559, 0.3333333333333333703, 0.3219752754296894559, 0.3333333333333333703, 0.3219752754296894559, 0.3333333333333333703, 0.3219752754296894559, 0.3333333333333333703, 0.3219752754296894559, 0.3333333333333333703, 0.3219752754296894559, 0.3333333333333333703, 0.3219752754296894559, 0.3333333333333333703, 0.3219752754296894559, 0.3333333333333333703, 0.3219752754296894559, 0.3333333333333333703, 0.3219752754296894559, 0.3333333333333333703, 0.3219752754296894559, 0.3333333333333333703, 0.3219752754296894559, 0.3333333333333333703, 0.3219752754296894559, 0.3333333333333333703, 0.3219752754296894559, 0.3333333333333333703, 0.3219752754296894559, 0.3333333333333333703, 0.3219752754296894559, 0.3333333333333333703, 0.3219752754296894559, 0.3333333333333333703, 0.3219752754296894559, 0.3333333333333333703, 0.3219752754296894559, 0.3333333333333333703, 0.3219752754296894559, 0.3333333333333333703, 0.3219752754296894559, 0.3333333333333333703, 0.3219752754296894559, 0.3333333333333333703, 0.3219752754296894559, 0.3333333333333333703, 0.3219752754296894559, 0.3333333333333333703, 0.3219752754296894559, 0.3333333333333333703, 0.3219752754296894559, 0.3333333333333333703, 0.3219752754296894559, 0.3333333333333333703, 0.3219752754296894559, 0.3333333333333333703, 0.3219752754296894559, 0.3333333333333333703, 0.3219752754296894559, 0.3333333333333333703, 0.3219752754296894559, 0.3333333333333333703, 0.3219752754296894559, 0.3333333333333333703, 0.3219752754296894559, 0.3333333333333333703, 0.3219752754296894559, 0.3333333333333333703, 0.3219752754296894559, 0.3333333333333333703, 0.3219752754296894559, 0.3333333333333333703, 0.3219752754296894559, 0.3333333333333333703, 0.3219752754296894559, 0.3333333333333333703, 0.3219752754296894559, 0.3333333333333333703, 0.3219752754296894559, 0.3333333333333333703, 0.3219752754296894559, 0.3333333333333333703, 0.3219752754296894559, 0.3333333333333333703, 0.3219752754296894559, 0.3333333333333333703, 0.3219752754296894559, 0.3333333333333333703, 0.3219752754296894559, 0.3333333333333333703, 0.3219752754296894559, 0.3333333333333333703, 0.3219752754296894559, 0.3333333333333333703, 0.3219752754296894559, 0.3333333333333333703, 0.3219752754296894559, 0.3333333333333333703, 0.3219752754296894559, 0.3333333333333333703, 0.3219752754296894559, 0.3333333333333333703, 0.3219752754296894559, 0.3333333333333333703, 0.3219752754296894559, 0.3333333333333333703, 0.3219752754296894559, 0.3333333333333333703, 0.3219752754296894559, 0.3333333333333333703, 0.3219752754296894559, 0.3333333333333333703, 0.3219752754296894559, 0.3333333333333333703, 0.3219752754296894559, 0.3333333333333333703, 0.3219752754296894559, 0.3333333333333333703, 0.3219752754296894559, 0.3333333333333333703, 0.3219752754296894559, 0.3333333333333333703, 0.3219752754296894559, 0.3333333333333333703, 0.3219752754296894559, 0.3333333333333333703, 0.3219752754296894559, 0.3333333333333333703, 0.3219752754296894559, 0.3333333333333333703, 0.3219752754296894559, 0.3333333333333333703, 0.3219752754296894559, 0.3333333333333333703, 0.3219752754296894559, 0.3333333333333333703, 0.3219752754296894559, 0.3333333333333333703, 0.3219752754296894559, 0.3333333333333333703, 0.3219752754296894559, 0.3333333333333333703, 0.3219752754296894559, 0.3333333333333333703, 0.3219752754296894559, 0.3333333333333333703, 0.3219752754296894559, 0.3333333333333333703, 0.3219752754296894559, 0.3333333333333333703, 0.3219752754296894559, 0.3333333333333333703, 0.3219752754296894559, 0.3333333333333333703, 0.3219752754296894559, 0.3333333333333333703, 0.3219752754296894559, 0.3333333333333333703, 0.3219752754296894559, 0.3333333333333333703, 0.3219752754296894559, 0.3333333333333333703, 0.3219752754296894559, 0.3333333333333333703, 0.3219752754296894559, 0.3333333333333333703, 0.3219752754296894559, 0.3333333333333333703, 0.3219752754296894559, 0.3333333333333333703, 0.3219752754296894559, 0.3333333333333333703, 0.3219752754296894559, 0.3333333333333333703, 0.3219752754296894559, 0.3333333333333333703, 0.3219752754296894559, 0.3333333333333333703, 0.3219752754296894559, 0.3333333333333333703, 0.3219752754296894559, 0.3333333333333333703, 0.3219752754296894559, 0.3333333333333333703, 0.3219752754296894559, 0.3333333333333333703, 0.3219752754296894559, 0.3333333333333333703, 0.3219752754296894559, 0.3333333333333333703, 0.3219752754296894559, 0.3333333333333333703, 0.3219752754296894559, 0.3333333333333333703, 0.3219752754296894559, 0.3333333333333333703, 0.3219752754296894559, 0.3333333333333333703, 0.3219752754296894559, 0.3333333333333333703, 0.3219752754296894559, 0.3333333333333333703, 0.3219752754296894559, 0.3333333333333333703, 0.3219752754296894559, 0.3333333333333333703, 0.3219752754296894559, 0.3333333333333333703, 0.3219752754296894559, 0.3333333333333333703, 0.3219752754296894559, 0.3333333333333333703, 0.3219752754296894559, 0.3333333333333333703, 0.3219752754296894559, 0.3333333333333333703, 0.3219752754296894559, 0.3333333333333333703, 0.3219752754296894559, 0.3333333333333333703, 0.3219752754296894559, 0.3333333333333333703, 0.3219752754296894559, 0.3333333333333333703, 0.3219752754296894559, 0.3333333333333333703, 0.3219752754296894559, 0.3333333333333333703, 0.3219752754296894559, 0.3333333333333333703, 0.3219752754296894559, 0.3333333333333333703, 0.3219752754296894559, 0.3333333333333333703, 0.3219752754296894559, 0.3333333333333333703, 0.3219752754296894559, 0.3333333333333333703, 0.3219752754296894559, 0.3333333333333333703, 0.3219752754296894559, 0.3333333333333333703, 0.3219752754296894559, 0.3333333333333333703, 0.3219752754296894559, 0.3333333333333333703, 0.3219752754296894559, 0.3333333333333333703, 0.3219752754296894559, 0.3333333333333333703, 0.3219752754296894559, 0.3333333333333333703, 0.3219752754296894559, 0.3333333333333333703, 0.3219752754296894559, 0.3333333333333333703, 0.3219752754296894559, 0.3333333333333333703, 0.3219752754296894559, 0.3333333333333333703, 0.3219752754296894559, 0.3333333333333333703, 0.3219752754296894559, 0.3333333333333333703, 0.3219752754296894559, 0.3333333333333333703, 0.3219752754296894559, 0.3333333333333333703, 0.3219752754296894559, 0.3333333333333333703, 0.3219752754296894559, 0.3333333333333333703, 0.3219752754296894559, 0.3333333333333333703, 0.3219752754296894559, 0.3333333333333333703, 0.3219752754296894559, 0.3333333333333333703, 0.3219752754296894559, 0.3333333333333333703, 0.3219752754296894559, 0.3333333333333333703, 0.3219752754296894559, 0.3333333333333333703, 0.3219752754296894559, 0.3333333333333333703, 0.3219752754296894559, 0.3333333333333333703, 0.3219752754296894559, 0.3333333333333333703, 0.3219752754296894559, 0.3333333333333333703, 0.3219752754296894559, 0.3333333333333333703, 0.3219752754296894559, 0.3333333333333333703, 0.3219752754296894559, 0.3333333333333333703, 0.3219752754296894559, 0.3333333333333333703, 0.3219752754296894559, 0.3333333333333333703, 0.3219752754296894559, 0.3333333333333333703, 0.3219752754296894559, 0.3333333333333333703, 0.3219752754296894559, 0.3333333333333333703, 0.3219752754296894559, 0.3333333333333333703, 0.3219752754296894559, 0.3333333333333333703, 0.3219752754296894559, 0.3333333333333333703, 0.3219752754296894559, 0.3333333333333333703, 0.3219752754296894559, 0.3333333333333333703, 0.3219752754296894559, 0.3333333333333333703, 0.3219752754296894559, 0.3333333333333333703, 0.3219752754296894559, 0.3333333333333333703, 0.3219752754296894559, 0.3333333333333333703, 0.3219752754296894559, 0.3333333333333333703, 0.3219752754296894559, 0.3333333333333333703, 0.3219752754296894559, 0.3333333333333333703, 0.3219752754296894559, 0.3333333333333333703, 0.3219752754296894559, 0.3333333333333333703, 0.3219752754296894559, 0.3333333333333333703, 0.3219752754296894559, 0.3333333333333333703, 0.3219752754296894559, 0.3333333333333333703, 0.3219752754296894559, 0.3333333333333333703, 0.3219752754296894559, 0.3333333333333333703, 0.3219752754296894559, 0.3333333333333333703, 0.3219752754296894559, 0.3333333333333333703, 0.3219752754296894559, 0.3333333333333333703, 0.3219752754296894559, 0.3333333333333333703, 0.3219752754296894559, 0.3333333333333333703, 0.3219752754296894559, 0.3333333333333333703, 0.3219752754296894559, 0.3333333333333333703, 0.3219752754296894559, 0.3333333333333333703, 0.3219752754296894559, 0.3333333333333333703, 0.3219752754296894559, 0.3333333333333333703, 0.3219752754296894559, 0.3333333333333333703, 0.3219752754296894559, 0.3333333333333333703, 0.3219752754296894559, 0.3333333333333333703, 0.3219752754296894559, 0.3333333333333333703, 0.3219752754296894559, 0.3333333333333333703, 0.3219752754296894559, 0.3333333333333333703, 0.3219752754296894559, 0.3333333333333333703, 0.3219752754296894559, 0.3333333333333333703, 0.3219752754296894559, 0.3333333333333333703, 0.3219752754296894559, 0.3333333333333333703, 0.3219752754296894559, 0.3333333333333333703, 0.3219752754296894559, 0.3333333333333333703, 0.3219752754296894559, 0.3333333333333333703, 0.3219752754296894559, 0.3333333333333333703, 0.3219752754296894559, 0.3333333333333333703, 0.3219752754296894559, 0.3333333333333333703, 0.3219752754296894559, 0.3333333333333333703, 0.3219752754296894559, 0.3333333333333333703, 0.3219752754296894559, 0.3333333333333333703, 0.3219752754296894559, 0.3333333333333333703, 0.3219752754296894559, 0.3333333333333333703, 0.3219752754296894559, 0.3333333333333333703, 0.3219752754296894559, 0.3333333333333333703, 0.3219752754296894559, 0.3333333333333333703, 0.3219752754296894559, 0.3333333333333333703, 0.3219752754296894559, 0.3333333333333333703, 0.3219752754296894559, 0.3333333333333333703, 0.3219752754296894559, 0.3333333333333333703, 0.3219752754296894559, 0.3333333333333333703, 0.3219752754296894559, 0.3333333333333333703, 0.3219752754296894559, 0.3333333333333333703, 0.3219752754296894559, 0.3333333333333333703, 0.3219752754296894559, 0.3333333333333333703),
 ( 0.3333333333333333703, 0.3219752754296894559, 0.3333333333333333703, 0.3219752754296894559, 0.3333333333333333703, 0.3219752754296894559, 0.3333333333333333703, 0.3219752754296894559, 0.3333333333333333703, 0.3219752754296894559, 0.3333333333333333703, 0.3219752754296894559, 0.3333333333333333703, 0.3219752754296894559, 0.3333333333333333703, 0.3219752754296894559, 0.3333333333333333703, 0.3219752754296894559, 0.3333333333333333703, 0.3219752754296894559, 0.3333333333333333703, 0.3219752754296894559, 0.3333333333333333703, 0.3219752754296894559, 0.3333333333333333703, 0.3219752754296894559, 0.3333333333333333703, 0.3219752754296894559, 0.3333333333333333703, 0.3219752754296894559, 0.3333333333333333703, 0.3219752754296894559, 0.3333333333333333703, 0.3219752754296894559, 0.3333333333333333703, 0.3219752754296894559, 0.3333333333333333703, 0.3219752754296894559, 0.3333333333333333703, 0.3219752754296894559, 0.3333333333333333703, 0.3219752754296894559, 0.3333333333333333703, 0.3219752754296894559, 0.3333333333333333703, 0.3219752754296894559, 0.3333333333333333703, 0.3219752754296894559, 0.3333333333333333703, 0.3219752754296894559, 0.3333333333333333703, 0.3219752754296894559, 0.3333333333333333703, 0.3219752754296894559, 0.3333333333333333703, 0.3219752754296894559, 0.3333333333333333703, 0.3219752754296894559, 0.3333333333333333703, 0.3219752754296894559, 0.3333333333333333703, 0.3219752754296894559, 0.3333333333333333703, 0.3219752754296894559, 0.3333333333333333703, 0.3219752754296894559, 0.3333333333333333703, 0.3219752754296894559, 0.3333333333333333703, 0.3219752754296894559, 0.3333333333333333703, 0.3219752754296894559, 0.3333333333333333703, 0.3219752754296894559, 0.3333333333333333703, 0.3219752754296894559, 0.3333333333333333703, 0.3219752754296894559, 0.3333333333333333703, 0.3219752754296894559, 0.3333333333333333703, 0.3219752754296894559, 0.3333333333333333703, 0.3219752754296894559, 0.3333333333333333703, 0.3219752754296894559, 0.3333333333333333703, 0.3219752754296894559, 0.3333333333333333703, 0.3219752754296894559, 0.3333333333333333703, 0.3219752754296894559, 0.3333333333333333703, 0.3219752754296894559, 0.3333333333333333703, 0.3219752754296894559, 0.3333333333333333703, 0.3219752754296894559, 0.3333333333333333703, 0.3219752754296894559, 0.3333333333333333703, 0.3219752754296894559, 0.3333333333333333703, 0.3219752754296894559, 0.3333333333333333703, 0.3219752754296894559, 0.3333333333333333703, 0.3219752754296894559, 0.3333333333333333703, 0.3219752754296894559, 0.3333333333333333703, 0.3219752754296894559, 0.3333333333333333703, 0.3219752754296894559, 0.3333333333333333703, 0.3219752754296894559, 0.3333333333333333703, 0.3219752754296894559, 0.3333333333333333703, 0.3219752754296894559, 0.3333333333333333703, 0.3219752754296894559, 0.3333333333333333703, 0.3219752754296894559, 0.3333333333333333703, 0.3219752754296894559, 0.3333333333333333703, 0.3219752754296894559, 0.3333333333333333703, 0.3219752754296894559, 0.3333333333333333703, 0.3219752754296894559, 0.3333333333333333703, 0.3219752754296894559, 0.3333333333333333703, 0.3219752754296894559, 0.3333333333333333703, 0.3219752754296894559, 0.3333333333333333703, 0.3219752754296894559, 0.3333333333333333703, 0.3219752754296894559, 0.3333333333333333703, 0.3219752754296894559, 0.3333333333333333703, 0.3219752754296894559, 0.3333333333333333703, 0.3219752754296894559, 0.3333333333333333703, 0.3219752754296894559, 0.3333333333333333703, 0.3219752754296894559, 0.3333333333333333703, 0.3219752754296894559, 0.3333333333333333703, 0.3219752754296894559, 0.3333333333333333703, 0.3219752754296894559, 0.3333333333333333703, 0.3219752754296894559, 0.3333333333333333703, 0.3219752754296894559, 0.3333333333333333703, 0.3219752754296894559, 0.3333333333333333703, 0.3219752754296894559, 0.3333333333333333703, 0.3219752754296894559, 0.3333333333333333703, 0.3219752754296894559, 0.3333333333333333703, 0.3219752754296894559, 0.3333333333333333703, 0.3219752754296894559, 0.3333333333333333703, 0.3219752754296894559, 0.3333333333333333703, 0.3219752754296894559, 0.3333333333333333703, 0.3219752754296894559, 0.3333333333333333703, 0.3219752754296894559, 0.3333333333333333703, 0.3219752754296894559, 0.3333333333333333703, 0.3219752754296894559, 0.3333333333333333703, 0.3219752754296894559, 0.3333333333333333703, 0.3219752754296894559, 0.3333333333333333703, 0.3219752754296894559, 0.3333333333333333703, 0.3219752754296894559, 0.3333333333333333703, 0.3219752754296894559, 0.3333333333333333703, 0.3219752754296894559, 0.3333333333333333703, 0.3219752754296894559, 0.3333333333333333703, 0.3219752754296894559, 0.3333333333333333703, 0.3219752754296894559, 0.3333333333333333703, 0.3219752754296894559, 0.3333333333333333703, 0.3219752754296894559, 0.3333333333333333703, 0.3219752754296894559, 0.3333333333333333703, 0.3219752754296894559, 0.3333333333333333703, 0.3219752754296894559, 0.3333333333333333703, 0.3219752754296894559, 0.3333333333333333703, 0.3219752754296894559, 0.3333333333333333703, 0.3219752754296894559, 0.3333333333333333703, 0.3219752754296894559, 0.3333333333333333703, 0.3219752754296894559, 0.3333333333333333703, 0.3219752754296894559, 0.3333333333333333703, 0.3219752754296894559, 0.3333333333333333703, 0.3219752754296894559, 0.3333333333333333703, 0.3219752754296894559, 0.3333333333333333703, 0.3219752754296894559, 0.3333333333333333703, 0.3219752754296894559, 0.3333333333333333703, 0.3219752754296894559, 0.3333333333333333703, 0.3219752754296894559, 0.3333333333333333703, 0.3219752754296894559, 0.3333333333333333703, 0.3219752754296894559, 0.3333333333333333703, 0.3219752754296894559, 0.3333333333333333703, 0.3219752754296894559, 0.3333333333333333703, 0.3219752754296894559, 0.3333333333333333703, 0.3219752754296894559, 0.3333333333333333703, 0.3219752754296894559, 0.3333333333333333703, 0.3219752754296894559, 0.3333333333333333703, 0.3219752754296894559, 0.3333333333333333703, 0.3219752754296894559, 0.3333333333333333703, 0.3219752754296894559, 0.3333333333333333703, 0.3219752754296894559, 0.3333333333333333703, 0.3219752754296894559, 0.3333333333333333703, 0.3219752754296894559, 0.3333333333333333703, 0.3219752754296894559, 0.3333333333333333703, 0.3219752754296894559, 0.3333333333333333703, 0.3219752754296894559, 0.3333333333333333703, 0.3219752754296894559, 0.3333333333333333703, 0.3219752754296894559, 0.3333333333333333703, 0.3219752754296894559, 0.3333333333333333703, 0.3219752754296894559, 0.3333333333333333703, 0.3219752754296894559, 0.3333333333333333703, 0.3219752754296894559, 0.3333333333333333703, 0.3219752754296894559, 0.3333333333333333703, 0.3219752754296894559, 0.3333333333333333703, 0.3219752754296894559, 0.3333333333333333703, 0.3219752754296894559, 0.3333333333333333703, 0.3219752754296894559, 0.3333333333333333703, 0.3219752754296894559, 0.3333333333333333703, 0.3219752754296894559, 0.3333333333333333703, 0.3219752754296894559, 0.3333333333333333703, 0.3219752754296894559, 0.3333333333333333703, 0.3219752754296894559, 0.3333333333333333703, 0.3219752754296894559, 0.3333333333333333703, 0.3219752754296894559, 0.3333333333333333703, 0.3219752754296894559, 0.3333333333333333703, 0.3219752754296894559, 0.3333333333333333703, 0.3219752754296894559, 0.3333333333333333703, 0.3219752754296894559, 0.3333333333333333703, 0.3219752754296894559, 0.3333333333333333703, 0.3219752754296894559, 0.3333333333333333703, 0.3219752754296894559, 0.3333333333333333703, 0.3219752754296894559, 0.3333333333333333703, 0.3219752754296894559, 0.3333333333333333703, 0.3219752754296894559, 0.3333333333333333703, 0.3219752754296894559, 0.3333333333333333703, 0.3219752754296894559, 0.3333333333333333703, 0.3219752754296894559, 0.3333333333333333703, 0.3219752754296894559, 0.3333333333333333703, 0.3219752754296894559, 0.3333333333333333703, 0.3219752754296894559, 0.3333333333333333703, 0.3219752754296894559, 0.3333333333333333703, 0.3219752754296894559, 0.3333333333333333703, 0.3219752754296894559, 0.3333333333333333703, 0.3219752754296894559, 0.3333333333333333703, 0.3219752754296894559, 0.3333333333333333703, 0.3219752754296894559, 0.3333333333333333703, 0.3219752754296894559, 0.3333333333333333703, 0.3219752754296894559, 0.3333333333333333703, 0.3219752754296894559, 0.3333333333333333703, 0.3219752754296894559, 0.3333333333333333703, 0.3219752754296894559, 0.3333333333333333703, 0.3219752754296894559, 0.3333333333333333703, 0.3219752754296894559, 0.3333333333333333703, 0.3219752754296894559, 0.3333333333333333703, 0.3219752754296894559, 0.3333333333333333703, 0.3219752754296894559, 0.3333333333333333703, 0.3219752754296894559, 0.3333333333333333703, 0.3219752754296894559, 0.3333333333333333703, 0.3219752754296894559, 0.3333333333333333703, 0.3219752754296894559, 0.3333333333333333703, 0.3219752754296894559, 0.3333333333333333703, 0.3219752754296894559, 0.3333333333333333703, 0.3219752754296894559, 0.3333333333333333703, 0.3219752754296894559, 0.3333333333333333703, 0.3219752754296894559, 0.3333333333333333703, 0.3219752754296894559, 0.3333333333333333703, 0.3219752754296894559, 0.3333333333333333703, 0.3219752754296894559, 0.3333333333333333703, 0.3219752754296894559, 0.3333333333333333703, 0.3219752754296894559, 0.3333333333333333703, 0.3219752754296894559, 0.3333333333333333703, 0.3219752754296894559, 0.3333333333333333703, 0.3219752754296894559, 0.3333333333333333703, 0.3219752754296894559, 0.3333333333333333703, 0.3219752754296894559, 0.3333333333333333703, 0.3219752754296894559, 0.3333333333333333703, 0.3219752754296894559, 0.3333333333333333703, 0.3219752754296894559, 0.3333333333333333703, 0.3219752754296894559, 0.3333333333333333703, 0.3219752754296894559, 0.3333333333333333703, 0.3219752754296894559, 0.3333333333333333703, 0.3219752754296894559, 0.3333333333333333703, 0.3219752754296894559, 0.3333333333333333703, 0.3219752754296894559, 0.3333333333333333703, 0.3219752754296894559, 0.3333333333333333703, 0.3219752754296894559, 0.3333333333333333703, 0.3219752754296894559, 0.3333333333333333703, 0.3219752754296894559, 0.3333333333333333703, 0.3219752754296894559, 0.3333333333333333703, 0.3219752754296894559, 0.3333333333333333703, 0.3219752754296894559, 0.3333333333333333703, 0.3219752754296894559, 0.3333333333333333703, 0.3219752754296894559, 0.3333333333333333703, 0.3219752754296894559, 0.3333333333333333703, 0.3219752754296894559, 0.3333333333333333703, 0.3219752754296894559, 0.3333333333333333703, 0.3219752754296894559, 0.3333333333333333703),
 ( 1.000000000000000000, 0.9659258262890683122, 1.000000000000000000, 0.9659258262890683122, 1.000000000000000000, 0.9659258262890683122, 1.000000000000000000, 0.9659258262890683122, 1.000000000000000000, 0.9659258262890683122, 1.000000000000000000, 0.9659258262890683122, 1.000000000000000000, 0.9659258262890683122, 1.000000000000000000, 0.9659258262890683122, 1.000000000000000000, 0.9659258262890683122, 1.000000000000000000, 0.9659258262890683122, 1.000000000000000000, 0.9659258262890683122, 1.000000000000000000, 0.9659258262890683122, 1.000000000000000000, 0.9659258262890683122, 1.000000000000000000, 0.9659258262890683122, 1.000000000000000000, 0.9659258262890683122, 1.000000000000000000, 0.9659258262890683122, 1.000000000000000000, 0.9659258262890683122, 1.000000000000000000, 0.9659258262890683122, 1.000000000000000000, 0.9659258262890683122, 1.000000000000000000, 0.9659258262890683122, 1.000000000000000000, 0.9659258262890683122, 1.000000000000000000, 0.9659258262890683122, 1.000000000000000000, 0.9659258262890683122, 1.000000000000000000, 0.9659258262890683122, 1.000000000000000000, 0.9659258262890683122, 1.000000000000000000, 0.9659258262890683122, 1.000000000000000000, 0.9659258262890683122, 1.000000000000000000, 0.9659258262890683122, 1.000000000000000000, 0.9659258262890683122, 1.000000000000000000, 0.9659258262890683122, 1.000000000000000000, 0.9659258262890683122, 1.000000000000000000, 0.9659258262890683122, 1.000000000000000000, 0.9659258262890683122, 1.000000000000000000, 0.9659258262890683122, 1.000000000000000000, 0.9659258262890683122, 1.000000000000000000, 0.9659258262890683122, 1.000000000000000000, 0.9659258262890683122, 1.000000000000000000, 0.9659258262890683122, 1.000000000000000000, 0.9659258262890683122, 1.000000000000000000, 0.9659258262890683122, 1.000000000000000000, 0.9659258262890683122, 1.000000000000000000, 0.9659258262890683122, 1.000000000000000000, 0.9659258262890683122, 1.000000000000000000, 0.9659258262890683122, 1.000000000000000000, 0.9659258262890683122, 1.000000000000000000, 0.9659258262890683122, 1.000000000000000000, 0.9659258262890683122, 1.000000000000000000, 0.9659258262890683122, 1.000000000000000000, 0.9659258262890683122, 1.000000000000000000, 0.9659258262890683122, 1.000000000000000000, 0.9659258262890683122, 1.000000000000000000, 0.9659258262890683122, 1.000000000000000000, 0.9659258262890683122, 1.000000000000000000, 0.9659258262890683122, 1.000000000000000000, 0.9659258262890683122, 1.000000000000000000, 0.9659258262890683122, 1.000000000000000000, 0.9659258262890683122, 1.000000000000000000, 0.9659258262890683122, 1.000000000000000000, 0.9659258262890683122, 1.000000000000000000, 0.9659258262890683122, 1.000000000000000000, 0.9659258262890683122, 1.000000000000000000, 0.9659258262890683122, 1.000000000000000000, 0.9659258262890683122, 1.000000000000000000, 0.9659258262890683122, 1.000000000000000000, 0.9659258262890683122, 1.000000000000000000, 0.9659258262890683122, 1.000000000000000000, 0.9659258262890683122, 1.000000000000000000, 0.9659258262890683122, 1.000000000000000000, 0.9659258262890683122, 1.000000000000000000, 0.9659258262890683122, 1.000000000000000000, 0.9659258262890683122, 1.000000000000000000, 0.9659258262890683122, 1.000000000000000000, 0.9659258262890683122, 1.000000000000000000, 0.9659258262890683122, 1.000000000000000000, 0.9659258262890683122, 1.000000000000000000, 0.9659258262890683122, 1.000000000000000000, 0.9659258262890683122, 1.000000000000000000, 0.9659258262890683122, 1.000000000000000000, 0.9659258262890683122, 1.000000000000000000, 0.9659258262890683122, 1.000000000000000000, 0.9659258262890683122, 1.000000000000000000, 0.9659258262890683122, 1.000000000000000000, 0.9659258262890683122, 1.000000000000000000, 0.9659258262890683122, 1.000000000000000000, 0.9659258262890683122, 1.000000000000000000, 0.9659258262890683122, 1.000000000000000000, 0.9659258262890683122, 1.000000000000000000, 0.9659258262890683122, 1.000000000000000000, 0.9659258262890683122, 1.000000000000000000, 0.9659258262890683122, 1.000000000000000000, 0.9659258262890683122, 1.000000000000000000, 0.9659258262890683122, 1.000000000000000000, 0.9659258262890683122, 1.000000000000000000, 0.9659258262890683122, 1.000000000000000000, 0.9659258262890683122, 1.000000000000000000, 0.9659258262890683122, 1.000000000000000000, 0.9659258262890683122, 1.000000000000000000, 0.9659258262890683122, 1.000000000000000000, 0.9659258262890683122, 1.000000000000000000, 0.9659258262890683122, 1.000000000000000000, 0.9659258262890683122, 1.000000000000000000, 0.9659258262890683122, 1.000000000000000000, 0.9659258262890683122, 1.000000000000000000, 0.9659258262890683122, 1.000000000000000000, 0.9659258262890683122, 1.000000000000000000, 0.9659258262890683122, 1.000000000000000000, 0.9659258262890683122, 1.000000000000000000, 0.9659258262890683122, 1.000000000000000000, 0.9659258262890683122, 1.000000000000000000, 0.9659258262890683122, 1.000000000000000000, 0.9659258262890683122, 1.000000000000000000, 0.9659258262890683122, 1.000000000000000000, 0.9659258262890683122, 1.000000000000000000, 0.9659258262890683122, 1.000000000000000000, 0.9659258262890683122, 1.000000000000000000, 0.9659258262890683122, 1.000000000000000000, 0.9659258262890683122, 1.000000000000000000, 0.9659258262890683122, 1.000000000000000000, 0.9659258262890683122, 1.000000000000000000, 0.9659258262890683122, 1.000000000000000000, 0.9659258262890683122, 1.000000000000000000, 0.9659258262890683122, 1.000000000000000000, 0.9659258262890683122, 1.000000000000000000, 0.9659258262890683122, 1.000000000000000000, 0.9659258262890683122, 1.000000000000000000, 0.9659258262890683122, 1.000000000000000000, 0.9659258262890683122, 1.000000000000000000, 0.9659258262890683122, 1.000000000000000000, 0.9659258262890683122, 1.000000000000000000, 0.9659258262890683122, 1.000000000000000000, 0.9659258262890683122, 1.000000000000000000, 0.9659258262890683122, 1.000000000000000000, 0.9659258262890683122, 1.000000000000000000, 0.9659258262890683122, 1.000000000000000000, 0.9659258262890683122, 1.000000000000000000, 0.9659258262890683122, 1.000000000000000000, 0.9659258262890683122, 1.000000000000000000, 0.9659258262890683122, 1.000000000000000000, 0.9659258262890683122, 1.000000000000000000, 0.9659258262890683122, 1.000000000000000000, 0.9659258262890683122, 1.000000000000000000, 0.9659258262890683122, 1.000000000000000000, 0.9659258262890683122, 1.000000000000000000, 0.9659258262890683122, 1.000000000000000000, 0.9659258262890683122, 1.000000000000000000, 0.9659258262890683122, 1.000000000000000000, 0.9659258262890683122, 1.000000000000000000, 0.9659258262890683122, 1.000000000000000000, 0.9659258262890683122, 1.000000000000000000, 0.9659258262890683122, 1.000000000000000000, 0.9659258262890683122, 1.000000000000000000, 0.9659258262890683122, 1.000000000000000000, 0.9659258262890683122, 1.000000000000000000, 0.9659258262890683122, 1.000000000000000000, 0.9659258262890683122, 1.000000000000000000, 0.9659258262890683122, 1.000000000000000000, 0.9659258262890683122, 1.000000000000000000, 0.9659258262890683122, 1.000000000000000000, 0.9659258262890683122, 1.000000000000000000, 0.9659258262890683122, 1.000000000000000000, 0.9659258262890683122, 1.000000000000000000, 0.9659258262890683122, 1.000000000000000000, 0.9659258262890683122, 1.000000000000000000, 0.9659258262890683122, 1.000000000000000000, 0.9659258262890683122, 1.000000000000000000, 0.9659258262890683122, 1.000000000000000000, 0.9659258262890683122, 1.000000000000000000, 0.9659258262890683122, 1.000000000000000000, 0.9659258262890683122, 1.000000000000000000, 0.9659258262890683122, 1.000000000000000000, 0.9659258262890683122, 1.000000000000000000, 0.9659258262890683122, 1.000000000000000000, 0.9659258262890683122, 1.000000000000000000, 0.9659258262890683122, 1.000000000000000000, 0.9659258262890683122, 1.000000000000000000, 0.9659258262890683122, 1.000000000000000000, 0.9659258262890683122, 1.000000000000000000, 0.9659258262890683122, 1.000000000000000000, 0.9659258262890683122, 1.000000000000000000, 0.9659258262890683122, 1.000000000000000000, 0.9659258262890683122, 1.000000000000000000, 0.9659258262890683122, 1.000000000000000000, 0.9659258262890683122, 1.000000000000000000, 0.9659258262890683122, 1.000000000000000000, 0.9659258262890683122, 1.000000000000000000, 0.9659258262890683122, 1.000000000000000000, 0.9659258262890683122, 1.000000000000000000, 0.9659258262890683122, 1.000000000000000000, 0.9659258262890683122, 1.000000000000000000, 0.9659258262890683122, 1.000000000000000000, 0.9659258262890683122, 1.000000000000000000, 0.9659258262890683122, 1.000000000000000000, 0.9659258262890683122, 1.000000000000000000, 0.9659258262890683122, 1.000000000000000000, 0.9659258262890683122, 1.000000000000000000, 0.9659258262890683122, 1.000000000000000000, 0.9659258262890683122, 1.000000000000000000, 0.9659258262890683122, 1.000000000000000000, 0.9659258262890683122, 1.000000000000000000, 0.9659258262890683122, 1.000000000000000000, 0.9659258262890683122, 1.000000000000000000, 0.9659258262890683122, 1.000000000000000000, 0.9659258262890683122, 1.000000000000000000, 0.9659258262890683122, 1.000000000000000000, 0.9659258262890683122, 1.000000000000000000, 0.9659258262890683122, 1.000000000000000000, 0.9659258262890683122, 1.000000000000000000, 0.9659258262890683122, 1.000000000000000000, 0.9659258262890683122, 1.000000000000000000, 0.9659258262890683122, 1.000000000000000000, 0.9659258262890683122, 1.000000000000000000, 0.9659258262890683122, 1.000000000000000000, 0.9659258262890683122, 1.000000000000000000, 0.9659258262890683122, 1.000000000000000000, 0.9659258262890683122, 1.000000000000000000, 0.9659258262890683122, 1.000000000000000000, 0.9659258262890683122, 1.000000000000000000, 0.9659258262890683122, 1.000000000000000000, 0.9659258262890683122, 1.000000000000000000, 0.9659258262890683122, 1.000000000000000000, 0.9659258262890683122, 1.000000000000000000, 0.9659258262890683122, 1.000000000000000000, 0.9659258262890683122, 1.000000000000000000, 0.9659258262890683122, 1.000000000000000000, 0.9659258262890683122, 1.000000000000000000, 0.9659258262890683122, 1.000000000000000000, 0.9659258262890683122, 1.000000000000000000, 0.9659258262890683122, 1.000000000000000000),
 ( 0.3333333333333333703, 0.3219752754296894559, 0.3333333333333333703, 0.3219752754296894559, 0.3333333333333333703, 0.3219752754296894559, 0.3333333333333333703, 0.3219752754296894559, 0.3333333333333333703, 0.3219752754296894559, 0.3333333333333333703, 0.3219752754296894559, 0.3333333333333333703, 0.3219752754296894559, 0.3333333333333333703, 0.3219752754296894559, 0.3333333333333333703, 0.3219752754296894559, 0.3333333333333333703, 0.3219752754296894559, 0.3333333333333333703, 0.3219752754296894559, 0.3333333333333333703, 0.3219752754296894559, 0.3333333333333333703, 0.3219752754296894559, 0.3333333333333333703, 0.3219752754296894559, 0.3333333333333333703, 0.3219752754296894559, 0.3333333333333333703, 0.3219752754296894559, 0.3333333333333333703, 0.3219752754296894559, 0.3333333333333333703, 0.3219752754296894559, 0.3333333333333333703, 0.3219752754296894559, 0.3333333333333333703, 0.3219752754296894559, 0.3333333333333333703, 0.3219752754296894559, 0.3333333333333333703, 0.3219752754296894559, 0.3333333333333333703, 0.3219752754296894559, 0.3333333333333333703, 0.3219752754296894559, 0.3333333333333333703, 0.3219752754296894559, 0.3333333333333333703, 0.3219752754296894559, 0.3333333333333333703, 0.3219752754296894559, 0.3333333333333333703, 0.3219752754296894559, 0.3333333333333333703, 0.3219752754296894559, 0.3333333333333333703, 0.3219752754296894559, 0.3333333333333333703, 0.3219752754296894559, 0.3333333333333333703, 0.3219752754296894559, 0.3333333333333333703, 0.3219752754296894559, 0.3333333333333333703, 0.3219752754296894559, 0.3333333333333333703, 0.3219752754296894559, 0.3333333333333333703, 0.3219752754296894559, 0.3333333333333333703, 0.3219752754296894559, 0.3333333333333333703, 0.3219752754296894559, 0.3333333333333333703, 0.3219752754296894559, 0.3333333333333333703, 0.3219752754296894559, 0.3333333333333333703, 0.3219752754296894559, 0.3333333333333333703, 0.3219752754296894559, 0.3333333333333333703, 0.3219752754296894559, 0.3333333333333333703, 0.3219752754296894559, 0.3333333333333333703, 0.3219752754296894559, 0.3333333333333333703, 0.3219752754296894559, 0.3333333333333333703, 0.3219752754296894559, 0.3333333333333333703, 0.3219752754296894559, 0.3333333333333333703, 0.3219752754296894559, 0.3333333333333333703, 0.3219752754296894559, 0.3333333333333333703, 0.3219752754296894559, 0.3333333333333333703, 0.3219752754296894559, 0.3333333333333333703, 0.3219752754296894559, 0.3333333333333333703, 0.3219752754296894559, 0.3333333333333333703, 0.3219752754296894559, 0.3333333333333333703, 0.3219752754296894559, 0.3333333333333333703, 0.3219752754296894559, 0.3333333333333333703, 0.3219752754296894559, 0.3333333333333333703, 0.3219752754296894559, 0.3333333333333333703, 0.3219752754296894559, 0.3333333333333333703, 0.3219752754296894559, 0.3333333333333333703, 0.3219752754296894559, 0.3333333333333333703, 0.3219752754296894559, 0.3333333333333333703, 0.3219752754296894559, 0.3333333333333333703, 0.3219752754296894559, 0.3333333333333333703, 0.3219752754296894559, 0.3333333333333333703, 0.3219752754296894559, 0.3333333333333333703, 0.3219752754296894559, 0.3333333333333333703, 0.3219752754296894559, 0.3333333333333333703, 0.3219752754296894559, 0.3333333333333333703, 0.3219752754296894559, 0.3333333333333333703, 0.3219752754296894559, 0.3333333333333333703, 0.3219752754296894559, 0.3333333333333333703, 0.3219752754296894559, 0.3333333333333333703, 0.3219752754296894559, 0.3333333333333333703, 0.3219752754296894559, 0.3333333333333333703, 0.3219752754296894559, 0.3333333333333333703, 0.3219752754296894559, 0.3333333333333333703, 0.3219752754296894559, 0.3333333333333333703, 0.3219752754296894559, 0.3333333333333333703, 0.3219752754296894559, 0.3333333333333333703, 0.3219752754296894559, 0.3333333333333333703, 0.3219752754296894559, 0.3333333333333333703, 0.3219752754296894559, 0.3333333333333333703, 0.3219752754296894559, 0.3333333333333333703, 0.3219752754296894559, 0.3333333333333333703, 0.3219752754296894559, 0.3333333333333333703, 0.3219752754296894559, 0.3333333333333333703, 0.3219752754296894559, 0.3333333333333333703, 0.3219752754296894559, 0.3333333333333333703, 0.3219752754296894559, 0.3333333333333333703, 0.3219752754296894559, 0.3333333333333333703, 0.3219752754296894559, 0.3333333333333333703, 0.3219752754296894559, 0.3333333333333333703, 0.3219752754296894559, 0.3333333333333333703, 0.3219752754296894559, 0.3333333333333333703, 0.3219752754296894559, 0.3333333333333333703, 0.3219752754296894559, 0.3333333333333333703, 0.3219752754296894559, 0.3333333333333333703, 0.3219752754296894559, 0.3333333333333333703, 0.3219752754296894559, 0.3333333333333333703, 0.3219752754296894559, 0.3333333333333333703, 0.3219752754296894559, 0.3333333333333333703, 0.3219752754296894559, 0.3333333333333333703, 0.3219752754296894559, 0.3333333333333333703, 0.3219752754296894559, 0.3333333333333333703, 0.3219752754296894559, 0.3333333333333333703, 0.3219752754296894559, 0.3333333333333333703, 0.3219752754296894559, 0.3333333333333333703, 0.3219752754296894559, 0.3333333333333333703, 0.3219752754296894559, 0.3333333333333333703, 0.3219752754296894559, 0.3333333333333333703, 0.3219752754296894559, 0.3333333333333333703, 0.3219752754296894559, 0.3333333333333333703, 0.3219752754296894559, 0.3333333333333333703, 0.3219752754296894559, 0.3333333333333333703, 0.3219752754296894559, 0.3333333333333333703, 0.3219752754296894559, 0.3333333333333333703, 0.3219752754296894559, 0.3333333333333333703, 0.3219752754296894559, 0.3333333333333333703, 0.3219752754296894559, 0.3333333333333333703, 0.3219752754296894559, 0.3333333333333333703, 0.3219752754296894559, 0.3333333333333333703, 0.3219752754296894559, 0.3333333333333333703, 0.3219752754296894559, 0.3333333333333333703, 0.3219752754296894559, 0.3333333333333333703, 0.3219752754296894559, 0.3333333333333333703, 0.3219752754296894559, 0.3333333333333333703, 0.3219752754296894559, 0.3333333333333333703, 0.3219752754296894559, 0.3333333333333333703, 0.3219752754296894559, 0.3333333333333333703, 0.3219752754296894559, 0.3333333333333333703, 0.3219752754296894559, 0.3333333333333333703, 0.3219752754296894559, 0.3333333333333333703, 0.3219752754296894559, 0.3333333333333333703, 0.3219752754296894559, 0.3333333333333333703, 0.3219752754296894559, 0.3333333333333333703, 0.3219752754296894559, 0.3333333333333333703, 0.3219752754296894559, 0.3333333333333333703, 0.3219752754296894559, 0.3333333333333333703, 0.3219752754296894559, 0.3333333333333333703, 0.3219752754296894559, 0.3333333333333333703, 0.3219752754296894559, 0.3333333333333333703, 0.3219752754296894559, 0.3333333333333333703, 0.3219752754296894559, 0.3333333333333333703, 0.3219752754296894559, 0.3333333333333333703, 0.3219752754296894559, 0.3333333333333333703, 0.3219752754296894559, 0.3333333333333333703, 0.3219752754296894559, 0.3333333333333333703, 0.3219752754296894559, 0.3333333333333333703, 0.3219752754296894559, 0.3333333333333333703, 0.3219752754296894559, 0.3333333333333333703, 0.3219752754296894559, 0.3333333333333333703, 0.3219752754296894559, 0.3333333333333333703, 0.3219752754296894559, 0.3333333333333333703, 0.3219752754296894559, 0.3333333333333333703, 0.3219752754296894559, 0.3333333333333333703, 0.3219752754296894559, 0.3333333333333333703, 0.3219752754296894559, 0.3333333333333333703, 0.3219752754296894559, 0.3333333333333333703, 0.3219752754296894559, 0.3333333333333333703, 0.3219752754296894559, 0.3333333333333333703, 0.3219752754296894559, 0.3333333333333333703, 0.3219752754296894559, 0.3333333333333333703, 0.3219752754296894559, 0.3333333333333333703, 0.3219752754296894559, 0.3333333333333333703, 0.3219752754296894559, 0.3333333333333333703, 0.3219752754296894559, 0.3333333333333333703, 0.3219752754296894559, 0.3333333333333333703, 0.3219752754296894559, 0.3333333333333333703, 0.3219752754296894559, 0.3333333333333333703, 0.3219752754296894559, 0.3333333333333333703, 0.3219752754296894559, 0.3333333333333333703, 0.3219752754296894559, 0.3333333333333333703, 0.3219752754296894559, 0.3333333333333333703, 0.3219752754296894559, 0.3333333333333333703, 0.3219752754296894559, 0.3333333333333333703, 0.3219752754296894559, 0.3333333333333333703, 0.3219752754296894559, 0.3333333333333333703, 0.3219752754296894559, 0.3333333333333333703, 0.3219752754296894559, 0.3333333333333333703, 0.3219752754296894559, 0.3333333333333333703, 0.3219752754296894559, 0.3333333333333333703, 0.3219752754296894559, 0.3333333333333333703, 0.3219752754296894559, 0.3333333333333333703, 0.3219752754296894559, 0.3333333333333333703, 0.3219752754296894559, 0.3333333333333333703, 0.3219752754296894559, 0.3333333333333333703, 0.3219752754296894559, 0.3333333333333333703, 0.3219752754296894559, 0.3333333333333333703, 0.3219752754296894559, 0.3333333333333333703, 0.3219752754296894559, 0.3333333333333333703, 0.3219752754296894559, 0.3333333333333333703, 0.3219752754296894559, 0.3333333333333333703, 0.3219752754296894559, 0.3333333333333333703, 0.3219752754296894559, 0.3333333333333333703, 0.3219752754296894559, 0.3333333333333333703, 0.3219752754296894559, 0.3333333333333333703, 0.3219752754296894559, 0.3333333333333333703, 0.3219752754296894559, 0.3333333333333333703, 0.3219752754296894559, 0.3333333333333333703, 0.3219752754296894559, 0.3333333333333333703, 0.3219752754296894559, 0.3333333333333333703, 0.3219752754296894559, 0.3333333333333333703, 0.3219752754296894559, 0.3333333333333333703, 0.3219752754296894559, 0.3333333333333333703, 0.3219752754296894559, 0.3333333333333333703, 0.3219752754296894559, 0.3333333333333333703, 0.3219752754296894559, 0.3333333333333333703, 0.3219752754296894559, 0.3333333333333333703, 0.3219752754296894559, 0.3333333333333333703, 0.3219752754296894559, 0.3333333333333333703, 0.3219752754296894559, 0.3333333333333333703, 0.3219752754296894559, 0.3333333333333333703, 0.3219752754296894559, 0.3333333333333333703, 0.3219752754296894559, 0.3333333333333333703, 0.3219752754296894559, 0.3333333333333333703, 0.3219752754296894559, 0.3333333333333333703, 0.3219752754296894559, 0.3333333333333333703, 0.3219752754296894559, 0.3333333333333333703, 0.3219752754296894559, 0.3333333333333333703, 0.3219752754296894559, 0.3333333333333333703, 0.3219752754296894559, 0.3333333333333333703, 0.3219752754296894559, 0.3333333333333333703, 0.3219752754296894559, 0.3333333333333333703, 0.3219752754296894559, 0.3333333333333333703, 0.3219752754296894559, 0.3333333333333333703, 0.3219752754296894559, 0.3333333333333333703),
 ( 0.3333333333333333703, 0.3219752754296894559, 0.3333333333333333703, 0.3219752754296894559, 0.3333333333333333703, 0.3219752754296894559, 0.3333333333333333703, 0.3219752754296894559, 0.3333333333333333703, 0.3219752754296894559, 0.3333333333333333703, 0.3219752754296894559, 0.3333333333333333703, 0.3219752754296894559, 0.3333333333333333703, 0.3219752754296894559, 0.3333333333333333703, 0.3219752754296894559, 0.3333333333333333703, 0.3219752754296894559, 0.3333333333333333703, 0.3219752754296894559, 0.3333333333333333703, 0.3219752754296894559, 0.3333333333333333703, 0.3219752754296894559, 0.3333333333333333703, 0.3219752754296894559, 0.3333333333333333703, 0.3219752754296894559, 0.3333333333333333703, 0.3219752754296894559, 0.3333333333333333703, 0.3219752754296894559, 0.3333333333333333703, 0.3219752754296894559, 0.3333333333333333703, 0.3219752754296894559, 0.3333333333333333703, 0.3219752754296894559, 0.3333333333333333703, 0.3219752754296894559, 0.3333333333333333703, 0.3219752754296894559, 0.3333333333333333703, 0.3219752754296894559, 0.3333333333333333703, 0.3219752754296894559, 0.3333333333333333703, 0.3219752754296894559, 0.3333333333333333703, 0.3219752754296894559, 0.3333333333333333703, 0.3219752754296894559, 0.3333333333333333703, 0.3219752754296894559, 0.3333333333333333703, 0.3219752754296894559, 0.3333333333333333703, 0.3219752754296894559, 0.3333333333333333703, 0.3219752754296894559, 0.3333333333333333703, 0.3219752754296894559, 0.3333333333333333703, 0.3219752754296894559, 0.3333333333333333703, 0.3219752754296894559, 0.3333333333333333703, 0.3219752754296894559, 0.3333333333333333703, 0.3219752754296894559, 0.3333333333333333703, 0.3219752754296894559, 0.3333333333333333703, 0.3219752754296894559, 0.3333333333333333703, 0.3219752754296894559, 0.3333333333333333703, 0.3219752754296894559, 0.3333333333333333703, 0.3219752754296894559, 0.3333333333333333703, 0.3219752754296894559, 0.3333333333333333703, 0.3219752754296894559, 0.3333333333333333703, 0.3219752754296894559, 0.3333333333333333703, 0.3219752754296894559, 0.3333333333333333703, 0.3219752754296894559, 0.3333333333333333703, 0.3219752754296894559, 0.3333333333333333703, 0.3219752754296894559, 0.3333333333333333703, 0.3219752754296894559, 0.3333333333333333703, 0.3219752754296894559, 0.3333333333333333703, 0.3219752754296894559, 0.3333333333333333703, 0.3219752754296894559, 0.3333333333333333703, 0.3219752754296894559, 0.3333333333333333703, 0.3219752754296894559, 0.3333333333333333703, 0.3219752754296894559, 0.3333333333333333703, 0.3219752754296894559, 0.3333333333333333703, 0.3219752754296894559, 0.3333333333333333703, 0.3219752754296894559, 0.3333333333333333703, 0.3219752754296894559, 0.3333333333333333703, 0.3219752754296894559, 0.3333333333333333703, 0.3219752754296894559, 0.3333333333333333703, 0.3219752754296894559, 0.3333333333333333703, 0.3219752754296894559, 0.3333333333333333703, 0.3219752754296894559, 0.3333333333333333703, 0.3219752754296894559, 0.3333333333333333703, 0.3219752754296894559, 0.3333333333333333703, 0.3219752754296894559, 0.3333333333333333703, 0.3219752754296894559, 0.3333333333333333703, 0.3219752754296894559, 0.3333333333333333703, 0.3219752754296894559, 0.3333333333333333703, 0.3219752754296894559, 0.3333333333333333703, 0.3219752754296894559, 0.3333333333333333703, 0.3219752754296894559, 0.3333333333333333703, 0.3219752754296894559, 0.3333333333333333703, 0.3219752754296894559, 0.3333333333333333703, 0.3219752754296894559, 0.3333333333333333703, 0.3219752754296894559, 0.3333333333333333703, 0.3219752754296894559, 0.3333333333333333703, 0.3219752754296894559, 0.3333333333333333703, 0.3219752754296894559, 0.3333333333333333703, 0.3219752754296894559, 0.3333333333333333703, 0.3219752754296894559, 0.3333333333333333703, 0.3219752754296894559, 0.3333333333333333703, 0.3219752754296894559, 0.3333333333333333703, 0.3219752754296894559, 0.3333333333333333703, 0.3219752754296894559, 0.3333333333333333703, 0.3219752754296894559, 0.3333333333333333703, 0.3219752754296894559, 0.3333333333333333703, 0.3219752754296894559, 0.3333333333333333703, 0.3219752754296894559, 0.3333333333333333703, 0.3219752754296894559, 0.3333333333333333703, 0.3219752754296894559, 0.3333333333333333703, 0.3219752754296894559, 0.3333333333333333703, 0.3219752754296894559, 0.3333333333333333703, 0.3219752754296894559, 0.3333333333333333703, 0.3219752754296894559, 0.3333333333333333703, 0.3219752754296894559, 0.3333333333333333703, 0.3219752754296894559, 0.3333333333333333703, 0.3219752754296894559, 0.3333333333333333703, 0.3219752754296894559, 0.3333333333333333703, 0.3219752754296894559, 0.3333333333333333703, 0.3219752754296894559, 0.3333333333333333703, 0.3219752754296894559, 0.3333333333333333703, 0.3219752754296894559, 0.3333333333333333703, 0.3219752754296894559, 0.3333333333333333703, 0.3219752754296894559, 0.3333333333333333703, 0.3219752754296894559, 0.3333333333333333703, 0.3219752754296894559, 0.3333333333333333703, 0.3219752754296894559, 0.3333333333333333703, 0.3219752754296894559, 0.3333333333333333703, 0.3219752754296894559, 0.3333333333333333703, 0.3219752754296894559, 0.3333333333333333703, 0.3219752754296894559, 0.3333333333333333703, 0.3219752754296894559, 0.3333333333333333703, 0.3219752754296894559, 0.3333333333333333703, 0.3219752754296894559, 0.3333333333333333703, 0.3219752754296894559, 0.3333333333333333703, 0.3219752754296894559, 0.3333333333333333703, 0.3219752754296894559, 0.3333333333333333703, 0.3219752754296894559, 0.3333333333333333703, 0.3219752754296894559, 0.3333333333333333703, 0.3219752754296894559, 0.3333333333333333703, 0.3219752754296894559, 0.3333333333333333703, 0.3219752754296894559, 0.3333333333333333703, 0.3219752754296894559, 0.3333333333333333703, 0.3219752754296894559, 0.3333333333333333703, 0.3219752754296894559, 0.3333333333333333703, 0.3219752754296894559, 0.3333333333333333703, 0.3219752754296894559, 0.3333333333333333703, 0.3219752754296894559, 0.3333333333333333703, 0.3219752754296894559, 0.3333333333333333703, 0.3219752754296894559, 0.3333333333333333703, 0.3219752754296894559, 0.3333333333333333703, 0.3219752754296894559, 0.3333333333333333703, 0.3219752754296894559, 0.3333333333333333703, 0.3219752754296894559, 0.3333333333333333703, 0.3219752754296894559, 0.3333333333333333703, 0.3219752754296894559, 0.3333333333333333703, 0.3219752754296894559, 0.3333333333333333703, 0.3219752754296894559, 0.3333333333333333703, 0.3219752754296894559, 0.3333333333333333703, 0.3219752754296894559, 0.3333333333333333703, 0.3219752754296894559, 0.3333333333333333703, 0.3219752754296894559, 0.3333333333333333703, 0.3219752754296894559, 0.3333333333333333703, 0.3219752754296894559, 0.3333333333333333703, 0.3219752754296894559, 0.3333333333333333703, 0.3219752754296894559, 0.3333333333333333703, 0.3219752754296894559, 0.3333333333333333703, 0.3219752754296894559, 0.3333333333333333703, 0.3219752754296894559, 0.3333333333333333703, 0.3219752754296894559, 0.3333333333333333703, 0.3219752754296894559, 0.3333333333333333703, 0.3219752754296894559, 0.3333333333333333703, 0.3219752754296894559, 0.3333333333333333703, 0.3219752754296894559, 0.3333333333333333703, 0.3219752754296894559, 0.3333333333333333703, 0.3219752754296894559, 0.3333333333333333703, 0.3219752754296894559, 0.3333333333333333703, 0.3219752754296894559, 0.3333333333333333703, 0.3219752754296894559, 0.3333333333333333703, 0.3219752754296894559, 0.3333333333333333703, 0.3219752754296894559, 0.3333333333333333703, 0.3219752754296894559, 0.3333333333333333703, 0.3219752754296894559, 0.3333333333333333703, 0.3219752754296894559, 0.3333333333333333703, 0.3219752754296894559, 0.3333333333333333703, 0.3219752754296894559, 0.3333333333333333703, 0.3219752754296894559, 0.3333333333333333703, 0.3219752754296894559, 0.3333333333333333703, 0.3219752754296894559, 0.3333333333333333703, 0.3219752754296894559, 0.3333333333333333703, 0.3219752754296894559, 0.3333333333333333703, 0.3219752754296894559, 0.3333333333333333703, 0.3219752754296894559, 0.3333333333333333703, 0.3219752754296894559, 0.3333333333333333703, 0.3219752754296894559, 0.3333333333333333703, 0.3219752754296894559, 0.3333333333333333703, 0.3219752754296894559, 0.3333333333333333703, 0.3219752754296894559, 0.3333333333333333703, 0.3219752754296894559, 0.3333333333333333703, 0.3219752754296894559, 0.3333333333333333703, 0.3219752754296894559, 0.3333333333333333703, 0.3219752754296894559, 0.3333333333333333703, 0.3219752754296894559, 0.3333333333333333703, 0.3219752754296894559, 0.3333333333333333703, 0.3219752754296894559, 0.3333333333333333703, 0.3219752754296894559, 0.3333333333333333703, 0.3219752754296894559, 0.3333333333333333703, 0.3219752754296894559, 0.3333333333333333703, 0.3219752754296894559, 0.3333333333333333703, 0.3219752754296894559, 0.3333333333333333703, 0.3219752754296894559, 0.3333333333333333703, 0.3219752754296894559, 0.3333333333333333703, 0.3219752754296894559, 0.3333333333333333703, 0.3219752754296894559, 0.3333333333333333703, 0.3219752754296894559, 0.3333333333333333703, 0.3219752754296894559, 0.3333333333333333703, 0.3219752754296894559, 0.3333333333333333703, 0.3219752754296894559, 0.3333333333333333703, 0.3219752754296894559, 0.3333333333333333703, 0.3219752754296894559, 0.3333333333333333703, 0.3219752754296894559, 0.3333333333333333703, 0.3219752754296894559, 0.3333333333333333703, 0.3219752754296894559, 0.3333333333333333703, 0.3219752754296894559, 0.3333333333333333703, 0.3219752754296894559, 0.3333333333333333703, 0.3219752754296894559, 0.3333333333333333703, 0.3219752754296894559, 0.3333333333333333703, 0.3219752754296894559, 0.3333333333333333703, 0.3219752754296894559, 0.3333333333333333703, 0.3219752754296894559, 0.3333333333333333703, 0.3219752754296894559, 0.3333333333333333703, 0.3219752754296894559, 0.3333333333333333703, 0.3219752754296894559, 0.3333333333333333703, 0.3219752754296894559, 0.3333333333333333703, 0.3219752754296894559, 0.3333333333333333703, 0.3219752754296894559, 0.3333333333333333703, 0.3219752754296894559, 0.3333333333333333703, 0.3219752754296894559, 0.3333333333333333703, 0.3219752754296894559, 0.3333333333333333703, 0.3219752754296894559, 0.3333333333333333703, 0.3219752754296894559, 0.3333333333333333703, 0.3219752754296894559, 0.3333333333333333703, 0.3219752754296894559, 0.3333333333333333703, 0.3219752754296894559, 0.3333333333333333703, 0.3219752754296894559, 0.3333333333333333703, 0.3219752754296894559, 0.3333333333333333703),
 ( 1.000000000000000000, 0.9659258262890683122, 1.000000000000000000, 0.9659258262890683122, 1.000000000000000000, 0.9659258262890683122, 1.000000000000000000, 0.9659258262890683122, 1.000000000000000000, 0.9659258262890683122, 1.000000000000000000, 0.9659258262890683122, 1.000000000000000000, 0.9659258262890683122, 1.000000000000000000, 0.9659258262890683122, 1.000000000000000000, 0.9659258262890683122, 1.000000000000000000, 0.9659258262890683122, 1.000000000000000000, 0.9659258262890683122, 1.000000000000000000, 0.9659258262890683122, 1.000000000000000000, 0.9659258262890683122, 1.000000000000000000, 0.9659258262890683122, 1.000000000000000000, 0.9659258262890683122, 1.000000000000000000, 0.9659258262890683122, 1.000000000000000000, 0.9659258262890683122, 1.000000000000000000, 0.9659258262890683122, 1.000000000000000000, 0.9659258262890683122, 1.000000000000000000, 0.9659258262890683122, 1.000000000000000000, 0.9659258262890683122, 1.000000000000000000, 0.9659258262890683122, 1.000000000000000000, 0.9659258262890683122, 1.000000000000000000, 0.9659258262890683122, 1.000000000000000000, 0.9659258262890683122, 1.000000000000000000, 0.9659258262890683122, 1.000000000000000000, 0.9659258262890683122, 1.000000000000000000, 0.9659258262890683122, 1.000000000000000000, 0.9659258262890683122, 1.000000000000000000, 0.9659258262890683122, 1.000000000000000000, 0.9659258262890683122, 1.000000000000000000, 0.9659258262890683122, 1.000000000000000000, 0.9659258262890683122, 1.000000000000000000, 0.9659258262890683122, 1.000000000000000000, 0.9659258262890683122, 1.000000000000000000, 0.9659258262890683122, 1.000000000000000000, 0.9659258262890683122, 1.000000000000000000, 0.9659258262890683122, 1.000000000000000000, 0.9659258262890683122, 1.000000000000000000, 0.9659258262890683122, 1.000000000000000000, 0.9659258262890683122, 1.000000000000000000, 0.9659258262890683122, 1.000000000000000000, 0.9659258262890683122, 1.000000000000000000, 0.9659258262890683122, 1.000000000000000000, 0.9659258262890683122, 1.000000000000000000, 0.9659258262890683122, 1.000000000000000000, 0.9659258262890683122, 1.000000000000000000, 0.9659258262890683122, 1.000000000000000000, 0.9659258262890683122, 1.000000000000000000, 0.9659258262890683122, 1.000000000000000000, 0.9659258262890683122, 1.000000000000000000, 0.9659258262890683122, 1.000000000000000000, 0.9659258262890683122, 1.000000000000000000, 0.9659258262890683122, 1.000000000000000000, 0.9659258262890683122, 1.000000000000000000, 0.9659258262890683122, 1.000000000000000000, 0.9659258262890683122, 1.000000000000000000, 0.9659258262890683122, 1.000000000000000000, 0.9659258262890683122, 1.000000000000000000, 0.9659258262890683122, 1.000000000000000000, 0.9659258262890683122, 1.000000000000000000, 0.9659258262890683122, 1.000000000000000000, 0.9659258262890683122, 1.000000000000000000, 0.9659258262890683122, 1.000000000000000000, 0.9659258262890683122, 1.000000000000000000, 0.9659258262890683122, 1.000000000000000000, 0.9659258262890683122, 1.000000000000000000, 0.9659258262890683122, 1.000000000000000000, 0.9659258262890683122, 1.000000000000000000, 0.9659258262890683122, 1.000000000000000000, 0.9659258262890683122, 1.000000000000000000, 0.9659258262890683122, 1.000000000000000000, 0.9659258262890683122, 1.000000000000000000, 0.9659258262890683122, 1.000000000000000000, 0.9659258262890683122, 1.000000000000000000, 0.9659258262890683122, 1.000000000000000000, 0.9659258262890683122, 1.000000000000000000, 0.9659258262890683122, 1.000000000000000000, 0.9659258262890683122, 1.000000000000000000, 0.9659258262890683122, 1.000000000000000000, 0.9659258262890683122, 1.000000000000000000, 0.9659258262890683122, 1.000000000000000000, 0.9659258262890683122, 1.000000000000000000, 0.9659258262890683122, 1.000000000000000000, 0.9659258262890683122, 1.000000000000000000, 0.9659258262890683122, 1.000000000000000000, 0.9659258262890683122, 1.000000000000000000, 0.9659258262890683122, 1.000000000000000000, 0.9659258262890683122, 1.000000000000000000, 0.9659258262890683122, 1.000000000000000000, 0.9659258262890683122, 1.000000000000000000, 0.9659258262890683122, 1.000000000000000000, 0.9659258262890683122, 1.000000000000000000, 0.9659258262890683122, 1.000000000000000000, 0.9659258262890683122, 1.000000000000000000, 0.9659258262890683122, 1.000000000000000000, 0.9659258262890683122, 1.000000000000000000, 0.9659258262890683122, 1.000000000000000000, 0.9659258262890683122, 1.000000000000000000, 0.9659258262890683122, 1.000000000000000000, 0.9659258262890683122, 1.000000000000000000, 0.9659258262890683122, 1.000000000000000000, 0.9659258262890683122, 1.000000000000000000, 0.9659258262890683122, 1.000000000000000000, 0.9659258262890683122, 1.000000000000000000, 0.9659258262890683122, 1.000000000000000000, 0.9659258262890683122, 1.000000000000000000, 0.9659258262890683122, 1.000000000000000000, 0.9659258262890683122, 1.000000000000000000, 0.9659258262890683122, 1.000000000000000000, 0.9659258262890683122, 1.000000000000000000, 0.9659258262890683122, 1.000000000000000000, 0.9659258262890683122, 1.000000000000000000, 0.9659258262890683122, 1.000000000000000000, 0.9659258262890683122, 1.000000000000000000, 0.9659258262890683122, 1.000000000000000000, 0.9659258262890683122, 1.000000000000000000, 0.9659258262890683122, 1.000000000000000000, 0.9659258262890683122, 1.000000000000000000, 0.9659258262890683122, 1.000000000000000000, 0.9659258262890683122, 1.000000000000000000, 0.9659258262890683122, 1.000000000000000000, 0.9659258262890683122, 1.000000000000000000, 0.9659258262890683122, 1.000000000000000000, 0.9659258262890683122, 1.000000000000000000, 0.9659258262890683122, 1.000000000000000000, 0.9659258262890683122, 1.000000000000000000, 0.9659258262890683122, 1.000000000000000000, 0.9659258262890683122, 1.000000000000000000, 0.9659258262890683122, 1.000000000000000000, 0.9659258262890683122, 1.000000000000000000, 0.9659258262890683122, 1.000000000000000000, 0.9659258262890683122, 1.000000000000000000, 0.9659258262890683122, 1.000000000000000000, 0.9659258262890683122, 1.000000000000000000, 0.9659258262890683122, 1.000000000000000000, 0.9659258262890683122, 1.000000000000000000, 0.9659258262890683122, 1.000000000000000000, 0.9659258262890683122, 1.000000000000000000, 0.9659258262890683122, 1.000000000000000000, 0.9659258262890683122, 1.000000000000000000, 0.9659258262890683122, 1.000000000000000000, 0.9659258262890683122, 1.000000000000000000, 0.9659258262890683122, 1.000000000000000000, 0.9659258262890683122, 1.000000000000000000, 0.9659258262890683122, 1.000000000000000000, 0.9659258262890683122, 1.000000000000000000, 0.9659258262890683122, 1.000000000000000000, 0.9659258262890683122, 1.000000000000000000, 0.9659258262890683122, 1.000000000000000000, 0.9659258262890683122, 1.000000000000000000, 0.9659258262890683122, 1.000000000000000000, 0.9659258262890683122, 1.000000000000000000, 0.9659258262890683122, 1.000000000000000000, 0.9659258262890683122, 1.000000000000000000, 0.9659258262890683122, 1.000000000000000000, 0.9659258262890683122, 1.000000000000000000, 0.9659258262890683122, 1.000000000000000000, 0.9659258262890683122, 1.000000000000000000, 0.9659258262890683122, 1.000000000000000000, 0.9659258262890683122, 1.000000000000000000, 0.9659258262890683122, 1.000000000000000000, 0.9659258262890683122, 1.000000000000000000, 0.9659258262890683122, 1.000000000000000000, 0.9659258262890683122, 1.000000000000000000, 0.9659258262890683122, 1.000000000000000000, 0.9659258262890683122, 1.000000000000000000, 0.9659258262890683122, 1.000000000000000000, 0.9659258262890683122, 1.000000000000000000, 0.9659258262890683122, 1.000000000000000000, 0.9659258262890683122, 1.000000000000000000, 0.9659258262890683122, 1.000000000000000000, 0.9659258262890683122, 1.000000000000000000, 0.9659258262890683122, 1.000000000000000000, 0.9659258262890683122, 1.000000000000000000, 0.9659258262890683122, 1.000000000000000000, 0.9659258262890683122, 1.000000000000000000, 0.9659258262890683122, 1.000000000000000000, 0.9659258262890683122, 1.000000000000000000, 0.9659258262890683122, 1.000000000000000000, 0.9659258262890683122, 1.000000000000000000, 0.9659258262890683122, 1.000000000000000000, 0.9659258262890683122, 1.000000000000000000, 0.9659258262890683122, 1.000000000000000000, 0.9659258262890683122, 1.000000000000000000, 0.9659258262890683122, 1.000000000000000000, 0.9659258262890683122, 1.000000000000000000, 0.9659258262890683122, 1.000000000000000000, 0.9659258262890683122, 1.000000000000000000, 0.9659258262890683122, 1.000000000000000000, 0.9659258262890683122, 1.000000000000000000, 0.9659258262890683122, 1.000000000000000000, 0.9659258262890683122, 1.000000000000000000, 0.9659258262890683122, 1.000000000000000000, 0.9659258262890683122, 1.000000000000000000, 0.9659258262890683122, 1.000000000000000000, 0.9659258262890683122, 1.000000000000000000, 0.9659258262890683122, 1.000000000000000000, 0.9659258262890683122, 1.000000000000000000, 0.9659258262890683122, 1.000000000000000000, 0.9659258262890683122, 1.000000000000000000, 0.9659258262890683122, 1.000000000000000000, 0.9659258262890683122, 1.000000000000000000, 0.9659258262890683122, 1.000000000000000000, 0.9659258262890683122, 1.000000000000000000, 0.9659258262890683122, 1.000000000000000000, 0.9659258262890683122, 1.000000000000000000, 0.9659258262890683122, 1.000000000000000000, 0.9659258262890683122, 1.000000000000000000, 0.9659258262890683122, 1.000000000000000000, 0.9659258262890683122, 1.000000000000000000, 0.9659258262890683122, 1.000000000000000000, 0.9659258262890683122, 1.000000000000000000, 0.9659258262890683122, 1.000000000000000000, 0.9659258262890683122, 1.000000000000000000, 0.9659258262890683122, 1.000000000000000000, 0.9659258262890683122, 1.000000000000000000, 0.9659258262890683122, 1.000000000000000000, 0.9659258262890683122, 1.000000000000000000, 0.9659258262890683122, 1.000000000000000000, 0.9659258262890683122, 1.000000000000000000, 0.9659258262890683122, 1.000000000000000000, 0.9659258262890683122, 1.000000000000000000, 0.9659258262890683122, 1.000000000000000000, 0.9659258262890683122, 1.000000000000000000, 0.9659258262890683122, 1.000000000000000000, 0.9659258262890683122, 1.000000000000000000, 0.9659258262890683122, 1.000000000000000000) ) ) 
 REPRESENTATION_ITEM ( '' )  SURFACE ( )  );
